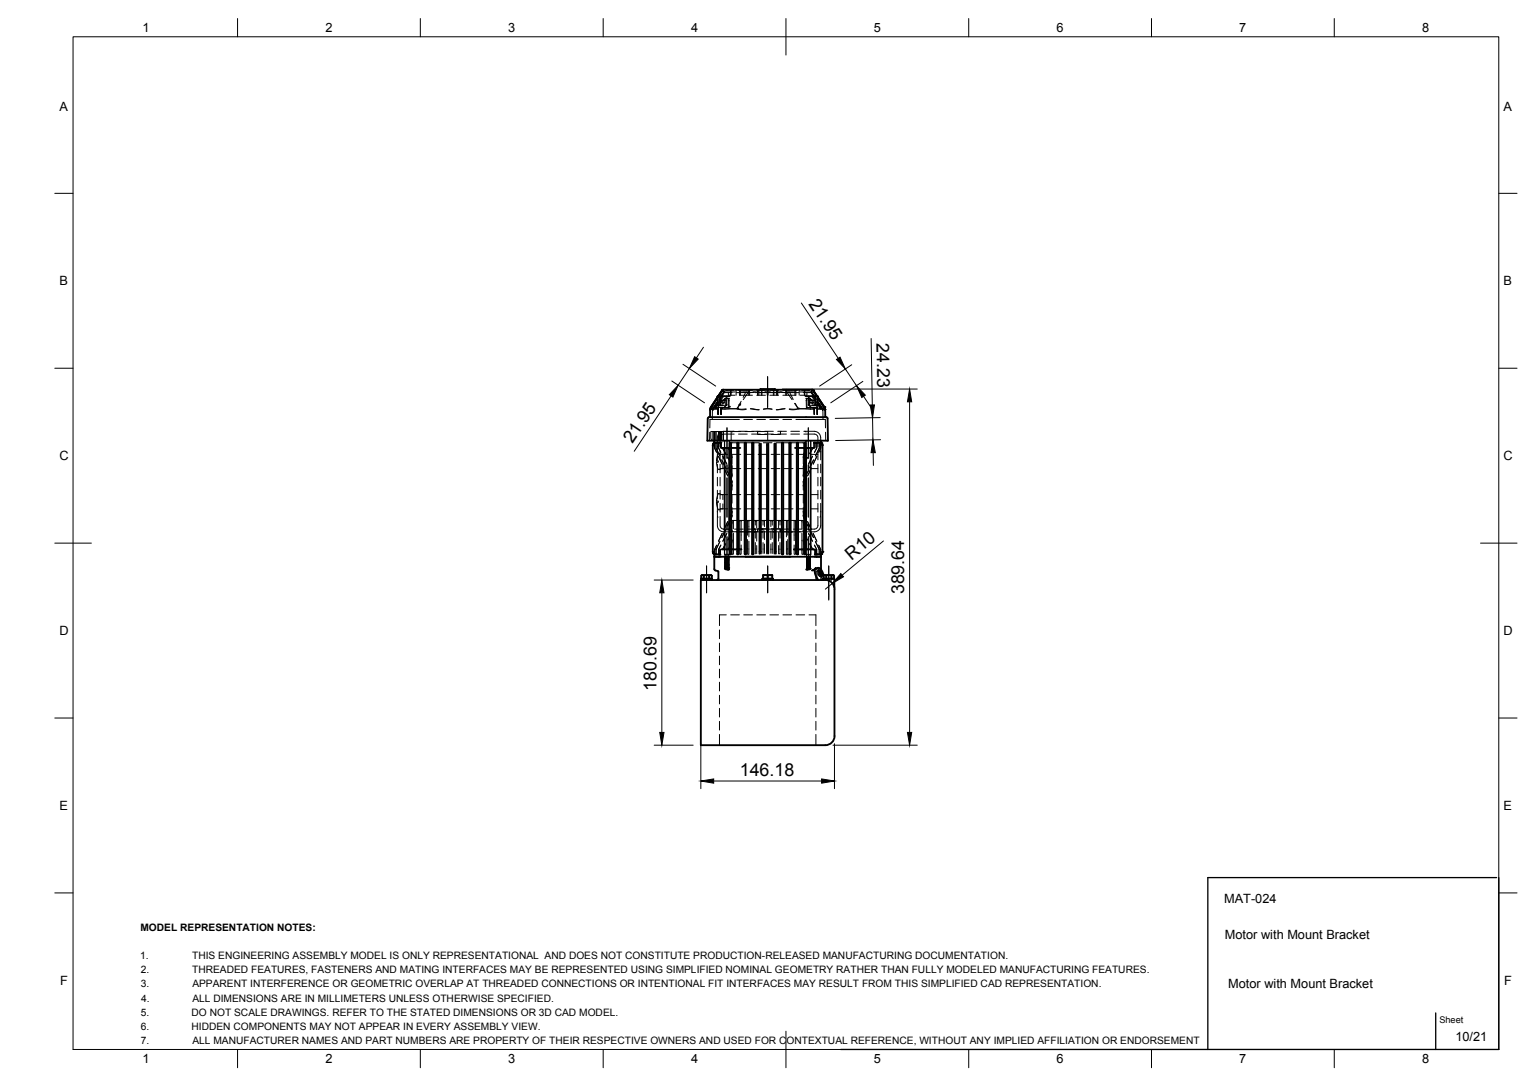
ISO-10303-21;
HEADER;
/* Generated by software containing ST-Developer
 * from STEP Tools, Inc. (www.steptools.com) 
 */

FILE_DESCRIPTION(
/* description */ ('STEP AP214'),
/* implementation_level */ '2;1');

FILE_NAME(
/* name */ 'Motor with Mount Bracket.step',
/* time_stamp */ '2026-11-14T06:34:07-08:00',
/* author */ (''),
/* organization */ (''),
/* preprocessor_version */ 'ST-DEVELOPER v20.2',
/* originating_system */ 'Autodesk Translation Framework v15.17.0.0',
/* authorisation */ '');

FILE_SCHEMA (('AUTOMOTIVE_DESIGN { 1 0 10303 214 3 1 1 }'));
ENDSEC;

DATA;
#10=MECHANICAL_DESIGN_GEOMETRIC_PRESENTATION_REPRESENTATION('',(#7258,#7259,#7260,#7261,#7262,#7263,#7264,#7265,#7266,#7267,#7268,#7269,#7270,#7271,#7272,#7273,#7274,#7275,#7276,#7277),#310623);
#905=B_SPLINE_SURFACE_WITH_KNOTS('',3,3,((#200297,#200298,#200299,#200300,
#200301,#200302,#200303,#200304,#200305,#200306,#200307,#200308,#200309),
(#200310,#200311,#200312,#200313,#200314,#200315,#200316,#200317,#200318,
#200319,#200320,#200321,#200322),(#200323,#200324,#200325,#200326,#200327,
#200328,#200329,#200330,#200331,#200332,#200333,#200334,#200335),(#200336,
#200337,#200338,#200339,#200340,#200341,#200342,#200343,#200344,#200345,
#200346,#200347,#200348),(#200349,#200350,#200351,#200352,#200353,#200354,
#200355,#200356,#200357,#200358,#200359,#200360,#200361),(#200362,#200363,
#200364,#200365,#200366,#200367,#200368,#200369,#200370,#200371,#200372,
#200373,#200374),(#200375,#200376,#200377,#200378,#200379,#200380,#200381,
#200382,#200383,#200384,#200385,#200386,#200387),(#200388,#200389,#200390,
#200391,#200392,#200393,#200394,#200395,#200396,#200397,#200398,#200399,
#200400),(#200401,#200402,#200403,#200404,#200405,#200406,#200407,#200408,
#200409,#200410,#200411,#200412,#200413),(#200414,#200415,#200416,#200417,
#200418,#200419,#200420,#200421,#200422,#200423,#200424,#200425,#200426),
(#200427,#200428,#200429,#200430,#200431,#200432,#200433,#200434,#200435,
#200436,#200437,#200438,#200439),(#200440,#200441,#200442,#200443,#200444,
#200445,#200446,#200447,#200448,#200449,#200450,#200451,#200452),(#200453,
#200454,#200455,#200456,#200457,#200458,#200459,#200460,#200461,#200462,
#200463,#200464,#200465),(#200466,#200467,#200468,#200469,#200470,#200471,
#200472,#200473,#200474,#200475,#200476,#200477,#200478),(#200479,#200480,
#200481,#200482,#200483,#200484,#200485,#200486,#200487,#200488,#200489,
#200490,#200491),(#200492,#200493,#200494,#200495,#200496,#200497,#200498,
#200499,#200500,#200501,#200502,#200503,#200504),(#200505,#200506,#200507,
#200508,#200509,#200510,#200511,#200512,#200513,#200514,#200515,#200516,
#200517),(#200518,#200519,#200520,#200521,#200522,#200523,#200524,#200525,
#200526,#200527,#200528,#200529,#200530),(#200531,#200532,#200533,#200534,
#200535,#200536,#200537,#200538,#200539,#200540,#200541,#200542,#200543),
(#200544,#200545,#200546,#200547,#200548,#200549,#200550,#200551,#200552,
#200553,#200554,#200555,#200556),(#200557,#200558,#200559,#200560,#200561,
#200562,#200563,#200564,#200565,#200566,#200567,#200568,#200569),(#200570,
#200571,#200572,#200573,#200574,#200575,#200576,#200577,#200578,#200579,
#200580,#200581,#200582),(#200583,#200584,#200585,#200586,#200587,#200588,
#200589,#200590,#200591,#200592,#200593,#200594,#200595),(#200596,#200597,
#200598,#200599,#200600,#200601,#200602,#200603,#200604,#200605,#200606,
#200607,#200608),(#200609,#200610,#200611,#200612,#200613,#200614,#200615,
#200616,#200617,#200618,#200619,#200620,#200621),(#200622,#200623,#200624,
#200625,#200626,#200627,#200628,#200629,#200630,#200631,#200632,#200633,
#200634),(#200635,#200636,#200637,#200638,#200639,#200640,#200641,#200642,
#200643,#200644,#200645,#200646,#200647),(#200648,#200649,#200650,#200651,
#200652,#200653,#200654,#200655,#200656,#200657,#200658,#200659,#200660)),
 .UNSPECIFIED.,.F.,.F.,.F.,(4,3,3,3,3,3,3,3,3,4),(4,3,3,3,4),(-3.98343850650087E-6,
0.125000000000275,0.250000000000551,0.375000000000826,0.500000000001101,
0.625000000001376,0.750000000001651,0.875000000001926,0.937500000002063,
1.0000000000022),(0.0305346534395145,0.148544372614449,0.266554091789383,
0.502573530139252,0.97461240683899),.UNSPECIFIED.);
#906=B_SPLINE_SURFACE_WITH_KNOTS('',3,3,((#200724,#200725,#200726,#200727,
#200728,#200729,#200730,#200731,#200732,#200733,#200734,#200735,#200736),
(#200737,#200738,#200739,#200740,#200741,#200742,#200743,#200744,#200745,
#200746,#200747,#200748,#200749),(#200750,#200751,#200752,#200753,#200754,
#200755,#200756,#200757,#200758,#200759,#200760,#200761,#200762),(#200763,
#200764,#200765,#200766,#200767,#200768,#200769,#200770,#200771,#200772,
#200773,#200774,#200775),(#200776,#200777,#200778,#200779,#200780,#200781,
#200782,#200783,#200784,#200785,#200786,#200787,#200788),(#200789,#200790,
#200791,#200792,#200793,#200794,#200795,#200796,#200797,#200798,#200799,
#200800,#200801),(#200802,#200803,#200804,#200805,#200806,#200807,#200808,
#200809,#200810,#200811,#200812,#200813,#200814),(#200815,#200816,#200817,
#200818,#200819,#200820,#200821,#200822,#200823,#200824,#200825,#200826,
#200827),(#200828,#200829,#200830,#200831,#200832,#200833,#200834,#200835,
#200836,#200837,#200838,#200839,#200840),(#200841,#200842,#200843,#200844,
#200845,#200846,#200847,#200848,#200849,#200850,#200851,#200852,#200853),
(#200854,#200855,#200856,#200857,#200858,#200859,#200860,#200861,#200862,
#200863,#200864,#200865,#200866),(#200867,#200868,#200869,#200870,#200871,
#200872,#200873,#200874,#200875,#200876,#200877,#200878,#200879),(#200880,
#200881,#200882,#200883,#200884,#200885,#200886,#200887,#200888,#200889,
#200890,#200891,#200892),(#200893,#200894,#200895,#200896,#200897,#200898,
#200899,#200900,#200901,#200902,#200903,#200904,#200905),(#200906,#200907,
#200908,#200909,#200910,#200911,#200912,#200913,#200914,#200915,#200916,
#200917,#200918),(#200919,#200920,#200921,#200922,#200923,#200924,#200925,
#200926,#200927,#200928,#200929,#200930,#200931),(#200932,#200933,#200934,
#200935,#200936,#200937,#200938,#200939,#200940,#200941,#200942,#200943,
#200944),(#200945,#200946,#200947,#200948,#200949,#200950,#200951,#200952,
#200953,#200954,#200955,#200956,#200957),(#200958,#200959,#200960,#200961,
#200962,#200963,#200964,#200965,#200966,#200967,#200968,#200969,#200970),
(#200971,#200972,#200973,#200974,#200975,#200976,#200977,#200978,#200979,
#200980,#200981,#200982,#200983),(#200984,#200985,#200986,#200987,#200988,
#200989,#200990,#200991,#200992,#200993,#200994,#200995,#200996),(#200997,
#200998,#200999,#201000,#201001,#201002,#201003,#201004,#201005,#201006,
#201007,#201008,#201009),(#201010,#201011,#201012,#201013,#201014,#201015,
#201016,#201017,#201018,#201019,#201020,#201021,#201022),(#201023,#201024,
#201025,#201026,#201027,#201028,#201029,#201030,#201031,#201032,#201033,
#201034,#201035),(#201036,#201037,#201038,#201039,#201040,#201041,#201042,
#201043,#201044,#201045,#201046,#201047,#201048),(#201049,#201050,#201051,
#201052,#201053,#201054,#201055,#201056,#201057,#201058,#201059,#201060,
#201061),(#201062,#201063,#201064,#201065,#201066,#201067,#201068,#201069,
#201070,#201071,#201072,#201073,#201074),(#201075,#201076,#201077,#201078,
#201079,#201080,#201081,#201082,#201083,#201084,#201085,#201086,#201087),
(#201088,#201089,#201090,#201091,#201092,#201093,#201094,#201095,#201096,
#201097,#201098,#201099,#201100),(#201101,#201102,#201103,#201104,#201105,
#201106,#201107,#201108,#201109,#201110,#201111,#201112,#201113),(#201114,
#201115,#201116,#201117,#201118,#201119,#201120,#201121,#201122,#201123,
#201124,#201125,#201126),(#201127,#201128,#201129,#201130,#201131,#201132,
#201133,#201134,#201135,#201136,#201137,#201138,#201139),(#201140,#201141,
#201142,#201143,#201144,#201145,#201146,#201147,#201148,#201149,#201150,
#201151,#201152),(#201153,#201154,#201155,#201156,#201157,#201158,#201159,
#201160,#201161,#201162,#201163,#201164,#201165),(#201166,#201167,#201168,
#201169,#201170,#201171,#201172,#201173,#201174,#201175,#201176,#201177,
#201178),(#201179,#201180,#201181,#201182,#201183,#201184,#201185,#201186,
#201187,#201188,#201189,#201190,#201191),(#201192,#201193,#201194,#201195,
#201196,#201197,#201198,#201199,#201200,#201201,#201202,#201203,#201204),
(#201205,#201206,#201207,#201208,#201209,#201210,#201211,#201212,#201213,
#201214,#201215,#201216,#201217),(#201218,#201219,#201220,#201221,#201222,
#201223,#201224,#201225,#201226,#201227,#201228,#201229,#201230),(#201231,
#201232,#201233,#201234,#201235,#201236,#201237,#201238,#201239,#201240,
#201241,#201242,#201243),(#201244,#201245,#201246,#201247,#201248,#201249,
#201250,#201251,#201252,#201253,#201254,#201255,#201256),(#201257,#201258,
#201259,#201260,#201261,#201262,#201263,#201264,#201265,#201266,#201267,
#201268,#201269),(#201270,#201271,#201272,#201273,#201274,#201275,#201276,
#201277,#201278,#201279,#201280,#201281,#201282)),.UNSPECIFIED.,.F.,.F.,
 .F.,(4,3,3,3,3,3,3,3,3,3,3,3,3,3,4),(4,3,3,3,4),(0.,0.0628750561902459,
0.125750112380492,0.251500224760983,0.377250337141475,0.503000449521967,
0.628750561902459,0.754500674282951,0.817375730473197,0.880250786663443,
0.943125842853689,0.974563370948812,0.990282134996373,0.998141517020154,
1.00600089904393),(0.0313847250337115,0.149350226349808,0.267315727665905,
0.503246730298099,0.975108735562486),.UNSPECIFIED.);
#907=B_SPLINE_SURFACE_WITH_KNOTS('',3,3,((#201360,#201361,#201362,#201363,
#201364,#201365,#201366,#201367,#201368,#201369,#201370,#201371,#201372),
(#201373,#201374,#201375,#201376,#201377,#201378,#201379,#201380,#201381,
#201382,#201383,#201384,#201385),(#201386,#201387,#201388,#201389,#201390,
#201391,#201392,#201393,#201394,#201395,#201396,#201397,#201398),(#201399,
#201400,#201401,#201402,#201403,#201404,#201405,#201406,#201407,#201408,
#201409,#201410,#201411),(#201412,#201413,#201414,#201415,#201416,#201417,
#201418,#201419,#201420,#201421,#201422,#201423,#201424),(#201425,#201426,
#201427,#201428,#201429,#201430,#201431,#201432,#201433,#201434,#201435,
#201436,#201437),(#201438,#201439,#201440,#201441,#201442,#201443,#201444,
#201445,#201446,#201447,#201448,#201449,#201450),(#201451,#201452,#201453,
#201454,#201455,#201456,#201457,#201458,#201459,#201460,#201461,#201462,
#201463),(#201464,#201465,#201466,#201467,#201468,#201469,#201470,#201471,
#201472,#201473,#201474,#201475,#201476),(#201477,#201478,#201479,#201480,
#201481,#201482,#201483,#201484,#201485,#201486,#201487,#201488,#201489),
(#201490,#201491,#201492,#201493,#201494,#201495,#201496,#201497,#201498,
#201499,#201500,#201501,#201502),(#201503,#201504,#201505,#201506,#201507,
#201508,#201509,#201510,#201511,#201512,#201513,#201514,#201515),(#201516,
#201517,#201518,#201519,#201520,#201521,#201522,#201523,#201524,#201525,
#201526,#201527,#201528),(#201529,#201530,#201531,#201532,#201533,#201534,
#201535,#201536,#201537,#201538,#201539,#201540,#201541),(#201542,#201543,
#201544,#201545,#201546,#201547,#201548,#201549,#201550,#201551,#201552,
#201553,#201554),(#201555,#201556,#201557,#201558,#201559,#201560,#201561,
#201562,#201563,#201564,#201565,#201566,#201567),(#201568,#201569,#201570,
#201571,#201572,#201573,#201574,#201575,#201576,#201577,#201578,#201579,
#201580),(#201581,#201582,#201583,#201584,#201585,#201586,#201587,#201588,
#201589,#201590,#201591,#201592,#201593),(#201594,#201595,#201596,#201597,
#201598,#201599,#201600,#201601,#201602,#201603,#201604,#201605,#201606),
(#201607,#201608,#201609,#201610,#201611,#201612,#201613,#201614,#201615,
#201616,#201617,#201618,#201619),(#201620,#201621,#201622,#201623,#201624,
#201625,#201626,#201627,#201628,#201629,#201630,#201631,#201632),(#201633,
#201634,#201635,#201636,#201637,#201638,#201639,#201640,#201641,#201642,
#201643,#201644,#201645),(#201646,#201647,#201648,#201649,#201650,#201651,
#201652,#201653,#201654,#201655,#201656,#201657,#201658),(#201659,#201660,
#201661,#201662,#201663,#201664,#201665,#201666,#201667,#201668,#201669,
#201670,#201671),(#201672,#201673,#201674,#201675,#201676,#201677,#201678,
#201679,#201680,#201681,#201682,#201683,#201684),(#201685,#201686,#201687,
#201688,#201689,#201690,#201691,#201692,#201693,#201694,#201695,#201696,
#201697),(#201698,#201699,#201700,#201701,#201702,#201703,#201704,#201705,
#201706,#201707,#201708,#201709,#201710),(#201711,#201712,#201713,#201714,
#201715,#201716,#201717,#201718,#201719,#201720,#201721,#201722,#201723)),
 .UNSPECIFIED.,.F.,.F.,.F.,(4,3,3,3,3,3,3,3,3,4),(4,3,3,3,4),(0.,0.125000000000521,
0.250000000001042,0.375000000001564,0.500000000002084,0.625000000002606,
0.750000000003127,0.875000000003648,0.937500000003908,1.00000000000417),
(0.035779394199433,0.153116210014097,0.27045302582876,0.505126657458087,
0.97447392071674),.UNSPECIFIED.);
#908=B_SPLINE_SURFACE_WITH_KNOTS('',3,3,((#201796,#201797,#201798,#201799,
#201800,#201801,#201802,#201803,#201804,#201805),(#201806,#201807,#201808,
#201809,#201810,#201811,#201812,#201813,#201814,#201815),(#201816,#201817,
#201818,#201819,#201820,#201821,#201822,#201823,#201824,#201825),(#201826,
#201827,#201828,#201829,#201830,#201831,#201832,#201833,#201834,#201835),
(#201836,#201837,#201838,#201839,#201840,#201841,#201842,#201843,#201844,
#201845),(#201846,#201847,#201848,#201849,#201850,#201851,#201852,#201853,
#201854,#201855),(#201856,#201857,#201858,#201859,#201860,#201861,#201862,
#201863,#201864,#201865),(#201866,#201867,#201868,#201869,#201870,#201871,
#201872,#201873,#201874,#201875),(#201876,#201877,#201878,#201879,#201880,
#201881,#201882,#201883,#201884,#201885),(#201886,#201887,#201888,#201889,
#201890,#201891,#201892,#201893,#201894,#201895),(#201896,#201897,#201898,
#201899,#201900,#201901,#201902,#201903,#201904,#201905),(#201906,#201907,
#201908,#201909,#201910,#201911,#201912,#201913,#201914,#201915),(#201916,
#201917,#201918,#201919,#201920,#201921,#201922,#201923,#201924,#201925),
(#201926,#201927,#201928,#201929,#201930,#201931,#201932,#201933,#201934,
#201935),(#201936,#201937,#201938,#201939,#201940,#201941,#201942,#201943,
#201944,#201945),(#201946,#201947,#201948,#201949,#201950,#201951,#201952,
#201953,#201954,#201955),(#201956,#201957,#201958,#201959,#201960,#201961,
#201962,#201963,#201964,#201965),(#201966,#201967,#201968,#201969,#201970,
#201971,#201972,#201973,#201974,#201975),(#201976,#201977,#201978,#201979,
#201980,#201981,#201982,#201983,#201984,#201985),(#201986,#201987,#201988,
#201989,#201990,#201991,#201992,#201993,#201994,#201995),(#201996,#201997,
#201998,#201999,#202000,#202001,#202002,#202003,#202004,#202005),(#202006,
#202007,#202008,#202009,#202010,#202011,#202012,#202013,#202014,#202015),
(#202016,#202017,#202018,#202019,#202020,#202021,#202022,#202023,#202024,
#202025),(#202026,#202027,#202028,#202029,#202030,#202031,#202032,#202033,
#202034,#202035),(#202036,#202037,#202038,#202039,#202040,#202041,#202042,
#202043,#202044,#202045),(#202046,#202047,#202048,#202049,#202050,#202051,
#202052,#202053,#202054,#202055),(#202056,#202057,#202058,#202059,#202060,
#202061,#202062,#202063,#202064,#202065),(#202066,#202067,#202068,#202069,
#202070,#202071,#202072,#202073,#202074,#202075),(#202076,#202077,#202078,
#202079,#202080,#202081,#202082,#202083,#202084,#202085),(#202086,#202087,
#202088,#202089,#202090,#202091,#202092,#202093,#202094,#202095),(#202096,
#202097,#202098,#202099,#202100,#202101,#202102,#202103,#202104,#202105),
(#202106,#202107,#202108,#202109,#202110,#202111,#202112,#202113,#202114,
#202115),(#202116,#202117,#202118,#202119,#202120,#202121,#202122,#202123,
#202124,#202125),(#202126,#202127,#202128,#202129,#202130,#202131,#202132,
#202133,#202134,#202135),(#202136,#202137,#202138,#202139,#202140,#202141,
#202142,#202143,#202144,#202145),(#202146,#202147,#202148,#202149,#202150,
#202151,#202152,#202153,#202154,#202155),(#202156,#202157,#202158,#202159,
#202160,#202161,#202162,#202163,#202164,#202165),(#202166,#202167,#202168,
#202169,#202170,#202171,#202172,#202173,#202174,#202175),(#202176,#202177,
#202178,#202179,#202180,#202181,#202182,#202183,#202184,#202185),(#202186,
#202187,#202188,#202189,#202190,#202191,#202192,#202193,#202194,#202195),
(#202196,#202197,#202198,#202199,#202200,#202201,#202202,#202203,#202204,
#202205),(#202206,#202207,#202208,#202209,#202210,#202211,#202212,#202213,
#202214,#202215),(#202216,#202217,#202218,#202219,#202220,#202221,#202222,
#202223,#202224,#202225),(#202226,#202227,#202228,#202229,#202230,#202231,
#202232,#202233,#202234,#202235),(#202236,#202237,#202238,#202239,#202240,
#202241,#202242,#202243,#202244,#202245),(#202246,#202247,#202248,#202249,
#202250,#202251,#202252,#202253,#202254,#202255),(#202256,#202257,#202258,
#202259,#202260,#202261,#202262,#202263,#202264,#202265),(#202266,#202267,
#202268,#202269,#202270,#202271,#202272,#202273,#202274,#202275),(#202276,
#202277,#202278,#202279,#202280,#202281,#202282,#202283,#202284,#202285),
(#202286,#202287,#202288,#202289,#202290,#202291,#202292,#202293,#202294,
#202295),(#202296,#202297,#202298,#202299,#202300,#202301,#202302,#202303,
#202304,#202305),(#202306,#202307,#202308,#202309,#202310,#202311,#202312,
#202313,#202314,#202315)),.UNSPECIFIED.,.F.,.F.,.F.,(4,3,3,3,3,3,3,3,3,
3,3,3,3,3,3,3,3,4),(4,3,3,4),(0.,0.00790626166828645,0.0158125233365729,
0.0316250466731458,0.0632500933462917,0.126500186692583,0.189750280038875,
0.253000373385167,0.37950056007775,0.506000746770334,0.632500933462917,
0.7590011201555,0.885501306848084,0.948751400194375,0.980376446867521,0.996188970204094,
1.00409523187238,1.01200149354067),(0.0341113530318832,0.269267250872974,
0.504423148714065,0.974734944396246),.UNSPECIFIED.);
#909=B_SPLINE_SURFACE_WITH_KNOTS('',3,3,((#202498,#202499,#202500,#202501),
(#202502,#202503,#202504,#202505),(#202506,#202507,#202508,#202509),(#202510,
#202511,#202512,#202513)),.UNSPECIFIED.,.F.,.F.,.F.,(4,4),(4,4),(0.,0.27458600745849),
(0.048728470569204,0.974637180848091),.UNSPECIFIED.);
#910=B_SPLINE_SURFACE_WITH_KNOTS('',3,3,((#202534,#202535,#202536,#202537),
(#202538,#202539,#202540,#202541),(#202542,#202543,#202544,#202545),(#202546,
#202547,#202548,#202549)),.UNSPECIFIED.,.F.,.F.,.F.,(4,4),(4,4),(0.,0.276208371820539),
(0.0491493978854403,0.974752225001403),.UNSPECIFIED.);
#911=B_SPLINE_SURFACE_WITH_KNOTS('',3,3,((#202753,#202754,#202755,#202756),
(#202757,#202758,#202759,#202760),(#202761,#202762,#202763,#202764),(#202765,
#202766,#202767,#202768)),.UNSPECIFIED.,.F.,.F.,.F.,(4,4),(4,4),(0.,0.107439860233905),
(0.0511874640850671,0.974440796609261),.UNSPECIFIED.);
#912=B_SPLINE_SURFACE_WITH_KNOTS('',3,3,((#202889,#202890,#202891,#202892),
(#202893,#202894,#202895,#202896),(#202897,#202898,#202899,#202900),(#202901,
#202902,#202903,#202904)),.UNSPECIFIED.,.F.,.F.,.F.,(4,4),(4,4),(0.,0.0948189441871283),
(0.0504405324641688,0.975107277906268),.UNSPECIFIED.);
#913=B_SPLINE_SURFACE_WITH_KNOTS('',3,3,((#202968,#202969,#202970,#202971,
#202972,#202973,#202974),(#202975,#202976,#202977,#202978,#202979,#202980,
#202981),(#202982,#202983,#202984,#202985,#202986,#202987,#202988),(#202989,
#202990,#202991,#202992,#202993,#202994,#202995),(#202996,#202997,#202998,
#202999,#203000,#203001,#203002),(#203003,#203004,#203005,#203006,#203007,
#203008,#203009),(#203010,#203011,#203012,#203013,#203014,#203015,#203016),
(#203017,#203018,#203019,#203020,#203021,#203022,#203023),(#203024,#203025,
#203026,#203027,#203028,#203029,#203030),(#203031,#203032,#203033,#203034,
#203035,#203036,#203037),(#203038,#203039,#203040,#203041,#203042,#203043,
#203044),(#203045,#203046,#203047,#203048,#203049,#203050,#203051),(#203052,
#203053,#203054,#203055,#203056,#203057,#203058),(#203059,#203060,#203061,
#203062,#203063,#203064,#203065),(#203066,#203067,#203068,#203069,#203070,
#203071,#203072),(#203073,#203074,#203075,#203076,#203077,#203078,#203079),
(#203080,#203081,#203082,#203083,#203084,#203085,#203086),(#203087,#203088,
#203089,#203090,#203091,#203092,#203093),(#203094,#203095,#203096,#203097,
#203098,#203099,#203100),(#203101,#203102,#203103,#203104,#203105,#203106,
#203107),(#203108,#203109,#203110,#203111,#203112,#203113,#203114),(#203115,
#203116,#203117,#203118,#203119,#203120,#203121),(#203122,#203123,#203124,
#203125,#203126,#203127,#203128),(#203129,#203130,#203131,#203132,#203133,
#203134,#203135),(#203136,#203137,#203138,#203139,#203140,#203141,#203142),
(#203143,#203144,#203145,#203146,#203147,#203148,#203149),(#203150,#203151,
#203152,#203153,#203154,#203155,#203156),(#203157,#203158,#203159,#203160,
#203161,#203162,#203163)),.UNSPECIFIED.,.F.,.F.,.F.,(4,3,3,3,3,3,3,3,3,
4),(4,3,4),(0.,0.0078125,0.015625,0.03125,0.0625,0.125,0.25,0.5,0.75,1.),
(0.0332750425089971,0.501824549528,0.970374056547004),.UNSPECIFIED.);
#914=B_SPLINE_SURFACE_WITH_KNOTS('',3,3,((#203245,#203246,#203247,#203248,
#203249,#203250,#203251),(#203252,#203253,#203254,#203255,#203256,#203257,
#203258),(#203259,#203260,#203261,#203262,#203263,#203264,#203265),(#203266,
#203267,#203268,#203269,#203270,#203271,#203272),(#203273,#203274,#203275,
#203276,#203277,#203278,#203279),(#203280,#203281,#203282,#203283,#203284,
#203285,#203286),(#203287,#203288,#203289,#203290,#203291,#203292,#203293),
(#203294,#203295,#203296,#203297,#203298,#203299,#203300),(#203301,#203302,
#203303,#203304,#203305,#203306,#203307),(#203308,#203309,#203310,#203311,
#203312,#203313,#203314),(#203315,#203316,#203317,#203318,#203319,#203320,
#203321),(#203322,#203323,#203324,#203325,#203326,#203327,#203328),(#203329,
#203330,#203331,#203332,#203333,#203334,#203335),(#203336,#203337,#203338,
#203339,#203340,#203341,#203342),(#203343,#203344,#203345,#203346,#203347,
#203348,#203349),(#203350,#203351,#203352,#203353,#203354,#203355,#203356),
(#203357,#203358,#203359,#203360,#203361,#203362,#203363),(#203364,#203365,
#203366,#203367,#203368,#203369,#203370),(#203371,#203372,#203373,#203374,
#203375,#203376,#203377),(#203378,#203379,#203380,#203381,#203382,#203383,
#203384),(#203385,#203386,#203387,#203388,#203389,#203390,#203391),(#203392,
#203393,#203394,#203395,#203396,#203397,#203398),(#203399,#203400,#203401,
#203402,#203403,#203404,#203405),(#203406,#203407,#203408,#203409,#203410,
#203411,#203412),(#203413,#203414,#203415,#203416,#203417,#203418,#203419),
(#203420,#203421,#203422,#203423,#203424,#203425,#203426),(#203427,#203428,
#203429,#203430,#203431,#203432,#203433),(#203434,#203435,#203436,#203437,
#203438,#203439,#203440),(#203441,#203442,#203443,#203444,#203445,#203446,
#203447),(#203448,#203449,#203450,#203451,#203452,#203453,#203454),(#203455,
#203456,#203457,#203458,#203459,#203460,#203461),(#203462,#203463,#203464,
#203465,#203466,#203467,#203468),(#203469,#203470,#203471,#203472,#203473,
#203474,#203475),(#203476,#203477,#203478,#203479,#203480,#203481,#203482),
(#203483,#203484,#203485,#203486,#203487,#203488,#203489),(#203490,#203491,
#203492,#203493,#203494,#203495,#203496),(#203497,#203498,#203499,#203500,
#203501,#203502,#203503),(#203504,#203505,#203506,#203507,#203508,#203509,
#203510),(#203511,#203512,#203513,#203514,#203515,#203516,#203517),(#203518,
#203519,#203520,#203521,#203522,#203523,#203524)),.UNSPECIFIED.,.F.,.F.,
 .F.,(4,3,3,3,3,3,3,3,3,3,3,3,3,4),(4,3,4),(0.,0.0078593752336461,0.0157187504672922,
0.0314375009345845,0.0628750018691691,0.125750003738338,0.251500007476676,
0.503000014953352,0.754500022430028,0.880250026168366,0.943125028037535,
0.974562528972119,0.990281279439412,1.0060000299067),(0.0284242133522742,
0.499005960311874,0.969587707271474),.UNSPECIFIED.);
#915=B_SPLINE_SURFACE_WITH_KNOTS('',3,3,((#203732,#203733,#203734,#203735,
#203736,#203737,#203738),(#203739,#203740,#203741,#203742,#203743,#203744,
#203745),(#203746,#203747,#203748,#203749,#203750,#203751,#203752),(#203753,
#203754,#203755,#203756,#203757,#203758,#203759),(#203760,#203761,#203762,
#203763,#203764,#203765,#203766),(#203767,#203768,#203769,#203770,#203771,
#203772,#203773),(#203774,#203775,#203776,#203777,#203778,#203779,#203780),
(#203781,#203782,#203783,#203784,#203785,#203786,#203787),(#203788,#203789,
#203790,#203791,#203792,#203793,#203794),(#203795,#203796,#203797,#203798,
#203799,#203800,#203801),(#203802,#203803,#203804,#203805,#203806,#203807,
#203808),(#203809,#203810,#203811,#203812,#203813,#203814,#203815),(#203816,
#203817,#203818,#203819,#203820,#203821,#203822),(#203823,#203824,#203825,
#203826,#203827,#203828,#203829),(#203830,#203831,#203832,#203833,#203834,
#203835,#203836),(#203837,#203838,#203839,#203840,#203841,#203842,#203843),
(#203844,#203845,#203846,#203847,#203848,#203849,#203850),(#203851,#203852,
#203853,#203854,#203855,#203856,#203857),(#203858,#203859,#203860,#203861,
#203862,#203863,#203864),(#203865,#203866,#203867,#203868,#203869,#203870,
#203871),(#203872,#203873,#203874,#203875,#203876,#203877,#203878),(#203879,
#203880,#203881,#203882,#203883,#203884,#203885),(#203886,#203887,#203888,
#203889,#203890,#203891,#203892),(#203893,#203894,#203895,#203896,#203897,
#203898,#203899),(#203900,#203901,#203902,#203903,#203904,#203905,#203906),
(#203907,#203908,#203909,#203910,#203911,#203912,#203913),(#203914,#203915,
#203916,#203917,#203918,#203919,#203920),(#203921,#203922,#203923,#203924,
#203925,#203926,#203927),(#203928,#203929,#203930,#203931,#203932,#203933,
#203934),(#203935,#203936,#203937,#203938,#203939,#203940,#203941),(#203942,
#203943,#203944,#203945,#203946,#203947,#203948),(#203949,#203950,#203951,
#203952,#203953,#203954,#203955),(#203956,#203957,#203958,#203959,#203960,
#203961,#203962),(#203963,#203964,#203965,#203966,#203967,#203968,#203969),
(#203970,#203971,#203972,#203973,#203974,#203975,#203976),(#203977,#203978,
#203979,#203980,#203981,#203982,#203983),(#203984,#203985,#203986,#203987,
#203988,#203989,#203990),(#203991,#203992,#203993,#203994,#203995,#203996,
#203997),(#203998,#203999,#204000,#204001,#204002,#204003,#204004),(#204005,
#204006,#204007,#204008,#204009,#204010,#204011),(#204012,#204013,#204014,
#204015,#204016,#204017,#204018),(#204019,#204020,#204021,#204022,#204023,
#204024,#204025),(#204026,#204027,#204028,#204029,#204030,#204031,#204032),
(#204033,#204034,#204035,#204036,#204037,#204038,#204039),(#204040,#204041,
#204042,#204043,#204044,#204045,#204046),(#204047,#204048,#204049,#204050,
#204051,#204052,#204053),(#204054,#204055,#204056,#204057,#204058,#204059,
#204060),(#204061,#204062,#204063,#204064,#204065,#204066,#204067),(#204068,
#204069,#204070,#204071,#204072,#204073,#204074),(#204075,#204076,#204077,
#204078,#204079,#204080,#204081),(#204082,#204083,#204084,#204085,#204086,
#204087,#204088),(#204089,#204090,#204091,#204092,#204093,#204094,#204095),
(#204096,#204097,#204098,#204099,#204100,#204101,#204102),(#204103,#204104,
#204105,#204106,#204107,#204108,#204109),(#204110,#204111,#204112,#204113,
#204114,#204115,#204116),(#204117,#204118,#204119,#204120,#204121,#204122,
#204123),(#204124,#204125,#204126,#204127,#204128,#204129,#204130),(#204131,
#204132,#204133,#204134,#204135,#204136,#204137),(#204138,#204139,#204140,
#204141,#204142,#204143,#204144),(#204145,#204146,#204147,#204148,#204149,
#204150,#204151),(#204152,#204153,#204154,#204155,#204156,#204157,#204158),
(#204159,#204160,#204161,#204162,#204163,#204164,#204165),(#204166,#204167,
#204168,#204169,#204170,#204171,#204172),(#204173,#204174,#204175,#204176,
#204177,#204178,#204179),(#204180,#204181,#204182,#204183,#204184,#204185,
#204186),(#204187,#204188,#204189,#204190,#204191,#204192,#204193),(#204194,
#204195,#204196,#204197,#204198,#204199,#204200),(#204201,#204202,#204203,
#204204,#204205,#204206,#204207),(#204208,#204209,#204210,#204211,#204212,
#204213,#204214),(#204215,#204216,#204217,#204218,#204219,#204220,#204221),
(#204222,#204223,#204224,#204225,#204226,#204227,#204228),(#204229,#204230,
#204231,#204232,#204233,#204234,#204235),(#204236,#204237,#204238,#204239,
#204240,#204241,#204242),(#204243,#204244,#204245,#204246,#204247,#204248,
#204249),(#204250,#204251,#204252,#204253,#204254,#204255,#204256),(#204257,
#204258,#204259,#204260,#204261,#204262,#204263),(#204264,#204265,#204266,
#204267,#204268,#204269,#204270),(#204271,#204272,#204273,#204274,#204275,
#204276,#204277),(#204278,#204279,#204280,#204281,#204282,#204283,#204284),
(#204285,#204286,#204287,#204288,#204289,#204290,#204291),(#204292,#204293,
#204294,#204295,#204296,#204297,#204298),(#204299,#204300,#204301,#204302,
#204303,#204304,#204305),(#204306,#204307,#204308,#204309,#204310,#204311,
#204312),(#204313,#204314,#204315,#204316,#204317,#204318,#204319),(#204320,
#204321,#204322,#204323,#204324,#204325,#204326),(#204327,#204328,#204329,
#204330,#204331,#204332,#204333),(#204334,#204335,#204336,#204337,#204338,
#204339,#204340),(#204341,#204342,#204343,#204344,#204345,#204346,#204347),
(#204348,#204349,#204350,#204351,#204352,#204353,#204354),(#204355,#204356,
#204357,#204358,#204359,#204360,#204361),(#204362,#204363,#204364,#204365,
#204366,#204367,#204368),(#204369,#204370,#204371,#204372,#204373,#204374,
#204375),(#204376,#204377,#204378,#204379,#204380,#204381,#204382),(#204383,
#204384,#204385,#204386,#204387,#204388,#204389),(#204390,#204391,#204392,
#204393,#204394,#204395,#204396),(#204397,#204398,#204399,#204400,#204401,
#204402,#204403),(#204404,#204405,#204406,#204407,#204408,#204409,#204410),
(#204411,#204412,#204413,#204414,#204415,#204416,#204417),(#204418,#204419,
#204420,#204421,#204422,#204423,#204424),(#204425,#204426,#204427,#204428,
#204429,#204430,#204431),(#204432,#204433,#204434,#204435,#204436,#204437,
#204438),(#204439,#204440,#204441,#204442,#204443,#204444,#204445),(#204446,
#204447,#204448,#204449,#204450,#204451,#204452),(#204453,#204454,#204455,
#204456,#204457,#204458,#204459),(#204460,#204461,#204462,#204463,#204464,
#204465,#204466),(#204467,#204468,#204469,#204470,#204471,#204472,#204473),
(#204474,#204475,#204476,#204477,#204478,#204479,#204480),(#204481,#204482,
#204483,#204484,#204485,#204486,#204487),(#204488,#204489,#204490,#204491,
#204492,#204493,#204494),(#204495,#204496,#204497,#204498,#204499,#204500,
#204501),(#204502,#204503,#204504,#204505,#204506,#204507,#204508),(#204509,
#204510,#204511,#204512,#204513,#204514,#204515),(#204516,#204517,#204518,
#204519,#204520,#204521,#204522),(#204523,#204524,#204525,#204526,#204527,
#204528,#204529),(#204530,#204531,#204532,#204533,#204534,#204535,#204536),
(#204537,#204538,#204539,#204540,#204541,#204542,#204543),(#204544,#204545,
#204546,#204547,#204548,#204549,#204550),(#204551,#204552,#204553,#204554,
#204555,#204556,#204557),(#204558,#204559,#204560,#204561,#204562,#204563,
#204564),(#204565,#204566,#204567,#204568,#204569,#204570,#204571),(#204572,
#204573,#204574,#204575,#204576,#204577,#204578),(#204579,#204580,#204581,
#204582,#204583,#204584,#204585),(#204586,#204587,#204588,#204589,#204590,
#204591,#204592),(#204593,#204594,#204595,#204596,#204597,#204598,#204599),
(#204600,#204601,#204602,#204603,#204604,#204605,#204606),(#204607,#204608,
#204609,#204610,#204611,#204612,#204613),(#204614,#204615,#204616,#204617,
#204618,#204619,#204620),(#204621,#204622,#204623,#204624,#204625,#204626,
#204627),(#204628,#204629,#204630,#204631,#204632,#204633,#204634),(#204635,
#204636,#204637,#204638,#204639,#204640,#204641),(#204642,#204643,#204644,
#204645,#204646,#204647,#204648),(#204649,#204650,#204651,#204652,#204653,
#204654,#204655),(#204656,#204657,#204658,#204659,#204660,#204661,#204662),
(#204663,#204664,#204665,#204666,#204667,#204668,#204669),(#204670,#204671,
#204672,#204673,#204674,#204675,#204676),(#204677,#204678,#204679,#204680,
#204681,#204682,#204683),(#204684,#204685,#204686,#204687,#204688,#204689,
#204690),(#204691,#204692,#204693,#204694,#204695,#204696,#204697),(#204698,
#204699,#204700,#204701,#204702,#204703,#204704),(#204705,#204706,#204707,
#204708,#204709,#204710,#204711),(#204712,#204713,#204714,#204715,#204716,
#204717,#204718),(#204719,#204720,#204721,#204722,#204723,#204724,#204725),
(#204726,#204727,#204728,#204729,#204730,#204731,#204732),(#204733,#204734,
#204735,#204736,#204737,#204738,#204739),(#204740,#204741,#204742,#204743,
#204744,#204745,#204746),(#204747,#204748,#204749,#204750,#204751,#204752,
#204753),(#204754,#204755,#204756,#204757,#204758,#204759,#204760),(#204761,
#204762,#204763,#204764,#204765,#204766,#204767),(#204768,#204769,#204770,
#204771,#204772,#204773,#204774),(#204775,#204776,#204777,#204778,#204779,
#204780,#204781),(#204782,#204783,#204784,#204785,#204786,#204787,#204788),
(#204789,#204790,#204791,#204792,#204793,#204794,#204795),(#204796,#204797,
#204798,#204799,#204800,#204801,#204802),(#204803,#204804,#204805,#204806,
#204807,#204808,#204809),(#204810,#204811,#204812,#204813,#204814,#204815,
#204816),(#204817,#204818,#204819,#204820,#204821,#204822,#204823),(#204824,
#204825,#204826,#204827,#204828,#204829,#204830)),.UNSPECIFIED.,.F.,.F.,
 .F.,(4,3,3,3,3,3,3,3,3,3,3,3,3,3,3,3,3,3,3,3,3,3,3,3,3,3,3,3,3,3,3,3,3,
3,3,3,3,3,3,3,3,3,3,3,3,3,3,3,3,3,3,3,4),(4,3,4),(0.,0.125100494684528,
0.156375618355659,0.164194399273443,0.165171746888165,0.166149094502889,
0.168103789732334,0.172013180191225,0.187650742026792,0.250200989369055,
0.281476113040187,0.297113674875754,0.299068370105199,0.301023065334645,
0.304932455793537,0.312751236711319,0.375301484053584,0.406576607724715,
0.422214169560281,0.430032950478064,0.431010298092787,0.431498971900149,
0.43198764570751,0.433942340936955,0.437851731395847,0.500401978738111,
0.562952226080375,0.566861616539267,0.568816311768712,0.569793659383435,
0.570771006998158,0.578589787915941,0.594227349751507,0.625502473422639,
0.688052720764903,0.695871501682686,0.699780892141577,0.7007582397563,0.701246913563662,
0.701735587371023,0.703690282600469,0.719327844436035,0.750602968107167,
0.813153215449431,0.828790777284997,0.832700167743888,0.834654862973334,
0.835632210588057,0.836120884395418,0.83660955820278,0.844428339120562,
0.875703462791694,1.00080395747622),(0.0460660594806178,0.548882757239649,
1.05169945499868),.UNSPECIFIED.);
#916=B_SPLINE_SURFACE_WITH_KNOTS('',3,1,((#204924,#204925),(#204926,#204927),
(#204928,#204929),(#204930,#204931),(#204932,#204933),(#204934,#204935),
(#204936,#204937),(#204938,#204939),(#204940,#204941),(#204942,#204943),
(#204944,#204945),(#204946,#204947),(#204948,#204949),(#204950,#204951),
(#204952,#204953),(#204954,#204955),(#204956,#204957),(#204958,#204959),
(#204960,#204961),(#204962,#204963),(#204964,#204965),(#204966,#204967),
(#204968,#204969),(#204970,#204971),(#204972,#204973),(#204974,#204975),
(#204976,#204977),(#204978,#204979),(#204980,#204981),(#204982,#204983),
(#204984,#204985),(#204986,#204987),(#204988,#204989),(#204990,#204991),
(#204992,#204993),(#204994,#204995),(#204996,#204997),(#204998,#204999),
(#205000,#205001),(#205002,#205003),(#205004,#205005),(#205006,#205007)),
 .UNSPECIFIED.,.F.,.F.,.F.,(4,1,1,1,2,1,1,1,2,1,1,1,2,1,1,1,2,1,1,1,2,1,
1,1,2,1,1,1,2,1,1,1,4),(2,2),(-0.130664626928687,0.0411596607520464,0.0823193215040928,
0.123478982256139,0.164638643008186,0.198458137911997,0.232277632815809,
0.26609712771962,0.299916622623432,0.332619014198497,0.365321405773562,
0.398023797348627,0.430726188923692,0.448044641692768,0.465363094461843,
0.482681547230919,0.499999999999994,0.517318452769073,0.534636905538152,
0.55195535830723,0.569273811076309,0.601976202651373,0.634678594226438,
0.667380985801503,0.700083377376568,0.73390287228038,0.767722367184191,
0.801541862088003,0.835361356991815,0.876521017743861,0.917680678495907,
0.958840339247954,1.12208155081997),(-0.184126650858872,1.18095881489235),
 .UNSPECIFIED.);
#917=B_SPLINE_SURFACE_WITH_KNOTS('',3,3,((#205068,#205069,#205070,#205071,
#205072,#205073,#205074),(#205075,#205076,#205077,#205078,#205079,#205080,
#205081),(#205082,#205083,#205084,#205085,#205086,#205087,#205088),(#205089,
#205090,#205091,#205092,#205093,#205094,#205095),(#205096,#205097,#205098,
#205099,#205100,#205101,#205102),(#205103,#205104,#205105,#205106,#205107,
#205108,#205109),(#205110,#205111,#205112,#205113,#205114,#205115,#205116),
(#205117,#205118,#205119,#205120,#205121,#205122,#205123),(#205124,#205125,
#205126,#205127,#205128,#205129,#205130),(#205131,#205132,#205133,#205134,
#205135,#205136,#205137),(#205138,#205139,#205140,#205141,#205142,#205143,
#205144)),.UNSPECIFIED.,.F.,.F.,.F.,(4,1,1,1,1,1,1,1,4),(4,3,4),(0.,0.124999999999998,
0.249999999999996,0.374999999999993,0.500000000000009,0.625000000000007,
0.75,0.875,1.),(0.,1.,1.01),.UNSPECIFIED.);
#918=B_SPLINE_SURFACE_WITH_KNOTS('',3,3,((#205150,#205151,#205152,#205153,
#205154,#205155,#205156),(#205157,#205158,#205159,#205160,#205161,#205162,
#205163),(#205164,#205165,#205166,#205167,#205168,#205169,#205170),(#205171,
#205172,#205173,#205174,#205175,#205176,#205177),(#205178,#205179,#205180,
#205181,#205182,#205183,#205184),(#205185,#205186,#205187,#205188,#205189,
#205190,#205191),(#205192,#205193,#205194,#205195,#205196,#205197,#205198),
(#205199,#205200,#205201,#205202,#205203,#205204,#205205),(#205206,#205207,
#205208,#205209,#205210,#205211,#205212),(#205213,#205214,#205215,#205216,
#205217,#205218,#205219),(#205220,#205221,#205222,#205223,#205224,#205225,
#205226),(#205227,#205228,#205229,#205230,#205231,#205232,#205233),(#205234,
#205235,#205236,#205237,#205238,#205239,#205240),(#205241,#205242,#205243,
#205244,#205245,#205246,#205247)),.UNSPECIFIED.,.F.,.F.,.F.,(4,3,1,1,1,
1,1,1,1,4),(4,3,4),(-0.01,0.,0.124999999999997,0.249999999999995,0.374999999999992,
0.49999999999999,0.624999999999988,0.749999999999985,0.874999999999983,
1.),(0.,1.,1.01),.UNSPECIFIED.);
#919=B_SPLINE_SURFACE_WITH_KNOTS('',3,3,((#205253,#205254,#205255,#205256,
#205257,#205258,#205259),(#205260,#205261,#205262,#205263,#205264,#205265,
#205266),(#205267,#205268,#205269,#205270,#205271,#205272,#205273),(#205274,
#205275,#205276,#205277,#205278,#205279,#205280),(#205281,#205282,#205283,
#205284,#205285,#205286,#205287),(#205288,#205289,#205290,#205291,#205292,
#205293,#205294),(#205295,#205296,#205297,#205298,#205299,#205300,#205301),
(#205302,#205303,#205304,#205305,#205306,#205307,#205308),(#205309,#205310,
#205311,#205312,#205313,#205314,#205315),(#205316,#205317,#205318,#205319,
#205320,#205321,#205322),(#205323,#205324,#205325,#205326,#205327,#205328,
#205329)),.UNSPECIFIED.,.F.,.F.,.F.,(4,1,1,1,1,1,1,1,4),(4,3,4),(0.,0.124999999999997,
0.249999999999998,0.375,0.5,0.625,0.75,0.875,1.),(0.,1.,1.01),
 .UNSPECIFIED.);
#920=B_SPLINE_SURFACE_WITH_KNOTS('',3,3,((#205335,#205336,#205337,#205338,
#205339,#205340,#205341),(#205342,#205343,#205344,#205345,#205346,#205347,
#205348),(#205349,#205350,#205351,#205352,#205353,#205354,#205355),(#205356,
#205357,#205358,#205359,#205360,#205361,#205362),(#205363,#205364,#205365,
#205366,#205367,#205368,#205369),(#205370,#205371,#205372,#205373,#205374,
#205375,#205376),(#205377,#205378,#205379,#205380,#205381,#205382,#205383),
(#205384,#205385,#205386,#205387,#205388,#205389,#205390),(#205391,#205392,
#205393,#205394,#205395,#205396,#205397),(#205398,#205399,#205400,#205401,
#205402,#205403,#205404),(#205405,#205406,#205407,#205408,#205409,#205410,
#205411),(#205412,#205413,#205414,#205415,#205416,#205417,#205418),(#205419,
#205420,#205421,#205422,#205423,#205424,#205425),(#205426,#205427,#205428,
#205429,#205430,#205431,#205432),(#205433,#205434,#205435,#205436,#205437,
#205438,#205439),(#205440,#205441,#205442,#205443,#205444,#205445,#205446),
(#205447,#205448,#205449,#205450,#205451,#205452,#205453)),
 .UNSPECIFIED.,.F.,.F.,.F.,(4,3,1,1,1,1,1,1,1,3,4),(4,3,4),(-0.01,0.,0.125,
0.25,0.375,0.5,0.625,0.75,0.875,1.,1.01),(0.,1.,1.01),.UNSPECIFIED.);
#921=B_SPLINE_SURFACE_WITH_KNOTS('',3,3,((#205503,#205504,#205505,#205506),
(#205507,#205508,#205509,#205510),(#205511,#205512,#205513,#205514),(#205515,
#205516,#205517,#205518),(#205519,#205520,#205521,#205522),(#205523,#205524,
#205525,#205526),(#205527,#205528,#205529,#205530)),.UNSPECIFIED.,.F.,.F.,
 .F.,(4,1,1,1,4),(4,4),(0.,0.25,0.5,0.75,1.),(0.,1.),.UNSPECIFIED.);
#922=B_SPLINE_SURFACE_WITH_KNOTS('',3,3,((#205531,#205532,#205533,#205534,
#205535,#205536,#205537),(#205538,#205539,#205540,#205541,#205542,#205543,
#205544),(#205545,#205546,#205547,#205548,#205549,#205550,#205551),(#205552,
#205553,#205554,#205555,#205556,#205557,#205558),(#205559,#205560,#205561,
#205562,#205563,#205564,#205565),(#205566,#205567,#205568,#205569,#205570,
#205571,#205572),(#205573,#205574,#205575,#205576,#205577,#205578,#205579)),
 .UNSPECIFIED.,.F.,.F.,.F.,(4,1,1,1,4),(4,3,4),(0.,0.25,0.5,0.75,1.),(0.,
1.,1.01),.UNSPECIFIED.);
#923=B_SPLINE_SURFACE_WITH_KNOTS('',3,3,((#205581,#205582,#205583,#205584,
#205585,#205586,#205587),(#205588,#205589,#205590,#205591,#205592,#205593,
#205594),(#205595,#205596,#205597,#205598,#205599,#205600,#205601),(#205602,
#205603,#205604,#205605,#205606,#205607,#205608),(#205609,#205610,#205611,
#205612,#205613,#205614,#205615),(#205616,#205617,#205618,#205619,#205620,
#205621,#205622),(#205623,#205624,#205625,#205626,#205627,#205628,#205629)),
 .UNSPECIFIED.,.F.,.F.,.F.,(4,1,1,1,4),(4,3,4),(0.,0.25,0.5,0.75,1.),(0.,
1.,1.01),.UNSPECIFIED.);
#924=B_SPLINE_SURFACE_WITH_KNOTS('',3,3,((#205630,#205631,#205632,#205633,
#205634,#205635,#205636),(#205637,#205638,#205639,#205640,#205641,#205642,
#205643),(#205644,#205645,#205646,#205647,#205648,#205649,#205650),(#205651,
#205652,#205653,#205654,#205655,#205656,#205657),(#205658,#205659,#205660,
#205661,#205662,#205663,#205664),(#205665,#205666,#205667,#205668,#205669,
#205670,#205671),(#205672,#205673,#205674,#205675,#205676,#205677,#205678)),
 .UNSPECIFIED.,.F.,.F.,.F.,(4,1,1,1,4),(4,3,4),(0.,0.25,0.5,0.75,1.),(0.,
1.,1.01),.UNSPECIFIED.);
#925=B_SPLINE_SURFACE_WITH_KNOTS('',3,3,((#205680,#205681,#205682,#205683,
#205684,#205685,#205686,#205687,#205688,#205689,#205690,#205691,#205692,
#205693,#205694,#205695),(#205696,#205697,#205698,#205699,#205700,#205701,
#205702,#205703,#205704,#205705,#205706,#205707,#205708,#205709,#205710,
#205711),(#205712,#205713,#205714,#205715,#205716,#205717,#205718,#205719,
#205720,#205721,#205722,#205723,#205724,#205725,#205726,#205727),(#205728,
#205729,#205730,#205731,#205732,#205733,#205734,#205735,#205736,#205737,
#205738,#205739,#205740,#205741,#205742,#205743),(#205744,#205745,#205746,
#205747,#205748,#205749,#205750,#205751,#205752,#205753,#205754,#205755,
#205756,#205757,#205758,#205759),(#205760,#205761,#205762,#205763,#205764,
#205765,#205766,#205767,#205768,#205769,#205770,#205771,#205772,#205773,
#205774,#205775),(#205776,#205777,#205778,#205779,#205780,#205781,#205782,
#205783,#205784,#205785,#205786,#205787,#205788,#205789,#205790,#205791),
(#205792,#205793,#205794,#205795,#205796,#205797,#205798,#205799,#205800,
#205801,#205802,#205803,#205804,#205805,#205806,#205807),(#205808,#205809,
#205810,#205811,#205812,#205813,#205814,#205815,#205816,#205817,#205818,
#205819,#205820,#205821,#205822,#205823),(#205824,#205825,#205826,#205827,
#205828,#205829,#205830,#205831,#205832,#205833,#205834,#205835,#205836,
#205837,#205838,#205839),(#205840,#205841,#205842,#205843,#205844,#205845,
#205846,#205847,#205848,#205849,#205850,#205851,#205852,#205853,#205854,
#205855),(#205856,#205857,#205858,#205859,#205860,#205861,#205862,#205863,
#205864,#205865,#205866,#205867,#205868,#205869,#205870,#205871),(#205872,
#205873,#205874,#205875,#205876,#205877,#205878,#205879,#205880,#205881,
#205882,#205883,#205884,#205885,#205886,#205887),(#205888,#205889,#205890,
#205891,#205892,#205893,#205894,#205895,#205896,#205897,#205898,#205899,
#205900,#205901,#205902,#205903),(#205904,#205905,#205906,#205907,#205908,
#205909,#205910,#205911,#205912,#205913,#205914,#205915,#205916,#205917,
#205918,#205919),(#205920,#205921,#205922,#205923,#205924,#205925,#205926,
#205927,#205928,#205929,#205930,#205931,#205932,#205933,#205934,#205935),
(#205936,#205937,#205938,#205939,#205940,#205941,#205942,#205943,#205944,
#205945,#205946,#205947,#205948,#205949,#205950,#205951),(#205952,#205953,
#205954,#205955,#205956,#205957,#205958,#205959,#205960,#205961,#205962,
#205963,#205964,#205965,#205966,#205967),(#205968,#205969,#205970,#205971,
#205972,#205973,#205974,#205975,#205976,#205977,#205978,#205979,#205980,
#205981,#205982,#205983),(#205984,#205985,#205986,#205987,#205988,#205989,
#205990,#205991,#205992,#205993,#205994,#205995,#205996,#205997,#205998,
#205999),(#206000,#206001,#206002,#206003,#206004,#206005,#206006,#206007,
#206008,#206009,#206010,#206011,#206012,#206013,#206014,#206015),(#206016,
#206017,#206018,#206019,#206020,#206021,#206022,#206023,#206024,#206025,
#206026,#206027,#206028,#206029,#206030,#206031),(#206032,#206033,#206034,
#206035,#206036,#206037,#206038,#206039,#206040,#206041,#206042,#206043,
#206044,#206045,#206046,#206047),(#206048,#206049,#206050,#206051,#206052,
#206053,#206054,#206055,#206056,#206057,#206058,#206059,#206060,#206061,
#206062,#206063),(#206064,#206065,#206066,#206067,#206068,#206069,#206070,
#206071,#206072,#206073,#206074,#206075,#206076,#206077,#206078,#206079),
(#206080,#206081,#206082,#206083,#206084,#206085,#206086,#206087,#206088,
#206089,#206090,#206091,#206092,#206093,#206094,#206095),(#206096,#206097,
#206098,#206099,#206100,#206101,#206102,#206103,#206104,#206105,#206106,
#206107,#206108,#206109,#206110,#206111),(#206112,#206113,#206114,#206115,
#206116,#206117,#206118,#206119,#206120,#206121,#206122,#206123,#206124,
#206125,#206126,#206127),(#206128,#206129,#206130,#206131,#206132,#206133,
#206134,#206135,#206136,#206137,#206138,#206139,#206140,#206141,#206142,
#206143),(#206144,#206145,#206146,#206147,#206148,#206149,#206150,#206151,
#206152,#206153,#206154,#206155,#206156,#206157,#206158,#206159),(#206160,
#206161,#206162,#206163,#206164,#206165,#206166,#206167,#206168,#206169,
#206170,#206171,#206172,#206173,#206174,#206175),(#206176,#206177,#206178,
#206179,#206180,#206181,#206182,#206183,#206184,#206185,#206186,#206187,
#206188,#206189,#206190,#206191),(#206192,#206193,#206194,#206195,#206196,
#206197,#206198,#206199,#206200,#206201,#206202,#206203,#206204,#206205,
#206206,#206207),(#206208,#206209,#206210,#206211,#206212,#206213,#206214,
#206215,#206216,#206217,#206218,#206219,#206220,#206221,#206222,#206223),
(#206224,#206225,#206226,#206227,#206228,#206229,#206230,#206231,#206232,
#206233,#206234,#206235,#206236,#206237,#206238,#206239),(#206240,#206241,
#206242,#206243,#206244,#206245,#206246,#206247,#206248,#206249,#206250,
#206251,#206252,#206253,#206254,#206255),(#206256,#206257,#206258,#206259,
#206260,#206261,#206262,#206263,#206264,#206265,#206266,#206267,#206268,
#206269,#206270,#206271),(#206272,#206273,#206274,#206275,#206276,#206277,
#206278,#206279,#206280,#206281,#206282,#206283,#206284,#206285,#206286,
#206287),(#206288,#206289,#206290,#206291,#206292,#206293,#206294,#206295,
#206296,#206297,#206298,#206299,#206300,#206301,#206302,#206303),(#206304,
#206305,#206306,#206307,#206308,#206309,#206310,#206311,#206312,#206313,
#206314,#206315,#206316,#206317,#206318,#206319),(#206320,#206321,#206322,
#206323,#206324,#206325,#206326,#206327,#206328,#206329,#206330,#206331,
#206332,#206333,#206334,#206335),(#206336,#206337,#206338,#206339,#206340,
#206341,#206342,#206343,#206344,#206345,#206346,#206347,#206348,#206349,
#206350,#206351),(#206352,#206353,#206354,#206355,#206356,#206357,#206358,
#206359,#206360,#206361,#206362,#206363,#206364,#206365,#206366,#206367)),
 .UNSPECIFIED.,.F.,.F.,.F.,(4,3,3,3,3,3,3,1,1,1,3,3,3,3,3,3,4),(4,3,3,3,
3,4),(-364.,-121.,-40.,-13.,-4.,-1.,0.,0.25,0.5,0.75,1.,2.,5.,14.,41.,122.,
365.),(-7.07,-3.03,-1.01,0.,1.,1.01),.UNSPECIFIED.);
#926=B_SPLINE_SURFACE_WITH_KNOTS('',3,3,((#206369,#206370,#206371,#206372,
#206373,#206374,#206375,#206376,#206377,#206378,#206379,#206380,#206381,
#206382,#206383,#206384),(#206385,#206386,#206387,#206388,#206389,#206390,
#206391,#206392,#206393,#206394,#206395,#206396,#206397,#206398,#206399,
#206400),(#206401,#206402,#206403,#206404,#206405,#206406,#206407,#206408,
#206409,#206410,#206411,#206412,#206413,#206414,#206415,#206416),(#206417,
#206418,#206419,#206420,#206421,#206422,#206423,#206424,#206425,#206426,
#206427,#206428,#206429,#206430,#206431,#206432),(#206433,#206434,#206435,
#206436,#206437,#206438,#206439,#206440,#206441,#206442,#206443,#206444,
#206445,#206446,#206447,#206448),(#206449,#206450,#206451,#206452,#206453,
#206454,#206455,#206456,#206457,#206458,#206459,#206460,#206461,#206462,
#206463,#206464),(#206465,#206466,#206467,#206468,#206469,#206470,#206471,
#206472,#206473,#206474,#206475,#206476,#206477,#206478,#206479,#206480),
(#206481,#206482,#206483,#206484,#206485,#206486,#206487,#206488,#206489,
#206490,#206491,#206492,#206493,#206494,#206495,#206496),(#206497,#206498,
#206499,#206500,#206501,#206502,#206503,#206504,#206505,#206506,#206507,
#206508,#206509,#206510,#206511,#206512),(#206513,#206514,#206515,#206516,
#206517,#206518,#206519,#206520,#206521,#206522,#206523,#206524,#206525,
#206526,#206527,#206528),(#206529,#206530,#206531,#206532,#206533,#206534,
#206535,#206536,#206537,#206538,#206539,#206540,#206541,#206542,#206543,
#206544),(#206545,#206546,#206547,#206548,#206549,#206550,#206551,#206552,
#206553,#206554,#206555,#206556,#206557,#206558,#206559,#206560),(#206561,
#206562,#206563,#206564,#206565,#206566,#206567,#206568,#206569,#206570,
#206571,#206572,#206573,#206574,#206575,#206576),(#206577,#206578,#206579,
#206580,#206581,#206582,#206583,#206584,#206585,#206586,#206587,#206588,
#206589,#206590,#206591,#206592),(#206593,#206594,#206595,#206596,#206597,
#206598,#206599,#206600,#206601,#206602,#206603,#206604,#206605,#206606,
#206607,#206608),(#206609,#206610,#206611,#206612,#206613,#206614,#206615,
#206616,#206617,#206618,#206619,#206620,#206621,#206622,#206623,#206624),
(#206625,#206626,#206627,#206628,#206629,#206630,#206631,#206632,#206633,
#206634,#206635,#206636,#206637,#206638,#206639,#206640),(#206641,#206642,
#206643,#206644,#206645,#206646,#206647,#206648,#206649,#206650,#206651,
#206652,#206653,#206654,#206655,#206656),(#206657,#206658,#206659,#206660,
#206661,#206662,#206663,#206664,#206665,#206666,#206667,#206668,#206669,
#206670,#206671,#206672),(#206673,#206674,#206675,#206676,#206677,#206678,
#206679,#206680,#206681,#206682,#206683,#206684,#206685,#206686,#206687,
#206688),(#206689,#206690,#206691,#206692,#206693,#206694,#206695,#206696,
#206697,#206698,#206699,#206700,#206701,#206702,#206703,#206704),(#206705,
#206706,#206707,#206708,#206709,#206710,#206711,#206712,#206713,#206714,
#206715,#206716,#206717,#206718,#206719,#206720),(#206721,#206722,#206723,
#206724,#206725,#206726,#206727,#206728,#206729,#206730,#206731,#206732,
#206733,#206734,#206735,#206736),(#206737,#206738,#206739,#206740,#206741,
#206742,#206743,#206744,#206745,#206746,#206747,#206748,#206749,#206750,
#206751,#206752),(#206753,#206754,#206755,#206756,#206757,#206758,#206759,
#206760,#206761,#206762,#206763,#206764,#206765,#206766,#206767,#206768),
(#206769,#206770,#206771,#206772,#206773,#206774,#206775,#206776,#206777,
#206778,#206779,#206780,#206781,#206782,#206783,#206784),(#206785,#206786,
#206787,#206788,#206789,#206790,#206791,#206792,#206793,#206794,#206795,
#206796,#206797,#206798,#206799,#206800),(#206801,#206802,#206803,#206804,
#206805,#206806,#206807,#206808,#206809,#206810,#206811,#206812,#206813,
#206814,#206815,#206816),(#206817,#206818,#206819,#206820,#206821,#206822,
#206823,#206824,#206825,#206826,#206827,#206828,#206829,#206830,#206831,
#206832),(#206833,#206834,#206835,#206836,#206837,#206838,#206839,#206840,
#206841,#206842,#206843,#206844,#206845,#206846,#206847,#206848),(#206849,
#206850,#206851,#206852,#206853,#206854,#206855,#206856,#206857,#206858,
#206859,#206860,#206861,#206862,#206863,#206864),(#206865,#206866,#206867,
#206868,#206869,#206870,#206871,#206872,#206873,#206874,#206875,#206876,
#206877,#206878,#206879,#206880),(#206881,#206882,#206883,#206884,#206885,
#206886,#206887,#206888,#206889,#206890,#206891,#206892,#206893,#206894,
#206895,#206896),(#206897,#206898,#206899,#206900,#206901,#206902,#206903,
#206904,#206905,#206906,#206907,#206908,#206909,#206910,#206911,#206912),
(#206913,#206914,#206915,#206916,#206917,#206918,#206919,#206920,#206921,
#206922,#206923,#206924,#206925,#206926,#206927,#206928),(#206929,#206930,
#206931,#206932,#206933,#206934,#206935,#206936,#206937,#206938,#206939,
#206940,#206941,#206942,#206943,#206944),(#206945,#206946,#206947,#206948,
#206949,#206950,#206951,#206952,#206953,#206954,#206955,#206956,#206957,
#206958,#206959,#206960)),.UNSPECIFIED.,.F.,.F.,.F.,(4,3,3,3,3,3,1,1,1,
3,3,3,3,3,4),(4,3,3,3,3,4),(-121.,-40.,-13.,-4.,-1.,0.,0.25,0.5,0.75,1.,
2.,5.,14.,41.,122.),(-7.07,-3.03,-1.01,0.,1.,1.01),.UNSPECIFIED.);
#927=B_SPLINE_SURFACE_WITH_KNOTS('',3,3,((#223433,#223434,#223435,#223436,
#223437,#223438,#223439),(#223440,#223441,#223442,#223443,#223444,#223445,
#223446),(#223447,#223448,#223449,#223450,#223451,#223452,#223453),(#223454,
#223455,#223456,#223457,#223458,#223459,#223460),(#223461,#223462,#223463,
#223464,#223465,#223466,#223467),(#223468,#223469,#223470,#223471,#223472,
#223473,#223474),(#223475,#223476,#223477,#223478,#223479,#223480,#223481),
(#223482,#223483,#223484,#223485,#223486,#223487,#223488),(#223489,#223490,
#223491,#223492,#223493,#223494,#223495),(#223496,#223497,#223498,#223499,
#223500,#223501,#223502),(#223503,#223504,#223505,#223506,#223507,#223508,
#223509),(#223510,#223511,#223512,#223513,#223514,#223515,#223516),(#223517,
#223518,#223519,#223520,#223521,#223522,#223523),(#223524,#223525,#223526,
#223527,#223528,#223529,#223530),(#223531,#223532,#223533,#223534,#223535,
#223536,#223537),(#223538,#223539,#223540,#223541,#223542,#223543,#223544),
(#223545,#223546,#223547,#223548,#223549,#223550,#223551),(#223552,#223553,
#223554,#223555,#223556,#223557,#223558),(#223559,#223560,#223561,#223562,
#223563,#223564,#223565),(#223566,#223567,#223568,#223569,#223570,#223571,
#223572),(#223573,#223574,#223575,#223576,#223577,#223578,#223579),(#223580,
#223581,#223582,#223583,#223584,#223585,#223586),(#223587,#223588,#223589,
#223590,#223591,#223592,#223593),(#223594,#223595,#223596,#223597,#223598,
#223599,#223600),(#223601,#223602,#223603,#223604,#223605,#223606,#223607),
(#223608,#223609,#223610,#223611,#223612,#223613,#223614),(#223615,#223616,
#223617,#223618,#223619,#223620,#223621),(#223622,#223623,#223624,#223625,
#223626,#223627,#223628),(#223629,#223630,#223631,#223632,#223633,#223634,
#223635),(#223636,#223637,#223638,#223639,#223640,#223641,#223642),(#223643,
#223644,#223645,#223646,#223647,#223648,#223649),(#223650,#223651,#223652,
#223653,#223654,#223655,#223656),(#223657,#223658,#223659,#223660,#223661,
#223662,#223663),(#223664,#223665,#223666,#223667,#223668,#223669,#223670),
(#223671,#223672,#223673,#223674,#223675,#223676,#223677),(#223678,#223679,
#223680,#223681,#223682,#223683,#223684),(#223685,#223686,#223687,#223688,
#223689,#223690,#223691),(#223692,#223693,#223694,#223695,#223696,#223697,
#223698),(#223699,#223700,#223701,#223702,#223703,#223704,#223705),(#223706,
#223707,#223708,#223709,#223710,#223711,#223712),(#223713,#223714,#223715,
#223716,#223717,#223718,#223719),(#223720,#223721,#223722,#223723,#223724,
#223725,#223726),(#223727,#223728,#223729,#223730,#223731,#223732,#223733),
(#223734,#223735,#223736,#223737,#223738,#223739,#223740),(#223741,#223742,
#223743,#223744,#223745,#223746,#223747),(#223748,#223749,#223750,#223751,
#223752,#223753,#223754),(#223755,#223756,#223757,#223758,#223759,#223760,
#223761),(#223762,#223763,#223764,#223765,#223766,#223767,#223768),(#223769,
#223770,#223771,#223772,#223773,#223774,#223775),(#223776,#223777,#223778,
#223779,#223780,#223781,#223782),(#223783,#223784,#223785,#223786,#223787,
#223788,#223789),(#223790,#223791,#223792,#223793,#223794,#223795,#223796),
(#223797,#223798,#223799,#223800,#223801,#223802,#223803),(#223804,#223805,
#223806,#223807,#223808,#223809,#223810),(#223811,#223812,#223813,#223814,
#223815,#223816,#223817),(#223818,#223819,#223820,#223821,#223822,#223823,
#223824),(#223825,#223826,#223827,#223828,#223829,#223830,#223831),(#223832,
#223833,#223834,#223835,#223836,#223837,#223838),(#223839,#223840,#223841,
#223842,#223843,#223844,#223845),(#223846,#223847,#223848,#223849,#223850,
#223851,#223852),(#223853,#223854,#223855,#223856,#223857,#223858,#223859),
(#223860,#223861,#223862,#223863,#223864,#223865,#223866),(#223867,#223868,
#223869,#223870,#223871,#223872,#223873),(#223874,#223875,#223876,#223877,
#223878,#223879,#223880),(#223881,#223882,#223883,#223884,#223885,#223886,
#223887),(#223888,#223889,#223890,#223891,#223892,#223893,#223894),(#223895,
#223896,#223897,#223898,#223899,#223900,#223901),(#223902,#223903,#223904,
#223905,#223906,#223907,#223908),(#223909,#223910,#223911,#223912,#223913,
#223914,#223915),(#223916,#223917,#223918,#223919,#223920,#223921,#223922),
(#223923,#223924,#223925,#223926,#223927,#223928,#223929),(#223930,#223931,
#223932,#223933,#223934,#223935,#223936),(#223937,#223938,#223939,#223940,
#223941,#223942,#223943),(#223944,#223945,#223946,#223947,#223948,#223949,
#223950),(#223951,#223952,#223953,#223954,#223955,#223956,#223957),(#223958,
#223959,#223960,#223961,#223962,#223963,#223964),(#223965,#223966,#223967,
#223968,#223969,#223970,#223971),(#223972,#223973,#223974,#223975,#223976,
#223977,#223978),(#223979,#223980,#223981,#223982,#223983,#223984,#223985),
(#223986,#223987,#223988,#223989,#223990,#223991,#223992),(#223993,#223994,
#223995,#223996,#223997,#223998,#223999),(#224000,#224001,#224002,#224003,
#224004,#224005,#224006),(#224007,#224008,#224009,#224010,#224011,#224012,
#224013),(#224014,#224015,#224016,#224017,#224018,#224019,#224020),(#224021,
#224022,#224023,#224024,#224025,#224026,#224027),(#224028,#224029,#224030,
#224031,#224032,#224033,#224034),(#224035,#224036,#224037,#224038,#224039,
#224040,#224041),(#224042,#224043,#224044,#224045,#224046,#224047,#224048),
(#224049,#224050,#224051,#224052,#224053,#224054,#224055),(#224056,#224057,
#224058,#224059,#224060,#224061,#224062),(#224063,#224064,#224065,#224066,
#224067,#224068,#224069),(#224070,#224071,#224072,#224073,#224074,#224075,
#224076),(#224077,#224078,#224079,#224080,#224081,#224082,#224083),(#224084,
#224085,#224086,#224087,#224088,#224089,#224090),(#224091,#224092,#224093,
#224094,#224095,#224096,#224097),(#224098,#224099,#224100,#224101,#224102,
#224103,#224104),(#224105,#224106,#224107,#224108,#224109,#224110,#224111),
(#224112,#224113,#224114,#224115,#224116,#224117,#224118),(#224119,#224120,
#224121,#224122,#224123,#224124,#224125),(#224126,#224127,#224128,#224129,
#224130,#224131,#224132),(#224133,#224134,#224135,#224136,#224137,#224138,
#224139),(#224140,#224141,#224142,#224143,#224144,#224145,#224146),(#224147,
#224148,#224149,#224150,#224151,#224152,#224153),(#224154,#224155,#224156,
#224157,#224158,#224159,#224160),(#224161,#224162,#224163,#224164,#224165,
#224166,#224167),(#224168,#224169,#224170,#224171,#224172,#224173,#224174),
(#224175,#224176,#224177,#224178,#224179,#224180,#224181),(#224182,#224183,
#224184,#224185,#224186,#224187,#224188),(#224189,#224190,#224191,#224192,
#224193,#224194,#224195),(#224196,#224197,#224198,#224199,#224200,#224201,
#224202),(#224203,#224204,#224205,#224206,#224207,#224208,#224209),(#224210,
#224211,#224212,#224213,#224214,#224215,#224216),(#224217,#224218,#224219,
#224220,#224221,#224222,#224223),(#224224,#224225,#224226,#224227,#224228,
#224229,#224230),(#224231,#224232,#224233,#224234,#224235,#224236,#224237),
(#224238,#224239,#224240,#224241,#224242,#224243,#224244),(#224245,#224246,
#224247,#224248,#224249,#224250,#224251),(#224252,#224253,#224254,#224255,
#224256,#224257,#224258),(#224259,#224260,#224261,#224262,#224263,#224264,
#224265),(#224266,#224267,#224268,#224269,#224270,#224271,#224272),(#224273,
#224274,#224275,#224276,#224277,#224278,#224279),(#224280,#224281,#224282,
#224283,#224284,#224285,#224286),(#224287,#224288,#224289,#224290,#224291,
#224292,#224293),(#224294,#224295,#224296,#224297,#224298,#224299,#224300),
(#224301,#224302,#224303,#224304,#224305,#224306,#224307),(#224308,#224309,
#224310,#224311,#224312,#224313,#224314),(#224315,#224316,#224317,#224318,
#224319,#224320,#224321),(#224322,#224323,#224324,#224325,#224326,#224327,
#224328),(#224329,#224330,#224331,#224332,#224333,#224334,#224335),(#224336,
#224337,#224338,#224339,#224340,#224341,#224342),(#224343,#224344,#224345,
#224346,#224347,#224348,#224349),(#224350,#224351,#224352,#224353,#224354,
#224355,#224356),(#224357,#224358,#224359,#224360,#224361,#224362,#224363),
(#224364,#224365,#224366,#224367,#224368,#224369,#224370),(#224371,#224372,
#224373,#224374,#224375,#224376,#224377),(#224378,#224379,#224380,#224381,
#224382,#224383,#224384),(#224385,#224386,#224387,#224388,#224389,#224390,
#224391),(#224392,#224393,#224394,#224395,#224396,#224397,#224398),(#224399,
#224400,#224401,#224402,#224403,#224404,#224405),(#224406,#224407,#224408,
#224409,#224410,#224411,#224412),(#224413,#224414,#224415,#224416,#224417,
#224418,#224419),(#224420,#224421,#224422,#224423,#224424,#224425,#224426),
(#224427,#224428,#224429,#224430,#224431,#224432,#224433),(#224434,#224435,
#224436,#224437,#224438,#224439,#224440),(#224441,#224442,#224443,#224444,
#224445,#224446,#224447),(#224448,#224449,#224450,#224451,#224452,#224453,
#224454),(#224455,#224456,#224457,#224458,#224459,#224460,#224461),(#224462,
#224463,#224464,#224465,#224466,#224467,#224468),(#224469,#224470,#224471,
#224472,#224473,#224474,#224475),(#224476,#224477,#224478,#224479,#224480,
#224481,#224482),(#224483,#224484,#224485,#224486,#224487,#224488,#224489),
(#224490,#224491,#224492,#224493,#224494,#224495,#224496),(#224497,#224498,
#224499,#224500,#224501,#224502,#224503),(#224504,#224505,#224506,#224507,
#224508,#224509,#224510),(#224511,#224512,#224513,#224514,#224515,#224516,
#224517),(#224518,#224519,#224520,#224521,#224522,#224523,#224524),(#224525,
#224526,#224527,#224528,#224529,#224530,#224531),(#224532,#224533,#224534,
#224535,#224536,#224537,#224538),(#224539,#224540,#224541,#224542,#224543,
#224544,#224545),(#224546,#224547,#224548,#224549,#224550,#224551,#224552),
(#224553,#224554,#224555,#224556,#224557,#224558,#224559),(#224560,#224561,
#224562,#224563,#224564,#224565,#224566),(#224567,#224568,#224569,#224570,
#224571,#224572,#224573),(#224574,#224575,#224576,#224577,#224578,#224579,
#224580),(#224581,#224582,#224583,#224584,#224585,#224586,#224587),(#224588,
#224589,#224590,#224591,#224592,#224593,#224594),(#224595,#224596,#224597,
#224598,#224599,#224600,#224601),(#224602,#224603,#224604,#224605,#224606,
#224607,#224608),(#224609,#224610,#224611,#224612,#224613,#224614,#224615),
(#224616,#224617,#224618,#224619,#224620,#224621,#224622),(#224623,#224624,
#224625,#224626,#224627,#224628,#224629),(#224630,#224631,#224632,#224633,
#224634,#224635,#224636),(#224637,#224638,#224639,#224640,#224641,#224642,
#224643),(#224644,#224645,#224646,#224647,#224648,#224649,#224650),(#224651,
#224652,#224653,#224654,#224655,#224656,#224657)),.UNSPECIFIED.,.F.,.F.,
 .F.,(4,3,3,3,3,3,3,3,3,3,3,3,3,3,3,3,3,3,3,3,3,3,3,3,3,3,3,3,3,3,3,3,3,
3,3,3,3,3,3,3,3,3,3,3,3,3,3,3,3,3,3,3,3,3,3,3,3,3,4),(4,3,4),(-0.00276391227871182,
0.0600815767561073,0.122927065790926,0.138638438049631,0.1396203988158,
0.140111379198885,0.140602359581969,0.142566281114307,0.146494124178983,
0.154349810308336,0.185772554825745,0.248618043860565,0.264329416119269,
0.272185102248622,0.276112945313298,0.277094906079467,0.278076866845636,
0.280040788377974,0.311463532895383,0.374309021930203,0.405731766447612,
0.421443138706317,0.421934119089401,0.422425099472486,0.423407060238655,
0.425370981770993,0.42929882483567,0.437154510965022,0.468577255482431,
0.499999999999841,0.53142274451725,0.56284548903466,0.570701175164012,0.574629018228689,
0.576592939761027,0.577574900527196,0.57806588091028,0.578556861293365,
0.59426823355207,0.625690978069479,0.688536467104298,0.719959211621708,
0.721923133154046,0.722905093920215,0.723887054686384,0.72781489775106,
0.735670583880413,0.751381956139117,0.814227445173936,0.845650189691346,
0.853505875820698,0.857433718885374,0.859397640417713,0.859888620800797,
0.860379601183882,0.861361561950051,0.877072934208755,0.939918423243574,
1.00276391227839),(-0.034810747309642,0.460156458726841,0.955123664763324),
 .UNSPECIFIED.);
#928=B_SPLINE_SURFACE_WITH_KNOTS('',3,3,((#224988,#224989,#224990,#224991),
(#224992,#224993,#224994,#224995),(#224996,#224997,#224998,#224999),(#225000,
#225001,#225002,#225003),(#225004,#225005,#225006,#225007),(#225008,#225009,
#225010,#225011),(#225012,#225013,#225014,#225015),(#225016,#225017,#225018,
#225019),(#225020,#225021,#225022,#225023),(#225024,#225025,#225026,#225027),
(#225028,#225029,#225030,#225031),(#225032,#225033,#225034,#225035),(#225036,
#225037,#225038,#225039),(#225040,#225041,#225042,#225043),(#225044,#225045,
#225046,#225047),(#225048,#225049,#225050,#225051),(#225052,#225053,#225054,
#225055),(#225056,#225057,#225058,#225059),(#225060,#225061,#225062,#225063),
(#225064,#225065,#225066,#225067),(#225068,#225069,#225070,#225071),(#225072,
#225073,#225074,#225075),(#225076,#225077,#225078,#225079),(#225080,#225081,
#225082,#225083),(#225084,#225085,#225086,#225087),(#225088,#225089,#225090,
#225091),(#225092,#225093,#225094,#225095),(#225096,#225097,#225098,#225099),
(#225100,#225101,#225102,#225103),(#225104,#225105,#225106,#225107),(#225108,
#225109,#225110,#225111),(#225112,#225113,#225114,#225115),(#225116,#225117,
#225118,#225119),(#225120,#225121,#225122,#225123),(#225124,#225125,#225126,
#225127),(#225128,#225129,#225130,#225131),(#225132,#225133,#225134,#225135),
(#225136,#225137,#225138,#225139),(#225140,#225141,#225142,#225143),(#225144,
#225145,#225146,#225147),(#225148,#225149,#225150,#225151),(#225152,#225153,
#225154,#225155),(#225156,#225157,#225158,#225159),(#225160,#225161,#225162,
#225163),(#225164,#225165,#225166,#225167),(#225168,#225169,#225170,#225171),
(#225172,#225173,#225174,#225175),(#225176,#225177,#225178,#225179),(#225180,
#225181,#225182,#225183),(#225184,#225185,#225186,#225187),(#225188,#225189,
#225190,#225191),(#225192,#225193,#225194,#225195),(#225196,#225197,#225198,
#225199),(#225200,#225201,#225202,#225203),(#225204,#225205,#225206,#225207),
(#225208,#225209,#225210,#225211),(#225212,#225213,#225214,#225215),(#225216,
#225217,#225218,#225219),(#225220,#225221,#225222,#225223),(#225224,#225225,
#225226,#225227),(#225228,#225229,#225230,#225231),(#225232,#225233,#225234,
#225235),(#225236,#225237,#225238,#225239),(#225240,#225241,#225242,#225243),
(#225244,#225245,#225246,#225247),(#225248,#225249,#225250,#225251),(#225252,
#225253,#225254,#225255),(#225256,#225257,#225258,#225259),(#225260,#225261,
#225262,#225263),(#225264,#225265,#225266,#225267),(#225268,#225269,#225270,
#225271),(#225272,#225273,#225274,#225275),(#225276,#225277,#225278,#225279),
(#225280,#225281,#225282,#225283),(#225284,#225285,#225286,#225287),(#225288,
#225289,#225290,#225291),(#225292,#225293,#225294,#225295),(#225296,#225297,
#225298,#225299),(#225300,#225301,#225302,#225303),(#225304,#225305,#225306,
#225307),(#225308,#225309,#225310,#225311),(#225312,#225313,#225314,#225315),
(#225316,#225317,#225318,#225319),(#225320,#225321,#225322,#225323),(#225324,
#225325,#225326,#225327),(#225328,#225329,#225330,#225331),(#225332,#225333,
#225334,#225335),(#225336,#225337,#225338,#225339),(#225340,#225341,#225342,
#225343),(#225344,#225345,#225346,#225347),(#225348,#225349,#225350,#225351),
(#225352,#225353,#225354,#225355),(#225356,#225357,#225358,#225359),(#225360,
#225361,#225362,#225363),(#225364,#225365,#225366,#225367),(#225368,#225369,
#225370,#225371),(#225372,#225373,#225374,#225375),(#225376,#225377,#225378,
#225379),(#225380,#225381,#225382,#225383),(#225384,#225385,#225386,#225387),
(#225388,#225389,#225390,#225391),(#225392,#225393,#225394,#225395),(#225396,
#225397,#225398,#225399),(#225400,#225401,#225402,#225403),(#225404,#225405,
#225406,#225407),(#225408,#225409,#225410,#225411),(#225412,#225413,#225414,
#225415),(#225416,#225417,#225418,#225419),(#225420,#225421,#225422,#225423),
(#225424,#225425,#225426,#225427),(#225428,#225429,#225430,#225431),(#225432,
#225433,#225434,#225435),(#225436,#225437,#225438,#225439),(#225440,#225441,
#225442,#225443),(#225444,#225445,#225446,#225447),(#225448,#225449,#225450,
#225451),(#225452,#225453,#225454,#225455),(#225456,#225457,#225458,#225459),
(#225460,#225461,#225462,#225463),(#225464,#225465,#225466,#225467),(#225468,
#225469,#225470,#225471),(#225472,#225473,#225474,#225475),(#225476,#225477,
#225478,#225479),(#225480,#225481,#225482,#225483),(#225484,#225485,#225486,
#225487),(#225488,#225489,#225490,#225491),(#225492,#225493,#225494,#225495),
(#225496,#225497,#225498,#225499),(#225500,#225501,#225502,#225503),(#225504,
#225505,#225506,#225507),(#225508,#225509,#225510,#225511),(#225512,#225513,
#225514,#225515),(#225516,#225517,#225518,#225519),(#225520,#225521,#225522,
#225523),(#225524,#225525,#225526,#225527),(#225528,#225529,#225530,#225531),
(#225532,#225533,#225534,#225535),(#225536,#225537,#225538,#225539),(#225540,
#225541,#225542,#225543),(#225544,#225545,#225546,#225547),(#225548,#225549,
#225550,#225551),(#225552,#225553,#225554,#225555),(#225556,#225557,#225558,
#225559),(#225560,#225561,#225562,#225563),(#225564,#225565,#225566,#225567),
(#225568,#225569,#225570,#225571),(#225572,#225573,#225574,#225575),(#225576,
#225577,#225578,#225579),(#225580,#225581,#225582,#225583),(#225584,#225585,
#225586,#225587),(#225588,#225589,#225590,#225591)),.UNSPECIFIED.,.F.,.F.,
 .F.,(4,3,3,3,3,3,3,3,3,3,3,3,3,3,3,3,3,3,3,3,3,3,3,3,3,3,3,3,3,3,3,3,3,
3,3,3,3,3,3,3,3,3,3,3,3,3,3,3,3,3,4),(4,4),(-0.00109644387045235,0.124177669566463,
0.139836933746078,0.147666565835885,0.151581381880788,0.15353878990324,
0.155496197925692,0.186814726284921,0.249451783003379,0.280770311362608,
0.296429575542222,0.300344391587126,0.302301799609578,0.302791151615191,
0.303280503620803,0.304259207632029,0.312088839721837,0.374725896440295,
0.406044424799524,0.421703688979138,0.42366109700159,0.424639801012816,
0.425618505024042,0.429533321068946,0.437362953158753,0.500000009877211,
0.562637066595668,0.570466698685476,0.574381514730379,0.575360218741605,
0.576338922752831,0.578296330775283,0.593955594954897,0.625274123314126,
0.687911180032584,0.695740812122391,0.696719516133617,0.69720886813923,
0.697698220144843,0.699655628167295,0.703570444212198,0.719229708391813,
0.750548236751042,0.8131852934695,0.844503821828729,0.84646122985118,0.848418637873632,
0.852333453918536,0.860163086008343,0.875822350187958,1.00109646362487),
(0.0477813279241126,1.03891804990681),.UNSPECIFIED.);
#929=B_SPLINE_SURFACE_WITH_KNOTS('',3,3,((#225984,#225985,#225986,#225987,
#225988,#225989,#225990,#225991,#225992,#225993,#225994,#225995,#225996),
(#225997,#225998,#225999,#226000,#226001,#226002,#226003,#226004,#226005,
#226006,#226007,#226008,#226009),(#226010,#226011,#226012,#226013,#226014,
#226015,#226016,#226017,#226018,#226019,#226020,#226021,#226022),(#226023,
#226024,#226025,#226026,#226027,#226028,#226029,#226030,#226031,#226032,
#226033,#226034,#226035),(#226036,#226037,#226038,#226039,#226040,#226041,
#226042,#226043,#226044,#226045,#226046,#226047,#226048),(#226049,#226050,
#226051,#226052,#226053,#226054,#226055,#226056,#226057,#226058,#226059,
#226060,#226061),(#226062,#226063,#226064,#226065,#226066,#226067,#226068,
#226069,#226070,#226071,#226072,#226073,#226074),(#226075,#226076,#226077,
#226078,#226079,#226080,#226081,#226082,#226083,#226084,#226085,#226086,
#226087),(#226088,#226089,#226090,#226091,#226092,#226093,#226094,#226095,
#226096,#226097,#226098,#226099,#226100),(#226101,#226102,#226103,#226104,
#226105,#226106,#226107,#226108,#226109,#226110,#226111,#226112,#226113),
(#226114,#226115,#226116,#226117,#226118,#226119,#226120,#226121,#226122,
#226123,#226124,#226125,#226126),(#226127,#226128,#226129,#226130,#226131,
#226132,#226133,#226134,#226135,#226136,#226137,#226138,#226139),(#226140,
#226141,#226142,#226143,#226144,#226145,#226146,#226147,#226148,#226149,
#226150,#226151,#226152),(#226153,#226154,#226155,#226156,#226157,#226158,
#226159,#226160,#226161,#226162,#226163,#226164,#226165),(#226166,#226167,
#226168,#226169,#226170,#226171,#226172,#226173,#226174,#226175,#226176,
#226177,#226178),(#226179,#226180,#226181,#226182,#226183,#226184,#226185,
#226186,#226187,#226188,#226189,#226190,#226191),(#226192,#226193,#226194,
#226195,#226196,#226197,#226198,#226199,#226200,#226201,#226202,#226203,
#226204),(#226205,#226206,#226207,#226208,#226209,#226210,#226211,#226212,
#226213,#226214,#226215,#226216,#226217),(#226218,#226219,#226220,#226221,
#226222,#226223,#226224,#226225,#226226,#226227,#226228,#226229,#226230),
(#226231,#226232,#226233,#226234,#226235,#226236,#226237,#226238,#226239,
#226240,#226241,#226242,#226243),(#226244,#226245,#226246,#226247,#226248,
#226249,#226250,#226251,#226252,#226253,#226254,#226255,#226256),(#226257,
#226258,#226259,#226260,#226261,#226262,#226263,#226264,#226265,#226266,
#226267,#226268,#226269),(#226270,#226271,#226272,#226273,#226274,#226275,
#226276,#226277,#226278,#226279,#226280,#226281,#226282),(#226283,#226284,
#226285,#226286,#226287,#226288,#226289,#226290,#226291,#226292,#226293,
#226294,#226295),(#226296,#226297,#226298,#226299,#226300,#226301,#226302,
#226303,#226304,#226305,#226306,#226307,#226308),(#226309,#226310,#226311,
#226312,#226313,#226314,#226315,#226316,#226317,#226318,#226319,#226320,
#226321),(#226322,#226323,#226324,#226325,#226326,#226327,#226328,#226329,
#226330,#226331,#226332,#226333,#226334),(#226335,#226336,#226337,#226338,
#226339,#226340,#226341,#226342,#226343,#226344,#226345,#226346,#226347)),
 .UNSPECIFIED.,.F.,.F.,.F.,(4,3,3,3,3,3,3,3,3,4),(4,3,3,3,4),(-2.09329281387815E-12,
0.0624999999980442,0.124999999998182,0.249999999998457,0.374999999998732,
0.499999999999007,0.624999999999282,0.749999999999557,0.874999999999832,
1.00000398343861),(0.0305346534395145,0.148544372614449,0.266554091789383,
0.502573530139252,0.97461240683899),.UNSPECIFIED.);
#930=B_SPLINE_SURFACE_WITH_KNOTS('',3,3,((#226418,#226419,#226420,#226421,
#226422,#226423,#226424,#226425,#226426,#226427,#226428,#226429,#226430),
(#226431,#226432,#226433,#226434,#226435,#226436,#226437,#226438,#226439,
#226440,#226441,#226442,#226443),(#226444,#226445,#226446,#226447,#226448,
#226449,#226450,#226451,#226452,#226453,#226454,#226455,#226456),(#226457,
#226458,#226459,#226460,#226461,#226462,#226463,#226464,#226465,#226466,
#226467,#226468,#226469),(#226470,#226471,#226472,#226473,#226474,#226475,
#226476,#226477,#226478,#226479,#226480,#226481,#226482),(#226483,#226484,
#226485,#226486,#226487,#226488,#226489,#226490,#226491,#226492,#226493,
#226494,#226495),(#226496,#226497,#226498,#226499,#226500,#226501,#226502,
#226503,#226504,#226505,#226506,#226507,#226508),(#226509,#226510,#226511,
#226512,#226513,#226514,#226515,#226516,#226517,#226518,#226519,#226520,
#226521),(#226522,#226523,#226524,#226525,#226526,#226527,#226528,#226529,
#226530,#226531,#226532,#226533,#226534),(#226535,#226536,#226537,#226538,
#226539,#226540,#226541,#226542,#226543,#226544,#226545,#226546,#226547),
(#226548,#226549,#226550,#226551,#226552,#226553,#226554,#226555,#226556,
#226557,#226558,#226559,#226560),(#226561,#226562,#226563,#226564,#226565,
#226566,#226567,#226568,#226569,#226570,#226571,#226572,#226573),(#226574,
#226575,#226576,#226577,#226578,#226579,#226580,#226581,#226582,#226583,
#226584,#226585,#226586),(#226587,#226588,#226589,#226590,#226591,#226592,
#226593,#226594,#226595,#226596,#226597,#226598,#226599),(#226600,#226601,
#226602,#226603,#226604,#226605,#226606,#226607,#226608,#226609,#226610,
#226611,#226612),(#226613,#226614,#226615,#226616,#226617,#226618,#226619,
#226620,#226621,#226622,#226623,#226624,#226625),(#226626,#226627,#226628,
#226629,#226630,#226631,#226632,#226633,#226634,#226635,#226636,#226637,
#226638),(#226639,#226640,#226641,#226642,#226643,#226644,#226645,#226646,
#226647,#226648,#226649,#226650,#226651),(#226652,#226653,#226654,#226655,
#226656,#226657,#226658,#226659,#226660,#226661,#226662,#226663,#226664),
(#226665,#226666,#226667,#226668,#226669,#226670,#226671,#226672,#226673,
#226674,#226675,#226676,#226677),(#226678,#226679,#226680,#226681,#226682,
#226683,#226684,#226685,#226686,#226687,#226688,#226689,#226690),(#226691,
#226692,#226693,#226694,#226695,#226696,#226697,#226698,#226699,#226700,
#226701,#226702,#226703),(#226704,#226705,#226706,#226707,#226708,#226709,
#226710,#226711,#226712,#226713,#226714,#226715,#226716),(#226717,#226718,
#226719,#226720,#226721,#226722,#226723,#226724,#226725,#226726,#226727,
#226728,#226729),(#226730,#226731,#226732,#226733,#226734,#226735,#226736,
#226737,#226738,#226739,#226740,#226741,#226742),(#226743,#226744,#226745,
#226746,#226747,#226748,#226749,#226750,#226751,#226752,#226753,#226754,
#226755),(#226756,#226757,#226758,#226759,#226760,#226761,#226762,#226763,
#226764,#226765,#226766,#226767,#226768),(#226769,#226770,#226771,#226772,
#226773,#226774,#226775,#226776,#226777,#226778,#226779,#226780,#226781),
(#226782,#226783,#226784,#226785,#226786,#226787,#226788,#226789,#226790,
#226791,#226792,#226793,#226794),(#226795,#226796,#226797,#226798,#226799,
#226800,#226801,#226802,#226803,#226804,#226805,#226806,#226807),(#226808,
#226809,#226810,#226811,#226812,#226813,#226814,#226815,#226816,#226817,
#226818,#226819,#226820),(#226821,#226822,#226823,#226824,#226825,#226826,
#226827,#226828,#226829,#226830,#226831,#226832,#226833),(#226834,#226835,
#226836,#226837,#226838,#226839,#226840,#226841,#226842,#226843,#226844,
#226845,#226846),(#226847,#226848,#226849,#226850,#226851,#226852,#226853,
#226854,#226855,#226856,#226857,#226858,#226859),(#226860,#226861,#226862,
#226863,#226864,#226865,#226866,#226867,#226868,#226869,#226870,#226871,
#226872),(#226873,#226874,#226875,#226876,#226877,#226878,#226879,#226880,
#226881,#226882,#226883,#226884,#226885),(#226886,#226887,#226888,#226889,
#226890,#226891,#226892,#226893,#226894,#226895,#226896,#226897,#226898),
(#226899,#226900,#226901,#226902,#226903,#226904,#226905,#226906,#226907,
#226908,#226909,#226910,#226911),(#226912,#226913,#226914,#226915,#226916,
#226917,#226918,#226919,#226920,#226921,#226922,#226923,#226924),(#226925,
#226926,#226927,#226928,#226929,#226930,#226931,#226932,#226933,#226934,
#226935,#226936,#226937),(#226938,#226939,#226940,#226941,#226942,#226943,
#226944,#226945,#226946,#226947,#226948,#226949,#226950),(#226951,#226952,
#226953,#226954,#226955,#226956,#226957,#226958,#226959,#226960,#226961,
#226962,#226963),(#226964,#226965,#226966,#226967,#226968,#226969,#226970,
#226971,#226972,#226973,#226974,#226975,#226976)),.UNSPECIFIED.,.F.,.F.,
 .F.,(4,3,3,3,3,3,3,3,3,3,3,3,3,3,4),(4,3,3,3,4),(-0.00600089904390221,
0.00185848297987854,0.00971786500365927,0.0254366290512207,0.0568741571463437,
0.11974921333659,0.182624269526835,0.245499325717081,0.371249438097573,
0.496999550478065,0.622749662858557,0.748499775239049,0.874249887619541,
0.937124943809787,1.00000000000003),(0.0313847250337115,0.149350226349808,
0.267315727665905,0.503246730298099,0.975108735562486),.UNSPECIFIED.);
#931=B_SPLINE_SURFACE_WITH_KNOTS('',3,3,((#227055,#227056,#227057,#227058,
#227059,#227060,#227061,#227062,#227063,#227064,#227065,#227066,#227067),
(#227068,#227069,#227070,#227071,#227072,#227073,#227074,#227075,#227076,
#227077,#227078,#227079,#227080),(#227081,#227082,#227083,#227084,#227085,
#227086,#227087,#227088,#227089,#227090,#227091,#227092,#227093),(#227094,
#227095,#227096,#227097,#227098,#227099,#227100,#227101,#227102,#227103,
#227104,#227105,#227106),(#227107,#227108,#227109,#227110,#227111,#227112,
#227113,#227114,#227115,#227116,#227117,#227118,#227119),(#227120,#227121,
#227122,#227123,#227124,#227125,#227126,#227127,#227128,#227129,#227130,
#227131,#227132),(#227133,#227134,#227135,#227136,#227137,#227138,#227139,
#227140,#227141,#227142,#227143,#227144,#227145),(#227146,#227147,#227148,
#227149,#227150,#227151,#227152,#227153,#227154,#227155,#227156,#227157,
#227158),(#227159,#227160,#227161,#227162,#227163,#227164,#227165,#227166,
#227167,#227168,#227169,#227170,#227171),(#227172,#227173,#227174,#227175,
#227176,#227177,#227178,#227179,#227180,#227181,#227182,#227183,#227184),
(#227185,#227186,#227187,#227188,#227189,#227190,#227191,#227192,#227193,
#227194,#227195,#227196,#227197),(#227198,#227199,#227200,#227201,#227202,
#227203,#227204,#227205,#227206,#227207,#227208,#227209,#227210),(#227211,
#227212,#227213,#227214,#227215,#227216,#227217,#227218,#227219,#227220,
#227221,#227222,#227223),(#227224,#227225,#227226,#227227,#227228,#227229,
#227230,#227231,#227232,#227233,#227234,#227235,#227236),(#227237,#227238,
#227239,#227240,#227241,#227242,#227243,#227244,#227245,#227246,#227247,
#227248,#227249),(#227250,#227251,#227252,#227253,#227254,#227255,#227256,
#227257,#227258,#227259,#227260,#227261,#227262),(#227263,#227264,#227265,
#227266,#227267,#227268,#227269,#227270,#227271,#227272,#227273,#227274,
#227275),(#227276,#227277,#227278,#227279,#227280,#227281,#227282,#227283,
#227284,#227285,#227286,#227287,#227288),(#227289,#227290,#227291,#227292,
#227293,#227294,#227295,#227296,#227297,#227298,#227299,#227300,#227301),
(#227302,#227303,#227304,#227305,#227306,#227307,#227308,#227309,#227310,
#227311,#227312,#227313,#227314),(#227315,#227316,#227317,#227318,#227319,
#227320,#227321,#227322,#227323,#227324,#227325,#227326,#227327),(#227328,
#227329,#227330,#227331,#227332,#227333,#227334,#227335,#227336,#227337,
#227338,#227339,#227340),(#227341,#227342,#227343,#227344,#227345,#227346,
#227347,#227348,#227349,#227350,#227351,#227352,#227353),(#227354,#227355,
#227356,#227357,#227358,#227359,#227360,#227361,#227362,#227363,#227364,
#227365,#227366),(#227367,#227368,#227369,#227370,#227371,#227372,#227373,
#227374,#227375,#227376,#227377,#227378,#227379),(#227380,#227381,#227382,
#227383,#227384,#227385,#227386,#227387,#227388,#227389,#227390,#227391,
#227392),(#227393,#227394,#227395,#227396,#227397,#227398,#227399,#227400,
#227401,#227402,#227403,#227404,#227405),(#227406,#227407,#227408,#227409,
#227410,#227411,#227412,#227413,#227414,#227415,#227416,#227417,#227418)),
 .UNSPECIFIED.,.F.,.F.,.F.,(4,3,3,3,3,3,3,3,3,4),(4,3,3,3,4),(7.97241441451061E-14,
0.0625000000003403,0.125000000000601,0.250000000001122,0.375000000001643,
0.500000000002164,0.625000000002685,0.750000000003206,0.875000000003727,
1.00000000000425),(0.035779394199433,0.153116210014097,0.27045302582876,
0.505126657458087,0.97447392071674),.UNSPECIFIED.);
#932=B_SPLINE_SURFACE_WITH_KNOTS('',3,3,((#227491,#227492,#227493,#227494,
#227495,#227496,#227497,#227498,#227499,#227500),(#227501,#227502,#227503,
#227504,#227505,#227506,#227507,#227508,#227509,#227510),(#227511,#227512,
#227513,#227514,#227515,#227516,#227517,#227518,#227519,#227520),(#227521,
#227522,#227523,#227524,#227525,#227526,#227527,#227528,#227529,#227530),
(#227531,#227532,#227533,#227534,#227535,#227536,#227537,#227538,#227539,
#227540),(#227541,#227542,#227543,#227544,#227545,#227546,#227547,#227548,
#227549,#227550),(#227551,#227552,#227553,#227554,#227555,#227556,#227557,
#227558,#227559,#227560),(#227561,#227562,#227563,#227564,#227565,#227566,
#227567,#227568,#227569,#227570),(#227571,#227572,#227573,#227574,#227575,
#227576,#227577,#227578,#227579,#227580),(#227581,#227582,#227583,#227584,
#227585,#227586,#227587,#227588,#227589,#227590),(#227591,#227592,#227593,
#227594,#227595,#227596,#227597,#227598,#227599,#227600),(#227601,#227602,
#227603,#227604,#227605,#227606,#227607,#227608,#227609,#227610),(#227611,
#227612,#227613,#227614,#227615,#227616,#227617,#227618,#227619,#227620),
(#227621,#227622,#227623,#227624,#227625,#227626,#227627,#227628,#227629,
#227630),(#227631,#227632,#227633,#227634,#227635,#227636,#227637,#227638,
#227639,#227640),(#227641,#227642,#227643,#227644,#227645,#227646,#227647,
#227648,#227649,#227650),(#227651,#227652,#227653,#227654,#227655,#227656,
#227657,#227658,#227659,#227660),(#227661,#227662,#227663,#227664,#227665,
#227666,#227667,#227668,#227669,#227670),(#227671,#227672,#227673,#227674,
#227675,#227676,#227677,#227678,#227679,#227680),(#227681,#227682,#227683,
#227684,#227685,#227686,#227687,#227688,#227689,#227690),(#227691,#227692,
#227693,#227694,#227695,#227696,#227697,#227698,#227699,#227700),(#227701,
#227702,#227703,#227704,#227705,#227706,#227707,#227708,#227709,#227710),
(#227711,#227712,#227713,#227714,#227715,#227716,#227717,#227718,#227719,
#227720),(#227721,#227722,#227723,#227724,#227725,#227726,#227727,#227728,
#227729,#227730),(#227731,#227732,#227733,#227734,#227735,#227736,#227737,
#227738,#227739,#227740),(#227741,#227742,#227743,#227744,#227745,#227746,
#227747,#227748,#227749,#227750),(#227751,#227752,#227753,#227754,#227755,
#227756,#227757,#227758,#227759,#227760),(#227761,#227762,#227763,#227764,
#227765,#227766,#227767,#227768,#227769,#227770),(#227771,#227772,#227773,
#227774,#227775,#227776,#227777,#227778,#227779,#227780),(#227781,#227782,
#227783,#227784,#227785,#227786,#227787,#227788,#227789,#227790),(#227791,
#227792,#227793,#227794,#227795,#227796,#227797,#227798,#227799,#227800),
(#227801,#227802,#227803,#227804,#227805,#227806,#227807,#227808,#227809,
#227810),(#227811,#227812,#227813,#227814,#227815,#227816,#227817,#227818,
#227819,#227820),(#227821,#227822,#227823,#227824,#227825,#227826,#227827,
#227828,#227829,#227830),(#227831,#227832,#227833,#227834,#227835,#227836,
#227837,#227838,#227839,#227840),(#227841,#227842,#227843,#227844,#227845,
#227846,#227847,#227848,#227849,#227850),(#227851,#227852,#227853,#227854,
#227855,#227856,#227857,#227858,#227859,#227860),(#227861,#227862,#227863,
#227864,#227865,#227866,#227867,#227868,#227869,#227870),(#227871,#227872,
#227873,#227874,#227875,#227876,#227877,#227878,#227879,#227880),(#227881,
#227882,#227883,#227884,#227885,#227886,#227887,#227888,#227889,#227890),
(#227891,#227892,#227893,#227894,#227895,#227896,#227897,#227898,#227899,
#227900),(#227901,#227902,#227903,#227904,#227905,#227906,#227907,#227908,
#227909,#227910),(#227911,#227912,#227913,#227914,#227915,#227916,#227917,
#227918,#227919,#227920),(#227921,#227922,#227923,#227924,#227925,#227926,
#227927,#227928,#227929,#227930),(#227931,#227932,#227933,#227934,#227935,
#227936,#227937,#227938,#227939,#227940),(#227941,#227942,#227943,#227944,
#227945,#227946,#227947,#227948,#227949,#227950),(#227951,#227952,#227953,
#227954,#227955,#227956,#227957,#227958,#227959,#227960),(#227961,#227962,
#227963,#227964,#227965,#227966,#227967,#227968,#227969,#227970),(#227971,
#227972,#227973,#227974,#227975,#227976,#227977,#227978,#227979,#227980),
(#227981,#227982,#227983,#227984,#227985,#227986,#227987,#227988,#227989,
#227990),(#227991,#227992,#227993,#227994,#227995,#227996,#227997,#227998,
#227999,#228000),(#228001,#228002,#228003,#228004,#228005,#228006,#228007,
#228008,#228009,#228010)),.UNSPECIFIED.,.F.,.F.,.F.,(4,3,3,3,3,3,3,3,3,
3,3,3,3,3,3,3,3,4),(4,3,3,4),(-0.00600093757051703,0.00190532409776943,
0.00981158576605589,0.0256241091026288,0.0572491557757747,0.120499249122066,
0.24699943581465,0.373499622507233,0.499999809199817,0.6264999958924,0.753000182584983,
0.816250275931275,0.879500369277567,0.942750462623858,0.974375509297004,
0.990188032633577,0.998094294301864,1.00600055597015),(0.0341113530318832,
0.269267250872974,0.504423148714065,0.974734944396246),.UNSPECIFIED.);
#933=B_SPLINE_SURFACE_WITH_KNOTS('',3,3,((#228207,#228208,#228209,#228210),
(#228211,#228212,#228213,#228214),(#228215,#228216,#228217,#228218),(#228219,
#228220,#228221,#228222)),.UNSPECIFIED.,.F.,.F.,.F.,(4,4),(4,4),(-2.26710392139532E-13,
0.274586007458263),(0.048728470569204,0.974637180848091),.UNSPECIFIED.);
#934=B_SPLINE_SURFACE_WITH_KNOTS('',3,3,((#228243,#228244,#228245,#228246),
(#228247,#228248,#228249,#228250),(#228251,#228252,#228253,#228254),(#228255,
#228256,#228257,#228258)),.UNSPECIFIED.,.F.,.F.,.F.,(4,4),(4,4),(0.723791628179461,
1.),(0.0491493978854403,0.974752225001403),.UNSPECIFIED.);
#935=B_SPLINE_SURFACE_WITH_KNOTS('',3,3,((#228461,#228462,#228463,#228464),
(#228465,#228466,#228467,#228468),(#228469,#228470,#228471,#228472),(#228473,
#228474,#228475,#228476)),.UNSPECIFIED.,.F.,.F.,.F.,(4,4),(4,4),(7.07266882820453E-16,
0.107439860233906),(0.0511874640850671,0.974440796609261),.UNSPECIFIED.);
#936=B_SPLINE_SURFACE_WITH_KNOTS('',3,3,((#228512,#228513,#228514,#228515),
(#228516,#228517,#228518,#228519),(#228520,#228521,#228522,#228523),(#228524,
#228525,#228526,#228527)),.UNSPECIFIED.,.F.,.F.,.F.,(4,4),(4,4),(0.905181055822597,
1.00000000000972),(0.0504405324641688,0.975107277906268),.UNSPECIFIED.);
#937=B_SPLINE_SURFACE_WITH_KNOTS('',3,3,((#228544,#228545,#228546,#228547,
#228548,#228549,#228550),(#228551,#228552,#228553,#228554,#228555,#228556,
#228557),(#228558,#228559,#228560,#228561,#228562,#228563,#228564),(#228565,
#228566,#228567,#228568,#228569,#228570,#228571),(#228572,#228573,#228574,
#228575,#228576,#228577,#228578),(#228579,#228580,#228581,#228582,#228583,
#228584,#228585),(#228586,#228587,#228588,#228589,#228590,#228591,#228592),
(#228593,#228594,#228595,#228596,#228597,#228598,#228599),(#228600,#228601,
#228602,#228603,#228604,#228605,#228606),(#228607,#228608,#228609,#228610,
#228611,#228612,#228613),(#228614,#228615,#228616,#228617,#228618,#228619,
#228620),(#228621,#228622,#228623,#228624,#228625,#228626,#228627),(#228628,
#228629,#228630,#228631,#228632,#228633,#228634),(#228635,#228636,#228637,
#228638,#228639,#228640,#228641),(#228642,#228643,#228644,#228645,#228646,
#228647,#228648),(#228649,#228650,#228651,#228652,#228653,#228654,#228655),
(#228656,#228657,#228658,#228659,#228660,#228661,#228662),(#228663,#228664,
#228665,#228666,#228667,#228668,#228669),(#228670,#228671,#228672,#228673,
#228674,#228675,#228676),(#228677,#228678,#228679,#228680,#228681,#228682,
#228683),(#228684,#228685,#228686,#228687,#228688,#228689,#228690),(#228691,
#228692,#228693,#228694,#228695,#228696,#228697),(#228698,#228699,#228700,
#228701,#228702,#228703,#228704),(#228705,#228706,#228707,#228708,#228709,
#228710,#228711),(#228712,#228713,#228714,#228715,#228716,#228717,#228718),
(#228719,#228720,#228721,#228722,#228723,#228724,#228725),(#228726,#228727,
#228728,#228729,#228730,#228731,#228732),(#228733,#228734,#228735,#228736,
#228737,#228738,#228739)),.UNSPECIFIED.,.F.,.F.,.F.,(4,3,3,3,3,3,3,3,3,
4),(4,3,4),(6.8818812944557E-15,0.250000000000005,0.5,0.75,0.875,0.9375,
0.96875,0.984375,0.9921875,1.),(0.0332750425089971,0.501824549528,0.970374056547004),
 .UNSPECIFIED.);
#938=B_SPLINE_SURFACE_WITH_KNOTS('',3,3,((#228821,#228822,#228823,#228824,
#228825,#228826,#228827),(#228828,#228829,#228830,#228831,#228832,#228833,
#228834),(#228835,#228836,#228837,#228838,#228839,#228840,#228841),(#228842,
#228843,#228844,#228845,#228846,#228847,#228848),(#228849,#228850,#228851,
#228852,#228853,#228854,#228855),(#228856,#228857,#228858,#228859,#228860,
#228861,#228862),(#228863,#228864,#228865,#228866,#228867,#228868,#228869),
(#228870,#228871,#228872,#228873,#228874,#228875,#228876),(#228877,#228878,
#228879,#228880,#228881,#228882,#228883),(#228884,#228885,#228886,#228887,
#228888,#228889,#228890),(#228891,#228892,#228893,#228894,#228895,#228896,
#228897),(#228898,#228899,#228900,#228901,#228902,#228903,#228904),(#228905,
#228906,#228907,#228908,#228909,#228910,#228911),(#228912,#228913,#228914,
#228915,#228916,#228917,#228918),(#228919,#228920,#228921,#228922,#228923,
#228924,#228925),(#228926,#228927,#228928,#228929,#228930,#228931,#228932),
(#228933,#228934,#228935,#228936,#228937,#228938,#228939),(#228940,#228941,
#228942,#228943,#228944,#228945,#228946),(#228947,#228948,#228949,#228950,
#228951,#228952,#228953),(#228954,#228955,#228956,#228957,#228958,#228959,
#228960),(#228961,#228962,#228963,#228964,#228965,#228966,#228967),(#228968,
#228969,#228970,#228971,#228972,#228973,#228974),(#228975,#228976,#228977,
#228978,#228979,#228980,#228981),(#228982,#228983,#228984,#228985,#228986,
#228987,#228988),(#228989,#228990,#228991,#228992,#228993,#228994,#228995),
(#228996,#228997,#228998,#228999,#229000,#229001,#229002),(#229003,#229004,
#229005,#229006,#229007,#229008,#229009),(#229010,#229011,#229012,#229013,
#229014,#229015,#229016),(#229017,#229018,#229019,#229020,#229021,#229022,
#229023),(#229024,#229025,#229026,#229027,#229028,#229029,#229030),(#229031,
#229032,#229033,#229034,#229035,#229036,#229037),(#229038,#229039,#229040,
#229041,#229042,#229043,#229044),(#229045,#229046,#229047,#229048,#229049,
#229050,#229051),(#229052,#229053,#229054,#229055,#229056,#229057,#229058),
(#229059,#229060,#229061,#229062,#229063,#229064,#229065),(#229066,#229067,
#229068,#229069,#229070,#229071,#229072),(#229073,#229074,#229075,#229076,
#229077,#229078,#229079),(#229080,#229081,#229082,#229083,#229084,#229085,
#229086),(#229087,#229088,#229089,#229090,#229091,#229092,#229093),(#229094,
#229095,#229096,#229097,#229098,#229099,#229100)),.UNSPECIFIED.,.F.,.F.,
 .F.,(4,3,3,3,3,3,3,3,3,3,3,3,3,4),(4,3,4),(-0.00600002990670325,0.009718720560589,
0.0254374710278812,0.0568749719624657,0.119749973831635,0.245499977569973,
0.496999985046649,0.748499992523325,0.874249996261663,0.937124998130832,
0.968562499065416,0.984281249532708,0.992140624766354,1.),(0.0284242133522742,
0.499005960311874,0.969587707271474),.UNSPECIFIED.);
#939=B_SPLINE_SURFACE_WITH_KNOTS('',3,3,((#229258,#229259,#229260,#229261,
#229262,#229263,#229264),(#229265,#229266,#229267,#229268,#229269,#229270,
#229271),(#229272,#229273,#229274,#229275,#229276,#229277,#229278),(#229279,
#229280,#229281,#229282,#229283,#229284,#229285),(#229286,#229287,#229288,
#229289,#229290,#229291,#229292),(#229293,#229294,#229295,#229296,#229297,
#229298,#229299),(#229300,#229301,#229302,#229303,#229304,#229305,#229306),
(#229307,#229308,#229309,#229310,#229311,#229312,#229313),(#229314,#229315,
#229316,#229317,#229318,#229319,#229320),(#229321,#229322,#229323,#229324,
#229325,#229326,#229327),(#229328,#229329,#229330,#229331,#229332,#229333,
#229334),(#229335,#229336,#229337,#229338,#229339,#229340,#229341),(#229342,
#229343,#229344,#229345,#229346,#229347,#229348),(#229349,#229350,#229351,
#229352,#229353,#229354,#229355),(#229356,#229357,#229358,#229359,#229360,
#229361,#229362),(#229363,#229364,#229365,#229366,#229367,#229368,#229369),
(#229370,#229371,#229372,#229373,#229374,#229375,#229376),(#229377,#229378,
#229379,#229380,#229381,#229382,#229383),(#229384,#229385,#229386,#229387,
#229388,#229389,#229390),(#229391,#229392,#229393,#229394,#229395,#229396,
#229397),(#229398,#229399,#229400,#229401,#229402,#229403,#229404),(#229405,
#229406,#229407,#229408,#229409,#229410,#229411),(#229412,#229413,#229414,
#229415,#229416,#229417,#229418),(#229419,#229420,#229421,#229422,#229423,
#229424,#229425),(#229426,#229427,#229428,#229429,#229430,#229431,#229432),
(#229433,#229434,#229435,#229436,#229437,#229438,#229439),(#229440,#229441,
#229442,#229443,#229444,#229445,#229446),(#229447,#229448,#229449,#229450,
#229451,#229452,#229453),(#229454,#229455,#229456,#229457,#229458,#229459,
#229460),(#229461,#229462,#229463,#229464,#229465,#229466,#229467),(#229468,
#229469,#229470,#229471,#229472,#229473,#229474),(#229475,#229476,#229477,
#229478,#229479,#229480,#229481),(#229482,#229483,#229484,#229485,#229486,
#229487,#229488),(#229489,#229490,#229491,#229492,#229493,#229494,#229495),
(#229496,#229497,#229498,#229499,#229500,#229501,#229502),(#229503,#229504,
#229505,#229506,#229507,#229508,#229509),(#229510,#229511,#229512,#229513,
#229514,#229515,#229516),(#229517,#229518,#229519,#229520,#229521,#229522,
#229523),(#229524,#229525,#229526,#229527,#229528,#229529,#229530),(#229531,
#229532,#229533,#229534,#229535,#229536,#229537),(#229538,#229539,#229540,
#229541,#229542,#229543,#229544),(#229545,#229546,#229547,#229548,#229549,
#229550,#229551),(#229552,#229553,#229554,#229555,#229556,#229557,#229558),
(#229559,#229560,#229561,#229562,#229563,#229564,#229565),(#229566,#229567,
#229568,#229569,#229570,#229571,#229572),(#229573,#229574,#229575,#229576,
#229577,#229578,#229579),(#229580,#229581,#229582,#229583,#229584,#229585,
#229586),(#229587,#229588,#229589,#229590,#229591,#229592,#229593),(#229594,
#229595,#229596,#229597,#229598,#229599,#229600),(#229601,#229602,#229603,
#229604,#229605,#229606,#229607),(#229608,#229609,#229610,#229611,#229612,
#229613,#229614),(#229615,#229616,#229617,#229618,#229619,#229620,#229621),
(#229622,#229623,#229624,#229625,#229626,#229627,#229628),(#229629,#229630,
#229631,#229632,#229633,#229634,#229635),(#229636,#229637,#229638,#229639,
#229640,#229641,#229642),(#229643,#229644,#229645,#229646,#229647,#229648,
#229649),(#229650,#229651,#229652,#229653,#229654,#229655,#229656),(#229657,
#229658,#229659,#229660,#229661,#229662,#229663),(#229664,#229665,#229666,
#229667,#229668,#229669,#229670),(#229671,#229672,#229673,#229674,#229675,
#229676,#229677),(#229678,#229679,#229680,#229681,#229682,#229683,#229684),
(#229685,#229686,#229687,#229688,#229689,#229690,#229691),(#229692,#229693,
#229694,#229695,#229696,#229697,#229698),(#229699,#229700,#229701,#229702,
#229703,#229704,#229705),(#229706,#229707,#229708,#229709,#229710,#229711,
#229712),(#229713,#229714,#229715,#229716,#229717,#229718,#229719),(#229720,
#229721,#229722,#229723,#229724,#229725,#229726),(#229727,#229728,#229729,
#229730,#229731,#229732,#229733),(#229734,#229735,#229736,#229737,#229738,
#229739,#229740),(#229741,#229742,#229743,#229744,#229745,#229746,#229747),
(#229748,#229749,#229750,#229751,#229752,#229753,#229754),(#229755,#229756,
#229757,#229758,#229759,#229760,#229761),(#229762,#229763,#229764,#229765,
#229766,#229767,#229768),(#229769,#229770,#229771,#229772,#229773,#229774,
#229775),(#229776,#229777,#229778,#229779,#229780,#229781,#229782),(#229783,
#229784,#229785,#229786,#229787,#229788,#229789),(#229790,#229791,#229792,
#229793,#229794,#229795,#229796),(#229797,#229798,#229799,#229800,#229801,
#229802,#229803),(#229804,#229805,#229806,#229807,#229808,#229809,#229810),
(#229811,#229812,#229813,#229814,#229815,#229816,#229817),(#229818,#229819,
#229820,#229821,#229822,#229823,#229824),(#229825,#229826,#229827,#229828,
#229829,#229830,#229831),(#229832,#229833,#229834,#229835,#229836,#229837,
#229838),(#229839,#229840,#229841,#229842,#229843,#229844,#229845),(#229846,
#229847,#229848,#229849,#229850,#229851,#229852),(#229853,#229854,#229855,
#229856,#229857,#229858,#229859),(#229860,#229861,#229862,#229863,#229864,
#229865,#229866),(#229867,#229868,#229869,#229870,#229871,#229872,#229873),
(#229874,#229875,#229876,#229877,#229878,#229879,#229880),(#229881,#229882,
#229883,#229884,#229885,#229886,#229887),(#229888,#229889,#229890,#229891,
#229892,#229893,#229894),(#229895,#229896,#229897,#229898,#229899,#229900,
#229901),(#229902,#229903,#229904,#229905,#229906,#229907,#229908),(#229909,
#229910,#229911,#229912,#229913,#229914,#229915),(#229916,#229917,#229918,
#229919,#229920,#229921,#229922),(#229923,#229924,#229925,#229926,#229927,
#229928,#229929),(#229930,#229931,#229932,#229933,#229934,#229935,#229936),
(#229937,#229938,#229939,#229940,#229941,#229942,#229943),(#229944,#229945,
#229946,#229947,#229948,#229949,#229950),(#229951,#229952,#229953,#229954,
#229955,#229956,#229957),(#229958,#229959,#229960,#229961,#229962,#229963,
#229964),(#229965,#229966,#229967,#229968,#229969,#229970,#229971),(#229972,
#229973,#229974,#229975,#229976,#229977,#229978),(#229979,#229980,#229981,
#229982,#229983,#229984,#229985),(#229986,#229987,#229988,#229989,#229990,
#229991,#229992),(#229993,#229994,#229995,#229996,#229997,#229998,#229999),
(#230000,#230001,#230002,#230003,#230004,#230005,#230006),(#230007,#230008,
#230009,#230010,#230011,#230012,#230013),(#230014,#230015,#230016,#230017,
#230018,#230019,#230020),(#230021,#230022,#230023,#230024,#230025,#230026,
#230027),(#230028,#230029,#230030,#230031,#230032,#230033,#230034),(#230035,
#230036,#230037,#230038,#230039,#230040,#230041),(#230042,#230043,#230044,
#230045,#230046,#230047,#230048),(#230049,#230050,#230051,#230052,#230053,
#230054,#230055),(#230056,#230057,#230058,#230059,#230060,#230061,#230062),
(#230063,#230064,#230065,#230066,#230067,#230068,#230069),(#230070,#230071,
#230072,#230073,#230074,#230075,#230076),(#230077,#230078,#230079,#230080,
#230081,#230082,#230083),(#230084,#230085,#230086,#230087,#230088,#230089,
#230090),(#230091,#230092,#230093,#230094,#230095,#230096,#230097),(#230098,
#230099,#230100,#230101,#230102,#230103,#230104),(#230105,#230106,#230107,
#230108,#230109,#230110,#230111),(#230112,#230113,#230114,#230115,#230116,
#230117,#230118),(#230119,#230120,#230121,#230122,#230123,#230124,#230125),
(#230126,#230127,#230128,#230129,#230130,#230131,#230132),(#230133,#230134,
#230135,#230136,#230137,#230138,#230139),(#230140,#230141,#230142,#230143,
#230144,#230145,#230146),(#230147,#230148,#230149,#230150,#230151,#230152,
#230153),(#230154,#230155,#230156,#230157,#230158,#230159,#230160),(#230161,
#230162,#230163,#230164,#230165,#230166,#230167),(#230168,#230169,#230170,
#230171,#230172,#230173,#230174),(#230175,#230176,#230177,#230178,#230179,
#230180,#230181),(#230182,#230183,#230184,#230185,#230186,#230187,#230188),
(#230189,#230190,#230191,#230192,#230193,#230194,#230195),(#230196,#230197,
#230198,#230199,#230200,#230201,#230202),(#230203,#230204,#230205,#230206,
#230207,#230208,#230209),(#230210,#230211,#230212,#230213,#230214,#230215,
#230216),(#230217,#230218,#230219,#230220,#230221,#230222,#230223),(#230224,
#230225,#230226,#230227,#230228,#230229,#230230),(#230231,#230232,#230233,
#230234,#230235,#230236,#230237),(#230238,#230239,#230240,#230241,#230242,
#230243,#230244),(#230245,#230246,#230247,#230248,#230249,#230250,#230251),
(#230252,#230253,#230254,#230255,#230256,#230257,#230258),(#230259,#230260,
#230261,#230262,#230263,#230264,#230265),(#230266,#230267,#230268,#230269,
#230270,#230271,#230272),(#230273,#230274,#230275,#230276,#230277,#230278,
#230279),(#230280,#230281,#230282,#230283,#230284,#230285,#230286),(#230287,
#230288,#230289,#230290,#230291,#230292,#230293),(#230294,#230295,#230296,
#230297,#230298,#230299,#230300),(#230301,#230302,#230303,#230304,#230305,
#230306,#230307),(#230308,#230309,#230310,#230311,#230312,#230313,#230314),
(#230315,#230316,#230317,#230318,#230319,#230320,#230321),(#230322,#230323,
#230324,#230325,#230326,#230327,#230328),(#230329,#230330,#230331,#230332,
#230333,#230334,#230335),(#230336,#230337,#230338,#230339,#230340,#230341,
#230342),(#230343,#230344,#230345,#230346,#230347,#230348,#230349),(#230350,
#230351,#230352,#230353,#230354,#230355,#230356)),.UNSPECIFIED.,.F.,.F.,
 .F.,(4,3,3,3,3,3,3,3,3,3,3,3,3,3,3,3,3,3,3,3,3,3,3,3,3,3,3,3,3,3,3,3,3,
3,3,3,3,3,3,3,3,3,3,3,3,3,3,3,3,3,3,3,4),(4,3,4),(-7.69660169486442E-5,
0.125023528667579,0.156298652338711,0.164117433256494,0.164606107063856,
0.165094780871217,0.16607212848594,0.168026823715385,0.171936214174277,
0.187573776009843,0.250124023352107,0.281399147023239,0.297036708858805,
0.298991404088251,0.299480077895612,0.299968751702973,0.300946099317697,
0.304855489776588,0.312674270694371,0.375224518036634,0.406499641707767,
0.422137203543333,0.429955984461115,0.430933332075839,0.431910679690562,
0.433865374920007,0.437774765378899,0.500325012721163,0.562875260063426,
0.566784650522318,0.568739345751764,0.569228019559125,0.569716693366486,
0.570694040981209,0.578512821898992,0.594150383734558,0.62542550740569,
0.687975754747954,0.695794535665737,0.699703926124629,0.701658621354074,
0.70361331658352,0.719250878419086,0.750526002090218,0.813076249432482,
0.828713811268048,0.832623201726939,0.834577896956385,0.835555244571108,
0.836532592185831,0.844351373103614,0.875626496774746,1.00072699145927),
(0.0460660594806178,0.548882757239649,1.05169945499868),.UNSPECIFIED.);
#940=B_SPLINE_SURFACE_WITH_KNOTS('',3,1,((#230431,#230432),(#230433,#230434),
(#230435,#230436),(#230437,#230438),(#230439,#230440),(#230441,#230442),
(#230443,#230444),(#230445,#230446),(#230447,#230448),(#230449,#230450),
(#230451,#230452),(#230453,#230454),(#230455,#230456),(#230457,#230458),
(#230459,#230460),(#230461,#230462),(#230463,#230464),(#230465,#230466),
(#230467,#230468),(#230469,#230470),(#230471,#230472),(#230473,#230474),
(#230475,#230476),(#230477,#230478),(#230479,#230480),(#230481,#230482),
(#230483,#230484),(#230485,#230486),(#230487,#230488),(#230489,#230490),
(#230491,#230492),(#230493,#230494),(#230495,#230496),(#230497,#230498),
(#230499,#230500),(#230501,#230502),(#230503,#230504),(#230505,#230506),
(#230507,#230508),(#230509,#230510),(#230511,#230512),(#230513,#230514)),
 .UNSPECIFIED.,.F.,.F.,.F.,(4,1,1,1,2,1,1,1,2,1,1,1,2,1,1,1,2,1,1,1,2,1,
1,1,2,1,1,1,2,1,1,1,4),(2,2),(-0.116364947985043,0.0349237439162043,0.0698474878324086,
0.104771231748613,0.139694975664817,0.174004779710855,0.208314583756892,
0.24262438780293,0.276934191848968,0.313293030205055,0.349651868561143,
0.38601070691723,0.422369545273318,0.441777158954989,0.46118477263666,0.480592386318331,
0.5,0.519407613681673,0.538815227363344,0.558222841045015,0.577630454726686,
0.613989293082773,0.65034813143886,0.686706969794946,0.723065808151033,
0.757375612197071,0.791685416243108,0.825995220289146,0.860305024335184,
0.895228768251388,0.930152512167592,0.965076256083796,1.11636494798509),
(-0.174247524918837,1.18461554289192),.UNSPECIFIED.);
#941=B_SPLINE_SURFACE_WITH_KNOTS('',3,3,((#230515,#230516,#230517,#230518),
(#230519,#230520,#230521,#230522),(#230523,#230524,#230525,#230526),(#230527,
#230528,#230529,#230530),(#230531,#230532,#230533,#230534),(#230535,#230536,
#230537,#230538),(#230539,#230540,#230541,#230542),(#230543,#230544,#230545,
#230546),(#230547,#230548,#230549,#230550),(#230551,#230552,#230553,#230554),
(#230555,#230556,#230557,#230558),(#230559,#230560,#230561,#230562),(#230563,
#230564,#230565,#230566),(#230567,#230568,#230569,#230570),(#230571,#230572,
#230573,#230574),(#230575,#230576,#230577,#230578),(#230579,#230580,#230581,
#230582),(#230583,#230584,#230585,#230586),(#230587,#230588,#230589,#230590),
(#230591,#230592,#230593,#230594),(#230595,#230596,#230597,#230598),(#230599,
#230600,#230601,#230602),(#230603,#230604,#230605,#230606),(#230607,#230608,
#230609,#230610),(#230611,#230612,#230613,#230614),(#230615,#230616,#230617,
#230618),(#230619,#230620,#230621,#230622),(#230623,#230624,#230625,#230626),
(#230627,#230628,#230629,#230630),(#230631,#230632,#230633,#230634),(#230635,
#230636,#230637,#230638),(#230639,#230640,#230641,#230642),(#230643,#230644,
#230645,#230646),(#230647,#230648,#230649,#230650),(#230651,#230652,#230653,
#230654),(#230655,#230656,#230657,#230658),(#230659,#230660,#230661,#230662),
(#230663,#230664,#230665,#230666),(#230667,#230668,#230669,#230670),(#230671,
#230672,#230673,#230674),(#230675,#230676,#230677,#230678),(#230679,#230680,
#230681,#230682)),.UNSPECIFIED.,.F.,.F.,.F.,(4,1,1,1,2,1,1,1,2,1,1,1,2,
1,1,1,2,1,1,1,2,1,1,1,2,1,1,1,2,1,1,1,4),(4,4),(-0.0947053917544244,0.0379780806838576,
0.0759561613677151,0.113934242051573,0.15191232273543,0.189669188200293,
0.227426053665157,0.26518291913002,0.302939784594882,0.333326792628875,
0.363713800662868,0.394100808696861,0.424487816730854,0.44336586254814,
0.462243908365427,0.481121954182713,0.5,0.518878045817286,0.537756091634573,
0.55663413745186,0.575512183269147,0.60589919130314,0.636286199337133,0.666673207371127,
0.697060215405119,0.734817080869983,0.772573946334846,0.810330811799709,
0.848087677264572,0.886065757948429,0.924043838632286,0.962021919316143,
1.09470538922058),(-0.176001360689901,1.1748817259388),.UNSPECIFIED.);
#942=B_SPLINE_SURFACE_WITH_KNOTS('',3,1,((#230683,#230684),(#230685,#230686),
(#230687,#230688),(#230689,#230690),(#230691,#230692),(#230693,#230694),
(#230695,#230696),(#230697,#230698),(#230699,#230700),(#230701,#230702),
(#230703,#230704),(#230705,#230706),(#230707,#230708),(#230709,#230710),
(#230711,#230712),(#230713,#230714),(#230715,#230716),(#230717,#230718),
(#230719,#230720),(#230721,#230722),(#230723,#230724),(#230725,#230726),
(#230727,#230728),(#230729,#230730),(#230731,#230732),(#230733,#230734),
(#230735,#230736),(#230737,#230738),(#230739,#230740),(#230741,#230742),
(#230743,#230744),(#230745,#230746),(#230747,#230748),(#230749,#230750),
(#230751,#230752),(#230753,#230754),(#230755,#230756),(#230757,#230758),
(#230759,#230760),(#230761,#230762),(#230763,#230764),(#230765,#230766)),
 .UNSPECIFIED.,.F.,.F.,.F.,(4,1,1,1,2,1,1,1,2,1,1,1,2,1,1,1,2,1,1,1,2,1,
1,1,2,1,1,1,2,1,1,1,4),(2,2),(-0.130664626928687,0.0411596607520464,0.0823193215040928,
0.123478982256139,0.164638643008186,0.198458137911997,0.232277632815809,
0.26609712771962,0.299916622623432,0.332619014198497,0.365321405773562,
0.398023797348627,0.430726188923692,0.448044641692768,0.465363094461843,
0.482681547230919,0.499999999999994,0.517318452769073,0.534636905538152,
0.55195535830723,0.569273811076309,0.601976202651373,0.634678594226438,
0.667380985801503,0.700083377376568,0.73390287228038,0.767722367184191,
0.801541862088003,0.835361356991815,0.876521017743861,0.917680678495907,
0.958840339247954,1.12208155081997),(-0.184126650858872,1.18095881489235),
 .UNSPECIFIED.);
#943=B_SPLINE_SURFACE_WITH_KNOTS('',3,3,((#230837,#230838,#230839,#230840,
#230841,#230842,#230843),(#230844,#230845,#230846,#230847,#230848,#230849,
#230850),(#230851,#230852,#230853,#230854,#230855,#230856,#230857),(#230858,
#230859,#230860,#230861,#230862,#230863,#230864),(#230865,#230866,#230867,
#230868,#230869,#230870,#230871),(#230872,#230873,#230874,#230875,#230876,
#230877,#230878),(#230879,#230880,#230881,#230882,#230883,#230884,#230885),
(#230886,#230887,#230888,#230889,#230890,#230891,#230892),(#230893,#230894,
#230895,#230896,#230897,#230898,#230899),(#230900,#230901,#230902,#230903,
#230904,#230905,#230906),(#230907,#230908,#230909,#230910,#230911,#230912,
#230913)),.UNSPECIFIED.,.F.,.F.,.F.,(4,1,1,1,1,1,1,1,4),(4,3,4),(0.,0.124999999999998,
0.249999999999996,0.374999999999993,0.500000000000009,0.625000000000007,
0.75,0.875,1.),(0.,1.,1.01),.UNSPECIFIED.);
#944=B_SPLINE_SURFACE_WITH_KNOTS('',3,3,((#230919,#230920,#230921,#230922,
#230923,#230924,#230925),(#230926,#230927,#230928,#230929,#230930,#230931,
#230932),(#230933,#230934,#230935,#230936,#230937,#230938,#230939),(#230940,
#230941,#230942,#230943,#230944,#230945,#230946),(#230947,#230948,#230949,
#230950,#230951,#230952,#230953),(#230954,#230955,#230956,#230957,#230958,
#230959,#230960),(#230961,#230962,#230963,#230964,#230965,#230966,#230967),
(#230968,#230969,#230970,#230971,#230972,#230973,#230974),(#230975,#230976,
#230977,#230978,#230979,#230980,#230981),(#230982,#230983,#230984,#230985,
#230986,#230987,#230988),(#230989,#230990,#230991,#230992,#230993,#230994,
#230995),(#230996,#230997,#230998,#230999,#231000,#231001,#231002),(#231003,
#231004,#231005,#231006,#231007,#231008,#231009),(#231010,#231011,#231012,
#231013,#231014,#231015,#231016)),.UNSPECIFIED.,.F.,.F.,.F.,(4,3,1,1,1,
1,1,1,1,4),(4,3,4),(-0.01,0.,0.124999999999997,0.249999999999995,0.374999999999992,
0.49999999999999,0.624999999999988,0.749999999999985,0.874999999999983,
1.),(0.,1.,1.01),.UNSPECIFIED.);
#945=B_SPLINE_SURFACE_WITH_KNOTS('',3,3,((#231022,#231023,#231024,#231025,
#231026,#231027,#231028),(#231029,#231030,#231031,#231032,#231033,#231034,
#231035),(#231036,#231037,#231038,#231039,#231040,#231041,#231042),(#231043,
#231044,#231045,#231046,#231047,#231048,#231049),(#231050,#231051,#231052,
#231053,#231054,#231055,#231056),(#231057,#231058,#231059,#231060,#231061,
#231062,#231063),(#231064,#231065,#231066,#231067,#231068,#231069,#231070),
(#231071,#231072,#231073,#231074,#231075,#231076,#231077),(#231078,#231079,
#231080,#231081,#231082,#231083,#231084),(#231085,#231086,#231087,#231088,
#231089,#231090,#231091),(#231092,#231093,#231094,#231095,#231096,#231097,
#231098)),.UNSPECIFIED.,.F.,.F.,.F.,(4,1,1,1,1,1,1,1,4),(4,3,4),(0.,0.124999999999997,
0.249999999999998,0.375,0.5,0.625,0.75,0.875,1.),(0.,1.,1.01),
 .UNSPECIFIED.);
#946=B_SPLINE_SURFACE_WITH_KNOTS('',3,3,((#231104,#231105,#231106,#231107,
#231108,#231109,#231110),(#231111,#231112,#231113,#231114,#231115,#231116,
#231117),(#231118,#231119,#231120,#231121,#231122,#231123,#231124),(#231125,
#231126,#231127,#231128,#231129,#231130,#231131),(#231132,#231133,#231134,
#231135,#231136,#231137,#231138),(#231139,#231140,#231141,#231142,#231143,
#231144,#231145),(#231146,#231147,#231148,#231149,#231150,#231151,#231152),
(#231153,#231154,#231155,#231156,#231157,#231158,#231159),(#231160,#231161,
#231162,#231163,#231164,#231165,#231166),(#231167,#231168,#231169,#231170,
#231171,#231172,#231173),(#231174,#231175,#231176,#231177,#231178,#231179,
#231180),(#231181,#231182,#231183,#231184,#231185,#231186,#231187),(#231188,
#231189,#231190,#231191,#231192,#231193,#231194),(#231195,#231196,#231197,
#231198,#231199,#231200,#231201),(#231202,#231203,#231204,#231205,#231206,
#231207,#231208),(#231209,#231210,#231211,#231212,#231213,#231214,#231215),
(#231216,#231217,#231218,#231219,#231220,#231221,#231222)),
 .UNSPECIFIED.,.F.,.F.,.F.,(4,3,1,1,1,1,1,1,1,3,4),(4,3,4),(-0.01,0.,0.125,
0.25,0.375,0.5,0.625,0.75,0.875,1.,1.01),(0.,1.,1.01),.UNSPECIFIED.);
#947=B_SPLINE_SURFACE_WITH_KNOTS('',3,3,((#231279,#231280,#231281,#231282),
(#231283,#231284,#231285,#231286),(#231287,#231288,#231289,#231290),(#231291,
#231292,#231293,#231294),(#231295,#231296,#231297,#231298),(#231299,#231300,
#231301,#231302),(#231303,#231304,#231305,#231306)),.UNSPECIFIED.,.F.,.F.,
 .F.,(4,1,1,1,4),(4,4),(0.,0.25,0.5,0.75,1.),(0.,1.),.UNSPECIFIED.);
#948=B_SPLINE_SURFACE_WITH_KNOTS('',3,3,((#231307,#231308,#231309,#231310,
#231311,#231312,#231313),(#231314,#231315,#231316,#231317,#231318,#231319,
#231320),(#231321,#231322,#231323,#231324,#231325,#231326,#231327),(#231328,
#231329,#231330,#231331,#231332,#231333,#231334),(#231335,#231336,#231337,
#231338,#231339,#231340,#231341),(#231342,#231343,#231344,#231345,#231346,
#231347,#231348),(#231349,#231350,#231351,#231352,#231353,#231354,#231355)),
 .UNSPECIFIED.,.F.,.F.,.F.,(4,1,1,1,4),(4,3,4),(0.,0.25,0.5,0.75,1.),(0.,
1.,1.01),.UNSPECIFIED.);
#949=B_SPLINE_SURFACE_WITH_KNOTS('',3,3,((#231357,#231358,#231359,#231360,
#231361,#231362,#231363),(#231364,#231365,#231366,#231367,#231368,#231369,
#231370),(#231371,#231372,#231373,#231374,#231375,#231376,#231377),(#231378,
#231379,#231380,#231381,#231382,#231383,#231384),(#231385,#231386,#231387,
#231388,#231389,#231390,#231391),(#231392,#231393,#231394,#231395,#231396,
#231397,#231398),(#231399,#231400,#231401,#231402,#231403,#231404,#231405)),
 .UNSPECIFIED.,.F.,.F.,.F.,(4,1,1,1,4),(4,3,4),(0.,0.25,0.5,0.75,1.),(0.,
1.,1.01),.UNSPECIFIED.);
#950=B_SPLINE_SURFACE_WITH_KNOTS('',3,3,((#231408,#231409,#231410,#231411,
#231412,#231413,#231414),(#231415,#231416,#231417,#231418,#231419,#231420,
#231421),(#231422,#231423,#231424,#231425,#231426,#231427,#231428),(#231429,
#231430,#231431,#231432,#231433,#231434,#231435),(#231436,#231437,#231438,
#231439,#231440,#231441,#231442),(#231443,#231444,#231445,#231446,#231447,
#231448,#231449),(#231450,#231451,#231452,#231453,#231454,#231455,#231456)),
 .UNSPECIFIED.,.F.,.F.,.F.,(4,1,1,1,4),(4,3,4),(0.,0.25,0.5,0.75,1.),(0.,
1.,1.01),.UNSPECIFIED.);
#951=B_SPLINE_SURFACE_WITH_KNOTS('',3,3,((#231458,#231459,#231460,#231461,
#231462,#231463,#231464,#231465,#231466,#231467,#231468,#231469,#231470,
#231471,#231472,#231473),(#231474,#231475,#231476,#231477,#231478,#231479,
#231480,#231481,#231482,#231483,#231484,#231485,#231486,#231487,#231488,
#231489),(#231490,#231491,#231492,#231493,#231494,#231495,#231496,#231497,
#231498,#231499,#231500,#231501,#231502,#231503,#231504,#231505),(#231506,
#231507,#231508,#231509,#231510,#231511,#231512,#231513,#231514,#231515,
#231516,#231517,#231518,#231519,#231520,#231521),(#231522,#231523,#231524,
#231525,#231526,#231527,#231528,#231529,#231530,#231531,#231532,#231533,
#231534,#231535,#231536,#231537),(#231538,#231539,#231540,#231541,#231542,
#231543,#231544,#231545,#231546,#231547,#231548,#231549,#231550,#231551,
#231552,#231553),(#231554,#231555,#231556,#231557,#231558,#231559,#231560,
#231561,#231562,#231563,#231564,#231565,#231566,#231567,#231568,#231569),
(#231570,#231571,#231572,#231573,#231574,#231575,#231576,#231577,#231578,
#231579,#231580,#231581,#231582,#231583,#231584,#231585),(#231586,#231587,
#231588,#231589,#231590,#231591,#231592,#231593,#231594,#231595,#231596,
#231597,#231598,#231599,#231600,#231601),(#231602,#231603,#231604,#231605,
#231606,#231607,#231608,#231609,#231610,#231611,#231612,#231613,#231614,
#231615,#231616,#231617),(#231618,#231619,#231620,#231621,#231622,#231623,
#231624,#231625,#231626,#231627,#231628,#231629,#231630,#231631,#231632,
#231633),(#231634,#231635,#231636,#231637,#231638,#231639,#231640,#231641,
#231642,#231643,#231644,#231645,#231646,#231647,#231648,#231649),(#231650,
#231651,#231652,#231653,#231654,#231655,#231656,#231657,#231658,#231659,
#231660,#231661,#231662,#231663,#231664,#231665),(#231666,#231667,#231668,
#231669,#231670,#231671,#231672,#231673,#231674,#231675,#231676,#231677,
#231678,#231679,#231680,#231681),(#231682,#231683,#231684,#231685,#231686,
#231687,#231688,#231689,#231690,#231691,#231692,#231693,#231694,#231695,
#231696,#231697),(#231698,#231699,#231700,#231701,#231702,#231703,#231704,
#231705,#231706,#231707,#231708,#231709,#231710,#231711,#231712,#231713),
(#231714,#231715,#231716,#231717,#231718,#231719,#231720,#231721,#231722,
#231723,#231724,#231725,#231726,#231727,#231728,#231729),(#231730,#231731,
#231732,#231733,#231734,#231735,#231736,#231737,#231738,#231739,#231740,
#231741,#231742,#231743,#231744,#231745),(#231746,#231747,#231748,#231749,
#231750,#231751,#231752,#231753,#231754,#231755,#231756,#231757,#231758,
#231759,#231760,#231761),(#231762,#231763,#231764,#231765,#231766,#231767,
#231768,#231769,#231770,#231771,#231772,#231773,#231774,#231775,#231776,
#231777),(#231778,#231779,#231780,#231781,#231782,#231783,#231784,#231785,
#231786,#231787,#231788,#231789,#231790,#231791,#231792,#231793),(#231794,
#231795,#231796,#231797,#231798,#231799,#231800,#231801,#231802,#231803,
#231804,#231805,#231806,#231807,#231808,#231809),(#231810,#231811,#231812,
#231813,#231814,#231815,#231816,#231817,#231818,#231819,#231820,#231821,
#231822,#231823,#231824,#231825),(#231826,#231827,#231828,#231829,#231830,
#231831,#231832,#231833,#231834,#231835,#231836,#231837,#231838,#231839,
#231840,#231841),(#231842,#231843,#231844,#231845,#231846,#231847,#231848,
#231849,#231850,#231851,#231852,#231853,#231854,#231855,#231856,#231857),
(#231858,#231859,#231860,#231861,#231862,#231863,#231864,#231865,#231866,
#231867,#231868,#231869,#231870,#231871,#231872,#231873),(#231874,#231875,
#231876,#231877,#231878,#231879,#231880,#231881,#231882,#231883,#231884,
#231885,#231886,#231887,#231888,#231889),(#231890,#231891,#231892,#231893,
#231894,#231895,#231896,#231897,#231898,#231899,#231900,#231901,#231902,
#231903,#231904,#231905),(#231906,#231907,#231908,#231909,#231910,#231911,
#231912,#231913,#231914,#231915,#231916,#231917,#231918,#231919,#231920,
#231921),(#231922,#231923,#231924,#231925,#231926,#231927,#231928,#231929,
#231930,#231931,#231932,#231933,#231934,#231935,#231936,#231937),(#231938,
#231939,#231940,#231941,#231942,#231943,#231944,#231945,#231946,#231947,
#231948,#231949,#231950,#231951,#231952,#231953),(#231954,#231955,#231956,
#231957,#231958,#231959,#231960,#231961,#231962,#231963,#231964,#231965,
#231966,#231967,#231968,#231969),(#231970,#231971,#231972,#231973,#231974,
#231975,#231976,#231977,#231978,#231979,#231980,#231981,#231982,#231983,
#231984,#231985),(#231986,#231987,#231988,#231989,#231990,#231991,#231992,
#231993,#231994,#231995,#231996,#231997,#231998,#231999,#232000,#232001),
(#232002,#232003,#232004,#232005,#232006,#232007,#232008,#232009,#232010,
#232011,#232012,#232013,#232014,#232015,#232016,#232017),(#232018,#232019,
#232020,#232021,#232022,#232023,#232024,#232025,#232026,#232027,#232028,
#232029,#232030,#232031,#232032,#232033),(#232034,#232035,#232036,#232037,
#232038,#232039,#232040,#232041,#232042,#232043,#232044,#232045,#232046,
#232047,#232048,#232049),(#232050,#232051,#232052,#232053,#232054,#232055,
#232056,#232057,#232058,#232059,#232060,#232061,#232062,#232063,#232064,
#232065),(#232066,#232067,#232068,#232069,#232070,#232071,#232072,#232073,
#232074,#232075,#232076,#232077,#232078,#232079,#232080,#232081),(#232082,
#232083,#232084,#232085,#232086,#232087,#232088,#232089,#232090,#232091,
#232092,#232093,#232094,#232095,#232096,#232097),(#232098,#232099,#232100,
#232101,#232102,#232103,#232104,#232105,#232106,#232107,#232108,#232109,
#232110,#232111,#232112,#232113),(#232114,#232115,#232116,#232117,#232118,
#232119,#232120,#232121,#232122,#232123,#232124,#232125,#232126,#232127,
#232128,#232129),(#232130,#232131,#232132,#232133,#232134,#232135,#232136,
#232137,#232138,#232139,#232140,#232141,#232142,#232143,#232144,#232145)),
 .UNSPECIFIED.,.F.,.F.,.F.,(4,3,3,3,3,3,3,1,1,1,3,3,3,3,3,3,4),(4,3,3,3,
3,4),(-364.,-121.,-40.,-13.,-4.,-1.,0.,0.25,0.5,0.75,1.,2.,5.,14.,41.,122.,
365.),(-7.07,-3.03,-1.01,0.,1.,1.01),.UNSPECIFIED.);
#952=B_SPLINE_SURFACE_WITH_KNOTS('',3,3,((#232147,#232148,#232149,#232150,
#232151,#232152,#232153,#232154,#232155,#232156,#232157,#232158,#232159,
#232160,#232161,#232162),(#232163,#232164,#232165,#232166,#232167,#232168,
#232169,#232170,#232171,#232172,#232173,#232174,#232175,#232176,#232177,
#232178),(#232179,#232180,#232181,#232182,#232183,#232184,#232185,#232186,
#232187,#232188,#232189,#232190,#232191,#232192,#232193,#232194),(#232195,
#232196,#232197,#232198,#232199,#232200,#232201,#232202,#232203,#232204,
#232205,#232206,#232207,#232208,#232209,#232210),(#232211,#232212,#232213,
#232214,#232215,#232216,#232217,#232218,#232219,#232220,#232221,#232222,
#232223,#232224,#232225,#232226),(#232227,#232228,#232229,#232230,#232231,
#232232,#232233,#232234,#232235,#232236,#232237,#232238,#232239,#232240,
#232241,#232242),(#232243,#232244,#232245,#232246,#232247,#232248,#232249,
#232250,#232251,#232252,#232253,#232254,#232255,#232256,#232257,#232258),
(#232259,#232260,#232261,#232262,#232263,#232264,#232265,#232266,#232267,
#232268,#232269,#232270,#232271,#232272,#232273,#232274),(#232275,#232276,
#232277,#232278,#232279,#232280,#232281,#232282,#232283,#232284,#232285,
#232286,#232287,#232288,#232289,#232290),(#232291,#232292,#232293,#232294,
#232295,#232296,#232297,#232298,#232299,#232300,#232301,#232302,#232303,
#232304,#232305,#232306),(#232307,#232308,#232309,#232310,#232311,#232312,
#232313,#232314,#232315,#232316,#232317,#232318,#232319,#232320,#232321,
#232322),(#232323,#232324,#232325,#232326,#232327,#232328,#232329,#232330,
#232331,#232332,#232333,#232334,#232335,#232336,#232337,#232338),(#232339,
#232340,#232341,#232342,#232343,#232344,#232345,#232346,#232347,#232348,
#232349,#232350,#232351,#232352,#232353,#232354),(#232355,#232356,#232357,
#232358,#232359,#232360,#232361,#232362,#232363,#232364,#232365,#232366,
#232367,#232368,#232369,#232370),(#232371,#232372,#232373,#232374,#232375,
#232376,#232377,#232378,#232379,#232380,#232381,#232382,#232383,#232384,
#232385,#232386),(#232387,#232388,#232389,#232390,#232391,#232392,#232393,
#232394,#232395,#232396,#232397,#232398,#232399,#232400,#232401,#232402),
(#232403,#232404,#232405,#232406,#232407,#232408,#232409,#232410,#232411,
#232412,#232413,#232414,#232415,#232416,#232417,#232418),(#232419,#232420,
#232421,#232422,#232423,#232424,#232425,#232426,#232427,#232428,#232429,
#232430,#232431,#232432,#232433,#232434),(#232435,#232436,#232437,#232438,
#232439,#232440,#232441,#232442,#232443,#232444,#232445,#232446,#232447,
#232448,#232449,#232450),(#232451,#232452,#232453,#232454,#232455,#232456,
#232457,#232458,#232459,#232460,#232461,#232462,#232463,#232464,#232465,
#232466),(#232467,#232468,#232469,#232470,#232471,#232472,#232473,#232474,
#232475,#232476,#232477,#232478,#232479,#232480,#232481,#232482),(#232483,
#232484,#232485,#232486,#232487,#232488,#232489,#232490,#232491,#232492,
#232493,#232494,#232495,#232496,#232497,#232498),(#232499,#232500,#232501,
#232502,#232503,#232504,#232505,#232506,#232507,#232508,#232509,#232510,
#232511,#232512,#232513,#232514),(#232515,#232516,#232517,#232518,#232519,
#232520,#232521,#232522,#232523,#232524,#232525,#232526,#232527,#232528,
#232529,#232530),(#232531,#232532,#232533,#232534,#232535,#232536,#232537,
#232538,#232539,#232540,#232541,#232542,#232543,#232544,#232545,#232546),
(#232547,#232548,#232549,#232550,#232551,#232552,#232553,#232554,#232555,
#232556,#232557,#232558,#232559,#232560,#232561,#232562),(#232563,#232564,
#232565,#232566,#232567,#232568,#232569,#232570,#232571,#232572,#232573,
#232574,#232575,#232576,#232577,#232578),(#232579,#232580,#232581,#232582,
#232583,#232584,#232585,#232586,#232587,#232588,#232589,#232590,#232591,
#232592,#232593,#232594),(#232595,#232596,#232597,#232598,#232599,#232600,
#232601,#232602,#232603,#232604,#232605,#232606,#232607,#232608,#232609,
#232610),(#232611,#232612,#232613,#232614,#232615,#232616,#232617,#232618,
#232619,#232620,#232621,#232622,#232623,#232624,#232625,#232626),(#232627,
#232628,#232629,#232630,#232631,#232632,#232633,#232634,#232635,#232636,
#232637,#232638,#232639,#232640,#232641,#232642),(#232643,#232644,#232645,
#232646,#232647,#232648,#232649,#232650,#232651,#232652,#232653,#232654,
#232655,#232656,#232657,#232658),(#232659,#232660,#232661,#232662,#232663,
#232664,#232665,#232666,#232667,#232668,#232669,#232670,#232671,#232672,
#232673,#232674),(#232675,#232676,#232677,#232678,#232679,#232680,#232681,
#232682,#232683,#232684,#232685,#232686,#232687,#232688,#232689,#232690),
(#232691,#232692,#232693,#232694,#232695,#232696,#232697,#232698,#232699,
#232700,#232701,#232702,#232703,#232704,#232705,#232706),(#232707,#232708,
#232709,#232710,#232711,#232712,#232713,#232714,#232715,#232716,#232717,
#232718,#232719,#232720,#232721,#232722),(#232723,#232724,#232725,#232726,
#232727,#232728,#232729,#232730,#232731,#232732,#232733,#232734,#232735,
#232736,#232737,#232738)),.UNSPECIFIED.,.F.,.F.,.F.,(4,3,3,3,3,3,1,1,1,
3,3,3,3,3,4),(4,3,3,3,3,4),(-121.,-40.,-13.,-4.,-1.,0.,0.25,0.5,0.75,1.,
2.,5.,14.,41.,122.),(-7.07,-3.03,-1.01,0.,1.,1.01),.UNSPECIFIED.);
#953=B_SPLINE_SURFACE_WITH_KNOTS('',1,3,((#244024,#244025,#244026,#244027,
#244028,#244029,#244030,#244031,#244032,#244033,#244034,#244035,#244036,
#244037,#244038,#244039,#244040,#244041,#244042,#244043,#244044,#244045,
#244046,#244047,#244048,#244049,#244050,#244051,#244052,#244053,#244054,
#244055,#244056,#244057,#244058,#244059,#244060,#244061,#244062,#244063,
#244064,#244065,#244066,#244067,#244068,#244069,#244070,#244071,#244072,
#244073,#244074,#244075,#244076,#244077,#244078,#244079,#244080,#244081,
#244082,#244083,#244084,#244085,#244086,#244087,#244088,#244089,#244090,
#244091,#244092,#244093,#244094,#244095,#244096,#244097,#244098,#244099,
#244100,#244101,#244102,#244103,#244104,#244105,#244106,#244107,#244108,
#244109,#244110,#244111,#244112,#244113,#244114,#244115,#244116,#244117,
#244118,#244119,#244120,#244121,#244122,#244123,#244124,#244125,#244126,
#244127,#244128,#244129,#244130,#244131,#244132,#244133,#244134,#244135,
#244136,#244137,#244138,#244139,#244140,#244141,#244142,#244143,#244144,
#244145,#244146,#244147,#244148,#244149,#244150,#244151,#244152,#244153,
#244154,#244155,#244156,#244157,#244158,#244159,#244160,#244161,#244162,
#244163,#244164,#244165,#244166,#244167,#244168,#244169,#244170,#244171,
#244172,#244173,#244174,#244175,#244176,#244177,#244178,#244179,#244180,
#244181,#244182,#244183,#244184,#244185,#244186,#244187,#244188,#244189,
#244190,#244191,#244192,#244193,#244194,#244195,#244196,#244197,#244198),
(#244199,#244200,#244201,#244202,#244203,#244204,#244205,#244206,#244207,
#244208,#244209,#244210,#244211,#244212,#244213,#244214,#244215,#244216,
#244217,#244218,#244219,#244220,#244221,#244222,#244223,#244224,#244225,
#244226,#244227,#244228,#244229,#244230,#244231,#244232,#244233,#244234,
#244235,#244236,#244237,#244238,#244239,#244240,#244241,#244242,#244243,
#244244,#244245,#244246,#244247,#244248,#244249,#244250,#244251,#244252,
#244253,#244254,#244255,#244256,#244257,#244258,#244259,#244260,#244261,
#244262,#244263,#244264,#244265,#244266,#244267,#244268,#244269,#244270,
#244271,#244272,#244273,#244274,#244275,#244276,#244277,#244278,#244279,
#244280,#244281,#244282,#244283,#244284,#244285,#244286,#244287,#244288,
#244289,#244290,#244291,#244292,#244293,#244294,#244295,#244296,#244297,
#244298,#244299,#244300,#244301,#244302,#244303,#244304,#244305,#244306,
#244307,#244308,#244309,#244310,#244311,#244312,#244313,#244314,#244315,
#244316,#244317,#244318,#244319,#244320,#244321,#244322,#244323,#244324,
#244325,#244326,#244327,#244328,#244329,#244330,#244331,#244332,#244333,
#244334,#244335,#244336,#244337,#244338,#244339,#244340,#244341,#244342,
#244343,#244344,#244345,#244346,#244347,#244348,#244349,#244350,#244351,
#244352,#244353,#244354,#244355,#244356,#244357,#244358,#244359,#244360,
#244361,#244362,#244363,#244364,#244365,#244366,#244367,#244368,#244369,
#244370,#244371,#244372,#244373)),.UNSPECIFIED.,.F.,.T.,.F.,(2,2),(4,1,
1,2,1,1,1,1,2,2,1,2,2,2,2,1,1,2,2,2,1,1,1,1,2,2,2,2,2,2,2,2,1,1,1,2,2,2,
2,1,1,1,2,2,2,1,1,1,2,2,2,2,2,2,2,1,2,2,2,2,2,1,1,2,2,2,2,1,2,2,2,1,1,2,
2,2,1,1,1,1,2,2,2,2,2,2,2,1,2,1,1,2,2,2,1,2,2,2,2,2,1,2,2,2,2,4),(0.,4.71475608888856),
(-0.000135430429350568,9.25560474171526E-5,0.000320542524184873,0.000548529000952593,
0.000776515477720314,0.00100450195448803,0.00111849519287189,0.00123248843125575,
0.00134648166963961,0.00146047490802347,0.0016884613847912,0.00191644786155891,
0.00203044109994277,0.00214443433832664,0.00225842757671049,0.00237242081509435,
0.00260040729186208,0.00271440053024594,0.0028283937686298,0.00294238700701366,
0.00305638024539752,0.00317037348378138,0.00328436672216524,0.0033983599605491,
0.00351235319893296,0.00362634643731682,0.00374033967570068,0.0039683261524684,
0.00419631262923612,0.00431030586761998,0.00436730248681191,0.00442429910600384,
0.0045382923443877,0.00465228558277156,0.00488027205953928,0.00499426529792314,
0.005108258536307,0.00522225177469086,0.00533624501307472,0.00556423148984244,
0.0056782247282263,0.00579221796661016,0.00590621120499402,0.00602020444337788,
0.00613419768176174,0.0062481909201456,0.00647617739691333,0.00659017063529719,
0.00670416387368105,0.00681815711206491,0.00693215035044876,0.00716013682721649,
0.00727413006560035,0.00738812330398421,0.00761610978075193,0.00784409625751965,
0.00795808949590351,0.00807208273428737,0.0081290793534793,0.00818607597267123,
0.00830006921105509,0.00852805568782281,0.00864204892620667,0.00875604216459053,
0.00887003540297439,0.00898402864135825,0.00921201511812597,0.00944000159489369,
0.00955399483327755,0.00966798807166141,0.00978198131004527,0.00989597454842913,
0.0101239610251968,0.0102379542635807,0.0103519475019646,0.0104659407403484,
0.0105799339787323,0.0106939272171161,0.0108079204555,0.0109219136938839,
0.0110359069322677,0.0111499001706516,0.0112638934090355,0.0114918798858032,
0.0117198663625709,0.0118338596009548,0.0118908562201467,0.0119478528393386,
0.0120618460777225,0.0121758393161063,0.0124038257928741,0.0125178190312579,
0.0126318122696418,0.0127458055080256,0.0129737919847934,0.0130877852231772,
0.0133157716999449,0.0134297649383288,0.0134867615575207,0.0135437581767127,
0.0137717446534804,0.0139997311302481,0.0142277176070158,0.0142847142262077,
0.0143417108453997,0.0144557040837835),.UNSPECIFIED.);
#954=B_SPLINE_SURFACE_WITH_KNOTS('',1,3,((#245024,#245025,#245026,#245027,
#245028,#245029,#245030,#245031,#245032,#245033,#245034,#245035,#245036,
#245037,#245038,#245039,#245040,#245041,#245042,#245043,#245044,#245045,
#245046,#245047,#245048,#245049,#245050,#245051,#245052,#245053,#245054,
#245055,#245056,#245057,#245058,#245059,#245060,#245061,#245062,#245063,
#245064,#245065,#245066,#245067,#245068,#245069,#245070,#245071,#245072,
#245073,#245074,#245075,#245076,#245077,#245078,#245079,#245080,#245081,
#245082,#245083,#245084,#245085,#245086,#245087,#245088,#245089,#245090,
#245091,#245092,#245093,#245094,#245095,#245096,#245097,#245098,#245099,
#245100,#245101,#245102,#245103,#245104,#245105,#245106,#245107,#245108,
#245109,#245110,#245111,#245112,#245113,#245114,#245115,#245116,#245117,
#245118,#245119,#245120,#245121,#245122,#245123,#245124,#245125,#245126,
#245127,#245128,#245129,#245130,#245131,#245132,#245133,#245134,#245135,
#245136,#245137,#245138,#245139,#245140,#245141,#245142,#245143,#245144,
#245145,#245146,#245147,#245148,#245149,#245150,#245151,#245152,#245153,
#245154,#245155,#245156,#245157,#245158,#245159,#245160,#245161,#245162,
#245163,#245164,#245165,#245166,#245167,#245168,#245169,#245170,#245171,
#245172,#245173,#245174,#245175,#245176,#245177,#245178,#245179,#245180,
#245181,#245182,#245183,#245184,#245185,#245186,#245187,#245188,#245189,
#245190,#245191,#245192,#245193,#245194,#245195,#245196,#245197,#245198),
(#245199,#245200,#245201,#245202,#245203,#245204,#245205,#245206,#245207,
#245208,#245209,#245210,#245211,#245212,#245213,#245214,#245215,#245216,
#245217,#245218,#245219,#245220,#245221,#245222,#245223,#245224,#245225,
#245226,#245227,#245228,#245229,#245230,#245231,#245232,#245233,#245234,
#245235,#245236,#245237,#245238,#245239,#245240,#245241,#245242,#245243,
#245244,#245245,#245246,#245247,#245248,#245249,#245250,#245251,#245252,
#245253,#245254,#245255,#245256,#245257,#245258,#245259,#245260,#245261,
#245262,#245263,#245264,#245265,#245266,#245267,#245268,#245269,#245270,
#245271,#245272,#245273,#245274,#245275,#245276,#245277,#245278,#245279,
#245280,#245281,#245282,#245283,#245284,#245285,#245286,#245287,#245288,
#245289,#245290,#245291,#245292,#245293,#245294,#245295,#245296,#245297,
#245298,#245299,#245300,#245301,#245302,#245303,#245304,#245305,#245306,
#245307,#245308,#245309,#245310,#245311,#245312,#245313,#245314,#245315,
#245316,#245317,#245318,#245319,#245320,#245321,#245322,#245323,#245324,
#245325,#245326,#245327,#245328,#245329,#245330,#245331,#245332,#245333,
#245334,#245335,#245336,#245337,#245338,#245339,#245340,#245341,#245342,
#245343,#245344,#245345,#245346,#245347,#245348,#245349,#245350,#245351,
#245352,#245353,#245354,#245355,#245356,#245357,#245358,#245359,#245360,
#245361,#245362,#245363,#245364,#245365,#245366,#245367,#245368,#245369,
#245370,#245371,#245372,#245373)),.UNSPECIFIED.,.F.,.T.,.F.,(2,2),(4,1,
1,2,1,1,1,1,2,2,1,2,2,2,2,1,1,2,2,2,1,1,1,1,2,2,2,2,2,2,2,2,1,1,1,2,2,2,
2,1,1,1,2,2,2,1,1,1,2,2,2,2,2,2,2,1,2,2,2,2,2,1,1,2,2,2,2,1,2,2,2,1,1,2,
2,2,1,1,1,1,2,2,2,2,2,2,2,1,2,1,1,2,2,2,1,2,2,2,2,2,1,2,2,2,2,4),(0.,5.46382276754873),
(-0.000135430429350568,9.25560474171526E-5,0.000320542524184873,0.000548529000952593,
0.000776515477720314,0.00100450195448803,0.00111849519287189,0.00123248843125575,
0.00134648166963961,0.00146047490802347,0.0016884613847912,0.00191644786155891,
0.00203044109994277,0.00214443433832664,0.00225842757671049,0.00237242081509435,
0.00260040729186208,0.00271440053024594,0.0028283937686298,0.00294238700701366,
0.00305638024539752,0.00317037348378138,0.00328436672216524,0.0033983599605491,
0.00351235319893296,0.00362634643731682,0.00374033967570068,0.0039683261524684,
0.00419631262923612,0.00431030586761998,0.00436730248681191,0.00442429910600384,
0.0045382923443877,0.00465228558277156,0.00488027205953928,0.00499426529792314,
0.005108258536307,0.00522225177469086,0.00533624501307472,0.00556423148984244,
0.0056782247282263,0.00579221796661016,0.00590621120499402,0.00602020444337788,
0.00613419768176174,0.0062481909201456,0.00647617739691333,0.00659017063529719,
0.00670416387368105,0.00681815711206491,0.00693215035044876,0.00716013682721649,
0.00727413006560035,0.00738812330398421,0.00761610978075193,0.00784409625751965,
0.00795808949590351,0.00807208273428737,0.0081290793534793,0.00818607597267123,
0.00830006921105509,0.00852805568782281,0.00864204892620667,0.00875604216459053,
0.00887003540297439,0.00898402864135825,0.00921201511812597,0.00944000159489369,
0.00955399483327755,0.00966798807166141,0.00978198131004527,0.00989597454842913,
0.0101239610251968,0.0102379542635807,0.0103519475019646,0.0104659407403484,
0.0105799339787323,0.0106939272171161,0.0108079204555,0.0109219136938839,
0.0110359069322677,0.0111499001706516,0.0112638934090355,0.0114918798858032,
0.0117198663625709,0.0118338596009548,0.0118908562201467,0.0119478528393386,
0.0120618460777225,0.0121758393161063,0.0124038257928741,0.0125178190312579,
0.0126318122696418,0.0127458055080256,0.0129737919847934,0.0130877852231772,
0.0133157716999449,0.0134297649383288,0.0134867615575207,0.0135437581767127,
0.0137717446534804,0.0139997311302481,0.0142277176070158,0.0142847142262077,
0.0143417108453997,0.0144557040837835),.UNSPECIFIED.);
#955=B_SPLINE_SURFACE_WITH_KNOTS('',1,3,((#249188,#249189,#249190,#249191,
#249192,#249193,#249194,#249195,#249196,#249197,#249198,#249199,#249200,
#249201,#249202,#249203,#249204,#249205,#249206,#249207,#249208,#249209,
#249210,#249211,#249212,#249213,#249214,#249215,#249216,#249217,#249218,
#249219,#249220,#249221,#249222,#249223,#249224,#249225,#249226,#249227,
#249228,#249229,#249230,#249231,#249232,#249233,#249234,#249235,#249236,
#249237,#249238,#249239,#249240,#249241,#249242,#249243,#249244,#249245,
#249246,#249247,#249248,#249249,#249250,#249251,#249252,#249253,#249254,
#249255,#249256,#249257,#249258,#249259,#249260,#249261,#249262,#249263,
#249264,#249265,#249266,#249267,#249268,#249269,#249270,#249271,#249272,
#249273,#249274,#249275,#249276,#249277,#249278,#249279,#249280,#249281,
#249282,#249283,#249284,#249285,#249286,#249287,#249288,#249289,#249290,
#249291,#249292,#249293,#249294,#249295,#249296,#249297,#249298,#249299,
#249300,#249301,#249302,#249303,#249304,#249305,#249306,#249307,#249308,
#249309,#249310,#249311,#249312,#249313,#249314,#249315,#249316,#249317,
#249318,#249319,#249320,#249321,#249322,#249323,#249324,#249325,#249326,
#249327,#249328,#249329,#249330,#249331,#249332,#249333,#249334,#249335,
#249336,#249337,#249338,#249339,#249340,#249341,#249342,#249343,#249344,
#249345,#249346,#249347,#249348,#249349,#249350,#249351,#249352,#249353,
#249354,#249355,#249356,#249357,#249358,#249359,#249360,#249361,#249362,
#249363,#249364,#249365,#249366),(#249367,#249368,#249369,#249370,#249371,
#249372,#249373,#249374,#249375,#249376,#249377,#249378,#249379,#249380,
#249381,#249382,#249383,#249384,#249385,#249386,#249387,#249388,#249389,
#249390,#249391,#249392,#249393,#249394,#249395,#249396,#249397,#249398,
#249399,#249400,#249401,#249402,#249403,#249404,#249405,#249406,#249407,
#249408,#249409,#249410,#249411,#249412,#249413,#249414,#249415,#249416,
#249417,#249418,#249419,#249420,#249421,#249422,#249423,#249424,#249425,
#249426,#249427,#249428,#249429,#249430,#249431,#249432,#249433,#249434,
#249435,#249436,#249437,#249438,#249439,#249440,#249441,#249442,#249443,
#249444,#249445,#249446,#249447,#249448,#249449,#249450,#249451,#249452,
#249453,#249454,#249455,#249456,#249457,#249458,#249459,#249460,#249461,
#249462,#249463,#249464,#249465,#249466,#249467,#249468,#249469,#249470,
#249471,#249472,#249473,#249474,#249475,#249476,#249477,#249478,#249479,
#249480,#249481,#249482,#249483,#249484,#249485,#249486,#249487,#249488,
#249489,#249490,#249491,#249492,#249493,#249494,#249495,#249496,#249497,
#249498,#249499,#249500,#249501,#249502,#249503,#249504,#249505,#249506,
#249507,#249508,#249509,#249510,#249511,#249512,#249513,#249514,#249515,
#249516,#249517,#249518,#249519,#249520,#249521,#249522,#249523,#249524,
#249525,#249526,#249527,#249528,#249529,#249530,#249531,#249532,#249533,
#249534,#249535,#249536,#249537,#249538,#249539,#249540,#249541,#249542,
#249543,#249544,#249545)),.UNSPECIFIED.,.F.,.T.,.F.,(2,2),(4,1,1,2,2,2,
2,1,1,1,2,2,2,1,1,2,2,2,2,2,2,2,2,2,1,1,1,2,2,2,1,2,2,2,1,2,2,2,1,1,1,1,
2,2,2,1,1,1,1,2,2,2,2,2,2,2,1,1,2,2,2,2,1,2,2,2,1,1,2,2,2,2,2,2,2,2,2,2,
1,1,1,2,2,2,1,1,2,2,2,1,2,2,2,2,2,1,2,2,2,2,2,1,1,1,2,2,4),(0.,5.45368304321453),
(-0.000118831294053002,0.000109147352845132,0.000337125999743267,0.000451115323192334,
0.000565104646641402,0.000679093970090469,0.000793083293539536,0.00102106194043767,
0.00113505126388674,0.0012490405873358,0.00136302991078487,0.00142002457250941,
0.00147701923423394,0.00170499788113207,0.00193297652803021,0.00204696585147928,
0.00216095517492835,0.00227494449837741,0.00238893382182648,0.00261691246872462,
0.00284489111562275,0.00290188577734728,0.00295888043907182,0.00307286976252088,
0.00330084840941902,0.00341483773286809,0.00352882705631715,0.00364281637976622,
0.00375680570321528,0.00387079502666435,0.00398478435011342,0.00421276299701156,
0.00444074164390969,0.00466872029080782,0.00489669893770596,0.00512467758460409,
0.00518167224632863,0.00523866690805316,0.00535265623150223,0.0054666455549513,
0.00558063487840036,0.00569462420184943,0.0058086135252985,0.00592260284874756,
0.00603659217219663,0.0061505814956457,0.00626457081909477,0.0064925494659929,
0.00660653878944197,0.00672052811289104,0.0068345174363401,0.00694850675978917,
0.00717648540668731,0.00729047473013637,0.00740446405358544,0.00763244270048357,
0.00786042134738171,0.00797441067083078,0.00808839999427985,0.00820238931772891,
0.00831637864117798,0.00854435728807612,0.00877233593497425,0.00888632525842331,
0.00900031458187238,0.00911430390532145,0.00922829322877052,0.00945627187566865,
0.00957026119911772,0.00968425052256679,0.00974124518429132,0.00979823984601585,
0.00991222916946492,0.0101402078163631,0.0103681864632612,0.0104251811249857,
0.0104821757867103,0.0105961651101593,0.0108241437570575,0.0109381330805065,
0.0110521224039556,0.0111661117274047,0.0112801010508537,0.0113940903743028,
0.0115080796977519,0.01173605834465,0.0118500476680991,0.0119640369915481,
0.0120780263149972,0.0121920156384463,0.0124199942853444,0.0126479729322425,
0.0127049675939671,0.0127619622556916,0.0128759515791407,0.0131039302260388,
0.0133319088729369,0.013445898196386,0.0135028928581105,0.0135598875198351,
0.0136738768432841,0.0137878661667332,0.0140158448136313,0.0141298341370804,
0.0142438234605295,0.0143578127839785,0.0144718021074276),.UNSPECIFIED.);
#956=B_SPLINE_SURFACE_WITH_KNOTS('',1,3,((#250322,#250323,#250324,#250325,
#250326,#250327,#250328,#250329,#250330,#250331,#250332,#250333,#250334,
#250335,#250336,#250337,#250338,#250339,#250340,#250341,#250342,#250343,
#250344,#250345,#250346,#250347,#250348,#250349,#250350,#250351,#250352,
#250353,#250354,#250355,#250356,#250357,#250358,#250359,#250360,#250361,
#250362,#250363,#250364,#250365,#250366,#250367,#250368,#250369,#250370,
#250371,#250372,#250373,#250374,#250375,#250376,#250377,#250378,#250379,
#250380,#250381,#250382,#250383,#250384,#250385,#250386,#250387,#250388,
#250389,#250390,#250391,#250392,#250393,#250394,#250395,#250396,#250397,
#250398,#250399,#250400,#250401,#250402,#250403,#250404,#250405,#250406,
#250407,#250408,#250409,#250410,#250411,#250412,#250413,#250414,#250415,
#250416,#250417,#250418,#250419,#250420,#250421,#250422,#250423,#250424,
#250425,#250426,#250427,#250428,#250429,#250430,#250431,#250432,#250433,
#250434,#250435,#250436,#250437,#250438,#250439,#250440,#250441,#250442,
#250443,#250444,#250445,#250446,#250447,#250448,#250449,#250450,#250451,
#250452,#250453,#250454,#250455,#250456,#250457,#250458,#250459,#250460,
#250461,#250462,#250463,#250464,#250465,#250466,#250467,#250468,#250469,
#250470,#250471,#250472,#250473,#250474,#250475,#250476,#250477,#250478,
#250479,#250480,#250481,#250482,#250483,#250484,#250485,#250486,#250487,
#250488,#250489,#250490,#250491,#250492,#250493,#250494,#250495,#250496,
#250497,#250498,#250499,#250500),(#250501,#250502,#250503,#250504,#250505,
#250506,#250507,#250508,#250509,#250510,#250511,#250512,#250513,#250514,
#250515,#250516,#250517,#250518,#250519,#250520,#250521,#250522,#250523,
#250524,#250525,#250526,#250527,#250528,#250529,#250530,#250531,#250532,
#250533,#250534,#250535,#250536,#250537,#250538,#250539,#250540,#250541,
#250542,#250543,#250544,#250545,#250546,#250547,#250548,#250549,#250550,
#250551,#250552,#250553,#250554,#250555,#250556,#250557,#250558,#250559,
#250560,#250561,#250562,#250563,#250564,#250565,#250566,#250567,#250568,
#250569,#250570,#250571,#250572,#250573,#250574,#250575,#250576,#250577,
#250578,#250579,#250580,#250581,#250582,#250583,#250584,#250585,#250586,
#250587,#250588,#250589,#250590,#250591,#250592,#250593,#250594,#250595,
#250596,#250597,#250598,#250599,#250600,#250601,#250602,#250603,#250604,
#250605,#250606,#250607,#250608,#250609,#250610,#250611,#250612,#250613,
#250614,#250615,#250616,#250617,#250618,#250619,#250620,#250621,#250622,
#250623,#250624,#250625,#250626,#250627,#250628,#250629,#250630,#250631,
#250632,#250633,#250634,#250635,#250636,#250637,#250638,#250639,#250640,
#250641,#250642,#250643,#250644,#250645,#250646,#250647,#250648,#250649,
#250650,#250651,#250652,#250653,#250654,#250655,#250656,#250657,#250658,
#250659,#250660,#250661,#250662,#250663,#250664,#250665,#250666,#250667,
#250668,#250669,#250670,#250671,#250672,#250673,#250674,#250675,#250676,
#250677,#250678,#250679)),.UNSPECIFIED.,.F.,.T.,.F.,(2,2),(4,1,1,2,2,2,
2,1,1,1,2,2,2,1,1,2,2,2,2,2,2,2,2,2,1,1,1,2,2,2,1,2,2,2,1,2,2,2,1,1,1,1,
2,2,2,1,1,1,1,2,2,2,2,2,2,2,1,1,2,2,2,2,1,2,2,2,1,1,2,2,2,2,2,2,2,2,2,2,
1,1,1,2,2,2,1,1,2,2,2,1,2,2,2,2,2,1,2,2,2,2,2,1,1,1,2,2,4),(0.,5.45368304321453),
(-0.000118831294053002,0.000109147352845132,0.000337125999743267,0.000451115323192334,
0.000565104646641402,0.000679093970090469,0.000793083293539536,0.00102106194043767,
0.00113505126388674,0.0012490405873358,0.00136302991078487,0.00142002457250941,
0.00147701923423394,0.00170499788113207,0.00193297652803021,0.00204696585147928,
0.00216095517492835,0.00227494449837741,0.00238893382182648,0.00261691246872462,
0.00284489111562275,0.00290188577734728,0.00295888043907182,0.00307286976252088,
0.00330084840941902,0.00341483773286809,0.00352882705631715,0.00364281637976622,
0.00375680570321528,0.00387079502666435,0.00398478435011342,0.00421276299701156,
0.00444074164390969,0.00466872029080782,0.00489669893770596,0.00512467758460409,
0.00518167224632863,0.00523866690805316,0.00535265623150223,0.0054666455549513,
0.00558063487840036,0.00569462420184943,0.0058086135252985,0.00592260284874756,
0.00603659217219663,0.0061505814956457,0.00626457081909477,0.0064925494659929,
0.00660653878944197,0.00672052811289104,0.0068345174363401,0.00694850675978917,
0.00717648540668731,0.00729047473013637,0.00740446405358544,0.00763244270048357,
0.00786042134738171,0.00797441067083078,0.00808839999427985,0.00820238931772891,
0.00831637864117798,0.00854435728807612,0.00877233593497425,0.00888632525842331,
0.00900031458187238,0.00911430390532145,0.00922829322877052,0.00945627187566865,
0.00957026119911772,0.00968425052256679,0.00974124518429132,0.00979823984601585,
0.00991222916946492,0.0101402078163631,0.0103681864632612,0.0104251811249857,
0.0104821757867103,0.0105961651101593,0.0108241437570575,0.0109381330805065,
0.0110521224039556,0.0111661117274047,0.0112801010508537,0.0113940903743028,
0.0115080796977519,0.01173605834465,0.0118500476680991,0.0119640369915481,
0.0120780263149972,0.0121920156384463,0.0124199942853444,0.0126479729322425,
0.0127049675939671,0.0127619622556916,0.0128759515791407,0.0131039302260388,
0.0133319088729369,0.013445898196386,0.0135028928581105,0.0135598875198351,
0.0136738768432841,0.0137878661667332,0.0140158448136313,0.0141298341370804,
0.0142438234605295,0.0143578127839785,0.0144718021074276),.UNSPECIFIED.);
#957=B_SPLINE_SURFACE_WITH_KNOTS('',1,3,((#250704,#250705,#250706,#250707,
#250708,#250709,#250710,#250711,#250712,#250713,#250714,#250715,#250716,
#250717,#250718,#250719,#250720,#250721,#250722,#250723,#250724,#250725,
#250726,#250727,#250728,#250729,#250730,#250731,#250732,#250733,#250734,
#250735,#250736,#250737,#250738,#250739,#250740,#250741,#250742,#250743,
#250744,#250745,#250746,#250747,#250748,#250749,#250750,#250751,#250752,
#250753,#250754,#250755,#250756,#250757,#250758,#250759,#250760,#250761,
#250762,#250763,#250764,#250765,#250766,#250767,#250768,#250769,#250770,
#250771,#250772,#250773,#250774,#250775,#250776,#250777,#250778,#250779,
#250780,#250781,#250782,#250783,#250784,#250785,#250786,#250787,#250788,
#250789,#250790,#250791,#250792,#250793,#250794,#250795,#250796,#250797,
#250798,#250799,#250800,#250801,#250802,#250803,#250804,#250805,#250806,
#250807,#250808,#250809,#250810,#250811,#250812,#250813,#250814,#250815,
#250816,#250817,#250818,#250819,#250820,#250821,#250822,#250823,#250824,
#250825,#250826,#250827,#250828,#250829,#250830,#250831,#250832,#250833,
#250834,#250835,#250836,#250837,#250838,#250839,#250840,#250841,#250842,
#250843,#250844,#250845,#250846,#250847,#250848,#250849,#250850,#250851,
#250852,#250853,#250854,#250855,#250856,#250857,#250858,#250859,#250860,
#250861,#250862,#250863,#250864,#250865,#250866,#250867,#250868,#250869,
#250870,#250871,#250872,#250873,#250874,#250875,#250876,#250877,#250878,
#250879,#250880,#250881,#250882),(#250883,#250884,#250885,#250886,#250887,
#250888,#250889,#250890,#250891,#250892,#250893,#250894,#250895,#250896,
#250897,#250898,#250899,#250900,#250901,#250902,#250903,#250904,#250905,
#250906,#250907,#250908,#250909,#250910,#250911,#250912,#250913,#250914,
#250915,#250916,#250917,#250918,#250919,#250920,#250921,#250922,#250923,
#250924,#250925,#250926,#250927,#250928,#250929,#250930,#250931,#250932,
#250933,#250934,#250935,#250936,#250937,#250938,#250939,#250940,#250941,
#250942,#250943,#250944,#250945,#250946,#250947,#250948,#250949,#250950,
#250951,#250952,#250953,#250954,#250955,#250956,#250957,#250958,#250959,
#250960,#250961,#250962,#250963,#250964,#250965,#250966,#250967,#250968,
#250969,#250970,#250971,#250972,#250973,#250974,#250975,#250976,#250977,
#250978,#250979,#250980,#250981,#250982,#250983,#250984,#250985,#250986,
#250987,#250988,#250989,#250990,#250991,#250992,#250993,#250994,#250995,
#250996,#250997,#250998,#250999,#251000,#251001,#251002,#251003,#251004,
#251005,#251006,#251007,#251008,#251009,#251010,#251011,#251012,#251013,
#251014,#251015,#251016,#251017,#251018,#251019,#251020,#251021,#251022,
#251023,#251024,#251025,#251026,#251027,#251028,#251029,#251030,#251031,
#251032,#251033,#251034,#251035,#251036,#251037,#251038,#251039,#251040,
#251041,#251042,#251043,#251044,#251045,#251046,#251047,#251048,#251049,
#251050,#251051,#251052,#251053,#251054,#251055,#251056,#251057,#251058,
#251059,#251060,#251061)),.UNSPECIFIED.,.F.,.T.,.F.,(2,2),(4,1,1,2,2,2,
2,1,1,1,2,2,2,1,1,2,2,2,2,2,2,2,2,2,1,1,1,2,2,2,1,2,2,2,1,2,2,2,1,1,1,1,
2,2,2,1,1,1,1,2,2,2,2,2,2,2,1,1,2,2,2,2,1,2,2,2,1,1,2,2,2,2,2,2,2,2,2,2,
1,1,1,2,2,2,1,1,2,2,2,1,2,2,2,2,2,1,2,2,2,2,2,1,1,1,2,2,4),(0.,5.45368304321453),
(-0.000118831294053002,0.000109147352845132,0.000337125999743267,0.000451115323192334,
0.000565104646641402,0.000679093970090469,0.000793083293539536,0.00102106194043767,
0.00113505126388674,0.0012490405873358,0.00136302991078487,0.00142002457250941,
0.00147701923423394,0.00170499788113207,0.00193297652803021,0.00204696585147928,
0.00216095517492835,0.00227494449837741,0.00238893382182648,0.00261691246872462,
0.00284489111562275,0.00290188577734728,0.00295888043907182,0.00307286976252088,
0.00330084840941902,0.00341483773286809,0.00352882705631715,0.00364281637976622,
0.00375680570321528,0.00387079502666435,0.00398478435011342,0.00421276299701156,
0.00444074164390969,0.00466872029080782,0.00489669893770596,0.00512467758460409,
0.00518167224632863,0.00523866690805316,0.00535265623150223,0.0054666455549513,
0.00558063487840036,0.00569462420184943,0.0058086135252985,0.00592260284874756,
0.00603659217219663,0.0061505814956457,0.00626457081909477,0.0064925494659929,
0.00660653878944197,0.00672052811289104,0.0068345174363401,0.00694850675978917,
0.00717648540668731,0.00729047473013637,0.00740446405358544,0.00763244270048357,
0.00786042134738171,0.00797441067083078,0.00808839999427985,0.00820238931772891,
0.00831637864117798,0.00854435728807612,0.00877233593497425,0.00888632525842331,
0.00900031458187238,0.00911430390532145,0.00922829322877052,0.00945627187566865,
0.00957026119911772,0.00968425052256679,0.00974124518429132,0.00979823984601585,
0.00991222916946492,0.0101402078163631,0.0103681864632612,0.0104251811249857,
0.0104821757867103,0.0105961651101593,0.0108241437570575,0.0109381330805065,
0.0110521224039556,0.0111661117274047,0.0112801010508537,0.0113940903743028,
0.0115080796977519,0.01173605834465,0.0118500476680991,0.0119640369915481,
0.0120780263149972,0.0121920156384463,0.0124199942853444,0.0126479729322425,
0.0127049675939671,0.0127619622556916,0.0128759515791407,0.0131039302260388,
0.0133319088729369,0.013445898196386,0.0135028928581105,0.0135598875198351,
0.0136738768432841,0.0137878661667332,0.0140158448136313,0.0141298341370804,
0.0142438234605295,0.0143578127839785,0.0144718021074276),.UNSPECIFIED.);
#958=B_SPLINE_SURFACE_WITH_KNOTS('',1,3,((#251106,#251107,#251108,#251109,
#251110,#251111,#251112,#251113,#251114,#251115,#251116,#251117,#251118,
#251119,#251120,#251121,#251122,#251123,#251124,#251125,#251126,#251127,
#251128,#251129,#251130,#251131,#251132,#251133,#251134,#251135,#251136,
#251137,#251138,#251139,#251140,#251141,#251142,#251143,#251144,#251145,
#251146,#251147,#251148,#251149,#251150,#251151,#251152,#251153,#251154,
#251155,#251156,#251157,#251158,#251159,#251160,#251161,#251162,#251163,
#251164,#251165,#251166,#251167,#251168,#251169,#251170,#251171,#251172,
#251173,#251174,#251175,#251176,#251177,#251178,#251179,#251180,#251181,
#251182,#251183,#251184,#251185,#251186,#251187,#251188,#251189,#251190,
#251191,#251192,#251193,#251194,#251195,#251196,#251197,#251198,#251199,
#251200,#251201,#251202,#251203,#251204,#251205,#251206,#251207,#251208,
#251209,#251210,#251211,#251212,#251213,#251214,#251215,#251216,#251217,
#251218,#251219,#251220,#251221,#251222,#251223,#251224,#251225,#251226,
#251227,#251228,#251229,#251230,#251231,#251232,#251233,#251234,#251235,
#251236,#251237,#251238,#251239,#251240,#251241,#251242,#251243,#251244,
#251245,#251246,#251247,#251248,#251249,#251250,#251251,#251252,#251253,
#251254,#251255,#251256,#251257,#251258,#251259,#251260,#251261,#251262,
#251263,#251264,#251265,#251266,#251267,#251268,#251269,#251270,#251271,
#251272,#251273,#251274,#251275,#251276,#251277,#251278,#251279,#251280,
#251281,#251282,#251283,#251284),(#251285,#251286,#251287,#251288,#251289,
#251290,#251291,#251292,#251293,#251294,#251295,#251296,#251297,#251298,
#251299,#251300,#251301,#251302,#251303,#251304,#251305,#251306,#251307,
#251308,#251309,#251310,#251311,#251312,#251313,#251314,#251315,#251316,
#251317,#251318,#251319,#251320,#251321,#251322,#251323,#251324,#251325,
#251326,#251327,#251328,#251329,#251330,#251331,#251332,#251333,#251334,
#251335,#251336,#251337,#251338,#251339,#251340,#251341,#251342,#251343,
#251344,#251345,#251346,#251347,#251348,#251349,#251350,#251351,#251352,
#251353,#251354,#251355,#251356,#251357,#251358,#251359,#251360,#251361,
#251362,#251363,#251364,#251365,#251366,#251367,#251368,#251369,#251370,
#251371,#251372,#251373,#251374,#251375,#251376,#251377,#251378,#251379,
#251380,#251381,#251382,#251383,#251384,#251385,#251386,#251387,#251388,
#251389,#251390,#251391,#251392,#251393,#251394,#251395,#251396,#251397,
#251398,#251399,#251400,#251401,#251402,#251403,#251404,#251405,#251406,
#251407,#251408,#251409,#251410,#251411,#251412,#251413,#251414,#251415,
#251416,#251417,#251418,#251419,#251420,#251421,#251422,#251423,#251424,
#251425,#251426,#251427,#251428,#251429,#251430,#251431,#251432,#251433,
#251434,#251435,#251436,#251437,#251438,#251439,#251440,#251441,#251442,
#251443,#251444,#251445,#251446,#251447,#251448,#251449,#251450,#251451,
#251452,#251453,#251454,#251455,#251456,#251457,#251458,#251459,#251460,
#251461,#251462,#251463)),.UNSPECIFIED.,.F.,.T.,.F.,(2,2),(4,1,1,2,2,2,
2,1,1,1,2,2,2,1,1,2,2,2,2,2,2,2,2,2,1,1,1,2,2,2,1,2,2,2,1,2,2,2,1,1,1,1,
2,2,2,1,1,1,1,2,2,2,2,2,2,2,1,1,2,2,2,2,1,2,2,2,1,1,2,2,2,2,2,2,2,2,2,2,
1,1,1,2,2,2,1,1,2,2,2,1,2,2,2,2,2,1,2,2,2,2,2,1,1,1,2,2,4),(0.,5.45368304321453),
(-0.000118831294053002,0.000109147352845132,0.000337125999743267,0.000451115323192334,
0.000565104646641402,0.000679093970090469,0.000793083293539536,0.00102106194043767,
0.00113505126388674,0.0012490405873358,0.00136302991078487,0.00142002457250941,
0.00147701923423394,0.00170499788113207,0.00193297652803021,0.00204696585147928,
0.00216095517492835,0.00227494449837741,0.00238893382182648,0.00261691246872462,
0.00284489111562275,0.00290188577734728,0.00295888043907182,0.00307286976252088,
0.00330084840941902,0.00341483773286809,0.00352882705631715,0.00364281637976622,
0.00375680570321528,0.00387079502666435,0.00398478435011342,0.00421276299701156,
0.00444074164390969,0.00466872029080782,0.00489669893770596,0.00512467758460409,
0.00518167224632863,0.00523866690805316,0.00535265623150223,0.0054666455549513,
0.00558063487840036,0.00569462420184943,0.0058086135252985,0.00592260284874756,
0.00603659217219663,0.0061505814956457,0.00626457081909477,0.0064925494659929,
0.00660653878944197,0.00672052811289104,0.0068345174363401,0.00694850675978917,
0.00717648540668731,0.00729047473013637,0.00740446405358544,0.00763244270048357,
0.00786042134738171,0.00797441067083078,0.00808839999427985,0.00820238931772891,
0.00831637864117798,0.00854435728807612,0.00877233593497425,0.00888632525842331,
0.00900031458187238,0.00911430390532145,0.00922829322877052,0.00945627187566865,
0.00957026119911772,0.00968425052256679,0.00974124518429132,0.00979823984601585,
0.00991222916946492,0.0101402078163631,0.0103681864632612,0.0104251811249857,
0.0104821757867103,0.0105961651101593,0.0108241437570575,0.0109381330805065,
0.0110521224039556,0.0111661117274047,0.0112801010508537,0.0113940903743028,
0.0115080796977519,0.01173605834465,0.0118500476680991,0.0119640369915481,
0.0120780263149972,0.0121920156384463,0.0124199942853444,0.0126479729322425,
0.0127049675939671,0.0127619622556916,0.0128759515791407,0.0131039302260388,
0.0133319088729369,0.013445898196386,0.0135028928581105,0.0135598875198351,
0.0136738768432841,0.0137878661667332,0.0140158448136313,0.0141298341370804,
0.0142438234605295,0.0143578127839785,0.0144718021074276),.UNSPECIFIED.);
#959=B_SPLINE_SURFACE_WITH_KNOTS('',1,3,((#251561,#251562,#251563,#251564,
#251565,#251566,#251567,#251568,#251569,#251570,#251571,#251572,#251573,
#251574,#251575,#251576,#251577,#251578,#251579,#251580,#251581,#251582,
#251583,#251584,#251585,#251586,#251587,#251588,#251589,#251590,#251591,
#251592,#251593,#251594,#251595,#251596,#251597,#251598,#251599,#251600,
#251601,#251602,#251603,#251604,#251605,#251606,#251607,#251608,#251609,
#251610,#251611,#251612,#251613,#251614,#251615,#251616,#251617,#251618,
#251619,#251620,#251621,#251622,#251623,#251624,#251625,#251626,#251627,
#251628,#251629,#251630,#251631,#251632,#251633,#251634,#251635,#251636,
#251637,#251638,#251639,#251640,#251641,#251642,#251643,#251644,#251645,
#251646,#251647,#251648,#251649,#251650,#251651,#251652,#251653,#251654,
#251655,#251656,#251657,#251658,#251659,#251660,#251661,#251662,#251663,
#251664,#251665,#251666,#251667,#251668,#251669,#251670,#251671,#251672,
#251673,#251674,#251675,#251676,#251677,#251678,#251679,#251680,#251681,
#251682,#251683,#251684,#251685,#251686,#251687,#251688,#251689,#251690,
#251691,#251692,#251693,#251694,#251695,#251696,#251697,#251698,#251699,
#251700,#251701,#251702,#251703,#251704,#251705,#251706,#251707,#251708,
#251709,#251710,#251711,#251712,#251713,#251714,#251715,#251716,#251717,
#251718,#251719,#251720,#251721,#251722,#251723,#251724,#251725,#251726,
#251727,#251728,#251729,#251730,#251731,#251732,#251733,#251734,#251735,
#251736,#251737,#251738,#251739,#251740,#251741,#251742,#251743,#251744,
#251745,#251746,#251747,#251748,#251749,#251750,#251751,#251752,#251753,
#251754,#251755,#251756,#251757,#251758,#251759,#251760,#251761,#251762,
#251763,#251764,#251765,#251766,#251767,#251768,#251769,#251770,#251771,
#251772,#251773,#251774,#251775,#251776,#251777,#251778,#251779,#251780,
#251781,#251782,#251783,#251784,#251785,#251786),(#251787,#251788,#251789,
#251790,#251791,#251792,#251793,#251794,#251795,#251796,#251797,#251798,
#251799,#251800,#251801,#251802,#251803,#251804,#251805,#251806,#251807,
#251808,#251809,#251810,#251811,#251812,#251813,#251814,#251815,#251816,
#251817,#251818,#251819,#251820,#251821,#251822,#251823,#251824,#251825,
#251826,#251827,#251828,#251829,#251830,#251831,#251832,#251833,#251834,
#251835,#251836,#251837,#251838,#251839,#251840,#251841,#251842,#251843,
#251844,#251845,#251846,#251847,#251848,#251849,#251850,#251851,#251852,
#251853,#251854,#251855,#251856,#251857,#251858,#251859,#251860,#251861,
#251862,#251863,#251864,#251865,#251866,#251867,#251868,#251869,#251870,
#251871,#251872,#251873,#251874,#251875,#251876,#251877,#251878,#251879,
#251880,#251881,#251882,#251883,#251884,#251885,#251886,#251887,#251888,
#251889,#251890,#251891,#251892,#251893,#251894,#251895,#251896,#251897,
#251898,#251899,#251900,#251901,#251902,#251903,#251904,#251905,#251906,
#251907,#251908,#251909,#251910,#251911,#251912,#251913,#251914,#251915,
#251916,#251917,#251918,#251919,#251920,#251921,#251922,#251923,#251924,
#251925,#251926,#251927,#251928,#251929,#251930,#251931,#251932,#251933,
#251934,#251935,#251936,#251937,#251938,#251939,#251940,#251941,#251942,
#251943,#251944,#251945,#251946,#251947,#251948,#251949,#251950,#251951,
#251952,#251953,#251954,#251955,#251956,#251957,#251958,#251959,#251960,
#251961,#251962,#251963,#251964,#251965,#251966,#251967,#251968,#251969,
#251970,#251971,#251972,#251973,#251974,#251975,#251976,#251977,#251978,
#251979,#251980,#251981,#251982,#251983,#251984,#251985,#251986,#251987,
#251988,#251989,#251990,#251991,#251992,#251993,#251994,#251995,#251996,
#251997,#251998,#251999,#252000,#252001,#252002,#252003,#252004,#252005,
#252006,#252007,#252008,#252009,#252010,#252011,#252012)),.UNSPECIFIED.,
 .F.,.T.,.F.,(2,2),(4,2,2,2,2,2,2,2,2,2,2,2,2,2,2,2,2,2,2,2,2,2,2,2,2,2,
2,2,2,2,2,2,2,2,2,2,2,2,2,2,2,2,2,2,2,2,2,2,2,2,2,2,2,2,2,2,2,2,2,2,2,2,
2,2,2,2,2,2,2,2,2,2,2,2,2,2,2,2,2,2,2,2,2,2,2,2,2,2,2,2,2,2,2,2,2,2,2,2,
2,2,2,2,2,2,2,2,2,2,2,2,2,2,4),(-1.02033811129603E-7,1.00000163088848),
(-0.000118831294053002,-4.84197060393493E-6,0.000109147352845132,0.000337125999743267,
0.000451115323192334,0.000565104646641402,0.000679093970090469,0.000793083293539536,
0.00102106194043767,0.00113505126388674,0.0012490405873358,0.00136302991078487,
0.00142002457250941,0.00147701923423394,0.00170499788113207,0.00193297652803021,
0.00204696585147928,0.00216095517492835,0.00227494449837741,0.00238893382182648,
0.00261691246872462,0.00284489111562275,0.00290188577734728,0.00295888043907182,
0.00307286976252088,0.00318685908596995,0.00330084840941902,0.00341483773286809,
0.00352882705631715,0.00364281637976622,0.00375680570321528,0.00387079502666435,
0.00398478435011342,0.00421276299701156,0.00444074164390969,0.00466872029080782,
0.00489669893770596,0.00512467758460409,0.00518167224632863,0.00523866690805316,
0.00535265623150223,0.0054666455549513,0.00558063487840036,0.00569462420184943,
0.0058086135252985,0.00592260284874756,0.00603659217219663,0.0061505814956457,
0.00626457081909477,0.0064925494659929,0.00660653878944197,0.00672052811289104,
0.0068345174363401,0.00694850675978917,0.00706249608323824,0.00717648540668731,
0.00729047473013637,0.00740446405358544,0.00763244270048357,0.00786042134738171,
0.00797441067083078,0.00808839999427985,0.00820238931772891,0.00831637864117798,
0.00854435728807612,0.00865834661152518,0.00877233593497425,0.00888632525842331,
0.00900031458187238,0.00911430390532145,0.00922829322877052,0.00945627187566865,
0.00957026119911772,0.00968425052256679,0.00974124518429132,0.00979823984601585,
0.00991222916946492,0.0101402078163631,0.0103681864632612,0.0104251811249857,
0.0104821757867103,0.0105961651101593,0.0107101544336084,0.0108241437570575,
0.0109381330805065,0.0110521224039556,0.0111661117274047,0.0112801010508537,
0.0113940903743028,0.0115080796977519,0.01173605834465,0.0118500476680991,
0.0119640369915481,0.0120780263149972,0.0121920156384463,0.0124199942853444,
0.0126479729322425,0.0127049675939671,0.0127619622556916,0.0128759515791407,
0.0129899409025897,0.0131039302260388,0.0133319088729369,0.013445898196386,
0.0135028928581105,0.0135598875198351,0.0136738768432841,0.0137878661667332,
0.0140158448136313,0.0141298341370804,0.0142438234605295,0.0143578127839785,
0.0144718021074276),.UNSPECIFIED.);
#960=B_SPLINE_SURFACE_WITH_KNOTS('',1,3,((#254568,#254569,#254570,#254571,
#254572,#254573,#254574,#254575,#254576,#254577,#254578,#254579,#254580,
#254581,#254582,#254583,#254584,#254585,#254586,#254587,#254588,#254589,
#254590,#254591,#254592,#254593,#254594,#254595,#254596,#254597,#254598,
#254599,#254600,#254601,#254602,#254603,#254604,#254605,#254606,#254607,
#254608,#254609,#254610,#254611,#254612,#254613,#254614,#254615,#254616,
#254617,#254618,#254619,#254620,#254621,#254622,#254623,#254624,#254625,
#254626,#254627,#254628,#254629,#254630,#254631,#254632,#254633,#254634,
#254635,#254636,#254637,#254638,#254639,#254640,#254641,#254642,#254643,
#254644,#254645,#254646,#254647,#254648,#254649,#254650,#254651,#254652,
#254653,#254654,#254655,#254656,#254657,#254658,#254659,#254660,#254661,
#254662,#254663,#254664,#254665,#254666,#254667,#254668,#254669,#254670,
#254671,#254672,#254673,#254674,#254675,#254676,#254677,#254678,#254679,
#254680,#254681,#254682,#254683,#254684,#254685,#254686,#254687,#254688,
#254689,#254690,#254691,#254692,#254693,#254694,#254695,#254696,#254697,
#254698,#254699,#254700,#254701,#254702,#254703,#254704,#254705,#254706,
#254707,#254708,#254709,#254710,#254711,#254712,#254713,#254714,#254715,
#254716,#254717,#254718,#254719,#254720,#254721,#254722,#254723,#254724,
#254725,#254726,#254727,#254728,#254729,#254730,#254731,#254732,#254733,
#254734,#254735,#254736,#254737,#254738,#254739,#254740,#254741,#254742,
#254743,#254744,#254745,#254746),(#254747,#254748,#254749,#254750,#254751,
#254752,#254753,#254754,#254755,#254756,#254757,#254758,#254759,#254760,
#254761,#254762,#254763,#254764,#254765,#254766,#254767,#254768,#254769,
#254770,#254771,#254772,#254773,#254774,#254775,#254776,#254777,#254778,
#254779,#254780,#254781,#254782,#254783,#254784,#254785,#254786,#254787,
#254788,#254789,#254790,#254791,#254792,#254793,#254794,#254795,#254796,
#254797,#254798,#254799,#254800,#254801,#254802,#254803,#254804,#254805,
#254806,#254807,#254808,#254809,#254810,#254811,#254812,#254813,#254814,
#254815,#254816,#254817,#254818,#254819,#254820,#254821,#254822,#254823,
#254824,#254825,#254826,#254827,#254828,#254829,#254830,#254831,#254832,
#254833,#254834,#254835,#254836,#254837,#254838,#254839,#254840,#254841,
#254842,#254843,#254844,#254845,#254846,#254847,#254848,#254849,#254850,
#254851,#254852,#254853,#254854,#254855,#254856,#254857,#254858,#254859,
#254860,#254861,#254862,#254863,#254864,#254865,#254866,#254867,#254868,
#254869,#254870,#254871,#254872,#254873,#254874,#254875,#254876,#254877,
#254878,#254879,#254880,#254881,#254882,#254883,#254884,#254885,#254886,
#254887,#254888,#254889,#254890,#254891,#254892,#254893,#254894,#254895,
#254896,#254897,#254898,#254899,#254900,#254901,#254902,#254903,#254904,
#254905,#254906,#254907,#254908,#254909,#254910,#254911,#254912,#254913,
#254914,#254915,#254916,#254917,#254918,#254919,#254920,#254921,#254922,
#254923,#254924,#254925)),.UNSPECIFIED.,.F.,.T.,.F.,(2,2),(4,1,1,2,2,2,
2,1,1,1,2,2,2,1,1,2,2,2,2,2,2,2,2,2,1,1,1,2,2,2,1,2,2,2,1,2,2,2,1,1,1,1,
2,2,2,1,1,1,1,2,2,2,2,2,2,2,1,1,2,2,2,2,1,2,2,2,1,1,2,2,2,2,2,2,2,2,2,2,
1,1,1,2,2,2,1,1,2,2,2,1,2,2,2,2,2,1,2,2,2,2,2,1,1,1,2,2,4),(0.,4.74723717073224),
(-0.000118831294053002,0.000109147352845132,0.000337125999743267,0.000451115323192334,
0.000565104646641402,0.000679093970090469,0.000793083293539536,0.00102106194043767,
0.00113505126388674,0.0012490405873358,0.00136302991078487,0.00142002457250941,
0.00147701923423394,0.00170499788113207,0.00193297652803021,0.00204696585147928,
0.00216095517492835,0.00227494449837741,0.00238893382182648,0.00261691246872462,
0.00284489111562275,0.00290188577734728,0.00295888043907182,0.00307286976252088,
0.00330084840941902,0.00341483773286809,0.00352882705631715,0.00364281637976622,
0.00375680570321528,0.00387079502666435,0.00398478435011342,0.00421276299701156,
0.00444074164390969,0.00466872029080782,0.00489669893770596,0.00512467758460409,
0.00518167224632863,0.00523866690805316,0.00535265623150223,0.0054666455549513,
0.00558063487840036,0.00569462420184943,0.0058086135252985,0.00592260284874756,
0.00603659217219663,0.0061505814956457,0.00626457081909477,0.0064925494659929,
0.00660653878944197,0.00672052811289104,0.0068345174363401,0.00694850675978917,
0.00717648540668731,0.00729047473013637,0.00740446405358544,0.00763244270048357,
0.00786042134738171,0.00797441067083078,0.00808839999427985,0.00820238931772891,
0.00831637864117798,0.00854435728807612,0.00877233593497425,0.00888632525842331,
0.00900031458187238,0.00911430390532145,0.00922829322877052,0.00945627187566865,
0.00957026119911772,0.00968425052256679,0.00974124518429132,0.00979823984601585,
0.00991222916946492,0.0101402078163631,0.0103681864632612,0.0104251811249857,
0.0104821757867103,0.0105961651101593,0.0108241437570575,0.0109381330805065,
0.0110521224039556,0.0111661117274047,0.0112801010508537,0.0113940903743028,
0.0115080796977519,0.01173605834465,0.0118500476680991,0.0119640369915481,
0.0120780263149972,0.0121920156384463,0.0124199942853444,0.0126479729322425,
0.0127049675939671,0.0127619622556916,0.0128759515791407,0.0131039302260388,
0.0133319088729369,0.013445898196386,0.0135028928581105,0.0135598875198351,
0.0136738768432841,0.0137878661667332,0.0140158448136313,0.0141298341370804,
0.0142438234605295,0.0143578127839785,0.0144718021074276),.UNSPECIFIED.);
#961=B_SPLINE_SURFACE_WITH_KNOTS('',1,3,((#254948,#254949,#254950,#254951,
#254952,#254953,#254954,#254955,#254956,#254957,#254958,#254959,#254960,
#254961,#254962,#254963,#254964,#254965,#254966,#254967,#254968,#254969,
#254970,#254971,#254972,#254973,#254974,#254975,#254976,#254977,#254978,
#254979,#254980,#254981,#254982,#254983,#254984,#254985,#254986,#254987,
#254988,#254989,#254990,#254991,#254992,#254993,#254994,#254995,#254996,
#254997,#254998,#254999,#255000,#255001,#255002,#255003,#255004,#255005,
#255006,#255007,#255008,#255009,#255010,#255011,#255012,#255013,#255014,
#255015,#255016,#255017,#255018,#255019,#255020,#255021,#255022,#255023,
#255024,#255025,#255026,#255027,#255028,#255029,#255030,#255031,#255032,
#255033,#255034,#255035,#255036,#255037,#255038,#255039,#255040,#255041,
#255042,#255043,#255044,#255045,#255046,#255047,#255048,#255049,#255050,
#255051,#255052,#255053,#255054,#255055,#255056,#255057,#255058,#255059,
#255060,#255061,#255062,#255063,#255064,#255065,#255066,#255067,#255068,
#255069,#255070,#255071,#255072,#255073,#255074,#255075,#255076,#255077,
#255078,#255079,#255080,#255081,#255082,#255083,#255084,#255085,#255086,
#255087,#255088,#255089,#255090,#255091,#255092,#255093,#255094,#255095,
#255096,#255097,#255098,#255099,#255100,#255101,#255102,#255103,#255104,
#255105,#255106,#255107,#255108,#255109,#255110,#255111,#255112,#255113,
#255114,#255115,#255116,#255117,#255118,#255119,#255120,#255121,#255122,
#255123,#255124,#255125,#255126),(#255127,#255128,#255129,#255130,#255131,
#255132,#255133,#255134,#255135,#255136,#255137,#255138,#255139,#255140,
#255141,#255142,#255143,#255144,#255145,#255146,#255147,#255148,#255149,
#255150,#255151,#255152,#255153,#255154,#255155,#255156,#255157,#255158,
#255159,#255160,#255161,#255162,#255163,#255164,#255165,#255166,#255167,
#255168,#255169,#255170,#255171,#255172,#255173,#255174,#255175,#255176,
#255177,#255178,#255179,#255180,#255181,#255182,#255183,#255184,#255185,
#255186,#255187,#255188,#255189,#255190,#255191,#255192,#255193,#255194,
#255195,#255196,#255197,#255198,#255199,#255200,#255201,#255202,#255203,
#255204,#255205,#255206,#255207,#255208,#255209,#255210,#255211,#255212,
#255213,#255214,#255215,#255216,#255217,#255218,#255219,#255220,#255221,
#255222,#255223,#255224,#255225,#255226,#255227,#255228,#255229,#255230,
#255231,#255232,#255233,#255234,#255235,#255236,#255237,#255238,#255239,
#255240,#255241,#255242,#255243,#255244,#255245,#255246,#255247,#255248,
#255249,#255250,#255251,#255252,#255253,#255254,#255255,#255256,#255257,
#255258,#255259,#255260,#255261,#255262,#255263,#255264,#255265,#255266,
#255267,#255268,#255269,#255270,#255271,#255272,#255273,#255274,#255275,
#255276,#255277,#255278,#255279,#255280,#255281,#255282,#255283,#255284,
#255285,#255286,#255287,#255288,#255289,#255290,#255291,#255292,#255293,
#255294,#255295,#255296,#255297,#255298,#255299,#255300,#255301,#255302,
#255303,#255304,#255305)),.UNSPECIFIED.,.F.,.T.,.F.,(2,2),(4,1,1,2,2,2,
2,1,1,1,2,2,2,1,1,2,2,2,2,2,2,2,2,2,1,1,1,2,2,2,1,2,2,2,1,2,2,2,1,1,1,1,
2,2,2,1,1,1,1,2,2,2,2,2,2,2,1,1,2,2,2,2,1,2,2,2,1,1,2,2,2,2,2,2,2,2,2,2,
1,1,1,2,2,2,1,1,2,2,2,1,2,2,2,2,2,1,2,2,2,2,2,1,1,1,2,2,4),(0.,4.74723717073224),
(-0.000118831294053002,0.000109147352845132,0.000337125999743267,0.000451115323192334,
0.000565104646641402,0.000679093970090469,0.000793083293539536,0.00102106194043767,
0.00113505126388674,0.0012490405873358,0.00136302991078487,0.00142002457250941,
0.00147701923423394,0.00170499788113207,0.00193297652803021,0.00204696585147928,
0.00216095517492835,0.00227494449837741,0.00238893382182648,0.00261691246872462,
0.00284489111562275,0.00290188577734728,0.00295888043907182,0.00307286976252088,
0.00330084840941902,0.00341483773286809,0.00352882705631715,0.00364281637976622,
0.00375680570321528,0.00387079502666435,0.00398478435011342,0.00421276299701156,
0.00444074164390969,0.00466872029080782,0.00489669893770596,0.00512467758460409,
0.00518167224632863,0.00523866690805316,0.00535265623150223,0.0054666455549513,
0.00558063487840036,0.00569462420184943,0.0058086135252985,0.00592260284874756,
0.00603659217219663,0.0061505814956457,0.00626457081909477,0.0064925494659929,
0.00660653878944197,0.00672052811289104,0.0068345174363401,0.00694850675978917,
0.00717648540668731,0.00729047473013637,0.00740446405358544,0.00763244270048357,
0.00786042134738171,0.00797441067083078,0.00808839999427985,0.00820238931772891,
0.00831637864117798,0.00854435728807612,0.00877233593497425,0.00888632525842331,
0.00900031458187238,0.00911430390532145,0.00922829322877052,0.00945627187566865,
0.00957026119911772,0.00968425052256679,0.00974124518429132,0.00979823984601585,
0.00991222916946492,0.0101402078163631,0.0103681864632612,0.0104251811249857,
0.0104821757867103,0.0105961651101593,0.0108241437570575,0.0109381330805065,
0.0110521224039556,0.0111661117274047,0.0112801010508537,0.0113940903743028,
0.0115080796977519,0.01173605834465,0.0118500476680991,0.0119640369915481,
0.0120780263149972,0.0121920156384463,0.0124199942853444,0.0126479729322425,
0.0127049675939671,0.0127619622556916,0.0128759515791407,0.0131039302260388,
0.0133319088729369,0.013445898196386,0.0135028928581105,0.0135598875198351,
0.0136738768432841,0.0137878661667332,0.0140158448136313,0.0141298341370804,
0.0142438234605295,0.0143578127839785,0.0144718021074276),.UNSPECIFIED.);
#962=B_SPLINE_SURFACE_WITH_KNOTS('',1,3,((#255358,#255359,#255360,#255361,
#255362,#255363,#255364,#255365,#255366,#255367,#255368,#255369,#255370,
#255371,#255372,#255373,#255374,#255375,#255376,#255377,#255378,#255379,
#255380,#255381,#255382,#255383,#255384,#255385,#255386,#255387,#255388,
#255389,#255390,#255391,#255392,#255393,#255394,#255395,#255396,#255397,
#255398,#255399,#255400,#255401,#255402,#255403,#255404,#255405,#255406,
#255407,#255408,#255409,#255410,#255411,#255412,#255413,#255414,#255415,
#255416,#255417,#255418,#255419,#255420,#255421,#255422,#255423,#255424,
#255425,#255426,#255427,#255428,#255429,#255430,#255431,#255432,#255433,
#255434,#255435,#255436,#255437,#255438,#255439,#255440,#255441,#255442,
#255443,#255444,#255445,#255446,#255447,#255448,#255449,#255450,#255451,
#255452,#255453,#255454,#255455,#255456,#255457,#255458,#255459,#255460,
#255461,#255462,#255463,#255464,#255465,#255466,#255467,#255468,#255469,
#255470,#255471,#255472,#255473,#255474,#255475,#255476,#255477,#255478,
#255479,#255480,#255481,#255482,#255483,#255484,#255485,#255486,#255487,
#255488,#255489,#255490,#255491,#255492,#255493,#255494,#255495,#255496,
#255497,#255498,#255499,#255500,#255501,#255502,#255503,#255504,#255505,
#255506,#255507,#255508,#255509,#255510,#255511,#255512,#255513,#255514,
#255515,#255516,#255517,#255518,#255519,#255520,#255521,#255522,#255523,
#255524,#255525,#255526,#255527,#255528,#255529,#255530,#255531,#255532,
#255533,#255534,#255535,#255536),(#255537,#255538,#255539,#255540,#255541,
#255542,#255543,#255544,#255545,#255546,#255547,#255548,#255549,#255550,
#255551,#255552,#255553,#255554,#255555,#255556,#255557,#255558,#255559,
#255560,#255561,#255562,#255563,#255564,#255565,#255566,#255567,#255568,
#255569,#255570,#255571,#255572,#255573,#255574,#255575,#255576,#255577,
#255578,#255579,#255580,#255581,#255582,#255583,#255584,#255585,#255586,
#255587,#255588,#255589,#255590,#255591,#255592,#255593,#255594,#255595,
#255596,#255597,#255598,#255599,#255600,#255601,#255602,#255603,#255604,
#255605,#255606,#255607,#255608,#255609,#255610,#255611,#255612,#255613,
#255614,#255615,#255616,#255617,#255618,#255619,#255620,#255621,#255622,
#255623,#255624,#255625,#255626,#255627,#255628,#255629,#255630,#255631,
#255632,#255633,#255634,#255635,#255636,#255637,#255638,#255639,#255640,
#255641,#255642,#255643,#255644,#255645,#255646,#255647,#255648,#255649,
#255650,#255651,#255652,#255653,#255654,#255655,#255656,#255657,#255658,
#255659,#255660,#255661,#255662,#255663,#255664,#255665,#255666,#255667,
#255668,#255669,#255670,#255671,#255672,#255673,#255674,#255675,#255676,
#255677,#255678,#255679,#255680,#255681,#255682,#255683,#255684,#255685,
#255686,#255687,#255688,#255689,#255690,#255691,#255692,#255693,#255694,
#255695,#255696,#255697,#255698,#255699,#255700,#255701,#255702,#255703,
#255704,#255705,#255706,#255707,#255708,#255709,#255710,#255711,#255712,
#255713,#255714,#255715)),.UNSPECIFIED.,.F.,.T.,.F.,(2,2),(4,1,1,2,2,2,
2,1,1,1,2,2,2,1,1,2,2,2,2,2,2,2,2,2,1,1,1,2,2,2,1,2,2,2,1,2,2,2,1,1,1,1,
2,2,2,1,1,1,1,2,2,2,2,2,2,2,1,1,2,2,2,2,1,2,2,2,1,1,2,2,2,2,2,2,2,2,2,2,
1,1,1,2,2,2,1,1,2,2,2,1,2,2,2,2,2,1,2,2,2,2,2,1,1,1,2,2,4),(0.,4.74723717073224),
(-0.000118831294053002,0.000109147352845132,0.000337125999743267,0.000451115323192334,
0.000565104646641402,0.000679093970090469,0.000793083293539536,0.00102106194043767,
0.00113505126388674,0.0012490405873358,0.00136302991078487,0.00142002457250941,
0.00147701923423394,0.00170499788113207,0.00193297652803021,0.00204696585147928,
0.00216095517492835,0.00227494449837741,0.00238893382182648,0.00261691246872462,
0.00284489111562275,0.00290188577734728,0.00295888043907182,0.00307286976252088,
0.00330084840941902,0.00341483773286809,0.00352882705631715,0.00364281637976622,
0.00375680570321528,0.00387079502666435,0.00398478435011342,0.00421276299701156,
0.00444074164390969,0.00466872029080782,0.00489669893770596,0.00512467758460409,
0.00518167224632863,0.00523866690805316,0.00535265623150223,0.0054666455549513,
0.00558063487840036,0.00569462420184943,0.0058086135252985,0.00592260284874756,
0.00603659217219663,0.0061505814956457,0.00626457081909477,0.0064925494659929,
0.00660653878944197,0.00672052811289104,0.0068345174363401,0.00694850675978917,
0.00717648540668731,0.00729047473013637,0.00740446405358544,0.00763244270048357,
0.00786042134738171,0.00797441067083078,0.00808839999427985,0.00820238931772891,
0.00831637864117798,0.00854435728807612,0.00877233593497425,0.00888632525842331,
0.00900031458187238,0.00911430390532145,0.00922829322877052,0.00945627187566865,
0.00957026119911772,0.00968425052256679,0.00974124518429132,0.00979823984601585,
0.00991222916946492,0.0101402078163631,0.0103681864632612,0.0104251811249857,
0.0104821757867103,0.0105961651101593,0.0108241437570575,0.0109381330805065,
0.0110521224039556,0.0111661117274047,0.0112801010508537,0.0113940903743028,
0.0115080796977519,0.01173605834465,0.0118500476680991,0.0119640369915481,
0.0120780263149972,0.0121920156384463,0.0124199942853444,0.0126479729322425,
0.0127049675939671,0.0127619622556916,0.0128759515791407,0.0131039302260388,
0.0133319088729369,0.013445898196386,0.0135028928581105,0.0135598875198351,
0.0136738768432841,0.0137878661667332,0.0140158448136313,0.0141298341370804,
0.0142438234605295,0.0143578127839785,0.0144718021074276),.UNSPECIFIED.);
#963=B_SPLINE_SURFACE_WITH_KNOTS('',1,3,((#255726,#255727,#255728,#255729,
#255730,#255731,#255732,#255733,#255734,#255735,#255736,#255737,#255738,
#255739,#255740,#255741,#255742,#255743,#255744,#255745,#255746,#255747,
#255748,#255749,#255750,#255751,#255752,#255753,#255754,#255755,#255756,
#255757,#255758,#255759,#255760,#255761,#255762,#255763,#255764,#255765,
#255766,#255767,#255768,#255769,#255770,#255771,#255772,#255773,#255774,
#255775,#255776,#255777,#255778,#255779,#255780,#255781,#255782,#255783,
#255784,#255785,#255786,#255787,#255788,#255789,#255790,#255791,#255792,
#255793,#255794,#255795,#255796,#255797,#255798,#255799,#255800,#255801,
#255802,#255803,#255804,#255805,#255806,#255807,#255808,#255809,#255810,
#255811,#255812,#255813,#255814,#255815,#255816,#255817,#255818,#255819,
#255820,#255821,#255822,#255823,#255824,#255825,#255826,#255827,#255828,
#255829,#255830,#255831,#255832,#255833,#255834,#255835,#255836,#255837,
#255838,#255839,#255840,#255841),(#255842,#255843,#255844,#255845,#255846,
#255847,#255848,#255849,#255850,#255851,#255852,#255853,#255854,#255855,
#255856,#255857,#255858,#255859,#255860,#255861,#255862,#255863,#255864,
#255865,#255866,#255867,#255868,#255869,#255870,#255871,#255872,#255873,
#255874,#255875,#255876,#255877,#255878,#255879,#255880,#255881,#255882,
#255883,#255884,#255885,#255886,#255887,#255888,#255889,#255890,#255891,
#255892,#255893,#255894,#255895,#255896,#255897,#255898,#255899,#255900,
#255901,#255902,#255903,#255904,#255905,#255906,#255907,#255908,#255909,
#255910,#255911,#255912,#255913,#255914,#255915,#255916,#255917,#255918,
#255919,#255920,#255921,#255922,#255923,#255924,#255925,#255926,#255927,
#255928,#255929,#255930,#255931,#255932,#255933,#255934,#255935,#255936,
#255937,#255938,#255939,#255940,#255941,#255942,#255943,#255944,#255945,
#255946,#255947,#255948,#255949,#255950,#255951,#255952,#255953,#255954,
#255955,#255956,#255957)),.UNSPECIFIED.,.F.,.F.,.F.,(2,2),(4,2,2,2,2,2,
2,2,2,2,2,2,2,2,2,2,2,2,2,2,2,2,2,2,2,2,2,2,2,2,2,2,2,2,2,2,2,2,2,2,2,2,
2,2,2,2,2,2,2,2,2,2,2,2,2,2,2,4),(0.,1.00000324318157),(0.00717648540668731,
0.00729047473013637,0.00740446405358544,0.00763244270048357,0.00786042134738171,
0.00797441067083078,0.00808839999427985,0.00820238931772891,0.00831637864117798,
0.00854435728807612,0.00865834661152518,0.00877233593497425,0.00888632525842331,
0.00900031458187238,0.00911430390532145,0.00922829322877052,0.00945627187566865,
0.00957026119911772,0.00968425052256679,0.00974124518429132,0.00979823984601585,
0.00991222916946492,0.0101402078163631,0.0103681864632612,0.0104251811249857,
0.0104821757867103,0.0105961651101593,0.0107101544336084,0.0108241437570575,
0.0109381330805065,0.0110521224039556,0.0111661117274047,0.0112801010508537,
0.0113940903743028,0.0115080796977519,0.01173605834465,0.0118500476680991,
0.0119640369915481,0.0120780263149972,0.0121920156384463,0.0124199942853444,
0.0126479729322425,0.0127049675939671,0.0127619622556916,0.0128759515791407,
0.0129899409025897,0.0131039302260388,0.0133319088729369,0.013445898196386,
0.0135028928581105,0.0135598875198351,0.0136738768432841,0.0137878661667332,
0.0140158448136313,0.0141298341370804,0.0142438234605295,0.0143578127839785,
0.0144718021074276),.UNSPECIFIED.);
#964=B_SPLINE_SURFACE_WITH_KNOTS('',1,3,((#258767,#258768,#258769,#258770,
#258771,#258772,#258773,#258774,#258775,#258776,#258777,#258778,#258779,
#258780,#258781,#258782,#258783,#258784,#258785,#258786,#258787,#258788,
#258789,#258790,#258791,#258792,#258793,#258794,#258795,#258796,#258797,
#258798,#258799,#258800,#258801,#258802,#258803,#258804,#258805,#258806,
#258807,#258808,#258809,#258810,#258811,#258812,#258813,#258814,#258815,
#258816,#258817,#258818,#258819,#258820,#258821,#258822,#258823,#258824,
#258825,#258826,#258827,#258828,#258829,#258830,#258831,#258832,#258833,
#258834,#258835,#258836,#258837,#258838,#258839,#258840,#258841,#258842,
#258843,#258844,#258845,#258846,#258847,#258848,#258849,#258850,#258851,
#258852,#258853,#258854,#258855,#258856,#258857,#258858,#258859,#258860,
#258861,#258862,#258863,#258864,#258865,#258866,#258867,#258868,#258869,
#258870,#258871,#258872,#258873,#258874,#258875,#258876,#258877,#258878,
#258879,#258880,#258881,#258882,#258883,#258884,#258885,#258886,#258887,
#258888,#258889,#258890,#258891,#258892,#258893,#258894,#258895,#258896,
#258897,#258898,#258899,#258900,#258901,#258902,#258903,#258904,#258905,
#258906,#258907,#258908,#258909,#258910,#258911,#258912,#258913,#258914,
#258915,#258916,#258917,#258918,#258919,#258920,#258921,#258922,#258923,
#258924,#258925,#258926,#258927,#258928,#258929,#258930,#258931,#258932,
#258933,#258934,#258935,#258936,#258937,#258938,#258939,#258940,#258941),
(#258942,#258943,#258944,#258945,#258946,#258947,#258948,#258949,#258950,
#258951,#258952,#258953,#258954,#258955,#258956,#258957,#258958,#258959,
#258960,#258961,#258962,#258963,#258964,#258965,#258966,#258967,#258968,
#258969,#258970,#258971,#258972,#258973,#258974,#258975,#258976,#258977,
#258978,#258979,#258980,#258981,#258982,#258983,#258984,#258985,#258986,
#258987,#258988,#258989,#258990,#258991,#258992,#258993,#258994,#258995,
#258996,#258997,#258998,#258999,#259000,#259001,#259002,#259003,#259004,
#259005,#259006,#259007,#259008,#259009,#259010,#259011,#259012,#259013,
#259014,#259015,#259016,#259017,#259018,#259019,#259020,#259021,#259022,
#259023,#259024,#259025,#259026,#259027,#259028,#259029,#259030,#259031,
#259032,#259033,#259034,#259035,#259036,#259037,#259038,#259039,#259040,
#259041,#259042,#259043,#259044,#259045,#259046,#259047,#259048,#259049,
#259050,#259051,#259052,#259053,#259054,#259055,#259056,#259057,#259058,
#259059,#259060,#259061,#259062,#259063,#259064,#259065,#259066,#259067,
#259068,#259069,#259070,#259071,#259072,#259073,#259074,#259075,#259076,
#259077,#259078,#259079,#259080,#259081,#259082,#259083,#259084,#259085,
#259086,#259087,#259088,#259089,#259090,#259091,#259092,#259093,#259094,
#259095,#259096,#259097,#259098,#259099,#259100,#259101,#259102,#259103,
#259104,#259105,#259106,#259107,#259108,#259109,#259110,#259111,#259112,
#259113,#259114,#259115,#259116)),.UNSPECIFIED.,.F.,.T.,.F.,(2,2),(4,1,
1,2,1,1,1,1,2,2,1,2,2,2,2,1,1,2,2,2,1,1,1,1,2,2,2,2,2,2,2,2,1,1,1,2,2,2,
2,1,1,1,2,2,2,1,1,1,2,2,2,2,2,2,2,1,2,2,2,2,2,1,1,2,2,2,2,1,2,2,2,1,1,2,
2,2,1,1,1,1,2,2,2,2,2,2,2,1,2,1,1,2,2,2,1,2,2,2,2,2,1,2,2,2,2,4),(0.,4.71475608888856),
(-0.000135430429350568,9.25560474171526E-5,0.000320542524184873,0.000548529000952593,
0.000776515477720314,0.00100450195448803,0.00111849519287189,0.00123248843125575,
0.00134648166963961,0.00146047490802347,0.0016884613847912,0.00191644786155891,
0.00203044109994277,0.00214443433832664,0.00225842757671049,0.00237242081509435,
0.00260040729186208,0.00271440053024594,0.0028283937686298,0.00294238700701366,
0.00305638024539752,0.00317037348378138,0.00328436672216524,0.0033983599605491,
0.00351235319893296,0.00362634643731682,0.00374033967570068,0.0039683261524684,
0.00419631262923612,0.00431030586761998,0.00436730248681191,0.00442429910600384,
0.0045382923443877,0.00465228558277156,0.00488027205953928,0.00499426529792314,
0.005108258536307,0.00522225177469086,0.00533624501307472,0.00556423148984244,
0.0056782247282263,0.00579221796661016,0.00590621120499402,0.00602020444337788,
0.00613419768176174,0.0062481909201456,0.00647617739691333,0.00659017063529719,
0.00670416387368105,0.00681815711206491,0.00693215035044876,0.00716013682721649,
0.00727413006560035,0.00738812330398421,0.00761610978075193,0.00784409625751965,
0.00795808949590351,0.00807208273428737,0.0081290793534793,0.00818607597267123,
0.00830006921105509,0.00852805568782281,0.00864204892620667,0.00875604216459053,
0.00887003540297439,0.00898402864135825,0.00921201511812597,0.00944000159489369,
0.00955399483327755,0.00966798807166141,0.00978198131004527,0.00989597454842913,
0.0101239610251968,0.0102379542635807,0.0103519475019646,0.0104659407403484,
0.0105799339787323,0.0106939272171161,0.0108079204555,0.0109219136938839,
0.0110359069322677,0.0111499001706516,0.0112638934090355,0.0114918798858032,
0.0117198663625709,0.0118338596009548,0.0118908562201467,0.0119478528393386,
0.0120618460777225,0.0121758393161063,0.0124038257928741,0.0125178190312579,
0.0126318122696418,0.0127458055080256,0.0129737919847934,0.0130877852231772,
0.0133157716999449,0.0134297649383288,0.0134867615575207,0.0135437581767127,
0.0137717446534804,0.0139997311302481,0.0142277176070158,0.0142847142262077,
0.0143417108453997,0.0144557040837835),.UNSPECIFIED.);
#965=B_SPLINE_SURFACE_WITH_KNOTS('',1,3,((#259139,#259140,#259141,#259142,
#259143,#259144,#259145,#259146,#259147,#259148,#259149,#259150,#259151,
#259152,#259153,#259154,#259155,#259156,#259157,#259158,#259159,#259160,
#259161,#259162,#259163,#259164,#259165,#259166,#259167,#259168,#259169,
#259170,#259171,#259172,#259173,#259174,#259175,#259176,#259177,#259178,
#259179,#259180,#259181,#259182,#259183,#259184,#259185,#259186,#259187,
#259188,#259189,#259190,#259191,#259192,#259193,#259194,#259195,#259196,
#259197,#259198,#259199,#259200,#259201,#259202,#259203,#259204,#259205,
#259206,#259207,#259208,#259209,#259210,#259211,#259212,#259213,#259214,
#259215,#259216,#259217,#259218,#259219,#259220,#259221,#259222,#259223,
#259224,#259225,#259226,#259227,#259228,#259229,#259230,#259231,#259232,
#259233,#259234,#259235,#259236,#259237,#259238,#259239,#259240,#259241,
#259242,#259243,#259244,#259245,#259246,#259247,#259248,#259249,#259250,
#259251,#259252,#259253,#259254,#259255,#259256,#259257,#259258,#259259,
#259260,#259261,#259262,#259263,#259264,#259265,#259266,#259267,#259268,
#259269,#259270,#259271,#259272,#259273,#259274,#259275,#259276,#259277,
#259278,#259279,#259280,#259281,#259282,#259283,#259284,#259285,#259286,
#259287,#259288,#259289,#259290,#259291,#259292,#259293,#259294,#259295,
#259296,#259297,#259298,#259299,#259300,#259301,#259302,#259303,#259304,
#259305,#259306,#259307,#259308,#259309,#259310,#259311,#259312,#259313),
(#259314,#259315,#259316,#259317,#259318,#259319,#259320,#259321,#259322,
#259323,#259324,#259325,#259326,#259327,#259328,#259329,#259330,#259331,
#259332,#259333,#259334,#259335,#259336,#259337,#259338,#259339,#259340,
#259341,#259342,#259343,#259344,#259345,#259346,#259347,#259348,#259349,
#259350,#259351,#259352,#259353,#259354,#259355,#259356,#259357,#259358,
#259359,#259360,#259361,#259362,#259363,#259364,#259365,#259366,#259367,
#259368,#259369,#259370,#259371,#259372,#259373,#259374,#259375,#259376,
#259377,#259378,#259379,#259380,#259381,#259382,#259383,#259384,#259385,
#259386,#259387,#259388,#259389,#259390,#259391,#259392,#259393,#259394,
#259395,#259396,#259397,#259398,#259399,#259400,#259401,#259402,#259403,
#259404,#259405,#259406,#259407,#259408,#259409,#259410,#259411,#259412,
#259413,#259414,#259415,#259416,#259417,#259418,#259419,#259420,#259421,
#259422,#259423,#259424,#259425,#259426,#259427,#259428,#259429,#259430,
#259431,#259432,#259433,#259434,#259435,#259436,#259437,#259438,#259439,
#259440,#259441,#259442,#259443,#259444,#259445,#259446,#259447,#259448,
#259449,#259450,#259451,#259452,#259453,#259454,#259455,#259456,#259457,
#259458,#259459,#259460,#259461,#259462,#259463,#259464,#259465,#259466,
#259467,#259468,#259469,#259470,#259471,#259472,#259473,#259474,#259475,
#259476,#259477,#259478,#259479,#259480,#259481,#259482,#259483,#259484,
#259485,#259486,#259487,#259488)),.UNSPECIFIED.,.F.,.T.,.F.,(2,2),(4,1,
1,2,1,1,1,1,2,2,1,2,2,2,2,1,1,2,2,2,1,1,1,1,2,2,2,2,2,2,2,2,1,1,1,2,2,2,
2,1,1,1,2,2,2,1,1,1,2,2,2,2,2,2,2,1,2,2,2,2,2,1,1,2,2,2,2,1,2,2,2,1,1,2,
2,2,1,1,1,1,2,2,2,2,2,2,2,1,2,1,1,2,2,2,1,2,2,2,2,2,1,2,2,2,2,4),(0.,4.71475608888856),
(-0.000135430429350568,9.25560474171526E-5,0.000320542524184873,0.000548529000952593,
0.000776515477720314,0.00100450195448803,0.00111849519287189,0.00123248843125575,
0.00134648166963961,0.00146047490802347,0.0016884613847912,0.00191644786155891,
0.00203044109994277,0.00214443433832664,0.00225842757671049,0.00237242081509435,
0.00260040729186208,0.00271440053024594,0.0028283937686298,0.00294238700701366,
0.00305638024539752,0.00317037348378138,0.00328436672216524,0.0033983599605491,
0.00351235319893296,0.00362634643731682,0.00374033967570068,0.0039683261524684,
0.00419631262923612,0.00431030586761998,0.00436730248681191,0.00442429910600384,
0.0045382923443877,0.00465228558277156,0.00488027205953928,0.00499426529792314,
0.005108258536307,0.00522225177469086,0.00533624501307472,0.00556423148984244,
0.0056782247282263,0.00579221796661016,0.00590621120499402,0.00602020444337788,
0.00613419768176174,0.0062481909201456,0.00647617739691333,0.00659017063529719,
0.00670416387368105,0.00681815711206491,0.00693215035044876,0.00716013682721649,
0.00727413006560035,0.00738812330398421,0.00761610978075193,0.00784409625751965,
0.00795808949590351,0.00807208273428737,0.0081290793534793,0.00818607597267123,
0.00830006921105509,0.00852805568782281,0.00864204892620667,0.00875604216459053,
0.00887003540297439,0.00898402864135825,0.00921201511812597,0.00944000159489369,
0.00955399483327755,0.00966798807166141,0.00978198131004527,0.00989597454842913,
0.0101239610251968,0.0102379542635807,0.0103519475019646,0.0104659407403484,
0.0105799339787323,0.0106939272171161,0.0108079204555,0.0109219136938839,
0.0110359069322677,0.0111499001706516,0.0112638934090355,0.0114918798858032,
0.0117198663625709,0.0118338596009548,0.0118908562201467,0.0119478528393386,
0.0120618460777225,0.0121758393161063,0.0124038257928741,0.0125178190312579,
0.0126318122696418,0.0127458055080256,0.0129737919847934,0.0130877852231772,
0.0133157716999449,0.0134297649383288,0.0134867615575207,0.0135437581767127,
0.0137717446534804,0.0139997311302481,0.0142277176070158,0.0142847142262077,
0.0143417108453997,0.0144557040837835),.UNSPECIFIED.);
#966=B_SPLINE_SURFACE_WITH_KNOTS('',1,3,((#259536,#259537,#259538,#259539,
#259540,#259541,#259542,#259543,#259544,#259545,#259546,#259547,#259548,
#259549,#259550,#259551,#259552,#259553,#259554,#259555,#259556,#259557,
#259558,#259559,#259560,#259561,#259562,#259563,#259564,#259565,#259566,
#259567,#259568,#259569,#259570,#259571,#259572,#259573,#259574,#259575,
#259576,#259577,#259578,#259579,#259580,#259581,#259582,#259583,#259584,
#259585,#259586,#259587,#259588,#259589,#259590,#259591,#259592,#259593,
#259594,#259595,#259596,#259597,#259598,#259599,#259600,#259601,#259602,
#259603,#259604,#259605,#259606,#259607,#259608,#259609,#259610,#259611,
#259612,#259613,#259614,#259615,#259616,#259617,#259618,#259619,#259620,
#259621,#259622,#259623,#259624,#259625,#259626,#259627,#259628,#259629,
#259630,#259631,#259632,#259633,#259634,#259635,#259636,#259637,#259638,
#259639,#259640,#259641,#259642,#259643,#259644,#259645,#259646,#259647,
#259648,#259649,#259650,#259651,#259652,#259653,#259654,#259655,#259656,
#259657,#259658,#259659,#259660,#259661,#259662,#259663,#259664,#259665,
#259666,#259667,#259668,#259669,#259670,#259671,#259672,#259673,#259674,
#259675,#259676,#259677,#259678,#259679,#259680,#259681,#259682,#259683,
#259684,#259685,#259686,#259687,#259688,#259689,#259690,#259691,#259692,
#259693,#259694,#259695,#259696,#259697,#259698,#259699,#259700,#259701,
#259702,#259703,#259704,#259705,#259706,#259707,#259708,#259709,#259710),
(#259711,#259712,#259713,#259714,#259715,#259716,#259717,#259718,#259719,
#259720,#259721,#259722,#259723,#259724,#259725,#259726,#259727,#259728,
#259729,#259730,#259731,#259732,#259733,#259734,#259735,#259736,#259737,
#259738,#259739,#259740,#259741,#259742,#259743,#259744,#259745,#259746,
#259747,#259748,#259749,#259750,#259751,#259752,#259753,#259754,#259755,
#259756,#259757,#259758,#259759,#259760,#259761,#259762,#259763,#259764,
#259765,#259766,#259767,#259768,#259769,#259770,#259771,#259772,#259773,
#259774,#259775,#259776,#259777,#259778,#259779,#259780,#259781,#259782,
#259783,#259784,#259785,#259786,#259787,#259788,#259789,#259790,#259791,
#259792,#259793,#259794,#259795,#259796,#259797,#259798,#259799,#259800,
#259801,#259802,#259803,#259804,#259805,#259806,#259807,#259808,#259809,
#259810,#259811,#259812,#259813,#259814,#259815,#259816,#259817,#259818,
#259819,#259820,#259821,#259822,#259823,#259824,#259825,#259826,#259827,
#259828,#259829,#259830,#259831,#259832,#259833,#259834,#259835,#259836,
#259837,#259838,#259839,#259840,#259841,#259842,#259843,#259844,#259845,
#259846,#259847,#259848,#259849,#259850,#259851,#259852,#259853,#259854,
#259855,#259856,#259857,#259858,#259859,#259860,#259861,#259862,#259863,
#259864,#259865,#259866,#259867,#259868,#259869,#259870,#259871,#259872,
#259873,#259874,#259875,#259876,#259877,#259878,#259879,#259880,#259881,
#259882,#259883,#259884,#259885)),.UNSPECIFIED.,.F.,.T.,.F.,(2,2),(4,1,
1,2,1,1,1,1,2,2,1,2,2,2,2,1,1,2,2,2,1,1,1,1,2,2,2,2,2,2,2,2,1,1,1,2,2,2,
2,1,1,1,2,2,2,1,1,1,2,2,2,2,2,2,2,1,2,2,2,2,2,1,1,2,2,2,2,1,2,2,2,1,1,2,
2,2,1,1,1,1,2,2,2,2,2,2,2,1,2,1,1,2,2,2,1,2,2,2,2,2,1,2,2,2,2,4),(0.,4.71475608888856),
(-0.000135430429350568,9.25560474171526E-5,0.000320542524184873,0.000548529000952593,
0.000776515477720314,0.00100450195448803,0.00111849519287189,0.00123248843125575,
0.00134648166963961,0.00146047490802347,0.0016884613847912,0.00191644786155891,
0.00203044109994277,0.00214443433832664,0.00225842757671049,0.00237242081509435,
0.00260040729186208,0.00271440053024594,0.0028283937686298,0.00294238700701366,
0.00305638024539752,0.00317037348378138,0.00328436672216524,0.0033983599605491,
0.00351235319893296,0.00362634643731682,0.00374033967570068,0.0039683261524684,
0.00419631262923612,0.00431030586761998,0.00436730248681191,0.00442429910600384,
0.0045382923443877,0.00465228558277156,0.00488027205953928,0.00499426529792314,
0.005108258536307,0.00522225177469086,0.00533624501307472,0.00556423148984244,
0.0056782247282263,0.00579221796661016,0.00590621120499402,0.00602020444337788,
0.00613419768176174,0.0062481909201456,0.00647617739691333,0.00659017063529719,
0.00670416387368105,0.00681815711206491,0.00693215035044876,0.00716013682721649,
0.00727413006560035,0.00738812330398421,0.00761610978075193,0.00784409625751965,
0.00795808949590351,0.00807208273428737,0.0081290793534793,0.00818607597267123,
0.00830006921105509,0.00852805568782281,0.00864204892620667,0.00875604216459053,
0.00887003540297439,0.00898402864135825,0.00921201511812597,0.00944000159489369,
0.00955399483327755,0.00966798807166141,0.00978198131004527,0.00989597454842913,
0.0101239610251968,0.0102379542635807,0.0103519475019646,0.0104659407403484,
0.0105799339787323,0.0106939272171161,0.0108079204555,0.0109219136938839,
0.0110359069322677,0.0111499001706516,0.0112638934090355,0.0114918798858032,
0.0117198663625709,0.0118338596009548,0.0118908562201467,0.0119478528393386,
0.0120618460777225,0.0121758393161063,0.0124038257928741,0.0125178190312579,
0.0126318122696418,0.0127458055080256,0.0129737919847934,0.0130877852231772,
0.0133157716999449,0.0134297649383288,0.0134867615575207,0.0135437581767127,
0.0137717446534804,0.0139997311302481,0.0142277176070158,0.0142847142262077,
0.0143417108453997,0.0144557040837835),.UNSPECIFIED.);
#967=B_SPLINE_SURFACE_WITH_KNOTS('',1,3,((#259896,#259897,#259898,#259899,
#259900,#259901,#259902,#259903,#259904,#259905,#259906,#259907,#259908,
#259909,#259910,#259911,#259912,#259913,#259914,#259915,#259916,#259917,
#259918,#259919,#259920,#259921,#259922,#259923,#259924,#259925,#259926,
#259927,#259928,#259929,#259930,#259931,#259932,#259933,#259934,#259935,
#259936,#259937,#259938,#259939,#259940,#259941,#259942,#259943,#259944,
#259945,#259946,#259947,#259948,#259949,#259950,#259951,#259952,#259953,
#259954,#259955,#259956,#259957,#259958,#259959,#259960,#259961,#259962,
#259963,#259964,#259965,#259966,#259967,#259968,#259969,#259970,#259971,
#259972,#259973,#259974,#259975,#259976,#259977,#259978,#259979,#259980,
#259981,#259982,#259983,#259984,#259985,#259986,#259987,#259988,#259989,
#259990,#259991,#259992,#259993,#259994,#259995,#259996,#259997,#259998,
#259999,#260000,#260001,#260002,#260003,#260004,#260005,#260006,#260007,
#260008,#260009),(#260010,#260011,#260012,#260013,#260014,#260015,#260016,
#260017,#260018,#260019,#260020,#260021,#260022,#260023,#260024,#260025,
#260026,#260027,#260028,#260029,#260030,#260031,#260032,#260033,#260034,
#260035,#260036,#260037,#260038,#260039,#260040,#260041,#260042,#260043,
#260044,#260045,#260046,#260047,#260048,#260049,#260050,#260051,#260052,
#260053,#260054,#260055,#260056,#260057,#260058,#260059,#260060,#260061,
#260062,#260063,#260064,#260065,#260066,#260067,#260068,#260069,#260070,
#260071,#260072,#260073,#260074,#260075,#260076,#260077,#260078,#260079,
#260080,#260081,#260082,#260083,#260084,#260085,#260086,#260087,#260088,
#260089,#260090,#260091,#260092,#260093,#260094,#260095,#260096,#260097,
#260098,#260099,#260100,#260101,#260102,#260103,#260104,#260105,#260106,
#260107,#260108,#260109,#260110,#260111,#260112,#260113,#260114,#260115,
#260116,#260117,#260118,#260119,#260120,#260121,#260122,#260123)),
 .UNSPECIFIED.,.F.,.F.,.F.,(2,2),(4,2,2,2,2,2,2,2,2,2,2,2,2,2,2,2,2,2,2,
2,2,2,2,2,2,2,2,2,2,2,2,2,2,2,2,2,2,2,2,2,2,2,2,2,2,2,2,2,2,2,2,2,2,2,2,
2,4),(0.,1.00000135803625),(0.00716013682721649,0.00727413006560035,0.00738812330398421,
0.00761610978075193,0.00784409625751965,0.00795808949590351,0.00807208273428737,
0.0081290793534793,0.00818607597267123,0.00830006921105509,0.00852805568782281,
0.00864204892620667,0.00875604216459053,0.00887003540297439,0.00898402864135825,
0.00921201511812597,0.00944000159489369,0.00955399483327755,0.00966798807166141,
0.00978198131004527,0.00989597454842913,0.0101239610251968,0.0102379542635807,
0.0103519475019646,0.0104659407403484,0.0105799339787323,0.0106939272171161,
0.0108079204555,0.0109219136938839,0.0110359069322677,0.0111499001706516,
0.0112638934090355,0.0114918798858032,0.0117198663625709,0.0118338596009548,
0.0118908562201467,0.0119478528393386,0.0120618460777225,0.0121758393161063,
0.0124038257928741,0.0125178190312579,0.0126318122696418,0.0127458055080256,
0.0128597987464095,0.0129737919847934,0.0130877852231772,0.0133157716999449,
0.0134297649383288,0.0134867615575207,0.0135437581767127,0.0136577514150965,
0.0137717446534804,0.0139997311302481,0.0142277176070158,0.0142847142262077,
0.0143417108453997,0.0144557040837835),.UNSPECIFIED.);
#968=B_SPLINE_SURFACE_WITH_KNOTS('',1,3,((#262733,#262734,#262735,#262736,
#262737,#262738,#262739,#262740,#262741,#262742,#262743,#262744,#262745,
#262746,#262747,#262748,#262749,#262750,#262751,#262752,#262753,#262754,
#262755,#262756,#262757,#262758,#262759,#262760,#262761,#262762,#262763,
#262764,#262765,#262766,#262767,#262768,#262769,#262770,#262771,#262772,
#262773,#262774,#262775,#262776,#262777,#262778,#262779,#262780,#262781,
#262782,#262783,#262784,#262785,#262786,#262787,#262788,#262789,#262790,
#262791,#262792,#262793,#262794,#262795,#262796,#262797,#262798,#262799,
#262800,#262801,#262802,#262803,#262804,#262805,#262806,#262807,#262808,
#262809,#262810,#262811,#262812,#262813,#262814,#262815,#262816,#262817,
#262818,#262819,#262820,#262821,#262822,#262823,#262824,#262825,#262826,
#262827,#262828,#262829,#262830,#262831,#262832,#262833,#262834,#262835,
#262836,#262837,#262838,#262839,#262840,#262841,#262842,#262843,#262844,
#262845,#262846,#262847,#262848,#262849,#262850,#262851,#262852,#262853,
#262854,#262855,#262856,#262857,#262858,#262859,#262860,#262861,#262862,
#262863,#262864,#262865,#262866,#262867,#262868,#262869,#262870,#262871,
#262872,#262873,#262874,#262875,#262876,#262877,#262878,#262879,#262880,
#262881,#262882,#262883,#262884,#262885,#262886,#262887,#262888,#262889,
#262890,#262891,#262892,#262893,#262894,#262895,#262896,#262897,#262898,
#262899,#262900,#262901,#262902,#262903,#262904,#262905,#262906,#262907),
(#262908,#262909,#262910,#262911,#262912,#262913,#262914,#262915,#262916,
#262917,#262918,#262919,#262920,#262921,#262922,#262923,#262924,#262925,
#262926,#262927,#262928,#262929,#262930,#262931,#262932,#262933,#262934,
#262935,#262936,#262937,#262938,#262939,#262940,#262941,#262942,#262943,
#262944,#262945,#262946,#262947,#262948,#262949,#262950,#262951,#262952,
#262953,#262954,#262955,#262956,#262957,#262958,#262959,#262960,#262961,
#262962,#262963,#262964,#262965,#262966,#262967,#262968,#262969,#262970,
#262971,#262972,#262973,#262974,#262975,#262976,#262977,#262978,#262979,
#262980,#262981,#262982,#262983,#262984,#262985,#262986,#262987,#262988,
#262989,#262990,#262991,#262992,#262993,#262994,#262995,#262996,#262997,
#262998,#262999,#263000,#263001,#263002,#263003,#263004,#263005,#263006,
#263007,#263008,#263009,#263010,#263011,#263012,#263013,#263014,#263015,
#263016,#263017,#263018,#263019,#263020,#263021,#263022,#263023,#263024,
#263025,#263026,#263027,#263028,#263029,#263030,#263031,#263032,#263033,
#263034,#263035,#263036,#263037,#263038,#263039,#263040,#263041,#263042,
#263043,#263044,#263045,#263046,#263047,#263048,#263049,#263050,#263051,
#263052,#263053,#263054,#263055,#263056,#263057,#263058,#263059,#263060,
#263061,#263062,#263063,#263064,#263065,#263066,#263067,#263068,#263069,
#263070,#263071,#263072,#263073,#263074,#263075,#263076,#263077,#263078,
#263079,#263080,#263081,#263082)),.UNSPECIFIED.,.F.,.T.,.F.,(2,2),(4,1,
1,2,1,1,1,1,2,2,1,2,2,2,2,1,1,2,2,2,1,1,1,1,2,2,2,2,2,2,2,2,1,1,1,2,2,2,
2,1,1,1,2,2,2,1,1,1,2,2,2,2,2,2,2,1,2,2,2,2,2,1,1,2,2,2,2,1,2,2,2,1,1,2,
2,2,1,1,1,1,2,2,2,2,2,2,2,1,2,1,1,2,2,2,1,2,2,2,2,2,1,2,2,2,2,4),(0.,5.46382276754873),
(-0.000135430429350568,9.25560474171526E-5,0.000320542524184873,0.000548529000952593,
0.000776515477720314,0.00100450195448803,0.00111849519287189,0.00123248843125575,
0.00134648166963961,0.00146047490802347,0.0016884613847912,0.00191644786155891,
0.00203044109994277,0.00214443433832664,0.00225842757671049,0.00237242081509435,
0.00260040729186208,0.00271440053024594,0.0028283937686298,0.00294238700701366,
0.00305638024539752,0.00317037348378138,0.00328436672216524,0.0033983599605491,
0.00351235319893296,0.00362634643731682,0.00374033967570068,0.0039683261524684,
0.00419631262923612,0.00431030586761998,0.00436730248681191,0.00442429910600384,
0.0045382923443877,0.00465228558277156,0.00488027205953928,0.00499426529792314,
0.005108258536307,0.00522225177469086,0.00533624501307472,0.00556423148984244,
0.0056782247282263,0.00579221796661016,0.00590621120499402,0.00602020444337788,
0.00613419768176174,0.0062481909201456,0.00647617739691333,0.00659017063529719,
0.00670416387368105,0.00681815711206491,0.00693215035044876,0.00716013682721649,
0.00727413006560035,0.00738812330398421,0.00761610978075193,0.00784409625751965,
0.00795808949590351,0.00807208273428737,0.0081290793534793,0.00818607597267123,
0.00830006921105509,0.00852805568782281,0.00864204892620667,0.00875604216459053,
0.00887003540297439,0.00898402864135825,0.00921201511812597,0.00944000159489369,
0.00955399483327755,0.00966798807166141,0.00978198131004527,0.00989597454842913,
0.0101239610251968,0.0102379542635807,0.0103519475019646,0.0104659407403484,
0.0105799339787323,0.0106939272171161,0.0108079204555,0.0109219136938839,
0.0110359069322677,0.0111499001706516,0.0112638934090355,0.0114918798858032,
0.0117198663625709,0.0118338596009548,0.0118908562201467,0.0119478528393386,
0.0120618460777225,0.0121758393161063,0.0124038257928741,0.0125178190312579,
0.0126318122696418,0.0127458055080256,0.0129737919847934,0.0130877852231772,
0.0133157716999449,0.0134297649383288,0.0134867615575207,0.0135437581767127,
0.0137717446534804,0.0139997311302481,0.0142277176070158,0.0142847142262077,
0.0143417108453997,0.0144557040837835),.UNSPECIFIED.);
#969=B_SPLINE_SURFACE_WITH_KNOTS('',1,3,((#263107,#263108,#263109,#263110,
#263111,#263112,#263113,#263114,#263115,#263116,#263117,#263118,#263119,
#263120,#263121,#263122,#263123,#263124,#263125,#263126,#263127,#263128,
#263129,#263130,#263131,#263132,#263133,#263134,#263135,#263136,#263137,
#263138,#263139,#263140,#263141,#263142,#263143,#263144,#263145,#263146,
#263147,#263148,#263149,#263150,#263151,#263152,#263153,#263154,#263155,
#263156,#263157,#263158,#263159,#263160,#263161,#263162,#263163,#263164,
#263165,#263166,#263167,#263168,#263169,#263170,#263171,#263172,#263173,
#263174,#263175,#263176,#263177,#263178,#263179,#263180,#263181,#263182,
#263183,#263184,#263185,#263186,#263187,#263188,#263189,#263190,#263191,
#263192,#263193,#263194,#263195,#263196,#263197,#263198,#263199,#263200,
#263201,#263202,#263203,#263204,#263205,#263206,#263207,#263208,#263209,
#263210,#263211,#263212,#263213,#263214,#263215,#263216,#263217,#263218,
#263219,#263220,#263221,#263222,#263223,#263224,#263225,#263226,#263227,
#263228,#263229,#263230,#263231,#263232,#263233,#263234,#263235,#263236,
#263237,#263238,#263239,#263240,#263241,#263242,#263243,#263244,#263245,
#263246,#263247,#263248,#263249,#263250,#263251,#263252,#263253,#263254,
#263255,#263256,#263257,#263258,#263259,#263260,#263261,#263262,#263263,
#263264,#263265,#263266,#263267,#263268,#263269,#263270,#263271,#263272,
#263273,#263274,#263275,#263276,#263277,#263278,#263279,#263280,#263281),
(#263282,#263283,#263284,#263285,#263286,#263287,#263288,#263289,#263290,
#263291,#263292,#263293,#263294,#263295,#263296,#263297,#263298,#263299,
#263300,#263301,#263302,#263303,#263304,#263305,#263306,#263307,#263308,
#263309,#263310,#263311,#263312,#263313,#263314,#263315,#263316,#263317,
#263318,#263319,#263320,#263321,#263322,#263323,#263324,#263325,#263326,
#263327,#263328,#263329,#263330,#263331,#263332,#263333,#263334,#263335,
#263336,#263337,#263338,#263339,#263340,#263341,#263342,#263343,#263344,
#263345,#263346,#263347,#263348,#263349,#263350,#263351,#263352,#263353,
#263354,#263355,#263356,#263357,#263358,#263359,#263360,#263361,#263362,
#263363,#263364,#263365,#263366,#263367,#263368,#263369,#263370,#263371,
#263372,#263373,#263374,#263375,#263376,#263377,#263378,#263379,#263380,
#263381,#263382,#263383,#263384,#263385,#263386,#263387,#263388,#263389,
#263390,#263391,#263392,#263393,#263394,#263395,#263396,#263397,#263398,
#263399,#263400,#263401,#263402,#263403,#263404,#263405,#263406,#263407,
#263408,#263409,#263410,#263411,#263412,#263413,#263414,#263415,#263416,
#263417,#263418,#263419,#263420,#263421,#263422,#263423,#263424,#263425,
#263426,#263427,#263428,#263429,#263430,#263431,#263432,#263433,#263434,
#263435,#263436,#263437,#263438,#263439,#263440,#263441,#263442,#263443,
#263444,#263445,#263446,#263447,#263448,#263449,#263450,#263451,#263452,
#263453,#263454,#263455,#263456)),.UNSPECIFIED.,.F.,.T.,.F.,(2,2),(4,1,
1,2,1,1,1,1,2,2,1,2,2,2,2,1,1,2,2,2,1,1,1,1,2,2,2,2,2,2,2,2,1,1,1,2,2,2,
2,1,1,1,2,2,2,1,1,1,2,2,2,2,2,2,2,1,2,2,2,2,2,1,1,2,2,2,2,1,2,2,2,1,1,2,
2,2,1,1,1,1,2,2,2,2,2,2,2,1,2,1,1,2,2,2,1,2,2,2,2,2,1,2,2,2,2,4),(0.,5.46382276754873),
(-0.000135430429350568,9.25560474171526E-5,0.000320542524184873,0.000548529000952593,
0.000776515477720314,0.00100450195448803,0.00111849519287189,0.00123248843125575,
0.00134648166963961,0.00146047490802347,0.0016884613847912,0.00191644786155891,
0.00203044109994277,0.00214443433832664,0.00225842757671049,0.00237242081509435,
0.00260040729186208,0.00271440053024594,0.0028283937686298,0.00294238700701366,
0.00305638024539752,0.00317037348378138,0.00328436672216524,0.0033983599605491,
0.00351235319893296,0.00362634643731682,0.00374033967570068,0.0039683261524684,
0.00419631262923612,0.00431030586761998,0.00436730248681191,0.00442429910600384,
0.0045382923443877,0.00465228558277156,0.00488027205953928,0.00499426529792314,
0.005108258536307,0.00522225177469086,0.00533624501307472,0.00556423148984244,
0.0056782247282263,0.00579221796661016,0.00590621120499402,0.00602020444337788,
0.00613419768176174,0.0062481909201456,0.00647617739691333,0.00659017063529719,
0.00670416387368105,0.00681815711206491,0.00693215035044876,0.00716013682721649,
0.00727413006560035,0.00738812330398421,0.00761610978075193,0.00784409625751965,
0.00795808949590351,0.00807208273428737,0.0081290793534793,0.00818607597267123,
0.00830006921105509,0.00852805568782281,0.00864204892620667,0.00875604216459053,
0.00887003540297439,0.00898402864135825,0.00921201511812597,0.00944000159489369,
0.00955399483327755,0.00966798807166141,0.00978198131004527,0.00989597454842913,
0.0101239610251968,0.0102379542635807,0.0103519475019646,0.0104659407403484,
0.0105799339787323,0.0106939272171161,0.0108079204555,0.0109219136938839,
0.0110359069322677,0.0111499001706516,0.0112638934090355,0.0114918798858032,
0.0117198663625709,0.0118338596009548,0.0118908562201467,0.0119478528393386,
0.0120618460777225,0.0121758393161063,0.0124038257928741,0.0125178190312579,
0.0126318122696418,0.0127458055080256,0.0129737919847934,0.0130877852231772,
0.0133157716999449,0.0134297649383288,0.0134867615575207,0.0135437581767127,
0.0137717446534804,0.0139997311302481,0.0142277176070158,0.0142847142262077,
0.0143417108453997,0.0144557040837835),.UNSPECIFIED.);
#970=B_SPLINE_SURFACE_WITH_KNOTS('',1,3,((#263501,#263502,#263503,#263504,
#263505,#263506,#263507,#263508,#263509,#263510,#263511,#263512,#263513,
#263514,#263515,#263516,#263517,#263518,#263519,#263520,#263521,#263522,
#263523,#263524,#263525,#263526,#263527,#263528,#263529,#263530,#263531,
#263532,#263533,#263534,#263535,#263536,#263537,#263538,#263539,#263540,
#263541,#263542,#263543,#263544,#263545,#263546,#263547,#263548,#263549,
#263550,#263551,#263552,#263553,#263554,#263555,#263556,#263557,#263558,
#263559,#263560,#263561,#263562,#263563,#263564,#263565,#263566,#263567,
#263568,#263569,#263570,#263571,#263572,#263573,#263574,#263575,#263576,
#263577,#263578,#263579,#263580,#263581,#263582,#263583,#263584,#263585,
#263586,#263587,#263588,#263589,#263590,#263591,#263592,#263593,#263594,
#263595,#263596,#263597,#263598,#263599,#263600,#263601,#263602,#263603,
#263604,#263605,#263606,#263607,#263608,#263609,#263610,#263611,#263612,
#263613,#263614,#263615,#263616,#263617,#263618,#263619,#263620,#263621,
#263622,#263623,#263624,#263625,#263626,#263627,#263628,#263629,#263630,
#263631,#263632,#263633,#263634,#263635,#263636,#263637,#263638,#263639,
#263640,#263641,#263642,#263643,#263644,#263645,#263646,#263647,#263648,
#263649,#263650,#263651,#263652,#263653,#263654,#263655,#263656,#263657,
#263658,#263659,#263660,#263661,#263662,#263663,#263664,#263665,#263666,
#263667,#263668,#263669,#263670,#263671,#263672,#263673,#263674,#263675),
(#263676,#263677,#263678,#263679,#263680,#263681,#263682,#263683,#263684,
#263685,#263686,#263687,#263688,#263689,#263690,#263691,#263692,#263693,
#263694,#263695,#263696,#263697,#263698,#263699,#263700,#263701,#263702,
#263703,#263704,#263705,#263706,#263707,#263708,#263709,#263710,#263711,
#263712,#263713,#263714,#263715,#263716,#263717,#263718,#263719,#263720,
#263721,#263722,#263723,#263724,#263725,#263726,#263727,#263728,#263729,
#263730,#263731,#263732,#263733,#263734,#263735,#263736,#263737,#263738,
#263739,#263740,#263741,#263742,#263743,#263744,#263745,#263746,#263747,
#263748,#263749,#263750,#263751,#263752,#263753,#263754,#263755,#263756,
#263757,#263758,#263759,#263760,#263761,#263762,#263763,#263764,#263765,
#263766,#263767,#263768,#263769,#263770,#263771,#263772,#263773,#263774,
#263775,#263776,#263777,#263778,#263779,#263780,#263781,#263782,#263783,
#263784,#263785,#263786,#263787,#263788,#263789,#263790,#263791,#263792,
#263793,#263794,#263795,#263796,#263797,#263798,#263799,#263800,#263801,
#263802,#263803,#263804,#263805,#263806,#263807,#263808,#263809,#263810,
#263811,#263812,#263813,#263814,#263815,#263816,#263817,#263818,#263819,
#263820,#263821,#263822,#263823,#263824,#263825,#263826,#263827,#263828,
#263829,#263830,#263831,#263832,#263833,#263834,#263835,#263836,#263837,
#263838,#263839,#263840,#263841,#263842,#263843,#263844,#263845,#263846,
#263847,#263848,#263849,#263850)),.UNSPECIFIED.,.F.,.T.,.F.,(2,2),(4,1,
1,2,1,1,1,1,2,2,1,2,2,2,2,1,1,2,2,2,1,1,1,1,2,2,2,2,2,2,2,2,1,1,1,2,2,2,
2,1,1,1,2,2,2,1,1,1,2,2,2,2,2,2,2,1,2,2,2,2,2,1,1,2,2,2,2,1,2,2,2,1,1,2,
2,2,1,1,1,1,2,2,2,2,2,2,2,1,2,1,1,2,2,2,1,2,2,2,2,2,1,2,2,2,2,4),(0.,5.46382276754873),
(-0.000135430429350568,9.25560474171526E-5,0.000320542524184873,0.000548529000952593,
0.000776515477720314,0.00100450195448803,0.00111849519287189,0.00123248843125575,
0.00134648166963961,0.00146047490802347,0.0016884613847912,0.00191644786155891,
0.00203044109994277,0.00214443433832664,0.00225842757671049,0.00237242081509435,
0.00260040729186208,0.00271440053024594,0.0028283937686298,0.00294238700701366,
0.00305638024539752,0.00317037348378138,0.00328436672216524,0.0033983599605491,
0.00351235319893296,0.00362634643731682,0.00374033967570068,0.0039683261524684,
0.00419631262923612,0.00431030586761998,0.00436730248681191,0.00442429910600384,
0.0045382923443877,0.00465228558277156,0.00488027205953928,0.00499426529792314,
0.005108258536307,0.00522225177469086,0.00533624501307472,0.00556423148984244,
0.0056782247282263,0.00579221796661016,0.00590621120499402,0.00602020444337788,
0.00613419768176174,0.0062481909201456,0.00647617739691333,0.00659017063529719,
0.00670416387368105,0.00681815711206491,0.00693215035044876,0.00716013682721649,
0.00727413006560035,0.00738812330398421,0.00761610978075193,0.00784409625751965,
0.00795808949590351,0.00807208273428737,0.0081290793534793,0.00818607597267123,
0.00830006921105509,0.00852805568782281,0.00864204892620667,0.00875604216459053,
0.00887003540297439,0.00898402864135825,0.00921201511812597,0.00944000159489369,
0.00955399483327755,0.00966798807166141,0.00978198131004527,0.00989597454842913,
0.0101239610251968,0.0102379542635807,0.0103519475019646,0.0104659407403484,
0.0105799339787323,0.0106939272171161,0.0108079204555,0.0109219136938839,
0.0110359069322677,0.0111499001706516,0.0112638934090355,0.0114918798858032,
0.0117198663625709,0.0118338596009548,0.0118908562201467,0.0119478528393386,
0.0120618460777225,0.0121758393161063,0.0124038257928741,0.0125178190312579,
0.0126318122696418,0.0127458055080256,0.0129737919847934,0.0130877852231772,
0.0133157716999449,0.0134297649383288,0.0134867615575207,0.0135437581767127,
0.0137717446534804,0.0139997311302481,0.0142277176070158,0.0142847142262077,
0.0143417108453997,0.0144557040837835),.UNSPECIFIED.);
#971=B_SPLINE_SURFACE_WITH_KNOTS('',1,3,((#263926,#263927,#263928,#263929,
#263930,#263931,#263932,#263933,#263934,#263935,#263936,#263937,#263938,
#263939,#263940,#263941,#263942,#263943,#263944,#263945,#263946,#263947,
#263948,#263949,#263950,#263951,#263952,#263953,#263954,#263955,#263956,
#263957,#263958,#263959,#263960,#263961,#263962,#263963,#263964,#263965,
#263966,#263967,#263968,#263969,#263970,#263971,#263972,#263973,#263974,
#263975,#263976,#263977,#263978,#263979,#263980,#263981,#263982,#263983,
#263984,#263985,#263986,#263987,#263988,#263989,#263990,#263991,#263992,
#263993,#263994,#263995,#263996,#263997,#263998,#263999,#264000,#264001,
#264002,#264003,#264004,#264005,#264006,#264007,#264008,#264009,#264010,
#264011,#264012,#264013,#264014,#264015,#264016,#264017,#264018,#264019,
#264020,#264021,#264022,#264023,#264024,#264025,#264026,#264027,#264028,
#264029,#264030,#264031,#264032,#264033,#264034,#264035,#264036,#264037,
#264038,#264039,#264040,#264041,#264042,#264043,#264044,#264045,#264046,
#264047,#264048,#264049,#264050,#264051,#264052,#264053,#264054,#264055,
#264056,#264057,#264058,#264059,#264060,#264061,#264062,#264063,#264064,
#264065,#264066,#264067,#264068,#264069,#264070,#264071,#264072,#264073,
#264074,#264075,#264076,#264077,#264078,#264079,#264080,#264081,#264082,
#264083,#264084,#264085,#264086,#264087,#264088,#264089,#264090,#264091,
#264092,#264093,#264094,#264095,#264096,#264097,#264098,#264099,#264100,
#264101,#264102,#264103,#264104,#264105,#264106,#264107,#264108,#264109,
#264110,#264111,#264112,#264113,#264114,#264115,#264116,#264117,#264118,
#264119,#264120,#264121,#264122,#264123,#264124,#264125,#264126,#264127,
#264128,#264129,#264130,#264131,#264132,#264133,#264134,#264135,#264136,
#264137,#264138,#264139,#264140,#264141,#264142,#264143,#264144,#264145,
#264146,#264147,#264148,#264149),(#264150,#264151,#264152,#264153,#264154,
#264155,#264156,#264157,#264158,#264159,#264160,#264161,#264162,#264163,
#264164,#264165,#264166,#264167,#264168,#264169,#264170,#264171,#264172,
#264173,#264174,#264175,#264176,#264177,#264178,#264179,#264180,#264181,
#264182,#264183,#264184,#264185,#264186,#264187,#264188,#264189,#264190,
#264191,#264192,#264193,#264194,#264195,#264196,#264197,#264198,#264199,
#264200,#264201,#264202,#264203,#264204,#264205,#264206,#264207,#264208,
#264209,#264210,#264211,#264212,#264213,#264214,#264215,#264216,#264217,
#264218,#264219,#264220,#264221,#264222,#264223,#264224,#264225,#264226,
#264227,#264228,#264229,#264230,#264231,#264232,#264233,#264234,#264235,
#264236,#264237,#264238,#264239,#264240,#264241,#264242,#264243,#264244,
#264245,#264246,#264247,#264248,#264249,#264250,#264251,#264252,#264253,
#264254,#264255,#264256,#264257,#264258,#264259,#264260,#264261,#264262,
#264263,#264264,#264265,#264266,#264267,#264268,#264269,#264270,#264271,
#264272,#264273,#264274,#264275,#264276,#264277,#264278,#264279,#264280,
#264281,#264282,#264283,#264284,#264285,#264286,#264287,#264288,#264289,
#264290,#264291,#264292,#264293,#264294,#264295,#264296,#264297,#264298,
#264299,#264300,#264301,#264302,#264303,#264304,#264305,#264306,#264307,
#264308,#264309,#264310,#264311,#264312,#264313,#264314,#264315,#264316,
#264317,#264318,#264319,#264320,#264321,#264322,#264323,#264324,#264325,
#264326,#264327,#264328,#264329,#264330,#264331,#264332,#264333,#264334,
#264335,#264336,#264337,#264338,#264339,#264340,#264341,#264342,#264343,
#264344,#264345,#264346,#264347,#264348,#264349,#264350,#264351,#264352,
#264353,#264354,#264355,#264356,#264357,#264358,#264359,#264360,#264361,
#264362,#264363,#264364,#264365,#264366,#264367,#264368,#264369,#264370,
#264371,#264372,#264373)),.UNSPECIFIED.,.F.,.T.,.F.,(2,2),(4,2,2,2,2,2,
2,2,2,2,2,2,2,2,2,2,2,2,2,2,2,2,2,2,2,2,2,2,2,2,2,2,2,2,2,2,2,2,2,2,2,2,
2,2,2,2,2,2,2,2,2,2,2,2,2,2,2,2,2,2,2,2,2,2,2,2,2,2,2,2,2,2,2,2,2,2,2,2,
2,2,2,2,2,2,2,2,2,2,2,2,2,2,2,2,2,2,2,2,2,2,2,2,2,2,2,2,2,2,2,2,2,4),(-1.37747249376985E-7,
1.00000777338949),(-0.000135430429350568,-2.14371909667077E-5,9.25560474171526E-5,
0.000320542524184873,0.000548529000952593,0.000776515477720314,0.00100450195448803,
0.00111849519287189,0.00123248843125575,0.00134648166963961,0.00146047490802347,
0.00157446814640733,0.0016884613847912,0.00191644786155891,0.00203044109994277,
0.00214443433832664,0.00225842757671049,0.00237242081509435,0.00260040729186208,
0.00271440053024594,0.0028283937686298,0.00294238700701366,0.00305638024539752,
0.00317037348378138,0.00328436672216524,0.0033983599605491,0.00351235319893296,
0.00362634643731682,0.00374033967570068,0.0039683261524684,0.00419631262923612,
0.00431030586761998,0.00436730248681191,0.00442429910600384,0.0045382923443877,
0.00465228558277156,0.00488027205953928,0.00499426529792314,0.005108258536307,
0.00522225177469086,0.00533624501307472,0.00545023825145858,0.00556423148984244,
0.0056782247282263,0.00579221796661016,0.00590621120499402,0.00602020444337788,
0.00613419768176174,0.0062481909201456,0.00647617739691333,0.00659017063529719,
0.00670416387368105,0.00681815711206491,0.00693215035044876,0.00704614358883263,
0.00716013682721649,0.00727413006560035,0.00738812330398421,0.00761610978075193,
0.00784409625751965,0.00795808949590351,0.00807208273428737,0.0081290793534793,
0.00818607597267123,0.00830006921105509,0.00852805568782281,0.00864204892620667,
0.00875604216459053,0.00887003540297439,0.00898402864135825,0.00921201511812597,
0.00944000159489369,0.00955399483327755,0.00966798807166141,0.00978198131004527,
0.00989597454842913,0.0101239610251968,0.0102379542635807,0.0103519475019646,
0.0104659407403484,0.0105799339787323,0.0106939272171161,0.0108079204555,
0.0109219136938839,0.0110359069322677,0.0111499001706516,0.0112638934090355,
0.0114918798858032,0.0117198663625709,0.0118338596009548,0.0118908562201467,
0.0119478528393386,0.0120618460777225,0.0121758393161063,0.0124038257928741,
0.0125178190312579,0.0126318122696418,0.0127458055080256,0.0128597987464095,
0.0129737919847934,0.0130877852231772,0.0133157716999449,0.0134297649383288,
0.0134867615575207,0.0135437581767127,0.0136577514150965,0.0137717446534804,
0.0139997311302481,0.0142277176070158,0.0142847142262077,0.0143417108453997,
0.0144557040837835),.UNSPECIFIED.);
#972=B_SPLINE_SURFACE_WITH_KNOTS('',1,3,((#266971,#266972,#266973,#266974,
#266975,#266976,#266977,#266978,#266979,#266980,#266981,#266982,#266983,
#266984,#266985,#266986,#266987,#266988,#266989,#266990,#266991,#266992,
#266993,#266994,#266995,#266996,#266997,#266998,#266999,#267000,#267001,
#267002,#267003,#267004,#267005,#267006,#267007,#267008,#267009,#267010,
#267011,#267012,#267013,#267014,#267015,#267016,#267017,#267018,#267019,
#267020,#267021,#267022,#267023,#267024,#267025,#267026,#267027,#267028,
#267029,#267030,#267031,#267032,#267033,#267034,#267035,#267036,#267037,
#267038,#267039,#267040,#267041,#267042,#267043,#267044,#267045,#267046,
#267047,#267048,#267049,#267050,#267051,#267052,#267053,#267054,#267055,
#267056,#267057,#267058,#267059,#267060,#267061,#267062,#267063,#267064,
#267065,#267066,#267067,#267068,#267069,#267070,#267071,#267072,#267073,
#267074,#267075,#267076,#267077,#267078,#267079,#267080,#267081,#267082,
#267083,#267084,#267085,#267086,#267087,#267088,#267089,#267090,#267091,
#267092,#267093,#267094,#267095,#267096,#267097,#267098,#267099,#267100,
#267101,#267102,#267103,#267104,#267105,#267106,#267107,#267108,#267109,
#267110,#267111,#267112,#267113,#267114,#267115,#267116,#267117,#267118,
#267119,#267120,#267121,#267122,#267123,#267124,#267125,#267126,#267127,
#267128,#267129,#267130,#267131,#267132,#267133,#267134,#267135,#267136,
#267137,#267138,#267139,#267140,#267141,#267142,#267143,#267144,#267145,
#267146,#267147,#267148,#267149,#267150,#267151,#267152,#267153,#267154,
#267155,#267156,#267157,#267158,#267159,#267160,#267161,#267162,#267163,
#267164,#267165,#267166,#267167,#267168,#267169,#267170,#267171,#267172,
#267173,#267174,#267175,#267176,#267177,#267178,#267179,#267180,#267181,
#267182,#267183,#267184,#267185,#267186,#267187,#267188,#267189,#267190,
#267191,#267192,#267193,#267194),(#267195,#267196,#267197,#267198,#267199,
#267200,#267201,#267202,#267203,#267204,#267205,#267206,#267207,#267208,
#267209,#267210,#267211,#267212,#267213,#267214,#267215,#267216,#267217,
#267218,#267219,#267220,#267221,#267222,#267223,#267224,#267225,#267226,
#267227,#267228,#267229,#267230,#267231,#267232,#267233,#267234,#267235,
#267236,#267237,#267238,#267239,#267240,#267241,#267242,#267243,#267244,
#267245,#267246,#267247,#267248,#267249,#267250,#267251,#267252,#267253,
#267254,#267255,#267256,#267257,#267258,#267259,#267260,#267261,#267262,
#267263,#267264,#267265,#267266,#267267,#267268,#267269,#267270,#267271,
#267272,#267273,#267274,#267275,#267276,#267277,#267278,#267279,#267280,
#267281,#267282,#267283,#267284,#267285,#267286,#267287,#267288,#267289,
#267290,#267291,#267292,#267293,#267294,#267295,#267296,#267297,#267298,
#267299,#267300,#267301,#267302,#267303,#267304,#267305,#267306,#267307,
#267308,#267309,#267310,#267311,#267312,#267313,#267314,#267315,#267316,
#267317,#267318,#267319,#267320,#267321,#267322,#267323,#267324,#267325,
#267326,#267327,#267328,#267329,#267330,#267331,#267332,#267333,#267334,
#267335,#267336,#267337,#267338,#267339,#267340,#267341,#267342,#267343,
#267344,#267345,#267346,#267347,#267348,#267349,#267350,#267351,#267352,
#267353,#267354,#267355,#267356,#267357,#267358,#267359,#267360,#267361,
#267362,#267363,#267364,#267365,#267366,#267367,#267368,#267369,#267370,
#267371,#267372,#267373,#267374,#267375,#267376,#267377,#267378,#267379,
#267380,#267381,#267382,#267383,#267384,#267385,#267386,#267387,#267388,
#267389,#267390,#267391,#267392,#267393,#267394,#267395,#267396,#267397,
#267398,#267399,#267400,#267401,#267402,#267403,#267404,#267405,#267406,
#267407,#267408,#267409,#267410,#267411,#267412,#267413,#267414,#267415,
#267416,#267417,#267418)),.UNSPECIFIED.,.F.,.T.,.F.,(2,2),(4,2,2,2,2,2,
2,2,2,2,2,2,2,2,2,2,2,2,2,2,2,2,2,2,2,2,2,2,2,2,2,2,2,2,2,2,2,2,2,2,2,2,
2,2,2,2,2,2,2,2,2,2,2,2,2,2,2,2,2,2,2,2,2,2,2,2,2,2,2,2,2,2,2,2,2,2,2,2,
2,2,2,2,2,2,2,2,2,2,2,2,2,2,2,2,2,2,2,2,2,2,2,2,2,2,2,2,2,2,2,2,2,4),(-3.14488534446183E-8,
1.00000561805477),(-0.000135430429350568,-2.14371909667077E-5,9.25560474171526E-5,
0.000320542524184873,0.000548529000952593,0.000776515477720314,0.00100450195448803,
0.00111849519287189,0.00123248843125575,0.00134648166963961,0.00146047490802347,
0.00157446814640733,0.0016884613847912,0.00191644786155891,0.00203044109994277,
0.00214443433832664,0.00225842757671049,0.00237242081509435,0.00260040729186208,
0.00271440053024594,0.0028283937686298,0.00294238700701366,0.00305638024539752,
0.00317037348378138,0.00328436672216524,0.0033983599605491,0.00351235319893296,
0.00362634643731682,0.00374033967570068,0.0039683261524684,0.00419631262923612,
0.00431030586761998,0.00436730248681191,0.00442429910600384,0.0045382923443877,
0.00465228558277156,0.00488027205953928,0.00499426529792314,0.005108258536307,
0.00522225177469086,0.00533624501307472,0.00545023825145858,0.00556423148984244,
0.0056782247282263,0.00579221796661016,0.00590621120499402,0.00602020444337788,
0.00613419768176174,0.0062481909201456,0.00647617739691333,0.00659017063529719,
0.00670416387368105,0.00681815711206491,0.00693215035044876,0.00704614358883263,
0.00716013682721649,0.00727413006560035,0.00738812330398421,0.00761610978075193,
0.00784409625751965,0.00795808949590351,0.00807208273428737,0.0081290793534793,
0.00818607597267123,0.00830006921105509,0.00852805568782281,0.00864204892620667,
0.00875604216459053,0.00887003540297439,0.00898402864135825,0.00921201511812597,
0.00944000159489369,0.00955399483327755,0.00966798807166141,0.00978198131004527,
0.00989597454842913,0.0101239610251968,0.0102379542635807,0.0103519475019646,
0.0104659407403484,0.0105799339787323,0.0106939272171161,0.0108079204555,
0.0109219136938839,0.0110359069322677,0.0111499001706516,0.0112638934090355,
0.0114918798858032,0.0117198663625709,0.0118338596009548,0.0118908562201467,
0.0119478528393386,0.0120618460777225,0.0121758393161063,0.0124038257928741,
0.0125178190312579,0.0126318122696418,0.0127458055080256,0.0128597987464095,
0.0129737919847934,0.0130877852231772,0.0133157716999449,0.0134297649383288,
0.0134867615575207,0.0135437581767127,0.0136577514150965,0.0137717446534804,
0.0139997311302481,0.0142277176070158,0.0142847142262077,0.0143417108453997,
0.0144557040837835),.UNSPECIFIED.);
#973=B_SPLINE_SURFACE_WITH_KNOTS('',1,3,((#267480,#267481,#267482,#267483,
#267484,#267485,#267486,#267487,#267488,#267489,#267490,#267491,#267492,
#267493,#267494,#267495,#267496,#267497,#267498,#267499,#267500,#267501,
#267502,#267503,#267504,#267505,#267506,#267507,#267508,#267509,#267510,
#267511,#267512,#267513,#267514,#267515,#267516,#267517,#267518,#267519,
#267520,#267521,#267522,#267523,#267524,#267525,#267526,#267527,#267528,
#267529,#267530,#267531,#267532,#267533,#267534,#267535,#267536,#267537,
#267538,#267539,#267540,#267541,#267542,#267543,#267544,#267545,#267546,
#267547,#267548,#267549,#267550,#267551,#267552,#267553,#267554,#267555,
#267556,#267557,#267558,#267559,#267560,#267561,#267562,#267563,#267564,
#267565,#267566,#267567,#267568,#267569,#267570,#267571,#267572,#267573,
#267574,#267575,#267576,#267577,#267578,#267579,#267580,#267581,#267582,
#267583,#267584,#267585,#267586,#267587,#267588,#267589,#267590,#267591,
#267592,#267593,#267594,#267595,#267596,#267597,#267598,#267599,#267600,
#267601,#267602,#267603,#267604,#267605,#267606,#267607,#267608,#267609,
#267610,#267611,#267612,#267613,#267614,#267615,#267616,#267617,#267618,
#267619,#267620,#267621,#267622,#267623,#267624,#267625,#267626,#267627,
#267628,#267629,#267630,#267631,#267632,#267633,#267634,#267635,#267636,
#267637,#267638,#267639,#267640,#267641,#267642,#267643,#267644,#267645,
#267646,#267647,#267648,#267649,#267650,#267651,#267652,#267653,#267654),
(#267655,#267656,#267657,#267658,#267659,#267660,#267661,#267662,#267663,
#267664,#267665,#267666,#267667,#267668,#267669,#267670,#267671,#267672,
#267673,#267674,#267675,#267676,#267677,#267678,#267679,#267680,#267681,
#267682,#267683,#267684,#267685,#267686,#267687,#267688,#267689,#267690,
#267691,#267692,#267693,#267694,#267695,#267696,#267697,#267698,#267699,
#267700,#267701,#267702,#267703,#267704,#267705,#267706,#267707,#267708,
#267709,#267710,#267711,#267712,#267713,#267714,#267715,#267716,#267717,
#267718,#267719,#267720,#267721,#267722,#267723,#267724,#267725,#267726,
#267727,#267728,#267729,#267730,#267731,#267732,#267733,#267734,#267735,
#267736,#267737,#267738,#267739,#267740,#267741,#267742,#267743,#267744,
#267745,#267746,#267747,#267748,#267749,#267750,#267751,#267752,#267753,
#267754,#267755,#267756,#267757,#267758,#267759,#267760,#267761,#267762,
#267763,#267764,#267765,#267766,#267767,#267768,#267769,#267770,#267771,
#267772,#267773,#267774,#267775,#267776,#267777,#267778,#267779,#267780,
#267781,#267782,#267783,#267784,#267785,#267786,#267787,#267788,#267789,
#267790,#267791,#267792,#267793,#267794,#267795,#267796,#267797,#267798,
#267799,#267800,#267801,#267802,#267803,#267804,#267805,#267806,#267807,
#267808,#267809,#267810,#267811,#267812,#267813,#267814,#267815,#267816,
#267817,#267818,#267819,#267820,#267821,#267822,#267823,#267824,#267825,
#267826,#267827,#267828,#267829)),.UNSPECIFIED.,.F.,.T.,.F.,(2,2),(4,1,
1,2,1,1,1,1,2,2,1,2,2,2,2,1,1,2,2,2,1,1,1,1,2,2,2,2,2,2,2,2,1,1,1,2,2,2,
2,1,1,1,2,2,2,1,1,1,2,2,2,2,2,2,2,1,2,2,2,2,2,1,1,2,2,2,2,1,2,2,2,1,1,2,
2,2,1,1,1,1,2,2,2,2,2,2,2,1,2,1,1,2,2,2,1,2,2,2,2,2,1,2,2,2,2,4),(0.,5.46382276754873),
(-0.000135430429350568,9.25560474171526E-5,0.000320542524184873,0.000548529000952593,
0.000776515477720314,0.00100450195448803,0.00111849519287189,0.00123248843125575,
0.00134648166963961,0.00146047490802347,0.0016884613847912,0.00191644786155891,
0.00203044109994277,0.00214443433832664,0.00225842757671049,0.00237242081509435,
0.00260040729186208,0.00271440053024594,0.0028283937686298,0.00294238700701366,
0.00305638024539752,0.00317037348378138,0.00328436672216524,0.0033983599605491,
0.00351235319893296,0.00362634643731682,0.00374033967570068,0.0039683261524684,
0.00419631262923612,0.00431030586761998,0.00436730248681191,0.00442429910600384,
0.0045382923443877,0.00465228558277156,0.00488027205953928,0.00499426529792314,
0.005108258536307,0.00522225177469086,0.00533624501307472,0.00556423148984244,
0.0056782247282263,0.00579221796661016,0.00590621120499402,0.00602020444337788,
0.00613419768176174,0.0062481909201456,0.00647617739691333,0.00659017063529719,
0.00670416387368105,0.00681815711206491,0.00693215035044876,0.00716013682721649,
0.00727413006560035,0.00738812330398421,0.00761610978075193,0.00784409625751965,
0.00795808949590351,0.00807208273428737,0.0081290793534793,0.00818607597267123,
0.00830006921105509,0.00852805568782281,0.00864204892620667,0.00875604216459053,
0.00887003540297439,0.00898402864135825,0.00921201511812597,0.00944000159489369,
0.00955399483327755,0.00966798807166141,0.00978198131004527,0.00989597454842913,
0.0101239610251968,0.0102379542635807,0.0103519475019646,0.0104659407403484,
0.0105799339787323,0.0106939272171161,0.0108079204555,0.0109219136938839,
0.0110359069322677,0.0111499001706516,0.0112638934090355,0.0114918798858032,
0.0117198663625709,0.0118338596009548,0.0118908562201467,0.0119478528393386,
0.0120618460777225,0.0121758393161063,0.0124038257928741,0.0125178190312579,
0.0126318122696418,0.0127458055080256,0.0129737919847934,0.0130877852231772,
0.0133157716999449,0.0134297649383288,0.0134867615575207,0.0135437581767127,
0.0137717446534804,0.0139997311302481,0.0142277176070158,0.0142847142262077,
0.0143417108453997,0.0144557040837835),.UNSPECIFIED.);
#974=B_SPLINE_SURFACE_WITH_KNOTS('',1,3,((#267830,#267831,#267832,#267833,
#267834,#267835,#267836,#267837,#267838,#267839,#267840,#267841,#267842,
#267843,#267844,#267845,#267846,#267847,#267848,#267849,#267850,#267851,
#267852,#267853,#267854,#267855,#267856,#267857,#267858,#267859,#267860,
#267861,#267862,#267863,#267864,#267865,#267866,#267867,#267868,#267869,
#267870,#267871,#267872,#267873,#267874,#267875,#267876,#267877,#267878,
#267879,#267880,#267881,#267882,#267883,#267884,#267885,#267886,#267887,
#267888,#267889,#267890,#267891,#267892,#267893,#267894,#267895,#267896,
#267897,#267898,#267899,#267900,#267901,#267902,#267903,#267904,#267905,
#267906,#267907,#267908,#267909,#267910,#267911,#267912,#267913,#267914,
#267915,#267916,#267917,#267918,#267919,#267920,#267921,#267922,#267923,
#267924,#267925,#267926,#267927,#267928,#267929,#267930,#267931,#267932,
#267933,#267934,#267935,#267936,#267937,#267938,#267939,#267940,#267941,
#267942,#267943,#267944,#267945,#267946,#267947,#267948,#267949,#267950,
#267951,#267952,#267953,#267954,#267955,#267956,#267957,#267958,#267959,
#267960,#267961,#267962,#267963,#267964,#267965,#267966,#267967,#267968,
#267969,#267970,#267971,#267972,#267973,#267974,#267975,#267976,#267977,
#267978,#267979,#267980,#267981,#267982,#267983,#267984,#267985,#267986,
#267987,#267988,#267989,#267990,#267991,#267992,#267993,#267994,#267995,
#267996,#267997,#267998,#267999,#268000,#268001,#268002,#268003,#268004),
(#268005,#268006,#268007,#268008,#268009,#268010,#268011,#268012,#268013,
#268014,#268015,#268016,#268017,#268018,#268019,#268020,#268021,#268022,
#268023,#268024,#268025,#268026,#268027,#268028,#268029,#268030,#268031,
#268032,#268033,#268034,#268035,#268036,#268037,#268038,#268039,#268040,
#268041,#268042,#268043,#268044,#268045,#268046,#268047,#268048,#268049,
#268050,#268051,#268052,#268053,#268054,#268055,#268056,#268057,#268058,
#268059,#268060,#268061,#268062,#268063,#268064,#268065,#268066,#268067,
#268068,#268069,#268070,#268071,#268072,#268073,#268074,#268075,#268076,
#268077,#268078,#268079,#268080,#268081,#268082,#268083,#268084,#268085,
#268086,#268087,#268088,#268089,#268090,#268091,#268092,#268093,#268094,
#268095,#268096,#268097,#268098,#268099,#268100,#268101,#268102,#268103,
#268104,#268105,#268106,#268107,#268108,#268109,#268110,#268111,#268112,
#268113,#268114,#268115,#268116,#268117,#268118,#268119,#268120,#268121,
#268122,#268123,#268124,#268125,#268126,#268127,#268128,#268129,#268130,
#268131,#268132,#268133,#268134,#268135,#268136,#268137,#268138,#268139,
#268140,#268141,#268142,#268143,#268144,#268145,#268146,#268147,#268148,
#268149,#268150,#268151,#268152,#268153,#268154,#268155,#268156,#268157,
#268158,#268159,#268160,#268161,#268162,#268163,#268164,#268165,#268166,
#268167,#268168,#268169,#268170,#268171,#268172,#268173,#268174,#268175,
#268176,#268177,#268178,#268179)),.UNSPECIFIED.,.F.,.T.,.F.,(2,2),(4,1,
1,2,1,1,1,1,2,2,1,2,2,2,2,1,1,2,2,2,1,1,1,1,2,2,2,2,2,2,2,2,1,1,1,2,2,2,
2,1,1,1,2,2,2,1,1,1,2,2,2,2,2,2,2,1,2,2,2,2,2,1,1,2,2,2,2,1,2,2,2,1,1,2,
2,2,1,1,1,1,2,2,2,2,2,2,2,1,2,1,1,2,2,2,1,2,2,2,2,2,1,2,2,2,2,4),(0.,5.46382276754873),
(-0.000135430429350568,9.25560474171526E-5,0.000320542524184873,0.000548529000952593,
0.000776515477720314,0.00100450195448803,0.00111849519287189,0.00123248843125575,
0.00134648166963961,0.00146047490802347,0.0016884613847912,0.00191644786155891,
0.00203044109994277,0.00214443433832664,0.00225842757671049,0.00237242081509435,
0.00260040729186208,0.00271440053024594,0.0028283937686298,0.00294238700701366,
0.00305638024539752,0.00317037348378138,0.00328436672216524,0.0033983599605491,
0.00351235319893296,0.00362634643731682,0.00374033967570068,0.0039683261524684,
0.00419631262923612,0.00431030586761998,0.00436730248681191,0.00442429910600384,
0.0045382923443877,0.00465228558277156,0.00488027205953928,0.00499426529792314,
0.005108258536307,0.00522225177469086,0.00533624501307472,0.00556423148984244,
0.0056782247282263,0.00579221796661016,0.00590621120499402,0.00602020444337788,
0.00613419768176174,0.0062481909201456,0.00647617739691333,0.00659017063529719,
0.00670416387368105,0.00681815711206491,0.00693215035044876,0.00716013682721649,
0.00727413006560035,0.00738812330398421,0.00761610978075193,0.00784409625751965,
0.00795808949590351,0.00807208273428737,0.0081290793534793,0.00818607597267123,
0.00830006921105509,0.00852805568782281,0.00864204892620667,0.00875604216459053,
0.00887003540297439,0.00898402864135825,0.00921201511812597,0.00944000159489369,
0.00955399483327755,0.00966798807166141,0.00978198131004527,0.00989597454842913,
0.0101239610251968,0.0102379542635807,0.0103519475019646,0.0104659407403484,
0.0105799339787323,0.0106939272171161,0.0108079204555,0.0109219136938839,
0.0110359069322677,0.0111499001706516,0.0112638934090355,0.0114918798858032,
0.0117198663625709,0.0118338596009548,0.0118908562201467,0.0119478528393386,
0.0120618460777225,0.0121758393161063,0.0124038257928741,0.0125178190312579,
0.0126318122696418,0.0127458055080256,0.0129737919847934,0.0130877852231772,
0.0133157716999449,0.0134297649383288,0.0134867615575207,0.0135437581767127,
0.0137717446534804,0.0139997311302481,0.0142277176070158,0.0142847142262077,
0.0143417108453997,0.0144557040837835),.UNSPECIFIED.);
#975=B_SPLINE_SURFACE_WITH_KNOTS('',1,3,((#268180,#268181,#268182,#268183,
#268184,#268185,#268186,#268187,#268188,#268189,#268190,#268191,#268192,
#268193,#268194,#268195,#268196,#268197,#268198,#268199,#268200,#268201,
#268202,#268203,#268204,#268205,#268206,#268207,#268208,#268209,#268210,
#268211,#268212,#268213,#268214,#268215,#268216,#268217,#268218,#268219,
#268220,#268221,#268222,#268223,#268224,#268225,#268226,#268227,#268228,
#268229,#268230,#268231,#268232,#268233,#268234,#268235,#268236,#268237,
#268238,#268239,#268240,#268241,#268242,#268243,#268244,#268245,#268246,
#268247,#268248,#268249,#268250,#268251,#268252,#268253,#268254,#268255,
#268256,#268257,#268258,#268259,#268260,#268261,#268262,#268263,#268264,
#268265,#268266,#268267,#268268,#268269,#268270,#268271,#268272,#268273,
#268274,#268275,#268276,#268277,#268278,#268279,#268280,#268281,#268282,
#268283,#268284,#268285,#268286,#268287,#268288,#268289,#268290,#268291),
(#268292,#268293,#268294,#268295,#268296,#268297,#268298,#268299,#268300,
#268301,#268302,#268303,#268304,#268305,#268306,#268307,#268308,#268309,
#268310,#268311,#268312,#268313,#268314,#268315,#268316,#268317,#268318,
#268319,#268320,#268321,#268322,#268323,#268324,#268325,#268326,#268327,
#268328,#268329,#268330,#268331,#268332,#268333,#268334,#268335,#268336,
#268337,#268338,#268339,#268340,#268341,#268342,#268343,#268344,#268345,
#268346,#268347,#268348,#268349,#268350,#268351,#268352,#268353,#268354,
#268355,#268356,#268357,#268358,#268359,#268360,#268361,#268362,#268363,
#268364,#268365,#268366,#268367,#268368,#268369,#268370,#268371,#268372,
#268373,#268374,#268375,#268376,#268377,#268378,#268379,#268380,#268381,
#268382,#268383,#268384,#268385,#268386,#268387,#268388,#268389,#268390,
#268391,#268392,#268393,#268394,#268395,#268396,#268397,#268398,#268399,
#268400,#268401,#268402,#268403)),.UNSPECIFIED.,.F.,.F.,.F.,(2,2),(4,2,
2,2,2,2,2,2,2,2,2,2,2,2,2,2,2,2,2,2,2,2,2,2,2,2,2,2,2,2,2,2,2,2,2,2,2,2,
2,2,2,2,2,2,2,2,2,2,2,2,2,2,2,2,2,4),(0.,1.),(-0.000135430429350568,-2.14371909667077E-5,
9.25560474171526E-5,0.000320542524184873,0.000548529000952593,0.000776515477720314,
0.00100450195448803,0.00111849519287189,0.00123248843125575,0.00134648166963961,
0.00146047490802347,0.00157446814640733,0.0016884613847912,0.00191644786155891,
0.00203044109994277,0.00214443433832664,0.00225842757671049,0.00237242081509435,
0.00260040729186208,0.00271440053024594,0.0028283937686298,0.00294238700701366,
0.00305638024539752,0.00317037348378138,0.00328436672216524,0.0033983599605491,
0.00351235319893296,0.00362634643731682,0.00374033967570068,0.0039683261524684,
0.00419631262923612,0.00431030586761998,0.00436730248681191,0.00442429910600384,
0.0045382923443877,0.00465228558277156,0.00488027205953928,0.00499426529792314,
0.005108258536307,0.00522225177469086,0.00533624501307472,0.00545023825145858,
0.00556423148984244,0.0056782247282263,0.00579221796661016,0.00590621120499402,
0.00602020444337788,0.00613419768176174,0.0062481909201456,0.00647617739691333,
0.00659017063529719,0.00670416387368105,0.00681815711206491,0.00693215035044876,
0.00704614358883263,0.00716013682721649),.UNSPECIFIED.);
#976=B_SPLINE_SURFACE_WITH_KNOTS('',1,3,((#268440,#268441,#268442,#268443,
#268444,#268445,#268446,#268447,#268448,#268449,#268450,#268451,#268452,
#268453,#268454,#268455,#268456,#268457,#268458,#268459,#268460,#268461,
#268462,#268463,#268464,#268465,#268466,#268467,#268468,#268469,#268470,
#268471,#268472,#268473,#268474,#268475,#268476,#268477,#268478,#268479,
#268480,#268481,#268482,#268483,#268484,#268485,#268486,#268487,#268488,
#268489,#268490,#268491,#268492,#268493,#268494,#268495,#268496,#268497,
#268498,#268499,#268500,#268501,#268502,#268503,#268504,#268505,#268506,
#268507,#268508,#268509,#268510,#268511,#268512,#268513,#268514,#268515,
#268516,#268517,#268518,#268519,#268520,#268521,#268522,#268523,#268524,
#268525,#268526,#268527,#268528,#268529,#268530,#268531,#268532,#268533,
#268534,#268535,#268536,#268537,#268538,#268539,#268540,#268541,#268542,
#268543,#268544,#268545,#268546,#268547,#268548,#268549,#268550,#268551,
#268552,#268553,#268554,#268555,#268556,#268557,#268558,#268559,#268560,
#268561,#268562,#268563,#268564,#268565,#268566,#268567,#268568,#268569,
#268570,#268571,#268572,#268573,#268574,#268575,#268576,#268577,#268578,
#268579,#268580,#268581,#268582,#268583,#268584,#268585,#268586,#268587,
#268588,#268589,#268590,#268591,#268592,#268593,#268594,#268595,#268596,
#268597,#268598,#268599,#268600,#268601,#268602,#268603,#268604,#268605,
#268606,#268607,#268608,#268609,#268610,#268611,#268612,#268613,#268614),
(#268615,#268616,#268617,#268618,#268619,#268620,#268621,#268622,#268623,
#268624,#268625,#268626,#268627,#268628,#268629,#268630,#268631,#268632,
#268633,#268634,#268635,#268636,#268637,#268638,#268639,#268640,#268641,
#268642,#268643,#268644,#268645,#268646,#268647,#268648,#268649,#268650,
#268651,#268652,#268653,#268654,#268655,#268656,#268657,#268658,#268659,
#268660,#268661,#268662,#268663,#268664,#268665,#268666,#268667,#268668,
#268669,#268670,#268671,#268672,#268673,#268674,#268675,#268676,#268677,
#268678,#268679,#268680,#268681,#268682,#268683,#268684,#268685,#268686,
#268687,#268688,#268689,#268690,#268691,#268692,#268693,#268694,#268695,
#268696,#268697,#268698,#268699,#268700,#268701,#268702,#268703,#268704,
#268705,#268706,#268707,#268708,#268709,#268710,#268711,#268712,#268713,
#268714,#268715,#268716,#268717,#268718,#268719,#268720,#268721,#268722,
#268723,#268724,#268725,#268726,#268727,#268728,#268729,#268730,#268731,
#268732,#268733,#268734,#268735,#268736,#268737,#268738,#268739,#268740,
#268741,#268742,#268743,#268744,#268745,#268746,#268747,#268748,#268749,
#268750,#268751,#268752,#268753,#268754,#268755,#268756,#268757,#268758,
#268759,#268760,#268761,#268762,#268763,#268764,#268765,#268766,#268767,
#268768,#268769,#268770,#268771,#268772,#268773,#268774,#268775,#268776,
#268777,#268778,#268779,#268780,#268781,#268782,#268783,#268784,#268785,
#268786,#268787,#268788,#268789)),.UNSPECIFIED.,.F.,.T.,.F.,(2,2),(4,1,
1,2,1,1,1,1,2,2,1,2,2,2,2,1,1,2,2,2,1,1,1,1,2,2,2,2,2,2,2,2,1,1,1,2,2,2,
2,1,1,1,2,2,2,1,1,1,2,2,2,2,2,2,2,1,2,2,2,2,2,1,1,2,2,2,2,1,2,2,2,1,1,2,
2,2,1,1,1,1,2,2,2,2,2,2,2,1,2,1,1,2,2,2,1,2,2,2,2,2,1,2,2,2,2,4),(0.,4.71475608888856),
(-0.000135430429350568,9.25560474171526E-5,0.000320542524184873,0.000548529000952593,
0.000776515477720314,0.00100450195448803,0.00111849519287189,0.00123248843125575,
0.00134648166963961,0.00146047490802347,0.0016884613847912,0.00191644786155891,
0.00203044109994277,0.00214443433832664,0.00225842757671049,0.00237242081509435,
0.00260040729186208,0.00271440053024594,0.0028283937686298,0.00294238700701366,
0.00305638024539752,0.00317037348378138,0.00328436672216524,0.0033983599605491,
0.00351235319893296,0.00362634643731682,0.00374033967570068,0.0039683261524684,
0.00419631262923612,0.00431030586761998,0.00436730248681191,0.00442429910600384,
0.0045382923443877,0.00465228558277156,0.00488027205953928,0.00499426529792314,
0.005108258536307,0.00522225177469086,0.00533624501307472,0.00556423148984244,
0.0056782247282263,0.00579221796661016,0.00590621120499402,0.00602020444337788,
0.00613419768176174,0.0062481909201456,0.00647617739691333,0.00659017063529719,
0.00670416387368105,0.00681815711206491,0.00693215035044876,0.00716013682721649,
0.00727413006560035,0.00738812330398421,0.00761610978075193,0.00784409625751965,
0.00795808949590351,0.00807208273428737,0.0081290793534793,0.00818607597267123,
0.00830006921105509,0.00852805568782281,0.00864204892620667,0.00875604216459053,
0.00887003540297439,0.00898402864135825,0.00921201511812597,0.00944000159489369,
0.00955399483327755,0.00966798807166141,0.00978198131004527,0.00989597454842913,
0.0101239610251968,0.0102379542635807,0.0103519475019646,0.0104659407403484,
0.0105799339787323,0.0106939272171161,0.0108079204555,0.0109219136938839,
0.0110359069322677,0.0111499001706516,0.0112638934090355,0.0114918798858032,
0.0117198663625709,0.0118338596009548,0.0118908562201467,0.0119478528393386,
0.0120618460777225,0.0121758393161063,0.0124038257928741,0.0125178190312579,
0.0126318122696418,0.0127458055080256,0.0129737919847934,0.0130877852231772,
0.0133157716999449,0.0134297649383288,0.0134867615575207,0.0135437581767127,
0.0137717446534804,0.0139997311302481,0.0142277176070158,0.0142847142262077,
0.0143417108453997,0.0144557040837835),.UNSPECIFIED.);
#977=B_SPLINE_SURFACE_WITH_KNOTS('',1,3,((#268791,#268792,#268793,#268794,
#268795,#268796,#268797,#268798,#268799,#268800,#268801,#268802,#268803,
#268804,#268805,#268806,#268807,#268808,#268809,#268810,#268811,#268812,
#268813,#268814,#268815,#268816,#268817,#268818,#268819,#268820,#268821,
#268822,#268823,#268824,#268825,#268826,#268827,#268828,#268829,#268830,
#268831,#268832,#268833,#268834,#268835,#268836,#268837,#268838,#268839,
#268840,#268841,#268842,#268843,#268844,#268845,#268846,#268847,#268848,
#268849,#268850,#268851,#268852,#268853,#268854,#268855,#268856,#268857,
#268858,#268859,#268860,#268861,#268862,#268863,#268864,#268865,#268866,
#268867,#268868,#268869,#268870,#268871,#268872,#268873,#268874,#268875,
#268876,#268877,#268878,#268879,#268880,#268881,#268882,#268883,#268884,
#268885,#268886,#268887,#268888,#268889,#268890,#268891,#268892,#268893,
#268894,#268895,#268896,#268897,#268898,#268899,#268900,#268901,#268902,
#268903,#268904,#268905,#268906,#268907,#268908,#268909,#268910,#268911,
#268912,#268913,#268914,#268915,#268916,#268917,#268918,#268919,#268920,
#268921,#268922,#268923,#268924,#268925,#268926,#268927,#268928,#268929,
#268930,#268931,#268932,#268933,#268934,#268935,#268936,#268937,#268938,
#268939,#268940,#268941,#268942,#268943,#268944,#268945,#268946,#268947,
#268948,#268949,#268950,#268951,#268952,#268953,#268954,#268955,#268956,
#268957,#268958,#268959,#268960,#268961,#268962,#268963,#268964,#268965),
(#268966,#268967,#268968,#268969,#268970,#268971,#268972,#268973,#268974,
#268975,#268976,#268977,#268978,#268979,#268980,#268981,#268982,#268983,
#268984,#268985,#268986,#268987,#268988,#268989,#268990,#268991,#268992,
#268993,#268994,#268995,#268996,#268997,#268998,#268999,#269000,#269001,
#269002,#269003,#269004,#269005,#269006,#269007,#269008,#269009,#269010,
#269011,#269012,#269013,#269014,#269015,#269016,#269017,#269018,#269019,
#269020,#269021,#269022,#269023,#269024,#269025,#269026,#269027,#269028,
#269029,#269030,#269031,#269032,#269033,#269034,#269035,#269036,#269037,
#269038,#269039,#269040,#269041,#269042,#269043,#269044,#269045,#269046,
#269047,#269048,#269049,#269050,#269051,#269052,#269053,#269054,#269055,
#269056,#269057,#269058,#269059,#269060,#269061,#269062,#269063,#269064,
#269065,#269066,#269067,#269068,#269069,#269070,#269071,#269072,#269073,
#269074,#269075,#269076,#269077,#269078,#269079,#269080,#269081,#269082,
#269083,#269084,#269085,#269086,#269087,#269088,#269089,#269090,#269091,
#269092,#269093,#269094,#269095,#269096,#269097,#269098,#269099,#269100,
#269101,#269102,#269103,#269104,#269105,#269106,#269107,#269108,#269109,
#269110,#269111,#269112,#269113,#269114,#269115,#269116,#269117,#269118,
#269119,#269120,#269121,#269122,#269123,#269124,#269125,#269126,#269127,
#269128,#269129,#269130,#269131,#269132,#269133,#269134,#269135,#269136,
#269137,#269138,#269139,#269140)),.UNSPECIFIED.,.F.,.T.,.F.,(2,2),(4,1,
1,2,1,1,1,1,2,2,1,2,2,2,2,1,1,2,2,2,1,1,1,1,2,2,2,2,2,2,2,2,1,1,1,2,2,2,
2,1,1,1,2,2,2,1,1,1,2,2,2,2,2,2,2,1,2,2,2,2,2,1,1,2,2,2,2,1,2,2,2,1,1,2,
2,2,1,1,1,1,2,2,2,2,2,2,2,1,2,1,1,2,2,2,1,2,2,2,2,2,1,2,2,2,2,4),(0.,4.71475608888856),
(-0.000135430429350568,9.25560474171526E-5,0.000320542524184873,0.000548529000952593,
0.000776515477720314,0.00100450195448803,0.00111849519287189,0.00123248843125575,
0.00134648166963961,0.00146047490802347,0.0016884613847912,0.00191644786155891,
0.00203044109994277,0.00214443433832664,0.00225842757671049,0.00237242081509435,
0.00260040729186208,0.00271440053024594,0.0028283937686298,0.00294238700701366,
0.00305638024539752,0.00317037348378138,0.00328436672216524,0.0033983599605491,
0.00351235319893296,0.00362634643731682,0.00374033967570068,0.0039683261524684,
0.00419631262923612,0.00431030586761998,0.00436730248681191,0.00442429910600384,
0.0045382923443877,0.00465228558277156,0.00488027205953928,0.00499426529792314,
0.005108258536307,0.00522225177469086,0.00533624501307472,0.00556423148984244,
0.0056782247282263,0.00579221796661016,0.00590621120499402,0.00602020444337788,
0.00613419768176174,0.0062481909201456,0.00647617739691333,0.00659017063529719,
0.00670416387368105,0.00681815711206491,0.00693215035044876,0.00716013682721649,
0.00727413006560035,0.00738812330398421,0.00761610978075193,0.00784409625751965,
0.00795808949590351,0.00807208273428737,0.0081290793534793,0.00818607597267123,
0.00830006921105509,0.00852805568782281,0.00864204892620667,0.00875604216459053,
0.00887003540297439,0.00898402864135825,0.00921201511812597,0.00944000159489369,
0.00955399483327755,0.00966798807166141,0.00978198131004527,0.00989597454842913,
0.0101239610251968,0.0102379542635807,0.0103519475019646,0.0104659407403484,
0.0105799339787323,0.0106939272171161,0.0108079204555,0.0109219136938839,
0.0110359069322677,0.0111499001706516,0.0112638934090355,0.0114918798858032,
0.0117198663625709,0.0118338596009548,0.0118908562201467,0.0119478528393386,
0.0120618460777225,0.0121758393161063,0.0124038257928741,0.0125178190312579,
0.0126318122696418,0.0127458055080256,0.0129737919847934,0.0130877852231772,
0.0133157716999449,0.0134297649383288,0.0134867615575207,0.0135437581767127,
0.0137717446534804,0.0139997311302481,0.0142277176070158,0.0142847142262077,
0.0143417108453997,0.0144557040837835),.UNSPECIFIED.);
#978=B_SPLINE_SURFACE_WITH_KNOTS('',1,3,((#269141,#269142,#269143,#269144,
#269145,#269146,#269147,#269148,#269149,#269150,#269151,#269152,#269153,
#269154,#269155,#269156,#269157,#269158,#269159,#269160,#269161,#269162,
#269163,#269164,#269165,#269166,#269167,#269168,#269169,#269170,#269171,
#269172,#269173,#269174,#269175,#269176,#269177,#269178,#269179,#269180,
#269181,#269182,#269183,#269184,#269185,#269186,#269187,#269188,#269189,
#269190,#269191,#269192,#269193,#269194,#269195,#269196,#269197,#269198,
#269199,#269200,#269201,#269202,#269203,#269204,#269205,#269206,#269207,
#269208,#269209,#269210,#269211,#269212,#269213,#269214,#269215,#269216,
#269217,#269218,#269219,#269220,#269221,#269222,#269223,#269224,#269225,
#269226,#269227,#269228,#269229,#269230,#269231,#269232,#269233,#269234,
#269235,#269236,#269237,#269238,#269239,#269240,#269241,#269242,#269243,
#269244,#269245,#269246,#269247,#269248,#269249,#269250,#269251,#269252),
(#269253,#269254,#269255,#269256,#269257,#269258,#269259,#269260,#269261,
#269262,#269263,#269264,#269265,#269266,#269267,#269268,#269269,#269270,
#269271,#269272,#269273,#269274,#269275,#269276,#269277,#269278,#269279,
#269280,#269281,#269282,#269283,#269284,#269285,#269286,#269287,#269288,
#269289,#269290,#269291,#269292,#269293,#269294,#269295,#269296,#269297,
#269298,#269299,#269300,#269301,#269302,#269303,#269304,#269305,#269306,
#269307,#269308,#269309,#269310,#269311,#269312,#269313,#269314,#269315,
#269316,#269317,#269318,#269319,#269320,#269321,#269322,#269323,#269324,
#269325,#269326,#269327,#269328,#269329,#269330,#269331,#269332,#269333,
#269334,#269335,#269336,#269337,#269338,#269339,#269340,#269341,#269342,
#269343,#269344,#269345,#269346,#269347,#269348,#269349,#269350,#269351,
#269352,#269353,#269354,#269355,#269356,#269357,#269358,#269359,#269360,
#269361,#269362,#269363,#269364)),.UNSPECIFIED.,.F.,.F.,.F.,(2,2),(4,2,
2,2,2,2,2,2,2,2,2,2,2,2,2,2,2,2,2,2,2,2,2,2,2,2,2,2,2,2,2,2,2,2,2,2,2,2,
2,2,2,2,2,2,2,2,2,2,2,2,2,2,2,2,2,4),(0.,1.),(-0.000118831294053002,-4.84197060393493E-6,
0.000109147352845132,0.000337125999743267,0.000451115323192334,0.000565104646641402,
0.000679093970090469,0.000793083293539536,0.00102106194043767,0.00113505126388674,
0.0012490405873358,0.00136302991078487,0.00142002457250941,0.00147701923423394,
0.00170499788113207,0.00193297652803021,0.00204696585147928,0.00216095517492835,
0.00227494449837741,0.00238893382182648,0.00261691246872462,0.00284489111562275,
0.00290188577734728,0.00295888043907182,0.00307286976252088,0.00318685908596995,
0.00330084840941902,0.00341483773286809,0.00352882705631715,0.00364281637976622,
0.00375680570321528,0.00387079502666435,0.00398478435011342,0.00421276299701156,
0.00444074164390969,0.00466872029080782,0.00489669893770596,0.00512467758460409,
0.00518167224632863,0.00523866690805316,0.00535265623150223,0.0054666455549513,
0.00558063487840036,0.00569462420184943,0.0058086135252985,0.00592260284874756,
0.00603659217219663,0.0061505814956457,0.00626457081909477,0.0064925494659929,
0.00660653878944197,0.00672052811289104,0.0068345174363401,0.00694850675978917,
0.00706249608323824,0.00717648540668731),.UNSPECIFIED.);
#979=B_SPLINE_SURFACE_WITH_KNOTS('',1,3,((#269442,#269443,#269444,#269445,
#269446,#269447,#269448,#269449,#269450,#269451,#269452,#269453,#269454,
#269455,#269456,#269457,#269458,#269459,#269460),(#269461,#269462,#269463,
#269464,#269465,#269466,#269467,#269468,#269469,#269470,#269471,#269472,
#269473,#269474,#269475,#269476,#269477,#269478,#269479)),.UNSPECIFIED.,
 .F.,.F.,.F.,(2,2),(4,2,2,2,2,1,1,1,2,2,4),(0.,4.74723717073224),(0.013418536150584,
0.013445898196386,0.0135028928581105,0.0135598875198351,0.0136738768432841,
0.0137878661667332,0.0140158448136313,0.0141298341370804,0.0142438234605295,
0.0143578127839785,0.0144718021074276),.UNSPECIFIED.);
#980=B_SPLINE_SURFACE_WITH_KNOTS('',1,3,((#269481,#269482,#269483,#269484,
#269485,#269486,#269487,#269488,#269489,#269490,#269491,#269492,#269493,
#269494,#269495,#269496,#269497,#269498,#269499,#269500,#269501,#269502,
#269503,#269504,#269505,#269506,#269507,#269508,#269509,#269510,#269511,
#269512,#269513,#269514,#269515,#269516,#269517,#269518,#269519,#269520,
#269521,#269522,#269523,#269524,#269525,#269526,#269527,#269528,#269529,
#269530,#269531,#269532,#269533,#269534,#269535,#269536,#269537,#269538,
#269539,#269540,#269541,#269542,#269543,#269544,#269545,#269546,#269547,
#269548,#269549,#269550,#269551,#269552,#269553,#269554,#269555,#269556,
#269557,#269558,#269559,#269560,#269561,#269562,#269563,#269564,#269565,
#269566,#269567,#269568,#269569,#269570,#269571,#269572,#269573,#269574,
#269575,#269576,#269577,#269578,#269579,#269580,#269581,#269582,#269583,
#269584,#269585,#269586,#269587,#269588,#269589,#269590,#269591,#269592,
#269593,#269594,#269595,#269596,#269597,#269598,#269599,#269600,#269601,
#269602,#269603,#269604,#269605,#269606,#269607,#269608,#269609,#269610,
#269611,#269612,#269613,#269614,#269615,#269616,#269617,#269618,#269619,
#269620,#269621,#269622,#269623,#269624,#269625,#269626,#269627,#269628,
#269629,#269630,#269631,#269632,#269633,#269634,#269635,#269636,#269637,
#269638,#269639,#269640,#269641,#269642,#269643,#269644,#269645,#269646,
#269647,#269648,#269649,#269650,#269651,#269652,#269653,#269654,#269655,
#269656,#269657,#269658,#269659),(#269660,#269661,#269662,#269663,#269664,
#269665,#269666,#269667,#269668,#269669,#269670,#269671,#269672,#269673,
#269674,#269675,#269676,#269677,#269678,#269679,#269680,#269681,#269682,
#269683,#269684,#269685,#269686,#269687,#269688,#269689,#269690,#269691,
#269692,#269693,#269694,#269695,#269696,#269697,#269698,#269699,#269700,
#269701,#269702,#269703,#269704,#269705,#269706,#269707,#269708,#269709,
#269710,#269711,#269712,#269713,#269714,#269715,#269716,#269717,#269718,
#269719,#269720,#269721,#269722,#269723,#269724,#269725,#269726,#269727,
#269728,#269729,#269730,#269731,#269732,#269733,#269734,#269735,#269736,
#269737,#269738,#269739,#269740,#269741,#269742,#269743,#269744,#269745,
#269746,#269747,#269748,#269749,#269750,#269751,#269752,#269753,#269754,
#269755,#269756,#269757,#269758,#269759,#269760,#269761,#269762,#269763,
#269764,#269765,#269766,#269767,#269768,#269769,#269770,#269771,#269772,
#269773,#269774,#269775,#269776,#269777,#269778,#269779,#269780,#269781,
#269782,#269783,#269784,#269785,#269786,#269787,#269788,#269789,#269790,
#269791,#269792,#269793,#269794,#269795,#269796,#269797,#269798,#269799,
#269800,#269801,#269802,#269803,#269804,#269805,#269806,#269807,#269808,
#269809,#269810,#269811,#269812,#269813,#269814,#269815,#269816,#269817,
#269818,#269819,#269820,#269821,#269822,#269823,#269824,#269825,#269826,
#269827,#269828,#269829,#269830,#269831,#269832,#269833,#269834,#269835,
#269836,#269837,#269838)),.UNSPECIFIED.,.F.,.T.,.F.,(2,2),(4,1,1,2,2,2,
2,1,1,1,2,2,2,1,1,2,2,2,2,2,2,2,2,2,1,1,1,2,2,2,1,2,2,2,1,2,2,2,1,1,1,1,
2,2,2,1,1,1,1,2,2,2,2,2,2,2,1,1,2,2,2,2,1,2,2,2,1,1,2,2,2,2,2,2,2,2,2,2,
1,1,1,2,2,2,1,1,2,2,2,1,2,2,2,2,2,1,2,2,2,2,2,1,1,1,2,2,4),(0.,4.74723717073224),
(-0.000118831294053002,0.000109147352845132,0.000337125999743267,0.000451115323192334,
0.000565104646641402,0.000679093970090469,0.000793083293539536,0.00102106194043767,
0.00113505126388674,0.0012490405873358,0.00136302991078487,0.00142002457250941,
0.00147701923423394,0.00170499788113207,0.00193297652803021,0.00204696585147928,
0.00216095517492835,0.00227494449837741,0.00238893382182648,0.00261691246872462,
0.00284489111562275,0.00290188577734728,0.00295888043907182,0.00307286976252088,
0.00330084840941902,0.00341483773286809,0.00352882705631715,0.00364281637976622,
0.00375680570321528,0.00387079502666435,0.00398478435011342,0.00421276299701156,
0.00444074164390969,0.00466872029080782,0.00489669893770596,0.00512467758460409,
0.00518167224632863,0.00523866690805316,0.00535265623150223,0.0054666455549513,
0.00558063487840036,0.00569462420184943,0.0058086135252985,0.00592260284874756,
0.00603659217219663,0.0061505814956457,0.00626457081909477,0.0064925494659929,
0.00660653878944197,0.00672052811289104,0.0068345174363401,0.00694850675978917,
0.00717648540668731,0.00729047473013637,0.00740446405358544,0.00763244270048357,
0.00786042134738171,0.00797441067083078,0.00808839999427985,0.00820238931772891,
0.00831637864117798,0.00854435728807612,0.00877233593497425,0.00888632525842331,
0.00900031458187238,0.00911430390532145,0.00922829322877052,0.00945627187566865,
0.00957026119911772,0.00968425052256679,0.00974124518429132,0.00979823984601585,
0.00991222916946492,0.0101402078163631,0.0103681864632612,0.0104251811249857,
0.0104821757867103,0.0105961651101593,0.0108241437570575,0.0109381330805065,
0.0110521224039556,0.0111661117274047,0.0112801010508537,0.0113940903743028,
0.0115080796977519,0.01173605834465,0.0118500476680991,0.0119640369915481,
0.0120780263149972,0.0121920156384463,0.0124199942853444,0.0126479729322425,
0.0127049675939671,0.0127619622556916,0.0128759515791407,0.0131039302260388,
0.0133319088729369,0.013445898196386,0.0135028928581105,0.0135598875198351,
0.0136738768432841,0.0137878661667332,0.0140158448136313,0.0141298341370804,
0.0142438234605295,0.0143578127839785,0.0144718021074276),.UNSPECIFIED.);
#981=B_SPLINE_SURFACE_WITH_KNOTS('',1,3,((#269839,#269840,#269841,#269842,
#269843,#269844,#269845,#269846,#269847,#269848,#269849,#269850,#269851,
#269852,#269853,#269854,#269855,#269856,#269857,#269858,#269859,#269860,
#269861,#269862,#269863,#269864,#269865,#269866,#269867,#269868,#269869,
#269870,#269871,#269872,#269873,#269874,#269875,#269876,#269877,#269878,
#269879,#269880,#269881,#269882,#269883,#269884,#269885,#269886,#269887,
#269888,#269889,#269890,#269891,#269892,#269893,#269894,#269895,#269896,
#269897,#269898,#269899,#269900,#269901,#269902,#269903,#269904,#269905,
#269906,#269907,#269908,#269909,#269910,#269911,#269912,#269913,#269914,
#269915,#269916,#269917,#269918,#269919,#269920,#269921,#269922,#269923,
#269924,#269925,#269926,#269927,#269928,#269929,#269930,#269931,#269932,
#269933,#269934,#269935,#269936,#269937,#269938,#269939,#269940,#269941,
#269942,#269943,#269944,#269945,#269946,#269947,#269948,#269949,#269950,
#269951,#269952,#269953,#269954,#269955,#269956,#269957,#269958,#269959,
#269960,#269961,#269962,#269963,#269964,#269965,#269966,#269967,#269968,
#269969,#269970,#269971,#269972,#269973,#269974,#269975,#269976,#269977,
#269978,#269979,#269980,#269981,#269982,#269983,#269984,#269985,#269986,
#269987,#269988,#269989,#269990,#269991,#269992,#269993,#269994,#269995,
#269996,#269997,#269998,#269999,#270000,#270001,#270002,#270003,#270004,
#270005,#270006,#270007,#270008,#270009,#270010,#270011,#270012,#270013,
#270014,#270015,#270016,#270017,#270018,#270019,#270020,#270021,#270022,
#270023,#270024,#270025,#270026,#270027,#270028,#270029,#270030,#270031,
#270032,#270033,#270034,#270035,#270036,#270037,#270038,#270039,#270040,
#270041,#270042,#270043,#270044,#270045,#270046,#270047,#270048,#270049,
#270050,#270051,#270052,#270053,#270054,#270055,#270056,#270057,#270058,
#270059,#270060,#270061,#270062,#270063,#270064),(#270065,#270066,#270067,
#270068,#270069,#270070,#270071,#270072,#270073,#270074,#270075,#270076,
#270077,#270078,#270079,#270080,#270081,#270082,#270083,#270084,#270085,
#270086,#270087,#270088,#270089,#270090,#270091,#270092,#270093,#270094,
#270095,#270096,#270097,#270098,#270099,#270100,#270101,#270102,#270103,
#270104,#270105,#270106,#270107,#270108,#270109,#270110,#270111,#270112,
#270113,#270114,#270115,#270116,#270117,#270118,#270119,#270120,#270121,
#270122,#270123,#270124,#270125,#270126,#270127,#270128,#270129,#270130,
#270131,#270132,#270133,#270134,#270135,#270136,#270137,#270138,#270139,
#270140,#270141,#270142,#270143,#270144,#270145,#270146,#270147,#270148,
#270149,#270150,#270151,#270152,#270153,#270154,#270155,#270156,#270157,
#270158,#270159,#270160,#270161,#270162,#270163,#270164,#270165,#270166,
#270167,#270168,#270169,#270170,#270171,#270172,#270173,#270174,#270175,
#270176,#270177,#270178,#270179,#270180,#270181,#270182,#270183,#270184,
#270185,#270186,#270187,#270188,#270189,#270190,#270191,#270192,#270193,
#270194,#270195,#270196,#270197,#270198,#270199,#270200,#270201,#270202,
#270203,#270204,#270205,#270206,#270207,#270208,#270209,#270210,#270211,
#270212,#270213,#270214,#270215,#270216,#270217,#270218,#270219,#270220,
#270221,#270222,#270223,#270224,#270225,#270226,#270227,#270228,#270229,
#270230,#270231,#270232,#270233,#270234,#270235,#270236,#270237,#270238,
#270239,#270240,#270241,#270242,#270243,#270244,#270245,#270246,#270247,
#270248,#270249,#270250,#270251,#270252,#270253,#270254,#270255,#270256,
#270257,#270258,#270259,#270260,#270261,#270262,#270263,#270264,#270265,
#270266,#270267,#270268,#270269,#270270,#270271,#270272,#270273,#270274,
#270275,#270276,#270277,#270278,#270279,#270280,#270281,#270282,#270283,
#270284,#270285,#270286,#270287,#270288,#270289,#270290)),.UNSPECIFIED.,
 .F.,.T.,.F.,(2,2),(4,2,2,2,2,2,2,2,2,2,2,2,2,2,2,2,2,2,2,2,2,2,2,2,2,2,
2,2,2,2,2,2,2,2,2,2,2,2,2,2,2,2,2,2,2,2,2,2,2,2,2,2,2,2,2,2,2,2,2,2,2,2,
2,2,2,2,2,2,2,2,2,2,2,2,2,2,2,2,2,2,2,2,2,2,2,2,2,2,2,2,2,2,2,2,2,2,2,2,
2,2,2,2,2,2,2,2,2,2,2,2,2,2,4),(-1.67052866871372E-8,1.00000923646777),
(-0.000118831294053002,-4.84197060393493E-6,0.000109147352845132,0.000337125999743267,
0.000451115323192334,0.000565104646641402,0.000679093970090469,0.000793083293539536,
0.00102106194043767,0.00113505126388674,0.0012490405873358,0.00136302991078487,
0.00142002457250941,0.00147701923423394,0.00170499788113207,0.00193297652803021,
0.00204696585147928,0.00216095517492835,0.00227494449837741,0.00238893382182648,
0.00261691246872462,0.00284489111562275,0.00290188577734728,0.00295888043907182,
0.00307286976252088,0.00318685908596995,0.00330084840941902,0.00341483773286809,
0.00352882705631715,0.00364281637976622,0.00375680570321528,0.00387079502666435,
0.00398478435011342,0.00421276299701156,0.00444074164390969,0.00466872029080782,
0.00489669893770596,0.00512467758460409,0.00518167224632863,0.00523866690805316,
0.00535265623150223,0.0054666455549513,0.00558063487840036,0.00569462420184943,
0.0058086135252985,0.00592260284874756,0.00603659217219663,0.0061505814956457,
0.00626457081909477,0.0064925494659929,0.00660653878944197,0.00672052811289104,
0.0068345174363401,0.00694850675978917,0.00706249608323824,0.00717648540668731,
0.00729047473013637,0.00740446405358544,0.00763244270048357,0.00786042134738171,
0.00797441067083078,0.00808839999427985,0.00820238931772891,0.00831637864117798,
0.00854435728807612,0.00865834661152518,0.00877233593497425,0.00888632525842331,
0.00900031458187238,0.00911430390532145,0.00922829322877052,0.00945627187566865,
0.00957026119911772,0.00968425052256679,0.00974124518429132,0.00979823984601585,
0.00991222916946492,0.0101402078163631,0.0103681864632612,0.0104251811249857,
0.0104821757867103,0.0105961651101593,0.0107101544336084,0.0108241437570575,
0.0109381330805065,0.0110521224039556,0.0111661117274047,0.0112801010508537,
0.0113940903743028,0.0115080796977519,0.01173605834465,0.0118500476680991,
0.0119640369915481,0.0120780263149972,0.0121920156384463,0.0124199942853444,
0.0126479729322425,0.0127049675939671,0.0127619622556916,0.0128759515791407,
0.0129899409025897,0.0131039302260388,0.0133319088729369,0.013445898196386,
0.0135028928581105,0.0135598875198351,0.0136738768432841,0.0137878661667332,
0.0140158448136313,0.0141298341370804,0.0142438234605295,0.0143578127839785,
0.0144718021074276),.UNSPECIFIED.);
#982=B_SPLINE_SURFACE_WITH_KNOTS('',1,3,((#270358,#270359,#270360,#270361,
#270362,#270363,#270364,#270365,#270366,#270367,#270368,#270369,#270370,
#270371,#270372,#270373,#270374,#270375,#270376,#270377,#270378,#270379,
#270380,#270381,#270382,#270383,#270384,#270385,#270386,#270387,#270388,
#270389,#270390,#270391,#270392,#270393,#270394,#270395,#270396,#270397,
#270398,#270399,#270400,#270401,#270402,#270403,#270404,#270405,#270406,
#270407,#270408,#270409,#270410,#270411,#270412,#270413,#270414,#270415,
#270416,#270417,#270418,#270419,#270420,#270421,#270422,#270423,#270424,
#270425,#270426,#270427,#270428,#270429,#270430,#270431,#270432,#270433,
#270434,#270435,#270436,#270437,#270438,#270439,#270440,#270441,#270442,
#270443,#270444,#270445,#270446,#270447,#270448,#270449,#270450,#270451,
#270452,#270453,#270454,#270455,#270456,#270457,#270458,#270459,#270460,
#270461,#270462,#270463,#270464,#270465,#270466,#270467,#270468,#270469,
#270470,#270471,#270472,#270473,#270474,#270475,#270476,#270477,#270478,
#270479,#270480,#270481,#270482,#270483,#270484,#270485,#270486,#270487,
#270488,#270489,#270490,#270491,#270492,#270493,#270494,#270495,#270496,
#270497,#270498,#270499,#270500,#270501,#270502,#270503,#270504,#270505,
#270506,#270507,#270508,#270509,#270510,#270511,#270512,#270513,#270514,
#270515,#270516,#270517,#270518,#270519,#270520,#270521,#270522,#270523,
#270524,#270525,#270526,#270527,#270528,#270529,#270530,#270531,#270532,
#270533,#270534,#270535,#270536),(#270537,#270538,#270539,#270540,#270541,
#270542,#270543,#270544,#270545,#270546,#270547,#270548,#270549,#270550,
#270551,#270552,#270553,#270554,#270555,#270556,#270557,#270558,#270559,
#270560,#270561,#270562,#270563,#270564,#270565,#270566,#270567,#270568,
#270569,#270570,#270571,#270572,#270573,#270574,#270575,#270576,#270577,
#270578,#270579,#270580,#270581,#270582,#270583,#270584,#270585,#270586,
#270587,#270588,#270589,#270590,#270591,#270592,#270593,#270594,#270595,
#270596,#270597,#270598,#270599,#270600,#270601,#270602,#270603,#270604,
#270605,#270606,#270607,#270608,#270609,#270610,#270611,#270612,#270613,
#270614,#270615,#270616,#270617,#270618,#270619,#270620,#270621,#270622,
#270623,#270624,#270625,#270626,#270627,#270628,#270629,#270630,#270631,
#270632,#270633,#270634,#270635,#270636,#270637,#270638,#270639,#270640,
#270641,#270642,#270643,#270644,#270645,#270646,#270647,#270648,#270649,
#270650,#270651,#270652,#270653,#270654,#270655,#270656,#270657,#270658,
#270659,#270660,#270661,#270662,#270663,#270664,#270665,#270666,#270667,
#270668,#270669,#270670,#270671,#270672,#270673,#270674,#270675,#270676,
#270677,#270678,#270679,#270680,#270681,#270682,#270683,#270684,#270685,
#270686,#270687,#270688,#270689,#270690,#270691,#270692,#270693,#270694,
#270695,#270696,#270697,#270698,#270699,#270700,#270701,#270702,#270703,
#270704,#270705,#270706,#270707,#270708,#270709,#270710,#270711,#270712,
#270713,#270714,#270715)),.UNSPECIFIED.,.F.,.T.,.F.,(2,2),(4,1,1,2,2,2,
2,1,1,1,2,2,2,1,1,2,2,2,2,2,2,2,2,2,1,1,1,2,2,2,1,2,2,2,1,2,2,2,1,1,1,1,
2,2,2,1,1,1,1,2,2,2,2,2,2,2,1,1,2,2,2,2,1,2,2,2,1,1,2,2,2,2,2,2,2,2,2,2,
1,1,1,2,2,2,1,1,2,2,2,1,2,2,2,2,2,1,2,2,2,2,2,1,1,1,2,2,4),(0.,5.45368304321453),
(-0.000118831294053002,0.000109147352845132,0.000337125999743267,0.000451115323192334,
0.000565104646641402,0.000679093970090469,0.000793083293539536,0.00102106194043767,
0.00113505126388674,0.0012490405873358,0.00136302991078487,0.00142002457250941,
0.00147701923423394,0.00170499788113207,0.00193297652803021,0.00204696585147928,
0.00216095517492835,0.00227494449837741,0.00238893382182648,0.00261691246872462,
0.00284489111562275,0.00290188577734728,0.00295888043907182,0.00307286976252088,
0.00330084840941902,0.00341483773286809,0.00352882705631715,0.00364281637976622,
0.00375680570321528,0.00387079502666435,0.00398478435011342,0.00421276299701156,
0.00444074164390969,0.00466872029080782,0.00489669893770596,0.00512467758460409,
0.00518167224632863,0.00523866690805316,0.00535265623150223,0.0054666455549513,
0.00558063487840036,0.00569462420184943,0.0058086135252985,0.00592260284874756,
0.00603659217219663,0.0061505814956457,0.00626457081909477,0.0064925494659929,
0.00660653878944197,0.00672052811289104,0.0068345174363401,0.00694850675978917,
0.00717648540668731,0.00729047473013637,0.00740446405358544,0.00763244270048357,
0.00786042134738171,0.00797441067083078,0.00808839999427985,0.00820238931772891,
0.00831637864117798,0.00854435728807612,0.00877233593497425,0.00888632525842331,
0.00900031458187238,0.00911430390532145,0.00922829322877052,0.00945627187566865,
0.00957026119911772,0.00968425052256679,0.00974124518429132,0.00979823984601585,
0.00991222916946492,0.0101402078163631,0.0103681864632612,0.0104251811249857,
0.0104821757867103,0.0105961651101593,0.0108241437570575,0.0109381330805065,
0.0110521224039556,0.0111661117274047,0.0112801010508537,0.0113940903743028,
0.0115080796977519,0.01173605834465,0.0118500476680991,0.0119640369915481,
0.0120780263149972,0.0121920156384463,0.0124199942853444,0.0126479729322425,
0.0127049675939671,0.0127619622556916,0.0128759515791407,0.0131039302260388,
0.0133319088729369,0.013445898196386,0.0135028928581105,0.0135598875198351,
0.0136738768432841,0.0137878661667332,0.0140158448136313,0.0141298341370804,
0.0142438234605295,0.0143578127839785,0.0144718021074276),.UNSPECIFIED.);
#983=B_SPLINE_SURFACE_WITH_KNOTS('',1,3,((#270716,#270717,#270718,#270719,
#270720,#270721,#270722,#270723,#270724,#270725,#270726,#270727,#270728,
#270729,#270730,#270731,#270732,#270733,#270734,#270735,#270736,#270737,
#270738,#270739,#270740,#270741,#270742,#270743,#270744,#270745,#270746,
#270747,#270748,#270749,#270750,#270751,#270752,#270753,#270754,#270755,
#270756,#270757,#270758,#270759,#270760,#270761,#270762,#270763,#270764,
#270765,#270766,#270767,#270768,#270769,#270770,#270771,#270772,#270773,
#270774,#270775,#270776,#270777,#270778,#270779,#270780,#270781,#270782,
#270783,#270784,#270785,#270786,#270787,#270788,#270789,#270790,#270791,
#270792,#270793,#270794,#270795,#270796,#270797,#270798,#270799,#270800,
#270801,#270802,#270803,#270804,#270805,#270806,#270807,#270808,#270809,
#270810,#270811,#270812,#270813,#270814,#270815,#270816,#270817,#270818,
#270819,#270820,#270821,#270822,#270823,#270824,#270825,#270826,#270827,
#270828,#270829,#270830,#270831,#270832,#270833,#270834,#270835,#270836,
#270837,#270838,#270839,#270840,#270841,#270842,#270843,#270844,#270845,
#270846,#270847,#270848,#270849,#270850,#270851,#270852,#270853,#270854,
#270855,#270856,#270857,#270858,#270859,#270860,#270861,#270862,#270863,
#270864,#270865,#270866,#270867,#270868,#270869,#270870,#270871,#270872,
#270873,#270874,#270875,#270876,#270877,#270878,#270879,#270880,#270881,
#270882,#270883,#270884,#270885,#270886,#270887,#270888,#270889,#270890,
#270891,#270892,#270893,#270894),(#270895,#270896,#270897,#270898,#270899,
#270900,#270901,#270902,#270903,#270904,#270905,#270906,#270907,#270908,
#270909,#270910,#270911,#270912,#270913,#270914,#270915,#270916,#270917,
#270918,#270919,#270920,#270921,#270922,#270923,#270924,#270925,#270926,
#270927,#270928,#270929,#270930,#270931,#270932,#270933,#270934,#270935,
#270936,#270937,#270938,#270939,#270940,#270941,#270942,#270943,#270944,
#270945,#270946,#270947,#270948,#270949,#270950,#270951,#270952,#270953,
#270954,#270955,#270956,#270957,#270958,#270959,#270960,#270961,#270962,
#270963,#270964,#270965,#270966,#270967,#270968,#270969,#270970,#270971,
#270972,#270973,#270974,#270975,#270976,#270977,#270978,#270979,#270980,
#270981,#270982,#270983,#270984,#270985,#270986,#270987,#270988,#270989,
#270990,#270991,#270992,#270993,#270994,#270995,#270996,#270997,#270998,
#270999,#271000,#271001,#271002,#271003,#271004,#271005,#271006,#271007,
#271008,#271009,#271010,#271011,#271012,#271013,#271014,#271015,#271016,
#271017,#271018,#271019,#271020,#271021,#271022,#271023,#271024,#271025,
#271026,#271027,#271028,#271029,#271030,#271031,#271032,#271033,#271034,
#271035,#271036,#271037,#271038,#271039,#271040,#271041,#271042,#271043,
#271044,#271045,#271046,#271047,#271048,#271049,#271050,#271051,#271052,
#271053,#271054,#271055,#271056,#271057,#271058,#271059,#271060,#271061,
#271062,#271063,#271064,#271065,#271066,#271067,#271068,#271069,#271070,
#271071,#271072,#271073)),.UNSPECIFIED.,.F.,.T.,.F.,(2,2),(4,1,1,2,2,2,
2,1,1,1,2,2,2,1,1,2,2,2,2,2,2,2,2,2,1,1,1,2,2,2,1,2,2,2,1,2,2,2,1,1,1,1,
2,2,2,1,1,1,1,2,2,2,2,2,2,2,1,1,2,2,2,2,1,2,2,2,1,1,2,2,2,2,2,2,2,2,2,2,
1,1,1,2,2,2,1,1,2,2,2,1,2,2,2,2,2,1,2,2,2,2,2,1,1,1,2,2,4),(0.,5.45368304321453),
(-0.000118831294053002,0.000109147352845132,0.000337125999743267,0.000451115323192334,
0.000565104646641402,0.000679093970090469,0.000793083293539536,0.00102106194043767,
0.00113505126388674,0.0012490405873358,0.00136302991078487,0.00142002457250941,
0.00147701923423394,0.00170499788113207,0.00193297652803021,0.00204696585147928,
0.00216095517492835,0.00227494449837741,0.00238893382182648,0.00261691246872462,
0.00284489111562275,0.00290188577734728,0.00295888043907182,0.00307286976252088,
0.00330084840941902,0.00341483773286809,0.00352882705631715,0.00364281637976622,
0.00375680570321528,0.00387079502666435,0.00398478435011342,0.00421276299701156,
0.00444074164390969,0.00466872029080782,0.00489669893770596,0.00512467758460409,
0.00518167224632863,0.00523866690805316,0.00535265623150223,0.0054666455549513,
0.00558063487840036,0.00569462420184943,0.0058086135252985,0.00592260284874756,
0.00603659217219663,0.0061505814956457,0.00626457081909477,0.0064925494659929,
0.00660653878944197,0.00672052811289104,0.0068345174363401,0.00694850675978917,
0.00717648540668731,0.00729047473013637,0.00740446405358544,0.00763244270048357,
0.00786042134738171,0.00797441067083078,0.00808839999427985,0.00820238931772891,
0.00831637864117798,0.00854435728807612,0.00877233593497425,0.00888632525842331,
0.00900031458187238,0.00911430390532145,0.00922829322877052,0.00945627187566865,
0.00957026119911772,0.00968425052256679,0.00974124518429132,0.00979823984601585,
0.00991222916946492,0.0101402078163631,0.0103681864632612,0.0104251811249857,
0.0104821757867103,0.0105961651101593,0.0108241437570575,0.0109381330805065,
0.0110521224039556,0.0111661117274047,0.0112801010508537,0.0113940903743028,
0.0115080796977519,0.01173605834465,0.0118500476680991,0.0119640369915481,
0.0120780263149972,0.0121920156384463,0.0124199942853444,0.0126479729322425,
0.0127049675939671,0.0127619622556916,0.0128759515791407,0.0131039302260388,
0.0133319088729369,0.013445898196386,0.0135028928581105,0.0135598875198351,
0.0136738768432841,0.0137878661667332,0.0140158448136313,0.0141298341370804,
0.0142438234605295,0.0143578127839785,0.0144718021074276),.UNSPECIFIED.);
#1016=SPHERICAL_SURFACE('',#95826,0.5);
#1017=SPHERICAL_SURFACE('',#96300,0.5);
#1018=SPHERICAL_SURFACE('',#97991,0.5);
#1019=SPHERICAL_SURFACE('',#98013,0.5);
#1020=SPHERICAL_SURFACE('',#98021,0.5);
#1021=SPHERICAL_SURFACE('',#98031,0.5);
#1022=SPHERICAL_SURFACE('',#99893,0.5);
#1023=SPHERICAL_SURFACE('',#99915,0.5);
#1024=SPHERICAL_SURFACE('',#99923,0.5);
#1025=SPHERICAL_SURFACE('',#99933,0.5);
#1026=SPHERICAL_SURFACE('',#101999,20.36);
#1027=SPHERICAL_SURFACE('',#102137,20.36);
#1028=SPHERICAL_SURFACE('',#102743,0.75);
#1029=SPHERICAL_SURFACE('',#102749,0.75);
#1030=SPHERICAL_SURFACE('',#102756,0.75);
#1031=SPHERICAL_SURFACE('',#102764,0.75);
#1032=SPHERICAL_SURFACE('',#102790,0.75);
#1033=SPHERICAL_SURFACE('',#102796,0.75);
#1034=SPHERICAL_SURFACE('',#102803,0.75);
#1035=SPHERICAL_SURFACE('',#102811,0.75);
#1036=SPHERICAL_SURFACE('',#103151,1.);
#1037=SPHERICAL_SURFACE('',#103161,1.);
#1038=SPHERICAL_SURFACE('',#103323,10.);
#1039=SPHERICAL_SURFACE('',#103325,10.);
#1068=(
BOUNDED_CURVE()
B_SPLINE_CURVE(3,(#134716,#134717,#134718,#134719,#134720,#134721),
 .UNSPECIFIED.,.F.,.F.)
B_SPLINE_CURVE_WITH_KNOTS((4,2,4),(0.,0.5,1.),.UNSPECIFIED.)
CURVE()
GEOMETRIC_REPRESENTATION_ITEM()
RATIONAL_B_SPLINE_CURVE((0.999999968420324,0.999999972427659,0.999999976025392,
0.999999982652427,0.99999998567993,0.999999988486397))
REPRESENTATION_ITEM('')
);
#1069=(
BOUNDED_CURVE()
B_SPLINE_CURVE(3,(#135210,#135211,#135212,#135213,#135214,#135215,#135216,
#135217,#135218,#135219,#135220,#135221,#135222,#135223),.UNSPECIFIED.,
 .F.,.F.)
B_SPLINE_CURVE_WITH_KNOTS((4,2,2,2,2,2,4),(0.,0.0419812889255314,0.201651074104609,
0.361320859283688,0.520990644462766,0.680660429641844,1.),.UNSPECIFIED.)
CURVE()
GEOMETRIC_REPRESENTATION_ITEM()
RATIONAL_B_SPLINE_CURVE((0.999998374495664,0.999998374493274,0.999998374583376,
0.999998375464702,0.999998377524268,0.999998384150543,0.999998388666334,
0.999998400123408,0.999998406847051,0.999998422090857,0.99999843067397,
0.999998457730094,0.999998478258162,0.999998498329814))
REPRESENTATION_ITEM('')
);
#1070=(
BOUNDED_CURVE()
B_SPLINE_CURVE(3,(#135565,#135566,#135567,#135568,#135569,#135570,#135571,
#135572,#135573,#135574),.UNSPECIFIED.,.F.,.F.)
B_SPLINE_CURVE_WITH_KNOTS((4,2,2,2,4),(4.71238898038469,5.10508806208341,
5.49778714378214,5.89048622548086,6.28318530717959),.UNSPECIFIED.)
CURVE()
GEOMETRIC_REPRESENTATION_ITEM()
RATIONAL_B_SPLINE_CURVE((1.,1.,1.,1.,1.,1.,1.,1.,1.,1.))
REPRESENTATION_ITEM('')
);
#1071=(
BOUNDED_CURVE()
B_SPLINE_CURVE(3,(#136470,#136471,#136472,#136473,#136474,#136475,#136476,
#136477,#136478,#136479),.UNSPECIFIED.,.F.,.F.)
B_SPLINE_CURVE_WITH_KNOTS((4,2,2,2,4),(0.,0.245429606613382,0.496953071075587,
0.748476535537792,1.),.UNSPECIFIED.)
CURVE()
GEOMETRIC_REPRESENTATION_ITEM()
RATIONAL_B_SPLINE_CURVE((0.999999984853823,0.999999984852031,0.99999998484993,
0.999999984845045,0.999999984842238,0.999999984836252,0.999999984832989,
0.999999984826274,0.999999984822825,0.99999998481928))
REPRESENTATION_ITEM('')
);
#1072=(
BOUNDED_CURVE()
B_SPLINE_CURVE(3,(#136618,#136619,#136620,#136621),.UNSPECIFIED.,.F.,.F.)
B_SPLINE_CURVE_WITH_KNOTS((4,4),(0.,0.038317388945353),.UNSPECIFIED.)
CURVE()
GEOMETRIC_REPRESENTATION_ITEM()
RATIONAL_B_SPLINE_CURVE((1.,1.,1.,1.))
REPRESENTATION_ITEM('')
);
#1073=(
BOUNDED_CURVE()
B_SPLINE_CURVE(3,(#136629,#136630,#136631,#136632),.UNSPECIFIED.,.F.,.F.)
B_SPLINE_CURVE_WITH_KNOTS((4,4),(0.,0.0385835973699829),.UNSPECIFIED.)
CURVE()
GEOMETRIC_REPRESENTATION_ITEM()
RATIONAL_B_SPLINE_CURVE((1.,1.,1.,1.))
REPRESENTATION_ITEM('')
);
#1074=(
BOUNDED_CURVE()
B_SPLINE_CURVE(3,(#136756,#136757,#136758,#136759),.UNSPECIFIED.,.F.,.F.)
B_SPLINE_CURVE_WITH_KNOTS((4,4),(0.,0.0372541843113205),.UNSPECIFIED.)
CURVE()
GEOMETRIC_REPRESENTATION_ITEM()
RATIONAL_B_SPLINE_CURVE((1.,1.,1.,1.))
REPRESENTATION_ITEM('')
);
#1075=(
BOUNDED_CURVE()
B_SPLINE_CURVE(3,(#136790,#136791,#136792,#136793),.UNSPECIFIED.,.F.,.F.)
B_SPLINE_CURVE_WITH_KNOTS((4,4),(0.,0.0369876550821707),.UNSPECIFIED.)
CURVE()
GEOMETRIC_REPRESENTATION_ITEM()
RATIONAL_B_SPLINE_CURVE((1.,1.,1.,1.))
REPRESENTATION_ITEM('')
);
#1076=(
BOUNDED_CURVE()
B_SPLINE_CURVE(3,(#136837,#136838,#136839,#136840,#136841,#136842,#136843,
#136844,#136845,#136846,#136847,#136848,#136849,#136850),.UNSPECIFIED.,
 .F.,.F.)
B_SPLINE_CURVE_WITH_KNOTS((4,2,2,2,2,2,4),(0.,0.245468499204218,0.371223749336846,
0.496978999469476,0.622734249602107,0.748489499734738,1.),.UNSPECIFIED.)
CURVE()
GEOMETRIC_REPRESENTATION_ITEM()
RATIONAL_B_SPLINE_CURVE((0.99999993495641,0.999999935048577,0.999999935181178,
0.999999935424418,0.999999935514307,0.999999935708972,0.999999935814682,
0.999999936034834,0.999999936149644,0.999999936388505,0.999999936513549,
0.999999936895779,0.999999937156295,0.999999937422256))
REPRESENTATION_ITEM('')
);
#1077=(
BOUNDED_CURVE()
B_SPLINE_CURVE(3,(#137033,#137034,#137035,#137036),.UNSPECIFIED.,.F.,.F.)
B_SPLINE_CURVE_WITH_KNOTS((4,4),(0.,0.0358270578054484),.UNSPECIFIED.)
CURVE()
GEOMETRIC_REPRESENTATION_ITEM()
RATIONAL_B_SPLINE_CURVE((1.,1.,1.,1.))
REPRESENTATION_ITEM('')
);
#1078=(
BOUNDED_CURVE()
B_SPLINE_CURVE(3,(#137068,#137069,#137070,#137071),.UNSPECIFIED.,.F.,.F.)
B_SPLINE_CURVE_WITH_KNOTS((4,4),(0.,0.0360938777358061),.UNSPECIFIED.)
CURVE()
GEOMETRIC_REPRESENTATION_ITEM()
RATIONAL_B_SPLINE_CURVE((1.,1.,1.,1.))
REPRESENTATION_ITEM('')
);
#1079=(
BOUNDED_CURVE()
B_SPLINE_CURVE(3,(#137082,#137083,#137084,#137085),.UNSPECIFIED.,.F.,.F.)
B_SPLINE_CURVE_WITH_KNOTS((4,4),(0.,1.),.UNSPECIFIED.)
CURVE()
GEOMETRIC_REPRESENTATION_ITEM()
RATIONAL_B_SPLINE_CURVE((0.999999995222607,0.999999995303701,0.999999995402298,
0.999999995544337))
REPRESENTATION_ITEM('')
);
#1080=(
BOUNDED_CURVE()
B_SPLINE_CURVE(3,(#137248,#137249,#137250,#137251),.UNSPECIFIED.,.F.,.F.)
B_SPLINE_CURVE_WITH_KNOTS((4,4),(0.,1.),.UNSPECIFIED.)
CURVE()
GEOMETRIC_REPRESENTATION_ITEM()
RATIONAL_B_SPLINE_CURVE((0.999999920677172,0.999999923035118,0.999999925829014,
0.999999929482952))
REPRESENTATION_ITEM('')
);
#1081=(
BOUNDED_CURVE()
B_SPLINE_CURVE(3,(#137464,#137465,#137466,#137467),.UNSPECIFIED.,.F.,.F.)
B_SPLINE_CURVE_WITH_KNOTS((4,4),(0.,1.),.UNSPECIFIED.)
CURVE()
GEOMETRIC_REPRESENTATION_ITEM()
RATIONAL_B_SPLINE_CURVE((0.999999954619029,0.999999952528045,0.999999951009961,
0.999999949748637))
REPRESENTATION_ITEM('')
);
#1082=(
BOUNDED_CURVE()
B_SPLINE_CURVE(3,(#137900,#137901,#137902,#137903),.UNSPECIFIED.,.F.,.F.)
B_SPLINE_CURVE_WITH_KNOTS((4,4),(-1.38777878078145E-17,0.0332202089949022),
 .UNSPECIFIED.)
CURVE()
GEOMETRIC_REPRESENTATION_ITEM()
RATIONAL_B_SPLINE_CURVE((1.,1.,1.,1.))
REPRESENTATION_ITEM('')
);
#1083=(
BOUNDED_CURVE()
B_SPLINE_CURVE(3,(#137941,#137942,#137943,#137944,#137945,#137946,#137947,
#137948,#137949,#137950,#137951,#137952),.UNSPECIFIED.,.F.,.F.)
B_SPLINE_CURVE_WITH_KNOTS((4,2,2,2,2,4),(0.,0.244321743484906,0.496214495656607,
0.622160871742453,0.748107247828304,1.),.UNSPECIFIED.)
CURVE()
GEOMETRIC_REPRESENTATION_ITEM()
RATIONAL_B_SPLINE_CURVE((0.999999971111316,0.999999971052111,0.999999970982043,
0.999999970817943,0.99999997072254,0.999999970569587,0.999999970516657,
0.999999970406767,0.999999970349674,0.999999970177141,0.999999970058889,
0.999999969937273))
REPRESENTATION_ITEM('')
);
#1084=(
BOUNDED_CURVE()
B_SPLINE_CURVE(3,(#138175,#138176,#138177,#138178,#138179,#138180),
 .UNSPECIFIED.,.F.,.F.)
B_SPLINE_CURVE_WITH_KNOTS((4,2,4),(0.,0.5,1.),.UNSPECIFIED.)
CURVE()
GEOMETRIC_REPRESENTATION_ITEM()
RATIONAL_B_SPLINE_CURVE((0.999999994912409,0.999999994848392,0.999999994777208,
0.999999994613678,0.999999994521381,0.999999994413334))
REPRESENTATION_ITEM('')
);
#1085=(
BOUNDED_CURVE()
B_SPLINE_CURVE(3,(#138365,#138366,#138367,#138368),.UNSPECIFIED.,.F.,.F.)
B_SPLINE_CURVE_WITH_KNOTS((4,4),(0.,1.),.UNSPECIFIED.)
CURVE()
GEOMETRIC_REPRESENTATION_ITEM()
RATIONAL_B_SPLINE_CURVE((0.999999987573952,0.999999987041702,0.999999986704629,
0.99999998643111))
REPRESENTATION_ITEM('')
);
#1086=(
BOUNDED_CURVE()
B_SPLINE_CURVE(3,(#138745,#138746,#138747,#138748),.UNSPECIFIED.,.F.,.F.)
B_SPLINE_CURVE_WITH_KNOTS((4,4),(0.,0.0430361525536219),.UNSPECIFIED.)
CURVE()
GEOMETRIC_REPRESENTATION_ITEM()
RATIONAL_B_SPLINE_CURVE((1.,1.,1.,1.))
REPRESENTATION_ITEM('')
);
#1087=(
BOUNDED_CURVE()
B_SPLINE_CURVE(3,(#138780,#138781,#138782,#138783),.UNSPECIFIED.,.F.,.F.)
B_SPLINE_CURVE_WITH_KNOTS((4,4),(-2.77555756156289E-17,0.0433026927553429),
 .UNSPECIFIED.)
CURVE()
GEOMETRIC_REPRESENTATION_ITEM()
RATIONAL_B_SPLINE_CURVE((1.,1.,1.,1.))
REPRESENTATION_ITEM('')
);
#1088=(
BOUNDED_CURVE()
B_SPLINE_CURVE(3,(#138796,#138797,#138798,#138799),.UNSPECIFIED.,.F.,.F.)
B_SPLINE_CURVE_WITH_KNOTS((4,4),(0.,1.),.UNSPECIFIED.)
CURVE()
GEOMETRIC_REPRESENTATION_ITEM()
RATIONAL_B_SPLINE_CURVE((0.999999999134233,0.999999999123191,0.999999999109547,
0.999999999086375))
REPRESENTATION_ITEM('')
);
#1089=(
BOUNDED_CURVE()
B_SPLINE_CURVE(3,(#138882,#138883,#138884,#138885),.UNSPECIFIED.,.F.,.F.)
B_SPLINE_CURVE_WITH_KNOTS((4,4),(0.,0.044753309356401),.UNSPECIFIED.)
CURVE()
GEOMETRIC_REPRESENTATION_ITEM()
RATIONAL_B_SPLINE_CURVE((1.,1.,1.,1.))
REPRESENTATION_ITEM('')
);
#1090=(
BOUNDED_CURVE()
B_SPLINE_CURVE(3,(#138892,#138893,#138894,#138895),.UNSPECIFIED.,.F.,.F.)
B_SPLINE_CURVE_WITH_KNOTS((4,4),(0.,0.0444870989094409),.UNSPECIFIED.)
CURVE()
GEOMETRIC_REPRESENTATION_ITEM()
RATIONAL_B_SPLINE_CURVE((1.,1.,1.,1.))
REPRESENTATION_ITEM('')
);
#1091=(
BOUNDED_CURVE()
B_SPLINE_CURVE(3,(#138927,#138928,#138929,#138930,#138931,#138932,#138933,
#138934,#138935,#138936),.UNSPECIFIED.,.F.,.F.)
B_SPLINE_CURVE_WITH_KNOTS((4,2,2,2,4),(0.,0.245398115008223,0.49693207667215,
0.748466038336073,1.),.UNSPECIFIED.)
CURVE()
GEOMETRIC_REPRESENTATION_ITEM()
RATIONAL_B_SPLINE_CURVE((0.999999977858779,0.999999977854974,0.999999977850512,
0.999999977840136,0.999999977834171,0.999999977821454,0.999999977814521,
0.999999977800252,0.999999977792922,0.999999977785388))
REPRESENTATION_ITEM('')
);
#1092=(
BOUNDED_CURVE()
B_SPLINE_CURVE(3,(#138951,#138952,#138953,#138954,#138955,#138956,#138957,
#138958,#138959,#138960),.UNSPECIFIED.,.F.,.F.)
B_SPLINE_CURVE_WITH_KNOTS((4,2,2,2,4),(0.,0.251502574391383,0.503005148782772,
0.754507723174155,1.),.UNSPECIFIED.)
CURVE()
GEOMETRIC_REPRESENTATION_ITEM()
RATIONAL_B_SPLINE_CURVE((0.999999995351172,0.999999995351771,0.999999995352353,
0.999999995353486,0.999999995354037,0.999999995355048,0.999999995355522,
0.999999995356347,0.999999995356702,0.999999995357005))
REPRESENTATION_ITEM('')
);
#1093=(
BOUNDED_CURVE()
B_SPLINE_CURVE(3,(#139039,#139040,#139041,#139042),.UNSPECIFIED.,.F.,.F.)
B_SPLINE_CURVE_WITH_KNOTS((4,4),(0.,0.0445045070401677),.UNSPECIFIED.)
CURVE()
GEOMETRIC_REPRESENTATION_ITEM()
RATIONAL_B_SPLINE_CURVE((1.,1.,1.,1.))
REPRESENTATION_ITEM('')
);
#1094=(
BOUNDED_CURVE()
B_SPLINE_CURVE(3,(#139088,#139089,#139090,#139091,#139092,#139093,#139094,
#139095),.UNSPECIFIED.,.F.,.F.)
B_SPLINE_CURVE_WITH_KNOTS((4,2,2,4),(0.,0.233211998637451,0.490844615148963,
1.),.UNSPECIFIED.)
CURVE()
GEOMETRIC_REPRESENTATION_ITEM()
RATIONAL_B_SPLINE_CURVE((0.999999996506968,0.999999996496103,0.99999999647882,
0.999999996429016,0.999999996394958,0.999999996273789,0.999999996166972,
0.999999996039415))
REPRESENTATION_ITEM('')
);
#1095=(
BOUNDED_CURVE()
B_SPLINE_CURVE(3,(#139100,#139101,#139102,#139103),.UNSPECIFIED.,.F.,.F.)
B_SPLINE_CURVE_WITH_KNOTS((4,4),(0.,1.),.UNSPECIFIED.)
CURVE()
GEOMETRIC_REPRESENTATION_ITEM()
RATIONAL_B_SPLINE_CURVE((0.999999998576403,0.999999998611592,0.999999998632289,
0.999999998649038))
REPRESENTATION_ITEM('')
);
#1096=(
BOUNDED_CURVE()
B_SPLINE_CURVE(3,(#139203,#139204,#139205,#139206),.UNSPECIFIED.,.F.,.F.)
B_SPLINE_CURVE_WITH_KNOTS((4,4),(0.,0.0433970829567688),.UNSPECIFIED.)
CURVE()
GEOMETRIC_REPRESENTATION_ITEM()
RATIONAL_B_SPLINE_CURVE((1.,1.,1.,1.))
REPRESENTATION_ITEM('')
);
#1097=(
BOUNDED_CURVE()
B_SPLINE_CURVE(3,(#139237,#139238,#139239,#139240),.UNSPECIFIED.,.F.,.F.)
B_SPLINE_CURVE_WITH_KNOTS((4,4),(-1.38777878078145E-17,0.0431305646498159),
 .UNSPECIFIED.)
CURVE()
GEOMETRIC_REPRESENTATION_ITEM()
RATIONAL_B_SPLINE_CURVE((1.,1.,1.,1.))
REPRESENTATION_ITEM('')
);
#1098=(
BOUNDED_CURVE()
B_SPLINE_CURVE(3,(#139284,#139285,#139286,#139287,#139288,#139289,#139290,
#139291,#139292,#139293,#139294,#139295,#139296,#139297),.UNSPECIFIED.,
 .F.,.F.)
B_SPLINE_CURVE_WITH_KNOTS((4,2,2,2,2,2,4),(0.,0.245486421447413,0.371238684539511,
0.496990947631609,0.622743210723706,0.748495473815804,1.),.UNSPECIFIED.)
CURVE()
GEOMETRIC_REPRESENTATION_ITEM()
RATIONAL_B_SPLINE_CURVE((0.999999936096482,0.999999936209566,0.999999936365119,
0.999999936644208,0.999999936746728,0.999999936967832,0.999999937086967,
0.999999937333646,0.999999937462032,0.999999937728739,0.999999937868259,
0.999999938292486,0.99999993858141,0.99999993887622))
REPRESENTATION_ITEM('')
);
#1099=(
BOUNDED_CURVE()
B_SPLINE_CURVE(3,(#139524,#139525,#139526,#139527),.UNSPECIFIED.,.F.,.F.)
B_SPLINE_CURVE_WITH_KNOTS((4,4),(0.,1.),.UNSPECIFIED.)
CURVE()
GEOMETRIC_REPRESENTATION_ITEM()
RATIONAL_B_SPLINE_CURVE((0.999999988352499,0.999999988581759,0.999999988864347,
0.999999989311818))
REPRESENTATION_ITEM('')
);
#1100=(
BOUNDED_CURVE()
B_SPLINE_CURVE(3,(#139703,#139704,#139705,#139706,#139707,#139708),
 .UNSPECIFIED.,.F.,.F.)
B_SPLINE_CURVE_WITH_KNOTS((4,2,4),(0.,0.500000000000001,1.),
 .UNSPECIFIED.)
CURVE()
GEOMETRIC_REPRESENTATION_ITEM()
RATIONAL_B_SPLINE_CURVE((0.999999994872226,0.999999994962405,0.999999995062978,
0.999999995295095,0.999999995426566,0.999999995581248))
REPRESENTATION_ITEM('')
);
#1101=(
BOUNDED_CURVE()
B_SPLINE_CURVE(3,(#139709,#139710,#139711,#139712,#139713,#139714),
 .UNSPECIFIED.,.F.,.F.)
B_SPLINE_CURVE_WITH_KNOTS((4,2,4),(0.,0.5,1.),.UNSPECIFIED.)
CURVE()
GEOMETRIC_REPRESENTATION_ITEM()
RATIONAL_B_SPLINE_CURVE((0.999999988435972,0.999999988660851,0.999999988852627,
0.999999989192075,0.999999989339638,0.999999989472243))
REPRESENTATION_ITEM('')
);
#1102=(
BOUNDED_CURVE()
B_SPLINE_CURVE(3,(#139852,#139853,#139854,#139855,#139856,#139857,#139858,
#139859,#139860,#139861),.UNSPECIFIED.,.F.,.F.)
B_SPLINE_CURVE_WITH_KNOTS((4,2,2,2,4),(1.18015353016497E-15,0.392699081698726,
0.785398163397449,1.17809724509617,1.5707963267949),.UNSPECIFIED.)
CURVE()
GEOMETRIC_REPRESENTATION_ITEM()
RATIONAL_B_SPLINE_CURVE((1.,1.,1.,1.,1.,1.,1.,1.,1.,1.))
REPRESENTATION_ITEM('')
);
#1103=(
BOUNDED_CURVE()
B_SPLINE_CURVE(3,(#139894,#139895,#139896,#139897,#139898,#139899,#139900,
#139901,#139902,#139903),.UNSPECIFIED.,.F.,.F.)
B_SPLINE_CURVE_WITH_KNOTS((4,2,2,2,4),(4.71238898038469,5.10508806208341,
5.49778714378214,5.89048622548086,6.28318530717959),.UNSPECIFIED.)
CURVE()
GEOMETRIC_REPRESENTATION_ITEM()
RATIONAL_B_SPLINE_CURVE((1.,1.,1.,1.,1.,1.,1.,1.,1.,1.))
REPRESENTATION_ITEM('')
);
#1104=(
BOUNDED_CURVE()
B_SPLINE_CURVE(3,(#139907,#139908,#139909,#139910,#139911,#139912,#139913,
#139914,#139915,#139916),.UNSPECIFIED.,.F.,.F.)
B_SPLINE_CURVE_WITH_KNOTS((4,2,2,2,4),(1.5707963267949,1.96349540849362,
2.35619449019234,2.74889357189107,3.1415926535898),.UNSPECIFIED.)
CURVE()
GEOMETRIC_REPRESENTATION_ITEM()
RATIONAL_B_SPLINE_CURVE((1.,1.,1.,1.,1.,1.,1.,1.,1.,1.))
REPRESENTATION_ITEM('')
);
#1105=(
BOUNDED_CURVE()
B_SPLINE_CURVE(3,(#140064,#140065,#140066,#140067,#140068,#140069,#140070,
#140071,#140072,#140073),.UNSPECIFIED.,.F.,.F.)
B_SPLINE_CURVE_WITH_KNOTS((4,2,2,2,4),(3.1415926535898,3.53429173528852,
3.92699081698724,4.31968989868597,4.71238898038469),.UNSPECIFIED.)
CURVE()
GEOMETRIC_REPRESENTATION_ITEM()
RATIONAL_B_SPLINE_CURVE((1.,1.,1.,1.,1.,1.,1.,1.,1.,1.))
REPRESENTATION_ITEM('')
);
#1106=(
BOUNDED_CURVE()
B_SPLINE_CURVE(3,(#140084,#140085,#140086,#140087,#140088,#140089,#140090,
#140091,#140092,#140093),.UNSPECIFIED.,.F.,.F.)
B_SPLINE_CURVE_WITH_KNOTS((4,2,2,2,4),(4.71238898038469,5.10508806208342,
5.49778714378214,5.89048622548086,6.28318530717959),.UNSPECIFIED.)
CURVE()
GEOMETRIC_REPRESENTATION_ITEM()
RATIONAL_B_SPLINE_CURVE((1.,1.,1.,1.,1.,1.,1.,1.,1.,1.))
REPRESENTATION_ITEM('')
);
#1107=(
BOUNDED_CURVE()
B_SPLINE_CURVE(3,(#140350,#140351,#140352,#140353,#140354,#140355,#140356,
#140357,#140358,#140359),.UNSPECIFIED.,.F.,.F.)
B_SPLINE_CURVE_WITH_KNOTS((4,2,2,2,4),(0.,0.392699081698724,0.785398163397448,
1.17809724509617,1.5707963267949),.UNSPECIFIED.)
CURVE()
GEOMETRIC_REPRESENTATION_ITEM()
RATIONAL_B_SPLINE_CURVE((1.,1.,1.,1.,1.,1.,1.,1.,1.,1.))
REPRESENTATION_ITEM('')
);
#1108=(
BOUNDED_CURVE()
B_SPLINE_CURVE(3,(#140374,#140375,#140376,#140377,#140378,#140379,#140380,
#140381,#140382,#140383),.UNSPECIFIED.,.F.,.F.)
B_SPLINE_CURVE_WITH_KNOTS((4,2,2,2,4),(1.5707963267949,1.96349540849362,
2.35619449019234,2.74889357189107,3.1415926535898),.UNSPECIFIED.)
CURVE()
GEOMETRIC_REPRESENTATION_ITEM()
RATIONAL_B_SPLINE_CURVE((1.,1.,1.,1.,1.,1.,1.,1.,1.,1.))
REPRESENTATION_ITEM('')
);
#1109=(
BOUNDED_CURVE()
B_SPLINE_CURVE(3,(#140585,#140586,#140587,#140588,#140589,#140590,#140591,
#140592,#140593,#140594),.UNSPECIFIED.,.F.,.F.)
B_SPLINE_CURVE_WITH_KNOTS((4,2,2,2,4),(3.1415926535898,3.53429173528852,
3.92699081698724,4.31968989868597,4.71238898038469),.UNSPECIFIED.)
CURVE()
GEOMETRIC_REPRESENTATION_ITEM()
RATIONAL_B_SPLINE_CURVE((1.,1.,1.,1.,1.,1.,1.,1.,1.,1.))
REPRESENTATION_ITEM('')
);
#1110=(
BOUNDED_CURVE()
B_SPLINE_CURVE(3,(#140633,#140634,#140635,#140636,#140637,#140638,#140639,
#140640,#140641,#140642),.UNSPECIFIED.,.F.,.F.)
B_SPLINE_CURVE_WITH_KNOTS((4,2,2,2,4),(3.1415926535898,3.53429173528852,
3.92699081698724,4.31968989868597,4.71238898038469),.UNSPECIFIED.)
CURVE()
GEOMETRIC_REPRESENTATION_ITEM()
RATIONAL_B_SPLINE_CURVE((1.,1.,1.,1.,1.,1.,1.,1.,1.,1.))
REPRESENTATION_ITEM('')
);
#1111=(
BOUNDED_CURVE()
B_SPLINE_CURVE(3,(#140676,#140677,#140678,#140679,#140680,#140681,#140682,
#140683,#140684,#140685),.UNSPECIFIED.,.F.,.F.)
B_SPLINE_CURVE_WITH_KNOTS((4,2,2,2,4),(1.5707963267949,1.96349540849362,
2.35619449019234,2.74889357189106,3.14159265358979),.UNSPECIFIED.)
CURVE()
GEOMETRIC_REPRESENTATION_ITEM()
RATIONAL_B_SPLINE_CURVE((1.,1.,1.,1.,1.,1.,1.,1.,1.,1.))
REPRESENTATION_ITEM('')
);
#1112=(
BOUNDED_CURVE()
B_SPLINE_CURVE(3,(#140968,#140969,#140970,#140971),.UNSPECIFIED.,.F.,.F.)
B_SPLINE_CURVE_WITH_KNOTS((4,4),(0.,0.00407947372412412),.UNSPECIFIED.)
CURVE()
GEOMETRIC_REPRESENTATION_ITEM()
RATIONAL_B_SPLINE_CURVE((1.,1.,1.,1.))
REPRESENTATION_ITEM('')
);
#1113=(
BOUNDED_CURVE()
B_SPLINE_CURVE(3,(#141029,#141030,#141031,#141032,#141033,#141034,#141035,
#141036,#141037,#141038),.UNSPECIFIED.,.F.,.F.)
B_SPLINE_CURVE_WITH_KNOTS((4,2,2,2,4),(-1.77635683940025E-15,0.392699081698723,
0.785398163397447,1.17809724509617,1.5707963267949),.UNSPECIFIED.)
CURVE()
GEOMETRIC_REPRESENTATION_ITEM()
RATIONAL_B_SPLINE_CURVE((1.,1.,1.,1.,1.,1.,1.,1.,1.,1.))
REPRESENTATION_ITEM('')
);
#1114=(
BOUNDED_CURVE()
B_SPLINE_CURVE(3,(#141072,#141073,#141074,#141075,#141076,#141077,#141078,
#141079,#141080,#141081),.UNSPECIFIED.,.F.,.F.)
B_SPLINE_CURVE_WITH_KNOTS((4,2,2,2,4),(4.71238898038469,5.10508806208342,
5.49778714378214,5.89048622548086,6.28318530717959),.UNSPECIFIED.)
CURVE()
GEOMETRIC_REPRESENTATION_ITEM()
RATIONAL_B_SPLINE_CURVE((1.,1.,1.,1.,1.,1.,1.,1.,1.,1.))
REPRESENTATION_ITEM('')
);
#1115=(
BOUNDED_CURVE()
B_SPLINE_CURVE(3,(#141085,#141086,#141087,#141088,#141089,#141090,#141091,
#141092,#141093,#141094),.UNSPECIFIED.,.F.,.F.)
B_SPLINE_CURVE_WITH_KNOTS((4,2,2,2,4),(1.5707963267949,1.96349540849362,
2.35619449019234,2.74889357189107,3.14159265358979),.UNSPECIFIED.)
CURVE()
GEOMETRIC_REPRESENTATION_ITEM()
RATIONAL_B_SPLINE_CURVE((1.,1.,1.,1.,1.,1.,1.,1.,1.,1.))
REPRESENTATION_ITEM('')
);
#1116=(
BOUNDED_CURVE()
B_SPLINE_CURVE(3,(#141118,#141119,#141120,#141121),.UNSPECIFIED.,.F.,.F.)
B_SPLINE_CURVE_WITH_KNOTS((4,4),(-1.00613961606655E-16,0.00454919832189776),
 .UNSPECIFIED.)
CURVE()
GEOMETRIC_REPRESENTATION_ITEM()
RATIONAL_B_SPLINE_CURVE((1.,1.,1.,1.))
REPRESENTATION_ITEM('')
);
#1117=(
BOUNDED_CURVE()
B_SPLINE_CURVE(3,(#141162,#141163,#141164,#141165),.UNSPECIFIED.,.F.,.F.)
B_SPLINE_CURVE_WITH_KNOTS((4,4),(1.7347234759768E-18,0.00426411906192034),
 .UNSPECIFIED.)
CURVE()
GEOMETRIC_REPRESENTATION_ITEM()
RATIONAL_B_SPLINE_CURVE((1.,1.,1.,1.))
REPRESENTATION_ITEM('')
);
#1118=(
BOUNDED_CURVE()
B_SPLINE_CURVE(3,(#141236,#141237,#141238,#141239,#141240,#141241,#141242,
#141243,#141244,#141245),.UNSPECIFIED.,.F.,.F.)
B_SPLINE_CURVE_WITH_KNOTS((4,2,2,2,4),(4.71238898038469,5.10508806208342,
5.49778714378214,5.89048622548086,6.28318530717959),.UNSPECIFIED.)
CURVE()
GEOMETRIC_REPRESENTATION_ITEM()
RATIONAL_B_SPLINE_CURVE((1.,1.,1.,1.,1.,1.,1.,1.,1.,1.))
REPRESENTATION_ITEM('')
);
#1119=(
BOUNDED_CURVE()
B_SPLINE_CURVE(3,(#141275,#141276,#141277,#141278,#141279,#141280,#141281,
#141282,#141283,#141284),.UNSPECIFIED.,.F.,.F.)
B_SPLINE_CURVE_WITH_KNOTS((4,2,2,2,4),(3.1415926535898,3.53429173528852,
3.92699081698724,4.31968989868597,4.71238898038469),.UNSPECIFIED.)
CURVE()
GEOMETRIC_REPRESENTATION_ITEM()
RATIONAL_B_SPLINE_CURVE((1.,1.,1.,1.,1.,1.,1.,1.,1.,1.))
REPRESENTATION_ITEM('')
);
#1120=(
BOUNDED_CURVE()
B_SPLINE_CURVE(3,(#141500,#141501,#141502,#141503,#141504,#141505,#141506,
#141507,#141508,#141509),.UNSPECIFIED.,.F.,.F.)
B_SPLINE_CURVE_WITH_KNOTS((4,2,2,2,4),(-1.77635683940025E-15,0.392699081698723,
0.785398163397447,1.17809724509617,1.5707963267949),.UNSPECIFIED.)
CURVE()
GEOMETRIC_REPRESENTATION_ITEM()
RATIONAL_B_SPLINE_CURVE((1.,1.,1.,1.,1.,1.,1.,1.,1.,1.))
REPRESENTATION_ITEM('')
);
#1121=(
BOUNDED_CURVE()
B_SPLINE_CURVE(3,(#141524,#141525,#141526,#141527,#141528,#141529,#141530,
#141531,#141532,#141533),.UNSPECIFIED.,.F.,.F.)
B_SPLINE_CURVE_WITH_KNOTS((4,2,2,2,4),(1.5707963267949,1.96349540849362,
2.35619449019234,2.74889357189107,3.14159265358979),.UNSPECIFIED.)
CURVE()
GEOMETRIC_REPRESENTATION_ITEM()
RATIONAL_B_SPLINE_CURVE((1.,1.,1.,1.,1.,1.,1.,1.,1.,1.))
REPRESENTATION_ITEM('')
);
#1122=(
BOUNDED_CURVE()
B_SPLINE_CURVE(3,(#141732,#141733,#141734,#141735,#141736,#141737,#141738,
#141739,#141740,#141741),.UNSPECIFIED.,.F.,.F.)
B_SPLINE_CURVE_WITH_KNOTS((4,2,2,2,4),(3.1415926535898,3.53429173528852,
3.92699081698724,4.31968989868597,4.71238898038469),.UNSPECIFIED.)
CURVE()
GEOMETRIC_REPRESENTATION_ITEM()
RATIONAL_B_SPLINE_CURVE((1.,1.,1.,1.,1.,1.,1.,1.,1.,1.))
REPRESENTATION_ITEM('')
);
#1123=(
BOUNDED_CURVE()
B_SPLINE_CURVE(3,(#141935,#141936,#141937,#141938,#141939,#141940,#141941,
#141942,#141943,#141944),.UNSPECIFIED.,.F.,.F.)
B_SPLINE_CURVE_WITH_KNOTS((4,2,2,2,4),(3.1415926535898,3.53429173528852,
3.92699081698724,4.31968989868597,4.71238898038469),.UNSPECIFIED.)
CURVE()
GEOMETRIC_REPRESENTATION_ITEM()
RATIONAL_B_SPLINE_CURVE((1.,1.,1.,1.,1.,1.,1.,1.,1.,1.))
REPRESENTATION_ITEM('')
);
#1124=(
BOUNDED_CURVE()
B_SPLINE_CURVE(3,(#141948,#141949,#141950,#141951,#141952,#141953,#141954,
#141955,#141956,#141957),.UNSPECIFIED.,.F.,.F.)
B_SPLINE_CURVE_WITH_KNOTS((4,2,2,2,4),(4.71238898038469,5.10508806208341,
5.49778714378214,5.89048622548086,6.28318530717959),.UNSPECIFIED.)
CURVE()
GEOMETRIC_REPRESENTATION_ITEM()
RATIONAL_B_SPLINE_CURVE((1.,1.,1.,1.,1.,1.,1.,1.,1.,1.))
REPRESENTATION_ITEM('')
);
#1125=(
BOUNDED_CURVE()
B_SPLINE_CURVE(3,(#142061,#142062,#142063,#142064,#142065,#142066,#142067,
#142068,#142069,#142070),.UNSPECIFIED.,.F.,.F.)
B_SPLINE_CURVE_WITH_KNOTS((4,2,2,2,4),(1.5707963267949,1.96349540849362,
2.35619449019234,2.74889357189107,3.14159265358979),.UNSPECIFIED.)
CURVE()
GEOMETRIC_REPRESENTATION_ITEM()
RATIONAL_B_SPLINE_CURVE((1.,1.,1.,1.,1.,1.,1.,1.,1.,1.))
REPRESENTATION_ITEM('')
);
#1126=(
BOUNDED_CURVE()
B_SPLINE_CURVE(3,(#142094,#142095,#142096,#142097),.UNSPECIFIED.,.F.,.F.)
B_SPLINE_CURVE_WITH_KNOTS((4,4),(-5.03069808033274E-17,0.00385726433182564),
 .UNSPECIFIED.)
CURVE()
GEOMETRIC_REPRESENTATION_ITEM()
RATIONAL_B_SPLINE_CURVE((1.,1.,1.,1.))
REPRESENTATION_ITEM('')
);
#1127=(
BOUNDED_CURVE()
B_SPLINE_CURVE(3,(#142138,#142139,#142140,#142141),.UNSPECIFIED.,.F.,.F.)
B_SPLINE_CURVE_WITH_KNOTS((4,4),(0.,0.00414272899747597),.UNSPECIFIED.)
CURVE()
GEOMETRIC_REPRESENTATION_ITEM()
RATIONAL_B_SPLINE_CURVE((1.,1.,1.,1.))
REPRESENTATION_ITEM('')
);
#1128=(
BOUNDED_CURVE()
B_SPLINE_CURVE(3,(#142159,#142160,#142161,#142162,#142163,#142164,#142165,
#142166,#142167,#142168),.UNSPECIFIED.,.F.,.F.)
B_SPLINE_CURVE_WITH_KNOTS((4,2,2,2,4),(-8.88178419700125E-16,0.392699081698724,
0.785398163397448,1.17809724509617,1.5707963267949),.UNSPECIFIED.)
CURVE()
GEOMETRIC_REPRESENTATION_ITEM()
RATIONAL_B_SPLINE_CURVE((1.,1.,1.,1.,1.,1.,1.,1.,1.,1.))
REPRESENTATION_ITEM('')
);
#1129=(
BOUNDED_CURVE()
B_SPLINE_CURVE(3,(#142266,#142267,#142268,#142269,#142270,#142271,#142272,
#142273,#142274,#142275),.UNSPECIFIED.,.F.,.F.)
B_SPLINE_CURVE_WITH_KNOTS((4,2,2,2,4),(4.71238898038469,5.10508806208341,
5.49778714378214,5.89048622548086,6.28318530717959),.UNSPECIFIED.)
CURVE()
GEOMETRIC_REPRESENTATION_ITEM()
RATIONAL_B_SPLINE_CURVE((1.,1.,1.,1.,1.,1.,1.,1.,1.,1.))
REPRESENTATION_ITEM('')
);
#1130=(
BOUNDED_CURVE()
B_SPLINE_CURVE(3,(#142412,#142413,#142414,#142415,#142416,#142417,#142418,
#142419,#142420,#142421),.UNSPECIFIED.,.F.,.F.)
B_SPLINE_CURVE_WITH_KNOTS((4,2,2,2,4),(1.5707963267949,1.96349540849362,
2.35619449019234,2.74889357189107,3.14159265358979),.UNSPECIFIED.)
CURVE()
GEOMETRIC_REPRESENTATION_ITEM()
RATIONAL_B_SPLINE_CURVE((1.,1.,1.,1.,1.,1.,1.,1.,1.,1.))
REPRESENTATION_ITEM('')
);
#1131=(
BOUNDED_CURVE()
B_SPLINE_CURVE(3,(#142528,#142529,#142530,#142531,#142532,#142533,#142534,
#142535,#142536,#142537),.UNSPECIFIED.,.F.,.F.)
B_SPLINE_CURVE_WITH_KNOTS((4,2,2,2,4),(-8.88178419700125E-16,0.392699081698724,
0.785398163397448,1.17809724509617,1.5707963267949),.UNSPECIFIED.)
CURVE()
GEOMETRIC_REPRESENTATION_ITEM()
RATIONAL_B_SPLINE_CURVE((1.,1.,1.,1.,1.,1.,1.,1.,1.,1.))
REPRESENTATION_ITEM('')
);
#1132=(
BOUNDED_CURVE()
B_SPLINE_CURVE(3,(#144003,#144004,#144005,#144006),.UNSPECIFIED.,.F.,.F.)
B_SPLINE_CURVE_WITH_KNOTS((4,4),(0.,1.),.UNSPECIFIED.)
CURVE()
GEOMETRIC_REPRESENTATION_ITEM()
RATIONAL_B_SPLINE_CURVE((0.999999927380708,0.999999923584106,0.999999920688567,
0.999999918247059))
REPRESENTATION_ITEM('')
);
#1133=(
BOUNDED_CURVE()
B_SPLINE_CURVE(3,(#144057,#144058,#144059,#144060),.UNSPECIFIED.,.F.,.F.)
B_SPLINE_CURVE_WITH_KNOTS((4,4),(0.,1.),.UNSPECIFIED.)
CURVE()
GEOMETRIC_REPRESENTATION_ITEM()
RATIONAL_B_SPLINE_CURVE((0.999999995487232,0.999999995342312,0.999999995242007,
0.999999995159558))
REPRESENTATION_ITEM('')
);
#1134=(
BOUNDED_CURVE()
B_SPLINE_CURVE(3,(#144253,#144254,#144255,#144256),.UNSPECIFIED.,.F.,.F.)
B_SPLINE_CURVE_WITH_KNOTS((4,4),(0.,1.),.UNSPECIFIED.)
CURVE()
GEOMETRIC_REPRESENTATION_ITEM()
RATIONAL_B_SPLINE_CURVE((0.999999999408156,0.999999999401785,0.999999999393965,
0.999999999382027))
REPRESENTATION_ITEM('')
);
#1135=(
BOUNDED_CURVE()
B_SPLINE_CURVE(3,(#144311,#144312,#144313,#144314),.UNSPECIFIED.,.F.,.F.)
B_SPLINE_CURVE_WITH_KNOTS((4,4),(0.,1.),.UNSPECIFIED.)
CURVE()
GEOMETRIC_REPRESENTATION_ITEM()
RATIONAL_B_SPLINE_CURVE((0.99999987960117,0.999999865674974,0.999999841276082,
0.999999808047049))
REPRESENTATION_ITEM('')
);
#1136=(
BOUNDED_CURVE()
B_SPLINE_CURVE(3,(#144668,#144669,#144670,#144671,#144672,#144673),
 .UNSPECIFIED.,.F.,.F.)
B_SPLINE_CURVE_WITH_KNOTS((4,2,4),(0.,0.5,1.),.UNSPECIFIED.)
CURVE()
GEOMETRIC_REPRESENTATION_ITEM()
RATIONAL_B_SPLINE_CURVE((0.999999999903741,0.999999999897905,0.999999999891833,
0.999999999879122,0.999999999872429,0.999999999865662))
REPRESENTATION_ITEM('')
);
#1137=(
BOUNDED_CURVE()
B_SPLINE_CURVE(3,(#144928,#144929,#144930,#144931,#144932,#144933),
 .UNSPECIFIED.,.F.,.F.)
B_SPLINE_CURVE_WITH_KNOTS((4,2,4),(0.,0.499999999999999,0.999999989281006),
 .UNSPECIFIED.)
CURVE()
GEOMETRIC_REPRESENTATION_ITEM()
RATIONAL_B_SPLINE_CURVE((0.999999999934743,0.999999999928937,0.999999999922868,
0.999999999909996,0.99999999990313,0.999999999896125))
REPRESENTATION_ITEM('')
);
#1138=(
BOUNDED_CURVE()
B_SPLINE_CURVE(3,(#145054,#145055,#145056,#145057),.UNSPECIFIED.,.F.,.F.)
B_SPLINE_CURVE_WITH_KNOTS((4,4),(0.,1.),.UNSPECIFIED.)
CURVE()
GEOMETRIC_REPRESENTATION_ITEM()
RATIONAL_B_SPLINE_CURVE((0.999999907463791,0.99999990228317,0.999999898054214,
0.999999894391216))
REPRESENTATION_ITEM('')
);
#1139=(
BOUNDED_CURVE()
B_SPLINE_CURVE(3,(#145708,#145709,#145710,#145711,#145712,#145713),
 .UNSPECIFIED.,.F.,.F.)
B_SPLINE_CURVE_WITH_KNOTS((4,2,4),(0.,0.5,1.),.UNSPECIFIED.)
CURVE()
GEOMETRIC_REPRESENTATION_ITEM()
RATIONAL_B_SPLINE_CURVE((0.999999998284567,0.999999998319219,0.99999999834714,
0.999999998395064,0.999999998415023,0.999999998432575))
REPRESENTATION_ITEM('')
);
#1140=(
BOUNDED_CURVE()
B_SPLINE_CURVE(3,(#145734,#145735,#145736,#145737,#145738,#145739),
 .UNSPECIFIED.,.F.,.F.)
B_SPLINE_CURVE_WITH_KNOTS((4,2,4),(0.,0.499999999999999,1.),
 .UNSPECIFIED.)
CURVE()
GEOMETRIC_REPRESENTATION_ITEM()
RATIONAL_B_SPLINE_CURVE((0.99999999988276,0.999999999875186,0.999999999867293,
0.999999999850728,0.999999999841986,0.999999999833128))
REPRESENTATION_ITEM('')
);
#1141=(
BOUNDED_CURVE()
B_SPLINE_CURVE(3,(#145935,#145936,#145937,#145938),.UNSPECIFIED.,.F.,.F.)
B_SPLINE_CURVE_WITH_KNOTS((4,4),(0.,1.),.UNSPECIFIED.)
CURVE()
GEOMETRIC_REPRESENTATION_ITEM()
RATIONAL_B_SPLINE_CURVE((0.999999985881004,0.999999986166315,0.999999986518015,
0.99999998707511))
REPRESENTATION_ITEM('')
);
#1142=(
BOUNDED_CURVE()
B_SPLINE_CURVE(3,(#146091,#146092,#146093,#146094,#146095,#146096,#146097,
#146098,#146099,#146100,#146101,#146102,#146103,#146104),.UNSPECIFIED.,
 .F.,.F.)
B_SPLINE_CURVE_WITH_KNOTS((4,2,2,2,2,2,4),(0.,0.245502202551198,0.371251835459332,
0.497001468367467,0.622751101275599,0.748500734183734,1.),.UNSPECIFIED.)
CURVE()
GEOMETRIC_REPRESENTATION_ITEM()
RATIONAL_B_SPLINE_CURVE((0.999999945516601,0.999999945630438,0.999999945782265,
0.999999946051757,0.999999946150377,0.999999946362488,0.999999946475958,
0.99999994671043,0.999999946832282,0.999999947085115,0.999999947217219,
0.999999947617593,0.999999947890007,0.999999948167728))
REPRESENTATION_ITEM('')
);
#1143=(
BOUNDED_CURVE()
B_SPLINE_CURVE(3,(#146180,#146181,#146182,#146183),.UNSPECIFIED.,.F.,.F.)
B_SPLINE_CURVE_WITH_KNOTS((4,4),(0.,1.),.UNSPECIFIED.)
CURVE()
GEOMETRIC_REPRESENTATION_ITEM()
RATIONAL_B_SPLINE_CURVE((0.999999999051513,0.999999999075715,0.999999999089916,
0.999999999101407))
REPRESENTATION_ITEM('')
);
#1144=(
BOUNDED_CURVE()
B_SPLINE_CURVE(3,(#146412,#146413,#146414,#146415,#146416,#146417,#146418,
#146419,#146420,#146421),.UNSPECIFIED.,.F.,.F.)
B_SPLINE_CURVE_WITH_KNOTS((4,2,2,2,4),(0.,0.251507516180303,0.50301503236061,
0.754522548540912,1.),.UNSPECIFIED.)
CURVE()
GEOMETRIC_REPRESENTATION_ITEM()
RATIONAL_B_SPLINE_CURVE((0.999999987939898,0.999999987944251,0.999999987948487,
0.999999987956739,0.999999987960767,0.999999987968182,0.999999987971664,
0.999999987977827,0.999999987980498,0.999999987982808))
REPRESENTATION_ITEM('')
);
#1145=(
BOUNDED_CURVE()
B_SPLINE_CURVE(3,(#146520,#146521,#146522,#146523,#146524,#146525,#146526,
#146527,#146528,#146529),.UNSPECIFIED.,.F.,.F.)
B_SPLINE_CURVE_WITH_KNOTS((4,2,2,2,4),(0.,0.24546127409179,0.496974182727859,
0.748487091363931,1.),.UNSPECIFIED.)
CURVE()
GEOMETRIC_REPRESENTATION_ITEM()
RATIONAL_B_SPLINE_CURVE((0.999999992164428,0.999999992163856,0.999999992163196,
0.999999992161673,0.999999992160813,0.999999992158981,0.999999992157986,
0.999999992155948,0.999999992154902,0.999999992153827))
REPRESENTATION_ITEM('')
);
#1146=(
BOUNDED_CURVE()
B_SPLINE_CURVE(3,(#146762,#146763,#146764,#146765),.UNSPECIFIED.,.F.,.F.)
B_SPLINE_CURVE_WITH_KNOTS((4,4),(0.,1.),.UNSPECIFIED.)
CURVE()
GEOMETRIC_REPRESENTATION_ITEM()
RATIONAL_B_SPLINE_CURVE((0.999999998598817,0.999999998581398,0.999999998559873,
0.999999998523147))
REPRESENTATION_ITEM('')
);
#1147=(
BOUNDED_CURVE()
B_SPLINE_CURVE(3,(#147003,#147004,#147005,#147006),.UNSPECIFIED.,.F.,.F.)
B_SPLINE_CURVE_WITH_KNOTS((4,4),(0.,1.),.UNSPECIFIED.)
CURVE()
GEOMETRIC_REPRESENTATION_ITEM()
RATIONAL_B_SPLINE_CURVE((0.99999998938962,0.999999988942626,0.999999988661227,
0.999999988432992))
REPRESENTATION_ITEM('')
);
#1148=(
BOUNDED_CURVE()
B_SPLINE_CURVE(3,(#147124,#147125,#147126,#147127,#147128,#147129),
 .UNSPECIFIED.,.F.,.F.)
B_SPLINE_CURVE_WITH_KNOTS((4,2,4),(0.,0.5,1.),.UNSPECIFIED.)
CURVE()
GEOMETRIC_REPRESENTATION_ITEM()
RATIONAL_B_SPLINE_CURVE((0.999999999894234,0.999999999887496,0.999999999880475,
0.999999999865743,0.999999999857971,0.999999999850097))
REPRESENTATION_ITEM('')
);
#1149=(
BOUNDED_CURVE()
B_SPLINE_CURVE(3,(#148141,#148142,#148143,#148144),.UNSPECIFIED.,.F.,.F.)
B_SPLINE_CURVE_WITH_KNOTS((4,4),(0.,1.),.UNSPECIFIED.)
CURVE()
GEOMETRIC_REPRESENTATION_ITEM()
RATIONAL_B_SPLINE_CURVE((0.999999927469661,0.999999923649506,0.999999920386278,
0.999999917494068))
REPRESENTATION_ITEM('')
);
#1150=(
BOUNDED_CURVE()
B_SPLINE_CURVE(3,(#148246,#148247,#148248,#148249),.UNSPECIFIED.,.F.,.F.)
B_SPLINE_CURVE_WITH_KNOTS((4,4),(0.,1.),.UNSPECIFIED.)
CURVE()
GEOMETRIC_REPRESENTATION_ITEM()
RATIONAL_B_SPLINE_CURVE((0.999999892411738,0.999999896151516,0.999999900365766,
0.999999905288505))
REPRESENTATION_ITEM('')
);
#1151=(
BOUNDED_CURVE()
B_SPLINE_CURVE(3,(#148262,#148263,#148264,#148265),.UNSPECIFIED.,.F.,.F.)
B_SPLINE_CURVE_WITH_KNOTS((4,4),(0.,1.),.UNSPECIFIED.)
CURVE()
GEOMETRIC_REPRESENTATION_ITEM()
RATIONAL_B_SPLINE_CURVE((0.999999978616913,0.999999978977049,0.999999979295994,
0.999999979585313))
REPRESENTATION_ITEM('')
);
#1152=(
BOUNDED_CURVE()
B_SPLINE_CURVE(3,(#148432,#148433,#148434,#148435),.UNSPECIFIED.,.F.,.F.)
B_SPLINE_CURVE_WITH_KNOTS((4,4),(0.,1.),.UNSPECIFIED.)
CURVE()
GEOMETRIC_REPRESENTATION_ITEM()
RATIONAL_B_SPLINE_CURVE((0.999999998794032,0.999999998776629,0.99999999875741,
0.999999998735649))
REPRESENTATION_ITEM('')
);
#1153=(
BOUNDED_CURVE()
B_SPLINE_CURVE(3,(#149798,#149799,#149800,#149801,#149802,#149803),
 .UNSPECIFIED.,.F.,.F.)
B_SPLINE_CURVE_WITH_KNOTS((4,2,4),(0.,0.5,1.),.UNSPECIFIED.)
CURVE()
GEOMETRIC_REPRESENTATION_ITEM()
RATIONAL_B_SPLINE_CURVE((0.999999996854374,0.999999996923258,0.999999996997747,
0.999999997161208,0.999999997250172,0.999999997348475))
REPRESENTATION_ITEM('')
);
#1154=(
BOUNDED_CURVE()
B_SPLINE_CURVE(3,(#150640,#150641,#150642,#150643,#150644,#150645),
 .UNSPECIFIED.,.F.,.F.)
B_SPLINE_CURVE_WITH_KNOTS((4,2,4),(0.,0.5,1.),.UNSPECIFIED.)
CURVE()
GEOMETRIC_REPRESENTATION_ITEM()
RATIONAL_B_SPLINE_CURVE((0.999999996756183,0.999999996827757,0.999999996905132,
0.999999997074846,0.999999997167179,0.999999997269145))
REPRESENTATION_ITEM('')
);
#1155=(
BOUNDED_CURVE()
B_SPLINE_CURVE(3,(#151836,#151837,#151838,#151839,#151840,#151841),
 .UNSPECIFIED.,.F.,.F.)
B_SPLINE_CURVE_WITH_KNOTS((4,2,4),(0.,0.5,1.),.UNSPECIFIED.)
CURVE()
GEOMETRIC_REPRESENTATION_ITEM()
RATIONAL_B_SPLINE_CURVE((0.999999999990438,0.999999999987754,0.999999999984833,
0.999999999978368,0.999999999974827,0.999999999970832))
REPRESENTATION_ITEM('')
);
#1156=(
BOUNDED_CURVE()
B_SPLINE_CURVE(3,(#151873,#151874,#151875,#151876),.UNSPECIFIED.,.F.,.F.)
B_SPLINE_CURVE_WITH_KNOTS((4,4),(0.,1.),.UNSPECIFIED.)
CURVE()
GEOMETRIC_REPRESENTATION_ITEM()
RATIONAL_B_SPLINE_CURVE((0.999999764205276,0.999999729074058,0.999999662874959,
0.999999569832623))
REPRESENTATION_ITEM('')
);
#1157=(
BOUNDED_CURVE()
B_SPLINE_CURVE(3,(#152419,#152420,#152421,#152422,#152423,#152424),
 .UNSPECIFIED.,.F.,.F.)
B_SPLINE_CURVE_WITH_KNOTS((4,2,4),(0.,0.5,1.),.UNSPECIFIED.)
CURVE()
GEOMETRIC_REPRESENTATION_ITEM()
RATIONAL_B_SPLINE_CURVE((0.999999938557239,0.999999946973332,0.999999954433094,
0.999999968051422,0.999999974205021,0.999999979856827))
REPRESENTATION_ITEM('')
);
#1158=(
BOUNDED_CURVE()
B_SPLINE_CURVE(3,(#152846,#152847,#152848,#152849,#152850,#152851,#152852,
#152853),.UNSPECIFIED.,.F.,.F.)
B_SPLINE_CURVE_WITH_KNOTS((4,2,2,4),(0.,0.230529842217703,0.489063635927588,
1.),.UNSPECIFIED.)
CURVE()
GEOMETRIC_REPRESENTATION_ITEM()
RATIONAL_B_SPLINE_CURVE((0.999999995461409,0.999999995444687,0.999999995419802,
0.999999995349838,0.999999995302614,0.999999995136626,0.999999994992415,
0.999999994821643))
REPRESENTATION_ITEM('')
);
#1159=(
BOUNDED_CURVE()
B_SPLINE_CURVE(3,(#165191,#165192,#165193,#165194,#165195,#165196,#165197,
#165198,#165199,#165200),.UNSPECIFIED.,.F.,.F.)
B_SPLINE_CURVE_WITH_KNOTS((4,2,2,2,4),(-8.88178419700125E-16,0.392699081698724,
0.785398163397448,1.17809724509617,1.5707963267949),.UNSPECIFIED.)
CURVE()
GEOMETRIC_REPRESENTATION_ITEM()
RATIONAL_B_SPLINE_CURVE((1.,1.,1.,1.,1.,1.,1.,1.,1.,1.))
REPRESENTATION_ITEM('')
);
#1160=(
BOUNDED_CURVE()
B_SPLINE_CURVE(3,(#165277,#165278,#165279,#165280,#165281,#165282,#165283,
#165284,#165285,#165286),.UNSPECIFIED.,.F.,.F.)
B_SPLINE_CURVE_WITH_KNOTS((4,2,2,2,4),(4.71238898038469,5.10508806208341,
5.49778714378214,5.89048622548086,6.28318530717959),.UNSPECIFIED.)
CURVE()
GEOMETRIC_REPRESENTATION_ITEM()
RATIONAL_B_SPLINE_CURVE((1.,1.,1.,1.,1.,1.,1.,1.,1.,1.))
REPRESENTATION_ITEM('')
);
#1161=(
BOUNDED_CURVE()
B_SPLINE_CURVE(3,(#165729,#165730,#165731,#165732),.UNSPECIFIED.,.F.,.F.)
B_SPLINE_CURVE_WITH_KNOTS((4,4),(-5.03069808033274E-17,0.00385726433182564),
 .UNSPECIFIED.)
CURVE()
GEOMETRIC_REPRESENTATION_ITEM()
RATIONAL_B_SPLINE_CURVE((1.,1.,1.,1.))
REPRESENTATION_ITEM('')
);
#1162=(
BOUNDED_CURVE()
B_SPLINE_CURVE(3,(#165857,#165858,#165859,#165860),.UNSPECIFIED.,.F.,.F.)
B_SPLINE_CURVE_WITH_KNOTS((4,4),(0.,0.00414272899747597),.UNSPECIFIED.)
CURVE()
GEOMETRIC_REPRESENTATION_ITEM()
RATIONAL_B_SPLINE_CURVE((1.,1.,1.,1.))
REPRESENTATION_ITEM('')
);
#1163=(
BOUNDED_CURVE()
B_SPLINE_CURVE(3,(#165944,#165945,#165946,#165947,#165948,#165949,#165950,
#165951,#165952,#165953),.UNSPECIFIED.,.F.,.F.)
B_SPLINE_CURVE_WITH_KNOTS((4,2,2,2,4),(-8.88178419700125E-16,0.392699081698724,
0.785398163397448,1.17809724509617,1.5707963267949),.UNSPECIFIED.)
CURVE()
GEOMETRIC_REPRESENTATION_ITEM()
RATIONAL_B_SPLINE_CURVE((1.,1.,1.,1.,1.,1.,1.,1.,1.,1.))
REPRESENTATION_ITEM('')
);
#1164=(
BOUNDED_CURVE()
B_SPLINE_CURVE(3,(#166125,#166126,#166127,#166128,#166129,#166130,#166131,
#166132,#166133,#166134),.UNSPECIFIED.,.F.,.F.)
B_SPLINE_CURVE_WITH_KNOTS((4,2,2,2,4),(4.71238898038469,5.10508806208341,
5.49778714378214,5.89048622548086,6.28318530717959),.UNSPECIFIED.)
CURVE()
GEOMETRIC_REPRESENTATION_ITEM()
RATIONAL_B_SPLINE_CURVE((1.,1.,1.,1.,1.,1.,1.,1.,1.,1.))
REPRESENTATION_ITEM('')
);
#1165=(
BOUNDED_CURVE()
B_SPLINE_CURVE(3,(#166770,#166771,#166772,#166773,#166774,#166775,#166776,
#166777,#166778,#166779),.UNSPECIFIED.,.F.,.F.)
B_SPLINE_CURVE_WITH_KNOTS((4,2,2,2,4),(3.1415926535898,3.53429173528852,
3.92699081698724,4.31968989868597,4.71238898038469),.UNSPECIFIED.)
CURVE()
GEOMETRIC_REPRESENTATION_ITEM()
RATIONAL_B_SPLINE_CURVE((1.,1.,1.,1.,1.,1.,1.,1.,1.,1.))
REPRESENTATION_ITEM('')
);
#1166=(
BOUNDED_CURVE()
B_SPLINE_CURVE(3,(#166847,#166848,#166849,#166850,#166851,#166852,#166853,
#166854,#166855,#166856),.UNSPECIFIED.,.F.,.F.)
B_SPLINE_CURVE_WITH_KNOTS((4,2,2,2,4),(1.5707963267949,1.96349540849362,
2.35619449019234,2.74889357189107,3.14159265358979),.UNSPECIFIED.)
CURVE()
GEOMETRIC_REPRESENTATION_ITEM()
RATIONAL_B_SPLINE_CURVE((1.,1.,1.,1.,1.,1.,1.,1.,1.,1.))
REPRESENTATION_ITEM('')
);
#1167=(
BOUNDED_CURVE()
B_SPLINE_CURVE(3,(#167521,#167522,#167523,#167524,#167525,#167526,#167527,
#167528,#167529,#167530),.UNSPECIFIED.,.F.,.F.)
B_SPLINE_CURVE_WITH_KNOTS((4,2,2,2,4),(3.1415926535898,3.53429173528852,
3.92699081698724,4.31968989868597,4.71238898038469),.UNSPECIFIED.)
CURVE()
GEOMETRIC_REPRESENTATION_ITEM()
RATIONAL_B_SPLINE_CURVE((1.,1.,1.,1.,1.,1.,1.,1.,1.,1.))
REPRESENTATION_ITEM('')
);
#1168=(
BOUNDED_CURVE()
B_SPLINE_CURVE(3,(#167735,#167736,#167737,#167738),.UNSPECIFIED.,.F.,.F.)
B_SPLINE_CURVE_WITH_KNOTS((4,4),(-1.00613961606655E-16,0.00454919832189776),
 .UNSPECIFIED.)
CURVE()
GEOMETRIC_REPRESENTATION_ITEM()
RATIONAL_B_SPLINE_CURVE((1.,1.,1.,1.))
REPRESENTATION_ITEM('')
);
#1169=(
BOUNDED_CURVE()
B_SPLINE_CURVE(3,(#167862,#167863,#167864,#167865),.UNSPECIFIED.,.F.,.F.)
B_SPLINE_CURVE_WITH_KNOTS((4,4),(1.7347234759768E-18,0.00426411906192034),
 .UNSPECIFIED.)
CURVE()
GEOMETRIC_REPRESENTATION_ITEM()
RATIONAL_B_SPLINE_CURVE((1.,1.,1.,1.))
REPRESENTATION_ITEM('')
);
#1170=(
BOUNDED_CURVE()
B_SPLINE_CURVE(3,(#168044,#168045,#168046,#168047,#168048,#168049,#168050,
#168051,#168052,#168053),.UNSPECIFIED.,.F.,.F.)
B_SPLINE_CURVE_WITH_KNOTS((4,2,2,2,4),(1.5707963267949,1.96349540849362,
2.35619449019234,2.74889357189107,3.14159265358979),.UNSPECIFIED.)
CURVE()
GEOMETRIC_REPRESENTATION_ITEM()
RATIONAL_B_SPLINE_CURVE((1.,1.,1.,1.,1.,1.,1.,1.,1.,1.))
REPRESENTATION_ITEM('')
);
#1171=(
BOUNDED_CURVE()
B_SPLINE_CURVE(3,(#168202,#168203,#168204,#168205),.UNSPECIFIED.,.F.,.F.)
B_SPLINE_CURVE_WITH_KNOTS((4,4),(0.,0.00407947372412412),.UNSPECIFIED.)
CURVE()
GEOMETRIC_REPRESENTATION_ITEM()
RATIONAL_B_SPLINE_CURVE((1.,1.,1.,1.))
REPRESENTATION_ITEM('')
);
#1172=(
BOUNDED_CURVE()
B_SPLINE_CURVE(3,(#169018,#169019,#169020,#169021,#169022,#169023,#169024,
#169025,#169026,#169027),.UNSPECIFIED.,.F.,.F.)
B_SPLINE_CURVE_WITH_KNOTS((4,2,2,2,4),(3.1415926535898,3.53429173528852,
3.92699081698724,4.31968989868597,4.71238898038469),.UNSPECIFIED.)
CURVE()
GEOMETRIC_REPRESENTATION_ITEM()
RATIONAL_B_SPLINE_CURVE((1.,1.,1.,1.,1.,1.,1.,1.,1.,1.))
REPRESENTATION_ITEM('')
);
#1173=(
BOUNDED_CURVE()
B_SPLINE_CURVE(3,(#169095,#169096,#169097,#169098,#169099,#169100,#169101,
#169102,#169103,#169104),.UNSPECIFIED.,.F.,.F.)
B_SPLINE_CURVE_WITH_KNOTS((4,2,2,2,4),(1.5707963267949,1.96349540849362,
2.35619449019234,2.74889357189107,3.1415926535898),.UNSPECIFIED.)
CURVE()
GEOMETRIC_REPRESENTATION_ITEM()
RATIONAL_B_SPLINE_CURVE((1.,1.,1.,1.,1.,1.,1.,1.,1.,1.))
REPRESENTATION_ITEM('')
);
#1174=(
BOUNDED_CURVE()
B_SPLINE_CURVE(3,(#169731,#169732,#169733,#169734,#169735,#169736,#169737,
#169738,#169739,#169740),.UNSPECIFIED.,.F.,.F.)
B_SPLINE_CURVE_WITH_KNOTS((4,2,2,2,4),(3.1415926535898,3.53429173528852,
3.92699081698724,4.31968989868597,4.71238898038469),.UNSPECIFIED.)
CURVE()
GEOMETRIC_REPRESENTATION_ITEM()
RATIONAL_B_SPLINE_CURVE((1.,1.,1.,1.,1.,1.,1.,1.,1.,1.))
REPRESENTATION_ITEM('')
);
#1175=(
BOUNDED_CURVE()
B_SPLINE_CURVE(3,(#170157,#170158,#170159,#170160,#170161,#170162,#170163,
#170164,#170165,#170166),.UNSPECIFIED.,.F.,.F.)
B_SPLINE_CURVE_WITH_KNOTS((4,2,2,2,4),(1.5707963267949,1.96349540849362,
2.35619449019234,2.74889357189107,3.1415926535898),.UNSPECIFIED.)
CURVE()
GEOMETRIC_REPRESENTATION_ITEM()
RATIONAL_B_SPLINE_CURVE((1.,1.,1.,1.,1.,1.,1.,1.,1.,1.))
REPRESENTATION_ITEM('')
);
#1176=(
BOUNDED_CURVE()
B_SPLINE_CURVE(3,(#171513,#171514,#171515,#171516),.UNSPECIFIED.,.F.,.F.)
B_SPLINE_CURVE_WITH_KNOTS((4,4),(0.,0.0433970829567688),.UNSPECIFIED.)
CURVE()
GEOMETRIC_REPRESENTATION_ITEM()
RATIONAL_B_SPLINE_CURVE((1.,1.,1.,1.))
REPRESENTATION_ITEM('')
);
#1177=(
BOUNDED_CURVE()
B_SPLINE_CURVE(3,(#171666,#171667,#171668,#171669),.UNSPECIFIED.,.F.,.F.)
B_SPLINE_CURVE_WITH_KNOTS((4,4),(-1.38777878078145E-17,0.0431305646498159),
 .UNSPECIFIED.)
CURVE()
GEOMETRIC_REPRESENTATION_ITEM()
RATIONAL_B_SPLINE_CURVE((1.,1.,1.,1.))
REPRESENTATION_ITEM('')
);
#1178=(
BOUNDED_CURVE()
B_SPLINE_CURVE(3,(#171908,#171909,#171910,#171911),.UNSPECIFIED.,.F.,.F.)
B_SPLINE_CURVE_WITH_KNOTS((4,4),(0.,0.0445045070401677),.UNSPECIFIED.)
CURVE()
GEOMETRIC_REPRESENTATION_ITEM()
RATIONAL_B_SPLINE_CURVE((1.,1.,1.,1.))
REPRESENTATION_ITEM('')
);
#1179=(
BOUNDED_CURVE()
B_SPLINE_CURVE(3,(#172016,#172017,#172018,#172019),.UNSPECIFIED.,.F.,.F.)
B_SPLINE_CURVE_WITH_KNOTS((4,4),(0.,0.044753309356401),.UNSPECIFIED.)
CURVE()
GEOMETRIC_REPRESENTATION_ITEM()
RATIONAL_B_SPLINE_CURVE((1.,1.,1.,1.))
REPRESENTATION_ITEM('')
);
#1180=(
BOUNDED_CURVE()
B_SPLINE_CURVE(3,(#172070,#172071,#172072,#172073),.UNSPECIFIED.,.F.,.F.)
B_SPLINE_CURVE_WITH_KNOTS((4,4),(0.,0.0444870989094409),.UNSPECIFIED.)
CURVE()
GEOMETRIC_REPRESENTATION_ITEM()
RATIONAL_B_SPLINE_CURVE((1.,1.,1.,1.))
REPRESENTATION_ITEM('')
);
#1181=(
BOUNDED_CURVE()
B_SPLINE_CURVE(3,(#172295,#172296,#172297,#172298),.UNSPECIFIED.,.F.,.F.)
B_SPLINE_CURVE_WITH_KNOTS((4,4),(-2.77555756156289E-17,0.0433026927553429),
 .UNSPECIFIED.)
CURVE()
GEOMETRIC_REPRESENTATION_ITEM()
RATIONAL_B_SPLINE_CURVE((1.,1.,1.,1.))
REPRESENTATION_ITEM('')
);
#1182=(
BOUNDED_CURVE()
B_SPLINE_CURVE(3,(#172425,#172426,#172427,#172428),.UNSPECIFIED.,.F.,.F.)
B_SPLINE_CURVE_WITH_KNOTS((4,4),(0.,0.0430361525536219),.UNSPECIFIED.)
CURVE()
GEOMETRIC_REPRESENTATION_ITEM()
RATIONAL_B_SPLINE_CURVE((1.,1.,1.,1.))
REPRESENTATION_ITEM('')
);
#1183=(
BOUNDED_CURVE()
B_SPLINE_CURVE(3,(#173780,#173781,#173782,#173783),.UNSPECIFIED.,.F.,.F.)
B_SPLINE_CURVE_WITH_KNOTS((4,4),(-1.38777878078145E-17,0.0332202089949022),
 .UNSPECIFIED.)
CURVE()
GEOMETRIC_REPRESENTATION_ITEM()
RATIONAL_B_SPLINE_CURVE((1.,1.,1.,1.))
REPRESENTATION_ITEM('')
);
#1184=(
BOUNDED_CURVE()
B_SPLINE_CURVE(3,(#175236,#175237,#175238,#175239),.UNSPECIFIED.,.F.,.F.)
B_SPLINE_CURVE_WITH_KNOTS((4,4),(0.,0.0360938777358061),.UNSPECIFIED.)
CURVE()
GEOMETRIC_REPRESENTATION_ITEM()
RATIONAL_B_SPLINE_CURVE((1.,1.,1.,1.))
REPRESENTATION_ITEM('')
);
#1185=(
BOUNDED_CURVE()
B_SPLINE_CURVE(3,(#175270,#175271,#175272,#175273),.UNSPECIFIED.,.F.,.F.)
B_SPLINE_CURVE_WITH_KNOTS((4,4),(0.,0.0358270578054484),.UNSPECIFIED.)
CURVE()
GEOMETRIC_REPRESENTATION_ITEM()
RATIONAL_B_SPLINE_CURVE((1.,1.,1.,1.))
REPRESENTATION_ITEM('')
);
#1186=(
BOUNDED_CURVE()
B_SPLINE_CURVE(3,(#175317,#175318,#175319,#175320),.UNSPECIFIED.,.F.,.F.)
B_SPLINE_CURVE_WITH_KNOTS((4,4),(0.,0.0372541843113205),.UNSPECIFIED.)
CURVE()
GEOMETRIC_REPRESENTATION_ITEM()
RATIONAL_B_SPLINE_CURVE((1.,1.,1.,1.))
REPRESENTATION_ITEM('')
);
#1187=(
BOUNDED_CURVE()
B_SPLINE_CURVE(3,(#175490,#175491,#175492,#175493),.UNSPECIFIED.,.F.,.F.)
B_SPLINE_CURVE_WITH_KNOTS((4,4),(0.,0.0369876550821707),.UNSPECIFIED.)
CURVE()
GEOMETRIC_REPRESENTATION_ITEM()
RATIONAL_B_SPLINE_CURVE((1.,1.,1.,1.))
REPRESENTATION_ITEM('')
);
#1188=(
BOUNDED_CURVE()
B_SPLINE_CURVE(3,(#175650,#175651,#175652,#175653),.UNSPECIFIED.,.F.,.F.)
B_SPLINE_CURVE_WITH_KNOTS((4,4),(0.,0.0385835973699829),.UNSPECIFIED.)
CURVE()
GEOMETRIC_REPRESENTATION_ITEM()
RATIONAL_B_SPLINE_CURVE((1.,1.,1.,1.))
REPRESENTATION_ITEM('')
);
#1189=(
BOUNDED_CURVE()
B_SPLINE_CURVE(3,(#175681,#175682,#175683,#175684),.UNSPECIFIED.,.F.,.F.)
B_SPLINE_CURVE_WITH_KNOTS((4,4),(0.,0.038317388945353),.UNSPECIFIED.)
CURVE()
GEOMETRIC_REPRESENTATION_ITEM()
RATIONAL_B_SPLINE_CURVE((1.,1.,1.,1.))
REPRESENTATION_ITEM('')
);
#1190=(
BOUNDED_CURVE()
B_SPLINE_CURVE(3,(#176882,#176883,#176884,#176885,#176886,#176887,#176888,
#176889,#176890,#176891),.UNSPECIFIED.,.F.,.F.)
B_SPLINE_CURVE_WITH_KNOTS((4,2,2,2,4),(4.71238898038469,5.10508806208341,
5.49778714378214,5.89048622548086,6.28318530717959),.UNSPECIFIED.)
CURVE()
GEOMETRIC_REPRESENTATION_ITEM()
RATIONAL_B_SPLINE_CURVE((1.,1.,1.,1.,1.,1.,1.,1.,1.,1.))
REPRESENTATION_ITEM('')
);
#1191=(
BOUNDED_CURVE()
B_SPLINE_CURVE(3,(#177941,#177942,#177943,#177944,#177945,#177946,#177947,
#177948,#177949,#177950),.UNSPECIFIED.,.F.,.F.)
B_SPLINE_CURVE_WITH_KNOTS((4,2,2,2,4),(1.5707963267949,1.96349540849362,
2.35619449019234,2.74889357189107,3.14159265358979),.UNSPECIFIED.)
CURVE()
GEOMETRIC_REPRESENTATION_ITEM()
RATIONAL_B_SPLINE_CURVE((1.,1.,1.,1.,1.,1.,1.,1.,1.,1.))
REPRESENTATION_ITEM('')
);
#1192=(
BOUNDED_CURVE()
B_SPLINE_CURVE(3,(#178325,#178326,#178327,#178328,#178329,#178330,#178331,
#178332,#178333,#178334),.UNSPECIFIED.,.F.,.F.)
B_SPLINE_CURVE_WITH_KNOTS((4,2,2,2,4),(1.5707963267949,1.96349540849362,
2.35619449019234,2.74889357189107,3.14159265358979),.UNSPECIFIED.)
CURVE()
GEOMETRIC_REPRESENTATION_ITEM()
RATIONAL_B_SPLINE_CURVE((1.,1.,1.,1.,1.,1.,1.,1.,1.,1.))
REPRESENTATION_ITEM('')
);
#1193=(
BOUNDED_CURVE()
B_SPLINE_CURVE(3,(#178526,#178527,#178528,#178529,#178530,#178531,#178532,
#178533,#178534,#178535),.UNSPECIFIED.,.F.,.F.)
B_SPLINE_CURVE_WITH_KNOTS((4,2,2,2,4),(3.1415926535898,3.53429173528852,
3.92699081698724,4.31968989868597,4.71238898038469),.UNSPECIFIED.)
CURVE()
GEOMETRIC_REPRESENTATION_ITEM()
RATIONAL_B_SPLINE_CURVE((1.,1.,1.,1.,1.,1.,1.,1.,1.,1.))
REPRESENTATION_ITEM('')
);
#1194=(
BOUNDED_CURVE()
B_SPLINE_CURVE(3,(#178822,#178823,#178824,#178825,#178826,#178827,#178828,
#178829,#178830,#178831),.UNSPECIFIED.,.F.,.F.)
B_SPLINE_CURVE_WITH_KNOTS((4,2,2,2,4),(4.71238898038469,5.10508806208342,
5.49778714378214,5.89048622548086,6.28318530717959),.UNSPECIFIED.)
CURVE()
GEOMETRIC_REPRESENTATION_ITEM()
RATIONAL_B_SPLINE_CURVE((1.,1.,1.,1.,1.,1.,1.,1.,1.,1.))
REPRESENTATION_ITEM('')
);
#1195=(
BOUNDED_CURVE()
B_SPLINE_CURVE(3,(#178949,#178950,#178951,#178952,#178953,#178954,#178955,
#178956,#178957,#178958),.UNSPECIFIED.,.F.,.F.)
B_SPLINE_CURVE_WITH_KNOTS((4,2,2,2,4),(-1.77635683940025E-15,0.392699081698723,
0.785398163397447,1.17809724509617,1.5707963267949),.UNSPECIFIED.)
CURVE()
GEOMETRIC_REPRESENTATION_ITEM()
RATIONAL_B_SPLINE_CURVE((1.,1.,1.,1.,1.,1.,1.,1.,1.,1.))
REPRESENTATION_ITEM('')
);
#1196=(
BOUNDED_CURVE()
B_SPLINE_CURVE(3,(#179176,#179177,#179178,#179179,#179180,#179181,#179182,
#179183,#179184,#179185),.UNSPECIFIED.,.F.,.F.)
B_SPLINE_CURVE_WITH_KNOTS((4,2,2,2,4),(4.71238898038469,5.10508806208342,
5.49778714378214,5.89048622548086,6.28318530717959),.UNSPECIFIED.)
CURVE()
GEOMETRIC_REPRESENTATION_ITEM()
RATIONAL_B_SPLINE_CURVE((1.,1.,1.,1.,1.,1.,1.,1.,1.,1.))
REPRESENTATION_ITEM('')
);
#1197=(
BOUNDED_CURVE()
B_SPLINE_CURVE(3,(#179405,#179406,#179407,#179408,#179409,#179410,#179411,
#179412,#179413,#179414),.UNSPECIFIED.,.F.,.F.)
B_SPLINE_CURVE_WITH_KNOTS((4,2,2,2,4),(-1.77635683940025E-15,0.392699081698723,
0.785398163397447,1.17809724509617,1.5707963267949),.UNSPECIFIED.)
CURVE()
GEOMETRIC_REPRESENTATION_ITEM()
RATIONAL_B_SPLINE_CURVE((1.,1.,1.,1.,1.,1.,1.,1.,1.,1.))
REPRESENTATION_ITEM('')
);
#1198=(
BOUNDED_CURVE()
B_SPLINE_CURVE(3,(#179630,#179631,#179632,#179633,#179634,#179635,#179636,
#179637,#179638,#179639),.UNSPECIFIED.,.F.,.F.)
B_SPLINE_CURVE_WITH_KNOTS((4,2,2,2,4),(1.5707963267949,1.96349540849362,
2.35619449019234,2.74889357189106,3.14159265358979),.UNSPECIFIED.)
CURVE()
GEOMETRIC_REPRESENTATION_ITEM()
RATIONAL_B_SPLINE_CURVE((1.,1.,1.,1.,1.,1.,1.,1.,1.,1.))
REPRESENTATION_ITEM('')
);
#1199=(
BOUNDED_CURVE()
B_SPLINE_CURVE(3,(#180140,#180141,#180142,#180143,#180144,#180145,#180146,
#180147,#180148,#180149),.UNSPECIFIED.,.F.,.F.)
B_SPLINE_CURVE_WITH_KNOTS((4,2,2,2,4),(3.1415926535898,3.53429173528852,
3.92699081698724,4.31968989868597,4.71238898038469),.UNSPECIFIED.)
CURVE()
GEOMETRIC_REPRESENTATION_ITEM()
RATIONAL_B_SPLINE_CURVE((1.,1.,1.,1.,1.,1.,1.,1.,1.,1.))
REPRESENTATION_ITEM('')
);
#1200=(
BOUNDED_CURVE()
B_SPLINE_CURVE(3,(#180362,#180363,#180364,#180365,#180366,#180367,#180368,
#180369,#180370,#180371),.UNSPECIFIED.,.F.,.F.)
B_SPLINE_CURVE_WITH_KNOTS((4,2,2,2,4),(4.71238898038469,5.10508806208341,
5.49778714378214,5.89048622548086,6.28318530717959),.UNSPECIFIED.)
CURVE()
GEOMETRIC_REPRESENTATION_ITEM()
RATIONAL_B_SPLINE_CURVE((1.,1.,1.,1.,1.,1.,1.,1.,1.,1.))
REPRESENTATION_ITEM('')
);
#1201=(
BOUNDED_CURVE()
B_SPLINE_CURVE(3,(#180489,#180490,#180491,#180492,#180493,#180494,#180495,
#180496,#180497,#180498),.UNSPECIFIED.,.F.,.F.)
B_SPLINE_CURVE_WITH_KNOTS((4,2,2,2,4),(0.,0.392699081698724,0.785398163397448,
1.17809724509617,1.5707963267949),.UNSPECIFIED.)
CURVE()
GEOMETRIC_REPRESENTATION_ITEM()
RATIONAL_B_SPLINE_CURVE((1.,1.,1.,1.,1.,1.,1.,1.,1.,1.))
REPRESENTATION_ITEM('')
);
#1202=(
BOUNDED_CURVE()
B_SPLINE_CURVE(3,(#180738,#180739,#180740,#180741,#180742,#180743,#180744,
#180745,#180746,#180747),.UNSPECIFIED.,.F.,.F.)
B_SPLINE_CURVE_WITH_KNOTS((4,2,2,2,4),(4.71238898038469,5.10508806208342,
5.49778714378214,5.89048622548086,6.28318530717959),.UNSPECIFIED.)
CURVE()
GEOMETRIC_REPRESENTATION_ITEM()
RATIONAL_B_SPLINE_CURVE((1.,1.,1.,1.,1.,1.,1.,1.,1.,1.))
REPRESENTATION_ITEM('')
);
#1203=(
BOUNDED_CURVE()
B_SPLINE_CURVE(3,(#180936,#180937,#180938,#180939,#180940,#180941,#180942,
#180943,#180944,#180945),.UNSPECIFIED.,.F.,.F.)
B_SPLINE_CURVE_WITH_KNOTS((4,2,2,2,4),(1.18015353016497E-15,0.392699081698726,
0.785398163397449,1.17809724509617,1.5707963267949),.UNSPECIFIED.)
CURVE()
GEOMETRIC_REPRESENTATION_ITEM()
RATIONAL_B_SPLINE_CURVE((1.,1.,1.,1.,1.,1.,1.,1.,1.,1.))
REPRESENTATION_ITEM('')
);
#1204=(
BOUNDED_CURVE()
B_SPLINE_CURVE(2,(#189315,#189316,#189317),.UNSPECIFIED.,.F.,.F.)
B_SPLINE_CURVE_WITH_KNOTS((3,3),(0.130611113351463,0.388312804292302),
 .UNSPECIFIED.)
CURVE()
GEOMETRIC_REPRESENTATION_ITEM()
RATIONAL_B_SPLINE_CURVE((1.30940107675848,1.51196612828735,1.30940107675849))
REPRESENTATION_ITEM('')
);
#1205=(
BOUNDED_CURVE()
B_SPLINE_CURVE(2,(#189320,#189321,#189322),.UNSPECIFIED.,.F.,.F.)
B_SPLINE_CURVE_WITH_KNOTS((3,3),(-1.16209721084497,-0.594066455576381),
 .UNSPECIFIED.)
CURVE()
GEOMETRIC_REPRESENTATION_ITEM()
RATIONAL_B_SPLINE_CURVE((2.95854811567268,3.41623710198805,2.95854811567267))
REPRESENTATION_ITEM('')
);
#1206=(
BOUNDED_CURVE()
B_SPLINE_CURVE(2,(#189327,#189328,#189329),.UNSPECIFIED.,.F.,.F.)
B_SPLINE_CURVE_WITH_KNOTS((3,3),(0.130611113351462,0.388312804292336),
 .UNSPECIFIED.)
CURVE()
GEOMETRIC_REPRESENTATION_ITEM()
RATIONAL_B_SPLINE_CURVE((1.30940107675853,1.51196612828747,1.30940107675849))
REPRESENTATION_ITEM('')
);
#1207=(
BOUNDED_CURVE()
B_SPLINE_CURVE(2,(#189330,#189331,#189332),.UNSPECIFIED.,.F.,.F.)
B_SPLINE_CURVE_WITH_KNOTS((3,3),(-1.16209721084502,-0.594066455576397),
 .UNSPECIFIED.)
CURVE()
GEOMETRIC_REPRESENTATION_ITEM()
RATIONAL_B_SPLINE_CURVE((2.95854811567274,3.41623710198818,2.95854811567276))
REPRESENTATION_ITEM('')
);
#1208=(
BOUNDED_CURVE()
B_SPLINE_CURVE(2,(#189337,#189338,#189339),.UNSPECIFIED.,.F.,.F.)
B_SPLINE_CURVE_WITH_KNOTS((3,3),(0.130611113351459,0.388312804292314),
 .UNSPECIFIED.)
CURVE()
GEOMETRIC_REPRESENTATION_ITEM()
RATIONAL_B_SPLINE_CURVE((1.30940107675849,1.51196612828739,1.3094010767585))
REPRESENTATION_ITEM('')
);
#1209=(
BOUNDED_CURVE()
B_SPLINE_CURVE(2,(#189340,#189341,#189342),.UNSPECIFIED.,.F.,.F.)
B_SPLINE_CURVE_WITH_KNOTS((3,3),(-1.16209721084514,-0.594066455576369),
 .UNSPECIFIED.)
CURVE()
GEOMETRIC_REPRESENTATION_ITEM()
RATIONAL_B_SPLINE_CURVE((2.95854811567259,3.4162371019884,2.95854811567281))
REPRESENTATION_ITEM('')
);
#1210=(
BOUNDED_CURVE()
B_SPLINE_CURVE(2,(#189347,#189348,#189349),.UNSPECIFIED.,.F.,.F.)
B_SPLINE_CURVE_WITH_KNOTS((3,3),(0.130611113351462,0.388312804292323),
 .UNSPECIFIED.)
CURVE()
GEOMETRIC_REPRESENTATION_ITEM()
RATIONAL_B_SPLINE_CURVE((1.30940107675851,1.51196612828743,1.30940107675851))
REPRESENTATION_ITEM('')
);
#1211=(
BOUNDED_CURVE()
B_SPLINE_CURVE(2,(#189350,#189351,#189352),.UNSPECIFIED.,.F.,.F.)
B_SPLINE_CURVE_WITH_KNOTS((3,3),(-1.16209721084512,-0.594066455576527),
 .UNSPECIFIED.)
CURVE()
GEOMETRIC_REPRESENTATION_ITEM()
RATIONAL_B_SPLINE_CURVE((2.95854811567258,3.41623710198823,2.95854811567305))
REPRESENTATION_ITEM('')
);
#1212=(
BOUNDED_CURVE()
B_SPLINE_CURVE(2,(#189357,#189358,#189359),.UNSPECIFIED.,.F.,.F.)
B_SPLINE_CURVE_WITH_KNOTS((3,3),(0.130611113351459,0.388312804292301),
 .UNSPECIFIED.)
CURVE()
GEOMETRIC_REPRESENTATION_ITEM()
RATIONAL_B_SPLINE_CURVE((1.30940107675849,1.51196612828738,1.30940107675852))
REPRESENTATION_ITEM('')
);
#1213=(
BOUNDED_CURVE()
B_SPLINE_CURVE(2,(#189360,#189361,#189362),.UNSPECIFIED.,.F.,.F.)
B_SPLINE_CURVE_WITH_KNOTS((3,3),(-1.16209721084525,-0.594066455576358),
 .UNSPECIFIED.)
CURVE()
GEOMETRIC_REPRESENTATION_ITEM()
RATIONAL_B_SPLINE_CURVE((2.95854811567222,3.41623710198829,2.95854811567264))
REPRESENTATION_ITEM('')
);
#1214=(
BOUNDED_CURVE()
B_SPLINE_CURVE(2,(#189364,#189365,#189366),.UNSPECIFIED.,.F.,.F.)
B_SPLINE_CURVE_WITH_KNOTS((3,3),(0.130611113351455,0.388312804292296),
 .UNSPECIFIED.)
CURVE()
GEOMETRIC_REPRESENTATION_ITEM()
RATIONAL_B_SPLINE_CURVE((1.30940107675851,1.51196612828741,1.30940107675853))
REPRESENTATION_ITEM('')
);
#1215=(
BOUNDED_CURVE()
B_SPLINE_CURVE(2,(#189367,#189368,#189369),.UNSPECIFIED.,.F.,.F.)
B_SPLINE_CURVE_WITH_KNOTS((3,3),(-1.16209721084501,-0.594066455576361),
 .UNSPECIFIED.)
CURVE()
GEOMETRIC_REPRESENTATION_ITEM()
RATIONAL_B_SPLINE_CURVE((2.95854811567265,3.41623710198812,2.95854811567266))
REPRESENTATION_ITEM('')
);
#1216=(
BOUNDED_CURVE()
B_SPLINE_CURVE(3,(#189448,#189449,#189450,#189451,#189452,#189453),
 .UNSPECIFIED.,.F.,.F.)
B_SPLINE_CURVE_WITH_KNOTS((4,2,4),(0.,0.5,1.),.UNSPECIFIED.)
CURVE()
GEOMETRIC_REPRESENTATION_ITEM()
RATIONAL_B_SPLINE_CURVE((0.999999993165193,0.99999999218853,0.99999999162755,
0.999999991625647,0.999999992188242,0.999999993165193))
REPRESENTATION_ITEM('')
);
#1217=(
BOUNDED_CURVE()
B_SPLINE_CURVE(3,(#195905,#195906,#195907,#195908),.UNSPECIFIED.,.F.,.F.)
B_SPLINE_CURVE_WITH_KNOTS((4,4),(0.,1.),.UNSPECIFIED.)
CURVE()
GEOMETRIC_REPRESENTATION_ITEM()
RATIONAL_B_SPLINE_CURVE((0.999999992674717,0.999999992656022,0.999999992624103,
0.999999992588127))
REPRESENTATION_ITEM('')
);
#1218=(
BOUNDED_CURVE()
B_SPLINE_CURVE(3,(#198545,#198546,#198547,#198548),.UNSPECIFIED.,.F.,.F.)
B_SPLINE_CURVE_WITH_KNOTS((4,4),(0.,1.),.UNSPECIFIED.)
CURVE()
GEOMETRIC_REPRESENTATION_ITEM()
RATIONAL_B_SPLINE_CURVE((0.999999999851496,0.999999999851229,0.999999999850917,
0.999999999850552))
REPRESENTATION_ITEM('')
);
#1219=(
BOUNDED_CURVE()
B_SPLINE_CURVE(3,(#198765,#198766,#198767,#198768,#198769,#198770,#198771,
#198772,#198773,#198774,#198775,#198776,#198777,#198778,#198779,#198780,
#198781,#198782,#198783,#198784),.UNSPECIFIED.,.F.,.F.)
B_SPLINE_CURVE_WITH_KNOTS((4,2,2,2,2,2,2,2,2,4),(0.,0.12500000000001,0.25,
0.37499999999999,0.437500000000004,0.5,0.62499999999999,0.75,0.87499999999999,
1.),.UNSPECIFIED.)
CURVE()
GEOMETRIC_REPRESENTATION_ITEM()
RATIONAL_B_SPLINE_CURVE((0.999999999812713,0.999999999813312,0.999999999814157,
0.999999999815449,0.999999999817637,0.999999999820964,0.999999999822179,
0.999999999824503,0.999999999825349,0.999999999827408,0.999999999828626,
0.999999999831746,0.999999999833571,0.999999999837455,0.999999999839621,
0.999999999844372,0.999999999846902,0.999999999851427,0.999999999853478,
0.999999999855875))
REPRESENTATION_ITEM('')
);
#1220=(
BOUNDED_CURVE()
B_SPLINE_CURVE(3,(#198941,#198942,#198943,#198944),.UNSPECIFIED.,.F.,.F.)
B_SPLINE_CURVE_WITH_KNOTS((4,4),(0.,1.),.UNSPECIFIED.)
CURVE()
GEOMETRIC_REPRESENTATION_ITEM()
RATIONAL_B_SPLINE_CURVE((0.999999998386268,0.999999998378396,0.999999998366988,
0.999999998354755))
REPRESENTATION_ITEM('')
);
#1221=(
BOUNDED_CURVE()
B_SPLINE_CURVE(3,(#199096,#199097,#199098,#199099,#199100,#199101),
 .UNSPECIFIED.,.F.,.F.)
B_SPLINE_CURVE_WITH_KNOTS((4,2,4),(0.,0.494420432466491,1.),
 .UNSPECIFIED.)
CURVE()
GEOMETRIC_REPRESENTATION_ITEM()
RATIONAL_B_SPLINE_CURVE((0.999999966703371,0.999999968198516,0.999999968156611,
0.999999966169366,0.999999964170887,0.999999961536821))
REPRESENTATION_ITEM('')
);
#1222=(
BOUNDED_CURVE()
B_SPLINE_CURVE(2,(#200177,#200178,#200179),.UNSPECIFIED.,.F.,.F.)
B_SPLINE_CURVE_WITH_KNOTS((3,3),(-0.866812823403001,-0.259568682604973),
 .UNSPECIFIED.)
CURVE()
GEOMETRIC_REPRESENTATION_ITEM()
RATIONAL_B_SPLINE_CURVE((1.00000103881537,1.00000117281535,1.00000060925137))
REPRESENTATION_ITEM('')
);
#1223=(
BOUNDED_CURVE()
B_SPLINE_CURVE(2,(#200193,#200194,#200195),.UNSPECIFIED.,.F.,.F.)
B_SPLINE_CURVE_WITH_KNOTS((3,3),(-1.23967788329125,-0.633513201114164),
 .UNSPECIFIED.)
CURVE()
GEOMETRIC_REPRESENTATION_ITEM()
RATIONAL_B_SPLINE_CURVE((1.00000061114393,1.00000117236832,1.00000103863036))
REPRESENTATION_ITEM('')
);
#1224=(
BOUNDED_CURVE()
B_SPLINE_CURVE(2,(#200212,#200213,#200214),.UNSPECIFIED.,.F.,.F.)
B_SPLINE_CURVE_WITH_KNOTS((3,3),(-1.24811202076719,-0.633513201181538),
 .UNSPECIFIED.)
CURVE()
GEOMETRIC_REPRESENTATION_ITEM()
RATIONAL_B_SPLINE_CURVE((1.00000059564287,1.00000117472449,1.00000103906851))
REPRESENTATION_ITEM('')
);
#1225=(
BOUNDED_CURVE()
B_SPLINE_CURVE(2,(#200228,#200229,#200230),.UNSPECIFIED.,.F.,.F.)
B_SPLINE_CURVE_WITH_KNOTS((3,3),(-0.866812823519123,-0.251975230958864),
 .UNSPECIFIED.)
CURVE()
GEOMETRIC_REPRESENTATION_ITEM()
RATIONAL_B_SPLINE_CURVE((1.00000103877905,1.00000117444993,1.00000059502701))
REPRESENTATION_ITEM('')
);
#1226=(
BOUNDED_CURVE()
B_SPLINE_CURVE(2,(#223366,#223367,#223368),.UNSPECIFIED.,.F.,.F.)
B_SPLINE_CURVE_WITH_KNOTS((3,3),(0.633513201322797,1.24075734212083),
 .UNSPECIFIED.)
CURVE()
GEOMETRIC_REPRESENTATION_ITEM()
RATIONAL_B_SPLINE_CURVE((1.00000103881537,1.00000117281535,1.00000060925137))
REPRESENTATION_ITEM('')
);
#1227=(
BOUNDED_CURVE()
B_SPLINE_CURVE(2,(#223382,#223383,#223384),.UNSPECIFIED.,.F.,.F.)
B_SPLINE_CURVE_WITH_KNOTS((3,3),(0.260648141434546,0.866812823611635),
 .UNSPECIFIED.)
CURVE()
GEOMETRIC_REPRESENTATION_ITEM()
RATIONAL_B_SPLINE_CURVE((1.00000061114393,1.00000117236832,1.00000103863036))
REPRESENTATION_ITEM('')
);
#1228=(
BOUNDED_CURVE()
B_SPLINE_CURVE(2,(#223401,#223402,#223403),.UNSPECIFIED.,.F.,.F.)
B_SPLINE_CURVE_WITH_KNOTS((3,3),(0.252214003958614,0.866812823544261),
 .UNSPECIFIED.)
CURVE()
GEOMETRIC_REPRESENTATION_ITEM()
RATIONAL_B_SPLINE_CURVE((1.00000059564287,1.00000117472449,1.00000103906851))
REPRESENTATION_ITEM('')
);
#1229=(
BOUNDED_CURVE()
B_SPLINE_CURVE(2,(#223417,#223418,#223419),.UNSPECIFIED.,.F.,.F.)
B_SPLINE_CURVE_WITH_KNOTS((3,3),(0.633513201206708,1.24835079376697),
 .UNSPECIFIED.)
CURVE()
GEOMETRIC_REPRESENTATION_ITEM()
RATIONAL_B_SPLINE_CURVE((1.00000103877905,1.00000117444993,1.00000059502701))
REPRESENTATION_ITEM('')
);
#1230=(
BOUNDED_CURVE()
B_SPLINE_CURVE(2,(#232817,#232818,#232819),.UNSPECIFIED.,.F.,.F.)
B_SPLINE_CURVE_WITH_KNOTS((3,3),(0.594066455576382,1.16209721084497),
 .UNSPECIFIED.)
CURVE()
GEOMETRIC_REPRESENTATION_ITEM()
RATIONAL_B_SPLINE_CURVE((2.95854811567267,3.41623710198805,2.95854811567268))
REPRESENTATION_ITEM('')
);
#1231=(
BOUNDED_CURVE()
B_SPLINE_CURVE(2,(#232822,#232823,#232824),.UNSPECIFIED.,.F.,.F.)
B_SPLINE_CURVE_WITH_KNOTS((3,3),(-0.388312804292316,-0.130611113351459),
 .UNSPECIFIED.)
CURVE()
GEOMETRIC_REPRESENTATION_ITEM()
RATIONAL_B_SPLINE_CURVE((1.30940107675847,1.51196612828737,1.30940107675848))
REPRESENTATION_ITEM('')
);
#1232=(
BOUNDED_CURVE()
B_SPLINE_CURVE(2,(#232829,#232830,#232831),.UNSPECIFIED.,.F.,.F.)
B_SPLINE_CURVE_WITH_KNOTS((3,3),(0.594066455576367,1.16209721084493),
 .UNSPECIFIED.)
CURVE()
GEOMETRIC_REPRESENTATION_ITEM()
RATIONAL_B_SPLINE_CURVE((2.95854811567267,3.41623710198805,2.95854811567278))
REPRESENTATION_ITEM('')
);
#1233=(
BOUNDED_CURVE()
B_SPLINE_CURVE(2,(#232832,#232833,#232834),.UNSPECIFIED.,.F.,.F.)
B_SPLINE_CURVE_WITH_KNOTS((3,3),(-0.388312804292315,-0.130611113351461),
 .UNSPECIFIED.)
CURVE()
GEOMETRIC_REPRESENTATION_ITEM()
RATIONAL_B_SPLINE_CURVE((1.30940107675852,1.51196612828742,1.30940107675851))
REPRESENTATION_ITEM('')
);
#1234=(
BOUNDED_CURVE()
B_SPLINE_CURVE(2,(#232839,#232840,#232841),.UNSPECIFIED.,.F.,.F.)
B_SPLINE_CURVE_WITH_KNOTS((3,3),(0.594066455576351,1.16209721084505),
 .UNSPECIFIED.)
CURVE()
GEOMETRIC_REPRESENTATION_ITEM()
RATIONAL_B_SPLINE_CURVE((2.95854811567277,3.41623710198832,2.95854811567269))
REPRESENTATION_ITEM('')
);
#1235=(
BOUNDED_CURVE()
B_SPLINE_CURVE(2,(#232842,#232843,#232844),.UNSPECIFIED.,.F.,.F.)
B_SPLINE_CURVE_WITH_KNOTS((3,3),(-0.388312804292322,-0.130611113351455),
 .UNSPECIFIED.)
CURVE()
GEOMETRIC_REPRESENTATION_ITEM()
RATIONAL_B_SPLINE_CURVE((1.30940107675848,1.5119661282874,1.30940107675849))
REPRESENTATION_ITEM('')
);
#1236=(
BOUNDED_CURVE()
B_SPLINE_CURVE(2,(#232849,#232850,#232851),.UNSPECIFIED.,.F.,.F.)
B_SPLINE_CURVE_WITH_KNOTS((3,3),(0.594066455576352,1.16209721084485),
 .UNSPECIFIED.)
CURVE()
GEOMETRIC_REPRESENTATION_ITEM()
RATIONAL_B_SPLINE_CURVE((2.95854811567277,3.41623710198815,2.95854811567302))
REPRESENTATION_ITEM('')
);
#1237=(
BOUNDED_CURVE()
B_SPLINE_CURVE(2,(#232852,#232853,#232854),.UNSPECIFIED.,.F.,.F.)
B_SPLINE_CURVE_WITH_KNOTS((3,3),(-0.388312804292316,-0.130611113351461),
 .UNSPECIFIED.)
CURVE()
GEOMETRIC_REPRESENTATION_ITEM()
RATIONAL_B_SPLINE_CURVE((1.30940107675852,1.51196612828743,1.30940107675851))
REPRESENTATION_ITEM('')
);
#1238=(
BOUNDED_CURVE()
B_SPLINE_CURVE(2,(#232859,#232860,#232861),.UNSPECIFIED.,.F.,.F.)
B_SPLINE_CURVE_WITH_KNOTS((3,3),(0.594066455576162,1.16209721084505),
 .UNSPECIFIED.)
CURVE()
GEOMETRIC_REPRESENTATION_ITEM()
RATIONAL_B_SPLINE_CURVE((2.95854811567234,3.41623710198832,2.95854811567258))
REPRESENTATION_ITEM('')
);
#1239=(
BOUNDED_CURVE()
B_SPLINE_CURVE(2,(#232862,#232863,#232864),.UNSPECIFIED.,.F.,.F.)
B_SPLINE_CURVE_WITH_KNOTS((3,3),(-0.388312804292327,-0.130611113351463),
 .UNSPECIFIED.)
CURVE()
GEOMETRIC_REPRESENTATION_ITEM()
RATIONAL_B_SPLINE_CURVE((1.30940107675851,1.51196612828743,1.30940107675852))
REPRESENTATION_ITEM('')
);
#1240=(
BOUNDED_CURVE()
B_SPLINE_CURVE(2,(#232866,#232867,#232868),.UNSPECIFIED.,.F.,.F.)
B_SPLINE_CURVE_WITH_KNOTS((3,3),(0.594066455576369,1.16209721084496),
 .UNSPECIFIED.)
CURVE()
GEOMETRIC_REPRESENTATION_ITEM()
RATIONAL_B_SPLINE_CURVE((2.95854811567278,3.4162371019882,2.95854811567281))
REPRESENTATION_ITEM('')
);
#1241=(
BOUNDED_CURVE()
B_SPLINE_CURVE(2,(#232869,#232870,#232871),.UNSPECIFIED.,.F.,.F.)
B_SPLINE_CURVE_WITH_KNOTS((3,3),(-0.388312804292311,-0.130611113351464),
 .UNSPECIFIED.)
CURVE()
GEOMETRIC_REPRESENTATION_ITEM()
RATIONAL_B_SPLINE_CURVE((1.30940107675851,1.51196612828742,1.30940107675852))
REPRESENTATION_ITEM('')
);
#1242=(
BOUNDED_CURVE()
B_SPLINE_CURVE(2,(#232916,#232917,#232918),.UNSPECIFIED.,.F.,.F.)
B_SPLINE_CURVE_WITH_KNOTS((3,3),(-1.46410161513778,-1.00000000000002),
 .UNSPECIFIED.)
CURVE()
GEOMETRIC_REPRESENTATION_ITEM()
RATIONAL_B_SPLINE_CURVE((1.39230484541328,1.50000000000003,1.50000000000003))
REPRESENTATION_ITEM('')
);
#1243=(
BOUNDED_CURVE()
B_SPLINE_CURVE(2,(#232919,#232920,#232921),.UNSPECIFIED.,.F.,.F.)
B_SPLINE_CURVE_WITH_KNOTS((3,3),(-1.00000000000002,-0.535898384862265),
 .UNSPECIFIED.)
CURVE()
GEOMETRIC_REPRESENTATION_ITEM()
RATIONAL_B_SPLINE_CURVE((1.50000000000001,1.50000000000001,1.39230484541328))
REPRESENTATION_ITEM('')
);
#1244=(
BOUNDED_CURVE()
B_SPLINE_CURVE(2,(#232924,#232925,#232926),.UNSPECIFIED.,.F.,.F.)
B_SPLINE_CURVE_WITH_KNOTS((3,3),(-1.00000000000002,-0.535898384862256),
 .UNSPECIFIED.)
CURVE()
GEOMETRIC_REPRESENTATION_ITEM()
RATIONAL_B_SPLINE_CURVE((1.50000000000003,1.50000000000003,1.39230484541329))
REPRESENTATION_ITEM('')
);
#1245=(
BOUNDED_CURVE()
B_SPLINE_CURVE(2,(#232927,#232928,#232929),.UNSPECIFIED.,.F.,.F.)
B_SPLINE_CURVE_WITH_KNOTS((3,3),(-1.46410161513777,-1.00000000000001),
 .UNSPECIFIED.)
CURVE()
GEOMETRIC_REPRESENTATION_ITEM()
RATIONAL_B_SPLINE_CURVE((1.39230484541327,1.50000000000001,1.50000000000001))
REPRESENTATION_ITEM('')
);
#1246=(
BOUNDED_CURVE()
B_SPLINE_CURVE(2,(#232932,#232933,#232934),.UNSPECIFIED.,.F.,.F.)
B_SPLINE_CURVE_WITH_KNOTS((3,3),(-1.00000000000001,-0.535898384862254),
 .UNSPECIFIED.)
CURVE()
GEOMETRIC_REPRESENTATION_ITEM()
RATIONAL_B_SPLINE_CURVE((1.50000000000001,1.50000000000001,1.39230484541328))
REPRESENTATION_ITEM('')
);
#1247=(
BOUNDED_CURVE()
B_SPLINE_CURVE(2,(#232935,#232936,#232937),.UNSPECIFIED.,.F.,.F.)
B_SPLINE_CURVE_WITH_KNOTS((3,3),(-1.46410161513775,-1.),.UNSPECIFIED.)
CURVE()
GEOMETRIC_REPRESENTATION_ITEM()
RATIONAL_B_SPLINE_CURVE((1.39230484541327,1.5,1.5))
REPRESENTATION_ITEM('')
);
#1248=(
BOUNDED_CURVE()
B_SPLINE_CURVE(2,(#232940,#232941,#232942),.UNSPECIFIED.,.F.,.F.)
B_SPLINE_CURVE_WITH_KNOTS((3,3),(-1.,-0.535898384862256),.UNSPECIFIED.)
CURVE()
GEOMETRIC_REPRESENTATION_ITEM()
RATIONAL_B_SPLINE_CURVE((1.5,1.5,1.39230484541327))
REPRESENTATION_ITEM('')
);
#1249=(
BOUNDED_CURVE()
B_SPLINE_CURVE(2,(#232943,#232944,#232945),.UNSPECIFIED.,.F.,.F.)
B_SPLINE_CURVE_WITH_KNOTS((3,3),(-1.46410161513776,-1.00000000000001),
 .UNSPECIFIED.)
CURVE()
GEOMETRIC_REPRESENTATION_ITEM()
RATIONAL_B_SPLINE_CURVE((1.39230484541327,1.5,1.5))
REPRESENTATION_ITEM('')
);
#1250=(
BOUNDED_CURVE()
B_SPLINE_CURVE(2,(#232948,#232949,#232950),.UNSPECIFIED.,.F.,.F.)
B_SPLINE_CURVE_WITH_KNOTS((3,3),(-1.00000000000001,-0.535898384862251),
 .UNSPECIFIED.)
CURVE()
GEOMETRIC_REPRESENTATION_ITEM()
RATIONAL_B_SPLINE_CURVE((1.5,1.50000000000001,1.39230484541327))
REPRESENTATION_ITEM('')
);
#1251=(
BOUNDED_CURVE()
B_SPLINE_CURVE(2,(#232951,#232952,#232953),.UNSPECIFIED.,.F.,.F.)
B_SPLINE_CURVE_WITH_KNOTS((3,3),(-1.46410161513775,-1.00000000000001),
 .UNSPECIFIED.)
CURVE()
GEOMETRIC_REPRESENTATION_ITEM()
RATIONAL_B_SPLINE_CURVE((1.39230484541326,1.49999999999999,1.49999999999999))
REPRESENTATION_ITEM('')
);
#1252=(
BOUNDED_CURVE()
B_SPLINE_CURVE(2,(#232956,#232957,#232958),.UNSPECIFIED.,.F.,.F.)
B_SPLINE_CURVE_WITH_KNOTS((3,3),(-1.00000000000001,-0.535898384862264),
 .UNSPECIFIED.)
CURVE()
GEOMETRIC_REPRESENTATION_ITEM()
RATIONAL_B_SPLINE_CURVE((1.49999999999999,1.49999999999999,1.39230484541326))
REPRESENTATION_ITEM('')
);
#1253=(
BOUNDED_CURVE()
B_SPLINE_CURVE(2,(#232959,#232960,#232961),.UNSPECIFIED.,.F.,.F.)
B_SPLINE_CURVE_WITH_KNOTS((3,3),(-1.46410161513776,-1.00000000000002),
 .UNSPECIFIED.)
CURVE()
GEOMETRIC_REPRESENTATION_ITEM()
RATIONAL_B_SPLINE_CURVE((1.39230484541327,1.5,1.50000000000001))
REPRESENTATION_ITEM('')
);
#1254=(
BOUNDED_CURVE()
B_SPLINE_CURVE(2,(#232977,#232978,#232979),.UNSPECIFIED.,.F.,.F.)
B_SPLINE_CURVE_WITH_KNOTS((3,3),(0.82874043787133,1.36602540378442),
 .UNSPECIFIED.)
CURVE()
GEOMETRIC_REPRESENTATION_ITEM()
RATIONAL_B_SPLINE_CURVE((1.73205080756822,1.86602540378445,1.86602540378445))
REPRESENTATION_ITEM('')
);
#1255=(
BOUNDED_CURVE()
B_SPLINE_CURVE(2,(#232980,#232981,#232982),.UNSPECIFIED.,.F.,.F.)
B_SPLINE_CURVE_WITH_KNOTS((3,3),(1.36602540378443,1.90331036969748),
 .UNSPECIFIED.)
CURVE()
GEOMETRIC_REPRESENTATION_ITEM()
RATIONAL_B_SPLINE_CURVE((1.86602540378443,1.86602540378443,1.73205080756823))
REPRESENTATION_ITEM('')
);
#1256=(
BOUNDED_CURVE()
B_SPLINE_CURVE(2,(#232985,#232986,#232987),.UNSPECIFIED.,.F.,.F.)
B_SPLINE_CURVE_WITH_KNOTS((3,3),(0.82874043787135,1.36602540378443),
 .UNSPECIFIED.)
CURVE()
GEOMETRIC_REPRESENTATION_ITEM()
RATIONAL_B_SPLINE_CURVE((1.73205080756821,1.86602540378443,1.86602540378443))
REPRESENTATION_ITEM('')
);
#1257=(
BOUNDED_CURVE()
B_SPLINE_CURVE(2,(#232988,#232989,#232990),.UNSPECIFIED.,.F.,.F.)
B_SPLINE_CURVE_WITH_KNOTS((3,3),(1.36602540378445,1.90331036969754),
 .UNSPECIFIED.)
CURVE()
GEOMETRIC_REPRESENTATION_ITEM()
RATIONAL_B_SPLINE_CURVE((1.86602540378445,1.86602540378445,1.73205080756823))
REPRESENTATION_ITEM('')
);
#1258=(
BOUNDED_CURVE()
B_SPLINE_CURVE(2,(#232993,#232994,#232995),.UNSPECIFIED.,.F.,.F.)
B_SPLINE_CURVE_WITH_KNOTS((3,3),(0.828740437871358,1.36602540378445),
 .UNSPECIFIED.)
CURVE()
GEOMETRIC_REPRESENTATION_ITEM()
RATIONAL_B_SPLINE_CURVE((1.73205080756824,1.86602540378446,1.86602540378445))
REPRESENTATION_ITEM('')
);
#1259=(
BOUNDED_CURVE()
B_SPLINE_CURVE(2,(#232996,#232997,#232998),.UNSPECIFIED.,.F.,.F.)
B_SPLINE_CURVE_WITH_KNOTS((3,3),(1.36602540378445,1.90331036969753),
 .UNSPECIFIED.)
CURVE()
GEOMETRIC_REPRESENTATION_ITEM()
RATIONAL_B_SPLINE_CURVE((1.86602540378444,1.86602540378444,1.73205080756822))
REPRESENTATION_ITEM('')
);
#1260=(
BOUNDED_CURVE()
B_SPLINE_CURVE(2,(#233001,#233002,#233003),.UNSPECIFIED.,.F.,.F.)
B_SPLINE_CURVE_WITH_KNOTS((3,3),(0.828740437871363,1.36602540378445),
 .UNSPECIFIED.)
CURVE()
GEOMETRIC_REPRESENTATION_ITEM()
RATIONAL_B_SPLINE_CURVE((1.73205080756823,1.86602540378444,1.86602540378444))
REPRESENTATION_ITEM('')
);
#1261=(
BOUNDED_CURVE()
B_SPLINE_CURVE(2,(#233004,#233005,#233006),.UNSPECIFIED.,.F.,.F.)
B_SPLINE_CURVE_WITH_KNOTS((3,3),(1.36602540378447,1.90331036969755),
 .UNSPECIFIED.)
CURVE()
GEOMETRIC_REPRESENTATION_ITEM()
RATIONAL_B_SPLINE_CURVE((1.86602540378447,1.86602540378447,1.73205080756825))
REPRESENTATION_ITEM('')
);
#1262=(
BOUNDED_CURVE()
B_SPLINE_CURVE(2,(#233009,#233010,#233011),.UNSPECIFIED.,.F.,.F.)
B_SPLINE_CURVE_WITH_KNOTS((3,3),(0.828740437871365,1.36602540378447),
 .UNSPECIFIED.)
CURVE()
GEOMETRIC_REPRESENTATION_ITEM()
RATIONAL_B_SPLINE_CURVE((1.73205080756825,1.86602540378447,1.86602540378447))
REPRESENTATION_ITEM('')
);
#1263=(
BOUNDED_CURVE()
B_SPLINE_CURVE(2,(#233012,#233013,#233014),.UNSPECIFIED.,.F.,.F.)
B_SPLINE_CURVE_WITH_KNOTS((3,3),(1.36602540378446,1.90331036969757),
 .UNSPECIFIED.)
CURVE()
GEOMETRIC_REPRESENTATION_ITEM()
RATIONAL_B_SPLINE_CURVE((1.8660254037845,1.8660254037845,1.73205080756827))
REPRESENTATION_ITEM('')
);
#1264=(
BOUNDED_CURVE()
B_SPLINE_CURVE(2,(#233017,#233018,#233019),.UNSPECIFIED.,.F.,.F.)
B_SPLINE_CURVE_WITH_KNOTS((3,3),(1.36602540378442,1.90331036969753),
 .UNSPECIFIED.)
CURVE()
GEOMETRIC_REPRESENTATION_ITEM()
RATIONAL_B_SPLINE_CURVE((1.86602540378445,1.86602540378446,1.73205080756824))
REPRESENTATION_ITEM('')
);
#1265=(
BOUNDED_CURVE()
B_SPLINE_CURVE(2,(#233020,#233021,#233022),.UNSPECIFIED.,.F.,.F.)
B_SPLINE_CURVE_WITH_KNOTS((3,3),(0.82874043787136,1.36602540378446),
 .UNSPECIFIED.)
CURVE()
GEOMETRIC_REPRESENTATION_ITEM()
RATIONAL_B_SPLINE_CURVE((1.73205080756826,1.86602540378449,1.8660254037845))
REPRESENTATION_ITEM('')
);
#1266=(
BOUNDED_CURVE()
B_SPLINE_CURVE(2,(#233050,#233051,#233052),.UNSPECIFIED.,.F.,.F.)
B_SPLINE_CURVE_WITH_KNOTS((3,3),(-1.46410161513776,-1.00000000000001),
 .UNSPECIFIED.)
CURVE()
GEOMETRIC_REPRESENTATION_ITEM()
RATIONAL_B_SPLINE_CURVE((1.39230484541327,1.50000000000001,1.50000000000001))
REPRESENTATION_ITEM('')
);
#1267=(
BOUNDED_CURVE()
B_SPLINE_CURVE(2,(#233053,#233054,#233055),.UNSPECIFIED.,.F.,.F.)
B_SPLINE_CURVE_WITH_KNOTS((3,3),(-1.,-0.535898384862256),.UNSPECIFIED.)
CURVE()
GEOMETRIC_REPRESENTATION_ITEM()
RATIONAL_B_SPLINE_CURVE((1.5,1.5,1.39230484541327))
REPRESENTATION_ITEM('')
);
#1268=(
BOUNDED_CURVE()
B_SPLINE_CURVE(2,(#233058,#233059,#233060),.UNSPECIFIED.,.F.,.F.)
B_SPLINE_CURVE_WITH_KNOTS((3,3),(-1.00000000000001,-0.535898384862251),
 .UNSPECIFIED.)
CURVE()
GEOMETRIC_REPRESENTATION_ITEM()
RATIONAL_B_SPLINE_CURVE((1.50000000000001,1.50000000000001,1.39230484541327))
REPRESENTATION_ITEM('')
);
#1269=(
BOUNDED_CURVE()
B_SPLINE_CURVE(2,(#233061,#233062,#233063),.UNSPECIFIED.,.F.,.F.)
B_SPLINE_CURVE_WITH_KNOTS((3,3),(-1.46410161513775,-1.),.UNSPECIFIED.)
CURVE()
GEOMETRIC_REPRESENTATION_ITEM()
RATIONAL_B_SPLINE_CURVE((1.39230484541326,1.5,1.5))
REPRESENTATION_ITEM('')
);
#1270=(
BOUNDED_CURVE()
B_SPLINE_CURVE(2,(#233066,#233067,#233068),.UNSPECIFIED.,.F.,.F.)
B_SPLINE_CURVE_WITH_KNOTS((3,3),(-1.,-0.535898384862256),.UNSPECIFIED.)
CURVE()
GEOMETRIC_REPRESENTATION_ITEM()
RATIONAL_B_SPLINE_CURVE((1.5,1.5,1.39230484541327))
REPRESENTATION_ITEM('')
);
#1271=(
BOUNDED_CURVE()
B_SPLINE_CURVE(2,(#233069,#233070,#233071),.UNSPECIFIED.,.F.,.F.)
B_SPLINE_CURVE_WITH_KNOTS((3,3),(-1.46410161513777,-1.),.UNSPECIFIED.)
CURVE()
GEOMETRIC_REPRESENTATION_ITEM()
RATIONAL_B_SPLINE_CURVE((1.39230484541326,1.5,1.5))
REPRESENTATION_ITEM('')
);
#1272=(
BOUNDED_CURVE()
B_SPLINE_CURVE(2,(#233074,#233075,#233076),.UNSPECIFIED.,.F.,.F.)
B_SPLINE_CURVE_WITH_KNOTS((3,3),(-1.,-0.535898384862258),.UNSPECIFIED.)
CURVE()
GEOMETRIC_REPRESENTATION_ITEM()
RATIONAL_B_SPLINE_CURVE((1.5,1.5,1.39230484541327))
REPRESENTATION_ITEM('')
);
#1273=(
BOUNDED_CURVE()
B_SPLINE_CURVE(2,(#233077,#233078,#233079),.UNSPECIFIED.,.F.,.F.)
B_SPLINE_CURVE_WITH_KNOTS((3,3),(-1.46410161513776,-1.),.UNSPECIFIED.)
CURVE()
GEOMETRIC_REPRESENTATION_ITEM()
RATIONAL_B_SPLINE_CURVE((1.39230484541327,1.50000000000001,1.50000000000001))
REPRESENTATION_ITEM('')
);
#1274=(
BOUNDED_CURVE()
B_SPLINE_CURVE(2,(#233082,#233083,#233084),.UNSPECIFIED.,.F.,.F.)
B_SPLINE_CURVE_WITH_KNOTS((3,3),(-1.,-0.535898384862256),.UNSPECIFIED.)
CURVE()
GEOMETRIC_REPRESENTATION_ITEM()
RATIONAL_B_SPLINE_CURVE((1.50000000000001,1.5,1.39230484541327))
REPRESENTATION_ITEM('')
);
#1275=(
BOUNDED_CURVE()
B_SPLINE_CURVE(2,(#233085,#233086,#233087),.UNSPECIFIED.,.F.,.F.)
B_SPLINE_CURVE_WITH_KNOTS((3,3),(-1.46410161513776,-1.00000000000001),
 .UNSPECIFIED.)
CURVE()
GEOMETRIC_REPRESENTATION_ITEM()
RATIONAL_B_SPLINE_CURVE((1.39230484541328,1.50000000000002,1.50000000000002))
REPRESENTATION_ITEM('')
);
#1276=(
BOUNDED_CURVE()
B_SPLINE_CURVE(2,(#233090,#233091,#233092),.UNSPECIFIED.,.F.,.F.)
B_SPLINE_CURVE_WITH_KNOTS((3,3),(-1.00000000000001,-0.535898384862248),
 .UNSPECIFIED.)
CURVE()
GEOMETRIC_REPRESENTATION_ITEM()
RATIONAL_B_SPLINE_CURVE((1.50000000000002,1.50000000000002,1.39230484541328))
REPRESENTATION_ITEM('')
);
#1277=(
BOUNDED_CURVE()
B_SPLINE_CURVE(2,(#233093,#233094,#233095),.UNSPECIFIED.,.F.,.F.)
B_SPLINE_CURVE_WITH_KNOTS((3,3),(-1.46410161513775,-1.),.UNSPECIFIED.)
CURVE()
GEOMETRIC_REPRESENTATION_ITEM()
RATIONAL_B_SPLINE_CURVE((1.39230484541327,1.5,1.5))
REPRESENTATION_ITEM('')
);
#1278=(
BOUNDED_CURVE()
B_SPLINE_CURVE(2,(#233111,#233112,#233113),.UNSPECIFIED.,.F.,.F.)
B_SPLINE_CURVE_WITH_KNOTS((3,3),(0.828740437871337,1.36602540378444),
 .UNSPECIFIED.)
CURVE()
GEOMETRIC_REPRESENTATION_ITEM()
RATIONAL_B_SPLINE_CURVE((1.73205080756821,1.86602540378444,1.86602540378444))
REPRESENTATION_ITEM('')
);
#1279=(
BOUNDED_CURVE()
B_SPLINE_CURVE(2,(#233114,#233115,#233116),.UNSPECIFIED.,.F.,.F.)
B_SPLINE_CURVE_WITH_KNOTS((3,3),(1.36602540378446,1.90331036969753),
 .UNSPECIFIED.)
CURVE()
GEOMETRIC_REPRESENTATION_ITEM()
RATIONAL_B_SPLINE_CURVE((1.86602540378447,1.86602540378447,1.73205080756826))
REPRESENTATION_ITEM('')
);
#1280=(
BOUNDED_CURVE()
B_SPLINE_CURVE(2,(#233119,#233120,#233121),.UNSPECIFIED.,.F.,.F.)
B_SPLINE_CURVE_WITH_KNOTS((3,3),(0.828740437871367,1.36602540378446),
 .UNSPECIFIED.)
CURVE()
GEOMETRIC_REPRESENTATION_ITEM()
RATIONAL_B_SPLINE_CURVE((1.73205080756825,1.86602540378447,1.86602540378447))
REPRESENTATION_ITEM('')
);
#1281=(
BOUNDED_CURVE()
B_SPLINE_CURVE(2,(#233122,#233123,#233124),.UNSPECIFIED.,.F.,.F.)
B_SPLINE_CURVE_WITH_KNOTS((3,3),(1.36602540378445,1.90331036969753),
 .UNSPECIFIED.)
CURVE()
GEOMETRIC_REPRESENTATION_ITEM()
RATIONAL_B_SPLINE_CURVE((1.86602540378445,1.86602540378445,1.73205080756823))
REPRESENTATION_ITEM('')
);
#1282=(
BOUNDED_CURVE()
B_SPLINE_CURVE(2,(#233127,#233128,#233129),.UNSPECIFIED.,.F.,.F.)
B_SPLINE_CURVE_WITH_KNOTS((3,3),(0.828740437871355,1.36602540378445),
 .UNSPECIFIED.)
CURVE()
GEOMETRIC_REPRESENTATION_ITEM()
RATIONAL_B_SPLINE_CURVE((1.73205080756823,1.86602540378445,1.86602540378445))
REPRESENTATION_ITEM('')
);
#1283=(
BOUNDED_CURVE()
B_SPLINE_CURVE(2,(#233130,#233131,#233132),.UNSPECIFIED.,.F.,.F.)
B_SPLINE_CURVE_WITH_KNOTS((3,3),(1.36602540378444,1.90331036969752),
 .UNSPECIFIED.)
CURVE()
GEOMETRIC_REPRESENTATION_ITEM()
RATIONAL_B_SPLINE_CURVE((1.86602540378444,1.86602540378444,1.73205080756823))
REPRESENTATION_ITEM('')
);
#1284=(
BOUNDED_CURVE()
B_SPLINE_CURVE(2,(#233135,#233136,#233137),.UNSPECIFIED.,.F.,.F.)
B_SPLINE_CURVE_WITH_KNOTS((3,3),(0.828740437871347,1.36602540378444),
 .UNSPECIFIED.)
CURVE()
GEOMETRIC_REPRESENTATION_ITEM()
RATIONAL_B_SPLINE_CURVE((1.73205080756822,1.86602540378444,1.86602540378444))
REPRESENTATION_ITEM('')
);
#1285=(
BOUNDED_CURVE()
B_SPLINE_CURVE(2,(#233138,#233139,#233140),.UNSPECIFIED.,.F.,.F.)
B_SPLINE_CURVE_WITH_KNOTS((3,3),(1.36602540378443,1.90331036969751),
 .UNSPECIFIED.)
CURVE()
GEOMETRIC_REPRESENTATION_ITEM()
RATIONAL_B_SPLINE_CURVE((1.86602540378443,1.86602540378444,1.73205080756823))
REPRESENTATION_ITEM('')
);
#1286=(
BOUNDED_CURVE()
B_SPLINE_CURVE(2,(#233143,#233144,#233145),.UNSPECIFIED.,.F.,.F.)
B_SPLINE_CURVE_WITH_KNOTS((3,3),(0.828740437871352,1.36602540378443),
 .UNSPECIFIED.)
CURVE()
GEOMETRIC_REPRESENTATION_ITEM()
RATIONAL_B_SPLINE_CURVE((1.73205080756822,1.86602540378443,1.86602540378443))
REPRESENTATION_ITEM('')
);
#1287=(
BOUNDED_CURVE()
B_SPLINE_CURVE(2,(#233146,#233147,#233148),.UNSPECIFIED.,.F.,.F.)
B_SPLINE_CURVE_WITH_KNOTS((3,3),(1.36602540378444,1.90331036969754),
 .UNSPECIFIED.)
CURVE()
GEOMETRIC_REPRESENTATION_ITEM()
RATIONAL_B_SPLINE_CURVE((1.86602540378445,1.86602540378445,1.73205080756823))
REPRESENTATION_ITEM('')
);
#1288=(
BOUNDED_CURVE()
B_SPLINE_CURVE(2,(#233151,#233152,#233153),.UNSPECIFIED.,.F.,.F.)
B_SPLINE_CURVE_WITH_KNOTS((3,3),(1.36602540378444,1.90331036969753),
 .UNSPECIFIED.)
CURVE()
GEOMETRIC_REPRESENTATION_ITEM()
RATIONAL_B_SPLINE_CURVE((1.86602540378444,1.86602540378444,1.73205080756822))
REPRESENTATION_ITEM('')
);
#1289=(
BOUNDED_CURVE()
B_SPLINE_CURVE(2,(#233154,#233155,#233156),.UNSPECIFIED.,.F.,.F.)
B_SPLINE_CURVE_WITH_KNOTS((3,3),(0.828740437871356,1.36602540378444),
 .UNSPECIFIED.)
CURVE()
GEOMETRIC_REPRESENTATION_ITEM()
RATIONAL_B_SPLINE_CURVE((1.73205080756823,1.86602540378445,1.86602540378445))
REPRESENTATION_ITEM('')
);
#1290=(
BOUNDED_CURVE()
B_SPLINE_CURVE(2,(#233174,#233175,#233176),.UNSPECIFIED.,.F.,.F.)
B_SPLINE_CURVE_WITH_KNOTS((3,3),(0.130611113351464,0.388312804292288),
 .UNSPECIFIED.)
CURVE()
GEOMETRIC_REPRESENTATION_ITEM()
RATIONAL_B_SPLINE_CURVE((1.30940107675847,1.51196612828731,1.30940107675848))
REPRESENTATION_ITEM('')
);
#1291=(
BOUNDED_CURVE()
B_SPLINE_CURVE(2,(#233179,#233180,#233181),.UNSPECIFIED.,.F.,.F.)
B_SPLINE_CURVE_WITH_KNOTS((3,3),(-1.16209721084502,-0.594066455576398),
 .UNSPECIFIED.)
CURVE()
GEOMETRIC_REPRESENTATION_ITEM()
RATIONAL_B_SPLINE_CURVE((2.95854811567252,3.41623710198795,2.95854811567259))
REPRESENTATION_ITEM('')
);
#1292=(
BOUNDED_CURVE()
B_SPLINE_CURVE(2,(#233186,#233187,#233188),.UNSPECIFIED.,.F.,.F.)
B_SPLINE_CURVE_WITH_KNOTS((3,3),(0.130611113351459,0.388312804292326),
 .UNSPECIFIED.)
CURVE()
GEOMETRIC_REPRESENTATION_ITEM()
RATIONAL_B_SPLINE_CURVE((1.30940107675853,1.51196612828746,1.30940107675851))
REPRESENTATION_ITEM('')
);
#1293=(
BOUNDED_CURVE()
B_SPLINE_CURVE(2,(#233189,#233190,#233191),.UNSPECIFIED.,.F.,.F.)
B_SPLINE_CURVE_WITH_KNOTS((3,3),(-1.16209721084504,-0.594066455576386),
 .UNSPECIFIED.)
CURVE()
GEOMETRIC_REPRESENTATION_ITEM()
RATIONAL_B_SPLINE_CURVE((2.95854811567252,3.416237101988,2.95854811567259))
REPRESENTATION_ITEM('')
);
#1294=(
BOUNDED_CURVE()
B_SPLINE_CURVE(2,(#233196,#233197,#233198),.UNSPECIFIED.,.F.,.F.)
B_SPLINE_CURVE_WITH_KNOTS((3,3),(0.130611113351456,0.388312804292303),
 .UNSPECIFIED.)
CURVE()
GEOMETRIC_REPRESENTATION_ITEM()
RATIONAL_B_SPLINE_CURVE((1.30940107675853,1.51196612828745,1.30940107675855))
REPRESENTATION_ITEM('')
);
#1295=(
BOUNDED_CURVE()
B_SPLINE_CURVE(2,(#233199,#233200,#233201),.UNSPECIFIED.,.F.,.F.)
B_SPLINE_CURVE_WITH_KNOTS((3,3),(-1.16209721084501,-0.594066455576338),
 .UNSPECIFIED.)
CURVE()
GEOMETRIC_REPRESENTATION_ITEM()
RATIONAL_B_SPLINE_CURVE((2.95854811567261,3.41623710198812,2.9585481156726))
REPRESENTATION_ITEM('')
);
#1296=(
BOUNDED_CURVE()
B_SPLINE_CURVE(2,(#233206,#233207,#233208),.UNSPECIFIED.,.F.,.F.)
B_SPLINE_CURVE_WITH_KNOTS((3,3),(0.130611113351459,0.388312804292329),
 .UNSPECIFIED.)
CURVE()
GEOMETRIC_REPRESENTATION_ITEM()
RATIONAL_B_SPLINE_CURVE((1.30940107675851,1.51196612828744,1.3094010767585))
REPRESENTATION_ITEM('')
);
#1297=(
BOUNDED_CURVE()
B_SPLINE_CURVE(2,(#233209,#233210,#233211),.UNSPECIFIED.,.F.,.F.)
B_SPLINE_CURVE_WITH_KNOTS((3,3),(-1.16209721084508,-0.594066455576527),
 .UNSPECIFIED.)
CURVE()
GEOMETRIC_REPRESENTATION_ITEM()
RATIONAL_B_SPLINE_CURVE((2.95854811567269,3.41623710198822,2.95854811567307))
REPRESENTATION_ITEM('')
);
#1298=(
BOUNDED_CURVE()
B_SPLINE_CURVE(2,(#233216,#233217,#233218),.UNSPECIFIED.,.F.,.F.)
B_SPLINE_CURVE_WITH_KNOTS((3,3),(0.130611113351453,0.388312804292305),
 .UNSPECIFIED.)
CURVE()
GEOMETRIC_REPRESENTATION_ITEM()
RATIONAL_B_SPLINE_CURVE((1.30940107675848,1.51196612828739,1.30940107675851))
REPRESENTATION_ITEM('')
);
#1299=(
BOUNDED_CURVE()
B_SPLINE_CURVE(2,(#233219,#233220,#233221),.UNSPECIFIED.,.F.,.F.)
B_SPLINE_CURVE_WITH_KNOTS((3,3),(-1.16209721084514,-0.594066455576349),
 .UNSPECIFIED.)
CURVE()
GEOMETRIC_REPRESENTATION_ITEM()
RATIONAL_B_SPLINE_CURVE((2.9585481156724,3.41623710198821,2.95854811567262))
REPRESENTATION_ITEM('')
);
#1300=(
BOUNDED_CURVE()
B_SPLINE_CURVE(2,(#233223,#233224,#233225),.UNSPECIFIED.,.F.,.F.)
B_SPLINE_CURVE_WITH_KNOTS((3,3),(0.130611113351457,0.388312804292304),
 .UNSPECIFIED.)
CURVE()
GEOMETRIC_REPRESENTATION_ITEM()
RATIONAL_B_SPLINE_CURVE((1.30940107675851,1.51196612828742,1.30940107675852))
REPRESENTATION_ITEM('')
);
#1301=(
BOUNDED_CURVE()
B_SPLINE_CURVE(2,(#233226,#233227,#233228),.UNSPECIFIED.,.F.,.F.)
B_SPLINE_CURVE_WITH_KNOTS((3,3),(-1.16209721084494,-0.594066455576379),
 .UNSPECIFIED.)
CURVE()
GEOMETRIC_REPRESENTATION_ITEM()
RATIONAL_B_SPLINE_CURVE((2.95854811567261,3.41623710198787,2.95854811567254))
REPRESENTATION_ITEM('')
);
#1302=(
BOUNDED_CURVE()
B_SPLINE_CURVE(2,(#234764,#234765,#234766),.UNSPECIFIED.,.F.,.F.)
B_SPLINE_CURVE_WITH_KNOTS((3,3),(-1.46410161513777,-1.00000000000001),
 .UNSPECIFIED.)
CURVE()
GEOMETRIC_REPRESENTATION_ITEM()
RATIONAL_B_SPLINE_CURVE((1.39230484541328,1.50000000000002,1.50000000000002))
REPRESENTATION_ITEM('')
);
#1303=(
BOUNDED_CURVE()
B_SPLINE_CURVE(2,(#234767,#234768,#234769),.UNSPECIFIED.,.F.,.F.)
B_SPLINE_CURVE_WITH_KNOTS((3,3),(-1.00000000000001,-0.535898384862261),
 .UNSPECIFIED.)
CURVE()
GEOMETRIC_REPRESENTATION_ITEM()
RATIONAL_B_SPLINE_CURVE((1.5,1.5,1.39230484541327))
REPRESENTATION_ITEM('')
);
#1304=(
BOUNDED_CURVE()
B_SPLINE_CURVE(2,(#234772,#234773,#234774),.UNSPECIFIED.,.F.,.F.)
B_SPLINE_CURVE_WITH_KNOTS((3,3),(-1.00000000000001,-0.535898384862254),
 .UNSPECIFIED.)
CURVE()
GEOMETRIC_REPRESENTATION_ITEM()
RATIONAL_B_SPLINE_CURVE((1.50000000000002,1.50000000000002,1.39230484541328))
REPRESENTATION_ITEM('')
);
#1305=(
BOUNDED_CURVE()
B_SPLINE_CURVE(2,(#234775,#234776,#234777),.UNSPECIFIED.,.F.,.F.)
B_SPLINE_CURVE_WITH_KNOTS((3,3),(-1.46410161513777,-1.),.UNSPECIFIED.)
CURVE()
GEOMETRIC_REPRESENTATION_ITEM()
RATIONAL_B_SPLINE_CURVE((1.39230484541327,1.50000000000001,1.50000000000001))
REPRESENTATION_ITEM('')
);
#1306=(
BOUNDED_CURVE()
B_SPLINE_CURVE(2,(#234780,#234781,#234782),.UNSPECIFIED.,.F.,.F.)
B_SPLINE_CURVE_WITH_KNOTS((3,3),(-1.,-0.535898384862249),.UNSPECIFIED.)
CURVE()
GEOMETRIC_REPRESENTATION_ITEM()
RATIONAL_B_SPLINE_CURVE((1.50000000000001,1.50000000000001,1.39230484541327))
REPRESENTATION_ITEM('')
);
#1307=(
BOUNDED_CURVE()
B_SPLINE_CURVE(2,(#234783,#234784,#234785),.UNSPECIFIED.,.F.,.F.)
B_SPLINE_CURVE_WITH_KNOTS((3,3),(-1.46410161513774,-0.99999999999999),
 .UNSPECIFIED.)
CURVE()
GEOMETRIC_REPRESENTATION_ITEM()
RATIONAL_B_SPLINE_CURVE((1.39230484541328,1.50000000000001,1.50000000000001))
REPRESENTATION_ITEM('')
);
#1308=(
BOUNDED_CURVE()
B_SPLINE_CURVE(2,(#234788,#234789,#234790),.UNSPECIFIED.,.F.,.F.)
B_SPLINE_CURVE_WITH_KNOTS((3,3),(-0.99999999999999,-0.535898384862251),
 .UNSPECIFIED.)
CURVE()
GEOMETRIC_REPRESENTATION_ITEM()
RATIONAL_B_SPLINE_CURVE((1.50000000000001,1.5,1.39230484541327))
REPRESENTATION_ITEM('')
);
#1309=(
BOUNDED_CURVE()
B_SPLINE_CURVE(2,(#234791,#234792,#234793),.UNSPECIFIED.,.F.,.F.)
B_SPLINE_CURVE_WITH_KNOTS((3,3),(-1.46410161513775,-1.),.UNSPECIFIED.)
CURVE()
GEOMETRIC_REPRESENTATION_ITEM()
RATIONAL_B_SPLINE_CURVE((1.39230484541327,1.5,1.5))
REPRESENTATION_ITEM('')
);
#1310=(
BOUNDED_CURVE()
B_SPLINE_CURVE(2,(#234796,#234797,#234798),.UNSPECIFIED.,.F.,.F.)
B_SPLINE_CURVE_WITH_KNOTS((3,3),(-1.,-0.53589838486225),.UNSPECIFIED.)
CURVE()
GEOMETRIC_REPRESENTATION_ITEM()
RATIONAL_B_SPLINE_CURVE((1.5,1.5,1.39230484541326))
REPRESENTATION_ITEM('')
);
#1311=(
BOUNDED_CURVE()
B_SPLINE_CURVE(2,(#234799,#234800,#234801),.UNSPECIFIED.,.F.,.F.)
B_SPLINE_CURVE_WITH_KNOTS((3,3),(-1.46410161513774,-1.),.UNSPECIFIED.)
CURVE()
GEOMETRIC_REPRESENTATION_ITEM()
RATIONAL_B_SPLINE_CURVE((1.39230484541326,1.49999999999999,1.49999999999999))
REPRESENTATION_ITEM('')
);
#1312=(
BOUNDED_CURVE()
B_SPLINE_CURVE(2,(#234804,#234805,#234806),.UNSPECIFIED.,.F.,.F.)
B_SPLINE_CURVE_WITH_KNOTS((3,3),(-1.,-0.535898384862254),.UNSPECIFIED.)
CURVE()
GEOMETRIC_REPRESENTATION_ITEM()
RATIONAL_B_SPLINE_CURVE((1.49999999999999,1.49999999999999,1.39230484541326))
REPRESENTATION_ITEM('')
);
#1313=(
BOUNDED_CURVE()
B_SPLINE_CURVE(2,(#234807,#234808,#234809),.UNSPECIFIED.,.F.,.F.)
B_SPLINE_CURVE_WITH_KNOTS((3,3),(-1.46410161513775,-1.00000000000001),
 .UNSPECIFIED.)
CURVE()
GEOMETRIC_REPRESENTATION_ITEM()
RATIONAL_B_SPLINE_CURVE((1.39230484541327,1.5,1.5))
REPRESENTATION_ITEM('')
);
#1314=(
BOUNDED_CURVE()
B_SPLINE_CURVE(2,(#234825,#234826,#234827),.UNSPECIFIED.,.F.,.F.)
B_SPLINE_CURVE_WITH_KNOTS((3,3),(0.828740437871318,1.36602540378443),
 .UNSPECIFIED.)
CURVE()
GEOMETRIC_REPRESENTATION_ITEM()
RATIONAL_B_SPLINE_CURVE((1.73205080756821,1.86602540378444,1.86602540378444))
REPRESENTATION_ITEM('')
);
#1315=(
BOUNDED_CURVE()
B_SPLINE_CURVE(2,(#234828,#234829,#234830),.UNSPECIFIED.,.F.,.F.)
B_SPLINE_CURVE_WITH_KNOTS((3,3),(1.36602540378443,1.90331036969749),
 .UNSPECIFIED.)
CURVE()
GEOMETRIC_REPRESENTATION_ITEM()
RATIONAL_B_SPLINE_CURVE((1.86602540378444,1.86602540378444,1.73205080756824))
REPRESENTATION_ITEM('')
);
#1316=(
BOUNDED_CURVE()
B_SPLINE_CURVE(2,(#234833,#234834,#234835),.UNSPECIFIED.,.F.,.F.)
B_SPLINE_CURVE_WITH_KNOTS((3,3),(0.828740437871351,1.36602540378443),
 .UNSPECIFIED.)
CURVE()
GEOMETRIC_REPRESENTATION_ITEM()
RATIONAL_B_SPLINE_CURVE((1.73205080756822,1.86602540378444,1.86602540378444))
REPRESENTATION_ITEM('')
);
#1317=(
BOUNDED_CURVE()
B_SPLINE_CURVE(2,(#234836,#234837,#234838),.UNSPECIFIED.,.F.,.F.)
B_SPLINE_CURVE_WITH_KNOTS((3,3),(1.36602540378444,1.90331036969753),
 .UNSPECIFIED.)
CURVE()
GEOMETRIC_REPRESENTATION_ITEM()
RATIONAL_B_SPLINE_CURVE((1.86602540378444,1.86602540378444,1.73205080756822))
REPRESENTATION_ITEM('')
);
#1318=(
BOUNDED_CURVE()
B_SPLINE_CURVE(2,(#234841,#234842,#234843),.UNSPECIFIED.,.F.,.F.)
B_SPLINE_CURVE_WITH_KNOTS((3,3),(0.82874043787136,1.36602540378444),
 .UNSPECIFIED.)
CURVE()
GEOMETRIC_REPRESENTATION_ITEM()
RATIONAL_B_SPLINE_CURVE((1.73205080756822,1.86602540378444,1.86602540378444))
REPRESENTATION_ITEM('')
);
#1319=(
BOUNDED_CURVE()
B_SPLINE_CURVE(2,(#234844,#234845,#234846),.UNSPECIFIED.,.F.,.F.)
B_SPLINE_CURVE_WITH_KNOTS((3,3),(1.36602540378446,1.90331036969753),
 .UNSPECIFIED.)
CURVE()
GEOMETRIC_REPRESENTATION_ITEM()
RATIONAL_B_SPLINE_CURVE((1.86602540378445,1.86602540378444,1.73205080756823))
REPRESENTATION_ITEM('')
);
#1320=(
BOUNDED_CURVE()
B_SPLINE_CURVE(2,(#234849,#234850,#234851),.UNSPECIFIED.,.F.,.F.)
B_SPLINE_CURVE_WITH_KNOTS((3,3),(0.82874043787137,1.36602540378446),
 .UNSPECIFIED.)
CURVE()
GEOMETRIC_REPRESENTATION_ITEM()
RATIONAL_B_SPLINE_CURVE((1.73205080756824,1.86602540378445,1.86602540378445))
REPRESENTATION_ITEM('')
);
#1321=(
BOUNDED_CURVE()
B_SPLINE_CURVE(2,(#234852,#234853,#234854),.UNSPECIFIED.,.F.,.F.)
B_SPLINE_CURVE_WITH_KNOTS((3,3),(1.36602540378446,1.90331036969755),
 .UNSPECIFIED.)
CURVE()
GEOMETRIC_REPRESENTATION_ITEM()
RATIONAL_B_SPLINE_CURVE((1.86602540378447,1.86602540378446,1.73205080756824))
REPRESENTATION_ITEM('')
);
#1322=(
BOUNDED_CURVE()
B_SPLINE_CURVE(2,(#234857,#234858,#234859),.UNSPECIFIED.,.F.,.F.)
B_SPLINE_CURVE_WITH_KNOTS((3,3),(0.828740437871358,1.36602540378446),
 .UNSPECIFIED.)
CURVE()
GEOMETRIC_REPRESENTATION_ITEM()
RATIONAL_B_SPLINE_CURVE((1.73205080756824,1.86602540378447,1.86602540378447))
REPRESENTATION_ITEM('')
);
#1323=(
BOUNDED_CURVE()
B_SPLINE_CURVE(2,(#234860,#234861,#234862),.UNSPECIFIED.,.F.,.F.)
B_SPLINE_CURVE_WITH_KNOTS((3,3),(1.36602540378446,1.90331036969755),
 .UNSPECIFIED.)
CURVE()
GEOMETRIC_REPRESENTATION_ITEM()
RATIONAL_B_SPLINE_CURVE((1.86602540378446,1.86602540378446,1.73205080756824))
REPRESENTATION_ITEM('')
);
#1324=(
BOUNDED_CURVE()
B_SPLINE_CURVE(2,(#234865,#234866,#234867),.UNSPECIFIED.,.F.,.F.)
B_SPLINE_CURVE_WITH_KNOTS((3,3),(1.36602540378443,1.90331036969752),
 .UNSPECIFIED.)
CURVE()
GEOMETRIC_REPRESENTATION_ITEM()
RATIONAL_B_SPLINE_CURVE((1.86602540378444,1.86602540378445,1.73205080756823))
REPRESENTATION_ITEM('')
);
#1325=(
BOUNDED_CURVE()
B_SPLINE_CURVE(2,(#234868,#234869,#234870),.UNSPECIFIED.,.F.,.F.)
B_SPLINE_CURVE_WITH_KNOTS((3,3),(0.828740437871363,1.36602540378446),
 .UNSPECIFIED.)
CURVE()
GEOMETRIC_REPRESENTATION_ITEM()
RATIONAL_B_SPLINE_CURVE((1.73205080756824,1.86602540378447,1.86602540378446))
REPRESENTATION_ITEM('')
);
#1326=(
BOUNDED_CURVE()
B_SPLINE_CURVE(2,(#234898,#234899,#234900),.UNSPECIFIED.,.F.,.F.)
B_SPLINE_CURVE_WITH_KNOTS((3,3),(-1.46410161513776,-1.00000000000001),
 .UNSPECIFIED.)
CURVE()
GEOMETRIC_REPRESENTATION_ITEM()
RATIONAL_B_SPLINE_CURVE((1.39230484541327,1.5,1.5))
REPRESENTATION_ITEM('')
);
#1327=(
BOUNDED_CURVE()
B_SPLINE_CURVE(2,(#234901,#234902,#234903),.UNSPECIFIED.,.F.,.F.)
B_SPLINE_CURVE_WITH_KNOTS((3,3),(-1.,-0.535898384862256),.UNSPECIFIED.)
CURVE()
GEOMETRIC_REPRESENTATION_ITEM()
RATIONAL_B_SPLINE_CURVE((1.5,1.5,1.39230484541327))
REPRESENTATION_ITEM('')
);
#1328=(
BOUNDED_CURVE()
B_SPLINE_CURVE(2,(#234906,#234907,#234908),.UNSPECIFIED.,.F.,.F.)
B_SPLINE_CURVE_WITH_KNOTS((3,3),(-1.00000000000001,-0.535898384862261),
 .UNSPECIFIED.)
CURVE()
GEOMETRIC_REPRESENTATION_ITEM()
RATIONAL_B_SPLINE_CURVE((1.5,1.5,1.39230484541327))
REPRESENTATION_ITEM('')
);
#1329=(
BOUNDED_CURVE()
B_SPLINE_CURVE(2,(#234909,#234910,#234911),.UNSPECIFIED.,.F.,.F.)
B_SPLINE_CURVE_WITH_KNOTS((3,3),(-1.46410161513776,-1.),.UNSPECIFIED.)
CURVE()
GEOMETRIC_REPRESENTATION_ITEM()
RATIONAL_B_SPLINE_CURVE((1.39230484541328,1.50000000000002,1.50000000000002))
REPRESENTATION_ITEM('')
);
#1330=(
BOUNDED_CURVE()
B_SPLINE_CURVE(2,(#234914,#234915,#234916),.UNSPECIFIED.,.F.,.F.)
B_SPLINE_CURVE_WITH_KNOTS((3,3),(-1.,-0.53589838486225),.UNSPECIFIED.)
CURVE()
GEOMETRIC_REPRESENTATION_ITEM()
RATIONAL_B_SPLINE_CURVE((1.50000000000002,1.50000000000002,1.39230484541328))
REPRESENTATION_ITEM('')
);
#1331=(
BOUNDED_CURVE()
B_SPLINE_CURVE(2,(#234917,#234918,#234919),.UNSPECIFIED.,.F.,.F.)
B_SPLINE_CURVE_WITH_KNOTS((3,3),(-1.46410161513775,-1.00000000000001),
 .UNSPECIFIED.)
CURVE()
GEOMETRIC_REPRESENTATION_ITEM()
RATIONAL_B_SPLINE_CURVE((1.39230484541327,1.5,1.50000000000001))
REPRESENTATION_ITEM('')
);
#1332=(
BOUNDED_CURVE()
B_SPLINE_CURVE(2,(#234922,#234923,#234924),.UNSPECIFIED.,.F.,.F.)
B_SPLINE_CURVE_WITH_KNOTS((3,3),(-1.00000000000001,-0.535898384862254),
 .UNSPECIFIED.)
CURVE()
GEOMETRIC_REPRESENTATION_ITEM()
RATIONAL_B_SPLINE_CURVE((1.50000000000001,1.50000000000001,1.39230484541327))
REPRESENTATION_ITEM('')
);
#1333=(
BOUNDED_CURVE()
B_SPLINE_CURVE(2,(#234925,#234926,#234927),.UNSPECIFIED.,.F.,.F.)
B_SPLINE_CURVE_WITH_KNOTS((3,3),(-1.46410161513775,-1.00000000000001),
 .UNSPECIFIED.)
CURVE()
GEOMETRIC_REPRESENTATION_ITEM()
RATIONAL_B_SPLINE_CURVE((1.39230484541328,1.50000000000001,1.50000000000001))
REPRESENTATION_ITEM('')
);
#1334=(
BOUNDED_CURVE()
B_SPLINE_CURVE(2,(#234930,#234931,#234932),.UNSPECIFIED.,.F.,.F.)
B_SPLINE_CURVE_WITH_KNOTS((3,3),(-1.00000000000001,-0.535898384862257),
 .UNSPECIFIED.)
CURVE()
GEOMETRIC_REPRESENTATION_ITEM()
RATIONAL_B_SPLINE_CURVE((1.5,1.5,1.39230484541327))
REPRESENTATION_ITEM('')
);
#1335=(
BOUNDED_CURVE()
B_SPLINE_CURVE(2,(#234933,#234934,#234935),.UNSPECIFIED.,.F.,.F.)
B_SPLINE_CURVE_WITH_KNOTS((3,3),(-1.46410161513775,-1.00000000000001),
 .UNSPECIFIED.)
CURVE()
GEOMETRIC_REPRESENTATION_ITEM()
RATIONAL_B_SPLINE_CURVE((1.39230484541328,1.50000000000001,1.50000000000001))
REPRESENTATION_ITEM('')
);
#1336=(
BOUNDED_CURVE()
B_SPLINE_CURVE(2,(#234938,#234939,#234940),.UNSPECIFIED.,.F.,.F.)
B_SPLINE_CURVE_WITH_KNOTS((3,3),(-1.00000000000001,-0.535898384862249),
 .UNSPECIFIED.)
CURVE()
GEOMETRIC_REPRESENTATION_ITEM()
RATIONAL_B_SPLINE_CURVE((1.50000000000002,1.50000000000002,1.39230484541328))
REPRESENTATION_ITEM('')
);
#1337=(
BOUNDED_CURVE()
B_SPLINE_CURVE(2,(#234941,#234942,#234943),.UNSPECIFIED.,.F.,.F.)
B_SPLINE_CURVE_WITH_KNOTS((3,3),(-1.46410161513775,-1.),.UNSPECIFIED.)
CURVE()
GEOMETRIC_REPRESENTATION_ITEM()
RATIONAL_B_SPLINE_CURVE((1.39230484541327,1.5,1.5))
REPRESENTATION_ITEM('')
);
#1338=(
BOUNDED_CURVE()
B_SPLINE_CURVE(2,(#234959,#234960,#234961),.UNSPECIFIED.,.F.,.F.)
B_SPLINE_CURVE_WITH_KNOTS((3,3),(0.828740437871322,1.36602540378445),
 .UNSPECIFIED.)
CURVE()
GEOMETRIC_REPRESENTATION_ITEM()
RATIONAL_B_SPLINE_CURVE((1.7320508075682,1.86602540378444,1.86602540378444))
REPRESENTATION_ITEM('')
);
#1339=(
BOUNDED_CURVE()
B_SPLINE_CURVE(2,(#234962,#234963,#234964),.UNSPECIFIED.,.F.,.F.)
B_SPLINE_CURVE_WITH_KNOTS((3,3),(1.36602540378446,1.90331036969753),
 .UNSPECIFIED.)
CURVE()
GEOMETRIC_REPRESENTATION_ITEM()
RATIONAL_B_SPLINE_CURVE((1.86602540378447,1.86602540378447,1.73205080756826))
REPRESENTATION_ITEM('')
);
#1340=(
BOUNDED_CURVE()
B_SPLINE_CURVE(2,(#234967,#234968,#234969),.UNSPECIFIED.,.F.,.F.)
B_SPLINE_CURVE_WITH_KNOTS((3,3),(0.828740437871366,1.36602540378446),
 .UNSPECIFIED.)
CURVE()
GEOMETRIC_REPRESENTATION_ITEM()
RATIONAL_B_SPLINE_CURVE((1.73205080756825,1.86602540378447,1.86602540378447))
REPRESENTATION_ITEM('')
);
#1341=(
BOUNDED_CURVE()
B_SPLINE_CURVE(2,(#234970,#234971,#234972),.UNSPECIFIED.,.F.,.F.)
B_SPLINE_CURVE_WITH_KNOTS((3,3),(1.36602540378446,1.90331036969754),
 .UNSPECIFIED.)
CURVE()
GEOMETRIC_REPRESENTATION_ITEM()
RATIONAL_B_SPLINE_CURVE((1.86602540378445,1.86602540378445,1.73205080756824))
REPRESENTATION_ITEM('')
);
#1342=(
BOUNDED_CURVE()
B_SPLINE_CURVE(2,(#234975,#234976,#234977),.UNSPECIFIED.,.F.,.F.)
B_SPLINE_CURVE_WITH_KNOTS((3,3),(0.828740437871359,1.36602540378446),
 .UNSPECIFIED.)
CURVE()
GEOMETRIC_REPRESENTATION_ITEM()
RATIONAL_B_SPLINE_CURVE((1.73205080756823,1.86602540378446,1.86602540378445))
REPRESENTATION_ITEM('')
);
#1343=(
BOUNDED_CURVE()
B_SPLINE_CURVE(2,(#234978,#234979,#234980),.UNSPECIFIED.,.F.,.F.)
B_SPLINE_CURVE_WITH_KNOTS((3,3),(1.36602540378444,1.90331036969751),
 .UNSPECIFIED.)
CURVE()
GEOMETRIC_REPRESENTATION_ITEM()
RATIONAL_B_SPLINE_CURVE((1.86602540378444,1.86602540378444,1.73205080756823))
REPRESENTATION_ITEM('')
);
#1344=(
BOUNDED_CURVE()
B_SPLINE_CURVE(2,(#234983,#234984,#234985),.UNSPECIFIED.,.F.,.F.)
B_SPLINE_CURVE_WITH_KNOTS((3,3),(0.828740437871355,1.36602540378444),
 .UNSPECIFIED.)
CURVE()
GEOMETRIC_REPRESENTATION_ITEM()
RATIONAL_B_SPLINE_CURVE((1.73205080756823,1.86602540378444,1.86602540378444))
REPRESENTATION_ITEM('')
);
#1345=(
BOUNDED_CURVE()
B_SPLINE_CURVE(2,(#234986,#234987,#234988),.UNSPECIFIED.,.F.,.F.)
B_SPLINE_CURVE_WITH_KNOTS((3,3),(1.36602540378447,1.90331036969758),
 .UNSPECIFIED.)
CURVE()
GEOMETRIC_REPRESENTATION_ITEM()
RATIONAL_B_SPLINE_CURVE((1.8660254037845,1.86602540378449,1.73205080756826))
REPRESENTATION_ITEM('')
);
#1346=(
BOUNDED_CURVE()
B_SPLINE_CURVE(2,(#234991,#234992,#234993),.UNSPECIFIED.,.F.,.F.)
B_SPLINE_CURVE_WITH_KNOTS((3,3),(0.828740437871367,1.36602540378446),
 .UNSPECIFIED.)
CURVE()
GEOMETRIC_REPRESENTATION_ITEM()
RATIONAL_B_SPLINE_CURVE((1.73205080756826,1.86602540378449,1.86602540378449))
REPRESENTATION_ITEM('')
);
#1347=(
BOUNDED_CURVE()
B_SPLINE_CURVE(2,(#234994,#234995,#234996),.UNSPECIFIED.,.F.,.F.)
B_SPLINE_CURVE_WITH_KNOTS((3,3),(1.36602540378445,1.90331036969752),
 .UNSPECIFIED.)
CURVE()
GEOMETRIC_REPRESENTATION_ITEM()
RATIONAL_B_SPLINE_CURVE((1.86602540378444,1.86602540378444,1.73205080756823))
REPRESENTATION_ITEM('')
);
#1348=(
BOUNDED_CURVE()
B_SPLINE_CURVE(2,(#234999,#235000,#235001),.UNSPECIFIED.,.F.,.F.)
B_SPLINE_CURVE_WITH_KNOTS((3,3),(1.36602540378445,1.90331036969753),
 .UNSPECIFIED.)
CURVE()
GEOMETRIC_REPRESENTATION_ITEM()
RATIONAL_B_SPLINE_CURVE((1.86602540378444,1.86602540378444,1.73205080756822))
REPRESENTATION_ITEM('')
);
#1349=(
BOUNDED_CURVE()
B_SPLINE_CURVE(2,(#235002,#235003,#235004),.UNSPECIFIED.,.F.,.F.)
B_SPLINE_CURVE_WITH_KNOTS((3,3),(0.828740437871357,1.36602540378444),
 .UNSPECIFIED.)
CURVE()
GEOMETRIC_REPRESENTATION_ITEM()
RATIONAL_B_SPLINE_CURVE((1.73205080756823,1.86602540378444,1.86602540378444))
REPRESENTATION_ITEM('')
);
#1350=(
BOUNDED_CURVE()
B_SPLINE_CURVE(2,(#235022,#235023,#235024),.UNSPECIFIED.,.F.,.F.)
B_SPLINE_CURVE_WITH_KNOTS((3,3),(0.594066455576395,1.16209721084489),
 .UNSPECIFIED.)
CURVE()
GEOMETRIC_REPRESENTATION_ITEM()
RATIONAL_B_SPLINE_CURVE((2.95854811567256,3.4162371019878,2.95854811567265))
REPRESENTATION_ITEM('')
);
#1351=(
BOUNDED_CURVE()
B_SPLINE_CURVE(2,(#235027,#235028,#235029),.UNSPECIFIED.,.F.,.F.)
B_SPLINE_CURVE_WITH_KNOTS((3,3),(-0.388312804292301,-0.130611113351461),
 .UNSPECIFIED.)
CURVE()
GEOMETRIC_REPRESENTATION_ITEM()
RATIONAL_B_SPLINE_CURVE((1.30940107675846,1.51196612828732,1.30940107675846))
REPRESENTATION_ITEM('')
);
#1352=(
BOUNDED_CURVE()
B_SPLINE_CURVE(2,(#235034,#235035,#235036),.UNSPECIFIED.,.F.,.F.)
B_SPLINE_CURVE_WITH_KNOTS((3,3),(0.594066455576358,1.16209721084491),
 .UNSPECIFIED.)
CURVE()
GEOMETRIC_REPRESENTATION_ITEM()
RATIONAL_B_SPLINE_CURVE((2.95854811567265,3.41623710198804,2.95854811567281))
REPRESENTATION_ITEM('')
);
#1353=(
BOUNDED_CURVE()
B_SPLINE_CURVE(2,(#235037,#235038,#235039),.UNSPECIFIED.,.F.,.F.)
B_SPLINE_CURVE_WITH_KNOTS((3,3),(-0.388312804292316,-0.130611113351459),
 .UNSPECIFIED.)
CURVE()
GEOMETRIC_REPRESENTATION_ITEM()
RATIONAL_B_SPLINE_CURVE((1.30940107675852,1.51196612828743,1.30940107675851))
REPRESENTATION_ITEM('')
);
#1354=(
BOUNDED_CURVE()
B_SPLINE_CURVE(2,(#235044,#235045,#235046),.UNSPECIFIED.,.F.,.F.)
B_SPLINE_CURVE_WITH_KNOTS((3,3),(0.59406645557637,1.16209721084499),
 .UNSPECIFIED.)
CURVE()
GEOMETRIC_REPRESENTATION_ITEM()
RATIONAL_B_SPLINE_CURVE((2.95854811567266,3.41623710198807,2.95854811567265))
REPRESENTATION_ITEM('')
);
#1355=(
BOUNDED_CURVE()
B_SPLINE_CURVE(2,(#235047,#235048,#235049),.UNSPECIFIED.,.F.,.F.)
B_SPLINE_CURVE_WITH_KNOTS((3,3),(-0.38831280429231,-0.130611113351455),
 .UNSPECIFIED.)
CURVE()
GEOMETRIC_REPRESENTATION_ITEM()
RATIONAL_B_SPLINE_CURVE((1.30940107675854,1.51196612828746,1.30940107675852))
REPRESENTATION_ITEM('')
);
#1356=(
BOUNDED_CURVE()
B_SPLINE_CURVE(2,(#235054,#235055,#235056),.UNSPECIFIED.,.F.,.F.)
B_SPLINE_CURVE_WITH_KNOTS((3,3),(0.594066455576365,1.16209721084486),
 .UNSPECIFIED.)
CURVE()
GEOMETRIC_REPRESENTATION_ITEM()
RATIONAL_B_SPLINE_CURVE((2.95854811567265,3.41623710198797,2.95854811567285))
REPRESENTATION_ITEM('')
);
#1357=(
BOUNDED_CURVE()
B_SPLINE_CURVE(2,(#235057,#235058,#235059),.UNSPECIFIED.,.F.,.F.)
B_SPLINE_CURVE_WITH_KNOTS((3,3),(-0.388312804292318,-0.13061111335146),
 .UNSPECIFIED.)
CURVE()
GEOMETRIC_REPRESENTATION_ITEM()
RATIONAL_B_SPLINE_CURVE((1.30940107675852,1.51196612828743,1.30940107675851))
REPRESENTATION_ITEM('')
);
#1358=(
BOUNDED_CURVE()
B_SPLINE_CURVE(2,(#235064,#235065,#235066),.UNSPECIFIED.,.F.,.F.)
B_SPLINE_CURVE_WITH_KNOTS((3,3),(0.594066455576169,1.16209721084492),
 .UNSPECIFIED.)
CURVE()
GEOMETRIC_REPRESENTATION_ITEM()
RATIONAL_B_SPLINE_CURVE((2.95854811567235,3.41623710198821,2.95854811567279))
REPRESENTATION_ITEM('')
);
#1359=(
BOUNDED_CURVE()
B_SPLINE_CURVE(2,(#235067,#235068,#235069),.UNSPECIFIED.,.F.,.F.)
B_SPLINE_CURVE_WITH_KNOTS((3,3),(-0.388312804292328,-0.130611113351469),
 .UNSPECIFIED.)
CURVE()
GEOMETRIC_REPRESENTATION_ITEM()
RATIONAL_B_SPLINE_CURVE((1.3094010767585,1.51196612828743,1.30940107675853))
REPRESENTATION_ITEM('')
);
#1360=(
BOUNDED_CURVE()
B_SPLINE_CURVE(2,(#235071,#235072,#235073),.UNSPECIFIED.,.F.,.F.)
B_SPLINE_CURVE_WITH_KNOTS((3,3),(0.594066455576378,1.16209721084502),
 .UNSPECIFIED.)
CURVE()
GEOMETRIC_REPRESENTATION_ITEM()
RATIONAL_B_SPLINE_CURVE((2.95854811567253,3.41623710198792,2.95854811567244))
REPRESENTATION_ITEM('')
);
#1361=(
BOUNDED_CURVE()
B_SPLINE_CURVE(2,(#235074,#235075,#235076),.UNSPECIFIED.,.F.,.F.)
B_SPLINE_CURVE_WITH_KNOTS((3,3),(-0.388312804292317,-0.13061111335146),
 .UNSPECIFIED.)
CURVE()
GEOMETRIC_REPRESENTATION_ITEM()
RATIONAL_B_SPLINE_CURVE((1.3094010767585,1.51196612828743,1.30940107675851))
REPRESENTATION_ITEM('')
);
#1362=(
BOUNDED_CURVE()
B_SPLINE_CURVE(3,(#235504,#235505,#235506,#235507,#235508,#235509,#235510,
#235511,#235512,#235513),.UNSPECIFIED.,.F.,.F.)
B_SPLINE_CURVE_WITH_KNOTS((4,2,2,2,4),(4.71238898038469,5.10508806208341,
5.49778714378214,5.89048622548086,6.28318530717959),.UNSPECIFIED.)
CURVE()
GEOMETRIC_REPRESENTATION_ITEM()
RATIONAL_B_SPLINE_CURVE((1.,1.,1.,1.,1.,1.,1.,1.,1.,1.))
REPRESENTATION_ITEM('')
);
#1363=(
BOUNDED_CURVE()
B_SPLINE_CURVE(3,(#235591,#235592,#235593,#235594,#235595,#235596,#235597,
#235598,#235599,#235600),.UNSPECIFIED.,.F.,.F.)
B_SPLINE_CURVE_WITH_KNOTS((4,2,2,2,4),(4.71238898038469,5.10508806208341,
5.49778714378214,5.89048622548086,6.28318530717959),.UNSPECIFIED.)
CURVE()
GEOMETRIC_REPRESENTATION_ITEM()
RATIONAL_B_SPLINE_CURVE((1.,1.,1.,1.,1.,1.,1.,1.,1.,1.))
REPRESENTATION_ITEM('')
);
#1364=(
BOUNDED_CURVE()
B_SPLINE_CURVE(2,(#238415,#238416,#238417),.UNSPECIFIED.,.F.,.F.)
B_SPLINE_CURVE_WITH_KNOTS((3,3),(0.809350832147077,0.812919471044032),
 .UNSPECIFIED.)
CURVE()
GEOMETRIC_REPRESENTATION_ITEM()
RATIONAL_B_SPLINE_CURVE((1.,0.934429088195473,0.933042650109519))
REPRESENTATION_ITEM('')
);
#1365=(
BOUNDED_CURVE()
B_SPLINE_CURVE(2,(#238425,#238426,#238427),.UNSPECIFIED.,.F.,.F.)
B_SPLINE_CURVE_WITH_KNOTS((3,3),(0.804347826086956,0.80995470719394),
 .UNSPECIFIED.)
CURVE()
GEOMETRIC_REPRESENTATION_ITEM()
RATIONAL_B_SPLINE_CURVE((1.,0.89633721073752,0.953092503428239))
REPRESENTATION_ITEM('')
);
#1366=(
BOUNDED_CURVE()
B_SPLINE_CURVE(2,(#238433,#238434,#238435,#238436,#238437,#238438,#238439),
 .UNSPECIFIED.,.F.,.F.)
B_SPLINE_CURVE_WITH_KNOTS((3,2,2,3),(0.76560213851751,0.772893587455772,
0.780185036394034,0.78020664750063),.UNSPECIFIED.)
CURVE()
GEOMETRIC_REPRESENTATION_ITEM()
RATIONAL_B_SPLINE_CURVE((1.,0.866025403784439,1.,0.866025403784439,1.,0.99960291304177,
0.999208179933552))
REPRESENTATION_ITEM('')
);
#1367=(
BOUNDED_CURVE()
B_SPLINE_CURVE(2,(#238453,#238454,#238455,#238456,#238457,#238458,#238459),
 .UNSPECIFIED.,.F.,.F.)
B_SPLINE_CURVE_WITH_KNOTS((3,2,2,3),(0.787646415600072,0.794767934270535,
0.802059383208806,0.809350832147077),.UNSPECIFIED.)
CURVE()
GEOMETRIC_REPRESENTATION_ITEM()
RATIONAL_B_SPLINE_CURVE((0.993900866577314,0.86914773779612,1.,0.866025403784439,
1.,0.866025403784439,1.))
REPRESENTATION_ITEM('')
);
#1368=(
BOUNDED_CURVE()
B_SPLINE_CURVE(2,(#238460,#238461,#238462,#238463,#238464,#238465,#238466,
#238467,#238468,#238469,#238470,#238471,#238472),.UNSPECIFIED.,.F.,.F.)
B_SPLINE_CURVE_WITH_KNOTS((3,2,2,2,2,2,3),(0.760869565217391,0.768115942028986,
0.77536231884058,0.782608695652174,0.789855072463768,0.797101449275362,
0.804347826086956),.UNSPECIFIED.)
CURVE()
GEOMETRIC_REPRESENTATION_ITEM()
RATIONAL_B_SPLINE_CURVE((1.,0.866025403784439,1.,0.866025403784439,1.,0.866025403784439,
1.,0.866025403784439,1.,0.866025403784439,1.,0.866025403784439,1.))
REPRESENTATION_ITEM('')
);
#1369=(
BOUNDED_CURVE()
B_SPLINE_CURVE(2,(#238477,#238478,#238479,#238480,#238481,#238482,#238483,
#238484,#238485,#238486,#238487,#238488,#238489),.UNSPECIFIED.,.F.,.F.)
B_SPLINE_CURVE_WITH_KNOTS((3,2,2,2,2,2,3),(0.721853444887938,0.7291448938262,
0.736436342764462,0.743727791702724,0.751019240640986,0.758310689579248,
0.76560213851751),.UNSPECIFIED.)
CURVE()
GEOMETRIC_REPRESENTATION_ITEM()
RATIONAL_B_SPLINE_CURVE((1.,0.866025403784439,1.,0.866025403784439,1.,0.866025403784439,
1.,0.866025403784439,1.,0.866025403784439,1.,0.866025403784439,1.))
REPRESENTATION_ITEM('')
);
#1370=(
BOUNDED_CURVE()
B_SPLINE_CURVE(2,(#238490,#238491,#238492,#238493,#238494,#238495,#238496,
#238497,#238498,#238499,#238500,#238501,#238502),.UNSPECIFIED.,.F.,.F.)
B_SPLINE_CURVE_WITH_KNOTS((3,2,2,2,2,2,3),(0.717391304347826,0.72463768115942,
0.731884057971015,0.739130434782609,0.746376811594203,0.753623188405797,
0.760869565217391),.UNSPECIFIED.)
CURVE()
GEOMETRIC_REPRESENTATION_ITEM()
RATIONAL_B_SPLINE_CURVE((1.,0.866025403784439,1.,0.866025403784439,1.,0.866025403784439,
1.,0.866025403784439,1.,0.866025403784439,1.,0.866025403784439,1.))
REPRESENTATION_ITEM('')
);
#1371=(
BOUNDED_CURVE()
B_SPLINE_CURVE(2,(#238507,#238508,#238509,#238510,#238511,#238512,#238513,
#238514,#238515,#238516,#238517,#238518,#238519),.UNSPECIFIED.,.F.,.F.)
B_SPLINE_CURVE_WITH_KNOTS((3,2,2,2,2,2,3),(0.678104751258366,0.685396200196628,
0.69268764913489,0.699979098073152,0.707270547011414,0.714561995949676,
0.721853444887938),.UNSPECIFIED.)
CURVE()
GEOMETRIC_REPRESENTATION_ITEM()
RATIONAL_B_SPLINE_CURVE((1.,0.866025403784439,1.,0.866025403784439,1.,0.866025403784439,
1.,0.866025403784439,1.,0.866025403784439,1.,0.866025403784439,1.))
REPRESENTATION_ITEM('')
);
#1372=(
BOUNDED_CURVE()
B_SPLINE_CURVE(2,(#238520,#238521,#238522,#238523,#238524,#238525,#238526,
#238527,#238528,#238529,#238530,#238531,#238532),.UNSPECIFIED.,.F.,.F.)
B_SPLINE_CURVE_WITH_KNOTS((3,2,2,2,2,2,3),(0.673913043478261,0.681159420289855,
0.688405797101449,0.695652173913044,0.702898550724638,0.710144927536232,
0.717391304347826),.UNSPECIFIED.)
CURVE()
GEOMETRIC_REPRESENTATION_ITEM()
RATIONAL_B_SPLINE_CURVE((1.,0.866025403784439,1.,0.866025403784439,1.,0.866025403784439,
1.,0.866025403784439,1.,0.866025403784439,1.,0.866025403784439,1.))
REPRESENTATION_ITEM('')
);
#1373=(
BOUNDED_CURVE()
B_SPLINE_CURVE(2,(#238537,#238538,#238539,#238540,#238541,#238542,#238543,
#238544,#238545,#238546,#238547,#238548,#238549),.UNSPECIFIED.,.F.,.F.)
B_SPLINE_CURVE_WITH_KNOTS((3,2,2,2,2,2,3),(0.634356057628794,0.641647506567056,
0.648938955505318,0.65623040444358,0.663521853381842,0.670813302320104,
0.678104751258366),.UNSPECIFIED.)
CURVE()
GEOMETRIC_REPRESENTATION_ITEM()
RATIONAL_B_SPLINE_CURVE((1.,0.866025403784439,1.,0.866025403784439,1.,0.866025403784439,
1.,0.866025403784439,1.,0.866025403784439,1.,0.866025403784439,1.))
REPRESENTATION_ITEM('')
);
#1374=(
BOUNDED_CURVE()
B_SPLINE_CURVE(2,(#238550,#238551,#238552,#238553,#238554,#238555,#238556,
#238557,#238558,#238559,#238560,#238561,#238562),.UNSPECIFIED.,.F.,.F.)
B_SPLINE_CURVE_WITH_KNOTS((3,2,2,2,2,2,3),(0.630434782608696,0.63768115942029,
0.644927536231884,0.652173913043478,0.659420289855073,0.666666666666667,
0.673913043478261),.UNSPECIFIED.)
CURVE()
GEOMETRIC_REPRESENTATION_ITEM()
RATIONAL_B_SPLINE_CURVE((1.,0.866025403784439,1.,0.866025403784439,1.,0.866025403784439,
1.,0.866025403784439,1.,0.866025403784439,1.,0.866025403784439,1.))
REPRESENTATION_ITEM('')
);
#1375=(
BOUNDED_CURVE()
B_SPLINE_CURVE(2,(#238567,#238568,#238569,#238570,#238571,#238572,#238573,
#238574,#238575,#238576,#238577,#238578,#238579),.UNSPECIFIED.,.F.,.F.)
B_SPLINE_CURVE_WITH_KNOTS((3,2,2,2,2,2,3),(0.590607363999222,0.597898812937484,
0.605190261875746,0.612481710814008,0.61977315975227,0.627064608690532,
0.634356057628794),.UNSPECIFIED.)
CURVE()
GEOMETRIC_REPRESENTATION_ITEM()
RATIONAL_B_SPLINE_CURVE((1.,0.866025403784439,1.,0.866025403784439,1.,0.866025403784439,
1.,0.866025403784439,1.,0.866025403784439,1.,0.866025403784439,1.))
REPRESENTATION_ITEM('')
);
#1376=(
BOUNDED_CURVE()
B_SPLINE_CURVE(2,(#238580,#238581,#238582,#238583,#238584,#238585,#238586,
#238587,#238588,#238589,#238590,#238591,#238592),.UNSPECIFIED.,.F.,.F.)
B_SPLINE_CURVE_WITH_KNOTS((3,2,2,2,2,2,3),(0.586956521739131,0.594202898550725,
0.601449275362319,0.608695652173913,0.615942028985507,0.623188405797102,
0.630434782608696),.UNSPECIFIED.)
CURVE()
GEOMETRIC_REPRESENTATION_ITEM()
RATIONAL_B_SPLINE_CURVE((1.,0.866025403784439,1.,0.866025403784439,1.,0.866025403784439,
1.,0.866025403784439,1.,0.866025403784439,1.,0.866025403784439,1.))
REPRESENTATION_ITEM('')
);
#1377=(
BOUNDED_CURVE()
B_SPLINE_CURVE(2,(#238597,#238598,#238599,#238600,#238601,#238602,#238603,
#238604,#238605,#238606,#238607,#238608,#238609),.UNSPECIFIED.,.F.,.F.)
B_SPLINE_CURVE_WITH_KNOTS((3,2,2,2,2,2,3),(0.54685867036965,0.554150119307912,
0.561441568246174,0.568733017184436,0.576024466122698,0.58331591506096,
0.590607363999222),.UNSPECIFIED.)
CURVE()
GEOMETRIC_REPRESENTATION_ITEM()
RATIONAL_B_SPLINE_CURVE((1.,0.866025403784439,1.,0.866025403784439,1.,0.866025403784439,
1.,0.866025403784439,1.,0.866025403784439,1.,0.866025403784439,1.))
REPRESENTATION_ITEM('')
);
#1378=(
BOUNDED_CURVE()
B_SPLINE_CURVE(2,(#238610,#238611,#238612,#238613,#238614,#238615,#238616,
#238617,#238618,#238619,#238620,#238621,#238622),.UNSPECIFIED.,.F.,.F.)
B_SPLINE_CURVE_WITH_KNOTS((3,2,2,2,2,2,3),(0.543478260869565,0.550724637681159,
0.557971014492754,0.565217391304348,0.572463768115942,0.579710144927536,
0.586956521739131),.UNSPECIFIED.)
CURVE()
GEOMETRIC_REPRESENTATION_ITEM()
RATIONAL_B_SPLINE_CURVE((1.,0.866025403784439,1.,0.866025403784439,1.,0.866025403784439,
1.,0.866025403784439,1.,0.866025403784439,1.,0.866025403784439,1.))
REPRESENTATION_ITEM('')
);
#1379=(
BOUNDED_CURVE()
B_SPLINE_CURVE(2,(#238627,#238628,#238629,#238630,#238631,#238632,#238633,
#238634,#238635,#238636,#238637,#238638,#238639),.UNSPECIFIED.,.F.,.F.)
B_SPLINE_CURVE_WITH_KNOTS((3,2,2,2,2,2,3),(0.503109976740078,0.51040142567834,
0.517692874616602,0.524984323554864,0.532275772493126,0.539567221431388,
0.54685867036965),.UNSPECIFIED.)
CURVE()
GEOMETRIC_REPRESENTATION_ITEM()
RATIONAL_B_SPLINE_CURVE((1.,0.866025403784439,1.,0.866025403784439,1.,0.866025403784439,
1.,0.866025403784439,1.,0.866025403784439,1.,0.866025403784439,1.))
REPRESENTATION_ITEM('')
);
#1380=(
BOUNDED_CURVE()
B_SPLINE_CURVE(2,(#238640,#238641,#238642,#238643,#238644,#238645,#238646,
#238647,#238648,#238649,#238650,#238651,#238652),.UNSPECIFIED.,.F.,.F.)
B_SPLINE_CURVE_WITH_KNOTS((3,2,2,2,2,2,3),(0.5,0.507246376811594,0.514492753623189,
0.521739130434783,0.528985507246377,0.536231884057971,0.543478260869565),
 .UNSPECIFIED.)
CURVE()
GEOMETRIC_REPRESENTATION_ITEM()
RATIONAL_B_SPLINE_CURVE((1.,0.866025403784439,1.,0.866025403784439,1.,0.866025403784439,
1.,0.866025403784439,1.,0.866025403784439,1.,0.866025403784439,1.))
REPRESENTATION_ITEM('')
);
#1381=(
BOUNDED_CURVE()
B_SPLINE_CURVE(2,(#238657,#238658,#238659,#238660,#238661,#238662,#238663,
#238664,#238665,#238666,#238667,#238668,#238669),.UNSPECIFIED.,.F.,.F.)
B_SPLINE_CURVE_WITH_KNOTS((3,2,2,2,2,2,3),(0.459361283110506,0.466652732048768,
0.47394418098703,0.481235629925292,0.488527078863554,0.495818527801816,
0.503109976740078),.UNSPECIFIED.)
CURVE()
GEOMETRIC_REPRESENTATION_ITEM()
RATIONAL_B_SPLINE_CURVE((1.,0.866025403784439,1.,0.866025403784439,1.,0.866025403784439,
1.,0.866025403784439,1.,0.866025403784439,1.,0.866025403784439,1.))
REPRESENTATION_ITEM('')
);
#1382=(
BOUNDED_CURVE()
B_SPLINE_CURVE(2,(#238670,#238671,#238672,#238673,#238674,#238675,#238676,
#238677,#238678,#238679,#238680,#238681,#238682),.UNSPECIFIED.,.F.,.F.)
B_SPLINE_CURVE_WITH_KNOTS((3,2,2,2,2,2,3),(0.456521739130435,0.463768115942029,
0.471014492753623,0.478260869565218,0.485507246376812,0.492753623188406,
0.5),.UNSPECIFIED.)
CURVE()
GEOMETRIC_REPRESENTATION_ITEM()
RATIONAL_B_SPLINE_CURVE((1.,0.866025403784439,1.,0.866025403784439,1.,0.866025403784439,
1.,0.866025403784439,1.,0.866025403784439,1.,0.866025403784439,1.))
REPRESENTATION_ITEM('')
);
#1383=(
BOUNDED_CURVE()
B_SPLINE_CURVE(2,(#238687,#238688,#238689,#238690,#238691,#238692,#238693,
#238694,#238695,#238696,#238697,#238698,#238699),.UNSPECIFIED.,.F.,.F.)
B_SPLINE_CURVE_WITH_KNOTS((3,2,2,2,2,2,3),(0.415612589480934,0.422904038419196,
0.430195487357458,0.43748693629572,0.444778385233982,0.452069834172244,
0.459361283110506),.UNSPECIFIED.)
CURVE()
GEOMETRIC_REPRESENTATION_ITEM()
RATIONAL_B_SPLINE_CURVE((1.,0.866025403784439,1.,0.866025403784439,1.,0.866025403784439,
1.,0.866025403784439,1.,0.866025403784439,1.,0.866025403784439,1.))
REPRESENTATION_ITEM('')
);
#1384=(
BOUNDED_CURVE()
B_SPLINE_CURVE(2,(#238700,#238701,#238702,#238703,#238704,#238705,#238706,
#238707,#238708,#238709,#238710,#238711,#238712),.UNSPECIFIED.,.F.,.F.)
B_SPLINE_CURVE_WITH_KNOTS((3,2,2,2,2,2,3),(0.41304347826087,0.420289855072464,
0.427536231884058,0.434782608695652,0.442028985507247,0.449275362318841,
0.456521739130435),.UNSPECIFIED.)
CURVE()
GEOMETRIC_REPRESENTATION_ITEM()
RATIONAL_B_SPLINE_CURVE((1.,0.866025403784439,1.,0.866025403784439,1.,0.866025403784439,
1.,0.866025403784439,1.,0.866025403784439,1.,0.866025403784439,1.))
REPRESENTATION_ITEM('')
);
#1385=(
BOUNDED_CURVE()
B_SPLINE_CURVE(2,(#238717,#238718,#238719,#238720,#238721,#238722,#238723,
#238724,#238725,#238726,#238727,#238728,#238729),.UNSPECIFIED.,.F.,.F.)
B_SPLINE_CURVE_WITH_KNOTS((3,2,2,2,2,2,3),(0.371863895851362,0.379155344789624,
0.386446793727886,0.393738242666148,0.40102969160441,0.408321140542672,
0.415612589480934),.UNSPECIFIED.)
CURVE()
GEOMETRIC_REPRESENTATION_ITEM()
RATIONAL_B_SPLINE_CURVE((1.,0.866025403784439,1.,0.866025403784439,1.,0.866025403784439,
1.,0.866025403784439,1.,0.866025403784439,1.,0.866025403784439,1.))
REPRESENTATION_ITEM('')
);
#1386=(
BOUNDED_CURVE()
B_SPLINE_CURVE(2,(#238730,#238731,#238732,#238733,#238734,#238735,#238736,
#238737,#238738,#238739,#238740,#238741,#238742),.UNSPECIFIED.,.F.,.F.)
B_SPLINE_CURVE_WITH_KNOTS((3,2,2,2,2,2,3),(0.369565217391304,0.376811594202899,
0.384057971014493,0.391304347826087,0.398550724637681,0.405797101449275,
0.41304347826087),.UNSPECIFIED.)
CURVE()
GEOMETRIC_REPRESENTATION_ITEM()
RATIONAL_B_SPLINE_CURVE((1.,0.866025403784439,1.,0.866025403784439,1.,0.866025403784439,
1.,0.866025403784439,1.,0.866025403784439,1.,0.866025403784439,1.))
REPRESENTATION_ITEM('')
);
#1387=(
BOUNDED_CURVE()
B_SPLINE_CURVE(2,(#238747,#238748,#238749,#238750,#238751,#238752,#238753,
#238754,#238755,#238756,#238757,#238758,#238759),.UNSPECIFIED.,.F.,.F.)
B_SPLINE_CURVE_WITH_KNOTS((3,2,2,2,2,2,3),(0.32811520222179,0.335406651160052,
0.342698100098314,0.349989549036576,0.357280997974838,0.3645724469131,0.371863895851362),
 .UNSPECIFIED.)
CURVE()
GEOMETRIC_REPRESENTATION_ITEM()
RATIONAL_B_SPLINE_CURVE((1.,0.866025403784439,1.,0.866025403784439,1.,0.866025403784439,
1.,0.866025403784439,1.,0.866025403784439,1.,0.866025403784439,1.))
REPRESENTATION_ITEM('')
);
#1388=(
BOUNDED_CURVE()
B_SPLINE_CURVE(2,(#238760,#238761,#238762,#238763,#238764,#238765,#238766,
#238767,#238768,#238769,#238770,#238771,#238772),.UNSPECIFIED.,.F.,.F.)
B_SPLINE_CURVE_WITH_KNOTS((3,2,2,2,2,2,3),(0.326086956521739,0.333333333333334,
0.340579710144927,0.347826086956522,0.355072463768116,0.36231884057971,
0.369565217391304),.UNSPECIFIED.)
CURVE()
GEOMETRIC_REPRESENTATION_ITEM()
RATIONAL_B_SPLINE_CURVE((1.,0.866025403784439,1.,0.866025403784439,1.,0.866025403784439,
1.,0.866025403784439,1.,0.866025403784439,1.,0.866025403784439,1.))
REPRESENTATION_ITEM('')
);
#1389=(
BOUNDED_CURVE()
B_SPLINE_CURVE(2,(#238777,#238778,#238779,#238780,#238781,#238782,#238783,
#238784,#238785,#238786,#238787,#238788,#238789),.UNSPECIFIED.,.F.,.F.)
B_SPLINE_CURVE_WITH_KNOTS((3,2,2,2,2,2,3),(0.284366508592218,0.29165795753048,
0.298949406468742,0.306240855407004,0.313532304345266,0.320823753283528,
0.32811520222179),.UNSPECIFIED.)
CURVE()
GEOMETRIC_REPRESENTATION_ITEM()
RATIONAL_B_SPLINE_CURVE((1.,0.866025403784439,1.,0.866025403784439,1.,0.866025403784439,
1.,0.866025403784439,1.,0.866025403784439,1.,0.866025403784439,1.))
REPRESENTATION_ITEM('')
);
#1390=(
BOUNDED_CURVE()
B_SPLINE_CURVE(2,(#238790,#238791,#238792,#238793,#238794,#238795,#238796,
#238797,#238798,#238799,#238800,#238801,#238802),.UNSPECIFIED.,.F.,.F.)
B_SPLINE_CURVE_WITH_KNOTS((3,2,2,2,2,2,3),(0.282608695652174,0.289855072463769,
0.297101449275363,0.304347826086956,0.311594202898551,0.318840579710145,
0.326086956521739),.UNSPECIFIED.)
CURVE()
GEOMETRIC_REPRESENTATION_ITEM()
RATIONAL_B_SPLINE_CURVE((1.,0.866025403784439,1.,0.866025403784439,1.,0.866025403784439,
1.,0.866025403784439,1.,0.866025403784439,1.,0.866025403784439,1.))
REPRESENTATION_ITEM('')
);
#1391=(
BOUNDED_CURVE()
B_SPLINE_CURVE(2,(#238807,#238808,#238809,#238810,#238811,#238812,#238813,
#238814,#238815,#238816,#238817,#238818,#238819),.UNSPECIFIED.,.F.,.F.)
B_SPLINE_CURVE_WITH_KNOTS((3,2,2,2,2,2,3),(0.240617814962646,0.247909263900908,
0.25520071283917,0.262492161777432,0.269783610715694,0.277075059653956,
0.284366508592218),.UNSPECIFIED.)
CURVE()
GEOMETRIC_REPRESENTATION_ITEM()
RATIONAL_B_SPLINE_CURVE((1.,0.866025403784439,1.,0.866025403784439,1.,0.866025403784439,
1.,0.866025403784439,1.,0.866025403784439,1.,0.866025403784439,1.))
REPRESENTATION_ITEM('')
);
#1392=(
BOUNDED_CURVE()
B_SPLINE_CURVE(2,(#238820,#238821,#238822,#238823,#238824,#238825,#238826,
#238827,#238828,#238829,#238830,#238831,#238832),.UNSPECIFIED.,.F.,.F.)
B_SPLINE_CURVE_WITH_KNOTS((3,2,2,2,2,2,3),(0.239130434782609,0.246376811594203,
0.253623188405797,0.260869565217392,0.268115942028985,0.27536231884058,
0.282608695652174),.UNSPECIFIED.)
CURVE()
GEOMETRIC_REPRESENTATION_ITEM()
RATIONAL_B_SPLINE_CURVE((1.,0.866025403784439,1.,0.866025403784439,1.,0.866025403784439,
1.,0.866025403784439,1.,0.866025403784439,1.,0.866025403784439,1.))
REPRESENTATION_ITEM('')
);
#1393=(
BOUNDED_CURVE()
B_SPLINE_CURVE(2,(#238837,#238838,#238839,#238840,#238841,#238842,#238843,
#238844,#238845,#238846,#238847,#238848,#238849),.UNSPECIFIED.,.F.,.F.)
B_SPLINE_CURVE_WITH_KNOTS((3,2,2,2,2,2,3),(0.196869121333074,0.204160570271336,
0.211452019209598,0.21874346814786,0.226034917086122,0.233326366024384,
0.240617814962646),.UNSPECIFIED.)
CURVE()
GEOMETRIC_REPRESENTATION_ITEM()
RATIONAL_B_SPLINE_CURVE((1.,0.866025403784439,1.,0.866025403784439,1.,0.866025403784439,
1.,0.866025403784439,1.,0.866025403784439,1.,0.866025403784439,1.))
REPRESENTATION_ITEM('')
);
#1394=(
BOUNDED_CURVE()
B_SPLINE_CURVE(2,(#238850,#238851,#238852,#238853,#238854,#238855,#238856,
#238857,#238858,#238859,#238860,#238861,#238862),.UNSPECIFIED.,.F.,.F.)
B_SPLINE_CURVE_WITH_KNOTS((3,2,2,2,2,2,3),(0.195652173913044,0.202898550724638,
0.210144927536232,0.217391304347826,0.224637681159421,0.231884057971014,
0.239130434782609),.UNSPECIFIED.)
CURVE()
GEOMETRIC_REPRESENTATION_ITEM()
RATIONAL_B_SPLINE_CURVE((1.,0.866025403784439,1.,0.866025403784439,1.,0.866025403784439,
1.,0.866025403784439,1.,0.866025403784439,1.,0.866025403784439,1.))
REPRESENTATION_ITEM('')
);
#1395=(
BOUNDED_CURVE()
B_SPLINE_CURVE(2,(#238867,#238868,#238869,#238870,#238871,#238872,#238873,
#238874,#238875,#238876,#238877,#238878,#238879),.UNSPECIFIED.,.F.,.F.)
B_SPLINE_CURVE_WITH_KNOTS((3,2,2,2,2,2,3),(0.153120427703502,0.160411876641764,
0.167703325580026,0.174994774518288,0.18228622345655,0.189577672394812,
0.196869121333074),.UNSPECIFIED.)
CURVE()
GEOMETRIC_REPRESENTATION_ITEM()
RATIONAL_B_SPLINE_CURVE((1.,0.866025403784439,1.,0.866025403784439,1.,0.866025403784439,
1.,0.866025403784439,1.,0.866025403784439,1.,0.866025403784439,1.))
REPRESENTATION_ITEM('')
);
#1396=(
BOUNDED_CURVE()
B_SPLINE_CURVE(2,(#238880,#238881,#238882,#238883,#238884,#238885,#238886,
#238887,#238888,#238889,#238890,#238891,#238892),.UNSPECIFIED.,.F.,.F.)
B_SPLINE_CURVE_WITH_KNOTS((3,2,2,2,2,2,3),(0.152173913043478,0.159420289855073,
0.166666666666667,0.173913043478261,0.181159420289855,0.18840579710145,
0.195652173913044),.UNSPECIFIED.)
CURVE()
GEOMETRIC_REPRESENTATION_ITEM()
RATIONAL_B_SPLINE_CURVE((1.,0.866025403784439,1.,0.866025403784439,1.,0.866025403784439,
1.,0.866025403784439,1.,0.866025403784439,1.,0.866025403784439,1.))
REPRESENTATION_ITEM('')
);
#1397=(
BOUNDED_CURVE()
B_SPLINE_CURVE(2,(#238897,#238898,#238899,#238900,#238901,#238902,#238903,
#238904,#238905,#238906,#238907,#238908,#238909),.UNSPECIFIED.,.F.,.F.)
B_SPLINE_CURVE_WITH_KNOTS((3,2,2,2,2,2,3),(0.10937173407393,0.116663183012192,
0.123954631950454,0.131246080888716,0.138537529826978,0.14582897876524,
0.153120427703502),.UNSPECIFIED.)
CURVE()
GEOMETRIC_REPRESENTATION_ITEM()
RATIONAL_B_SPLINE_CURVE((1.,0.866025403784439,1.,0.866025403784439,1.,0.866025403784439,
1.,0.866025403784439,1.,0.866025403784439,1.,0.866025403784439,1.))
REPRESENTATION_ITEM('')
);
#1398=(
BOUNDED_CURVE()
B_SPLINE_CURVE(2,(#238910,#238911,#238912,#238913,#238914,#238915,#238916,
#238917,#238918,#238919,#238920,#238921,#238922),.UNSPECIFIED.,.F.,.F.)
B_SPLINE_CURVE_WITH_KNOTS((3,2,2,2,2,2,3),(0.108695652173913,0.115942028985507,
0.123188405797102,0.130434782608696,0.13768115942029,0.144927536231884,
0.152173913043478),.UNSPECIFIED.)
CURVE()
GEOMETRIC_REPRESENTATION_ITEM()
RATIONAL_B_SPLINE_CURVE((1.,0.866025403784439,1.,0.866025403784439,1.,0.866025403784439,
1.,0.866025403784439,1.,0.866025403784439,1.,0.866025403784439,1.))
REPRESENTATION_ITEM('')
);
#1399=(
BOUNDED_CURVE()
B_SPLINE_CURVE(2,(#238927,#238928,#238929,#238930,#238931,#238932,#238933,
#238934,#238935,#238936,#238937,#238938,#238939),.UNSPECIFIED.,.F.,.F.)
B_SPLINE_CURVE_WITH_KNOTS((3,2,2,2,2,2,3),(0.065623040444358,0.07291448938262,
0.080205938320882,0.087497387259144,0.094788836197406,0.102080285135668,
0.10937173407393),.UNSPECIFIED.)
CURVE()
GEOMETRIC_REPRESENTATION_ITEM()
RATIONAL_B_SPLINE_CURVE((1.,0.866025403784439,1.,0.866025403784439,1.,0.866025403784439,
1.,0.866025403784439,1.,0.866025403784439,1.,0.866025403784439,1.))
REPRESENTATION_ITEM('')
);
#1400=(
BOUNDED_CURVE()
B_SPLINE_CURVE(2,(#238940,#238941,#238942,#238943,#238944,#238945,#238946,
#238947,#238948,#238949,#238950,#238951,#238952),.UNSPECIFIED.,.F.,.F.)
B_SPLINE_CURVE_WITH_KNOTS((3,2,2,2,2,2,3),(0.065217391304348,0.0724637681159422,
0.0797101449275364,0.0869565217391306,0.0942028985507248,0.101449275362319,
0.108695652173913),.UNSPECIFIED.)
CURVE()
GEOMETRIC_REPRESENTATION_ITEM()
RATIONAL_B_SPLINE_CURVE((1.,0.866025403784439,1.,0.866025403784439,1.,0.866025403784439,
1.,0.866025403784439,1.,0.866025403784439,1.,0.866025403784439,1.))
REPRESENTATION_ITEM('')
);
#1401=(
BOUNDED_CURVE()
B_SPLINE_CURVE(2,(#238959,#238960,#238961,#238962,#238963),
 .UNSPECIFIED.,.F.,.F.)
B_SPLINE_CURVE_WITH_KNOTS((3,2,3),(0.0118893770663295,0.014582897876524,
0.021874346814786),.UNSPECIFIED.)
CURVE()
GEOMETRIC_REPRESENTATION_ITEM()
RATIONAL_B_SPLINE_CURVE((0.937582367981151,0.950508689562319,1.,0.866025403784439,
1.))
REPRESENTATION_ITEM('')
);
#1402=(
BOUNDED_CURVE()
B_SPLINE_CURVE(2,(#240349,#240350,#240351),.UNSPECIFIED.,.F.,.F.)
B_SPLINE_CURVE_WITH_KNOTS((3,3),(0.809350832147077,0.812919456587346),
 .UNSPECIFIED.)
CURVE()
GEOMETRIC_REPRESENTATION_ITEM()
RATIONAL_B_SPLINE_CURVE((1.,0.934429353825615,0.933042661343594))
REPRESENTATION_ITEM('')
);
#1403=(
BOUNDED_CURVE()
B_SPLINE_CURVE(2,(#240369,#240370,#240371),.UNSPECIFIED.,.F.,.F.)
B_SPLINE_CURVE_WITH_KNOTS((3,3),(0.804347826086956,0.809954707839571),
 .UNSPECIFIED.)
CURVE()
GEOMETRIC_REPRESENTATION_ITEM()
RATIONAL_B_SPLINE_CURVE((1.,0.896337198800779,0.953092516498953))
REPRESENTATION_ITEM('')
);
#1404=(
BOUNDED_CURVE()
B_SPLINE_CURVE(2,(#240377,#240378,#240379,#240380,#240381,#240382,#240383),
 .UNSPECIFIED.,.F.,.F.)
B_SPLINE_CURVE_WITH_KNOTS((3,2,2,3),(0.76560213851751,0.772893587455772,
0.780185036394034,0.780206648355897),.UNSPECIFIED.)
CURVE()
GEOMETRIC_REPRESENTATION_ITEM()
RATIONAL_B_SPLINE_CURVE((1.,0.866025403784439,1.,0.866025403784439,1.,0.99960289732691,
0.999208148690144))
REPRESENTATION_ITEM('')
);
#1405=(
BOUNDED_CURVE()
B_SPLINE_CURVE(2,(#240397,#240398,#240399,#240400,#240401,#240402,#240403),
 .UNSPECIFIED.,.F.,.F.)
B_SPLINE_CURVE_WITH_KNOTS((3,2,2,3),(0.787646397966073,0.794767934270535,
0.802059383208806,0.809350832147077),.UNSPECIFIED.)
CURVE()
GEOMETRIC_REPRESENTATION_ITEM()
RATIONAL_B_SPLINE_CURVE((0.99390148439558,0.869147413785358,1.,0.866025403784439,
1.,0.866025403784439,1.))
REPRESENTATION_ITEM('')
);
#1406=(
BOUNDED_CURVE()
B_SPLINE_CURVE(2,(#240404,#240405,#240406,#240407,#240408,#240409,#240410,
#240411,#240412,#240413,#240414,#240415,#240416),.UNSPECIFIED.,.F.,.F.)
B_SPLINE_CURVE_WITH_KNOTS((3,2,2,2,2,2,3),(0.760869565217391,0.768115942028986,
0.77536231884058,0.782608695652174,0.789855072463768,0.797101449275362,
0.804347826086956),.UNSPECIFIED.)
CURVE()
GEOMETRIC_REPRESENTATION_ITEM()
RATIONAL_B_SPLINE_CURVE((1.,0.866025403784439,1.,0.866025403784439,1.,0.866025403784439,
1.,0.866025403784439,1.,0.866025403784439,1.,0.866025403784439,1.))
REPRESENTATION_ITEM('')
);
#1407=(
BOUNDED_CURVE()
B_SPLINE_CURVE(2,(#240421,#240422,#240423,#240424,#240425,#240426,#240427,
#240428,#240429,#240430,#240431,#240432,#240433),.UNSPECIFIED.,.F.,.F.)
B_SPLINE_CURVE_WITH_KNOTS((3,2,2,2,2,2,3),(0.721853444887938,0.7291448938262,
0.736436342764462,0.743727791702724,0.751019240640986,0.758310689579248,
0.76560213851751),.UNSPECIFIED.)
CURVE()
GEOMETRIC_REPRESENTATION_ITEM()
RATIONAL_B_SPLINE_CURVE((1.,0.866025403784439,1.,0.866025403784439,1.,0.866025403784439,
1.,0.866025403784439,1.,0.866025403784439,1.,0.866025403784439,1.))
REPRESENTATION_ITEM('')
);
#1408=(
BOUNDED_CURVE()
B_SPLINE_CURVE(2,(#240434,#240435,#240436,#240437,#240438,#240439,#240440,
#240441,#240442,#240443,#240444,#240445,#240446),.UNSPECIFIED.,.F.,.F.)
B_SPLINE_CURVE_WITH_KNOTS((3,2,2,2,2,2,3),(0.717391304347826,0.724637681159421,
0.731884057971015,0.739130434782609,0.746376811594203,0.753623188405797,
0.760869565217391),.UNSPECIFIED.)
CURVE()
GEOMETRIC_REPRESENTATION_ITEM()
RATIONAL_B_SPLINE_CURVE((1.,0.866025403784439,1.,0.866025403784439,1.,0.866025403784439,
1.,0.866025403784439,1.,0.866025403784439,1.,0.866025403784439,1.))
REPRESENTATION_ITEM('')
);
#1409=(
BOUNDED_CURVE()
B_SPLINE_CURVE(2,(#240451,#240452,#240453,#240454,#240455,#240456,#240457,
#240458,#240459,#240460,#240461,#240462,#240463),.UNSPECIFIED.,.F.,.F.)
B_SPLINE_CURVE_WITH_KNOTS((3,2,2,2,2,2,3),(0.678104751258366,0.685396200196628,
0.69268764913489,0.699979098073152,0.707270547011414,0.714561995949676,
0.721853444887938),.UNSPECIFIED.)
CURVE()
GEOMETRIC_REPRESENTATION_ITEM()
RATIONAL_B_SPLINE_CURVE((1.,0.866025403784439,1.,0.866025403784439,1.,0.866025403784439,
1.,0.866025403784439,1.,0.866025403784439,1.,0.866025403784439,1.))
REPRESENTATION_ITEM('')
);
#1410=(
BOUNDED_CURVE()
B_SPLINE_CURVE(2,(#240464,#240465,#240466,#240467,#240468,#240469,#240470,
#240471,#240472,#240473,#240474,#240475,#240476),.UNSPECIFIED.,.F.,.F.)
B_SPLINE_CURVE_WITH_KNOTS((3,2,2,2,2,2,3),(0.673913043478261,0.681159420289855,
0.688405797101449,0.695652173913044,0.702898550724638,0.710144927536232,
0.717391304347826),.UNSPECIFIED.)
CURVE()
GEOMETRIC_REPRESENTATION_ITEM()
RATIONAL_B_SPLINE_CURVE((1.,0.866025403784439,1.,0.866025403784439,1.,0.866025403784439,
1.,0.866025403784439,1.,0.866025403784439,1.,0.866025403784439,1.))
REPRESENTATION_ITEM('')
);
#1411=(
BOUNDED_CURVE()
B_SPLINE_CURVE(2,(#240481,#240482,#240483,#240484,#240485,#240486,#240487,
#240488,#240489,#240490,#240491,#240492,#240493),.UNSPECIFIED.,.F.,.F.)
B_SPLINE_CURVE_WITH_KNOTS((3,2,2,2,2,2,3),(0.634356057628794,0.641647506567056,
0.648938955505318,0.65623040444358,0.663521853381842,0.670813302320104,
0.678104751258366),.UNSPECIFIED.)
CURVE()
GEOMETRIC_REPRESENTATION_ITEM()
RATIONAL_B_SPLINE_CURVE((1.,0.866025403784439,1.,0.866025403784439,1.,0.866025403784439,
1.,0.866025403784439,1.,0.866025403784439,1.,0.866025403784439,1.))
REPRESENTATION_ITEM('')
);
#1412=(
BOUNDED_CURVE()
B_SPLINE_CURVE(2,(#240494,#240495,#240496,#240497,#240498,#240499,#240500,
#240501,#240502,#240503,#240504,#240505,#240506),.UNSPECIFIED.,.F.,.F.)
B_SPLINE_CURVE_WITH_KNOTS((3,2,2,2,2,2,3),(0.630434782608696,0.63768115942029,
0.644927536231884,0.652173913043478,0.659420289855073,0.666666666666667,
0.673913043478261),.UNSPECIFIED.)
CURVE()
GEOMETRIC_REPRESENTATION_ITEM()
RATIONAL_B_SPLINE_CURVE((1.,0.866025403784439,1.,0.866025403784439,1.,0.866025403784439,
1.,0.866025403784439,1.,0.866025403784439,1.,0.866025403784439,1.))
REPRESENTATION_ITEM('')
);
#1413=(
BOUNDED_CURVE()
B_SPLINE_CURVE(2,(#240511,#240512,#240513,#240514,#240515,#240516,#240517,
#240518,#240519,#240520,#240521,#240522,#240523),.UNSPECIFIED.,.F.,.F.)
B_SPLINE_CURVE_WITH_KNOTS((3,2,2,2,2,2,3),(0.590607363999222,0.597898812937484,
0.605190261875746,0.612481710814008,0.61977315975227,0.627064608690532,
0.634356057628794),.UNSPECIFIED.)
CURVE()
GEOMETRIC_REPRESENTATION_ITEM()
RATIONAL_B_SPLINE_CURVE((1.,0.866025403784439,1.,0.866025403784439,1.,0.866025403784439,
1.,0.866025403784439,1.,0.866025403784439,1.,0.866025403784439,1.))
REPRESENTATION_ITEM('')
);
#1414=(
BOUNDED_CURVE()
B_SPLINE_CURVE(2,(#240524,#240525,#240526,#240527,#240528,#240529,#240530,
#240531,#240532,#240533,#240534,#240535,#240536),.UNSPECIFIED.,.F.,.F.)
B_SPLINE_CURVE_WITH_KNOTS((3,2,2,2,2,2,3),(0.586956521739131,0.594202898550725,
0.601449275362319,0.608695652173913,0.615942028985507,0.623188405797101,
0.630434782608696),.UNSPECIFIED.)
CURVE()
GEOMETRIC_REPRESENTATION_ITEM()
RATIONAL_B_SPLINE_CURVE((1.,0.866025403784439,1.,0.866025403784439,1.,0.866025403784439,
1.,0.866025403784439,1.,0.866025403784439,1.,0.866025403784439,1.))
REPRESENTATION_ITEM('')
);
#1415=(
BOUNDED_CURVE()
B_SPLINE_CURVE(2,(#240541,#240542,#240543,#240544,#240545,#240546,#240547,
#240548,#240549,#240550,#240551,#240552,#240553),.UNSPECIFIED.,.F.,.F.)
B_SPLINE_CURVE_WITH_KNOTS((3,2,2,2,2,2,3),(0.54685867036965,0.554150119307912,
0.561441568246174,0.568733017184436,0.576024466122698,0.58331591506096,
0.590607363999222),.UNSPECIFIED.)
CURVE()
GEOMETRIC_REPRESENTATION_ITEM()
RATIONAL_B_SPLINE_CURVE((1.,0.866025403784439,1.,0.866025403784439,1.,0.866025403784439,
1.,0.866025403784439,1.,0.866025403784439,1.,0.866025403784439,1.))
REPRESENTATION_ITEM('')
);
#1416=(
BOUNDED_CURVE()
B_SPLINE_CURVE(2,(#240554,#240555,#240556,#240557,#240558,#240559,#240560,
#240561,#240562,#240563,#240564,#240565,#240566),.UNSPECIFIED.,.F.,.F.)
B_SPLINE_CURVE_WITH_KNOTS((3,2,2,2,2,2,3),(0.543478260869565,0.55072463768116,
0.557971014492754,0.565217391304348,0.572463768115942,0.579710144927536,
0.586956521739131),.UNSPECIFIED.)
CURVE()
GEOMETRIC_REPRESENTATION_ITEM()
RATIONAL_B_SPLINE_CURVE((1.,0.866025403784439,1.,0.866025403784439,1.,0.866025403784439,
1.,0.866025403784439,1.,0.866025403784439,1.,0.866025403784439,1.))
REPRESENTATION_ITEM('')
);
#1417=(
BOUNDED_CURVE()
B_SPLINE_CURVE(2,(#240571,#240572,#240573,#240574,#240575,#240576,#240577,
#240578,#240579,#240580,#240581,#240582,#240583),.UNSPECIFIED.,.F.,.F.)
B_SPLINE_CURVE_WITH_KNOTS((3,2,2,2,2,2,3),(0.503109976740078,0.51040142567834,
0.517692874616602,0.524984323554864,0.532275772493126,0.539567221431388,
0.54685867036965),.UNSPECIFIED.)
CURVE()
GEOMETRIC_REPRESENTATION_ITEM()
RATIONAL_B_SPLINE_CURVE((1.,0.866025403784439,1.,0.866025403784439,1.,0.866025403784439,
1.,0.866025403784439,1.,0.866025403784439,1.,0.866025403784439,1.))
REPRESENTATION_ITEM('')
);
#1418=(
BOUNDED_CURVE()
B_SPLINE_CURVE(2,(#240584,#240585,#240586,#240587,#240588,#240589,#240590,
#240591,#240592,#240593,#240594,#240595,#240596),.UNSPECIFIED.,.F.,.F.)
B_SPLINE_CURVE_WITH_KNOTS((3,2,2,2,2,2,3),(0.5,0.507246376811594,0.514492753623189,
0.521739130434783,0.528985507246377,0.536231884057971,0.543478260869565),
 .UNSPECIFIED.)
CURVE()
GEOMETRIC_REPRESENTATION_ITEM()
RATIONAL_B_SPLINE_CURVE((1.,0.866025403784439,1.,0.866025403784439,1.,0.866025403784439,
1.,0.866025403784439,1.,0.866025403784439,1.,0.866025403784439,1.))
REPRESENTATION_ITEM('')
);
#1419=(
BOUNDED_CURVE()
B_SPLINE_CURVE(2,(#240601,#240602,#240603,#240604,#240605,#240606,#240607,
#240608,#240609,#240610,#240611,#240612,#240613),.UNSPECIFIED.,.F.,.F.)
B_SPLINE_CURVE_WITH_KNOTS((3,2,2,2,2,2,3),(0.459361283110506,0.466652732048768,
0.47394418098703,0.481235629925292,0.488527078863554,0.495818527801816,
0.503109976740078),.UNSPECIFIED.)
CURVE()
GEOMETRIC_REPRESENTATION_ITEM()
RATIONAL_B_SPLINE_CURVE((1.,0.866025403784439,1.,0.866025403784439,1.,0.866025403784439,
1.,0.866025403784439,1.,0.866025403784439,1.,0.866025403784439,1.))
REPRESENTATION_ITEM('')
);
#1420=(
BOUNDED_CURVE()
B_SPLINE_CURVE(2,(#240614,#240615,#240616,#240617,#240618,#240619,#240620,
#240621,#240622,#240623,#240624,#240625,#240626),.UNSPECIFIED.,.F.,.F.)
B_SPLINE_CURVE_WITH_KNOTS((3,2,2,2,2,2,3),(0.456521739130435,0.463768115942029,
0.471014492753623,0.478260869565218,0.485507246376812,0.492753623188406,
0.5),.UNSPECIFIED.)
CURVE()
GEOMETRIC_REPRESENTATION_ITEM()
RATIONAL_B_SPLINE_CURVE((1.,0.866025403784439,1.,0.866025403784439,1.,0.866025403784439,
1.,0.866025403784439,1.,0.866025403784439,1.,0.866025403784439,1.))
REPRESENTATION_ITEM('')
);
#1421=(
BOUNDED_CURVE()
B_SPLINE_CURVE(2,(#240631,#240632,#240633,#240634,#240635,#240636,#240637,
#240638,#240639,#240640,#240641,#240642,#240643),.UNSPECIFIED.,.F.,.F.)
B_SPLINE_CURVE_WITH_KNOTS((3,2,2,2,2,2,3),(0.415612589480934,0.422904038419196,
0.430195487357458,0.43748693629572,0.444778385233982,0.452069834172244,
0.459361283110506),.UNSPECIFIED.)
CURVE()
GEOMETRIC_REPRESENTATION_ITEM()
RATIONAL_B_SPLINE_CURVE((1.,0.866025403784439,1.,0.866025403784439,1.,0.866025403784439,
1.,0.866025403784439,1.,0.866025403784439,1.,0.866025403784439,1.))
REPRESENTATION_ITEM('')
);
#1422=(
BOUNDED_CURVE()
B_SPLINE_CURVE(2,(#240644,#240645,#240646,#240647,#240648,#240649,#240650,
#240651,#240652,#240653,#240654,#240655,#240656),.UNSPECIFIED.,.F.,.F.)
B_SPLINE_CURVE_WITH_KNOTS((3,2,2,2,2,2,3),(0.413043478260869,0.420289855072464,
0.427536231884058,0.434782608695652,0.442028985507246,0.449275362318841,
0.456521739130435),.UNSPECIFIED.)
CURVE()
GEOMETRIC_REPRESENTATION_ITEM()
RATIONAL_B_SPLINE_CURVE((1.,0.866025403784439,1.,0.866025403784439,1.,0.866025403784439,
1.,0.866025403784439,1.,0.866025403784439,1.,0.866025403784439,1.))
REPRESENTATION_ITEM('')
);
#1423=(
BOUNDED_CURVE()
B_SPLINE_CURVE(2,(#240661,#240662,#240663,#240664,#240665,#240666,#240667,
#240668,#240669,#240670,#240671,#240672,#240673),.UNSPECIFIED.,.F.,.F.)
B_SPLINE_CURVE_WITH_KNOTS((3,2,2,2,2,2,3),(0.371863895851362,0.379155344789624,
0.386446793727886,0.393738242666148,0.40102969160441,0.408321140542672,
0.415612589480934),.UNSPECIFIED.)
CURVE()
GEOMETRIC_REPRESENTATION_ITEM()
RATIONAL_B_SPLINE_CURVE((1.,0.866025403784439,1.,0.866025403784439,1.,0.866025403784439,
1.,0.866025403784439,1.,0.866025403784439,1.,0.866025403784439,1.))
REPRESENTATION_ITEM('')
);
#1424=(
BOUNDED_CURVE()
B_SPLINE_CURVE(2,(#240674,#240675,#240676,#240677,#240678,#240679,#240680,
#240681,#240682,#240683,#240684,#240685,#240686),.UNSPECIFIED.,.F.,.F.)
B_SPLINE_CURVE_WITH_KNOTS((3,2,2,2,2,2,3),(0.369565217391304,0.376811594202899,
0.384057971014493,0.391304347826087,0.398550724637682,0.405797101449275,
0.413043478260869),.UNSPECIFIED.)
CURVE()
GEOMETRIC_REPRESENTATION_ITEM()
RATIONAL_B_SPLINE_CURVE((1.,0.866025403784439,1.,0.866025403784439,1.,0.866025403784439,
1.,0.866025403784439,1.,0.866025403784439,1.,0.866025403784439,1.))
REPRESENTATION_ITEM('')
);
#1425=(
BOUNDED_CURVE()
B_SPLINE_CURVE(2,(#240691,#240692,#240693,#240694,#240695,#240696,#240697,
#240698,#240699,#240700,#240701,#240702,#240703),.UNSPECIFIED.,.F.,.F.)
B_SPLINE_CURVE_WITH_KNOTS((3,2,2,2,2,2,3),(0.32811520222179,0.335406651160052,
0.342698100098314,0.349989549036576,0.357280997974838,0.3645724469131,0.371863895851362),
 .UNSPECIFIED.)
CURVE()
GEOMETRIC_REPRESENTATION_ITEM()
RATIONAL_B_SPLINE_CURVE((1.,0.866025403784439,1.,0.866025403784439,1.,0.866025403784439,
1.,0.866025403784439,1.,0.866025403784439,1.,0.866025403784439,1.))
REPRESENTATION_ITEM('')
);
#1426=(
BOUNDED_CURVE()
B_SPLINE_CURVE(2,(#240704,#240705,#240706,#240707,#240708,#240709,#240710,
#240711,#240712,#240713,#240714,#240715,#240716),.UNSPECIFIED.,.F.,.F.)
B_SPLINE_CURVE_WITH_KNOTS((3,2,2,2,2,2,3),(0.326086956521739,0.333333333333334,
0.340579710144927,0.347826086956522,0.355072463768116,0.36231884057971,
0.369565217391304),.UNSPECIFIED.)
CURVE()
GEOMETRIC_REPRESENTATION_ITEM()
RATIONAL_B_SPLINE_CURVE((1.,0.866025403784439,1.,0.866025403784439,1.,0.866025403784439,
1.,0.866025403784439,1.,0.866025403784439,1.,0.866025403784439,1.))
REPRESENTATION_ITEM('')
);
#1427=(
BOUNDED_CURVE()
B_SPLINE_CURVE(2,(#240721,#240722,#240723,#240724,#240725,#240726,#240727,
#240728,#240729,#240730,#240731,#240732,#240733),.UNSPECIFIED.,.F.,.F.)
B_SPLINE_CURVE_WITH_KNOTS((3,2,2,2,2,2,3),(0.284366508592218,0.29165795753048,
0.298949406468742,0.306240855407004,0.313532304345266,0.320823753283528,
0.32811520222179),.UNSPECIFIED.)
CURVE()
GEOMETRIC_REPRESENTATION_ITEM()
RATIONAL_B_SPLINE_CURVE((1.,0.866025403784439,1.,0.866025403784439,1.,0.866025403784439,
1.,0.866025403784439,1.,0.866025403784439,1.,0.866025403784439,1.))
REPRESENTATION_ITEM('')
);
#1428=(
BOUNDED_CURVE()
B_SPLINE_CURVE(2,(#240734,#240735,#240736,#240737,#240738,#240739,#240740,
#240741,#240742,#240743,#240744,#240745,#240746),.UNSPECIFIED.,.F.,.F.)
B_SPLINE_CURVE_WITH_KNOTS((3,2,2,2,2,2,3),(0.282608695652174,0.289855072463769,
0.297101449275363,0.304347826086956,0.311594202898551,0.318840579710145,
0.326086956521739),.UNSPECIFIED.)
CURVE()
GEOMETRIC_REPRESENTATION_ITEM()
RATIONAL_B_SPLINE_CURVE((1.,0.866025403784439,1.,0.866025403784439,1.,0.866025403784439,
1.,0.866025403784439,1.,0.866025403784439,1.,0.866025403784439,1.))
REPRESENTATION_ITEM('')
);
#1429=(
BOUNDED_CURVE()
B_SPLINE_CURVE(2,(#240751,#240752,#240753,#240754,#240755,#240756,#240757,
#240758,#240759,#240760,#240761,#240762,#240763),.UNSPECIFIED.,.F.,.F.)
B_SPLINE_CURVE_WITH_KNOTS((3,2,2,2,2,2,3),(0.240617814962646,0.247909263900908,
0.25520071283917,0.262492161777432,0.269783610715694,0.277075059653956,
0.284366508592218),.UNSPECIFIED.)
CURVE()
GEOMETRIC_REPRESENTATION_ITEM()
RATIONAL_B_SPLINE_CURVE((1.,0.866025403784439,1.,0.866025403784439,1.,0.866025403784439,
1.,0.866025403784439,1.,0.866025403784439,1.,0.866025403784439,1.))
REPRESENTATION_ITEM('')
);
#1430=(
BOUNDED_CURVE()
B_SPLINE_CURVE(2,(#240764,#240765,#240766,#240767,#240768,#240769,#240770,
#240771,#240772,#240773,#240774,#240775,#240776),.UNSPECIFIED.,.F.,.F.)
B_SPLINE_CURVE_WITH_KNOTS((3,2,2,2,2,2,3),(0.239130434782609,0.246376811594203,
0.253623188405797,0.260869565217392,0.268115942028985,0.27536231884058,
0.282608695652174),.UNSPECIFIED.)
CURVE()
GEOMETRIC_REPRESENTATION_ITEM()
RATIONAL_B_SPLINE_CURVE((1.,0.866025403784439,1.,0.866025403784439,1.,0.866025403784439,
1.,0.866025403784439,1.,0.866025403784439,1.,0.866025403784439,1.))
REPRESENTATION_ITEM('')
);
#1431=(
BOUNDED_CURVE()
B_SPLINE_CURVE(2,(#240781,#240782,#240783,#240784,#240785,#240786,#240787,
#240788,#240789,#240790,#240791,#240792,#240793),.UNSPECIFIED.,.F.,.F.)
B_SPLINE_CURVE_WITH_KNOTS((3,2,2,2,2,2,3),(0.196869121333074,0.204160570271336,
0.211452019209598,0.21874346814786,0.226034917086122,0.233326366024384,
0.240617814962646),.UNSPECIFIED.)
CURVE()
GEOMETRIC_REPRESENTATION_ITEM()
RATIONAL_B_SPLINE_CURVE((1.,0.866025403784439,1.,0.866025403784439,1.,0.866025403784439,
1.,0.866025403784439,1.,0.866025403784439,1.,0.866025403784439,1.))
REPRESENTATION_ITEM('')
);
#1432=(
BOUNDED_CURVE()
B_SPLINE_CURVE(2,(#240794,#240795,#240796,#240797,#240798,#240799,#240800,
#240801,#240802,#240803,#240804,#240805,#240806),.UNSPECIFIED.,.F.,.F.)
B_SPLINE_CURVE_WITH_KNOTS((3,2,2,2,2,2,3),(0.195652173913044,0.202898550724638,
0.210144927536232,0.217391304347826,0.224637681159421,0.231884057971015,
0.239130434782609),.UNSPECIFIED.)
CURVE()
GEOMETRIC_REPRESENTATION_ITEM()
RATIONAL_B_SPLINE_CURVE((1.,0.866025403784439,1.,0.866025403784439,1.,0.866025403784439,
1.,0.866025403784439,1.,0.866025403784439,1.,0.866025403784439,1.))
REPRESENTATION_ITEM('')
);
#1433=(
BOUNDED_CURVE()
B_SPLINE_CURVE(2,(#240811,#240812,#240813,#240814,#240815,#240816,#240817,
#240818,#240819,#240820,#240821,#240822,#240823),.UNSPECIFIED.,.F.,.F.)
B_SPLINE_CURVE_WITH_KNOTS((3,2,2,2,2,2,3),(0.153120427703502,0.160411876641764,
0.167703325580026,0.174994774518288,0.18228622345655,0.189577672394812,
0.196869121333074),.UNSPECIFIED.)
CURVE()
GEOMETRIC_REPRESENTATION_ITEM()
RATIONAL_B_SPLINE_CURVE((1.,0.866025403784439,1.,0.866025403784439,1.,0.866025403784439,
1.,0.866025403784439,1.,0.866025403784439,1.,0.866025403784439,1.))
REPRESENTATION_ITEM('')
);
#1434=(
BOUNDED_CURVE()
B_SPLINE_CURVE(2,(#240824,#240825,#240826,#240827,#240828,#240829,#240830,
#240831,#240832,#240833,#240834,#240835,#240836),.UNSPECIFIED.,.F.,.F.)
B_SPLINE_CURVE_WITH_KNOTS((3,2,2,2,2,2,3),(0.152173913043478,0.159420289855073,
0.166666666666667,0.173913043478261,0.181159420289855,0.18840579710145,
0.195652173913044),.UNSPECIFIED.)
CURVE()
GEOMETRIC_REPRESENTATION_ITEM()
RATIONAL_B_SPLINE_CURVE((1.,0.866025403784439,1.,0.866025403784439,1.,0.866025403784439,
1.,0.866025403784439,1.,0.866025403784439,1.,0.866025403784439,1.))
REPRESENTATION_ITEM('')
);
#1435=(
BOUNDED_CURVE()
B_SPLINE_CURVE(2,(#240841,#240842,#240843,#240844,#240845,#240846,#240847,
#240848,#240849,#240850,#240851,#240852,#240853),.UNSPECIFIED.,.F.,.F.)
B_SPLINE_CURVE_WITH_KNOTS((3,2,2,2,2,2,3),(0.10937173407393,0.116663183012192,
0.123954631950454,0.131246080888716,0.138537529826978,0.14582897876524,
0.153120427703502),.UNSPECIFIED.)
CURVE()
GEOMETRIC_REPRESENTATION_ITEM()
RATIONAL_B_SPLINE_CURVE((1.,0.866025403784439,1.,0.866025403784439,1.,0.866025403784439,
1.,0.866025403784439,1.,0.866025403784439,1.,0.866025403784439,1.))
REPRESENTATION_ITEM('')
);
#1436=(
BOUNDED_CURVE()
B_SPLINE_CURVE(2,(#240854,#240855,#240856,#240857,#240858,#240859,#240860,
#240861,#240862,#240863,#240864,#240865,#240866),.UNSPECIFIED.,.F.,.F.)
B_SPLINE_CURVE_WITH_KNOTS((3,2,2,2,2,2,3),(0.108695652173913,0.115942028985507,
0.123188405797102,0.130434782608696,0.13768115942029,0.144927536231884,
0.152173913043478),.UNSPECIFIED.)
CURVE()
GEOMETRIC_REPRESENTATION_ITEM()
RATIONAL_B_SPLINE_CURVE((1.,0.866025403784439,1.,0.866025403784439,1.,0.866025403784439,
1.,0.866025403784439,1.,0.866025403784439,1.,0.866025403784439,1.))
REPRESENTATION_ITEM('')
);
#1437=(
BOUNDED_CURVE()
B_SPLINE_CURVE(2,(#240871,#240872,#240873,#240874,#240875,#240876,#240877,
#240878,#240879,#240880,#240881,#240882,#240883),.UNSPECIFIED.,.F.,.F.)
B_SPLINE_CURVE_WITH_KNOTS((3,2,2,2,2,2,3),(0.065623040444358,0.07291448938262,
0.080205938320882,0.087497387259144,0.094788836197406,0.102080285135668,
0.10937173407393),.UNSPECIFIED.)
CURVE()
GEOMETRIC_REPRESENTATION_ITEM()
RATIONAL_B_SPLINE_CURVE((1.,0.866025403784439,1.,0.866025403784439,1.,0.866025403784439,
1.,0.866025403784439,1.,0.866025403784439,1.,0.866025403784439,1.))
REPRESENTATION_ITEM('')
);
#1438=(
BOUNDED_CURVE()
B_SPLINE_CURVE(2,(#240884,#240885,#240886,#240887,#240888,#240889,#240890,
#240891,#240892,#240893,#240894,#240895,#240896),.UNSPECIFIED.,.F.,.F.)
B_SPLINE_CURVE_WITH_KNOTS((3,2,2,2,2,2,3),(0.065217391304348,0.0724637681159421,
0.0797101449275364,0.0869565217391305,0.0942028985507248,0.101449275362319,
0.108695652173913),.UNSPECIFIED.)
CURVE()
GEOMETRIC_REPRESENTATION_ITEM()
RATIONAL_B_SPLINE_CURVE((1.,0.866025403784439,1.,0.866025403784439,1.,0.866025403784439,
1.,0.866025403784439,1.,0.866025403784439,1.,0.866025403784439,1.))
REPRESENTATION_ITEM('')
);
#1439=(
BOUNDED_CURVE()
B_SPLINE_CURVE(2,(#240903,#240904,#240905,#240906,#240907),
 .UNSPECIFIED.,.F.,.F.)
B_SPLINE_CURVE_WITH_KNOTS((3,2,3),(0.0118893770663288,0.014582897876524,
0.021874346814786),.UNSPECIFIED.)
CURVE()
GEOMETRIC_REPRESENTATION_ITEM()
RATIONAL_B_SPLINE_CURVE((0.937582367981144,0.950508689562306,1.,0.866025403784439,
1.))
REPRESENTATION_ITEM('')
);
#1440=(
BOUNDED_CURVE()
B_SPLINE_CURVE(2,(#242295,#242296,#242297),.UNSPECIFIED.,.F.,.F.)
B_SPLINE_CURVE_WITH_KNOTS((3,3),(0.809350832147077,0.81291946675533),
 .UNSPECIFIED.)
CURVE()
GEOMETRIC_REPRESENTATION_ITEM()
RATIONAL_B_SPLINE_CURVE((1.,0.934429166996968,0.933042653441986))
REPRESENTATION_ITEM('')
);
#1441=(
BOUNDED_CURVE()
B_SPLINE_CURVE(2,(#242305,#242306,#242307),.UNSPECIFIED.,.F.,.F.)
B_SPLINE_CURVE_WITH_KNOTS((3,3),(0.804347826086956,0.809954704477924),
 .UNSPECIFIED.)
CURVE()
GEOMETRIC_REPRESENTATION_ITEM()
RATIONAL_B_SPLINE_CURVE((1.,0.896337260952566,0.953092448442884))
REPRESENTATION_ITEM('')
);
#1442=(
BOUNDED_CURVE()
B_SPLINE_CURVE(2,(#242313,#242314,#242315,#242316,#242317,#242318,#242319),
 .UNSPECIFIED.,.F.,.F.)
B_SPLINE_CURVE_WITH_KNOTS((3,2,2,3),(0.76560213851751,0.772893587455772,
0.780185036394034,0.780206651397652),.UNSPECIFIED.)
CURVE()
GEOMETRIC_REPRESENTATION_ITEM()
RATIONAL_B_SPLINE_CURVE((1.,0.866025403784439,1.,0.866025403784439,1.,0.999602841437075,
0.999208037573154))
REPRESENTATION_ITEM('')
);
#1443=(
BOUNDED_CURVE()
B_SPLINE_CURVE(2,(#242333,#242334,#242335,#242336,#242337,#242338,#242339),
 .UNSPECIFIED.,.F.,.F.)
B_SPLINE_CURVE_WITH_KNOTS((3,2,2,3),(0.787646407455994,0.794767934270535,
0.802059383208806,0.809350832147077),.UNSPECIFIED.)
CURVE()
GEOMETRIC_REPRESENTATION_ITEM()
RATIONAL_B_SPLINE_CURVE((0.993901151909826,0.86914758815514,1.,0.866025403784439,
1.,0.866025403784439,1.))
REPRESENTATION_ITEM('')
);
#1444=(
BOUNDED_CURVE()
B_SPLINE_CURVE(2,(#242340,#242341,#242342,#242343,#242344,#242345,#242346,
#242347,#242348,#242349,#242350,#242351,#242352),.UNSPECIFIED.,.F.,.F.)
B_SPLINE_CURVE_WITH_KNOTS((3,2,2,2,2,2,3),(0.760869565217391,0.768115942028986,
0.77536231884058,0.782608695652174,0.789855072463768,0.797101449275362,
0.804347826086956),.UNSPECIFIED.)
CURVE()
GEOMETRIC_REPRESENTATION_ITEM()
RATIONAL_B_SPLINE_CURVE((1.,0.866025403784439,1.,0.866025403784439,1.,0.866025403784439,
1.,0.866025403784439,1.,0.866025403784439,1.,0.866025403784439,1.))
REPRESENTATION_ITEM('')
);
#1445=(
BOUNDED_CURVE()
B_SPLINE_CURVE(2,(#242357,#242358,#242359,#242360,#242361,#242362,#242363,
#242364,#242365,#242366,#242367,#242368,#242369),.UNSPECIFIED.,.F.,.F.)
B_SPLINE_CURVE_WITH_KNOTS((3,2,2,2,2,2,3),(0.721853444887938,0.7291448938262,
0.736436342764462,0.743727791702724,0.751019240640986,0.758310689579248,
0.76560213851751),.UNSPECIFIED.)
CURVE()
GEOMETRIC_REPRESENTATION_ITEM()
RATIONAL_B_SPLINE_CURVE((1.,0.866025403784439,1.,0.866025403784439,1.,0.866025403784439,
1.,0.866025403784439,1.,0.866025403784439,1.,0.866025403784439,1.))
REPRESENTATION_ITEM('')
);
#1446=(
BOUNDED_CURVE()
B_SPLINE_CURVE(2,(#242370,#242371,#242372,#242373,#242374,#242375,#242376,
#242377,#242378,#242379,#242380,#242381,#242382),.UNSPECIFIED.,.F.,.F.)
B_SPLINE_CURVE_WITH_KNOTS((3,2,2,2,2,2,3),(0.717391304347826,0.72463768115942,
0.731884057971015,0.739130434782609,0.746376811594203,0.753623188405797,
0.760869565217391),.UNSPECIFIED.)
CURVE()
GEOMETRIC_REPRESENTATION_ITEM()
RATIONAL_B_SPLINE_CURVE((1.,0.866025403784439,1.,0.866025403784439,1.,0.866025403784439,
1.,0.866025403784439,1.,0.866025403784439,1.,0.866025403784439,1.))
REPRESENTATION_ITEM('')
);
#1447=(
BOUNDED_CURVE()
B_SPLINE_CURVE(2,(#242387,#242388,#242389,#242390,#242391,#242392,#242393,
#242394,#242395,#242396,#242397,#242398,#242399),.UNSPECIFIED.,.F.,.F.)
B_SPLINE_CURVE_WITH_KNOTS((3,2,2,2,2,2,3),(0.678104751258366,0.685396200196628,
0.69268764913489,0.699979098073152,0.707270547011414,0.714561995949676,
0.721853444887938),.UNSPECIFIED.)
CURVE()
GEOMETRIC_REPRESENTATION_ITEM()
RATIONAL_B_SPLINE_CURVE((1.,0.866025403784439,1.,0.866025403784439,1.,0.866025403784439,
1.,0.866025403784439,1.,0.866025403784439,1.,0.866025403784439,1.))
REPRESENTATION_ITEM('')
);
#1448=(
BOUNDED_CURVE()
B_SPLINE_CURVE(2,(#242400,#242401,#242402,#242403,#242404,#242405,#242406,
#242407,#242408,#242409,#242410,#242411,#242412),.UNSPECIFIED.,.F.,.F.)
B_SPLINE_CURVE_WITH_KNOTS((3,2,2,2,2,2,3),(0.673913043478261,0.681159420289855,
0.688405797101449,0.695652173913044,0.702898550724638,0.710144927536232,
0.717391304347826),.UNSPECIFIED.)
CURVE()
GEOMETRIC_REPRESENTATION_ITEM()
RATIONAL_B_SPLINE_CURVE((1.,0.866025403784439,1.,0.866025403784439,1.,0.866025403784439,
1.,0.866025403784439,1.,0.866025403784439,1.,0.866025403784439,1.))
REPRESENTATION_ITEM('')
);
#1449=(
BOUNDED_CURVE()
B_SPLINE_CURVE(2,(#242417,#242418,#242419,#242420,#242421,#242422,#242423,
#242424,#242425,#242426,#242427,#242428,#242429),.UNSPECIFIED.,.F.,.F.)
B_SPLINE_CURVE_WITH_KNOTS((3,2,2,2,2,2,3),(0.634356057628794,0.641647506567056,
0.648938955505318,0.65623040444358,0.663521853381842,0.670813302320104,
0.678104751258366),.UNSPECIFIED.)
CURVE()
GEOMETRIC_REPRESENTATION_ITEM()
RATIONAL_B_SPLINE_CURVE((1.,0.866025403784439,1.,0.866025403784439,1.,0.866025403784439,
1.,0.866025403784439,1.,0.866025403784439,1.,0.866025403784439,1.))
REPRESENTATION_ITEM('')
);
#1450=(
BOUNDED_CURVE()
B_SPLINE_CURVE(2,(#242430,#242431,#242432,#242433,#242434,#242435,#242436,
#242437,#242438,#242439,#242440,#242441,#242442),.UNSPECIFIED.,.F.,.F.)
B_SPLINE_CURVE_WITH_KNOTS((3,2,2,2,2,2,3),(0.630434782608696,0.63768115942029,
0.644927536231884,0.652173913043478,0.659420289855073,0.666666666666667,
0.673913043478261),.UNSPECIFIED.)
CURVE()
GEOMETRIC_REPRESENTATION_ITEM()
RATIONAL_B_SPLINE_CURVE((1.,0.866025403784439,1.,0.866025403784439,1.,0.866025403784439,
1.,0.866025403784439,1.,0.866025403784439,1.,0.866025403784439,1.))
REPRESENTATION_ITEM('')
);
#1451=(
BOUNDED_CURVE()
B_SPLINE_CURVE(2,(#242447,#242448,#242449,#242450,#242451,#242452,#242453,
#242454,#242455,#242456,#242457,#242458,#242459),.UNSPECIFIED.,.F.,.F.)
B_SPLINE_CURVE_WITH_KNOTS((3,2,2,2,2,2,3),(0.590607363999222,0.597898812937484,
0.605190261875746,0.612481710814008,0.61977315975227,0.627064608690532,
0.634356057628794),.UNSPECIFIED.)
CURVE()
GEOMETRIC_REPRESENTATION_ITEM()
RATIONAL_B_SPLINE_CURVE((1.,0.866025403784439,1.,0.866025403784439,1.,0.866025403784439,
1.,0.866025403784439,1.,0.866025403784439,1.,0.866025403784439,1.))
REPRESENTATION_ITEM('')
);
#1452=(
BOUNDED_CURVE()
B_SPLINE_CURVE(2,(#242460,#242461,#242462,#242463,#242464,#242465,#242466,
#242467,#242468,#242469,#242470,#242471,#242472),.UNSPECIFIED.,.F.,.F.)
B_SPLINE_CURVE_WITH_KNOTS((3,2,2,2,2,2,3),(0.586956521739131,0.594202898550725,
0.601449275362319,0.608695652173913,0.615942028985507,0.623188405797101,
0.630434782608696),.UNSPECIFIED.)
CURVE()
GEOMETRIC_REPRESENTATION_ITEM()
RATIONAL_B_SPLINE_CURVE((1.,0.866025403784439,1.,0.866025403784439,1.,0.866025403784439,
1.,0.866025403784439,1.,0.866025403784439,1.,0.866025403784439,1.))
REPRESENTATION_ITEM('')
);
#1453=(
BOUNDED_CURVE()
B_SPLINE_CURVE(2,(#242477,#242478,#242479,#242480,#242481,#242482,#242483,
#242484,#242485,#242486,#242487,#242488,#242489),.UNSPECIFIED.,.F.,.F.)
B_SPLINE_CURVE_WITH_KNOTS((3,2,2,2,2,2,3),(0.54685867036965,0.554150119307912,
0.561441568246174,0.568733017184436,0.576024466122698,0.58331591506096,
0.590607363999222),.UNSPECIFIED.)
CURVE()
GEOMETRIC_REPRESENTATION_ITEM()
RATIONAL_B_SPLINE_CURVE((1.,0.866025403784439,1.,0.866025403784439,1.,0.866025403784439,
1.,0.866025403784439,1.,0.866025403784439,1.,0.866025403784439,1.))
REPRESENTATION_ITEM('')
);
#1454=(
BOUNDED_CURVE()
B_SPLINE_CURVE(2,(#242490,#242491,#242492,#242493,#242494,#242495,#242496,
#242497,#242498,#242499,#242500,#242501,#242502),.UNSPECIFIED.,.F.,.F.)
B_SPLINE_CURVE_WITH_KNOTS((3,2,2,2,2,2,3),(0.543478260869565,0.55072463768116,
0.557971014492754,0.565217391304348,0.572463768115942,0.579710144927536,
0.586956521739131),.UNSPECIFIED.)
CURVE()
GEOMETRIC_REPRESENTATION_ITEM()
RATIONAL_B_SPLINE_CURVE((1.,0.866025403784439,1.,0.866025403784439,1.,0.866025403784439,
1.,0.866025403784439,1.,0.866025403784439,1.,0.866025403784439,1.))
REPRESENTATION_ITEM('')
);
#1455=(
BOUNDED_CURVE()
B_SPLINE_CURVE(2,(#242507,#242508,#242509,#242510,#242511,#242512,#242513,
#242514,#242515,#242516,#242517,#242518,#242519),.UNSPECIFIED.,.F.,.F.)
B_SPLINE_CURVE_WITH_KNOTS((3,2,2,2,2,2,3),(0.503109976740078,0.51040142567834,
0.517692874616602,0.524984323554864,0.532275772493126,0.539567221431388,
0.54685867036965),.UNSPECIFIED.)
CURVE()
GEOMETRIC_REPRESENTATION_ITEM()
RATIONAL_B_SPLINE_CURVE((1.,0.866025403784439,1.,0.866025403784439,1.,0.866025403784439,
1.,0.866025403784439,1.,0.866025403784439,1.,0.866025403784439,1.))
REPRESENTATION_ITEM('')
);
#1456=(
BOUNDED_CURVE()
B_SPLINE_CURVE(2,(#242520,#242521,#242522,#242523,#242524,#242525,#242526,
#242527,#242528,#242529,#242530,#242531,#242532),.UNSPECIFIED.,.F.,.F.)
B_SPLINE_CURVE_WITH_KNOTS((3,2,2,2,2,2,3),(0.5,0.507246376811594,0.514492753623188,
0.521739130434783,0.528985507246377,0.536231884057971,0.543478260869565),
 .UNSPECIFIED.)
CURVE()
GEOMETRIC_REPRESENTATION_ITEM()
RATIONAL_B_SPLINE_CURVE((1.,0.866025403784439,1.,0.866025403784439,1.,0.866025403784439,
1.,0.866025403784439,1.,0.866025403784439,1.,0.866025403784439,1.))
REPRESENTATION_ITEM('')
);
#1457=(
BOUNDED_CURVE()
B_SPLINE_CURVE(2,(#242537,#242538,#242539,#242540,#242541,#242542,#242543,
#242544,#242545,#242546,#242547,#242548,#242549),.UNSPECIFIED.,.F.,.F.)
B_SPLINE_CURVE_WITH_KNOTS((3,2,2,2,2,2,3),(0.459361283110506,0.466652732048768,
0.47394418098703,0.481235629925292,0.488527078863554,0.495818527801816,
0.503109976740078),.UNSPECIFIED.)
CURVE()
GEOMETRIC_REPRESENTATION_ITEM()
RATIONAL_B_SPLINE_CURVE((1.,0.866025403784439,1.,0.866025403784439,1.,0.866025403784439,
1.,0.866025403784439,1.,0.866025403784439,1.,0.866025403784439,1.))
REPRESENTATION_ITEM('')
);
#1458=(
BOUNDED_CURVE()
B_SPLINE_CURVE(2,(#242550,#242551,#242552,#242553,#242554,#242555,#242556,
#242557,#242558,#242559,#242560,#242561,#242562),.UNSPECIFIED.,.F.,.F.)
B_SPLINE_CURVE_WITH_KNOTS((3,2,2,2,2,2,3),(0.456521739130435,0.463768115942029,
0.471014492753623,0.478260869565218,0.485507246376812,0.492753623188406,
0.5),.UNSPECIFIED.)
CURVE()
GEOMETRIC_REPRESENTATION_ITEM()
RATIONAL_B_SPLINE_CURVE((1.,0.866025403784439,1.,0.866025403784439,1.,0.866025403784439,
1.,0.866025403784439,1.,0.866025403784439,1.,0.866025403784439,1.))
REPRESENTATION_ITEM('')
);
#1459=(
BOUNDED_CURVE()
B_SPLINE_CURVE(2,(#242567,#242568,#242569,#242570,#242571,#242572,#242573,
#242574,#242575,#242576,#242577,#242578,#242579),.UNSPECIFIED.,.F.,.F.)
B_SPLINE_CURVE_WITH_KNOTS((3,2,2,2,2,2,3),(0.415612589480934,0.422904038419196,
0.430195487357458,0.43748693629572,0.444778385233982,0.452069834172244,
0.459361283110506),.UNSPECIFIED.)
CURVE()
GEOMETRIC_REPRESENTATION_ITEM()
RATIONAL_B_SPLINE_CURVE((1.,0.866025403784439,1.,0.866025403784439,1.,0.866025403784439,
1.,0.866025403784439,1.,0.866025403784439,1.,0.866025403784439,1.))
REPRESENTATION_ITEM('')
);
#1460=(
BOUNDED_CURVE()
B_SPLINE_CURVE(2,(#242580,#242581,#242582,#242583,#242584,#242585,#242586,
#242587,#242588,#242589,#242590,#242591,#242592),.UNSPECIFIED.,.F.,.F.)
B_SPLINE_CURVE_WITH_KNOTS((3,2,2,2,2,2,3),(0.41304347826087,0.420289855072464,
0.427536231884058,0.434782608695652,0.442028985507247,0.449275362318841,
0.456521739130435),.UNSPECIFIED.)
CURVE()
GEOMETRIC_REPRESENTATION_ITEM()
RATIONAL_B_SPLINE_CURVE((1.,0.866025403784439,1.,0.866025403784439,1.,0.866025403784439,
1.,0.866025403784439,1.,0.866025403784439,1.,0.866025403784439,1.))
REPRESENTATION_ITEM('')
);
#1461=(
BOUNDED_CURVE()
B_SPLINE_CURVE(2,(#242597,#242598,#242599,#242600,#242601,#242602,#242603,
#242604,#242605,#242606,#242607,#242608,#242609),.UNSPECIFIED.,.F.,.F.)
B_SPLINE_CURVE_WITH_KNOTS((3,2,2,2,2,2,3),(0.371863895851362,0.379155344789624,
0.386446793727886,0.393738242666148,0.40102969160441,0.408321140542672,
0.415612589480934),.UNSPECIFIED.)
CURVE()
GEOMETRIC_REPRESENTATION_ITEM()
RATIONAL_B_SPLINE_CURVE((1.,0.866025403784439,1.,0.866025403784439,1.,0.866025403784439,
1.,0.866025403784439,1.,0.866025403784439,1.,0.866025403784439,1.))
REPRESENTATION_ITEM('')
);
#1462=(
BOUNDED_CURVE()
B_SPLINE_CURVE(2,(#242610,#242611,#242612,#242613,#242614,#242615,#242616,
#242617,#242618,#242619,#242620,#242621,#242622),.UNSPECIFIED.,.F.,.F.)
B_SPLINE_CURVE_WITH_KNOTS((3,2,2,2,2,2,3),(0.369565217391304,0.376811594202899,
0.384057971014493,0.391304347826087,0.398550724637681,0.405797101449275,
0.41304347826087),.UNSPECIFIED.)
CURVE()
GEOMETRIC_REPRESENTATION_ITEM()
RATIONAL_B_SPLINE_CURVE((1.,0.866025403784439,1.,0.866025403784439,1.,0.866025403784439,
1.,0.866025403784439,1.,0.866025403784439,1.,0.866025403784439,1.))
REPRESENTATION_ITEM('')
);
#1463=(
BOUNDED_CURVE()
B_SPLINE_CURVE(2,(#242627,#242628,#242629,#242630,#242631,#242632,#242633,
#242634,#242635,#242636,#242637,#242638,#242639),.UNSPECIFIED.,.F.,.F.)
B_SPLINE_CURVE_WITH_KNOTS((3,2,2,2,2,2,3),(0.32811520222179,0.335406651160052,
0.342698100098314,0.349989549036576,0.357280997974838,0.3645724469131,0.371863895851362),
 .UNSPECIFIED.)
CURVE()
GEOMETRIC_REPRESENTATION_ITEM()
RATIONAL_B_SPLINE_CURVE((1.,0.866025403784439,1.,0.866025403784439,1.,0.866025403784439,
1.,0.866025403784439,1.,0.866025403784439,1.,0.866025403784439,1.))
REPRESENTATION_ITEM('')
);
#1464=(
BOUNDED_CURVE()
B_SPLINE_CURVE(2,(#242640,#242641,#242642,#242643,#242644,#242645,#242646,
#242647,#242648,#242649,#242650,#242651,#242652),.UNSPECIFIED.,.F.,.F.)
B_SPLINE_CURVE_WITH_KNOTS((3,2,2,2,2,2,3),(0.326086956521739,0.333333333333334,
0.340579710144927,0.347826086956522,0.355072463768116,0.36231884057971,
0.369565217391304),.UNSPECIFIED.)
CURVE()
GEOMETRIC_REPRESENTATION_ITEM()
RATIONAL_B_SPLINE_CURVE((1.,0.866025403784439,1.,0.866025403784439,1.,0.866025403784439,
1.,0.866025403784439,1.,0.866025403784439,1.,0.866025403784439,1.))
REPRESENTATION_ITEM('')
);
#1465=(
BOUNDED_CURVE()
B_SPLINE_CURVE(2,(#242657,#242658,#242659,#242660,#242661,#242662,#242663,
#242664,#242665,#242666,#242667,#242668,#242669),.UNSPECIFIED.,.F.,.F.)
B_SPLINE_CURVE_WITH_KNOTS((3,2,2,2,2,2,3),(0.284366508592218,0.29165795753048,
0.298949406468742,0.306240855407004,0.313532304345266,0.320823753283528,
0.32811520222179),.UNSPECIFIED.)
CURVE()
GEOMETRIC_REPRESENTATION_ITEM()
RATIONAL_B_SPLINE_CURVE((1.,0.866025403784439,1.,0.866025403784439,1.,0.866025403784439,
1.,0.866025403784439,1.,0.866025403784439,1.,0.866025403784439,1.))
REPRESENTATION_ITEM('')
);
#1466=(
BOUNDED_CURVE()
B_SPLINE_CURVE(2,(#242670,#242671,#242672,#242673,#242674,#242675,#242676,
#242677,#242678,#242679,#242680,#242681,#242682),.UNSPECIFIED.,.F.,.F.)
B_SPLINE_CURVE_WITH_KNOTS((3,2,2,2,2,2,3),(0.282608695652174,0.289855072463769,
0.297101449275363,0.304347826086956,0.311594202898551,0.318840579710145,
0.326086956521739),.UNSPECIFIED.)
CURVE()
GEOMETRIC_REPRESENTATION_ITEM()
RATIONAL_B_SPLINE_CURVE((1.,0.866025403784439,1.,0.866025403784439,1.,0.866025403784439,
1.,0.866025403784439,1.,0.866025403784439,1.,0.866025403784439,1.))
REPRESENTATION_ITEM('')
);
#1467=(
BOUNDED_CURVE()
B_SPLINE_CURVE(2,(#242687,#242688,#242689,#242690,#242691,#242692,#242693,
#242694,#242695,#242696,#242697,#242698,#242699),.UNSPECIFIED.,.F.,.F.)
B_SPLINE_CURVE_WITH_KNOTS((3,2,2,2,2,2,3),(0.240617814962646,0.247909263900908,
0.25520071283917,0.262492161777432,0.269783610715694,0.277075059653956,
0.284366508592218),.UNSPECIFIED.)
CURVE()
GEOMETRIC_REPRESENTATION_ITEM()
RATIONAL_B_SPLINE_CURVE((1.,0.866025403784439,1.,0.866025403784439,1.,0.866025403784439,
1.,0.866025403784439,1.,0.866025403784439,1.,0.866025403784439,1.))
REPRESENTATION_ITEM('')
);
#1468=(
BOUNDED_CURVE()
B_SPLINE_CURVE(2,(#242700,#242701,#242702,#242703,#242704,#242705,#242706,
#242707,#242708,#242709,#242710,#242711,#242712),.UNSPECIFIED.,.F.,.F.)
B_SPLINE_CURVE_WITH_KNOTS((3,2,2,2,2,2,3),(0.239130434782609,0.246376811594203,
0.253623188405797,0.260869565217392,0.268115942028985,0.27536231884058,
0.282608695652174),.UNSPECIFIED.)
CURVE()
GEOMETRIC_REPRESENTATION_ITEM()
RATIONAL_B_SPLINE_CURVE((1.,0.866025403784439,1.,0.866025403784439,1.,0.866025403784439,
1.,0.866025403784439,1.,0.866025403784439,1.,0.866025403784439,1.))
REPRESENTATION_ITEM('')
);
#1469=(
BOUNDED_CURVE()
B_SPLINE_CURVE(2,(#242717,#242718,#242719,#242720,#242721,#242722,#242723,
#242724,#242725,#242726,#242727,#242728,#242729),.UNSPECIFIED.,.F.,.F.)
B_SPLINE_CURVE_WITH_KNOTS((3,2,2,2,2,2,3),(0.196869121333074,0.204160570271336,
0.211452019209598,0.21874346814786,0.226034917086122,0.233326366024384,
0.240617814962646),.UNSPECIFIED.)
CURVE()
GEOMETRIC_REPRESENTATION_ITEM()
RATIONAL_B_SPLINE_CURVE((1.,0.866025403784439,1.,0.866025403784439,1.,0.866025403784439,
1.,0.866025403784439,1.,0.866025403784439,1.,0.866025403784439,1.))
REPRESENTATION_ITEM('')
);
#1470=(
BOUNDED_CURVE()
B_SPLINE_CURVE(2,(#242730,#242731,#242732,#242733,#242734,#242735,#242736,
#242737,#242738,#242739,#242740,#242741,#242742),.UNSPECIFIED.,.F.,.F.)
B_SPLINE_CURVE_WITH_KNOTS((3,2,2,2,2,2,3),(0.195652173913044,0.202898550724638,
0.210144927536232,0.217391304347826,0.224637681159421,0.231884057971014,
0.239130434782609),.UNSPECIFIED.)
CURVE()
GEOMETRIC_REPRESENTATION_ITEM()
RATIONAL_B_SPLINE_CURVE((1.,0.866025403784439,1.,0.866025403784439,1.,0.866025403784439,
1.,0.866025403784439,1.,0.866025403784439,1.,0.866025403784439,1.))
REPRESENTATION_ITEM('')
);
#1471=(
BOUNDED_CURVE()
B_SPLINE_CURVE(2,(#242747,#242748,#242749,#242750,#242751,#242752,#242753,
#242754,#242755,#242756,#242757,#242758,#242759),.UNSPECIFIED.,.F.,.F.)
B_SPLINE_CURVE_WITH_KNOTS((3,2,2,2,2,2,3),(0.153120427703502,0.160411876641764,
0.167703325580026,0.174994774518288,0.18228622345655,0.189577672394812,
0.196869121333074),.UNSPECIFIED.)
CURVE()
GEOMETRIC_REPRESENTATION_ITEM()
RATIONAL_B_SPLINE_CURVE((1.,0.866025403784439,1.,0.866025403784439,1.,0.866025403784439,
1.,0.866025403784439,1.,0.866025403784439,1.,0.866025403784439,1.))
REPRESENTATION_ITEM('')
);
#1472=(
BOUNDED_CURVE()
B_SPLINE_CURVE(2,(#242760,#242761,#242762,#242763,#242764,#242765,#242766,
#242767,#242768,#242769,#242770,#242771,#242772),.UNSPECIFIED.,.F.,.F.)
B_SPLINE_CURVE_WITH_KNOTS((3,2,2,2,2,2,3),(0.152173913043478,0.159420289855073,
0.166666666666667,0.173913043478261,0.181159420289855,0.18840579710145,
0.195652173913044),.UNSPECIFIED.)
CURVE()
GEOMETRIC_REPRESENTATION_ITEM()
RATIONAL_B_SPLINE_CURVE((1.,0.866025403784439,1.,0.866025403784439,1.,0.866025403784439,
1.,0.866025403784439,1.,0.866025403784439,1.,0.866025403784439,1.))
REPRESENTATION_ITEM('')
);
#1473=(
BOUNDED_CURVE()
B_SPLINE_CURVE(2,(#242777,#242778,#242779,#242780,#242781,#242782,#242783,
#242784,#242785,#242786,#242787,#242788,#242789),.UNSPECIFIED.,.F.,.F.)
B_SPLINE_CURVE_WITH_KNOTS((3,2,2,2,2,2,3),(0.10937173407393,0.116663183012192,
0.123954631950454,0.131246080888716,0.138537529826978,0.14582897876524,
0.153120427703502),.UNSPECIFIED.)
CURVE()
GEOMETRIC_REPRESENTATION_ITEM()
RATIONAL_B_SPLINE_CURVE((1.,0.866025403784439,1.,0.866025403784439,1.,0.866025403784439,
1.,0.866025403784439,1.,0.866025403784439,1.,0.866025403784439,1.))
REPRESENTATION_ITEM('')
);
#1474=(
BOUNDED_CURVE()
B_SPLINE_CURVE(2,(#242790,#242791,#242792,#242793,#242794,#242795,#242796,
#242797,#242798,#242799,#242800,#242801,#242802),.UNSPECIFIED.,.F.,.F.)
B_SPLINE_CURVE_WITH_KNOTS((3,2,2,2,2,2,3),(0.108695652173913,0.115942028985507,
0.123188405797102,0.130434782608696,0.13768115942029,0.144927536231884,
0.152173913043478),.UNSPECIFIED.)
CURVE()
GEOMETRIC_REPRESENTATION_ITEM()
RATIONAL_B_SPLINE_CURVE((1.,0.866025403784439,1.,0.866025403784439,1.,0.866025403784439,
1.,0.866025403784439,1.,0.866025403784439,1.,0.866025403784439,1.))
REPRESENTATION_ITEM('')
);
#1475=(
BOUNDED_CURVE()
B_SPLINE_CURVE(2,(#242807,#242808,#242809,#242810,#242811,#242812,#242813,
#242814,#242815,#242816,#242817,#242818,#242819),.UNSPECIFIED.,.F.,.F.)
B_SPLINE_CURVE_WITH_KNOTS((3,2,2,2,2,2,3),(0.065623040444358,0.07291448938262,
0.080205938320882,0.087497387259144,0.094788836197406,0.102080285135668,
0.10937173407393),.UNSPECIFIED.)
CURVE()
GEOMETRIC_REPRESENTATION_ITEM()
RATIONAL_B_SPLINE_CURVE((1.,0.866025403784439,1.,0.866025403784439,1.,0.866025403784439,
1.,0.866025403784439,1.,0.866025403784439,1.,0.866025403784439,1.))
REPRESENTATION_ITEM('')
);
#1476=(
BOUNDED_CURVE()
B_SPLINE_CURVE(2,(#242820,#242821,#242822,#242823,#242824,#242825,#242826,
#242827,#242828,#242829,#242830,#242831,#242832),.UNSPECIFIED.,.F.,.F.)
B_SPLINE_CURVE_WITH_KNOTS((3,2,2,2,2,2,3),(0.065217391304348,0.0724637681159422,
0.0797101449275364,0.0869565217391306,0.0942028985507248,0.101449275362319,
0.108695652173913),.UNSPECIFIED.)
CURVE()
GEOMETRIC_REPRESENTATION_ITEM()
RATIONAL_B_SPLINE_CURVE((1.,0.866025403784439,1.,0.866025403784439,1.,0.866025403784439,
1.,0.866025403784439,1.,0.866025403784439,1.,0.866025403784439,1.))
REPRESENTATION_ITEM('')
);
#1477=(
BOUNDED_CURVE()
B_SPLINE_CURVE(2,(#242839,#242840,#242841,#242842,#242843),
 .UNSPECIFIED.,.F.,.F.)
B_SPLINE_CURVE_WITH_KNOTS((3,2,3),(0.0118893770663289,0.014582897876524,
0.021874346814786),.UNSPECIFIED.)
CURVE()
GEOMETRIC_REPRESENTATION_ITEM()
RATIONAL_B_SPLINE_CURVE((0.937582367981145,0.950508689562308,1.,0.866025403784439,
1.))
REPRESENTATION_ITEM('')
);
#1478=(
BOUNDED_CURVE()
B_SPLINE_CURVE(2,(#242849,#242850,#242851),.UNSPECIFIED.,.F.,.F.)
B_SPLINE_CURVE_WITH_KNOTS((3,3),(0.809350832147077,0.812919467682267),
 .UNSPECIFIED.)
CURVE()
GEOMETRIC_REPRESENTATION_ITEM()
RATIONAL_B_SPLINE_CURVE((1.,0.934429149965244,0.933042652721709))
REPRESENTATION_ITEM('')
);
#1479=(
BOUNDED_CURVE()
B_SPLINE_CURVE(2,(#242859,#242860,#242861),.UNSPECIFIED.,.F.,.F.)
B_SPLINE_CURVE_WITH_KNOTS((3,3),(0.804347826086957,0.809954707320484),
 .UNSPECIFIED.)
CURVE()
GEOMETRIC_REPRESENTATION_ITEM()
RATIONAL_B_SPLINE_CURVE((1.,0.896337208397912,0.953092505990106))
REPRESENTATION_ITEM('')
);
#1480=(
BOUNDED_CURVE()
B_SPLINE_CURVE(2,(#242867,#242868,#242869,#242870,#242871,#242872,#242873),
 .UNSPECIFIED.,.F.,.F.)
B_SPLINE_CURVE_WITH_KNOTS((3,2,2,3),(0.76560213851751,0.772893587455772,
0.780185036394034,0.780206571546235),.UNSPECIFIED.)
CURVE()
GEOMETRIC_REPRESENTATION_ITEM()
RATIONAL_B_SPLINE_CURVE((1.,0.866025403784439,1.,0.866025403784439,1.,0.99960430864359,
0.999210954620584))
REPRESENTATION_ITEM('')
);
#1481=(
BOUNDED_CURVE()
B_SPLINE_CURVE(2,(#242887,#242888,#242889,#242890,#242891,#242892,#242893),
 .UNSPECIFIED.,.F.,.F.)
B_SPLINE_CURVE_WITH_KNOTS((3,2,2,3),(0.787646418746451,0.794767934270535,
0.802059383208806,0.809350832147077),.UNSPECIFIED.)
CURVE()
GEOMETRIC_REPRESENTATION_ITEM()
RATIONAL_B_SPLINE_CURVE((0.993900756342288,0.869147795608333,1.,0.866025403784439,
1.,0.866025403784439,1.))
REPRESENTATION_ITEM('')
);
#1482=(
BOUNDED_CURVE()
B_SPLINE_CURVE(2,(#242894,#242895,#242896,#242897,#242898,#242899,#242900,
#242901,#242902,#242903,#242904,#242905,#242906),.UNSPECIFIED.,.F.,.F.)
B_SPLINE_CURVE_WITH_KNOTS((3,2,2,2,2,2,3),(0.760869565217391,0.768115942028986,
0.77536231884058,0.782608695652174,0.789855072463768,0.797101449275362,
0.804347826086957),.UNSPECIFIED.)
CURVE()
GEOMETRIC_REPRESENTATION_ITEM()
RATIONAL_B_SPLINE_CURVE((1.,0.866025403784439,1.,0.866025403784439,1.,0.866025403784439,
1.,0.866025403784439,1.,0.866025403784439,1.,0.866025403784439,1.))
REPRESENTATION_ITEM('')
);
#1483=(
BOUNDED_CURVE()
B_SPLINE_CURVE(2,(#242911,#242912,#242913,#242914,#242915,#242916,#242917,
#242918,#242919,#242920,#242921,#242922,#242923),.UNSPECIFIED.,.F.,.F.)
B_SPLINE_CURVE_WITH_KNOTS((3,2,2,2,2,2,3),(0.721853444887938,0.7291448938262,
0.736436342764462,0.743727791702724,0.751019240640986,0.758310689579248,
0.76560213851751),.UNSPECIFIED.)
CURVE()
GEOMETRIC_REPRESENTATION_ITEM()
RATIONAL_B_SPLINE_CURVE((1.,0.866025403784439,1.,0.866025403784439,1.,0.866025403784439,
1.,0.866025403784439,1.,0.866025403784439,1.,0.866025403784439,1.))
REPRESENTATION_ITEM('')
);
#1484=(
BOUNDED_CURVE()
B_SPLINE_CURVE(2,(#242924,#242925,#242926,#242927,#242928,#242929,#242930,
#242931,#242932,#242933,#242934,#242935,#242936),.UNSPECIFIED.,.F.,.F.)
B_SPLINE_CURVE_WITH_KNOTS((3,2,2,2,2,2,3),(0.717391304347826,0.72463768115942,
0.731884057971015,0.739130434782609,0.746376811594203,0.753623188405797,
0.760869565217391),.UNSPECIFIED.)
CURVE()
GEOMETRIC_REPRESENTATION_ITEM()
RATIONAL_B_SPLINE_CURVE((1.,0.866025403784439,1.,0.866025403784439,1.,0.866025403784439,
1.,0.866025403784439,1.,0.866025403784439,1.,0.866025403784439,1.))
REPRESENTATION_ITEM('')
);
#1485=(
BOUNDED_CURVE()
B_SPLINE_CURVE(2,(#242941,#242942,#242943,#242944,#242945,#242946,#242947,
#242948,#242949,#242950,#242951,#242952,#242953),.UNSPECIFIED.,.F.,.F.)
B_SPLINE_CURVE_WITH_KNOTS((3,2,2,2,2,2,3),(0.678104751258366,0.685396200196628,
0.69268764913489,0.699979098073152,0.707270547011414,0.714561995949676,
0.721853444887938),.UNSPECIFIED.)
CURVE()
GEOMETRIC_REPRESENTATION_ITEM()
RATIONAL_B_SPLINE_CURVE((1.,0.866025403784439,1.,0.866025403784439,1.,0.866025403784439,
1.,0.866025403784439,1.,0.866025403784439,1.,0.866025403784439,1.))
REPRESENTATION_ITEM('')
);
#1486=(
BOUNDED_CURVE()
B_SPLINE_CURVE(2,(#242954,#242955,#242956,#242957,#242958,#242959,#242960,
#242961,#242962,#242963,#242964,#242965,#242966),.UNSPECIFIED.,.F.,.F.)
B_SPLINE_CURVE_WITH_KNOTS((3,2,2,2,2,2,3),(0.673913043478261,0.681159420289855,
0.688405797101449,0.695652173913044,0.702898550724638,0.710144927536232,
0.717391304347826),.UNSPECIFIED.)
CURVE()
GEOMETRIC_REPRESENTATION_ITEM()
RATIONAL_B_SPLINE_CURVE((1.,0.866025403784439,1.,0.866025403784439,1.,0.866025403784439,
1.,0.866025403784439,1.,0.866025403784439,1.,0.866025403784439,1.))
REPRESENTATION_ITEM('')
);
#1487=(
BOUNDED_CURVE()
B_SPLINE_CURVE(2,(#242971,#242972,#242973,#242974,#242975,#242976,#242977,
#242978,#242979,#242980,#242981,#242982,#242983),.UNSPECIFIED.,.F.,.F.)
B_SPLINE_CURVE_WITH_KNOTS((3,2,2,2,2,2,3),(0.634356057628794,0.641647506567056,
0.648938955505318,0.65623040444358,0.663521853381842,0.670813302320104,
0.678104751258366),.UNSPECIFIED.)
CURVE()
GEOMETRIC_REPRESENTATION_ITEM()
RATIONAL_B_SPLINE_CURVE((1.,0.866025403784439,1.,0.866025403784439,1.,0.866025403784439,
1.,0.866025403784439,1.,0.866025403784439,1.,0.866025403784439,1.))
REPRESENTATION_ITEM('')
);
#1488=(
BOUNDED_CURVE()
B_SPLINE_CURVE(2,(#242984,#242985,#242986,#242987,#242988,#242989,#242990,
#242991,#242992,#242993,#242994,#242995,#242996),.UNSPECIFIED.,.F.,.F.)
B_SPLINE_CURVE_WITH_KNOTS((3,2,2,2,2,2,3),(0.630434782608696,0.63768115942029,
0.644927536231884,0.652173913043478,0.659420289855073,0.666666666666667,
0.673913043478261),.UNSPECIFIED.)
CURVE()
GEOMETRIC_REPRESENTATION_ITEM()
RATIONAL_B_SPLINE_CURVE((1.,0.866025403784439,1.,0.866025403784439,1.,0.866025403784439,
1.,0.866025403784439,1.,0.866025403784439,1.,0.866025403784439,1.))
REPRESENTATION_ITEM('')
);
#1489=(
BOUNDED_CURVE()
B_SPLINE_CURVE(2,(#243001,#243002,#243003,#243004,#243005,#243006,#243007,
#243008,#243009,#243010,#243011,#243012,#243013),.UNSPECIFIED.,.F.,.F.)
B_SPLINE_CURVE_WITH_KNOTS((3,2,2,2,2,2,3),(0.590607363999222,0.597898812937484,
0.605190261875746,0.612481710814008,0.61977315975227,0.627064608690532,
0.634356057628794),.UNSPECIFIED.)
CURVE()
GEOMETRIC_REPRESENTATION_ITEM()
RATIONAL_B_SPLINE_CURVE((1.,0.866025403784439,1.,0.866025403784439,1.,0.866025403784439,
1.,0.866025403784439,1.,0.866025403784439,1.,0.866025403784439,1.))
REPRESENTATION_ITEM('')
);
#1490=(
BOUNDED_CURVE()
B_SPLINE_CURVE(2,(#243014,#243015,#243016,#243017,#243018,#243019,#243020,
#243021,#243022,#243023,#243024,#243025,#243026),.UNSPECIFIED.,.F.,.F.)
B_SPLINE_CURVE_WITH_KNOTS((3,2,2,2,2,2,3),(0.586956521739131,0.594202898550725,
0.601449275362319,0.608695652173913,0.615942028985507,0.623188405797101,
0.630434782608696),.UNSPECIFIED.)
CURVE()
GEOMETRIC_REPRESENTATION_ITEM()
RATIONAL_B_SPLINE_CURVE((1.,0.866025403784439,1.,0.866025403784439,1.,0.866025403784439,
1.,0.866025403784439,1.,0.866025403784439,1.,0.866025403784439,1.))
REPRESENTATION_ITEM('')
);
#1491=(
BOUNDED_CURVE()
B_SPLINE_CURVE(2,(#243031,#243032,#243033,#243034,#243035,#243036,#243037,
#243038,#243039,#243040,#243041,#243042,#243043),.UNSPECIFIED.,.F.,.F.)
B_SPLINE_CURVE_WITH_KNOTS((3,2,2,2,2,2,3),(0.54685867036965,0.554150119307912,
0.561441568246174,0.568733017184436,0.576024466122698,0.58331591506096,
0.590607363999222),.UNSPECIFIED.)
CURVE()
GEOMETRIC_REPRESENTATION_ITEM()
RATIONAL_B_SPLINE_CURVE((1.,0.866025403784439,1.,0.866025403784439,1.,0.866025403784439,
1.,0.866025403784439,1.,0.866025403784439,1.,0.866025403784439,1.))
REPRESENTATION_ITEM('')
);
#1492=(
BOUNDED_CURVE()
B_SPLINE_CURVE(2,(#243044,#243045,#243046,#243047,#243048,#243049,#243050,
#243051,#243052,#243053,#243054,#243055,#243056),.UNSPECIFIED.,.F.,.F.)
B_SPLINE_CURVE_WITH_KNOTS((3,2,2,2,2,2,3),(0.543478260869565,0.55072463768116,
0.557971014492754,0.565217391304348,0.572463768115942,0.579710144927536,
0.586956521739131),.UNSPECIFIED.)
CURVE()
GEOMETRIC_REPRESENTATION_ITEM()
RATIONAL_B_SPLINE_CURVE((1.,0.866025403784439,1.,0.866025403784439,1.,0.866025403784439,
1.,0.866025403784439,1.,0.866025403784439,1.,0.866025403784439,1.))
REPRESENTATION_ITEM('')
);
#1493=(
BOUNDED_CURVE()
B_SPLINE_CURVE(2,(#243061,#243062,#243063,#243064,#243065,#243066,#243067,
#243068,#243069,#243070,#243071,#243072,#243073),.UNSPECIFIED.,.F.,.F.)
B_SPLINE_CURVE_WITH_KNOTS((3,2,2,2,2,2,3),(0.503109976740078,0.51040142567834,
0.517692874616602,0.524984323554864,0.532275772493126,0.539567221431388,
0.54685867036965),.UNSPECIFIED.)
CURVE()
GEOMETRIC_REPRESENTATION_ITEM()
RATIONAL_B_SPLINE_CURVE((1.,0.866025403784439,1.,0.866025403784439,1.,0.866025403784439,
1.,0.866025403784439,1.,0.866025403784439,1.,0.866025403784439,1.))
REPRESENTATION_ITEM('')
);
#1494=(
BOUNDED_CURVE()
B_SPLINE_CURVE(2,(#243074,#243075,#243076,#243077,#243078,#243079,#243080,
#243081,#243082,#243083,#243084,#243085,#243086),.UNSPECIFIED.,.F.,.F.)
B_SPLINE_CURVE_WITH_KNOTS((3,2,2,2,2,2,3),(0.5,0.507246376811594,0.514492753623189,
0.521739130434783,0.528985507246377,0.536231884057971,0.543478260869565),
 .UNSPECIFIED.)
CURVE()
GEOMETRIC_REPRESENTATION_ITEM()
RATIONAL_B_SPLINE_CURVE((1.,0.866025403784439,1.,0.866025403784439,1.,0.866025403784439,
1.,0.866025403784439,1.,0.866025403784439,1.,0.866025403784439,1.))
REPRESENTATION_ITEM('')
);
#1495=(
BOUNDED_CURVE()
B_SPLINE_CURVE(2,(#243091,#243092,#243093,#243094,#243095,#243096,#243097,
#243098,#243099,#243100,#243101,#243102,#243103),.UNSPECIFIED.,.F.,.F.)
B_SPLINE_CURVE_WITH_KNOTS((3,2,2,2,2,2,3),(0.459361283110506,0.466652732048768,
0.47394418098703,0.481235629925292,0.488527078863554,0.495818527801816,
0.503109976740078),.UNSPECIFIED.)
CURVE()
GEOMETRIC_REPRESENTATION_ITEM()
RATIONAL_B_SPLINE_CURVE((1.,0.866025403784439,1.,0.866025403784439,1.,0.866025403784439,
1.,0.866025403784439,1.,0.866025403784439,1.,0.866025403784439,1.))
REPRESENTATION_ITEM('')
);
#1496=(
BOUNDED_CURVE()
B_SPLINE_CURVE(2,(#243104,#243105,#243106,#243107,#243108,#243109,#243110,
#243111,#243112,#243113,#243114,#243115,#243116),.UNSPECIFIED.,.F.,.F.)
B_SPLINE_CURVE_WITH_KNOTS((3,2,2,2,2,2,3),(0.456521739130435,0.463768115942029,
0.471014492753623,0.478260869565218,0.485507246376812,0.492753623188406,
0.5),.UNSPECIFIED.)
CURVE()
GEOMETRIC_REPRESENTATION_ITEM()
RATIONAL_B_SPLINE_CURVE((1.,0.866025403784439,1.,0.866025403784439,1.,0.866025403784439,
1.,0.866025403784439,1.,0.866025403784439,1.,0.866025403784439,1.))
REPRESENTATION_ITEM('')
);
#1497=(
BOUNDED_CURVE()
B_SPLINE_CURVE(2,(#243121,#243122,#243123,#243124,#243125,#243126,#243127,
#243128,#243129,#243130,#243131,#243132,#243133),.UNSPECIFIED.,.F.,.F.)
B_SPLINE_CURVE_WITH_KNOTS((3,2,2,2,2,2,3),(0.415612589480934,0.422904038419196,
0.430195487357458,0.43748693629572,0.444778385233982,0.452069834172244,
0.459361283110506),.UNSPECIFIED.)
CURVE()
GEOMETRIC_REPRESENTATION_ITEM()
RATIONAL_B_SPLINE_CURVE((1.,0.866025403784439,1.,0.866025403784439,1.,0.866025403784439,
1.,0.866025403784439,1.,0.866025403784439,1.,0.866025403784439,1.))
REPRESENTATION_ITEM('')
);
#1498=(
BOUNDED_CURVE()
B_SPLINE_CURVE(2,(#243134,#243135,#243136,#243137,#243138,#243139,#243140,
#243141,#243142,#243143,#243144,#243145,#243146),.UNSPECIFIED.,.F.,.F.)
B_SPLINE_CURVE_WITH_KNOTS((3,2,2,2,2,2,3),(0.41304347826087,0.420289855072464,
0.427536231884058,0.434782608695652,0.442028985507247,0.449275362318841,
0.456521739130435),.UNSPECIFIED.)
CURVE()
GEOMETRIC_REPRESENTATION_ITEM()
RATIONAL_B_SPLINE_CURVE((1.,0.866025403784439,1.,0.866025403784439,1.,0.866025403784439,
1.,0.866025403784439,1.,0.866025403784439,1.,0.866025403784439,1.))
REPRESENTATION_ITEM('')
);
#1499=(
BOUNDED_CURVE()
B_SPLINE_CURVE(2,(#243151,#243152,#243153,#243154,#243155,#243156,#243157,
#243158,#243159,#243160,#243161,#243162,#243163),.UNSPECIFIED.,.F.,.F.)
B_SPLINE_CURVE_WITH_KNOTS((3,2,2,2,2,2,3),(0.371863895851362,0.379155344789624,
0.386446793727886,0.393738242666148,0.40102969160441,0.408321140542672,
0.415612589480934),.UNSPECIFIED.)
CURVE()
GEOMETRIC_REPRESENTATION_ITEM()
RATIONAL_B_SPLINE_CURVE((1.,0.866025403784439,1.,0.866025403784439,1.,0.866025403784439,
1.,0.866025403784439,1.,0.866025403784439,1.,0.866025403784439,1.))
REPRESENTATION_ITEM('')
);
#1500=(
BOUNDED_CURVE()
B_SPLINE_CURVE(2,(#243164,#243165,#243166,#243167,#243168,#243169,#243170,
#243171,#243172,#243173,#243174,#243175,#243176),.UNSPECIFIED.,.F.,.F.)
B_SPLINE_CURVE_WITH_KNOTS((3,2,2,2,2,2,3),(0.369565217391304,0.376811594202899,
0.384057971014493,0.391304347826087,0.398550724637682,0.405797101449275,
0.41304347826087),.UNSPECIFIED.)
CURVE()
GEOMETRIC_REPRESENTATION_ITEM()
RATIONAL_B_SPLINE_CURVE((1.,0.866025403784439,1.,0.866025403784439,1.,0.866025403784439,
1.,0.866025403784439,1.,0.866025403784439,1.,0.866025403784439,1.))
REPRESENTATION_ITEM('')
);
#1501=(
BOUNDED_CURVE()
B_SPLINE_CURVE(2,(#243181,#243182,#243183,#243184,#243185,#243186,#243187,
#243188,#243189,#243190,#243191,#243192,#243193),.UNSPECIFIED.,.F.,.F.)
B_SPLINE_CURVE_WITH_KNOTS((3,2,2,2,2,2,3),(0.32811520222179,0.335406651160052,
0.342698100098314,0.349989549036576,0.357280997974838,0.3645724469131,0.371863895851362),
 .UNSPECIFIED.)
CURVE()
GEOMETRIC_REPRESENTATION_ITEM()
RATIONAL_B_SPLINE_CURVE((1.,0.866025403784439,1.,0.866025403784439,1.,0.866025403784439,
1.,0.866025403784439,1.,0.866025403784439,1.,0.866025403784439,1.))
REPRESENTATION_ITEM('')
);
#1502=(
BOUNDED_CURVE()
B_SPLINE_CURVE(2,(#243194,#243195,#243196,#243197,#243198,#243199,#243200,
#243201,#243202,#243203,#243204,#243205,#243206),.UNSPECIFIED.,.F.,.F.)
B_SPLINE_CURVE_WITH_KNOTS((3,2,2,2,2,2,3),(0.326086956521739,0.333333333333334,
0.340579710144927,0.347826086956522,0.355072463768116,0.36231884057971,
0.369565217391304),.UNSPECIFIED.)
CURVE()
GEOMETRIC_REPRESENTATION_ITEM()
RATIONAL_B_SPLINE_CURVE((1.,0.866025403784439,1.,0.866025403784439,1.,0.866025403784439,
1.,0.866025403784439,1.,0.866025403784439,1.,0.866025403784439,1.))
REPRESENTATION_ITEM('')
);
#1503=(
BOUNDED_CURVE()
B_SPLINE_CURVE(2,(#243211,#243212,#243213,#243214,#243215,#243216,#243217,
#243218,#243219,#243220,#243221,#243222,#243223),.UNSPECIFIED.,.F.,.F.)
B_SPLINE_CURVE_WITH_KNOTS((3,2,2,2,2,2,3),(0.284366508592218,0.29165795753048,
0.298949406468742,0.306240855407004,0.313532304345266,0.320823753283528,
0.32811520222179),.UNSPECIFIED.)
CURVE()
GEOMETRIC_REPRESENTATION_ITEM()
RATIONAL_B_SPLINE_CURVE((1.,0.866025403784439,1.,0.866025403784439,1.,0.866025403784439,
1.,0.866025403784439,1.,0.866025403784439,1.,0.866025403784439,1.))
REPRESENTATION_ITEM('')
);
#1504=(
BOUNDED_CURVE()
B_SPLINE_CURVE(2,(#243224,#243225,#243226,#243227,#243228,#243229,#243230,
#243231,#243232,#243233,#243234,#243235,#243236),.UNSPECIFIED.,.F.,.F.)
B_SPLINE_CURVE_WITH_KNOTS((3,2,2,2,2,2,3),(0.282608695652174,0.289855072463769,
0.297101449275363,0.304347826086956,0.311594202898551,0.318840579710145,
0.326086956521739),.UNSPECIFIED.)
CURVE()
GEOMETRIC_REPRESENTATION_ITEM()
RATIONAL_B_SPLINE_CURVE((1.,0.866025403784439,1.,0.866025403784439,1.,0.866025403784439,
1.,0.866025403784439,1.,0.866025403784439,1.,0.866025403784439,1.))
REPRESENTATION_ITEM('')
);
#1505=(
BOUNDED_CURVE()
B_SPLINE_CURVE(2,(#243241,#243242,#243243,#243244,#243245,#243246,#243247,
#243248,#243249,#243250,#243251,#243252,#243253),.UNSPECIFIED.,.F.,.F.)
B_SPLINE_CURVE_WITH_KNOTS((3,2,2,2,2,2,3),(0.240617814962646,0.247909263900908,
0.25520071283917,0.262492161777432,0.269783610715694,0.277075059653956,
0.284366508592218),.UNSPECIFIED.)
CURVE()
GEOMETRIC_REPRESENTATION_ITEM()
RATIONAL_B_SPLINE_CURVE((1.,0.866025403784439,1.,0.866025403784439,1.,0.866025403784439,
1.,0.866025403784439,1.,0.866025403784439,1.,0.866025403784439,1.))
REPRESENTATION_ITEM('')
);
#1506=(
BOUNDED_CURVE()
B_SPLINE_CURVE(2,(#243254,#243255,#243256,#243257,#243258,#243259,#243260,
#243261,#243262,#243263,#243264,#243265,#243266),.UNSPECIFIED.,.F.,.F.)
B_SPLINE_CURVE_WITH_KNOTS((3,2,2,2,2,2,3),(0.239130434782609,0.246376811594203,
0.253623188405797,0.260869565217392,0.268115942028985,0.27536231884058,
0.282608695652174),.UNSPECIFIED.)
CURVE()
GEOMETRIC_REPRESENTATION_ITEM()
RATIONAL_B_SPLINE_CURVE((1.,0.866025403784439,1.,0.866025403784439,1.,0.866025403784439,
1.,0.866025403784439,1.,0.866025403784439,1.,0.866025403784439,1.))
REPRESENTATION_ITEM('')
);
#1507=(
BOUNDED_CURVE()
B_SPLINE_CURVE(2,(#243271,#243272,#243273,#243274,#243275,#243276,#243277,
#243278,#243279,#243280,#243281,#243282,#243283),.UNSPECIFIED.,.F.,.F.)
B_SPLINE_CURVE_WITH_KNOTS((3,2,2,2,2,2,3),(0.196869121333074,0.204160570271336,
0.211452019209598,0.21874346814786,0.226034917086122,0.233326366024384,
0.240617814962646),.UNSPECIFIED.)
CURVE()
GEOMETRIC_REPRESENTATION_ITEM()
RATIONAL_B_SPLINE_CURVE((1.,0.866025403784439,1.,0.866025403784439,1.,0.866025403784439,
1.,0.866025403784439,1.,0.866025403784439,1.,0.866025403784439,1.))
REPRESENTATION_ITEM('')
);
#1508=(
BOUNDED_CURVE()
B_SPLINE_CURVE(2,(#243284,#243285,#243286,#243287,#243288,#243289,#243290,
#243291,#243292,#243293,#243294,#243295,#243296),.UNSPECIFIED.,.F.,.F.)
B_SPLINE_CURVE_WITH_KNOTS((3,2,2,2,2,2,3),(0.195652173913044,0.202898550724638,
0.210144927536232,0.217391304347826,0.224637681159421,0.231884057971015,
0.239130434782609),.UNSPECIFIED.)
CURVE()
GEOMETRIC_REPRESENTATION_ITEM()
RATIONAL_B_SPLINE_CURVE((1.,0.866025403784439,1.,0.866025403784439,1.,0.866025403784439,
1.,0.866025403784439,1.,0.866025403784439,1.,0.866025403784439,1.))
REPRESENTATION_ITEM('')
);
#1509=(
BOUNDED_CURVE()
B_SPLINE_CURVE(2,(#243301,#243302,#243303,#243304,#243305,#243306,#243307,
#243308,#243309,#243310,#243311,#243312,#243313),.UNSPECIFIED.,.F.,.F.)
B_SPLINE_CURVE_WITH_KNOTS((3,2,2,2,2,2,3),(0.153120427703502,0.160411876641764,
0.167703325580026,0.174994774518288,0.18228622345655,0.189577672394812,
0.196869121333074),.UNSPECIFIED.)
CURVE()
GEOMETRIC_REPRESENTATION_ITEM()
RATIONAL_B_SPLINE_CURVE((1.,0.866025403784439,1.,0.866025403784439,1.,0.866025403784439,
1.,0.866025403784439,1.,0.866025403784439,1.,0.866025403784439,1.))
REPRESENTATION_ITEM('')
);
#1510=(
BOUNDED_CURVE()
B_SPLINE_CURVE(2,(#243314,#243315,#243316,#243317,#243318,#243319,#243320,
#243321,#243322,#243323,#243324,#243325,#243326),.UNSPECIFIED.,.F.,.F.)
B_SPLINE_CURVE_WITH_KNOTS((3,2,2,2,2,2,3),(0.152173913043478,0.159420289855073,
0.166666666666667,0.173913043478261,0.181159420289855,0.18840579710145,
0.195652173913044),.UNSPECIFIED.)
CURVE()
GEOMETRIC_REPRESENTATION_ITEM()
RATIONAL_B_SPLINE_CURVE((1.,0.866025403784439,1.,0.866025403784439,1.,0.866025403784439,
1.,0.866025403784439,1.,0.866025403784439,1.,0.866025403784439,1.))
REPRESENTATION_ITEM('')
);
#1511=(
BOUNDED_CURVE()
B_SPLINE_CURVE(2,(#243331,#243332,#243333,#243334,#243335,#243336,#243337,
#243338,#243339,#243340,#243341,#243342,#243343),.UNSPECIFIED.,.F.,.F.)
B_SPLINE_CURVE_WITH_KNOTS((3,2,2,2,2,2,3),(0.10937173407393,0.116663183012192,
0.123954631950454,0.131246080888716,0.138537529826978,0.14582897876524,
0.153120427703502),.UNSPECIFIED.)
CURVE()
GEOMETRIC_REPRESENTATION_ITEM()
RATIONAL_B_SPLINE_CURVE((1.,0.866025403784439,1.,0.866025403784439,1.,0.866025403784439,
1.,0.866025403784439,1.,0.866025403784439,1.,0.866025403784439,1.))
REPRESENTATION_ITEM('')
);
#1512=(
BOUNDED_CURVE()
B_SPLINE_CURVE(2,(#243344,#243345,#243346,#243347,#243348,#243349,#243350,
#243351,#243352,#243353,#243354,#243355,#243356),.UNSPECIFIED.,.F.,.F.)
B_SPLINE_CURVE_WITH_KNOTS((3,2,2,2,2,2,3),(0.108695652173913,0.115942028985507,
0.123188405797102,0.130434782608696,0.13768115942029,0.144927536231884,
0.152173913043478),.UNSPECIFIED.)
CURVE()
GEOMETRIC_REPRESENTATION_ITEM()
RATIONAL_B_SPLINE_CURVE((1.,0.866025403784439,1.,0.866025403784439,1.,0.866025403784439,
1.,0.866025403784439,1.,0.866025403784439,1.,0.866025403784439,1.))
REPRESENTATION_ITEM('')
);
#1513=(
BOUNDED_CURVE()
B_SPLINE_CURVE(2,(#243361,#243362,#243363,#243364,#243365,#243366,#243367,
#243368,#243369,#243370,#243371,#243372,#243373),.UNSPECIFIED.,.F.,.F.)
B_SPLINE_CURVE_WITH_KNOTS((3,2,2,2,2,2,3),(0.065623040444358,0.07291448938262,
0.080205938320882,0.087497387259144,0.094788836197406,0.102080285135668,
0.10937173407393),.UNSPECIFIED.)
CURVE()
GEOMETRIC_REPRESENTATION_ITEM()
RATIONAL_B_SPLINE_CURVE((1.,0.866025403784439,1.,0.866025403784439,1.,0.866025403784439,
1.,0.866025403784439,1.,0.866025403784439,1.,0.866025403784439,1.))
REPRESENTATION_ITEM('')
);
#1514=(
BOUNDED_CURVE()
B_SPLINE_CURVE(2,(#243374,#243375,#243376,#243377,#243378,#243379,#243380,
#243381,#243382,#243383,#243384,#243385,#243386),.UNSPECIFIED.,.F.,.F.)
B_SPLINE_CURVE_WITH_KNOTS((3,2,2,2,2,2,3),(0.065217391304348,0.0724637681159422,
0.0797101449275364,0.0869565217391306,0.0942028985507248,0.101449275362319,
0.108695652173913),.UNSPECIFIED.)
CURVE()
GEOMETRIC_REPRESENTATION_ITEM()
RATIONAL_B_SPLINE_CURVE((1.,0.866025403784439,1.,0.866025403784439,1.,0.866025403784439,
1.,0.866025403784439,1.,0.866025403784439,1.,0.866025403784439,1.))
REPRESENTATION_ITEM('')
);
#1515=(
BOUNDED_CURVE()
B_SPLINE_CURVE(2,(#243393,#243394,#243395,#243396,#243397),
 .UNSPECIFIED.,.F.,.F.)
B_SPLINE_CURVE_WITH_KNOTS((3,2,3),(0.0118893770663285,0.014582897876524,
0.021874346814786),.UNSPECIFIED.)
CURVE()
GEOMETRIC_REPRESENTATION_ITEM()
RATIONAL_B_SPLINE_CURVE((0.937582367981142,0.950508689562301,1.,0.866025403784439,
1.))
REPRESENTATION_ITEM('')
);
#1516=(
BOUNDED_CURVE()
B_SPLINE_CURVE(2,(#243949,#243950,#243951),.UNSPECIFIED.,.F.,.F.)
B_SPLINE_CURVE_WITH_KNOTS((3,3),(0.305379135947461,0.795630657118022),
 .UNSPECIFIED.)
CURVE()
GEOMETRIC_REPRESENTATION_ITEM()
RATIONAL_B_SPLINE_CURVE((1.45513171305057,1.68024137247218,1.45513171305058))
REPRESENTATION_ITEM('')
);
#1517=(
BOUNDED_CURVE()
B_SPLINE_CURVE(2,(#243954,#243955,#243956),.UNSPECIFIED.,.F.,.F.)
B_SPLINE_CURVE_WITH_KNOTS((3,3),(-1.92744743716646,-0.984663180908388),
 .UNSPECIFIED.)
CURVE()
GEOMETRIC_REPRESENTATION_ITEM()
RATIONAL_B_SPLINE_CURVE((2.94675698395174,3.40262187584188,2.94675698395181))
REPRESENTATION_ITEM('')
);
#1518=(
BOUNDED_CURVE()
B_SPLINE_CURVE(2,(#243961,#243962,#243963),.UNSPECIFIED.,.F.,.F.)
B_SPLINE_CURVE_WITH_KNOTS((3,3),(0.313853530401117,0.810060947929668),
 .UNSPECIFIED.)
CURVE()
GEOMETRIC_REPRESENTATION_ITEM()
RATIONAL_B_SPLINE_CURVE((1.46945873729773,1.69678479508373,1.46945873729773))
REPRESENTATION_ITEM('')
);
#1519=(
BOUNDED_CURVE()
B_SPLINE_CURVE(2,(#243964,#243965,#243966),.UNSPECIFIED.,.F.,.F.)
B_SPLINE_CURVE_WITH_KNOTS((3,3),(-1.9274474371665,-0.98466318090834),
 .UNSPECIFIED.)
CURVE()
GEOMETRIC_REPRESENTATION_ITEM()
RATIONAL_B_SPLINE_CURVE((2.94675698395173,3.40262187584197,2.94675698395179))
REPRESENTATION_ITEM('')
);
#1520=(
BOUNDED_CURVE()
B_SPLINE_CURVE(2,(#243971,#243972,#243973),.UNSPECIFIED.,.F.,.F.)
B_SPLINE_CURVE_WITH_KNOTS((3,3),(0.337455036462552,0.850307797466422),
 .UNSPECIFIED.)
CURVE()
GEOMETRIC_REPRESENTATION_ITEM()
RATIONAL_B_SPLINE_CURVE((1.5095308677303,1.74305610566815,1.5095308677303))
REPRESENTATION_ITEM('')
);
#1521=(
BOUNDED_CURVE()
B_SPLINE_CURVE(2,(#243974,#243975,#243976),.UNSPECIFIED.,.F.,.F.)
B_SPLINE_CURVE_WITH_KNOTS((3,3),(-1.75023669514897,-0.881692746819963),
 .UNSPECIFIED.)
CURVE()
GEOMETRIC_REPRESENTATION_ITEM()
RATIONAL_B_SPLINE_CURVE((2.72423919983985,3.14568047072895,2.72423919983986))
REPRESENTATION_ITEM('')
);
#1522=(
BOUNDED_CURVE()
B_SPLINE_CURVE(2,(#243981,#243982,#243983),.UNSPECIFIED.,.F.,.F.)
B_SPLINE_CURVE_WITH_KNOTS((3,3),(0.296747814710797,0.78094561467123),
 .UNSPECIFIED.)
CURVE()
GEOMETRIC_REPRESENTATION_ITEM()
RATIONAL_B_SPLINE_CURVE((1.44057579043547,1.66343364079194,1.44057579043547))
REPRESENTATION_ITEM('')
);
#1523=(
BOUNDED_CURVE()
B_SPLINE_CURVE(2,(#243984,#243985,#243986),.UNSPECIFIED.,.F.,.F.)
B_SPLINE_CURVE_WITH_KNOTS((3,3),(-1.65890795248092,-0.828567311293231),
 .UNSPECIFIED.)
CURVE()
GEOMETRIC_REPRESENTATION_ITEM()
RATIONAL_B_SPLINE_CURVE((2.60974794608846,3.01347735838248,2.60974794608845))
REPRESENTATION_ITEM('')
);
#1524=(
BOUNDED_CURVE()
B_SPLINE_CURVE(2,(#243991,#243992,#243993),.UNSPECIFIED.,.F.,.F.)
B_SPLINE_CURVE_WITH_KNOTS((3,3),(0.327461385305039,0.833256095326246),
 .UNSPECIFIED.)
CURVE()
GEOMETRIC_REPRESENTATION_ITEM()
RATIONAL_B_SPLINE_CURVE((1.49253377429497,1.72342955272753,1.49253377429496))
REPRESENTATION_ITEM('')
);
#1525=(
BOUNDED_CURVE()
B_SPLINE_CURVE(2,(#243994,#243995,#243996),.UNSPECIFIED.,.F.,.F.)
B_SPLINE_CURVE_WITH_KNOTS((3,3),(-1.63785199431076,-0.816312569741005),
 .UNSPECIFIED.)
CURVE()
GEOMETRIC_REPRESENTATION_ITEM()
RATIONAL_B_SPLINE_CURVE((2.58337319633923,2.9830224206474,2.58337319633922))
REPRESENTATION_ITEM('')
);
#1526=(
BOUNDED_CURVE()
B_SPLINE_CURVE(2,(#243998,#243999,#244000),.UNSPECIFIED.,.F.,.F.)
B_SPLINE_CURVE_WITH_KNOTS((3,3),(0.336410883504879,0.848525565411443),
 .UNSPECIFIED.)
CURVE()
GEOMETRIC_REPRESENTATION_ITEM()
RATIONAL_B_SPLINE_CURVE((1.50775306979144,1.74100328143105,1.50775306979145))
REPRESENTATION_ITEM('')
);
#1527=(
BOUNDED_CURVE()
B_SPLINE_CURVE(2,(#244001,#244002,#244003),.UNSPECIFIED.,.F.,.F.)
B_SPLINE_CURVE_WITH_KNOTS((3,3),(-1.93645569281037,-0.989894173396402),
 .UNSPECIFIED.)
CURVE()
GEOMETRIC_REPRESENTATION_ITEM()
RATIONAL_B_SPLINE_CURVE((2.9580792886783,3.41569574720537,2.9580792886783))
REPRESENTATION_ITEM('')
);
#1528=(
BOUNDED_CURVE()
B_SPLINE_CURVE(2,(#247964,#247965,#247966),.UNSPECIFIED.,.F.,.F.)
B_SPLINE_CURVE_WITH_KNOTS((3,3),(-1.19817642475198,-1.13405670867392),
 .UNSPECIFIED.)
CURVE()
GEOMETRIC_REPRESENTATION_ITEM()
RATIONAL_B_SPLINE_CURVE((1.00675929761165,1.00683091269735,1.00687550567357))
REPRESENTATION_ITEM('')
);
#1529=(
BOUNDED_CURVE()
B_SPLINE_CURVE(3,(#248095,#248096,#248097,#248098,#248099,#248100),
 .UNSPECIFIED.,.F.,.F.)
B_SPLINE_CURVE_WITH_KNOTS((4,2,4),(0.,0.5,1.),.UNSPECIFIED.)
CURVE()
GEOMETRIC_REPRESENTATION_ITEM()
RATIONAL_B_SPLINE_CURVE((0.99999997576651,0.999999976303432,0.999999976712256,
0.999999977274856,0.999999977413013,0.999999977414642))
REPRESENTATION_ITEM('')
);
#1530=(
BOUNDED_CURVE()
B_SPLINE_CURVE(3,(#248243,#248244,#248245,#248246,#248247,#248248),
 .UNSPECIFIED.,.F.,.F.)
B_SPLINE_CURVE_WITH_KNOTS((4,2,4),(0.,0.5,1.),.UNSPECIFIED.)
CURVE()
GEOMETRIC_REPRESENTATION_ITEM()
RATIONAL_B_SPLINE_CURVE((0.999999975766518,0.999999976303441,0.999999976712265,
0.999999977274864,0.999999977413021,0.99999997741465))
REPRESENTATION_ITEM('')
);
#1531=(
BOUNDED_CURVE()
B_SPLINE_CURVE(2,(#252039,#252040,#252041,#252042,#252043,#252044,#252045,
#252046,#252047,#252048,#252049,#252050,#252051),.UNSPECIFIED.,.F.,.F.)
B_SPLINE_CURVE_WITH_KNOTS((3,2,2,2,2,2,3),(0.021874346814786,0.029165795753048,
0.03645724469131,0.043748693629572,0.051040142567834,0.058331591506096,
0.065623040444358),.UNSPECIFIED.)
CURVE()
GEOMETRIC_REPRESENTATION_ITEM()
RATIONAL_B_SPLINE_CURVE((1.,0.866025403784439,1.,0.866025403784439,1.,0.866025403784439,
1.,0.866025403784439,1.,0.866025403784439,1.,0.866025403784439,1.))
REPRESENTATION_ITEM('')
);
#1532=(
BOUNDED_CURVE()
B_SPLINE_CURVE(2,(#252052,#252053,#252054,#252055,#252056,#252057,#252058,
#252059,#252060,#252061,#252062,#252063,#252064),.UNSPECIFIED.,.F.,.F.)
B_SPLINE_CURVE_WITH_KNOTS((3,2,2,2,2,2,3),(0.0217391304347828,0.028985507246377,
0.0362318840579712,0.0434782608695654,0.0507246376811596,0.0579710144927538,
0.065217391304348),.UNSPECIFIED.)
CURVE()
GEOMETRIC_REPRESENTATION_ITEM()
RATIONAL_B_SPLINE_CURVE((1.,0.866025403784442,1.,0.866025403784439,1.,0.866025403784439,
1.,0.866025403784439,1.,0.866025403784439,1.,0.866025403784439,1.))
REPRESENTATION_ITEM('')
);
#1533=(
BOUNDED_CURVE()
B_SPLINE_CURVE(2,(#256140,#256141,#256142,#256143,#256144,#256145,#256146,
#256147,#256148,#256149,#256150,#256151,#256152),.UNSPECIFIED.,.F.,.F.)
B_SPLINE_CURVE_WITH_KNOTS((3,2,2,2,2,2,3),(0.021874346814786,0.029165795753048,
0.03645724469131,0.043748693629572,0.051040142567834,0.058331591506096,
0.065623040444358),.UNSPECIFIED.)
CURVE()
GEOMETRIC_REPRESENTATION_ITEM()
RATIONAL_B_SPLINE_CURVE((1.,0.866025403784439,1.,0.866025403784439,1.,0.866025403784439,
1.,0.866025403784439,1.,0.866025403784439,1.,0.866025403784439,1.))
REPRESENTATION_ITEM('')
);
#1534=(
BOUNDED_CURVE()
B_SPLINE_CURVE(2,(#256153,#256154,#256155,#256156,#256157,#256158,#256159,
#256160,#256161,#256162,#256163,#256164,#256165),.UNSPECIFIED.,.F.,.F.)
B_SPLINE_CURVE_WITH_KNOTS((3,2,2,2,2,2,3),(0.0217391304347828,0.028985507246377,
0.0362318840579712,0.0434782608695654,0.0507246376811596,0.0579710144927538,
0.065217391304348),.UNSPECIFIED.)
CURVE()
GEOMETRIC_REPRESENTATION_ITEM()
RATIONAL_B_SPLINE_CURVE((1.,0.866025403784442,1.,0.866025403784439,1.,0.866025403784439,
1.,0.866025403784439,1.,0.866025403784439,1.,0.866025403784439,1.))
REPRESENTATION_ITEM('')
);
#1535=(
BOUNDED_CURVE()
B_SPLINE_CURVE(2,(#260278,#260279,#260280,#260281,#260282,#260283,#260284,
#260285,#260286,#260287,#260288,#260289,#260290),.UNSPECIFIED.,.F.,.F.)
B_SPLINE_CURVE_WITH_KNOTS((3,2,2,2,2,2,3),(0.021874346814786,0.029165795753048,
0.03645724469131,0.043748693629572,0.051040142567834,0.058331591506096,
0.065623040444358),.UNSPECIFIED.)
CURVE()
GEOMETRIC_REPRESENTATION_ITEM()
RATIONAL_B_SPLINE_CURVE((1.,0.866025403784439,1.,0.866025403784439,1.,0.866025403784439,
1.,0.866025403784439,1.,0.866025403784439,1.,0.866025403784439,1.))
REPRESENTATION_ITEM('')
);
#1536=(
BOUNDED_CURVE()
B_SPLINE_CURVE(2,(#260291,#260292,#260293,#260294,#260295,#260296,#260297,
#260298,#260299,#260300,#260301,#260302,#260303),.UNSPECIFIED.,.F.,.F.)
B_SPLINE_CURVE_WITH_KNOTS((3,2,2,2,2,2,3),(0.0217391304347828,0.028985507246377,
0.0362318840579711,0.0434782608695653,0.0507246376811596,0.0579710144927538,
0.065217391304348),.UNSPECIFIED.)
CURVE()
GEOMETRIC_REPRESENTATION_ITEM()
RATIONAL_B_SPLINE_CURVE((1.,0.866025403784441,1.,0.866025403784439,1.,0.866025403784439,
1.,0.866025403784439,1.,0.866025403784439,1.,0.866025403784439,1.))
REPRESENTATION_ITEM('')
);
#1537=(
BOUNDED_CURVE()
B_SPLINE_CURVE(2,(#264429,#264430,#264431,#264432,#264433,#264434,#264435,
#264436,#264437,#264438,#264439,#264440,#264441),.UNSPECIFIED.,.F.,.F.)
B_SPLINE_CURVE_WITH_KNOTS((3,2,2,2,2,2,3),(0.021874346814786,0.029165795753048,
0.03645724469131,0.043748693629572,0.051040142567834,0.058331591506096,
0.065623040444358),.UNSPECIFIED.)
CURVE()
GEOMETRIC_REPRESENTATION_ITEM()
RATIONAL_B_SPLINE_CURVE((1.,0.866025403784439,1.,0.866025403784439,1.,0.866025403784439,
1.,0.866025403784439,1.,0.866025403784439,1.,0.866025403784439,1.))
REPRESENTATION_ITEM('')
);
#1538=(
BOUNDED_CURVE()
B_SPLINE_CURVE(2,(#264442,#264443,#264444,#264445,#264446,#264447,#264448,
#264449,#264450,#264451,#264452,#264453,#264454),.UNSPECIFIED.,.F.,.F.)
B_SPLINE_CURVE_WITH_KNOTS((3,2,2,2,2,2,3),(0.0217391304347828,0.028985507246377,
0.0362318840579712,0.0434782608695654,0.0507246376811596,0.0579710144927538,
0.065217391304348),.UNSPECIFIED.)
CURVE()
GEOMETRIC_REPRESENTATION_ITEM()
RATIONAL_B_SPLINE_CURVE((1.,0.866025403784442,1.,0.866025403784439,1.,0.866025403784439,
1.,0.866025403784439,1.,0.866025403784439,1.,0.866025403784439,1.))
REPRESENTATION_ITEM('')
);
#1771=ELLIPSE('',#94133,0.937885965405836,0.86675406492929);
#1772=ELLIPSE('',#94142,1.46972525436131,1.19984572304843);
#1773=ELLIPSE('',#94157,1.04665693996376,1.00906146746166);
#1774=ELLIPSE('',#94159,1.37504974877692,1.13183911208508);
#1775=ELLIPSE('',#94174,1.14567646024684,1.02014379851209);
#1776=ELLIPSE('',#94176,1.25196838933939,1.02863480032067);
#1777=ELLIPSE('',#94203,1.29935811091585,1.07153805568279);
#1778=ELLIPSE('',#94205,1.09610411986708,1.01541339803192);
#1779=ELLIPSE('',#94218,1.42337813156552,1.16710237101683);
#1780=ELLIPSE('',#94264,0.908597175301873,0.820141976513812);
#1781=ELLIPSE('',#94283,1.06703722879645,0.943876034909289);
#1782=ELLIPSE('',#94284,1.14336482056826,1.01842172929862);
#1783=ELLIPSE('',#94297,1.3737241452667,1.13065652311915);
#1784=ELLIPSE('',#94298,1.04669178748828,1.00873018684506);
#1785=ELLIPSE('',#94310,1.46903943622045,1.1992965413372);
#1786=ELLIPSE('',#94324,1.47061008469222,1.20045580538409);
#1787=ELLIPSE('',#94336,1.04558723045975,1.0088761098663);
#1788=ELLIPSE('',#94337,1.37669607957637,1.13307292819281);
#1789=ELLIPSE('',#94350,1.14413769841436,1.02008736650461);
#1790=ELLIPSE('',#94351,1.25359260924378,1.03019400968285);
#1791=ELLIPSE('',#94415,0.455015549306865,0.414682781673397);
#1792=ELLIPSE('',#94434,0.470322150347728,0.437408695773927);
#1793=ELLIPSE('',#94470,2.23591051322783,1.82312386243465);
#1794=ELLIPSE('',#94471,1.49234872661747,1.21529881462133);
#1795=ELLIPSE('',#94499,0.796819240888165,0.626540578311605);
#1796=ELLIPSE('',#94501,0.817675517046813,0.657962952441664);
#1797=ELLIPSE('',#94642,1.14142675533965,1.0183769149773);
#1798=ELLIPSE('',#94644,1.25155489583491,1.02861695892357);
#1799=ELLIPSE('',#94658,1.04546867609948,1.00852772291651);
#1800=ELLIPSE('',#94660,1.37581189656266,1.13221924904961);
#1801=ELLIPSE('',#94675,1.47003669918833,1.19998639117251);
#1802=ELLIPSE('',#94690,2.24478172556828,1.82751302619863);
#1803=ELLIPSE('',#94692,6.74379813677969,5.49640701624088);
#1804=ELLIPSE('',#94693,6.74471830677379,5.49677536022385);
#1805=ELLIPSE('',#94694,2.24478717905741,1.82751618959032);
#1806=ELLIPSE('',#94697,2.19060648404767,1.80054773483043);
#1807=ELLIPSE('',#94699,2.19081358780445,1.80064181344396);
#1808=ELLIPSE('',#94703,1.43187143532244,1.37961189378668);
#1809=ELLIPSE('',#94705,2.14457779788183,1.77729531483311);
#1810=ELLIPSE('',#94708,1.45260602254477,1.42951177173056);
#1811=ELLIPSE('',#94712,1.45276135118972,1.42923490730472);
#1812=ELLIPSE('',#94719,1.48146874195372,1.44883544422854);
#1813=ELLIPSE('',#94723,1.48049428484162,1.44867655321776);
#1814=ELLIPSE('',#94726,1.59183749500213,1.48024250564481);
#1815=ELLIPSE('',#94730,1.59230054944377,1.48054973563609);
#1816=ELLIPSE('',#94736,1.34503947636183,1.23514518656413);
#1817=ELLIPSE('',#94748,1.52235692825161,1.4619644584823);
#1818=ELLIPSE('',#94753,1.44688208751335,1.42026986218873);
#1819=ELLIPSE('',#94761,1.43683810397249,1.39553674726878);
#1820=ELLIPSE('',#94764,2.21081023708958,1.81065351492543);
#1821=ELLIPSE('',#94783,1.4677889282425,1.40956355520622);
#1822=ELLIPSE('',#94784,1.59354891790328,1.48067275522773);
#1823=ELLIPSE('',#94787,1.48261995869119,1.44952139994979);
#1824=ELLIPSE('',#94792,1.48262920837846,1.44930064696724);
#1825=ELLIPSE('',#94799,1.45380901900664,1.43054003732522);
#1826=ELLIPSE('',#94801,1.45322066357761,1.43028995785239);
#1827=ELLIPSE('',#94806,2.14181401024915,1.77588874339951);
#1828=ELLIPSE('',#94808,1.43208157244053,1.38029189146704);
#1829=ELLIPSE('',#94812,2.18879207398525,1.79962727559316);
#1830=ELLIPSE('',#94814,2.18901509550273,1.79974914074665);
#1831=ELLIPSE('',#94817,2.2444282619244,1.82733890923556);
#1832=ELLIPSE('',#94819,2.24443876108746,1.82734353773875);
#1833=ELLIPSE('',#94820,6.74573450851259,5.50047048351084);
#1834=ELLIPSE('',#94821,6.74598671172703,5.50057144500526);
#1835=ELLIPSE('',#94826,2.24510297414266,1.8276717674473);
#1836=ELLIPSE('',#94828,6.74390240939121,5.49585078304806);
#1837=ELLIPSE('',#94829,6.74404990886307,5.4959097928901);
#1838=ELLIPSE('',#94830,2.24510748390125,1.82767438434328);
#1839=ELLIPSE('',#94833,2.19238797298482,1.80144123645576);
#1840=ELLIPSE('',#94835,2.19259034569564,1.80153305864657);
#1841=ELLIPSE('',#94839,1.4316254101432,1.37881184106309);
#1842=ELLIPSE('',#94841,2.14692927256853,1.77849116248874);
#1843=ELLIPSE('',#94843,1.45181104759523,1.42845526063355);
#1844=ELLIPSE('',#94848,1.45196348821223,1.42817952802932);
#1845=ELLIPSE('',#94855,1.47984354908539,1.44816756164213);
#1846=ELLIPSE('',#94857,1.47888863188348,1.44801453428131);
#1847=ELLIPSE('',#94861,1.58904382174786,1.4795419860971);
#1848=ELLIPSE('',#94864,1.58949098795625,1.47983751651523);
#1849=ELLIPSE('',#94887,0.749685754907703,0.60185647341446);
#1850=ELLIPSE('',#94890,1.41328440310968,1.18460827309285);
#1851=ELLIPSE('',#94952,2.88179127866164,2.12564226548654);
#1852=ELLIPSE('',#94953,1.43722552537773,1.32204636451836);
#1853=ELLIPSE('',#94954,0.987429753876356,0.693960884248331);
#1854=ELLIPSE('',#94958,1.87599164352097,1.3631837367251);
#1855=ELLIPSE('',#94976,0.977632591669663,0.93380624359465);
#1856=ELLIPSE('',#94979,0.523318313869799,0.469519600058616);
#1857=ELLIPSE('',#95067,17.5713723065032,4.52112060210991);
#1858=ELLIPSE('',#95068,4.50277672631039,3.19320827117429);
#1859=ELLIPSE('',#95108,9.1303217691259,3.27937044288807);
#1860=ELLIPSE('',#95112,5.58690768783904,2.31976556616765);
#1861=ELLIPSE('',#95177,7.49339813124813,6.10504954200232);
#1862=ELLIPSE('',#95180,7.49235439337033,6.10463249190312);
#1863=ELLIPSE('',#95265,1.25100010657953,1.02769269305806);
#1864=ELLIPSE('',#95282,1.14675177068285,1.02017737933149);
#1865=ELLIPSE('',#95308,1.37382679960868,1.13091857689604);
#1866=ELLIPSE('',#95320,1.04756140277279,1.00921649017983);
#1867=ELLIPSE('',#95333,1.46893565132849,1.19930046752296);
#1868=ELLIPSE('',#95338,7.49433291871596,6.10831258037442);
#1869=ELLIPSE('',#95344,7.4940138380099,6.10818593644246);
#1870=ELLIPSE('',#95364,7.49253505210954,6.10416626992353);
#1871=ELLIPSE('',#95367,7.49234362041712,6.10409043317082);
#1872=ELLIPSE('',#95375,1.47091283278985,1.20059247389518);
#1873=ELLIPSE('',#95388,1.04442811078714,1.00835504871987);
#1874=ELLIPSE('',#95400,1.3774591382642,1.13345236867699);
#1875=ELLIPSE('',#95426,1.13994052039406,1.01834002153806);
#1876=ELLIPSE('',#95434,1.25321023290178,1.03018791386508);
#1877=ELLIPSE('',#95475,11.6751690359376,3.71302998352787);
#1878=ELLIPSE('',#95715,0.678690131415711,0.494805844211885);
#1879=ELLIPSE('',#95726,34.5904711318704,5.84597391203818);
#1880=ELLIPSE('',#96078,11.7565014068008,3.72593447424617);
#1881=ELLIPSE('',#96110,7.46086400325983,6.09136338114254);
#1882=ELLIPSE('',#96116,7.53518791407952,6.1247960459708);
#1883=ELLIPSE('',#96150,7.45763201025,6.09058811436398);
#1884=ELLIPSE('',#96203,9.1303217691259,3.27937044288807);
#1885=ELLIPSE('',#96205,6.16525689027633,2.36185455359168);
#1886=ELLIPSE('',#96212,1.33669592490101,1.1019523707532);
#1887=ELLIPSE('',#96213,1.25109689071003,1.02773417463857);
#1888=ELLIPSE('',#96221,5.58690768783904,2.31976556616765);
#1889=ELLIPSE('',#96224,1.44645360831276,1.18341499862822);
#1890=ELLIPSE('',#96225,1.37376569032744,1.13089346959656);
#1891=ELLIPSE('',#96233,1.49685474119579,1.21828695523177);
#1892=ELLIPSE('',#96234,1.46882736484448,1.19925664387663);
#1893=ELLIPSE('',#96242,1.47121822864674,1.20071603818299);
#1894=ELLIPSE('',#96243,1.49679583489779,1.21835526315613);
#1895=ELLIPSE('',#96251,1.37792699674947,1.13364466418821);
#1896=ELLIPSE('',#96252,1.44801280663984,1.18476784522542);
#1897=ELLIPSE('',#96262,1.25404132664573,1.03054296143257);
#1898=ELLIPSE('',#96263,1.3394502339077,1.10450276996805);
#1899=ELLIPSE('',#96432,0.979743096898815,0.937213104467219);
#1900=ELLIPSE('',#96433,0.523318313830269,0.469519600018551);
#1901=ELLIPSE('',#96496,1.43722552532624,1.32204636444341);
#1902=ELLIPSE('',#96498,0.987429753852244,0.693960884240177);
#1903=ELLIPSE('',#96500,1.01009247479397,0.982994833669031);
#1904=ELLIPSE('',#96682,0.749685755431834,0.601856473637416);
#1905=ELLIPSE('',#96752,1.58949098802822,1.479837516555);
#1906=ELLIPSE('',#96760,1.47888863176487,1.4480145341903);
#1907=ELLIPSE('',#96787,1.45196348827863,1.42817952812272);
#1908=ELLIPSE('',#96802,2.14692927256853,1.77849116248874);
#1909=ELLIPSE('',#96814,2.19259034569564,1.80153305864657);
#1910=ELLIPSE('',#96822,7.53325800757047,6.12058869275862);
#1911=ELLIPSE('',#96825,6.74390240934933,5.49585078303102);
#1912=ELLIPSE('',#96829,6.74404990885783,5.49590979288799);
#1913=ELLIPSE('',#96832,2.24510748390125,1.82767438434328);
#1914=ELLIPSE('',#96845,2.24443876108746,1.82734353773875);
#1915=ELLIPSE('',#96848,6.7457345089557,5.50047048368992);
#1916=ELLIPSE('',#96852,6.7459867118041,5.50057144503682);
#1917=ELLIPSE('',#96854,7.46237077505305,6.09538628449527);
#1918=ELLIPSE('',#96863,2.18901509550273,1.79974914074665);
#1919=ELLIPSE('',#96875,1.43208157237843,1.38029189134632);
#1920=ELLIPSE('',#96889,1.45322066372077,1.43028995804929);
#1921=ELLIPSE('',#96916,1.48262920850352,1.44930064705618);
#1922=ELLIPSE('',#96937,1.59354891806686,1.48067275531);
#1923=ELLIPSE('',#96964,4.50277672631039,3.19320827117429);
#1924=ELLIPSE('',#97067,7.540726371712,6.12413561514585);
#1925=ELLIPSE('',#97070,6.743798136932,5.49640701630224);
#1926=ELLIPSE('',#97074,6.74471830680559,5.49677536023675);
#1927=ELLIPSE('',#97084,1.49663539150943,1.21824685106957);
#1928=ELLIPSE('',#97085,2.24478717905741,1.82751618959032);
#1929=ELLIPSE('',#97089,2.19081358780445,1.80064181344396);
#1930=ELLIPSE('',#97090,1.47034339388813,1.20011049466526);
#1931=ELLIPSE('',#97093,1.4468541246316,1.18395401892993);
#1932=ELLIPSE('',#97094,2.14457779788183,1.77729531483311);
#1933=ELLIPSE('',#97098,1.45276135105947,1.42923490713001);
#1934=ELLIPSE('',#97099,1.37628311373034,1.13241299577346);
#1935=ELLIPSE('',#97105,1.33772997969343,1.1031395948871);
#1936=ELLIPSE('',#97106,1.48049428500572,1.4486765533338);
#1937=ELLIPSE('',#97110,1.59230054967801,1.48054973575714);
#1938=ELLIPSE('',#97111,1.25239319344149,1.02897532635693);
#1939=ELLIPSE('',#97183,17.5713723091178,4.52112060324491);
#1940=ELLIPSE('',#97197,0.872532027987849,0.761015579916806);
#1941=ELLIPSE('',#97198,0.872242253742692,0.756153787356879);
#1942=ELLIPSE('',#97289,2.88179127901306,2.12564226561543);
#1943=ELLIPSE('',#97336,1.58904382162818,1.47954198603725);
#1944=ELLIPSE('',#97338,1.25368354036916,1.03023294677774);
#1945=ELLIPSE('',#97342,1.47984354894719,1.44816756153839);
#1946=ELLIPSE('',#97343,1.33964027941621,1.10428915808927);
#1947=ELLIPSE('',#97350,1.45181104761723,1.42845526066408);
#1948=ELLIPSE('',#97352,1.37663299645276,1.13304702413717);
#1949=ELLIPSE('',#97356,1.4316254101432,1.37881184106309);
#1950=ELLIPSE('',#97357,1.44858750676641,1.18492005208182);
#1951=ELLIPSE('',#97361,2.19238797298482,1.80144123645576);
#1952=ELLIPSE('',#97363,1.47050130285363,1.20041179042018);
#1953=ELLIPSE('',#97367,2.24510297414266,1.8276717674473);
#1954=ELLIPSE('',#97368,1.49718443147311,1.21851081499056);
#1955=ELLIPSE('',#97372,2.2444282619244,1.82733890923556);
#1956=ELLIPSE('',#97374,1.496455657919,1.21812538939567);
#1957=ELLIPSE('',#97378,2.18879207398525,1.79962727559316);
#1958=ELLIPSE('',#97379,1.46934753477481,1.19942122868132);
#1959=ELLIPSE('',#97383,2.14181401024915,1.77588874339951);
#1960=ELLIPSE('',#97385,1.44549176500332,1.18299703423917);
#1961=ELLIPSE('',#97389,1.45380901901781,1.43054003733421);
#1962=ELLIPSE('',#97390,1.37419951292197,1.13085206801441);
#1963=ELLIPSE('',#97397,1.48261995859359,1.44952139988389);
#1964=ELLIPSE('',#97399,1.33548546759184,1.10135868188479);
#1965=ELLIPSE('',#97403,1.46778892822304,1.40956355519549);
#1966=ELLIPSE('',#97409,0.470344661252933,0.437456112172233);
#1967=ELLIPSE('',#97411,0.455017224729773,0.414686073541653);
#1968=ELLIPSE('',#97416,2.23591051322783,1.82312386243465);
#1969=ELLIPSE('',#97419,2.21081023703135,1.81065351490182);
#1970=ELLIPSE('',#97421,1.47966360607638,1.20670524509602);
#1971=ELLIPSE('',#97426,1.43683810399907,1.39553674731997);
#1972=ELLIPSE('',#97427,1.42375962264705,1.16725779022872);
#1973=ELLIPSE('',#97431,1.44688208750104,1.42026986217179);
#1974=ELLIPSE('',#97433,1.39004657997782,1.14302890167313);
#1975=ELLIPSE('',#97437,1.52235692801125,1.4619644583464);
#1976=ELLIPSE('',#97438,1.30002012621557,1.07181606140101);
#1977=ELLIPSE('',#97445,1.34503947637202,1.23514518658134);
#1978=ELLIPSE('',#97451,1.59183749527776,1.48024250578175);
#1979=ELLIPSE('',#97453,1.25206291218026,1.02867529869755);
#1980=ELLIPSE('',#97457,1.48146874171335,1.4488354440584);
#1981=ELLIPSE('',#97458,1.33790496197122,1.1029159114908);
#1982=ELLIPSE('',#97465,1.45260602245606,1.42951177160569);
#1983=ELLIPSE('',#97468,1.37498779933069,1.13181366553965);
#1984=ELLIPSE('',#97472,1.4318714352199,1.37961189358987);
#1985=ELLIPSE('',#97473,1.44743072160946,1.18410503354282);
#1986=ELLIPSE('',#97477,2.19060648404767,1.80054773483043);
#1987=ELLIPSE('',#97480,1.46961676159926,1.19980182022532);
#1988=ELLIPSE('',#97484,2.24478172556828,1.82751302619863);
#1989=ELLIPSE('',#97485,1.49702492666268,1.21840253533698);
#1990=ELLIPSE('',#97642,0.872188006859956,0.755196727163197);
#1991=ELLIPSE('',#97644,1.49262340192896,1.21540966767209);
#1992=ELLIPSE('',#97677,0.937885965402937,0.866754064923446);
#1993=ELLIPSE('',#97692,0.908597175301873,0.820141976513812);
#1994=ELLIPSE('',#98012,3.52383305788943,2.05269137889129);
#1995=ELLIPSE('',#98075,61.9730832448324,42.9788571518931);
#1996=ELLIPSE('',#99192,13.1271153497978,2.2815651398259);
#1997=ELLIPSE('',#99195,1.19618791882944,0.501602687323024);
#1998=ELLIPSE('',#99196,1.29981244177848,1.04628846257511);
#1999=ELLIPSE('',#99204,12.6883691454053,2.13068730228645);
#2000=ELLIPSE('',#99207,1.1878650987102,0.0615784629608745);
#2001=ELLIPSE('',#99209,9.77817556377705,5.31069546080688);
#2002=ELLIPSE('',#99212,88.5846814729442,33.7972522652792);
#2003=ELLIPSE('',#99914,3.52785922818763,2.05416344169751);
#2004=ELLIPSE('',#99983,61.9730832448324,42.9788571518931);
#2005=ELLIPSE('',#101082,2.92401254191216,2.73356722767542);
#2006=ELLIPSE('',#101109,5.10101304780922,2.0080086469997);
#2007=ELLIPSE('',#101114,5.6075381031809,3.56592930826501);
#2008=ELLIPSE('',#101127,13.1302942292056,2.28259278464871);
#2009=ELLIPSE('',#101129,4.57456085127438,4.1484359323234);
#2010=ELLIPSE('',#101131,1.29981239432824,1.04628842702785);
#2011=ELLIPSE('',#101132,1.19618830369613,0.501602775052797);
#2012=ELLIPSE('',#101140,12.6871422926546,2.13028400375921);
#2013=ELLIPSE('',#101142,9.77817556377705,5.31069546080688);
#2014=ELLIPSE('',#101144,1.18790481732873,0.0615825826882351);
#2015=ELLIPSE('',#101147,88.5846058090516,33.7973158081396);
#2016=ELLIPSE('',#102738,0.922279678089193,0.749999999999809);
#2017=ELLIPSE('',#102739,1.28870175757961,0.749999999999421);
#2018=ELLIPSE('',#102741,1.2887017575839,0.750000000003065);
#2019=ELLIPSE('',#102777,0.859134505046975,0.499999999989815);
#2020=ELLIPSE('',#102778,0.614853118726872,0.500000000000419);
#2021=ELLIPSE('',#102780,0.859134505053703,0.499999999999708);
#2022=ELLIPSE('',#102785,1.28870175757994,0.749999999999587);
#2023=ELLIPSE('',#102786,0.922279678089253,0.749999999999816);
#2024=ELLIPSE('',#102789,1.28870175760062,0.750000000020496);
#2025=ELLIPSE('',#102824,0.859134505046725,0.499999999989502);
#2026=ELLIPSE('',#102825,0.614853118726913,0.500000000000432);
#2027=ELLIPSE('',#102827,0.859134505054217,0.500000000000012);
#2028=ELLIPSE('',#103055,20.4666308011442,7.0000000000003);
#2029=ELLIPSE('',#103124,2.41725606676382,0.463770738124485);
#2030=ELLIPSE('',#103128,18.7300337971543,16.644499908438);
#2031=ELLIPSE('',#103129,18.4563717977211,16.4307217995611);
#2032=ELLIPSE('',#103137,1.99975887730092,1.99623716560152);
#2033=ELLIPSE('',#103142,2.00289288489225,1.97864499243066);
#2034=ELLIPSE('',#103145,1.70825186416551,1.63934150110833);
#2035=ELLIPSE('',#103294,2.05999726017368,1.96170207629362);
#2036=ELLIPSE('',#103328,14.1421356237285,9.99999999999842);
#2037=ELLIPSE('',#103330,14.14213562373,9.99999999999928);
#2038=(
BOUNDED_SURFACE()
B_SPLINE_SURFACE(3,2,((#131389,#131390,#131391),(#131392,#131393,#131394),
(#131395,#131396,#131397),(#131398,#131399,#131400)),.UNSPECIFIED.,.F.,
 .F.,.F.)
B_SPLINE_SURFACE_WITH_KNOTS((4,4),(3,3),(0.,0.00040046484477139),(0.,1.),
 .UNSPECIFIED.)
GEOMETRIC_REPRESENTATION_ITEM()
RATIONAL_B_SPLINE_SURFACE(((1.,0.707106781186548,1.),(1.,0.718332690797356,
1.),(1.,0.721890377876178,1.),(1.,0.71893387489533,1.)))
REPRESENTATION_ITEM('')
SURFACE()
);
#2039=(
BOUNDED_SURFACE()
B_SPLINE_SURFACE(3,2,((#131632,#131633,#131634),(#131635,#131636,#131637),
(#131638,#131639,#131640),(#131641,#131642,#131643),(#131644,#131645,#131646),
(#131647,#131648,#131649),(#131650,#131651,#131652),(#131653,#131654,#131655)),
 .UNSPECIFIED.,.F.,.F.,.F.)
B_SPLINE_SURFACE_WITH_KNOTS((4,2,2,4),(3,3),(-6.93889390390723E-18,0.000883592517330617,
0.00132538877599593,0.00176718503466124),(0.,1.),.UNSPECIFIED.)
GEOMETRIC_REPRESENTATION_ITEM()
RATIONAL_B_SPLINE_SURFACE(((1.,0.714572220188102,1.),(1.,0.766482020905858,
1.),(1.,0.804713539964754,1.),(1.,0.843200382681728,1.),(1.,0.852495764772597,
1.),(1.,0.865090875406593,1.),(1.,0.86808633519291,1.),(1.,0.868041451421723,
1.)))
REPRESENTATION_ITEM('')
SURFACE()
);
#2040=(
BOUNDED_SURFACE()
B_SPLINE_SURFACE(3,2,((#131704,#131705,#131706),(#131707,#131708,#131709),
(#131710,#131711,#131712),(#131713,#131714,#131715),(#131716,#131717,#131718),
(#131719,#131720,#131721),(#131722,#131723,#131724),(#131725,#131726,#131727),
(#131728,#131729,#131730),(#131731,#131732,#131733)),.UNSPECIFIED.,.F.,
 .F.,.F.)
B_SPLINE_SURFACE_WITH_KNOTS((4,2,2,2,4),(3,3),(-4.62791697325438E-16,0.00043428534736775,
0.000868570694735964,0.00130285604210418,0.00173714138947239),(0.,1.),
 .UNSPECIFIED.)
GEOMETRIC_REPRESENTATION_ITEM()
RATIONAL_B_SPLINE_SURFACE(((1.,0.823084066989561,1.),(1.,0.819254444805576,
1.),(1.,0.813299508531675,1.),(1.,0.797300511206505,1.),(1.,0.787129420739965,
1.),(1.,0.761999300344554,1.),(1.,0.746886433981532,1.),(1.,0.710597168436061,
1.),(1.,0.68930848675479,1.),(1.,0.664389729441784,1.)))
REPRESENTATION_ITEM('')
SURFACE()
);
#2041=(
BOUNDED_SURFACE()
B_SPLINE_SURFACE(3,2,((#131793,#131794,#131795),(#131796,#131797,#131798),
(#131799,#131800,#131801),(#131802,#131803,#131804)),.UNSPECIFIED.,.F.,
 .F.,.F.)
B_SPLINE_SURFACE_WITH_KNOTS((4,4),(3,3),(0.,0.000503800937603746),(0.,1.),
 .UNSPECIFIED.)
GEOMETRIC_REPRESENTATION_ITEM()
RATIONAL_B_SPLINE_SURFACE(((1.,0.816955285488328,1.),(1.,0.819071576866324,
1.),(1.,0.821113754793722,1.),(1.,0.823084066989369,1.)))
REPRESENTATION_ITEM('')
SURFACE()
);
#2042=(
BOUNDED_SURFACE()
B_SPLINE_SURFACE(3,2,((#131810,#131811,#131812),(#131813,#131814,#131815),
(#131816,#131817,#131818),(#131819,#131820,#131821),(#131822,#131823,#131824),
(#131825,#131826,#131827),(#131828,#131829,#131830),(#131831,#131832,#131833),
(#131834,#131835,#131836),(#131837,#131838,#131839)),.UNSPECIFIED.,.F.,
 .F.,.F.)
B_SPLINE_SURFACE_WITH_KNOTS((4,2,2,2,4),(3,3),(-7.15573433840433E-18,0.000392138229924569,
0.000784276459849145,0.00117641468977372,0.00156855291969829),(0.,1.),
 .UNSPECIFIED.)
GEOMETRIC_REPRESENTATION_ITEM()
RATIONAL_B_SPLINE_SURFACE(((1.,0.761454662564716,1.),(1.,0.777350220421001,
1.),(1.,0.789525254479917,1.),(1.,0.80808932428192,1.),(1.,0.814267286660623,
1.),(1.,0.822043050215882,1.),(1.,0.8235601071816,1.),(1.,0.82291335354639,
1.),(1.,0.820747192732019,1.),(1.,0.816955285488498,1.)))
REPRESENTATION_ITEM('')
SURFACE()
);
#2043=(
BOUNDED_SURFACE()
B_SPLINE_SURFACE(3,2,((#131914,#131915,#131916),(#131917,#131918,#131919),
(#131920,#131921,#131922),(#131923,#131924,#131925),(#131926,#131927,#131928),
(#131929,#131930,#131931)),.UNSPECIFIED.,.F.,.F.,.F.)
B_SPLINE_SURFACE_WITH_KNOTS((4,2,4),(3,3),(-9.86081875875566E-17,0.000795696580732677,
0.00159139316146545),(0.,1.),.UNSPECIFIED.)
GEOMETRIC_REPRESENTATION_ITEM()
RATIONAL_B_SPLINE_SURFACE(((1.,0.707106781186548,1.),(1.,0.682426263182222,
1.),(1.,0.657497772192221,1.),(1.,0.621173394621865,1.),(1.,0.609936188780092,
1.),(1.,0.610093408676581,1.)))
REPRESENTATION_ITEM('')
SURFACE()
);
#2044=(
BOUNDED_SURFACE()
B_SPLINE_SURFACE(3,2,((#131953,#131954,#131955),(#131956,#131957,#131958),
(#131959,#131960,#131961),(#131962,#131963,#131964),(#131965,#131966,#131967),
(#131968,#131969,#131970),(#131971,#131972,#131973),(#131974,#131975,#131976),
(#131977,#131978,#131979),(#131980,#131981,#131982)),.UNSPECIFIED.,.F.,
 .F.,.F.)
B_SPLINE_SURFACE_WITH_KNOTS((4,2,2,2,4),(3,3),(0.,0.000399257182160439,
0.000798514364320879,0.00119777154648132,0.00159702872864176),(0.,1.),
 .UNSPECIFIED.)
GEOMETRIC_REPRESENTATION_ITEM()
RATIONAL_B_SPLINE_SURFACE(((1.,0.805613398857371,1.),(1.,0.805643268651268,
1.),(1.,0.802937363700045,1.),(1.,0.792810049002322,1.),(1.,0.785336419192136,
1.),(1.,0.767086380955436,1.),(1.,0.756158224894836,1.),(1.,0.732687821688199,
1.),(1.,0.719866291289219,1.),(1.,0.707106781186559,1.)))
REPRESENTATION_ITEM('')
SURFACE()
);
#2045=(
BOUNDED_SURFACE()
B_SPLINE_SURFACE(3,2,((#132088,#132089,#132090),(#132091,#132092,#132093),
(#132094,#132095,#132096),(#132097,#132098,#132099),(#132100,#132101,#132102),
(#132103,#132104,#132105),(#132106,#132107,#132108),(#132109,#132110,#132111),
(#132112,#132113,#132114),(#132115,#132116,#132117)),.UNSPECIFIED.,.F.,
 .F.,.F.)
B_SPLINE_SURFACE_WITH_KNOTS((4,2,2,2,4),(3,3),(0.,0.000408971318093432,
0.000817942636186865,0.0012269139542803,0.00163588527237373),(0.,1.),
 .UNSPECIFIED.)
GEOMETRIC_REPRESENTATION_ITEM()
RATIONAL_B_SPLINE_SURFACE(((1.,0.707106781186548,1.),(1.,0.688859876352089,
1.),(1.,0.670469148037181,1.),(1.,0.634232875326911,1.),(1.,0.617116919953528,
1.),(1.,0.586509610415134,1.),(1.,0.573603373050602,1.),(1.,0.555466576286827,
1.),(1.,0.550482231415542,1.),(1.,0.55046727607882,1.)))
REPRESENTATION_ITEM('')
SURFACE()
);
#2046=(
BOUNDED_SURFACE()
B_SPLINE_SURFACE(3,2,((#132223,#132224,#132225),(#132226,#132227,#132228),
(#132229,#132230,#132231),(#132232,#132233,#132234),(#132235,#132236,#132237),
(#132238,#132239,#132240)),.UNSPECIFIED.,.F.,.F.,.F.)
B_SPLINE_SURFACE_WITH_KNOTS((4,2,4),(3,3),(0.,0.0008117357936932,0.0016234715873864),
(0.,1.),.UNSPECIFIED.)
GEOMETRIC_REPRESENTATION_ITEM()
RATIONAL_B_SPLINE_SURFACE(((1.,0.707106781186543,1.),(1.,0.739826804639566,
1.),(1.,0.771134330273905,1.),(1.,0.817260896513624,1.),(1.,0.831377708695547,
1.),(1.,0.831289505264087,1.)))
REPRESENTATION_ITEM('')
SURFACE()
);
#2047=(
BOUNDED_SURFACE()
B_SPLINE_SURFACE(3,2,((#132262,#132263,#132264),(#132265,#132266,#132267),
(#132268,#132269,#132270),(#132271,#132272,#132273),(#132274,#132275,#132276),
(#132277,#132278,#132279),(#132280,#132281,#132282),(#132283,#132284,#132285),
(#132286,#132287,#132288),(#132289,#132290,#132291)),.UNSPECIFIED.,.F.,
 .F.,.F.)
B_SPLINE_SURFACE_WITH_KNOTS((4,2,2,2,4),(3,3),(0.,0.000403813407730069,
0.00080762681546014,0.00121144022319021,0.00161525363092028),(0.,1.),
 .UNSPECIFIED.)
GEOMETRIC_REPRESENTATION_ITEM()
RATIONAL_B_SPLINE_SURFACE(((1.,0.574616980402532,1.),(1.,0.574559944255782,
1.),(1.,0.578580805360036,1.),(1.,0.593205211704828,1.),(1.,0.603887596362185,
1.),(1.,0.629170763939607,1.),(1.,0.643946507952345,1.),(1.,0.674809145535283,
1.),(1.,0.691194307570675,1.),(1.,0.707106781186543,1.)))
REPRESENTATION_ITEM('')
SURFACE()
);
#2048=(
BOUNDED_SURFACE()
B_SPLINE_SURFACE(3,2,((#132373,#132374,#132375),(#132376,#132377,#132378),
(#132379,#132380,#132381),(#132382,#132383,#132384),(#132385,#132386,#132387),
(#132388,#132389,#132390),(#132391,#132392,#132393),(#132394,#132395,#132396),
(#132397,#132398,#132399),(#132400,#132401,#132402)),.UNSPECIFIED.,.F.,
 .F.,.F.)
B_SPLINE_SURFACE_WITH_KNOTS((4,2,2,2,4),(3,3),(-3.25260651745651E-18,0.000393055033931551,
0.000786110067863104,0.00117916510179466,0.00157222013572621),(0.,1.),
 .UNSPECIFIED.)
GEOMETRIC_REPRESENTATION_ITEM()
RATIONAL_B_SPLINE_SURFACE(((1.,0.759233451646328,1.),(1.,0.765853834182409,
1.),(1.,0.77182063876785,1.),(1.,0.782085007421256,1.),(1.,0.786377884755709,
1.),(1.,0.792439775573655,1.),(1.,0.794229619467717,1.),(1.,0.793882695203775,
1.),(1.,0.791736824593394,1.),(1.,0.786683372191859,1.)))
REPRESENTATION_ITEM('')
SURFACE()
);
#2049=(
BOUNDED_SURFACE()
B_SPLINE_SURFACE(3,2,((#132459,#132460,#132461),(#132462,#132463,#132464),
(#132465,#132466,#132467),(#132468,#132469,#132470)),.UNSPECIFIED.,.F.,
 .F.,.F.)
B_SPLINE_SURFACE_WITH_KNOTS((4,4),(3,3),(2.16840434497101E-19,0.000504355062152837),
(0.,1.),.UNSPECIFIED.)
GEOMETRIC_REPRESENTATION_ITEM()
RATIONAL_B_SPLINE_SURFACE(((1.,0.759233451646319,1.),(1.,0.762871393877082,
1.),(1.,0.766403968732707,1.),(1.,0.769836971136898,1.)))
REPRESENTATION_ITEM('')
SURFACE()
);
#2050=(
BOUNDED_SURFACE()
B_SPLINE_SURFACE(3,2,((#132476,#132477,#132478),(#132479,#132480,#132481),
(#132482,#132483,#132484),(#132485,#132486,#132487),(#132488,#132489,#132490),
(#132491,#132492,#132493)),.UNSPECIFIED.,.F.,.F.,.F.)
B_SPLINE_SURFACE_WITH_KNOTS((4,2,4),(3,3),(-7.10152422978005E-18,0.000826467086096255,
0.00165293417219252),(0.,1.),.UNSPECIFIED.)
GEOMETRIC_REPRESENTATION_ITEM()
RATIONAL_B_SPLINE_SURFACE(((1.,0.634315526883885,1.),(1.,0.669226935131166,
1.),(1.,0.696507858185965,1.),(1.,0.739984504397939,1.),(1.,0.756420113602562,
1.),(1.,0.769836971137166,1.)))
REPRESENTATION_ITEM('')
SURFACE()
);
#2051=(
BOUNDED_SURFACE()
B_SPLINE_SURFACE(3,2,((#132531,#132532,#132533),(#132534,#132535,#132536),
(#132537,#132538,#132539),(#132540,#132541,#132542),(#132543,#132544,#132545),
(#132546,#132547,#132548),(#132549,#132550,#132551),(#132552,#132553,#132554),
(#132555,#132556,#132557),(#132558,#132559,#132560)),.UNSPECIFIED.,.F.,
 .F.,.F.)
B_SPLINE_SURFACE_WITH_KNOTS((4,2,2,2,4),(3,3),(-9.01822866961737E-5,0.000428050429885702,
0.000856100859773762,0.00128415128966182,0.0018023840062437),(-0.000709751295981599,
1.),.UNSPECIFIED.)
GEOMETRIC_REPRESENTATION_ITEM()
RATIONAL_B_SPLINE_SURFACE(((1.00018329866537,0.870871200656103,1.),(1.00017803427841,
0.874579814490897,1.),(1.00017912606777,0.873810679327735,1.),(1.00019317825117,
0.863911307902413,1.),(1.000204118,0.856204559855697,1.),(1.00023569027009,
0.833962775819186,1.),(1.00025618433367,0.819525279404997,1.),(1.00031175778272,
0.780375333947188,1.),(1.00034836088001,0.754589472410892,1.),(1.00039261225142,
0.723415614990589,1.)))
REPRESENTATION_ITEM('')
SURFACE()
);
#2052=(
BOUNDED_SURFACE()
B_SPLINE_SURFACE(3,2,((#132586,#132587,#132588),(#132589,#132590,#132591),
(#132592,#132593,#132594),(#132595,#132596,#132597)),.UNSPECIFIED.,.F.,
 .F.,.F.)
B_SPLINE_SURFACE_WITH_KNOTS((4,4),(3,3),(0.,0.000504208024932662),(0.,1.),
 .UNSPECIFIED.)
GEOMETRIC_REPRESENTATION_ITEM()
RATIONAL_B_SPLINE_SURFACE(((1.,0.872490094680101,1.),(1.,0.873532316568381,
1.),(1.,0.874514063294085,1.),(1.,0.875436198637085,1.)))
REPRESENTATION_ITEM('')
SURFACE()
);
#2053=(
BOUNDED_SURFACE()
B_SPLINE_SURFACE(3,2,((#132603,#132604,#132605),(#132606,#132607,#132608),
(#132609,#132610,#132611),(#132612,#132613,#132614),(#132615,#132616,#132617),
(#132618,#132619,#132620),(#132621,#132622,#132623),(#132624,#132625,#132626),
(#132627,#132628,#132629),(#132630,#132631,#132632),(#132633,#132634,#132635),
(#132636,#132637,#132638)),.UNSPECIFIED.,.F.,.F.,.F.)
B_SPLINE_SURFACE_WITH_KNOTS((4,2,2,2,2,4),(3,3),(0.,0.000471787629256711,
0.000943575258513421,0.00117946907314178,0.00141536288777013,0.00188715051702685),
(0.,1.),.UNSPECIFIED.)
GEOMETRIC_REPRESENTATION_ITEM()
RATIONAL_B_SPLINE_SURFACE(((1.,0.688859710774758,1.),(1.,0.717278497414175,
1.),(1.,0.742415568607548,1.),(1.,0.786827943379553,1.),(1.,0.806155596178757,
1.),(1.,0.829868996905786,1.),(1.,0.837032764561711,1.),(1.,0.849395444084014,
1.),(1.,0.854694123459555,1.),(1.,0.86824784980175,1.),(1.,0.873676740317145,
1.),(1.,0.875436198637081,1.)))
REPRESENTATION_ITEM('')
SURFACE()
);
#2054=(
BOUNDED_SURFACE()
B_SPLINE_SURFACE(3,2,((#132703,#132704,#132705),(#132706,#132707,#132708),
(#132709,#132710,#132711),(#132712,#132713,#132714)),.UNSPECIFIED.,.F.,
 .F.,.F.)
B_SPLINE_SURFACE_WITH_KNOTS((4,4),(3,3),(0.000909429960036056,0.00157021148057203),
(0.,1.),.UNSPECIFIED.)
GEOMETRIC_REPRESENTATION_ITEM()
RATIONAL_B_SPLINE_SURFACE(((1.,0.72569894652024,1.),(1.,0.728856973451895,
1.),(1.,0.724481780670466,1.),(1.,0.707106781186543,1.)))
REPRESENTATION_ITEM('')
SURFACE()
);
#2055=(
BOUNDED_SURFACE()
B_SPLINE_SURFACE(3,2,((#132727,#132728,#132729),(#132730,#132731,#132732),
(#132733,#132734,#132735),(#132736,#132737,#132738)),.UNSPECIFIED.,.F.,
 .F.,.F.)
B_SPLINE_SURFACE_WITH_KNOTS((4,4),(3,3),(-1.50704101975485E-17,0.000358861832009556),
(0.,1.),.UNSPECIFIED.)
GEOMETRIC_REPRESENTATION_ITEM()
RATIONAL_B_SPLINE_SURFACE(((1.,0.707106781186544,1.),(1.,0.693584131808955,
1.),(1.,0.67719600445086,1.),(1.,0.65799444631037,1.)))
REPRESENTATION_ITEM('')
SURFACE()
);
#2056=(
BOUNDED_SURFACE()
B_SPLINE_SURFACE(3,2,((#133123,#133124,#133125),(#133126,#133127,#133128),
(#133129,#133130,#133131),(#133132,#133133,#133134)),.UNSPECIFIED.,.F.,
 .F.,.F.)
B_SPLINE_SURFACE_WITH_KNOTS((4,4),(3,3),(5.42101086242752E-20,0.000113625826113285),
(0.,1.),.UNSPECIFIED.)
GEOMETRIC_REPRESENTATION_ITEM()
RATIONAL_B_SPLINE_SURFACE(((1.,0.691935594449019,1.),(1.,0.697297182114951,
1.),(1.,0.702351867303478,1.),(1.,0.70710678118654,1.)))
REPRESENTATION_ITEM('')
SURFACE()
);
#2057=(
BOUNDED_SURFACE()
B_SPLINE_SURFACE(3,2,((#133147,#133148,#133149),(#133150,#133151,#133152),
(#133153,#133154,#133155),(#133156,#133157,#133158),(#133159,#133160,#133161),
(#133162,#133163,#133164)),.UNSPECIFIED.,.F.,.F.,.F.)
B_SPLINE_SURFACE_WITH_KNOTS((4,2,4),(3,3),(0.,0.000500133683539797,0.00100026736707959),
(0.,1.),.UNSPECIFIED.)
GEOMETRIC_REPRESENTATION_ITEM()
RATIONAL_B_SPLINE_SURFACE(((1.,0.707106781186538,1.),(1.,0.722794581177,
1.),(1.,0.731463278267736,1.),(1.,0.737752025312339,1.),(1.,0.735567484186947,
1.),(1.,0.732423362569068,1.)))
REPRESENTATION_ITEM('')
SURFACE()
);
#2058=(
BOUNDED_SURFACE()
B_SPLINE_SURFACE(3,2,((#133347,#133348,#133349),(#133350,#133351,#133352),
(#133353,#133354,#133355),(#133356,#133357,#133358),(#133359,#133360,#133361),
(#133362,#133363,#133364)),.UNSPECIFIED.,.F.,.F.,.F.)
B_SPLINE_SURFACE_WITH_KNOTS((4,2,4),(3,3),(0.,0.000635851334990063,0.00127170266998013),
(0.,1.),.UNSPECIFIED.)
GEOMETRIC_REPRESENTATION_ITEM()
RATIONAL_B_SPLINE_SURFACE(((1.,0.549598954535088,1.),(1.,0.549481216714779,
1.),(1.,0.561870616792487,1.),(1.,0.602538835999935,1.),(1.,0.629604434612806,
1.),(1.,0.65799444631184,1.)))
REPRESENTATION_ITEM('')
SURFACE()
);
#2059=(
BOUNDED_SURFACE()
B_SPLINE_SURFACE(3,2,((#133389,#133390,#133391),(#133392,#133393,#133394),
(#133395,#133396,#133397),(#133398,#133399,#133400),(#133401,#133402,#133403),
(#133404,#133405,#133406),(#133407,#133408,#133409),(#133410,#133411,#133412)),
 .UNSPECIFIED.,.F.,.F.,.F.)
B_SPLINE_SURFACE_WITH_KNOTS((4,2,2,4),(3,3),(0.,0.000399389907139719,0.000798779814279438,
0.00159755962855888),(0.,1.),.UNSPECIFIED.)
GEOMETRIC_REPRESENTATION_ITEM()
RATIONAL_B_SPLINE_SURFACE(((1.,0.707106781186543,1.),(1.,0.719972059607527,
1.),(1.,0.732679659198347,1.),(1.,0.756479572209125,1.),(1.,0.767365377234031,
1.),(1.,0.79501980381119,1.),(1.,0.806340389868128,1.),(1.,0.806206028026398,
1.)))
REPRESENTATION_ITEM('')
SURFACE()
);
#2060=(
BOUNDED_SURFACE()
B_SPLINE_SURFACE(3,2,((#133427,#133428,#133429),(#133430,#133431,#133432),
(#133433,#133434,#133435),(#133436,#133437,#133438),(#133439,#133440,#133441),
(#133442,#133443,#133444),(#133445,#133446,#133447),(#133448,#133449,#133450),
(#133451,#133452,#133453),(#133454,#133455,#133456)),.UNSPECIFIED.,.F.,
 .F.,.F.)
B_SPLINE_SURFACE_WITH_KNOTS((4,2,2,2,4),(3,3),(0.,0.000397955182835291,
0.000795910365670582,0.00119386554850587,0.00159182073134117),(0.,1.),
 .UNSPECIFIED.)
GEOMETRIC_REPRESENTATION_ITEM()
RATIONAL_B_SPLINE_SURFACE(((1.,0.60931006565052,1.),(1.,0.60928110676943,
1.),(1.,0.611992414032709,1.),(1.,0.622151576786515,1.),(1.,0.629646305612374,
1.),(1.,0.647895096091951,1.),(1.,0.658798646820943,1.),(1.,0.682038372243284,
1.),(1.,0.694657643733687,1.),(1.,0.707106781186553,1.)))
REPRESENTATION_ITEM('')
SURFACE()
);
#2061=(
BOUNDED_SURFACE()
B_SPLINE_SURFACE(3,2,((#133485,#133486,#133487),(#133488,#133489,#133490),
(#133491,#133492,#133493),(#133494,#133495,#133496),(#133497,#133498,#133499),
(#133500,#133501,#133502),(#133503,#133504,#133505),(#133506,#133507,#133508),
(#133509,#133510,#133511),(#133512,#133513,#133514)),.UNSPECIFIED.,.F.,
 .F.,.F.)
B_SPLINE_SURFACE_WITH_KNOTS((4,2,2,2,4),(3,3),(0.,0.00039329942356206,0.000786598847124121,
0.00117989827068618,0.00157319769424824),(0.,1.),.UNSPECIFIED.)
GEOMETRIC_REPRESENTATION_ITEM()
RATIONAL_B_SPLINE_SURFACE(((1.,0.825370895892916,1.),(1.,0.829081051796027,
1.),(1.,0.831084991111337,1.),(1.,0.831059675364535,1.),(1.,0.829021889329635,
1.),(1.,0.819977402296451,1.),(1.,0.812885056457023,1.),(1.,0.792515337687537,
1.),(1.,0.779105591645567,1.),(1.,0.762081632340355,1.)))
REPRESENTATION_ITEM('')
SURFACE()
);
#2062=(
BOUNDED_SURFACE()
B_SPLINE_SURFACE(3,2,((#133527,#133528,#133529),(#133530,#133531,#133532),
(#133533,#133534,#133535),(#133536,#133537,#133538)),.UNSPECIFIED.,.F.,
 .F.,.F.)
B_SPLINE_SURFACE_WITH_KNOTS((4,4),(3,3),(-2.62810606610486E-16,0.000504136652582459),
(0.,1.),.UNSPECIFIED.)
GEOMETRIC_REPRESENTATION_ITEM()
RATIONAL_B_SPLINE_SURFACE(((1.,0.831517473467334,1.),(1.,0.829540548856785,
1.),(1.,0.827492428459287,1.),(1.,0.825370895892945,1.)))
REPRESENTATION_ITEM('')
SURFACE()
);
#2063=(
BOUNDED_SURFACE()
B_SPLINE_SURFACE(3,2,((#133542,#133543,#133544),(#133545,#133546,#133547),
(#133548,#133549,#133550),(#133551,#133552,#133553),(#133554,#133555,#133556),
(#133557,#133558,#133559),(#133560,#133561,#133562),(#133563,#133564,#133565),
(#133566,#133567,#133568),(#133569,#133570,#133571),(#133572,#133573,#133574),
(#133575,#133576,#133577)),.UNSPECIFIED.,.F.,.F.,.F.)
B_SPLINE_SURFACE_WITH_KNOTS((4,2,2,2,2,4),(3,3),(-0.000176150978763801,
0.000440377446917856,0.000880754893835713,0.00110094361729464,0.00132113234075357,
0.00193766076643857),(0.,1.00051287559994),.UNSPECIFIED.)
GEOMETRIC_REPRESENTATION_ITEM()
RATIONAL_B_SPLINE_SURFACE(((1.,0.629431973271816,1.00038011059806),(1.,
0.671936522340933,1.00033651150585),(1.,0.704322705400091,1.00030329133971),
(1.,0.750691692792477,1.00025572829526),(1.,0.766670204641027,1.00023933831756),
(1.,0.786800026967206,1.00021869012815),(1.,0.792954061695274,1.00021237761965),
(1.,0.80379124513689,1.00020126136573),(1.,0.808563806838397,1.00019636590484),
(1.,0.824745084867243,1.00017976793948),(1.,0.832099980342898,1.00017222364662),
(1.,0.835028609003294,1.00016921960226)))
REPRESENTATION_ITEM('')
SURFACE()
);
#2064=(
BOUNDED_SURFACE()
B_SPLINE_SURFACE(3,2,((#133645,#133646,#133647),(#133648,#133649,#133650),
(#133651,#133652,#133653),(#133654,#133655,#133656),(#133657,#133658,#133659),
(#133660,#133661,#133662),(#133663,#133664,#133665),(#133666,#133667,#133668),
(#133669,#133670,#133671),(#133672,#133673,#133674)),.UNSPECIFIED.,.F.,
 .F.,.F.)
B_SPLINE_SURFACE_WITH_KNOTS((4,2,2,2,4),(3,3),(-0.000135704889425893,0.000453061765036137,
0.000906123530072295,0.00135918529510845,0.00194795194957144),(-0.000781731935573401,
1.00013570488943),.UNSPECIFIED.)
GEOMETRIC_REPRESENTATION_ITEM()
RATIONAL_B_SPLINE_SURFACE(((1.00019390081514,0.8759631402042,1.00003363851682),
(1.00018914318116,0.879006562062377,1.00003281314767),(1.00019402369835,
0.875884532760928,1.00003365983498),(1.00021859753591,0.860164837917186,
1.00003792298079),(1.00023473046334,0.84984472834809,1.00004072177124),
(1.00027794935235,0.822197937521576,1.0000482195186),(1.00030475494617,
0.805050605368179,1.00005286983644),(1.00037753551171,0.758493437481938,
1.00006549603544),(1.00042634862193,0.727268066383258,1.0000739642857),
(1.00048406431786,0.690347779692363,1.00008397698424)))
REPRESENTATION_ITEM('')
SURFACE()
);
#2065=(
BOUNDED_SURFACE()
B_SPLINE_SURFACE(3,2,((#133726,#133727,#133728),(#133729,#133730,#133731),
(#133732,#133733,#133734),(#133735,#133736,#133737)),.UNSPECIFIED.,.F.,
 .F.,.F.)
B_SPLINE_SURFACE_WITH_KNOTS((4,4),(3,3),(0.,0.000503779257761556),(0.,1.),
 .UNSPECIFIED.)
GEOMETRIC_REPRESENTATION_ITEM()
RATIONAL_B_SPLINE_SURFACE(((1.,0.877279917170998,1.),(1.,0.877311423474687,
1.),(1.,0.877285649811871,1.),(1.,0.877202574460126,1.)))
REPRESENTATION_ITEM('')
SURFACE()
);
#2066=(
BOUNDED_SURFACE()
B_SPLINE_SURFACE(3,2,((#133741,#133742,#133743),(#133744,#133745,#133746),
(#133747,#133748,#133749),(#133750,#133751,#133752),(#133753,#133754,#133755),
(#133756,#133757,#133758),(#133759,#133760,#133761),(#133762,#133763,#133764),
(#133765,#133766,#133767),(#133768,#133769,#133770)),.UNSPECIFIED.,.F.,
 .F.,.F.)
B_SPLINE_SURFACE_WITH_KNOTS((4,2,2,2,4),(3,3),(-0.000155617325212005,0.000907880296577857,
0.00113485037072232,0.00136182044486679,0.00197137791837065),(0.,1.00015561732522),
 .UNSPECIFIED.)
GEOMETRIC_REPRESENTATION_ITEM()
RATIONAL_B_SPLINE_SURFACE(((1.,0.68550557359324,1.00009788156287),(1.,0.752540961090915,
1.00007701782747),(1.,0.80291249495684,1.00006134046074),(1.,0.8425596182679,
1.00004900090217),(1.,0.848571644906788,1.00004712975116),(1.,0.858970162163407,
1.00004389337228),(1.,0.8633849038709,1.00004251935169),(1.,0.876162786879574,
1.00003854243174),(1.,0.879321122197454,1.00003755944835),(1.,0.875948401811248,
1.0000386091558)))
REPRESENTATION_ITEM('')
SURFACE()
);
#2067=(
BOUNDED_SURFACE()
B_SPLINE_SURFACE(3,2,((#133838,#133839,#133840),(#133841,#133842,#133843),
(#133844,#133845,#133846),(#133847,#133848,#133849),(#133850,#133851,#133852),
(#133853,#133854,#133855),(#133856,#133857,#133858),(#133859,#133860,#133861),
(#133862,#133863,#133864),(#133865,#133866,#133867)),.UNSPECIFIED.,.F.,
 .F.,.F.)
B_SPLINE_SURFACE_WITH_KNOTS((4,2,2,2,4),(3,3),(-8.34022521184474E-16,0.000443043867974425,
0.000886087735949684,0.00132913160392494,0.00177217547190021),(0.,1.),
 .UNSPECIFIED.)
GEOMETRIC_REPRESENTATION_ITEM()
RATIONAL_B_SPLINE_SURFACE(((1.,0.834143101464621,1.),(1.,0.83044410875076,
1.),(1.,0.824302497883951,1.),(1.,0.80744078994961,1.),(1.,0.79657978834944,
1.),(1.,0.769588124839812,1.),(1.,0.753384767045469,1.),(1.,0.714346006222175,
1.),(1.,0.691706791956038,1.),(1.,0.665108204576645,1.)))
REPRESENTATION_ITEM('')
SURFACE()
);
#2068=(
BOUNDED_SURFACE()
B_SPLINE_SURFACE(3,2,((#133880,#133881,#133882),(#133883,#133884,#133885),
(#133886,#133887,#133888),(#133889,#133890,#133891)),.UNSPECIFIED.,.F.,
 .F.,.F.)
B_SPLINE_SURFACE_WITH_KNOTS((4,4),(3,3),(0.,0.000504125640440226),(0.,1.),
 .UNSPECIFIED.)
GEOMETRIC_REPRESENTATION_ITEM()
RATIONAL_B_SPLINE_SURFACE(((1.,0.828190603154496,1.),(1.,0.830246482056442,
1.),(1.,0.832229943187683,1.),(1.,0.834143101464675,1.)))
REPRESENTATION_ITEM('')
SURFACE()
);
#2069=(
BOUNDED_SURFACE()
B_SPLINE_SURFACE(3,2,((#133895,#133896,#133897),(#133898,#133899,#133900),
(#133901,#133902,#133903),(#133904,#133905,#133906),(#133907,#133908,#133909),
(#133910,#133911,#133912),(#133913,#133914,#133915),(#133916,#133917,#133918)),
 .UNSPECIFIED.,.F.,.F.,.F.)
B_SPLINE_SURFACE_WITH_KNOTS((4,2,2,4),(3,3),(0.,0.000394166264145648,0.000788332528291295,
0.00157666505658259),(0.,1.),.UNSPECIFIED.)
GEOMETRIC_REPRESENTATION_ITEM()
RATIONAL_B_SPLINE_SURFACE(((1.,0.760827176127386,1.),(1.,0.778398802886113,
1.),(1.,0.792083552136379,1.),(1.,0.813520155171949,1.),(1.,0.820889309284053,
1.),(1.,0.835705990917082,1.),(1.,0.835268319089816,1.),(1.,0.828190603154679,
1.)))
REPRESENTATION_ITEM('')
SURFACE()
);
#2070=(
BOUNDED_SURFACE()
B_SPLINE_SURFACE(3,2,((#133945,#133946,#133947),(#133948,#133949,#133950),
(#133951,#133952,#133953),(#133954,#133955,#133956),(#133957,#133958,#133959),
(#133960,#133961,#133962)),.UNSPECIFIED.,.F.,.F.,.F.)
B_SPLINE_SURFACE_WITH_KNOTS((4,2,4),(3,3),(0.,0.000795474163050539,0.00159094832610108),
(0.,1.),.UNSPECIFIED.)
GEOMETRIC_REPRESENTATION_ITEM()
RATIONAL_B_SPLINE_SURFACE(((1.,0.707106781186543,1.),(1.,0.682590952101739,
1.),(1.,0.657853637690047,1.),(1.,0.62184399984072,1.),(1.,0.610720170210845,
1.),(1.,0.610875747200839,1.)))
REPRESENTATION_ITEM('')
SURFACE()
);
#2071=(
BOUNDED_SURFACE()
B_SPLINE_SURFACE(3,2,((#133975,#133976,#133977),(#133978,#133979,#133980),
(#133981,#133982,#133983),(#133984,#133985,#133986),(#133987,#133988,#133989),
(#133990,#133991,#133992),(#133993,#133994,#133995),(#133996,#133997,#133998),
(#133999,#134000,#134001),(#134002,#134003,#134004)),.UNSPECIFIED.,.F.,
 .F.,.F.)
B_SPLINE_SURFACE_WITH_KNOTS((4,2,2,2,4),(3,3),(0.,0.000399133477242608,
0.000798266954485216,0.00119740043172782,0.00159653390897044),(0.,1.),
 .UNSPECIFIED.)
GEOMETRIC_REPRESENTATION_ITEM()
RATIONAL_B_SPLINE_SURFACE(((1.,0.805020333414601,1.),(1.,0.805049923545582,
1.),(1.,0.802360394037482,1.),(1.,0.792292516045722,1.),(1.,0.784862653088995,
1.),(1.,0.766719225973379,1.),(1.,0.755854623801483,1.),(1.,0.732526059701691,
1.),(1.,0.719783513455905,1.),(1.,0.707106781186554,1.)))
REPRESENTATION_ITEM('')
SURFACE()
);
#2072=(
BOUNDED_SURFACE()
B_SPLINE_SURFACE(3,2,((#134060,#134061,#134062),(#134063,#134064,#134065),
(#134066,#134067,#134068),(#134069,#134070,#134071),(#134072,#134073,#134074),
(#134075,#134076,#134077),(#134078,#134079,#134080),(#134081,#134082,#134083)),
 .UNSPECIFIED.,.F.,.F.,.F.)
B_SPLINE_SURFACE_WITH_KNOTS((4,2,2,4),(3,3),(-3.14418630020796E-18,0.000761037462531171,
0.00114155619379676,0.00152207492506235),(0.,1.),.UNSPECIFIED.)
GEOMETRIC_REPRESENTATION_ITEM()
RATIONAL_B_SPLINE_SURFACE(((1.,0.691935594449023,1.),(1.,0.657938057153071,
1.),(1.,0.623321566128117,1.),(1.,0.582569634693765,1.),(1.,0.571407182182735,
1.),(1.,0.5555307216223,1.),(1.,0.551373498869702,1.),(1.,0.551334230064852,
1.)))
REPRESENTATION_ITEM('')
SURFACE()
);
#2073=(
BOUNDED_SURFACE()
B_SPLINE_SURFACE(3,2,((#134122,#134123,#134124),(#134125,#134126,#134127),
(#134128,#134129,#134130),(#134131,#134132,#134133),(#134134,#134135,#134136),
(#134137,#134138,#134139)),.UNSPECIFIED.,.F.,.F.,.F.)
B_SPLINE_SURFACE_WITH_KNOTS((4,2,4),(3,3),(4.71238898038469,5.49778714378214,
6.28318530717959),(0.,1.),.UNSPECIFIED.)
GEOMETRIC_REPRESENTATION_ITEM()
RATIONAL_B_SPLINE_SURFACE(((1.,0.707106781186548,1.),(1.,0.699025295935929,
1.),(1.,0.690860049127223,1.),(1.,0.679082711198032,1.),(1.,0.675526278180878,
1.),(1.,0.675590207615665,1.)))
REPRESENTATION_ITEM('')
SURFACE()
);
#2074=(
BOUNDED_SURFACE()
B_SPLINE_SURFACE(3,2,((#134152,#134153,#134154),(#134155,#134156,#134157),
(#134158,#134159,#134160),(#134161,#134162,#134163),(#134164,#134165,#134166),
(#134167,#134168,#134169)),.UNSPECIFIED.,.F.,.F.,.F.)
B_SPLINE_SURFACE_WITH_KNOTS((4,2,4),(3,3),(1.41124413247309E-15,0.78539816339745,
1.5707963267949),(0.,1.),.UNSPECIFIED.)
GEOMETRIC_REPRESENTATION_ITEM()
RATIONAL_B_SPLINE_SURFACE(((1.,0.73727733681012,1.),(1.,0.737326538316275,
1.),(1.,0.734106258287724,1.),(1.,0.723033691556635,1.),(1.,0.715202981902879,
1.),(1.,0.707106781186548,1.)))
REPRESENTATION_ITEM('')
SURFACE()
);
#2075=(
BOUNDED_SURFACE()
B_SPLINE_SURFACE(3,2,((#134195,#134196,#134197),(#134198,#134199,#134200),
(#134201,#134202,#134203),(#134204,#134205,#134206),(#134207,#134208,#134209),
(#134210,#134211,#134212)),.UNSPECIFIED.,.F.,.F.,.F.)
B_SPLINE_SURFACE_WITH_KNOTS((4,2,4),(3,3),(3.1415926535898,3.72828696246945,
4.31498127134909),(0.,1.),.UNSPECIFIED.)
GEOMETRIC_REPRESENTATION_ITEM()
RATIONAL_B_SPLINE_SURFACE(((1.,0.737277336810115,1.),(1.,0.73729299178243,
1.),(1.,0.735539930277599,1.),(1.,0.729097328045697,1.),(1.,0.724411344440144,
1.),(1.,0.71893387489533,1.)))
REPRESENTATION_ITEM('')
SURFACE()
);
#2076=(
BOUNDED_SURFACE()
B_SPLINE_SURFACE(3,2,((#134225,#134226,#134227),(#134228,#134229,#134230),
(#134231,#134232,#134233),(#134234,#134235,#134236),(#134237,#134238,#134239),
(#134240,#134241,#134242)),.UNSPECIFIED.,.F.,.F.,.F.)
B_SPLINE_SURFACE_WITH_KNOTS((4,2,4),(3,3),(0.,0.00169934430350512,0.00339868860701024),
(0.,1.),.UNSPECIFIED.)
GEOMETRIC_REPRESENTATION_ITEM()
RATIONAL_B_SPLINE_SURFACE(((1.,0.707106781186547,1.),(1.,0.74482559038907,
1.),(1.,0.778551967557851,1.),(1.,0.840511428018892,1.),(1.,0.868726285027217,
1.),(1.,0.894799245647903,1.)))
REPRESENTATION_ITEM('')
SURFACE()
);
#2077=(
BOUNDED_SURFACE()
B_SPLINE_SURFACE(3,2,((#134277,#134278,#134279),(#134280,#134281,#134282),
(#134283,#134284,#134285),(#134286,#134287,#134288),(#134289,#134290,#134291),
(#134292,#134293,#134294)),.UNSPECIFIED.,.F.,.F.,.F.)
B_SPLINE_SURFACE_WITH_KNOTS((4,2,4),(3,3),(4.71238898038469,5.49778714378214,
6.28318530717959),(0.,1.),.UNSPECIFIED.)
GEOMETRIC_REPRESENTATION_ITEM()
RATIONAL_B_SPLINE_SURFACE(((1.,0.707106781186548,1.),(1.,0.699025295935929,
1.),(1.,0.690860049127223,1.),(1.,0.679082711198032,1.),(1.,0.675526278180878,
1.),(1.,0.675590207615665,1.)))
REPRESENTATION_ITEM('')
SURFACE()
);
#2078=(
BOUNDED_SURFACE()
B_SPLINE_SURFACE(3,2,((#134307,#134308,#134309),(#134310,#134311,#134312),
(#134313,#134314,#134315),(#134316,#134317,#134318),(#134319,#134320,#134321),
(#134322,#134323,#134324)),.UNSPECIFIED.,.F.,.F.,.F.)
B_SPLINE_SURFACE_WITH_KNOTS((4,2,4),(3,3),(3.1415926535898,3.92699081698724,
4.71238898038469),(0.,1.),.UNSPECIFIED.)
GEOMETRIC_REPRESENTATION_ITEM()
RATIONAL_B_SPLINE_SURFACE(((1.,0.73727733681012,1.),(1.,0.737326538316634,
1.),(1.,0.734106258287243,1.),(1.,0.723033691557116,1.),(1.,0.715202981902516,
1.),(1.,0.707106781186548,1.)))
REPRESENTATION_ITEM('')
SURFACE()
);
#2079=(
BOUNDED_SURFACE()
B_SPLINE_SURFACE(3,2,((#134339,#134340,#134341),(#134342,#134343,#134344),
(#134345,#134346,#134347),(#134348,#134349,#134350),(#134351,#134352,#134353),
(#134354,#134355,#134356)),.UNSPECIFIED.,.F.,.F.,.F.)
B_SPLINE_SURFACE_WITH_KNOTS((4,2,4),(3,3),(-3.25260651745651E-18,0.00101351621082632,
0.00202703242165263),(0.,1.),.UNSPECIFIED.)
GEOMETRIC_REPRESENTATION_ITEM()
RATIONAL_B_SPLINE_SURFACE(((1.,0.893214344719542,1.),(1.,0.912305000874927,
1.),(1.,0.927255525935639,1.),(1.,0.94789383214718,1.),(1.,0.953590869545161,
1.),(1.,0.953555223991885,1.)))
REPRESENTATION_ITEM('')
SURFACE()
);
#2080=(
BOUNDED_SURFACE()
B_SPLINE_SURFACE(3,2,((#134395,#134396,#134397),(#134398,#134399,#134400),
(#134401,#134402,#134403),(#134404,#134405,#134406),(#134407,#134408,#134409),
(#134410,#134411,#134412)),.UNSPECIFIED.,.F.,.F.,.F.)
B_SPLINE_SURFACE_WITH_KNOTS((4,2,4),(3,3),(4.71238898038469,5.49778714378214,
6.28318530717959),(0.,1.),.UNSPECIFIED.)
GEOMETRIC_REPRESENTATION_ITEM()
RATIONAL_B_SPLINE_SURFACE(((1.,0.707106781186543,1.),(1.,0.715202981902221,
1.),(1.,0.723033691557525,1.),(1.,0.734106258286841,1.),(1.,0.737326538316939,
1.),(1.,0.737277336810125,1.)))
REPRESENTATION_ITEM('')
SURFACE()
);
#2081=(
BOUNDED_SURFACE()
B_SPLINE_SURFACE(3,2,((#134425,#134426,#134427),(#134428,#134429,#134430),
(#134431,#134432,#134433),(#134434,#134435,#134436),(#134437,#134438,#134439),
(#134440,#134441,#134442)),.UNSPECIFIED.,.F.,.F.,.F.)
B_SPLINE_SURFACE_WITH_KNOTS((4,2,4),(3,3),(3.1415926535898,3.92699081698724,
4.71238898038469),(0.,1.),.UNSPECIFIED.)
GEOMETRIC_REPRESENTATION_ITEM()
RATIONAL_B_SPLINE_SURFACE(((1.,0.675590207615659,1.),(1.,0.675526278181242,
1.),(1.,0.679082711197541,1.),(1.,0.690860049127717,1.),(1.,0.699025295935567,
1.),(1.,0.707106781186543,1.)))
REPRESENTATION_ITEM('')
SURFACE()
);
#2082=(
BOUNDED_SURFACE()
B_SPLINE_SURFACE(3,2,((#134455,#134456,#134457),(#134458,#134459,#134460),
(#134461,#134462,#134463),(#134464,#134465,#134466),(#134467,#134468,#134469),
(#134470,#134471,#134472)),.UNSPECIFIED.,.F.,.F.,.F.)
B_SPLINE_SURFACE_WITH_KNOTS((4,2,4),(3,3),(0.,0.00162565899344706,0.00325131798689413),
(0.,1.),.UNSPECIFIED.)
GEOMETRIC_REPRESENTATION_ITEM()
RATIONAL_B_SPLINE_SURFACE(((1.,0.893214344719539,1.),(1.,0.868075018581634,
1.),(1.,0.841018189595232,1.),(1.,0.782003386508022,1.),(1.,0.750058517040659,
1.),(1.,0.714668958264373,1.)))
REPRESENTATION_ITEM('')
SURFACE()
);
#2083=(
BOUNDED_SURFACE()
B_SPLINE_SURFACE(3,2,((#134511,#134512,#134513),(#134514,#134515,#134516),
(#134517,#134518,#134519),(#134520,#134521,#134522),(#134523,#134524,#134525),
(#134526,#134527,#134528)),.UNSPECIFIED.,.F.,.F.,.F.)
B_SPLINE_SURFACE_WITH_KNOTS((4,2,4),(3,3),(1.5707963267949,2.35619449019234,
3.1415926535898),(0.,1.),.UNSPECIFIED.)
GEOMETRIC_REPRESENTATION_ITEM()
RATIONAL_B_SPLINE_SURFACE(((1.,0.707106781186543,1.),(1.,0.71520298190223,
1.),(1.,0.723033691557516,1.),(1.,0.734106258286857,1.),(1.,0.737326538316932,
1.),(1.,0.737277336810125,1.)))
REPRESENTATION_ITEM('')
SURFACE()
);
#2084=(
BOUNDED_SURFACE()
B_SPLINE_SURFACE(3,2,((#134541,#134542,#134543),(#134544,#134545,#134546),
(#134547,#134548,#134549),(#134550,#134551,#134552),(#134553,#134554,#134555),
(#134556,#134557,#134558)),.UNSPECIFIED.,.F.,.F.,.F.)
B_SPLINE_SURFACE_WITH_KNOTS((4,2,4),(3,3),(3.1415926535898,3.92699081698724,
4.71238898038469),(0.,1.),.UNSPECIFIED.)
GEOMETRIC_REPRESENTATION_ITEM()
RATIONAL_B_SPLINE_SURFACE(((1.,0.675590207615659,1.),(1.,0.675526278181249,
1.),(1.,0.679082711197525,1.),(1.,0.69086004912773,1.),(1.,0.699025295935556,
1.),(1.,0.707106781186543,1.)))
REPRESENTATION_ITEM('')
SURFACE()
);
#2085=(
BOUNDED_SURFACE()
B_SPLINE_SURFACE(3,2,((#134603,#134604,#134605),(#134606,#134607,#134608),
(#134609,#134610,#134611),(#134612,#134613,#134614),(#134615,#134616,#134617),
(#134618,#134619,#134620)),.UNSPECIFIED.,.F.,.F.,.F.)
B_SPLINE_SURFACE_WITH_KNOTS((4,2,4),(3,3),(4.71238898038469,5.49778714378214,
6.28318530717959),(0.,1.),.UNSPECIFIED.)
GEOMETRIC_REPRESENTATION_ITEM()
RATIONAL_B_SPLINE_SURFACE(((1.,0.707106781186543,1.),(1.,0.699025295935225,
1.),(1.,0.690860049128176,1.),(1.,0.679082711197064,1.),(1.,0.6755262781816,
1.),(1.,0.675590207615662,1.)))
REPRESENTATION_ITEM('')
SURFACE()
);
#2086=(
BOUNDED_SURFACE()
B_SPLINE_SURFACE(3,2,((#134633,#134634,#134635),(#134636,#134637,#134638),
(#134639,#134640,#134641),(#134642,#134643,#134644),(#134645,#134646,#134647),
(#134648,#134649,#134650)),.UNSPECIFIED.,.F.,.F.,.F.)
B_SPLINE_SURFACE_WITH_KNOTS((4,2,4),(3,3),(0.,0.785398163397448,1.5707963267949),
(0.,1.),.UNSPECIFIED.)
GEOMETRIC_REPRESENTATION_ITEM()
RATIONAL_B_SPLINE_SURFACE(((1.,0.737277336810127,1.),(1.,0.737326538316762,
1.),(1.,0.734106258287074,1.),(1.,0.723033691557295,1.),(1.,0.715202981902387,
1.),(1.,0.707106781186548,1.)))
REPRESENTATION_ITEM('')
SURFACE()
);
#2087=(
BOUNDED_SURFACE()
B_SPLINE_SURFACE(3,2,((#134676,#134677,#134678),(#134679,#134680,#134681),
(#134682,#134683,#134684),(#134685,#134686,#134687)),.UNSPECIFIED.,.F.,
 .F.,.F.)
B_SPLINE_SURFACE_WITH_KNOTS((4,4),(3,3),(3.1415926535898,3.72189740710945),
(0.,1.),.UNSPECIFIED.)
GEOMETRIC_REPRESENTATION_ITEM()
RATIONAL_B_SPLINE_SURFACE(((1.,0.737277336810124,1.),(1.,0.737285953283754,
1.),(1.,0.735586930398308,1.),(1.,0.732423362569238,1.)))
REPRESENTATION_ITEM('')
SURFACE()
);
#2088=(
BOUNDED_SURFACE()
B_SPLINE_SURFACE(3,2,((#134695,#134696,#134697),(#134698,#134699,#134700),
(#134701,#134702,#134703),(#134704,#134705,#134706),(#134707,#134708,#134709),
(#134710,#134711,#134712)),.UNSPECIFIED.,.F.,.F.,.F.)
B_SPLINE_SURFACE_WITH_KNOTS((4,2,4),(3,3),(0.,0.00168309713341273,0.00336619426682545),
(0.,1.),.UNSPECIFIED.)
GEOMETRIC_REPRESENTATION_ITEM()
RATIONAL_B_SPLINE_SURFACE(((1.,0.707106781186545,1.),(1.,0.744273762477552,
1.),(1.,0.7776417896067,1.),(1.,0.83910580954319,1.),(1.,0.867185102973278,
1.),(1.,0.89321434471954,1.)))
REPRESENTATION_ITEM('')
SURFACE()
);
#2089=(
BOUNDED_SURFACE()
B_SPLINE_SURFACE(3,2,((#134756,#134757,#134758),(#134759,#134760,#134761),
(#134762,#134763,#134764),(#134765,#134766,#134767),(#134768,#134769,#134770),
(#134771,#134772,#134773)),.UNSPECIFIED.,.F.,.F.,.F.)
B_SPLINE_SURFACE_WITH_KNOTS((4,2,4),(3,3),(4.71238898038469,5.49778714378214,
6.28318530717959),(0.,1.),.UNSPECIFIED.)
GEOMETRIC_REPRESENTATION_ITEM()
RATIONAL_B_SPLINE_SURFACE(((1.,0.707106781186543,1.),(1.,0.699025295935037,
1.),(1.,0.690860049128415,1.),(1.,0.679082711196836,1.),(1.,0.675526278181767,
1.),(1.,0.675590207615662,1.)))
REPRESENTATION_ITEM('')
SURFACE()
);
#2090=(
BOUNDED_SURFACE()
B_SPLINE_SURFACE(3,2,((#134786,#134787,#134788),(#134789,#134790,#134791),
(#134792,#134793,#134794),(#134795,#134796,#134797),(#134798,#134799,#134800),
(#134801,#134802,#134803)),.UNSPECIFIED.,.F.,.F.,.F.)
B_SPLINE_SURFACE_WITH_KNOTS((4,2,4),(3,3),(3.1415926535898,3.92699081698724,
4.71238898038469),(0.,1.),.UNSPECIFIED.)
GEOMETRIC_REPRESENTATION_ITEM()
RATIONAL_B_SPLINE_SURFACE(((1.,0.737277336810123,1.),(1.,0.737326538316937,
1.),(1.,0.73410625828684,1.),(1.,0.723033691557529,1.),(1.,0.715202981902217,
1.),(1.,0.707106781186543,1.)))
REPRESENTATION_ITEM('')
SURFACE()
);
#2091=(
BOUNDED_SURFACE()
B_SPLINE_SURFACE(3,2,((#134816,#134817,#134818),(#134819,#134820,#134821),
(#134822,#134823,#134824),(#134825,#134826,#134827),(#134828,#134829,#134830),
(#134831,#134832,#134833)),.UNSPECIFIED.,.F.,.F.,.F.)
B_SPLINE_SURFACE_WITH_KNOTS((4,2,4),(3,3),(9.63948754967748E-5,0.00173129457116097,
0.00336619426682516),(0.,1.),.UNSPECIFIED.)
GEOMETRIC_REPRESENTATION_ITEM()
RATIONAL_B_SPLINE_SURFACE(((1.,0.88872394157032,1.),(1.,0.863203710383462,
1.),(1.,0.835728844788038,1.),(1.,0.775725241916869,1.),(1.,0.743211702946043,
1.),(1.,0.707106781186548,1.)))
REPRESENTATION_ITEM('')
SURFACE()
);
#2092=(
BOUNDED_SURFACE()
B_SPLINE_SURFACE(3,2,((#134855,#134856,#134857),(#134858,#134859,#134860),
(#134861,#134862,#134863),(#134864,#134865,#134866)),.UNSPECIFIED.,.F.,
 .F.,.F.)
B_SPLINE_SURFACE_WITH_KNOTS((4,4),(3,3),(2.22847122787664,3.14161440295379),
(-2.1749363990258E-5,1.),.UNSPECIFIED.)
GEOMETRIC_REPRESENTATION_ITEM()
RATIONAL_B_SPLINE_SURFACE(((1.00001193202905,0.725692460307629,1.),(1.00001161526324,
0.732974645844473,1.),(1.00001142611057,0.737323110435419,1.),(1.00001142835037,
0.737271619087495,0.999999999999999)))
REPRESENTATION_ITEM('')
SURFACE()
);
#2093=(
BOUNDED_SURFACE()
B_SPLINE_SURFACE(3,2,((#134887,#134888,#134889),(#134890,#134891,#134892),
(#134893,#134894,#134895),(#134896,#134897,#134898),(#134899,#134900,#134901),
(#134902,#134903,#134904)),.UNSPECIFIED.,.F.,.F.,.F.)
B_SPLINE_SURFACE_WITH_KNOTS((4,2,4),(3,3),(4.71238898038469,5.49778714378214,
6.28318530717959),(0.,1.),.UNSPECIFIED.)
GEOMETRIC_REPRESENTATION_ITEM()
RATIONAL_B_SPLINE_SURFACE(((1.,0.707106781186538,1.),(1.,0.715202981902668,
1.),(1.,0.723033691556936,1.),(1.,0.734106258287417,1.),(1.,0.737326538316498,
1.),(1.,0.737277336810125,1.)))
REPRESENTATION_ITEM('')
SURFACE()
);
#2094=(
BOUNDED_SURFACE()
B_SPLINE_SURFACE(3,2,((#134917,#134918,#134919),(#134920,#134921,#134922),
(#134923,#134924,#134925),(#134926,#134927,#134928),(#134929,#134930,#134931),
(#134932,#134933,#134934)),.UNSPECIFIED.,.F.,.F.,.F.)
B_SPLINE_SURFACE_WITH_KNOTS((4,2,4),(3,3),(0.,0.785398163397448,1.5707963267949),
(0.,1.),.UNSPECIFIED.)
GEOMETRIC_REPRESENTATION_ITEM()
RATIONAL_B_SPLINE_SURFACE(((1.,0.675590207615664,1.),(1.,0.675526278181461,
1.),(1.,0.679082711197251,1.),(1.,0.690860049128011,1.),(1.,0.699025295935341,
1.),(1.,0.707106781186543,1.)))
REPRESENTATION_ITEM('')
SURFACE()
);
#2095=(
BOUNDED_SURFACE()
B_SPLINE_SURFACE(3,2,((#134977,#134978,#134979),(#134980,#134981,#134982),
(#134983,#134984,#134985),(#134986,#134987,#134988),(#134989,#134990,#134991),
(#134992,#134993,#134994)),.UNSPECIFIED.,.F.,.F.,.F.)
B_SPLINE_SURFACE_WITH_KNOTS((4,2,4),(3,3),(1.5707963267949,2.35619449019234,
3.1415926535898),(0.,1.),.UNSPECIFIED.)
GEOMETRIC_REPRESENTATION_ITEM()
RATIONAL_B_SPLINE_SURFACE(((1.,0.707106781186543,1.),(1.,0.715202981902222,
1.),(1.,0.723033691557528,1.),(1.,0.73410625828684,1.),(1.,0.737326538316928,
1.),(1.,0.737277336810125,1.)))
REPRESENTATION_ITEM('')
SURFACE()
);
#2096=(
BOUNDED_SURFACE()
B_SPLINE_SURFACE(3,2,((#135007,#135008,#135009),(#135010,#135011,#135012),
(#135013,#135014,#135015),(#135016,#135017,#135018),(#135019,#135020,#135021),
(#135022,#135023,#135024)),.UNSPECIFIED.,.F.,.F.,.F.)
B_SPLINE_SURFACE_WITH_KNOTS((4,2,4),(3,3),(0.,0.785398163397448,1.5707963267949),
(0.,1.),.UNSPECIFIED.)
GEOMETRIC_REPRESENTATION_ITEM()
RATIONAL_B_SPLINE_SURFACE(((1.,0.675590207615664,1.),(1.,0.675526278181762,
1.),(1.,0.679082711196844,1.),(1.,0.690860049128418,1.),(1.,0.699025295935035,
1.),(1.,0.707106781186543,1.)))
REPRESENTATION_ITEM('')
SURFACE()
);
#2097=(
BOUNDED_SURFACE()
B_SPLINE_SURFACE(3,2,((#135086,#135087,#135088),(#135089,#135090,#135091),
(#135092,#135093,#135094),(#135095,#135096,#135097)),.UNSPECIFIED.,.F.,
 .F.,.F.)
B_SPLINE_SURFACE_WITH_KNOTS((4,4),(3,3),(0.,0.000650162698700256),(0.,1.),
 .UNSPECIFIED.)
GEOMETRIC_REPRESENTATION_ITEM()
RATIONAL_B_SPLINE_SURFACE(((1.,0.690549802660026,1.),(1.,0.689437188232559,
1.),(1.,0.688863085247593,1.),(1.,0.688859710772113,1.)))
REPRESENTATION_ITEM('')
SURFACE()
);
#2098=(
BOUNDED_SURFACE()
B_SPLINE_SURFACE(3,2,((#135103,#135104,#135105),(#135106,#135107,#135108),
(#135109,#135110,#135111),(#135112,#135113,#135114)),.UNSPECIFIED.,.F.,
 .F.,.F.)
B_SPLINE_SURFACE_WITH_KNOTS((4,4),(3,3),(-6.93889390390723E-18,0.0331958858056162),
(0.,1.),.UNSPECIFIED.)
GEOMETRIC_REPRESENTATION_ITEM()
RATIONAL_B_SPLINE_SURFACE(((1.,0.685275128444715,1.),(1.,0.687584548418076,
1.),(1.,0.689209215689052,1.),(1.,0.690549802660031,1.)))
REPRESENTATION_ITEM('')
SURFACE()
);
#2099=(
BOUNDED_SURFACE()
B_SPLINE_SURFACE(3,2,((#135126,#135127,#135128),(#135129,#135130,#135131),
(#135132,#135133,#135134),(#135135,#135136,#135137),(#135138,#135139,#135140),
(#135141,#135142,#135143),(#135144,#135145,#135146),(#135147,#135148,#135149),
(#135150,#135151,#135152),(#135153,#135154,#135155),(#135156,#135157,#135158),
(#135159,#135160,#135161),(#135162,#135163,#135164),(#135165,#135166,#135167)),
 .UNSPECIFIED.,.F.,.F.,.F.)
B_SPLINE_SURFACE_WITH_KNOTS((4,2,2,2,2,2,4),(3,3),(-9.99593665452618E-5,
0.000249898416362892,0.000374847624544338,0.000499796832725785,0.000624746040907231,
0.000749695249088677,0.00109955303199673),(-0.00121399112232759,1.00003012118409),
 .UNSPECIFIED.)
GEOMETRIC_REPRESENTATION_ITEM()
RATIONAL_B_SPLINE_SURFACE(((1.00075881319157,0.687462263241503,1.0000188051834),
(1.0007674207464,0.683917008974209,1.00001901849894),(1.00077151552536,
0.682230463507457,1.00001911997723),(1.00077025819397,0.682748329448053,
1.00001908881759),(1.00076928167011,0.683150537212566,1.00001906461702),
(1.00076613988363,0.684444566951248,1.00001898675613),(1.00076399876361,
0.685326445139633,1.00001893369412),(1.00075856649934,0.687563870106642,
1.00001879906978),(1.000755378547,0.688876914504211,1.00001872006479),(1.0007481508392,
0.69185384145156,1.00001854094512),(1.00074408123656,0.693530017369103,
1.00001844009075),(1.00072783192001,0.700222737891797,1.0000180373943),
(1.00071354413798,0.706107547365276,1.00001768330931),(1.00070077601211,
0.711366445349713,1.00001736688499)))
REPRESENTATION_ITEM('')
SURFACE()
);
#2100=(
BOUNDED_SURFACE()
B_SPLINE_SURFACE(3,2,((#135420,#135421,#135422),(#135423,#135424,#135425),
(#135426,#135427,#135428),(#135429,#135430,#135431),(#135432,#135433,#135434),
(#135435,#135436,#135437)),.UNSPECIFIED.,.F.,.F.,.F.)
B_SPLINE_SURFACE_WITH_KNOTS((4,2,4),(3,3),(0.0202634924775631,0.0220347355863407,
0.0238059786951184),(0.,1.),.UNSPECIFIED.)
GEOMETRIC_REPRESENTATION_ITEM()
RATIONAL_B_SPLINE_SURFACE(((1.,0.707106781186538,1.),(1.,0.681614664404396,
1.),(1.,0.655059254259685,1.),(1.,0.598852069172831,1.),(1.,0.569209502658738,
1.),(1.,0.537299608347133,1.)))
REPRESENTATION_ITEM('')
SURFACE()
);
#2101=(
BOUNDED_SURFACE()
B_SPLINE_SURFACE(3,2,((#135836,#135837,#135838),(#135839,#135840,#135841),
(#135842,#135843,#135844),(#135845,#135846,#135847),(#135848,#135849,#135850),
(#135851,#135852,#135853),(#135854,#135855,#135856),(#135857,#135858,#135859),
(#135860,#135861,#135862),(#135863,#135864,#135865)),.UNSPECIFIED.,.F.,
 .F.,.F.)
B_SPLINE_SURFACE_WITH_KNOTS((4,2,2,2,4),(3,3),(-4.08272591082004E-15,0.000408890006701704,
0.000817780013407491,0.00122667002011328,0.00163556002681907),(0.,1.),
 .UNSPECIFIED.)
GEOMETRIC_REPRESENTATION_ITEM()
RATIONAL_B_SPLINE_SURFACE(((1.,0.707106781186878,1.),(1.,0.688891921544893,
1.),(1.,0.670532818962991,1.),(1.,0.634368444020432,1.),(1.,0.617287210907485,
1.),(1.,0.586753298958185,1.),(1.,0.573879231151052,1.),(1.,0.555793216592158,
1.),(1.,0.550823008344725,1.),(1.,0.550808342809435,1.)))
REPRESENTATION_ITEM('')
SURFACE()
);
#2102=(
BOUNDED_SURFACE()
B_SPLINE_SURFACE(3,2,((#135947,#135948,#135949),(#135950,#135951,#135952),
(#135953,#135954,#135955),(#135956,#135957,#135958),(#135959,#135960,#135961),
(#135962,#135963,#135964),(#135965,#135966,#135967),(#135968,#135969,#135970),
(#135971,#135972,#135973),(#135974,#135975,#135976)),.UNSPECIFIED.,.F.,
 .F.,.F.)
B_SPLINE_SURFACE_WITH_KNOTS((4,2,2,2,4),(3,3),(-5.38853734303535E-5,0.000399221470224828,
0.000798442940449655,0.00119766441067448,0.00165077125432966),(-5.38853734303535E-5,
1.),.UNSPECIFIED.)
GEOMETRIC_REPRESENTATION_ITEM()
RATIONAL_B_SPLINE_SURFACE(((1.00002098681007,0.805264316328848,1.),(1.00002089216129,
0.806142558161274,1.),(1.00002118366649,0.803437694284019,1.),(1.00002234668521,
0.79264609497424,1.),(1.00002315070481,0.785185632613891,1.),(1.00002511413113,
0.766967086537006,1.),(1.0000262898705,0.756057452790845,1.),(1.00002898535259,
0.731046193594127,1.),(1.00003056885291,0.716352964024592,1.),(1.00003212218393,
0.701939674122364,1.)))
REPRESENTATION_ITEM('')
SURFACE()
);
#2103=(
BOUNDED_SURFACE()
B_SPLINE_SURFACE(3,2,((#136069,#136070,#136071),(#136072,#136073,#136074),
(#136075,#136076,#136077),(#136078,#136079,#136080),(#136081,#136082,#136083),
(#136084,#136085,#136086)),.UNSPECIFIED.,.F.,.F.,.F.)
B_SPLINE_SURFACE_WITH_KNOTS((4,2,4),(3,3),(-1.94017978766281E-16,0.000795637462001992,
0.00159127492400417),(0.,1.),.UNSPECIFIED.)
GEOMETRIC_REPRESENTATION_ITEM()
RATIONAL_B_SPLINE_SURFACE(((1.,0.707106781186555,1.),(1.,0.682471170316176,
1.),(1.,0.657591859959034,1.),(1.,0.621346223380964,1.),(1.,0.610136165392898,
1.),(1.,0.610293066582478,1.)))
REPRESENTATION_ITEM('')
SURFACE()
);
#2104=(
BOUNDED_SURFACE()
B_SPLINE_SURFACE(3,2,((#136124,#136125,#136126),(#136127,#136128,#136129),
(#136130,#136131,#136132),(#136133,#136134,#136135),(#136136,#136137,#136138),
(#136139,#136140,#136141),(#136142,#136143,#136144),(#136145,#136146,#136147)),
 .UNSPECIFIED.,.F.,.F.,.F.)
B_SPLINE_SURFACE_WITH_KNOTS((4,2,2,4),(3,3),(0.,0.000393730579424048,0.000787461158848096,
0.00157492231769619),(0.,1.),.UNSPECIFIED.)
GEOMETRIC_REPRESENTATION_ITEM()
RATIONAL_B_SPLINE_SURFACE(((1.,0.761354724782829,1.),(1.,0.778699482201342,
1.),(1.,0.792177303062869,1.),(1.,0.813203501689393,1.),(1.,0.820397856397578,
1.),(1.,0.834724000629532,1.),(1.,0.834081767050111,1.),(1.,0.826892724830075,
1.)))
REPRESENTATION_ITEM('')
SURFACE()
);
#2105=(
BOUNDED_SURFACE()
B_SPLINE_SURFACE(3,2,((#136167,#136168,#136169),(#136170,#136171,#136172),
(#136173,#136174,#136175),(#136176,#136177,#136178)),.UNSPECIFIED.,.F.,
 .F.,.F.)
B_SPLINE_SURFACE_WITH_KNOTS((4,4),(3,3),(-2.30501381870419E-16,0.000504122926429285),
(0.,1.),.UNSPECIFIED.)
GEOMETRIC_REPRESENTATION_ITEM()
RATIONAL_B_SPLINE_SURFACE(((1.,0.832929291663028,1.),(1.,0.830988393206304,
1.),(1.,0.828976922242354,1.),(1.,0.82689272482991,1.)))
REPRESENTATION_ITEM('')
SURFACE()
);
#2106=(
BOUNDED_SURFACE()
B_SPLINE_SURFACE(3,2,((#136184,#136185,#136186),(#136187,#136188,#136189),
(#136190,#136191,#136192),(#136193,#136194,#136195),(#136196,#136197,#136198),
(#136199,#136200,#136201),(#136202,#136203,#136204),(#136205,#136206,#136207),
(#136208,#136209,#136210),(#136211,#136212,#136213)),.UNSPECIFIED.,.F.,
 .F.,.F.)
B_SPLINE_SURFACE_WITH_KNOTS((4,2,2,2,4),(3,3),(-1.86157513015761E-16,0.000442340065143073,
0.000884680130286332,0.00132702019542959,0.00176936026057285),(0.,1.),
 .UNSPECIFIED.)
GEOMETRIC_REPRESENTATION_ITEM()
RATIONAL_B_SPLINE_SURFACE(((1.,0.83292929166297,1.),(1.,0.829173169481911,
1.),(1.,0.823008202027213,1.),(1.,0.806154887727085,1.),(1.,0.795326013033949,
1.),(1.,0.768452086196073,1.),(1.,0.752322946736307,1.),(1.,0.713492386952618,
1.),(1.,0.69094524448308,1.),(1.,0.664473794614023,1.)))
REPRESENTATION_ITEM('')
SURFACE()
);
#2107=(
BOUNDED_SURFACE()
B_SPLINE_SURFACE(3,2,((#136301,#136302,#136303),(#136304,#136305,#136306),
(#136307,#136308,#136309),(#136310,#136311,#136312),(#136313,#136314,#136315),
(#136316,#136317,#136318),(#136319,#136320,#136321),(#136322,#136323,#136324),
(#136325,#136326,#136327),(#136328,#136329,#136330)),.UNSPECIFIED.,.F.,
 .F.,.F.)
B_SPLINE_SURFACE_WITH_KNOTS((4,2,2,2,4),(3,3),(-0.000154485852495398,0.000906588491342359,
0.00113323561417795,0.00135988273701354,0.00196766283517968),(-0.000154485852495398,
1.),.UNSPECIFIED.)
GEOMETRIC_REPRESENTATION_ITEM()
RATIONAL_B_SPLINE_SURFACE(((1.00009689723556,0.686387996056344,1.),(1.00007625016334,
0.753213119168533,1.),(1.00006074765387,0.803387647186572,1.),(1.00004855990641,
0.842833807662968,1.),(1.00004671134296,0.848816761518043,1.),(1.00004351687879,
0.859155779998294,1.),(1.0000421620718,0.863540670176529,1.),(1.00003825071871,
0.876199929974803,1.),(1.00003729591827,0.879290182030031,1.),(1.00003834620117,
0.875890896968986,1.)))
REPRESENTATION_ITEM('')
SURFACE()
);
#2108=(
BOUNDED_SURFACE()
B_SPLINE_SURFACE(3,2,((#136411,#136412,#136413),(#136414,#136415,#136416),
(#136417,#136418,#136419),(#136420,#136421,#136422)),.UNSPECIFIED.,.F.,
 .F.,.F.)
B_SPLINE_SURFACE_WITH_KNOTS((4,4),(3,3),(-2.91650384398601E-17,0.000810744804887501),
(0.,1.),.UNSPECIFIED.)
GEOMETRIC_REPRESENTATION_ITEM()
RATIONAL_B_SPLINE_SURFACE(((1.,0.804104907750019,1.),(1.,0.778265384411316,
1.),(1.,0.743775615594857,1.),(1.,0.707106781186549,1.)))
REPRESENTATION_ITEM('')
SURFACE()
);
#2109=(
BOUNDED_SURFACE()
B_SPLINE_SURFACE(3,2,((#136439,#136440,#136441),(#136442,#136443,#136444),
(#136445,#136446,#136447),(#136448,#136449,#136450),(#136451,#136452,#136453),
(#136454,#136455,#136456),(#136457,#136458,#136459),(#136460,#136461,#136462),
(#136463,#136464,#136465),(#136466,#136467,#136468)),.UNSPECIFIED.,.F.,
 .F.,.F.)
B_SPLINE_SURFACE_WITH_KNOTS((4,2,2,2,4),(3,3),(0.00807567872552143,0.00870243807057167,
0.0093291974156219,0.00995595676067213,0.0105827161057224),(0.,1.),
 .UNSPECIFIED.)
GEOMETRIC_REPRESENTATION_ITEM()
RATIONAL_B_SPLINE_SURFACE(((1.,0.707106781186547,1.),(1.,0.707175173315664,
1.),(1.,0.707241719347897,1.),(1.,0.707371272007346,1.),(1.,0.70743422794471,
1.),(1.,0.707549712034256,1.),(1.,0.707603875852248,1.),(1.,0.707699291327501,
1.),(1.,0.707740674853624,1.),(1.,0.707775806502368,1.)))
REPRESENTATION_ITEM('')
SURFACE()
);
#2110=(
BOUNDED_SURFACE()
B_SPLINE_SURFACE(3,2,((#136516,#136517,#136518),(#136519,#136520,#136521),
(#136522,#136523,#136524),(#136525,#136526,#136527),(#136528,#136529,#136530),
(#136531,#136532,#136533),(#136534,#136535,#136536),(#136537,#136538,#136539),
(#136540,#136541,#136542),(#136543,#136544,#136545),(#136546,#136547,#136548),
(#136549,#136550,#136551)),.UNSPECIFIED.,.F.,.F.,.F.)
B_SPLINE_SURFACE_WITH_KNOTS((4,2,2,2,2,4),(3,3),(0.00807567643991074,0.0087258483708248,
0.00905093433628183,0.00937602030173886,0.0100261922326529,0.010676364163567),
(0.,1.),.UNSPECIFIED.)
GEOMETRIC_REPRESENTATION_ITEM()
RATIONAL_B_SPLINE_SURFACE(((1.,0.707106781186547,1.),(1.,0.707170635637275,
1.),(1.,0.707232744268554,1.),(1.,0.70732338528182,1.),(1.,0.707353375007997,
1.),(1.,0.707410998957093,1.),(1.,0.707438747129451,1.),(1.,0.707518900645085,
1.),(1.,0.707568814651682,1.),(1.,0.707655521042551,1.),(1.,0.707692858707996,
1.),(1.,0.707723858215708,1.)))
REPRESENTATION_ITEM('')
SURFACE()
);
#2111=(
BOUNDED_SURFACE()
B_SPLINE_SURFACE(3,2,((#136601,#136602,#136603),(#136604,#136605,#136606),
(#136607,#136608,#136609),(#136610,#136611,#136612)),.UNSPECIFIED.,.F.,
 .F.,.F.)
B_SPLINE_SURFACE_WITH_KNOTS((4,4),(3,3),(0.,0.000650122897330092),(0.,1.),
 .UNSPECIFIED.)
GEOMETRIC_REPRESENTATION_ITEM()
RATIONAL_B_SPLINE_SURFACE(((1.,0.713892198341303,1.),(1.,0.714340614318511,
1.),(1.,0.714570777789516,1.),(1.,0.714572220188112,1.)))
REPRESENTATION_ITEM('')
SURFACE()
);
#2112=(
BOUNDED_SURFACE()
B_SPLINE_SURFACE(3,2,((#136660,#136661,#136662),(#136663,#136664,#136665),
(#136666,#136667,#136668),(#136669,#136670,#136671)),.UNSPECIFIED.,.F.,
 .F.,.F.)
B_SPLINE_SURFACE_WITH_KNOTS((4,4),(3,3),(0.,0.000650368158908551),(0.,1.),
 .UNSPECIFIED.)
GEOMETRIC_REPRESENTATION_ITEM()
RATIONAL_B_SPLINE_SURFACE(((1.,0.66438972944168,1.),(1.,0.664393217905862,
1.),(1.,0.665747114157887,1.),(1.,0.66841287307604,1.)))
REPRESENTATION_ITEM('')
SURFACE()
);
#2113=(
BOUNDED_SURFACE()
B_SPLINE_SURFACE(3,2,((#136794,#136795,#136796),(#136797,#136798,#136799),
(#136800,#136801,#136802),(#136803,#136804,#136805),(#136806,#136807,#136808),
(#136809,#136810,#136811),(#136812,#136813,#136814),(#136815,#136816,#136817),
(#136818,#136819,#136820),(#136821,#136822,#136823),(#136824,#136825,#136826),
(#136827,#136828,#136829),(#136830,#136831,#136832),(#136833,#136834,#136835)),
 .UNSPECIFIED.,.F.,.F.,.F.)
B_SPLINE_SURFACE_WITH_KNOTS((4,2,2,2,2,2,4),(3,3),(0.00807831625971351,
0.00883535021604665,0.00921386719421322,0.00959238417237979,0.00997090115054636,
0.0103494181287129,0.0111064520850461),(0.,1.),.UNSPECIFIED.)
GEOMETRIC_REPRESENTATION_ITEM()
RATIONAL_B_SPLINE_SURFACE(((1.,0.707106781186548,1.),(1.,0.705861961062141,
1.),(1.,0.704642623504988,1.),(1.,0.702853606538468,1.),(1.,0.702268342990035,
1.),(1.,0.701150362247141,1.),(1.,0.700612993986993,1.),(1.,0.699582583564998,
1.),(1.,0.699087807793684,1.),(1.,0.698176683118393,1.),(1.,0.697755963868462,
1.),(1.,0.696598958196255,1.),(1.,0.695966377684547,1.),(1.,0.695533955710884,
1.)))
REPRESENTATION_ITEM('')
SURFACE()
);
#2114=(
BOUNDED_SURFACE()
B_SPLINE_SURFACE(3,2,((#136852,#136853,#136854),(#136855,#136856,#136857),
(#136858,#136859,#136860),(#136861,#136862,#136863)),.UNSPECIFIED.,.F.,
 .F.,.F.)
B_SPLINE_SURFACE_WITH_KNOTS((4,4),(3,3),(0.0316780996002149,0.0322721596780966),
(0.0854777406552673,1.),.UNSPECIFIED.)
GEOMETRIC_REPRESENTATION_ITEM()
RATIONAL_B_SPLINE_SURFACE(((0.96702384016161,0.807106741558701,1.),(0.966583587972177,
0.804531496904019,1.),(0.966125339262662,0.801850982035457,1.),(0.96564868941755,
0.799062830164232,1.)))
REPRESENTATION_ITEM('')
SURFACE()
);
#2115=(
BOUNDED_SURFACE()
B_SPLINE_SURFACE(3,2,((#136881,#136882,#136883),(#136884,#136885,#136886),
(#136887,#136888,#136889),(#136890,#136891,#136892),(#136893,#136894,#136895),
(#136896,#136897,#136898),(#136899,#136900,#136901),(#136902,#136903,#136904),
(#136905,#136906,#136907),(#136908,#136909,#136910),(#136911,#136912,#136913),
(#136914,#136915,#136916)),.UNSPECIFIED.,.F.,.F.,.F.)
B_SPLINE_SURFACE_WITH_KNOTS((4,2,2,2,2,4),(3,3),(0.00807807165860127,0.00885401549830484,
0.00962995933800841,0.0100179312578602,0.010405903177712,0.0111818470174155),
(0.,1.),.UNSPECIFIED.)
GEOMETRIC_REPRESENTATION_ITEM()
RATIONAL_B_SPLINE_SURFACE(((1.,0.707106781186548,1.),(1.,0.708323960348238,
1.),(1.,0.709510365636766,1.),(1.,0.711820403892163,1.),(1.,0.712901935204825,
1.),(1.,0.714375984986412,1.),(1.,0.714843782196838,1.),(1.,0.715700614088123,
1.),(1.,0.716094239791898,1.),(1.,0.71717000694229,1.),(1.,0.717742537382462,
1.),(1.,0.718120418666571,1.)))
REPRESENTATION_ITEM('')
SURFACE()
);
#2116=(
BOUNDED_SURFACE()
B_SPLINE_SURFACE(3,2,((#136965,#136966,#136967),(#136968,#136969,#136970),
(#136971,#136972,#136973),(#136974,#136975,#136976)),.UNSPECIFIED.,.F.,
 .F.,.F.)
B_SPLINE_SURFACE_WITH_KNOTS((4,4),(3,3),(-6.50599722386063E-5,0.000715659694624667),
(0.,1.00019764385803),.UNSPECIFIED.)
GEOMETRIC_REPRESENTATION_ITEM()
RATIONAL_B_SPLINE_SURFACE(((1.,0.755595413549798,1.00009661013077),(1.,
0.759778183122694,1.00009495673334),(1.,0.761738166948689,1.00009418197581),
(1.,0.761362101277913,1.00009433062995)))
REPRESENTATION_ITEM('')
SURFACE()
);
#2117=(
BOUNDED_SURFACE()
B_SPLINE_SURFACE(3,2,((#137090,#137091,#137092),(#137093,#137094,#137095),
(#137096,#137097,#137098),(#137099,#137100,#137101)),.UNSPECIFIED.,.F.,
 .F.,.F.)
B_SPLINE_SURFACE_WITH_KNOTS((4,4),(3,3),(-6.51392861930307E-5,0.000716532148123338),
(0.,1.00012789259532),.UNSPECIFIED.)
GEOMETRIC_REPRESENTATION_ITEM()
RATIONAL_B_SPLINE_SURFACE(((1.,0.610140967503591,1.00009972016695),(1.,
0.609358872291236,1.00009992021532),(1.,0.613297600455477,1.00009891274699),
(1.,0.621522254435954,1.0000968090023)))
REPRESENTATION_ITEM('')
SURFACE()
);
#2118=(
BOUNDED_SURFACE()
B_SPLINE_SURFACE(3,2,((#137171,#137172,#137173),(#137174,#137175,#137176),
(#137177,#137178,#137179),(#137180,#137181,#137182)),.UNSPECIFIED.,.F.,
 .F.,.F.)
B_SPLINE_SURFACE_WITH_KNOTS((4,4),(3,3),(-6.51938878740145E-5,0.000717132766614092),
(0.,1.00014042207762),.UNSPECIFIED.)
GEOMETRIC_REPRESENTATION_ITEM()
RATIONAL_B_SPLINE_SURFACE(((1.,0.795313299193259,1.00005748506358),(1.,
0.802685972468766,1.00005541449138),(1.,0.806177096184803,1.00005443402969),
(1.,0.805504544806421,1.00005462291181)))
REPRESENTATION_ITEM('')
SURFACE()
);
#2119=(
BOUNDED_SURFACE()
B_SPLINE_SURFACE(3,2,((#137256,#137257,#137258),(#137259,#137260,#137261),
(#137262,#137263,#137264),(#137265,#137266,#137267)),.UNSPECIFIED.,.F.,
 .F.,.F.)
B_SPLINE_SURFACE_WITH_KNOTS((4,4),(3,3),(-3.51472717058904E-5,0.00068864672702981),
(0.,1.00003514727171),.UNSPECIFIED.)
GEOMETRIC_REPRESENTATION_ITEM()
RATIONAL_B_SPLINE_SURFACE(((1.,0.550503741378763,1.00003159713427),(1.,
0.549804011257131,1.00003164632147),(1.,0.556145239310861,1.00003120056774),
(1.,0.568324276981185,1.00003034444785)))
REPRESENTATION_ITEM('')
SURFACE()
);
#2120=(
BOUNDED_SURFACE()
B_SPLINE_SURFACE(3,2,((#137355,#137356,#137357),(#137358,#137359,#137360),
(#137361,#137362,#137363),(#137364,#137365,#137366)),.UNSPECIFIED.,.F.,
 .F.,.F.)
B_SPLINE_SURFACE_WITH_KNOTS((4,4),(3,3),(0.,0.000921798889909707),(0.,1.),
 .UNSPECIFIED.)
GEOMETRIC_REPRESENTATION_ITEM()
RATIONAL_B_SPLINE_SURFACE(((1.,0.831289505264087,1.),(1.,0.831333394817592,
1.),(1.,0.824011622363235,1.),(1.,0.810617639934149,1.)))
REPRESENTATION_ITEM('')
SURFACE()
);
#2121=(
BOUNDED_SURFACE()
B_SPLINE_SURFACE(3,2,((#137438,#137439,#137440),(#137441,#137442,#137443),
(#137444,#137445,#137446),(#137447,#137448,#137449)),.UNSPECIFIED.,.F.,
 .F.,.F.)
B_SPLINE_SURFACE_WITH_KNOTS((4,4),(3,3),(-6.52563961816919E-5,0.000717820357998483),
(0.,1.00007660676733),.UNSPECIFIED.)
GEOMETRIC_REPRESENTATION_ITEM()
RATIONAL_B_SPLINE_SURFACE(((1.,0.590666869146129,1.00006271537583),(1.,
0.579347829852759,1.00006444960585),(1.,0.573596789585218,1.00006533074306),
(0.999999999999999,0.574723554882887,1.00006515810736)))
REPRESENTATION_ITEM('')
SURFACE()
);
#2122=(
BOUNDED_SURFACE()
B_SPLINE_SURFACE(3,2,((#137468,#137469,#137470),(#137471,#137472,#137473),
(#137474,#137475,#137476),(#137477,#137478,#137479)),.UNSPECIFIED.,.F.,
 .F.,.F.)
B_SPLINE_SURFACE_WITH_KNOTS((4,4),(3,3),(-6.51209638471727E-5,0.000716330602318899),
(0.,1.00017301493665),.UNSPECIFIED.)
GEOMETRIC_REPRESENTATION_ITEM()
RATIONAL_B_SPLINE_SURFACE(((1.,0.786579319308494,1.0000738499311),(1.,0.787125222591245,
1.00007366103225),(1.,0.784342967102359,1.00007462377577),(1.,0.778244201129582,
1.00007673413099)))
REPRESENTATION_ITEM('')
SURFACE()
);
#2123=(
BOUNDED_SURFACE()
B_SPLINE_SURFACE(3,2,((#137596,#137597,#137598),(#137599,#137600,#137601),
(#137602,#137603,#137604),(#137605,#137606,#137607),(#137608,#137609,#137610),
(#137611,#137612,#137613),(#137614,#137615,#137616),(#137617,#137618,#137619),
(#137620,#137621,#137622),(#137623,#137624,#137625),(#137626,#137627,#137628),
(#137629,#137630,#137631),(#137632,#137633,#137634),(#137635,#137636,#137637)),
 .UNSPECIFIED.,.F.,.F.,.F.)
B_SPLINE_SURFACE_WITH_KNOTS((4,2,2,2,2,2,4),(3,3),(0.00807568025026493,
0.00898700204274496,0.00944266293898498,0.009898323835225,0.010353984731465,
0.010809645627705,0.0117209674201851),(0.,1.),.UNSPECIFIED.)
GEOMETRIC_REPRESENTATION_ITEM()
RATIONAL_B_SPLINE_SURFACE(((1.,0.707106781186546,1.),(1.,0.707214557916128,
1.),(1.,0.707322930753557,1.),(1.,0.707478596210236,1.),(1.,0.707528365558662,
1.),(1.,0.70762361150633,1.),(1.,0.70766951928712,1.),(1.,0.70775397022188,
1.),(1.,0.707792549798564,1.),(1.,0.707862266510969,1.),(1.,0.707893578069266,
1.),(1.,0.707972242595767,1.),(1.,0.70800597758526,1.),(1.,0.708018339291814,
1.)))
REPRESENTATION_ITEM('')
SURFACE()
);
#2124=(
BOUNDED_SURFACE()
B_SPLINE_SURFACE(3,2,((#137654,#137655,#137656),(#137657,#137658,#137659),
(#137660,#137661,#137662),(#137663,#137664,#137665)),.UNSPECIFIED.,.F.,
 .F.,.F.)
B_SPLINE_SURFACE_WITH_KNOTS((4,4),(3,3),(0.0370067204754696,0.0375452288399126),
(0.,0.906596046514924),.UNSPECIFIED.)
GEOMETRIC_REPRESENTATION_ITEM()
RATIONAL_B_SPLINE_SURFACE(((1.,0.74984328911729,0.953268748425464),(1.,
0.745960134338133,0.952543344408728),(1.,0.741971405566699,0.951798218335465),
(1.,0.737872605222811,0.951032530022135)))
REPRESENTATION_ITEM('')
SURFACE()
);
#2125=(
BOUNDED_SURFACE()
B_SPLINE_SURFACE(3,2,((#137680,#137681,#137682),(#137683,#137684,#137685),
(#137686,#137687,#137688),(#137689,#137690,#137691),(#137692,#137693,#137694),
(#137695,#137696,#137697),(#137698,#137699,#137700),(#137701,#137702,#137703),
(#137704,#137705,#137706),(#137707,#137708,#137709),(#137710,#137711,#137712),
(#137713,#137714,#137715)),.UNSPECIFIED.,.F.,.F.,.F.)
B_SPLINE_SURFACE_WITH_KNOTS((4,2,2,2,2,4),(3,3),(0.00807589507756136,0.00894079878156724,
0.00980570248557312,0.010238154337576,0.010670606189579,0.0115355098935849),
(0.,1.),.UNSPECIFIED.)
GEOMETRIC_REPRESENTATION_ITEM()
RATIONAL_B_SPLINE_SURFACE(((1.,0.707106781186548,1.),(1.,0.706684802682679,
1.),(1.,0.706265611788784,1.),(1.,0.705449765784865,1.),(1.,0.705070572349072,
1.),(1.,0.704559600788765,1.),(1.,0.704402907652403,1.),(1.,0.7041166887103,
1.),(1.,0.703986299022118,1.),(1.,0.703645597188673,1.),(1.,0.703488957328521,
1.),(1.,0.703406029216022,1.)))
REPRESENTATION_ITEM('')
SURFACE()
);
#2126=(
BOUNDED_SURFACE()
B_SPLINE_SURFACE(3,2,((#137779,#137780,#137781),(#137782,#137783,#137784),
(#137785,#137786,#137787),(#137788,#137789,#137790)),.UNSPECIFIED.,.F.,
 .F.,.F.)
B_SPLINE_SURFACE_WITH_KNOTS((4,4),(3,3),(-6.50851503337948E-5,0.000715936653671955),
(0.,1.00015557324313),.UNSPECIFIED.)
GEOMETRIC_REPRESENTATION_ITEM()
RATIONAL_B_SPLINE_SURFACE(((0.999999999999999,0.64270572393334,1.00011117085856),
(1.,0.636685742162938,1.00011304395473),(1.,0.633761479841935,1.00011395382868),
(1.,0.634327701648552,1.00011377765075)))
REPRESENTATION_ITEM('')
SURFACE()
);
#2127=(
BOUNDED_SURFACE()
B_SPLINE_SURFACE(3,2,((#137844,#137845,#137846),(#137847,#137848,#137849),
(#137850,#137851,#137852),(#137853,#137854,#137855)),.UNSPECIFIED.,.F.,
 .F.,.F.)
B_SPLINE_SURFACE_WITH_KNOTS((4,4),(3,3),(0.,0.000650274811908555),(0.,1.),
 .UNSPECIFIED.)
GEOMETRIC_REPRESENTATION_ITEM()
RATIONAL_B_SPLINE_SURFACE(((1.,0.73939111071482,1.),(1.,0.73938749716724,
1.),(1.,0.738423154307972,1.),(1.,0.736495153922513,1.)))
REPRESENTATION_ITEM('')
SURFACE()
);
#2128=(
BOUNDED_SURFACE()
B_SPLINE_SURFACE(3,2,((#137904,#137905,#137906),(#137907,#137908,#137909),
(#137910,#137911,#137912),(#137913,#137914,#137915),(#137916,#137917,#137918),
(#137919,#137920,#137921),(#137922,#137923,#137924),(#137925,#137926,#137927),
(#137928,#137929,#137930),(#137931,#137932,#137933),(#137934,#137935,#137936),
(#137937,#137938,#137939)),.UNSPECIFIED.,.F.,.F.,.F.)
B_SPLINE_SURFACE_WITH_KNOTS((4,2,2,2,2,4),(3,3),(0.00807907499033046,0.00872002967587247,
0.00904050701864348,0.00936098436141448,0.0100019390469565,0.0106428937324985),
(0.,1.),.UNSPECIFIED.)
GEOMETRIC_REPRESENTATION_ITEM()
RATIONAL_B_SPLINE_SURFACE(((1.,0.707106781186548,1.),(1.,0.708291653108703,
1.),(1.,0.709443749235048,1.),(1.,0.71112469687116,1.),(1.,0.711680940824733,
1.),(1.,0.712751570007901,1.),(1.,0.713267249229028,1.),(1.,0.714757432797168,
1.),(1.,0.715686917775259,1.),(1.,0.717310091250008,1.),(1.,0.718010566750711,
1.),(1.,0.718598488256614,1.)))
REPRESENTATION_ITEM('')
SURFACE()
);
#2129=(
BOUNDED_SURFACE()
B_SPLINE_SURFACE(3,2,((#137954,#137955,#137956),(#137957,#137958,#137959),
(#137960,#137961,#137962),(#137963,#137964,#137965)),.UNSPECIFIED.,.F.,
 .F.,.F.)
B_SPLINE_SURFACE_WITH_KNOTS((4,4),(3,3),(0.0283524505452003,0.0289409470909155),
(0.,0.920633110097118),.UNSPECIFIED.)
GEOMETRIC_REPRESENTATION_ITEM()
RATIONAL_B_SPLINE_SURFACE(((1.,0.864312975626627,0.978461885750618),(1.,
0.86308788835206,0.978267423016934),(1.,0.861770510916135,0.978058310717099),
(1.,0.860360064997711,0.977834425305256)))
REPRESENTATION_ITEM('')
SURFACE()
);
#2130=(
BOUNDED_SURFACE()
B_SPLINE_SURFACE(3,2,((#137981,#137982,#137983),(#137984,#137985,#137986),
(#137987,#137988,#137989),(#137990,#137991,#137992),(#137993,#137994,#137995),
(#137996,#137997,#137998),(#137999,#138000,#138001),(#138002,#138003,#138004),
(#138005,#138006,#138007),(#138008,#138009,#138010)),.UNSPECIFIED.,.F.,
 .F.,.F.)
B_SPLINE_SURFACE_WITH_KNOTS((4,2,2,2,4),(3,3),(0.00807856278467327,0.00871080510931882,
0.00934304743396438,0.00997528975860994,0.0106075320832555),(0.,1.),
 .UNSPECIFIED.)
GEOMETRIC_REPRESENTATION_ITEM()
RATIONAL_B_SPLINE_SURFACE(((1.,0.707106781186548,1.),(1.,0.706030220592194,
1.),(1.,0.704978540375902,1.),(1.,0.702923837367757,1.),(1.,0.701922380471311,
1.),(1.,0.700080728636545,1.),(1.,0.699214393311896,1.),(1.,0.697689255248067,
1.),(1.,0.697026914527849,1.),(1.,0.696465765714756,1.)))
REPRESENTATION_ITEM('')
SURFACE()
);
#2131=(
BOUNDED_SURFACE()
B_SPLINE_SURFACE(3,2,((#138152,#138153,#138154),(#138155,#138156,#138157),
(#138158,#138159,#138160),(#138161,#138162,#138163)),.UNSPECIFIED.,.F.,
 .F.,.F.)
B_SPLINE_SURFACE_WITH_KNOTS((4,4),(3,3),(0.00489732211254449,0.00554953903232782),
(0.,1.),.UNSPECIFIED.)
GEOMETRIC_REPRESENTATION_ITEM()
RATIONAL_B_SPLINE_SURFACE(((1.,0.565840417962196,1.),(1.,0.555341099754398,
1.),(1.,0.549566935115175,1.),(1.,0.549598954535096,1.)))
REPRESENTATION_ITEM('')
SURFACE()
);
#2132=(
BOUNDED_SURFACE()
B_SPLINE_SURFACE(3,2,((#138187,#138188,#138189),(#138190,#138191,#138192),
(#138193,#138194,#138195),(#138196,#138197,#138198)),.UNSPECIFIED.,.F.,
 .F.,.F.)
B_SPLINE_SURFACE_WITH_KNOTS((4,4),(3,3),(-6.51926395977061E-5,0.000717119035574751),
(0.,1.00013881592609),.UNSPECIFIED.)
GEOMETRIC_REPRESENTATION_ITEM()
RATIONAL_B_SPLINE_SURFACE(((1.,0.806095432842625,1.00005383408413),(1.,
0.806773570717767,1.00005364581145),(1.,0.803329499666744,1.00005460199528),
(0.999999999999999,0.795829536739348,1.00005668422387)))
REPRESENTATION_ITEM('')
SURFACE()
);
#2133=(
BOUNDED_SURFACE()
B_SPLINE_SURFACE(3,2,((#138272,#138273,#138274),(#138275,#138276,#138277),
(#138278,#138279,#138280),(#138281,#138282,#138283)),.UNSPECIFIED.,.F.,
 .F.,.F.)
B_SPLINE_SURFACE_WITH_KNOTS((4,4),(3,3),(-6.51439314691727E-5,0.000716583246160882),
(0.,1.00012692018127),.UNSPECIFIED.)
GEOMETRIC_REPRESENTATION_ITEM()
RATIONAL_B_SPLINE_SURFACE(((1.,0.620818202688319,1.0000962516449),(1.,0.612618963298309,
1.0000983329428),(1.,0.608569430840875,1.00009936087759),(1.,0.609356995261979,
1.00009916096195)))
REPRESENTATION_ITEM('')
SURFACE()
);
#2134=(
BOUNDED_SURFACE()
B_SPLINE_SURFACE(3,2,((#138369,#138370,#138371),(#138372,#138373,#138374),
(#138375,#138376,#138377),(#138378,#138379,#138380)),.UNSPECIFIED.,.F.,
 .F.,.F.)
B_SPLINE_SURFACE_WITH_KNOTS((4,4),(3,3),(0.,0.00065060314950297),(0.,1.),
 .UNSPECIFIED.)
GEOMETRIC_REPRESENTATION_ITEM()
RATIONAL_B_SPLINE_SURFACE(((1.,0.762081632339421,1.),(1.,0.762075781187422,
1.),(1.,0.760455646763466,1.),(1.,0.757216058458816,1.)))
REPRESENTATION_ITEM('')
SURFACE()
);
#2135=(
BOUNDED_SURFACE()
B_SPLINE_SURFACE(3,2,((#138521,#138522,#138523),(#138524,#138525,#138526),
(#138527,#138528,#138529),(#138530,#138531,#138532),(#138533,#138534,#138535),
(#138536,#138537,#138538),(#138539,#138540,#138541),(#138542,#138543,#138544),
(#138545,#138546,#138547),(#138548,#138549,#138550),(#138551,#138552,#138553),
(#138554,#138555,#138556),(#138557,#138558,#138559),(#138560,#138561,#138562)),
 .UNSPECIFIED.,.F.,.F.,.F.)
B_SPLINE_SURFACE_WITH_KNOTS((4,2,2,2,2,2,4),(3,3),(0.00807895877935271,
0.00883634587130868,0.00921503941728666,0.00959373296326465,0.00997242650924264,
0.0103511200552206,0.0111085071471766),(0.,1.),.UNSPECIFIED.)
GEOMETRIC_REPRESENTATION_ITEM()
RATIONAL_B_SPLINE_SURFACE(((1.,0.707106781186548,1.),(1.,0.708496200821205,
1.),(1.,0.70985049824013,1.),(1.,0.711828637936002,1.),(1.,0.712474210732742,
1.),(1.,0.71370482119381,1.),(1.,0.714294998379545,1.),(1.,0.715424510819791,
1.),(1.,0.715965704866287,1.),(1.,0.716960611510995,1.),(1.,0.71741913219781,
1.),(1.,0.71867831515119,1.),(1.,0.719364099598229,1.),(1.,0.719832136235989,
1.)))
REPRESENTATION_ITEM('')
SURFACE()
);
#2136=(
BOUNDED_SURFACE()
B_SPLINE_SURFACE(3,2,((#138579,#138580,#138581),(#138582,#138583,#138584),
(#138585,#138586,#138587),(#138588,#138589,#138590)),.UNSPECIFIED.,.F.,
 .F.,.F.)
B_SPLINE_SURFACE_WITH_KNOTS((4,4),(3,3),(0.0154746506919765,0.0160816000283851),
(0.0845570889131019,1.),.UNSPECIFIED.)
GEOMETRIC_REPRESENTATION_ITEM()
RATIONAL_B_SPLINE_SURFACE(((0.967520924037566,0.807945871955148,1.),(0.96800421232544,
0.810803635237245,1.),(0.968468725982054,0.813550381031034,1.),(0.968914883389343,
0.81618858329783,1.)))
REPRESENTATION_ITEM('')
SURFACE()
);
#2137=(
BOUNDED_SURFACE()
B_SPLINE_SURFACE(3,2,((#138610,#138611,#138612),(#138613,#138614,#138615),
(#138616,#138617,#138618),(#138619,#138620,#138621),(#138622,#138623,#138624),
(#138625,#138626,#138627),(#138628,#138629,#138630),(#138631,#138632,#138633),
(#138634,#138635,#138636),(#138637,#138638,#138639),(#138640,#138641,#138642),
(#138643,#138644,#138645),(#138646,#138647,#138648),(#138649,#138650,#138651)),
 .UNSPECIFIED.,.F.,.F.,.F.)
B_SPLINE_SURFACE_WITH_KNOTS((4,2,2,2,2,2,4),(3,3),(0.00807922902311453,
0.00881773053780572,0.00918698129515131,0.0095562320524969,0.0099254828098425,
0.0102947335671881,0.0110332350818793),(0.,1.),.UNSPECIFIED.)
GEOMETRIC_REPRESENTATION_ITEM()
RATIONAL_B_SPLINE_SURFACE(((1.,0.707106781186548,1.),(1.,0.705699386801107,
1.),(1.,0.704319784944778,1.),(1.,0.702293838625036,1.),(1.,0.701628229397446,
1.),(1.,0.700355977320158,1.),(1.,0.699743668156969,1.),(1.,0.698567591087498,
1.),(1.,0.698000119405105,1.),(1.,0.696949115865192,1.),(1.,0.696462203809247,
1.),(1.,0.695116916536575,1.),(1.,0.694367821279467,1.),(1.,0.693837065201558,
1.)))
REPRESENTATION_ITEM('')
SURFACE()
);
#2138=(
BOUNDED_SURFACE()
B_SPLINE_SURFACE(3,2,((#138691,#138692,#138693),(#138694,#138695,#138696),
(#138697,#138698,#138699),(#138700,#138701,#138702)),.UNSPECIFIED.,.F.,
 .F.,.F.)
B_SPLINE_SURFACE_WITH_KNOTS((4,4),(3,3),(0.,0.0006503810773206),(0.,1.),
 .UNSPECIFIED.)
GEOMETRIC_REPRESENTATION_ITEM()
RATIONAL_B_SPLINE_SURFACE(((1.,0.667763418073535,1.),(1.,0.665075430476096,
1.),(1.,0.663677894706716,1.),(1.,0.663670476501713,1.)))
REPRESENTATION_ITEM('')
SURFACE()
);
#2139=(
BOUNDED_SURFACE()
B_SPLINE_SURFACE(3,2,((#138804,#138805,#138806),(#138807,#138808,#138809),
(#138810,#138811,#138812),(#138813,#138814,#138815)),.UNSPECIFIED.,.F.,
 .F.,.F.)
B_SPLINE_SURFACE_WITH_KNOTS((4,4),(3,3),(0.,0.000650124307745721),(0.,1.),
 .UNSPECIFIED.)
GEOMETRIC_REPRESENTATION_ITEM()
RATIONAL_B_SPLINE_SURFACE(((1.,0.715240287646145,1.),(1.,0.715239393380683,
1.),(1.,0.714992351911572,1.),(1.,0.71449972514277,1.)))
REPRESENTATION_ITEM('')
SURFACE()
);
#2140=(
BOUNDED_SURFACE()
B_SPLINE_SURFACE(3,2,((#138896,#138897,#138898),(#138899,#138900,#138901),
(#138902,#138903,#138904),(#138905,#138906,#138907),(#138908,#138909,#138910),
(#138911,#138912,#138913),(#138914,#138915,#138916),(#138917,#138918,#138919),
(#138920,#138921,#138922),(#138923,#138924,#138925)),.UNSPECIFIED.,.F.,
 .F.,.F.)
B_SPLINE_SURFACE_WITH_KNOTS((4,2,2,2,4),(3,3),(0.00807569195610403,0.00870260410927289,
0.00932951626244174,0.0099564284156106,0.0105833405687795),(0.,1.),
 .UNSPECIFIED.)
GEOMETRIC_REPRESENTATION_ITEM()
RATIONAL_B_SPLINE_SURFACE(((1.,0.707106781186548,1.),(1.,0.707206112905989,
1.),(1.,0.707302756119535,1.),(1.,0.707490889447615,1.),(1.,0.707582303244654,
1.),(1.,0.707749976398179,1.),(1.,0.707828611057685,1.),(1.,0.70796711497316,
1.),(1.,0.708027180199908,1.),(1.,0.708078164615097,1.)))
REPRESENTATION_ITEM('')
SURFACE()
);
#2141=(
BOUNDED_SURFACE()
B_SPLINE_SURFACE(3,2,((#138938,#138939,#138940),(#138941,#138942,#138943),
(#138944,#138945,#138946),(#138947,#138948,#138949)),.UNSPECIFIED.,.F.,
 .F.,.F.)
B_SPLINE_SURFACE_WITH_KNOTS((4,4),(3,3),(0.0237206528291238,0.0242322821884044),
(0.0789621674491627,1.),.UNSPECIFIED.)
GEOMETRIC_REPRESENTATION_ITEM()
RATIONAL_B_SPLINE_SURFACE(((0.978911250155251,0.866462949751686,1.),(0.978926955451664,
0.866562397986968,1.),(0.9789317875721,0.866592995680722,1.),(0.978925751378407,
0.866554773618892,1.)))
REPRESENTATION_ITEM('')
SURFACE()
);
#2142=(
BOUNDED_SURFACE()
B_SPLINE_SURFACE(3,2,((#138962,#138963,#138964),(#138965,#138966,#138967),
(#138968,#138969,#138970),(#138971,#138972,#138973),(#138974,#138975,#138976),
(#138977,#138978,#138979),(#138980,#138981,#138982),(#138983,#138984,#138985),
(#138986,#138987,#138988),(#138989,#138990,#138991)),.UNSPECIFIED.,.F.,
 .F.,.F.)
B_SPLINE_SURFACE_WITH_KNOTS((4,2,2,2,4),(3,3),(0.00807567041695258,0.00870229794915108,
0.00932892548134959,0.00995555301354809,0.0105821805457466),(0.,1.),
 .UNSPECIFIED.)
GEOMETRIC_REPRESENTATION_ITEM()
RATIONAL_B_SPLINE_SURFACE(((1.,0.707106781186548,1.),(1.,0.707144476742774,
1.),(1.,0.707181156772813,1.),(1.,0.707252569458078,1.),(1.,0.707287275051322,
1.),(1.,0.707350941456054,1.),(1.,0.707380803865577,1.),(1.,0.707433415861318,
1.),(1.,0.707456236659423,1.),(1.,0.707475611987371,1.)))
REPRESENTATION_ITEM('')
SURFACE()
);
#2143=(
BOUNDED_SURFACE()
B_SPLINE_SURFACE(3,2,((#139022,#139023,#139024),(#139025,#139026,#139027),
(#139028,#139029,#139030),(#139031,#139032,#139033)),.UNSPECIFIED.,.F.,
 .F.,.F.)
B_SPLINE_SURFACE_WITH_KNOTS((4,4),(3,3),(0.,0.000650121463573334),(0.,1.),
 .UNSPECIFIED.)
GEOMETRIC_REPRESENTATION_ITEM()
RATIONAL_B_SPLINE_SURFACE(((1.,0.713284154090124,1.),(1.,0.713692564168438,
1.),(1.,0.713902215282654,1.),(1.,0.713903527556066,1.)))
REPRESENTATION_ITEM('')
SURFACE()
);
#2144=(
BOUNDED_SURFACE()
B_SPLINE_SURFACE(3,2,((#139104,#139105,#139106),(#139107,#139108,#139109),
(#139110,#139111,#139112),(#139113,#139114,#139115)),.UNSPECIFIED.,.F.,
 .F.,.F.)
B_SPLINE_SURFACE_WITH_KNOTS((4,4),(3,3),(0.,0.000650359837711272),(0.,1.),
 .UNSPECIFIED.)
GEOMETRIC_REPRESENTATION_ITEM()
RATIONAL_B_SPLINE_SURFACE(((1.,0.665108204576639,1.),(1.,0.66511166059484,
1.),(1.,0.666441892349684,1.),(1.,0.669061697655964,1.)))
REPRESENTATION_ITEM('')
SURFACE()
);
#2145=(
BOUNDED_SURFACE()
B_SPLINE_SURFACE(3,2,((#139241,#139242,#139243),(#139244,#139245,#139246),
(#139247,#139248,#139249),(#139250,#139251,#139252),(#139253,#139254,#139255),
(#139256,#139257,#139258),(#139259,#139260,#139261),(#139262,#139263,#139264),
(#139265,#139266,#139267),(#139268,#139269,#139270),(#139271,#139272,#139273),
(#139274,#139275,#139276),(#139277,#139278,#139279),(#139280,#139281,#139282)),
 .UNSPECIFIED.,.F.,.F.,.F.)
B_SPLINE_SURFACE_WITH_KNOTS((4,2,2,2,2,2,4),(3,3),(0.00807931853788568,
0.00881187542632408,0.00917815387054328,0.00954443231476248,0.00991071075898168,
0.0102769892032009,0.0110095460916393),(0.,1.),.UNSPECIFIED.)
GEOMETRIC_REPRESENTATION_ITEM()
RATIONAL_B_SPLINE_SURFACE(((1.,0.707106781186552,1.),(1.,0.705694108475444,
1.),(1.,0.704309639709031,1.),(1.,0.702276829363826,1.),(1.,0.701608277715413,
1.),(1.,0.700330266875156,1.),(1.,0.699715065357364,1.),(1.,0.698533028725346,
1.),(1.,0.697962156582885,1.),(1.,0.696902668323859,1.),(1.,0.696411414935025,
1.),(1.,0.695052392645847,1.),(1.,0.69429223033984,1.),(1.,0.69374733452232,
1.)))
REPRESENTATION_ITEM('')
SURFACE()
);
#2146=(
BOUNDED_SURFACE()
B_SPLINE_SURFACE(3,2,((#139299,#139300,#139301),(#139302,#139303,#139304),
(#139305,#139306,#139307),(#139308,#139309,#139310)),.UNSPECIFIED.,.F.,
 .F.,.F.)
B_SPLINE_SURFACE_WITH_KNOTS((4,4),(3,3),(0.0318721040045715,0.0324798405467945),
(0.0842204782052437,1.),.UNSPECIFIED.)
GEOMETRIC_REPRESENTATION_ITEM()
RATIONAL_B_SPLINE_SURFACE(((0.96952117077485,0.819053335514945,1.),(0.96908988447244,
0.816492875686171,1.),(0.968640411425079,0.813824444819121,1.),(0.968172353055208,
0.811045676639188,1.)))
REPRESENTATION_ITEM('')
SURFACE()
);
#2147=(
BOUNDED_SURFACE()
B_SPLINE_SURFACE(3,2,((#139330,#139331,#139332),(#139333,#139334,#139335),
(#139336,#139337,#139338),(#139339,#139340,#139341),(#139342,#139343,#139344),
(#139345,#139346,#139347),(#139348,#139349,#139350),(#139351,#139352,#139353),
(#139354,#139355,#139356),(#139357,#139358,#139359),(#139360,#139361,#139362),
(#139363,#139364,#139365),(#139366,#139367,#139368),(#139369,#139370,#139371)),
 .UNSPECIFIED.,.F.,.F.,.F.)
B_SPLINE_SURFACE_WITH_KNOTS((4,2,2,2,2,2,4),(3,3),(0.00807909221698663,
0.00882982802565525,0.00920519592998956,0.00958056383432386,0.00995593173865817,
0.0103312996429925,0.0110820354516611),(0.,1.),.UNSPECIFIED.)
GEOMETRIC_REPRESENTATION_ITEM()
RATIONAL_B_SPLINE_SURFACE(((1.,0.707106781186556,1.),(1.,0.708510771074171,
1.),(1.,0.709878889431803,1.),(1.,0.711876867675041,1.),(1.,0.712529775389558,
1.),(1.,0.713774284861137,1.),(1.,0.714371256763372,1.),(1.,0.715514222535529,
1.),(1.,0.716062813357328,1.),(1.,0.717072969030255,1.),(1.,0.717538977439758,
1.),(1.,0.718820706504871,1.),(1.,0.719523481892828,1.),(1.,0.720009098745653,
1.)))
REPRESENTATION_ITEM('')
SURFACE()
);
#2148=(
BOUNDED_SURFACE()
B_SPLINE_SURFACE(3,2,((#139411,#139412,#139413),(#139414,#139415,#139416),
(#139417,#139418,#139419),(#139420,#139421,#139422)),.UNSPECIFIED.,.F.,
 .F.,.F.)
B_SPLINE_SURFACE_WITH_KNOTS((4,4),(3,3),(-6.50587846610038E-5,0.000715646631271042),
(0.,1.00019802018696),.UNSPECIFIED.)
GEOMETRIC_REPRESENTATION_ITEM()
RATIONAL_B_SPLINE_SURFACE(((1.,0.755032712249889,1.00009701693624),(1.,
0.75916874975514,1.0000953788984),(1.,0.761106752395798,1.00009461137111),
(1.,0.760734912009425,1.00009475863492)))
REPRESENTATION_ITEM('')
SURFACE()
);
#2149=(
BOUNDED_SURFACE()
B_SPLINE_SURFACE(3,2,((#139534,#139535,#139536),(#139537,#139538,#139539),
(#139540,#139541,#139542),(#139543,#139544,#139545)),.UNSPECIFIED.,.F.,
 .F.,.F.)
B_SPLINE_SURFACE_WITH_KNOTS((4,4),(3,3),(-6.5137241604418E-5,0.000716509657648589),
(0.,1.00012888352926),.UNSPECIFIED.)
GEOMETRIC_REPRESENTATION_ITEM()
RATIONAL_B_SPLINE_SURFACE(((1.,0.610922104164594,1.00010029146475),(1.,
0.610147227047923,1.00010049120254),(1.,0.614050298485334,1.0000994851193),
(1.,0.622205101827845,1.00009738307963)))
REPRESENTATION_ITEM('')
SURFACE()
);
#2150=(
BOUNDED_SURFACE()
B_SPLINE_SURFACE(3,2,((#139622,#139623,#139624),(#139625,#139626,#139627),
(#139628,#139629,#139630),(#139631,#139632,#139633)),.UNSPECIFIED.,.F.,
 .F.,.F.)
B_SPLINE_SURFACE_WITH_KNOTS((4,4),(3,3),(-6.51913040321435E-5,0.00071710434435357),
(0.,1.00014170095501),.UNSPECIFIED.)
GEOMETRIC_REPRESENTATION_ITEM()
RATIONAL_B_SPLINE_SURFACE(((1.,0.794778369766658,1.00005816020198),(1.,
0.80210956676765,1.00005608252675),(1.,0.805580179391815,1.0000550989485),
(1.,0.804911641151859,1.00005528841352)))
REPRESENTATION_ITEM('')
SURFACE()
);
#2151=(
BOUNDED_SURFACE()
B_SPLINE_SURFACE(3,2,((#139715,#139716,#139717),(#139718,#139719,#139720),
(#139721,#139722,#139723),(#139724,#139725,#139726)),.UNSPECIFIED.,.F.,
 .F.,.F.)
B_SPLINE_SURFACE_WITH_KNOTS((4,4),(3,3),(-3.67368196064713E-5,0.0006901971826107),
(0.,1.00003673681961),.UNSPECIFIED.)
GEOMETRIC_REPRESENTATION_ITEM()
RATIONAL_B_SPLINE_SURFACE(((1.,0.551374288254534,1.00003296216369),(1.,
0.550645752158029,1.00003301569188),(1.,0.556973926885096,1.00003255073786),
(0.999999999999999,0.569158328192581,1.00003165550555)))
REPRESENTATION_ITEM('')
SURFACE()
);
#2152=(
BOUNDED_SURFACE()
B_SPLINE_SURFACE(3,2,((#139820,#139821,#139822),(#139823,#139824,#139825),
(#139826,#139827,#139828),(#139829,#139830,#139831),(#139832,#139833,#139834),
(#139835,#139836,#139837),(#139838,#139839,#139840),(#139841,#139842,#139843),
(#139844,#139845,#139846),(#139847,#139848,#139849)),.UNSPECIFIED.,.F.,
 .F.,.F.)
B_SPLINE_SURFACE_WITH_KNOTS((4,2,2,2,4),(3,3),(1.18015353016497E-15,0.392699081698726,
0.785398163397449,1.17809724509617,1.5707963267949),(0.,1.),
 .UNSPECIFIED.)
GEOMETRIC_REPRESENTATION_ITEM()
RATIONAL_B_SPLINE_SURFACE(((1.,0.67559020761567,1.),(1.,0.675585785528194,
1.),(1.,0.676431027860885,1.),(1.,0.679650528045421,1.),(1.,0.682027045382314,
1.),(1.,0.687915714942951,1.),(1.,0.691424416305301,1.),(1.,0.699004971484679,
1.),(1.,0.703073130220216,1.),(1.,0.707106781186548,1.)))
REPRESENTATION_ITEM('')
SURFACE()
);
#2153=(
BOUNDED_SURFACE()
B_SPLINE_SURFACE(3,2,((#139862,#139863,#139864),(#139865,#139866,#139867),
(#139868,#139869,#139870),(#139871,#139872,#139873),(#139874,#139875,#139876),
(#139877,#139878,#139879),(#139880,#139881,#139882),(#139883,#139884,#139885),
(#139886,#139887,#139888),(#139889,#139890,#139891)),.UNSPECIFIED.,.F.,
 .F.,.F.)
B_SPLINE_SURFACE_WITH_KNOTS((4,2,2,2,4),(3,3),(4.71238898038469,5.10508806208341,
5.49778714378214,5.89048622548086,6.28318530717959),(0.,1.),
 .UNSPECIFIED.)
GEOMETRIC_REPRESENTATION_ITEM()
RATIONAL_B_SPLINE_SURFACE(((1.,0.707106781186548,1.),(1.,0.71114164850559,
1.),(1.,0.71513624913423,1.),(1.,0.722468048845566,1.),(1.,0.725801833007554,
1.),(1.,0.731338116836806,1.),(1.,0.733539335051299,1.),(1.,0.736509240245015,
1.),(1.,0.737280525008035,1.),(1.,0.73727733681012,1.)))
REPRESENTATION_ITEM('')
SURFACE()
);
#2154=(
BOUNDED_SURFACE()
B_SPLINE_SURFACE(3,2,((#140139,#140140,#140141),(#140142,#140143,#140144),
(#140145,#140146,#140147),(#140148,#140149,#140150),(#140151,#140152,#140153),
(#140154,#140155,#140156),(#140157,#140158,#140159),(#140160,#140161,#140162),
(#140163,#140164,#140165),(#140166,#140167,#140168)),.UNSPECIFIED.,.F.,
 .F.,.F.)
B_SPLINE_SURFACE_WITH_KNOTS((4,2,2,2,4),(3,3),(4.71238898038469,5.10508806208342,
5.49778714378214,5.89048622548086,6.28318530717959),(0.,1.),
 .UNSPECIFIED.)
GEOMETRIC_REPRESENTATION_ITEM()
RATIONAL_B_SPLINE_SURFACE(((1.,0.707106781186548,1.),(1.,0.711141648505921,
1.),(1.,0.715136249133786,1.),(1.,0.722468048846019,1.),(1.,0.725801833007554,
1.),(1.,0.731338116836806,1.),(1.,0.733539335051135,1.),(1.,0.736509240245178,
1.),(1.,0.737280525007913,1.),(1.,0.73727733681012,1.)))
REPRESENTATION_ITEM('')
SURFACE()
);
#2155=(
BOUNDED_SURFACE()
B_SPLINE_SURFACE(3,2,((#140170,#140171,#140172),(#140173,#140174,#140175),
(#140176,#140177,#140178),(#140179,#140180,#140181),(#140182,#140183,#140184),
(#140185,#140186,#140187)),.UNSPECIFIED.,.F.,.F.,.F.)
B_SPLINE_SURFACE_WITH_KNOTS((4,2,4),(3,3),(0.,0.00070803381389838,0.00141606762779676),
(0.,1.),.UNSPECIFIED.)
GEOMETRIC_REPRESENTATION_ITEM()
RATIONAL_B_SPLINE_SURFACE(((1.,0.800108937437262,1.),(1.,0.794442999342884,
1.),(1.,0.785169683107043,1.),(1.,0.763289065038484,1.),(1.,0.750458153314313,
1.),(1.,0.737277336810115,1.)))
REPRESENTATION_ITEM('')
SURFACE()
);
#2156=(
BOUNDED_SURFACE()
B_SPLINE_SURFACE(3,2,((#140318,#140319,#140320),(#140321,#140322,#140323),
(#140324,#140325,#140326),(#140327,#140328,#140329),(#140330,#140331,#140332),
(#140333,#140334,#140335),(#140336,#140337,#140338),(#140339,#140340,#140341),
(#140342,#140343,#140344),(#140345,#140346,#140347)),.UNSPECIFIED.,.F.,
 .F.,.F.)
B_SPLINE_SURFACE_WITH_KNOTS((4,2,2,2,4),(3,3),(0.,0.392699081698724,0.785398163397448,
1.17809724509617,1.5707963267949),(0.,1.),.UNSPECIFIED.)
GEOMETRIC_REPRESENTATION_ITEM()
RATIONAL_B_SPLINE_SURFACE(((1.,0.67559020761567,1.),(1.,0.675585785528568,
1.),(1.,0.676431027860386,1.),(1.,0.679650528045925,1.),(1.,0.682027045382314,
1.),(1.,0.687915714942951,1.),(1.,0.69142441630529,1.),(1.,0.69900497148469,
1.),(1.,0.703073130220208,1.),(1.,0.707106781186548,1.)))
REPRESENTATION_ITEM('')
SURFACE()
);
#2157=(
BOUNDED_SURFACE()
B_SPLINE_SURFACE(3,2,((#140602,#140603,#140604),(#140605,#140606,#140607),
(#140608,#140609,#140610),(#140611,#140612,#140613),(#140614,#140615,#140616),
(#140617,#140618,#140619),(#140620,#140621,#140622),(#140623,#140624,#140625),
(#140626,#140627,#140628),(#140629,#140630,#140631)),.UNSPECIFIED.,.F.,
 .F.,.F.)
B_SPLINE_SURFACE_WITH_KNOTS((4,2,2,2,4),(3,3),(3.1415926535898,3.53429173528852,
3.92699081698724,4.31968989868597,4.71238898038469),(0.,1.),
 .UNSPECIFIED.)
GEOMETRIC_REPRESENTATION_ITEM()
RATIONAL_B_SPLINE_SURFACE(((1.,0.737277336810125,1.),(1.,0.737280525008216,
1.),(1.,0.736509240244793,1.),(1.,0.733539335051535,1.),(1.,0.731338116837053,
1.),(1.,0.725801833007317,1.),(1.,0.722468048845379,1.),(1.,0.715136249134436,
1.),(1.,0.711141648505436,1.),(1.,0.707106781186548,1.)))
REPRESENTATION_ITEM('')
SURFACE()
);
#2158=(
BOUNDED_SURFACE()
B_SPLINE_SURFACE(3,2,((#140644,#140645,#140646),(#140647,#140648,#140649),
(#140650,#140651,#140652),(#140653,#140654,#140655),(#140656,#140657,#140658),
(#140659,#140660,#140661),(#140662,#140663,#140664),(#140665,#140666,#140667),
(#140668,#140669,#140670),(#140671,#140672,#140673)),.UNSPECIFIED.,.F.,
 .F.,.F.)
B_SPLINE_SURFACE_WITH_KNOTS((4,2,2,2,4),(3,3),(1.5707963267949,1.96349540849362,
2.35619449019234,2.74889357189106,3.14159265358979),(0.,1.),
 .UNSPECIFIED.)
GEOMETRIC_REPRESENTATION_ITEM()
RATIONAL_B_SPLINE_SURFACE(((1.,0.707106781186548,1.),(1.,0.703073130219847,
1.),(1.,0.699004971485165,1.),(1.,0.691424416304824,1.),(1.,0.687915714942826,
1.),(1.,0.682027045382428,1.),(1.,0.679650528045614,1.),(1.,0.676431027860685,
1.),(1.,0.675585785528338,1.),(1.,0.675590207615664,1.)))
REPRESENTATION_ITEM('')
SURFACE()
);
#2159=(
BOUNDED_SURFACE()
B_SPLINE_SURFACE(3,2,((#140835,#140836,#140837),(#140838,#140839,#140840),
(#140841,#140842,#140843),(#140844,#140845,#140846),(#140847,#140848,#140849),
(#140850,#140851,#140852),(#140853,#140854,#140855),(#140856,#140857,#140858),
(#140859,#140860,#140861),(#140862,#140863,#140864),(#140865,#140866,#140867),
(#140868,#140869,#140870)),.UNSPECIFIED.,.F.,.F.,.F.)
B_SPLINE_SURFACE_WITH_KNOTS((4,2,2,2,2,4),(3,3),(0.00373720614906648,0.00431441150266452,
0.00489161685626256,0.00518021953306157,0.00546882220986059,0.00604602756345863),
(0.,1.),.UNSPECIFIED.)
GEOMETRIC_REPRESENTATION_ITEM()
RATIONAL_B_SPLINE_SURFACE(((1.,0.702399276808564,1.),(1.,0.697901374758016,
1.),(1.,0.693446103155503,1.),(1.,0.685742881148842,1.),(1.,0.682394877642487,
1.),(1.,0.6786862147386,1.),(1.,0.677675780152448,1.),(1.,0.676083839724519,
1.),(1.,0.675500346164623,1.),(1.,0.674441428307327,1.),(1.,0.674627601820987,
1.),(1.,0.675590207615657,1.)))
REPRESENTATION_ITEM('')
SURFACE()
);
#2160=(
BOUNDED_SURFACE()
B_SPLINE_SURFACE(3,2,((#140872,#140873,#140874),(#140875,#140876,#140877),
(#140878,#140879,#140880),(#140881,#140882,#140883),(#140884,#140885,#140886),
(#140887,#140888,#140889),(#140890,#140891,#140892),(#140893,#140894,#140895),
(#140896,#140897,#140898),(#140899,#140900,#140901)),.UNSPECIFIED.,.F.,
 .F.,.F.)
B_SPLINE_SURFACE_WITH_KNOTS((4,2,2,2,4),(3,3),(1.5707963267949,1.96349540849362,
2.35619449019234,2.74889357189107,3.1415926535898),(0.,1.),
 .UNSPECIFIED.)
GEOMETRIC_REPRESENTATION_ITEM()
RATIONAL_B_SPLINE_SURFACE(((1.,0.707106781186548,1.),(1.,0.711141648505595,
1.),(1.,0.715136249134216,1.),(1.,0.722468048845599,1.),(1.,0.725801833007891,
1.),(1.,0.731338116836469,1.),(1.,0.733539335051304,1.),(1.,0.73650924024502,
1.),(1.,0.737280525008041,1.),(1.,0.737277336810125,1.)))
REPRESENTATION_ITEM('')
SURFACE()
);
#2161=(
BOUNDED_SURFACE()
B_SPLINE_SURFACE(3,2,((#140998,#140999,#141000),(#141001,#141002,#141003),
(#141004,#141005,#141006),(#141007,#141008,#141009),(#141010,#141011,#141012),
(#141013,#141014,#141015),(#141016,#141017,#141018),(#141019,#141020,#141021),
(#141022,#141023,#141024),(#141025,#141026,#141027)),.UNSPECIFIED.,.F.,
 .F.,.F.)
B_SPLINE_SURFACE_WITH_KNOTS((4,2,2,2,4),(3,3),(-1.77635683940025E-15,0.392699081698723,
0.785398163397447,1.17809724509617,1.5707963267949),(0.,1.),
 .UNSPECIFIED.)
GEOMETRIC_REPRESENTATION_ITEM()
RATIONAL_B_SPLINE_SURFACE(((1.,0.675590207615668,1.),(1.,0.675585785528724,
1.),(1.,0.676431027860173,1.),(1.,0.679650528046127,1.),(1.,0.682027045382925,
1.),(1.,0.687915714942339,1.),(1.,0.69142441630503,1.),(1.,0.699004971484955,
1.),(1.,0.703073130220009,1.),(1.,0.70710678118655,1.)))
REPRESENTATION_ITEM('')
SURFACE()
);
#2162=(
BOUNDED_SURFACE()
B_SPLINE_SURFACE(3,2,((#141040,#141041,#141042),(#141043,#141044,#141045),
(#141046,#141047,#141048),(#141049,#141050,#141051),(#141052,#141053,#141054),
(#141055,#141056,#141057),(#141058,#141059,#141060),(#141061,#141062,#141063),
(#141064,#141065,#141066),(#141067,#141068,#141069)),.UNSPECIFIED.,.F.,
 .F.,.F.)
B_SPLINE_SURFACE_WITH_KNOTS((4,2,2,2,4),(3,3),(4.71238898038469,5.10508806208342,
5.49778714378214,5.89048622548086,6.28318530717959),(0.,1.),
 .UNSPECIFIED.)
GEOMETRIC_REPRESENTATION_ITEM()
RATIONAL_B_SPLINE_SURFACE(((1.,0.707106781186545,1.),(1.,0.711141648505882,
1.),(1.,0.715136249133832,1.),(1.,0.722468048845978,1.),(1.,0.725801833007229,
1.),(1.,0.731338116837136,1.),(1.,0.733539335051522,1.),(1.,0.736509240244802,
1.),(1.,0.737280525008203,1.),(1.,0.737277336810123,1.)))
REPRESENTATION_ITEM('')
SURFACE()
);
#2163=(
BOUNDED_SURFACE()
B_SPLINE_SURFACE(3,2,((#141204,#141205,#141206),(#141207,#141208,#141209),
(#141210,#141211,#141212),(#141213,#141214,#141215),(#141216,#141217,#141218),
(#141219,#141220,#141221),(#141222,#141223,#141224),(#141225,#141226,#141227),
(#141228,#141229,#141230),(#141231,#141232,#141233)),.UNSPECIFIED.,.F.,
 .F.,.F.)
B_SPLINE_SURFACE_WITH_KNOTS((4,2,2,2,4),(3,3),(4.71238898038469,5.10508806208342,
5.49778714378214,5.89048622548086,6.28318530717959),(0.,1.),
 .UNSPECIFIED.)
GEOMETRIC_REPRESENTATION_ITEM()
RATIONAL_B_SPLINE_SURFACE(((1.,0.707106781186545,1.),(1.,0.711141648505767,
1.),(1.,0.715136249133983,1.),(1.,0.722468048845823,1.),(1.,0.725801833007033,
1.),(1.,0.731338116837333,1.),(1.,0.73353933505153,1.),(1.,0.736509240244789,
1.),(1.,0.737280525008216,1.),(1.,0.737277336810123,1.)))
REPRESENTATION_ITEM('')
SURFACE()
);
#2164=(
BOUNDED_SURFACE()
B_SPLINE_SURFACE(3,2,((#141417,#141418,#141419),(#141420,#141421,#141422),
(#141423,#141424,#141425),(#141426,#141427,#141428)),.UNSPECIFIED.,.F.,
 .F.,.F.)
B_SPLINE_SURFACE_WITH_KNOTS((4,4),(3,3),(-5.74627151417317E-18,0.000655078443521525),
(0.,1.),.UNSPECIFIED.)
GEOMETRIC_REPRESENTATION_ITEM()
RATIONAL_B_SPLINE_SURFACE(((1.,0.773398994756356,1.),(1.,0.76231666392952,
1.),(1.,0.750153503473797,1.),(1.,0.737277336810164,1.)))
REPRESENTATION_ITEM('')
SURFACE()
);
#2165=(
BOUNDED_SURFACE()
B_SPLINE_SURFACE(3,2,((#141430,#141431,#141432),(#141433,#141434,#141435),
(#141436,#141437,#141438),(#141439,#141440,#141441)),.UNSPECIFIED.,.F.,
 .F.,.F.)
B_SPLINE_SURFACE_WITH_KNOTS((4,4),(3,3),(-8.23993651088983E-18,0.000144871551798125),
(0.,0.546238879221174),.UNSPECIFIED.)
GEOMETRIC_REPRESENTATION_ITEM()
RATIONAL_B_SPLINE_SURFACE(((1.,0.941669523342704,0.947063795072844),(1.,
0.94316141436526,0.948417719357794),(1.,0.944606420735039,0.949729094777561),
(1.,0.946004055482066,0.950997479396062)))
REPRESENTATION_ITEM('')
SURFACE()
);
#2166=(
BOUNDED_SURFACE()
B_SPLINE_SURFACE(3,2,((#141468,#141469,#141470),(#141471,#141472,#141473),
(#141474,#141475,#141476),(#141477,#141478,#141479),(#141480,#141481,#141482),
(#141483,#141484,#141485),(#141486,#141487,#141488),(#141489,#141490,#141491),
(#141492,#141493,#141494),(#141495,#141496,#141497)),.UNSPECIFIED.,.F.,
 .F.,.F.)
B_SPLINE_SURFACE_WITH_KNOTS((4,2,2,2,4),(3,3),(-1.77635683940025E-15,0.392699081698723,
0.785398163397447,1.17809724509617,1.5707963267949),(0.,1.),
 .UNSPECIFIED.)
GEOMETRIC_REPRESENTATION_ITEM()
RATIONAL_B_SPLINE_SURFACE(((1.,0.675590207615662,1.),(1.,0.675585785528387,
1.),(1.,0.676431027860615,1.),(1.,0.679650528045674,1.),(1.,0.682027045382935,
1.),(1.,0.687915714942327,1.),(1.,0.691424416304369,1.),(1.,0.699004971485606,
1.),(1.,0.703073130219524,1.),(1.,0.707106781186548,1.)))
REPRESENTATION_ITEM('')
SURFACE()
);
#2167=(
BOUNDED_SURFACE()
B_SPLINE_SURFACE(3,2,((#141760,#141761,#141762),(#141763,#141764,#141765),
(#141766,#141767,#141768),(#141769,#141770,#141771),(#141772,#141773,#141774),
(#141775,#141776,#141777)),.UNSPECIFIED.,.F.,.F.,.F.)
B_SPLINE_SURFACE_WITH_KNOTS((4,2,4),(3,3),(0.00432986646256736,0.00505584518302534,
0.00578182390348332),(0.,1.),.UNSPECIFIED.)
GEOMETRIC_REPRESENTATION_ITEM()
RATIONAL_B_SPLINE_SURFACE(((1.,0.737277336810087,1.),(1.,0.750110373322841,
1.),(1.,0.762782449795825,1.),(1.,0.783852338027907,1.),(1.,0.792419881107176,
1.),(1.,0.79736306112227,1.)))
REPRESENTATION_ITEM('')
SURFACE()
);
#2168=(
BOUNDED_SURFACE()
B_SPLINE_SURFACE(3,2,((#141903,#141904,#141905),(#141906,#141907,#141908),
(#141909,#141910,#141911),(#141912,#141913,#141914),(#141915,#141916,#141917),
(#141918,#141919,#141920),(#141921,#141922,#141923),(#141924,#141925,#141926),
(#141927,#141928,#141929),(#141930,#141931,#141932)),.UNSPECIFIED.,.F.,
 .F.,.F.)
B_SPLINE_SURFACE_WITH_KNOTS((4,2,2,2,4),(3,3),(3.1415926535898,3.53429173528852,
3.92699081698724,4.31968989868597,4.71238898038469),(0.,1.),
 .UNSPECIFIED.)
GEOMETRIC_REPRESENTATION_ITEM()
RATIONAL_B_SPLINE_SURFACE(((1.,0.73727733681012,1.),(1.,0.737280525007918,
1.),(1.,0.736509240245177,1.),(1.,0.733539335051133,1.),(1.,0.731338116836513,
1.),(1.,0.725801833007847,1.),(1.,0.722468048844965,1.),(1.,0.715136249134831,
1.),(1.,0.711141648505139,1.),(1.,0.707106781186548,1.)))
REPRESENTATION_ITEM('')
SURFACE()
);
#2169=(
BOUNDED_SURFACE()
B_SPLINE_SURFACE(3,2,((#142170,#142171,#142172),(#142173,#142174,#142175),
(#142176,#142177,#142178),(#142179,#142180,#142181),(#142182,#142183,#142184),
(#142185,#142186,#142187),(#142188,#142189,#142190),(#142191,#142192,#142193),
(#142194,#142195,#142196),(#142197,#142198,#142199)),.UNSPECIFIED.,.F.,
 .F.,.F.)
B_SPLINE_SURFACE_WITH_KNOTS((4,2,2,2,4),(3,3),(1.5707963267949,1.96349540849362,
2.35619449019234,2.74889357189107,3.14159265358979),(0.,1.),
 .UNSPECIFIED.)
GEOMETRIC_REPRESENTATION_ITEM()
RATIONAL_B_SPLINE_SURFACE(((1.,0.707106781186548,1.),(1.,0.703073130219484,
1.),(1.,0.699004971485652,1.),(1.,0.691424416304328,1.),(1.,0.687915714942076,
1.),(1.,0.682027045383186,1.),(1.,0.679650528045925,1.),(1.,0.676431027860385,
1.),(1.,0.675585785528569,1.),(1.,0.67559020761567,1.)))
REPRESENTATION_ITEM('')
SURFACE()
);
#2170=(
BOUNDED_SURFACE()
B_SPLINE_SURFACE(3,2,((#142207,#142208,#142209),(#142210,#142211,#142212),
(#142213,#142214,#142215),(#142216,#142217,#142218),(#142219,#142220,#142221),
(#142222,#142223,#142224),(#142225,#142226,#142227),(#142228,#142229,#142230),
(#142231,#142232,#142233),(#142234,#142235,#142236)),.UNSPECIFIED.,.F.,
 .F.,.F.)
B_SPLINE_SURFACE_WITH_KNOTS((4,2,2,2,4),(3,3),(3.1415926535898,3.53429173528852,
3.92699081698724,4.31968989868597,4.71238898038469),(0.,1.),
 .UNSPECIFIED.)
GEOMETRIC_REPRESENTATION_ITEM()
RATIONAL_B_SPLINE_SURFACE(((1.,0.73727733681012,1.),(1.,0.737280525007918,
1.),(1.,0.736509240245186,1.),(1.,0.733539335051142,1.),(1.,0.731338116837293,
1.),(1.,0.725801833007076,1.),(1.,0.722468048845319,1.),(1.,0.715136249134486,
1.),(1.,0.711141648505406,1.),(1.,0.707106781186552,1.)))
REPRESENTATION_ITEM('')
SURFACE()
);
#2171=(
BOUNDED_SURFACE()
B_SPLINE_SURFACE(3,2,((#142380,#142381,#142382),(#142383,#142384,#142385),
(#142386,#142387,#142388),(#142389,#142390,#142391),(#142392,#142393,#142394),
(#142395,#142396,#142397),(#142398,#142399,#142400),(#142401,#142402,#142403),
(#142404,#142405,#142406),(#142407,#142408,#142409)),.UNSPECIFIED.,.F.,
 .F.,.F.)
B_SPLINE_SURFACE_WITH_KNOTS((4,2,2,2,4),(3,3),(1.5707963267949,1.96349540849362,
2.35619449019234,2.74889357189107,3.14159265358979),(0.,1.),
 .UNSPECIFIED.)
GEOMETRIC_REPRESENTATION_ITEM()
RATIONAL_B_SPLINE_SURFACE(((1.,0.707106781186543,1.),(1.,0.703073130219691,
1.),(1.,0.699004971485369,1.),(1.,0.691424416304591,1.),(1.,0.687915714942475,
1.),(1.,0.682027045382777,1.),(1.,0.679650528045923,1.),(1.,0.676431027860383,
1.),(1.,0.675585785528567,1.),(1.,0.675590207615659,1.)))
REPRESENTATION_ITEM('')
SURFACE()
);
#2172=(
BOUNDED_SURFACE()
B_SPLINE_SURFACE(2,2,((#142574,#142575,#142576),(#142577,#142578,#142579),
(#142580,#142581,#142582)),.UNSPECIFIED.,.F.,.F.,.F.)
B_SPLINE_SURFACE_WITH_KNOTS((3,3),(3,3),(-1.5707963267949,-1.75915766232281E-16),
(2.36370134837197,3.14159265358979),.UNSPECIFIED.)
GEOMETRIC_REPRESENTATION_ITEM()
RATIONAL_B_SPLINE_SURFACE(((1.,0.925309396359852,1.),(0.707106781186554,
0.654292548861688,0.707106781186554),(1.,0.925309396359852,1.)))
REPRESENTATION_ITEM('')
SURFACE()
);
#2173=(
BOUNDED_SURFACE()
B_SPLINE_SURFACE(2,2,((#142590,#142591,#142592),(#142593,#142594,#142595),
(#142596,#142597,#142598)),.UNSPECIFIED.,.F.,.F.,.F.)
B_SPLINE_SURFACE_WITH_KNOTS((3,3),(3,3),(-1.5707963267949,0.),(1.5707963267949,
2.40432329481773),.UNSPECIFIED.)
GEOMETRIC_REPRESENTATION_ITEM()
RATIONAL_B_SPLINE_SURFACE(((1.,0.914403878918655,1.),(0.707106781186554,
0.64658118352667,0.707106781186554),(1.,0.914403878918655,1.)))
REPRESENTATION_ITEM('')
SURFACE()
);
#2174=(
BOUNDED_SURFACE()
B_SPLINE_SURFACE(3,2,((#142680,#142681,#142682),(#142683,#142684,#142685),
(#142686,#142687,#142688),(#142689,#142690,#142691),(#142692,#142693,#142694),
(#142695,#142696,#142697),(#142698,#142699,#142700),(#142701,#142702,#142703),
(#142704,#142705,#142706),(#142707,#142708,#142709)),.UNSPECIFIED.,.F.,
 .F.,.F.)
B_SPLINE_SURFACE_WITH_KNOTS((4,2,2,2,4),(3,3),(0.00328497804042337,0.00367780251889487,
0.00407062699736637,0.00446345147583787,0.00485627595430937),(0.,1.),
 .UNSPECIFIED.)
GEOMETRIC_REPRESENTATION_ITEM()
RATIONAL_B_SPLINE_SURFACE(((1.,0.801783725737274,1.),(1.,0.801875346909261,
1.),(1.,0.796940392589261,1.),(1.,0.780100098278086,1.),(1.,0.768150144755555,
1.),(1.,0.743627445145758,1.),(1.,0.730956034974261,1.),(1.,0.712691010436091,
1.),(1.,0.706946596929733,1.),(1.,0.707106781186548,1.)))
REPRESENTATION_ITEM('')
SURFACE()
);
#2175=(
BOUNDED_SURFACE()
B_SPLINE_SURFACE(3,2,((#142721,#142722,#142723),(#142724,#142725,#142726),
(#142727,#142728,#142729),(#142730,#142731,#142732),(#142733,#142734,#142735),
(#142736,#142737,#142738)),.UNSPECIFIED.,.F.,.F.,.F.)
B_SPLINE_SURFACE_WITH_KNOTS((4,2,4),(3,3),(-1.97866896478604E-18,0.00038804539867497,
0.000776090797349943),(0.,1.),.UNSPECIFIED.)
GEOMETRIC_REPRESENTATION_ITEM()
RATIONAL_B_SPLINE_SURFACE(((1.,0.889512696472455,1.),(1.,0.863343118435834,
1.),(1.,0.832896241151233,1.),(1.,0.770252595987774,1.),(1.,0.738321744191135,
1.),(1.,0.707106781186616,1.)))
REPRESENTATION_ITEM('')
SURFACE()
);
#2176=(
BOUNDED_SURFACE()
B_SPLINE_SURFACE(3,2,((#142752,#142753,#142754),(#142755,#142756,#142757),
(#142758,#142759,#142760),(#142761,#142762,#142763)),.UNSPECIFIED.,.F.,
 .F.,.F.)
B_SPLINE_SURFACE_WITH_KNOTS((4,4),(3,3),(-3.41523684332934E-18,0.000418670815451504),
(0.,1.),.UNSPECIFIED.)
GEOMETRIC_REPRESENTATION_ITEM()
RATIONAL_B_SPLINE_SURFACE(((1.,0.80178372573727,1.),(1.,0.801581038760284,
1.),(1.,0.797360979426379,1.),(1.,0.782160982635977,1.)))
REPRESENTATION_ITEM('')
SURFACE()
);
#2177=(
BOUNDED_SURFACE()
B_SPLINE_SURFACE(3,2,((#142770,#142771,#142772),(#142773,#142774,#142775),
(#142776,#142777,#142778),(#142779,#142780,#142781),(#142782,#142783,#142784),
(#142785,#142786,#142787)),.UNSPECIFIED.,.F.,.F.,.F.)
B_SPLINE_SURFACE_WITH_KNOTS((4,2,4),(3,3),(0.,0.00138008432392828,0.00276016864785656),
(0.,1.),.UNSPECIFIED.)
GEOMETRIC_REPRESENTATION_ITEM()
RATIONAL_B_SPLINE_SURFACE(((1.,0.889512696472458,1.),(1.,0.875621469665309,
1.),(1.,0.859481975708513,1.),(1.,0.823331923932046,1.),(1.,0.803217377248123,
1.),(1.,0.782160982635976,1.)))
REPRESENTATION_ITEM('')
SURFACE()
);
#2178=(
BOUNDED_SURFACE()
B_SPLINE_SURFACE(3,2,((#142799,#142800,#142801),(#142802,#142803,#142804),
(#142805,#142806,#142807),(#142808,#142809,#142810),(#142811,#142812,#142813),
(#142814,#142815,#142816),(#142817,#142818,#142819),(#142820,#142821,#142822),
(#142823,#142824,#142825),(#142826,#142827,#142828),(#142829,#142830,#142831),
(#142832,#142833,#142834)),.UNSPECIFIED.,.F.,.F.,.F.)
B_SPLINE_SURFACE_WITH_KNOTS((4,2,2,2,2,4),(3,3),(0.,0.000250417359226946,
0.000375626038840418,0.000500834718453891,0.000751252077680836,0.00100166943690778),
(-0.00140468204160171,1.),.UNSPECIFIED.)
GEOMETRIC_REPRESENTATION_ITEM()
RATIONAL_B_SPLINE_SURFACE(((1.0008239995229,0.706695359341974,1.),(1.00080388922191,
0.713853670046833,1.),(1.00078381509905,0.720999103057124,1.),(1.00075782359272,
0.7302508431544,1.),(1.00074967829203,0.73315018280726,1.),(1.00073524706918,
0.738287011792902,1.),(1.00072896513201,0.740523082654128,1.),(1.00071294399062,
0.746225847024512,1.),(1.00070666903946,0.748459431199004,1.),(1.00070405563711,
0.749389678142165,1.),(1.00070770913775,0.748089205673413,1.),(1.00071606406546,
0.745115248770045,1.)))
REPRESENTATION_ITEM('')
SURFACE()
);
#2179=(
BOUNDED_SURFACE()
B_SPLINE_SURFACE(3,2,((#142836,#142837,#142838),(#142839,#142840,#142841),
(#142842,#142843,#142844),(#142845,#142846,#142847),(#142848,#142849,#142850),
(#142851,#142852,#142853),(#142854,#142855,#142856),(#142857,#142858,#142859),
(#142860,#142861,#142862),(#142863,#142864,#142865),(#142866,#142867,#142868),
(#142869,#142870,#142871)),.UNSPECIFIED.,.F.,.F.,.F.)
B_SPLINE_SURFACE_WITH_KNOTS((4,2,2,2,2,4),(3,3),(-2.00577401909819E-18,
0.000253295312002929,0.000379942968004394,0.00050659062400586,0.000759885936008791,
0.00101318124801172),(0.,1.),.UNSPECIFIED.)
GEOMETRIC_REPRESENTATION_ITEM()
RATIONAL_B_SPLINE_SURFACE(((1.,0.619253049823351,1.),(1.,0.611711019709536,
1.),(1.,0.608322651255403,1.),(1.,0.610256821027379,1.),(1.,0.612081873728276,
1.),(1.,0.61778814027945,1.),(1.,0.621690668847742,1.),(1.,0.636005795097188,
1.),(1.,0.648854597242623,1.),(1.,0.676998182563378,1.),(1.,0.692438011698887,
1.),(1.,0.707106781186548,1.)))
REPRESENTATION_ITEM('')
SURFACE()
);
#2180=(
BOUNDED_SURFACE()
B_SPLINE_SURFACE(3,2,((#142878,#142879,#142880),(#142881,#142882,#142883),
(#142884,#142885,#142886),(#142887,#142888,#142889)),.UNSPECIFIED.,.F.,
 .F.,.F.)
B_SPLINE_SURFACE_WITH_KNOTS((4,4),(3,3),(0.00165976994196512,0.00175987143987977),
(0.,1.),.UNSPECIFIED.)
GEOMETRIC_REPRESENTATION_ITEM()
RATIONAL_B_SPLINE_SURFACE(((1.,0.707106781186549,1.),(1.,0.714158119082749,
1.),(1.,0.721010468727715,1.),(1.,0.727682857483054,1.)))
REPRESENTATION_ITEM('')
SURFACE()
);
#2181=(
BOUNDED_SURFACE()
B_SPLINE_SURFACE(3,2,((#142891,#142892,#142893),(#142894,#142895,#142896),
(#142897,#142898,#142899),(#142900,#142901,#142902),(#142903,#142904,#142905),
(#142906,#142907,#142908),(#142909,#142910,#142911),(#142912,#142913,#142914),
(#142915,#142916,#142917),(#142918,#142919,#142920)),.UNSPECIFIED.,.F.,
 .F.,.F.)
B_SPLINE_SURFACE_WITH_KNOTS((4,2,2,2,4),(3,3),(0.00166905748884283,0.00189688228523533,
0.00212470708162783,0.00235253187802032,0.00258035667441282),(0.,1.),
 .UNSPECIFIED.)
GEOMETRIC_REPRESENTATION_ITEM()
RATIONAL_B_SPLINE_SURFACE(((1.,0.727682857482998,1.),(1.,0.742747587336582,
1.),(1.,0.756565090576503,1.),(1.,0.779563382898484,1.),(1.,0.788904601358709,
1.),(1.,0.801793098601248,1.),(1.,0.805447378128131,1.),(1.,0.806422615061365,
1.),(1.,0.803776299349016,1.),(1.,0.798143461625347,1.)))
REPRESENTATION_ITEM('')
SURFACE()
);
#2182=(
BOUNDED_SURFACE()
B_SPLINE_SURFACE(3,2,((#142922,#142923,#142924),(#142925,#142926,#142927),
(#142928,#142929,#142930),(#142931,#142932,#142933),(#142934,#142935,#142936),
(#142937,#142938,#142939)),.UNSPECIFIED.,.F.,.F.,.F.)
B_SPLINE_SURFACE_WITH_KNOTS((4,2,4),(3,3),(0.19058679356565,0.194723599184011,
0.198860404802373),(0.,1.),.UNSPECIFIED.)
GEOMETRIC_REPRESENTATION_ITEM()
RATIONAL_B_SPLINE_SURFACE(((1.,0.954062806827576,1.),(1.,0.95589180838713,
1.),(1.,0.957713181483215,1.),(1.,0.961295526062221,1.),(1.,0.963047831711069,
1.),(1.,0.964700553047209,1.)))
REPRESENTATION_ITEM('')
SURFACE()
);
#2183=(
BOUNDED_SURFACE()
B_SPLINE_SURFACE(2,2,((#142973,#142974,#142975),(#142976,#142977,#142978),
(#142979,#142980,#142981)),.UNSPECIFIED.,.F.,.F.,.F.)
B_SPLINE_SURFACE_WITH_KNOTS((3,3),(3,3),(-3.74064361396611E-16,1.57079632679501),
(0.,1.5707963267949),.UNSPECIFIED.)
GEOMETRIC_REPRESENTATION_ITEM()
RATIONAL_B_SPLINE_SURFACE(((1.,0.707106781186548,1.),(0.707106781186506,
0.49999999999997,0.707106781186506),(1.,0.707106781186548,1.)))
REPRESENTATION_ITEM('')
SURFACE()
);
#2184=(
BOUNDED_SURFACE()
B_SPLINE_SURFACE(2,2,((#142993,#142994,#142995),(#142996,#142997,#142998),
(#142999,#143000,#143001)),.UNSPECIFIED.,.F.,.F.,.F.)
B_SPLINE_SURFACE_WITH_KNOTS((3,3),(3,3),(0.,1.57079632679501),(1.5707963267949,
3.14159265358979),.UNSPECIFIED.)
GEOMETRIC_REPRESENTATION_ITEM()
RATIONAL_B_SPLINE_SURFACE(((1.,0.707106781186548,1.),(0.707106781186506,
0.49999999999997,0.707106781186506),(1.,0.707106781186548,1.)))
REPRESENTATION_ITEM('')
SURFACE()
);
#2185=(
BOUNDED_SURFACE()
B_SPLINE_SURFACE(2,2,((#143024,#143025,#143026),(#143027,#143028,#143029),
(#143030,#143031,#143032)),.UNSPECIFIED.,.F.,.F.,.F.)
B_SPLINE_SURFACE_WITH_KNOTS((3,3),(3,3),(-3.74064361396611E-16,1.57079632679492),
(0.,1.5707963267949),.UNSPECIFIED.)
GEOMETRIC_REPRESENTATION_ITEM()
RATIONAL_B_SPLINE_SURFACE(((1.,0.707106781186548,1.),(0.707106781186552,
0.500000000000003,0.707106781186552),(1.,0.707106781186548,1.)))
REPRESENTATION_ITEM('')
SURFACE()
);
#2186=(
BOUNDED_SURFACE()
B_SPLINE_SURFACE(2,2,((#143044,#143045,#143046),(#143047,#143048,#143049),
(#143050,#143051,#143052)),.UNSPECIFIED.,.F.,.F.,.F.)
B_SPLINE_SURFACE_WITH_KNOTS((3,3),(3,3),(0.,1.57079632679492),(1.5707963267949,
3.14159265358979),.UNSPECIFIED.)
GEOMETRIC_REPRESENTATION_ITEM()
RATIONAL_B_SPLINE_SURFACE(((1.,0.707106781186548,1.),(0.707106781186552,
0.500000000000003,0.707106781186552),(1.,0.707106781186548,1.)))
REPRESENTATION_ITEM('')
SURFACE()
);
#2187=(
BOUNDED_SURFACE()
B_SPLINE_SURFACE(2,2,((#143072,#143073,#143074),(#143075,#143076,#143077),
(#143078,#143079,#143080)),.UNSPECIFIED.,.F.,.F.,.F.)
B_SPLINE_SURFACE_WITH_KNOTS((3,3),(3,3),(-3.74064361396611E-16,1.57079632679492),
(0.,1.5707963267949),.UNSPECIFIED.)
GEOMETRIC_REPRESENTATION_ITEM()
RATIONAL_B_SPLINE_SURFACE(((1.,0.707106781186548,1.),(0.707106781186552,
0.500000000000003,0.707106781186552),(1.,0.707106781186548,1.)))
REPRESENTATION_ITEM('')
SURFACE()
);
#2188=(
BOUNDED_SURFACE()
B_SPLINE_SURFACE(3,2,((#143089,#143090,#143091),(#143092,#143093,#143094),
(#143095,#143096,#143097),(#143098,#143099,#143100),(#143101,#143102,#143103),
(#143104,#143105,#143106),(#143107,#143108,#143109),(#143110,#143111,#143112),
(#143113,#143114,#143115),(#143116,#143117,#143118)),.UNSPECIFIED.,.F.,
 .F.,.F.)
B_SPLINE_SURFACE_WITH_KNOTS((4,2,2,2,4),(3,3),(0.00116892975483561,0.00173273620432837,
0.00229654265382113,0.00286034910331391,0.00342415555280667),(-8.73672651670295E-5,
1.),.UNSPECIFIED.)
GEOMETRIC_REPRESENTATION_ITEM()
RATIONAL_B_SPLINE_SURFACE(((1.00005118303036,0.707081191907034,1.),(1.00004250803408,
0.75672791175003,1.),(1.00003576403205,0.795323614743255,1.),(1.0000266067815,
0.847730260009664,1.),(1.00002422236724,0.86137618483401,1.),(1.00002421067414,
0.861443104051655,1.),(1.0000265855687,0.847851660205381,1.),(1.00003574715403,
0.795420207077597,1.),(1.00004250128307,0.756766547571557,1.),(1.00005118303036,
0.707081191907034,1.)))
REPRESENTATION_ITEM('')
SURFACE()
);
#2189=(
BOUNDED_SURFACE()
B_SPLINE_SURFACE(3,2,((#143124,#143125,#143126),(#143127,#143128,#143129),
(#143130,#143131,#143132),(#143133,#143134,#143135),(#143136,#143137,#143138),
(#143139,#143140,#143141),(#143142,#143143,#143144),(#143145,#143146,#143147),
(#143148,#143149,#143150),(#143151,#143152,#143153)),.UNSPECIFIED.,.F.,
 .F.,.F.)
B_SPLINE_SURFACE_WITH_KNOTS((4,2,2,2,4),(3,3),(4.71238898038469,5.10508806208341,
5.49778714378214,5.89048622548086,6.28318530717959),(0.,1.),
 .UNSPECIFIED.)
GEOMETRIC_REPRESENTATION_ITEM()
RATIONAL_B_SPLINE_SURFACE(((1.,0.707106781186548,1.),(1.,0.71355026185156,
1.),(1.,0.719894264862189,1.),(1.,0.73149075639733,1.),(1.,0.73673812929671,
1.),(1.,0.745429366938189,1.),(1.,0.748871927696634,1.),(1.,0.753512297096161,
1.),(1.,0.754714219730837,1.),(1.,0.754709580222772,1.)))
REPRESENTATION_ITEM('')
SURFACE()
);
#2190=(
BOUNDED_SURFACE()
B_SPLINE_SURFACE(3,2,((#143170,#143171,#143172),(#143173,#143174,#143175),
(#143176,#143177,#143178),(#143179,#143180,#143181),(#143182,#143183,#143184),
(#143185,#143186,#143187),(#143188,#143189,#143190),(#143191,#143192,#143193),
(#143194,#143195,#143196),(#143197,#143198,#143199)),.UNSPECIFIED.,.F.,
 .F.,.F.)
B_SPLINE_SURFACE_WITH_KNOTS((4,2,2,2,4),(3,3),(8.78519494496445E-16,0.392699081698725,
0.785398163397449,1.17809724509617,1.5707963267949),(0.,1.),
 .UNSPECIFIED.)
GEOMETRIC_REPRESENTATION_ITEM()
RATIONAL_B_SPLINE_SURFACE(((1.,0.754709580222768,1.),(1.,0.754714219644573,
1.),(1.,0.753512297211018,1.),(1.,0.748871927581762,1.),(1.,0.745429367161016,
1.),(1.,0.736738129073881,1.),(1.,0.73149075671205,1.),(1.,0.719894264547496,
1.),(1.,0.713550262087909,1.),(1.,0.707106781186548,1.)))
REPRESENTATION_ITEM('')
SURFACE()
);
#2191=(
BOUNDED_SURFACE()
B_SPLINE_SURFACE(3,2,((#143854,#143855,#143856),(#143857,#143858,#143859),
(#143860,#143861,#143862),(#143863,#143864,#143865),(#143866,#143867,#143868),
(#143869,#143870,#143871),(#143872,#143873,#143874),(#143875,#143876,#143877),
(#143878,#143879,#143880),(#143881,#143882,#143883)),.UNSPECIFIED.,.F.,
 .F.,.F.)
B_SPLINE_SURFACE_WITH_KNOTS((4,2,2,2,4),(3,3),(0.00116892975483565,0.00173273620432837,
0.00229654265382108,0.0028603491033138,0.00342415555280651),(-8.73672651410431E-5,
1.),.UNSPECIFIED.)
GEOMETRIC_REPRESENTATION_ITEM()
RATIONAL_B_SPLINE_SURFACE(((1.00005118303034,0.707081191907037,1.),(1.00004250803407,
0.756727911750281,1.),(1.00003576403204,0.795323614742893,1.),(1.00002660678149,
0.847730260009987,1.),(1.00002422236723,0.861376184832614,1.),(1.00002421067413,
0.861443104052995,1.),(1.00002658556869,0.847851660205354,1.),(1.00003574715402,
0.795420207077597,1.),(1.00004250128306,0.756766547571537,1.),(1.00005118303034,
0.707081191907037,1.)))
REPRESENTATION_ITEM('')
SURFACE()
);
#2192=(
BOUNDED_SURFACE()
B_SPLINE_SURFACE(3,2,((#143900,#143901,#143902),(#143903,#143904,#143905),
(#143906,#143907,#143908),(#143909,#143910,#143911),(#143912,#143913,#143914),
(#143915,#143916,#143917),(#143918,#143919,#143920),(#143921,#143922,#143923),
(#143924,#143925,#143926),(#143927,#143928,#143929)),.UNSPECIFIED.,.F.,
 .F.,.F.)
B_SPLINE_SURFACE_WITH_KNOTS((4,2,2,2,4),(3,3),(0.00108313181642967,0.00175636478508591,
0.00242959775374216,0.0031028307223984,0.00377606369105465),(-0.000209460012303618,
1.),.UNSPECIFIED.)
GEOMETRIC_REPRESENTATION_ITEM()
RATIONAL_B_SPLINE_SURFACE(((1.00012272453493,0.707045431769336,1.),(1.00009434426229,
0.774791710231057,1.),(1.00007166829574,0.828921293970649,1.),(1.0000403086156,
0.903779687679754,1.),(1.00003179560244,0.924101020320101,1.),(1.00003154660919,
0.92469538973271,1.),(1.00003985538718,0.90486158494707,1.),(1.00007114262335,
0.830176121522528,1.),(1.00009383870822,0.775998513536341,1.),(1.00012272453493,
0.707045431769336,1.)))
REPRESENTATION_ITEM('')
SURFACE()
);
#2193=(
BOUNDED_SURFACE()
B_SPLINE_SURFACE(3,2,((#143938,#143939,#143940),(#143941,#143942,#143943),
(#143944,#143945,#143946),(#143947,#143948,#143949),(#143950,#143951,#143952),
(#143953,#143954,#143955),(#143956,#143957,#143958),(#143959,#143960,#143961),
(#143962,#143963,#143964),(#143965,#143966,#143967)),.UNSPECIFIED.,.F.,
 .F.,.F.)
B_SPLINE_SURFACE_WITH_KNOTS((4,2,2,2,4),(3,3),(0.00131180726843869,0.00173116479138241,
0.00215052231432612,0.00256987983726984,0.00298923736021356),(-7.19536616060548E-6,
1.),.UNSPECIFIED.)
GEOMETRIC_REPRESENTATION_ITEM()
RATIONAL_B_SPLINE_SURFACE(((1.00000421497824,0.707104673712593,1.),(1.00000380693473,
0.735459277067922,1.),(1.00000349584298,0.757076784024011,1.),(1.00000307861086,
0.78606989643,1.),(1.00000297270686,0.793429076618424,1.),(1.00000297242631,
0.793448571747567,1.),(1.00000307812254,0.786103829136133,1.),(1.0000034951559,
0.757124528684544,1.),(1.00000380600669,0.735523766261729,1.),(1.00000421497824,
0.707104673712593,1.)))
REPRESENTATION_ITEM('')
SURFACE()
);
#2194=(
BOUNDED_SURFACE()
B_SPLINE_SURFACE(3,2,((#143988,#143989,#143990),(#143991,#143992,#143993),
(#143994,#143995,#143996),(#143997,#143998,#143999)),.UNSPECIFIED.,.F.,
 .F.,.F.)
B_SPLINE_SURFACE_WITH_KNOTS((4,4),(3,3),(-3.51851606259766E-5,0.000688755160509476),
(0.,1.00003518516063),.UNSPECIFIED.)
GEOMETRIC_REPRESENTATION_ITEM()
RATIONAL_B_SPLINE_SURFACE(((1.,0.568606220888424,1.00003035731882),(1.,
0.556584756681385,1.00003120327312),(1.,0.550157943671747,1.00003165553002),
(1.,0.550842070368378,1.0000316073878)))
REPRESENTATION_ITEM('')
SURFACE()
);
#2195=(
BOUNDED_SURFACE()
B_SPLINE_SURFACE(3,2,((#144019,#144020,#144021),(#144022,#144023,#144024),
(#144025,#144026,#144027),(#144028,#144029,#144030)),.UNSPECIFIED.,.F.,
 .F.,.F.)
B_SPLINE_SURFACE_WITH_KNOTS((4,4),(3,3),(-6.51893458122614E-5,0.000717082803934822),
(0.,1.00014047630858),.UNSPECIFIED.)
GEOMETRIC_REPRESENTATION_ITEM()
RATIONAL_B_SPLINE_SURFACE(((1.,0.80532666321776,1.00005469398346),(1.,0.805999592802023,
1.00005450492213),(1.,0.80258142750598,1.00005546526462),(1.,0.795135566176566,
1.00005755719884)))
REPRESENTATION_ITEM('')
SURFACE()
);
#2196=(
BOUNDED_SURFACE()
B_SPLINE_SURFACE(3,2,((#144042,#144043,#144044),(#144045,#144046,#144047),
(#144048,#144049,#144050),(#144051,#144052,#144053)),.UNSPECIFIED.,.F.,
 .F.,.F.)
B_SPLINE_SURFACE_WITH_KNOTS((4,4),(3,3),(-6.51412822692208E-5,0.000716554104961429),
(0.,1.00012817146333),.UNSPECIFIED.)
GEOMETRIC_REPRESENTATION_ITEM()
RATIONAL_B_SPLINE_SURFACE(((1.,0.62167678976432,1.00009698047894),(1.,0.613563994562104,
1.0000990601366),(1.,0.609559936451189,1.00010008654858),(1.,0.610338513229397,
1.00009988696593)))
REPRESENTATION_ITEM('')
SURFACE()
);
#2197=(
BOUNDED_SURFACE()
B_SPLINE_SURFACE(3,2,((#144072,#144073,#144074),(#144075,#144076,#144077),
(#144078,#144079,#144080),(#144081,#144082,#144083)),.UNSPECIFIED.,.F.,
 .F.,.F.)
B_SPLINE_SURFACE_WITH_KNOTS((4,4),(3,3),(0.,0.000650589467290063),(0.,1.),
 .UNSPECIFIED.)
GEOMETRIC_REPRESENTATION_ITEM()
RATIONAL_B_SPLINE_SURFACE(((1.,0.761354724782838,1.),(1.,0.761348936155314,
1.),(1.,0.759749503531854,1.),(1.,0.756551244268667,1.)))
REPRESENTATION_ITEM('')
SURFACE()
);
#2198=(
BOUNDED_SURFACE()
B_SPLINE_SURFACE(3,2,((#144085,#144086,#144087),(#144088,#144089,#144090),
(#144091,#144092,#144093),(#144094,#144095,#144096),(#144097,#144098,#144099),
(#144100,#144101,#144102),(#144103,#144104,#144105),(#144106,#144107,#144108),
(#144109,#144110,#144111),(#144112,#144113,#144114),(#144115,#144116,#144117),
(#144118,#144119,#144120),(#144121,#144122,#144123),(#144124,#144125,#144126)),
 .UNSPECIFIED.,.F.,.F.,.F.)
B_SPLINE_SURFACE_WITH_KNOTS((4,2,2,2,2,2,4),(3,3),(0.00807902625150492,
0.00883280378349999,0.00920969254949752,0.00958658131549505,0.00996347008149258,
0.0103403588474901,0.0110941363794852),(0.,1.),.UNSPECIFIED.)
GEOMETRIC_REPRESENTATION_ITEM()
RATIONAL_B_SPLINE_SURFACE(((1.,0.707106781186548,1.),(1.,0.708503208405905,
1.),(1.,0.709864127404626,1.),(1.,0.711851747119499,1.),(1.,0.712500882329163,
1.),(1.,0.713738228851022,1.),(1.,0.714331705876986,1.),(1.,0.715467776552351,
1.),(1.,0.716012641761659,1.),(1.,0.71701515809269,1.),(1.,0.717477434704573,
1.),(1.,0.718748007011303,1.),(1.,0.719442582755427,1.),(1.,0.719919801430648,
1.)))
REPRESENTATION_ITEM('')
SURFACE()
);
#2199=(
BOUNDED_SURFACE()
B_SPLINE_SURFACE(3,2,((#144143,#144144,#144145),(#144146,#144147,#144148),
(#144149,#144150,#144151),(#144152,#144153,#144154)),.UNSPECIFIED.,.F.,
 .F.,.F.)
B_SPLINE_SURFACE_WITH_KNOTS((4,4),(3,3),(0.0156098999423859,0.0162171358932854),
(0.0843742085712764,1.),.UNSPECIFIED.)
GEOMETRIC_REPRESENTATION_ITEM()
RATIONAL_B_SPLINE_SURFACE(((0.967873953213285,0.809621640719886,1.),(0.968348523789084,
0.812433937177747,1.),(0.968804462122364,0.815135819310926,1.),(0.969242174215226,
0.817729693080374,1.)))
REPRESENTATION_ITEM('')
SURFACE()
);
#2200=(
BOUNDED_SURFACE()
B_SPLINE_SURFACE(3,2,((#144174,#144175,#144176),(#144177,#144178,#144179),
(#144180,#144181,#144182),(#144183,#144184,#144185),(#144186,#144187,#144188),
(#144189,#144190,#144191),(#144192,#144193,#144194),(#144195,#144196,#144197),
(#144198,#144199,#144200),(#144201,#144202,#144203),(#144204,#144205,#144206),
(#144207,#144208,#144209),(#144210,#144211,#144212),(#144213,#144214,#144215)),
 .UNSPECIFIED.,.F.,.F.,.F.)
B_SPLINE_SURFACE_WITH_KNOTS((4,2,2,2,2,2,4),(3,3),(0.00807927244133089,
0.00881458117408921,0.00918223554046837,0.00954988990684753,0.0099175442732267,
0.0102851986396059,0.0110205073723642),(0.,1.),.UNSPECIFIED.)
GEOMETRIC_REPRESENTATION_ITEM()
RATIONAL_B_SPLINE_SURFACE(((1.,0.707106781186548,1.),(1.,0.705697402766896,
1.),(1.,0.704316028414221,1.),(1.,0.702287640598182,1.),(1.,0.70162085852966,
1.),(1.,0.700346303389684,1.),(1.,0.699732822392533,1.),(1.,0.69855427952325,
1.),(1.,0.697985323371657,1.),(1.,0.696930428409623,1.),(1.,0.69644149384419,
1.),(1.,0.695089684342733,1.),(1.,0.694335092820993,1.),(1.,0.693797102764879,
1.)))
REPRESENTATION_ITEM('')
SURFACE()
);
#2201=(
BOUNDED_SURFACE()
B_SPLINE_SURFACE(3,2,((#144217,#144218,#144219),(#144220,#144221,#144222),
(#144223,#144224,#144225),(#144226,#144227,#144228)),.UNSPECIFIED.,.F.,
 .F.,.F.)
B_SPLINE_SURFACE_WITH_KNOTS((4,4),(3,3),(-1.0842021724855E-19,0.000650371461981817),
(0.,1.),.UNSPECIFIED.)
GEOMETRIC_REPRESENTATION_ITEM()
RATIONAL_B_SPLINE_SURFACE(((1.,0.668488966322264,1.),(1.,0.665851831765851,
1.),(1.,0.664481097979681,1.),(1.,0.664473794614064,1.)))
REPRESENTATION_ITEM('')
SURFACE()
);
#2202=(
BOUNDED_SURFACE()
B_SPLINE_SURFACE(3,2,((#144257,#144258,#144259),(#144260,#144261,#144262),
(#144263,#144264,#144265),(#144266,#144267,#144268)),.UNSPECIFIED.,.F.,
 .F.,.F.)
B_SPLINE_SURFACE_WITH_KNOTS((4,4),(3,3),(0.,0.000650122732446382),(0.,1.),
 .UNSPECIFIED.)
GEOMETRIC_REPRESENTATION_ITEM()
RATIONAL_B_SPLINE_SURFACE(((1.,0.714558059459819,1.),(1.,0.714557241617472,
1.),(1.,0.714330794970796,1.),(1.,0.71387929067142,1.)))
REPRESENTATION_ITEM('')
SURFACE()
);
#2203=(
BOUNDED_SURFACE()
B_SPLINE_SURFACE(3,2,((#144273,#144274,#144275),(#144276,#144277,#144278),
(#144279,#144280,#144281),(#144282,#144283,#144284),(#144285,#144286,#144287),
(#144288,#144289,#144290)),.UNSPECIFIED.,.F.,.F.,.F.)
B_SPLINE_SURFACE_WITH_KNOTS((4,2,4),(3,3),(0.,0.000414679582686121,0.000829359165372242),
(0.,1.),.UNSPECIFIED.)
GEOMETRIC_REPRESENTATION_ITEM()
RATIONAL_B_SPLINE_SURFACE(((1.,0.807089511457031,1.),(1.,0.806982451123016,
1.),(1.,0.808254776113455,1.),(1.,0.809251473726326,1.),(1.,0.80886183729917,
1.),(1.,0.804104907750028,1.)))
REPRESENTATION_ITEM('')
SURFACE()
);
#2204=(
BOUNDED_SURFACE()
B_SPLINE_SURFACE(3,2,((#144297,#144298,#144299),(#144300,#144301,#144302),
(#144303,#144304,#144305),(#144306,#144307,#144308)),.UNSPECIFIED.,.F.,
 .F.,.F.)
B_SPLINE_SURFACE_WITH_KNOTS((4,4),(3,3),(2.16840434497101E-19,0.000794016598505311),
(0.,1.),.UNSPECIFIED.)
GEOMETRIC_REPRESENTATION_ITEM()
RATIONAL_B_SPLINE_SURFACE(((1.,0.917068097704896,1.),(1.,0.931812274712855,
1.),(1.,0.942532558511199,1.),(1.,0.948460216910911,1.)))
REPRESENTATION_ITEM('')
SURFACE()
);
#2205=(
BOUNDED_SURFACE()
B_SPLINE_SURFACE(3,2,((#144328,#144329,#144330),(#144331,#144332,#144333),
(#144334,#144335,#144336),(#144337,#144338,#144339)),.UNSPECIFIED.,.F.,
 .F.,.F.)
B_SPLINE_SURFACE_WITH_KNOTS((4,4),(3,3),(0.,0.038317388945353),(0.,1.),
 .UNSPECIFIED.)
GEOMETRIC_REPRESENTATION_ITEM()
RATIONAL_B_SPLINE_SURFACE(((1.,0.716457303923414,1.),(1.,0.715285870443621,
1.),(1.,0.714517981140503,1.),(1.,0.713892198341303,1.)))
REPRESENTATION_ITEM('')
SURFACE()
);
#2206=(
BOUNDED_SURFACE()
B_SPLINE_SURFACE(3,2,((#144341,#144342,#144343),(#144344,#144345,#144346),
(#144347,#144348,#144349),(#144350,#144351,#144352)),.UNSPECIFIED.,.F.,
 .F.,.F.)
B_SPLINE_SURFACE_WITH_KNOTS((4,4),(3,3),(0.,0.0385835973699829),(0.,1.),
 .UNSPECIFIED.)
GEOMETRIC_REPRESENTATION_ITEM()
RATIONAL_B_SPLINE_SURFACE(((1.,0.713879290671428,1.),(1.,0.71450712730611,
1.),(1.,0.715277846561214,1.),(1.,0.716457303923418,1.)))
REPRESENTATION_ITEM('')
SURFACE()
);
#2207=(
BOUNDED_SURFACE()
B_SPLINE_SURFACE(3,2,((#144354,#144355,#144356),(#144357,#144358,#144359),
(#144360,#144361,#144362),(#144363,#144364,#144365)),.UNSPECIFIED.,.F.,
 .F.,.F.)
B_SPLINE_SURFACE_WITH_KNOTS((4,4),(3,3),(0.,0.00195778753723149),(0.,1.),
 .UNSPECIFIED.)
GEOMETRIC_REPRESENTATION_ITEM()
RATIONAL_B_SPLINE_SURFACE(((1.,0.707106781186543,1.),(1.,0.710074099671655,
1.),(1.,0.713236629341983,1.),(1.,0.716457303923398,1.)))
REPRESENTATION_ITEM('')
SURFACE()
);
#2208=(
BOUNDED_SURFACE()
B_SPLINE_SURFACE(3,2,((#144373,#144374,#144375),(#144376,#144377,#144378),
(#144379,#144380,#144381),(#144382,#144383,#144384)),.UNSPECIFIED.,.F.,
 .F.,.F.)
B_SPLINE_SURFACE_WITH_KNOTS((4,4),(3,3),(-4.11996825544492E-18,0.00195778789380024),
(0.,1.),.UNSPECIFIED.)
GEOMETRIC_REPRESENTATION_ITEM()
RATIONAL_B_SPLINE_SURFACE(((1.,0.716457303923414,1.),(1.,0.713268765085681,
1.),(1.,0.710104564531573,1.),(1.,0.707106781186529,1.)))
REPRESENTATION_ITEM('')
SURFACE()
);
#2209=(
BOUNDED_SURFACE()
B_SPLINE_SURFACE(3,2,((#144386,#144387,#144388),(#144389,#144390,#144391),
(#144392,#144393,#144394),(#144395,#144396,#144397),(#144398,#144399,#144400),
(#144401,#144402,#144403)),.UNSPECIFIED.,.F.,.F.,.F.)
B_SPLINE_SURFACE_WITH_KNOTS((4,2,4),(3,3),(0.024832888249526,0.028058706716499,
0.0312845251834718),(0.,1.),.UNSPECIFIED.)
GEOMETRIC_REPRESENTATION_ITEM()
RATIONAL_B_SPLINE_SURFACE(((1.,0.973275621725783,1.),(1.,0.974072863725218,
1.),(1.,0.974738796346974,1.),(1.,0.975743605366306,1.),(1.,0.976080910223402,
1.),(1.,0.976217656750926,1.)))
REPRESENTATION_ITEM('')
SURFACE()
);
#2210=(
BOUNDED_SURFACE()
B_SPLINE_SURFACE(3,2,((#144437,#144438,#144439),(#144440,#144441,#144442),
(#144443,#144444,#144445),(#144446,#144447,#144448)),.UNSPECIFIED.,.F.,
 .F.,.F.)
B_SPLINE_SURFACE_WITH_KNOTS((4,4),(3,3),(0.,0.0369876550821707),(0.,1.),
 .UNSPECIFIED.)
GEOMETRIC_REPRESENTATION_ITEM()
RATIONAL_B_SPLINE_SURFACE(((1.,0.668412873076039,1.),(1.,0.66485630627401,
1.),(1.,0.660493096380151,1.),(1.,0.653853118868808,1.)))
REPRESENTATION_ITEM('')
SURFACE()
);
#2211=(
BOUNDED_SURFACE()
B_SPLINE_SURFACE(3,2,((#144450,#144451,#144452),(#144453,#144454,#144455),
(#144456,#144457,#144458),(#144459,#144460,#144461),(#144462,#144463,#144464),
(#144465,#144466,#144467)),.UNSPECIFIED.,.F.,.F.,.F.)
B_SPLINE_SURFACE_WITH_KNOTS((4,2,4),(3,3),(0.,0.00108572934543333,0.00217145869086666),
(0.,1.),.UNSPECIFIED.)
GEOMETRIC_REPRESENTATION_ITEM()
RATIONAL_B_SPLINE_SURFACE(((1.,0.707106781186548,1.),(1.,0.698862672165929,
1.),(1.,0.690309395332211,1.),(1.,0.672521089753096,1.),(1.,0.663221545283971,
1.),(1.,0.653853118868808,1.)))
REPRESENTATION_ITEM('')
SURFACE()
);
#2212=(
BOUNDED_SURFACE()
B_SPLINE_SURFACE(3,2,((#144473,#144474,#144475),(#144476,#144477,#144478),
(#144479,#144480,#144481),(#144482,#144483,#144484),(#144485,#144486,#144487),
(#144488,#144489,#144490)),.UNSPECIFIED.,.F.,.F.,.F.)
B_SPLINE_SURFACE_WITH_KNOTS((4,2,4),(3,3),(-3.59995409638982E-5,0.00108574887884081,
0.00220749732422829),(0.,1.00003599956655),.UNSPECIFIED.)
GEOMETRIC_REPRESENTATION_ITEM()
RATIONAL_B_SPLINE_SURFACE(((1.,0.652908618523184,1.00002499027857),(1.,
0.662597041194131,1.00002429272054),(1.,0.672048287583566,1.00002361223899),
(1.,0.690435350993111,1.00002228838636),(1.,0.699430385989609,1.00002164075164),
(1.,0.70791464495416,1.00002102989235)))
REPRESENTATION_ITEM('')
SURFACE()
);
#2213=(
BOUNDED_SURFACE()
B_SPLINE_SURFACE(3,2,((#144517,#144518,#144519),(#144520,#144521,#144522),
(#144523,#144524,#144525),(#144526,#144527,#144528)),.UNSPECIFIED.,.F.,
 .F.,.F.)
B_SPLINE_SURFACE_WITH_KNOTS((4,4),(3,3),(0.,0.0372541843113205),(0.,1.),
 .UNSPECIFIED.)
GEOMETRIC_REPRESENTATION_ITEM()
RATIONAL_B_SPLINE_SURFACE(((1.,0.653853118868809,1.),(1.,0.660540277946251,
1.),(1.,0.664920252154014,1.),(1.,0.668488966322263,1.)))
REPRESENTATION_ITEM('')
SURFACE()
);
#2214=(
BOUNDED_SURFACE()
B_SPLINE_SURFACE(3,2,((#144534,#144535,#144536),(#144537,#144538,#144539),
(#144540,#144541,#144542),(#144543,#144544,#144545)),.UNSPECIFIED.,.F.,
 .F.,.F.)
B_SPLINE_SURFACE_WITH_KNOTS((4,4),(3,3),(0.,0.0358270578054484),(0.,1.),
 .UNSPECIFIED.)
GEOMETRIC_REPRESENTATION_ITEM()
RATIONAL_B_SPLINE_SURFACE(((1.,0.773031559588625,1.),(1.,0.765796148320668,
1.),(1.,0.760773695826815,1.),(1.,0.756642830410354,1.)))
REPRESENTATION_ITEM('')
SURFACE()
);
#2215=(
BOUNDED_SURFACE()
B_SPLINE_SURFACE(3,2,((#144547,#144548,#144549),(#144550,#144551,#144552),
(#144553,#144554,#144555),(#144556,#144557,#144558)),.UNSPECIFIED.,.F.,
 .F.,.F.)
B_SPLINE_SURFACE_WITH_KNOTS((4,4),(3,3),(0.,0.0360938777358061),(0.,1.),
 .UNSPECIFIED.)
GEOMETRIC_REPRESENTATION_ITEM()
RATIONAL_B_SPLINE_SURFACE(((1.,0.756551244268665,1.),(1.,0.760698019999951,
1.),(1.,0.765742819248909,1.),(1.,0.77303155958863,1.)))
REPRESENTATION_ITEM('')
SURFACE()
);
#2216=(
BOUNDED_SURFACE()
B_SPLINE_SURFACE(3,2,((#144560,#144561,#144562),(#144563,#144564,#144565),
(#144566,#144567,#144568),(#144569,#144570,#144571),(#144572,#144573,#144574),
(#144575,#144576,#144577)),.UNSPECIFIED.,.F.,.F.,.F.)
B_SPLINE_SURFACE_WITH_KNOTS((4,2,4),(3,3),(-2.53870287234617E-5,0.00117590500970525,
0.00237716614312564),(0.,1.00002538702872),.UNSPECIFIED.)
GEOMETRIC_REPRESENTATION_ITEM()
RATIONAL_B_SPLINE_SURFACE(((1.,0.706372183938724,1.0000149086756),(1.,0.717843868865426,
1.00001432621161),(1.,0.729214574731599,1.00001374887474),(1.,0.751742343795836,
1.0000126050485),(1.,0.762975777222459,1.0000120346815),(1.,0.773705940022985,
1.0000114898676)))
REPRESENTATION_ITEM('')
SURFACE()
);
#2217=(
BOUNDED_SURFACE()
B_SPLINE_SURFACE(3,2,((#144609,#144610,#144611),(#144612,#144613,#144614),
(#144615,#144616,#144617),(#144618,#144619,#144620),(#144621,#144622,#144623),
(#144624,#144625,#144626)),.UNSPECIFIED.,.F.,.F.,.F.)
B_SPLINE_SURFACE_WITH_KNOTS((4,2,4),(3,3),(0.,0.00117596609447381,0.00235193218894761),
(0.,1.),.UNSPECIFIED.)
GEOMETRIC_REPRESENTATION_ITEM()
RATIONAL_B_SPLINE_SURFACE(((1.,0.773031559588625,1.),(1.,0.762507689934388,
1.),(1.,0.751714784265694,1.),(1.,0.729663967046365,1.),(1.,0.718328240933523,
1.),(1.,0.707106781186548,1.)))
REPRESENTATION_ITEM('')
SURFACE()
);
#2218=(
BOUNDED_SURFACE()
B_SPLINE_SURFACE(3,2,((#144633,#144634,#144635),(#144636,#144637,#144638),
(#144639,#144640,#144641),(#144642,#144643,#144644),(#144645,#144646,#144647),
(#144648,#144649,#144650)),.UNSPECIFIED.,.F.,.F.,.F.)
B_SPLINE_SURFACE_WITH_KNOTS((4,2,4),(3,3),(0.0131958327712131,0.0172517018793722,
0.0213075709875312),(0.,1.),.UNSPECIFIED.)
GEOMETRIC_REPRESENTATION_ITEM()
RATIONAL_B_SPLINE_SURFACE(((1.,0.962986864031359,1.),(1.,0.964634124968522,
1.),(1.,0.966223563289428,1.),(1.,0.969200421482677,1.),(1.,0.970562510847277,
1.),(1.,0.97174760310377,1.)))
REPRESENTATION_ITEM('')
SURFACE()
);
#2219=(
BOUNDED_SURFACE()
B_SPLINE_SURFACE(3,2,((#144674,#144675,#144676),(#144677,#144678,#144679),
(#144680,#144681,#144682),(#144683,#144684,#144685)),.UNSPECIFIED.,.F.,
 .F.,.F.)
B_SPLINE_SURFACE_WITH_KNOTS((4,4),(3,3),(0.,0.0319950621716305),(0.,1.),
 .UNSPECIFIED.)
GEOMETRIC_REPRESENTATION_ITEM()
RATIONAL_B_SPLINE_SURFACE(((1.,0.619604282534389,1.),(1.,0.612421729644488,
1.),(1.,0.603704627405285,1.),(1.,0.591243989422539,1.)))
REPRESENTATION_ITEM('')
SURFACE()
);
#2220=(
BOUNDED_SURFACE()
B_SPLINE_SURFACE(3,2,((#144687,#144688,#144689),(#144690,#144691,#144692),
(#144693,#144694,#144695),(#144696,#144697,#144698),(#144699,#144700,#144701),
(#144702,#144703,#144704)),.UNSPECIFIED.,.F.,.F.,.F.)
B_SPLINE_SURFACE_WITH_KNOTS((4,2,4),(3,3),(0.,0.00145467289932797,0.00290934579865593),
(0.,1.),.UNSPECIFIED.)
GEOMETRIC_REPRESENTATION_ITEM()
RATIONAL_B_SPLINE_SURFACE(((1.,0.707106781186548,1.),(1.,0.689351003959322,
1.),(1.,0.670875374619751,1.),(1.,0.63219865253591,1.),(1.,0.61183462187758,
1.),(1.,0.591243989422533,1.)))
REPRESENTATION_ITEM('')
SURFACE()
);
#2221=(
BOUNDED_SURFACE()
B_SPLINE_SURFACE(3,2,((#144710,#144711,#144712),(#144713,#144714,#144715),
(#144716,#144717,#144718),(#144719,#144720,#144721),(#144722,#144723,#144724),
(#144725,#144726,#144727)),.UNSPECIFIED.,.F.,.F.,.F.)
B_SPLINE_SURFACE_WITH_KNOTS((4,2,4),(3,3),(-0.000112903673830276,0.00145505538520654,
0.00302301461672063),(0.,1.00011290384629),.UNSPECIFIED.)
GEOMETRIC_REPRESENTATION_ITEM()
RATIONAL_B_SPLINE_SURFACE(((0.999999999999999,0.586393787062724,1.00009339546458),
(1.,0.608684432923124,1.00008836206527),(1.,0.630255928913141,1.00008349105554),
(1.,0.671993040490121,1.00007406649468),(1.,0.692297992883085,1.00006948148023),
(1.,0.711173028308929,1.00006521935203)))
REPRESENTATION_ITEM('')
SURFACE()
);
#2222=(
BOUNDED_SURFACE()
B_SPLINE_SURFACE(3,2,((#144757,#144758,#144759),(#144760,#144761,#144762),
(#144763,#144764,#144765),(#144766,#144767,#144768)),.UNSPECIFIED.,.F.,
 .F.,.F.)
B_SPLINE_SURFACE_WITH_KNOTS((4,4),(3,3),(0.,0.0322629186945109),(0.,1.),
 .UNSPECIFIED.)
GEOMETRIC_REPRESENTATION_ITEM()
RATIONAL_B_SPLINE_SURFACE(((1.,0.591243989422541,1.),(1.,0.603807915079894,
1.),(1.,0.612569262394175,1.),(1.,0.619783312569531,1.)))
REPRESENTATION_ITEM('')
SURFACE()
);
#2223=(
BOUNDED_SURFACE()
B_SPLINE_SURFACE(3,2,((#144785,#144786,#144787),(#144788,#144789,#144790),
(#144791,#144792,#144793),(#144794,#144795,#144796)),.UNSPECIFIED.,.F.,
 .F.,.F.)
B_SPLINE_SURFACE_WITH_KNOTS((4,4),(3,3),(0.,0.0298008594779328),(0.,1.),
 .UNSPECIFIED.)
GEOMETRIC_REPRESENTATION_ITEM()
RATIONAL_B_SPLINE_SURFACE(((1.,0.819627815321769,1.),(1.,0.81028158060527,
1.),(1.,0.803135207628788,1.),(1.,0.797103929716951,1.)))
REPRESENTATION_ITEM('')
SURFACE()
);
#2224=(
BOUNDED_SURFACE()
B_SPLINE_SURFACE(3,2,((#144798,#144799,#144800),(#144801,#144802,#144803),
(#144804,#144805,#144806),(#144807,#144808,#144809)),.UNSPECIFIED.,.F.,
 .F.,.F.)
B_SPLINE_SURFACE_WITH_KNOTS((4,4),(3,3),(0.,0.0300693678107436),(0.,1.),
 .UNSPECIFIED.)
GEOMETRIC_REPRESENTATION_ITEM()
RATIONAL_B_SPLINE_SURFACE(((1.,0.79694160937888,1.),(1.,0.803005840650144,
1.),(1.,0.810197796192684,1.),(1.,0.819627815321757,1.)))
REPRESENTATION_ITEM('')
SURFACE()
);
#2225=(
BOUNDED_SURFACE()
B_SPLINE_SURFACE(3,2,((#144811,#144812,#144813),(#144814,#144815,#144816),
(#144817,#144818,#144819),(#144820,#144821,#144822),(#144823,#144824,#144825),
(#144826,#144827,#144828)),.UNSPECIFIED.,.F.,.F.,.F.)
B_SPLINE_SURFACE_WITH_KNOTS((4,2,4),(3,3),(-8.43401684374147E-5,0.00160216910094088,
0.00328860201455053),(0.,1.00008434016844),.UNSPECIFIED.)
GEOMETRIC_REPRESENTATION_ITEM()
RATIONAL_B_SPLINE_SURFACE(((1.,0.703841529342767,1.0000499561106),(1.,0.725491849855086,
1.00004630412724),(1.,0.746131243723142,1.00004282266733),(1.,0.785697186856154,
1.00003614867071),(1.,0.804770925859817,1.00003293130599),(1.,0.822243584210538,
1.0000299840121)))
REPRESENTATION_ITEM('')
SURFACE()
);
#2226=(
BOUNDED_SURFACE()
B_SPLINE_SURFACE(3,2,((#144863,#144864,#144865),(#144866,#144867,#144868),
(#144869,#144870,#144871),(#144872,#144873,#144874),(#144875,#144876,#144877),
(#144878,#144879,#144880)),.UNSPECIFIED.,.F.,.F.,.F.)
B_SPLINE_SURFACE_WITH_KNOTS((4,2,4),(3,3),(0.,0.00160286774303482,0.00320573548606963),
(0.,1.),.UNSPECIFIED.)
GEOMETRIC_REPRESENTATION_ITEM()
RATIONAL_B_SPLINE_SURFACE(((1.,0.819627815321769,1.),(1.,0.802865620897526,
1.),(1.,0.785107826354221,1.),(1.,0.747495184421159,1.),(1.,0.727508688529169,
1.),(1.,0.707106781186548,1.)))
REPRESENTATION_ITEM('')
SURFACE()
);
#2227=(
BOUNDED_SURFACE()
B_SPLINE_SURFACE(3,2,((#144893,#144894,#144895),(#144896,#144897,#144898),
(#144899,#144900,#144901),(#144902,#144903,#144904),(#144905,#144906,#144907),
(#144908,#144909,#144910)),.UNSPECIFIED.,.F.,.F.,.F.)
B_SPLINE_SURFACE_WITH_KNOTS((4,2,4),(3,3),(0.28787290846928,0.292960043496213,
0.298047178523145),(0.,1.),.UNSPECIFIED.)
GEOMETRIC_REPRESENTATION_ITEM()
RATIONAL_B_SPLINE_SURFACE(((1.,0.948000837587232,1.),(1.,0.950253148926149,
1.),(1.,0.952526342948766,1.),(1.,0.957029990073055,1.),(1.,0.959243464400477,
1.),(1.,0.961372004230729,1.)))
REPRESENTATION_ITEM('')
SURFACE()
);
#2228=(
BOUNDED_SURFACE()
B_SPLINE_SURFACE(3,2,((#144934,#144935,#144936),(#144937,#144938,#144939),
(#144940,#144941,#144942),(#144943,#144944,#144945)),.UNSPECIFIED.,.F.,
 .F.,.F.)
B_SPLINE_SURFACE_WITH_KNOTS((4,4),(3,3),(1.38777878078145E-17,0.0238258198664154),
(0.,1.),.UNSPECIFIED.)
GEOMETRIC_REPRESENTATION_ITEM()
RATIONAL_B_SPLINE_SURFACE(((1.,0.566606711022863,1.),(1.,0.557709627588123,
1.),(1.,0.547241836069268,1.),(1.,0.533775524284033,1.)))
REPRESENTATION_ITEM('')
SURFACE()
);
#2229=(
BOUNDED_SURFACE()
B_SPLINE_SURFACE(3,2,((#144947,#144948,#144949),(#144950,#144951,#144952),
(#144953,#144954,#144955),(#144956,#144957,#144958),(#144959,#144960,#144961),
(#144962,#144963,#144964)),.UNSPECIFIED.,.F.,.F.,.F.)
B_SPLINE_SURFACE_WITH_KNOTS((4,2,4),(3,3),(0.,0.00196532227871992,0.00393064455743984),
(0.,1.),.UNSPECIFIED.)
GEOMETRIC_REPRESENTATION_ITEM()
RATIONAL_B_SPLINE_SURFACE(((1.,0.70710678118655,1.),(1.,0.681045297773967,
1.),(1.,0.653805231917789,1.),(1.,0.596033371554667,1.),(1.,0.565216504169612,
1.),(1.,0.533775524284038,1.)))
REPRESENTATION_ITEM('')
SURFACE()
);
#2230=(
BOUNDED_SURFACE()
B_SPLINE_SURFACE(3,2,((#144970,#144971,#144972),(#144973,#144974,#144975),
(#144976,#144977,#144978),(#144979,#144980,#144981),(#144982,#144983,#144984),
(#144985,#144986,#144987)),.UNSPECIFIED.,.F.,.F.,.F.)
B_SPLINE_SURFACE_WITH_KNOTS((4,2,4),(3,3),(-0.000393284609852448,0.00196642364705715,
0.00432613202352569),(0.,1.00045991623863),.UNSPECIFIED.)
GEOMETRIC_REPRESENTATION_ITEM()
RATIONAL_B_SPLINE_SURFACE(((1.,0.514485821122662,1.0004465917099),(1.,0.552975432690279,
1.00041118771514),(1.,0.589408021414007,1.0003776758368),(1.,0.658978456167228,
1.00031368269146),(1.,0.692168964479326,1.00028315298398),(1.,0.722275405990915,
1.0002554601013)))
REPRESENTATION_ITEM('')
SURFACE()
);
#2231=(
BOUNDED_SURFACE()
B_SPLINE_SURFACE(3,2,((#145020,#145021,#145022),(#145023,#145024,#145025),
(#145026,#145027,#145028),(#145029,#145030,#145031)),.UNSPECIFIED.,.F.,
 .F.,.F.)
B_SPLINE_SURFACE_WITH_KNOTS((4,4),(3,3),(0.,0.0240963563036403),(0.,1.),
 .UNSPECIFIED.)
GEOMETRIC_REPRESENTATION_ITEM()
RATIONAL_B_SPLINE_SURFACE(((1.,0.533775524284036,1.),(1.,0.547394060950047,
1.),(1.,0.557948204678947,1.),(1.,0.566908467907053,1.)))
REPRESENTATION_ITEM('')
SURFACE()
);
#2232=(
BOUNDED_SURFACE()
B_SPLINE_SURFACE(3,2,((#145058,#145059,#145060),(#145061,#145062,#145063),
(#145064,#145065,#145066),(#145067,#145068,#145069)),.UNSPECIFIED.,.F.,
 .F.,.F.)
B_SPLINE_SURFACE_WITH_KNOTS((4,4),(3,3),(0.,8.95703543583319E-5),(0.,1.),
 .UNSPECIFIED.)
GEOMETRIC_REPRESENTATION_ITEM()
RATIONAL_B_SPLINE_SURFACE(((1.,0.821022196159299,1.),(1.,0.818079073177133,
1.),(1.,0.814610488520586,1.),(1.,0.810617639934139,1.)))
REPRESENTATION_ITEM('')
SURFACE()
);
#2233=(
BOUNDED_SURFACE()
B_SPLINE_SURFACE(3,2,((#145071,#145072,#145073),(#145074,#145075,#145076),
(#145077,#145078,#145079),(#145080,#145081,#145082),(#145083,#145084,#145085),
(#145086,#145087,#145088),(#145089,#145090,#145091),(#145092,#145093,#145094)),
 .UNSPECIFIED.,.F.,.F.,.F.)
B_SPLINE_SURFACE_WITH_KNOTS((4,2,2,4),(3,3),(0.,0.000301902853038141,0.000452854279557211,
0.000603805706076282),(0.,1.),.UNSPECIFIED.)
GEOMETRIC_REPRESENTATION_ITEM()
RATIONAL_B_SPLINE_SURFACE(((1.,0.702399276808562,1.),(1.,0.672208297052869,
1.),(1.,0.639172707788597,1.),(1.,0.593013313775285,1.),(1.,0.577958663413849,
1.),(1.,0.550545486207946,1.),(1.,0.538469268822416,1.),(1.,0.528679393385783,
1.)))
REPRESENTATION_ITEM('')
SURFACE()
);
#2234=(
BOUNDED_SURFACE()
B_SPLINE_SURFACE(3,2,((#145096,#145097,#145098),(#145099,#145100,#145101),
(#145102,#145103,#145104),(#145105,#145106,#145107)),.UNSPECIFIED.,.F.,
 .F.,.F.)
B_SPLINE_SURFACE_WITH_KNOTS((4,4),(3,3),(0.,0.024690830875569),(0.,1.),
 .UNSPECIFIED.)
GEOMETRIC_REPRESENTATION_ITEM()
RATIONAL_B_SPLINE_SURFACE(((1.,0.821022196159299,1.),(1.,0.827229968384993,
1.),(1.,0.834396885388283,1.),(1.,0.84317661051583,1.)))
REPRESENTATION_ITEM('')
SURFACE()
);
#2235=(
BOUNDED_SURFACE()
B_SPLINE_SURFACE(3,2,((#145109,#145110,#145111),(#145112,#145113,#145114),
(#145115,#145116,#145117),(#145118,#145119,#145120),(#145121,#145122,#145123),
(#145124,#145125,#145126)),.UNSPECIFIED.,.F.,.F.,.F.)
B_SPLINE_SURFACE_WITH_KNOTS((4,2,4),(3,3),(-0.000125633631190664,0.00192660600180124,
0.00397876574878657),(0.,1.00012563363119),.UNSPECIFIED.)
GEOMETRIC_REPRESENTATION_ITEM()
RATIONAL_B_SPLINE_SURFACE(((1.,0.702058786892261,1.00007486287297),(1.,
0.729454174087526,1.00006797930903),(1.,0.755057429332917,1.00006154604917),
(1.,0.803448625603955,1.00004938692576),(1.,0.826420664059153,1.00004361480455),
(1.,0.846952528006408,1.0000384558193)))
REPRESENTATION_ITEM('')
SURFACE()
);
#2236=(
BOUNDED_SURFACE()
B_SPLINE_SURFACE(3,2,((#145167,#145168,#145169),(#145170,#145171,#145172),
(#145173,#145174,#145175),(#145176,#145177,#145178),(#145179,#145180,#145181),
(#145182,#145183,#145184)),.UNSPECIFIED.,.F.,.F.,.F.)
B_SPLINE_SURFACE_WITH_KNOTS((4,2,4),(3,3),(-0.000277756685671561,0.00176358033920161,
0.00380491746723071),(0.,1.00027775678883),.UNSPECIFIED.)
GEOMETRIC_REPRESENTATION_ITEM()
RATIONAL_B_SPLINE_SURFACE(((1.,0.541612572103269,1.00025464044002),(1.,
0.573730160641759,1.00023679868351),(1.,0.60443290548972,1.00021974289187),
(1.,0.66339296977674,1.00018698977562),(1.,0.691792553884413,1.00017121342105),
(1.,0.717755310902421,1.00015679075701)))
REPRESENTATION_ITEM('')
SURFACE()
);
#2237=(
BOUNDED_SURFACE()
B_SPLINE_SURFACE(3,2,((#145186,#145187,#145188),(#145189,#145190,#145191),
(#145192,#145193,#145194),(#145195,#145196,#145197)),.UNSPECIFIED.,.F.,
 .F.,.F.)
B_SPLINE_SURFACE_WITH_KNOTS((4,4),(3,3),(0.,0.0278605201857756),(0.,1.),
 .UNSPECIFIED.)
GEOMETRIC_REPRESENTATION_ITEM()
RATIONAL_B_SPLINE_SURFACE(((1.,0.55476848021506,1.),(1.,0.56887897086178,
1.),(1.,0.579290070452688,1.),(1.,0.587985430396658,1.)))
REPRESENTATION_ITEM('')
SURFACE()
);
#2238=(
BOUNDED_SURFACE()
B_SPLINE_SURFACE(3,2,((#145198,#145199,#145200),(#145201,#145202,#145203),
(#145204,#145205,#145206),(#145207,#145208,#145209)),.UNSPECIFIED.,.F.,
 .F.,.F.)
B_SPLINE_SURFACE_WITH_KNOTS((4,4),(3,3),(-1.38777878078145E-17,0.0333345287175385),
(0.,1.),.UNSPECIFIED.)
GEOMETRIC_REPRESENTATION_ITEM()
RATIONAL_B_SPLINE_SURFACE(((1.,0.779737900546642,1.),(1.,0.785266544814036,
1.),(1.,0.791920621206337,1.),(1.,0.801085834760578,1.)))
REPRESENTATION_ITEM('')
SURFACE()
);
#2239=(
BOUNDED_SURFACE()
B_SPLINE_SURFACE(3,2,((#145211,#145212,#145213),(#145214,#145215,#145216),
(#145217,#145218,#145219),(#145220,#145221,#145222)),.UNSPECIFIED.,.F.,
 .F.,.F.)
B_SPLINE_SURFACE_WITH_KNOTS((4,4),(3,3),(0.,9.64176041888312E-5),(0.,1.),
 .UNSPECIFIED.)
GEOMETRIC_REPRESENTATION_ITEM()
RATIONAL_B_SPLINE_SURFACE(((1.,0.801085834760579,1.),(1.,0.800109483270879,
1.),(1.,0.799128688610329,1.),(1.,0.798143461627153,1.)))
REPRESENTATION_ITEM('')
SURFACE()
);
#2240=(
BOUNDED_SURFACE()
B_SPLINE_SURFACE(3,2,((#145223,#145224,#145225),(#145226,#145227,#145228),
(#145229,#145230,#145231),(#145232,#145233,#145234)),.UNSPECIFIED.,.F.,
 .F.,.F.)
B_SPLINE_SURFACE_WITH_KNOTS((4,4),(3,3),(0.,0.0333425790106738),(0.,1.),
 .UNSPECIFIED.)
GEOMETRIC_REPRESENTATION_ITEM()
RATIONAL_B_SPLINE_SURFACE(((1.,0.619253049823353,1.),(1.,0.62903050118076,
1.),(1.,0.635777469330956,1.),(1.,0.641321251913794,1.)))
REPRESENTATION_ITEM('')
SURFACE()
);
#2241=(
BOUNDED_SURFACE()
B_SPLINE_SURFACE(3,2,((#145235,#145236,#145237),(#145238,#145239,#145240),
(#145241,#145242,#145243),(#145244,#145245,#145246)),.UNSPECIFIED.,.F.,
 .F.,.F.)
B_SPLINE_SURFACE_WITH_KNOTS((4,4),(3,3),(-1.38777878078145E-17,0.0332202089949022),
(0.,1.),.UNSPECIFIED.)
GEOMETRIC_REPRESENTATION_ITEM()
RATIONAL_B_SPLINE_SURFACE(((1.,0.736495153922513,1.),(1.,0.738798609451216,
1.),(1.,0.741580133014481,1.),(1.,0.745472778587061,1.)))
REPRESENTATION_ITEM('')
SURFACE()
);
#2242=(
BOUNDED_SURFACE()
B_SPLINE_SURFACE(3,2,((#145285,#145286,#145287),(#145288,#145289,#145290),
(#145291,#145292,#145293),(#145294,#145295,#145296)),.UNSPECIFIED.,.F.,
 .F.,.F.)
B_SPLINE_SURFACE_WITH_KNOTS((4,4),(3,3),(-3.41800396632663E-5,0.000687703280430334),
(0.,1.00003418003966),.UNSPECIFIED.)
GEOMETRIC_REPRESENTATION_ITEM()
RATIONAL_B_SPLINE_SURFACE(((1.,0.549976566282829,1.00003076363763),(1.,
0.549294416403988,1.00003081026945),(1.,0.555643671106273,1.00003037623389),
(1.,0.567819410633178,1.00002954389937)))
REPRESENTATION_ITEM('')
SURFACE()
);
#2243=(
BOUNDED_SURFACE()
B_SPLINE_SURFACE(3,2,((#145300,#145301,#145302),(#145303,#145304,#145305),
(#145306,#145307,#145308),(#145309,#145310,#145311),(#145312,#145313,#145314),
(#145315,#145316,#145317)),.UNSPECIFIED.,.F.,.F.,.F.)
B_SPLINE_SURFACE_WITH_KNOTS((4,2,4),(3,3),(1.38777878078145E-17,0.0146992078328598,
0.0293984156657196),(0.,1.),.UNSPECIFIED.)
GEOMETRIC_REPRESENTATION_ITEM()
RATIONAL_B_SPLINE_SURFACE(((1.,0.566144048133053,1.),(1.,0.560653267979146,
1.),(1.,0.554543800692172,1.),(1.,0.540492753126539,1.),(1.,0.532555598048173,
1.),(1.,0.523250899838466,1.)))
REPRESENTATION_ITEM('')
SURFACE()
);
#2244=(
BOUNDED_SURFACE()
B_SPLINE_SURFACE(3,2,((#145326,#145327,#145328),(#145329,#145330,#145331),
(#145332,#145333,#145334),(#145335,#145336,#145337),(#145338,#145339,#145340),
(#145341,#145342,#145343)),.UNSPECIFIED.,.F.,.F.,.F.)
B_SPLINE_SURFACE_WITH_KNOTS((4,2,4),(3,3),(0.,0.00207126900955203,0.00414253801910405),
(0.,1.),.UNSPECIFIED.)
GEOMETRIC_REPRESENTATION_ITEM()
RATIONAL_B_SPLINE_SURFACE(((1.,0.707106781186548,1.),(1.,0.679626330234824,
1.),(1.,0.650848145227602,1.),(1.,0.589569252159033,1.),(1.,0.556778618705704,
1.),(1.,0.523250899838466,1.)))
REPRESENTATION_ITEM('')
SURFACE()
);
#2245=(
BOUNDED_SURFACE()
B_SPLINE_SURFACE(3,2,((#145356,#145357,#145358),(#145359,#145360,#145361),
(#145362,#145363,#145364),(#145365,#145366,#145367),(#145368,#145369,#145370),
(#145371,#145372,#145373)),.UNSPECIFIED.,.F.,.F.,.F.)
B_SPLINE_SURFACE_WITH_KNOTS((4,2,4),(3,3),(-0.000414433024293954,0.00207216577676188,
0.00455876470887616),(0.,1.00057450279771),.UNSPECIFIED.)
GEOMETRIC_REPRESENTATION_ITEM()
RATIONAL_B_SPLINE_SURFACE(((1.,0.502594029997045,1.00057152224273),(1.,
0.543754583372273,1.00052422853659),(1.,0.582517660127345,1.0004796895445),
(1.,0.656326486548337,1.00039488278995),(1.,0.691338987574868,1.00035465323036),
(1.,0.723071803322265,1.00031819204751)))
REPRESENTATION_ITEM('')
SURFACE()
);
#2246=(
BOUNDED_SURFACE()
B_SPLINE_SURFACE(3,2,((#145406,#145407,#145408),(#145409,#145410,#145411),
(#145412,#145413,#145414),(#145415,#145416,#145417),(#145418,#145419,#145420),
(#145421,#145422,#145423)),.UNSPECIFIED.,.F.,.F.,.F.)
B_SPLINE_SURFACE_WITH_KNOTS((4,2,4),(3,3),(0.,0.0145632072393804,0.0291264144787609),
(0.,1.),.UNSPECIFIED.)
GEOMETRIC_REPRESENTATION_ITEM()
RATIONAL_B_SPLINE_SURFACE(((1.,0.523250899838464,1.),(1.,0.532471350763147,
1.),(1.,0.540347653844846,1.),(1.,0.554302832144208,1.),(1.,0.560377433574518,
1.),(1.,0.565840417962188,1.)))
REPRESENTATION_ITEM('')
SURFACE()
);
#2247=(
BOUNDED_SURFACE()
B_SPLINE_SURFACE(3,2,((#145430,#145431,#145432),(#145433,#145434,#145435),
(#145436,#145437,#145438),(#145439,#145440,#145441),(#145442,#145443,#145444),
(#145445,#145446,#145447)),.UNSPECIFIED.,.F.,.F.,.F.)
B_SPLINE_SURFACE_WITH_KNOTS((4,2,4),(3,3),(0.320579494062015,0.325851056440119,
0.331122618818223),(0.,1.),.UNSPECIFIED.)
GEOMETRIC_REPRESENTATION_ITEM()
RATIONAL_B_SPLINE_SURFACE(((1.,0.944716550693843,1.),(1.,0.947183014496352,
1.),(1.,0.949681733718157,1.),(1.,0.954674150124444,1.),(1.,0.957142659869515,
1.),(1.,0.959530911310534,1.)))
REPRESENTATION_ITEM('')
SURFACE()
);
#2248=(
BOUNDED_SURFACE()
B_SPLINE_SURFACE(3,2,((#145499,#145500,#145501),(#145502,#145503,#145504),
(#145505,#145506,#145507),(#145508,#145509,#145510),(#145511,#145512,#145513),
(#145514,#145515,#145516)),.UNSPECIFIED.,.F.,.F.,.F.)
B_SPLINE_SURFACE_WITH_KNOTS((4,2,4),(3,3),(0.,0.0176980703187956,0.0353961406375911),
(0.,1.),.UNSPECIFIED.)
GEOMETRIC_REPRESENTATION_ITEM()
RATIONAL_B_SPLINE_SURFACE(((1.,0.797648081014877,1.),(1.,0.801243745289675,
1.),(1.,0.805251011590647,1.),(1.,0.814487862093865,1.),(1.,0.819714636457853,
1.),(1.,0.825853968826193,1.)))
REPRESENTATION_ITEM('')
SURFACE()
);
#2249=(
BOUNDED_SURFACE()
B_SPLINE_SURFACE(3,2,((#145518,#145519,#145520),(#145521,#145522,#145523),
(#145524,#145525,#145526),(#145527,#145528,#145529),(#145530,#145531,#145532),
(#145533,#145534,#145535)),.UNSPECIFIED.,.F.,.F.,.F.)
B_SPLINE_SURFACE_WITH_KNOTS((4,2,4),(3,3),(-9.9063038639367E-5,0.00167878022781669,
0.00345653198876773),(0.,1.00009906303864),.UNSPECIFIED.)
GEOMETRIC_REPRESENTATION_ITEM()
RATIONAL_B_SPLINE_SURFACE(((0.999999999999999,0.70321690031505,1.00005880047134),
(1.,0.726378747565388,1.0000542115054),(1.,0.748363388483742,1.00004985577474),
(1.,0.790366013422709,1.00004153395942),(1.,0.810543585884598,1.00003753625614),
(1.,0.828922930782749,1.00003389482864)))
REPRESENTATION_ITEM('')
SURFACE()
);
#2250=(
BOUNDED_SURFACE()
B_SPLINE_SURFACE(3,2,((#145541,#145542,#145543),(#145544,#145545,#145546),
(#145547,#145548,#145549),(#145550,#145551,#145552),(#145553,#145554,#145555),
(#145556,#145557,#145558)),.UNSPECIFIED.,.F.,.F.,.F.)
B_SPLINE_SURFACE_WITH_KNOTS((4,2,4),(3,3),(-3.90312782094781E-18,0.00167965794371986,
0.00335931588743972),(0.,1.),.UNSPECIFIED.)
GEOMETRIC_REPRESENTATION_ITEM()
RATIONAL_B_SPLINE_SURFACE(((1.,0.825853968826192,1.),(1.,0.808295365083271,
1.),(1.,0.789625920673805,1.),(1.,0.749928217285841,1.),(1.,0.728769006116152,
1.),(1.,0.707106781186548,1.)))
REPRESENTATION_ITEM('')
SURFACE()
);
#2251=(
BOUNDED_SURFACE()
B_SPLINE_SURFACE(3,2,((#145567,#145568,#145569),(#145570,#145571,#145572),
(#145573,#145574,#145575),(#145576,#145577,#145578),(#145579,#145580,#145581),
(#145582,#145583,#145584)),.UNSPECIFIED.,.F.,.F.,.F.)
B_SPLINE_SURFACE_WITH_KNOTS((4,2,4),(3,3),(0.,0.0178323395635859,0.0356646791271718),
(0.,1.),.UNSPECIFIED.)
GEOMETRIC_REPRESENTATION_ITEM()
RATIONAL_B_SPLINE_SURFACE(((1.,0.825853968826192,1.),(1.,0.819668171116131,
1.),(1.,0.814408476706928,1.),(1.,0.80512037347301,1.),(1.,0.801094867709694,
1.),(1.,0.79748483152198,1.)))
REPRESENTATION_ITEM('')
SURFACE()
);
#2252=(
BOUNDED_SURFACE()
B_SPLINE_SURFACE(3,2,((#145593,#145594,#145595),(#145596,#145597,#145598),
(#145599,#145600,#145601),(#145602,#145603,#145604)),.UNSPECIFIED.,.F.,
 .F.,.F.)
B_SPLINE_SURFACE_WITH_KNOTS((4,4),(3,3),(-6.51957114117417E-5,0.000717152825529202),
(0.,1.0001395156952),.UNSPECIFIED.)
GEOMETRIC_REPRESENTATION_ITEM()
RATIONAL_B_SPLINE_SURFACE(((1.,0.795687417707187,1.00005700962391),(1.,
0.80308940810469,1.00005494423624),(1.,0.806595093358397,1.00005396604001),
(1.,0.80591968995395,1.00005415449876)))
REPRESENTATION_ITEM('')
SURFACE()
);
#2253=(
BOUNDED_SURFACE()
B_SPLINE_SURFACE(3,2,((#145638,#145639,#145640),(#145641,#145642,#145643),
(#145644,#145645,#145646),(#145647,#145648,#145649),(#145650,#145651,#145652),
(#145653,#145654,#145655)),.UNSPECIFIED.,.F.,.F.,.F.)
B_SPLINE_SURFACE_WITH_KNOTS((4,2,4),(3,3),(0.,0.0188568492058762,0.0377136984117525),
(0.,1.),.UNSPECIFIED.)
GEOMETRIC_REPRESENTATION_ITEM()
RATIONAL_B_SPLINE_SURFACE(((1.,0.583115115460263,1.),(1.,0.591477165975886,
1.),(1.,0.59822556054293,1.),(1.,0.609817503669346,1.),(1.,0.614651018359553,
1.),(1.,0.618903611686376,1.)))
REPRESENTATION_ITEM('')
SURFACE()
);
#2254=(
BOUNDED_SURFACE()
B_SPLINE_SURFACE(3,2,((#145673,#145674,#145675),(#145676,#145677,#145678),
(#145679,#145680,#145681),(#145682,#145683,#145684)),.UNSPECIFIED.,.F.,
 .F.,.F.)
B_SPLINE_SURFACE_WITH_KNOTS((4,4),(3,3),(-6.51408174375087E-5,0.000716548991812596),
(0.,1.00012715075799),.UNSPECIFIED.)
GEOMETRIC_REPRESENTATION_ITEM()
RATIONAL_B_SPLINE_SURFACE(((1.,0.609559938200355,1.00009928949961),(1.,
0.608772413245087,1.0000994897684),(1.,0.612737943163139,1.00009848132813),
(1.,0.621014916147782,1.00009637648136)))
REPRESENTATION_ITEM('')
SURFACE()
);
#2255=(
BOUNDED_SURFACE()
B_SPLINE_SURFACE(3,2,((#145688,#145689,#145690),(#145691,#145692,#145693),
(#145694,#145695,#145696),(#145697,#145698,#145699),(#145700,#145701,#145702),
(#145703,#145704,#145705)),.UNSPECIFIED.,.F.,.F.,.F.)
B_SPLINE_SURFACE_WITH_KNOTS((4,2,4),(3,3),(0.,0.018990790064314,0.0379815801286281),
(0.,1.),.UNSPECIFIED.)
GEOMETRIC_REPRESENTATION_ITEM()
RATIONAL_B_SPLINE_SURFACE(((1.,0.619084183929308,1.),(1.,0.61481875400451,
1.),(1.,0.609968099232784,1.),(1.,0.598321687913226,1.),(1.,0.591536257853193,
1.),(1.,0.583115115460264,1.)))
REPRESENTATION_ITEM('')
SURFACE()
);
#2256=(
BOUNDED_SURFACE()
B_SPLINE_SURFACE(3,2,((#145714,#145715,#145716),(#145717,#145718,#145719),
(#145720,#145721,#145722),(#145723,#145724,#145725),(#145726,#145727,#145728),
(#145729,#145730,#145731)),.UNSPECIFIED.,.F.,.F.,.F.)
B_SPLINE_SURFACE_WITH_KNOTS((4,2,4),(3,3),(0.,0.00151694200897944,0.00303388401795888),
(0.,1.),.UNSPECIFIED.)
GEOMETRIC_REPRESENTATION_ITEM()
RATIONAL_B_SPLINE_SURFACE(((1.,0.70710678118655,1.),(1.,0.688185240537986,
1.),(1.,0.6684652198449,1.),(1.,0.627083641349078,1.),(1.,0.605243055947471,
1.),(1.,0.583115115460264,1.)))
REPRESENTATION_ITEM('')
SURFACE()
);
#2257=(
BOUNDED_SURFACE()
B_SPLINE_SURFACE(3,2,((#145744,#145745,#145746),(#145747,#145748,#145749),
(#145750,#145751,#145752),(#145753,#145754,#145755),(#145756,#145757,#145758),
(#145759,#145760,#145761)),.UNSPECIFIED.,.F.,.F.,.F.)
B_SPLINE_SURFACE_WITH_KNOTS((4,2,4),(3,3),(-0.000134068678628998,0.00151741931723474,
0.00316890735964793),(0.,1.00013406872517),.UNSPECIFIED.)
GEOMETRIC_REPRESENTATION_ITEM()
RATIONAL_B_SPLINE_SURFACE(((1.,0.577176787432037,1.00011337473816),(1.,
0.601399673404762,1.00010687967528),(1.,0.624769559778014,1.00010061333353),
(1.,0.669881131114838,1.00008851723181),(1.,0.691769778729462,1.00008264806565),
(1.,0.712034386796128,1.00007721436531)))
REPRESENTATION_ITEM('')
SURFACE()
);
#2258=(
BOUNDED_SURFACE()
B_SPLINE_SURFACE(3,2,((#145790,#145791,#145792),(#145793,#145794,#145795),
(#145796,#145797,#145798),(#145799,#145800,#145801),(#145802,#145803,#145804),
(#145805,#145806,#145807),(#145808,#145809,#145810),(#145811,#145812,#145813)),
 .UNSPECIFIED.,.F.,.F.,.F.)
B_SPLINE_SURFACE_WITH_KNOTS((4,2,2,4),(3,3),(0.017818580704263,0.0199004486313254,
0.0219823165583878,0.0261460524125126),(0.,1.),.UNSPECIFIED.)
GEOMETRIC_REPRESENTATION_ITEM()
RATIONAL_B_SPLINE_SURFACE(((1.,0.961171308030857,1.),(1.,0.962092810628593,
1.),(1.,0.963001088261132,1.),(1.,0.964780402726978,1.),(1.,0.965653853257041,
1.),(1.,0.968176214233281,1.),(1.,0.969729042204957,1.),(1.,0.971089731516655,
1.)))
REPRESENTATION_ITEM('')
SURFACE()
);
#2259=(
BOUNDED_SURFACE()
B_SPLINE_SURFACE(3,2,((#145859,#145860,#145861),(#145862,#145863,#145864),
(#145865,#145866,#145867),(#145868,#145869,#145870)),.UNSPECIFIED.,.F.,
 .F.,.F.)
B_SPLINE_SURFACE_WITH_KNOTS((4,4),(3,3),(-8.32667268468867E-17,0.0417901757617077),
(0.,1.),.UNSPECIFIED.)
GEOMETRIC_REPRESENTATION_ITEM()
RATIONAL_B_SPLINE_SURFACE(((1.,0.757216058458815,1.),(1.,0.76211005468913,
1.),(1.,0.768141195659961,1.),(1.,0.777664586555055,1.)))
REPRESENTATION_ITEM('')
SURFACE()
);
#2260=(
BOUNDED_SURFACE()
B_SPLINE_SURFACE(3,2,((#145872,#145873,#145874),(#145875,#145876,#145877),
(#145878,#145879,#145880),(#145881,#145882,#145883),(#145884,#145885,#145886),
(#145887,#145888,#145889)),.UNSPECIFIED.,.F.,.F.,.F.)
B_SPLINE_SURFACE_WITH_KNOTS((4,2,4),(3,3),(-2.92956119863222E-5,0.00120613678608598,
0.00244151698435041),(0.,1.00002929561199),.UNSPECIFIED.)
GEOMETRIC_REPRESENTATION_ITEM()
RATIONAL_B_SPLINE_SURFACE(((1.,0.706220266280328,1.00001721291418),(1.,
0.718564407685336,1.00001648965582),(1.,0.730784372547602,1.00001577367312),
(1.,0.754961474849659,1.00001435710711),(1.,0.767001288465581,1.00001365167969),
(1.,0.778473732954666,1.00001297949513)))
REPRESENTATION_ITEM('')
SURFACE()
);
#2261=(
BOUNDED_SURFACE()
B_SPLINE_SURFACE(3,2,((#145895,#145896,#145897),(#145898,#145899,#145900),
(#145901,#145902,#145903),(#145904,#145905,#145906),(#145907,#145908,#145909),
(#145910,#145911,#145912)),.UNSPECIFIED.,.F.,.F.,.F.)
B_SPLINE_SURFACE_WITH_KNOTS((4,2,4),(3,3),(0.,0.00120620763625507,0.00241241527251014),
(0.,1.),.UNSPECIFIED.)
GEOMETRIC_REPRESENTATION_ITEM()
RATIONAL_B_SPLINE_SURFACE(((1.,0.777664586555049,1.),(1.,0.766436783957212,
1.),(1.,0.754901973237173,1.),(1.,0.73129895059372,1.),(1.,0.719146552484787,
1.),(1.,0.707106781186548,1.)))
REPRESENTATION_ITEM('')
SURFACE()
);
#2262=(
BOUNDED_SURFACE()
B_SPLINE_SURFACE(3,2,((#145921,#145922,#145923),(#145924,#145925,#145926),
(#145927,#145928,#145929),(#145930,#145931,#145932)),.UNSPECIFIED.,.F.,
 .F.,.F.)
B_SPLINE_SURFACE_WITH_KNOTS((4,4),(3,3),(0.,0.0420570108120997),(0.,1.),
 .UNSPECIFIED.)
GEOMETRIC_REPRESENTATION_ITEM()
RATIONAL_B_SPLINE_SURFACE(((1.,0.777664586555049,1.),(1.,0.768081385918698,
1.),(1.,0.762031405880593,1.),(1.,0.757123446310248,1.)))
REPRESENTATION_ITEM('')
SURFACE()
);
#2263=(
BOUNDED_SURFACE()
B_SPLINE_SURFACE(3,2,((#145939,#145940,#145941),(#145942,#145943,#145944),
(#145945,#145946,#145947),(#145948,#145949,#145950)),.UNSPECIFIED.,.F.,
 .F.,.F.)
B_SPLINE_SURFACE_WITH_KNOTS((4,4),(3,3),(-6.50609804213592E-5,0.000715670784634903),
(0.,1.00019732104438),.UNSPECIFIED.)
GEOMETRIC_REPRESENTATION_ITEM()
RATIONAL_B_SPLINE_SURFACE(((1.,0.756066809424476,1.00009626630384),(1.,
0.760288887453374,1.00009460009415),(1.,0.762267398805321,1.0000938192903),
(1.,0.761887769744426,1.00009396910791)))
REPRESENTATION_ITEM('')
SURFACE()
);
#2264=(
BOUNDED_SURFACE()
B_SPLINE_SURFACE(3,2,((#145955,#145956,#145957),(#145958,#145959,#145960),
(#145961,#145962,#145963),(#145964,#145965,#145966),(#145967,#145968,#145969),
(#145970,#145971,#145972),(#145973,#145974,#145975),(#145976,#145977,#145978),
(#145979,#145980,#145981),(#145982,#145983,#145984),(#145985,#145986,#145987),
(#145988,#145989,#145990),(#145991,#145992,#145993),(#145994,#145995,#145996)),
 .UNSPECIFIED.,.F.,.F.,.F.)
B_SPLINE_SURFACE_WITH_KNOTS((4,2,2,2,2,2,4),(3,3),(0.00808011141552929,
0.00881517523662049,0.00918270714716608,0.00955023905771168,0.00991777096825728,
0.0102853028788029,0.0110203666998941),(0.,1.),.UNSPECIFIED.)
GEOMETRIC_REPRESENTATION_ITEM()
RATIONAL_B_SPLINE_SURFACE(((1.,0.707106781186548,1.),(1.,0.708672362536739,
1.),(1.,0.710198222857537,1.),(1.,0.712427305746575,1.),(1.,0.71315813872198,
1.),(1.,0.714551782754775,1.),(1.,0.715220876802376,1.),(1.,0.71650348303418,
1.),(1.,0.717121230234592,1.),(1.,0.718264550261012,1.),(1.,0.718793336138408,
1.),(1.,0.720253112545596,1.),(1.,0.721064801594907,1.),(1.,0.721643051700349,
1.)))
REPRESENTATION_ITEM('')
SURFACE()
);
#2265=(
BOUNDED_SURFACE()
B_SPLINE_SURFACE(3,2,((#146035,#146036,#146037),(#146038,#146039,#146040),
(#146041,#146042,#146043),(#146044,#146045,#146046)),.UNSPECIFIED.,.F.,
 .F.,.F.)
B_SPLINE_SURFACE_WITH_KNOTS((4,4),(3,3),(0.,0.0430361525536219),(0.,1.),
 .UNSPECIFIED.)
GEOMETRIC_REPRESENTATION_ITEM()
RATIONAL_B_SPLINE_SURFACE(((1.,0.649397749909071,1.),(1.,0.658290092659334,
1.),(1.,0.663526138769308,1.),(1.,0.667763418073535,1.)))
REPRESENTATION_ITEM('')
SURFACE()
);
#2266=(
BOUNDED_SURFACE()
B_SPLINE_SURFACE(3,2,((#146048,#146049,#146050),(#146051,#146052,#146053),
(#146054,#146055,#146056),(#146057,#146058,#146059),(#146060,#146061,#146062),
(#146063,#146064,#146065),(#146066,#146067,#146068),(#146069,#146070,#146071),
(#146072,#146073,#146074),(#146075,#146076,#146077),(#146078,#146079,#146080),
(#146081,#146082,#146083),(#146084,#146085,#146086),(#146087,#146088,#146089)),
 .UNSPECIFIED.,.F.,.F.,.F.)
B_SPLINE_SURFACE_WITH_KNOTS((4,2,2,2,2,2,4),(3,3),(0.0080803797182093,0.00879690254712659,
0.00915516396158524,0.00951342537604388,0.00987168679050253,0.0102299482049612,
0.0109464710338785),(0.,1.),.UNSPECIFIED.)
GEOMETRIC_REPRESENTATION_ITEM()
RATIONAL_B_SPLINE_SURFACE(((1.,0.707106781186548,1.),(1.,0.705537440672151,
1.),(1.,0.703998083945123,1.),(1.,0.701735656940981,1.),(1.,0.700989163179782,
1.),(1.,0.699560461823081,1.),(1.,0.698871897343629,1.),(1.,0.697546947950716,
1.),(1.,0.696905752213842,1.),(1.,0.695707159507179,1.),(1.,0.695149875554341,
1.),(1.,0.693602432259692,1.),(1.,0.692727265033204,1.),(1.,0.692079067931822,
1.)))
REPRESENTATION_ITEM('')
SURFACE()
);
#2267=(
BOUNDED_SURFACE()
B_SPLINE_SURFACE(3,2,((#146151,#146152,#146153),(#146154,#146155,#146156),
(#146157,#146158,#146159),(#146160,#146161,#146162)),.UNSPECIFIED.,.F.,
 .F.,.F.)
B_SPLINE_SURFACE_WITH_KNOTS((4,4),(3,3),(0.,0.000650375609766158),(0.,1.),
 .UNSPECIFIED.)
GEOMETRIC_REPRESENTATION_ITEM()
RATIONAL_B_SPLINE_SURFACE(((1.,0.663756004792833,1.),(1.,0.663759519746911,
1.),(1.,0.665134391960157,1.),(1.,0.66784082710355,1.)))
REPRESENTATION_ITEM('')
SURFACE()
);
#2268=(
BOUNDED_SURFACE()
B_SPLINE_SURFACE(3,2,((#146166,#146167,#146168),(#146169,#146170,#146171),
(#146172,#146173,#146174),(#146175,#146176,#146177)),.UNSPECIFIED.,.F.,
 .F.,.F.)
B_SPLINE_SURFACE_WITH_KNOTS((4,4),(3,3),(-2.77555756156289E-17,0.0433026927553429),
(0.,1.),.UNSPECIFIED.)
GEOMETRIC_REPRESENTATION_ITEM()
RATIONAL_B_SPLINE_SURFACE(((1.,0.667840827103545,1.),(1.,0.66359300941018,
1.),(1.,0.658343952018749,1.),(1.,0.649397749909072,1.)))
REPRESENTATION_ITEM('')
SURFACE()
);
#2269=(
BOUNDED_SURFACE()
B_SPLINE_SURFACE(3,2,((#146184,#146185,#146186),(#146187,#146188,#146189),
(#146190,#146191,#146192),(#146193,#146194,#146195),(#146196,#146197,#146198),
(#146199,#146200,#146201)),.UNSPECIFIED.,.F.,.F.,.F.)
B_SPLINE_SURFACE_WITH_KNOTS((4,2,4),(3,3),(0.,0.00110388220976991,0.00220776441953981),
(0.,1.),.UNSPECIFIED.)
GEOMETRIC_REPRESENTATION_ITEM()
RATIONAL_B_SPLINE_SURFACE(((1.,0.707106781186548,1.),(1.,0.69822152219183,
1.),(1.,0.68897986867167,1.),(1.,0.66970545013756,1.),(1.,0.659601845960695,
1.),(1.,0.649397749909072,1.)))
REPRESENTATION_ITEM('')
SURFACE()
);
#2270=(
BOUNDED_SURFACE()
B_SPLINE_SURFACE(3,2,((#146215,#146216,#146217),(#146218,#146219,#146220),
(#146221,#146222,#146223),(#146224,#146225,#146226),(#146227,#146228,#146229),
(#146230,#146231,#146232)),.UNSPECIFIED.,.F.,.F.,.F.)
B_SPLINE_SURFACE_WITH_KNOTS((4,2,4),(3,3),(-4.18082381682501E-5,0.00110390261829224,
0.00224961359036052),(0.,1.00004180835378),.UNSPECIFIED.)
GEOMETRIC_REPRESENTATION_ITEM()
RATIONAL_B_SPLINE_SURFACE(((1.,0.648223184306046,1.00002941441912),(1.,
0.658829102191687,1.00002852758719),(1.,0.669145628051642,1.00002766495326),
(1.,0.68916060951258,1.00002599136641),(1.,0.698923845802076,1.00002517499674),
(1.,0.708101577151724,1.00002440758506)))
REPRESENTATION_ITEM('')
SURFACE()
);
#2271=(
BOUNDED_SURFACE()
B_SPLINE_SURFACE(3,2,((#146258,#146259,#146260),(#146261,#146262,#146263),
(#146264,#146265,#146266),(#146267,#146268,#146269),(#146270,#146271,#146272),
(#146273,#146274,#146275)),.UNSPECIFIED.,.F.,.F.,.F.)
B_SPLINE_SURFACE_WITH_KNOTS((4,2,4),(3,3),(0.012499301108314,0.0157975372010094,
0.0190957732937049),(0.,1.),.UNSPECIFIED.)
GEOMETRIC_REPRESENTATION_ITEM()
RATIONAL_B_SPLINE_SURFACE(((1.,0.976191060180328,1.),(1.,0.976018964367352,
1.),(1.,0.975629721882182,1.),(1.,0.974451430140223,1.),(1.,0.97367913510036,
1.),(1.,0.972768244198254,1.)))
REPRESENTATION_ITEM('')
SURFACE()
);
#2272=(
BOUNDED_SURFACE()
B_SPLINE_SURFACE(3,2,((#146300,#146301,#146302),(#146303,#146304,#146305),
(#146306,#146307,#146308),(#146309,#146310,#146311)),.UNSPECIFIED.,.F.,
 .F.,.F.)
B_SPLINE_SURFACE_WITH_KNOTS((4,4),(3,3),(0.,0.0444870989094409),(0.,1.),
 .UNSPECIFIED.)
GEOMETRIC_REPRESENTATION_ITEM()
RATIONAL_B_SPLINE_SURFACE(((1.,0.71449972514277,1.),(1.,0.715296138993144,
1.),(1.,0.71628014758797,1.),(1.,0.717952606100523,1.)))
REPRESENTATION_ITEM('')
SURFACE()
);
#2273=(
BOUNDED_SURFACE()
B_SPLINE_SURFACE(3,2,((#146313,#146314,#146315),(#146316,#146317,#146318),
(#146319,#146320,#146321),(#146322,#146323,#146324)),.UNSPECIFIED.,.F.,
 .F.,.F.)
B_SPLINE_SURFACE_WITH_KNOTS((4,4),(3,3),(0.,0.00196035438616165),(0.,1.),
 .UNSPECIFIED.)
GEOMETRIC_REPRESENTATION_ITEM()
RATIONAL_B_SPLINE_SURFACE(((1.,0.707106781186548,1.),(1.,0.710533388681839,
1.),(1.,0.714200483631581,1.),(1.,0.717952606100467,1.)))
REPRESENTATION_ITEM('')
SURFACE()
);
#2274=(
BOUNDED_SURFACE()
B_SPLINE_SURFACE(3,2,((#146330,#146331,#146332),(#146333,#146334,#146335),
(#146336,#146337,#146338),(#146339,#146340,#146341)),.UNSPECIFIED.,.F.,
 .F.,.F.)
B_SPLINE_SURFACE_WITH_KNOTS((4,4),(3,3),(-3.90312782094781E-18,0.0019603544817943),
(0.,1.),.UNSPECIFIED.)
GEOMETRIC_REPRESENTATION_ITEM()
RATIONAL_B_SPLINE_SURFACE(((1.,0.717952606100523,1.),(1.,0.714237876912109,
1.),(1.,0.710568615888393,1.),(1.,0.707106781186514,1.)))
REPRESENTATION_ITEM('')
SURFACE()
);
#2275=(
BOUNDED_SURFACE()
B_SPLINE_SURFACE(3,2,((#146345,#146346,#146347),(#146348,#146349,#146350),
(#146351,#146352,#146353),(#146354,#146355,#146356)),.UNSPECIFIED.,.F.,
 .F.,.F.)
B_SPLINE_SURFACE_WITH_KNOTS((4,4),(3,3),(0.,0.044753309356401),(0.,1.),
 .UNSPECIFIED.)
GEOMETRIC_REPRESENTATION_ITEM()
RATIONAL_B_SPLINE_SURFACE(((1.,0.717952606100523,1.),(1.,0.716270361073643,
1.),(1.,0.715283994577086,1.),(1.,0.714485667734334,1.)))
REPRESENTATION_ITEM('')
SURFACE()
);
#2276=(
BOUNDED_SURFACE()
B_SPLINE_SURFACE(3,2,((#146363,#146364,#146365),(#146366,#146367,#146368),
(#146369,#146370,#146371),(#146372,#146373,#146374)),.UNSPECIFIED.,.F.,
 .F.,.F.)
B_SPLINE_SURFACE_WITH_KNOTS((4,4),(3,3),(0.,0.000650124428678587),(0.,1.),
 .UNSPECIFIED.)
GEOMETRIC_REPRESENTATION_ITEM()
RATIONAL_B_SPLINE_SURFACE(((1.,0.714485667734326,1.),(1.,0.714973119513317,
1.),(1.,0.715223297464931,1.),(1.,0.715224866856049,1.)))
REPRESENTATION_ITEM('')
SURFACE()
);
#2277=(
BOUNDED_SURFACE()
B_SPLINE_SURFACE(3,2,((#146379,#146380,#146381),(#146382,#146383,#146384),
(#146385,#146386,#146387),(#146388,#146389,#146390),(#146391,#146392,#146393),
(#146394,#146395,#146396),(#146397,#146398,#146399),(#146400,#146401,#146402),
(#146403,#146404,#146405),(#146406,#146407,#146408)),.UNSPECIFIED.,.F.,
 .F.,.F.)
B_SPLINE_SURFACE_WITH_KNOTS((4,2,2,2,4),(3,3),(0.00807569768389314,0.00867847980331418,
0.00928126192273523,0.00988404404215627,0.0104868261615773),(0.,1.),
 .UNSPECIFIED.)
GEOMETRIC_REPRESENTATION_ITEM()
RATIONAL_B_SPLINE_SURFACE(((1.,0.707106781186548,1.),(1.,0.707212493429049,
1.),(1.,0.707315385014487,1.),(1.,0.707515784384109,1.),(1.,0.707613608127955,
1.),(1.,0.707793680404111,1.),(1.,0.707878261047732,1.),(1.,0.708029744860286,
1.),(1.,0.7080959680978,1.),(1.,0.708153025875396,1.)))
REPRESENTATION_ITEM('')
SURFACE()
);
#2278=(
BOUNDED_SURFACE()
B_SPLINE_SURFACE(3,2,((#146476,#146477,#146478),(#146479,#146480,#146481),
(#146482,#146483,#146484),(#146485,#146486,#146487)),.UNSPECIFIED.,.F.,
 .F.,.F.)
B_SPLINE_SURFACE_WITH_KNOTS((4,4),(3,3),(0.,0.0445045070401677),(0.,1.),
 .UNSPECIFIED.)
GEOMETRIC_REPRESENTATION_ITEM()
RATIONAL_B_SPLINE_SURFACE(((1.,0.71617462512364,1.),(1.,0.714773807595299,
1.),(1.,0.713950503107743,1.),(1.,0.713284154090124,1.)))
REPRESENTATION_ITEM('')
SURFACE()
);
#2279=(
BOUNDED_SURFACE()
B_SPLINE_SURFACE(3,2,((#146489,#146490,#146491),(#146492,#146493,#146494),
(#146495,#146496,#146497),(#146498,#146499,#146500),(#146501,#146502,#146503),
(#146504,#146505,#146506),(#146507,#146508,#146509),(#146510,#146511,#146512),
(#146513,#146514,#146515),(#146516,#146517,#146518)),.UNSPECIFIED.,.F.,
 .F.,.F.)
B_SPLINE_SURFACE_WITH_KNOTS((4,2,2,2,4),(3,3),(0.0080756712423913,0.00867825313759154,
0.00928083503279179,0.00988341692799203,0.0104859988231923),(0.,1.),
 .UNSPECIFIED.)
GEOMETRIC_REPRESENTATION_ITEM()
RATIONAL_B_SPLINE_SURFACE(((1.,0.707106781186548,1.),(1.,0.707146901961909,
1.),(1.,0.707185957443845,1.),(1.,0.707262034097608,1.),(1.,0.707299176477847,
1.),(1.,0.7073675568103,1.),(1.,0.707399679105567,1.),(1.,0.707457223307409,
1.),(1.,0.707482383732919,1.),(1.,0.707504065565917,1.)))
REPRESENTATION_ITEM('')
SURFACE()
);
#2280=(
BOUNDED_SURFACE()
B_SPLINE_SURFACE(3,2,((#146545,#146546,#146547),(#146548,#146549,#146550),
(#146551,#146552,#146553),(#146554,#146555,#146556)),.UNSPECIFIED.,.F.,
 .F.,.F.)
B_SPLINE_SURFACE_WITH_KNOTS((4,4),(3,3),(0.,0.000650121327073412),(0.,1.),
 .UNSPECIFIED.)
GEOMETRIC_REPRESENTATION_ITEM()
RATIONAL_B_SPLINE_SURFACE(((1.,0.713890629234418,1.),(1.,0.713889885788569,
1.),(1.,0.71368362023966,1.),(1.,0.713272398106985,1.)))
REPRESENTATION_ITEM('')
SURFACE()
);
#2281=(
BOUNDED_SURFACE()
B_SPLINE_SURFACE(3,2,((#146560,#146561,#146562),(#146563,#146564,#146565),
(#146566,#146567,#146568),(#146569,#146570,#146571)),.UNSPECIFIED.,.F.,
 .F.,.F.)
B_SPLINE_SURFACE_WITH_KNOTS((4,4),(3,3),(0.,0.0447707136167657),(0.,1.),
 .UNSPECIFIED.)
GEOMETRIC_REPRESENTATION_ITEM()
RATIONAL_B_SPLINE_SURFACE(((1.,0.713272398106993,1.),(1.,0.713940344609358,
1.),(1.,0.714765614654658,1.),(1.,0.71617462512364,1.)))
REPRESENTATION_ITEM('')
SURFACE()
);
#2282=(
BOUNDED_SURFACE()
B_SPLINE_SURFACE(3,2,((#146578,#146579,#146580),(#146581,#146582,#146583),
(#146584,#146585,#146586),(#146587,#146588,#146589)),.UNSPECIFIED.,.F.,
 .F.,.F.)
B_SPLINE_SURFACE_WITH_KNOTS((4,4),(3,3),(0.,0.00195732360009946),(0.,1.),
 .UNSPECIFIED.)
GEOMETRIC_REPRESENTATION_ITEM()
RATIONAL_B_SPLINE_SURFACE(((1.,0.707106781186548,1.),(1.,0.709967301734631,
1.),(1.,0.713032729764421,1.),(1.,0.716174625123614,1.)))
REPRESENTATION_ITEM('')
SURFACE()
);
#2283=(
BOUNDED_SURFACE()
B_SPLINE_SURFACE(3,2,((#146597,#146598,#146599),(#146600,#146601,#146602),
(#146603,#146604,#146605),(#146606,#146607,#146608)),.UNSPECIFIED.,.F.,
 .F.,.F.)
B_SPLINE_SURFACE_WITH_KNOTS((4,4),(3,3),(0.,0.00195732365556561),(0.,1.),
 .UNSPECIFIED.)
GEOMETRIC_REPRESENTATION_ITEM()
RATIONAL_B_SPLINE_SURFACE(((1.,0.71617462512364,1.),(1.,0.713064019807532,
1.),(1.,0.709996713322441,1.),(1.,0.707106781186534,1.)))
REPRESENTATION_ITEM('')
SURFACE()
);
#2284=(
BOUNDED_SURFACE()
B_SPLINE_SURFACE(3,2,((#146610,#146611,#146612),(#146613,#146614,#146615),
(#146616,#146617,#146618),(#146619,#146620,#146621),(#146622,#146623,#146624),
(#146625,#146626,#146627),(#146628,#146629,#146630),(#146631,#146632,#146633)),
 .UNSPECIFIED.,.F.,.F.,.F.)
B_SPLINE_SURFACE_WITH_KNOTS((4,2,2,4),(3,3),(0.023727979672696,0.0269788291349169,
0.0286042538660274,0.0302296785971378),(0.,1.),.UNSPECIFIED.)
GEOMETRIC_REPRESENTATION_ITEM()
RATIONAL_B_SPLINE_SURFACE(((1.,0.972985060853882,1.),(1.,0.973867966894579,
1.),(1.,0.974606628833735,1.),(1.,0.975438732489742,1.),(1.,0.975670772749385,
1.),(1.,0.976026965697327,1.),(1.,0.976152018462137,1.),(1.,0.976223679017856,
1.)))
REPRESENTATION_ITEM('')
SURFACE()
);
#2285=(
BOUNDED_SURFACE()
B_SPLINE_SURFACE(3,2,((#146667,#146668,#146669),(#146670,#146671,#146672),
(#146673,#146674,#146675),(#146676,#146677,#146678)),.UNSPECIFIED.,.F.,
 .F.,.F.)
B_SPLINE_SURFACE_WITH_KNOTS((4,4),(3,3),(-1.38777878078145E-17,0.0431305646498159),
(0.,1.),.UNSPECIFIED.)
GEOMETRIC_REPRESENTATION_ITEM()
RATIONAL_B_SPLINE_SURFACE(((1.,0.669061697655964,1.),(1.,0.66495869705799,
1.),(1.,0.659888610517475,1.),(1.,0.65126854630498,1.)))
REPRESENTATION_ITEM('')
SURFACE()
);
#2286=(
BOUNDED_SURFACE()
B_SPLINE_SURFACE(3,2,((#146680,#146681,#146682),(#146683,#146684,#146685),
(#146686,#146687,#146688),(#146689,#146690,#146691),(#146692,#146693,#146694),
(#146695,#146696,#146697)),.UNSPECIFIED.,.F.,.F.,.F.)
B_SPLINE_SURFACE_WITH_KNOTS((4,2,4),(3,3),(0.,0.00109598668217933,0.00219197336435865),
(0.,1.),.UNSPECIFIED.)
GEOMETRIC_REPRESENTATION_ITEM()
RATIONAL_B_SPLINE_SURFACE(((1.,0.707106781186548,1.),(1.,0.698507203291837,
1.),(1.,0.689563761715544,1.),(1.,0.670914228806854,1.),(1.,0.661139818833385,
1.),(1.,0.65126854630498,1.)))
REPRESENTATION_ITEM('')
SURFACE()
);
#2287=(
BOUNDED_SURFACE()
B_SPLINE_SURFACE(3,2,((#146703,#146704,#146705),(#146706,#146707,#146708),
(#146709,#146710,#146711),(#146712,#146713,#146714),(#146715,#146716,#146717),
(#146718,#146719,#146720)),.UNSPECIFIED.,.F.,.F.,.F.)
B_SPLINE_SURFACE_WITH_KNOTS((4,2,4),(3,3),(-4.05963276307181E-5,0.00109600456666539,
0.0022326050184341),(0.,1.00004059633081),.UNSPECIFIED.)
GEOMETRIC_REPRESENTATION_ITEM()
RATIONAL_B_SPLINE_SURFACE(((1.,0.650157040100188,1.00002840468107),(1.,
0.660408047293388,1.00002757237451),(1.,0.670380682621654,1.0000267626697),
(1.,0.689731025456819,1.00002519156386),(1.,0.699171182287062,1.0000244250924),
(1.,0.708048211870778,1.00002370434275)))
REPRESENTATION_ITEM('')
SURFACE()
);
#2288=(
BOUNDED_SURFACE()
B_SPLINE_SURFACE(3,2,((#146748,#146749,#146750),(#146751,#146752,#146753),
(#146754,#146755,#146756),(#146757,#146758,#146759)),.UNSPECIFIED.,.F.,
 .F.,.F.)
B_SPLINE_SURFACE_WITH_KNOTS((4,4),(3,3),(0.,0.0433970829567688),(0.,1.),
 .UNSPECIFIED.)
GEOMETRIC_REPRESENTATION_ITEM()
RATIONAL_B_SPLINE_SURFACE(((1.,0.651268546304981,1.),(1.,0.659940697395559,
1.),(1.,0.665023311775857,1.),(1.,0.669136477740405,1.)))
REPRESENTATION_ITEM('')
SURFACE()
);
#2289=(
BOUNDED_SURFACE()
B_SPLINE_SURFACE(3,2,((#146766,#146767,#146768),(#146769,#146770,#146771),
(#146772,#146773,#146774),(#146775,#146776,#146777)),.UNSPECIFIED.,.F.,
 .F.,.F.)
B_SPLINE_SURFACE_WITH_KNOTS((4,4),(3,3),(0.,0.000650363027228679),(0.,1.),
 .UNSPECIFIED.)
GEOMETRIC_REPRESENTATION_ITEM()
RATIONAL_B_SPLINE_SURFACE(((1.,0.66913647774042,1.),(1.,0.666544790513632,
1.),(1.,0.665198010610878,1.),(1.,0.665190809887722,1.)))
REPRESENTATION_ITEM('')
SURFACE()
);
#2290=(
BOUNDED_SURFACE()
B_SPLINE_SURFACE(3,2,((#146782,#146783,#146784),(#146785,#146786,#146787),
(#146788,#146789,#146790),(#146791,#146792,#146793),(#146794,#146795,#146796),
(#146797,#146798,#146799),(#146800,#146801,#146802),(#146803,#146804,#146805),
(#146806,#146807,#146808),(#146809,#146810,#146811),(#146812,#146813,#146814),
(#146815,#146816,#146817),(#146818,#146819,#146820),(#146821,#146822,#146823)),
 .UNSPECIFIED.,.F.,.F.,.F.)
B_SPLINE_SURFACE_WITH_KNOTS((4,2,2,2,2,2,4),(3,3),(0.00808046157075938,
0.00879095475051749,0.00914620134039654,0.0095014479302756,0.00985669452015465,
0.0102119411100337,0.0109224342897918),(0.,1.),.UNSPECIFIED.)
GEOMETRIC_REPRESENTATION_ITEM()
RATIONAL_B_SPLINE_SURFACE(((1.,0.707106781186552,1.),(1.,0.705538120216095,
1.),(1.,0.703999772329756,1.),(1.,0.701739154413458,1.),(1.,0.700992634705956,
1.),(1.,0.699563445722461,1.),(1.,0.698874516085242,1.),(1.,0.697548436732303,
1.),(1.,0.696906638208049,1.),(1.,0.695703451829647,1.),(1.,0.695143596113536,
1.),(1.,0.693587190992306,1.),(1.,0.692704331853457,1.),(1.,0.69204248906153,
1.)))
REPRESENTATION_ITEM('')
SURFACE()
);
#2291=(
BOUNDED_SURFACE()
B_SPLINE_SURFACE(3,2,((#146895,#146896,#146897),(#146898,#146899,#146900),
(#146901,#146902,#146903),(#146904,#146905,#146906)),.UNSPECIFIED.,.F.,
 .F.,.F.)
B_SPLINE_SURFACE_WITH_KNOTS((4,4),(3,3),(0.,0.0419168978153696),(0.,1.),
 .UNSPECIFIED.)
GEOMETRIC_REPRESENTATION_ITEM()
RATIONAL_B_SPLINE_SURFACE(((1.,0.776159951988518,1.),(1.,0.766788671732685,
1.),(1.,0.760870494736068,1.),(1.,0.756069167758398,1.)))
REPRESENTATION_ITEM('')
SURFACE()
);
#2292=(
BOUNDED_SURFACE()
B_SPLINE_SURFACE(3,2,((#146908,#146909,#146910),(#146911,#146912,#146913),
(#146914,#146915,#146916),(#146917,#146918,#146919),(#146920,#146921,#146922),
(#146923,#146924,#146925),(#146926,#146927,#146928),(#146929,#146930,#146931),
(#146932,#146933,#146934),(#146935,#146936,#146937),(#146938,#146939,#146940),
(#146941,#146942,#146943),(#146944,#146945,#146946),(#146947,#146948,#146949)),
 .UNSPECIFIED.,.F.,.F.,.F.)
B_SPLINE_SURFACE_WITH_KNOTS((4,2,2,2,2,2,4),(3,3),(0.00808024661615471,
0.00880850598034447,0.00917263566243935,0.00953676534453423,0.00990089502662911,
0.010265024708724,0.0109932840729137),(0.,1.),.UNSPECIFIED.)
GEOMETRIC_REPRESENTATION_ITEM()
RATIONAL_B_SPLINE_SURFACE(((1.,0.707106781186552,1.),(1.,0.7086803042033,
1.),(1.,0.710213526000588,1.),(1.,0.712453026336305,1.),(1.,0.713188114139461,
1.),(1.,0.714590095265908,1.),(1.,0.715263343050717,1.),(1.,0.716554408796435,
1.),(1.,0.71717678241798,1.),(1.,0.718331565221162,1.),(1.,0.718866152975084,
1.),(1.,0.720344053893136,1.),(1.,0.721169771392395,1.),(1.,0.721765931188049,
1.)))
REPRESENTATION_ITEM('')
SURFACE()
);
#2293=(
BOUNDED_SURFACE()
B_SPLINE_SURFACE(3,2,((#146974,#146975,#146976),(#146977,#146978,#146979),
(#146980,#146981,#146982),(#146983,#146984,#146985)),.UNSPECIFIED.,.F.,
 .F.,.F.)
B_SPLINE_SURFACE_WITH_KNOTS((4,4),(3,3),(0.,0.000650577858517379),(0.,1.),
 .UNSPECIFIED.)
GEOMETRIC_REPRESENTATION_ITEM()
RATIONAL_B_SPLINE_SURFACE(((1.,0.760728353039955,1.),(1.,0.760722617942438,
1.),(1.,0.759141109939139,1.),(1.,0.755978609126096,1.)))
REPRESENTATION_ITEM('')
SURFACE()
);
#2294=(
BOUNDED_SURFACE()
B_SPLINE_SURFACE(3,2,((#146989,#146990,#146991),(#146992,#146993,#146994),
(#146995,#146996,#146997),(#146998,#146999,#147000)),.UNSPECIFIED.,.F.,
 .F.,.F.)
B_SPLINE_SURFACE_WITH_KNOTS((4,4),(3,3),(0.,0.0421837023697854),(0.,1.),
 .UNSPECIFIED.)
GEOMETRIC_REPRESENTATION_ITEM()
RATIONAL_B_SPLINE_SURFACE(((1.,0.755978609126094,1.),(1.,0.760793534959097,
1.),(1.,0.766730014383061,1.),(1.,0.776159951988524,1.)))
REPRESENTATION_ITEM('')
SURFACE()
);
#2295=(
BOUNDED_SURFACE()
B_SPLINE_SURFACE(3,2,((#147007,#147008,#147009),(#147010,#147011,#147012),
(#147013,#147014,#147015),(#147016,#147017,#147018),(#147019,#147020,#147021),
(#147022,#147023,#147024)),.UNSPECIFIED.,.F.,.F.,.F.)
B_SPLINE_SURFACE_WITH_KNOTS((4,2,4),(3,3),(-2.81603468776107E-5,0.00119589979970271,
0.00241995509742885),(0.,1.00002816034688),.UNSPECIFIED.)
GEOMETRIC_REPRESENTATION_ITEM()
RATIONAL_B_SPLINE_SURFACE(((1.,0.706267412093565,1.00001654322313),(1.,
0.718312133068377,1.00001586485609),(1.,0.730249727038935,1.00001519252251),
(1.,0.753894775002322,1.00001386081701),(1.,0.765682964669419,1.00001319689799),
(1.,0.776930652130126,1.00001256342043)))
REPRESENTATION_ITEM('')
SURFACE()
);
#2296=(
BOUNDED_SURFACE()
B_SPLINE_SURFACE(3,2,((#147056,#147057,#147058),(#147059,#147060,#147061),
(#147062,#147063,#147064),(#147065,#147066,#147067),(#147068,#147069,#147070),
(#147071,#147072,#147073)),.UNSPECIFIED.,.F.,.F.,.F.)
B_SPLINE_SURFACE_WITH_KNOTS((4,2,4),(3,3),(0.,0.00119596402151854,0.00239192804303707),
(0.,1.),.UNSPECIFIED.)
GEOMETRIC_REPRESENTATION_ITEM()
RATIONAL_B_SPLINE_SURFACE(((1.,0.776159951988518,1.),(1.,0.765146332033717,
1.),(1.,0.753844155392208,1.),(1.,0.730744284614809,1.),(1.,0.718864587348138,
1.),(1.,0.707106781186548,1.)))
REPRESENTATION_ITEM('')
SURFACE()
);
#2297=(
BOUNDED_SURFACE()
B_SPLINE_SURFACE(3,2,((#147080,#147081,#147082),(#147083,#147084,#147085),
(#147086,#147087,#147088),(#147089,#147090,#147091),(#147092,#147093,#147094),
(#147095,#147096,#147097),(#147098,#147099,#147100),(#147101,#147102,#147103)),
 .UNSPECIFIED.,.F.,.F.,.F.)
B_SPLINE_SURFACE_WITH_KNOTS((4,2,2,4),(3,3),(0.0758061741912965,0.0799264930317429,
0.081986652451966,0.0840468118721892),(0.,1.),.UNSPECIFIED.)
GEOMETRIC_REPRESENTATION_ITEM()
RATIONAL_B_SPLINE_SURFACE(((1.,0.961573839605902,1.),(1.,0.963379794804551,
1.),(1.,0.965135301445735,1.),(1.,0.967619049505042,1.),(1.,0.968423938543271,
1.),(1.,0.96994350882013,1.),(1.,0.970660771468208,1.),(1.,0.971327129982678,
1.)))
REPRESENTATION_ITEM('')
SURFACE()
);
#2298=(
BOUNDED_SURFACE()
B_SPLINE_SURFACE(3,2,((#147130,#147131,#147132),(#147133,#147134,#147135),
(#147136,#147137,#147138),(#147139,#147140,#147141),(#147142,#147143,#147144),
(#147145,#147146,#147147)),.UNSPECIFIED.,.F.,.F.,.F.)
B_SPLINE_SURFACE_WITH_KNOTS((4,2,4),(3,3),(-1.38777878078145E-17,0.0189537577590876,
0.0379075155181751),(0.,1.),.UNSPECIFIED.)
GEOMETRIC_REPRESENTATION_ITEM()
RATIONAL_B_SPLINE_SURFACE(((1.,0.620304161933054,1.),(1.,0.616101722702546,
1.),(1.,0.61132314280393,1.),(1.,0.599852065362239,1.),(1.,0.593169697629851,
1.),(1.,0.584878694958868,1.)))
REPRESENTATION_ITEM('')
SURFACE()
);
#2299=(
BOUNDED_SURFACE()
B_SPLINE_SURFACE(3,2,((#147149,#147150,#147151),(#147152,#147153,#147154),
(#147155,#147156,#147157),(#147158,#147159,#147160),(#147161,#147162,#147163),
(#147164,#147165,#147166)),.UNSPECIFIED.,.F.,.F.,.F.)
B_SPLINE_SURFACE_WITH_KNOTS((4,2,4),(3,3),(-1.06251812903579E-17,0.00150294083257491,
0.00300588166514984),(0.,1.),.UNSPECIFIED.)
GEOMETRIC_REPRESENTATION_ITEM()
RATIONAL_B_SPLINE_SURFACE(((1.,0.707106781186548,1.),(1.,0.688447591630839,
1.),(1.,0.669002122235948,1.),(1.,0.628207099426844,1.),(1.,0.606682052630604,
1.),(1.,0.584878694958868,1.)))
REPRESENTATION_ITEM('')
SURFACE()
);
#2300=(
BOUNDED_SURFACE()
B_SPLINE_SURFACE(3,2,((#147172,#147173,#147174),(#147175,#147176,#147177),
(#147178,#147179,#147180),(#147181,#147182,#147183),(#147184,#147185,#147186),
(#147187,#147188,#147189)),.UNSPECIFIED.,.F.,.F.,.F.)
B_SPLINE_SURFACE_WITH_KNOTS((4,2,4),(3,3),(-0.000128927283350436,0.00150339017752321,
0.00313570783234569),(0.,1.00012892747725),.UNSPECIFIED.)
GEOMETRIC_REPRESENTATION_ITEM()
RATIONAL_B_SPLINE_SURFACE(((1.,0.579199953812914,1.00010850537676),(1.,
0.603005180155982,1.0001023670812),(1.,0.625981897604081,1.00009644242077),
(1.,0.670345420760658,1.00008500306653),(1.,0.691877771030212,1.00007945084333),
(1.,0.711824716728862,1.00007430742455)))
REPRESENTATION_ITEM('')
SURFACE()
);
#2301=(
BOUNDED_SURFACE()
B_SPLINE_SURFACE(3,2,((#147220,#147221,#147222),(#147223,#147224,#147225),
(#147226,#147227,#147228),(#147229,#147230,#147231),(#147232,#147233,#147234),
(#147235,#147236,#147237)),.UNSPECIFIED.,.F.,.F.,.F.)
B_SPLINE_SURFACE_WITH_KNOTS((4,2,4),(3,3),(0.,0.0190876722191456,0.0381753444382913),
(0.,1.),.UNSPECIFIED.)
GEOMETRIC_REPRESENTATION_ITEM()
RATIONAL_B_SPLINE_SURFACE(((1.,0.584878694958869,1.),(1.,0.593227971935905,
1.),(1.,0.599946751815832,1.),(1.,0.611471310523657,1.),(1.,0.616266665820404,
1.),(1.,0.620481653466,1.)))
REPRESENTATION_ITEM('')
SURFACE()
);
#2302=(
BOUNDED_SURFACE()
B_SPLINE_SURFACE(3,2,((#147246,#147247,#147248),(#147249,#147250,#147251),
(#147252,#147253,#147254),(#147255,#147256,#147257)),.UNSPECIFIED.,.F.,
 .F.,.F.)
B_SPLINE_SURFACE_WITH_KNOTS((4,4),(3,3),(-6.51391992791641E-5,0.000716531192070805),
(0.,1.00012915786925),.UNSPECIFIED.)
GEOMETRIC_REPRESENTATION_ITEM()
RATIONAL_B_SPLINE_SURFACE(((1.,0.622358323103107,1.00009755078866),(1.,
0.614314362823104,1.0000996286702),(1.,0.610346508423654,1.00010065362944),
(1.,0.611117930705946,1.00010045435892)))
REPRESENTATION_ITEM('')
SURFACE()
);
#2303=(
BOUNDED_SURFACE()
B_SPLINE_SURFACE(3,2,((#147285,#147286,#147287),(#147288,#147289,#147290),
(#147291,#147292,#147293),(#147294,#147295,#147296),(#147297,#147298,#147299),
(#147300,#147301,#147302)),.UNSPECIFIED.,.F.,.F.,.F.)
B_SPLINE_SURFACE_WITH_KNOTS((4,2,4),(3,3),(0.,0.0178083890192188,0.0356167780384377),
(0.,1.),.UNSPECIFIED.)
GEOMETRIC_REPRESENTATION_ITEM()
RATIONAL_B_SPLINE_SURFACE(((1.,0.824689321081978,1.),(1.,0.818552442915159,
1.),(1.,0.813336414682689,1.),(1.,0.80412734431217,1.),(1.,0.800137214821899,
1.),(1.,0.796559406694623,1.)))
REPRESENTATION_ITEM('')
SURFACE()
);
#2304=(
BOUNDED_SURFACE()
B_SPLINE_SURFACE(3,2,((#147355,#147356,#147357),(#147358,#147359,#147360),
(#147361,#147362,#147363),(#147364,#147365,#147366)),.UNSPECIFIED.,.F.,
 .F.,.F.)
B_SPLINE_SURFACE_WITH_KNOTS((4,4),(3,3),(-6.5186839171593E-5,0.000717055230887516),
(0.,1.00014173624585),.UNSPECIFIED.)
GEOMETRIC_REPRESENTATION_ITEM()
RATIONAL_B_SPLINE_SURFACE(((1.,0.804734778555417,1.00005535231887),(1.,
0.805403669437747,1.0000551627067),(1.,0.802005595787365,1.00005612596711),
(1.,0.794601667527971,1.0000582247771)))
REPRESENTATION_ITEM('')
SURFACE()
);
#2305=(
BOUNDED_SURFACE()
B_SPLINE_SURFACE(3,2,((#147370,#147371,#147372),(#147373,#147374,#147375),
(#147376,#147377,#147378),(#147379,#147380,#147381),(#147382,#147383,#147384),
(#147385,#147386,#147387)),.UNSPECIFIED.,.F.,.F.,.F.)
B_SPLINE_SURFACE_WITH_KNOTS((4,2,4),(3,3),(0.,0.0179426259581151,0.0358852519162302),
(0.,1.),.UNSPECIFIED.)
GEOMETRIC_REPRESENTATION_ITEM()
RATIONAL_B_SPLINE_SURFACE(((1.,0.796398016704685,1.),(1.,0.799989941027341,
1.),(1.,0.80399801610487,1.),(1.,0.81325769888663,1.),(1.,0.81850629826423,
1.),(1.,0.824689321081979,1.)))
REPRESENTATION_ITEM('')
SURFACE()
);
#2306=(
BOUNDED_SURFACE()
B_SPLINE_SURFACE(3,2,((#147396,#147397,#147398),(#147399,#147400,#147401),
(#147402,#147403,#147404),(#147405,#147406,#147407),(#147408,#147409,#147410),
(#147411,#147412,#147413)),.UNSPECIFIED.,.F.,.F.,.F.)
B_SPLINE_SURFACE_WITH_KNOTS((4,2,4),(3,3),(-9.67458881849461E-5,0.0016638050806964,
0.00342426416910809),(0.,1.00009674588818),.UNSPECIFIED.)
GEOMETRIC_REPRESENTATION_ITEM()
RATIONAL_B_SPLINE_SURFACE(((1.,0.703317663028854,1.0000574055924),(1.,0.726192599003532,
1.0000529794804),(1.,0.747928069556768,1.00004877384559),(1.,0.789487375132482,
1.00004073246173),(1.,0.809468493425914,1.00003686627966),(1.,0.827689223724241,
1.00003334071819)))
REPRESENTATION_ITEM('')
SURFACE()
);
#2307=(
BOUNDED_SURFACE()
B_SPLINE_SURFACE(3,2,((#147448,#147449,#147450),(#147451,#147452,#147453),
(#147454,#147455,#147456),(#147457,#147458,#147459),(#147460,#147461,#147462),
(#147463,#147464,#147465)),.UNSPECIFIED.,.F.,.F.,.F.)
B_SPLINE_SURFACE_WITH_KNOTS((4,2,4),(3,3),(0.,0.00166463949867057,0.00332927899734113),
(0.,1.),.UNSPECIFIED.)
GEOMETRIC_REPRESENTATION_ITEM()
RATIONAL_B_SPLINE_SURFACE(((1.,0.824689321081979,1.),(1.,0.807273117786527,
1.),(1.,0.78876985537206,1.),(1.,0.749461319834452,1.),(1.,0.728524445804063,
1.),(1.,0.707106781186548,1.)))
REPRESENTATION_ITEM('')
SURFACE()
);
#2308=(
BOUNDED_SURFACE()
B_SPLINE_SURFACE(3,2,((#147473,#147474,#147475),(#147476,#147477,#147478),
(#147479,#147480,#147481),(#147482,#147483,#147484),(#147485,#147486,#147487),
(#147488,#147489,#147490)),.UNSPECIFIED.,.F.,.F.,.F.)
B_SPLINE_SURFACE_WITH_KNOTS((4,2,4),(3,3),(0.312244141975826,0.317485429411984,
0.322726716848141),(0.,1.),.UNSPECIFIED.)
GEOMETRIC_REPRESENTATION_ITEM()
RATIONAL_B_SPLINE_SURFACE(((1.,0.945205509755643,1.),(1.,0.94765942841632,
1.),(1.,0.950143082313928,1.),(1.,0.955101624050304,1.),(1.,0.957550590969702,
1.),(1.,0.959916006973269,1.)))
REPRESENTATION_ITEM('')
SURFACE()
);
#2309=(
BOUNDED_SURFACE()
B_SPLINE_SURFACE(3,2,((#147517,#147518,#147519),(#147520,#147521,#147522),
(#147523,#147524,#147525),(#147526,#147527,#147528),(#147529,#147530,#147531),
(#147532,#147533,#147534)),.UNSPECIFIED.,.F.,.F.,.F.)
B_SPLINE_SURFACE_WITH_KNOTS((4,2,4),(3,3),(0.,0.0147014688781887,0.0294029377563774),
(0.,1.),.UNSPECIFIED.)
GEOMETRIC_REPRESENTATION_ITEM()
RATIONAL_B_SPLINE_SURFACE(((1.,0.567371969128416,1.),(1.,0.561922702387361,
1.),(1.,0.555858739311734,1.),(1.,0.541909480588213,1.),(1.,0.534028604774054,
1.),(1.,0.524787419125872,1.)))
REPRESENTATION_ITEM('')
SURFACE()
);
#2310=(
BOUNDED_SURFACE()
B_SPLINE_SURFACE(3,2,((#147536,#147537,#147538),(#147539,#147540,#147541),
(#147542,#147543,#147544),(#147545,#147546,#147547)),.UNSPECIFIED.,.F.,
 .F.,.F.)
B_SPLINE_SURFACE_WITH_KNOTS((4,4),(3,3),(-3.67928601655754E-5,0.000690322634236133),
(0.,1.00003679286017),.UNSPECIFIED.)
GEOMETRIC_REPRESENTATION_ITEM()
RATIONAL_B_SPLINE_SURFACE(((1.,0.569438382608578,1.00003168318676),(1.,
0.557411392496524,1.00003256820149),(1.,0.550996682930264,1.00003304023252),
(1.,0.551710399363625,1.00003298771318)))
REPRESENTATION_ITEM('')
SURFACE()
);
#2311=(
BOUNDED_SURFACE()
B_SPLINE_SURFACE(3,2,((#147575,#147576,#147577),(#147578,#147579,#147580),
(#147581,#147582,#147583),(#147584,#147585,#147586),(#147587,#147588,#147589),
(#147590,#147591,#147592)),.UNSPECIFIED.,.F.,.F.,.F.)
B_SPLINE_SURFACE_WITH_KNOTS((4,2,4),(3,3),(0.,0.002055311285568,0.00411062257113599),
(0.,1.),.UNSPECIFIED.)
GEOMETRIC_REPRESENTATION_ITEM()
RATIONAL_B_SPLINE_SURFACE(((1.,0.707106781186549,1.),(1.,0.67983601545864,
1.),(1.,0.651283059470391,1.),(1.,0.590515772030266,1.),(1.,0.55801180255865,
1.),(1.,0.524787419125864,1.)))
REPRESENTATION_ITEM('')
SURFACE()
);
#2312=(
BOUNDED_SURFACE()
B_SPLINE_SURFACE(3,2,((#147598,#147599,#147600),(#147601,#147602,#147603),
(#147604,#147605,#147606),(#147607,#147608,#147609),(#147610,#147611,#147612),
(#147613,#147614,#147615)),.UNSPECIFIED.,.F.,.F.,.F.)
B_SPLINE_SURFACE_WITH_KNOTS((4,2,4),(3,3),(-0.000411246537817809,0.00205623335330194,
0.00452371337726426),(0.,1.00055466892243),.UNSPECIFIED.)
GEOMETRIC_REPRESENTATION_ITEM()
RATIONAL_B_SPLINE_SURFACE(((1.,0.50433079517456,1.00054986460745),(1.,0.545103499610019,
1.00050463390338),(1.,0.583527669535412,1.00046200851752),(1.,0.656716898757763,
1.00038081693571),(1.,0.691464019865608,1.00034227063927),(1.,0.722954371107003,
1.00030733720088)))
REPRESENTATION_ITEM('')
SURFACE()
);
#2313=(
BOUNDED_SURFACE()
B_SPLINE_SURFACE(3,2,((#147649,#147650,#147651),(#147652,#147653,#147654),
(#147655,#147656,#147657),(#147658,#147659,#147660),(#147661,#147662,#147663),
(#147664,#147665,#147666)),.UNSPECIFIED.,.F.,.F.,.F.)
B_SPLINE_SURFACE_WITH_KNOTS((4,2,4),(3,3),(-6.93889390390723E-18,0.0148367096635454,
0.0296734193270908),(0.,1.),.UNSPECIFIED.)
GEOMETRIC_REPRESENTATION_ITEM()
RATIONAL_B_SPLINE_SURFACE(((1.,0.524787419125867,1.),(1.,0.534113414550019,
1.),(1.,0.542054608658765,1.),(1.,0.556098130983184,1.),(1.,0.562195863398439,
1.),(1.,0.56767185832395,1.)))
REPRESENTATION_ITEM('')
SURFACE()
);
#2314=(
BOUNDED_SURFACE()
B_SPLINE_SURFACE(3,2,((#147673,#147674,#147675),(#147676,#147677,#147678),
(#147679,#147680,#147681),(#147682,#147683,#147684)),.UNSPECIFIED.,.F.,
 .F.,.F.)
B_SPLINE_SURFACE_WITH_KNOTS((4,4),(3,3),(0.,0.000433489251034108),(0.,1.),
 .UNSPECIFIED.)
GEOMETRIC_REPRESENTATION_ITEM()
RATIONAL_B_SPLINE_SURFACE(((1.,0.843391445812886,1.),(1.,0.83955525384858,
1.),(1.,0.835558949072738,1.),(1.,0.831408647420015,1.)))
REPRESENTATION_ITEM('')
SURFACE()
);
#2315=(
BOUNDED_SURFACE()
B_SPLINE_SURFACE(3,2,((#147715,#147716,#147717),(#147718,#147719,#147720),
(#147721,#147722,#147723),(#147724,#147725,#147726),(#147727,#147728,#147729),
(#147730,#147731,#147732),(#147733,#147734,#147735),(#147736,#147737,#147738),
(#147739,#147740,#147741),(#147742,#147743,#147744)),.UNSPECIFIED.,.F.,
 .F.,.F.)
B_SPLINE_SURFACE_WITH_KNOTS((4,2,2,2,4),(3,3),(1.5707963267949,1.96349540849362,
2.35619449019234,2.74889357189107,3.1415926535898),(0.,1.),
 .UNSPECIFIED.)
GEOMETRIC_REPRESENTATION_ITEM()
RATIONAL_B_SPLINE_SURFACE(((1.,0.707106781186548,1.),(1.,0.700666378834291,
1.),(1.,0.694134907060803,1.),(1.,0.681903435451243,1.),(1.,0.676209154064001,
1.),(1.,0.666616044204474,1.),(1.,0.662724068472647,1.),(1.,0.657443209221265,
1.),(1.,0.656051196071914,1.),(1.,0.656059028990508,1.)))
REPRESENTATION_ITEM('')
SURFACE()
);
#2316=(
BOUNDED_SURFACE()
B_SPLINE_SURFACE(3,2,((#147783,#147784,#147785),(#147786,#147787,#147788),
(#147789,#147790,#147791),(#147792,#147793,#147794),(#147795,#147796,#147797),
(#147798,#147799,#147800),(#147801,#147802,#147803),(#147804,#147805,#147806),
(#147807,#147808,#147809),(#147810,#147811,#147812)),.UNSPECIFIED.,.F.,
 .F.,.F.)
B_SPLINE_SURFACE_WITH_KNOTS((4,2,2,2,4),(3,3),(0.,0.000174105410412539,
0.000348210820825077,0.000522316231237617,0.000696421641650155),(0.,1.),
 .UNSPECIFIED.)
GEOMETRIC_REPRESENTATION_ITEM()
RATIONAL_B_SPLINE_SURFACE(((1.,0.4747595709467,1.),(1.,0.487194273605061,
1.),(1.,0.503322485825965,1.),(1.,0.54047069549172,1.),(1.,0.560568699342516,
1.),(1.,0.602438533850501,1.),(1.,0.623450047599376,1.),(1.,0.665484286819028,
1.),(1.,0.686628698725959,1.),(1.,0.707106781186548,1.)))
REPRESENTATION_ITEM('')
SURFACE()
);
#2317=(
BOUNDED_SURFACE()
B_SPLINE_SURFACE(3,2,((#147814,#147815,#147816),(#147817,#147818,#147819),
(#147820,#147821,#147822),(#147823,#147824,#147825),(#147826,#147827,#147828),
(#147829,#147830,#147831),(#147832,#147833,#147834),(#147835,#147836,#147837)),
 .UNSPECIFIED.,.F.,.F.,.F.)
B_SPLINE_SURFACE_WITH_KNOTS((4,2,2,4),(3,3),(0.,0.00267885639561352,0.00401828459342028,
0.00535771279122705),(0.,1.),.UNSPECIFIED.)
GEOMETRIC_REPRESENTATION_ITEM()
RATIONAL_B_SPLINE_SURFACE(((1.,0.707106781186871,1.),(1.,0.673473842386368,
1.),(1.,0.638019211186003,1.),(1.,0.580269195298477,1.),(1.,0.560144321783745,
1.),(1.,0.518526712842715,1.),(1.,0.497044145980004,1.),(1.,0.474759570947005,
1.)))
REPRESENTATION_ITEM('')
SURFACE()
);
#2318=(
BOUNDED_SURFACE()
B_SPLINE_SURFACE(3,2,((#147854,#147855,#147856),(#147857,#147858,#147859),
(#147860,#147861,#147862),(#147863,#147864,#147865),(#147866,#147867,#147868),
(#147869,#147870,#147871),(#147872,#147873,#147874),(#147875,#147876,#147877),
(#147878,#147879,#147880),(#147881,#147882,#147883)),.UNSPECIFIED.,.F.,
 .F.,.F.)
B_SPLINE_SURFACE_WITH_KNOTS((4,2,2,2,4),(3,3),(-0.000563963881013773,0.00140990970253443,
0.00281981940506887,0.0042297291076033,0.0062036026911515),(0.,1.00067621131492),
 .UNSPECIFIED.)
GEOMETRIC_REPRESENTATION_ITEM()
RATIONAL_B_SPLINE_SURFACE(((1.,0.431302648803683,1.00076911916729),(1.,
0.465713233921,1.00072258151327),(1.,0.498089262024449,1.0006787954402),
(1.,0.550868342653017,1.00060741581717),(1.,0.572053437981938,1.00057876461484),
(1.,0.613155696744348,1.00052317698995),(1.,0.632943112728916,1.00049641604078),
(1.,0.678527474844668,1.00043476671789),(1.,0.703702763966988,1.00040071908717),
(1.,0.727897090333189,1.00036799813268)))
REPRESENTATION_ITEM('')
SURFACE()
);
#2319=(
BOUNDED_SURFACE()
B_SPLINE_SURFACE(3,2,((#147929,#147930,#147931),(#147932,#147933,#147934),
(#147935,#147936,#147937),(#147938,#147939,#147940),(#147941,#147942,#147943),
(#147944,#147945,#147946)),.UNSPECIFIED.,.F.,.F.,.F.)
B_SPLINE_SURFACE_WITH_KNOTS((4,2,4),(3,3),(0.00191966951912585,0.00217079434687949,
0.00242191917463315),(0.,1.),.UNSPECIFIED.)
GEOMETRIC_REPRESENTATION_ITEM()
RATIONAL_B_SPLINE_SURFACE(((1.,0.460674285272032,1.),(1.,0.480581991146479,
1.),(1.,0.508992468088204,1.),(1.,0.568988175192947,1.),(1.,0.601196374063936,
1.),(1.,0.631879234223659,1.)))
REPRESENTATION_ITEM('')
SURFACE()
);
#2320=(
BOUNDED_SURFACE()
B_SPLINE_SURFACE(3,2,((#147955,#147956,#147957),(#147958,#147959,#147960),
(#147961,#147962,#147963),(#147964,#147965,#147966)),.UNSPECIFIED.,.F.,
 .F.,.F.)
B_SPLINE_SURFACE_WITH_KNOTS((4,4),(3,3),(-6.9931040125315E-18,0.000203650363220118),
(0.,1.),.UNSPECIFIED.)
GEOMETRIC_REPRESENTATION_ITEM()
RATIONAL_B_SPLINE_SURFACE(((1.,0.707106781186548,1.),(1.,0.683088481213104,
1.),(1.,0.658130799535722,1.),(1.,0.631879234223615,1.)))
REPRESENTATION_ITEM('')
SURFACE()
);
#2321=(
BOUNDED_SURFACE()
B_SPLINE_SURFACE(3,2,((#147988,#147989,#147990),(#147991,#147992,#147993),
(#147994,#147995,#147996),(#147997,#147998,#147999),(#148000,#148001,#148002),
(#148003,#148004,#148005),(#148006,#148007,#148008),(#148009,#148010,#148011),
(#148012,#148013,#148014),(#148015,#148016,#148017)),.UNSPECIFIED.,.F.,
 .F.,.F.)
B_SPLINE_SURFACE_WITH_KNOTS((4,2,2,2,4),(3,3),(0.00116892975483546,0.00173273620432841,
0.00229654265382136,0.0028603491033143,0.00342415555280725),(0.,1.00008736726511),
 .UNSPECIFIED.)
GEOMETRIC_REPRESENTATION_ITEM()
RATIONAL_B_SPLINE_SURFACE(((1.,0.707081191907056,1.00005118303032),(1.,
0.756727911750155,1.00004250803406),(1.,0.795323614743188,1.00003576403202),
(1.,0.847730260009882,1.00002660678148),(1.,0.86137618483429,1.00002422236722),
(1.,0.861443104051581,1.00002421067412),(1.,0.847851660205464,1.00002658556868),
(1.,0.795420207077645,1.00003574715401),(1.,0.756766547571617,1.00004250128304),
(1.,0.707081191907056,1.00005118303032)))
REPRESENTATION_ITEM('')
SURFACE()
);
#2322=(
BOUNDED_SURFACE()
B_SPLINE_SURFACE(3,2,((#148038,#148039,#148040),(#148041,#148042,#148043),
(#148044,#148045,#148046),(#148047,#148048,#148049),(#148050,#148051,#148052),
(#148053,#148054,#148055),(#148056,#148057,#148058),(#148059,#148060,#148061),
(#148062,#148063,#148064),(#148065,#148066,#148067)),.UNSPECIFIED.,.F.,
 .F.,.F.)
B_SPLINE_SURFACE_WITH_KNOTS((4,2,2,2,4),(3,3),(3.1415926535898,3.53429173528852,
3.92699081698724,4.31968989868597,4.71238898038469),(0.,1.),
 .UNSPECIFIED.)
GEOMETRIC_REPRESENTATION_ITEM()
RATIONAL_B_SPLINE_SURFACE(((1.,0.754709580222767,1.),(1.,0.754714219730801,
1.),(1.,0.753512297096199,1.),(1.,0.748871927696587,1.),(1.,0.745429366938708,
1.),(1.,0.736738129296182,1.),(1.,0.731490756397336,1.),(1.,0.719894264862173,
1.),(1.,0.71355026185156,1.),(1.,0.707106781186543,1.)))
REPRESENTATION_ITEM('')
SURFACE()
);
#2323=(
BOUNDED_SURFACE()
B_SPLINE_SURFACE(3,2,((#148080,#148081,#148082),(#148083,#148084,#148085),
(#148086,#148087,#148088),(#148089,#148090,#148091)),.UNSPECIFIED.,.F.,
 .F.,.F.)
B_SPLINE_SURFACE_WITH_KNOTS((4,4),(3,3),(-2.71050543121376E-20,0.00022779825406313),
(0.,1.),.UNSPECIFIED.)
GEOMETRIC_REPRESENTATION_ITEM()
RATIONAL_B_SPLINE_SURFACE(((1.,0.800108937437274,1.),(1.,0.815261773270244,
1.),(1.,0.827452668690902,1.),(1.,0.835963592436001,1.)))
REPRESENTATION_ITEM('')
SURFACE()
);
#2324=(
BOUNDED_SURFACE()
B_SPLINE_SURFACE(3,2,((#148093,#148094,#148095),(#148096,#148097,#148098),
(#148099,#148100,#148101),(#148102,#148103,#148104),(#148105,#148106,#148107),
(#148108,#148109,#148110)),.UNSPECIFIED.,.F.,.F.,.F.)
B_SPLINE_SURFACE_WITH_KNOTS((4,2,4),(3,3),(0.,0.000488238270881924,0.000976476541763847),
(0.,1.),.UNSPECIFIED.)
GEOMETRIC_REPRESENTATION_ITEM()
RATIONAL_B_SPLINE_SURFACE(((1.,0.807089511457258,1.),(1.,0.816558112905035,
1.),(1.,0.821286794224823,1.),(1.,0.825205555407875,1.),(1.,0.824318362071196,
1.),(1.,0.822092089912778,1.)))
REPRESENTATION_ITEM('')
SURFACE()
);
#2325=(
BOUNDED_SURFACE()
B_SPLINE_SURFACE(3,2,((#148112,#148113,#148114),(#148115,#148116,#148117),
(#148118,#148119,#148120),(#148121,#148122,#148123)),.UNSPECIFIED.,.F.,
 .F.,.F.)
B_SPLINE_SURFACE_WITH_KNOTS((4,4),(3,3),(0.,0.000103369667661675),(0.,1.),
 .UNSPECIFIED.)
GEOMETRIC_REPRESENTATION_ITEM()
RATIONAL_B_SPLINE_SURFACE(((1.,0.835735574810027,1.),(1.,0.831946521393585,
1.),(1.,0.827395718030991,1.),(1.,0.822092089912784,1.)))
REPRESENTATION_ITEM('')
SURFACE()
);
#2326=(
BOUNDED_SURFACE()
B_SPLINE_SURFACE(3,2,((#148127,#148128,#148129),(#148130,#148131,#148132),
(#148133,#148134,#148135),(#148136,#148137,#148138)),.UNSPECIFIED.,.F.,
 .F.,.F.)
B_SPLINE_SURFACE_WITH_KNOTS((4,4),(3,3),(0.,0.0206148669995797),(0.,1.),
 .UNSPECIFIED.)
GEOMETRIC_REPRESENTATION_ITEM()
RATIONAL_B_SPLINE_SURFACE(((1.,0.835735574810025,1.),(1.,0.841493793210698,
1.),(1.,0.847990686938055,1.),(1.,0.855596390789697,1.)))
REPRESENTATION_ITEM('')
SURFACE()
);
#2327=(
BOUNDED_SURFACE()
B_SPLINE_SURFACE(3,2,((#148145,#148146,#148147),(#148148,#148149,#148150),
(#148151,#148152,#148153),(#148154,#148155,#148156),(#148157,#148158,#148159),
(#148160,#148161,#148162)),.UNSPECIFIED.,.F.,.F.,.F.)
B_SPLINE_SURFACE_WITH_KNOTS((4,2,4),(3,3),(-0.000138519827310576,0.00213206083322637,
0.00440235036966729),(0.,1.00013851982731),.UNSPECIFIED.)
GEOMETRIC_REPRESENTATION_ITEM()
RATIONAL_B_SPLINE_SURFACE(((1.,0.701536032441349,1.00008268635449),(1.,
0.731888497336716,1.0000742775181),(1.,0.759999697565549,1.0000664896009),
(1.,0.812818114669199,1.00005185680486),(1.,0.837690840276735,1.00004496607355),
(1.,0.859613164458893,1.00003889272043)))
REPRESENTATION_ITEM('')
SURFACE()
);
#2328=(
BOUNDED_SURFACE()
B_SPLINE_SURFACE(3,2,((#148200,#148201,#148202),(#148203,#148204,#148205),
(#148206,#148207,#148208),(#148209,#148210,#148211),(#148212,#148213,#148214),
(#148215,#148216,#148217),(#148218,#148219,#148220),(#148221,#148222,#148223)),
 .UNSPECIFIED.,.F.,.F.,.F.)
B_SPLINE_SURFACE_WITH_KNOTS((4,2,2,4),(3,3),(0.,0.00213290337237644,0.00319935505856466,
0.00426580674475288),(0.,1.),.UNSPECIFIED.)
GEOMETRIC_REPRESENTATION_ITEM()
RATIONAL_B_SPLINE_SURFACE(((1.,0.855596390789701,1.),(1.,0.834565892891844,
1.),(1.,0.811730594666637,1.),(1.,0.77446817058652,1.),(1.,0.761499431653623,
1.),(1.,0.734903385695778,1.),(1.,0.721225679237929,1.),(1.,0.707106781186545,
1.)))
REPRESENTATION_ITEM('')
SURFACE()
);
#2329=(
BOUNDED_SURFACE()
B_SPLINE_SURFACE(3,2,((#148234,#148235,#148236),(#148237,#148238,#148239),
(#148240,#148241,#148242),(#148243,#148244,#148245)),.UNSPECIFIED.,.F.,
 .F.,.F.)
B_SPLINE_SURFACE_WITH_KNOTS((4,4),(3,3),(-2.08166817117217E-17,0.0203430832871546),
(0.,1.),.UNSPECIFIED.)
GEOMETRIC_REPRESENTATION_ITEM()
RATIONAL_B_SPLINE_SURFACE(((1.,0.855596390789699,1.),(1.,0.848090845809161,
1.),(1.,0.841665513049531,1.),(1.,0.835963592435998,1.)))
REPRESENTATION_ITEM('')
SURFACE()
);
#2330=(
BOUNDED_SURFACE()
B_SPLINE_SURFACE(3,2,((#148266,#148267,#148268),(#148269,#148270,#148271),
(#148272,#148273,#148274),(#148275,#148276,#148277),(#148278,#148279,#148280),
(#148281,#148282,#148283),(#148284,#148285,#148286),(#148287,#148288,#148289)),
 .UNSPECIFIED.,.F.,.F.,.F.)
B_SPLINE_SURFACE_WITH_KNOTS((4,2,2,4),(3,3),(-1.5368565794982E-17,0.000158339556725866,
0.000316679113451747,0.000633358226903509),(0.,1.),.UNSPECIFIED.)
GEOMETRIC_REPRESENTATION_ITEM()
RATIONAL_B_SPLINE_SURFACE(((1.,0.507397370006824,1.),(1.,0.519070630879541,
1.),(1.,0.533426892711081,1.),(1.,0.565658432465259,1.),(1.,0.583100719918817,
1.),(1.,0.636529920575075,1.),(1.,0.673198940992506,1.),(1.,0.707106781186548,
1.)))
REPRESENTATION_ITEM('')
SURFACE()
);
#2331=(
BOUNDED_SURFACE()
B_SPLINE_SURFACE(3,2,((#148293,#148294,#148295),(#148296,#148297,#148298),
(#148299,#148300,#148301),(#148302,#148303,#148304)),.UNSPECIFIED.,.F.,
 .F.,.F.)
B_SPLINE_SURFACE_WITH_KNOTS((4,4),(3,3),(0.,0.0125680158145827),(0.,1.),
 .UNSPECIFIED.)
GEOMETRIC_REPRESENTATION_ITEM()
RATIONAL_B_SPLINE_SURFACE(((1.,0.507397370006812,1.),(1.,0.500416139715127,
1.),(1.,0.49272006913241,1.),(1.,0.484030052331115,1.)))
REPRESENTATION_ITEM('')
SURFACE()
);
#2332=(
BOUNDED_SURFACE()
B_SPLINE_SURFACE(3,2,((#148306,#148307,#148308),(#148309,#148310,#148311),
(#148312,#148313,#148314),(#148315,#148316,#148317),(#148318,#148319,#148320),
(#148321,#148322,#148323),(#148324,#148325,#148326),(#148327,#148328,#148329)),
 .UNSPECIFIED.,.F.,.F.,.F.)
B_SPLINE_SURFACE_WITH_KNOTS((4,2,2,4),(3,3),(-5.42101086242752E-20,0.00250485829616721,
0.00375728744425081,0.00500971659233441),(0.,1.),.UNSPECIFIED.)
GEOMETRIC_REPRESENTATION_ITEM()
RATIONAL_B_SPLINE_SURFACE(((1.,0.70710678118722,1.),(1.,0.674452105060394,
1.),(1.,0.640073400404409,1.),(1.,0.584341050151977,1.),(1.,0.564951135845581,
1.),(1.,0.525261922605914,1.),(1.,0.504912110655119,1.),(1.,0.484030052331115,
1.)))
REPRESENTATION_ITEM('')
SURFACE()
);
#2333=(
BOUNDED_SURFACE()
B_SPLINE_SURFACE(3,2,((#148346,#148347,#148348),(#148349,#148350,#148351),
(#148352,#148353,#148354),(#148355,#148356,#148357),(#148358,#148359,#148360),
(#148361,#148362,#148363),(#148364,#148365,#148366),(#148367,#148368,#148369),
(#148370,#148371,#148372),(#148373,#148374,#148375)),.UNSPECIFIED.,.F.,
 .F.,.F.)
B_SPLINE_SURFACE_WITH_KNOTS((4,2,2,2,4),(3,3),(-0.000453575048684217,0.00125260629929845,
0.00250521259859689,0.00375781889789535,0.00546400047376828),(0.,1.00045357527164),
 .UNSPECIFIED.)
GEOMETRIC_REPRESENTATION_ITEM()
RATIONAL_B_SPLINE_SURFACE(((1.,0.460833248862991,1.00048910541122),(1.,
0.4899429330804,1.00046269854536),(1.,0.517846279275575,1.0004373860097),
(1.,0.564400235579759,1.00039515456295),(1.,0.583541342515348,1.00037779069739),
(1.,0.620882778440762,1.00034391639351),(1.,0.63899642320703,1.00032748459082),
(1.,0.680146964965137,1.0002901548545),(1.,0.702746029066762,1.00026965410123),
(1.,0.724519821938228,1.00024990199319)))
REPRESENTATION_ITEM('')
SURFACE()
);
#2334=(
BOUNDED_SURFACE()
B_SPLINE_SURFACE(3,2,((#148418,#148419,#148420),(#148421,#148422,#148423),
(#148424,#148425,#148426),(#148427,#148428,#148429)),.UNSPECIFIED.,.F.,
 .F.,.F.)
B_SPLINE_SURFACE_WITH_KNOTS((4,4),(3,3),(0.,0.01284355850178),(0.,1.),
 .UNSPECIFIED.)
GEOMETRIC_REPRESENTATION_ITEM()
RATIONAL_B_SPLINE_SURFACE(((1.,0.484030052331127,1.),(1.,0.492910462848522,
1.),(1.,0.500753390328389,1.),(1.,0.507855360856573,1.)))
REPRESENTATION_ITEM('')
SURFACE()
);
#2335=(
BOUNDED_SURFACE()
B_SPLINE_SURFACE(3,2,((#148436,#148437,#148438),(#148439,#148440,#148441),
(#148442,#148443,#148444),(#148445,#148446,#148447),(#148448,#148449,#148450),
(#148451,#148452,#148453),(#148454,#148455,#148456),(#148457,#148458,#148459),
(#148460,#148461,#148462),(#148463,#148464,#148465)),.UNSPECIFIED.,.F.,
 .F.,.F.)
B_SPLINE_SURFACE_WITH_KNOTS((4,2,2,2,4),(3,3),(0.,0.000158019212117338,
0.000316038424234677,0.000474057636352015,0.000632076848469353),(0.,1.),
 .UNSPECIFIED.)
GEOMETRIC_REPRESENTATION_ITEM()
RATIONAL_B_SPLINE_SURFACE(((1.,0.707106781186548,1.),(1.,0.690072170678528,
1.),(1.,0.67275310971826,1.),(1.,0.637401910188738,1.),(1.,0.619074074320766,
1.),(1.,0.5836606862513,1.),(1.,0.566468213012793,1.),(1.,0.53406367243224,
1.),(1.,0.519473083497879,1.),(1.,0.507855360856575,1.)))
REPRESENTATION_ITEM('')
SURFACE()
);
#2336=(
BOUNDED_SURFACE()
B_SPLINE_SURFACE(3,2,((#148482,#148483,#148484),(#148485,#148486,#148487),
(#148488,#148489,#148490),(#148491,#148492,#148493),(#148494,#148495,#148496),
(#148497,#148498,#148499),(#148500,#148501,#148502),(#148503,#148504,#148505),
(#148506,#148507,#148508),(#148509,#148510,#148511)),.UNSPECIFIED.,.F.,
 .F.,.F.)
B_SPLINE_SURFACE_WITH_KNOTS((4,2,2,2,4),(3,3),(1.5707963267949,1.96349540849362,
2.35619449019234,2.74889357189107,3.1415926535898),(0.,1.),
 .UNSPECIFIED.)
GEOMETRIC_REPRESENTATION_ITEM()
RATIONAL_B_SPLINE_SURFACE(((1.,0.707106781186548,1.),(1.,0.700666378834307,
1.),(1.,0.694134907060781,1.),(1.,0.681903435451265,1.),(1.,0.676209154064001,
1.),(1.,0.666616044204474,1.),(1.,0.662724068472647,1.),(1.,0.657443209221265,
1.),(1.,0.656051196071904,1.),(1.,0.656059028990508,1.)))
REPRESENTATION_ITEM('')
SURFACE()
);
#2337=(
BOUNDED_SURFACE()
B_SPLINE_SURFACE(3,2,((#148566,#148567,#148568),(#148569,#148570,#148571),
(#148572,#148573,#148574),(#148575,#148576,#148577),(#148578,#148579,#148580),
(#148581,#148582,#148583),(#148584,#148585,#148586),(#148587,#148588,#148589),
(#148590,#148591,#148592),(#148593,#148594,#148595)),.UNSPECIFIED.,.F.,
 .F.,.F.)
B_SPLINE_SURFACE_WITH_KNOTS((4,2,2,2,4),(3,3),(3.1415926535898,3.53429173528852,
3.92699081698724,4.31968989868597,4.71238898038469),(0.,1.),
 .UNSPECIFIED.)
GEOMETRIC_REPRESENTATION_ITEM()
RATIONAL_B_SPLINE_SURFACE(((1.,0.754709580222772,1.),(1.,0.754714219730806,
1.),(1.,0.753512297096203,1.),(1.,0.748871927696591,1.),(1.,0.745429366938691,
1.),(1.,0.736738129296209,1.),(1.,0.73149075639733,1.),(1.,0.719894264862189,
1.),(1.,0.713550261851557,1.),(1.,0.707106781186548,1.)))
REPRESENTATION_ITEM('')
SURFACE()
);
#2338=(
BOUNDED_SURFACE()
B_SPLINE_SURFACE(3,2,((#148612,#148613,#148614),(#148615,#148616,#148617),
(#148618,#148619,#148620),(#148621,#148622,#148623),(#148624,#148625,#148626),
(#148627,#148628,#148629)),.UNSPECIFIED.,.F.,.F.,.F.)
B_SPLINE_SURFACE_WITH_KNOTS((4,2,4),(3,3),(-3.07642366442762E-17,0.000324428028333684,
0.000648856056667399),(0.,1.),.UNSPECIFIED.)
GEOMETRIC_REPRESENTATION_ITEM()
RATIONAL_B_SPLINE_SURFACE(((1.,0.872575378690131,1.),(1.,0.857798601408145,
1.),(1.,0.834121076196936,1.),(1.,0.776835192876573,1.),(1.,0.743446077163894,
1.),(1.,0.707106781186548,1.)))
REPRESENTATION_ITEM('')
SURFACE()
);
#2339=(
BOUNDED_SURFACE()
B_SPLINE_SURFACE(3,2,((#148638,#148639,#148640),(#148641,#148642,#148643),
(#148644,#148645,#148646),(#148647,#148648,#148649)),.UNSPECIFIED.,.F.,
 .F.,.F.)
B_SPLINE_SURFACE_WITH_KNOTS((4,4),(3,3),(-3.46944695195361E-18,0.00904291806877092),
(0.,1.),.UNSPECIFIED.)
GEOMETRIC_REPRESENTATION_ITEM()
RATIONAL_B_SPLINE_SURFACE(((1.,0.872575378690133,1.),(1.,0.875691129720726,
1.),(1.,0.878972255663315,1.),(1.,0.882443751548002,1.)))
REPRESENTATION_ITEM('')
SURFACE()
);
#2340=(
BOUNDED_SURFACE()
B_SPLINE_SURFACE(3,2,((#148656,#148657,#148658),(#148659,#148660,#148661),
(#148662,#148663,#148664),(#148665,#148666,#148667),(#148668,#148669,#148670),
(#148671,#148672,#148673),(#148674,#148675,#148676),(#148677,#148678,#148679)),
 .UNSPECIFIED.,.F.,.F.,.F.)
B_SPLINE_SURFACE_WITH_KNOTS((4,2,2,4),(3,3),(-0.000144062567305207,0.0026640399986995,
0.00399605999804924,0.00547189964699229),(0.,1.00014406256731),
 .UNSPECIFIED.)
GEOMETRIC_REPRESENTATION_ITEM()
RATIONAL_B_SPLINE_SURFACE(((1.,0.701472497284949,1.0000860132769),(1.,0.73797281472355,
1.00007549661803),(1.,0.771217551452112,1.00006591797378),(1.,0.816811286567555,
1.00005278127272),(1.,0.831011743157808,1.00004868976425),(1.,0.859267298198093,
1.00004054862865),(1.,0.873224671977378,1.00003652715845),(1.,0.886265321053273,
1.00003276981968)))
REPRESENTATION_ITEM('')
SURFACE()
);
#2341=(
BOUNDED_SURFACE()
B_SPLINE_SURFACE(3,2,((#148726,#148727,#148728),(#148729,#148730,#148731),
(#148732,#148733,#148734),(#148735,#148736,#148737),(#148738,#148739,#148740),
(#148741,#148742,#148743),(#148744,#148745,#148746),(#148747,#148748,#148749)),
 .UNSPECIFIED.,.F.,.F.,.F.)
B_SPLINE_SURFACE_WITH_KNOTS((4,2,2,4),(3,3),(0.,0.00133214690895888,0.00266429381791776,
0.00532858763583552),(0.,1.),.UNSPECIFIED.)
GEOMETRIC_REPRESENTATION_ITEM()
RATIONAL_B_SPLINE_SURFACE(((1.,0.882443751548025,1.),(1.,0.870504695835311,
1.),(1.,0.857867656996629,1.),(1.,0.831237498116469,1.),(1.,0.81724531074011,
1.),(1.,0.773060112442974,1.),(1.,0.741342239036411,1.),(1.,0.707106781185704,
1.)))
REPRESENTATION_ITEM('')
SURFACE()
);
#2342=(
BOUNDED_SURFACE()
B_SPLINE_SURFACE(3,2,((#148760,#148761,#148762),(#148763,#148764,#148765),
(#148766,#148767,#148768),(#148769,#148770,#148771)),.UNSPECIFIED.,.F.,
 .F.,.F.)
B_SPLINE_SURFACE_WITH_KNOTS((4,4),(3,3),(0.,0.00876509433037234),(0.,1.),
 .UNSPECIFIED.)
GEOMETRIC_REPRESENTATION_ITEM()
RATIONAL_B_SPLINE_SURFACE(((1.,0.882443751548025,1.),(1.,0.879078911067312,
1.),(1.,0.875892933141997,1.),(1.,0.872863017557589,1.)))
REPRESENTATION_ITEM('')
SURFACE()
);
#2343=(
BOUNDED_SURFACE()
B_SPLINE_SURFACE(3,2,((#148777,#148778,#148779),(#148780,#148781,#148782),
(#148783,#148784,#148785),(#148786,#148787,#148788),(#148789,#148790,#148791),
(#148792,#148793,#148794)),.UNSPECIFIED.,.F.,.F.,.F.)
B_SPLINE_SURFACE_WITH_KNOTS((4,2,4),(3,3),(0.,0.000324772070278169,0.000649544140556338),
(0.,1.),.UNSPECIFIED.)
GEOMETRIC_REPRESENTATION_ITEM()
RATIONAL_B_SPLINE_SURFACE(((1.,0.707106781186543,1.),(1.,0.743104095569232,
1.),(1.,0.776957430466177,1.),(1.,0.834022397797079,1.),(1.,0.857828418485942,
1.),(1.,0.872863017557589,1.)))
REPRESENTATION_ITEM('')
SURFACE()
);
#2344=(
BOUNDED_SURFACE()
B_SPLINE_SURFACE(3,2,((#148823,#148824,#148825),(#148826,#148827,#148828),
(#148829,#148830,#148831),(#148832,#148833,#148834),(#148835,#148836,#148837),
(#148838,#148839,#148840)),.UNSPECIFIED.,.F.,.F.,.F.)
B_SPLINE_SURFACE_WITH_KNOTS((4,2,4),(3,3),(0.,0.000315675390911493,0.000631350781822986),
(0.,1.),.UNSPECIFIED.)
GEOMETRIC_REPRESENTATION_ITEM()
RATIONAL_B_SPLINE_SURFACE(((1.,0.860139545375527,1.),(1.,0.846673137247607,
1.),(1.,0.824923291377528,1.),(1.,0.771907958235216,1.),(1.,0.740773829846737,
1.),(1.,0.70710678118655,1.)))
REPRESENTATION_ITEM('')
SURFACE()
);
#2345=(
BOUNDED_SURFACE()
B_SPLINE_SURFACE(3,2,((#148842,#148843,#148844),(#148845,#148846,#148847),
(#148848,#148849,#148850),(#148851,#148852,#148853)),.UNSPECIFIED.,.F.,
 .F.,.F.)
B_SPLINE_SURFACE_WITH_KNOTS((4,4),(3,3),(0.,0.0135233968444947),(0.,1.),
 .UNSPECIFIED.)
GEOMETRIC_REPRESENTATION_ITEM()
RATIONAL_B_SPLINE_SURFACE(((1.,0.860139545375529,1.),(1.,0.864525021855929,
1.),(1.,0.869269442591942,1.),(1.,0.874466916621369,1.)))
REPRESENTATION_ITEM('')
SURFACE()
);
#2346=(
BOUNDED_SURFACE()
B_SPLINE_SURFACE(3,2,((#148860,#148861,#148862),(#148863,#148864,#148865),
(#148866,#148867,#148868),(#148869,#148870,#148871),(#148872,#148873,#148874),
(#148875,#148876,#148877),(#148878,#148879,#148880),(#148881,#148882,#148883)),
 .UNSPECIFIED.,.F.,.F.,.F.)
B_SPLINE_SURFACE_WITH_KNOTS((4,2,2,4),(3,3),(-0.000144843990829094,0.00249252731595781,
0.00373879097393672,0.00512986098279815),(0.,1.00014484399083),
 .UNSPECIFIED.)
GEOMETRIC_REPRESENTATION_ITEM()
RATIONAL_B_SPLINE_SURFACE(((1.,0.70137438171017,1.00008650825263),(1.,0.736070522946198,
1.00007645719751),(1.,0.767818414112902,1.00006726021499),(1.,0.811420652293743,
1.00005462917062),(1.,0.824998507459968,1.00005069582916),(1.,0.852223941818717,
1.00004280894803),(1.,0.865751049224885,1.00003889030759),(1.,0.878438086880466,
1.00003521502526)))
REPRESENTATION_ITEM('')
SURFACE()
);
#2347=(
BOUNDED_SURFACE()
B_SPLINE_SURFACE(3,2,((#148933,#148934,#148935),(#148936,#148937,#148938),
(#148939,#148940,#148941),(#148942,#148943,#148944),(#148945,#148946,#148947),
(#148948,#148949,#148950),(#148951,#148952,#148953),(#148954,#148955,#148956),
(#148957,#148958,#148959),(#148960,#148961,#148962)),.UNSPECIFIED.,.F.,
 .F.,.F.)
B_SPLINE_SURFACE_WITH_KNOTS((4,2,2,2,4),(3,3),(-0.000328574018954638,0.00116432048255243,
0.00232864096510486,0.0034929614476573,0.00498585604475646),(0.,1.00032857411453),
 .UNSPECIFIED.)
GEOMETRIC_REPRESENTATION_ITEM()
RATIONAL_B_SPLINE_SURFACE(((1.,0.483022826201985,1.00033973063422),(1.,
0.508075627896709,1.00032326722996),(1.,0.53225061289853,1.00030738068138),
(1.,0.573877072079261,1.00028002592744),(1.,0.591639012002754,1.00026835370008),
(1.,0.626354777911338,1.00024554029599),(1.,0.643300055532478,1.00023440473681),
(1.,0.680527266030163,1.00020994094136),(1.,0.700545105936671,1.00019678625332),
(1.,0.719876715686407,1.0001840825202)))
REPRESENTATION_ITEM('')
SURFACE()
);
#2348=(
BOUNDED_SURFACE()
B_SPLINE_SURFACE(3,2,((#149004,#149005,#149006),(#149007,#149008,#149009),
(#149010,#149011,#149012),(#149013,#149014,#149015)),.UNSPECIFIED.,.F.,
 .F.,.F.)
B_SPLINE_SURFACE_WITH_KNOTS((4,4),(3,3),(-1.7347234759768E-18,0.0170848224870981),
(0.,1.),.UNSPECIFIED.)
GEOMETRIC_REPRESENTATION_ITEM()
RATIONAL_B_SPLINE_SURFACE(((1.,0.499602392377301,1.),(1.,0.510855798801923,
1.),(1.,0.520331406035946,1.),(1.,0.528679393385783,1.)))
REPRESENTATION_ITEM('')
SURFACE()
);
#2349=(
BOUNDED_SURFACE()
B_SPLINE_SURFACE(3,2,((#149027,#149028,#149029),(#149030,#149031,#149032),
(#149033,#149034,#149035),(#149036,#149037,#149038),(#149039,#149040,#149041),
(#149042,#149043,#149044),(#149045,#149046,#149047),(#149048,#149049,#149050)),
 .UNSPECIFIED.,.F.,.F.,.F.)
B_SPLINE_SURFACE_WITH_KNOTS((4,2,2,4),(3,3),(0.,0.001434338214324,0.002868676428648,
0.005737352857296),(0.,1.),.UNSPECIFIED.)
GEOMETRIC_REPRESENTATION_ITEM()
RATIONAL_B_SPLINE_SURFACE(((1.,0.45339384727684,1.),(1.,0.47771228976057,
1.),(1.,0.501151853233145,1.),(1.,0.546461020466456,1.),(1.,0.568350660511087,
1.),(1.,0.632070189677047,1.),(1.,0.670684004768455,1.),(1.,0.707106781186548,
1.)))
REPRESENTATION_ITEM('')
SURFACE()
);
#2350=(
BOUNDED_SURFACE()
B_SPLINE_SURFACE(3,2,((#149061,#149062,#149063),(#149064,#149065,#149066),
(#149067,#149068,#149069),(#149070,#149071,#149072)),.UNSPECIFIED.,.F.,
 .F.,.F.)
B_SPLINE_SURFACE_WITH_KNOTS((4,4),(3,3),(0.,0.00407947372412412),(0.,1.),
 .UNSPECIFIED.)
GEOMETRIC_REPRESENTATION_ITEM()
RATIONAL_B_SPLINE_SURFACE(((1.,0.453393847276564,1.),(1.,0.456475766016567,
1.),(1.,0.459447353892611,1.),(1.,0.462319489161104,1.)))
REPRESENTATION_ITEM('')
SURFACE()
);
#2351=(
BOUNDED_SURFACE()
B_SPLINE_SURFACE(3,2,((#149078,#149079,#149080),(#149081,#149082,#149083),
(#149084,#149085,#149086),(#149087,#149088,#149089),(#149090,#149091,#149092),
(#149093,#149094,#149095),(#149096,#149097,#149098),(#149099,#149100,#149101)),
 .UNSPECIFIED.,.F.,.F.,.F.)
B_SPLINE_SURFACE_WITH_KNOTS((4,2,2,4),(3,3),(0.,0.000337961269725901,0.000506941904588851,
0.000675922539451801),(0.,1.),.UNSPECIFIED.)
GEOMETRIC_REPRESENTATION_ITEM()
RATIONAL_B_SPLINE_SURFACE(((1.,0.707106781186548,1.),(1.,0.66833529952704,
1.),(1.,0.625126311995779,1.),(1.,0.560329805282816,1.),(1.,0.53845874286336,
1.),(1.,0.497198802480914,1.),(1.,0.478168468596388,1.),(1.,0.462319489161107,
1.)))
REPRESENTATION_ITEM('')
SURFACE()
);
#2352=(
BOUNDED_SURFACE()
B_SPLINE_SURFACE(3,2,((#149126,#149127,#149128),(#149129,#149130,#149131),
(#149132,#149133,#149134),(#149135,#149136,#149137),(#149138,#149139,#149140),
(#149141,#149142,#149143),(#149144,#149145,#149146),(#149147,#149148,#149149),
(#149150,#149151,#149152),(#149153,#149154,#149155)),.UNSPECIFIED.,.F.,
 .F.,.F.)
B_SPLINE_SURFACE_WITH_KNOTS((4,2,2,2,4),(3,3),(1.5707963267949,1.96349540849362,
2.35619449019234,2.74889357189107,3.14159265358979),(0.,1.),
 .UNSPECIFIED.)
GEOMETRIC_REPRESENTATION_ITEM()
RATIONAL_B_SPLINE_SURFACE(((1.,0.70710678118655,1.),(1.,0.7006663788345,
1.),(1.,0.694134907060529,1.),(1.,0.681903435451519,1.),(1.,0.676209154063276,
1.),(1.,0.666616044205195,1.),(1.,0.662724068472661,1.),(1.,0.657443209221257,
1.),(1.,0.656051196071916,1.),(1.,0.656059028990507,1.)))
REPRESENTATION_ITEM('')
SURFACE()
);
#2353=(
BOUNDED_SURFACE()
B_SPLINE_SURFACE(3,2,((#149194,#149195,#149196),(#149197,#149198,#149199),
(#149200,#149201,#149202),(#149203,#149204,#149205),(#149206,#149207,#149208),
(#149209,#149210,#149211),(#149212,#149213,#149214),(#149215,#149216,#149217),
(#149218,#149219,#149220),(#149221,#149222,#149223)),.UNSPECIFIED.,.F.,
 .F.,.F.)
B_SPLINE_SURFACE_WITH_KNOTS((4,2,2,2,4),(3,3),(0.,0.000175112702239915,
0.000350225404479831,0.000525338106719747,0.000700450808959663),(0.,1.),
 .UNSPECIFIED.)
GEOMETRIC_REPRESENTATION_ITEM()
RATIONAL_B_SPLINE_SURFACE(((1.,0.441891116431771,1.),(1.,0.459945578495206,
1.),(1.,0.481391225572596,1.),(1.,0.52725624746098,1.),(1.,0.550835433567685,
1.),(1.,0.597437830540943,1.),(1.,0.62070290968502,1.),(1.,0.665021344579013,
1.),(1.,0.68636937449165,1.),(1.,0.707106781186548,1.)))
REPRESENTATION_ITEM('')
SURFACE()
);
#2354=(
BOUNDED_SURFACE()
B_SPLINE_SURFACE(3,2,((#149225,#149226,#149227),(#149228,#149229,#149230),
(#149231,#149232,#149233),(#149234,#149235,#149236)),.UNSPECIFIED.,.F.,
 .F.,.F.)
B_SPLINE_SURFACE_WITH_KNOTS((4,4),(3,3),(1.7347234759768E-18,0.00426411906192034),
(0.,1.),.UNSPECIFIED.)
GEOMETRIC_REPRESENTATION_ITEM()
RATIONAL_B_SPLINE_SURFACE(((1.,0.441891116431774,1.),(1.,0.438589787881315,
1.),(1.,0.435168043398159,1.),(1.,0.431612184895232,1.)))
REPRESENTATION_ITEM('')
SURFACE()
);
#2355=(
BOUNDED_SURFACE()
B_SPLINE_SURFACE(3,2,((#149243,#149244,#149245),(#149246,#149247,#149248),
(#149249,#149250,#149251),(#149252,#149253,#149254),(#149255,#149256,#149257),
(#149258,#149259,#149260),(#149261,#149262,#149263),(#149264,#149265,#149266),
(#149267,#149268,#149269),(#149270,#149271,#149272)),.UNSPECIFIED.,.F.,
 .F.,.F.)
B_SPLINE_SURFACE_WITH_KNOTS((4,2,2,2,4),(3,3),(-0.000627077628646835,0.00156769407161709,
0.00313538814323418,0.00470308221485126,0.00689785374126868),(0.,1.00120059479706),
 .UNSPECIFIED.)
GEOMETRIC_REPRESENTATION_ITEM()
RATIONAL_B_SPLINE_SURFACE(((1.,0.729847250011682,1.00064868797209),(1.,
0.70323368126333,1.00071259219644),(1.,0.675527972127855,1.00077911885691),
(1.,0.62520314302849,1.00089995831287),(1.,0.603398245983805,1.00095231600475),
(1.,0.55753734457264,1.001062436724),(1.,0.533442814445538,1.00112029225901),
(1.,0.47370313538274,1.00126373855474),(1.,0.436994504158806,1.00135188293805),
(1.,0.398153145892338,1.00144514840334)))
REPRESENTATION_ITEM('')
SURFACE()
);
#2356=(
BOUNDED_SURFACE()
B_SPLINE_SURFACE(3,2,((#149328,#149329,#149330),(#149331,#149332,#149333),
(#149334,#149335,#149336),(#149337,#149338,#149339),(#149340,#149341,#149342),
(#149343,#149344,#149345),(#149346,#149347,#149348),(#149349,#149350,#149351),
(#149352,#149353,#149354),(#149355,#149356,#149357),(#149358,#149359,#149360),
(#149361,#149362,#149363)),.UNSPECIFIED.,.F.,.F.,.F.)
B_SPLINE_SURFACE_WITH_KNOTS((4,2,2,2,2,4),(3,3),(-0.000627228261712472,
0.0015680710888481,0.00235210663327216,0.0031361421776962,0.00470421326654431,
0.00689951279093165),(0.,1.00121732095691),.UNSPECIFIED.)
GEOMETRIC_REPRESENTATION_ITEM()
RATIONAL_B_SPLINE_SURFACE(((1.,0.398113494737596,1.00146537811308),(1.,
0.437012270486998,1.00137067352324),(1.,0.473696248960092,1.00128136117168),
(1.,0.520905142750056,1.00116642442016),(1.,0.533089323815758,1.00113676030225),
(1.,0.557031366991619,1.00107847000043),(1.,0.568823900888959,1.00104975940313),
(1.,0.603302051221277,1.00096581745322),(1.,0.625142666027295,1.00091264337699),
(1.,0.675522559468756,1.00078998637681),(1.,0.703234839482815,1.00072251689836),
(1.,0.729837417574121,1.00065774914672)))
REPRESENTATION_ITEM('')
SURFACE()
);
#2357=(
BOUNDED_SURFACE()
B_SPLINE_SURFACE(3,2,((#149415,#149416,#149417),(#149418,#149419,#149420),
(#149421,#149422,#149423),(#149424,#149425,#149426)),.UNSPECIFIED.,.F.,
 .F.,.F.)
B_SPLINE_SURFACE_WITH_KNOTS((4,4),(3,3),(-1.00613961606655E-16,0.00454919832189776),
(0.,1.),.UNSPECIFIED.)
GEOMETRIC_REPRESENTATION_ITEM()
RATIONAL_B_SPLINE_SURFACE(((1.,0.43161218489519,1.),(1.,0.4354057728044,
1.),(1.,0.439046733702441,1.),(1.,0.442551630563568,1.)))
REPRESENTATION_ITEM('')
SURFACE()
);
#2358=(
BOUNDED_SURFACE()
B_SPLINE_SURFACE(3,2,((#149433,#149434,#149435),(#149436,#149437,#149438),
(#149439,#149440,#149441),(#149442,#149443,#149444),(#149445,#149446,#149447),
(#149448,#149449,#149450),(#149451,#149452,#149453),(#149454,#149455,#149456)),
 .UNSPECIFIED.,.F.,.F.,.F.)
B_SPLINE_SURFACE_WITH_KNOTS((4,2,2,4),(3,3),(0.,0.000350059279280428,0.000525088918920643,
0.000700118558560857),(0.,1.),.UNSPECIFIED.)
GEOMETRIC_REPRESENTATION_ITEM()
RATIONAL_B_SPLINE_SURFACE(((1.,0.707106781186548,1.),(1.,0.666269021153261,
1.),(1.,0.620643690025591,1.),(1.,0.551020195303415,1.),(1.,0.527243635346707,
1.),(1.,0.48184496425994,1.),(1.,0.460546552679624,1.),(1.,0.442551630563558,
1.)))
REPRESENTATION_ITEM('')
SURFACE()
);
#2359=(
BOUNDED_SURFACE()
B_SPLINE_SURFACE(3,2,((#149477,#149478,#149479),(#149480,#149481,#149482),
(#149483,#149484,#149485),(#149486,#149487,#149488),(#149489,#149490,#149491),
(#149492,#149493,#149494),(#149495,#149496,#149497),(#149498,#149499,#149500),
(#149501,#149502,#149503),(#149504,#149505,#149506)),.UNSPECIFIED.,.F.,
 .F.,.F.)
B_SPLINE_SURFACE_WITH_KNOTS((4,2,2,2,4),(3,3),(0.00131180726843867,0.00173116479138242,
0.00215052231432617,0.00256987983726992,0.00298923736021366),(0.,1.00000719536586),
 .UNSPECIFIED.)
GEOMETRIC_REPRESENTATION_ITEM()
RATIONAL_B_SPLINE_SURFACE(((1.,0.70710467371268,1.00000421497806),(1.,0.735459277069437,
1.00000380693457),(1.,0.75707678402216,1.00000349584283),(1.,0.786069896432003,
1.00000307861073),(1.,0.793429076618853,1.00000297270674),(1.,0.793448571747271,
1.00000297242619),(1.,0.786103829137559,1.00000307812241),(1.,0.757124528683257,
1.00000349515575),(1.,0.735523766262829,1.00000380600653),(1.,0.70710467371268,
1.00000421497806)))
REPRESENTATION_ITEM('')
SURFACE()
);
#2360=(
BOUNDED_SURFACE()
B_SPLINE_SURFACE(3,2,((#149527,#149528,#149529),(#149530,#149531,#149532),
(#149533,#149534,#149535),(#149536,#149537,#149538),(#149539,#149540,#149541),
(#149542,#149543,#149544),(#149545,#149546,#149547),(#149548,#149549,#149550),
(#149551,#149552,#149553),(#149554,#149555,#149556)),.UNSPECIFIED.,.F.,
 .F.,.F.)
B_SPLINE_SURFACE_WITH_KNOTS((4,2,2,2,4),(3,3),(3.1415926535898,3.53429173528852,
3.92699081698724,4.31968989868597,4.71238898038469),(0.,1.),
 .UNSPECIFIED.)
GEOMETRIC_REPRESENTATION_ITEM()
RATIONAL_B_SPLINE_SURFACE(((1.,0.754709580222776,1.),(1.,0.75471421973084,
1.),(1.,0.753512297096162,1.),(1.,0.748871927696637,1.),(1.,0.745429366938649,
1.),(1.,0.736738129296255,1.),(1.,0.73149075639724,1.),(1.,0.719894264862275,
1.),(1.,0.713550261851491,1.),(1.,0.707106781186548,1.)))
REPRESENTATION_ITEM('')
SURFACE()
);
#2361=(
BOUNDED_SURFACE()
B_SPLINE_SURFACE(3,2,((#149596,#149597,#149598),(#149599,#149600,#149601),
(#149602,#149603,#149604),(#149605,#149606,#149607),(#149608,#149609,#149610),
(#149611,#149612,#149613)),.UNSPECIFIED.,.F.,.F.,.F.)
B_SPLINE_SURFACE_WITH_KNOTS((4,2,4),(3,3),(-3.80119597236557E-5,0.000488761174293955,
0.00101555203427385),(-3.80296856860089E-5,1.),.UNSPECIFIED.)
GEOMETRIC_REPRESENTATION_ITEM()
RATIONAL_B_SPLINE_SURFACE(((1.00001434166179,0.81144122631948,1.),(1.00001374938095,
0.819228311950262,1.),(1.00001345333693,0.823120587367281,1.),(1.00001327853937,
0.825418760007561,1.),(1.00001340351003,0.823775692776788,1.),(1.00001365395156,
0.820482981788876,1.)))
REPRESENTATION_ITEM('')
SURFACE()
);
#2362=(
BOUNDED_SURFACE()
B_SPLINE_SURFACE(3,2,((#149641,#149642,#149643),(#149644,#149645,#149646),
(#149647,#149648,#149649),(#149650,#149651,#149652)),.UNSPECIFIED.,.F.,
 .F.,.F.)
B_SPLINE_SURFACE_WITH_KNOTS((4,4),(3,3),(0.,0.000106239733749475),(0.,1.),
 .UNSPECIFIED.)
GEOMETRIC_REPRESENTATION_ITEM()
RATIONAL_B_SPLINE_SURFACE(((1.,0.835215680136664,1.),(1.,0.831333836917881,
1.),(1.,0.826651097750167,1.),(1.,0.821176675475199,1.)))
REPRESENTATION_ITEM('')
SURFACE()
);
#2363=(
BOUNDED_SURFACE()
B_SPLINE_SURFACE(3,2,((#149656,#149657,#149658),(#149659,#149660,#149661),
(#149662,#149663,#149664),(#149665,#149666,#149667),(#149668,#149669,#149670),
(#149671,#149672,#149673)),.UNSPECIFIED.,.F.,.F.,.F.)
B_SPLINE_SURFACE_WITH_KNOTS((4,2,4),(3,3),(0.,0.0130414224518927,0.0260828449037854),
(0.,1.),.UNSPECIFIED.)
GEOMETRIC_REPRESENTATION_ITEM()
RATIONAL_B_SPLINE_SURFACE(((1.,0.835215680136663,1.),(1.,0.838844513950773,
1.),(1.,0.842771271110783,1.),(1.,0.851396246528345,1.),(1.,0.856094111052002,
1.),(1.,0.861290731803024,1.)))
REPRESENTATION_ITEM('')
SURFACE()
);
#2364=(
BOUNDED_SURFACE()
B_SPLINE_SURFACE(3,2,((#149682,#149683,#149684),(#149685,#149686,#149687),
(#149688,#149689,#149690),(#149691,#149692,#149693),(#149694,#149695,#149696),
(#149697,#149698,#149699)),.UNSPECIFIED.,.F.,.F.,.F.)
B_SPLINE_SURFACE_WITH_KNOTS((4,2,4),(3,3),(-0.00015233523741089,0.0022325368353913,
0.00461734601372613),(0.,1.00015233523741),.UNSPECIFIED.)
GEOMETRIC_REPRESENTATION_ITEM()
RATIONAL_B_SPLINE_SURFACE(((1.,0.700994279879693,1.00009109821472),(1.,
0.732815663384495,1.0000814031787),(1.,0.762177009942305,1.0000724576433),
(1.,0.817213761356616,1.00005568957012),(1.,0.843031394120544,1.00004782369969),
(1.,0.865639026170535,1.00004093582169)))
REPRESENTATION_ITEM('')
SURFACE()
);
#2365=(
BOUNDED_SURFACE()
B_SPLINE_SURFACE(3,2,((#149743,#149744,#149745),(#149746,#149747,#149748),
(#149749,#149750,#149751),(#149752,#149753,#149754),(#149755,#149756,#149757),
(#149758,#149759,#149760),(#149761,#149762,#149763),(#149764,#149765,#149766)),
 .UNSPECIFIED.,.F.,.F.,.F.)
B_SPLINE_SURFACE_WITH_KNOTS((4,2,2,4),(3,3),(0.,0.00223318354977648,0.00334977532466471,
0.00446636709955295),(0.,1.),.UNSPECIFIED.)
GEOMETRIC_REPRESENTATION_ITEM()
RATIONAL_B_SPLINE_SURFACE(((1.,0.861290731803006,1.),(1.,0.839613661895165,
1.),(1.,0.815980432119487,1.),(1.,0.777267373295742,1.),(1.,0.763786842194511,
1.),(1.,0.736109943319361,1.),(1.,0.721853181403518,1.),(1.,0.707106781186545,
1.)))
REPRESENTATION_ITEM('')
SURFACE()
);
#2366=(
BOUNDED_SURFACE()
B_SPLINE_SURFACE(3,2,((#149779,#149780,#149781),(#149782,#149783,#149784),
(#149785,#149786,#149787),(#149788,#149789,#149790),(#149791,#149792,#149793),
(#149794,#149795,#149796)),.UNSPECIFIED.,.F.,.F.,.F.)
B_SPLINE_SURFACE_WITH_KNOTS((4,2,4),(3,3),(0.,0.0129055642122842,0.0258111284245685),
(0.,1.),.UNSPECIFIED.)
GEOMETRIC_REPRESENTATION_ITEM()
RATIONAL_B_SPLINE_SURFACE(((1.,0.861290731803006,1.),(1.,0.856148221578915,
1.),(1.,0.851494227257712,1.),(1.,0.842943112520738,1.),(1.,0.839046328378941,
1.),(1.,0.835442841040481,1.)))
REPRESENTATION_ITEM('')
SURFACE()
);
#2367=(
BOUNDED_SURFACE()
B_SPLINE_SURFACE(3,2,((#149804,#149805,#149806),(#149807,#149808,#149809),
(#149810,#149811,#149812),(#149813,#149814,#149815)),.UNSPECIFIED.,.F.,
 .F.,.F.)
B_SPLINE_SURFACE_WITH_KNOTS((4,4),(3,3),(0.,0.000212668013534773),(0.,1.),
 .UNSPECIFIED.)
GEOMETRIC_REPRESENTATION_ITEM()
RATIONAL_B_SPLINE_SURFACE(((1.,0.802684671197877,1.),(1.,0.816456497832501,
1.),(1.,0.82752079624252,1.),(1.,0.835442841040483,1.)))
REPRESENTATION_ITEM('')
SURFACE()
);
#2368=(
BOUNDED_SURFACE()
B_SPLINE_SURFACE(3,2,((#149817,#149818,#149819),(#149820,#149821,#149822),
(#149823,#149824,#149825),(#149826,#149827,#149828)),.UNSPECIFIED.,.F.,
 .F.,.F.)
B_SPLINE_SURFACE_WITH_KNOTS((4,4),(3,3),(-1.1328828500301E-15,0.000723745383907254),
(0.,1.),.UNSPECIFIED.)
GEOMETRIC_REPRESENTATION_ITEM()
RATIONAL_B_SPLINE_SURFACE(((1.,0.802684671198269,1.),(1.,0.797620722711664,
1.),(1.,0.787749610789602,1.),(1.,0.773398994756355,1.)))
REPRESENTATION_ITEM('')
SURFACE()
);
#2369=(
BOUNDED_SURFACE()
B_SPLINE_SURFACE(3,2,((#149848,#149849,#149850),(#149851,#149852,#149853),
(#149854,#149855,#149856),(#149857,#149858,#149859),(#149860,#149861,#149862),
(#149863,#149864,#149865),(#149866,#149867,#149868),(#149869,#149870,#149871)),
 .UNSPECIFIED.,.F.,.F.,.F.)
B_SPLINE_SURFACE_WITH_KNOTS((4,2,2,4),(3,3),(-6.50521303491303E-18,0.000158176853950714,
0.000316353707901435,0.000632707415802875),(0.,1.),.UNSPECIFIED.)
GEOMETRIC_REPRESENTATION_ITEM()
RATIONAL_B_SPLINE_SURFACE(((1.,0.50825434412561,1.),(1.,0.519857702736613,
1.),(1.,0.534132547044037,1.),(1.,0.566198696596924,1.),(1.,0.583560620774966,
1.),(1.,0.636763258069658,1.),(1.,0.673308410857549,1.),(1.,0.707106781186552,
1.)))
REPRESENTATION_ITEM('')
SURFACE()
);
#2370=(
BOUNDED_SURFACE()
B_SPLINE_SURFACE(3,2,((#149875,#149876,#149877),(#149878,#149879,#149880),
(#149881,#149882,#149883),(#149884,#149885,#149886)),.UNSPECIFIED.,.F.,
 .F.,.F.)
B_SPLINE_SURFACE_WITH_KNOTS((4,4),(3,3),(-6.93889390390723E-18,0.0177935197894076),
(0.,1.),.UNSPECIFIED.)
GEOMETRIC_REPRESENTATION_ITEM()
RATIONAL_B_SPLINE_SURFACE(((1.,0.508254344125608,1.),(1.,0.498412666571477,
1.),(1.,0.487173250319529,1.),(1.,0.473671517629131,1.)))
REPRESENTATION_ITEM('')
SURFACE()
);
#2371=(
BOUNDED_SURFACE()
B_SPLINE_SURFACE(3,2,((#149888,#149889,#149890),(#149891,#149892,#149893),
(#149894,#149895,#149896),(#149897,#149898,#149899),(#149900,#149901,#149902),
(#149903,#149904,#149905),(#149906,#149907,#149908),(#149909,#149910,#149911)),
 .UNSPECIFIED.,.F.,.F.,.F.)
B_SPLINE_SURFACE_WITH_KNOTS((4,2,2,4),(3,3),(0.,0.00262348010799063,0.00393522016198593,
0.00524696021598125),(0.,1.),.UNSPECIFIED.)
GEOMETRIC_REPRESENTATION_ITEM()
RATIONAL_B_SPLINE_SURFACE(((1.,0.70710678118732,1.),(1.,0.673159051373371,
1.),(1.,0.637356734328886,1.),(1.,0.579048422068377,1.),(1.,0.558729842945168,
1.),(1.,0.517089292555981,1.),(1.,0.495689661102028,1.),(1.,0.473671517629131,
1.)))
REPRESENTATION_ITEM('')
SURFACE()
);
#2372=(
BOUNDED_SURFACE()
B_SPLINE_SURFACE(3,2,((#149928,#149929,#149930),(#149931,#149932,#149933),
(#149934,#149935,#149936),(#149937,#149938,#149939),(#149940,#149941,#149942),
(#149943,#149944,#149945),(#149946,#149947,#149948),(#149949,#149950,#149951),
(#149952,#149953,#149954),(#149955,#149956,#149957)),.UNSPECIFIED.,.F.,
 .F.,.F.)
B_SPLINE_SURFACE_WITH_KNOTS((4,2,2,2,4),(3,3),(-4.33680868994201E-18,0.00131184996336558,
0.00262369992673117,0.00393554989009676,0.00524739985346235),(0.,1.),
 .UNSPECIFIED.)
GEOMETRIC_REPRESENTATION_ITEM()
RATIONAL_B_SPLINE_SURFACE(((1.,0.473671517629133,1.),(1.,0.495707594803631,
1.),(1.,0.517034522428114,1.),(1.,0.558412152901823,1.),(1.,0.578466470542957,
1.),(1.,0.617536962037478,1.),(1.,0.636393525150058,1.),(1.,0.672664546785766,
1.),(1.,0.690145348310819,1.),(1.,0.707106781186548,1.)))
REPRESENTATION_ITEM('')
SURFACE()
);
#2373=(
BOUNDED_SURFACE()
B_SPLINE_SURFACE(3,2,((#149970,#149971,#149972),(#149973,#149974,#149975),
(#149976,#149977,#149978),(#149979,#149980,#149981)),.UNSPECIFIED.,.F.,
 .F.,.F.)
B_SPLINE_SURFACE_WITH_KNOTS((4,4),(3,3),(0.,0.0180689587739334),(0.,1.),
 .UNSPECIFIED.)
GEOMETRIC_REPRESENTATION_ITEM()
RATIONAL_B_SPLINE_SURFACE(((1.,0.473671517629134,1.),(1.,0.487381853083234,
1.),(1.,0.49876090260372,1.),(1.,0.508709923441297,1.)))
REPRESENTATION_ITEM('')
SURFACE()
);
#2374=(
BOUNDED_SURFACE()
B_SPLINE_SURFACE(3,2,((#149988,#149989,#149990),(#149991,#149992,#149993),
(#149994,#149995,#149996),(#149997,#149998,#149999),(#150000,#150001,#150002),
(#150003,#150004,#150005),(#150006,#150007,#150008),(#150009,#150010,#150011),
(#150012,#150013,#150014),(#150015,#150016,#150017)),.UNSPECIFIED.,.F.,
 .F.,.F.)
B_SPLINE_SURFACE_WITH_KNOTS((4,2,2,2,4),(3,3),(0.,0.000157845161260656,
0.000315690322521312,0.000473535483781968,0.000631380645042625),(0.,1.),
 .UNSPECIFIED.)
GEOMETRIC_REPRESENTATION_ITEM()
RATIONAL_B_SPLINE_SURFACE(((1.,0.707106781186548,1.),(1.,0.690126575842363,
1.),(1.,0.672866331348439,1.),(1.,0.637644189799934,1.),(1.,0.619386686649187,
1.),(1.,0.584119465416144,1.),(1.,0.567005655158962,1.),(1.,0.534765171917349,
1.),(1.,0.520258799319389,1.),(1.,0.508709923441296,1.)))
REPRESENTATION_ITEM('')
SURFACE()
);
#2375=(
BOUNDED_SURFACE()
B_SPLINE_SURFACE(3,2,((#150034,#150035,#150036),(#150037,#150038,#150039),
(#150040,#150041,#150042),(#150043,#150044,#150045),(#150046,#150047,#150048),
(#150049,#150050,#150051),(#150052,#150053,#150054),(#150055,#150056,#150057),
(#150058,#150059,#150060),(#150061,#150062,#150063)),.UNSPECIFIED.,.F.,
 .F.,.F.)
B_SPLINE_SURFACE_WITH_KNOTS((4,2,2,2,4),(3,3),(1.5707963267949,1.96349540849362,
2.35619449019234,2.74889357189107,3.14159265358979),(0.,1.),
 .UNSPECIFIED.)
GEOMETRIC_REPRESENTATION_ITEM()
RATIONAL_B_SPLINE_SURFACE(((1.,0.707106781186548,1.),(1.,0.700666378834645,
1.),(1.,0.694134907060333,1.),(1.,0.681903435451719,1.),(1.,0.676209154063922,
1.),(1.,0.666616044204548,1.),(1.,0.662724068472644,1.),(1.,0.657443209221262,
1.),(1.,0.656051196071901,1.),(1.,0.656059028990513,1.)))
REPRESENTATION_ITEM('')
SURFACE()
);
#2376=(
BOUNDED_SURFACE()
B_SPLINE_SURFACE(3,2,((#150118,#150119,#150120),(#150121,#150122,#150123),
(#150124,#150125,#150126),(#150127,#150128,#150129),(#150130,#150131,#150132),
(#150133,#150134,#150135),(#150136,#150137,#150138),(#150139,#150140,#150141),
(#150142,#150143,#150144),(#150145,#150146,#150147)),.UNSPECIFIED.,.F.,
 .F.,.F.)
B_SPLINE_SURFACE_WITH_KNOTS((4,2,2,2,4),(3,3),(3.1415926535898,3.53429173528852,
3.92699081698724,4.31968989868597,4.71238898038469),(0.,1.),
 .UNSPECIFIED.)
GEOMETRIC_REPRESENTATION_ITEM()
RATIONAL_B_SPLINE_SURFACE(((1.,0.754709580222772,1.),(1.,0.754714219730848,
1.),(1.,0.753512297096158,1.),(1.,0.748871927696634,1.),(1.,0.745429366938649,
1.),(1.,0.736738129296255,1.),(1.,0.731490756397077,1.),(1.,0.719894264862441,
1.),(1.,0.713550261851367,1.),(1.,0.707106781186548,1.)))
REPRESENTATION_ITEM('')
SURFACE()
);
#2377=(
BOUNDED_SURFACE()
B_SPLINE_SURFACE(3,2,((#150164,#150165,#150166),(#150167,#150168,#150169),
(#150170,#150171,#150172),(#150173,#150174,#150175),(#150176,#150177,#150178),
(#150179,#150180,#150181)),.UNSPECIFIED.,.F.,.F.,.F.)
B_SPLINE_SURFACE_WITH_KNOTS((4,2,4),(3,3),(0.,0.000324038763230374,0.000648077526460748),
(0.,1.),.UNSPECIFIED.)
GEOMETRIC_REPRESENTATION_ITEM()
RATIONAL_B_SPLINE_SURFACE(((1.,0.87207744658335,1.),(1.,0.857354948275163,
1.),(1.,0.833755771861677,1.),(1.,0.776640613237984,1.),(1.,0.743340108181467,
1.),(1.,0.707106781186543,1.)))
REPRESENTATION_ITEM('')
SURFACE()
);
#2378=(
BOUNDED_SURFACE()
B_SPLINE_SURFACE(3,2,((#150190,#150191,#150192),(#150193,#150194,#150195),
(#150196,#150197,#150198),(#150199,#150200,#150201)),.UNSPECIFIED.,.F.,
 .F.,.F.)
B_SPLINE_SURFACE_WITH_KNOTS((4,4),(3,3),(0.,0.0141656229616797),(0.,1.),
 .UNSPECIFIED.)
GEOMETRIC_REPRESENTATION_ITEM()
RATIONAL_B_SPLINE_SURFACE(((1.,0.872077446583348,1.),(1.,0.876947206822174,
1.),(1.,0.882221222508023,1.),(1.,0.887998771276578,1.)))
REPRESENTATION_ITEM('')
SURFACE()
);
#2379=(
BOUNDED_SURFACE()
B_SPLINE_SURFACE(3,2,((#150208,#150209,#150210),(#150211,#150212,#150213),
(#150214,#150215,#150216),(#150217,#150218,#150219),(#150220,#150221,#150222),
(#150223,#150224,#150225),(#150226,#150227,#150228),(#150229,#150230,#150231)),
 .UNSPECIFIED.,.F.,.F.,.F.)
B_SPLINE_SURFACE_WITH_KNOTS((4,2,2,4),(3,3),(-0.000151407848110819,0.00278824321172774,
0.00418236481759161,0.0057276222743267),(0.,1.00015140784811),
 .UNSPECIFIED.)
GEOMETRIC_REPRESENTATION_ITEM()
RATIONAL_B_SPLINE_SURFACE(((1.,0.701236390783137,1.00009047031033),(1.,
0.739120426865072,1.00007899842957),(1.,0.773512306563008,1.00006858402857),
(1.,0.820586923934616,1.00005432909554),(1.,0.835217331499987,1.00004989877849),
(1.,0.864264001665827,1.00004110299084),(1.,0.878586452051055,1.00003676592805),
(1.,0.891923360613614,1.0000327273028)))
REPRESENTATION_ITEM('')
SURFACE()
);
#2380=(
BOUNDED_SURFACE()
B_SPLINE_SURFACE(3,2,((#150278,#150279,#150280),(#150281,#150282,#150283),
(#150284,#150285,#150286),(#150287,#150288,#150289),(#150290,#150291,#150292),
(#150293,#150294,#150295),(#150296,#150297,#150298),(#150299,#150300,#150301)),
 .UNSPECIFIED.,.F.,.F.,.F.)
B_SPLINE_SURFACE_WITH_KNOTS((4,2,2,4),(3,3),(-8.78076470147105E-5,0.00139422219513554,
0.00278844439027108,0.0056649682329014),(0.,1.00008807945236),
 .UNSPECIFIED.)
GEOMETRIC_REPRESENTATION_ITEM()
RATIONAL_B_SPLINE_SURFACE(((1.,0.890287745294558,1.00001932679062),(1.,
0.87740523386917,1.00002159615973),(1.,0.863663500716923,1.00002401688839),
(1.,0.835397058527914,1.00002899627389),(1.,0.820967815861932,1.00003153811347),
(1.,0.774347259046824,1.0000397507397),(1.,0.740581186868133,1.00004569893399),
(0.999999999999999,0.703701983503653,1.00005219553406)))
REPRESENTATION_ITEM('')
SURFACE()
);
#2381=(
BOUNDED_SURFACE()
B_SPLINE_SURFACE(3,2,((#150350,#150351,#150352),(#150353,#150354,#150355),
(#150356,#150357,#150358),(#150359,#150360,#150361)),.UNSPECIFIED.,.F.,
 .F.,.F.)
B_SPLINE_SURFACE_WITH_KNOTS((4,4),(3,3),(0.,0.0138879247081574),(0.,1.),
 .UNSPECIFIED.)
GEOMETRIC_REPRESENTATION_ITEM()
RATIONAL_B_SPLINE_SURFACE(((1.,0.887998771276556,1.),(1.,0.882334484690674,
1.),(1.,0.877154223922122,1.),(1.,0.872364293278347,1.)))
REPRESENTATION_ITEM('')
SURFACE()
);
#2382=(
BOUNDED_SURFACE()
B_SPLINE_SURFACE(3,2,((#150367,#150368,#150369),(#150370,#150371,#150372),
(#150373,#150374,#150375),(#150376,#150377,#150378),(#150379,#150380,#150381),
(#150382,#150383,#150384)),.UNSPECIFIED.,.F.,.F.,.F.)
B_SPLINE_SURFACE_WITH_KNOTS((4,2,4),(3,3),(0.,0.000324353517959648,0.000648707035919297),
(0.,1.),.UNSPECIFIED.)
GEOMETRIC_REPRESENTATION_ITEM()
RATIONAL_B_SPLINE_SURFACE(((1.,0.707106781186548,1.),(1.,0.742998991655634,
1.),(1.,0.776756965569408,1.),(1.,0.833658724502819,1.),(1.,0.857385369677227,
1.),(1.,0.872364293278349,1.)))
REPRESENTATION_ITEM('')
SURFACE()
);
#2383=(
BOUNDED_SURFACE()
B_SPLINE_SURFACE(3,2,((#150411,#150412,#150413),(#150414,#150415,#150416),
(#150417,#150418,#150419),(#150420,#150421,#150422)),.UNSPECIFIED.,.F.,
 .F.,.F.)
B_SPLINE_SURFACE_WITH_KNOTS((4,4),(3,3),(0.00167806205423436,0.0019221164224989),
(0.,1.),.UNSPECIFIED.)
GEOMETRIC_REPRESENTATION_ITEM()
RATIONAL_B_SPLINE_SURFACE(((1.,0.83648401963888,1.),(1.,0.827500667105214,
1.),(1.,0.81402442184051,1.),(1.,0.797363061122239,1.)))
REPRESENTATION_ITEM('')
SURFACE()
);
#2384=(
BOUNDED_SURFACE()
B_SPLINE_SURFACE(3,2,((#150424,#150425,#150426),(#150427,#150428,#150429),
(#150430,#150431,#150432),(#150433,#150434,#150435),(#150436,#150437,#150438),
(#150439,#150440,#150441),(#150442,#150443,#150444),(#150445,#150446,#150447),
(#150448,#150449,#150450),(#150451,#150452,#150453)),.UNSPECIFIED.,.F.,
 .F.,.F.)
B_SPLINE_SURFACE_WITH_KNOTS((4,2,2,2,4),(3,3),(0.,0.000158289020679031,
0.000316578041358062,0.000474867062037094,0.000633156082716125),(0.,1.),
 .UNSPECIFIED.)
GEOMETRIC_REPRESENTATION_ITEM()
RATIONAL_B_SPLINE_SURFACE(((1.,0.707106781186548,1.),(1.,0.689988873362392,
1.),(1.,0.672579653000586,1.),(1.,0.63703033863955,1.),(1.,0.61859446393025,
1.),(1.,0.582956103977724,1.),(1.,0.565642356156971,1.),(1.,0.532984405418804,
1.),(1.,0.518263379167526,1.),(1.,0.506538946041792,1.)))
REPRESENTATION_ITEM('')
SURFACE()
);
#2385=(
BOUNDED_SURFACE()
B_SPLINE_SURFACE(3,2,((#150456,#150457,#150458),(#150459,#150460,#150461),
(#150462,#150463,#150464),(#150465,#150466,#150467),(#150468,#150469,#150470),
(#150471,#150472,#150473)),.UNSPECIFIED.,.F.,.F.,.F.)
B_SPLINE_SURFACE_WITH_KNOTS((4,2,4),(3,3),(0.,0.000518347860385374,0.00103669572077075),
(0.,1.),.UNSPECIFIED.)
GEOMETRIC_REPRESENTATION_ITEM()
RATIONAL_B_SPLINE_SURFACE(((1.,0.819851970694872,1.),(1.,0.821199393891468,
1.),(1.,0.820620061026224,1.),(1.,0.813565992888811,1.),(1.,0.807280082867884,
1.),(1.,0.797551754323293,1.)))
REPRESENTATION_ITEM('')
SURFACE()
);
#2386=(
BOUNDED_SURFACE()
B_SPLINE_SURFACE(3,2,((#150504,#150505,#150506),(#150507,#150508,#150509),
(#150510,#150511,#150512),(#150513,#150514,#150515),(#150516,#150517,#150518),
(#150519,#150520,#150521)),.UNSPECIFIED.,.F.,.F.,.F.)
B_SPLINE_SURFACE_WITH_KNOTS((4,2,4),(3,3),(0.,0.0127570403976527,0.0255140807953054),
(0.,1.),.UNSPECIFIED.)
GEOMETRIC_REPRESENTATION_ITEM()
RATIONAL_B_SPLINE_SURFACE(((1.,0.83648401963888,1.),(1.,0.840071262854844,
1.),(1.,0.843946769546665,1.),(1.,0.852439323016447,1.),(1.,0.857056062862677,
1.),(1.,0.862148985649771,1.)))
REPRESENTATION_ITEM('')
SURFACE()
);
#2387=(
BOUNDED_SURFACE()
B_SPLINE_SURFACE(3,2,((#150523,#150524,#150525),(#150526,#150527,#150528),
(#150529,#150530,#150531),(#150532,#150533,#150534),(#150535,#150536,#150537),
(#150538,#150539,#150540)),.UNSPECIFIED.,.F.,.F.,.F.)
B_SPLINE_SURFACE_WITH_KNOTS((4,2,4),(3,3),(-0.000152927716596379,0.00224843555189379,
0.00464973688355988),(0.,1.0001529277166),.UNSPECIFIED.)
GEOMETRIC_REPRESENTATION_ITEM()
RATIONAL_B_SPLINE_SURFACE(((1.,0.700973962712928,1.00009145873817),(1.,
0.732997839700047,1.0000816640614),(1.,0.76252859926943,1.00007263191814),
(1.,0.817862932084816,1.00005570761181),(1.,0.843804501741489,1.00004777324178),
(1.,0.866501623387319,1.00004083120381)))
REPRESENTATION_ITEM('')
SURFACE()
);
#2388=(
BOUNDED_SURFACE()
B_SPLINE_SURFACE(3,2,((#150584,#150585,#150586),(#150587,#150588,#150589),
(#150590,#150591,#150592),(#150593,#150594,#150595),(#150596,#150597,#150598),
(#150599,#150600,#150601),(#150602,#150603,#150604),(#150605,#150606,#150607)),
 .UNSPECIFIED.,.F.,.F.,.F.)
B_SPLINE_SURFACE_WITH_KNOTS((4,2,2,4),(3,3),(2.16840434497101E-19,0.00224905873968498,
0.00337358810952747,0.00449811747936996),(0.,1.),.UNSPECIFIED.)
GEOMETRIC_REPRESENTATION_ITEM()
RATIONAL_B_SPLINE_SURFACE(((1.,0.862148985649768,1.),(1.,0.840377424690098,
1.),(1.,0.816625499326475,1.),(1.,0.777693385283957,1.),(1.,0.764135973582955,
1.),(1.,0.736295007876384,1.),(1.,0.721949804627483,1.),(1.,0.707106781186548,
1.)))
REPRESENTATION_ITEM('')
SURFACE()
);
#2389=(
BOUNDED_SURFACE()
B_SPLINE_SURFACE(3,2,((#150620,#150621,#150622),(#150623,#150624,#150625),
(#150626,#150627,#150628),(#150629,#150630,#150631),(#150632,#150633,#150634),
(#150635,#150636,#150637)),.UNSPECIFIED.,.F.,.F.,.F.)
B_SPLINE_SURFACE_WITH_KNOTS((4,2,4),(3,3),(0.,0.0128929585057523,0.0257859170115046),
(0.,1.),.UNSPECIFIED.)
GEOMETRIC_REPRESENTATION_ITEM()
RATIONAL_B_SPLINE_SURFACE(((1.,0.862148985649771,1.),(1.,0.857001824466315,
1.),(1.,0.852340953158334,1.),(1.,0.843773924789864,1.),(1.,0.839868090827823,
1.),(1.,0.83625514626814,1.)))
REPRESENTATION_ITEM('')
SURFACE()
);
#2390=(
BOUNDED_SURFACE()
B_SPLINE_SURFACE(3,2,((#150646,#150647,#150648),(#150649,#150650,#150651),
(#150652,#150653,#150654),(#150655,#150656,#150657)),.UNSPECIFIED.,.F.,
 .F.,.F.)
B_SPLINE_SURFACE_WITH_KNOTS((4,4),(3,3),(-1.68213967061126E-16,0.000120540380538488),
(0.,1.),.UNSPECIFIED.)
GEOMETRIC_REPRESENTATION_ITEM()
RATIONAL_B_SPLINE_SURFACE(((1.,0.819851970694933,1.),(1.,0.826338730586804,
1.),(1.,0.831810971765196,1.),(1.,0.836255146268139,1.)))
REPRESENTATION_ITEM('')
SURFACE()
);
#2391=(
BOUNDED_SURFACE()
B_SPLINE_SURFACE(3,2,((#150659,#150660,#150661),(#150662,#150663,#150664),
(#150665,#150666,#150667),(#150668,#150669,#150670),(#150671,#150672,#150673),
(#150674,#150675,#150676),(#150677,#150678,#150679),(#150680,#150681,#150682),
(#150683,#150684,#150685),(#150686,#150687,#150688)),.UNSPECIFIED.,.F.,
 .F.,.F.)
B_SPLINE_SURFACE_WITH_KNOTS((4,2,2,2,4),(3,3),(4.71238898038469,5.10508806208341,
5.49778714378214,5.89048622548086,6.28318530717959),(0.,1.),
 .UNSPECIFIED.)
GEOMETRIC_REPRESENTATION_ITEM()
RATIONAL_B_SPLINE_SURFACE(((1.,0.707106781186552,1.),(1.,0.713550261851678,
1.),(1.,0.71989426486204,1.),(1.,0.731490756397489,1.),(1.,0.736738129296849,
1.),(1.,0.745429366938066,1.),(1.,0.748871927696599,1.),(1.,0.753512297096214,
1.),(1.,0.754714219730812,1.),(1.,0.754709580222777,1.)))
REPRESENTATION_ITEM('')
SURFACE()
);
#2392=(
BOUNDED_SURFACE()
B_SPLINE_SURFACE(3,2,((#150724,#150725,#150726),(#150727,#150728,#150729),
(#150730,#150731,#150732),(#150733,#150734,#150735),(#150736,#150737,#150738),
(#150739,#150740,#150741),(#150742,#150743,#150744),(#150745,#150746,#150747),
(#150748,#150749,#150750),(#150751,#150752,#150753)),.UNSPECIFIED.,.F.,
 .F.,.F.)
B_SPLINE_SURFACE_WITH_KNOTS((4,2,2,2,4),(3,3),(0.00108313181642978,0.00175636478508586,
0.00242959775374195,0.00310283072239804,0.00377606369105412),(0.,1.00020946001193),
 .UNSPECIFIED.)
GEOMETRIC_REPRESENTATION_ITEM()
RATIONAL_B_SPLINE_SURFACE(((1.,0.707045431769442,1.00012272453471),(1.,
0.774791710231453,1.00009434426212),(1.,0.828921293970199,1.00007166829561),
(1.,0.90377968768014,1.00004030861553),(1.,0.924101020320238,1.00003179560238),
(1.,0.924695389732398,1.00003154660913),(1.,0.904861584946617,1.0000398553871),
(1.,0.830176121522932,1.00007114262322),(1.,0.775998513536094,1.00009383870805),
(1.,0.707045431769442,1.00012272453471)))
REPRESENTATION_ITEM('')
SURFACE()
);
#2393=(
BOUNDED_SURFACE()
B_SPLINE_SURFACE(3,2,((#150784,#150785,#150786),(#150787,#150788,#150789),
(#150790,#150791,#150792),(#150793,#150794,#150795),(#150796,#150797,#150798),
(#150799,#150800,#150801),(#150802,#150803,#150804),(#150805,#150806,#150807),
(#150808,#150809,#150810),(#150811,#150812,#150813)),.UNSPECIFIED.,.F.,
 .F.,.F.)
B_SPLINE_SURFACE_WITH_KNOTS((4,2,2,2,4),(3,3),(-8.88178419700125E-16,0.392699081698724,
0.785398163397448,1.17809724509617,1.5707963267949),(0.,1.),
 .UNSPECIFIED.)
GEOMETRIC_REPRESENTATION_ITEM()
RATIONAL_B_SPLINE_SURFACE(((1.,0.656059028990513,1.),(1.,0.656051196071901,
1.),(1.,0.657443209221259,1.),(1.,0.662724068472642,1.),(1.,0.666616044204551,
1.),(1.,0.676209154063925,1.),(1.,0.681903435451265,1.),(1.,0.694134907060781,
1.),(1.,0.70066637883431,1.),(1.,0.707106781186548,1.)))
REPRESENTATION_ITEM('')
SURFACE()
);
#2394=(
BOUNDED_SURFACE()
B_SPLINE_SURFACE(3,2,((#150830,#150831,#150832),(#150833,#150834,#150835),
(#150836,#150837,#150838),(#150839,#150840,#150841),(#150842,#150843,#150844),
(#150845,#150846,#150847),(#150848,#150849,#150850),(#150851,#150852,#150853),
(#150854,#150855,#150856),(#150857,#150858,#150859)),.UNSPECIFIED.,.F.,
 .F.,.F.)
B_SPLINE_SURFACE_WITH_KNOTS((4,2,2,2,4),(3,3),(-6.16097884514888E-17,0.000175529658750937,
0.000351059317501936,0.000526588976252934,0.000702118635003933),(0.,1.),
 .UNSPECIFIED.)
GEOMETRIC_REPRESENTATION_ITEM()
RATIONAL_B_SPLINE_SURFACE(((1.,0.440584280700845,1.),(1.,0.458788905458512,
1.),(1.,0.480391768923104,1.),(1.,0.526541516020855,1.),(1.,0.550240391579637,
1.),(1.,0.597052366816548,1.),(1.,0.620407250394368,1.),(1.,0.664886737818671,
1.),(1.,0.686305427599538,1.),(1.,0.707106781186548,1.)))
REPRESENTATION_ITEM('')
SURFACE()
);
#2395=(
BOUNDED_SURFACE()
B_SPLINE_SURFACE(3,2,((#150872,#150873,#150874),(#150875,#150876,#150877),
(#150878,#150879,#150880),(#150881,#150882,#150883)),.UNSPECIFIED.,.F.,
 .F.,.F.)
B_SPLINE_SURFACE_WITH_KNOTS((4,4),(3,3),(0.,0.00414272899747597),(0.,1.),
 .UNSPECIFIED.)
GEOMETRIC_REPRESENTATION_ITEM()
RATIONAL_B_SPLINE_SURFACE(((1.,0.440584280700845,1.),(1.,0.437364321804866,
1.),(1.,0.434030421143282,1.),(1.,0.43057004911423,1.)))
REPRESENTATION_ITEM('')
SURFACE()
);
#2396=(
BOUNDED_SURFACE()
B_SPLINE_SURFACE(3,2,((#150890,#150891,#150892),(#150893,#150894,#150895),
(#150896,#150897,#150898),(#150899,#150900,#150901),(#150902,#150903,#150904),
(#150905,#150906,#150907),(#150908,#150909,#150910),(#150911,#150912,#150913),
(#150914,#150915,#150916),(#150917,#150918,#150919)),.UNSPECIFIED.,.F.,
 .F.,.F.)
B_SPLINE_SURFACE_WITH_KNOTS((4,2,2,2,4),(3,3),(-0.000629686196911106,0.00157421549227777,
0.00314843098455553,0.0047226464768333,0.00692654799509362),(0.,1.00122484286925),
 .UNSPECIFIED.)
GEOMETRIC_REPRESENTATION_ITEM()
RATIONAL_B_SPLINE_SURFACE(((1.,0.729910044545915,1.00066163551199),(1.,
0.703216914697168,1.00072702529149),(1.,0.675425262315014,1.00079510610598),
(1.,0.62493198685998,1.00091879876276),(1.,0.603050731781505,1.00097240096126),
(1.,0.557017477276785,1.00108516796832),(1.,0.532829811862376,1.00114442014733),
(1.,0.472843951657849,1.00129136665359),(1.,0.435970647158995,1.00138169466175),
(1.,0.396939037364919,1.00147730983961)))
REPRESENTATION_ITEM('')
SURFACE()
);
#2397=(
BOUNDED_SURFACE()
B_SPLINE_SURFACE(3,2,((#150975,#150976,#150977),(#150978,#150979,#150980),
(#150981,#150982,#150983),(#150984,#150985,#150986),(#150987,#150988,#150989),
(#150990,#150991,#150992),(#150993,#150994,#150995),(#150996,#150997,#150998),
(#150999,#151000,#151001),(#151002,#151003,#151004),(#151005,#151006,#151007),
(#151008,#151009,#151010)),.UNSPECIFIED.,.F.,.F.,.F.)
B_SPLINE_SURFACE_WITH_KNOTS((4,2,2,2,2,4),(3,3),(-0.000629845251684256,
0.00157461356268982,0.00236192034403473,0.00314922712537965,0.00472384068806947,
0.00692829967583523),(0.,1.00123997501886),.UNSPECIFIED.)
GEOMETRIC_REPRESENTATION_ITEM()
RATIONAL_B_SPLINE_SURFACE(((1.,0.396902198869997,1.00149565241467),(1.,
0.435987544303699,1.00139872271078),(1.,0.47283780294273,1.00130733591048),
(1.,0.520247360808013,1.00118976257566),(1.,0.532482074736246,1.0011594210964),
(1.,0.556521348730162,1.00109980489795),(1.,0.568360302311468,1.00107044488457),
(1.,0.602961724073934,1.00098463508736),(1.,0.624876074265694,1.00093028859378),
(1.,0.67542036326162,1.00080494128238),(1.,0.703218088558977,1.00073600431248),
(1.,0.72990104380667,1.0006698319166)))
REPRESENTATION_ITEM('')
SURFACE()
);
#2398=(
BOUNDED_SURFACE()
B_SPLINE_SURFACE(3,2,((#151062,#151063,#151064),(#151065,#151066,#151067),
(#151068,#151069,#151070),(#151071,#151072,#151073)),.UNSPECIFIED.,.F.,
 .F.,.F.)
B_SPLINE_SURFACE_WITH_KNOTS((4,4),(3,3),(-5.03069808033274E-17,0.00385726433182564),
(0.,1.),.UNSPECIFIED.)
GEOMETRIC_REPRESENTATION_ITEM()
RATIONAL_B_SPLINE_SURFACE(((1.,0.430570049114201,1.),(1.,0.433791974258431,
1.),(1.,0.436904245661489,1.),(1.,0.439917019807019,1.)))
REPRESENTATION_ITEM('')
SURFACE()
);
#2399=(
BOUNDED_SURFACE()
B_SPLINE_SURFACE(3,2,((#151080,#151081,#151082),(#151083,#151084,#151085),
(#151086,#151087,#151088),(#151089,#151090,#151091),(#151092,#151093,#151094),
(#151095,#151096,#151097),(#151098,#151099,#151100),(#151101,#151102,#151103)),
 .UNSPECIFIED.,.F.,.F.,.F.)
B_SPLINE_SURFACE_WITH_KNOTS((4,2,2,4),(3,3),(0.,0.000351812098911224,0.000527718148366836,
0.000703624197822447),(0.,1.),.UNSPECIFIED.)
GEOMETRIC_REPRESENTATION_ITEM()
RATIONAL_B_SPLINE_SURFACE(((1.,0.707106781186548,1.),(1.,0.666004685610564,
1.),(1.,0.620075381085077,1.),(1.,0.549819108711631,1.),(1.,0.525790037137517,
1.),(1.,0.479829608303299,1.),(1.,0.458216765529125,1.),(1.,0.439917019807004,
1.)))
REPRESENTATION_ITEM('')
SURFACE()
);
#2400=(
BOUNDED_SURFACE()
B_SPLINE_SURFACE(3,2,((#151131,#151132,#151133),(#151134,#151135,#151136),
(#151137,#151138,#151139),(#151140,#151141,#151142),(#151143,#151144,#151145),
(#151146,#151147,#151148)),.UNSPECIFIED.,.F.,.F.,.F.)
B_SPLINE_SURFACE_WITH_KNOTS((4,2,4),(3,3),(-6.47810798060089E-18,0.000325048915579083,
0.000650097831158172),(0.,1.),.UNSPECIFIED.)
GEOMETRIC_REPRESENTATION_ITEM()
RATIONAL_B_SPLINE_SURFACE(((1.,0.873361457045401,1.),(1.,0.85849847792363,
1.),(1.,0.834696857457215,1.),(1.,0.77714142509596,1.),(1.,0.743612803250452,
1.),(1.,0.707106781186552,1.)))
REPRESENTATION_ITEM('')
SURFACE()
);
#2401=(
BOUNDED_SURFACE()
B_SPLINE_SURFACE(3,2,((#151150,#151151,#151152),(#151153,#151154,#151155),
(#151156,#151157,#151158),(#151159,#151160,#151161)),.UNSPECIFIED.,.F.,
 .F.,.F.)
B_SPLINE_SURFACE_WITH_KNOTS((4,4),(3,3),(-6.93889390390723E-18,0.0135258923233721),
(0.,1.),.UNSPECIFIED.)
GEOMETRIC_REPRESENTATION_ITEM()
RATIONAL_B_SPLINE_SURFACE(((1.,0.873361457045398,1.),(1.,0.878048383336236,
1.),(1.,0.883106305929072,1.),(1.,0.888620714475961,1.)))
REPRESENTATION_ITEM('')
SURFACE()
);
#2402=(
BOUNDED_SURFACE()
B_SPLINE_SURFACE(3,2,((#151168,#151169,#151170),(#151171,#151172,#151173),
(#151174,#151175,#151176),(#151177,#151178,#151179),(#151180,#151181,#151182),
(#151183,#151184,#151185),(#151186,#151187,#151188),(#151189,#151190,#151191)),
 .UNSPECIFIED.,.F.,.F.,.F.)
B_SPLINE_SURFACE_WITH_KNOTS((4,2,2,4),(3,3),(-0.000151078666148884,0.00280275939636971,
0.00420413909455456,0.00575632475223853),(0.,1.00015107866615),
 .UNSPECIFIED.)
GEOMETRIC_REPRESENTATION_ITEM()
RATIONAL_B_SPLINE_SURFACE(((1.,0.701255881851812,1.00009026772578),(1.,
0.739278029586967,1.00007877905505),(1.,0.773783756716406,1.00006835289659),
(1.,0.82101132809148,1.00005408273962),(1.,0.835689666549691,1.00004964757202),
(1.,0.864812919803629,1.00004084776751),(1.,0.879165644906446,1.00003651098639),
(1.,0.892526157585967,1.00003247400952)))
REPRESENTATION_ITEM('')
SURFACE()
);
#2403=(
BOUNDED_SURFACE()
B_SPLINE_SURFACE(3,2,((#151241,#151242,#151243),(#151244,#151245,#151246),
(#151247,#151248,#151249),(#151250,#151251,#151252),(#151253,#151254,#151255),
(#151256,#151257,#151258),(#151259,#151260,#151261),(#151262,#151263,#151264)),
 .UNSPECIFIED.,.F.,.F.,.F.)
B_SPLINE_SURFACE_WITH_KNOTS((4,2,2,4),(3,3),(-9.4832710962814E-5,0.00140148291572316,
0.00280296583144632,0.00570103232705891),(0.,1.00009510066417),
 .UNSPECIFIED.)
GEOMETRIC_REPRESENTATION_ITEM()
RATIONAL_B_SPLINE_SURFACE(((1.,0.891085304843231,1.0000207157197),(1.,0.878122527114681,
1.00002318125724),(1.,0.864284413164116,1.00002581328489),(1.,0.835864397104656,
1.0000312188097),(1.,0.821386039943232,1.00003397261246),(1.,0.774524182759367,
1.00004288579995),(1.,0.740570301233833,1.00004934387332),(1.,0.703433195559746,
1.00005640740015)))
REPRESENTATION_ITEM('')
SURFACE()
);
#2404=(
BOUNDED_SURFACE()
B_SPLINE_SURFACE(3,2,((#151313,#151314,#151315),(#151316,#151317,#151318),
(#151319,#151320,#151321),(#151322,#151323,#151324)),.UNSPECIFIED.,.F.,
 .F.,.F.)
B_SPLINE_SURFACE_WITH_KNOTS((4,4),(3,3),(-6.93889390390723E-18,0.0138038180377133),
(0.,1.),.UNSPECIFIED.)
GEOMETRIC_REPRESENTATION_ITEM()
RATIONAL_B_SPLINE_SURFACE(((1.,0.888620714475959,1.),(1.,0.882992994712188,
1.),(1.,0.877840677983261,1.),(1.,0.873073026815702,1.)))
REPRESENTATION_ITEM('')
SURFACE()
);
#2405=(
BOUNDED_SURFACE()
B_SPLINE_SURFACE(3,2,((#151331,#151332,#151333),(#151334,#151335,#151336),
(#151337,#151338,#151339),(#151340,#151341,#151342),(#151343,#151344,#151345),
(#151346,#151347,#151348)),.UNSPECIFIED.,.F.,.F.,.F.)
B_SPLINE_SURFACE_WITH_KNOTS((4,2,4),(3,3),(0.,0.000324950456877623,0.000649900913755246),
(0.,1.),.UNSPECIFIED.)
GEOMETRIC_REPRESENTATION_ITEM()
RATIONAL_B_SPLINE_SURFACE(((1.,0.707106781186552,1.),(1.,0.743148709395921,
1.),(1.,0.777042261126144,1.),(1.,0.834175818048995,1.),(1.,0.858015095896893,
1.),(1.,0.873073026815704,1.)))
REPRESENTATION_ITEM('')
SURFACE()
);
#2406=(
BOUNDED_SURFACE()
B_SPLINE_SURFACE(3,2,((#151361,#151362,#151363),(#151364,#151365,#151366),
(#151367,#151368,#151369),(#151370,#151371,#151372),(#151373,#151374,#151375),
(#151376,#151377,#151378),(#151379,#151380,#151381),(#151382,#151383,#151384),
(#151385,#151386,#151387),(#151388,#151389,#151390)),.UNSPECIFIED.,.F.,
 .F.,.F.)
B_SPLINE_SURFACE_WITH_KNOTS((4,2,2,2,4),(3,3),(4.71238898038469,5.10508806208341,
5.49778714378214,5.89048622548086,6.28318530717959),(0.,1.),
 .UNSPECIFIED.)
GEOMETRIC_REPRESENTATION_ITEM()
RATIONAL_B_SPLINE_SURFACE(((1.,0.707106781186552,1.),(1.,0.713550261851565,
1.),(1.,0.719894264862192,1.),(1.,0.731490756397333,1.),(1.,0.736738129296254,
1.),(1.,0.745429366938654,1.),(1.,0.748871927696603,1.),(1.,0.753512297096217,
1.),(1.,0.754714219730812,1.),(1.,0.754709580222777,1.)))
REPRESENTATION_ITEM('')
SURFACE()
);
#2407=(
BOUNDED_SURFACE()
B_SPLINE_SURFACE(3,2,((#151448,#151449,#151450),(#151451,#151452,#151453),
(#151454,#151455,#151456),(#151457,#151458,#151459),(#151460,#151461,#151462),
(#151463,#151464,#151465),(#151466,#151467,#151468),(#151469,#151470,#151471),
(#151472,#151473,#151474),(#151475,#151476,#151477)),.UNSPECIFIED.,.F.,
 .F.,.F.)
B_SPLINE_SURFACE_WITH_KNOTS((4,2,2,2,4),(3,3),(-8.88178419700125E-16,0.392699081698724,
0.785398163397448,1.17809724509617,1.5707963267949),(0.,1.),
 .UNSPECIFIED.)
GEOMETRIC_REPRESENTATION_ITEM()
RATIONAL_B_SPLINE_SURFACE(((1.,0.656059028990507,1.),(1.,0.65605119607191,
1.),(1.,0.657443209221259,1.),(1.,0.662724068472642,1.),(1.,0.666616044204551,
1.),(1.,0.676209154063925,1.),(1.,0.681903435451068,1.),(1.,0.694134907060979,
1.),(1.,0.70066637883416,1.),(1.,0.707106781186548,1.)))
REPRESENTATION_ITEM('')
SURFACE()
);
#2408=(
BOUNDED_SURFACE()
B_SPLINE_SURFACE(3,2,((#151494,#151495,#151496),(#151497,#151498,#151499),
(#151500,#151501,#151502),(#151503,#151504,#151505),(#151506,#151507,#151508),
(#151509,#151510,#151511),(#151512,#151513,#151514),(#151515,#151516,#151517)),
 .UNSPECIFIED.,.F.,.F.,.F.)
B_SPLINE_SURFACE_WITH_KNOTS((4,2,2,4),(3,3),(-2.83789918648081E-17,0.000158415844625727,
0.000316831689251482,0.000633663378502992),(0.,1.),.UNSPECIFIED.)
GEOMETRIC_REPRESENTATION_ITEM()
RATIONAL_B_SPLINE_SURFACE(((1.,0.506999357883079,1.),(1.,0.518705031372287,
1.),(1.,0.533099046918872,1.),(1.,0.565407295868411,1.),(1.,0.582886848388227,
1.),(1.,0.636421215472814,1.),(1.,0.67314781771756,1.),(1.,0.707106781186543,
1.)))
REPRESENTATION_ITEM('')
SURFACE()
);
#2409=(
BOUNDED_SURFACE()
B_SPLINE_SURFACE(3,2,((#151528,#151529,#151530),(#151531,#151532,#151533),
(#151534,#151535,#151536),(#151537,#151538,#151539)),.UNSPECIFIED.,.F.,
 .F.,.F.)
B_SPLINE_SURFACE_WITH_KNOTS((4,4),(3,3),(6.93889390390723E-18,0.0177264565684137),
(0.,1.),.UNSPECIFIED.)
GEOMETRIC_REPRESENTATION_ITEM()
RATIONAL_B_SPLINE_SURFACE(((1.,0.506999357883079,1.),(1.,0.497142617029225,
1.),(1.,0.485892200859361,1.),(1.,0.472392340793768,1.)))
REPRESENTATION_ITEM('')
SURFACE()
);
#2410=(
BOUNDED_SURFACE()
B_SPLINE_SURFACE(3,2,((#151546,#151547,#151548),(#151549,#151550,#151551),
(#151552,#151553,#151554),(#151555,#151556,#151557),(#151558,#151559,#151560),
(#151561,#151562,#151563),(#151564,#151565,#151566),(#151567,#151568,#151569)),
 .UNSPECIFIED.,.F.,.F.,.F.)
B_SPLINE_SURFACE_WITH_KNOTS((4,2,2,4),(3,3),(0.,0.00263855694108943,0.00395783541163415,
0.00527711388217887),(0.,1.),.UNSPECIFIED.)
GEOMETRIC_REPRESENTATION_ITEM()
RATIONAL_B_SPLINE_SURFACE(((1.,0.707106781186999,1.),(1.,0.673000035720727,
1.),(1.,0.63702309328796,1.),(1.,0.578397249219397,1.),(1.,0.557964247865131,
1.),(1.,0.516081850109694,1.),(1.,0.494551837223282,1.),(1.,0.472392340793768,
1.)))
REPRESENTATION_ITEM('')
SURFACE()
);
#2411=(
BOUNDED_SURFACE()
B_SPLINE_SURFACE(3,2,((#151586,#151587,#151588),(#151589,#151590,#151591),
(#151592,#151593,#151594),(#151595,#151596,#151597),(#151598,#151599,#151600),
(#151601,#151602,#151603),(#151604,#151605,#151606),(#151607,#151608,#151609)),
 .UNSPECIFIED.,.F.,.F.,.F.)
B_SPLINE_SURFACE_WITH_KNOTS((4,2,2,4),(3,3),(-0.00052775387520704,0.0013193848583342,
0.00263876971666841,0.00580529337667048),(0.,1.00056372827132),
 .UNSPECIFIED.)
GEOMETRIC_REPRESENTATION_ITEM()
RATIONAL_B_SPLINE_SURFACE(((1.,0.445116797210528,1.00062560669739),(1.,
0.477005124809063,1.0005896539938),(1.,0.507425993631993,1.00055535578622),
(1.,0.557401754212246,1.00049901028798),(1.,0.577581621789236,1.00047625836425),
(1.,0.644406491906409,1.00040091622722),(1.,0.687357348800982,1.0003524910026),
(1.,0.727074127757439,1.00030771206032)))
REPRESENTATION_ITEM('')
SURFACE()
);
#2412=(
BOUNDED_SURFACE()
B_SPLINE_SURFACE(3,2,((#151654,#151655,#151656),(#151657,#151658,#151659),
(#151660,#151661,#151662),(#151663,#151664,#151665)),.UNSPECIFIED.,.F.,
 .F.,.F.)
B_SPLINE_SURFACE_WITH_KNOTS((4,4),(3,3),(0.,0.0174508326761739),(0.,1.),
 .UNSPECIFIED.)
GEOMETRIC_REPRESENTATION_ITEM()
RATIONAL_B_SPLINE_SURFACE(((1.,0.472392340793765,1.),(1.,0.485682667654673,
1.),(1.,0.49679147679375,1.),(1.,0.506538946041787,1.)))
REPRESENTATION_ITEM('')
SURFACE()
);
#2413=(
BOUNDED_SURFACE()
B_SPLINE_SURFACE(3,2,((#151677,#151678,#151679),(#151680,#151681,#151682),
(#151683,#151684,#151685),(#151686,#151687,#151688),(#151689,#151690,#151691),
(#151692,#151693,#151694)),.UNSPECIFIED.,.F.,.F.,.F.)
B_SPLINE_SURFACE_WITH_KNOTS((4,2,4),(3,3),(0.269041526988586,0.27511900362718,
0.281196480265774),(0.,1.),.UNSPECIFIED.)
GEOMETRIC_REPRESENTATION_ITEM()
RATIONAL_B_SPLINE_SURFACE(((1.,0.936757701036177,1.),(1.,0.939378149853558,
1.),(1.,0.942051042550488,1.),(1.,0.947449038066665,1.),(1.,0.950158897999453,
1.),(1.,0.952840299126697,1.)))
REPRESENTATION_ITEM('')
SURFACE()
);
#2414=(
BOUNDED_SURFACE()
B_SPLINE_SURFACE(3,2,((#151695,#151696,#151697),(#151698,#151699,#151700),
(#151701,#151702,#151703),(#151704,#151705,#151706),(#151707,#151708,#151709),
(#151710,#151711,#151712)),.UNSPECIFIED.,.F.,.F.,.F.)
B_SPLINE_SURFACE_WITH_KNOTS((4,2,4),(3,3),(0.0740543944727613,0.0811932403219739,
0.0883320861711864),(0.,1.),.UNSPECIFIED.)
GEOMETRIC_REPRESENTATION_ITEM()
RATIONAL_B_SPLINE_SURFACE(((1.,0.918849788108586,1.),(1.,0.921623427170992,
1.),(1.,0.924482745526459,1.),(1.,0.930368049939493,1.),(1.,0.933390296558584,
1.),(1.,0.936467000373499,1.)))
REPRESENTATION_ITEM('')
SURFACE()
);
#2415=(
BOUNDED_SURFACE()
B_SPLINE_SURFACE(3,2,((#151730,#151731,#151732),(#151733,#151734,#151735),
(#151736,#151737,#151738),(#151739,#151740,#151741),(#151742,#151743,#151744),
(#151745,#151746,#151747)),.UNSPECIFIED.,.F.,.F.,.F.)
B_SPLINE_SURFACE_WITH_KNOTS((4,2,4),(3,3),(4.71238898038469,5.49778714378214,
6.28318530717959),(0.,1.),.UNSPECIFIED.)
GEOMETRIC_REPRESENTATION_ITEM()
RATIONAL_B_SPLINE_SURFACE(((1.,0.707106781186552,1.),(1.,0.720039765645528,
1.),(1.,0.732392511163776,1.),(1.,0.749774985071127,1.),(1.,0.754782222113857,
1.),(1.,0.754709580222772,1.)))
REPRESENTATION_ITEM('')
SURFACE()
);
#2416=(
BOUNDED_SURFACE()
B_SPLINE_SURFACE(3,2,((#151752,#151753,#151754),(#151755,#151756,#151757),
(#151758,#151759,#151760),(#151761,#151762,#151763),(#151764,#151765,#151766),
(#151767,#151768,#151769)),.UNSPECIFIED.,.F.,.F.,.F.)
B_SPLINE_SURFACE_WITH_KNOTS((4,2,4),(3,3),(0.,0.785398163397448,1.5707963267949),
(0.,1.),.UNSPECIFIED.)
GEOMETRIC_REPRESENTATION_ITEM()
RATIONAL_B_SPLINE_SURFACE(((1.,0.656059028990507,1.),(1.,0.655948674699742,
1.),(1.,0.661819490286637,1.),(1.,0.681005707981833,1.),(1.,0.694211427469263,
1.),(1.,0.707106781186548,1.)))
REPRESENTATION_ITEM('')
SURFACE()
);
#2417=(
BOUNDED_SURFACE()
B_SPLINE_SURFACE(3,2,((#151772,#151773,#151774),(#151775,#151776,#151777),
(#151778,#151779,#151780),(#151781,#151782,#151783),(#151784,#151785,#151786),
(#151787,#151788,#151789)),.UNSPECIFIED.,.F.,.F.,.F.)
B_SPLINE_SURFACE_WITH_KNOTS((4,2,4),(3,3),(1.5707963267949,2.35619449019234,
3.1415926535898),(0.,1.),.UNSPECIFIED.)
GEOMETRIC_REPRESENTATION_ITEM()
RATIONAL_B_SPLINE_SURFACE(((1.,0.707106781186548,1.),(1.,0.72003976564552,
1.),(1.,0.732392511163791,1.),(1.,0.749774985071113,1.),(1.,0.75478222211386,
1.),(1.,0.754709580222772,1.)))
REPRESENTATION_ITEM('')
SURFACE()
);
#2418=(
BOUNDED_SURFACE()
B_SPLINE_SURFACE(3,2,((#151794,#151795,#151796),(#151797,#151798,#151799),
(#151800,#151801,#151802),(#151803,#151804,#151805),(#151806,#151807,#151808),
(#151809,#151810,#151811)),.UNSPECIFIED.,.F.,.F.,.F.)
B_SPLINE_SURFACE_WITH_KNOTS((4,2,4),(3,3),(0.,0.785398163397448,1.5707963267949),
(0.,1.),.UNSPECIFIED.)
GEOMETRIC_REPRESENTATION_ITEM()
RATIONAL_B_SPLINE_SURFACE(((1.,0.656059028990507,1.),(1.,0.655948674699894,
1.),(1.,0.661819490286433,1.),(1.,0.681005707982038,1.),(1.,0.694211427469109,
1.),(1.,0.707106781186548,1.)))
REPRESENTATION_ITEM('')
SURFACE()
);
#2419=(
BOUNDED_SURFACE()
B_SPLINE_SURFACE(3,2,((#151816,#151817,#151818),(#151819,#151820,#151821),
(#151822,#151823,#151824),(#151825,#151826,#151827),(#151828,#151829,#151830),
(#151831,#151832,#151833)),.UNSPECIFIED.,.F.,.F.,.F.)
B_SPLINE_SURFACE_WITH_KNOTS((4,2,4),(3,3),(-4.77048955893622E-18,0.00191432655883667,
0.00382865311767335),(0.,1.),.UNSPECIFIED.)
GEOMETRIC_REPRESENTATION_ITEM()
RATIONAL_B_SPLINE_SURFACE(((1.,0.903978945212085,1.),(1.,0.877037193452108,
1.),(1.,0.847703426978615,1.),(1.,0.782785838918396,1.),(1.,0.74722569047758,
1.),(1.,0.707106781186548,1.)))
REPRESENTATION_ITEM('')
SURFACE()
);
#2420=(
BOUNDED_SURFACE()
B_SPLINE_SURFACE(3,2,((#151842,#151843,#151844),(#151845,#151846,#151847),
(#151848,#151849,#151850),(#151851,#151852,#151853),(#151854,#151855,#151856),
(#151857,#151858,#151859)),.UNSPECIFIED.,.F.,.F.,.F.)
B_SPLINE_SURFACE_WITH_KNOTS((4,2,4),(3,3),(0.,0.000512893057734432,0.00102578611546886),
(0.,1.),.UNSPECIFIED.)
GEOMETRIC_REPRESENTATION_ITEM()
RATIONAL_B_SPLINE_SURFACE(((1.,0.813073674901549,1.),(1.,0.812982901655522,
1.),(1.,0.811992001632673,1.),(1.,0.803971289951385,1.),(1.,0.796694115012665,
1.),(1.,0.78334887142417,1.)))
REPRESENTATION_ITEM('')
SURFACE()
);
#2421=(
BOUNDED_SURFACE()
B_SPLINE_SURFACE(3,2,((#151861,#151862,#151863),(#151864,#151865,#151866),
(#151867,#151868,#151869),(#151870,#151871,#151872)),.UNSPECIFIED.,.F.,
 .F.,.F.)
B_SPLINE_SURFACE_WITH_KNOTS((4,4),(3,3),(0.,0.00123332093723591),(0.,1.),
 .UNSPECIFIED.)
GEOMETRIC_REPRESENTATION_ITEM()
RATIONAL_B_SPLINE_SURFACE(((1.,0.903978945212084,1.),(1.,0.925250261712233,
1.),(1.,0.940236171156205,1.),(1.,0.947923524237147,1.)))
REPRESENTATION_ITEM('')
SURFACE()
);
#2422=(
BOUNDED_SURFACE()
B_SPLINE_SURFACE(3,2,((#151877,#151878,#151879),(#151880,#151881,#151882),
(#151883,#151884,#151885),(#151886,#151887,#151888)),.UNSPECIFIED.,.F.,
 .F.,.F.)
B_SPLINE_SURFACE_WITH_KNOTS((4,4),(3,3),(-2.22874639202747E-5,0.000633198052120762),
(-2.22874639202404E-5,1.),.UNSPECIFIED.)
GEOMETRIC_REPRESENTATION_ITEM()
RATIONAL_B_SPLINE_SURFACE(((1.00000954900466,0.785776329440857,1.),(1.00001060519385,
0.762081637234299,1.),(1.0000118597036,0.733937794771298,1.),(1.00001319156803,
0.70405856681235,1.)))
REPRESENTATION_ITEM('')
SURFACE()
);
#2423=(
BOUNDED_SURFACE()
B_SPLINE_SURFACE(3,2,((#151893,#151894,#151895),(#151896,#151897,#151898),
(#151899,#151900,#151901),(#151902,#151903,#151904),(#151905,#151906,#151907),
(#151908,#151909,#151910),(#151911,#151912,#151913),(#151914,#151915,#151916),
(#151917,#151918,#151919),(#151920,#151921,#151922)),.UNSPECIFIED.,.F.,
 .F.,.F.)
B_SPLINE_SURFACE_WITH_KNOTS((4,2,2,2,4),(3,3),(0.,0.000408689684844658,
0.000817379369689317,0.00122606905453398,0.00163475873937863),(0.,1.),
 .UNSPECIFIED.)
GEOMETRIC_REPRESENTATION_ITEM()
RATIONAL_B_SPLINE_SURFACE(((1.,0.707106781186864,1.),(1.,0.688970136944317,
1.),(1.,0.670689426918774,1.),(1.,0.634705388858963,1.),(1.,0.617712576312848,
1.),(1.,0.58736619029857,1.),(1.,0.574575334017929,1.),(1.,0.556620432342278,
1.),(1.,0.551687087704826,1.),(1.,0.55167311003777,1.)))
REPRESENTATION_ITEM('')
SURFACE()
);
#2424=(
BOUNDED_SURFACE()
B_SPLINE_SURFACE(3,2,((#151925,#151926,#151927),(#151928,#151929,#151930),
(#151931,#151932,#151933),(#151934,#151935,#151936),(#151937,#151938,#151939),
(#151940,#151941,#151942),(#151943,#151944,#151945),(#151946,#151947,#151948),
(#151949,#151950,#151951),(#151952,#151953,#151954)),.UNSPECIFIED.,.F.,
 .F.,.F.)
B_SPLINE_SURFACE_WITH_KNOTS((4,2,2,2,4),(3,3),(-5.33083174934941E-5,0.000399098307138592,
0.000798196614277184,0.00119729492141578,0.00164970154604786),(-5.33083174934941E-5,
1.),.UNSPECIFIED.)
GEOMETRIC_REPRESENTATION_ITEM()
RATIONAL_B_SPLINE_SURFACE(((1.00002082472519,0.804676585507141,1.),(1.00002073272724,
0.805539470966454,1.),(1.00002101939354,0.802850713304667,1.),(1.00002216245292,
0.792129502840601,1.),(1.0000229532041,0.784712731694325,1.),(1.00002488425564,
0.766600628144248,1.),(1.00002604063762,0.755754459706965,1.),(1.00002868939129,
0.730910741180952,1.),(1.00003024414844,0.716328052911061,1.),(1.00003176891541,
0.702026654549035,1.)))
REPRESENTATION_ITEM('')
SURFACE()
);
#2425=(
BOUNDED_SURFACE()
B_SPLINE_SURFACE(3,2,((#151960,#151961,#151962),(#151963,#151964,#151965),
(#151966,#151967,#151968),(#151969,#151970,#151971)),.UNSPECIFIED.,.F.,
 .F.,.F.)
B_SPLINE_SURFACE_WITH_KNOTS((4,4),(3,3),(0.00330239163309442,0.00410592895993832),
(0.,1.),.UNSPECIFIED.)
GEOMETRIC_REPRESENTATION_ITEM()
RATIONAL_B_SPLINE_SURFACE(((1.,0.707106781186551,1.),(1.,0.682330721002586,
1.),(1.,0.657517255942454,1.),(1.,0.639433225268795,1.)))
REPRESENTATION_ITEM('')
SURFACE()
);
#2426=(
BOUNDED_SURFACE()
B_SPLINE_SURFACE(3,2,((#151977,#151978,#151979),(#151980,#151981,#151982),
(#151983,#151984,#151985),(#151986,#151987,#151988)),.UNSPECIFIED.,.F.,
 .F.,.F.)
B_SPLINE_SURFACE_WITH_KNOTS((4,4),(3,3),(-3.25260651745652E-19,0.0007884708222344),
(0.,1.),.UNSPECIFIED.)
GEOMETRIC_REPRESENTATION_ITEM()
RATIONAL_B_SPLINE_SURFACE(((1.,0.639433225268789,1.),(1.,0.625985289878347,
1.),(1.,0.614551947533885,1.),(1.,0.61107365918432,1.)))
REPRESENTATION_ITEM('')
SURFACE()
);
#2427=(
BOUNDED_SURFACE()
B_SPLINE_SURFACE(3,2,((#151991,#151992,#151993),(#151994,#151995,#151996),
(#151997,#151998,#151999),(#152000,#152001,#152002),(#152003,#152004,#152005),
(#152006,#152007,#152008)),.UNSPECIFIED.,.F.,.F.,.F.)
B_SPLINE_SURFACE_WITH_KNOTS((4,2,4),(3,3),(0.,0.000792989481313416,0.00158597896262684),
(0.,1.),.UNSPECIFIED.)
GEOMETRIC_REPRESENTATION_ITEM()
RATIONAL_B_SPLINE_SURFACE(((1.,0.760728353039959,1.),(1.,0.798498231399495,
1.),(1.,0.82089578223655,1.),(1.,0.844341385725833,1.),(1.,0.844813563409958,
1.),(1.,0.837989542743388,1.)))
REPRESENTATION_ITEM('')
SURFACE()
);
#2428=(
BOUNDED_SURFACE()
B_SPLINE_SURFACE(3,2,((#152010,#152011,#152012),(#152013,#152014,#152015),
(#152016,#152017,#152018),(#152019,#152020,#152021)),.UNSPECIFIED.,.F.,
 .F.,.F.)
B_SPLINE_SURFACE_WITH_KNOTS((4,4),(3,3),(0.,0.000504443591143906),(0.,1.),
 .UNSPECIFIED.)
GEOMETRIC_REPRESENTATION_ITEM()
RATIONAL_B_SPLINE_SURFACE(((1.,0.843854525156016,1.),(1.,0.841969285469978,
1.),(1.,0.840014967913779,1.),(1.,0.837989542743208,1.)))
REPRESENTATION_ITEM('')
SURFACE()
);
#2429=(
BOUNDED_SURFACE()
B_SPLINE_SURFACE(3,2,((#152024,#152025,#152026),(#152027,#152028,#152029),
(#152030,#152031,#152032),(#152033,#152034,#152035),(#152036,#152037,#152038),
(#152039,#152040,#152041),(#152042,#152043,#152044),(#152045,#152046,#152047),
(#152048,#152049,#152050),(#152051,#152052,#152053)),.UNSPECIFIED.,.F.,
 .F.,.F.)
B_SPLINE_SURFACE_WITH_KNOTS((4,2,2,2,4),(3,3),(-0.000180960259681038,0.00045240064920256,
0.00090480129840513,0.0013572019476077,0.0019905628564913),(-0.000555000723925246,
1.),.UNSPECIFIED.)
GEOMETRIC_REPRESENTATION_ITEM()
RATIONAL_B_SPLINE_SURFACE(((1.00017007065858,0.846783390316832,1.),(1.00017222379657,
0.844843628895718,1.),(1.00018057705553,0.837318180189595,1.),(1.00020429784683,
0.815948125808373,1.),(1.00021713987135,0.804378749442043,1.),(1.00024916216878,
0.775529870463418,1.),(1.00026828613008,0.758301098979412,1.),(1.00032368050176,
0.708396324719543,1.),(1.00036234037351,0.673567656857712,1.),(1.00041151994587,
0.629261793605653,1.)))
REPRESENTATION_ITEM('')
SURFACE()
);
#2430=(
BOUNDED_SURFACE()
B_SPLINE_SURFACE(3,2,((#152056,#152057,#152058),(#152059,#152060,#152061),
(#152062,#152063,#152064),(#152065,#152066,#152067),(#152068,#152069,#152070),
(#152071,#152072,#152073),(#152074,#152075,#152076),(#152077,#152078,#152079),
(#152080,#152081,#152082),(#152083,#152084,#152085),(#152086,#152087,#152088),
(#152089,#152090,#152091)),.UNSPECIFIED.,.F.,.F.,.F.)
B_SPLINE_SURFACE_WITH_KNOTS((4,2,2,2,2,4),(3,3),(0.,0.000464847896993965,
0.00092969579398793,0.00116211974248491,0.00139454369098189,0.00185939158797586),
(0.,1.),.UNSPECIFIED.)
GEOMETRIC_REPRESENTATION_ITEM()
RATIONAL_B_SPLINE_SURFACE(((1.,0.713890629234418,1.),(1.,0.74043984709427,
1.),(1.,0.764405928904485,1.),(1.,0.806784773788238,1.),(1.,0.825414433535011,
1.),(1.,0.847876574774264,1.),(1.,0.854606009430438,1.),(1.,0.866028143804753,
1.),(1.,0.87079122929337,1.),(1.,0.882487982894785,1.),(1.,0.886433234017275,
1.),(1.,0.886392435203049,1.)))
REPRESENTATION_ITEM('')
SURFACE()
);
#2431=(
BOUNDED_SURFACE()
B_SPLINE_SURFACE(3,2,((#152093,#152094,#152095),(#152096,#152097,#152098),
(#152099,#152100,#152101),(#152102,#152103,#152104)),.UNSPECIFIED.,.F.,
 .F.,.F.)
B_SPLINE_SURFACE_WITH_KNOTS((4,4),(3,3),(0.,0.000504070263719173),(0.,1.),
 .UNSPECIFIED.)
GEOMETRIC_REPRESENTATION_ITEM()
RATIONAL_B_SPLINE_SURFACE(((1.,0.886316114436169,1.),(1.,0.886398092028818,
1.),(1.,0.886423525277845,1.),(1.,0.886392435202391,1.)))
REPRESENTATION_ITEM('')
SURFACE()
);
#2432=(
BOUNDED_SURFACE()
B_SPLINE_SURFACE(3,2,((#152107,#152108,#152109),(#152110,#152111,#152112),
(#152113,#152114,#152115),(#152116,#152117,#152118),(#152119,#152120,#152121),
(#152122,#152123,#152124),(#152125,#152126,#152127),(#152128,#152129,#152130)),
 .UNSPECIFIED.,.F.,.F.,.F.)
B_SPLINE_SURFACE_WITH_KNOTS((4,2,2,4),(3,3),(-0.00017279642425018,0.000466811173310166,
0.000933622346620337,0.00204004111749139),(-0.000172796424253642,1.),
 .UNSPECIFIED.)
GEOMETRIC_REPRESENTATION_ITEM()
RATIONAL_B_SPLINE_SURFACE(((1.00003993733279,0.884438196676905,1.),(1.00003842620951,
0.888810750363417,1.),(1.00003959918162,0.885416663590792,1.),(1.00004581699226,
0.867424941052306,1.),(1.00004978263944,0.855950030055177,1.),(1.00006709382113,
0.805858768736276,1.),(1.0000858454205,0.751599545903121,1.),(1.0001089190889,
0.684834077514369,1.)))
REPRESENTATION_ITEM('')
SURFACE()
);
#2433=(
BOUNDED_SURFACE()
B_SPLINE_SURFACE(3,2,((#152133,#152134,#152135),(#152136,#152137,#152138),
(#152139,#152140,#152141),(#152142,#152143,#152144),(#152145,#152146,#152147),
(#152148,#152149,#152150),(#152151,#152152,#152153),(#152154,#152155,#152156)),
 .UNSPECIFIED.,.F.,.F.,.F.)
B_SPLINE_SURFACE_WITH_KNOTS((4,2,2,4),(3,3),(-0.00017992504535195,0.000899625226760169,
0.00134943784014025,0.00197917549887237),(-0.000964860374386562,1.),
 .UNSPECIFIED.)
GEOMETRIC_REPRESENTATION_ITEM()
RATIONAL_B_SPLINE_SURFACE(((1.00071732884499,0.628273238267874,1.),(1.00057400293934,
0.702546112070203,1.),(1.00047742991241,0.75259119087058,1.),(1.00038270957014,
0.801676190515576,1.),(1.00036092726382,0.812963992823138,1.),(1.00031924704205,
0.83456308781941,1.),(1.00030545716438,0.841709136113667,1.),(1.00029954974065,
0.844770420362849,1.)))
REPRESENTATION_ITEM('')
SURFACE()
);
#2434=(
BOUNDED_SURFACE()
B_SPLINE_SURFACE(3,2,((#152158,#152159,#152160),(#152161,#152162,#152163),
(#152164,#152165,#152166),(#152167,#152168,#152169)),.UNSPECIFIED.,.F.,
 .F.,.F.)
B_SPLINE_SURFACE_WITH_KNOTS((4,4),(3,3),(-2.16840434497101E-19,0.000504456607560921),
(0.,1.),.UNSPECIFIED.)
GEOMETRIC_REPRESENTATION_ITEM()
RATIONAL_B_SPLINE_SURFACE(((1.,0.835211735760659,1.),(1.,0.83730162444359,
1.),(1.,0.839319452171524,1.),(1.,0.841267344812682,1.)))
REPRESENTATION_ITEM('')
SURFACE()
);
#2435=(
BOUNDED_SURFACE()
B_SPLINE_SURFACE(3,2,((#152172,#152173,#152174),(#152175,#152176,#152177),
(#152178,#152179,#152180),(#152181,#152182,#152183),(#152184,#152185,#152186),
(#152187,#152188,#152189),(#152190,#152191,#152192),(#152193,#152194,#152195),
(#152196,#152197,#152198),(#152199,#152200,#152201)),.UNSPECIFIED.,.F.,
 .F.,.F.)
B_SPLINE_SURFACE_WITH_KNOTS((4,2,2,2,4),(3,3),(0.,0.00039540981677153,0.00079081963354306,
0.00118622945031459,0.00158163926708612),(0.,1.),.UNSPECIFIED.)
GEOMETRIC_REPRESENTATION_ITEM()
RATIONAL_B_SPLINE_SURFACE(((1.,0.835211735760644,1.),(1.,0.838806334780784,
1.),(1.,0.840513202341181,1.),(1.,0.839504260685003,1.),(1.,0.836771095032971,
1.),(1.,0.825966649242057,1.),(1.,0.817815337411177,1.),(1.,0.795024845130666,
1.),(1.,0.780342956064905,1.),(1.,0.761980581628842,1.)))
REPRESENTATION_ITEM('')
SURFACE()
);
#2436=(
BOUNDED_SURFACE()
B_SPLINE_SURFACE(3,2,((#152204,#152205,#152206),(#152207,#152208,#152209),
(#152210,#152211,#152212),(#152213,#152214,#152215)),.UNSPECIFIED.,.F.,
 .F.,.F.)
B_SPLINE_SURFACE_WITH_KNOTS((4,4),(3,3),(0.,0.000372129922795447),(0.,1.),
 .UNSPECIFIED.)
GEOMETRIC_REPRESENTATION_ITEM()
RATIONAL_B_SPLINE_SURFACE(((1.,0.609511474287707,1.),(1.,0.609908567799612,
1.),(1.,0.612427474748796,1.),(1.,0.616304832905386,1.)))
REPRESENTATION_ITEM('')
SURFACE()
);
#2437=(
BOUNDED_SURFACE()
B_SPLINE_SURFACE(3,2,((#152217,#152218,#152219),(#152220,#152221,#152222),
(#152223,#152224,#152225),(#152226,#152227,#152228),(#152229,#152230,#152231),
(#152232,#152233,#152234)),.UNSPECIFIED.,.F.,.F.,.F.)
B_SPLINE_SURFACE_WITH_KNOTS((4,2,4),(3,3),(0.0033044647217104,0.00391466500066162,
0.00452486527961284),(0.,1.),.UNSPECIFIED.)
GEOMETRIC_REPRESENTATION_ITEM()
RATIONAL_B_SPLINE_SURFACE(((1.,0.707106781186548,1.),(1.,0.688071275370979,
1.),(1.,0.668909963668733,1.),(1.,0.636714772442526,1.),(1.,0.623520947306417,
1.),(1.,0.61630483290538,1.)))
REPRESENTATION_ITEM('')
SURFACE()
);
#2438=(
BOUNDED_SURFACE()
B_SPLINE_SURFACE(3,2,((#152246,#152247,#152248),(#152249,#152250,#152251),
(#152252,#152253,#152254),(#152255,#152256,#152257),(#152258,#152259,#152260),
(#152261,#152262,#152263),(#152264,#152265,#152266),(#152267,#152268,#152269)),
 .UNSPECIFIED.,.F.,.F.,.F.)
B_SPLINE_SURFACE_WITH_KNOTS((4,2,2,4),(3,3),(-1.29128478743024E-16,0.000399353616616221,
0.00079870723323257,0.00159741446646527),(0.,1.),.UNSPECIFIED.)
GEOMETRIC_REPRESENTATION_ITEM()
RATIONAL_B_SPLINE_SURFACE(((1.,0.70710678118656,1.),(1.,0.719948338626786,
1.),(1.,0.732633692835949,1.),(1.,0.756391361283625,1.),(1.,0.767258343653063,
1.),(1.,0.794863148134095,1.),(1.,0.806163077037293,1.),(1.,0.806028661642745,
1.)))
REPRESENTATION_ITEM('')
SURFACE()
);
#2439=(
BOUNDED_SURFACE()
B_SPLINE_SURFACE(3,2,((#152272,#152273,#152274),(#152275,#152276,#152277),
(#152278,#152279,#152280),(#152281,#152282,#152283),(#152284,#152285,#152286),
(#152287,#152288,#152289),(#152290,#152291,#152292),(#152293,#152294,#152295),
(#152296,#152297,#152298),(#152299,#152300,#152301)),.UNSPECIFIED.,.F.,
 .F.,.F.)
B_SPLINE_SURFACE_WITH_KNOTS((4,2,2,2,4),(3,3),(0.,0.000409091700616903,
0.000818183401233805,0.00122727510185071,0.00163636680246761),(0.,1.),
 .UNSPECIFIED.)
GEOMETRIC_REPRESENTATION_ITEM()
RATIONAL_B_SPLINE_SURFACE(((1.,0.549942215762897,1.),(1.,0.54985788278214,
1.),(1.,0.554957454495403,1.),(1.,0.573078296428378,1.),(1.,0.58619337630722,
1.),(1.,0.61662144853447,1.),(1.,0.634085743304818,1.),(1.,0.670152902628418,
1.),(1.,0.688944445542904,1.),(1.,0.707106781186548,1.)))
REPRESENTATION_ITEM('')
SURFACE()
);
#2440=(
BOUNDED_SURFACE()
B_SPLINE_SURFACE(3,2,((#152306,#152307,#152308),(#152309,#152310,#152311),
(#152312,#152313,#152314),(#152315,#152316,#152317)),.UNSPECIFIED.,.F.,
 .F.,.F.)
B_SPLINE_SURFACE_WITH_KNOTS((4,4),(3,3),(0.,0.000344272120907045),(0.,1.),
 .UNSPECIFIED.)
GEOMETRIC_REPRESENTATION_ITEM()
RATIONAL_B_SPLINE_SURFACE(((1.,0.707106781186548,1.),(1.,0.722743638846974,
1.),(1.,0.737730816488031,1.),(1.,0.752153393551655,1.)))
REPRESENTATION_ITEM('')
SURFACE()
);
#2441=(
BOUNDED_SURFACE()
B_SPLINE_SURFACE(3,2,((#152319,#152320,#152321),(#152322,#152323,#152324),
(#152325,#152326,#152327),(#152328,#152329,#152330),(#152331,#152332,#152333),
(#152334,#152335,#152336)),.UNSPECIFIED.,.F.,.F.,.F.)
B_SPLINE_SURFACE_WITH_KNOTS((4,2,4),(3,3),(-1.54498809579185E-17,0.000643111039450966,
0.00128622207890195),(0.,1.),.UNSPECIFIED.)
GEOMETRIC_REPRESENTATION_ITEM()
RATIONAL_B_SPLINE_SURFACE(((1.,0.752153393551656,1.),(1.,0.774602351077688,
1.),(1.,0.786049290204429,1.),(1.,0.797170335299084,1.),(1.,0.797315472489739,
1.),(1.,0.797551754323297,1.)))
REPRESENTATION_ITEM('')
SURFACE()
);
#2442=(
BOUNDED_SURFACE()
B_SPLINE_SURFACE(3,2,((#152337,#152338,#152339),(#152340,#152341,#152342),
(#152343,#152344,#152345),(#152346,#152347,#152348)),.UNSPECIFIED.,.F.,
 .F.,.F.)
B_SPLINE_SURFACE_WITH_KNOTS((4,4),(3,3),(0.,0.00096907076046529),(0.,1.),
 .UNSPECIFIED.)
GEOMETRIC_REPRESENTATION_ITEM()
RATIONAL_B_SPLINE_SURFACE(((1.,0.903978945212084,1.),(1.,0.920702565586523,
1.),(1.,0.933513016958348,1.),(1.,0.941989694367876,1.)))
REPRESENTATION_ITEM('')
SURFACE()
);
#2443=(
BOUNDED_SURFACE()
B_SPLINE_SURFACE(3,2,((#152357,#152358,#152359),(#152360,#152361,#152362),
(#152363,#152364,#152365),(#152366,#152367,#152368),(#152369,#152370,#152371),
(#152372,#152373,#152374)),.UNSPECIFIED.,.F.,.F.,.F.)
B_SPLINE_SURFACE_WITH_KNOTS((4,2,4),(3,3),(4.71238898038469,5.49778714378214,
6.28318530717959),(0.,1.),.UNSPECIFIED.)
GEOMETRIC_REPRESENTATION_ITEM()
RATIONAL_B_SPLINE_SURFACE(((1.,0.707106781186552,1.),(1.,0.694211427469738,
1.),(1.,0.681005707981193,1.),(1.,0.661819490287278,1.),(1.,0.65594867469926,
1.),(1.,0.656059028990507,1.)))
REPRESENTATION_ITEM('')
SURFACE()
);
#2444=(
BOUNDED_SURFACE()
B_SPLINE_SURFACE(3,2,((#152379,#152380,#152381),(#152382,#152383,#152384),
(#152385,#152386,#152387),(#152388,#152389,#152390),(#152391,#152392,#152393),
(#152394,#152395,#152396)),.UNSPECIFIED.,.F.,.F.,.F.)
B_SPLINE_SURFACE_WITH_KNOTS((4,2,4),(3,3),(0.,0.785398163397448,1.5707963267949),
(0.,1.),.UNSPECIFIED.)
GEOMETRIC_REPRESENTATION_ITEM()
RATIONAL_B_SPLINE_SURFACE(((1.,0.754709580222772,1.),(1.,0.754782222114301,
1.),(1.,0.749774985070531,1.),(1.,0.732392511164381,1.),(1.,0.720039765645079,
1.),(1.,0.707106781186548,1.)))
REPRESENTATION_ITEM('')
SURFACE()
);
#2445=(
BOUNDED_SURFACE()
B_SPLINE_SURFACE(3,2,((#152399,#152400,#152401),(#152402,#152403,#152404),
(#152405,#152406,#152407),(#152408,#152409,#152410),(#152411,#152412,#152413),
(#152414,#152415,#152416)),.UNSPECIFIED.,.F.,.F.,.F.)
B_SPLINE_SURFACE_WITH_KNOTS((4,2,4),(3,3),(0.,0.00191432655883665,0.0038286531176733),
(0.,1.),.UNSPECIFIED.)
GEOMETRIC_REPRESENTATION_ITEM()
RATIONAL_B_SPLINE_SURFACE(((1.,0.707106781186548,1.),(1.,0.747225690478532,
1.),(1.,0.78278583891712,1.),(1.,0.847703426979888,1.),(1.,0.877037193451153,
1.),(1.,0.903978945212084,1.)))
REPRESENTATION_ITEM('')
SURFACE()
);
#2446=(
BOUNDED_SURFACE()
B_SPLINE_SURFACE(3,2,((#152427,#152428,#152429),(#152430,#152431,#152432),
(#152433,#152434,#152435),(#152436,#152437,#152438),(#152439,#152440,#152441),
(#152442,#152443,#152444)),.UNSPECIFIED.,.F.,.F.,.F.)
B_SPLINE_SURFACE_WITH_KNOTS((4,2,4),(3,3),(4.71238898038469,5.49778714378214,
6.28318530717959),(0.,1.),.UNSPECIFIED.)
GEOMETRIC_REPRESENTATION_ITEM()
RATIONAL_B_SPLINE_SURFACE(((1.,0.707106781186548,1.),(1.,0.694211427468419,
1.),(1.,0.68100570798296,1.),(1.,0.661819490285511,1.),(1.,0.655948674700594,
1.),(1.,0.656059028990501,1.)))
REPRESENTATION_ITEM('')
SURFACE()
);
#2447=(
BOUNDED_SURFACE()
B_SPLINE_SURFACE(3,2,((#152449,#152450,#152451),(#152452,#152453,#152454),
(#152455,#152456,#152457),(#152458,#152459,#152460),(#152461,#152462,#152463),
(#152464,#152465,#152466)),.UNSPECIFIED.,.F.,.F.,.F.)
B_SPLINE_SURFACE_WITH_KNOTS((4,2,4),(3,3),(3.1415926535898,3.92699081698724,
4.71238898038469),(0.,1.),.UNSPECIFIED.)
GEOMETRIC_REPRESENTATION_ITEM()
RATIONAL_B_SPLINE_SURFACE(((1.,0.754709580222777,1.),(1.,0.754782222115066,
1.),(1.,0.749774985069503,1.),(1.,0.732392511165393,1.),(1.,0.720039765644325,
1.),(1.,0.707106781186548,1.)))
REPRESENTATION_ITEM('')
SURFACE()
);
#2448=(
BOUNDED_SURFACE()
B_SPLINE_SURFACE(3,2,((#152474,#152475,#152476),(#152477,#152478,#152479),
(#152480,#152481,#152482),(#152483,#152484,#152485),(#152486,#152487,#152488),
(#152489,#152490,#152491)),.UNSPECIFIED.,.F.,.F.,.F.)
B_SPLINE_SURFACE_WITH_KNOTS((4,2,4),(3,3),(4.71238898038469,5.49778714378214,
6.28318530717959),(0.,1.),.UNSPECIFIED.)
GEOMETRIC_REPRESENTATION_ITEM()
RATIONAL_B_SPLINE_SURFACE(((1.,0.707106781186548,1.),(1.,0.720039765645103,
1.),(1.,0.732392511164345,1.),(1.,0.749774985070558,1.),(1.,0.754782222114279,
1.),(1.,0.754709580222763,1.)))
REPRESENTATION_ITEM('')
SURFACE()
);
#2449=(
BOUNDED_SURFACE()
B_SPLINE_SURFACE(3,2,((#152496,#152497,#152498),(#152499,#152500,#152501),
(#152502,#152503,#152504),(#152505,#152506,#152507),(#152508,#152509,#152510),
(#152511,#152512,#152513)),.UNSPECIFIED.,.F.,.F.,.F.)
B_SPLINE_SURFACE_WITH_KNOTS((4,2,4),(3,3),(8.78519494496442E-16,0.785398163397449,
1.5707963267949),(0.,1.),.UNSPECIFIED.)
GEOMETRIC_REPRESENTATION_ITEM()
RATIONAL_B_SPLINE_SURFACE(((1.,0.656059028990513,1.),(1.,0.655948674700453,
1.),(1.,0.661819490285707,1.),(1.,0.681005707982772,1.),(1.,0.694211427468564,
1.),(1.,0.707106781186548,1.)))
REPRESENTATION_ITEM('')
SURFACE()
);
#2450=(
BOUNDED_SURFACE()
B_SPLINE_SURFACE(3,2,((#152516,#152517,#152518),(#152519,#152520,#152521),
(#152522,#152523,#152524),(#152525,#152526,#152527),(#152528,#152529,#152530),
(#152531,#152532,#152533)),.UNSPECIFIED.,.F.,.F.,.F.)
B_SPLINE_SURFACE_WITH_KNOTS((4,2,4),(3,3),(1.5707963267949,2.35619449019234,
3.1415926535898),(0.,1.),.UNSPECIFIED.)
GEOMETRIC_REPRESENTATION_ITEM()
RATIONAL_B_SPLINE_SURFACE(((1.,0.707106781186548,1.),(1.,0.720039765645106,
1.),(1.,0.732392511164342,1.),(1.,0.749774985070554,1.),(1.,0.754782222114274,
1.),(1.,0.754709580222767,1.)))
REPRESENTATION_ITEM('')
SURFACE()
);
#2451=(
BOUNDED_SURFACE()
B_SPLINE_SURFACE(3,2,((#152538,#152539,#152540),(#152541,#152542,#152543),
(#152544,#152545,#152546),(#152547,#152548,#152549),(#152550,#152551,#152552),
(#152553,#152554,#152555)),.UNSPECIFIED.,.F.,.F.,.F.)
B_SPLINE_SURFACE_WITH_KNOTS((4,2,4),(3,3),(8.78519494496442E-16,0.785398163397449,
1.5707963267949),(0.,1.),.UNSPECIFIED.)
GEOMETRIC_REPRESENTATION_ITEM()
RATIONAL_B_SPLINE_SURFACE(((1.,0.656059028990513,1.),(1.,0.65594867470042,
1.),(1.,0.661819490285751,1.),(1.,0.681005707982728,1.),(1.,0.694211427468597,
1.),(1.,0.707106781186548,1.)))
REPRESENTATION_ITEM('')
SURFACE()
);
#2452=(
BOUNDED_SURFACE()
B_SPLINE_SURFACE(3,2,((#152560,#152561,#152562),(#152563,#152564,#152565),
(#152566,#152567,#152568),(#152569,#152570,#152571),(#152572,#152573,#152574),
(#152575,#152576,#152577),(#152578,#152579,#152580),(#152581,#152582,#152583)),
 .UNSPECIFIED.,.F.,.F.,.F.)
B_SPLINE_SURFACE_WITH_KNOTS((4,2,2,4),(3,3),(0.,0.00103600378053286,0.00207200756106572,
0.00414401512213144),(0.,1.),.UNSPECIFIED.)
GEOMETRIC_REPRESENTATION_ITEM()
RATIONAL_B_SPLINE_SURFACE(((1.,0.917068097704898,1.),(1.,0.902969174287913,
1.),(1.,0.888154932928049,1.),(1.,0.856959094818643,1.),(1.,0.840579087750432,
1.),(1.,0.788725570722382,1.),(1.,0.750598222445163,1.),(1.,0.707106781186548,
1.)))
REPRESENTATION_ITEM('')
SURFACE()
);
#2453=(
BOUNDED_SURFACE()
B_SPLINE_SURFACE(2,2,((#152592,#152593,#152594),(#152595,#152596,#152597),
(#152598,#152599,#152600)),.UNSPECIFIED.,.F.,.F.,.F.)
B_SPLINE_SURFACE_WITH_KNOTS((3,3),(3,3),(0.,1.5707963267949),(0.,1.5707963267949),
 .UNSPECIFIED.)
GEOMETRIC_REPRESENTATION_ITEM()
RATIONAL_B_SPLINE_SURFACE(((1.,0.707106781186547,1.),(0.707106781186621,
0.500000000000052,0.707106781186621),(1.,0.707106781186547,1.)))
REPRESENTATION_ITEM('')
SURFACE()
);
#2454=(
BOUNDED_SURFACE()
B_SPLINE_SURFACE(3,2,((#152601,#152602,#152603),(#152604,#152605,#152606),
(#152607,#152608,#152609),(#152610,#152611,#152612),(#152613,#152614,#152615),
(#152616,#152617,#152618)),.UNSPECIFIED.,.F.,.F.,.F.)
B_SPLINE_SURFACE_WITH_KNOTS((4,2,4),(3,3),(0.283188163394013,0.288276169473932,
0.293364175553851),(0.,1.),.UNSPECIFIED.)
GEOMETRIC_REPRESENTATION_ITEM()
RATIONAL_B_SPLINE_SURFACE(((1.,0.948000855586274,1.),(1.,0.950253931198463,
1.),(1.,0.952523267214703,1.),(1.,0.957028867337525,1.),(1.,0.959243070764605,
1.),(1.,0.961372018922465,1.)))
REPRESENTATION_ITEM('')
SURFACE()
);
#2455=(
BOUNDED_SURFACE()
B_SPLINE_SURFACE(3,2,((#152640,#152641,#152642),(#152643,#152644,#152645),
(#152646,#152647,#152648),(#152649,#152650,#152651),(#152652,#152653,#152654),
(#152655,#152656,#152657)),.UNSPECIFIED.,.F.,.F.,.F.)
B_SPLINE_SURFACE_WITH_KNOTS((4,2,4),(3,3),(0.0131888298509929,0.0172446796820237,
0.0213005295130545),(0.,1.),.UNSPECIFIED.)
GEOMETRIC_REPRESENTATION_ITEM()
RATIONAL_B_SPLINE_SURFACE(((1.,0.962986864789684,1.),(1.,0.964634105108703,
1.),(1.,0.96622351418111,1.),(1.,0.969200309542686,1.),(1.,0.970562566403692,
1.),(1.,0.971747603318281,1.)))
REPRESENTATION_ITEM('')
SURFACE()
);
#2456=(
BOUNDED_SURFACE()
B_SPLINE_SURFACE(3,2,((#152674,#152675,#152676),(#152677,#152678,#152679),
(#152680,#152681,#152682),(#152683,#152684,#152685),(#152686,#152687,#152688),
(#152689,#152690,#152691),(#152692,#152693,#152694),(#152695,#152696,#152697)),
 .UNSPECIFIED.,.F.,.F.,.F.)
B_SPLINE_SURFACE_WITH_KNOTS((4,2,2,4),(3,3),(0.0122567706991037,0.0155118977534076,
0.0171394612805594,0.0187670248077113),(0.,1.),.UNSPECIFIED.)
GEOMETRIC_REPRESENTATION_ITEM()
RATIONAL_B_SPLINE_SURFACE(((1.,0.976217638119343,1.),(1.,0.976078404720299,
1.),(1.,0.975752989031438,1.),(1.,0.975002468017128,1.),(1.,0.974707022042782,
1.),(1.,0.97404359369431,1.),(1.,0.973675473821347,1.),(1.,0.973275528580344,
1.)))
REPRESENTATION_ITEM('')
SURFACE()
);
#2457=(
BOUNDED_SURFACE()
B_SPLINE_SURFACE(3,2,((#152745,#152746,#152747),(#152748,#152749,#152750),
(#152751,#152752,#152753),(#152754,#152755,#152756),(#152757,#152758,#152759),
(#152760,#152761,#152762)),.UNSPECIFIED.,.F.,.F.,.F.)
B_SPLINE_SURFACE_WITH_KNOTS((4,2,4),(3,3),(0.320593732793275,0.325865292398914,
0.331136852004555),(0.,1.),.UNSPECIFIED.)
GEOMETRIC_REPRESENTATION_ITEM()
RATIONAL_B_SPLINE_SURFACE(((1.,0.944716550630948,1.),(1.,0.947183012056064,
1.),(1.,0.949681743560583,1.),(1.,0.954674153969892,1.),(1.,0.957142661330136,
1.),(1.,0.959530911256235,1.)))
REPRESENTATION_ITEM('')
SURFACE()
);
#2458=(
BOUNDED_SURFACE()
B_SPLINE_SURFACE(3,2,((#152798,#152799,#152800),(#152801,#152802,#152803),
(#152804,#152805,#152806),(#152807,#152808,#152809),(#152810,#152811,#152812),
(#152813,#152814,#152815)),.UNSPECIFIED.,.F.,.F.,.F.)
B_SPLINE_SURFACE_WITH_KNOTS((4,2,4),(3,3),(0.0161036610523817,0.0202680863362144,
0.0244325116200472),(0.,1.),.UNSPECIFIED.)
GEOMETRIC_REPRESENTATION_ITEM()
RATIONAL_B_SPLINE_SURFACE(((1.,0.961171400688072,1.),(1.,0.963011198169074,
1.),(1.,0.964799382389448,1.),(1.,0.968173271553358,1.),(1.,0.969728922082773,
1.),(1.,0.971089741366958,1.)))
REPRESENTATION_ITEM('')
SURFACE()
);
#2459=(
BOUNDED_SURFACE()
B_SPLINE_SURFACE(3,2,((#152833,#152834,#152835),(#152836,#152837,#152838),
(#152839,#152840,#152841),(#152842,#152843,#152844)),.UNSPECIFIED.,.F.,
 .F.,.F.)
B_SPLINE_SURFACE_WITH_KNOTS((4,4),(3,3),(0.0324061838408421,0.0330259723062236),
(0.0834883624373275,1.),.UNSPECIFIED.)
GEOMETRIC_REPRESENTATION_ITEM()
RATIONAL_B_SPLINE_SURFACE(((0.97106385378676,0.826705510992856,1.),(0.97062009002177,
0.824047872538613,1.),(0.970157734863912,0.821278892860728,1.),(0.969676371182953,
0.8183960738252,1.)))
REPRESENTATION_ITEM('')
SURFACE()
);
#2460=(
BOUNDED_SURFACE()
B_SPLINE_SURFACE(3,2,((#152854,#152855,#152856),(#152857,#152858,#152859),
(#152860,#152861,#152862),(#152863,#152864,#152865),(#152866,#152867,#152868),
(#152869,#152870,#152871),(#152872,#152873,#152874),(#152875,#152876,#152877)),
 .UNSPECIFIED.,.F.,.F.,.F.)
B_SPLINE_SURFACE_WITH_KNOTS((4,2,2,4),(3,3),(0.0238269657788709,0.0270983492768517,
0.0287340410258421,0.0303697327748325),(0.,1.),.UNSPECIFIED.)
GEOMETRIC_REPRESENTATION_ITEM()
RATIONAL_B_SPLINE_SURFACE(((1.,0.972768240458926,1.),(1.,0.973679370262107,
1.),(1.,0.974448100441956,1.),(1.,0.975326902749563,1.),(1.,0.975574944117527,
1.),(1.,0.975963474394985,1.),(1.,0.976104268047958,1.),(1.,0.976191081059459,
1.)))
REPRESENTATION_ITEM('')
SURFACE()
);
#2461=(
BOUNDED_SURFACE()
B_SPLINE_SURFACE(3,2,((#152904,#152905,#152906),(#152907,#152908,#152909),
(#152910,#152911,#152912),(#152913,#152914,#152915)),.UNSPECIFIED.,.F.,
 .F.,.F.)
B_SPLINE_SURFACE_WITH_KNOTS((4,4),(3,3),(0.0242632023351278,0.0247749981337221),
(0.078087948024069,1.),.UNSPECIFIED.)
GEOMETRIC_REPRESENTATION_ITEM()
RATIONAL_B_SPLINE_SURFACE(((0.980707816377885,0.876471439509661,1.),(0.980713728265565,
0.876509293543672,1.),(0.98070899383337,0.876478978800394,1.),(0.980693615408901,
0.876380510183544,1.)))
REPRESENTATION_ITEM('')
SURFACE()
);
#2462=(
BOUNDED_SURFACE()
B_SPLINE_SURFACE(3,2,((#152923,#152924,#152925),(#152926,#152927,#152928),
(#152929,#152930,#152931),(#152932,#152933,#152934),(#152935,#152936,#152937),
(#152938,#152939,#152940)),.UNSPECIFIED.,.F.,.F.,.F.)
B_SPLINE_SURFACE_WITH_KNOTS((4,2,4),(3,3),(0.0123698333451925,0.0156488944469233,
0.018927955548654),(0.,1.),.UNSPECIFIED.)
GEOMETRIC_REPRESENTATION_ITEM()
RATIONAL_B_SPLINE_SURFACE(((1.,0.976223664541016,1.),(1.,0.976080968954893,
1.),(1.,0.975725566325668,1.),(1.,0.974611093487067,1.),(1.,0.973867270455976,
1.),(1.,0.972985060473524,1.)))
REPRESENTATION_ITEM('')
SURFACE()
);
#2463=(
BOUNDED_SURFACE()
B_SPLINE_SURFACE(3,2,((#152961,#152962,#152963),(#152964,#152965,#152966),
(#152967,#152968,#152969),(#152970,#152971,#152972)),.UNSPECIFIED.,.F.,
 .F.,.F.)
B_SPLINE_SURFACE_WITH_KNOTS((4,4),(3,3),(0.0160154644119955,0.0166352988433916),
(0.0831643362494566,1.),.UNSPECIFIED.)
GEOMETRIC_REPRESENTATION_ITEM()
RATIONAL_B_SPLINE_SURFACE(((0.970304695662226,0.821466113499056,1.),(0.970770685596721,
0.824267734695772,1.),(0.971217880665933,0.826956357544095,1.),(0.971646673892332,
0.829534344970778,1.)))
REPRESENTATION_ITEM('')
SURFACE()
);
#2464=(
BOUNDED_SURFACE()
B_SPLINE_SURFACE(3,2,((#152982,#152983,#152984),(#152985,#152986,#152987),
(#152988,#152989,#152990),(#152991,#152992,#152993),(#152994,#152995,#152996),
(#152997,#152998,#152999),(#153000,#153001,#153002),(#153003,#153004,#153005)),
 .UNSPECIFIED.,.F.,.F.,.F.)
B_SPLINE_SURFACE_WITH_KNOTS((4,2,2,4),(3,3),(0.0125275809691397,0.0146002660392865,
0.0166729511094333,0.0208183212497269),(0.,1.),.UNSPECIFIED.)
GEOMETRIC_REPRESENTATION_ITEM()
RATIONAL_B_SPLINE_SURFACE(((1.,0.971326932216839,1.),(1.,0.970663335907126,
1.),(1.,0.969949535519179,1.),(1.,0.968438208203061,1.),(1.,0.967638304877362,
1.),(1.,0.965155032314022,1.),(1.,0.963392662012641,1.),(1.,0.961573369372794,
1.)))
REPRESENTATION_ITEM('')
SURFACE()
);
#2465=(
BOUNDED_SURFACE()
B_SPLINE_SURFACE(3,2,((#153041,#153042,#153043),(#153044,#153045,#153046),
(#153047,#153048,#153049),(#153050,#153051,#153052),(#153053,#153054,#153055),
(#153056,#153057,#153058)),.UNSPECIFIED.,.F.,.F.,.F.)
B_SPLINE_SURFACE_WITH_KNOTS((4,2,4),(3,3),(0.312823500866356,0.318064669632816,
0.323305838399276),(0.,1.),.UNSPECIFIED.)
GEOMETRIC_REPRESENTATION_ITEM()
RATIONAL_B_SPLINE_SURFACE(((1.,0.945205507217168,1.),(1.,0.947659322083022,
1.),(1.,0.950143491189858,1.),(1.,0.955101782056076,1.),(1.,0.957550650194803,
1.),(1.,0.959916004770377,1.)))
REPRESENTATION_ITEM('')
SURFACE()
);
#2466=(
BOUNDED_SURFACE()
B_SPLINE_SURFACE(3,2,((#153082,#153083,#153084),(#153085,#153086,#153087),
(#153088,#153089,#153090),(#153091,#153092,#153093)),.UNSPECIFIED.,.F.,
 .F.,.F.)
B_SPLINE_SURFACE_WITH_KNOTS((4,4),(3,3),(0.419404298305653,0.433181348372439),
(0.,1.),.UNSPECIFIED.)
GEOMETRIC_REPRESENTATION_ITEM()
RATIONAL_B_SPLINE_SURFACE(((1.,0.914650799019394,1.),(1.,0.919810342661608,
1.),(1.,0.925303402418372,1.),(1.,0.931052782541994,1.)))
REPRESENTATION_ITEM('')
SURFACE()
);
#2467=(
BOUNDED_SURFACE()
B_SPLINE_SURFACE(3,2,((#153113,#153114,#153115),(#153116,#153117,#153118),
(#153119,#153120,#153121),(#153122,#153123,#153124)),.UNSPECIFIED.,.F.,
 .F.,.F.)
B_SPLINE_SURFACE_WITH_KNOTS((4,4),(3,3),(0.419208811459411,0.43319545022518),
(0.,1.),.UNSPECIFIED.)
GEOMETRIC_REPRESENTATION_ITEM()
RATIONAL_B_SPLINE_SURFACE(((1.,0.914416798650558,1.),(1.,0.91964499776707,
1.),(1.,0.925217323809603,1.),(1.,0.931054338234342,1.)))
REPRESENTATION_ITEM('')
SURFACE()
);
#2468=(
BOUNDED_SURFACE()
B_SPLINE_SURFACE(3,2,((#153131,#153132,#153133),(#153134,#153135,#153136),
(#153137,#153138,#153139),(#153140,#153141,#153142)),.UNSPECIFIED.,.F.,
 .F.,.F.)
B_SPLINE_SURFACE_WITH_KNOTS((4,4),(3,3),(0.,0.000244695081784474),(0.27005445281224,
1.),.UNSPECIFIED.)
GEOMETRIC_REPRESENTATION_ITEM()
RATIONAL_B_SPLINE_SURFACE(((0.938257063314061,0.885684283219602,1.),(0.937405524229094,
0.884107676953533,1.),(0.936533776434415,0.882493654696909,1.),(0.935642351405452,
0.88084320046503,1.)))
REPRESENTATION_ITEM('')
SURFACE()
);
#2469=(
BOUNDED_SURFACE()
B_SPLINE_SURFACE(2,2,((#153148,#153149,#153150),(#153151,#153152,#153153),
(#153154,#153155,#153156)),.UNSPECIFIED.,.F.,.F.,.F.)
B_SPLINE_SURFACE_WITH_KNOTS((3,3),(3,3),(-1.5707963267949,2.46935726117696E-16),
(0.,1.5707963267949),.UNSPECIFIED.)
GEOMETRIC_REPRESENTATION_ITEM()
RATIONAL_B_SPLINE_SURFACE(((1.,0.707106781186548,1.),(0.707106781186554,
0.500000000000005,0.707106781186554),(1.,0.707106781186548,1.)))
REPRESENTATION_ITEM('')
SURFACE()
);
#2470=(
BOUNDED_SURFACE()
B_SPLINE_SURFACE(3,2,((#153162,#153163,#153164),(#153165,#153166,#153167),
(#153168,#153169,#153170),(#153171,#153172,#153173)),.UNSPECIFIED.,.F.,
 .F.,.F.)
B_SPLINE_SURFACE_WITH_KNOTS((4,4),(3,3),(0.38512996553569,0.397461118597566),
(0.,1.),.UNSPECIFIED.)
GEOMETRIC_REPRESENTATION_ITEM()
RATIONAL_B_SPLINE_SURFACE(((1.,0.93107684669709,1.),(1.,0.936225605355842,
1.),(1.,0.941660652469138,1.),(1.,0.947109873173451,1.)))
REPRESENTATION_ITEM('')
SURFACE()
);
#2471=(
BOUNDED_SURFACE()
B_SPLINE_SURFACE(3,2,((#153183,#153184,#153185),(#153186,#153187,#153188),
(#153189,#153190,#153191),(#153192,#153193,#153194)),.UNSPECIFIED.,.F.,
 .F.,.F.)
B_SPLINE_SURFACE_WITH_KNOTS((4,4),(3,3),(0.385104144430477,0.397435259869197),
(0.,1.),.UNSPECIFIED.)
GEOMETRIC_REPRESENTATION_ITEM()
RATIONAL_B_SPLINE_SURFACE(((1.,0.931076847239609,1.),(1.,0.936225547402437,
1.),(1.,0.941660619426866,1.),(1.,0.947109873449768,1.)))
REPRESENTATION_ITEM('')
SURFACE()
);
#2472=(
BOUNDED_SURFACE()
B_SPLINE_SURFACE(3,2,((#153213,#153214,#153215),(#153216,#153217,#153218),
(#153219,#153220,#153221),(#153222,#153223,#153224)),.UNSPECIFIED.,.F.,
 .F.,.F.)
B_SPLINE_SURFACE_WITH_KNOTS((4,4),(3,3),(0.404488952792596,0.419203847024178),
(0.,1.),.UNSPECIFIED.)
GEOMETRIC_REPRESENTATION_ITEM()
RATIONAL_B_SPLINE_SURFACE(((1.,0.909299925506085,1.),(1.,0.914893743921987,
1.),(1.,0.920902622704526,1.),(1.,0.927264329586823,1.)))
REPRESENTATION_ITEM('')
SURFACE()
);
#2473=(
BOUNDED_SURFACE()
B_SPLINE_SURFACE(3,2,((#153234,#153235,#153236),(#153237,#153238,#153239),
(#153240,#153241,#153242),(#153243,#153244,#153245)),.UNSPECIFIED.,.F.,
 .F.,.F.)
B_SPLINE_SURFACE_WITH_KNOTS((4,4),(3,3),(0.404502936988592,0.419217840791179),
(0.,1.),.UNSPECIFIED.)
GEOMETRIC_REPRESENTATION_ITEM()
RATIONAL_B_SPLINE_SURFACE(((1.,0.909299925389086,1.),(1.,0.914893755639716,
1.),(1.,0.920902631303307,1.),(1.,0.927264329485076,1.)))
REPRESENTATION_ITEM('')
SURFACE()
);
#2474=(
BOUNDED_SURFACE()
B_SPLINE_SURFACE(3,2,((#153266,#153267,#153268),(#153269,#153270,#153271),
(#153272,#153273,#153274),(#153275,#153276,#153277),(#153278,#153279,#153280),
(#153281,#153282,#153283)),.UNSPECIFIED.,.F.,.F.,.F.)
B_SPLINE_SURFACE_WITH_KNOTS((4,2,4),(3,3),(0.369267573830044,0.375649620241937,
0.382031666653828),(0.,1.),.UNSPECIFIED.)
GEOMETRIC_REPRESENTATION_ITEM()
RATIONAL_B_SPLINE_SURFACE(((1.,0.927093956641406,1.),(1.,0.929854789980195,
1.),(1.,0.932694024545401,1.),(1.,0.938495042437814,1.),(1.,0.941445780893249,
1.),(1.,0.944420998665188,1.)))
REPRESENTATION_ITEM('')
SURFACE()
);
#2475=(
BOUNDED_SURFACE()
B_SPLINE_SURFACE(3,2,((#153311,#153312,#153313),(#153314,#153315,#153316),
(#153317,#153318,#153319),(#153320,#153321,#153322),(#153323,#153324,#153325),
(#153326,#153327,#153328)),.UNSPECIFIED.,.F.,.F.,.F.)
B_SPLINE_SURFACE_WITH_KNOTS((4,2,4),(3,3),(0.369297600957186,0.375679664308256,
0.382061727659326),(0.,1.),.UNSPECIFIED.)
GEOMETRIC_REPRESENTATION_ITEM()
RATIONAL_B_SPLINE_SURFACE(((1.,0.927093956100417,1.),(1.,0.929854781017749,
1.),(1.,0.932694090912752,1.),(1.,0.938495064212398,1.),(1.,0.941445786720263,
1.),(1.,0.944420998446809,1.)))
REPRESENTATION_ITEM('')
SURFACE()
);
#2476=(
BOUNDED_SURFACE()
B_SPLINE_SURFACE(3,2,((#153335,#153336,#153337),(#153338,#153339,#153340),
(#153341,#153342,#153343),(#153344,#153345,#153346),(#153347,#153348,#153349),
(#153350,#153351,#153352)),.UNSPECIFIED.,.F.,.F.,.F.)
B_SPLINE_SURFACE_WITH_KNOTS((4,2,4),(3,3),(0.370125164623157,0.376536577097884,
0.382947989572612),(0.,1.),.UNSPECIFIED.)
GEOMETRIC_REPRESENTATION_ITEM()
RATIONAL_B_SPLINE_SURFACE(((1.,0.926591820711723,1.),(1.,0.929356779319319,
1.),(1.,0.932200966596534,1.),(1.,0.938014929520768,1.),(1.,0.94097390228205,
1.),(1.,0.943959859033813,1.)))
REPRESENTATION_ITEM('')
SURFACE()
);
#2477=(
BOUNDED_SURFACE()
B_SPLINE_SURFACE(3,2,((#153380,#153381,#153382),(#153383,#153384,#153385),
(#153386,#153387,#153388),(#153389,#153390,#153391),(#153392,#153393,#153394),
(#153395,#153396,#153397)),.UNSPECIFIED.,.F.,.F.,.F.)
B_SPLINE_SURFACE_WITH_KNOTS((4,2,4),(3,3),(0.370163239489449,0.376574672522443,
0.382986105555437),(0.,1.),.UNSPECIFIED.)
GEOMETRIC_REPRESENTATION_ITEM()
RATIONAL_B_SPLINE_SURFACE(((1.,0.926591820049981,1.),(1.,0.929356768176447,
1.),(1.,0.932201048041363,1.),(1.,0.938014956099503,1.),(1.,0.940973909290998,
1.),(1.,0.943959858771035,1.)))
REPRESENTATION_ITEM('')
SURFACE()
);
#2478=(
BOUNDED_SURFACE()
B_SPLINE_SURFACE(3,2,((#153423,#153424,#153425),(#153426,#153427,#153428),
(#153429,#153430,#153431),(#153432,#153433,#153434)),.UNSPECIFIED.,.F.,
 .F.,.F.)
B_SPLINE_SURFACE_WITH_KNOTS((4,4),(3,3),(0.405561464018681,0.420324995017399),
(0.,1.),.UNSPECIFIED.)
GEOMETRIC_REPRESENTATION_ITEM()
RATIONAL_B_SPLINE_SURFACE(((1.,0.908824629255916,1.),(1.,0.914415103092982,
1.),(1.,0.920421753472993,1.),(1.,0.926785562004255,1.)))
REPRESENTATION_ITEM('')
SURFACE()
);
#2479=(
BOUNDED_SURFACE()
B_SPLINE_SURFACE(3,2,((#153444,#153445,#153446),(#153447,#153448,#153449),
(#153450,#153451,#153452),(#153453,#153454,#153455)),.UNSPECIFIED.,.F.,
 .F.,.F.)
B_SPLINE_SURFACE_WITH_KNOTS((4,4),(3,3),(0.410308427502393,0.42507565892922),
(0.,1.),.UNSPECIFIED.)
GEOMETRIC_REPRESENTATION_ITEM()
RATIONAL_B_SPLINE_SURFACE(((1.,0.908824587192128,1.),(1.,0.914419456338754,
1.),(1.,0.920423871098494,1.),(1.,0.926785532009406,1.)))
REPRESENTATION_ITEM('')
SURFACE()
);
#2480=(
BOUNDED_SURFACE()
B_SPLINE_SURFACE(3,2,((#153537,#153538,#153539),(#153540,#153541,#153542),
(#153543,#153544,#153545),(#153546,#153547,#153548)),.UNSPECIFIED.,.F.,
 .F.,.F.)
B_SPLINE_SURFACE_WITH_KNOTS((4,4),(3,3),(0.410308427502393,0.42507565892922),
(0.,1.),.UNSPECIFIED.)
GEOMETRIC_REPRESENTATION_ITEM()
RATIONAL_B_SPLINE_SURFACE(((1.,0.908824587192128,1.),(1.,0.914419456338754,
1.),(1.,0.920423871098494,1.),(1.,0.926785532009406,1.)))
REPRESENTATION_ITEM('')
SURFACE()
);
#2481=(
BOUNDED_SURFACE()
B_SPLINE_SURFACE(3,2,((#153800,#153801,#153802),(#153803,#153804,#153805),
(#153806,#153807,#153808),(#153809,#153810,#153811)),.UNSPECIFIED.,.F.,
 .F.,.F.)
B_SPLINE_SURFACE_WITH_KNOTS((4,4),(3,3),(0.405561464018681,0.420324995017399),
(0.,1.),.UNSPECIFIED.)
GEOMETRIC_REPRESENTATION_ITEM()
RATIONAL_B_SPLINE_SURFACE(((1.,0.908824629255916,1.),(1.,0.914415103092982,
1.),(1.,0.920421753472993,1.),(1.,0.926785562004255,1.)))
REPRESENTATION_ITEM('')
SURFACE()
);
#2482=(
BOUNDED_SURFACE()
B_SPLINE_SURFACE(3,2,((#154434,#154435,#154436),(#154437,#154438,#154439),
(#154440,#154441,#154442),(#154443,#154444,#154445),(#154446,#154447,#154448),
(#154449,#154450,#154451)),.UNSPECIFIED.,.F.,.F.,.F.)
B_SPLINE_SURFACE_WITH_KNOTS((4,2,4),(3,3),(0.370163239489449,0.376574672522443,
0.382986105555437),(0.,1.),.UNSPECIFIED.)
GEOMETRIC_REPRESENTATION_ITEM()
RATIONAL_B_SPLINE_SURFACE(((1.,0.926591820049981,1.),(1.,0.929356768176447,
1.),(1.,0.932201048041363,1.),(1.,0.938014956099503,1.),(1.,0.940973909290998,
1.),(1.,0.943959858771035,1.)))
REPRESENTATION_ITEM('')
SURFACE()
);
#2483=(
BOUNDED_SURFACE()
B_SPLINE_SURFACE(3,2,((#154619,#154620,#154621),(#154622,#154623,#154624),
(#154625,#154626,#154627),(#154628,#154629,#154630),(#154631,#154632,#154633),
(#154634,#154635,#154636)),.UNSPECIFIED.,.F.,.F.,.F.)
B_SPLINE_SURFACE_WITH_KNOTS((4,2,4),(3,3),(0.370125164623157,0.376536577097884,
0.382947989572612),(0.,1.),.UNSPECIFIED.)
GEOMETRIC_REPRESENTATION_ITEM()
RATIONAL_B_SPLINE_SURFACE(((1.,0.926591820711723,1.),(1.,0.929356779319319,
1.),(1.,0.932200966596534,1.),(1.,0.938014929520768,1.),(1.,0.94097390228205,
1.),(1.,0.943959859033813,1.)))
REPRESENTATION_ITEM('')
SURFACE()
);
#2484=(
BOUNDED_SURFACE()
B_SPLINE_SURFACE(3,2,((#154835,#154836,#154837),(#154838,#154839,#154840),
(#154841,#154842,#154843),(#154844,#154845,#154846),(#154847,#154848,#154849),
(#154850,#154851,#154852)),.UNSPECIFIED.,.F.,.F.,.F.)
B_SPLINE_SURFACE_WITH_KNOTS((4,2,4),(3,3),(0.369297600957186,0.375679664308256,
0.382061727659326),(0.,1.),.UNSPECIFIED.)
GEOMETRIC_REPRESENTATION_ITEM()
RATIONAL_B_SPLINE_SURFACE(((1.,0.927093956100417,1.),(1.,0.929854781017749,
1.),(1.,0.932694090912752,1.),(1.,0.938495064212398,1.),(1.,0.941445786720263,
1.),(1.,0.944420998446809,1.)))
REPRESENTATION_ITEM('')
SURFACE()
);
#2485=(
BOUNDED_SURFACE()
B_SPLINE_SURFACE(3,2,((#154999,#155000,#155001),(#155002,#155003,#155004),
(#155005,#155006,#155007),(#155008,#155009,#155010),(#155011,#155012,#155013),
(#155014,#155015,#155016)),.UNSPECIFIED.,.F.,.F.,.F.)
B_SPLINE_SURFACE_WITH_KNOTS((4,2,4),(3,3),(0.369267573830044,0.375649620241937,
0.382031666653828),(0.,1.),.UNSPECIFIED.)
GEOMETRIC_REPRESENTATION_ITEM()
RATIONAL_B_SPLINE_SURFACE(((1.,0.927093956641406,1.),(1.,0.929854789980195,
1.),(1.,0.932694024545401,1.),(1.,0.938495042437814,1.),(1.,0.941445780893249,
1.),(1.,0.944420998665188,1.)))
REPRESENTATION_ITEM('')
SURFACE()
);
#2486=(
BOUNDED_SURFACE()
B_SPLINE_SURFACE(3,2,((#155557,#155558,#155559),(#155560,#155561,#155562),
(#155563,#155564,#155565),(#155566,#155567,#155568)),.UNSPECIFIED.,.F.,
 .F.,.F.)
B_SPLINE_SURFACE_WITH_KNOTS((4,4),(3,3),(0.404502936988592,0.419217840791179),
(0.,1.),.UNSPECIFIED.)
GEOMETRIC_REPRESENTATION_ITEM()
RATIONAL_B_SPLINE_SURFACE(((1.,0.909299925389086,1.),(1.,0.914893755639716,
1.),(1.,0.920902631303307,1.),(1.,0.927264329485076,1.)))
REPRESENTATION_ITEM('')
SURFACE()
);
#2487=(
BOUNDED_SURFACE()
B_SPLINE_SURFACE(3,2,((#155817,#155818,#155819),(#155820,#155821,#155822),
(#155823,#155824,#155825),(#155826,#155827,#155828)),.UNSPECIFIED.,.F.,
 .F.,.F.)
B_SPLINE_SURFACE_WITH_KNOTS((4,4),(3,3),(0.404488952792596,0.419203847024178),
(0.,1.00010378411472),.UNSPECIFIED.)
GEOMETRIC_REPRESENTATION_ITEM()
RATIONAL_B_SPLINE_SURFACE(((1.,0.909290512279149,1.00001882840776),(1.,
0.914884911244543,1.00001766718827),(1.,0.920894413653247,1.0000164198065),
(1.,0.927256780779661,1.00001509918122)))
REPRESENTATION_ITEM('')
SURFACE()
);
#2488=(
BOUNDED_SURFACE()
B_SPLINE_SURFACE(3,2,((#156265,#156266,#156267),(#156268,#156269,#156270),
(#156271,#156272,#156273),(#156274,#156275,#156276)),.UNSPECIFIED.,.F.,
 .F.,.F.)
B_SPLINE_SURFACE_WITH_KNOTS((4,4),(3,3),(0.385104144430477,0.397435259869197),
(0.,1.),.UNSPECIFIED.)
GEOMETRIC_REPRESENTATION_ITEM()
RATIONAL_B_SPLINE_SURFACE(((1.,0.931076847239609,1.),(1.,0.936225547402437,
1.),(1.,0.941660619426866,1.),(1.,0.947109873449768,1.)))
REPRESENTATION_ITEM('')
SURFACE()
);
#2489=(
BOUNDED_SURFACE()
B_SPLINE_SURFACE(3,2,((#156429,#156430,#156431),(#156432,#156433,#156434),
(#156435,#156436,#156437),(#156438,#156439,#156440)),.UNSPECIFIED.,.F.,
 .F.,.F.)
B_SPLINE_SURFACE_WITH_KNOTS((4,4),(3,3),(0.38512996553569,0.397461118597566),
(0.,1.),.UNSPECIFIED.)
GEOMETRIC_REPRESENTATION_ITEM()
RATIONAL_B_SPLINE_SURFACE(((1.,0.93107684669709,1.),(1.,0.936225605355842,
1.),(1.,0.941660652469138,1.),(1.,0.947109873173451,1.)))
REPRESENTATION_ITEM('')
SURFACE()
);
#2490=(
BOUNDED_SURFACE()
B_SPLINE_SURFACE(2,2,((#156689,#156690,#156691),(#156692,#156693,#156694),
(#156695,#156696,#156697)),.UNSPECIFIED.,.F.,.F.,.F.)
B_SPLINE_SURFACE_WITH_KNOTS((3,3),(3,3),(-1.5707963267949,2.46935726117696E-16),
(-1.5707963267949,0.),.UNSPECIFIED.)
GEOMETRIC_REPRESENTATION_ITEM()
RATIONAL_B_SPLINE_SURFACE(((1.,0.707106781186548,1.),(0.707106781186554,
0.500000000000005,0.707106781186554),(1.,0.707106781186548,1.)))
REPRESENTATION_ITEM('')
SURFACE()
);
#2491=(
BOUNDED_SURFACE()
B_SPLINE_SURFACE(3,2,((#156786,#156787,#156788),(#156789,#156790,#156791),
(#156792,#156793,#156794),(#156795,#156796,#156797)),.UNSPECIFIED.,.F.,
 .F.,.F.)
B_SPLINE_SURFACE_WITH_KNOTS((4,4),(3,3),(0.,0.000244695081784474),(0.,0.729945547187775),
 .UNSPECIFIED.)
GEOMETRIC_REPRESENTATION_ITEM()
RATIONAL_B_SPLINE_SURFACE(((1.,0.8856842832196,0.938257063314063),(1.,0.884107676953531,
0.937405524229096),(1.,0.882493654696906,0.936533776434417),(1.,0.880843200465028,
0.935642351405454)))
REPRESENTATION_ITEM('')
SURFACE()
);
#2492=(
BOUNDED_SURFACE()
B_SPLINE_SURFACE(3,2,((#156852,#156853,#156854),(#156855,#156856,#156857),
(#156858,#156859,#156860),(#156861,#156862,#156863)),.UNSPECIFIED.,.F.,
 .F.,.F.)
B_SPLINE_SURFACE_WITH_KNOTS((4,4),(3,3),(0.419208811459411,0.43319545022518),
(0.,1.),.UNSPECIFIED.)
GEOMETRIC_REPRESENTATION_ITEM()
RATIONAL_B_SPLINE_SURFACE(((1.,0.914416798650558,1.),(1.,0.91964499776707,
1.),(1.,0.925217323809603,1.),(1.,0.931054338234342,1.)))
REPRESENTATION_ITEM('')
SURFACE()
);
#2493=(
BOUNDED_SURFACE()
B_SPLINE_SURFACE(3,2,((#157146,#157147,#157148),(#157149,#157150,#157151),
(#157152,#157153,#157154),(#157155,#157156,#157157)),.UNSPECIFIED.,.F.,
 .F.,.F.)
B_SPLINE_SURFACE_WITH_KNOTS((4,4),(3,3),(0.419404298305653,0.433181348372439),
(0.,1.),.UNSPECIFIED.)
GEOMETRIC_REPRESENTATION_ITEM()
RATIONAL_B_SPLINE_SURFACE(((1.,0.914650799019394,1.),(1.,0.919810342661608,
1.),(1.,0.925303402418372,1.),(1.,0.931052782541994,1.)))
REPRESENTATION_ITEM('')
SURFACE()
);
#2494=(
BOUNDED_SURFACE()
B_SPLINE_SURFACE(3,2,((#157401,#157402,#157403),(#157404,#157405,#157406),
(#157407,#157408,#157409),(#157410,#157411,#157412),(#157413,#157414,#157415),
(#157416,#157417,#157418)),.UNSPECIFIED.,.F.,.F.,.F.)
B_SPLINE_SURFACE_WITH_KNOTS((4,2,4),(3,3),(0.312823500866356,0.318064669632816,
0.323305838399276),(-5.72660618870878E-8,1.),.UNSPECIFIED.)
GEOMETRIC_REPRESENTATION_ITEM()
RATIONAL_B_SPLINE_SURFACE(((1.00000000627573,0.945205504079303,1.),(1.00000000599469,
0.947659319085678,1.),(1.00000000571017,0.950143488334772,1.),(1.00000000514229,
0.955101779484932,1.),(1.00000000486181,0.957550647763896,1.),(1.00000000459091,
0.959916002474924,1.)))
REPRESENTATION_ITEM('')
SURFACE()
);
#2495=(
BOUNDED_SURFACE()
B_SPLINE_SURFACE(3,2,((#157744,#157745,#157746),(#157747,#157748,#157749),
(#157750,#157751,#157752),(#157753,#157754,#157755),(#157756,#157757,#157758),
(#157759,#157760,#157761),(#157762,#157763,#157764),(#157765,#157766,#157767)),
 .UNSPECIFIED.,.F.,.F.,.F.)
B_SPLINE_SURFACE_WITH_KNOTS((4,2,2,4),(3,3),(0.0125275809691397,0.0146002660392865,
0.0166729511094333,0.0208183212497269),(0.,1.),.UNSPECIFIED.)
GEOMETRIC_REPRESENTATION_ITEM()
RATIONAL_B_SPLINE_SURFACE(((1.,0.971326932216839,1.),(1.,0.970663335907126,
1.),(1.,0.969949535519179,1.),(1.,0.968438208203061,1.),(1.,0.967638304877362,
1.),(1.,0.965155032314022,1.),(1.,0.963392662012641,1.),(1.,0.961573369372794,
1.)))
REPRESENTATION_ITEM('')
SURFACE()
);
#2496=(
BOUNDED_SURFACE()
B_SPLINE_SURFACE(3,2,((#157998,#157999,#158000),(#158001,#158002,#158003),
(#158004,#158005,#158006),(#158007,#158008,#158009)),.UNSPECIFIED.,.F.,
 .F.,.F.)
B_SPLINE_SURFACE_WITH_KNOTS((4,4),(3,3),(0.0160154644119955,0.0166352988433916),
(0.,0.916835663750545),.UNSPECIFIED.)
GEOMETRIC_REPRESENTATION_ITEM()
RATIONAL_B_SPLINE_SURFACE(((1.,0.821466113499055,0.970304695662227),(1.,
0.824267734695769,0.970770685596721),(1.,0.826956357544096,0.971217880665933),
(1.,0.829534344970778,0.971646673892332)))
REPRESENTATION_ITEM('')
SURFACE()
);
#2497=(
BOUNDED_SURFACE()
B_SPLINE_SURFACE(3,2,((#158282,#158283,#158284),(#158285,#158286,#158287),
(#158288,#158289,#158290),(#158291,#158292,#158293),(#158294,#158295,#158296),
(#158297,#158298,#158299)),.UNSPECIFIED.,.F.,.F.,.F.)
B_SPLINE_SURFACE_WITH_KNOTS((4,2,4),(3,3),(0.0123698333451925,0.0156488944469233,
0.018927955548654),(0.,1.00002228978397),.UNSPECIFIED.)
GEOMETRIC_REPRESENTATION_ITEM()
RATIONAL_B_SPLINE_SURFACE(((1.,0.976223134571635,1.00000105996239),(1.,
0.976080435804858,1.00000106632384),(1.,0.975725025253786,1.00000108216789),
(1.,0.974610527573826,1.00000113185171),(1.,0.97386668796308,1.00000116501176),
(1.,0.972984458316358,1.00000120434118)))
REPRESENTATION_ITEM('')
SURFACE()
);
#2498=(
BOUNDED_SURFACE()
B_SPLINE_SURFACE(3,2,((#158421,#158422,#158423),(#158424,#158425,#158426),
(#158427,#158428,#158429),(#158430,#158431,#158432)),.UNSPECIFIED.,.F.,
 .F.,.F.)
B_SPLINE_SURFACE_WITH_KNOTS((4,4),(3,3),(0.0242632023351278,0.0247749981337221),
(0.,0.921912051975923),.UNSPECIFIED.)
GEOMETRIC_REPRESENTATION_ITEM()
RATIONAL_B_SPLINE_SURFACE(((1.,0.876471439509662,0.980707816377883),(1.,
0.876509293543674,0.980713728265564),(1.,0.876478978800395,0.980708993833368),
(1.,0.876380510183545,0.980693615408899)))
REPRESENTATION_ITEM('')
SURFACE()
);
#2499=(
BOUNDED_SURFACE()
B_SPLINE_SURFACE(3,2,((#158594,#158595,#158596),(#158597,#158598,#158599),
(#158600,#158601,#158602),(#158603,#158604,#158605),(#158606,#158607,#158608),
(#158609,#158610,#158611),(#158612,#158613,#158614),(#158615,#158616,#158617)),
 .UNSPECIFIED.,.F.,.F.,.F.)
B_SPLINE_SURFACE_WITH_KNOTS((4,2,2,4),(3,3),(0.0238269657788709,0.0270983492768517,
0.0287340410258421,0.0303697327748325),(0.,1.),.UNSPECIFIED.)
GEOMETRIC_REPRESENTATION_ITEM()
RATIONAL_B_SPLINE_SURFACE(((1.,0.972768240458926,1.),(1.,0.973679370262107,
1.),(1.,0.974448100441956,1.),(1.,0.975326902749563,1.),(1.,0.975574944117527,
1.),(1.,0.975963474394985,1.),(1.,0.976104268047958,1.),(1.,0.976191081059459,
1.)))
REPRESENTATION_ITEM('')
SURFACE()
);
#2500=(
BOUNDED_SURFACE()
B_SPLINE_SURFACE(3,2,((#158773,#158774,#158775),(#158776,#158777,#158778),
(#158779,#158780,#158781),(#158782,#158783,#158784)),.UNSPECIFIED.,.F.,
 .F.,.F.)
B_SPLINE_SURFACE_WITH_KNOTS((4,4),(3,3),(0.0324061838408421,0.0330259723062236),
(0.,0.916511637562676),.UNSPECIFIED.)
GEOMETRIC_REPRESENTATION_ITEM()
RATIONAL_B_SPLINE_SURFACE(((1.,0.826705510992856,0.971063853786761),(1.,
0.824047872538611,0.970620090021771),(1.,0.821278892860727,0.970157734863913),
(1.,0.818396073825199,0.969676371182954)))
REPRESENTATION_ITEM('')
SURFACE()
);
#2501=(
BOUNDED_SURFACE()
B_SPLINE_SURFACE(3,2,((#158996,#158997,#158998),(#158999,#159000,#159001),
(#159002,#159003,#159004),(#159005,#159006,#159007),(#159008,#159009,#159010),
(#159011,#159012,#159013)),.UNSPECIFIED.,.F.,.F.,.F.)
B_SPLINE_SURFACE_WITH_KNOTS((4,2,4),(3,3),(0.0161036610523817,0.0202680863362144,
0.0244325116200472),(0.,1.),.UNSPECIFIED.)
GEOMETRIC_REPRESENTATION_ITEM()
RATIONAL_B_SPLINE_SURFACE(((1.,0.961171400688072,1.),(1.,0.963011198169074,
1.),(1.,0.964799382389448,1.),(1.,0.968173271553358,1.),(1.,0.969728922082773,
1.),(1.,0.971089741366958,1.)))
REPRESENTATION_ITEM('')
SURFACE()
);
#2502=(
BOUNDED_SURFACE()
B_SPLINE_SURFACE(3,2,((#159339,#159340,#159341),(#159342,#159343,#159344),
(#159345,#159346,#159347),(#159348,#159349,#159350),(#159351,#159352,#159353),
(#159354,#159355,#159356)),.UNSPECIFIED.,.F.,.F.,.F.)
B_SPLINE_SURFACE_WITH_KNOTS((4,2,4),(3,3),(0.320593732793275,0.325865292398914,
0.331136852004555),(0.,1.),.UNSPECIFIED.)
GEOMETRIC_REPRESENTATION_ITEM()
RATIONAL_B_SPLINE_SURFACE(((1.,0.944716550630948,1.),(1.,0.947183012056064,
1.),(1.,0.949681743560583,1.),(1.,0.954674153969892,1.),(1.,0.957142661330136,
1.),(1.,0.959530911256235,1.)))
REPRESENTATION_ITEM('')
SURFACE()
);
#2503=(
BOUNDED_SURFACE()
B_SPLINE_SURFACE(3,2,((#159807,#159808,#159809),(#159810,#159811,#159812),
(#159813,#159814,#159815),(#159816,#159817,#159818),(#159819,#159820,#159821),
(#159822,#159823,#159824),(#159825,#159826,#159827),(#159828,#159829,#159830)),
 .UNSPECIFIED.,.F.,.F.,.F.)
B_SPLINE_SURFACE_WITH_KNOTS((4,2,2,4),(3,3),(0.0122567706991037,0.0155118977534076,
0.0171394612805594,0.0187670248077113),(0.,1.00001496733849),
 .UNSPECIFIED.)
GEOMETRIC_REPRESENTATION_ITEM()
RATIONAL_B_SPLINE_SURFACE(((1.,0.976217282160683,1.00000071192798),(1.,
0.976078046677685,1.00000071609595),(1.,0.975752626118217,1.0000007258373),
(1.,0.975002093870605,1.00000074830424),(1.,0.97470664347422,1.00000075714846),
(1.,0.974043205195991,1.00000077700827),(1.,0.973675079813253,1.00000078802798),
(1.,0.973275128586134,1.00000080000039)))
REPRESENTATION_ITEM('')
SURFACE()
);
#2504=(
BOUNDED_SURFACE()
B_SPLINE_SURFACE(3,2,((#159910,#159911,#159912),(#159913,#159914,#159915),
(#159916,#159917,#159918),(#159919,#159920,#159921),(#159922,#159923,#159924),
(#159925,#159926,#159927)),.UNSPECIFIED.,.F.,.F.,.F.)
B_SPLINE_SURFACE_WITH_KNOTS((4,2,4),(3,3),(0.0131888298509929,0.0172446796820237,
0.0213005295130545),(0.,1.),.UNSPECIFIED.)
GEOMETRIC_REPRESENTATION_ITEM()
RATIONAL_B_SPLINE_SURFACE(((1.,0.962986864789684,1.),(1.,0.964634105108703,
1.),(1.,0.96622351418111,1.),(1.,0.969200309542686,1.),(1.,0.970562566403692,
1.),(1.,0.971747603318281,1.)))
REPRESENTATION_ITEM('')
SURFACE()
);
#2505=(
BOUNDED_SURFACE()
B_SPLINE_SURFACE(3,2,((#160107,#160108,#160109),(#160110,#160111,#160112),
(#160113,#160114,#160115),(#160116,#160117,#160118),(#160119,#160120,#160121),
(#160122,#160123,#160124)),.UNSPECIFIED.,.F.,.F.,.F.)
B_SPLINE_SURFACE_WITH_KNOTS((4,2,4),(3,3),(0.283188163394013,0.288276169473932,
0.293364175553851),(0.,1.),.UNSPECIFIED.)
GEOMETRIC_REPRESENTATION_ITEM()
RATIONAL_B_SPLINE_SURFACE(((1.,0.948000855586274,1.),(1.,0.950253931198463,
1.),(1.,0.952523267214703,1.),(1.,0.957028867337525,1.),(1.,0.959243070764605,
1.),(1.,0.961372018922465,1.)))
REPRESENTATION_ITEM('')
SURFACE()
);
#2506=(
BOUNDED_SURFACE()
B_SPLINE_SURFACE(2,2,((#160355,#160356,#160357),(#160358,#160359,#160360),
(#160361,#160362,#160363)),.UNSPECIFIED.,.F.,.F.,.F.)
B_SPLINE_SURFACE_WITH_KNOTS((3,3),(3,3),(0.,1.5707963267949),(-1.5707963267949,
0.),.UNSPECIFIED.)
GEOMETRIC_REPRESENTATION_ITEM()
RATIONAL_B_SPLINE_SURFACE(((1.,0.707106781186547,1.),(0.707106781186621,
0.500000000000052,0.707106781186621),(1.,0.707106781186547,1.)))
REPRESENTATION_ITEM('')
SURFACE()
);
#2507=(
BOUNDED_SURFACE()
B_SPLINE_SURFACE(3,2,((#160372,#160373,#160374),(#160375,#160376,#160377),
(#160378,#160379,#160380),(#160381,#160382,#160383),(#160384,#160385,#160386),
(#160387,#160388,#160389),(#160390,#160391,#160392),(#160393,#160394,#160395)),
 .UNSPECIFIED.,.F.,.F.,.F.)
B_SPLINE_SURFACE_WITH_KNOTS((4,2,2,4),(3,3),(0.,0.00103600378053286,0.00207200756106572,
0.00414401512213144),(0.,1.),.UNSPECIFIED.)
GEOMETRIC_REPRESENTATION_ITEM()
RATIONAL_B_SPLINE_SURFACE(((1.,0.917068097704898,1.),(1.,0.902969174287913,
1.),(1.,0.888154932928049,1.),(1.,0.856959094818643,1.),(1.,0.840579087750432,
1.),(1.,0.788725570722382,1.),(1.,0.750598222445163,1.),(1.,0.707106781186548,
1.)))
REPRESENTATION_ITEM('')
SURFACE()
);
#2508=(
BOUNDED_SURFACE()
B_SPLINE_SURFACE(3,2,((#160489,#160490,#160491),(#160492,#160493,#160494),
(#160495,#160496,#160497),(#160498,#160499,#160500),(#160501,#160502,#160503),
(#160504,#160505,#160506)),.UNSPECIFIED.,.F.,.F.,.F.)
B_SPLINE_SURFACE_WITH_KNOTS((4,2,4),(3,3),(8.78519494496442E-16,0.785398163397449,
1.5707963267949),(0.,1.),.UNSPECIFIED.)
GEOMETRIC_REPRESENTATION_ITEM()
RATIONAL_B_SPLINE_SURFACE(((1.,0.656059028990513,1.),(1.,0.65594867470042,
1.),(1.,0.661819490285751,1.),(1.,0.681005707982728,1.),(1.,0.694211427468597,
1.),(1.,0.707106781186548,1.)))
REPRESENTATION_ITEM('')
SURFACE()
);
#2509=(
BOUNDED_SURFACE()
B_SPLINE_SURFACE(3,2,((#160578,#160579,#160580),(#160581,#160582,#160583),
(#160584,#160585,#160586),(#160587,#160588,#160589),(#160590,#160591,#160592),
(#160593,#160594,#160595)),.UNSPECIFIED.,.F.,.F.,.F.)
B_SPLINE_SURFACE_WITH_KNOTS((4,2,4),(3,3),(1.5707963267949,2.35619449019234,
3.1415926535898),(0.,1.),.UNSPECIFIED.)
GEOMETRIC_REPRESENTATION_ITEM()
RATIONAL_B_SPLINE_SURFACE(((1.,0.707106781186548,1.),(1.,0.720039765645106,
1.),(1.,0.732392511164342,1.),(1.,0.749774985070554,1.),(1.,0.754782222114274,
1.),(1.,0.754709580222767,1.)))
REPRESENTATION_ITEM('')
SURFACE()
);
#2510=(
BOUNDED_SURFACE()
B_SPLINE_SURFACE(3,2,((#160799,#160800,#160801),(#160802,#160803,#160804),
(#160805,#160806,#160807),(#160808,#160809,#160810),(#160811,#160812,#160813),
(#160814,#160815,#160816)),.UNSPECIFIED.,.F.,.F.,.F.)
B_SPLINE_SURFACE_WITH_KNOTS((4,2,4),(3,3),(8.78519494496442E-16,0.785398163397449,
1.5707963267949),(0.,1.),.UNSPECIFIED.)
GEOMETRIC_REPRESENTATION_ITEM()
RATIONAL_B_SPLINE_SURFACE(((1.,0.656059028990513,1.),(1.,0.655948674700453,
1.),(1.,0.661819490285707,1.),(1.,0.681005707982772,1.),(1.,0.694211427468564,
1.),(1.,0.707106781186548,1.)))
REPRESENTATION_ITEM('')
SURFACE()
);
#2511=(
BOUNDED_SURFACE()
B_SPLINE_SURFACE(3,2,((#160888,#160889,#160890),(#160891,#160892,#160893),
(#160894,#160895,#160896),(#160897,#160898,#160899),(#160900,#160901,#160902),
(#160903,#160904,#160905)),.UNSPECIFIED.,.F.,.F.,.F.)
B_SPLINE_SURFACE_WITH_KNOTS((4,2,4),(3,3),(4.71238898038469,5.49778714378214,
6.28318530717959),(0.,1.),.UNSPECIFIED.)
GEOMETRIC_REPRESENTATION_ITEM()
RATIONAL_B_SPLINE_SURFACE(((1.,0.707106781186548,1.),(1.,0.720039765645103,
1.),(1.,0.732392511164345,1.),(1.,0.749774985070558,1.),(1.,0.754782222114279,
1.),(1.,0.754709580222763,1.)))
REPRESENTATION_ITEM('')
SURFACE()
);
#2512=(
BOUNDED_SURFACE()
B_SPLINE_SURFACE(3,2,((#161058,#161059,#161060),(#161061,#161062,#161063),
(#161064,#161065,#161066),(#161067,#161068,#161069),(#161070,#161071,#161072),
(#161073,#161074,#161075)),.UNSPECIFIED.,.F.,.F.,.F.)
B_SPLINE_SURFACE_WITH_KNOTS((4,2,4),(3,3),(3.1415926535898,3.92699081698724,
4.71238898038469),(0.,1.),.UNSPECIFIED.)
GEOMETRIC_REPRESENTATION_ITEM()
RATIONAL_B_SPLINE_SURFACE(((1.,0.754709580222777,1.),(1.,0.754782222115066,
1.),(1.,0.749774985069503,1.),(1.,0.732392511165393,1.),(1.,0.720039765644325,
1.),(1.,0.707106781186548,1.)))
REPRESENTATION_ITEM('')
SURFACE()
);
#2513=(
BOUNDED_SURFACE()
B_SPLINE_SURFACE(3,2,((#161141,#161142,#161143),(#161144,#161145,#161146),
(#161147,#161148,#161149),(#161150,#161151,#161152),(#161153,#161154,#161155),
(#161156,#161157,#161158)),.UNSPECIFIED.,.F.,.F.,.F.)
B_SPLINE_SURFACE_WITH_KNOTS((4,2,4),(3,3),(4.71232237546293,5.49778714378214,
6.28325191210135),(-6.66049217571579E-5,1.),.UNSPECIFIED.)
GEOMETRIC_REPRESENTATION_ITEM()
RATIONAL_B_SPLINE_SURFACE(((1.00003901842147,0.707090554001954,1.),(1.0000407364626,
0.694193300415841,1.),(1.0000424959016,0.680985274981482,1.),(1.00004505208164,
0.661796152210739,1.),(1.00004583420842,0.655924763411915,1.),(1.00004581937076,
0.656036149035425,1.)))
REPRESENTATION_ITEM('')
SURFACE()
);
#2514=(
BOUNDED_SURFACE()
B_SPLINE_SURFACE(3,2,((#161302,#161303,#161304),(#161305,#161306,#161307),
(#161308,#161309,#161310),(#161311,#161312,#161313),(#161314,#161315,#161316),
(#161317,#161318,#161319)),.UNSPECIFIED.,.F.,.F.,.F.)
B_SPLINE_SURFACE_WITH_KNOTS((4,2,4),(3,3),(0.,0.00191432655883665,0.0038286531176733),
(0.,1.),.UNSPECIFIED.)
GEOMETRIC_REPRESENTATION_ITEM()
RATIONAL_B_SPLINE_SURFACE(((1.,0.707106781186548,1.),(1.,0.747225690478532,
1.),(1.,0.78278583891712,1.),(1.,0.847703426979888,1.),(1.,0.877037193451153,
1.),(1.,0.903978945212084,1.)))
REPRESENTATION_ITEM('')
SURFACE()
);
#2515=(
BOUNDED_SURFACE()
B_SPLINE_SURFACE(3,2,((#161410,#161411,#161412),(#161413,#161414,#161415),
(#161416,#161417,#161418),(#161419,#161420,#161421),(#161422,#161423,#161424),
(#161425,#161426,#161427)),.UNSPECIFIED.,.F.,.F.,.F.)
B_SPLINE_SURFACE_WITH_KNOTS((4,2,4),(3,3),(0.,0.785398163397448,1.5707963267949),
(0.,1.),.UNSPECIFIED.)
GEOMETRIC_REPRESENTATION_ITEM()
RATIONAL_B_SPLINE_SURFACE(((1.,0.754709580222772,1.),(1.,0.754782222114301,
1.),(1.,0.749774985070531,1.),(1.,0.732392511164381,1.),(1.,0.720039765645079,
1.),(1.,0.707106781186548,1.)))
REPRESENTATION_ITEM('')
SURFACE()
);
#2516=(
BOUNDED_SURFACE()
B_SPLINE_SURFACE(3,2,((#161493,#161494,#161495),(#161496,#161497,#161498),
(#161499,#161500,#161501),(#161502,#161503,#161504),(#161505,#161506,#161507),
(#161508,#161509,#161510)),.UNSPECIFIED.,.F.,.F.,.F.)
B_SPLINE_SURFACE_WITH_KNOTS((4,2,4),(3,3),(4.71232237546302,5.49778714378214,
6.28325191210126),(-6.6604921673139E-5,1.),.UNSPECIFIED.)
GEOMETRIC_REPRESENTATION_ITEM()
RATIONAL_B_SPLINE_SURFACE(((1.00003901842142,0.707090554001977,0.999999999999999),
(1.00004073646254,0.694193300417183,1.),(1.00004249590154,0.68098527497974,
1.),(1.00004505208158,0.661796152212536,1.),(1.00004583420837,0.65592476341061,
1.),(1.0000458193707,0.65603614903546,1.)))
REPRESENTATION_ITEM('')
SURFACE()
);
#2517=(
BOUNDED_SURFACE()
B_SPLINE_SURFACE(3,2,((#161723,#161724,#161725),(#161726,#161727,#161728),
(#161729,#161730,#161731),(#161732,#161733,#161734)),.UNSPECIFIED.,.F.,
 .F.,.F.)
B_SPLINE_SURFACE_WITH_KNOTS((4,4),(3,3),(0.,0.00096907076046529),(0.,1.),
 .UNSPECIFIED.)
GEOMETRIC_REPRESENTATION_ITEM()
RATIONAL_B_SPLINE_SURFACE(((1.,0.903978945212084,1.),(1.,0.920702565586523,
1.),(1.,0.933513016958348,1.),(1.,0.941989694367876,1.)))
REPRESENTATION_ITEM('')
SURFACE()
);
#2518=(
BOUNDED_SURFACE()
B_SPLINE_SURFACE(3,2,((#161807,#161808,#161809),(#161810,#161811,#161812),
(#161813,#161814,#161815),(#161816,#161817,#161818),(#161819,#161820,#161821),
(#161822,#161823,#161824)),.UNSPECIFIED.,.F.,.F.,.F.)
B_SPLINE_SURFACE_WITH_KNOTS((4,2,4),(3,3),(-0.000128622207890212,0.000643111039450966,
0.00141484428679216),(-0.00251732068448168,1.),.UNSPECIFIED.)
GEOMETRIC_REPRESENTATION_ITEM()
RATIONAL_B_SPLINE_SURFACE(((1.00132581435537,0.736661609395596,1.),(1.00116195192182,
0.769208601633366,1.),(1.0010854898064,0.784395803624051,1.),(1.00101813210278,
0.797774652021856,1.),(1.00102381299662,0.796646290850486,1.),(1.00102082699956,
0.797239381168936,1.)))
REPRESENTATION_ITEM('')
SURFACE()
);
#2519=(
BOUNDED_SURFACE()
B_SPLINE_SURFACE(3,2,((#161873,#161874,#161875),(#161876,#161877,#161878),
(#161879,#161880,#161881),(#161882,#161883,#161884)),.UNSPECIFIED.,.F.,
 .F.,.F.)
B_SPLINE_SURFACE_WITH_KNOTS((4,4),(3,3),(0.,0.000344272120907045),(0.,1.),
 .UNSPECIFIED.)
GEOMETRIC_REPRESENTATION_ITEM()
RATIONAL_B_SPLINE_SURFACE(((1.,0.707106781186548,1.),(1.,0.722743638846974,
1.),(1.,0.737730816488031,1.),(1.,0.752153393551655,1.)))
REPRESENTATION_ITEM('')
SURFACE()
);
#2520=(
BOUNDED_SURFACE()
B_SPLINE_SURFACE(3,2,((#161893,#161894,#161895),(#161896,#161897,#161898),
(#161899,#161900,#161901),(#161902,#161903,#161904),(#161905,#161906,#161907),
(#161908,#161909,#161910),(#161911,#161912,#161913),(#161914,#161915,#161916),
(#161917,#161918,#161919),(#161920,#161921,#161922)),.UNSPECIFIED.,.F.,
 .F.,.F.)
B_SPLINE_SURFACE_WITH_KNOTS((4,2,2,2,4),(3,3),(0.,0.000409091700616903,
0.000818183401233805,0.00122727510185071,0.00163636680246761),(0.,1.),
 .UNSPECIFIED.)
GEOMETRIC_REPRESENTATION_ITEM()
RATIONAL_B_SPLINE_SURFACE(((1.,0.549942215762897,1.),(1.,0.54985788278214,
1.),(1.,0.554957454495403,1.),(1.,0.573078296428378,1.),(1.,0.58619337630722,
1.),(1.,0.61662144853447,1.),(1.,0.634085743304818,1.),(1.,0.670152902628418,
1.),(1.,0.688944445542904,1.),(1.,0.707106781186548,1.)))
REPRESENTATION_ITEM('')
SURFACE()
);
#2521=(
BOUNDED_SURFACE()
B_SPLINE_SURFACE(3,2,((#162039,#162040,#162041),(#162042,#162043,#162044),
(#162045,#162046,#162047),(#162048,#162049,#162050),(#162051,#162052,#162053),
(#162054,#162055,#162056),(#162057,#162058,#162059),(#162060,#162061,#162062)),
 .UNSPECIFIED.,.F.,.F.,.F.)
B_SPLINE_SURFACE_WITH_KNOTS((4,2,2,4),(3,3),(-0.000109471601813517,0.000399353616616221,
0.00079870723323257,0.00170688606827854),(-0.000609991948385842,1.),
 .UNSPECIFIED.)
GEOMETRIC_REPRESENTATION_ITEM()
RATIONAL_B_SPLINE_SURFACE(((1.00037046105782,0.696339387097673,1.),(1.00035043066668,
0.712757957212574,1.),(1.00033035655321,0.729212365766033,1.),(1.00029737990511,
0.756242761975451,1.),(1.00028411427462,0.767116373116637,1.),(1.00024733719763,
0.797261916093909,1.),(1.00023300379127,0.809010764906677,1.),(1.00023765398644,
0.805199079207076,1.)))
REPRESENTATION_ITEM('')
SURFACE()
);
#2522=(
BOUNDED_SURFACE()
B_SPLINE_SURFACE(3,2,((#162155,#162156,#162157),(#162158,#162159,#162160),
(#162161,#162162,#162163),(#162164,#162165,#162166),(#162167,#162168,#162169),
(#162170,#162171,#162172)),.UNSPECIFIED.,.F.,.F.,.F.)
B_SPLINE_SURFACE_WITH_KNOTS((4,2,4),(3,3),(0.0033044647217104,0.00391466500066162,
0.00452486527961284),(0.,1.),.UNSPECIFIED.)
GEOMETRIC_REPRESENTATION_ITEM()
RATIONAL_B_SPLINE_SURFACE(((1.,0.707106781186548,1.),(1.,0.688071275370979,
1.),(1.,0.668909963668733,1.),(1.,0.636714772442526,1.),(1.,0.623520947306417,
1.),(1.,0.61630483290538,1.)))
REPRESENTATION_ITEM('')
SURFACE()
);
#2523=(
BOUNDED_SURFACE()
B_SPLINE_SURFACE(3,2,((#162206,#162207,#162208),(#162209,#162210,#162211),
(#162212,#162213,#162214),(#162215,#162216,#162217)),.UNSPECIFIED.,.F.,
 .F.,.F.)
B_SPLINE_SURFACE_WITH_KNOTS((4,4),(3,3),(-3.72129922795447E-5,0.000409342915074972),
(0.,1.00007018282617),.UNSPECIFIED.)
GEOMETRIC_REPRESENTATION_ITEM()
RATIONAL_B_SPLINE_SURFACE(((1.,0.609429354571442,1.00005482270343),(1.,
0.60938746827453,1.00005482858282),(1.,0.612511139640593,1.00005439012666),
(1.,0.617481186158951,1.00005369250283)))
REPRESENTATION_ITEM('')
SURFACE()
);
#2524=(
BOUNDED_SURFACE()
B_SPLINE_SURFACE(3,2,((#162238,#162239,#162240),(#162241,#162242,#162243),
(#162244,#162245,#162246),(#162247,#162248,#162249),(#162250,#162251,#162252),
(#162253,#162254,#162255),(#162256,#162257,#162258),(#162259,#162260,#162261),
(#162262,#162263,#162264),(#162265,#162266,#162267)),.UNSPECIFIED.,.F.,
 .F.,.F.)
B_SPLINE_SURFACE_WITH_KNOTS((4,2,2,2,4),(3,3),(0.,0.00039540981677153,0.00079081963354306,
0.00118622945031459,0.00158163926708612),(0.,1.),.UNSPECIFIED.)
GEOMETRIC_REPRESENTATION_ITEM()
RATIONAL_B_SPLINE_SURFACE(((1.,0.835211735760644,1.),(1.,0.838806334780784,
1.),(1.,0.840513202341181,1.),(1.,0.839504260685003,1.),(1.,0.836771095032971,
1.),(1.,0.825966649242057,1.),(1.,0.817815337411177,1.),(1.,0.795024845130666,
1.),(1.,0.780342956064905,1.),(1.,0.761980581628842,1.)))
REPRESENTATION_ITEM('')
SURFACE()
);
#2525=(
BOUNDED_SURFACE()
B_SPLINE_SURFACE(3,2,((#162380,#162381,#162382),(#162383,#162384,#162385),
(#162386,#162387,#162388),(#162389,#162390,#162391)),.UNSPECIFIED.,.F.,
 .F.,.F.)
B_SPLINE_SURFACE_WITH_KNOTS((4,4),(3,3),(-2.16840434497101E-19,0.000504456607560921),
(0.,1.),.UNSPECIFIED.)
GEOMETRIC_REPRESENTATION_ITEM()
RATIONAL_B_SPLINE_SURFACE(((1.,0.835211735760659,1.),(1.,0.83730162444359,
1.),(1.,0.839319452171524,1.),(1.,0.841267344812682,1.)))
REPRESENTATION_ITEM('')
SURFACE()
);
#2526=(
BOUNDED_SURFACE()
B_SPLINE_SURFACE(3,2,((#162395,#162396,#162397),(#162398,#162399,#162400),
(#162401,#162402,#162403),(#162404,#162405,#162406),(#162407,#162408,#162409),
(#162410,#162411,#162412),(#162413,#162414,#162415),(#162416,#162417,#162418)),
 .UNSPECIFIED.,.F.,.F.,.F.)
B_SPLINE_SURFACE_WITH_KNOTS((4,2,2,4),(3,3),(-0.000179925045351958,0.000899625226760169,
0.00134943784014025,0.00197917549887236),(0.,1.00242125618315),
 .UNSPECIFIED.)
GEOMETRIC_REPRESENTATION_ITEM()
RATIONAL_B_SPLINE_SURFACE(((1.,0.627732378823926,1.00180271055912),(1.,
0.702113319059347,1.00144251993621),(1.,0.752231213046251,1.00119982341481),
(1.,0.801387630970335,1.00096178285313),(1.,0.812691856939329,1.00090704199908),
(1.,0.834322378444833,1.0008022959312),(1.,0.841478824181795,1.00076764075422),
(1.,0.8445445625749,1.00075279487814)))
REPRESENTATION_ITEM('')
SURFACE()
);
#2527=(
BOUNDED_SURFACE()
B_SPLINE_SURFACE(3,2,((#162525,#162526,#162527),(#162528,#162529,#162530),
(#162531,#162532,#162533),(#162534,#162535,#162536),(#162537,#162538,#162539),
(#162540,#162541,#162542),(#162543,#162544,#162545),(#162546,#162547,#162548)),
 .UNSPECIFIED.,.F.,.F.,.F.)
B_SPLINE_SURFACE_WITH_KNOTS((4,2,2,4),(3,3),(-5.14996031930615E-18,0.000466811173310166,
0.000933622346620337,0.00186724469324068),(-0.00180391133637782,1.),
 .UNSPECIFIED.)
GEOMETRIC_REPRESENTATION_ITEM()
RATIONAL_B_SPLINE_SURFACE(((1.00041089117644,0.886111038786231,1.),(1.00041028049095,
0.886280305833524,1.),(1.0004242246253,0.882415333629096,1.),(1.0004790873429,
0.867208733256615,1.),(1.00052055430255,0.855715108594697,1.),(1.00068168753861,
0.811052925699315,1.),(1.00083807861781,0.767705152435299,1.),(1.00102927155329,
0.714711157767394,1.)))
REPRESENTATION_ITEM('')
SURFACE()
);
#2528=(
BOUNDED_SURFACE()
B_SPLINE_SURFACE(3,2,((#162647,#162648,#162649),(#162650,#162651,#162652),
(#162653,#162654,#162655),(#162656,#162657,#162658)),.UNSPECIFIED.,.F.,
 .F.,.F.)
B_SPLINE_SURFACE_WITH_KNOTS((4,4),(3,3),(0.,0.000504070263719173),(0.,1.),
 .UNSPECIFIED.)
GEOMETRIC_REPRESENTATION_ITEM()
RATIONAL_B_SPLINE_SURFACE(((1.,0.886316114436169,1.),(1.,0.886398092028818,
1.),(1.,0.886423525277845,1.),(1.,0.886392435202391,1.)))
REPRESENTATION_ITEM('')
SURFACE()
);
#2529=(
BOUNDED_SURFACE()
B_SPLINE_SURFACE(3,2,((#162662,#162663,#162664),(#162665,#162666,#162667),
(#162668,#162669,#162670),(#162671,#162672,#162673),(#162674,#162675,#162676),
(#162677,#162678,#162679),(#162680,#162681,#162682),(#162683,#162684,#162685),
(#162686,#162687,#162688),(#162689,#162690,#162691),(#162692,#162693,#162694),
(#162695,#162696,#162697)),.UNSPECIFIED.,.F.,.F.,.F.)
B_SPLINE_SURFACE_WITH_KNOTS((4,2,2,2,2,4),(3,3),(0.,0.000464847896993965,
0.00092969579398793,0.00116211974248491,0.00139454369098189,0.00185939158797586),
(0.,1.),.UNSPECIFIED.)
GEOMETRIC_REPRESENTATION_ITEM()
RATIONAL_B_SPLINE_SURFACE(((1.,0.713890629234418,1.),(1.,0.74043984709427,
1.),(1.,0.764405928904485,1.),(1.,0.806784773788238,1.),(1.,0.825414433535011,
1.),(1.,0.847876574774264,1.),(1.,0.854606009430438,1.),(1.,0.866028143804753,
1.),(1.,0.87079122929337,1.),(1.,0.882487982894785,1.),(1.,0.886433234017274,
1.),(1.,0.886392435203049,1.)))
REPRESENTATION_ITEM('')
SURFACE()
);
#2530=(
BOUNDED_SURFACE()
B_SPLINE_SURFACE(3,2,((#162835,#162836,#162837),(#162838,#162839,#162840),
(#162841,#162842,#162843),(#162844,#162845,#162846),(#162847,#162848,#162849),
(#162850,#162851,#162852),(#162853,#162854,#162855),(#162856,#162857,#162858),
(#162859,#162860,#162861),(#162862,#162863,#162864)),.UNSPECIFIED.,.F.,
 .F.,.F.)
B_SPLINE_SURFACE_WITH_KNOTS((4,2,2,2,4),(3,3),(-1.01915004213637E-17,0.00045240064920256,
0.00090480129840513,0.0013572019476077,0.00180960259681027),(0.,1.),
 .UNSPECIFIED.)
GEOMETRIC_REPRESENTATION_ITEM()
RATIONAL_B_SPLINE_SURFACE(((1.,0.843854525155974,1.),(1.,0.840228746359808,
1.),(1.,0.833848718540882,1.),(1.,0.81605021807051,1.),(1.,0.804487259154749,
1.),(1.,0.775654382443571,1.),(1.,0.758435167636249,1.),(1.,0.716870923938366,
1.),(1.,0.693173303079418,1.),(1.,0.665190809887608,1.)))
REPRESENTATION_ITEM('')
SURFACE()
);
#2531=(
BOUNDED_SURFACE()
B_SPLINE_SURFACE(3,2,((#162989,#162990,#162991),(#162992,#162993,#162994),
(#162995,#162996,#162997),(#162998,#162999,#163000)),.UNSPECIFIED.,.F.,
 .F.,.F.)
B_SPLINE_SURFACE_WITH_KNOTS((4,4),(3,3),(0.,0.000504443591143906),(0.,1.),
 .UNSPECIFIED.)
GEOMETRIC_REPRESENTATION_ITEM()
RATIONAL_B_SPLINE_SURFACE(((1.,0.843854525156016,1.),(1.,0.841969285469978,
1.),(1.,0.840014967913779,1.),(1.,0.837989542743208,1.)))
REPRESENTATION_ITEM('')
SURFACE()
);
#2532=(
BOUNDED_SURFACE()
B_SPLINE_SURFACE(3,2,((#163004,#163005,#163006),(#163007,#163008,#163009),
(#163010,#163011,#163012),(#163013,#163014,#163015),(#163016,#163017,#163018),
(#163019,#163020,#163021)),.UNSPECIFIED.,.F.,.F.,.F.)
B_SPLINE_SURFACE_WITH_KNOTS((4,2,4),(3,3),(-0.000158597896262736,0.000792989481313416,
0.00174457685888895),(-0.00240453499929849,1.),.UNSPECIFIED.)
GEOMETRIC_REPRESENTATION_ITEM()
RATIONAL_B_SPLINE_SURFACE(((1.00127175946673,0.735549811688094,1.),(1.00101661270767,
0.788605134055686,1.),(1.00087469807204,0.81811492195007,1.),(1.00073907087598,
0.846317297066205,1.),(1.00074935587393,0.844178630349327,1.),(1.00080479888491,
0.832649787767144,1.)))
REPRESENTATION_ITEM('')
SURFACE()
);
#2533=(
BOUNDED_SURFACE()
B_SPLINE_SURFACE(3,2,((#163108,#163109,#163110),(#163111,#163112,#163113),
(#163114,#163115,#163116),(#163117,#163118,#163119)),.UNSPECIFIED.,.F.,
 .F.,.F.)
B_SPLINE_SURFACE_WITH_KNOTS((4,4),(3,3),(-3.25260651745652E-19,0.0007884708222344),
(0.,1.),.UNSPECIFIED.)
GEOMETRIC_REPRESENTATION_ITEM()
RATIONAL_B_SPLINE_SURFACE(((1.,0.639433225268789,1.),(1.,0.625985289878347,
1.),(1.,0.614551947533885,1.),(1.,0.61107365918432,1.)))
REPRESENTATION_ITEM('')
SURFACE()
);
#2534=(
BOUNDED_SURFACE()
B_SPLINE_SURFACE(3,2,((#163168,#163169,#163170),(#163171,#163172,#163173),
(#163174,#163175,#163176),(#163177,#163178,#163179)),.UNSPECIFIED.,.F.,
 .F.,.F.)
B_SPLINE_SURFACE_WITH_KNOTS((4,4),(3,3),(0.00330239163309442,0.00410592895993832),
(0.,1.),.UNSPECIFIED.)
GEOMETRIC_REPRESENTATION_ITEM()
RATIONAL_B_SPLINE_SURFACE(((1.,0.707106781186551,1.),(1.,0.682330721002586,
1.),(1.,0.657517255942454,1.),(1.,0.639433225268795,1.)))
REPRESENTATION_ITEM('')
SURFACE()
);
#2535=(
BOUNDED_SURFACE()
B_SPLINE_SURFACE(3,2,((#163214,#163215,#163216),(#163217,#163218,#163219),
(#163220,#163221,#163222),(#163223,#163224,#163225),(#163226,#163227,#163228),
(#163229,#163230,#163231),(#163232,#163233,#163234),(#163235,#163236,#163237),
(#163238,#163239,#163240),(#163241,#163242,#163243)),.UNSPECIFIED.,.F.,
 .F.,.F.)
B_SPLINE_SURFACE_WITH_KNOTS((4,2,2,2,4),(3,3),(-0.000159639322855436,0.000399098307138592,
0.000798196614277184,0.00119729492141578,0.0017560325514098),(0.,1.00227173482475),
 .UNSPECIFIED.)
GEOMETRIC_REPRESENTATION_ITEM()
RATIONAL_B_SPLINE_SURFACE(((1.,0.803036549228823,1.00089489746064),(1.,
0.806208297931994,1.00088048671667),(1.,0.80375514797508,1.00089163252905),
(1.,0.791668382001202,1.00094654838341),(1.,0.784235158170282,1.00098032101028),
(1.,0.766082876391421,1.00106279535161),(1.,0.755212647809181,1.00111218390526),
(1.,0.727204596596005,1.00123943763589),(1.,0.708752138742072,1.00132327581811),
(1.,0.691327715635498,1.00140244315565)))
REPRESENTATION_ITEM('')
SURFACE()
);
#2536=(
BOUNDED_SURFACE()
B_SPLINE_SURFACE(3,2,((#163315,#163316,#163317),(#163318,#163319,#163320),
(#163321,#163322,#163323),(#163324,#163325,#163326),(#163327,#163328,#163329),
(#163330,#163331,#163332),(#163333,#163334,#163335),(#163336,#163337,#163338),
(#163339,#163340,#163341),(#163342,#163343,#163344)),.UNSPECIFIED.,.F.,
 .F.,.F.)
B_SPLINE_SURFACE_WITH_KNOTS((4,2,2,2,4),(3,3),(0.,0.000408689684844658,
0.000817379369689317,0.00122606905453398,0.00163475873937863),(0.,1.),
 .UNSPECIFIED.)
GEOMETRIC_REPRESENTATION_ITEM()
RATIONAL_B_SPLINE_SURFACE(((1.,0.707106781186864,1.),(1.,0.688970136944317,
1.),(1.,0.670689426918774,1.),(1.,0.634705388858963,1.),(1.,0.617712576312848,
1.),(1.,0.58736619029857,1.),(1.,0.574575334017929,1.),(1.,0.556620432342278,
1.),(1.,0.551687087704826,1.),(1.,0.55167311003777,1.)))
REPRESENTATION_ITEM('')
SURFACE()
);
#2537=(
BOUNDED_SURFACE()
B_SPLINE_SURFACE(3,2,((#163467,#163468,#163469),(#163470,#163471,#163472),
(#163473,#163474,#163475),(#163476,#163477,#163478)),.UNSPECIFIED.,.F.,
 .F.,.F.)
B_SPLINE_SURFACE_WITH_KNOTS((4,4),(3,3),(-6.10910588200899E-5,0.000672001647020572),
(-0.000116090865111071,1.),.UNSPECIFIED.)
GEOMETRIC_REPRESENTATION_ITEM()
RATIONAL_B_SPLINE_SURFACE(((1.00004877735551,0.789917339908843,1.),(1.00005479149462,
0.764014616617302,1.),(1.00006214451632,0.73234536470319,1.),(1.00006995490833,
0.698706232130948,1.)))
REPRESENTATION_ITEM('')
SURFACE()
);
#2538=(
BOUNDED_SURFACE()
B_SPLINE_SURFACE(3,2,((#163526,#163527,#163528),(#163529,#163530,#163531),
(#163532,#163533,#163534),(#163535,#163536,#163537)),.UNSPECIFIED.,.F.,
 .F.,.F.)
B_SPLINE_SURFACE_WITH_KNOTS((4,4),(3,3),(0.,0.00123332093723591),(0.,1.),
 .UNSPECIFIED.)
GEOMETRIC_REPRESENTATION_ITEM()
RATIONAL_B_SPLINE_SURFACE(((1.,0.903978945212084,1.),(1.,0.925250261712233,
1.),(1.,0.940236171156205,1.),(1.,0.947923524237147,1.)))
REPRESENTATION_ITEM('')
SURFACE()
);
#2539=(
BOUNDED_SURFACE()
B_SPLINE_SURFACE(3,2,((#163612,#163613,#163614),(#163615,#163616,#163617),
(#163618,#163619,#163620),(#163621,#163622,#163623),(#163624,#163625,#163626),
(#163627,#163628,#163629)),.UNSPECIFIED.,.F.,.F.,.F.)
B_SPLINE_SURFACE_WITH_KNOTS((4,2,4),(3,3),(-2.91766628346879E-5,0.000512893057734432,
0.00105496277830351),(-0.00146324405675922,1.00002917666283),
 .UNSPECIFIED.)
GEOMETRIC_REPRESENTATION_ITEM()
RATIONAL_B_SPLINE_SURFACE(((1.00054781718412,0.812801839713216,1.00001090767416),
(1.0005478023828,0.812806897568977,1.00001090737945),(1.00055033964304,
0.811939873927939,1.00001095789923),(1.00057518372836,0.80345024052436,
1.00001145257373),(1.00059830034578,0.795550911371957,1.00001191285233),
(1.00064180365305,0.780685114305911,1.00001277905353)))
REPRESENTATION_ITEM('')
SURFACE()
);
#2540=(
BOUNDED_SURFACE()
B_SPLINE_SURFACE(3,2,((#163651,#163652,#163653),(#163654,#163655,#163656),
(#163657,#163658,#163659),(#163660,#163661,#163662),(#163663,#163664,#163665),
(#163666,#163667,#163668)),.UNSPECIFIED.,.F.,.F.,.F.)
B_SPLINE_SURFACE_WITH_KNOTS((4,2,4),(3,3),(-4.77048955893622E-18,0.00191432655883667,
0.00382865311767335),(0.,1.),.UNSPECIFIED.)
GEOMETRIC_REPRESENTATION_ITEM()
RATIONAL_B_SPLINE_SURFACE(((1.,0.903978945212085,1.),(1.,0.877037193452108,
1.),(1.,0.847703426978615,1.),(1.,0.782785838918396,1.),(1.,0.74722569047758,
1.),(1.,0.707106781186548,1.)))
REPRESENTATION_ITEM('')
SURFACE()
);
#2541=(
BOUNDED_SURFACE()
B_SPLINE_SURFACE(3,2,((#163760,#163761,#163762),(#163763,#163764,#163765),
(#163766,#163767,#163768),(#163769,#163770,#163771),(#163772,#163773,#163774),
(#163775,#163776,#163777)),.UNSPECIFIED.,.F.,.F.,.F.)
B_SPLINE_SURFACE_WITH_KNOTS((4,2,4),(3,3),(0.,0.785398163397448,1.5707963267949),
(0.,1.),.UNSPECIFIED.)
GEOMETRIC_REPRESENTATION_ITEM()
RATIONAL_B_SPLINE_SURFACE(((1.,0.656059028990507,1.),(1.,0.655948674699894,
1.),(1.,0.661819490286433,1.),(1.,0.681005707982038,1.),(1.,0.694211427469109,
1.),(1.,0.707106781186548,1.)))
REPRESENTATION_ITEM('')
SURFACE()
);
#2542=(
BOUNDED_SURFACE()
B_SPLINE_SURFACE(3,2,((#163849,#163850,#163851),(#163852,#163853,#163854),
(#163855,#163856,#163857),(#163858,#163859,#163860),(#163861,#163862,#163863),
(#163864,#163865,#163866)),.UNSPECIFIED.,.F.,.F.,.F.)
B_SPLINE_SURFACE_WITH_KNOTS((4,2,4),(3,3),(1.5707963267949,2.35619449019234,
3.1415926535898),(0.,1.),.UNSPECIFIED.)
GEOMETRIC_REPRESENTATION_ITEM()
RATIONAL_B_SPLINE_SURFACE(((1.,0.707106781186548,1.),(1.,0.72003976564552,
1.),(1.,0.732392511163791,1.),(1.,0.749774985071113,1.),(1.,0.75478222211386,
1.),(1.,0.754709580222772,1.)))
REPRESENTATION_ITEM('')
SURFACE()
);
#2543=(
BOUNDED_SURFACE()
B_SPLINE_SURFACE(3,2,((#164070,#164071,#164072),(#164073,#164074,#164075),
(#164076,#164077,#164078),(#164079,#164080,#164081),(#164082,#164083,#164084),
(#164085,#164086,#164087)),.UNSPECIFIED.,.F.,.F.,.F.)
B_SPLINE_SURFACE_WITH_KNOTS((4,2,4),(3,3),(0.,0.785398163397448,1.5707963267949),
(0.,1.),.UNSPECIFIED.)
GEOMETRIC_REPRESENTATION_ITEM()
RATIONAL_B_SPLINE_SURFACE(((1.,0.656059028990507,1.),(1.,0.655948674699742,
1.),(1.,0.661819490286637,1.),(1.,0.681005707981833,1.),(1.,0.694211427469263,
1.),(1.,0.707106781186548,1.)))
REPRESENTATION_ITEM('')
SURFACE()
);
#2544=(
BOUNDED_SURFACE()
B_SPLINE_SURFACE(3,2,((#164159,#164160,#164161),(#164162,#164163,#164164),
(#164165,#164166,#164167),(#164168,#164169,#164170),(#164171,#164172,#164173),
(#164174,#164175,#164176)),.UNSPECIFIED.,.F.,.F.,.F.)
B_SPLINE_SURFACE_WITH_KNOTS((4,2,4),(3,3),(4.71238898038469,5.49778714378214,
6.28318530717959),(0.,1.),.UNSPECIFIED.)
GEOMETRIC_REPRESENTATION_ITEM()
RATIONAL_B_SPLINE_SURFACE(((1.,0.707106781186552,1.),(1.,0.720039765645528,
1.),(1.,0.732392511163776,1.),(1.,0.749774985071127,1.),(1.,0.754782222113857,
1.),(1.,0.754709580222772,1.)))
REPRESENTATION_ITEM('')
SURFACE()
);
#2545=(
BOUNDED_SURFACE()
B_SPLINE_SURFACE(3,2,((#164411,#164412,#164413),(#164414,#164415,#164416),
(#164417,#164418,#164419),(#164420,#164421,#164422),(#164423,#164424,#164425),
(#164426,#164427,#164428)),.UNSPECIFIED.,.F.,.F.,.F.)
B_SPLINE_SURFACE_WITH_KNOTS((4,2,4),(3,3),(0.0740543944727613,0.0811932403219739,
0.0883320861711864),(0.,1.),.UNSPECIFIED.)
GEOMETRIC_REPRESENTATION_ITEM()
RATIONAL_B_SPLINE_SURFACE(((1.,0.918849788108586,1.),(1.,0.921623427170992,
1.),(1.,0.924482745526459,1.),(1.,0.930368049939493,1.),(1.,0.933390296558584,
1.),(1.,0.936467000373499,1.)))
REPRESENTATION_ITEM('')
SURFACE()
);
#2546=(
BOUNDED_SURFACE()
B_SPLINE_SURFACE(3,2,((#164641,#164642,#164643),(#164644,#164645,#164646),
(#164647,#164648,#164649),(#164650,#164651,#164652),(#164653,#164654,#164655),
(#164656,#164657,#164658)),.UNSPECIFIED.,.F.,.F.,.F.)
B_SPLINE_SURFACE_WITH_KNOTS((4,2,4),(3,3),(0.269041526988586,0.27511900362718,
0.281196480265774),(0.,1.),.UNSPECIFIED.)
GEOMETRIC_REPRESENTATION_ITEM()
RATIONAL_B_SPLINE_SURFACE(((1.,0.936757701036177,1.),(1.,0.939378149853558,
1.),(1.,0.942051042550488,1.),(1.,0.947449038066665,1.),(1.,0.950158897999453,
1.),(1.,0.952840299126697,1.)))
REPRESENTATION_ITEM('')
SURFACE()
);
#2547=(
BOUNDED_SURFACE()
B_SPLINE_SURFACE(3,2,((#164959,#164960,#164961),(#164962,#164963,#164964),
(#164965,#164966,#164967),(#164968,#164969,#164970)),.UNSPECIFIED.,.F.,
 .F.,.F.)
B_SPLINE_SURFACE_WITH_KNOTS((4,4),(3,3),(0.,0.0174508326761739),(0.,1.),
 .UNSPECIFIED.)
GEOMETRIC_REPRESENTATION_ITEM()
RATIONAL_B_SPLINE_SURFACE(((1.,0.472392340793765,1.),(1.,0.485682667654673,
1.),(1.,0.49679147679375,1.),(1.,0.506538946041787,1.)))
REPRESENTATION_ITEM('')
SURFACE()
);
#2548=(
BOUNDED_SURFACE()
B_SPLINE_SURFACE(3,2,((#164996,#164997,#164998),(#164999,#165000,#165001),
(#165002,#165003,#165004),(#165005,#165006,#165007),(#165008,#165009,#165010),
(#165011,#165012,#165013),(#165014,#165015,#165016),(#165017,#165018,#165019)),
 .UNSPECIFIED.,.F.,.F.,.F.)
B_SPLINE_SURFACE_WITH_KNOTS((4,2,2,4),(3,3),(0.,0.0013193848583342,0.00263876971666841,
0.00527753943333681),(0.,1.),.UNSPECIFIED.)
GEOMETRIC_REPRESENTATION_ITEM()
RATIONAL_B_SPLINE_SURFACE(((1.,0.472392340793765,1.),(1.,0.494569863951139,
1.),(1.,0.516028114800238,1.),(1.,0.557651118782376,1.),(1.,0.577819616806839,
1.),(1.,0.636749517047671,1.),(1.,0.673107462854922,1.),(1.,0.707106781186548,
1.)))
REPRESENTATION_ITEM('')
SURFACE()
);
#2549=(
BOUNDED_SURFACE()
B_SPLINE_SURFACE(3,2,((#165054,#165055,#165056),(#165057,#165058,#165059),
(#165060,#165061,#165062),(#165063,#165064,#165065),(#165066,#165067,#165068),
(#165069,#165070,#165071),(#165072,#165073,#165074),(#165075,#165076,#165077)),
 .UNSPECIFIED.,.F.,.F.,.F.)
B_SPLINE_SURFACE_WITH_KNOTS((4,2,2,4),(3,3),(-0.000342067638939368,0.00263855694108943,
0.00395783541163415,0.00561918145328965),(-0.00153661657981784,1.),
 .UNSPECIFIED.)
GEOMETRIC_REPRESENTATION_ITEM()
RATIONAL_B_SPLINE_SURFACE(((1.00086096519304,0.71985035032541,1.),(1.00097794016698,
0.681787838351873,1.),(1.00110163105103,0.641540034937012,1.),(1.00129767452272,
0.577749407442451,1.),(1.00136056639245,0.557285008399528,1.),(1.00150619096957,
0.509900195875283,1.),(1.00159023347395,0.482553587266646,1.),(1.00167739996307,
0.454190464588956,1.)))
REPRESENTATION_ITEM('')
SURFACE()
);
#2550=(
BOUNDED_SURFACE()
B_SPLINE_SURFACE(3,2,((#165096,#165097,#165098),(#165099,#165100,#165101),
(#165102,#165103,#165104),(#165105,#165106,#165107)),.UNSPECIFIED.,.F.,
 .F.,.F.)
B_SPLINE_SURFACE_WITH_KNOTS((4,4),(3,3),(6.93889390390723E-18,0.0177264565684137),
(0.,1.),.UNSPECIFIED.)
GEOMETRIC_REPRESENTATION_ITEM()
RATIONAL_B_SPLINE_SURFACE(((1.,0.506999357883079,1.),(1.,0.497142617029225,
1.),(1.,0.485892200859361,1.),(1.,0.472392340793768,1.)))
REPRESENTATION_ITEM('')
SURFACE()
);
#2551=(
BOUNDED_SURFACE()
B_SPLINE_SURFACE(3,2,((#165114,#165115,#165116),(#165117,#165118,#165119),
(#165120,#165121,#165122),(#165123,#165124,#165125),(#165126,#165127,#165128),
(#165129,#165130,#165131),(#165132,#165133,#165134),(#165135,#165136,#165137)),
 .UNSPECIFIED.,.F.,.F.,.F.)
B_SPLINE_SURFACE_WITH_KNOTS((4,2,2,4),(3,3),(-2.83789918648081E-17,0.000158415844625727,
0.000316831689251482,0.000633663378502992),(0.,1.),.UNSPECIFIED.)
GEOMETRIC_REPRESENTATION_ITEM()
RATIONAL_B_SPLINE_SURFACE(((1.,0.506999357883079,1.),(1.,0.518705031372287,
1.),(1.,0.533099046918872,1.),(1.,0.565407295868411,1.),(1.,0.582886848388227,
1.),(1.,0.636421215472814,1.),(1.,0.67314781771756,1.),(1.,0.707106781186543,
1.)))
REPRESENTATION_ITEM('')
SURFACE()
);
#2552=(
BOUNDED_SURFACE()
B_SPLINE_SURFACE(3,2,((#165157,#165158,#165159),(#165160,#165161,#165162),
(#165163,#165164,#165165),(#165166,#165167,#165168),(#165169,#165170,#165171),
(#165172,#165173,#165174),(#165175,#165176,#165177),(#165178,#165179,#165180),
(#165181,#165182,#165183),(#165184,#165185,#165186)),.UNSPECIFIED.,.F.,
 .F.,.F.)
B_SPLINE_SURFACE_WITH_KNOTS((4,2,2,2,4),(3,3),(-8.88178419700125E-16,0.392699081698724,
0.785398163397448,1.17809724509617,1.5707963267949),(0.,1.),
 .UNSPECIFIED.)
GEOMETRIC_REPRESENTATION_ITEM()
RATIONAL_B_SPLINE_SURFACE(((1.,0.656059028990507,1.),(1.,0.65605119607191,
1.),(1.,0.657443209221259,1.),(1.,0.662724068472642,1.),(1.,0.666616044204551,
1.),(1.,0.676209154063925,1.),(1.,0.681903435451068,1.),(1.,0.694134907060979,
1.),(1.,0.70066637883416,1.),(1.,0.707106781186548,1.)))
REPRESENTATION_ITEM('')
SURFACE()
);
#2553=(
BOUNDED_SURFACE()
B_SPLINE_SURFACE(3,2,((#165246,#165247,#165248),(#165249,#165250,#165251),
(#165252,#165253,#165254),(#165255,#165256,#165257),(#165258,#165259,#165260),
(#165261,#165262,#165263),(#165264,#165265,#165266),(#165267,#165268,#165269),
(#165270,#165271,#165272),(#165273,#165274,#165275)),.UNSPECIFIED.,.F.,
 .F.,.F.)
B_SPLINE_SURFACE_WITH_KNOTS((4,2,2,2,4),(3,3),(4.71238898038469,5.10508806208341,
5.49778714378214,5.89048622548086,6.28318530717959),(0.,1.),
 .UNSPECIFIED.)
GEOMETRIC_REPRESENTATION_ITEM()
RATIONAL_B_SPLINE_SURFACE(((1.,0.707106781186552,1.),(1.,0.713550261851565,
1.),(1.,0.719894264862192,1.),(1.,0.731490756397333,1.),(1.,0.736738129296254,
1.),(1.,0.745429366938654,1.),(1.,0.748871927696603,1.),(1.,0.753512297096217,
1.),(1.,0.754714219730812,1.),(1.,0.754709580222777,1.)))
REPRESENTATION_ITEM('')
SURFACE()
);
#2554=(
BOUNDED_SURFACE()
B_SPLINE_SURFACE(3,2,((#165292,#165293,#165294),(#165295,#165296,#165297),
(#165298,#165299,#165300),(#165301,#165302,#165303),(#165304,#165305,#165306),
(#165307,#165308,#165309)),.UNSPECIFIED.,.F.,.F.,.F.)
B_SPLINE_SURFACE_WITH_KNOTS((4,2,4),(3,3),(-6.49900913755202E-5,0.000324950456877623,
0.000714891005130771),(-0.0004124377275279,1.),.UNSPECIFIED.)
GEOMETRIC_REPRESENTATION_ITEM()
RATIONAL_B_SPLINE_SURFACE(((1.0002597372525,0.685119431172141,1.),(1.00022332133393,
0.7292666031402,1.),(1.00018870296933,0.771234592847265,1.),(1.00013212596193,
0.839823137995945,1.),(1.00010945519713,0.867307001975368,1.),(1.00009818284526,
0.880972521781153,1.)))
REPRESENTATION_ITEM('')
SURFACE()
);
#2555=(
BOUNDED_SURFACE()
B_SPLINE_SURFACE(3,2,((#165334,#165335,#165336),(#165337,#165338,#165339),
(#165340,#165341,#165342),(#165343,#165344,#165345)),.UNSPECIFIED.,.F.,
 .F.,.F.)
B_SPLINE_SURFACE_WITH_KNOTS((4,4),(3,3),(-6.93889390390723E-18,0.0138038180377133),
(0.,1.),.UNSPECIFIED.)
GEOMETRIC_REPRESENTATION_ITEM()
RATIONAL_B_SPLINE_SURFACE(((1.,0.888620714475959,1.),(1.,0.882992994712188,
1.),(1.,0.877840677983261,1.),(1.,0.873073026815702,1.)))
REPRESENTATION_ITEM('')
SURFACE()
);
#2556=(
BOUNDED_SURFACE()
B_SPLINE_SURFACE(3,2,((#165352,#165353,#165354),(#165355,#165356,#165357),
(#165358,#165359,#165360),(#165361,#165362,#165363),(#165364,#165365,#165366),
(#165367,#165368,#165369),(#165370,#165371,#165372),(#165373,#165374,#165375)),
 .UNSPECIFIED.,.F.,.F.,.F.)
B_SPLINE_SURFACE_WITH_KNOTS((4,2,2,4),(3,3),(0.,0.00140148291572316,0.00280296583144632,
0.00560593166289265),(0.,1.),.UNSPECIFIED.)
GEOMETRIC_REPRESENTATION_ITEM()
RATIONAL_B_SPLINE_SURFACE(((1.,0.888620714475959,1.),(1.,0.876376872535401,
1.),(1.,0.863367339892611,1.),(1.,0.835880005025182,1.),(1.,0.821403024634208,
1.),(1.,0.775582050820272,1.),(1.,0.742820617730576,1.),(1.,0.707106781185993,
1.)))
REPRESENTATION_ITEM('')
SURFACE()
);
#2557=(
BOUNDED_SURFACE()
B_SPLINE_SURFACE(3,2,((#165401,#165402,#165403),(#165404,#165405,#165406),
(#165407,#165408,#165409),(#165410,#165411,#165412),(#165413,#165414,#165415),
(#165416,#165417,#165418),(#165419,#165420,#165421),(#165422,#165423,#165424)),
 .UNSPECIFIED.,.F.,.F.,.F.)
B_SPLINE_SURFACE_WITH_KNOTS((4,2,2,4),(3,3),(0.,0.00280275939636971,0.00420413909455456,
0.00560551879273941),(0.,1.),.UNSPECIFIED.)
GEOMETRIC_REPRESENTATION_ITEM()
RATIONAL_B_SPLINE_SURFACE(((1.,0.707106781186548,1.),(1.,0.742840106247676,
1.),(1.,0.77545596336237,1.),(1.,0.821038365376531,1.),(1.,0.835714486585925,
1.),(1.,0.863346562356171,1.),(1.,0.876386389875133,1.),(1.,0.888620714475965,
1.)))
REPRESENTATION_ITEM('')
SURFACE()
);
#2558=(
BOUNDED_SURFACE()
B_SPLINE_SURFACE(3,2,((#165443,#165444,#165445),(#165446,#165447,#165448),
(#165449,#165450,#165451),(#165452,#165453,#165454)),.UNSPECIFIED.,.F.,
 .F.,.F.)
B_SPLINE_SURFACE_WITH_KNOTS((4,4),(3,3),(-6.93889390390723E-18,0.0135258923233721),
(0.,1.),.UNSPECIFIED.)
GEOMETRIC_REPRESENTATION_ITEM()
RATIONAL_B_SPLINE_SURFACE(((1.,0.873361457045398,1.),(1.,0.878048383336236,
1.),(1.,0.883106305929072,1.),(1.,0.888620714475961,1.)))
REPRESENTATION_ITEM('')
SURFACE()
);
#2559=(
BOUNDED_SURFACE()
B_SPLINE_SURFACE(3,2,((#165461,#165462,#165463),(#165464,#165465,#165466),
(#165467,#165468,#165469),(#165470,#165471,#165472),(#165473,#165474,#165475),
(#165476,#165477,#165478)),.UNSPECIFIED.,.F.,.F.,.F.)
B_SPLINE_SURFACE_WITH_KNOTS((4,2,4),(3,3),(-6.47810798060089E-18,0.000325048915579083,
0.000650097831158172),(0.,1.),.UNSPECIFIED.)
GEOMETRIC_REPRESENTATION_ITEM()
RATIONAL_B_SPLINE_SURFACE(((1.,0.873361457045401,1.),(1.,0.85849847792363,
1.),(1.,0.834696857457215,1.),(1.,0.77714142509596,1.),(1.,0.743612803250452,
1.),(1.,0.707106781186552,1.)))
REPRESENTATION_ITEM('')
SURFACE()
);
#2560=(
BOUNDED_SURFACE()
B_SPLINE_SURFACE(3,2,((#165671,#165672,#165673),(#165674,#165675,#165676),
(#165677,#165678,#165679),(#165680,#165681,#165682),(#165683,#165684,#165685),
(#165686,#165687,#165688),(#165689,#165690,#165691),(#165692,#165693,#165694)),
 .UNSPECIFIED.,.F.,.F.,.F.)
B_SPLINE_SURFACE_WITH_KNOTS((4,2,2,4),(3,3),(0.,0.000351812098911224,0.000527718148366836,
0.000703624197822447),(0.,1.),.UNSPECIFIED.)
GEOMETRIC_REPRESENTATION_ITEM()
RATIONAL_B_SPLINE_SURFACE(((1.,0.707106781186548,1.),(1.,0.666004685610564,
1.),(1.,0.620075381085077,1.),(1.,0.549819108711631,1.),(1.,0.525790037137517,
1.),(1.,0.479829608303299,1.),(1.,0.458216765529125,1.),(1.,0.439917019807004,
1.)))
REPRESENTATION_ITEM('')
SURFACE()
);
#2561=(
BOUNDED_SURFACE()
B_SPLINE_SURFACE(3,2,((#165716,#165717,#165718),(#165719,#165720,#165721),
(#165722,#165723,#165724),(#165725,#165726,#165727)),.UNSPECIFIED.,.F.,
 .F.,.F.)
B_SPLINE_SURFACE_WITH_KNOTS((4,4),(3,3),(-5.03069808033274E-17,0.00385726433182564),
(0.,1.),.UNSPECIFIED.)
GEOMETRIC_REPRESENTATION_ITEM()
RATIONAL_B_SPLINE_SURFACE(((1.,0.430570049114201,1.),(1.,0.433791974258431,
1.),(1.,0.436904245661489,1.),(1.,0.439917019807019,1.)))
REPRESENTATION_ITEM('')
SURFACE()
);
#2562=(
BOUNDED_SURFACE()
B_SPLINE_SURFACE(3,2,((#165734,#165735,#165736),(#165737,#165738,#165739),
(#165740,#165741,#165742),(#165743,#165744,#165745),(#165746,#165747,#165748),
(#165749,#165750,#165751),(#165752,#165753,#165754),(#165755,#165756,#165757),
(#165758,#165759,#165760),(#165761,#165762,#165763),(#165764,#165765,#165766),
(#165767,#165768,#165769)),.UNSPECIFIED.,.F.,.F.,.F.)
B_SPLINE_SURFACE_WITH_KNOTS((4,2,2,2,2,4),(3,3),(0.,0.00157461356268982,
0.00236192034403473,0.00314922712537965,0.00472384068806947,0.0062984542507593),
(0.,1.),.UNSPECIFIED.)
GEOMETRIC_REPRESENTATION_ITEM()
RATIONAL_B_SPLINE_SURFACE(((1.,0.430570049114667,1.),(1.,0.457560960025303,
1.),(1.,0.483459257940472,1.),(1.,0.520841505371429,1.),(1.,0.533061067348069,
1.),(1.,0.557070570158285,1.),(1.,0.5688948619132,1.),(1.,0.603453431912179,
1.),(1.,0.625340642509566,1.),(1.,0.667408719974356,1.),(1.,0.687583394050722,
1.),(1.,0.707106781186543,1.)))
REPRESENTATION_ITEM('')
SURFACE()
);
#2563=(
BOUNDED_SURFACE()
B_SPLINE_SURFACE(3,2,((#165795,#165796,#165797),(#165798,#165799,#165800),
(#165801,#165802,#165803),(#165804,#165805,#165806),(#165807,#165808,#165809),
(#165810,#165811,#165812),(#165813,#165814,#165815),(#165816,#165817,#165818),
(#165819,#165820,#165821),(#165822,#165823,#165824)),.UNSPECIFIED.,.F.,
 .F.,.F.)
B_SPLINE_SURFACE_WITH_KNOTS((4,2,2,2,4),(3,3),(0.,0.00157421549227777,0.00314843098455553,
0.0047226464768333,0.00629686196911106),(0.,1.),.UNSPECIFIED.)
GEOMETRIC_REPRESENTATION_ITEM()
RATIONAL_B_SPLINE_SURFACE(((1.,0.707106781187362,1.),(1.,0.68758289696825,
1.),(1.,0.667417078226011,1.),(1.,0.625390824237668,1.),(1.,0.60353633747147,
1.),(1.,0.557559397493831,1.),(1.,0.533401321926016,1.),(1.,0.483474255638482,
1.),(1.,0.457551920277023,1.),(1.,0.430570049114227,1.)))
REPRESENTATION_ITEM('')
SURFACE()
);
#2564=(
BOUNDED_SURFACE()
B_SPLINE_SURFACE(3,2,((#165843,#165844,#165845),(#165846,#165847,#165848),
(#165849,#165850,#165851),(#165852,#165853,#165854)),.UNSPECIFIED.,.F.,
 .F.,.F.)
B_SPLINE_SURFACE_WITH_KNOTS((4,4),(3,3),(0.,0.00414272899747597),(0.,1.),
 .UNSPECIFIED.)
GEOMETRIC_REPRESENTATION_ITEM()
RATIONAL_B_SPLINE_SURFACE(((1.,0.440584280700845,1.),(1.,0.437364321804866,
1.),(1.,0.434030421143282,1.),(1.,0.43057004911423,1.)))
REPRESENTATION_ITEM('')
SURFACE()
);
#2565=(
BOUNDED_SURFACE()
B_SPLINE_SURFACE(3,2,((#165861,#165862,#165863),(#165864,#165865,#165866),
(#165867,#165868,#165869),(#165870,#165871,#165872),(#165873,#165874,#165875),
(#165876,#165877,#165878),(#165879,#165880,#165881),(#165882,#165883,#165884),
(#165885,#165886,#165887),(#165888,#165889,#165890)),.UNSPECIFIED.,.F.,
 .F.,.F.)
B_SPLINE_SURFACE_WITH_KNOTS((4,2,2,2,4),(3,3),(-6.16097884514888E-17,0.000175529658750937,
0.000351059317501936,0.000526588976252934,0.000702118635003933),(0.,1.),
 .UNSPECIFIED.)
GEOMETRIC_REPRESENTATION_ITEM()
RATIONAL_B_SPLINE_SURFACE(((1.,0.440584280700845,1.),(1.,0.458788905458512,
1.),(1.,0.480391768923104,1.),(1.,0.526541516020855,1.),(1.,0.550240391579637,
1.),(1.,0.597052366816548,1.),(1.,0.620407250394368,1.),(1.,0.664886737818671,
1.),(1.,0.686305427599538,1.),(1.,0.707106781186548,1.)))
REPRESENTATION_ITEM('')
SURFACE()
);
#2566=(
BOUNDED_SURFACE()
B_SPLINE_SURFACE(3,2,((#165910,#165911,#165912),(#165913,#165914,#165915),
(#165916,#165917,#165918),(#165919,#165920,#165921),(#165922,#165923,#165924),
(#165925,#165926,#165927),(#165928,#165929,#165930),(#165931,#165932,#165933),
(#165934,#165935,#165936),(#165937,#165938,#165939)),.UNSPECIFIED.,.F.,
 .F.,.F.)
B_SPLINE_SURFACE_WITH_KNOTS((4,2,2,2,4),(3,3),(-8.88178419700125E-16,0.392699081698724,
0.785398163397448,1.17809724509617,1.5707963267949),(0.,1.),
 .UNSPECIFIED.)
GEOMETRIC_REPRESENTATION_ITEM()
RATIONAL_B_SPLINE_SURFACE(((1.,0.656059028990513,1.),(1.,0.656051196071901,
1.),(1.,0.657443209221259,1.),(1.,0.662724068472642,1.),(1.,0.666616044204551,
1.),(1.,0.676209154063925,1.),(1.,0.681903435451265,1.),(1.,0.694134907060781,
1.),(1.,0.70066637883431,1.),(1.,0.707106781186548,1.)))
REPRESENTATION_ITEM('')
SURFACE()
);
#2567=(
BOUNDED_SURFACE()
B_SPLINE_SURFACE(3,2,((#165987,#165988,#165989),(#165990,#165991,#165992),
(#165993,#165994,#165995),(#165996,#165997,#165998),(#165999,#166000,#166001),
(#166002,#166003,#166004),(#166005,#166006,#166007),(#166008,#166009,#166010),
(#166011,#166012,#166013),(#166014,#166015,#166016)),.UNSPECIFIED.,.F.,
 .F.,.F.)
B_SPLINE_SURFACE_WITH_KNOTS((4,2,2,2,4),(3,3),(0.00108313181642978,0.00175636478508586,
0.00242959775374195,0.00310283072239804,0.00377606369105412),(-0.000209460012389645,
1.),.UNSPECIFIED.)
GEOMETRIC_REPRESENTATION_ITEM()
RATIONAL_B_SPLINE_SURFACE(((1.00012272453498,0.707045431769307,1.),(1.00009434426233,
0.774791710231349,1.),(1.00007166829577,0.82892129397012,1.),(1.00004030861562,
0.903779687680096,1.),(1.00003179560245,0.924101020320203,1.),(1.0000315466092,
0.924695389732363,1.),(1.00003985538719,0.904861584947119,1.),(1.00007114262338,
0.830176121522307,1.),(1.00009383870826,0.775998513536397,1.),(1.00012272453498,
0.707045431769307,1.)))
REPRESENTATION_ITEM('')
SURFACE()
);
#2568=(
BOUNDED_SURFACE()
B_SPLINE_SURFACE(3,2,((#166095,#166096,#166097),(#166098,#166099,#166100),
(#166101,#166102,#166103),(#166104,#166105,#166106),(#166107,#166108,#166109),
(#166110,#166111,#166112),(#166113,#166114,#166115),(#166116,#166117,#166118),
(#166119,#166120,#166121),(#166122,#166123,#166124)),.UNSPECIFIED.,.F.,
 .F.,.F.)
B_SPLINE_SURFACE_WITH_KNOTS((4,2,2,2,4),(3,3),(4.71238898038469,5.10508806208341,
5.49778714378214,5.89048622548086,6.28318530717959),(0.,1.),
 .UNSPECIFIED.)
GEOMETRIC_REPRESENTATION_ITEM()
RATIONAL_B_SPLINE_SURFACE(((1.,0.707106781186552,1.),(1.,0.713550261851678,
1.),(1.,0.71989426486204,1.),(1.,0.731490756397489,1.),(1.,0.736738129296849,
1.),(1.,0.745429366938066,1.),(1.,0.748871927696599,1.),(1.,0.753512297096214,
1.),(1.,0.754714219730812,1.),(1.,0.754709580222777,1.)))
REPRESENTATION_ITEM('')
SURFACE()
);
#2569=(
BOUNDED_SURFACE()
B_SPLINE_SURFACE(3,2,((#166135,#166136,#166137),(#166138,#166139,#166140),
(#166141,#166142,#166143),(#166144,#166145,#166146)),.UNSPECIFIED.,.F.,
 .F.,.F.)
B_SPLINE_SURFACE_WITH_KNOTS((4,4),(3,3),(-1.68213967061126E-16,0.000120540380538488),
(0.,1.),.UNSPECIFIED.)
GEOMETRIC_REPRESENTATION_ITEM()
RATIONAL_B_SPLINE_SURFACE(((1.,0.819851970694933,1.),(1.,0.826338730586804,
1.),(1.,0.831810971765196,1.),(1.,0.836255146268139,1.)))
REPRESENTATION_ITEM('')
SURFACE()
);
#2570=(
BOUNDED_SURFACE()
B_SPLINE_SURFACE(3,2,((#166155,#166156,#166157),(#166158,#166159,#166160),
(#166161,#166162,#166163),(#166164,#166165,#166166),(#166167,#166168,#166169),
(#166170,#166171,#166172)),.UNSPECIFIED.,.F.,.F.,.F.)
B_SPLINE_SURFACE_WITH_KNOTS((4,2,4),(3,3),(0.,0.0128929585057523,0.0257859170115046),
(0.,1.),.UNSPECIFIED.)
GEOMETRIC_REPRESENTATION_ITEM()
RATIONAL_B_SPLINE_SURFACE(((1.,0.862148985649771,1.),(1.,0.857001824466315,
1.),(1.,0.852340953158334,1.),(1.,0.843773924789864,1.),(1.,0.839868090827823,
1.),(1.,0.83625514626814,1.)))
REPRESENTATION_ITEM('')
SURFACE()
);
#2571=(
BOUNDED_SURFACE()
B_SPLINE_SURFACE(3,2,((#166182,#166183,#166184),(#166185,#166186,#166187),
(#166188,#166189,#166190),(#166191,#166192,#166193),(#166194,#166195,#166196),
(#166197,#166198,#166199),(#166200,#166201,#166202),(#166203,#166204,#166205)),
 .UNSPECIFIED.,.F.,.F.,.F.)
B_SPLINE_SURFACE_WITH_KNOTS((4,2,2,4),(3,3),(-0.000114297678441313,0.00224905873968498,
0.00337358810952747,0.00461247683191633),(-0.000114359352546393,1.),
 .UNSPECIFIED.)
GEOMETRIC_REPRESENTATION_ITEM()
RATIONAL_B_SPLINE_SURFACE(((1.0000307769399,0.865437591192138,1.),(1.00003596191931,
0.842767913115381,1.),(1.0000416442543,0.817923705527529,1.),(1.00005085149573,
0.777667962443431,1.),(1.00005395268399,0.764109000325605,1.),(1.00006064498396,
0.734849041160352,1.),(1.00006427096229,0.718995600871095,1.),(1.00006803721689,
0.702528847114332,1.)))
REPRESENTATION_ITEM('')
SURFACE()
);
#2572=(
BOUNDED_SURFACE()
B_SPLINE_SURFACE(3,2,((#166228,#166229,#166230),(#166231,#166232,#166233),
(#166234,#166235,#166236),(#166237,#166238,#166239),(#166240,#166241,#166242),
(#166243,#166244,#166245)),.UNSPECIFIED.,.F.,.F.,.F.)
B_SPLINE_SURFACE_WITH_KNOTS((4,2,4),(3,3),(0.,0.00224843555189379,0.00449687110378757),
(0.,1.),.UNSPECIFIED.)
GEOMETRIC_REPRESENTATION_ITEM()
RATIONAL_B_SPLINE_SURFACE(((1.,0.707106781186548,1.),(1.,0.736791791485942,
1.),(1.,0.764326610725229,1.),(1.,0.81612979408374,1.),(1.,0.840519041516535,
1.),(1.,0.862148985649773,1.)))
REPRESENTATION_ITEM('')
SURFACE()
);
#2573=(
BOUNDED_SURFACE()
B_SPLINE_SURFACE(3,2,((#166273,#166274,#166275),(#166276,#166277,#166278),
(#166279,#166280,#166281),(#166282,#166283,#166284),(#166285,#166286,#166287),
(#166288,#166289,#166290)),.UNSPECIFIED.,.F.,.F.,.F.)
B_SPLINE_SURFACE_WITH_KNOTS((4,2,4),(3,3),(0.,0.0127570403976527,0.0255140807953054),
(0.,1.),.UNSPECIFIED.)
GEOMETRIC_REPRESENTATION_ITEM()
RATIONAL_B_SPLINE_SURFACE(((1.,0.83648401963888,1.),(1.,0.840071262854844,
1.),(1.,0.843946769546665,1.),(1.,0.852439323016447,1.),(1.,0.857056062862677,
1.),(1.,0.862148985649771,1.)))
REPRESENTATION_ITEM('')
SURFACE()
);
#2574=(
BOUNDED_SURFACE()
B_SPLINE_SURFACE(3,2,((#166346,#166347,#166348),(#166349,#166350,#166351),
(#166352,#166353,#166354),(#166355,#166356,#166357),(#166358,#166359,#166360),
(#166361,#166362,#166363)),.UNSPECIFIED.,.F.,.F.,.F.)
B_SPLINE_SURFACE_WITH_KNOTS((4,2,4),(3,3),(0.,0.000518347860385374,0.00103669572077075),
(0.,1.),.UNSPECIFIED.)
GEOMETRIC_REPRESENTATION_ITEM()
RATIONAL_B_SPLINE_SURFACE(((1.,0.819851970694872,1.),(1.,0.821199393891468,
1.),(1.,0.820620061026224,1.),(1.,0.813565992888811,1.),(1.,0.807280082867884,
1.),(1.,0.797551754323293,1.)))
REPRESENTATION_ITEM('')
SURFACE()
);
#2575=(
BOUNDED_SURFACE()
B_SPLINE_SURFACE(3,2,((#166377,#166378,#166379),(#166380,#166381,#166382),
(#166383,#166384,#166385),(#166386,#166387,#166388),(#166389,#166390,#166391),
(#166392,#166393,#166394),(#166395,#166396,#166397),(#166398,#166399,#166400),
(#166401,#166402,#166403),(#166404,#166405,#166406)),.UNSPECIFIED.,.F.,
 .F.,.F.)
B_SPLINE_SURFACE_WITH_KNOTS((4,2,2,2,4),(3,3),(0.,0.000158289020679031,
0.000316578041358062,0.000474867062037094,0.000633156082716125),(-0.000663546784200084,
1.),.UNSPECIFIED.)
GEOMETRIC_REPRESENTATION_ITEM()
RATIONAL_B_SPLINE_SURFACE(((1.00038895462537,0.70691243283309,1.),(1.00041168676458,
0.689783166476245,1.),(1.00043480575931,0.672362394282253,1.),(1.00048201433009,
0.636789491287992,1.),(1.00050649669526,0.618341383513315,1.),(1.00055382351628,
0.582679375841648,1.),(1.00057681572595,0.565354139539206,1.),(1.00062018464055,
0.532674518722848,1.),(1.00063973378298,0.517943724381941,1.),(1.00065530352718,
0.50621151154631,1.)))
REPRESENTATION_ITEM('')
SURFACE()
);
#2576=(
BOUNDED_SURFACE()
B_SPLINE_SURFACE(3,2,((#166442,#166443,#166444),(#166445,#166446,#166447),
(#166448,#166449,#166450),(#166451,#166452,#166453)),.UNSPECIFIED.,.F.,
 .F.,.F.)
B_SPLINE_SURFACE_WITH_KNOTS((4,4),(3,3),(0.00167806205423436,0.0019221164224989),
(0.,1.),.UNSPECIFIED.)
GEOMETRIC_REPRESENTATION_ITEM()
RATIONAL_B_SPLINE_SURFACE(((1.,0.83648401963888,1.),(1.,0.827500667105214,
1.),(1.,0.81402442184051,1.),(1.,0.797363061122239,1.)))
REPRESENTATION_ITEM('')
SURFACE()
);
#2577=(
BOUNDED_SURFACE()
B_SPLINE_SURFACE(3,2,((#166471,#166472,#166473),(#166474,#166475,#166476),
(#166477,#166478,#166479),(#166480,#166481,#166482),(#166483,#166484,#166485),
(#166486,#166487,#166488)),.UNSPECIFIED.,.F.,.F.,.F.)
B_SPLINE_SURFACE_WITH_KNOTS((4,2,4),(3,3),(-6.48707035919281E-5,0.000324353517959648,
0.000713577739511227),(-0.000405636278254878,1.),.UNSPECIFIED.)
GEOMETRIC_REPRESENTATION_ITEM()
RATIONAL_B_SPLINE_SURFACE(((1.00025537797947,0.685213092166142,1.),(1.00021971394,
0.729173705886148,1.),(1.00018580256851,0.770973926060662,1.),(1.0001303846956,
0.839283734482019,1.),(1.0001081970018,0.866632981809814,1.),(1.00009717328087,
0.88022116601206,1.)))
REPRESENTATION_ITEM('')
SURFACE()
);
#2578=(
BOUNDED_SURFACE()
B_SPLINE_SURFACE(3,2,((#166571,#166572,#166573),(#166574,#166575,#166576),
(#166577,#166578,#166579),(#166580,#166581,#166582)),.UNSPECIFIED.,.F.,
 .F.,.F.)
B_SPLINE_SURFACE_WITH_KNOTS((4,4),(3,3),(0.,0.0138879247081574),(0.,1.),
 .UNSPECIFIED.)
GEOMETRIC_REPRESENTATION_ITEM()
RATIONAL_B_SPLINE_SURFACE(((1.,0.887998771276556,1.),(1.,0.882334484690674,
1.),(1.,0.877154223922122,1.),(1.,0.872364293278347,1.)))
REPRESENTATION_ITEM('')
SURFACE()
);
#2579=(
BOUNDED_SURFACE()
B_SPLINE_SURFACE(3,2,((#166589,#166590,#166591),(#166592,#166593,#166594),
(#166595,#166596,#166597),(#166598,#166599,#166600),(#166601,#166602,#166603),
(#166604,#166605,#166606),(#166607,#166608,#166609),(#166610,#166611,#166612)),
 .UNSPECIFIED.,.F.,.F.,.F.)
B_SPLINE_SURFACE_WITH_KNOTS((4,2,2,4),(3,3),(0.,0.00139422219513554,0.00278844439027108,
0.00557688878054216),(-0.000307172053122608,1.),.UNSPECIFIED.)
GEOMETRIC_REPRESENTATION_ITEM()
RATIONAL_B_SPLINE_SURFACE(((1.00006882843044,0.887964367629177,1.),(1.00007633423115,
0.875746783638711,1.),(1.00008430612713,0.862770512034486,1.),(1.00010114500028,
0.835360998417529,1.),(1.00011001146245,0.820928594689669,1.),(1.00013806798131,
0.775259533038872,1.),(1.00015813805149,0.742590431185938,1.),(1.00017999249442,
0.707016812574673,1.)))
REPRESENTATION_ITEM('')
SURFACE()
);
#2580=(
BOUNDED_SURFACE()
B_SPLINE_SURFACE(3,2,((#166638,#166639,#166640),(#166641,#166642,#166643),
(#166644,#166645,#166646),(#166647,#166648,#166649),(#166650,#166651,#166652),
(#166653,#166654,#166655),(#166656,#166657,#166658),(#166659,#166660,#166661)),
 .UNSPECIFIED.,.F.,.F.,.F.)
B_SPLINE_SURFACE_WITH_KNOTS((4,2,2,4),(3,3),(0.,0.00278824321172774,0.00418236481759161,
0.00557648642345548),(0.,1.),.UNSPECIFIED.)
GEOMETRIC_REPRESENTATION_ITEM()
RATIONAL_B_SPLINE_SURFACE(((1.,0.707106781186548,1.),(1.,0.742695591047798,
1.),(1.,0.775190977638611,1.),(1.,0.820614084370083,1.),(1.,0.835242277112269,
1.),(1.,0.862791265741296,1.),(1.,0.875794541967241,1.),(1.,0.887998771276056,
1.)))
REPRESENTATION_ITEM('')
SURFACE()
);
#2581=(
BOUNDED_SURFACE()
B_SPLINE_SURFACE(3,2,((#166680,#166681,#166682),(#166683,#166684,#166685),
(#166686,#166687,#166688),(#166689,#166690,#166691)),.UNSPECIFIED.,.F.,
 .F.,.F.)
B_SPLINE_SURFACE_WITH_KNOTS((4,4),(3,3),(0.,0.0141656229616797),(0.,1.),
 .UNSPECIFIED.)
GEOMETRIC_REPRESENTATION_ITEM()
RATIONAL_B_SPLINE_SURFACE(((1.,0.872077446583348,1.),(1.,0.876947206822174,
1.),(1.,0.882221222508023,1.),(1.,0.887998771276578,1.)))
REPRESENTATION_ITEM('')
SURFACE()
);
#2582=(
BOUNDED_SURFACE()
B_SPLINE_SURFACE(3,2,((#166698,#166699,#166700),(#166701,#166702,#166703),
(#166704,#166705,#166706),(#166707,#166708,#166709),(#166710,#166711,#166712),
(#166713,#166714,#166715)),.UNSPECIFIED.,.F.,.F.,.F.)
B_SPLINE_SURFACE_WITH_KNOTS((4,2,4),(3,3),(-6.48077526460634E-5,0.000324038763230374,
0.000712885279106823),(-0.000106163867131493,1.),.UNSPECIFIED.)
GEOMETRIC_REPRESENTATION_ITEM()
RATIONAL_B_SPLINE_SURFACE(((1.00002552144573,0.879801638625688,1.),(1.00002832831616,
0.866582120070106,1.),(1.00003408916573,0.839450244950509,1.),(1.00004864326935,
0.770904778322745,1.),(1.00005737063385,0.729801506857169,1.),(1.00006688410924,
0.684995888682771,1.)))
REPRESENTATION_ITEM('')
SURFACE()
);
#2583=(
BOUNDED_SURFACE()
B_SPLINE_SURFACE(3,2,((#166738,#166739,#166740),(#166741,#166742,#166743),
(#166744,#166745,#166746),(#166747,#166748,#166749),(#166750,#166751,#166752),
(#166753,#166754,#166755),(#166756,#166757,#166758),(#166759,#166760,#166761),
(#166762,#166763,#166764),(#166765,#166766,#166767)),.UNSPECIFIED.,.F.,
 .F.,.F.)
B_SPLINE_SURFACE_WITH_KNOTS((4,2,2,2,4),(3,3),(3.1415926535898,3.53429173528852,
3.92699081698724,4.31968989868597,4.71238898038469),(0.,1.),
 .UNSPECIFIED.)
GEOMETRIC_REPRESENTATION_ITEM()
RATIONAL_B_SPLINE_SURFACE(((1.,0.754709580222772,1.),(1.,0.754714219730848,
1.),(1.,0.753512297096158,1.),(1.,0.748871927696634,1.),(1.,0.745429366938649,
1.),(1.,0.736738129296255,1.),(1.,0.731490756397077,1.),(1.,0.719894264862441,
1.),(1.,0.713550261851367,1.),(1.,0.707106781186548,1.)))
REPRESENTATION_ITEM('')
SURFACE()
);
#2584=(
BOUNDED_SURFACE()
B_SPLINE_SURFACE(3,2,((#166816,#166817,#166818),(#166819,#166820,#166821),
(#166822,#166823,#166824),(#166825,#166826,#166827),(#166828,#166829,#166830),
(#166831,#166832,#166833),(#166834,#166835,#166836),(#166837,#166838,#166839),
(#166840,#166841,#166842),(#166843,#166844,#166845)),.UNSPECIFIED.,.F.,
 .F.,.F.)
B_SPLINE_SURFACE_WITH_KNOTS((4,2,2,2,4),(3,3),(1.5706633618744,1.96349540849362,
2.35619449019234,2.74889357189107,3.14172561851029),(0.,1.0001329649205),
 .UNSPECIFIED.)
GEOMETRIC_REPRESENTATION_ITEM()
RATIONAL_B_SPLINE_SURFACE(((1.,0.707074379515176,1.00007789766368),(1.,
0.700631001612551,1.00007961115014),(1.,0.694096308749504,1.00008134891997),
(1.,0.681861139767303,1.00008460261652),(1.,0.676166101239835,1.00008611709721),
(1.,0.666571715833371,1.00008866853059),(1.,0.662679222605223,1.0000897036607),
(1.,0.657396767036559,1.00009110842327),(1.,0.656004520314218,1.00009147866321),
(0.999999999999999,0.65601330534573,1.00009147632701)))
REPRESENTATION_ITEM('')
SURFACE()
);
#2585=(
BOUNDED_SURFACE()
B_SPLINE_SURFACE(3,2,((#166862,#166863,#166864),(#166865,#166866,#166867),
(#166868,#166869,#166870),(#166871,#166872,#166873),(#166874,#166875,#166876),
(#166877,#166878,#166879),(#166880,#166881,#166882),(#166883,#166884,#166885),
(#166886,#166887,#166888),(#166889,#166890,#166891)),.UNSPECIFIED.,.F.,
 .F.,.F.)
B_SPLINE_SURFACE_WITH_KNOTS((4,2,2,2,4),(3,3),(0.,0.000157845161260656,
0.000315690322521312,0.000473535483781968,0.000631380645042625),(-0.000656128803624682,
1.),.UNSPECIFIED.)
GEOMETRIC_REPRESENTATION_ITEM()
RATIONAL_B_SPLINE_SURFACE(((1.00038460353849,0.706914605509298,1.),(1.00040690056226,
0.689923258963295,1.),(1.00042956531064,0.672651689525801,1.),(1.00047581616045,
0.637406437715701,1.),(1.00049979042774,0.619136955291255,1.),(1.00054610047252,
0.583846594218537,1.),(1.00056857293538,0.566721555097505,1.),(1.00061090851415,
0.534459917946195,1.),(1.00062995710208,0.519944027299337,1.),(1.00064512214601,
0.508387573871131,1.)))
REPRESENTATION_ITEM('')
SURFACE()
);
#2586=(
BOUNDED_SURFACE()
B_SPLINE_SURFACE(3,2,((#166913,#166914,#166915),(#166916,#166917,#166918),
(#166919,#166920,#166921),(#166922,#166923,#166924)),.UNSPECIFIED.,.F.,
 .F.,.F.)
B_SPLINE_SURFACE_WITH_KNOTS((4,4),(3,3),(0.,0.0180689587739334),(0.,1.),
 .UNSPECIFIED.)
GEOMETRIC_REPRESENTATION_ITEM()
RATIONAL_B_SPLINE_SURFACE(((1.,0.473671517629134,1.),(1.,0.487381853083234,
1.),(1.,0.49876090260372,1.),(1.,0.508709923441297,1.)))
REPRESENTATION_ITEM('')
SURFACE()
);
#2587=(
BOUNDED_SURFACE()
B_SPLINE_SURFACE(3,2,((#166931,#166932,#166933),(#166934,#166935,#166936),
(#166937,#166938,#166939),(#166940,#166941,#166942),(#166943,#166944,#166945),
(#166946,#166947,#166948),(#166949,#166950,#166951),(#166952,#166953,#166954),
(#166955,#166956,#166957),(#166958,#166959,#166960)),.UNSPECIFIED.,.F.,
 .F.,.F.)
B_SPLINE_SURFACE_WITH_KNOTS((4,2,2,2,4),(3,3),(-4.33680868994201E-18,0.00131184996336558,
0.00262369992673117,0.00393554989009676,0.00524739985346235),(0.,1.),
 .UNSPECIFIED.)
GEOMETRIC_REPRESENTATION_ITEM()
RATIONAL_B_SPLINE_SURFACE(((1.,0.473671517629133,1.),(1.,0.495707594803631,
1.),(1.,0.517034522428114,1.),(1.,0.558412152901823,1.),(1.,0.578466470542957,
1.),(1.,0.617536962037478,1.),(1.,0.636393525150058,1.),(1.,0.672664546785766,
1.),(1.,0.690145348310819,1.),(1.,0.707106781186548,1.)))
REPRESENTATION_ITEM('')
SURFACE()
);
#2588=(
BOUNDED_SURFACE()
B_SPLINE_SURFACE(3,2,((#166983,#166984,#166985),(#166986,#166987,#166988),
(#166989,#166990,#166991),(#166992,#166993,#166994),(#166995,#166996,#166997),
(#166998,#166999,#167000),(#167001,#167002,#167003),(#167004,#167005,#167006)),
 .UNSPECIFIED.,.F.,.F.,.F.)
B_SPLINE_SURFACE_WITH_KNOTS((4,2,2,4),(3,3),(0.,0.00262348010799063,0.00393522016198593,
0.00524696021598125),(0.,1.),.UNSPECIFIED.)
GEOMETRIC_REPRESENTATION_ITEM()
RATIONAL_B_SPLINE_SURFACE(((1.,0.70710678118732,1.),(1.,0.673159051373371,
1.),(1.,0.637356734328886,1.),(1.,0.579048422068377,1.),(1.,0.558729842945168,
1.),(1.,0.517089292555981,1.),(1.,0.495689661102028,1.),(1.,0.473671517629131,
1.)))
REPRESENTATION_ITEM('')
SURFACE()
);
#2589=(
BOUNDED_SURFACE()
B_SPLINE_SURFACE(3,2,((#167025,#167026,#167027),(#167028,#167029,#167030),
(#167031,#167032,#167033),(#167034,#167035,#167036)),.UNSPECIFIED.,.F.,
 .F.,.F.)
B_SPLINE_SURFACE_WITH_KNOTS((4,4),(3,3),(-6.93889390390723E-18,0.0177935197894076),
(0.,1.),.UNSPECIFIED.)
GEOMETRIC_REPRESENTATION_ITEM()
RATIONAL_B_SPLINE_SURFACE(((1.,0.508254344125608,1.),(1.,0.498412666571477,
1.),(1.,0.487173250319529,1.),(1.,0.473671517629131,1.)))
REPRESENTATION_ITEM('')
SURFACE()
);
#2590=(
BOUNDED_SURFACE()
B_SPLINE_SURFACE(3,2,((#167072,#167073,#167074),(#167075,#167076,#167077),
(#167078,#167079,#167080),(#167081,#167082,#167083),(#167084,#167085,#167086),
(#167087,#167088,#167089),(#167090,#167091,#167092),(#167093,#167094,#167095)),
 .UNSPECIFIED.,.F.,.F.,.F.)
B_SPLINE_SURFACE_WITH_KNOTS((4,2,2,4),(3,3),(-6.50521303491303E-18,0.000158176853950714,
0.000316353707901435,0.000632707415802875),(0.,1.),.UNSPECIFIED.)
GEOMETRIC_REPRESENTATION_ITEM()
RATIONAL_B_SPLINE_SURFACE(((1.,0.50825434412561,1.),(1.,0.519857702736613,
1.),(1.,0.534132547044037,1.),(1.,0.566198696596924,1.),(1.,0.583560620774966,
1.),(1.,0.636763258069658,1.),(1.,0.673308410857549,1.),(1.,0.707106781186552,
1.)))
REPRESENTATION_ITEM('')
SURFACE()
);
#2591=(
BOUNDED_SURFACE()
B_SPLINE_SURFACE(3,2,((#167226,#167227,#167228),(#167229,#167230,#167231),
(#167232,#167233,#167234),(#167235,#167236,#167237)),.UNSPECIFIED.,.F.,
 .F.,.F.)
B_SPLINE_SURFACE_WITH_KNOTS((4,4),(3,3),(-1.1328828500301E-15,0.000723745383907254),
(0.,1.),.UNSPECIFIED.)
GEOMETRIC_REPRESENTATION_ITEM()
RATIONAL_B_SPLINE_SURFACE(((1.,0.802684671198269,1.),(1.,0.797620722711664,
1.),(1.,0.787749610789602,1.),(1.,0.773398994756355,1.)))
REPRESENTATION_ITEM('')
SURFACE()
);
#2592=(
BOUNDED_SURFACE()
B_SPLINE_SURFACE(3,2,((#167258,#167259,#167260),(#167261,#167262,#167263),
(#167264,#167265,#167266),(#167267,#167268,#167269)),.UNSPECIFIED.,.F.,
 .F.,.F.)
B_SPLINE_SURFACE_WITH_KNOTS((4,4),(3,3),(-2.12668013510612E-5,0.00023393481488825),
(-2.58890273307494E-5,1.),.UNSPECIFIED.)
GEOMETRIC_REPRESENTATION_ITEM()
RATIONAL_B_SPLINE_SURFACE(((1.00001043498075,0.798467114731324,1.),(1.00000954588804,
0.815638341296739,1.),(1.00000885543353,0.828973228358054,1.),(1.00000840251418,
0.837720550997796,0.999999999999999)))
REPRESENTATION_ITEM('')
SURFACE()
);
#2593=(
BOUNDED_SURFACE()
B_SPLINE_SURFACE(3,2,((#167274,#167275,#167276),(#167277,#167278,#167279),
(#167280,#167281,#167282),(#167283,#167284,#167285),(#167286,#167287,#167288),
(#167289,#167290,#167291)),.UNSPECIFIED.,.F.,.F.,.F.)
B_SPLINE_SURFACE_WITH_KNOTS((4,2,4),(3,3),(0.,0.0129055642122842,0.0258111284245685),
(0.,1.),.UNSPECIFIED.)
GEOMETRIC_REPRESENTATION_ITEM()
RATIONAL_B_SPLINE_SURFACE(((1.,0.861290731803006,1.),(1.,0.856148221578915,
1.),(1.,0.851494227257712,1.),(1.,0.842943112520738,1.),(1.,0.839046328378941,
1.),(1.,0.835442841040481,1.)))
REPRESENTATION_ITEM('')
SURFACE()
);
#2594=(
BOUNDED_SURFACE()
B_SPLINE_SURFACE(3,2,((#167301,#167302,#167303),(#167304,#167305,#167306),
(#167307,#167308,#167309),(#167310,#167311,#167312),(#167313,#167314,#167315),
(#167316,#167317,#167318),(#167319,#167320,#167321),(#167322,#167323,#167324)),
 .UNSPECIFIED.,.F.,.F.,.F.)
B_SPLINE_SURFACE_WITH_KNOTS((4,2,2,4),(3,3),(-0.000118679703551729,0.00223318354977648,
0.00334977532466471,0.00458504680310467),(-0.000118679703551729,1.),
 .UNSPECIFIED.)
GEOMETRIC_REPRESENTATION_ITEM()
RATIONAL_B_SPLINE_SURFACE(((1.00003211137202,0.864714137900249,1.),(1.00003747888505,
0.842100696538067,1.),(1.00004335836542,0.817330326405749,1.),(1.00005287395854,
0.777240939453633,1.),(1.00005607406915,0.763758808486968,1.),(1.00006299338349,
0.734607596724851,1.),(1.00006674915501,0.718784455078024,1.),(1.00007064938466,
0.702352708408401,0.999999999999999)))
REPRESENTATION_ITEM('')
SURFACE()
);
#2595=(
BOUNDED_SURFACE()
B_SPLINE_SURFACE(3,2,((#167347,#167348,#167349),(#167350,#167351,#167352),
(#167353,#167354,#167355),(#167356,#167357,#167358),(#167359,#167360,#167361),
(#167362,#167363,#167364)),.UNSPECIFIED.,.F.,.F.,.F.)
B_SPLINE_SURFACE_WITH_KNOTS((4,2,4),(3,3),(4.33680868994202E-19,0.0022325368353913,
0.00446507367078261),(0.,1.),.UNSPECIFIED.)
GEOMETRIC_REPRESENTATION_ITEM()
RATIONAL_B_SPLINE_SURFACE(((1.,0.707106781186548,1.),(1.,0.736599220372578,
1.),(1.,0.763970742639471,1.),(1.,0.815484818127782,1.),(1.,0.839751912193024,
1.),(1.,0.861290731802537,1.)))
REPRESENTATION_ITEM('')
SURFACE()
);
#2596=(
BOUNDED_SURFACE()
B_SPLINE_SURFACE(3,2,((#167392,#167393,#167394),(#167395,#167396,#167397),
(#167398,#167399,#167400),(#167401,#167402,#167403),(#167404,#167405,#167406),
(#167407,#167408,#167409)),.UNSPECIFIED.,.F.,.F.,.F.)
B_SPLINE_SURFACE_WITH_KNOTS((4,2,4),(3,3),(0.,0.0130414224518927,0.0260828449037854),
(0.,1.),.UNSPECIFIED.)
GEOMETRIC_REPRESENTATION_ITEM()
RATIONAL_B_SPLINE_SURFACE(((1.,0.835215680136663,1.),(1.,0.838844513950773,
1.),(1.,0.842771271110783,1.),(1.,0.851396246528345,1.),(1.,0.856094111052002,
1.),(1.,0.861290731803024,1.)))
REPRESENTATION_ITEM('')
SURFACE()
);
#2597=(
BOUNDED_SURFACE()
B_SPLINE_SURFACE(3,2,((#167419,#167420,#167421),(#167422,#167423,#167424),
(#167425,#167426,#167427),(#167428,#167429,#167430)),.UNSPECIFIED.,.F.,
 .F.,.F.)
B_SPLINE_SURFACE_WITH_KNOTS((4,4),(3,3),(0.,0.000106239733749475),(0.,1.),
 .UNSPECIFIED.)
GEOMETRIC_REPRESENTATION_ITEM()
RATIONAL_B_SPLINE_SURFACE(((1.,0.835215680136664,1.),(1.,0.831333836917881,
1.),(1.,0.826651097750167,1.),(1.,0.821176675475199,1.)))
REPRESENTATION_ITEM('')
SURFACE()
);
#2598=(
BOUNDED_SURFACE()
B_SPLINE_SURFACE(3,2,((#167437,#167438,#167439),(#167440,#167441,#167442),
(#167443,#167444,#167445),(#167446,#167447,#167448),(#167449,#167450,#167451),
(#167452,#167453,#167454)),.UNSPECIFIED.,.F.,.F.,.F.)
B_SPLINE_SURFACE_WITH_KNOTS((4,2,4),(3,3),(0.,0.000488761174293955,0.00097752234858791),
(0.,1.),.UNSPECIFIED.)
GEOMETRIC_REPRESENTATION_ITEM()
RATIONAL_B_SPLINE_SURFACE(((1.,0.813073674901529,1.),(1.,0.819782614828204,
1.),(1.,0.82321022732318,1.),(1.,0.825342446816795,1.),(1.,0.824005064313242,
1.),(1.,0.821176675475194,1.)))
REPRESENTATION_ITEM('')
SURFACE()
);
#2599=(
BOUNDED_SURFACE()
B_SPLINE_SURFACE(3,2,((#167489,#167490,#167491),(#167492,#167493,#167494),
(#167495,#167496,#167497),(#167498,#167499,#167500),(#167501,#167502,#167503),
(#167504,#167505,#167506),(#167507,#167508,#167509),(#167510,#167511,#167512),
(#167513,#167514,#167515),(#167516,#167517,#167518)),.UNSPECIFIED.,.F.,
 .F.,.F.)
B_SPLINE_SURFACE_WITH_KNOTS((4,2,2,2,4),(3,3),(3.1415926535898,3.53429173528852,
3.92699081698724,4.31968989868597,4.71238898038469),(0.,1.),
 .UNSPECIFIED.)
GEOMETRIC_REPRESENTATION_ITEM()
RATIONAL_B_SPLINE_SURFACE(((1.,0.754709580222776,1.),(1.,0.75471421973084,
1.),(1.,0.753512297096162,1.),(1.,0.748871927696637,1.),(1.,0.745429366938649,
1.),(1.,0.736738129296255,1.),(1.,0.73149075639724,1.),(1.,0.719894264862275,
1.),(1.,0.713550261851491,1.),(1.,0.707106781186548,1.)))
REPRESENTATION_ITEM('')
SURFACE()
);
#2600=(
BOUNDED_SURFACE()
B_SPLINE_SURFACE(3,2,((#167546,#167547,#167548),(#167549,#167550,#167551),
(#167552,#167553,#167554),(#167555,#167556,#167557),(#167558,#167559,#167560),
(#167561,#167562,#167563),(#167564,#167565,#167566),(#167567,#167568,#167569),
(#167570,#167571,#167572),(#167573,#167574,#167575)),.UNSPECIFIED.,.F.,
 .F.,.F.)
B_SPLINE_SURFACE_WITH_KNOTS((4,2,2,2,4),(3,3),(0.00131180726843867,0.00173116479138242,
0.00215052231432617,0.00256987983726992,0.00298923736021366),(-7.19536585550859E-6,
1.),.UNSPECIFIED.)
GEOMETRIC_REPRESENTATION_ITEM()
RATIONAL_B_SPLINE_SURFACE(((1.00000421497806,0.707104673712682,1.),(1.00000380693457,
0.735459277069438,1.),(1.00000349584283,0.757076784022164,1.),(1.00000307861073,
0.786069896432006,1.),(1.00000297270674,0.793429076618855,1.),(1.00000297242619,
0.793448571747273,1.),(1.00000307812241,0.786103829137561,1.),(1.00000349515575,
0.757124528683259,1.),(1.00000380600652,0.735523766262835,1.),(1.00000421497806,
0.707104673712682,1.)))
REPRESENTATION_ITEM('')
SURFACE()
);
#2601=(
BOUNDED_SURFACE()
B_SPLINE_SURFACE(3,2,((#167676,#167677,#167678),(#167679,#167680,#167681),
(#167682,#167683,#167684),(#167685,#167686,#167687),(#167688,#167689,#167690),
(#167691,#167692,#167693),(#167694,#167695,#167696),(#167697,#167698,#167699)),
 .UNSPECIFIED.,.F.,.F.,.F.)
B_SPLINE_SURFACE_WITH_KNOTS((4,2,2,4),(3,3),(0.,0.000350059279280428,0.000525088918920643,
0.000700118558560857),(0.,1.),.UNSPECIFIED.)
GEOMETRIC_REPRESENTATION_ITEM()
RATIONAL_B_SPLINE_SURFACE(((1.,0.707106781186548,1.),(1.,0.666269021153261,
1.),(1.,0.620643690025591,1.),(1.,0.551020195303415,1.),(1.,0.527243635346707,
1.),(1.,0.48184496425994,1.),(1.,0.460546552679624,1.),(1.,0.442551630563558,
1.)))
REPRESENTATION_ITEM('')
SURFACE()
);
#2602=(
BOUNDED_SURFACE()
B_SPLINE_SURFACE(3,2,((#167721,#167722,#167723),(#167724,#167725,#167726),
(#167727,#167728,#167729),(#167730,#167731,#167732)),.UNSPECIFIED.,.F.,
 .F.,.F.)
B_SPLINE_SURFACE_WITH_KNOTS((4,4),(3,3),(-1.00613961606655E-16,0.00454919832189776),
(0.,1.),.UNSPECIFIED.)
GEOMETRIC_REPRESENTATION_ITEM()
RATIONAL_B_SPLINE_SURFACE(((1.,0.43161218489519,1.),(1.,0.4354057728044,
1.),(1.,0.439046733702441,1.),(1.,0.442551630563568,1.)))
REPRESENTATION_ITEM('')
SURFACE()
);
#2603=(
BOUNDED_SURFACE()
B_SPLINE_SURFACE(3,2,((#167739,#167740,#167741),(#167742,#167743,#167744),
(#167745,#167746,#167747),(#167748,#167749,#167750),(#167751,#167752,#167753),
(#167754,#167755,#167756),(#167757,#167758,#167759),(#167760,#167761,#167762),
(#167763,#167764,#167765),(#167766,#167767,#167768),(#167769,#167770,#167771),
(#167772,#167773,#167774)),.UNSPECIFIED.,.F.,.F.,.F.)
B_SPLINE_SURFACE_WITH_KNOTS((4,2,2,2,2,4),(3,3),(0.,0.0015680710888481,
0.00235210663327216,0.0031361421776962,0.00470421326654431,0.00627228435539241),
(0.,1.),.UNSPECIFIED.)
GEOMETRIC_REPRESENTATION_ITEM()
RATIONAL_B_SPLINE_SURFACE(((1.,0.431612184896198,1.),(1.,0.458478767119797,
1.),(1.,0.484262778995081,1.),(1.,0.521487645866883,1.),(1.,0.533657012907055,
1.),(1.,0.557569946367873,1.),(1.,0.569348142420323,1.),(1.,0.603784372807714,
1.),(1.,0.625598432901225,1.),(1.,0.667530632490446,1.),(1.,0.687642674416921,
1.),(1.,0.707106781186545,1.)))
REPRESENTATION_ITEM('')
SURFACE()
);
#2604=(
BOUNDED_SURFACE()
B_SPLINE_SURFACE(3,2,((#167800,#167801,#167802),(#167803,#167804,#167805),
(#167806,#167807,#167808),(#167809,#167810,#167811),(#167812,#167813,#167814),
(#167815,#167816,#167817),(#167818,#167819,#167820),(#167821,#167822,#167823),
(#167824,#167825,#167826),(#167827,#167828,#167829)),.UNSPECIFIED.,.F.,
 .F.,.F.)
B_SPLINE_SURFACE_WITH_KNOTS((4,2,2,2,4),(3,3),(0.,0.00156769407161709,0.00313538814323418,
0.00470308221485126,0.00627077628646835),(0.,1.),.UNSPECIFIED.)
GEOMETRIC_REPRESENTATION_ITEM()
RATIONAL_B_SPLINE_SURFACE(((1.,0.707106781185944,1.),(1.,0.687642132810167,
1.),(1.,0.6675396507768,1.),(1.,0.625652582590125,1.),(1.,0.603873832998886,
1.),(1.,0.558067925921433,1.),(1.,0.534002288872959,1.),(1.,0.484278918307038,
1.),(1.,0.458469143464434,1.),(1.,0.431612184895232,1.)))
REPRESENTATION_ITEM('')
SURFACE()
);
#2605=(
BOUNDED_SURFACE()
B_SPLINE_SURFACE(3,2,((#167848,#167849,#167850),(#167851,#167852,#167853),
(#167854,#167855,#167856),(#167857,#167858,#167859)),.UNSPECIFIED.,.F.,
 .F.,.F.)
B_SPLINE_SURFACE_WITH_KNOTS((4,4),(3,3),(1.7347234759768E-18,0.00426411906192034),
(0.,1.),.UNSPECIFIED.)
GEOMETRIC_REPRESENTATION_ITEM()
RATIONAL_B_SPLINE_SURFACE(((1.,0.441891116431774,1.),(1.,0.438589787881315,
1.),(1.,0.435168043398159,1.),(1.,0.431612184895232,1.)))
REPRESENTATION_ITEM('')
SURFACE()
);
#2606=(
BOUNDED_SURFACE()
B_SPLINE_SURFACE(3,2,((#167866,#167867,#167868),(#167869,#167870,#167871),
(#167872,#167873,#167874),(#167875,#167876,#167877),(#167878,#167879,#167880),
(#167881,#167882,#167883),(#167884,#167885,#167886),(#167887,#167888,#167889),
(#167890,#167891,#167892),(#167893,#167894,#167895)),.UNSPECIFIED.,.F.,
 .F.,.F.)
B_SPLINE_SURFACE_WITH_KNOTS((4,2,2,2,4),(3,3),(0.,0.000175112702239915,
0.000350225404479831,0.000525338106719747,0.000700450808959663),(0.,1.),
 .UNSPECIFIED.)
GEOMETRIC_REPRESENTATION_ITEM()
RATIONAL_B_SPLINE_SURFACE(((1.,0.441891116431771,1.),(1.,0.459945578495206,
1.),(1.,0.481391225572596,1.),(1.,0.52725624746098,1.),(1.,0.550835433567685,
1.),(1.,0.597437830540943,1.),(1.,0.62070290968502,1.),(1.,0.665021344579013,
1.),(1.,0.68636937449165,1.),(1.,0.707106781186548,1.)))
REPRESENTATION_ITEM('')
SURFACE()
);
#2607=(
BOUNDED_SURFACE()
B_SPLINE_SURFACE(3,2,((#168014,#168015,#168016),(#168017,#168018,#168019),
(#168020,#168021,#168022),(#168023,#168024,#168025),(#168026,#168027,#168028),
(#168029,#168030,#168031),(#168032,#168033,#168034),(#168035,#168036,#168037),
(#168038,#168039,#168040),(#168041,#168042,#168043)),.UNSPECIFIED.,.F.,
 .F.,.F.)
B_SPLINE_SURFACE_WITH_KNOTS((4,2,2,2,4),(3,3),(1.57066336187496,1.96349540849362,
2.35619449019234,2.74889357189107,3.14172561850969),(0.,1.00013296491993),
 .UNSPECIFIED.)
GEOMETRIC_REPRESENTATION_ITEM()
RATIONAL_B_SPLINE_SURFACE(((1.,0.707074379515315,1.00007789766335),(1.,
0.700631001612556,1.0000796111498),(1.,0.694096308749865,1.00008134891963),
(1.,0.681861139767284,1.00008460261615),(1.,0.676166101239372,1.00008611709684),
(1.,0.666571715834207,1.00008866853021),(1.,0.662679222605431,1.00008970366031),
(1.,0.657396767036752,1.00009110842288),(1.,0.656004520314433,1.00009147866283),
(1.,0.656013305345919,1.00009147632662)))
REPRESENTATION_ITEM('')
SURFACE()
);
#2608=(
BOUNDED_SURFACE()
B_SPLINE_SURFACE(3,2,((#168068,#168069,#168070),(#168071,#168072,#168073),
(#168074,#168075,#168076),(#168077,#168078,#168079),(#168080,#168081,#168082),
(#168083,#168084,#168085),(#168086,#168087,#168088),(#168089,#168090,#168091)),
 .UNSPECIFIED.,.F.,.F.,.F.)
B_SPLINE_SURFACE_WITH_KNOTS((4,2,2,4),(3,3),(0.,0.000337961269725901,0.000506941904588851,
0.000675922539451801),(0.,1.),.UNSPECIFIED.)
GEOMETRIC_REPRESENTATION_ITEM()
RATIONAL_B_SPLINE_SURFACE(((1.,0.707106781186548,1.),(1.,0.66833529952704,
1.),(1.,0.625126311995779,1.),(1.,0.560329805282816,1.),(1.,0.53845874286336,
1.),(1.,0.497198802480914,1.),(1.,0.478168468596388,1.),(1.,0.462319489161107,
1.)))
REPRESENTATION_ITEM('')
SURFACE()
);
#2609=(
BOUNDED_SURFACE()
B_SPLINE_SURFACE(3,2,((#168189,#168190,#168191),(#168192,#168193,#168194),
(#168195,#168196,#168197),(#168198,#168199,#168200)),.UNSPECIFIED.,.F.,
 .F.,.F.)
B_SPLINE_SURFACE_WITH_KNOTS((4,4),(3,3),(0.,0.00407947372412412),(0.,1.),
 .UNSPECIFIED.)
GEOMETRIC_REPRESENTATION_ITEM()
RATIONAL_B_SPLINE_SURFACE(((1.,0.453393847276564,1.),(1.,0.456475766016567,
1.),(1.,0.459447353892611,1.),(1.,0.462319489161104,1.)))
REPRESENTATION_ITEM('')
SURFACE()
);
#2610=(
BOUNDED_SURFACE()
B_SPLINE_SURFACE(3,2,((#168207,#168208,#168209),(#168210,#168211,#168212),
(#168213,#168214,#168215),(#168216,#168217,#168218),(#168219,#168220,#168221),
(#168222,#168223,#168224),(#168225,#168226,#168227),(#168228,#168229,#168230)),
 .UNSPECIFIED.,.F.,.F.,.F.)
B_SPLINE_SURFACE_WITH_KNOTS((4,2,2,4),(3,3),(0.,0.001434338214324,0.002868676428648,
0.005737352857296),(0.,1.),.UNSPECIFIED.)
GEOMETRIC_REPRESENTATION_ITEM()
RATIONAL_B_SPLINE_SURFACE(((1.,0.45339384727684,1.),(1.,0.47771228976057,
1.),(1.,0.501151853233145,1.),(1.,0.546461020466456,1.),(1.,0.568350660511087,
1.),(1.,0.632070189677047,1.),(1.,0.670684004768455,1.),(1.,0.707106781186548,
1.)))
REPRESENTATION_ITEM('')
SURFACE()
);
#2611=(
BOUNDED_SURFACE()
B_SPLINE_SURFACE(3,2,((#168399,#168400,#168401),(#168402,#168403,#168404),
(#168405,#168406,#168407),(#168408,#168409,#168410)),.UNSPECIFIED.,.F.,
 .F.,.F.)
B_SPLINE_SURFACE_WITH_KNOTS((4,4),(3,3),(-1.7347234759768E-18,0.0170848224870981),
(0.,1.),.UNSPECIFIED.)
GEOMETRIC_REPRESENTATION_ITEM()
RATIONAL_B_SPLINE_SURFACE(((1.,0.499602392377301,1.),(1.,0.510855798801923,
1.),(1.,0.520331406035946,1.),(1.,0.528679393385783,1.)))
REPRESENTATION_ITEM('')
SURFACE()
);
#2612=(
BOUNDED_SURFACE()
B_SPLINE_SURFACE(3,2,((#168436,#168437,#168438),(#168439,#168440,#168441),
(#168442,#168443,#168444),(#168445,#168446,#168447),(#168448,#168449,#168450),
(#168451,#168452,#168453),(#168454,#168455,#168456),(#168457,#168458,#168459),
(#168460,#168461,#168462),(#168463,#168464,#168465)),.UNSPECIFIED.,.F.,
 .F.,.F.)
B_SPLINE_SURFACE_WITH_KNOTS((4,2,2,2,4),(3,3),(-1.8702487475375E-18,0.00116432048255243,
0.00232864096510486,0.0034929614476573,0.00465728193020974),(0.,1.),
 .UNSPECIFIED.)
GEOMETRIC_REPRESENTATION_ITEM()
RATIONAL_B_SPLINE_SURFACE(((1.,0.499602392377304,1.),(1.,0.518836986211321,
1.),(1.,0.537549820773013,1.),(1.,0.574017039053458,1.),(1.,0.591773144780234,
1.),(1.,0.62647750773349,1.),(1.,0.643417219403868,1.),(1.,0.676030436791849,
1.),(1.,0.691791372953169,1.),(1.,0.707106781186548,1.)))
REPRESENTATION_ITEM('')
SURFACE()
);
#2613=(
BOUNDED_SURFACE()
B_SPLINE_SURFACE(3,2,((#168516,#168517,#168518),(#168519,#168520,#168521),
(#168522,#168523,#168524),(#168525,#168526,#168527),(#168528,#168529,#168530),
(#168531,#168532,#168533),(#168534,#168535,#168536),(#168537,#168538,#168539)),
 .UNSPECIFIED.,.F.,.F.,.F.)
B_SPLINE_SURFACE_WITH_KNOTS((4,2,2,4),(3,3),(-4.33680868994202E-19,0.00249252731595781,
0.00373879097393672,0.00498505463191562),(0.,1.),.UNSPECIFIED.)
GEOMETRIC_REPRESENTATION_ITEM()
RATIONAL_B_SPLINE_SURFACE(((1.,0.70710678118655,1.),(1.,0.739588972045703,
1.),(1.,0.769477992255324,1.),(1.,0.811447962923272,1.),(1.,0.825023851703587,
1.),(1.,0.850750710603259,1.),(1.,0.862945608551043,1.),(1.,0.874466916621005,
1.)))
REPRESENTATION_ITEM('')
SURFACE()
);
#2614=(
BOUNDED_SURFACE()
B_SPLINE_SURFACE(3,2,((#168555,#168556,#168557),(#168558,#168559,#168560),
(#168561,#168562,#168563),(#168564,#168565,#168566)),.UNSPECIFIED.,.F.,
 .F.,.F.)
B_SPLINE_SURFACE_WITH_KNOTS((4,4),(3,3),(0.,0.0135233968444947),(0.,1.),
 .UNSPECIFIED.)
GEOMETRIC_REPRESENTATION_ITEM()
RATIONAL_B_SPLINE_SURFACE(((1.,0.860139545375529,1.),(1.,0.864525021855929,
1.),(1.,0.869269442591942,1.),(1.,0.874466916621369,1.)))
REPRESENTATION_ITEM('')
SURFACE()
);
#2615=(
BOUNDED_SURFACE()
B_SPLINE_SURFACE(3,2,((#168573,#168574,#168575),(#168576,#168577,#168578),
(#168579,#168580,#168581),(#168582,#168583,#168584),(#168585,#168586,#168587),
(#168588,#168589,#168590)),.UNSPECIFIED.,.F.,.F.,.F.)
B_SPLINE_SURFACE_WITH_KNOTS((4,2,4),(3,3),(0.,0.000315675390911493,0.000631350781822986),
(0.,1.),.UNSPECIFIED.)
GEOMETRIC_REPRESENTATION_ITEM()
RATIONAL_B_SPLINE_SURFACE(((1.,0.860139545375527,1.),(1.,0.846673137247607,
1.),(1.,0.824923291377528,1.),(1.,0.771907958235216,1.),(1.,0.740773829846737,
1.),(1.,0.70710678118655,1.)))
REPRESENTATION_ITEM('')
SURFACE()
);
#2616=(
BOUNDED_SURFACE()
B_SPLINE_SURFACE(3,2,((#168713,#168714,#168715),(#168716,#168717,#168718),
(#168719,#168720,#168721),(#168722,#168723,#168724),(#168725,#168726,#168727),
(#168728,#168729,#168730)),.UNSPECIFIED.,.F.,.F.,.F.)
B_SPLINE_SURFACE_WITH_KNOTS((4,2,4),(3,3),(-6.4954414055628E-5,0.000324772070278169,
0.000714498554611972),(-0.000410438713922671,1.),.UNSPECIFIED.)
GEOMETRIC_REPRESENTATION_ITEM()
RATIONAL_B_SPLINE_SURFACE(((1.00025845542913,0.685147355296338,1.),(1.0002222617227,
0.729238842293541,1.),(1.00018785201525,0.771157046260518,1.),(1.00013161693134,
0.839663113063761,1.),(1.00010908866185,0.867107246289421,1.),(1.00009788969732,
0.880749921969343,1.)))
REPRESENTATION_ITEM('')
SURFACE()
);
#2617=(
BOUNDED_SURFACE()
B_SPLINE_SURFACE(3,2,((#168813,#168814,#168815),(#168816,#168817,#168818),
(#168819,#168820,#168821),(#168822,#168823,#168824)),.UNSPECIFIED.,.F.,
 .F.,.F.)
B_SPLINE_SURFACE_WITH_KNOTS((4,4),(3,3),(0.,0.00876509433037234),(0.,1.),
 .UNSPECIFIED.)
GEOMETRIC_REPRESENTATION_ITEM()
RATIONAL_B_SPLINE_SURFACE(((1.,0.882443751548025,1.),(1.,0.879078911067312,
1.),(1.,0.875892933141997,1.),(1.,0.872863017557589,1.)))
REPRESENTATION_ITEM('')
SURFACE()
);
#2618=(
BOUNDED_SURFACE()
B_SPLINE_SURFACE(3,2,((#168831,#168832,#168833),(#168834,#168835,#168836),
(#168837,#168838,#168839),(#168840,#168841,#168842),(#168843,#168844,#168845),
(#168846,#168847,#168848),(#168849,#168850,#168851),(#168852,#168853,#168854)),
 .UNSPECIFIED.,.F.,.F.,.F.)
B_SPLINE_SURFACE_WITH_KNOTS((4,2,2,4),(3,3),(-4.21496351932344E-5,0.00133214690895888,
0.00266429381791776,0.00537073727101886),(-0.000298701407012629,1.),
 .UNSPECIFIED.)
GEOMETRIC_REPRESENTATION_ITEM()
RATIONAL_B_SPLINE_SURFACE(((1.00006957344384,0.883540147100468,1.),(1.0000769064979,
0.871265256709866,1.),(1.00008468386698,0.858246621887947,1.),(1.00010084930836,
0.831187088519705,1.),(1.00010921077731,0.81719072165729,1.),(1.00013589350388,
0.772526173817441,1.),(1.00015516908062,0.740260546179961,1.),(1.00017599959926,
0.705392081983662,0.999999999999999)))
REPRESENTATION_ITEM('')
SURFACE()
);
#2619=(
BOUNDED_SURFACE()
B_SPLINE_SURFACE(3,2,((#168886,#168887,#168888),(#168889,#168890,#168891),
(#168892,#168893,#168894),(#168895,#168896,#168897),(#168898,#168899,#168900),
(#168901,#168902,#168903),(#168904,#168905,#168906),(#168907,#168908,#168909)),
 .UNSPECIFIED.,.F.,.F.,.F.)
B_SPLINE_SURFACE_WITH_KNOTS((4,2,2,4),(3,3),(0.,0.0026640399986995,0.00399605999804924,
0.00532807999739899),(0.,1.),.UNSPECIFIED.)
GEOMETRIC_REPRESENTATION_ITEM()
RATIONAL_B_SPLINE_SURFACE(((1.,0.707106781186548,1.),(1.,0.741415034329509,
1.),(1.,0.772836788298617,1.),(1.,0.816837673402558,1.),(1.,0.831036084533252,
1.),(1.,0.857840517676878,1.),(1.,0.87051456122688,1.),(1.,0.882443751548482,
1.)))
REPRESENTATION_ITEM('')
SURFACE()
);
#2620=(
BOUNDED_SURFACE()
B_SPLINE_SURFACE(3,2,((#168928,#168929,#168930),(#168931,#168932,#168933),
(#168934,#168935,#168936),(#168937,#168938,#168939)),.UNSPECIFIED.,.F.,
 .F.,.F.)
B_SPLINE_SURFACE_WITH_KNOTS((4,4),(3,3),(-3.46944695195361E-18,0.00904291806877092),
(0.,1.),.UNSPECIFIED.)
GEOMETRIC_REPRESENTATION_ITEM()
RATIONAL_B_SPLINE_SURFACE(((1.,0.872575378690133,1.),(1.,0.875691129720726,
1.),(1.,0.878972255663315,1.),(1.,0.882443751548002,1.)))
REPRESENTATION_ITEM('')
SURFACE()
);
#2621=(
BOUNDED_SURFACE()
B_SPLINE_SURFACE(3,2,((#168946,#168947,#168948),(#168949,#168950,#168951),
(#168952,#168953,#168954),(#168955,#168956,#168957),(#168958,#168959,#168960),
(#168961,#168962,#168963)),.UNSPECIFIED.,.F.,.F.,.F.)
B_SPLINE_SURFACE_WITH_KNOTS((4,2,4),(3,3),(-6.48856056667737E-5,0.000324428028333684,
0.000713741662334142),(-0.000106621799618699,1.),.UNSPECIFIED.)
GEOMETRIC_REPRESENTATION_ITEM()
RATIONAL_B_SPLINE_SURFACE(((1.00002551905035,0.880329114491097,1.),(1.00002834928183,
0.867056821704917,1.),(1.0000341546752,0.839832589011995,1.),(1.0000488152557,
0.771082199518792,1.),(1.00005760311273,0.729871785430903,1.),(1.00006718666931,
0.68492996016543,1.)))
REPRESENTATION_ITEM('')
SURFACE()
);
#2622=(
BOUNDED_SURFACE()
B_SPLINE_SURFACE(3,2,((#168986,#168987,#168988),(#168989,#168990,#168991),
(#168992,#168993,#168994),(#168995,#168996,#168997),(#168998,#168999,#169000),
(#169001,#169002,#169003),(#169004,#169005,#169006),(#169007,#169008,#169009),
(#169010,#169011,#169012),(#169013,#169014,#169015)),.UNSPECIFIED.,.F.,
 .F.,.F.)
B_SPLINE_SURFACE_WITH_KNOTS((4,2,2,2,4),(3,3),(3.1415926535898,3.53429173528852,
3.92699081698724,4.31968989868597,4.71238898038469),(0.,1.),
 .UNSPECIFIED.)
GEOMETRIC_REPRESENTATION_ITEM()
RATIONAL_B_SPLINE_SURFACE(((1.,0.754709580222772,1.),(1.,0.754714219730806,
1.),(1.,0.753512297096203,1.),(1.,0.748871927696591,1.),(1.,0.745429366938691,
1.),(1.,0.736738129296209,1.),(1.,0.73149075639733,1.),(1.,0.719894264862189,
1.),(1.,0.713550261851557,1.),(1.,0.707106781186548,1.)))
REPRESENTATION_ITEM('')
SURFACE()
);
#2623=(
BOUNDED_SURFACE()
B_SPLINE_SURFACE(3,2,((#169064,#169065,#169066),(#169067,#169068,#169069),
(#169070,#169071,#169072),(#169073,#169074,#169075),(#169076,#169077,#169078),
(#169079,#169080,#169081),(#169082,#169083,#169084),(#169085,#169086,#169087),
(#169088,#169089,#169090),(#169091,#169092,#169093)),.UNSPECIFIED.,.F.,
 .F.,.F.)
B_SPLINE_SURFACE_WITH_KNOTS((4,2,2,2,4),(3,3),(1.57066336187449,1.96349540849362,
2.35619449019234,2.74889357189107,3.1417256185102),(0.,1.00013296492041),
 .UNSPECIFIED.)
GEOMETRIC_REPRESENTATION_ITEM()
RATIONAL_B_SPLINE_SURFACE(((1.,0.707074379515197,1.00007789766363),(1.,
0.700631001612236,1.00007961115009),(1.,0.694096308749978,1.00008134891992),
(1.,0.681861139766877,1.00008460261646),(1.,0.676166101239942,1.00008611709715),
(1.,0.666571715833326,1.00008866853053),(1.,0.662679222605256,1.00008970366064),
(1.,0.657396767036593,1.00009110842321),(1.,0.656004520314252,1.00009147866316),
(1.,0.656013305345755,1.00009147632695)))
REPRESENTATION_ITEM('')
SURFACE()
);
#2624=(
BOUNDED_SURFACE()
B_SPLINE_SURFACE(3,2,((#169110,#169111,#169112),(#169113,#169114,#169115),
(#169116,#169117,#169118),(#169119,#169120,#169121),(#169122,#169123,#169124),
(#169125,#169126,#169127),(#169128,#169129,#169130),(#169131,#169132,#169133),
(#169134,#169135,#169136),(#169137,#169138,#169139)),.UNSPECIFIED.,.F.,
 .F.,.F.)
B_SPLINE_SURFACE_WITH_KNOTS((4,2,2,2,4),(3,3),(0.,0.000158019212117338,
0.000316038424234677,0.000474057636352015,0.000632076848469353),(-0.000659009817274179,
1.),.UNSPECIFIED.)
GEOMETRIC_REPRESENTATION_ITEM()
RATIONAL_B_SPLINE_SURFACE(((1.00038629341672,0.706913761679937,1.),(1.00040876016389,
0.689867925196359,1.),(1.00043160206942,0.672537450804892,1.),(1.00047822635013,
0.637162954487827,1.),(1.000502398717,0.618823040396089,1.),(1.00054910501744,
0.583386314556222,1.),(1.0005717799679,0.566182511309068,1.),(1.00061451793483,
0.533756615818148,1.),(1.00063376129073,0.519156411542439,1.),(1.0006490837683,
0.507531032707861,1.)))
REPRESENTATION_ITEM('')
SURFACE()
);
#2625=(
BOUNDED_SURFACE()
B_SPLINE_SURFACE(3,2,((#169161,#169162,#169163),(#169164,#169165,#169166),
(#169167,#169168,#169169),(#169170,#169171,#169172)),.UNSPECIFIED.,.F.,
 .F.,.F.)
B_SPLINE_SURFACE_WITH_KNOTS((4,4),(3,3),(0.,0.01284355850178),(0.,1.),
 .UNSPECIFIED.)
GEOMETRIC_REPRESENTATION_ITEM()
RATIONAL_B_SPLINE_SURFACE(((1.,0.484030052331127,1.),(1.,0.492910462848522,
1.),(1.,0.500753390328389,1.),(1.,0.507855360856573,1.)))
REPRESENTATION_ITEM('')
SURFACE()
);
#2626=(
BOUNDED_SURFACE()
B_SPLINE_SURFACE(3,2,((#169179,#169180,#169181),(#169182,#169183,#169184),
(#169185,#169186,#169187),(#169188,#169189,#169190),(#169191,#169192,#169193),
(#169194,#169195,#169196),(#169197,#169198,#169199),(#169200,#169201,#169202),
(#169203,#169204,#169205),(#169206,#169207,#169208)),.UNSPECIFIED.,.F.,
 .F.,.F.)
B_SPLINE_SURFACE_WITH_KNOTS((4,2,2,2,4),(3,3),(-4.33680868994201E-18,0.00125260629929845,
0.00250521259859689,0.00375781889789535,0.0050104251971938),(0.,1.),
 .UNSPECIFIED.)
GEOMETRIC_REPRESENTATION_ITEM()
RATIONAL_B_SPLINE_SURFACE(((1.,0.484030052331112,1.),(1.,0.504928485114276,
1.),(1.,0.525198247435633,1.),(1.,0.564597723285694,1.),(1.,0.583730152224629,
1.),(1.,0.62105465867689,1.),(1.,0.639160091266653,1.),(1.,0.67398655458045,
1.),(1.,0.690790819130117,1.),(1.,0.707106781186548,1.)))
REPRESENTATION_ITEM('')
SURFACE()
);
#2627=(
BOUNDED_SURFACE()
B_SPLINE_SURFACE(3,2,((#169231,#169232,#169233),(#169234,#169235,#169236),
(#169237,#169238,#169239),(#169240,#169241,#169242),(#169243,#169244,#169245),
(#169246,#169247,#169248),(#169249,#169250,#169251),(#169252,#169253,#169254)),
 .UNSPECIFIED.,.F.,.F.,.F.)
B_SPLINE_SURFACE_WITH_KNOTS((4,2,2,4),(3,3),(-5.42101086242752E-20,0.00250485829616721,
0.00375728744425081,0.00500971659233441),(0.,1.),.UNSPECIFIED.)
GEOMETRIC_REPRESENTATION_ITEM()
RATIONAL_B_SPLINE_SURFACE(((1.,0.70710678118722,1.),(1.,0.674452105060394,
1.),(1.,0.640073400404409,1.),(1.,0.584341050151977,1.),(1.,0.564951135845581,
1.),(1.,0.525261922605914,1.),(1.,0.504912110655119,1.),(1.,0.484030052331115,
1.)))
REPRESENTATION_ITEM('')
SURFACE()
);
#2628=(
BOUNDED_SURFACE()
B_SPLINE_SURFACE(3,2,((#169270,#169271,#169272),(#169273,#169274,#169275),
(#169276,#169277,#169278),(#169279,#169280,#169281)),.UNSPECIFIED.,.F.,
 .F.,.F.)
B_SPLINE_SURFACE_WITH_KNOTS((4,4),(3,3),(0.,0.0125680158145827),(0.,1.),
 .UNSPECIFIED.)
GEOMETRIC_REPRESENTATION_ITEM()
RATIONAL_B_SPLINE_SURFACE(((1.,0.507397370006812,1.),(1.,0.500416139715127,
1.),(1.,0.49272006913241,1.),(1.,0.484030052331115,1.)))
REPRESENTATION_ITEM('')
SURFACE()
);
#2629=(
BOUNDED_SURFACE()
B_SPLINE_SURFACE(3,2,((#169311,#169312,#169313),(#169314,#169315,#169316),
(#169317,#169318,#169319),(#169320,#169321,#169322),(#169323,#169324,#169325),
(#169326,#169327,#169328),(#169329,#169330,#169331),(#169332,#169333,#169334)),
 .UNSPECIFIED.,.F.,.F.,.F.)
B_SPLINE_SURFACE_WITH_KNOTS((4,2,2,4),(3,3),(-1.5368565794982E-17,0.000158339556725866,
0.000316679113451747,0.000633358226903509),(0.,1.),.UNSPECIFIED.)
GEOMETRIC_REPRESENTATION_ITEM()
RATIONAL_B_SPLINE_SURFACE(((1.,0.507397370006824,1.),(1.,0.519070630879541,
1.),(1.,0.533426892711081,1.),(1.,0.565658432465259,1.),(1.,0.583100719918817,
1.),(1.,0.636529920575075,1.),(1.,0.673198940992506,1.),(1.,0.707106781186548,
1.)))
REPRESENTATION_ITEM('')
SURFACE()
);
#2630=(
BOUNDED_SURFACE()
B_SPLINE_SURFACE(3,2,((#169453,#169454,#169455),(#169456,#169457,#169458),
(#169459,#169460,#169461),(#169462,#169463,#169464)),.UNSPECIFIED.,.F.,
 .F.,.F.)
B_SPLINE_SURFACE_WITH_KNOTS((4,4),(3,3),(-2.08166817117217E-17,0.0203430832871546),
(0.,1.),.UNSPECIFIED.)
GEOMETRIC_REPRESENTATION_ITEM()
RATIONAL_B_SPLINE_SURFACE(((1.,0.855596390789699,1.),(1.,0.848090845809161,
1.),(1.,0.841665513049531,1.),(1.,0.835963592435998,1.)))
REPRESENTATION_ITEM('')
SURFACE()
);
#2631=(
BOUNDED_SURFACE()
B_SPLINE_SURFACE(3,2,((#169473,#169474,#169475),(#169476,#169477,#169478),
(#169479,#169480,#169481),(#169482,#169483,#169484),(#169485,#169486,#169487),
(#169488,#169489,#169490),(#169491,#169492,#169493),(#169494,#169495,#169496)),
 .UNSPECIFIED.,.F.,.F.,.F.)
B_SPLINE_SURFACE_WITH_KNOTS((4,2,2,4),(3,3),(-0.000280270643381287,0.00213290337237644,
0.00319935505856466,0.00454607738813407),(-0.00139944814386632,1.),
 .UNSPECIFIED.)
GEOMETRIC_REPRESENTATION_ITEM()
RATIONAL_B_SPLINE_SURFACE(((1.0003817605577,0.863603178378214,1.),(1.00044695755931,
0.840309352917159,1.),(1.00051853483077,0.814735961086389,1.),(1.00063212358804,
0.774152550486465,1.),(1.00066847254068,0.76116566247594,1.),(1.00075281158742,
0.731032696452739,1.),(1.00080157579018,0.713610042037807,1.),(1.00085238418929,
0.695457029605283,1.)))
REPRESENTATION_ITEM('')
SURFACE()
);
#2632=(
BOUNDED_SURFACE()
B_SPLINE_SURFACE(3,2,((#169516,#169517,#169518),(#169519,#169520,#169521),
(#169522,#169523,#169524),(#169525,#169526,#169527),(#169528,#169529,#169530),
(#169531,#169532,#169533)),.UNSPECIFIED.,.F.,.F.,.F.)
B_SPLINE_SURFACE_WITH_KNOTS((4,2,4),(3,3),(0.,0.00213206083322637,0.00426412166645274),
(0.,1.),.UNSPECIFIED.)
GEOMETRIC_REPRESENTATION_ITEM()
RATIONAL_B_SPLINE_SURFACE(((1.,0.707106781186545,1.),(1.,0.735348751818402,
1.),(1.,0.761643947187706,1.),(1.,0.811236415877723,1.),(1.,0.834679252508647,
1.),(1.,0.855596390789698,1.)))
REPRESENTATION_ITEM('')
SURFACE()
);
#2633=(
BOUNDED_SURFACE()
B_SPLINE_SURFACE(3,2,((#169558,#169559,#169560),(#169561,#169562,#169563),
(#169564,#169565,#169566),(#169567,#169568,#169569)),.UNSPECIFIED.,.F.,
 .F.,.F.)
B_SPLINE_SURFACE_WITH_KNOTS((4,4),(3,3),(0.,0.0206148669995797),(0.,1.),
 .UNSPECIFIED.)
GEOMETRIC_REPRESENTATION_ITEM()
RATIONAL_B_SPLINE_SURFACE(((1.,0.835735574810025,1.),(1.,0.841493793210698,
1.),(1.,0.847990686938055,1.),(1.,0.855596390789697,1.)))
REPRESENTATION_ITEM('')
SURFACE()
);
#2634=(
BOUNDED_SURFACE()
B_SPLINE_SURFACE(3,2,((#169576,#169577,#169578),(#169579,#169580,#169581),
(#169582,#169583,#169584),(#169585,#169586,#169587)),.UNSPECIFIED.,.F.,
 .F.,.F.)
B_SPLINE_SURFACE_WITH_KNOTS((4,4),(3,3),(0.,0.000103369667661675),(0.,1.),
 .UNSPECIFIED.)
GEOMETRIC_REPRESENTATION_ITEM()
RATIONAL_B_SPLINE_SURFACE(((1.,0.835735574810027,1.),(1.,0.831946521393585,
1.),(1.,0.827395718030991,1.),(1.,0.822092089912784,1.)))
REPRESENTATION_ITEM('')
SURFACE()
);
#2635=(
BOUNDED_SURFACE()
B_SPLINE_SURFACE(3,2,((#169594,#169595,#169596),(#169597,#169598,#169599),
(#169600,#169601,#169602),(#169603,#169604,#169605),(#169606,#169607,#169608),
(#169609,#169610,#169611)),.UNSPECIFIED.,.F.,.F.,.F.)
B_SPLINE_SURFACE_WITH_KNOTS((4,2,4),(3,3),(0.,0.000488238270881924,0.000976476541763847),
(0.,1.),.UNSPECIFIED.)
GEOMETRIC_REPRESENTATION_ITEM()
RATIONAL_B_SPLINE_SURFACE(((1.,0.807089511457258,1.),(1.,0.816558112905035,
1.),(1.,0.821286794224823,1.),(1.,0.825205555407875,1.),(1.,0.824318362071196,
1.),(1.,0.822092089912778,1.)))
REPRESENTATION_ITEM('')
SURFACE()
);
#2636=(
BOUNDED_SURFACE()
B_SPLINE_SURFACE(3,2,((#169662,#169663,#169664),(#169665,#169666,#169667),
(#169668,#169669,#169670),(#169671,#169672,#169673)),.UNSPECIFIED.,.F.,
 .F.,.F.)
B_SPLINE_SURFACE_WITH_KNOTS((4,4),(3,3),(-2.2779825405953E-5,0.000250578079469443),
(-9.62977912475538E-5,1.),.UNSPECIFIED.)
GEOMETRIC_REPRESENTATION_ITEM()
RATIONAL_B_SPLINE_SURFACE(((1.00003939441504,0.795455251195445,1.),(1.00003575677157,
0.814342722165374,1.),(1.00003292074913,0.829067994671566,1.),(1.00003112533526,
0.838390191208877,1.)))
REPRESENTATION_ITEM('')
SURFACE()
);
#2637=(
BOUNDED_SURFACE()
B_SPLINE_SURFACE(3,2,((#169699,#169700,#169701),(#169702,#169703,#169704),
(#169705,#169706,#169707),(#169708,#169709,#169710),(#169711,#169712,#169713),
(#169714,#169715,#169716),(#169717,#169718,#169719),(#169720,#169721,#169722),
(#169723,#169724,#169725),(#169726,#169727,#169728)),.UNSPECIFIED.,.F.,
 .F.,.F.)
B_SPLINE_SURFACE_WITH_KNOTS((4,2,2,2,4),(3,3),(3.1415926535898,3.53429173528852,
3.92699081698724,4.31968989868597,4.71238898038469),(0.,1.),
 .UNSPECIFIED.)
GEOMETRIC_REPRESENTATION_ITEM()
RATIONAL_B_SPLINE_SURFACE(((1.,0.754709580222767,1.),(1.,0.754714219730801,
1.),(1.,0.753512297096199,1.),(1.,0.748871927696587,1.),(1.,0.745429366938708,
1.),(1.,0.736738129296182,1.),(1.,0.731490756397336,1.),(1.,0.719894264862173,
1.),(1.,0.71355026185156,1.),(1.,0.707106781186543,1.)))
REPRESENTATION_ITEM('')
SURFACE()
);
#2638=(
BOUNDED_SURFACE()
B_SPLINE_SURFACE(3,2,((#169756,#169757,#169758),(#169759,#169760,#169761),
(#169762,#169763,#169764),(#169765,#169766,#169767),(#169768,#169769,#169770),
(#169771,#169772,#169773),(#169774,#169775,#169776),(#169777,#169778,#169779),
(#169780,#169781,#169782),(#169783,#169784,#169785)),.UNSPECIFIED.,.F.,
 .F.,.F.)
B_SPLINE_SURFACE_WITH_KNOTS((4,2,2,2,4),(3,3),(0.00116892975483546,0.00173273620432841,
0.00229654265382136,0.0028603491033143,0.00342415555280725),(-8.73672651017134E-5,
1.),.UNSPECIFIED.)
GEOMETRIC_REPRESENTATION_ITEM()
RATIONAL_B_SPLINE_SURFACE(((1.00005118303032,0.707081191907057,1.),(1.00004250803405,
0.756727911750157,1.),(1.00003576403202,0.795323614743189,1.),(1.00002660678148,
0.847730260009883,1.),(1.00002422236722,0.86137618483429,1.),(1.00002421067412,
0.861443104051582,1.),(1.00002658556867,0.847851660205465,1.),(1.00003574715401,
0.795420207077646,1.),(1.00004250128304,0.756766547571618,1.),(1.00005118303032,
0.707081191907057,1.)))
REPRESENTATION_ITEM('')
SURFACE()
);
#2639=(
BOUNDED_SURFACE()
B_SPLINE_SURFACE(3,2,((#169873,#169874,#169875),(#169876,#169877,#169878),
(#169879,#169880,#169881),(#169882,#169883,#169884)),.UNSPECIFIED.,.F.,
 .F.,.F.)
B_SPLINE_SURFACE_WITH_KNOTS((4,4),(3,3),(-6.9931040125315E-18,0.000203650363220118),
(0.,1.),.UNSPECIFIED.)
GEOMETRIC_REPRESENTATION_ITEM()
RATIONAL_B_SPLINE_SURFACE(((1.,0.707106781186548,1.),(1.,0.683088481213104,
1.),(1.,0.658130799535722,1.),(1.,0.631879234223615,1.)))
REPRESENTATION_ITEM('')
SURFACE()
);
#2640=(
BOUNDED_SURFACE()
B_SPLINE_SURFACE(3,2,((#169891,#169892,#169893),(#169894,#169895,#169896),
(#169897,#169898,#169899),(#169900,#169901,#169902),(#169903,#169904,#169905),
(#169906,#169907,#169908)),.UNSPECIFIED.,.F.,.F.,.F.)
B_SPLINE_SURFACE_WITH_KNOTS((4,2,4),(3,3),(0.00191966951912585,0.00217079434687949,
0.00242191917463315),(0.,1.),.UNSPECIFIED.)
GEOMETRIC_REPRESENTATION_ITEM()
RATIONAL_B_SPLINE_SURFACE(((1.,0.460674285272032,1.),(1.,0.480581991146479,
1.),(1.,0.508992468088204,1.),(1.,0.568988175192947,1.),(1.,0.601196374063936,
1.),(1.,0.631879234223659,1.)))
REPRESENTATION_ITEM('')
SURFACE()
);
#2641=(
BOUNDED_SURFACE()
B_SPLINE_SURFACE(3,2,((#169936,#169937,#169938),(#169939,#169940,#169941),
(#169942,#169943,#169944),(#169945,#169946,#169947),(#169948,#169949,#169950),
(#169951,#169952,#169953),(#169954,#169955,#169956),(#169957,#169958,#169959),
(#169960,#169961,#169962),(#169963,#169964,#169965)),.UNSPECIFIED.,.F.,
 .F.,.F.)
B_SPLINE_SURFACE_WITH_KNOTS((4,2,2,2,4),(3,3),(0.,0.00140990970253443,0.00281981940506887,
0.0042297291076033,0.00563963881013773),(0.,1.),.UNSPECIFIED.)
GEOMETRIC_REPRESENTATION_ITEM()
RATIONAL_B_SPLINE_SURFACE(((1.,0.460674285271834,1.),(1.,0.484432802265468,
1.),(1.,0.507218999550826,1.),(1.,0.55117184532966,1.),(1.,0.572342624738,
1.),(1.,0.613417108469756,1.),(1.,0.633191153021656,1.),(1.,0.671152451591827,
1.),(1.,0.689411349760462,1.),(1.,0.707106781186548,1.)))
REPRESENTATION_ITEM('')
SURFACE()
);
#2642=(
BOUNDED_SURFACE()
B_SPLINE_SURFACE(3,2,((#169988,#169989,#169990),(#169991,#169992,#169993),
(#169994,#169995,#169996),(#169997,#169998,#169999),(#170000,#170001,#170002),
(#170003,#170004,#170005),(#170006,#170007,#170008),(#170009,#170010,#170011)),
 .UNSPECIFIED.,.F.,.F.,.F.)
B_SPLINE_SURFACE_WITH_KNOTS((4,2,2,4),(3,3),(0.,0.00267885639561352,0.00401828459342028,
0.00535771279122705),(0.,1.),.UNSPECIFIED.)
GEOMETRIC_REPRESENTATION_ITEM()
RATIONAL_B_SPLINE_SURFACE(((1.,0.707106781186871,1.),(1.,0.673473842386368,
1.),(1.,0.638019211186003,1.),(1.,0.580269195298477,1.),(1.,0.560144321783745,
1.),(1.,0.518526712842715,1.),(1.,0.497044145980004,1.),(1.,0.474759570947005,
1.)))
REPRESENTATION_ITEM('')
SURFACE()
);
#2643=(
BOUNDED_SURFACE()
B_SPLINE_SURFACE(3,2,((#170027,#170028,#170029),(#170030,#170031,#170032),
(#170033,#170034,#170035),(#170036,#170037,#170038),(#170039,#170040,#170041),
(#170042,#170043,#170044),(#170045,#170046,#170047),(#170048,#170049,#170050),
(#170051,#170052,#170053),(#170054,#170055,#170056)),.UNSPECIFIED.,.F.,
 .F.,.F.)
B_SPLINE_SURFACE_WITH_KNOTS((4,2,2,2,4),(3,3),(0.,0.000174105410412539,
0.000348210820825077,0.000522316231237617,0.000696421641650155),(-0.000483059379797502,
1.),.UNSPECIFIED.)
GEOMETRIC_REPRESENTATION_ITEM()
RATIONAL_B_SPLINE_SURFACE(((1.0005076897577,0.474505848630797,1.),(1.000495670555,
0.486946557988912,1.),(1.0004800812597,0.503082561094009,1.),(1.00044417434065,
0.540248715550885,1.),(1.00042474790251,0.560356427930957,1.),(1.00038427712958,
0.602246488055232,1.),(1.00036396770606,0.623268151612906,1.),(1.00032333802193,
0.665322695866086,1.),(1.00030290014099,0.686477321779519,1.),(1.00028310632439,
0.706965296369921,1.)))
REPRESENTATION_ITEM('')
SURFACE()
);
#2644=(
BOUNDED_SURFACE()
B_SPLINE_SURFACE(3,2,((#170127,#170128,#170129),(#170130,#170131,#170132),
(#170133,#170134,#170135),(#170136,#170137,#170138),(#170139,#170140,#170141),
(#170142,#170143,#170144),(#170145,#170146,#170147),(#170148,#170149,#170150),
(#170151,#170152,#170153),(#170154,#170155,#170156)),.UNSPECIFIED.,.F.,
 .F.,.F.)
B_SPLINE_SURFACE_WITH_KNOTS((4,2,2,2,4),(3,3),(1.57066336187483,1.96349540849362,
2.35619449019234,2.74889357189107,3.14172561850986),(0.,1.00013296492006),
 .UNSPECIFIED.)
GEOMETRIC_REPRESENTATION_ITEM()
RATIONAL_B_SPLINE_SURFACE(((1.,0.707074379515281,1.00007789766343),(1.,
0.700631001612311,1.00007961114988),(1.,0.6940963087501,1.00008134891971),
(1.,0.681861139766965,1.00008460261624),(1.,0.676166101240053,1.00008611709693),
(1.,0.666571715833441,1.0000886685303),(1.,0.662679222605372,1.00008970366041),
(1.,0.657396767036713,1.00009110842297),(1.,0.656004520314383,1.00009147866292),
(1.,0.656013305345874,1.00009147632672)))
REPRESENTATION_ITEM('')
SURFACE()
);
#2645=(
BOUNDED_SURFACE()
B_SPLINE_SURFACE(3,2,((#170183,#170184,#170185),(#170186,#170187,#170188),
(#170189,#170190,#170191),(#170192,#170193,#170194)),.UNSPECIFIED.,.F.,
 .F.,.F.)
B_SPLINE_SURFACE_WITH_KNOTS((4,4),(3,3),(0.,0.000433489251034108),(0.,1.),
 .UNSPECIFIED.)
GEOMETRIC_REPRESENTATION_ITEM()
RATIONAL_B_SPLINE_SURFACE(((1.,0.843391445812886,1.),(1.,0.83955525384858,
1.),(1.,0.835558949072738,1.),(1.,0.831408647420015,1.)))
REPRESENTATION_ITEM('')
SURFACE()
);
#2646=(
BOUNDED_SURFACE()
B_SPLINE_SURFACE(3,2,((#170199,#170200,#170201),(#170202,#170203,#170204),
(#170205,#170206,#170207),(#170208,#170209,#170210),(#170211,#170212,#170213),
(#170214,#170215,#170216)),.UNSPECIFIED.,.F.,.F.,.F.)
B_SPLINE_SURFACE_WITH_KNOTS((4,2,4),(3,3),(-6.93889390390723E-18,0.0148367096635454,
0.0296734193270908),(0.,1.),.UNSPECIFIED.)
GEOMETRIC_REPRESENTATION_ITEM()
RATIONAL_B_SPLINE_SURFACE(((1.,0.524787419125867,1.),(1.,0.534113414550019,
1.),(1.,0.542054608658765,1.),(1.,0.556098130983184,1.),(1.,0.562195863398439,
1.),(1.,0.56767185832395,1.)))
REPRESENTATION_ITEM('')
SURFACE()
);
#2647=(
BOUNDED_SURFACE()
B_SPLINE_SURFACE(3,2,((#170228,#170229,#170230),(#170231,#170232,#170233),
(#170234,#170235,#170236),(#170237,#170238,#170239),(#170240,#170241,#170242),
(#170243,#170244,#170245)),.UNSPECIFIED.,.F.,.F.,.F.)
B_SPLINE_SURFACE_WITH_KNOTS((4,2,4),(3,3),(-0.000210164559996447,0.00205623335330194,
0.00432263126660034),(-0.000445187292128403,1.),.UNSPECIFIED.)
GEOMETRIC_REPRESENTATION_ITEM()
RATIONAL_B_SPLINE_SURFACE(((1.0004324500486,0.514305488672343,1.),(1.00039941933963,
0.551403031161431,1.),(1.00036812081892,0.58655511350849,1.),(1.00030827208983,
0.653772585966662,1.),(1.00027973535443,0.68582284425181,1.),(1.00025355847735,
0.71522269184906,1.)))
REPRESENTATION_ITEM('')
SURFACE()
);
#2648=(
BOUNDED_SURFACE()
B_SPLINE_SURFACE(3,2,((#170277,#170278,#170279),(#170280,#170281,#170282),
(#170283,#170284,#170285),(#170286,#170287,#170288),(#170289,#170290,#170291),
(#170292,#170293,#170294)),.UNSPECIFIED.,.F.,.F.,.F.)
B_SPLINE_SURFACE_WITH_KNOTS((4,2,4),(3,3),(0.,0.002055311285568,0.00411062257113599),
(0.,1.),.UNSPECIFIED.)
GEOMETRIC_REPRESENTATION_ITEM()
RATIONAL_B_SPLINE_SURFACE(((1.,0.707106781186549,1.),(1.,0.67983601545864,
1.),(1.,0.651283059470391,1.),(1.,0.590515772030266,1.),(1.,0.55801180255865,
1.),(1.,0.524787419125864,1.)))
REPRESENTATION_ITEM('')
SURFACE()
);
#2649=(
BOUNDED_SURFACE()
B_SPLINE_SURFACE(3,2,((#170376,#170377,#170378),(#170379,#170380,#170381),
(#170382,#170383,#170384),(#170385,#170386,#170387)),.UNSPECIFIED.,.F.,
 .F.,.F.)
B_SPLINE_SURFACE_WITH_KNOTS((4,4),(3,3),(-3.67928601881599E-5,0.000690322634258718),
(-3.67928601881599E-5,1.),.UNSPECIFIED.)
GEOMETRIC_REPRESENTATION_ITEM()
RATIONAL_B_SPLINE_SURFACE(((1.00003168318678,0.569438382609689,1.),(1.00003256820151,
0.557411392496539,1.),(1.00003304023254,0.550996682929833,1.),(1.0000329877132,
0.551710399363681,1.)))
REPRESENTATION_ITEM('')
SURFACE()
);
#2650=(
BOUNDED_SURFACE()
B_SPLINE_SURFACE(3,2,((#170389,#170390,#170391),(#170392,#170393,#170394),
(#170395,#170396,#170397),(#170398,#170399,#170400),(#170401,#170402,#170403),
(#170404,#170405,#170406)),.UNSPECIFIED.,.F.,.F.,.F.)
B_SPLINE_SURFACE_WITH_KNOTS((4,2,4),(3,3),(-3.37037386498138E-5,0.0147014688781887,
0.0294366414950272),(0.,1.00003370373865),.UNSPECIFIED.)
GEOMETRIC_REPRESENTATION_ITEM()
RATIONAL_B_SPLINE_SURFACE(((1.,0.567394857543477,1.00002916082132),(1.,
0.561935737478507,1.00002952880683),(1.,0.555859760262213,1.00002993837313),
(1.,0.541878051053617,1.00003088084487),(1.,0.533976759333239,1.00003141345102),
(1.,0.524707821662759,1.00003203824672)))
REPRESENTATION_ITEM('')
SURFACE()
);
#2651=(
BOUNDED_SURFACE()
B_SPLINE_SURFACE(3,2,((#170433,#170434,#170435),(#170436,#170437,#170438),
(#170439,#170440,#170441),(#170442,#170443,#170444),(#170445,#170446,#170447),
(#170448,#170449,#170450)),.UNSPECIFIED.,.F.,.F.,.F.)
B_SPLINE_SURFACE_WITH_KNOTS((4,2,4),(3,3),(0.312244141975826,0.317485429411984,
0.322726716848141),(0.,1.),.UNSPECIFIED.)
GEOMETRIC_REPRESENTATION_ITEM()
RATIONAL_B_SPLINE_SURFACE(((1.,0.945205509755643,1.),(1.,0.94765942841632,
1.),(1.,0.950143082313928,1.),(1.,0.955101624050304,1.),(1.,0.957550590969702,
1.),(1.,0.959916006973269,1.)))
REPRESENTATION_ITEM('')
SURFACE()
);
#2652=(
BOUNDED_SURFACE()
B_SPLINE_SURFACE(3,2,((#170550,#170551,#170552),(#170553,#170554,#170555),
(#170556,#170557,#170558),(#170559,#170560,#170561),(#170562,#170563,#170564),
(#170565,#170566,#170567)),.UNSPECIFIED.,.F.,.F.,.F.)
B_SPLINE_SURFACE_WITH_KNOTS((4,2,4),(3,3),(0.,0.00166463949867057,0.00332927899734113),
(0.,1.),.UNSPECIFIED.)
GEOMETRIC_REPRESENTATION_ITEM()
RATIONAL_B_SPLINE_SURFACE(((1.,0.824689321081979,1.),(1.,0.807273117786527,
1.),(1.,0.78876985537206,1.),(1.,0.749461319834452,1.),(1.,0.728524445804063,
1.),(1.,0.707106781186548,1.)))
REPRESENTATION_ITEM('')
SURFACE()
);
#2653=(
BOUNDED_SURFACE()
B_SPLINE_SURFACE(3,2,((#170584,#170585,#170586),(#170587,#170588,#170589),
(#170590,#170591,#170592),(#170593,#170594,#170595),(#170596,#170597,#170598),
(#170599,#170600,#170601)),.UNSPECIFIED.,.F.,.F.,.F.)
B_SPLINE_SURFACE_WITH_KNOTS((4,2,4),(3,3),(0.,0.0016638050806964,0.0033276101613928),
(0.,1.),.UNSPECIFIED.)
GEOMETRIC_REPRESENTATION_ITEM()
RATIONAL_B_SPLINE_SURFACE(((1.,0.707106781186548,1.),(1.,0.728604788113201,
1.),(1.,0.749094258011124,1.),(1.,0.788367019884298,1.),(1.,0.807290696029469,
1.),(1.,0.824689321081979,1.)))
REPRESENTATION_ITEM('')
SURFACE()
);
#2654=(
BOUNDED_SURFACE()
B_SPLINE_SURFACE(3,2,((#170620,#170621,#170622),(#170623,#170624,#170625),
(#170626,#170627,#170628),(#170629,#170630,#170631),(#170632,#170633,#170634),
(#170635,#170636,#170637)),.UNSPECIFIED.,.F.,.F.,.F.)
B_SPLINE_SURFACE_WITH_KNOTS((4,2,4),(3,3),(0.,0.0179426259581151,0.0358852519162302),
(0.,1.),.UNSPECIFIED.)
GEOMETRIC_REPRESENTATION_ITEM()
RATIONAL_B_SPLINE_SURFACE(((1.,0.796398016704685,1.),(1.,0.799989941027341,
1.),(1.,0.80399801610487,1.),(1.,0.81325769888663,1.),(1.,0.81850629826423,
1.),(1.,0.824689321081979,1.)))
REPRESENTATION_ITEM('')
SURFACE()
);
#2655=(
BOUNDED_SURFACE()
B_SPLINE_SURFACE(3,2,((#170647,#170648,#170649),(#170650,#170651,#170652),
(#170653,#170654,#170655),(#170656,#170657,#170658)),.UNSPECIFIED.,.F.,
 .F.,.F.)
B_SPLINE_SURFACE_WITH_KNOTS((4,4),(3,3),(-6.51868391715497E-5,0.000717055230887523),
(-0.00014173624593116,1.),.UNSPECIFIED.)
GEOMETRIC_REPRESENTATION_ITEM()
RATIONAL_B_SPLINE_SURFACE(((1.0000553523189,0.804734778555401,1.),(1.00005516270673,
0.805403669437731,1.),(1.00005612596714,0.802005595787349,1.),(1.00005822477713,
0.794601667527954,1.)))
REPRESENTATION_ITEM('')
SURFACE()
);
#2656=(
BOUNDED_SURFACE()
B_SPLINE_SURFACE(3,2,((#170677,#170678,#170679),(#170680,#170681,#170682),
(#170683,#170684,#170685),(#170686,#170687,#170688),(#170689,#170690,#170691),
(#170692,#170693,#170694)),.UNSPECIFIED.,.F.,.F.,.F.)
B_SPLINE_SURFACE_WITH_KNOTS((4,2,4),(3,3),(0.,0.0178083890192188,0.0356167780384377),
(0.,1.),.UNSPECIFIED.)
GEOMETRIC_REPRESENTATION_ITEM()
RATIONAL_B_SPLINE_SURFACE(((1.,0.824689321081978,1.),(1.,0.818552442915159,
1.),(1.,0.813336414682689,1.),(1.,0.80412734431217,1.),(1.,0.800137214821899,
1.),(1.,0.796559406694623,1.)))
REPRESENTATION_ITEM('')
SURFACE()
);
#2657=(
BOUNDED_SURFACE()
B_SPLINE_SURFACE(3,2,((#170763,#170764,#170765),(#170766,#170767,#170768),
(#170769,#170770,#170771),(#170772,#170773,#170774)),.UNSPECIFIED.,.F.,
 .F.,.F.)
B_SPLINE_SURFACE_WITH_KNOTS((4,4),(3,3),(-6.51391992791641E-5,0.00071653119207077),
(-0.000129157869248124,1.),.UNSPECIFIED.)
GEOMETRIC_REPRESENTATION_ITEM()
RATIONAL_B_SPLINE_SURFACE(((1.00009755078865,0.622358323103109,1.),(1.00009962867019,
0.614314362823106,1.),(1.00010065362943,0.610346508423656,1.),(1.00010045435892,
0.611117930705948,1.)))
REPRESENTATION_ITEM('')
SURFACE()
);
#2658=(
BOUNDED_SURFACE()
B_SPLINE_SURFACE(3,2,((#170778,#170779,#170780),(#170781,#170782,#170783),
(#170784,#170785,#170786),(#170787,#170788,#170789),(#170790,#170791,#170792),
(#170793,#170794,#170795)),.UNSPECIFIED.,.F.,.F.,.F.)
B_SPLINE_SURFACE_WITH_KNOTS((4,2,4),(3,3),(0.,0.0190876722191456,0.0381753444382913),
(0.,1.),.UNSPECIFIED.)
GEOMETRIC_REPRESENTATION_ITEM()
RATIONAL_B_SPLINE_SURFACE(((1.,0.584878694958869,1.),(1.,0.593227971935905,
1.),(1.,0.599946751815832,1.),(1.,0.611471310523657,1.),(1.,0.616266665820404,
1.),(1.,0.620481653466,1.)))
REPRESENTATION_ITEM('')
SURFACE()
);
#2659=(
BOUNDED_SURFACE()
B_SPLINE_SURFACE(3,2,((#170805,#170806,#170807),(#170808,#170809,#170810),
(#170811,#170812,#170813),(#170814,#170815,#170816),(#170817,#170818,#170819),
(#170820,#170821,#170822)),.UNSPECIFIED.,.F.,.F.,.F.)
B_SPLINE_SURFACE_WITH_KNOTS((4,2,4),(3,3),(-3.90312782094781E-18,0.00150339017752321,
0.00300678035504644),(0.,1.),.UNSPECIFIED.)
GEOMETRIC_REPRESENTATION_ITEM()
RATIONAL_B_SPLINE_SURFACE(((1.,0.58487869495887,1.),(1.,0.60668052563981,
1.),(1.,0.627781895260115,1.),(1.,0.668636131517873,1.),(1.,0.688512443471572,
1.),(1.,0.707106781186547,1.)))
REPRESENTATION_ITEM('')
SURFACE()
);
#2660=(
BOUNDED_SURFACE()
B_SPLINE_SURFACE(3,2,((#170845,#170846,#170847),(#170848,#170849,#170850),
(#170851,#170852,#170853),(#170854,#170855,#170856),(#170857,#170858,#170859),
(#170860,#170861,#170862)),.UNSPECIFIED.,.F.,.F.,.F.)
B_SPLINE_SURFACE_WITH_KNOTS((4,2,4),(3,3),(-1.06251812903579E-17,0.00150294083257491,
0.00300588166514984),(0.,1.),.UNSPECIFIED.)
GEOMETRIC_REPRESENTATION_ITEM()
RATIONAL_B_SPLINE_SURFACE(((1.,0.707106781186548,1.),(1.,0.688447591630839,
1.),(1.,0.669002122235948,1.),(1.,0.628207099426844,1.),(1.,0.606682052630604,
1.),(1.,0.584878694958868,1.)))
REPRESENTATION_ITEM('')
SURFACE()
);
#2661=(
BOUNDED_SURFACE()
B_SPLINE_SURFACE(3,2,((#170982,#170983,#170984),(#170985,#170986,#170987),
(#170988,#170989,#170990),(#170991,#170992,#170993),(#170994,#170995,#170996),
(#170997,#170998,#170999)),.UNSPECIFIED.,.F.,.F.,.F.)
B_SPLINE_SURFACE_WITH_KNOTS((4,2,4),(3,3),(-1.83478794364492E-5,0.0189537577590876,
0.0379258633976115),(0.,1.00001834787944),.UNSPECIFIED.)
GEOMETRIC_REPRESENTATION_ITEM()
RATIONAL_B_SPLINE_SURFACE(((0.999999999999999,0.620309398234657,1.00001393303477),
(1.,0.616103929910579,1.00001408735762),(1.,0.611321563705418,1.00001426285018),
(1.,0.599839171198574,1.00001468420528),(1.,0.593149294515289,1.00001492969539),
(0.999999999999999,0.584846995484289,1.00001523435455)))
REPRESENTATION_ITEM('')
SURFACE()
);
#2662=(
BOUNDED_SURFACE()
B_SPLINE_SURFACE(3,2,((#171026,#171027,#171028),(#171029,#171030,#171031),
(#171032,#171033,#171034),(#171035,#171036,#171037),(#171038,#171039,#171040),
(#171041,#171042,#171043),(#171044,#171045,#171046),(#171047,#171048,#171049)),
 .UNSPECIFIED.,.F.,.F.,.F.)
B_SPLINE_SURFACE_WITH_KNOTS((4,2,2,4),(3,3),(0.0758061741912965,0.0799264930317429,
0.081986652451966,0.0840468118721892),(0.,1.00000233834524),
 .UNSPECIFIED.)
GEOMETRIC_REPRESENTATION_ITEM()
RATIONAL_B_SPLINE_SURFACE(((1.,0.961573749752273,1.00000017970768),(1.,
0.963379709173868,1.00000017126177),(1.,0.965135219920033,1.00000016305179),
(1.,0.9676189737872,1.00000015143604),(1.,0.968423864707538,1.00000014767181),
(1.,0.969943438537677,1.00000014056524),(1.,0.970660702862963,1.00000013721081),
(1.,0.971327062935609,1.00000013409445)))
REPRESENTATION_ITEM('')
SURFACE()
);
#2663=(
BOUNDED_SURFACE()
B_SPLINE_SURFACE(3,2,((#171155,#171156,#171157),(#171158,#171159,#171160),
(#171161,#171162,#171163),(#171164,#171165,#171166),(#171167,#171168,#171169),
(#171170,#171171,#171172)),.UNSPECIFIED.,.F.,.F.,.F.)
B_SPLINE_SURFACE_WITH_KNOTS((4,2,4),(3,3),(-0.00011033835690659,0.00119596402151854,
0.00250226639994571),(-0.000284389303992256,1.),.UNSPECIFIED.)
GEOMETRIC_REPRESENTATION_ITEM()
RATIONAL_B_SPLINE_SURFACE(((1.00012562153941,0.779138072972314,1.),(1.00013243243221,
0.767163479163878,1.),(1.00013944174136,0.754840038985303,1.),(1.00015379669844,
0.729601823486879,1.),(1.00016119800703,0.716589188185346,1.),(1.00016848829712,
0.703771740441114,1.)))
REPRESENTATION_ITEM('')
SURFACE()
);
#2664=(
BOUNDED_SURFACE()
B_SPLINE_SURFACE(3,2,((#171194,#171195,#171196),(#171197,#171198,#171199),
(#171200,#171201,#171202),(#171203,#171204,#171205),(#171206,#171207,#171208),
(#171209,#171210,#171211)),.UNSPECIFIED.,.F.,.F.,.F.)
B_SPLINE_SURFACE_WITH_KNOTS((4,2,4),(3,3),(0.,0.00119589979970271,0.00239179959940542),
(0.,1.),.UNSPECIFIED.)
GEOMETRIC_REPRESENTATION_ITEM()
RATIONAL_B_SPLINE_SURFACE(((1.,0.707106781186548,1.),(1.,0.718869254063191,
1.),(1.,0.730529301274249,1.),(1.,0.753629773858896,1.),(1.,0.765147260447909,
1.),(1.,0.776159951988232,1.)))
REPRESENTATION_ITEM('')
SURFACE()
);
#2665=(
BOUNDED_SURFACE()
B_SPLINE_SURFACE(3,2,((#171227,#171228,#171229),(#171230,#171231,#171232),
(#171233,#171234,#171235),(#171236,#171237,#171238)),.UNSPECIFIED.,.F.,
 .F.,.F.)
B_SPLINE_SURFACE_WITH_KNOTS((4,4),(3,3),(0.,0.0421837023697854),(0.,1.),
 .UNSPECIFIED.)
GEOMETRIC_REPRESENTATION_ITEM()
RATIONAL_B_SPLINE_SURFACE(((1.,0.755978609126094,1.),(1.,0.760793534959097,
1.),(1.,0.766730014383061,1.),(1.,0.776159951988524,1.)))
REPRESENTATION_ITEM('')
SURFACE()
);
#2666=(
BOUNDED_SURFACE()
B_SPLINE_SURFACE(3,2,((#171245,#171246,#171247),(#171248,#171249,#171250),
(#171251,#171252,#171253),(#171254,#171255,#171256)),.UNSPECIFIED.,.F.,
 .F.,.F.)
B_SPLINE_SURFACE_WITH_KNOTS((4,4),(3,3),(0.,0.000650577858517379),(0.,1.),
 .UNSPECIFIED.)
GEOMETRIC_REPRESENTATION_ITEM()
RATIONAL_B_SPLINE_SURFACE(((1.,0.760728353039955,1.),(1.,0.760722617942438,
1.),(1.,0.759141109939139,1.),(1.,0.755978609126096,1.)))
REPRESENTATION_ITEM('')
SURFACE()
);
#2667=(
BOUNDED_SURFACE()
B_SPLINE_SURFACE(3,2,((#171263,#171264,#171265),(#171266,#171267,#171268),
(#171269,#171270,#171271),(#171272,#171273,#171274),(#171275,#171276,#171277),
(#171278,#171279,#171280),(#171281,#171282,#171283),(#171284,#171285,#171286),
(#171287,#171288,#171289),(#171290,#171291,#171292),(#171293,#171294,#171295),
(#171296,#171297,#171298),(#171299,#171300,#171301),(#171302,#171303,#171304)),
 .UNSPECIFIED.,.F.,.F.,.F.)
B_SPLINE_SURFACE_WITH_KNOTS((4,2,2,2,2,2,4),(3,3),(0.00808024661615471,
0.00880850598034447,0.00917263566243935,0.00953676534453423,0.00990089502662911,
0.010265024708724,0.0109932840729137),(0.,1.),.UNSPECIFIED.)
GEOMETRIC_REPRESENTATION_ITEM()
RATIONAL_B_SPLINE_SURFACE(((1.,0.707106781186552,1.),(1.,0.7086803042033,
1.),(1.,0.710213526000588,1.),(1.,0.712453026336305,1.),(1.,0.713188114139461,
1.),(1.,0.714590095265908,1.),(1.,0.715263343050717,1.),(1.,0.716554408796435,
1.),(1.,0.71717678241798,1.),(1.,0.718331565221162,1.),(1.,0.718866152975084,
1.),(1.,0.720344053893136,1.),(1.,0.721169771392395,1.),(1.,0.721765931188049,
1.)))
REPRESENTATION_ITEM('')
SURFACE()
);
#2668=(
BOUNDED_SURFACE()
B_SPLINE_SURFACE(3,2,((#171347,#171348,#171349),(#171350,#171351,#171352),
(#171353,#171354,#171355),(#171356,#171357,#171358)),.UNSPECIFIED.,.F.,
 .F.,.F.)
B_SPLINE_SURFACE_WITH_KNOTS((4,4),(3,3),(0.,0.0419168978153696),(0.,1.),
 .UNSPECIFIED.)
GEOMETRIC_REPRESENTATION_ITEM()
RATIONAL_B_SPLINE_SURFACE(((1.,0.776159951988518,1.),(1.,0.766788671732685,
1.),(1.,0.760870494736068,1.),(1.,0.756069167758398,1.)))
REPRESENTATION_ITEM('')
SURFACE()
);
#2669=(
BOUNDED_SURFACE()
B_SPLINE_SURFACE(3,2,((#171401,#171402,#171403),(#171404,#171405,#171406),
(#171407,#171408,#171409),(#171410,#171411,#171412),(#171413,#171414,#171415),
(#171416,#171417,#171418),(#171419,#171420,#171421),(#171422,#171423,#171424),
(#171425,#171426,#171427),(#171428,#171429,#171430),(#171431,#171432,#171433),
(#171434,#171435,#171436),(#171437,#171438,#171439),(#171440,#171441,#171442)),
 .UNSPECIFIED.,.F.,.F.,.F.)
B_SPLINE_SURFACE_WITH_KNOTS((4,2,2,2,2,2,4),(3,3),(0.00808046157075938,
0.00879095475051749,0.00914620134039654,0.0095014479302756,0.00985669452015465,
0.0102119411100337,0.0109224342897918),(0.,1.),.UNSPECIFIED.)
GEOMETRIC_REPRESENTATION_ITEM()
RATIONAL_B_SPLINE_SURFACE(((1.,0.707106781186552,1.),(1.,0.705538120216095,
1.),(1.,0.703999772329756,1.),(1.,0.701739154413458,1.),(1.,0.700992634705956,
1.),(1.,0.699563445722461,1.),(1.,0.698874516085242,1.),(1.,0.697548436732303,
1.),(1.,0.696906638208049,1.),(1.,0.695703451829647,1.),(1.,0.695143596113536,
1.),(1.,0.693587190992306,1.),(1.,0.692704331853457,1.),(1.,0.69204248906153,
1.)))
REPRESENTATION_ITEM('')
SURFACE()
);
#2670=(
BOUNDED_SURFACE()
B_SPLINE_SURFACE(3,2,((#171485,#171486,#171487),(#171488,#171489,#171490),
(#171491,#171492,#171493),(#171494,#171495,#171496)),.UNSPECIFIED.,.F.,
 .F.,.F.)
B_SPLINE_SURFACE_WITH_KNOTS((4,4),(3,3),(0.,0.000650363027228679),(0.,1.),
 .UNSPECIFIED.)
GEOMETRIC_REPRESENTATION_ITEM()
RATIONAL_B_SPLINE_SURFACE(((1.,0.66913647774042,1.),(1.,0.666544790513632,
1.),(1.,0.665198010610878,1.),(1.,0.665190809887722,1.)))
REPRESENTATION_ITEM('')
SURFACE()
);
#2671=(
BOUNDED_SURFACE()
B_SPLINE_SURFACE(3,2,((#171500,#171501,#171502),(#171503,#171504,#171505),
(#171506,#171507,#171508),(#171509,#171510,#171511)),.UNSPECIFIED.,.F.,
 .F.,.F.)
B_SPLINE_SURFACE_WITH_KNOTS((4,4),(3,3),(0.,0.0433970829567688),(0.,1.),
 .UNSPECIFIED.)
GEOMETRIC_REPRESENTATION_ITEM()
RATIONAL_B_SPLINE_SURFACE(((1.,0.651268546304981,1.),(1.,0.659940697395559,
1.),(1.,0.665023311775857,1.),(1.,0.669136477740405,1.)))
REPRESENTATION_ITEM('')
SURFACE()
);
#2672=(
BOUNDED_SURFACE()
B_SPLINE_SURFACE(3,2,((#171518,#171519,#171520),(#171521,#171522,#171523),
(#171524,#171525,#171526),(#171527,#171528,#171529),(#171530,#171531,#171532),
(#171533,#171534,#171535)),.UNSPECIFIED.,.F.,.F.,.F.)
B_SPLINE_SURFACE_WITH_KNOTS((4,2,4),(3,3),(-0.00017231904915643,0.00109600456666539,
0.00236432773995983),(-0.000172319052339097,1.),.UNSPECIFIED.)
GEOMETRIC_REPRESENTATION_ITEM()
RATIONAL_B_SPLINE_SURFACE(((1.00012181741146,0.646535279167556,1.),(1.00011784985333,
0.658047523674751,1.),(1.0001140008242,0.669215845107308,1.),(1.00010655811155,
0.690811578565519,1.),(1.00010293762449,0.701316763613497,1.),(1.00009957515527,
0.711073285509502,1.)))
REPRESENTATION_ITEM('')
SURFACE()
);
#2673=(
BOUNDED_SURFACE()
B_SPLINE_SURFACE(3,2,((#171555,#171556,#171557),(#171558,#171559,#171560),
(#171561,#171562,#171563),(#171564,#171565,#171566),(#171567,#171568,#171569),
(#171570,#171571,#171572)),.UNSPECIFIED.,.F.,.F.,.F.)
B_SPLINE_SURFACE_WITH_KNOTS((4,2,4),(3,3),(0.,0.00109598668217933,0.00219197336435865),
(0.,1.),.UNSPECIFIED.)
GEOMETRIC_REPRESENTATION_ITEM()
RATIONAL_B_SPLINE_SURFACE(((1.,0.707106781186548,1.),(1.,0.698507203291837,
1.),(1.,0.689563761715544,1.),(1.,0.670914228806854,1.),(1.,0.661139818833385,
1.),(1.,0.65126854630498,1.)))
REPRESENTATION_ITEM('')
SURFACE()
);
#2674=(
BOUNDED_SURFACE()
B_SPLINE_SURFACE(3,2,((#171653,#171654,#171655),(#171656,#171657,#171658),
(#171659,#171660,#171661),(#171662,#171663,#171664)),.UNSPECIFIED.,.F.,
 .F.,.F.)
B_SPLINE_SURFACE_WITH_KNOTS((4,4),(3,3),(-1.38777878078145E-17,0.0431305646498159),
(0.,1.),.UNSPECIFIED.)
GEOMETRIC_REPRESENTATION_ITEM()
RATIONAL_B_SPLINE_SURFACE(((1.,0.669061697655964,1.),(1.,0.66495869705799,
1.),(1.,0.659888610517475,1.),(1.,0.65126854630498,1.)))
REPRESENTATION_ITEM('')
SURFACE()
);
#2675=(
BOUNDED_SURFACE()
B_SPLINE_SURFACE(3,2,((#171688,#171689,#171690),(#171691,#171692,#171693),
(#171694,#171695,#171696),(#171697,#171698,#171699),(#171700,#171701,#171702),
(#171703,#171704,#171705),(#171706,#171707,#171708),(#171709,#171710,#171711)),
 .UNSPECIFIED.,.F.,.F.,.F.)
B_SPLINE_SURFACE_WITH_KNOTS((4,2,2,4),(3,3),(0.023727979672696,0.0269788291349169,
0.0286042538660274,0.0302296785971378),(0.,1.),.UNSPECIFIED.)
GEOMETRIC_REPRESENTATION_ITEM()
RATIONAL_B_SPLINE_SURFACE(((1.,0.972985060853882,1.),(1.,0.973867966894579,
1.),(1.,0.974606628833735,1.),(1.,0.975438732489742,1.),(1.,0.975670772749385,
1.),(1.,0.976026965697327,1.),(1.,0.976152018462137,1.),(1.,0.976223679017856,
1.)))
REPRESENTATION_ITEM('')
SURFACE()
);
#2676=(
BOUNDED_SURFACE()
B_SPLINE_SURFACE(3,2,((#171754,#171755,#171756),(#171757,#171758,#171759),
(#171760,#171761,#171762),(#171763,#171764,#171765)),.UNSPECIFIED.,.F.,
 .F.,.F.)
B_SPLINE_SURFACE_WITH_KNOTS((4,4),(3,3),(0.,0.00195732365556561),(0.,1.),
 .UNSPECIFIED.)
GEOMETRIC_REPRESENTATION_ITEM()
RATIONAL_B_SPLINE_SURFACE(((1.,0.71617462512364,1.),(1.,0.713064019807532,
1.),(1.,0.709996713322441,1.),(1.,0.707106781186534,1.)))
REPRESENTATION_ITEM('')
SURFACE()
);
#2677=(
BOUNDED_SURFACE()
B_SPLINE_SURFACE(3,2,((#171775,#171776,#171777),(#171778,#171779,#171780),
(#171781,#171782,#171783),(#171784,#171785,#171786)),.UNSPECIFIED.,.F.,
 .F.,.F.)
B_SPLINE_SURFACE_WITH_KNOTS((4,4),(3,3),(0.,0.00195732360009946),(0.,1.),
 .UNSPECIFIED.)
GEOMETRIC_REPRESENTATION_ITEM()
RATIONAL_B_SPLINE_SURFACE(((1.,0.707106781186548,1.),(1.,0.709967301734631,
1.),(1.,0.713032729764421,1.),(1.,0.716174625123614,1.)))
REPRESENTATION_ITEM('')
SURFACE()
);
#2678=(
BOUNDED_SURFACE()
B_SPLINE_SURFACE(3,2,((#171790,#171791,#171792),(#171793,#171794,#171795),
(#171796,#171797,#171798),(#171799,#171800,#171801)),.UNSPECIFIED.,.F.,
 .F.,.F.)
B_SPLINE_SURFACE_WITH_KNOTS((4,4),(3,3),(0.,0.0447707136167657),(0.,1.),
 .UNSPECIFIED.)
GEOMETRIC_REPRESENTATION_ITEM()
RATIONAL_B_SPLINE_SURFACE(((1.,0.713272398106993,1.),(1.,0.713940344609358,
1.),(1.,0.714765614654658,1.),(1.,0.71617462512364,1.)))
REPRESENTATION_ITEM('')
SURFACE()
);
#2679=(
BOUNDED_SURFACE()
B_SPLINE_SURFACE(3,2,((#171808,#171809,#171810),(#171811,#171812,#171813),
(#171814,#171815,#171816),(#171817,#171818,#171819)),.UNSPECIFIED.,.F.,
 .F.,.F.)
B_SPLINE_SURFACE_WITH_KNOTS((4,4),(3,3),(0.,0.000650121327073412),(0.,1.),
 .UNSPECIFIED.)
GEOMETRIC_REPRESENTATION_ITEM()
RATIONAL_B_SPLINE_SURFACE(((1.,0.713890629234418,1.),(1.,0.713889885788569,
1.),(1.,0.71368362023966,1.),(1.,0.713272398106985,1.)))
REPRESENTATION_ITEM('')
SURFACE()
);
#2680=(
BOUNDED_SURFACE()
B_SPLINE_SURFACE(3,2,((#171826,#171827,#171828),(#171829,#171830,#171831),
(#171832,#171833,#171834),(#171835,#171836,#171837),(#171838,#171839,#171840),
(#171841,#171842,#171843),(#171844,#171845,#171846),(#171847,#171848,#171849),
(#171850,#171851,#171852),(#171853,#171854,#171855)),.UNSPECIFIED.,.F.,
 .F.,.F.)
B_SPLINE_SURFACE_WITH_KNOTS((4,2,2,2,4),(3,3),(0.0080756712423913,0.00867825313759154,
0.00928083503279179,0.00988341692799203,0.0104859988231923),(0.,1.),
 .UNSPECIFIED.)
GEOMETRIC_REPRESENTATION_ITEM()
RATIONAL_B_SPLINE_SURFACE(((1.,0.707106781186548,1.),(1.,0.707146901961909,
1.),(1.,0.707185957443845,1.),(1.,0.707262034097608,1.),(1.,0.707299176477847,
1.),(1.,0.7073675568103,1.),(1.,0.707399679105567,1.),(1.,0.707457223307409,
1.),(1.,0.707482383732919,1.),(1.,0.707504065565917,1.)))
REPRESENTATION_ITEM('')
SURFACE()
);
#2681=(
BOUNDED_SURFACE()
B_SPLINE_SURFACE(3,2,((#171883,#171884,#171885),(#171886,#171887,#171888),
(#171889,#171890,#171891),(#171892,#171893,#171894)),.UNSPECIFIED.,.F.,
 .F.,.F.)
B_SPLINE_SURFACE_WITH_KNOTS((4,4),(3,3),(0.,0.0445045070401677),(0.,1.),
 .UNSPECIFIED.)
GEOMETRIC_REPRESENTATION_ITEM()
RATIONAL_B_SPLINE_SURFACE(((1.,0.71617462512364,1.),(1.,0.714773807595299,
1.),(1.,0.713950503107743,1.),(1.,0.713284154090124,1.)))
REPRESENTATION_ITEM('')
SURFACE()
);
#2682=(
BOUNDED_SURFACE()
B_SPLINE_SURFACE(3,2,((#171928,#171929,#171930),(#171931,#171932,#171933),
(#171934,#171935,#171936),(#171937,#171938,#171939),(#171940,#171941,#171942),
(#171943,#171944,#171945),(#171946,#171947,#171948),(#171949,#171950,#171951),
(#171952,#171953,#171954),(#171955,#171956,#171957)),.UNSPECIFIED.,.F.,
 .F.,.F.)
B_SPLINE_SURFACE_WITH_KNOTS((4,2,2,2,4),(3,3),(0.00807569768389314,0.00867847980331418,
0.00928126192273523,0.00988404404215627,0.0104868261615773),(0.,1.),
 .UNSPECIFIED.)
GEOMETRIC_REPRESENTATION_ITEM()
RATIONAL_B_SPLINE_SURFACE(((1.,0.707106781186548,1.),(1.,0.707212493429049,
1.),(1.,0.707315385014487,1.),(1.,0.707515784384109,1.),(1.,0.707613608127955,
1.),(1.,0.707793680404111,1.),(1.,0.707878261047732,1.),(1.,0.708029744860286,
1.),(1.,0.7080959680978,1.),(1.,0.708153025875396,1.)))
REPRESENTATION_ITEM('')
SURFACE()
);
#2683=(
BOUNDED_SURFACE()
B_SPLINE_SURFACE(3,2,((#171988,#171989,#171990),(#171991,#171992,#171993),
(#171994,#171995,#171996),(#171997,#171998,#171999)),.UNSPECIFIED.,.F.,
 .F.,.F.)
B_SPLINE_SURFACE_WITH_KNOTS((4,4),(3,3),(0.,0.000650124428678587),(0.,1.),
 .UNSPECIFIED.)
GEOMETRIC_REPRESENTATION_ITEM()
RATIONAL_B_SPLINE_SURFACE(((1.,0.714485667734326,1.),(1.,0.714973119513317,
1.),(1.,0.715223297464931,1.),(1.,0.715224866856049,1.)))
REPRESENTATION_ITEM('')
SURFACE()
);
#2684=(
BOUNDED_SURFACE()
B_SPLINE_SURFACE(3,2,((#172003,#172004,#172005),(#172006,#172007,#172008),
(#172009,#172010,#172011),(#172012,#172013,#172014)),.UNSPECIFIED.,.F.,
 .F.,.F.)
B_SPLINE_SURFACE_WITH_KNOTS((4,4),(3,3),(0.,0.044753309356401),(0.,1.),
 .UNSPECIFIED.)
GEOMETRIC_REPRESENTATION_ITEM()
RATIONAL_B_SPLINE_SURFACE(((1.,0.717952606100523,1.),(1.,0.716270361073643,
1.),(1.,0.715283994577086,1.),(1.,0.714485667734334,1.)))
REPRESENTATION_ITEM('')
SURFACE()
);
#2685=(
BOUNDED_SURFACE()
B_SPLINE_SURFACE(3,2,((#172021,#172022,#172023),(#172024,#172025,#172026),
(#172027,#172028,#172029),(#172030,#172031,#172032)),.UNSPECIFIED.,.F.,
 .F.,.F.)
B_SPLINE_SURFACE_WITH_KNOTS((4,4),(3,3),(-3.90312782094781E-18,0.0019603544817943),
(0.,1.),.UNSPECIFIED.)
GEOMETRIC_REPRESENTATION_ITEM()
RATIONAL_B_SPLINE_SURFACE(((1.,0.717952606100523,1.),(1.,0.714237876912109,
1.),(1.,0.710568615888393,1.),(1.,0.707106781186514,1.)))
REPRESENTATION_ITEM('')
SURFACE()
);
#2686=(
BOUNDED_SURFACE()
B_SPLINE_SURFACE(3,2,((#172040,#172041,#172042),(#172043,#172044,#172045),
(#172046,#172047,#172048),(#172049,#172050,#172051)),.UNSPECIFIED.,.F.,
 .F.,.F.)
B_SPLINE_SURFACE_WITH_KNOTS((4,4),(3,3),(0.,0.00196035438616165),(0.,1.),
 .UNSPECIFIED.)
GEOMETRIC_REPRESENTATION_ITEM()
RATIONAL_B_SPLINE_SURFACE(((1.,0.707106781186548,1.),(1.,0.710533388681839,
1.),(1.,0.714200483631581,1.),(1.,0.717952606100467,1.)))
REPRESENTATION_ITEM('')
SURFACE()
);
#2687=(
BOUNDED_SURFACE()
B_SPLINE_SURFACE(3,2,((#172057,#172058,#172059),(#172060,#172061,#172062),
(#172063,#172064,#172065),(#172066,#172067,#172068)),.UNSPECIFIED.,.F.,
 .F.,.F.)
B_SPLINE_SURFACE_WITH_KNOTS((4,4),(3,3),(0.,0.0444870989094409),(0.,1.),
 .UNSPECIFIED.)
GEOMETRIC_REPRESENTATION_ITEM()
RATIONAL_B_SPLINE_SURFACE(((1.,0.71449972514277,1.),(1.,0.715296138993144,
1.),(1.,0.71628014758797,1.),(1.,0.717952606100523,1.)))
REPRESENTATION_ITEM('')
SURFACE()
);
#2688=(
BOUNDED_SURFACE()
B_SPLINE_SURFACE(3,2,((#172101,#172102,#172103),(#172104,#172105,#172106),
(#172107,#172108,#172109),(#172110,#172111,#172112),(#172113,#172114,#172115),
(#172116,#172117,#172118)),.UNSPECIFIED.,.F.,.F.,.F.)
B_SPLINE_SURFACE_WITH_KNOTS((4,2,4),(3,3),(0.012499301108314,0.0157975372010094,
0.0190957732937049),(0.,1.),.UNSPECIFIED.)
GEOMETRIC_REPRESENTATION_ITEM()
RATIONAL_B_SPLINE_SURFACE(((1.,0.976191060180328,1.),(1.,0.976018964367352,
1.),(1.,0.975629721882182,1.),(1.,0.974451430140223,1.),(1.,0.97367913510036,
1.),(1.,0.972768244198254,1.)))
REPRESENTATION_ITEM('')
SURFACE()
);
#2689=(
BOUNDED_SURFACE()
B_SPLINE_SURFACE(3,2,((#172209,#172210,#172211),(#172212,#172213,#172214),
(#172215,#172216,#172217),(#172218,#172219,#172220),(#172221,#172222,#172223),
(#172224,#172225,#172226)),.UNSPECIFIED.,.F.,.F.,.F.)
B_SPLINE_SURFACE_WITH_KNOTS((4,2,4),(3,3),(-0.00018317133585458,0.00110390261829224,
0.00239097668804685),(-0.000183171451462374,1.),.UNSPECIFIED.)
GEOMETRIC_REPRESENTATION_ITEM()
RATIONAL_B_SPLINE_SURFACE(((1.00013033238588,0.644233899891368,1.),(1.00012593769652,
0.656230008786567,1.),(1.00012167569773,0.667863914494213,1.),(1.00011343748823,
0.690351615044338,1.),(1.00010943132374,0.701287174225601,1.),(1.00010571535824,
0.711430582116219,1.)))
REPRESENTATION_ITEM('')
SURFACE()
);
#2690=(
BOUNDED_SURFACE()
B_SPLINE_SURFACE(3,2,((#172248,#172249,#172250),(#172251,#172252,#172253),
(#172254,#172255,#172256),(#172257,#172258,#172259),(#172260,#172261,#172262),
(#172263,#172264,#172265)),.UNSPECIFIED.,.F.,.F.,.F.)
B_SPLINE_SURFACE_WITH_KNOTS((4,2,4),(3,3),(0.,0.00110388220976991,0.00220776441953981),
(0.,1.),.UNSPECIFIED.)
GEOMETRIC_REPRESENTATION_ITEM()
RATIONAL_B_SPLINE_SURFACE(((1.,0.707106781186548,1.),(1.,0.69822152219183,
1.),(1.,0.68897986867167,1.),(1.,0.66970545013756,1.),(1.,0.659601845960695,
1.),(1.,0.649397749909072,1.)))
REPRESENTATION_ITEM('')
SURFACE()
);
#2691=(
BOUNDED_SURFACE()
B_SPLINE_SURFACE(3,2,((#172281,#172282,#172283),(#172284,#172285,#172286),
(#172287,#172288,#172289),(#172290,#172291,#172292)),.UNSPECIFIED.,.F.,
 .F.,.F.)
B_SPLINE_SURFACE_WITH_KNOTS((4,4),(3,3),(-2.77555756156289E-17,0.0433026927553429),
(0.,1.),.UNSPECIFIED.)
GEOMETRIC_REPRESENTATION_ITEM()
RATIONAL_B_SPLINE_SURFACE(((1.,0.667840827103545,1.),(1.,0.66359300941018,
1.),(1.,0.658343952018749,1.),(1.,0.649397749909072,1.)))
REPRESENTATION_ITEM('')
SURFACE()
);
#2692=(
BOUNDED_SURFACE()
B_SPLINE_SURFACE(3,2,((#172299,#172300,#172301),(#172302,#172303,#172304),
(#172305,#172306,#172307),(#172308,#172309,#172310)),.UNSPECIFIED.,.F.,
 .F.,.F.)
B_SPLINE_SURFACE_WITH_KNOTS((4,4),(3,3),(0.,0.000650375609766158),(0.,1.),
 .UNSPECIFIED.)
GEOMETRIC_REPRESENTATION_ITEM()
RATIONAL_B_SPLINE_SURFACE(((1.,0.663756004792833,1.),(1.,0.663759519746911,
1.),(1.,0.665134391960157,1.),(1.,0.66784082710355,1.)))
REPRESENTATION_ITEM('')
SURFACE()
);
#2693=(
BOUNDED_SURFACE()
B_SPLINE_SURFACE(3,2,((#172317,#172318,#172319),(#172320,#172321,#172322),
(#172323,#172324,#172325),(#172326,#172327,#172328),(#172329,#172330,#172331),
(#172332,#172333,#172334),(#172335,#172336,#172337),(#172338,#172339,#172340),
(#172341,#172342,#172343),(#172344,#172345,#172346),(#172347,#172348,#172349),
(#172350,#172351,#172352),(#172353,#172354,#172355),(#172356,#172357,#172358)),
 .UNSPECIFIED.,.F.,.F.,.F.)
B_SPLINE_SURFACE_WITH_KNOTS((4,2,2,2,2,2,4),(3,3),(0.0080803797182093,0.00879690254712659,
0.00915516396158524,0.00951342537604388,0.00987168679050253,0.0102299482049612,
0.0109464710338785),(0.,1.),.UNSPECIFIED.)
GEOMETRIC_REPRESENTATION_ITEM()
RATIONAL_B_SPLINE_SURFACE(((1.,0.707106781186548,1.),(1.,0.705537440672151,
1.),(1.,0.703998083945123,1.),(1.,0.701735656940981,1.),(1.,0.700989163179782,
1.),(1.,0.699560461823081,1.),(1.,0.698871897343629,1.),(1.,0.697546947950716,
1.),(1.,0.696905752213842,1.),(1.,0.695707159507179,1.),(1.,0.695149875554341,
1.),(1.,0.693602432259692,1.),(1.,0.692727265033204,1.),(1.,0.692079067931822,
1.)))
REPRESENTATION_ITEM('')
SURFACE()
);
#2694=(
BOUNDED_SURFACE()
B_SPLINE_SURFACE(3,2,((#172395,#172396,#172397),(#172398,#172399,#172400),
(#172401,#172402,#172403),(#172404,#172405,#172406)),.UNSPECIFIED.,.F.,
 .F.,.F.)
B_SPLINE_SURFACE_WITH_KNOTS((4,4),(3,3),(0.,0.0430361525536219),(0.,1.),
 .UNSPECIFIED.)
GEOMETRIC_REPRESENTATION_ITEM()
RATIONAL_B_SPLINE_SURFACE(((1.,0.649397749909071,1.),(1.,0.658290092659334,
1.),(1.,0.663526138769308,1.),(1.,0.667763418073535,1.)))
REPRESENTATION_ITEM('')
SURFACE()
);
#2695=(
BOUNDED_SURFACE()
B_SPLINE_SURFACE(3,2,((#172448,#172449,#172450),(#172451,#172452,#172453),
(#172454,#172455,#172456),(#172457,#172458,#172459),(#172460,#172461,#172462),
(#172463,#172464,#172465),(#172466,#172467,#172468),(#172469,#172470,#172471),
(#172472,#172473,#172474),(#172475,#172476,#172477),(#172478,#172479,#172480),
(#172481,#172482,#172483),(#172484,#172485,#172486),(#172487,#172488,#172489)),
 .UNSPECIFIED.,.F.,.F.,.F.)
B_SPLINE_SURFACE_WITH_KNOTS((4,2,2,2,2,2,4),(3,3),(0.00808011141552929,
0.00881517523662049,0.00918270714716608,0.00955023905771168,0.00991777096825728,
0.0102853028788029,0.0110203666998941),(0.,1.),.UNSPECIFIED.)
GEOMETRIC_REPRESENTATION_ITEM()
RATIONAL_B_SPLINE_SURFACE(((1.,0.707106781186548,1.),(1.,0.708672362536739,
1.),(1.,0.710198222857537,1.),(1.,0.712427305746575,1.),(1.,0.71315813872198,
1.),(1.,0.714551782754775,1.),(1.,0.715220876802376,1.),(1.,0.71650348303418,
1.),(1.,0.717121230234592,1.),(1.,0.718264550261012,1.),(1.,0.718793336138408,
1.),(1.,0.720253112545596,1.),(1.,0.721064801594907,1.),(1.,0.721643051700349,
1.)))
REPRESENTATION_ITEM('')
SURFACE()
);
#2696=(
BOUNDED_SURFACE()
B_SPLINE_SURFACE(3,2,((#172532,#172533,#172534),(#172535,#172536,#172537),
(#172538,#172539,#172540),(#172541,#172542,#172543)),.UNSPECIFIED.,.F.,
 .F.,.F.)
B_SPLINE_SURFACE_WITH_KNOTS((4,4),(3,3),(-6.5060980421357E-5,0.000715670784634951),
(-0.000197321044369628,1.),.UNSPECIFIED.)
GEOMETRIC_REPRESENTATION_ITEM()
RATIONAL_B_SPLINE_SURFACE(((1.00009626630384,0.756066809424477,1.),(1.00009460009415,
0.760288887453376,1.),(1.0000938192903,0.762267398805323,1.),(1.0000939691079,
0.761887769744427,1.)))
REPRESENTATION_ITEM('')
SURFACE()
);
#2697=(
BOUNDED_SURFACE()
B_SPLINE_SURFACE(3,2,((#172547,#172548,#172549),(#172550,#172551,#172552),
(#172553,#172554,#172555),(#172556,#172557,#172558)),.UNSPECIFIED.,.F.,
 .F.,.F.)
B_SPLINE_SURFACE_WITH_KNOTS((4,4),(3,3),(0.,0.0420570108120997),(0.,1.),
 .UNSPECIFIED.)
GEOMETRIC_REPRESENTATION_ITEM()
RATIONAL_B_SPLINE_SURFACE(((1.,0.777664586555049,1.),(1.,0.768081385918698,
1.),(1.,0.762031405880593,1.),(1.,0.757123446310248,1.)))
REPRESENTATION_ITEM('')
SURFACE()
);
#2698=(
BOUNDED_SURFACE()
B_SPLINE_SURFACE(3,2,((#172565,#172566,#172567),(#172568,#172569,#172570),
(#172571,#172572,#172573),(#172574,#172575,#172576),(#172577,#172578,#172579),
(#172580,#172581,#172582)),.UNSPECIFIED.,.F.,.F.,.F.)
B_SPLINE_SURFACE_WITH_KNOTS((4,2,4),(3,3),(0.,0.00120620763625507,0.00241241527251014),
(0.,1.),.UNSPECIFIED.)
GEOMETRIC_REPRESENTATION_ITEM()
RATIONAL_B_SPLINE_SURFACE(((1.,0.777664586555049,1.),(1.,0.766436783957212,
1.),(1.,0.754901973237173,1.),(1.,0.73129895059372,1.),(1.,0.719146552484787,
1.),(1.,0.707106781186548,1.)))
REPRESENTATION_ITEM('')
SURFACE()
);
#2699=(
BOUNDED_SURFACE()
B_SPLINE_SURFACE(3,2,((#172602,#172603,#172604),(#172605,#172606,#172607),
(#172608,#172609,#172610),(#172611,#172612,#172613),(#172614,#172615,#172616),
(#172617,#172618,#172619)),.UNSPECIFIED.,.F.,.F.,.F.)
B_SPLINE_SURFACE_WITH_KNOTS((4,2,4),(3,3),(0.,0.00120613678608598,0.00241227357217196),
(0.,1.),.UNSPECIFIED.)
GEOMETRIC_REPRESENTATION_ITEM()
RATIONAL_B_SPLINE_SURFACE(((1.,0.707106781186548,1.),(1.,0.719152101713129,
1.),(1.,0.731078910702522,1.),(1.,0.754682512407923,1.),(1.,0.766438100601174,
1.),(1.,0.777664586554854,1.)))
REPRESENTATION_ITEM('')
SURFACE()
);
#2700=(
BOUNDED_SURFACE()
B_SPLINE_SURFACE(3,2,((#172700,#172701,#172702),(#172703,#172704,#172705),
(#172706,#172707,#172708),(#172709,#172710,#172711)),.UNSPECIFIED.,.F.,
 .F.,.F.)
B_SPLINE_SURFACE_WITH_KNOTS((4,4),(3,3),(-8.32667268468867E-17,0.0417901757617077),
(0.,1.),.UNSPECIFIED.)
GEOMETRIC_REPRESENTATION_ITEM()
RATIONAL_B_SPLINE_SURFACE(((1.,0.757216058458815,1.),(1.,0.76211005468913,
1.),(1.,0.768141195659961,1.),(1.,0.777664586555055,1.)))
REPRESENTATION_ITEM('')
SURFACE()
);
#2701=(
BOUNDED_SURFACE()
B_SPLINE_SURFACE(3,2,((#172735,#172736,#172737),(#172738,#172739,#172740),
(#172741,#172742,#172743),(#172744,#172745,#172746),(#172747,#172748,#172749),
(#172750,#172751,#172752),(#172753,#172754,#172755),(#172756,#172757,#172758)),
 .UNSPECIFIED.,.F.,.F.,.F.)
B_SPLINE_SURFACE_WITH_KNOTS((4,2,2,4),(3,3),(0.017818580704263,0.0199004486313254,
0.0219823165583878,0.0261460524125126),(0.,1.),.UNSPECIFIED.)
GEOMETRIC_REPRESENTATION_ITEM()
RATIONAL_B_SPLINE_SURFACE(((1.,0.961171308030857,1.),(1.,0.962092810628593,
1.),(1.,0.963001088261132,1.),(1.,0.964780402726978,1.),(1.,0.965653853257041,
1.),(1.,0.968176214233281,1.),(1.,0.969729042204957,1.),(1.,0.971089731516655,
1.)))
REPRESENTATION_ITEM('')
SURFACE()
);
#2702=(
BOUNDED_SURFACE()
B_SPLINE_SURFACE(3,2,((#172864,#172865,#172866),(#172867,#172868,#172869),
(#172870,#172871,#172872),(#172873,#172874,#172875),(#172876,#172877,#172878),
(#172879,#172880,#172881)),.UNSPECIFIED.,.F.,.F.,.F.)
B_SPLINE_SURFACE_WITH_KNOTS((4,2,4),(3,3),(-1.5178830414797E-17,0.00151741931723474,
0.0030348386344695),(0.,1.),.UNSPECIFIED.)
GEOMETRIC_REPRESENTATION_ITEM()
RATIONAL_B_SPLINE_SURFACE(((1.,0.583115115460263,1.),(1.,0.605241592753533,
1.),(1.,0.62665070495839,1.),(1.,0.668094537904905,1.),(1.,0.688253312209368,
1.),(1.,0.70710678118655,1.)))
REPRESENTATION_ITEM('')
SURFACE()
);
#2703=(
BOUNDED_SURFACE()
B_SPLINE_SURFACE(3,2,((#172906,#172907,#172908),(#172909,#172910,#172911),
(#172912,#172913,#172914),(#172915,#172916,#172917),(#172918,#172919,#172920),
(#172921,#172922,#172923)),.UNSPECIFIED.,.F.,.F.,.F.)
B_SPLINE_SURFACE_WITH_KNOTS((4,2,4),(3,3),(0.,0.00151694200897944,0.00303388401795888),
(0.,1.),.UNSPECIFIED.)
GEOMETRIC_REPRESENTATION_ITEM()
RATIONAL_B_SPLINE_SURFACE(((1.,0.70710678118655,1.),(1.,0.688185240537986,
1.),(1.,0.6684652198449,1.),(1.,0.627083641349078,1.),(1.,0.605243055947471,
1.),(1.,0.583115115460264,1.)))
REPRESENTATION_ITEM('')
SURFACE()
);
#2704=(
BOUNDED_SURFACE()
B_SPLINE_SURFACE(3,2,((#172939,#172940,#172941),(#172942,#172943,#172944),
(#172945,#172946,#172947),(#172948,#172949,#172950),(#172951,#172952,#172953),
(#172954,#172955,#172956)),.UNSPECIFIED.,.F.,.F.,.F.)
B_SPLINE_SURFACE_WITH_KNOTS((4,2,4),(3,3),(-1.94201995013153E-5,0.018990790064314,
0.0380010003281294),(0.,1.0000194201995),.UNSPECIFIED.)
GEOMETRIC_REPRESENTATION_ITEM()
RATIONAL_B_SPLINE_SURFACE(((1.,0.619089870519235,1.00001479470141),(1.,
0.61482119355377,1.00001496049853),(1.,0.60996647972793,1.00001514905755),
(1.,0.5983079322478,1.00001560188019),(1.,0.59151444641303,1.00001586574189),
(0.999999999999999,0.58308117916846,1.00001619329335)))
REPRESENTATION_ITEM('')
SURFACE()
);
#2705=(
BOUNDED_SURFACE()
B_SPLINE_SURFACE(3,2,((#172966,#172967,#172968),(#172969,#172970,#172971),
(#172972,#172973,#172974),(#172975,#172976,#172977)),.UNSPECIFIED.,.F.,
 .F.,.F.)
B_SPLINE_SURFACE_WITH_KNOTS((4,4),(3,3),(-6.51408174375083E-5,0.000716548991812596),
(-0.000127150757950157,1.),.UNSPECIFIED.)
GEOMETRIC_REPRESENTATION_ITEM()
RATIONAL_B_SPLINE_SURFACE(((1.00009928949958,0.60955993820037,1.),(1.00009948976837,
0.608772413245102,1.),(1.0000984813281,0.612737943163154,1.),(1.00009637648133,
0.621014916147796,1.)))
REPRESENTATION_ITEM('')
SURFACE()
);
#2706=(
BOUNDED_SURFACE()
B_SPLINE_SURFACE(3,2,((#172992,#172993,#172994),(#172995,#172996,#172997),
(#172998,#172999,#173000),(#173001,#173002,#173003),(#173004,#173005,#173006),
(#173007,#173008,#173009)),.UNSPECIFIED.,.F.,.F.,.F.)
B_SPLINE_SURFACE_WITH_KNOTS((4,2,4),(3,3),(0.,0.0188568492058762,0.0377136984117525),
(0.,1.),.UNSPECIFIED.)
GEOMETRIC_REPRESENTATION_ITEM()
RATIONAL_B_SPLINE_SURFACE(((1.,0.583115115460263,1.),(1.,0.591477165975886,
1.),(1.,0.59822556054293,1.),(1.,0.609817503669346,1.),(1.,0.614651018359553,
1.),(1.,0.618903611686376,1.)))
REPRESENTATION_ITEM('')
SURFACE()
);
#2707=(
BOUNDED_SURFACE()
B_SPLINE_SURFACE(3,2,((#173094,#173095,#173096),(#173097,#173098,#173099),
(#173100,#173101,#173102),(#173103,#173104,#173105)),.UNSPECIFIED.,.F.,
 .F.,.F.)
B_SPLINE_SURFACE_WITH_KNOTS((4,4),(3,3),(-6.51957114117336E-5,0.000717152825529202),
(-0.000139515695195982,1.),.UNSPECIFIED.)
GEOMETRIC_REPRESENTATION_ITEM()
RATIONAL_B_SPLINE_SURFACE(((1.00005700962391,0.795687417707188,1.),(1.00005494423624,
0.80308940810469,1.),(1.00005396604001,0.806595093358397,1.),(1.00005415449876,
0.805919689953951,1.)))
REPRESENTATION_ITEM('')
SURFACE()
);
#2708=(
BOUNDED_SURFACE()
B_SPLINE_SURFACE(3,2,((#173109,#173110,#173111),(#173112,#173113,#173114),
(#173115,#173116,#173117),(#173118,#173119,#173120),(#173121,#173122,#173123),
(#173124,#173125,#173126)),.UNSPECIFIED.,.F.,.F.,.F.)
B_SPLINE_SURFACE_WITH_KNOTS((4,2,4),(3,3),(0.,0.0178323395635859,0.0356646791271718),
(0.,1.),.UNSPECIFIED.)
GEOMETRIC_REPRESENTATION_ITEM()
RATIONAL_B_SPLINE_SURFACE(((1.,0.825853968826192,1.),(1.,0.819668171116131,
1.),(1.,0.814408476706928,1.),(1.,0.80512037347301,1.),(1.,0.801094867709694,
1.),(1.,0.79748483152198,1.)))
REPRESENTATION_ITEM('')
SURFACE()
);
#2709=(
BOUNDED_SURFACE()
B_SPLINE_SURFACE(3,2,((#173136,#173137,#173138),(#173139,#173140,#173141),
(#173142,#173143,#173144),(#173145,#173146,#173147),(#173148,#173149,#173150),
(#173151,#173152,#173153)),.UNSPECIFIED.,.F.,.F.,.F.)
B_SPLINE_SURFACE_WITH_KNOTS((4,2,4),(3,3),(-3.90312782094781E-18,0.00167965794371986,
0.00335931588743972),(0.,1.),.UNSPECIFIED.)
GEOMETRIC_REPRESENTATION_ITEM()
RATIONAL_B_SPLINE_SURFACE(((1.,0.825853968826192,1.),(1.,0.808295365083271,
1.),(1.,0.789625920673805,1.),(1.,0.749928217285841,1.),(1.,0.728769006116152,
1.),(1.,0.707106781186548,1.)))
REPRESENTATION_ITEM('')
SURFACE()
);
#2710=(
BOUNDED_SURFACE()
B_SPLINE_SURFACE(3,2,((#173168,#173169,#173170),(#173171,#173172,#173173),
(#173174,#173175,#173176),(#173177,#173178,#173179),(#173180,#173181,#173182),
(#173183,#173184,#173185)),.UNSPECIFIED.,.F.,.F.,.F.)
B_SPLINE_SURFACE_WITH_KNOTS((4,2,4),(3,3),(0.,0.00167878022781669,0.00335756045563338),
(0.,1.),.UNSPECIFIED.)
GEOMETRIC_REPRESENTATION_ITEM()
RATIONAL_B_SPLINE_SURFACE(((1.,0.707106781186548,1.),(1.,0.728852565122502,
1.),(1.,0.749558440272865,1.),(1.,0.789217732831704,1.),(1.,0.808313359696353,
1.),(1.,0.825853968826191,1.)))
REPRESENTATION_ITEM('')
SURFACE()
);
#2711=(
BOUNDED_SURFACE()
B_SPLINE_SURFACE(3,2,((#173302,#173303,#173304),(#173305,#173306,#173307),
(#173308,#173309,#173310),(#173311,#173312,#173313),(#173314,#173315,#173316),
(#173317,#173318,#173319)),.UNSPECIFIED.,.F.,.F.,.F.)
B_SPLINE_SURFACE_WITH_KNOTS((4,2,4),(3,3),(0.,0.0176980703187956,0.0353961406375911),
(0.,1.),.UNSPECIFIED.)
GEOMETRIC_REPRESENTATION_ITEM()
RATIONAL_B_SPLINE_SURFACE(((1.,0.797648081014877,1.),(1.,0.801243745289675,
1.),(1.,0.805251011590647,1.),(1.,0.814487862093865,1.),(1.,0.819714636457853,
1.),(1.,0.825853968826193,1.)))
REPRESENTATION_ITEM('')
SURFACE()
);
#2712=(
BOUNDED_SURFACE()
B_SPLINE_SURFACE(3,2,((#173361,#173362,#173363),(#173364,#173365,#173366),
(#173367,#173368,#173369),(#173370,#173371,#173372),(#173373,#173374,#173375),
(#173376,#173377,#173378)),.UNSPECIFIED.,.F.,.F.,.F.)
B_SPLINE_SURFACE_WITH_KNOTS((4,2,4),(3,3),(0.320579494062015,0.325851056440119,
0.331122618818223),(0.,1.),.UNSPECIFIED.)
GEOMETRIC_REPRESENTATION_ITEM()
RATIONAL_B_SPLINE_SURFACE(((1.,0.944716550693843,1.),(1.,0.947183014496352,
1.),(1.,0.949681733718157,1.),(1.,0.954674150124444,1.),(1.,0.957142659869515,
1.),(1.,0.959530911310534,1.)))
REPRESENTATION_ITEM('')
SURFACE()
);
#2713=(
BOUNDED_SURFACE()
B_SPLINE_SURFACE(3,2,((#173512,#173513,#173514),(#173515,#173516,#173517),
(#173518,#173519,#173520),(#173521,#173522,#173523),(#173524,#173525,#173526),
(#173527,#173528,#173529)),.UNSPECIFIED.,.F.,.F.,.F.)
B_SPLINE_SURFACE_WITH_KNOTS((4,2,4),(3,3),(0.,0.0145632072393804,0.0291264144787609),
(0.,1.),.UNSPECIFIED.)
GEOMETRIC_REPRESENTATION_ITEM()
RATIONAL_B_SPLINE_SURFACE(((1.,0.523250899838464,1.),(1.,0.532471350763147,
1.),(1.,0.540347653844846,1.),(1.,0.554302832144208,1.),(1.,0.560377433574518,
1.),(1.,0.565840417962188,1.)))
REPRESENTATION_ITEM('')
SURFACE()
);
#2714=(
BOUNDED_SURFACE()
B_SPLINE_SURFACE(3,2,((#173582,#173583,#173584),(#173585,#173586,#173587),
(#173588,#173589,#173590),(#173591,#173592,#173593),(#173594,#173595,#173596),
(#173597,#173598,#173599)),.UNSPECIFIED.,.F.,.F.,.F.)
B_SPLINE_SURFACE_WITH_KNOTS((4,2,4),(3,3),(-0.000106024816734168,0.00207216577676188,
0.00425035650131637),(-0.000106024947792593,1.),.UNSPECIFIED.)
GEOMETRIC_REPRESENTATION_ITEM()
RATIONAL_B_SPLINE_SURFACE(((1.00010220266629,0.518025387314371,1.),(1.00009466956028,
0.553550545186674,1.),(1.00008751550017,0.587288171340496,1.),(1.00007381194872,
0.651912355251542,1.),(1.00006726786479,0.682773412363203,1.),(1.00006122918042,
0.711251070175717,1.)))
REPRESENTATION_ITEM('')
SURFACE()
);
#2715=(
BOUNDED_SURFACE()
B_SPLINE_SURFACE(3,2,((#173631,#173632,#173633),(#173634,#173635,#173636),
(#173637,#173638,#173639),(#173640,#173641,#173642),(#173643,#173644,#173645),
(#173646,#173647,#173648)),.UNSPECIFIED.,.F.,.F.,.F.)
B_SPLINE_SURFACE_WITH_KNOTS((4,2,4),(3,3),(0.,0.00207126900955203,0.00414253801910405),
(0.,1.),.UNSPECIFIED.)
GEOMETRIC_REPRESENTATION_ITEM()
RATIONAL_B_SPLINE_SURFACE(((1.,0.707106781186548,1.),(1.,0.679626330234824,
1.),(1.,0.650848145227602,1.),(1.,0.589569252159033,1.),(1.,0.556778618705704,
1.),(1.,0.523250899838466,1.)))
REPRESENTATION_ITEM('')
SURFACE()
);
#2716=(
BOUNDED_SURFACE()
B_SPLINE_SURFACE(3,2,((#173673,#173674,#173675),(#173676,#173677,#173678),
(#173679,#173680,#173681),(#173682,#173683,#173684),(#173685,#173686,#173687),
(#173688,#173689,#173690)),.UNSPECIFIED.,.F.,.F.,.F.)
B_SPLINE_SURFACE_WITH_KNOTS((4,2,4),(3,3),(-3.45632130015141E-5,0.0146992078328598,
0.029432978878721),(0.,1.000034563213),.UNSPECIFIED.)
GEOMETRIC_REPRESENTATION_ITEM()
RATIONAL_B_SPLINE_SURFACE(((1.,0.566167776253824,1.00002998927111),(1.,
0.560666809856082,1.00003036953326),(1.,0.554544924441235,1.00003079271732),
(1.,0.540460350933127,1.00003176633355),(1.,0.532502109028823,1.00003231645837),
(1.,0.523168760654905,1.00003296163938)))
REPRESENTATION_ITEM('')
SURFACE()
);
#2717=(
BOUNDED_SURFACE()
B_SPLINE_SURFACE(3,2,((#173700,#173701,#173702),(#173703,#173704,#173705),
(#173706,#173707,#173708),(#173709,#173710,#173711)),.UNSPECIFIED.,.F.,
 .F.,.F.)
B_SPLINE_SURFACE_WITH_KNOTS((4,4),(3,3),(-3.41800396463488E-5,0.000687703280413445),
(-3.41800396463774E-5,1.),.UNSPECIFIED.)
GEOMETRIC_REPRESENTATION_ITEM()
RATIONAL_B_SPLINE_SURFACE(((1.00003076363761,0.549976566282789,1.),(1.00003081026943,
0.549294416404309,1.),(1.00003037623388,0.555643671106268,1.),(1.00002954389936,
0.56781941063233,1.)))
REPRESENTATION_ITEM('')
SURFACE()
);
#2718=(
BOUNDED_SURFACE()
B_SPLINE_SURFACE(3,2,((#173748,#173749,#173750),(#173751,#173752,#173753),
(#173754,#173755,#173756),(#173757,#173758,#173759)),.UNSPECIFIED.,.F.,
 .F.,.F.)
B_SPLINE_SURFACE_WITH_KNOTS((4,4),(3,3),(-1.38777878078145E-17,0.0332202089949022),
(0.,1.),.UNSPECIFIED.)
GEOMETRIC_REPRESENTATION_ITEM()
RATIONAL_B_SPLINE_SURFACE(((1.,0.736495153922513,1.),(1.,0.738798609451216,
1.),(1.,0.741580133014481,1.),(1.,0.745472778587061,1.)))
REPRESENTATION_ITEM('')
SURFACE()
);
#2719=(
BOUNDED_SURFACE()
B_SPLINE_SURFACE(3,2,((#173784,#173785,#173786),(#173787,#173788,#173789),
(#173790,#173791,#173792),(#173793,#173794,#173795)),.UNSPECIFIED.,.F.,
 .F.,.F.)
B_SPLINE_SURFACE_WITH_KNOTS((4,4),(3,3),(0.,0.0333425790106738),(0.,1.),
 .UNSPECIFIED.)
GEOMETRIC_REPRESENTATION_ITEM()
RATIONAL_B_SPLINE_SURFACE(((1.,0.619253049823353,1.),(1.,0.62903050118076,
1.),(1.,0.635777469330956,1.),(1.,0.641321251913794,1.)))
REPRESENTATION_ITEM('')
SURFACE()
);
#2720=(
BOUNDED_SURFACE()
B_SPLINE_SURFACE(3,2,((#173820,#173821,#173822),(#173823,#173824,#173825),
(#173826,#173827,#173828),(#173829,#173830,#173831)),.UNSPECIFIED.,.F.,
 .F.,.F.)
B_SPLINE_SURFACE_WITH_KNOTS((4,4),(3,3),(0.,9.64176041888312E-5),(0.,1.),
 .UNSPECIFIED.)
GEOMETRIC_REPRESENTATION_ITEM()
RATIONAL_B_SPLINE_SURFACE(((1.,0.801085834760579,1.),(1.,0.800109483270879,
1.),(1.,0.799128688610329,1.),(1.,0.798143461627153,1.)))
REPRESENTATION_ITEM('')
SURFACE()
);
#2721=(
BOUNDED_SURFACE()
B_SPLINE_SURFACE(3,2,((#173843,#173844,#173845),(#173846,#173847,#173848),
(#173849,#173850,#173851),(#173852,#173853,#173854)),.UNSPECIFIED.,.F.,
 .F.,.F.)
B_SPLINE_SURFACE_WITH_KNOTS((4,4),(3,3),(-1.38777878078145E-17,0.0333345287175385),
(0.,1.),.UNSPECIFIED.)
GEOMETRIC_REPRESENTATION_ITEM()
RATIONAL_B_SPLINE_SURFACE(((1.,0.779737900546642,1.),(1.,0.785266544814036,
1.),(1.,0.791920621206337,1.),(1.,0.801085834760578,1.)))
REPRESENTATION_ITEM('')
SURFACE()
);
#2722=(
BOUNDED_SURFACE()
B_SPLINE_SURFACE(3,2,((#173881,#173882,#173883),(#173884,#173885,#173886),
(#173887,#173888,#173889),(#173890,#173891,#173892)),.UNSPECIFIED.,.F.,
 .F.,.F.)
B_SPLINE_SURFACE_WITH_KNOTS((4,4),(3,3),(0.,0.0278605201857756),(0.,1.),
 .UNSPECIFIED.)
GEOMETRIC_REPRESENTATION_ITEM()
RATIONAL_B_SPLINE_SURFACE(((1.,0.55476848021506,1.),(1.,0.56887897086178,
1.),(1.,0.579290070452688,1.),(1.,0.587985430396658,1.)))
REPRESENTATION_ITEM('')
SURFACE()
);
#2723=(
BOUNDED_SURFACE()
B_SPLINE_SURFACE(3,2,((#173922,#173923,#173924),(#173925,#173926,#173927),
(#173928,#173929,#173930),(#173931,#173932,#173933),(#173934,#173935,#173936),
(#173937,#173938,#173939)),.UNSPECIFIED.,.F.,.F.,.F.)
B_SPLINE_SURFACE_WITH_KNOTS((4,2,4),(3,3),(-1.95156391047391E-18,0.00176358033920161,
0.00352716067840323),(0.,1.),.UNSPECIFIED.)
GEOMETRIC_REPRESENTATION_ITEM()
RATIONAL_B_SPLINE_SURFACE(((1.,0.554768480215054,1.),(1.,0.582178779071266,
1.),(1.,0.608552864303934,1.),(1.,0.659476319336264,1.),(1.,0.684131843499319,
1.),(1.,0.707106781186548,1.)))
REPRESENTATION_ITEM('')
SURFACE()
);
#2724=(
BOUNDED_SURFACE()
B_SPLINE_SURFACE(3,2,((#174089,#174090,#174091),(#174092,#174093,#174094),
(#174095,#174096,#174097),(#174098,#174099,#174100),(#174101,#174102,#174103),
(#174104,#174105,#174106)),.UNSPECIFIED.,.F.,.F.,.F.)
B_SPLINE_SURFACE_WITH_KNOTS((4,2,4),(3,3),(0.,0.00192660600180124,0.00385321200360248),
(0.,1.),.UNSPECIFIED.)
GEOMETRIC_REPRESENTATION_ITEM()
RATIONAL_B_SPLINE_SURFACE(((1.,0.707106781186548,1.),(1.,0.732617243564259,
1.),(1.,0.7565692429617,1.),(1.,0.801993213239136,1.),(1.,0.823627327095932,
1.),(1.,0.843176610515832,1.)))
REPRESENTATION_ITEM('')
SURFACE()
);
#2725=(
BOUNDED_SURFACE()
B_SPLINE_SURFACE(3,2,((#174125,#174126,#174127),(#174128,#174129,#174130),
(#174131,#174132,#174133),(#174134,#174135,#174136)),.UNSPECIFIED.,.F.,
 .F.,.F.)
B_SPLINE_SURFACE_WITH_KNOTS((4,4),(3,3),(0.,0.024690830875569),(0.,1.),
 .UNSPECIFIED.)
GEOMETRIC_REPRESENTATION_ITEM()
RATIONAL_B_SPLINE_SURFACE(((1.,0.821022196159299,1.),(1.,0.827229968384993,
1.),(1.,0.834396885388283,1.),(1.,0.84317661051583,1.)))
REPRESENTATION_ITEM('')
SURFACE()
);
#2726=(
BOUNDED_SURFACE()
B_SPLINE_SURFACE(3,2,((#174163,#174164,#174165),(#174166,#174167,#174168),
(#174169,#174170,#174171),(#174172,#174173,#174174),(#174175,#174176,#174177),
(#174178,#174179,#174180),(#174181,#174182,#174183),(#174184,#174185,#174186)),
 .UNSPECIFIED.,.F.,.F.,.F.)
B_SPLINE_SURFACE_WITH_KNOTS((4,2,2,4),(3,3),(0.,0.000301902853038141,0.000452854279557211,
0.000603805706076282),(0.,1.),.UNSPECIFIED.)
GEOMETRIC_REPRESENTATION_ITEM()
RATIONAL_B_SPLINE_SURFACE(((1.,0.702399276808562,1.),(1.,0.672208297052869,
1.),(1.,0.639172707788597,1.),(1.,0.593013313775285,1.),(1.,0.577958663413849,
1.),(1.,0.550545486207946,1.),(1.,0.538469268822416,1.),(1.,0.528679393385783,
1.)))
REPRESENTATION_ITEM('')
SURFACE()
);
#2727=(
BOUNDED_SURFACE()
B_SPLINE_SURFACE(3,2,((#174264,#174265,#174266),(#174267,#174268,#174269),
(#174270,#174271,#174272),(#174273,#174274,#174275)),.UNSPECIFIED.,.F.,
 .F.,.F.)
B_SPLINE_SURFACE_WITH_KNOTS((4,4),(3,3),(0.,8.95703543583319E-5),(0.,1.),
 .UNSPECIFIED.)
GEOMETRIC_REPRESENTATION_ITEM()
RATIONAL_B_SPLINE_SURFACE(((1.,0.821022196159299,1.),(1.,0.818079073177133,
1.),(1.,0.814610488520586,1.),(1.,0.810617639934139,1.)))
REPRESENTATION_ITEM('')
SURFACE()
);
#2728=(
BOUNDED_SURFACE()
B_SPLINE_SURFACE(3,2,((#174299,#174300,#174301),(#174302,#174303,#174304),
(#174305,#174306,#174307),(#174308,#174309,#174310)),.UNSPECIFIED.,.F.,
 .F.,.F.)
B_SPLINE_SURFACE_WITH_KNOTS((4,4),(3,3),(0.,0.0240963563036403),(0.,1.),
 .UNSPECIFIED.)
GEOMETRIC_REPRESENTATION_ITEM()
RATIONAL_B_SPLINE_SURFACE(((1.,0.533775524284036,1.),(1.,0.547394060950047,
1.),(1.,0.557948204678947,1.),(1.,0.566908467907053,1.)))
REPRESENTATION_ITEM('')
SURFACE()
);
#2729=(
BOUNDED_SURFACE()
B_SPLINE_SURFACE(3,2,((#174339,#174340,#174341),(#174342,#174343,#174344),
(#174345,#174346,#174347),(#174348,#174349,#174350),(#174351,#174352,#174353),
(#174354,#174355,#174356)),.UNSPECIFIED.,.F.,.F.,.F.)
B_SPLINE_SURFACE_WITH_KNOTS((4,2,4),(3,3),(0.,0.00196642364705715,0.0039328472941143),
(0.,1.),.UNSPECIFIED.)
GEOMETRIC_REPRESENTATION_ITEM()
RATIONAL_B_SPLINE_SURFACE(((1.,0.533775524284043,1.),(1.,0.565273803175765,
1.),(1.,0.595391641981992,1.),(1.,0.653340354191305,1.),(1.,0.681207781927973,
1.),(1.,0.707106781186552,1.)))
REPRESENTATION_ITEM('')
SURFACE()
);
#2730=(
BOUNDED_SURFACE()
B_SPLINE_SURFACE(3,2,((#174388,#174389,#174390),(#174391,#174392,#174393),
(#174394,#174395,#174396),(#174397,#174398,#174399),(#174400,#174401,#174402),
(#174403,#174404,#174405)),.UNSPECIFIED.,.F.,.F.,.F.)
B_SPLINE_SURFACE_WITH_KNOTS((4,2,4),(3,3),(0.,0.00196532227871992,0.00393064455743984),
(0.,1.),.UNSPECIFIED.)
GEOMETRIC_REPRESENTATION_ITEM()
RATIONAL_B_SPLINE_SURFACE(((1.,0.70710678118655,1.),(1.,0.681045297773967,
1.),(1.,0.653805231917789,1.),(1.,0.596033371554667,1.),(1.,0.565216504169612,
1.),(1.,0.533775524284038,1.)))
REPRESENTATION_ITEM('')
SURFACE()
);
#2731=(
BOUNDED_SURFACE()
B_SPLINE_SURFACE(3,2,((#174467,#174468,#174469),(#174470,#174471,#174472),
(#174473,#174474,#174475),(#174476,#174477,#174478)),.UNSPECIFIED.,.F.,
 .F.,.F.)
B_SPLINE_SURFACE_WITH_KNOTS((4,4),(3,3),(1.38777878078145E-17,0.0238258198664154),
(0.,1.),.UNSPECIFIED.)
GEOMETRIC_REPRESENTATION_ITEM()
RATIONAL_B_SPLINE_SURFACE(((1.,0.566606711022863,1.),(1.,0.557709627588123,
1.),(1.,0.547241836069268,1.),(1.,0.533775524284033,1.)))
REPRESENTATION_ITEM('')
SURFACE()
);
#2732=(
BOUNDED_SURFACE()
B_SPLINE_SURFACE(3,2,((#174505,#174506,#174507),(#174508,#174509,#174510),
(#174511,#174512,#174513),(#174514,#174515,#174516),(#174517,#174518,#174519),
(#174520,#174521,#174522)),.UNSPECIFIED.,.F.,.F.,.F.)
B_SPLINE_SURFACE_WITH_KNOTS((4,2,4),(3,3),(0.28787290846928,0.292960043496213,
0.298047178523145),(0.,1.),.UNSPECIFIED.)
GEOMETRIC_REPRESENTATION_ITEM()
RATIONAL_B_SPLINE_SURFACE(((1.,0.948000837587232,1.),(1.,0.950253148926149,
1.),(1.,0.952526342948766,1.),(1.,0.957029990073055,1.),(1.,0.959243464400477,
1.),(1.,0.961372004230729,1.)))
REPRESENTATION_ITEM('')
SURFACE()
);
#2733=(
BOUNDED_SURFACE()
B_SPLINE_SURFACE(3,2,((#174589,#174590,#174591),(#174592,#174593,#174594),
(#174595,#174596,#174597),(#174598,#174599,#174600),(#174601,#174602,#174603),
(#174604,#174605,#174606)),.UNSPECIFIED.,.F.,.F.,.F.)
B_SPLINE_SURFACE_WITH_KNOTS((4,2,4),(3,3),(0.,0.00160286774303482,0.00320573548606963),
(0.,1.),.UNSPECIFIED.)
GEOMETRIC_REPRESENTATION_ITEM()
RATIONAL_B_SPLINE_SURFACE(((1.,0.819627815321769,1.),(1.,0.802865620897526,
1.),(1.,0.785107826354221,1.),(1.,0.747495184421159,1.),(1.,0.727508688529169,
1.),(1.,0.707106781186548,1.)))
REPRESENTATION_ITEM('')
SURFACE()
);
#2734=(
BOUNDED_SURFACE()
B_SPLINE_SURFACE(3,2,((#174631,#174632,#174633),(#174634,#174635,#174636),
(#174637,#174638,#174639),(#174640,#174641,#174642),(#174643,#174644,#174645),
(#174646,#174647,#174648)),.UNSPECIFIED.,.F.,.F.,.F.)
B_SPLINE_SURFACE_WITH_KNOTS((4,2,4),(3,3),(0.,0.00160216910094088,0.00320433820188177),
(0.,1.),.UNSPECIFIED.)
GEOMETRIC_REPRESENTATION_ITEM()
RATIONAL_B_SPLINE_SURFACE(((1.,0.707106781186548,1.),(1.,0.727576984679287,
1.),(1.,0.747141913282259,1.),(1.,0.784726895243881,1.),(1.,0.80287971578069,
1.),(1.,0.819627815322113,1.)))
REPRESENTATION_ITEM('')
SURFACE()
);
#2735=(
BOUNDED_SURFACE()
B_SPLINE_SURFACE(3,2,((#174664,#174665,#174666),(#174667,#174668,#174669),
(#174670,#174671,#174672),(#174673,#174674,#174675)),.UNSPECIFIED.,.F.,
 .F.,.F.)
B_SPLINE_SURFACE_WITH_KNOTS((4,4),(3,3),(0.,0.0300693678107436),(0.,1.),
 .UNSPECIFIED.)
GEOMETRIC_REPRESENTATION_ITEM()
RATIONAL_B_SPLINE_SURFACE(((1.,0.79694160937888,1.),(1.,0.803005840650144,
1.),(1.,0.810197796192684,1.),(1.,0.819627815321757,1.)))
REPRESENTATION_ITEM('')
SURFACE()
);
#2736=(
BOUNDED_SURFACE()
B_SPLINE_SURFACE(3,2,((#174702,#174703,#174704),(#174705,#174706,#174707),
(#174708,#174709,#174710),(#174711,#174712,#174713)),.UNSPECIFIED.,.F.,
 .F.,.F.)
B_SPLINE_SURFACE_WITH_KNOTS((4,4),(3,3),(0.,0.0298008594779328),(0.,1.),
 .UNSPECIFIED.)
GEOMETRIC_REPRESENTATION_ITEM()
RATIONAL_B_SPLINE_SURFACE(((1.,0.819627815321769,1.),(1.,0.81028158060527,
1.),(1.,0.803135207628788,1.),(1.,0.797103929716951,1.)))
REPRESENTATION_ITEM('')
SURFACE()
);
#2737=(
BOUNDED_SURFACE()
B_SPLINE_SURFACE(3,2,((#174764,#174765,#174766),(#174767,#174768,#174769),
(#174770,#174771,#174772),(#174773,#174774,#174775)),.UNSPECIFIED.,.F.,
 .F.,.F.)
B_SPLINE_SURFACE_WITH_KNOTS((4,4),(3,3),(0.,0.0322629186945109),(0.,1.),
 .UNSPECIFIED.)
GEOMETRIC_REPRESENTATION_ITEM()
RATIONAL_B_SPLINE_SURFACE(((1.,0.591243989422541,1.),(1.,0.603807915079894,
1.),(1.,0.612569262394175,1.),(1.,0.619783312569531,1.)))
REPRESENTATION_ITEM('')
SURFACE()
);
#2738=(
BOUNDED_SURFACE()
B_SPLINE_SURFACE(3,2,((#174804,#174805,#174806),(#174807,#174808,#174809),
(#174810,#174811,#174812),(#174813,#174814,#174815),(#174816,#174817,#174818),
(#174819,#174820,#174821)),.UNSPECIFIED.,.F.,.F.,.F.)
B_SPLINE_SURFACE_WITH_KNOTS((4,2,4),(3,3),(-4.11996825544492E-18,0.00145505538520654,
0.00291011077041309),(0.,1.),.UNSPECIFIED.)
GEOMETRIC_REPRESENTATION_ITEM()
RATIONAL_B_SPLINE_SURFACE(((1.,0.591243989422539,1.),(1.,0.611831201619161,
1.),(1.,0.631800177390031,1.),(1.,0.67052755959961,1.),(1.,0.68940594547505,
1.),(1.,0.707106781186548,1.)))
REPRESENTATION_ITEM('')
SURFACE()
);
#2739=(
BOUNDED_SURFACE()
B_SPLINE_SURFACE(3,2,((#174844,#174845,#174846),(#174847,#174848,#174849),
(#174850,#174851,#174852),(#174853,#174854,#174855),(#174856,#174857,#174858),
(#174859,#174860,#174861)),.UNSPECIFIED.,.F.,.F.,.F.)
B_SPLINE_SURFACE_WITH_KNOTS((4,2,4),(3,3),(0.,0.00145467289932797,0.00290934579865593),
(0.,1.),.UNSPECIFIED.)
GEOMETRIC_REPRESENTATION_ITEM()
RATIONAL_B_SPLINE_SURFACE(((1.,0.707106781186548,1.),(1.,0.689351003959322,
1.),(1.,0.670875374619751,1.),(1.,0.63219865253591,1.),(1.,0.61183462187758,
1.),(1.,0.591243989422533,1.)))
REPRESENTATION_ITEM('')
SURFACE()
);
#2740=(
BOUNDED_SURFACE()
B_SPLINE_SURFACE(3,2,((#174975,#174976,#174977),(#174978,#174979,#174980),
(#174981,#174982,#174983),(#174984,#174985,#174986)),.UNSPECIFIED.,.F.,
 .F.,.F.)
B_SPLINE_SURFACE_WITH_KNOTS((4,4),(3,3),(0.,0.0319950621716305),(0.,1.),
 .UNSPECIFIED.)
GEOMETRIC_REPRESENTATION_ITEM()
RATIONAL_B_SPLINE_SURFACE(((1.,0.619604282534389,1.),(1.,0.612421729644488,
1.),(1.,0.603704627405285,1.),(1.,0.591243989422539,1.)))
REPRESENTATION_ITEM('')
SURFACE()
);
#2741=(
BOUNDED_SURFACE()
B_SPLINE_SURFACE(3,2,((#175013,#175014,#175015),(#175016,#175017,#175018),
(#175019,#175020,#175021),(#175022,#175023,#175024),(#175025,#175026,#175027),
(#175028,#175029,#175030)),.UNSPECIFIED.,.F.,.F.,.F.)
B_SPLINE_SURFACE_WITH_KNOTS((4,2,4),(3,3),(0.0131958327712131,0.0172517018793722,
0.0213075709875312),(0.,1.),.UNSPECIFIED.)
GEOMETRIC_REPRESENTATION_ITEM()
RATIONAL_B_SPLINE_SURFACE(((1.,0.962986864031359,1.),(1.,0.964634124968522,
1.),(1.,0.966223563289428,1.),(1.,0.969200421482677,1.),(1.,0.970562510847277,
1.),(1.,0.97174760310377,1.)))
REPRESENTATION_ITEM('')
SURFACE()
);
#2742=(
BOUNDED_SURFACE()
B_SPLINE_SURFACE(3,2,((#175133,#175134,#175135),(#175136,#175137,#175138),
(#175139,#175140,#175141),(#175142,#175143,#175144),(#175145,#175146,#175147),
(#175148,#175149,#175150)),.UNSPECIFIED.,.F.,.F.,.F.)
B_SPLINE_SURFACE_WITH_KNOTS((4,2,4),(3,3),(0.,0.00117596609447381,0.00235193218894761),
(0.,1.),.UNSPECIFIED.)
GEOMETRIC_REPRESENTATION_ITEM()
RATIONAL_B_SPLINE_SURFACE(((1.,0.773031559588625,1.),(1.,0.762507689934388,
1.),(1.,0.751714784265694,1.),(1.,0.729663967046365,1.),(1.,0.718328240933523,
1.),(1.,0.707106781186548,1.)))
REPRESENTATION_ITEM('')
SURFACE()
);
#2743=(
BOUNDED_SURFACE()
B_SPLINE_SURFACE(3,2,((#175172,#175173,#175174),(#175175,#175176,#175177),
(#175178,#175179,#175180),(#175181,#175182,#175183),(#175184,#175185,#175186),
(#175187,#175188,#175189)),.UNSPECIFIED.,.F.,.F.,.F.)
B_SPLINE_SURFACE_WITH_KNOTS((4,2,4),(3,3),(0.,0.00117590500970525,0.00235181001941051),
(0.,1.),.UNSPECIFIED.)
GEOMETRIC_REPRESENTATION_ITEM()
RATIONAL_B_SPLINE_SURFACE(((1.,0.707106781186548,1.),(1.,0.718331568550412,
1.),(1.,0.729459486848599,1.),(1.,0.751510898082342,1.),(1.,0.762507564122321,
1.),(1.,0.773031559588357,1.)))
REPRESENTATION_ITEM('')
SURFACE()
);
#2744=(
BOUNDED_SURFACE()
B_SPLINE_SURFACE(3,2,((#175205,#175206,#175207),(#175208,#175209,#175210),
(#175211,#175212,#175213),(#175214,#175215,#175216)),.UNSPECIFIED.,.F.,
 .F.,.F.)
B_SPLINE_SURFACE_WITH_KNOTS((4,4),(3,3),(0.,0.0360938777358061),(0.,1.),
 .UNSPECIFIED.)
GEOMETRIC_REPRESENTATION_ITEM()
RATIONAL_B_SPLINE_SURFACE(((1.,0.756551244268665,1.),(1.,0.760698019999951,
1.),(1.,0.765742819248909,1.),(1.,0.77303155958863,1.)))
REPRESENTATION_ITEM('')
SURFACE()
);
#2745=(
BOUNDED_SURFACE()
B_SPLINE_SURFACE(3,2,((#175240,#175241,#175242),(#175243,#175244,#175245),
(#175246,#175247,#175248),(#175249,#175250,#175251)),.UNSPECIFIED.,.F.,
 .F.,.F.)
B_SPLINE_SURFACE_WITH_KNOTS((4,4),(3,3),(0.,0.0358270578054484),(0.,1.),
 .UNSPECIFIED.)
GEOMETRIC_REPRESENTATION_ITEM()
RATIONAL_B_SPLINE_SURFACE(((1.,0.773031559588625,1.),(1.,0.765796148320668,
1.),(1.,0.760773695826815,1.),(1.,0.756642830410354,1.)))
REPRESENTATION_ITEM('')
SURFACE()
);
#2746=(
BOUNDED_SURFACE()
B_SPLINE_SURFACE(3,2,((#175301,#175302,#175303),(#175304,#175305,#175306),
(#175307,#175308,#175309),(#175310,#175311,#175312)),.UNSPECIFIED.,.F.,
 .F.,.F.)
B_SPLINE_SURFACE_WITH_KNOTS((4,4),(3,3),(0.,0.0372541843113205),(0.,1.),
 .UNSPECIFIED.)
GEOMETRIC_REPRESENTATION_ITEM()
RATIONAL_B_SPLINE_SURFACE(((1.,0.653853118868809,1.),(1.,0.660540277946251,
1.),(1.,0.664920252154014,1.),(1.,0.668488966322263,1.)))
REPRESENTATION_ITEM('')
SURFACE()
);
#2747=(
BOUNDED_SURFACE()
B_SPLINE_SURFACE(3,2,((#175336,#175337,#175338),(#175339,#175340,#175341),
(#175342,#175343,#175344),(#175345,#175346,#175347),(#175348,#175349,#175350),
(#175351,#175352,#175353)),.UNSPECIFIED.,.F.,.F.,.F.)
B_SPLINE_SURFACE_WITH_KNOTS((4,2,4),(3,3),(-0.000172720172426045,0.00108574887884081,
0.00234421795569043),(-0.000172720198008812,1.),.UNSPECIFIED.)
GEOMETRIC_REPRESENTATION_ITEM()
RATIONAL_B_SPLINE_SURFACE(((1.00012114331385,0.649307622257087,1.),(1.00011736582696,
0.660242900607159,1.),(1.00011369038462,0.670882774756897,1.),(1.0001065636278,
0.691513705317947,1.),(1.00010308656314,0.70157930476702,1.),(1.00009984815327,
0.710954033119057,1.)))
REPRESENTATION_ITEM('')
SURFACE()
);
#2748=(
BOUNDED_SURFACE()
B_SPLINE_SURFACE(3,2,((#175373,#175374,#175375),(#175376,#175377,#175378),
(#175379,#175380,#175381),(#175382,#175383,#175384),(#175385,#175386,#175387),
(#175388,#175389,#175390)),.UNSPECIFIED.,.F.,.F.,.F.)
B_SPLINE_SURFACE_WITH_KNOTS((4,2,4),(3,3),(0.,0.00108572934543333,0.00217145869086666),
(0.,1.),.UNSPECIFIED.)
GEOMETRIC_REPRESENTATION_ITEM()
RATIONAL_B_SPLINE_SURFACE(((1.,0.707106781186548,1.),(1.,0.698862672165929,
1.),(1.,0.690309395332211,1.),(1.,0.672521089753096,1.),(1.,0.663221545283971,
1.),(1.,0.653853118868808,1.)))
REPRESENTATION_ITEM('')
SURFACE()
);
#2749=(
BOUNDED_SURFACE()
B_SPLINE_SURFACE(3,2,((#175477,#175478,#175479),(#175480,#175481,#175482),
(#175483,#175484,#175485),(#175486,#175487,#175488)),.UNSPECIFIED.,.F.,
 .F.,.F.)
B_SPLINE_SURFACE_WITH_KNOTS((4,4),(3,3),(0.,0.0369876550821707),(0.,1.),
 .UNSPECIFIED.)
GEOMETRIC_REPRESENTATION_ITEM()
RATIONAL_B_SPLINE_SURFACE(((1.,0.668412873076039,1.),(1.,0.66485630627401,
1.),(1.,0.660493096380151,1.),(1.,0.653853118868808,1.)))
REPRESENTATION_ITEM('')
SURFACE()
);
#2750=(
BOUNDED_SURFACE()
B_SPLINE_SURFACE(3,2,((#175554,#175555,#175556),(#175557,#175558,#175559),
(#175560,#175561,#175562),(#175563,#175564,#175565),(#175566,#175567,#175568),
(#175569,#175570,#175571)),.UNSPECIFIED.,.F.,.F.,.F.)
B_SPLINE_SURFACE_WITH_KNOTS((4,2,4),(3,3),(0.024832888249526,0.028058706716499,
0.0312845251834718),(0.,1.),.UNSPECIFIED.)
GEOMETRIC_REPRESENTATION_ITEM()
RATIONAL_B_SPLINE_SURFACE(((1.,0.973275621725783,1.),(1.,0.974072863725218,
1.),(1.,0.974738796346974,1.),(1.,0.975743605366306,1.),(1.,0.976080910223402,
1.),(1.,0.976217656750926,1.)))
REPRESENTATION_ITEM('')
SURFACE()
);
#2751=(
BOUNDED_SURFACE()
B_SPLINE_SURFACE(3,2,((#175587,#175588,#175589),(#175590,#175591,#175592),
(#175593,#175594,#175595),(#175596,#175597,#175598)),.UNSPECIFIED.,.F.,
 .F.,.F.)
B_SPLINE_SURFACE_WITH_KNOTS((4,4),(3,3),(-4.11996825544492E-18,0.00195778789380024),
(0.,1.),.UNSPECIFIED.)
GEOMETRIC_REPRESENTATION_ITEM()
RATIONAL_B_SPLINE_SURFACE(((1.,0.716457303923414,1.),(1.,0.713268765085681,
1.),(1.,0.710104564531573,1.),(1.,0.707106781186529,1.)))
REPRESENTATION_ITEM('')
SURFACE()
);
#2752=(
BOUNDED_SURFACE()
B_SPLINE_SURFACE(3,2,((#175608,#175609,#175610),(#175611,#175612,#175613),
(#175614,#175615,#175616),(#175617,#175618,#175619)),.UNSPECIFIED.,.F.,
 .F.,.F.)
B_SPLINE_SURFACE_WITH_KNOTS((4,4),(3,3),(0.,0.00195778753723149),(0.,1.),
 .UNSPECIFIED.)
GEOMETRIC_REPRESENTATION_ITEM()
RATIONAL_B_SPLINE_SURFACE(((1.,0.707106781186543,1.),(1.,0.710074099671655,
1.),(1.,0.713236629341983,1.),(1.,0.716457303923398,1.)))
REPRESENTATION_ITEM('')
SURFACE()
);
#2753=(
BOUNDED_SURFACE()
B_SPLINE_SURFACE(3,2,((#175623,#175624,#175625),(#175626,#175627,#175628),
(#175629,#175630,#175631),(#175632,#175633,#175634)),.UNSPECIFIED.,.F.,
 .F.,.F.)
B_SPLINE_SURFACE_WITH_KNOTS((4,4),(3,3),(0.,0.0385835973699829),(0.,1.),
 .UNSPECIFIED.)
GEOMETRIC_REPRESENTATION_ITEM()
RATIONAL_B_SPLINE_SURFACE(((1.,0.713879290671428,1.),(1.,0.71450712730611,
1.),(1.,0.715277846561214,1.),(1.,0.716457303923418,1.)))
REPRESENTATION_ITEM('')
SURFACE()
);
#2754=(
BOUNDED_SURFACE()
B_SPLINE_SURFACE(3,2,((#175654,#175655,#175656),(#175657,#175658,#175659),
(#175660,#175661,#175662),(#175663,#175664,#175665)),.UNSPECIFIED.,.F.,
 .F.,.F.)
B_SPLINE_SURFACE_WITH_KNOTS((4,4),(3,3),(0.,0.038317388945353),(0.,1.),
 .UNSPECIFIED.)
GEOMETRIC_REPRESENTATION_ITEM()
RATIONAL_B_SPLINE_SURFACE(((1.,0.716457303923414,1.),(1.,0.715285870443621,
1.),(1.,0.714517981140503,1.),(1.,0.713892198341303,1.)))
REPRESENTATION_ITEM('')
SURFACE()
);
#2755=(
BOUNDED_SURFACE()
B_SPLINE_SURFACE(3,2,((#175747,#175748,#175749),(#175750,#175751,#175752),
(#175753,#175754,#175755),(#175756,#175757,#175758)),.UNSPECIFIED.,.F.,
 .F.,.F.)
B_SPLINE_SURFACE_WITH_KNOTS((4,4),(3,3),(-1.62187915626604E-5,0.000794016598505311),
(0.,1.00001621879156),.UNSPECIFIED.)
GEOMETRIC_REPRESENTATION_ITEM()
RATIONAL_B_SPLINE_SURFACE(((1.,0.916158202477454,1.00000271962528),(1.,
0.931371211352859,1.00000222615204),(1.,0.942410544587803,1.00000186806275),
(1.,0.948459380997912,1.00000167185311)))
REPRESENTATION_ITEM('')
SURFACE()
);
#2756=(
BOUNDED_SURFACE()
B_SPLINE_SURFACE(3,2,((#175770,#175771,#175772),(#175773,#175774,#175775),
(#175776,#175777,#175778),(#175779,#175780,#175781),(#175782,#175783,#175784),
(#175785,#175786,#175787)),.UNSPECIFIED.,.F.,.F.,.F.)
B_SPLINE_SURFACE_WITH_KNOTS((4,2,4),(3,3),(-2.35539541778838E-5,0.000414679582686121,
0.000852913119550131),(-0.00068744155822166,1.00002355395418),
 .UNSPECIFIED.)
GEOMETRIC_REPRESENTATION_ITEM()
RATIONAL_B_SPLINE_SURFACE(((1.00026536769246,0.806984358134055,1.00000908631671),
(1.00026576129372,0.806698071587169,1.00000909979381),(1.00026384744406,
0.80809011338651,1.00000903426268),(1.00026239826983,0.809144172726734,
1.00000898464226),(1.00026303812725,0.808678771345985,1.00000900655128),
(1.00027069226676,0.803111519968988,1.00000926863268)))
REPRESENTATION_ITEM('')
SURFACE()
);
#2757=(
BOUNDED_SURFACE()
B_SPLINE_SURFACE(3,2,((#175807,#175808,#175809),(#175810,#175811,#175812),
(#175813,#175814,#175815),(#175816,#175817,#175818)),.UNSPECIFIED.,.F.,
 .F.,.F.)
B_SPLINE_SURFACE_WITH_KNOTS((4,4),(3,3),(0.,0.000650122732446382),(0.,1.),
 .UNSPECIFIED.)
GEOMETRIC_REPRESENTATION_ITEM()
RATIONAL_B_SPLINE_SURFACE(((1.,0.714558059459819,1.),(1.,0.714557241617472,
1.),(1.,0.714330794970796,1.),(1.,0.71387929067142,1.)))
REPRESENTATION_ITEM('')
SURFACE()
);
#2758=(
BOUNDED_SURFACE()
B_SPLINE_SURFACE(3,2,((#175826,#175827,#175828),(#175829,#175830,#175831),
(#175832,#175833,#175834),(#175835,#175836,#175837)),.UNSPECIFIED.,.F.,
 .F.,.F.)
B_SPLINE_SURFACE_WITH_KNOTS((4,4),(3,3),(-1.0842021724855E-19,0.000650371461981817),
(0.,1.),.UNSPECIFIED.)
GEOMETRIC_REPRESENTATION_ITEM()
RATIONAL_B_SPLINE_SURFACE(((1.,0.668488966322264,1.),(1.,0.665851831765851,
1.),(1.,0.664481097979681,1.),(1.,0.664473794614064,1.)))
REPRESENTATION_ITEM('')
SURFACE()
);
#2759=(
BOUNDED_SURFACE()
B_SPLINE_SURFACE(3,2,((#175843,#175844,#175845),(#175846,#175847,#175848),
(#175849,#175850,#175851),(#175852,#175853,#175854),(#175855,#175856,#175857),
(#175858,#175859,#175860),(#175861,#175862,#175863),(#175864,#175865,#175866),
(#175867,#175868,#175869),(#175870,#175871,#175872),(#175873,#175874,#175875),
(#175876,#175877,#175878),(#175879,#175880,#175881),(#175882,#175883,#175884)),
 .UNSPECIFIED.,.F.,.F.,.F.)
B_SPLINE_SURFACE_WITH_KNOTS((4,2,2,2,2,2,4),(3,3),(0.00807927244133089,
0.00881458117408921,0.00918223554046837,0.00954988990684753,0.0099175442732267,
0.0102851986396059,0.0110205073723642),(0.,1.),.UNSPECIFIED.)
GEOMETRIC_REPRESENTATION_ITEM()
RATIONAL_B_SPLINE_SURFACE(((1.,0.707106781186548,1.),(1.,0.705697402766896,
1.),(1.,0.704316028414221,1.),(1.,0.702287640598182,1.),(1.,0.70162085852966,
1.),(1.,0.700346303389684,1.),(1.,0.699732822392533,1.),(1.,0.69855427952325,
1.),(1.,0.697985323371657,1.),(1.,0.696930428409623,1.),(1.,0.69644149384419,
1.),(1.,0.695089684342733,1.),(1.,0.694335092820993,1.),(1.,0.693797102764879,
1.)))
REPRESENTATION_ITEM('')
SURFACE()
);
#2760=(
BOUNDED_SURFACE()
B_SPLINE_SURFACE(3,2,((#176024,#176025,#176026),(#176027,#176028,#176029),
(#176030,#176031,#176032),(#176033,#176034,#176035)),.UNSPECIFIED.,.F.,
 .F.,.F.)
B_SPLINE_SURFACE_WITH_KNOTS((4,4),(3,3),(0.0156098999423859,0.0162171358932854),
(0.,0.915625791428726),.UNSPECIFIED.)
GEOMETRIC_REPRESENTATION_ITEM()
RATIONAL_B_SPLINE_SURFACE(((1.,0.809621640719886,0.967873953213285),(1.,
0.812433937177746,0.968348523789085),(1.,0.815135819310926,0.968804462122364),
(1.,0.817729693080373,0.969242174215226)))
REPRESENTATION_ITEM('')
SURFACE()
);
#2761=(
BOUNDED_SURFACE()
B_SPLINE_SURFACE(3,2,((#176070,#176071,#176072),(#176073,#176074,#176075),
(#176076,#176077,#176078),(#176079,#176080,#176081),(#176082,#176083,#176084),
(#176085,#176086,#176087),(#176088,#176089,#176090),(#176091,#176092,#176093),
(#176094,#176095,#176096),(#176097,#176098,#176099),(#176100,#176101,#176102),
(#176103,#176104,#176105),(#176106,#176107,#176108),(#176109,#176110,#176111)),
 .UNSPECIFIED.,.F.,.F.,.F.)
B_SPLINE_SURFACE_WITH_KNOTS((4,2,2,2,2,2,4),(3,3),(0.00807902625150492,
0.00883280378349999,0.00920969254949752,0.00958658131549505,0.00996347008149258,
0.0103403588474901,0.0110941363794852),(0.,1.),.UNSPECIFIED.)
GEOMETRIC_REPRESENTATION_ITEM()
RATIONAL_B_SPLINE_SURFACE(((1.,0.707106781186548,1.),(1.,0.708503208405905,
1.),(1.,0.709864127404626,1.),(1.,0.711851747119499,1.),(1.,0.712500882329163,
1.),(1.,0.713738228851022,1.),(1.,0.714331705876986,1.),(1.,0.715467776552351,
1.),(1.,0.716012641761659,1.),(1.,0.71701515809269,1.),(1.,0.717477434704573,
1.),(1.,0.718748007011303,1.),(1.,0.719442582755427,1.),(1.,0.719919801430648,
1.)))
REPRESENTATION_ITEM('')
SURFACE()
);
#2762=(
BOUNDED_SURFACE()
B_SPLINE_SURFACE(3,2,((#176211,#176212,#176213),(#176214,#176215,#176216),
(#176217,#176218,#176219),(#176220,#176221,#176222)),.UNSPECIFIED.,.F.,
 .F.,.F.)
B_SPLINE_SURFACE_WITH_KNOTS((4,4),(3,3),(0.,0.000650589467290063),(0.,1.),
 .UNSPECIFIED.)
GEOMETRIC_REPRESENTATION_ITEM()
RATIONAL_B_SPLINE_SURFACE(((1.,0.761354724782838,1.),(1.,0.761348936155314,
1.),(1.,0.759749503531854,1.),(1.,0.756551244268667,1.)))
REPRESENTATION_ITEM('')
SURFACE()
);
#2763=(
BOUNDED_SURFACE()
B_SPLINE_SURFACE(3,2,((#176230,#176231,#176232),(#176233,#176234,#176235),
(#176236,#176237,#176238),(#176239,#176240,#176241)),.UNSPECIFIED.,.F.,
 .F.,.F.)
B_SPLINE_SURFACE_WITH_KNOTS((4,4),(3,3),(-6.51412822692206E-5,0.000716554104961429),
(-0.000128171463349183,1.),.UNSPECIFIED.)
GEOMETRIC_REPRESENTATION_ITEM()
RATIONAL_B_SPLINE_SURFACE(((1.00009698047895,0.621676789764313,1.),(1.00009906013662,
0.613563994562098,1.),(1.00010008654859,0.609559936451183,1.),(1.00009988696594,
0.610338513229391,1.)))
REPRESENTATION_ITEM('')
SURFACE()
);
#2764=(
BOUNDED_SURFACE()
B_SPLINE_SURFACE(3,2,((#176291,#176292,#176293),(#176294,#176295,#176296),
(#176297,#176298,#176299),(#176300,#176301,#176302)),.UNSPECIFIED.,.F.,
 .F.,.F.)
B_SPLINE_SURFACE_WITH_KNOTS((4,4),(3,3),(-6.51893458122614E-5,0.000717082803934875),
(-0.000140476308568739,1.),.UNSPECIFIED.)
GEOMETRIC_REPRESENTATION_ITEM()
RATIONAL_B_SPLINE_SURFACE(((1.00005469398346,0.805326663217762,1.),(1.00005450492213,
0.805999592802024,1.),(1.00005546526461,0.802581427505982,1.),(1.00005755719884,
0.795135566176566,1.)))
REPRESENTATION_ITEM('')
SURFACE()
);
#2765=(
BOUNDED_SURFACE()
B_SPLINE_SURFACE(3,2,((#176310,#176311,#176312),(#176313,#176314,#176315),
(#176316,#176317,#176318),(#176319,#176320,#176321)),.UNSPECIFIED.,.F.,
 .F.,.F.)
B_SPLINE_SURFACE_WITH_KNOTS((4,4),(3,3),(-3.51851606592903E-5,0.00068875516054279),
(-3.51851606592598E-5,1.),.UNSPECIFIED.)
GEOMETRIC_REPRESENTATION_ITEM()
RATIONAL_B_SPLINE_SURFACE(((1.00003035731885,0.568606220890069,1.),(1.00003120327315,
0.556584756681408,1.),(1.00003165553005,0.550157943671109,1.),(1.00003160738783,
0.550842070368458,1.)))
REPRESENTATION_ITEM('')
SURFACE()
);
#2766=(
BOUNDED_SURFACE()
B_SPLINE_SURFACE(3,2,((#176408,#176409,#176410),(#176411,#176412,#176413),
(#176414,#176415,#176416),(#176417,#176418,#176419),(#176420,#176421,#176422),
(#176423,#176424,#176425),(#176426,#176427,#176428),(#176429,#176430,#176431),
(#176432,#176433,#176434),(#176435,#176436,#176437)),.UNSPECIFIED.,.F.,
 .F.,.F.)
B_SPLINE_SURFACE_WITH_KNOTS((4,2,2,2,4),(3,3),(0.00131180726843869,0.00173116479138241,
0.00215052231432612,0.00256987983726984,0.00298923736021356),(0.,1.00000719536613),
 .UNSPECIFIED.)
GEOMETRIC_REPRESENTATION_ITEM()
RATIONAL_B_SPLINE_SURFACE(((1.,0.707104673712603,1.00000421497822),(1.,
0.735459277067931,1.00000380693471),(1.,0.757076784024019,1.00000349584296),
(1.,0.786069896430007,1.00000307861084),(1.,0.793429076618431,1.00000297270685),
(1.,0.793448571747574,1.0000029724263),(1.,0.78610382913614,1.00000307812252),
(1.,0.757124528684552,1.00000349515588),(1.,0.735523766261738,1.00000380600667),
(1.,0.707104673712603,1.00000421497822)))
REPRESENTATION_ITEM('')
SURFACE()
);
#2767=(
BOUNDED_SURFACE()
B_SPLINE_SURFACE(3,2,((#176476,#176477,#176478),(#176479,#176480,#176481),
(#176482,#176483,#176484),(#176485,#176486,#176487),(#176488,#176489,#176490),
(#176491,#176492,#176493),(#176494,#176495,#176496),(#176497,#176498,#176499),
(#176500,#176501,#176502),(#176503,#176504,#176505)),.UNSPECIFIED.,.F.,
 .F.,.F.)
B_SPLINE_SURFACE_WITH_KNOTS((4,2,2,2,4),(3,3),(0.00108313181642967,0.00175636478508591,
0.00242959775374216,0.0031028307223984,0.00377606369105465),(0.,1.00020946001139),
 .UNSPECIFIED.)
GEOMETRIC_REPRESENTATION_ITEM()
RATIONAL_B_SPLINE_SURFACE(((1.,0.707045431769604,1.00012272453439),(1.,
0.774791710231264,1.00009434426188),(1.,0.828921293970805,1.00007166829543),
(1.,0.903779687679842,1.00004030861543),(1.,0.92410102032017,1.0000317956023),
(1.,0.924695389732779,1.00003154660905),(1.,0.904861584947158,1.000039855387),
(1.,0.830176121522683,1.00007114262304),(1.,0.775998513536546,1.00009383870781),
(1.,0.707045431769604,1.00012272453439)))
REPRESENTATION_ITEM('')
SURFACE()
);
#2768=(
BOUNDED_SURFACE()
B_SPLINE_SURFACE(3,2,((#176567,#176568,#176569),(#176570,#176571,#176572),
(#176573,#176574,#176575),(#176576,#176577,#176578),(#176579,#176580,#176581),
(#176582,#176583,#176584),(#176585,#176586,#176587),(#176588,#176589,#176590),
(#176591,#176592,#176593),(#176594,#176595,#176596)),.UNSPECIFIED.,.F.,
 .F.,.F.)
B_SPLINE_SURFACE_WITH_KNOTS((4,2,2,2,4),(3,3),(0.00116892975483565,0.00173273620432837,
0.00229654265382108,0.0028603491033138,0.00342415555280651),(0.,1.00008736726516),
 .UNSPECIFIED.)
GEOMETRIC_REPRESENTATION_ITEM()
RATIONAL_B_SPLINE_SURFACE(((1.,0.707081191907032,1.00005118303035),(1.,
0.756727911750276,1.00004250803408),(1.,0.79532361474289,1.00003576403205),
(1.,0.847730260009984,1.0000266067815),(1.,0.861376184832611,1.00002422236723),
(1.,0.861443104052992,1.00002421067414),(1.,0.847851660205351,1.00002658556869),
(1.,0.795420207077594,1.00003574715403),(1.,0.756766547571532,1.00004250128307),
(1.,0.707081191907032,1.00005118303035)))
REPRESENTATION_ITEM('')
SURFACE()
);
#2769=(
BOUNDED_SURFACE()
B_SPLINE_SURFACE(3,2,((#176718,#176719,#176720),(#176721,#176722,#176723),
(#176724,#176725,#176726),(#176727,#176728,#176729),(#176730,#176731,#176732),
(#176733,#176734,#176735),(#176736,#176737,#176738),(#176739,#176740,#176741),
(#176742,#176743,#176744),(#176745,#176746,#176747)),.UNSPECIFIED.,.F.,
 .F.,.F.)
B_SPLINE_SURFACE_WITH_KNOTS((4,2,2,2,4),(3,3),(8.78519494496445E-16,0.392699081698725,
0.785398163397449,1.17809724509617,1.5707963267949),(0.,1.),
 .UNSPECIFIED.)
GEOMETRIC_REPRESENTATION_ITEM()
RATIONAL_B_SPLINE_SURFACE(((1.,0.754709580222768,1.),(1.,0.754714219644573,
1.),(1.,0.753512297211018,1.),(1.,0.748871927581762,1.),(1.,0.745429367161016,
1.),(1.,0.736738129073881,1.),(1.,0.73149075671205,1.),(1.,0.719894264547496,
1.),(1.,0.713550262087909,1.),(1.,0.707106781186548,1.)))
REPRESENTATION_ITEM('')
SURFACE()
);
#2770=(
BOUNDED_SURFACE()
B_SPLINE_SURFACE(3,2,((#176850,#176851,#176852),(#176853,#176854,#176855),
(#176856,#176857,#176858),(#176859,#176860,#176861),(#176862,#176863,#176864),
(#176865,#176866,#176867),(#176868,#176869,#176870),(#176871,#176872,#176873),
(#176874,#176875,#176876),(#176877,#176878,#176879)),.UNSPECIFIED.,.F.,
 .F.,.F.)
B_SPLINE_SURFACE_WITH_KNOTS((4,2,2,2,4),(3,3),(4.71238898038469,5.10508806208341,
5.49778714378214,5.89048622548086,6.28318530717959),(0.,1.),
 .UNSPECIFIED.)
GEOMETRIC_REPRESENTATION_ITEM()
RATIONAL_B_SPLINE_SURFACE(((1.,0.707106781186548,1.),(1.,0.71355026185156,
1.),(1.,0.719894264862189,1.),(1.,0.73149075639733,1.),(1.,0.73673812929671,
1.),(1.,0.745429366938189,1.),(1.,0.748871927696634,1.),(1.,0.753512297096161,
1.),(1.,0.754714219730837,1.),(1.,0.754709580222772,1.)))
REPRESENTATION_ITEM('')
SURFACE()
);
#2771=(
BOUNDED_SURFACE()
B_SPLINE_SURFACE(3,2,((#176896,#176897,#176898),(#176899,#176900,#176901),
(#176902,#176903,#176904),(#176905,#176906,#176907),(#176908,#176909,#176910),
(#176911,#176912,#176913),(#176914,#176915,#176916),(#176917,#176918,#176919),
(#176920,#176921,#176922),(#176923,#176924,#176925)),.UNSPECIFIED.,.F.,
 .F.,.F.)
B_SPLINE_SURFACE_WITH_KNOTS((4,2,2,2,4),(3,3),(0.00116892975483561,0.00173273620432837,
0.00229654265382113,0.00286034910331391,0.00342415555280667),(0.,1.00008736726517),
 .UNSPECIFIED.)
GEOMETRIC_REPRESENTATION_ITEM()
RATIONAL_B_SPLINE_SURFACE(((1.,0.707081191907034,1.00005118303036),(1.,
0.75672791175003,1.00004250803408),(1.,0.795323614743255,1.00003576403205),
(1.,0.847730260009664,1.0000266067815),(1.,0.861376184834009,1.00002422236724),
(1.,0.861443104051655,1.00002421067414),(1.,0.847851660205381,1.0000265855687),
(1.,0.795420207077597,1.00003574715403),(1.,0.756766547571556,1.00004250128307),
(1.,0.707081191907034,1.00005118303036)))
REPRESENTATION_ITEM('')
SURFACE()
);
#2772=(
BOUNDED_SURFACE()
B_SPLINE_SURFACE(2,2,((#176985,#176986,#176987),(#176988,#176989,#176990),
(#176991,#176992,#176993)),.UNSPECIFIED.,.F.,.F.,.F.)
B_SPLINE_SURFACE_WITH_KNOTS((3,3),(3,3),(-3.74064361396611E-16,1.57079632679492),
(-1.5707963267949,0.),.UNSPECIFIED.)
GEOMETRIC_REPRESENTATION_ITEM()
RATIONAL_B_SPLINE_SURFACE(((1.,0.707106781186548,1.),(0.707106781186552,
0.500000000000003,0.707106781186552),(1.,0.707106781186548,1.)))
REPRESENTATION_ITEM('')
SURFACE()
);
#2773=(
BOUNDED_SURFACE()
B_SPLINE_SURFACE(2,2,((#177001,#177002,#177003),(#177004,#177005,#177006),
(#177007,#177008,#177009)),.UNSPECIFIED.,.F.,.F.,.F.)
B_SPLINE_SURFACE_WITH_KNOTS((3,3),(3,3),(0.,1.57079632679492),(-3.14159265358979,
-1.5707963267949),.UNSPECIFIED.)
GEOMETRIC_REPRESENTATION_ITEM()
RATIONAL_B_SPLINE_SURFACE(((1.,0.707106781186548,1.),(0.707106781186552,
0.500000000000003,0.707106781186552),(1.,0.707106781186548,1.)))
REPRESENTATION_ITEM('')
SURFACE()
);
#2774=(
BOUNDED_SURFACE()
B_SPLINE_SURFACE(2,2,((#177029,#177030,#177031),(#177032,#177033,#177034),
(#177035,#177036,#177037)),.UNSPECIFIED.,.F.,.F.,.F.)
B_SPLINE_SURFACE_WITH_KNOTS((3,3),(3,3),(-3.74064361396611E-16,1.57079632679492),
(-1.5707963267949,0.),.UNSPECIFIED.)
GEOMETRIC_REPRESENTATION_ITEM()
RATIONAL_B_SPLINE_SURFACE(((1.,0.707106781186548,1.),(0.707106781186552,
0.500000000000003,0.707106781186552),(1.,0.707106781186548,1.)))
REPRESENTATION_ITEM('')
SURFACE()
);
#2775=(
BOUNDED_SURFACE()
B_SPLINE_SURFACE(2,2,((#177045,#177046,#177047),(#177048,#177049,#177050),
(#177051,#177052,#177053)),.UNSPECIFIED.,.F.,.F.,.F.)
B_SPLINE_SURFACE_WITH_KNOTS((3,3),(3,3),(0.,1.57079632679501),(-3.14159265358979,
-1.5707963267949),.UNSPECIFIED.)
GEOMETRIC_REPRESENTATION_ITEM()
RATIONAL_B_SPLINE_SURFACE(((1.,0.707106781186548,1.),(0.707106781186506,
0.49999999999997,0.707106781186506),(1.,0.707106781186548,1.)))
REPRESENTATION_ITEM('')
SURFACE()
);
#2776=(
BOUNDED_SURFACE()
B_SPLINE_SURFACE(2,2,((#177073,#177074,#177075),(#177076,#177077,#177078),
(#177079,#177080,#177081)),.UNSPECIFIED.,.F.,.F.,.F.)
B_SPLINE_SURFACE_WITH_KNOTS((3,3),(3,3),(-3.74064361396611E-16,1.57079632679501),
(-1.5707963267949,0.),.UNSPECIFIED.)
GEOMETRIC_REPRESENTATION_ITEM()
RATIONAL_B_SPLINE_SURFACE(((1.,0.707106781186548,1.),(0.707106781186506,
0.49999999999997,0.707106781186506),(1.,0.707106781186548,1.)))
REPRESENTATION_ITEM('')
SURFACE()
);
#2777=(
BOUNDED_SURFACE()
B_SPLINE_SURFACE(3,2,((#177091,#177092,#177093),(#177094,#177095,#177096),
(#177097,#177098,#177099),(#177100,#177101,#177102),(#177103,#177104,#177105),
(#177106,#177107,#177108)),.UNSPECIFIED.,.F.,.F.,.F.)
B_SPLINE_SURFACE_WITH_KNOTS((4,2,4),(3,3),(0.19058679356565,0.194723599184011,
0.198860404802373),(0.,1.),.UNSPECIFIED.)
GEOMETRIC_REPRESENTATION_ITEM()
RATIONAL_B_SPLINE_SURFACE(((1.,0.954062806827576,1.),(1.,0.95589180838713,
1.),(1.,0.957713181483215,1.),(1.,0.961295526062221,1.),(1.,0.963047831711069,
1.),(1.,0.964700553047209,1.)))
REPRESENTATION_ITEM('')
SURFACE()
);
#2778=(
BOUNDED_SURFACE()
B_SPLINE_SURFACE(3,2,((#177180,#177181,#177182),(#177183,#177184,#177185),
(#177186,#177187,#177188),(#177189,#177190,#177191),(#177192,#177193,#177194),
(#177195,#177196,#177197),(#177198,#177199,#177200),(#177201,#177202,#177203),
(#177204,#177205,#177206),(#177207,#177208,#177209)),.UNSPECIFIED.,.F.,
 .F.,.F.)
B_SPLINE_SURFACE_WITH_KNOTS((4,2,2,2,4),(3,3),(0.00166905748884283,0.00189688228523533,
0.00212470708162783,0.00235253187802032,0.00258035667441282),(0.,1.),
 .UNSPECIFIED.)
GEOMETRIC_REPRESENTATION_ITEM()
RATIONAL_B_SPLINE_SURFACE(((1.,0.727682857482998,1.),(1.,0.742747587336582,
1.),(1.,0.756565090576503,1.),(1.,0.779563382898484,1.),(1.,0.788904601358709,
1.),(1.,0.801793098601248,1.),(1.,0.805447378128131,1.),(1.,0.806422615061365,
1.),(1.,0.803776299349016,1.),(1.,0.798143461625347,1.)))
REPRESENTATION_ITEM('')
SURFACE()
);
#2779=(
BOUNDED_SURFACE()
B_SPLINE_SURFACE(3,2,((#177347,#177348,#177349),(#177350,#177351,#177352),
(#177353,#177354,#177355),(#177356,#177357,#177358)),.UNSPECIFIED.,.F.,
 .F.,.F.)
B_SPLINE_SURFACE_WITH_KNOTS((4,4),(3,3),(0.00165976994196512,0.00175987143987977),
(0.,1.),.UNSPECIFIED.)
GEOMETRIC_REPRESENTATION_ITEM()
RATIONAL_B_SPLINE_SURFACE(((1.,0.707106781186549,1.),(1.,0.714158119082749,
1.),(1.,0.721010468727715,1.),(1.,0.727682857483054,1.)))
REPRESENTATION_ITEM('')
SURFACE()
);
#2780=(
BOUNDED_SURFACE()
B_SPLINE_SURFACE(3,2,((#177385,#177386,#177387),(#177388,#177389,#177390),
(#177391,#177392,#177393),(#177394,#177395,#177396),(#177397,#177398,#177399),
(#177400,#177401,#177402),(#177403,#177404,#177405),(#177406,#177407,#177408),
(#177409,#177410,#177411),(#177412,#177413,#177414),(#177415,#177416,#177417),
(#177418,#177419,#177420)),.UNSPECIFIED.,.F.,.F.,.F.)
B_SPLINE_SURFACE_WITH_KNOTS((4,2,2,2,2,4),(3,3),(-2.00577401909819E-18,
0.000253295312002929,0.000379942968004394,0.00050659062400586,0.000759885936008791,
0.00107305843962858),(-0.000819314453937797,1.),.UNSPECIFIED.)
GEOMETRIC_REPRESENTATION_ITEM()
RATIONAL_B_SPLINE_SURFACE(((1.00062441413186,0.618941098343779,1.),(1.000636782846,
0.611392888935679,1.),(1.00064233967356,0.608001744342297,1.),(1.00063916769033,
0.609937498807523,1.),(1.00063617465599,0.611764046800477,1.),(1.0006268165417,
0.617474988578315,1.),(1.00062041650623,0.621380714544669,1.),(1.00059694010773,
0.635707569383962,1.),(1.00057586843891,0.64856689873871,1.),(1.00052425844524,
0.680062738598407,1.),(1.00049229616275,0.699568242459855,1.),(1.00046353459627,
0.717120457208093,1.)))
REPRESENTATION_ITEM('')
SURFACE()
);
#2781=(
BOUNDED_SURFACE()
B_SPLINE_SURFACE(3,2,((#177478,#177479,#177480),(#177481,#177482,#177483),
(#177484,#177485,#177486),(#177487,#177488,#177489),(#177490,#177491,#177492),
(#177493,#177494,#177495),(#177496,#177497,#177498),(#177499,#177500,#177501),
(#177502,#177503,#177504),(#177505,#177506,#177507),(#177508,#177509,#177510),
(#177511,#177512,#177513)),.UNSPECIFIED.,.F.,.F.,.F.)
B_SPLINE_SURFACE_WITH_KNOTS((4,2,2,2,2,4),(3,3),(0.,0.000250417359226946,
0.000375626038840418,0.000500834718453891,0.000751252077680836,0.00100166943690778),
(0.,1.00140468204324),.UNSPECIFIED.)
GEOMETRIC_REPRESENTATION_ITEM()
RATIONAL_B_SPLINE_SURFACE(((1.,0.706695359341495,1.00082399952386),(1.,
0.713853670046366,1.00080388922285),(1.,0.720999103056668,1.00078381509997),
(1.,0.73025084315396,1.0007578235936),(1.,0.733150182806824,1.00074967829291),
(1.,0.738287011792474,1.00073524707003),(1.,0.740523082653704,1.00072896513286),
(1.,0.746225847024098,1.00071294399145),(1.,0.748459431198593,1.00070666904028),
(1.,0.749389678141756,1.00070405563793),(1.,0.748089205673001,1.00070770913858),
(1.,0.745115248769628,1.0007160640663)))
REPRESENTATION_ITEM('')
SURFACE()
);
#2782=(
BOUNDED_SURFACE()
B_SPLINE_SURFACE(3,2,((#177610,#177611,#177612),(#177613,#177614,#177615),
(#177616,#177617,#177618),(#177619,#177620,#177621),(#177622,#177623,#177624),
(#177625,#177626,#177627)),.UNSPECIFIED.,.F.,.F.,.F.)
B_SPLINE_SURFACE_WITH_KNOTS((4,2,4),(3,3),(0.,0.00138008432392828,0.00276016864785656),
(0.,1.),.UNSPECIFIED.)
GEOMETRIC_REPRESENTATION_ITEM()
RATIONAL_B_SPLINE_SURFACE(((1.,0.889512696472458,1.),(1.,0.875621469665309,
1.),(1.,0.859481975708513,1.),(1.,0.823331923932046,1.),(1.,0.803217377248123,
1.),(1.,0.782160982635976,1.)))
REPRESENTATION_ITEM('')
SURFACE()
);
#2783=(
BOUNDED_SURFACE()
B_SPLINE_SURFACE(3,2,((#177678,#177679,#177680),(#177681,#177682,#177683),
(#177684,#177685,#177686),(#177687,#177688,#177689)),.UNSPECIFIED.,.F.,
 .F.,.F.)
B_SPLINE_SURFACE_WITH_KNOTS((4,4),(3,3),(-3.41523684332934E-18,0.000418670815451504),
(0.,1.),.UNSPECIFIED.)
GEOMETRIC_REPRESENTATION_ITEM()
RATIONAL_B_SPLINE_SURFACE(((1.,0.80178372573727,1.),(1.,0.801581038760284,
1.),(1.,0.797360979426379,1.),(1.,0.782160982635977,1.)))
REPRESENTATION_ITEM('')
SURFACE()
);
#2784=(
BOUNDED_SURFACE()
B_SPLINE_SURFACE(3,2,((#177736,#177737,#177738),(#177739,#177740,#177741),
(#177742,#177743,#177744),(#177745,#177746,#177747),(#177748,#177749,#177750),
(#177751,#177752,#177753)),.UNSPECIFIED.,.F.,.F.,.F.)
B_SPLINE_SURFACE_WITH_KNOTS((4,2,4),(3,3),(-1.97866896478604E-18,0.00038804539867497,
0.000776090797349943),(0.,1.),.UNSPECIFIED.)
GEOMETRIC_REPRESENTATION_ITEM()
RATIONAL_B_SPLINE_SURFACE(((1.,0.889512696472455,1.),(1.,0.863343118435834,
1.),(1.,0.832896241151233,1.),(1.,0.770252595987774,1.),(1.,0.738321744191135,
1.),(1.,0.707106781186616,1.)))
REPRESENTATION_ITEM('')
SURFACE()
);
#2785=(
BOUNDED_SURFACE()
B_SPLINE_SURFACE(3,2,((#177788,#177789,#177790),(#177791,#177792,#177793),
(#177794,#177795,#177796),(#177797,#177798,#177799),(#177800,#177801,#177802),
(#177803,#177804,#177805),(#177806,#177807,#177808),(#177809,#177810,#177811),
(#177812,#177813,#177814),(#177815,#177816,#177817)),.UNSPECIFIED.,.F.,
 .F.,.F.)
B_SPLINE_SURFACE_WITH_KNOTS((4,2,2,2,4),(3,3),(0.00312784824903477,0.00367780251889487,
0.00407062699736637,0.00446345147583787,0.00501340574569797),(0.,1.00073967576989),
 .UNSPECIFIED.)
GEOMETRIC_REPRESENTATION_ITEM()
RATIONAL_B_SPLINE_SURFACE(((1.,0.799013820880279,1.00029732921356),(1.,
0.805121639253135,1.00028829360304),(1.,0.800160744451582,1.00029563251041),
(1.,0.77993744364898,1.00032554988159),(1.,0.767978651035377,1.00034324113985),
(1.,0.743437812578867,1.00037954566701),(1.,0.730757029672295,1.00039830500273),
(1.,0.708822787991186,1.00043075345694),(1.,0.70267339919749,1.00043985056472),
(1.,0.710079976844615,1.00042889363267)))
REPRESENTATION_ITEM('')
SURFACE()
);
#2786=(
BOUNDED_SURFACE()
B_SPLINE_SURFACE(2,2,((#177886,#177887,#177888),(#177889,#177890,#177891),
(#177892,#177893,#177894)),.UNSPECIFIED.,.F.,.F.,.F.)
B_SPLINE_SURFACE_WITH_KNOTS((3,3),(3,3),(-1.5707963267949,0.),(-2.40432329481773,
-1.5707963267949),.UNSPECIFIED.)
GEOMETRIC_REPRESENTATION_ITEM()
RATIONAL_B_SPLINE_SURFACE(((1.,0.914403878918655,1.),(0.707106781186554,
0.64658118352667,0.707106781186554),(1.,0.914403878918655,1.)))
REPRESENTATION_ITEM('')
SURFACE()
);
#2787=(
BOUNDED_SURFACE()
B_SPLINE_SURFACE(2,2,((#177902,#177903,#177904),(#177905,#177906,#177907),
(#177908,#177909,#177910)),.UNSPECIFIED.,.F.,.F.,.F.)
B_SPLINE_SURFACE_WITH_KNOTS((3,3),(3,3),(-1.5707963267949,-1.75915766232281E-16),
(-3.14159265358979,-2.36370134837197),.UNSPECIFIED.)
GEOMETRIC_REPRESENTATION_ITEM()
RATIONAL_B_SPLINE_SURFACE(((1.,0.925309396359852,1.),(0.707106781186554,
0.654292548861688,0.707106781186554),(1.,0.925309396359852,1.)))
REPRESENTATION_ITEM('')
SURFACE()
);
#2788=(
BOUNDED_SURFACE()
B_SPLINE_SURFACE(3,2,((#177954,#177955,#177956),(#177957,#177958,#177959),
(#177960,#177961,#177962),(#177963,#177964,#177965),(#177966,#177967,#177968),
(#177969,#177970,#177971),(#177972,#177973,#177974),(#177975,#177976,#177977),
(#177978,#177979,#177980),(#177981,#177982,#177983)),.UNSPECIFIED.,.F.,
 .F.,.F.)
B_SPLINE_SURFACE_WITH_KNOTS((4,2,2,2,4),(3,3),(1.57071221042854,1.96349540849362,
2.35619449019234,2.74889357189107,3.14167676995614),(0.,1.00008411636635),
 .UNSPECIFIED.)
GEOMETRIC_REPRESENTATION_ITEM()
RATIONAL_B_SPLINE_SURFACE(((1.,0.707084736317511,1.00004927793526),(1.,
0.703049896773505,1.00004995672734),(1.,0.698980464825185,1.000050641339),
(1.,0.691398460047746,1.00005191688038),(1.,0.68788946354642,1.00005250720845),
(1.,0.682000298653236,1.00005349795876),(1.,0.679623581412379,1.00005389780039),
(1.,0.676403465575794,1.00005443952928),(1.,0.675558134885499,1.00005458174157),
(1.,0.675562922401557,1.00005458093616)))
REPRESENTATION_ITEM('')
SURFACE()
);
#2789=(
BOUNDED_SURFACE()
B_SPLINE_SURFACE(3,2,((#178188,#178189,#178190),(#178191,#178192,#178193),
(#178194,#178195,#178196),(#178197,#178198,#178199),(#178200,#178201,#178202),
(#178203,#178204,#178205),(#178206,#178207,#178208),(#178209,#178210,#178211),
(#178212,#178213,#178214),(#178215,#178216,#178217)),.UNSPECIFIED.,.F.,
 .F.,.F.)
B_SPLINE_SURFACE_WITH_KNOTS((4,2,2,2,4),(3,3),(3.1415926535898,3.53429173528852,
3.92699081698724,4.31968989868597,4.71238898038469),(0.,1.),
 .UNSPECIFIED.)
GEOMETRIC_REPRESENTATION_ITEM()
RATIONAL_B_SPLINE_SURFACE(((1.,0.73727733681012,1.),(1.,0.737280525007918,
1.),(1.,0.736509240245186,1.),(1.,0.733539335051142,1.),(1.,0.731338116837293,
1.),(1.,0.725801833007076,1.),(1.,0.722468048845319,1.),(1.,0.715136249134486,
1.),(1.,0.711141648505406,1.),(1.,0.707106781186552,1.)))
REPRESENTATION_ITEM('')
SURFACE()
);
#2790=(
BOUNDED_SURFACE()
B_SPLINE_SURFACE(3,2,((#178292,#178293,#178294),(#178295,#178296,#178297),
(#178298,#178299,#178300),(#178301,#178302,#178303),(#178304,#178305,#178306),
(#178307,#178308,#178309),(#178310,#178311,#178312),(#178313,#178314,#178315),
(#178316,#178317,#178318),(#178319,#178320,#178321)),.UNSPECIFIED.,.F.,
 .F.,.F.)
B_SPLINE_SURFACE_WITH_KNOTS((4,2,2,2,4),(3,3),(1.57071221043463,1.96349540849362,
2.35619449019234,2.74889357189107,3.14167676995005),(0.,1.00008411636026),
 .UNSPECIFIED.)
GEOMETRIC_REPRESENTATION_ITEM()
RATIONAL_B_SPLINE_SURFACE(((0.999999999999999,0.707084736319112,1.00004927793169),
(1.,0.70304989677498,1.00004995672372),(1.,0.698980464827243,1.00005064133533),
(1.,0.691398460049362,1.00005191687662),(1.,0.687889463547922,1.00005250720465),
(1.,0.682000298655582,1.00005349795488),(1.,0.679623581414333,1.00005389779649),
(1.,0.676403465577792,1.00005443952534),(1.,0.675558134887503,1.00005458173762),
(1.,0.675562922403545,1.0000545809322)))
REPRESENTATION_ITEM('')
SURFACE()
);
#2791=(
BOUNDED_SURFACE()
B_SPLINE_SURFACE(3,2,((#178536,#178537,#178538),(#178539,#178540,#178541),
(#178542,#178543,#178544),(#178545,#178546,#178547),(#178548,#178549,#178550),
(#178551,#178552,#178553),(#178554,#178555,#178556),(#178557,#178558,#178559),
(#178560,#178561,#178562),(#178563,#178564,#178565)),.UNSPECIFIED.,.F.,
 .F.,.F.)
B_SPLINE_SURFACE_WITH_KNOTS((4,2,2,2,4),(3,3),(3.1415926535898,3.53429173528852,
3.92699081698724,4.31968989868597,4.71238898038469),(0.,1.),
 .UNSPECIFIED.)
GEOMETRIC_REPRESENTATION_ITEM()
RATIONAL_B_SPLINE_SURFACE(((1.,0.73727733681012,1.),(1.,0.737280525007918,
1.),(1.,0.736509240245177,1.),(1.,0.733539335051133,1.),(1.,0.731338116836513,
1.),(1.,0.725801833007847,1.),(1.,0.722468048844965,1.),(1.,0.715136249134831,
1.),(1.,0.711141648505139,1.),(1.,0.707106781186548,1.)))
REPRESENTATION_ITEM('')
SURFACE()
);
#2792=(
BOUNDED_SURFACE()
B_SPLINE_SURFACE(3,2,((#178674,#178675,#178676),(#178677,#178678,#178679),
(#178680,#178681,#178682),(#178683,#178684,#178685),(#178686,#178687,#178688),
(#178689,#178690,#178691)),.UNSPECIFIED.,.F.,.F.,.F.)
B_SPLINE_SURFACE_WITH_KNOTS((4,2,4),(3,3),(0.00432986646256736,0.00505584518302534,
0.00578182390348332),(0.,1.),.UNSPECIFIED.)
GEOMETRIC_REPRESENTATION_ITEM()
RATIONAL_B_SPLINE_SURFACE(((1.,0.737277336810087,1.),(1.,0.750110373322841,
1.),(1.,0.762782449795825,1.),(1.,0.783852338027907,1.),(1.,0.792419881107176,
1.),(1.,0.79736306112227,1.)))
REPRESENTATION_ITEM('')
SURFACE()
);
#2793=(
BOUNDED_SURFACE()
B_SPLINE_SURFACE(3,2,((#178959,#178960,#178961),(#178962,#178963,#178964),
(#178965,#178966,#178967),(#178968,#178969,#178970),(#178971,#178972,#178973),
(#178974,#178975,#178976),(#178977,#178978,#178979),(#178980,#178981,#178982),
(#178983,#178984,#178985),(#178986,#178987,#178988)),.UNSPECIFIED.,.F.,
 .F.,.F.)
B_SPLINE_SURFACE_WITH_KNOTS((4,2,2,2,4),(3,3),(-1.77635683940025E-15,0.392699081698723,
0.785398163397447,1.17809724509617,1.5707963267949),(0.,1.),
 .UNSPECIFIED.)
GEOMETRIC_REPRESENTATION_ITEM()
RATIONAL_B_SPLINE_SURFACE(((1.,0.675590207615662,1.),(1.,0.675585785528387,
1.),(1.,0.676431027860615,1.),(1.,0.679650528045674,1.),(1.,0.682027045382935,
1.),(1.,0.687915714942327,1.),(1.,0.691424416304369,1.),(1.,0.699004971485606,
1.),(1.,0.703073130219524,1.),(1.,0.707106781186548,1.)))
REPRESENTATION_ITEM('')
SURFACE()
);
#2794=(
BOUNDED_SURFACE()
B_SPLINE_SURFACE(3,2,((#179098,#179099,#179100),(#179101,#179102,#179103),
(#179104,#179105,#179106),(#179107,#179108,#179109)),.UNSPECIFIED.,.F.,
 .F.,.F.)
B_SPLINE_SURFACE_WITH_KNOTS((4,4),(3,3),(-8.23993651088983E-18,0.000144871551798125),
(0.453761120778822,1.),.UNSPECIFIED.)
GEOMETRIC_REPRESENTATION_ITEM()
RATIONAL_B_SPLINE_SURFACE(((0.947063795072845,0.941669523342704,1.),(0.948417719357794,
0.943161414365259,1.),(0.949729094777561,0.944606420735039,1.),(0.950997479396062,
0.946004055482066,1.)))
REPRESENTATION_ITEM('')
SURFACE()
);
#2795=(
BOUNDED_SURFACE()
B_SPLINE_SURFACE(3,2,((#179111,#179112,#179113),(#179114,#179115,#179116),
(#179117,#179118,#179119),(#179120,#179121,#179122)),.UNSPECIFIED.,.F.,
 .F.,.F.)
B_SPLINE_SURFACE_WITH_KNOTS((4,4),(3,3),(-5.74627151417317E-18,0.000655078443521525),
(0.,1.),.UNSPECIFIED.)
GEOMETRIC_REPRESENTATION_ITEM()
RATIONAL_B_SPLINE_SURFACE(((1.,0.773398994756356,1.),(1.,0.76231666392952,
1.),(1.,0.750153503473797,1.),(1.,0.737277336810164,1.)))
REPRESENTATION_ITEM('')
SURFACE()
);
#2796=(
BOUNDED_SURFACE()
B_SPLINE_SURFACE(3,2,((#179189,#179190,#179191),(#179192,#179193,#179194),
(#179195,#179196,#179197),(#179198,#179199,#179200),(#179201,#179202,#179203),
(#179204,#179205,#179206),(#179207,#179208,#179209),(#179210,#179211,#179212),
(#179213,#179214,#179215),(#179216,#179217,#179218)),.UNSPECIFIED.,.F.,
 .F.,.F.)
B_SPLINE_SURFACE_WITH_KNOTS((4,2,2,2,4),(3,3),(4.71238898038469,5.10508806208342,
5.49778714378214,5.89048622548086,6.28318530717959),(0.,1.),
 .UNSPECIFIED.)
GEOMETRIC_REPRESENTATION_ITEM()
RATIONAL_B_SPLINE_SURFACE(((1.,0.707106781186545,1.),(1.,0.711141648505767,
1.),(1.,0.715136249133983,1.),(1.,0.722468048845823,1.),(1.,0.725801833007033,
1.),(1.,0.731338116837333,1.),(1.,0.73353933505153,1.),(1.,0.736509240244789,
1.),(1.,0.737280525008216,1.),(1.,0.737277336810123,1.)))
REPRESENTATION_ITEM('')
SURFACE()
);
#2797=(
BOUNDED_SURFACE()
B_SPLINE_SURFACE(3,2,((#179415,#179416,#179417),(#179418,#179419,#179420),
(#179421,#179422,#179423),(#179424,#179425,#179426),(#179427,#179428,#179429),
(#179430,#179431,#179432),(#179433,#179434,#179435),(#179436,#179437,#179438),
(#179439,#179440,#179441),(#179442,#179443,#179444)),.UNSPECIFIED.,.F.,
 .F.,.F.)
B_SPLINE_SURFACE_WITH_KNOTS((4,2,2,2,4),(3,3),(4.71238898038469,5.10508806208342,
5.49778714378214,5.89048622548086,6.28318530717959),(0.,1.),
 .UNSPECIFIED.)
GEOMETRIC_REPRESENTATION_ITEM()
RATIONAL_B_SPLINE_SURFACE(((1.,0.707106781186545,1.),(1.,0.711141648505882,
1.),(1.,0.715136249133832,1.),(1.,0.722468048845978,1.),(1.,0.725801833007229,
1.),(1.,0.731338116837136,1.),(1.,0.733539335051522,1.),(1.,0.736509240244802,
1.),(1.,0.737280525008203,1.),(1.,0.737277336810123,1.)))
REPRESENTATION_ITEM('')
SURFACE()
);
#2798=(
BOUNDED_SURFACE()
B_SPLINE_SURFACE(3,2,((#179517,#179518,#179519),(#179520,#179521,#179522),
(#179523,#179524,#179525),(#179526,#179527,#179528),(#179529,#179530,#179531),
(#179532,#179533,#179534),(#179535,#179536,#179537),(#179538,#179539,#179540),
(#179541,#179542,#179543),(#179544,#179545,#179546)),.UNSPECIFIED.,.F.,
 .F.,.F.)
B_SPLINE_SURFACE_WITH_KNOTS((4,2,2,2,4),(3,3),(-1.77635683940025E-15,0.392699081698723,
0.785398163397447,1.17809724509617,1.5707963267949),(0.,1.),
 .UNSPECIFIED.)
GEOMETRIC_REPRESENTATION_ITEM()
RATIONAL_B_SPLINE_SURFACE(((1.,0.675590207615668,1.),(1.,0.675585785528724,
1.),(1.,0.676431027860173,1.),(1.,0.679650528046127,1.),(1.,0.682027045382925,
1.),(1.,0.687915714942339,1.),(1.,0.69142441630503,1.),(1.,0.699004971484955,
1.),(1.,0.703073130220009,1.),(1.,0.70710678118655,1.)))
REPRESENTATION_ITEM('')
SURFACE()
);
#2799=(
BOUNDED_SURFACE()
B_SPLINE_SURFACE(3,2,((#179770,#179771,#179772),(#179773,#179774,#179775),
(#179776,#179777,#179778),(#179779,#179780,#179781),(#179782,#179783,#179784),
(#179785,#179786,#179787),(#179788,#179789,#179790),(#179791,#179792,#179793),
(#179794,#179795,#179796),(#179797,#179798,#179799)),.UNSPECIFIED.,.F.,
 .F.,.F.)
B_SPLINE_SURFACE_WITH_KNOTS((4,2,2,2,4),(3,3),(1.5707963267949,1.96349540849362,
2.35619449019234,2.74889357189107,3.1415926535898),(0.,1.),
 .UNSPECIFIED.)
GEOMETRIC_REPRESENTATION_ITEM()
RATIONAL_B_SPLINE_SURFACE(((1.,0.707106781186548,1.),(1.,0.711141648505595,
1.),(1.,0.715136249134216,1.),(1.,0.722468048845599,1.),(1.,0.725801833007891,
1.),(1.,0.731338116836469,1.),(1.,0.733539335051304,1.),(1.,0.73650924024502,
1.),(1.,0.737280525008041,1.),(1.,0.737277336810125,1.)))
REPRESENTATION_ITEM('')
SURFACE()
);
#2800=(
BOUNDED_SURFACE()
B_SPLINE_SURFACE(3,2,((#179872,#179873,#179874),(#179875,#179876,#179877),
(#179878,#179879,#179880),(#179881,#179882,#179883),(#179884,#179885,#179886),
(#179887,#179888,#179889),(#179890,#179891,#179892),(#179893,#179894,#179895),
(#179896,#179897,#179898),(#179899,#179900,#179901),(#179902,#179903,#179904),
(#179905,#179906,#179907)),.UNSPECIFIED.,.F.,.F.,.F.)
B_SPLINE_SURFACE_WITH_KNOTS((4,2,2,2,2,4),(3,3),(0.00373720614906648,0.00431441150266452,
0.00489161685626256,0.00518021953306157,0.00546882220986059,0.00604602756345863),
(0.,1.),.UNSPECIFIED.)
GEOMETRIC_REPRESENTATION_ITEM()
RATIONAL_B_SPLINE_SURFACE(((1.,0.702399276808564,1.),(1.,0.697901374758016,
1.),(1.,0.693446103155503,1.),(1.,0.685742881148842,1.),(1.,0.682394877642487,
1.),(1.,0.6786862147386,1.),(1.,0.677675780152448,1.),(1.,0.676083839724519,
1.),(1.,0.675500346164623,1.),(1.,0.674441428307327,1.),(1.,0.674627601820987,
1.),(1.,0.675590207615657,1.)))
REPRESENTATION_ITEM('')
SURFACE()
);
#2801=(
BOUNDED_SURFACE()
B_SPLINE_SURFACE(3,2,((#180151,#180152,#180153),(#180154,#180155,#180156),
(#180157,#180158,#180159),(#180160,#180161,#180162),(#180163,#180164,#180165),
(#180166,#180167,#180168),(#180169,#180170,#180171),(#180172,#180173,#180174),
(#180175,#180176,#180177),(#180178,#180179,#180180)),.UNSPECIFIED.,.F.,
 .F.,.F.)
B_SPLINE_SURFACE_WITH_KNOTS((4,2,2,2,4),(3,3),(1.5707122104307,1.96349540849362,
2.35619449019234,2.74889357189106,3.14167676995398),(0.,1.0000841163642),
 .UNSPECIFIED.)
GEOMETRIC_REPRESENTATION_ITEM()
RATIONAL_B_SPLINE_SURFACE(((1.,0.70708473631808,1.000049277934),(1.,0.703049896774256,
1.00004995672606),(1.,0.698980464825608,1.0000506413377),(1.,0.691398460048643,
1.00005191687905),(1.,0.687889463547443,1.00005250720711),(1.,0.682000298653572,
1.00005349795739),(1.,0.67962358141276,1.00005389779901),(1.,0.676403465576801,
1.00005443952789),(1.,0.675558134885977,1.00005458174018),(1.,0.675562922402261,
1.00005458093476)))
REPRESENTATION_ITEM('')
SURFACE()
);
#2802=(
BOUNDED_SURFACE()
B_SPLINE_SURFACE(3,2,((#180256,#180257,#180258),(#180259,#180260,#180261),
(#180262,#180263,#180264),(#180265,#180266,#180267),(#180268,#180269,#180270),
(#180271,#180272,#180273),(#180274,#180275,#180276),(#180277,#180278,#180279),
(#180280,#180281,#180282),(#180283,#180284,#180285)),.UNSPECIFIED.,.F.,
 .F.,.F.)
B_SPLINE_SURFACE_WITH_KNOTS((4,2,2,2,4),(3,3),(3.1415926535898,3.53429173528852,
3.92699081698724,4.31968989868597,4.71238898038469),(0.,1.),
 .UNSPECIFIED.)
GEOMETRIC_REPRESENTATION_ITEM()
RATIONAL_B_SPLINE_SURFACE(((1.,0.737277336810125,1.),(1.,0.737280525008216,
1.),(1.,0.736509240244793,1.),(1.,0.733539335051535,1.),(1.,0.731338116837053,
1.),(1.,0.725801833007317,1.),(1.,0.722468048845379,1.),(1.,0.715136249134436,
1.),(1.,0.711141648505436,1.),(1.,0.707106781186548,1.)))
REPRESENTATION_ITEM('')
SURFACE()
);
#2803=(
BOUNDED_SURFACE()
B_SPLINE_SURFACE(3,2,((#180499,#180500,#180501),(#180502,#180503,#180504),
(#180505,#180506,#180507),(#180508,#180509,#180510),(#180511,#180512,#180513),
(#180514,#180515,#180516),(#180517,#180518,#180519),(#180520,#180521,#180522),
(#180523,#180524,#180525),(#180526,#180527,#180528)),.UNSPECIFIED.,.F.,
 .F.,.F.)
B_SPLINE_SURFACE_WITH_KNOTS((4,2,2,2,4),(3,3),(0.,0.392699081698724,0.785398163397448,
1.17809724509617,1.5707963267949),(0.,1.),.UNSPECIFIED.)
GEOMETRIC_REPRESENTATION_ITEM()
RATIONAL_B_SPLINE_SURFACE(((1.,0.67559020761567,1.),(1.,0.675585785528568,
1.),(1.,0.676431027860386,1.),(1.,0.679650528045925,1.),(1.,0.682027045382314,
1.),(1.,0.687915714942951,1.),(1.,0.69142441630529,1.),(1.,0.69900497148469,
1.),(1.,0.703073130220208,1.),(1.,0.707106781186548,1.)))
REPRESENTATION_ITEM('')
SURFACE()
);
#2804=(
BOUNDED_SURFACE()
B_SPLINE_SURFACE(3,2,((#180669,#180670,#180671),(#180672,#180673,#180674),
(#180675,#180676,#180677),(#180678,#180679,#180680),(#180681,#180682,#180683),
(#180684,#180685,#180686)),.UNSPECIFIED.,.F.,.F.,.F.)
B_SPLINE_SURFACE_WITH_KNOTS((4,2,4),(3,3),(-0.000141606762778327,0.00070803381389838,
0.00155767439057644),(0.,1.00109719399777),.UNSPECIFIED.)
GEOMETRIC_REPRESENTATION_ITEM()
RATIONAL_B_SPLINE_SURFACE(((1.,0.802844010548984,1.0004326367365),(1.,0.797864106908113,
1.00044356457727),(1.,0.787124435107925,1.00046713158414),(1.,0.7608388846863,
1.00052481228045),(1.,0.744970654526623,1.00055963333422),(1.,0.729042216494434,
1.00059458650742)))
REPRESENTATION_ITEM('')
SURFACE()
);
#2805=(
BOUNDED_SURFACE()
B_SPLINE_SURFACE(3,2,((#180705,#180706,#180707),(#180708,#180709,#180710),
(#180711,#180712,#180713),(#180714,#180715,#180716),(#180717,#180718,#180719),
(#180720,#180721,#180722),(#180723,#180724,#180725),(#180726,#180727,#180728),
(#180729,#180730,#180731),(#180732,#180733,#180734)),.UNSPECIFIED.,.F.,
 .F.,.F.)
B_SPLINE_SURFACE_WITH_KNOTS((4,2,2,2,4),(3,3),(4.71238898038469,5.10508806208342,
5.49778714378214,5.89048622548086,6.28318530717959),(0.,1.),
 .UNSPECIFIED.)
GEOMETRIC_REPRESENTATION_ITEM()
RATIONAL_B_SPLINE_SURFACE(((1.,0.707106781186548,1.),(1.,0.711141648505921,
1.),(1.,0.715136249133786,1.),(1.,0.722468048846019,1.),(1.,0.725801833007554,
1.),(1.,0.731338116836806,1.),(1.,0.733539335051135,1.),(1.,0.736509240245178,
1.),(1.,0.737280525007913,1.),(1.,0.73727733681012,1.)))
REPRESENTATION_ITEM('')
SURFACE()
);
#2806=(
BOUNDED_SURFACE()
B_SPLINE_SURFACE(3,2,((#180946,#180947,#180948),(#180949,#180950,#180951),
(#180952,#180953,#180954),(#180955,#180956,#180957),(#180958,#180959,#180960),
(#180961,#180962,#180963),(#180964,#180965,#180966),(#180967,#180968,#180969),
(#180970,#180971,#180972),(#180973,#180974,#180975)),.UNSPECIFIED.,.F.,
 .F.,.F.)
B_SPLINE_SURFACE_WITH_KNOTS((4,2,2,2,4),(3,3),(4.71238898038469,5.10508806208341,
5.49778714378214,5.89048622548086,6.28318530717959),(0.,1.),
 .UNSPECIFIED.)
GEOMETRIC_REPRESENTATION_ITEM()
RATIONAL_B_SPLINE_SURFACE(((1.,0.707106781186548,1.),(1.,0.71114164850559,
1.),(1.,0.71513624913423,1.),(1.,0.722468048845566,1.),(1.,0.725801833007554,
1.),(1.,0.731338116836806,1.),(1.,0.733539335051299,1.),(1.,0.736509240245015,
1.),(1.,0.737280525008035,1.),(1.,0.73727733681012,1.)))
REPRESENTATION_ITEM('')
SURFACE()
);
#2807=(
BOUNDED_SURFACE()
B_SPLINE_SURFACE(3,2,((#181048,#181049,#181050),(#181051,#181052,#181053),
(#181054,#181055,#181056),(#181057,#181058,#181059),(#181060,#181061,#181062),
(#181063,#181064,#181065),(#181066,#181067,#181068),(#181069,#181070,#181071),
(#181072,#181073,#181074),(#181075,#181076,#181077)),.UNSPECIFIED.,.F.,
 .F.,.F.)
B_SPLINE_SURFACE_WITH_KNOTS((4,2,2,2,4),(3,3),(1.18015353016497E-15,0.392699081698726,
0.785398163397449,1.17809724509617,1.5707963267949),(0.,1.),
 .UNSPECIFIED.)
GEOMETRIC_REPRESENTATION_ITEM()
RATIONAL_B_SPLINE_SURFACE(((1.,0.67559020761567,1.),(1.,0.675585785528194,
1.),(1.,0.676431027860885,1.),(1.,0.679650528045421,1.),(1.,0.682027045382314,
1.),(1.,0.687915714942951,1.),(1.,0.691424416305301,1.),(1.,0.699004971484679,
1.),(1.,0.703073130220216,1.),(1.,0.707106781186548,1.)))
REPRESENTATION_ITEM('')
SURFACE()
);
#2808=(
BOUNDED_SURFACE()
B_SPLINE_SURFACE(3,2,((#181164,#181165,#181166),(#181167,#181168,#181169),
(#181170,#181171,#181172),(#181173,#181174,#181175)),.UNSPECIFIED.,.F.,
 .F.,.F.)
B_SPLINE_SURFACE_WITH_KNOTS((4,4),(3,3),(-3.67368196280255E-5,0.000690197182632251),
(-3.67368196280259E-5,1.),.UNSPECIFIED.)
GEOMETRIC_REPRESENTATION_ITEM()
RATIONAL_B_SPLINE_SURFACE(((1.00003296216371,0.551374288254589,1.),(1.0000330156919,
0.550645752157623,1.),(1.00003255073788,0.5569739268851,1.),(1.00003165550557,
0.569158328193655,1.)))
REPRESENTATION_ITEM('')
SURFACE()
);
#2809=(
BOUNDED_SURFACE()
B_SPLINE_SURFACE(3,2,((#181187,#181188,#181189),(#181190,#181191,#181192),
(#181193,#181194,#181195),(#181196,#181197,#181198)),.UNSPECIFIED.,.F.,
 .F.,.F.)
B_SPLINE_SURFACE_WITH_KNOTS((4,4),(3,3),(-6.51913040321377E-5,0.000717104344353579),
(-0.000141700954976534,1.),.UNSPECIFIED.)
GEOMETRIC_REPRESENTATION_ITEM()
RATIONAL_B_SPLINE_SURFACE(((1.00005816020197,0.794778369766663,1.),(1.00005608252674,
0.802109566767656,1.),(1.00005509894849,0.805580179391821,1.),(1.00005528841351,
0.804911641151865,1.)))
REPRESENTATION_ITEM('')
SURFACE()
);
#2810=(
BOUNDED_SURFACE()
B_SPLINE_SURFACE(3,2,((#181286,#181287,#181288),(#181289,#181290,#181291),
(#181292,#181293,#181294),(#181295,#181296,#181297)),.UNSPECIFIED.,.F.,
 .F.,.F.)
B_SPLINE_SURFACE_WITH_KNOTS((4,4),(3,3),(-6.5137241604418E-5,0.000716509657648598),
(-0.000128883529287276,1.),.UNSPECIFIED.)
GEOMETRIC_REPRESENTATION_ITEM()
RATIONAL_B_SPLINE_SURFACE(((1.00010029146477,0.610922104164585,1.),(1.00010049120256,
0.610147227047914,1.),(1.00009948511932,0.614050298485325,1.),(1.00009738307965,
0.622205101827837,1.)))
REPRESENTATION_ITEM('')
SURFACE()
);
#2811=(
BOUNDED_SURFACE()
B_SPLINE_SURFACE(3,2,((#181345,#181346,#181347),(#181348,#181349,#181350),
(#181351,#181352,#181353),(#181354,#181355,#181356)),.UNSPECIFIED.,.F.,
 .F.,.F.)
B_SPLINE_SURFACE_WITH_KNOTS((4,4),(3,3),(-6.50587846610001E-5,0.000715646631271033),
(-0.000198020186981615,1.),.UNSPECIFIED.)
GEOMETRIC_REPRESENTATION_ITEM()
RATIONAL_B_SPLINE_SURFACE(((1.00009701693625,0.755032712249884,1.),(1.00009537889841,
0.759168749755136,1.),(1.00009461137112,0.761106752395794,1.),(1.00009475863492,
0.760734912009421,1.)))
REPRESENTATION_ITEM('')
SURFACE()
);
#2812=(
BOUNDED_SURFACE()
B_SPLINE_SURFACE(3,2,((#181360,#181361,#181362),(#181363,#181364,#181365),
(#181366,#181367,#181368),(#181369,#181370,#181371),(#181372,#181373,#181374),
(#181375,#181376,#181377),(#181378,#181379,#181380),(#181381,#181382,#181383),
(#181384,#181385,#181386),(#181387,#181388,#181389),(#181390,#181391,#181392),
(#181393,#181394,#181395),(#181396,#181397,#181398),(#181399,#181400,#181401)),
 .UNSPECIFIED.,.F.,.F.,.F.)
B_SPLINE_SURFACE_WITH_KNOTS((4,2,2,2,2,2,4),(3,3),(0.00807909221698663,
0.00882982802565525,0.00920519592998956,0.00958056383432386,0.00995593173865817,
0.0103312996429925,0.0110820354516611),(0.,1.),.UNSPECIFIED.)
GEOMETRIC_REPRESENTATION_ITEM()
RATIONAL_B_SPLINE_SURFACE(((1.,0.707106781186556,1.),(1.,0.708510771074171,
1.),(1.,0.709878889431803,1.),(1.,0.711876867675041,1.),(1.,0.712529775389558,
1.),(1.,0.713774284861137,1.),(1.,0.714371256763372,1.),(1.,0.715514222535529,
1.),(1.,0.716062813357328,1.),(1.,0.717072969030255,1.),(1.,0.717538977439758,
1.),(1.,0.718820706504871,1.),(1.,0.719523481892828,1.),(1.,0.720009098745653,
1.)))
REPRESENTATION_ITEM('')
SURFACE()
);
#2813=(
BOUNDED_SURFACE()
B_SPLINE_SURFACE(3,2,((#181447,#181448,#181449),(#181450,#181451,#181452),
(#181453,#181454,#181455),(#181456,#181457,#181458)),.UNSPECIFIED.,.F.,
 .F.,.F.)
B_SPLINE_SURFACE_WITH_KNOTS((4,4),(3,3),(0.0318721040045715,0.0324798405467945),
(0.,0.915779521794752),.UNSPECIFIED.)
GEOMETRIC_REPRESENTATION_ITEM()
RATIONAL_B_SPLINE_SURFACE(((1.,0.819053335514945,0.969521170774848),(1.,
0.81649287568617,0.969089884472439),(1.,0.813824444819125,0.968640411425078),
(1.,0.811045676639188,0.968172353055207)))
REPRESENTATION_ITEM('')
SURFACE()
);
#2814=(
BOUNDED_SURFACE()
B_SPLINE_SURFACE(3,2,((#181591,#181592,#181593),(#181594,#181595,#181596),
(#181597,#181598,#181599),(#181600,#181601,#181602),(#181603,#181604,#181605),
(#181606,#181607,#181608),(#181609,#181610,#181611),(#181612,#181613,#181614),
(#181615,#181616,#181617),(#181618,#181619,#181620),(#181621,#181622,#181623),
(#181624,#181625,#181626),(#181627,#181628,#181629),(#181630,#181631,#181632)),
 .UNSPECIFIED.,.F.,.F.,.F.)
B_SPLINE_SURFACE_WITH_KNOTS((4,2,2,2,2,2,4),(3,3),(0.00807931853788568,
0.00881187542632408,0.00917815387054328,0.00954443231476248,0.00991071075898168,
0.0102769892032009,0.0110095460916393),(0.,1.),.UNSPECIFIED.)
GEOMETRIC_REPRESENTATION_ITEM()
RATIONAL_B_SPLINE_SURFACE(((1.,0.707106781186552,1.),(1.,0.705694108475444,
1.),(1.,0.704309639709031,1.),(1.,0.702276829363826,1.),(1.,0.701608277715413,
1.),(1.,0.700330266875156,1.),(1.,0.699715065357364,1.),(1.,0.698533028725346,
1.),(1.,0.697962156582885,1.),(1.,0.696902668323859,1.),(1.,0.696411414935025,
1.),(1.,0.695052392645847,1.),(1.,0.69429223033984,1.),(1.,0.69374733452232,
1.)))
REPRESENTATION_ITEM('')
SURFACE()
);
#2815=(
BOUNDED_SURFACE()
B_SPLINE_SURFACE(3,2,((#181733,#181734,#181735),(#181736,#181737,#181738),
(#181739,#181740,#181741),(#181742,#181743,#181744)),.UNSPECIFIED.,.F.,
 .F.,.F.)
B_SPLINE_SURFACE_WITH_KNOTS((4,4),(3,3),(0.,0.000650359837711272),(0.,1.),
 .UNSPECIFIED.)
GEOMETRIC_REPRESENTATION_ITEM()
RATIONAL_B_SPLINE_SURFACE(((1.,0.665108204576639,1.),(1.,0.66511166059484,
1.),(1.,0.666441892349684,1.),(1.,0.669061697655964,1.)))
REPRESENTATION_ITEM('')
SURFACE()
);
#2816=(
BOUNDED_SURFACE()
B_SPLINE_SURFACE(3,2,((#181783,#181784,#181785),(#181786,#181787,#181788),
(#181789,#181790,#181791),(#181792,#181793,#181794)),.UNSPECIFIED.,.F.,
 .F.,.F.)
B_SPLINE_SURFACE_WITH_KNOTS((4,4),(3,3),(0.,0.000650121463573334),(0.,1.),
 .UNSPECIFIED.)
GEOMETRIC_REPRESENTATION_ITEM()
RATIONAL_B_SPLINE_SURFACE(((1.,0.713284154090124,1.),(1.,0.713692564168438,
1.),(1.,0.713902215282654,1.),(1.,0.713903527556066,1.)))
REPRESENTATION_ITEM('')
SURFACE()
);
#2817=(
BOUNDED_SURFACE()
B_SPLINE_SURFACE(3,2,((#181798,#181799,#181800),(#181801,#181802,#181803),
(#181804,#181805,#181806),(#181807,#181808,#181809),(#181810,#181811,#181812),
(#181813,#181814,#181815),(#181816,#181817,#181818),(#181819,#181820,#181821),
(#181822,#181823,#181824),(#181825,#181826,#181827)),.UNSPECIFIED.,.F.,
 .F.,.F.)
B_SPLINE_SURFACE_WITH_KNOTS((4,2,2,2,4),(3,3),(0.00807567041695258,0.00870229794915108,
0.00932892548134959,0.00995555301354809,0.0105821805457466),(0.,1.),
 .UNSPECIFIED.)
GEOMETRIC_REPRESENTATION_ITEM()
RATIONAL_B_SPLINE_SURFACE(((1.,0.707106781186548,1.),(1.,0.707144476742774,
1.),(1.,0.707181156772813,1.),(1.,0.707252569458078,1.),(1.,0.707287275051322,
1.),(1.,0.707350941456054,1.),(1.,0.707380803865577,1.),(1.,0.707433415861318,
1.),(1.,0.707456236659423,1.),(1.,0.707475611987371,1.)))
REPRESENTATION_ITEM('')
SURFACE()
);
#2818=(
BOUNDED_SURFACE()
B_SPLINE_SURFACE(3,2,((#181942,#181943,#181944),(#181945,#181946,#181947),
(#181948,#181949,#181950),(#181951,#181952,#181953)),.UNSPECIFIED.,.F.,
 .F.,.F.)
B_SPLINE_SURFACE_WITH_KNOTS((4,4),(3,3),(0.0237206528291238,0.0242322821884044),
(0.,0.921037832550836),.UNSPECIFIED.)
GEOMETRIC_REPRESENTATION_ITEM()
RATIONAL_B_SPLINE_SURFACE(((1.,0.866462949751686,0.97891125015525),(1.,
0.866562397986968,0.978926955451664),(1.,0.866592995680722,0.9789317875721),
(1.,0.866554773618892,0.978925751378407)))
REPRESENTATION_ITEM('')
SURFACE()
);
#2819=(
BOUNDED_SURFACE()
B_SPLINE_SURFACE(3,2,((#182017,#182018,#182019),(#182020,#182021,#182022),
(#182023,#182024,#182025),(#182026,#182027,#182028),(#182029,#182030,#182031),
(#182032,#182033,#182034),(#182035,#182036,#182037),(#182038,#182039,#182040),
(#182041,#182042,#182043),(#182044,#182045,#182046)),.UNSPECIFIED.,.F.,
 .F.,.F.)
B_SPLINE_SURFACE_WITH_KNOTS((4,2,2,2,4),(3,3),(0.00807569195610403,0.00870260410927289,
0.00932951626244174,0.0099564284156106,0.0105833405687795),(0.,1.),
 .UNSPECIFIED.)
GEOMETRIC_REPRESENTATION_ITEM()
RATIONAL_B_SPLINE_SURFACE(((1.,0.707106781186548,1.),(1.,0.707206112905989,
1.),(1.,0.707302756119535,1.),(1.,0.707490889447615,1.),(1.,0.707582303244654,
1.),(1.,0.707749976398179,1.),(1.,0.707828611057685,1.),(1.,0.70796711497316,
1.),(1.,0.708027180199908,1.),(1.,0.708078164615097,1.)))
REPRESENTATION_ITEM('')
SURFACE()
);
#2820=(
BOUNDED_SURFACE()
B_SPLINE_SURFACE(3,2,((#182150,#182151,#182152),(#182153,#182154,#182155),
(#182156,#182157,#182158),(#182159,#182160,#182161)),.UNSPECIFIED.,.F.,
 .F.,.F.)
B_SPLINE_SURFACE_WITH_KNOTS((4,4),(3,3),(0.,0.000650124307745721),(0.,1.),
 .UNSPECIFIED.)
GEOMETRIC_REPRESENTATION_ITEM()
RATIONAL_B_SPLINE_SURFACE(((1.,0.715240287646145,1.),(1.,0.715239393380683,
1.),(1.,0.714992351911572,1.),(1.,0.71449972514277,1.)))
REPRESENTATION_ITEM('')
SURFACE()
);
#2821=(
BOUNDED_SURFACE()
B_SPLINE_SURFACE(3,2,((#182209,#182210,#182211),(#182212,#182213,#182214),
(#182215,#182216,#182217),(#182218,#182219,#182220)),.UNSPECIFIED.,.F.,
 .F.,.F.)
B_SPLINE_SURFACE_WITH_KNOTS((4,4),(3,3),(0.,0.0006503810773206),(0.,1.),
 .UNSPECIFIED.)
GEOMETRIC_REPRESENTATION_ITEM()
RATIONAL_B_SPLINE_SURFACE(((1.,0.667763418073535,1.),(1.,0.665075430476096,
1.),(1.,0.663677894706716,1.),(1.,0.663670476501713,1.)))
REPRESENTATION_ITEM('')
SURFACE()
);
#2822=(
BOUNDED_SURFACE()
B_SPLINE_SURFACE(3,2,((#182224,#182225,#182226),(#182227,#182228,#182229),
(#182230,#182231,#182232),(#182233,#182234,#182235),(#182236,#182237,#182238),
(#182239,#182240,#182241),(#182242,#182243,#182244),(#182245,#182246,#182247),
(#182248,#182249,#182250),(#182251,#182252,#182253),(#182254,#182255,#182256),
(#182257,#182258,#182259),(#182260,#182261,#182262),(#182263,#182264,#182265)),
 .UNSPECIFIED.,.F.,.F.,.F.)
B_SPLINE_SURFACE_WITH_KNOTS((4,2,2,2,2,2,4),(3,3),(0.00807922902311453,
0.00881773053780572,0.00918698129515131,0.0095562320524969,0.0099254828098425,
0.0102947335671881,0.0110332350818793),(0.,1.),.UNSPECIFIED.)
GEOMETRIC_REPRESENTATION_ITEM()
RATIONAL_B_SPLINE_SURFACE(((1.,0.707106781186548,1.),(1.,0.705699386801107,
1.),(1.,0.704319784944778,1.),(1.,0.702293838625036,1.),(1.,0.701628229397446,
1.),(1.,0.700355977320158,1.),(1.,0.699743668156969,1.),(1.,0.698567591087498,
1.),(1.,0.698000119405105,1.),(1.,0.696949115865192,1.),(1.,0.696462203809247,
1.),(1.,0.695116916536575,1.),(1.,0.694367821279467,1.),(1.,0.693837065201558,
1.)))
REPRESENTATION_ITEM('')
SURFACE()
);
#2823=(
BOUNDED_SURFACE()
B_SPLINE_SURFACE(3,2,((#182373,#182374,#182375),(#182376,#182377,#182378),
(#182379,#182380,#182381),(#182382,#182383,#182384)),.UNSPECIFIED.,.F.,
 .F.,.F.)
B_SPLINE_SURFACE_WITH_KNOTS((4,4),(3,3),(0.0154746506919765,0.0160816000283851),
(0.,0.915442911086902),.UNSPECIFIED.)
GEOMETRIC_REPRESENTATION_ITEM()
RATIONAL_B_SPLINE_SURFACE(((1.,0.807945871955147,0.967520924037568),(1.,
0.810803635237244,0.968004212325442),(1.,0.813550381031034,0.968468725982056),
(1.,0.816188583297829,0.968914883389344)))
REPRESENTATION_ITEM('')
SURFACE()
);
#2824=(
BOUNDED_SURFACE()
B_SPLINE_SURFACE(3,2,((#182419,#182420,#182421),(#182422,#182423,#182424),
(#182425,#182426,#182427),(#182428,#182429,#182430),(#182431,#182432,#182433),
(#182434,#182435,#182436),(#182437,#182438,#182439),(#182440,#182441,#182442),
(#182443,#182444,#182445),(#182446,#182447,#182448),(#182449,#182450,#182451),
(#182452,#182453,#182454),(#182455,#182456,#182457),(#182458,#182459,#182460)),
 .UNSPECIFIED.,.F.,.F.,.F.)
B_SPLINE_SURFACE_WITH_KNOTS((4,2,2,2,2,2,4),(3,3),(0.00807895877935271,
0.00883634587130868,0.00921503941728666,0.00959373296326465,0.00997242650924264,
0.0103511200552206,0.0111085071471766),(0.,1.),.UNSPECIFIED.)
GEOMETRIC_REPRESENTATION_ITEM()
RATIONAL_B_SPLINE_SURFACE(((1.,0.707106781186548,1.),(1.,0.708496200821205,
1.),(1.,0.70985049824013,1.),(1.,0.711828637936002,1.),(1.,0.712474210732742,
1.),(1.,0.71370482119381,1.),(1.,0.714294998379545,1.),(1.,0.715424510819791,
1.),(1.,0.715965704866287,1.),(1.,0.716960611510995,1.),(1.,0.71741913219781,
1.),(1.,0.71867831515119,1.),(1.,0.719364099598229,1.),(1.,0.719832136235989,
1.)))
REPRESENTATION_ITEM('')
SURFACE()
);
#2825=(
BOUNDED_SURFACE()
B_SPLINE_SURFACE(3,2,((#182582,#182583,#182584),(#182585,#182586,#182587),
(#182588,#182589,#182590),(#182591,#182592,#182593)),.UNSPECIFIED.,.F.,
 .F.,.F.)
B_SPLINE_SURFACE_WITH_KNOTS((4,4),(3,3),(0.,0.00065060314950297),(0.,1.),
 .UNSPECIFIED.)
GEOMETRIC_REPRESENTATION_ITEM()
RATIONAL_B_SPLINE_SURFACE(((1.,0.762081632339421,1.),(1.,0.762075781187422,
1.),(1.,0.760455646763466,1.),(1.,0.757216058458816,1.)))
REPRESENTATION_ITEM('')
SURFACE()
);
#2826=(
BOUNDED_SURFACE()
B_SPLINE_SURFACE(3,2,((#182605,#182606,#182607),(#182608,#182609,#182610),
(#182611,#182612,#182613),(#182614,#182615,#182616)),.UNSPECIFIED.,.F.,
 .F.,.F.)
B_SPLINE_SURFACE_WITH_KNOTS((4,4),(3,3),(-6.51439314691719E-5,0.0007165832461609),
(-0.00012692018125823,1.),.UNSPECIFIED.)
GEOMETRIC_REPRESENTATION_ITEM()
RATIONAL_B_SPLINE_SURFACE(((1.00009625164489,0.620818202688323,1.),(1.00009833294279,
0.612618963298313,1.),(1.00009936087757,0.608569430840879,1.),(1.00009916096194,
0.609356995261984,1.)))
REPRESENTATION_ITEM('')
SURFACE()
);
#2827=(
BOUNDED_SURFACE()
B_SPLINE_SURFACE(3,2,((#182759,#182760,#182761),(#182762,#182763,#182764),
(#182765,#182766,#182767),(#182768,#182769,#182770)),.UNSPECIFIED.,.F.,
 .F.,.F.)
B_SPLINE_SURFACE_WITH_KNOTS((4,4),(3,3),(-6.51926395977004E-5,0.000717119035574768),
(-0.000138815926047248,1.),.UNSPECIFIED.)
GEOMETRIC_REPRESENTATION_ITEM()
RATIONAL_B_SPLINE_SURFACE(((1.00005383408411,0.806095432842632,1.),(1.00005364581143,
0.806773570717775,1.),(1.00005460199526,0.803329499666753,1.),(1.00005668422386,
0.795829536739356,1.)))
REPRESENTATION_ITEM('')
SURFACE()
);
#2828=(
BOUNDED_SURFACE()
B_SPLINE_SURFACE(3,2,((#182776,#182777,#182778),(#182779,#182780,#182781),
(#182782,#182783,#182784),(#182785,#182786,#182787)),.UNSPECIFIED.,.F.,
 .F.,.F.)
B_SPLINE_SURFACE_WITH_KNOTS((4,4),(3,3),(0.00485453262895891,0.0055923285159134),
(0.,1.00004278948359),.UNSPECIFIED.)
GEOMETRIC_REPRESENTATION_ITEM()
RATIONAL_B_SPLINE_SURFACE(((1.,0.567949101515402,1.00003697446966),(1.,
0.55537551727941,1.00003805050401),(1.,0.548757935635794,1.00003861682981),
(1.,0.549661265383694,1.00003853952379)))
REPRESENTATION_ITEM('')
SURFACE()
);
#2829=(
BOUNDED_SURFACE()
B_SPLINE_SURFACE(3,2,((#183025,#183026,#183027),(#183028,#183029,#183030),
(#183031,#183032,#183033),(#183034,#183035,#183036),(#183037,#183038,#183039),
(#183040,#183041,#183042),(#183043,#183044,#183045),(#183046,#183047,#183048),
(#183049,#183050,#183051),(#183052,#183053,#183054)),.UNSPECIFIED.,.F.,
 .F.,.F.)
B_SPLINE_SURFACE_WITH_KNOTS((4,2,2,2,4),(3,3),(0.00807856278467327,0.00871080510931882,
0.00934304743396438,0.00997528975860994,0.0106075320832555),(0.,1.),
 .UNSPECIFIED.)
GEOMETRIC_REPRESENTATION_ITEM()
RATIONAL_B_SPLINE_SURFACE(((1.,0.707106781186548,1.),(1.,0.706030220592194,
1.),(1.,0.704978540375902,1.),(1.,0.702923837367757,1.),(1.,0.701922380471311,
1.),(1.,0.700080728636545,1.),(1.,0.699214393311896,1.),(1.,0.697689255248067,
1.),(1.,0.697026914527849,1.),(1.,0.696465765714756,1.)))
REPRESENTATION_ITEM('')
SURFACE()
);
#2830=(
BOUNDED_SURFACE()
B_SPLINE_SURFACE(3,2,((#183211,#183212,#183213),(#183214,#183215,#183216),
(#183217,#183218,#183219),(#183220,#183221,#183222)),.UNSPECIFIED.,.F.,
 .F.,.F.)
B_SPLINE_SURFACE_WITH_KNOTS((4,4),(3,3),(0.0283524505452003,0.0289409470909155),
(0.0793668899028847,1.),.UNSPECIFIED.)
GEOMETRIC_REPRESENTATION_ITEM()
RATIONAL_B_SPLINE_SURFACE(((0.978461885750617,0.864312975626627,1.),(0.978267423016933,
0.863087888352061,1.),(0.978058310717098,0.861770510916135,1.),(0.977834425305255,
0.860360064997711,1.)))
REPRESENTATION_ITEM('')
SURFACE()
);
#2831=(
BOUNDED_SURFACE()
B_SPLINE_SURFACE(3,2,((#183319,#183320,#183321),(#183322,#183323,#183324),
(#183325,#183326,#183327),(#183328,#183329,#183330),(#183331,#183332,#183333),
(#183334,#183335,#183336),(#183337,#183338,#183339),(#183340,#183341,#183342),
(#183343,#183344,#183345),(#183346,#183347,#183348),(#183349,#183350,#183351),
(#183352,#183353,#183354)),.UNSPECIFIED.,.F.,.F.,.F.)
B_SPLINE_SURFACE_WITH_KNOTS((4,2,2,2,2,4),(3,3),(0.00807907499033046,0.00872002967587247,
0.00904050701864348,0.00936098436141448,0.0100019390469565,0.0106428937324985),
(0.,1.),.UNSPECIFIED.)
GEOMETRIC_REPRESENTATION_ITEM()
RATIONAL_B_SPLINE_SURFACE(((1.,0.707106781186548,1.),(1.,0.708291653108703,
1.),(1.,0.709443749235048,1.),(1.,0.71112469687116,1.),(1.,0.711680940824733,
1.),(1.,0.712751570007901,1.),(1.,0.713267249229028,1.),(1.,0.714757432797168,
1.),(1.,0.715686917775259,1.),(1.,0.717310091250008,1.),(1.,0.718010566750711,
1.),(1.,0.718598488256614,1.)))
REPRESENTATION_ITEM('')
SURFACE()
);
#2832=(
BOUNDED_SURFACE()
B_SPLINE_SURFACE(3,2,((#183462,#183463,#183464),(#183465,#183466,#183467),
(#183468,#183469,#183470),(#183471,#183472,#183473)),.UNSPECIFIED.,.F.,
 .F.,.F.)
B_SPLINE_SURFACE_WITH_KNOTS((4,4),(3,3),(0.,0.000650274811908555),(0.,1.),
 .UNSPECIFIED.)
GEOMETRIC_REPRESENTATION_ITEM()
RATIONAL_B_SPLINE_SURFACE(((1.,0.73939111071482,1.),(1.,0.73938749716724,
1.),(1.,0.738423154307972,1.),(1.,0.736495153922513,1.)))
REPRESENTATION_ITEM('')
SURFACE()
);
#2833=(
BOUNDED_SURFACE()
B_SPLINE_SURFACE(3,2,((#183547,#183548,#183549),(#183550,#183551,#183552),
(#183553,#183554,#183555),(#183556,#183557,#183558)),.UNSPECIFIED.,.F.,
 .F.,.F.)
B_SPLINE_SURFACE_WITH_KNOTS((4,4),(3,3),(-6.5085150333794E-5,0.000715936653671951),
(-0.00015557324309298,1.),.UNSPECIFIED.)
GEOMETRIC_REPRESENTATION_ITEM()
RATIONAL_B_SPLINE_SURFACE(((1.00011117085853,0.642705723933352,1.),(1.00011304395471,
0.636685742162949,1.),(1.00011395382865,0.633761479841946,1.),(1.00011377765073,
0.634327701648564,1.)))
REPRESENTATION_ITEM('')
SURFACE()
);
#2834=(
BOUNDED_SURFACE()
B_SPLINE_SURFACE(3,2,((#183562,#183563,#183564),(#183565,#183566,#183567),
(#183568,#183569,#183570),(#183571,#183572,#183573),(#183574,#183575,#183576),
(#183577,#183578,#183579),(#183580,#183581,#183582),(#183583,#183584,#183585),
(#183586,#183587,#183588),(#183589,#183590,#183591),(#183592,#183593,#183594),
(#183595,#183596,#183597)),.UNSPECIFIED.,.F.,.F.,.F.)
B_SPLINE_SURFACE_WITH_KNOTS((4,2,2,2,2,4),(3,3),(0.00807589507756136,0.00894079878156724,
0.00980570248557312,0.010238154337576,0.010670606189579,0.0115355098935849),
(0.,1.),.UNSPECIFIED.)
GEOMETRIC_REPRESENTATION_ITEM()
RATIONAL_B_SPLINE_SURFACE(((1.,0.707106781186548,1.),(1.,0.706684802682679,
1.),(1.,0.706265611788784,1.),(1.,0.705449765784865,1.),(1.,0.705070572349072,
1.),(1.,0.704559600788765,1.),(1.,0.704402907652403,1.),(1.,0.7041166887103,
1.),(1.,0.703986299022118,1.),(1.,0.703645597188673,1.),(1.,0.703488957328521,
1.),(1.,0.703406029216022,1.)))
REPRESENTATION_ITEM('')
SURFACE()
);
#2835=(
BOUNDED_SURFACE()
B_SPLINE_SURFACE(3,2,((#183769,#183770,#183771),(#183772,#183773,#183774),
(#183775,#183776,#183777),(#183778,#183779,#183780)),.UNSPECIFIED.,.F.,
 .F.,.F.)
B_SPLINE_SURFACE_WITH_KNOTS((4,4),(3,3),(0.0370067204754696,0.0375452288399126),
(0.093403953485077,1.),.UNSPECIFIED.)
GEOMETRIC_REPRESENTATION_ITEM()
RATIONAL_B_SPLINE_SURFACE(((0.953268748425463,0.74984328911729,1.),(0.952543344408727,
0.745960134338133,1.),(0.951798218335464,0.741971405566697,1.),(0.951032530022134,
0.737872605222811,1.)))
REPRESENTATION_ITEM('')
SURFACE()
);
#2836=(
BOUNDED_SURFACE()
B_SPLINE_SURFACE(3,2,((#183865,#183866,#183867),(#183868,#183869,#183870),
(#183871,#183872,#183873),(#183874,#183875,#183876),(#183877,#183878,#183879),
(#183880,#183881,#183882),(#183883,#183884,#183885),(#183886,#183887,#183888),
(#183889,#183890,#183891),(#183892,#183893,#183894),(#183895,#183896,#183897),
(#183898,#183899,#183900),(#183901,#183902,#183903),(#183904,#183905,#183906)),
 .UNSPECIFIED.,.F.,.F.,.F.)
B_SPLINE_SURFACE_WITH_KNOTS((4,2,2,2,2,2,4),(3,3),(0.00807568025026493,
0.00898700204274496,0.00944266293898498,0.009898323835225,0.010353984731465,
0.010809645627705,0.0117209674201851),(0.,1.),.UNSPECIFIED.)
GEOMETRIC_REPRESENTATION_ITEM()
RATIONAL_B_SPLINE_SURFACE(((1.,0.707106781186546,1.),(1.,0.707214557916128,
1.),(1.,0.707322930753557,1.),(1.,0.707478596210236,1.),(1.,0.707528365558662,
1.),(1.,0.70762361150633,1.),(1.,0.70766951928712,1.),(1.,0.70775397022188,
1.),(1.,0.707792549798564,1.),(1.,0.707862266510969,1.),(1.,0.707893578069266,
1.),(1.,0.707972242595767,1.),(1.,0.70800597758526,1.),(1.,0.708018339291814,
1.)))
REPRESENTATION_ITEM('')
SURFACE()
);
#2837=(
BOUNDED_SURFACE()
B_SPLINE_SURFACE(3,2,((#184041,#184042,#184043),(#184044,#184045,#184046),
(#184047,#184048,#184049),(#184050,#184051,#184052)),.UNSPECIFIED.,.F.,
 .F.,.F.)
B_SPLINE_SURFACE_WITH_KNOTS((4,4),(3,3),(-6.51209638471711E-5,0.0007163306023189),
(-0.000173014936682415,1.),.UNSPECIFIED.)
GEOMETRIC_REPRESENTATION_ITEM()
RATIONAL_B_SPLINE_SURFACE(((1.00007384993111,0.786579319308486,1.),(1.00007366103227,
0.787125222591237,1.),(1.00007462377578,0.784342967102351,1.),(1.000076734131,
0.778244201129574,1.)))
REPRESENTATION_ITEM('')
SURFACE()
);
#2838=(
BOUNDED_SURFACE()
B_SPLINE_SURFACE(3,2,((#184058,#184059,#184060),(#184061,#184062,#184063),
(#184064,#184065,#184066),(#184067,#184068,#184069)),.UNSPECIFIED.,.F.,
 .F.,.F.)
B_SPLINE_SURFACE_WITH_KNOTS((4,4),(3,3),(-6.52563961816873E-5,0.000717820357998492),
(-7.66067673815307E-5,1.),.UNSPECIFIED.)
GEOMETRIC_REPRESENTATION_ITEM()
RATIONAL_B_SPLINE_SURFACE(((1.00006271537587,0.590666869146107,1.),(1.00006444960589,
0.579347829852736,1.),(1.0000653307431,0.573596789585195,1.),(1.00006515810741,
0.574723554882865,1.)))
REPRESENTATION_ITEM('')
SURFACE()
);
#2839=(
BOUNDED_SURFACE()
B_SPLINE_SURFACE(3,2,((#184193,#184194,#184195),(#184196,#184197,#184198),
(#184199,#184200,#184201),(#184202,#184203,#184204)),.UNSPECIFIED.,.F.,
 .F.,.F.)
B_SPLINE_SURFACE_WITH_KNOTS((4,4),(3,3),(0.,0.000921798889909707),(0.,1.),
 .UNSPECIFIED.)
GEOMETRIC_REPRESENTATION_ITEM()
RATIONAL_B_SPLINE_SURFACE(((1.,0.831289505264087,1.),(1.,0.831333394817592,
1.),(1.,0.824011622363235,1.),(1.,0.810617639934149,1.)))
REPRESENTATION_ITEM('')
SURFACE()
);
#2840=(
BOUNDED_SURFACE()
B_SPLINE_SURFACE(3,2,((#184372,#184373,#184374),(#184375,#184376,#184377),
(#184378,#184379,#184380),(#184381,#184382,#184383)),.UNSPECIFIED.,.F.,
 .F.,.F.)
B_SPLINE_SURFACE_WITH_KNOTS((4,4),(3,3),(-3.51472716647773E-5,0.000688646726988702),
(-3.51472716647773E-5,1.),.UNSPECIFIED.)
GEOMETRIC_REPRESENTATION_ITEM()
RATIONAL_B_SPLINE_SURFACE(((1.00003159713423,0.550503741378662,1.),(1.00003164632144,
0.54980401125791,1.),(1.00003120056771,0.556145239310851,1.),(1.00003034444782,
0.568324276979128,1.)))
REPRESENTATION_ITEM('')
SURFACE()
);
#2841=(
BOUNDED_SURFACE()
B_SPLINE_SURFACE(3,2,((#184396,#184397,#184398),(#184399,#184400,#184401),
(#184402,#184403,#184404),(#184405,#184406,#184407)),.UNSPECIFIED.,.F.,
 .F.,.F.)
B_SPLINE_SURFACE_WITH_KNOTS((4,4),(3,3),(-6.51938878740144E-5,0.000717132766614092),
(-0.000140422077604399,1.),.UNSPECIFIED.)
GEOMETRIC_REPRESENTATION_ITEM()
RATIONAL_B_SPLINE_SURFACE(((1.00005748506357,0.795313299193262,1.),(1.00005541449137,
0.802685972468769,1.),(1.00005443402968,0.806177096184806,1.),(1.00005462291181,
0.805504544806424,1.)))
REPRESENTATION_ITEM('')
SURFACE()
);
#2842=(
BOUNDED_SURFACE()
B_SPLINE_SURFACE(3,2,((#184496,#184497,#184498),(#184499,#184500,#184501),
(#184502,#184503,#184504),(#184505,#184506,#184507)),.UNSPECIFIED.,.F.,
 .F.,.F.)
B_SPLINE_SURFACE_WITH_KNOTS((4,4),(3,3),(-6.51392861930307E-5,0.000716532148123338),
(-0.000127892595311363,1.),.UNSPECIFIED.)
GEOMETRIC_REPRESENTATION_ITEM()
RATIONAL_B_SPLINE_SURFACE(((1.00009972016694,0.610140967503593,1.),(1.00009992021532,
0.609358872291238,1.),(1.00009891274698,0.613297600455479,1.),(1.0000968090023,
0.621522254435956,1.)))
REPRESENTATION_ITEM('')
SURFACE()
);
#2843=(
BOUNDED_SURFACE()
B_SPLINE_SURFACE(3,2,((#184567,#184568,#184569),(#184570,#184571,#184572),
(#184573,#184574,#184575),(#184576,#184577,#184578)),.UNSPECIFIED.,.F.,
 .F.,.F.)
B_SPLINE_SURFACE_WITH_KNOTS((4,4),(3,3),(-6.5059972238603E-5,0.000715659694624669),
(-0.000197643858000933,1.),.UNSPECIFIED.)
GEOMETRIC_REPRESENTATION_ITEM()
RATIONAL_B_SPLINE_SURFACE(((1.00009661013076,0.755595413549805,1.),(1.00009495673333,
0.759778183122702,1.),(1.0000941819758,0.761738166948696,1.),(1.00009433062994,
0.761362101277921,1.)))
REPRESENTATION_ITEM('')
SURFACE()
);
#2844=(
BOUNDED_SURFACE()
B_SPLINE_SURFACE(3,2,((#184582,#184583,#184584),(#184585,#184586,#184587),
(#184588,#184589,#184590),(#184591,#184592,#184593),(#184594,#184595,#184596),
(#184597,#184598,#184599),(#184600,#184601,#184602),(#184603,#184604,#184605),
(#184606,#184607,#184608),(#184609,#184610,#184611),(#184612,#184613,#184614),
(#184615,#184616,#184617)),.UNSPECIFIED.,.F.,.F.,.F.)
B_SPLINE_SURFACE_WITH_KNOTS((4,2,2,2,2,4),(3,3),(0.00807807165860127,0.00885401549830484,
0.00962995933800841,0.0100179312578602,0.010405903177712,0.0111818470174155),
(0.,1.),.UNSPECIFIED.)
GEOMETRIC_REPRESENTATION_ITEM()
RATIONAL_B_SPLINE_SURFACE(((1.,0.707106781186548,1.),(1.,0.708323960348238,
1.),(1.,0.709510365636766,1.),(1.,0.711820403892163,1.),(1.,0.712901935204825,
1.),(1.,0.714375984986412,1.),(1.,0.714843782196838,1.),(1.,0.715700614088123,
1.),(1.,0.716094239791898,1.),(1.,0.71717000694229,1.),(1.,0.717742537382462,
1.),(1.,0.718120418666571,1.)))
REPRESENTATION_ITEM('')
SURFACE()
);
#2845=(
BOUNDED_SURFACE()
B_SPLINE_SURFACE(3,2,((#184765,#184766,#184767),(#184768,#184769,#184770),
(#184771,#184772,#184773),(#184774,#184775,#184776)),.UNSPECIFIED.,.F.,
 .F.,.F.)
B_SPLINE_SURFACE_WITH_KNOTS((4,4),(3,3),(0.0316780996002149,0.032272159678108),
(0.,0.914522259344732),.UNSPECIFIED.)
GEOMETRIC_REPRESENTATION_ITEM()
RATIONAL_B_SPLINE_SURFACE(((1.,0.807106741558702,0.96702384016161),(1.,
0.804531496903973,0.966583587972169),(1.,0.801850982035351,0.966125339262643),
(1.,0.799062830164071,0.965648689417522)))
REPRESENTATION_ITEM('')
SURFACE()
);
#2846=(
BOUNDED_SURFACE()
B_SPLINE_SURFACE(3,2,((#184867,#184868,#184869),(#184870,#184871,#184872),
(#184873,#184874,#184875),(#184876,#184877,#184878),(#184879,#184880,#184881),
(#184882,#184883,#184884),(#184885,#184886,#184887),(#184888,#184889,#184890),
(#184891,#184892,#184893),(#184894,#184895,#184896),(#184897,#184898,#184899),
(#184900,#184901,#184902),(#184903,#184904,#184905),(#184906,#184907,#184908)),
 .UNSPECIFIED.,.F.,.F.,.F.)
B_SPLINE_SURFACE_WITH_KNOTS((4,2,2,2,2,2,4),(3,3),(0.00807831625971351,
0.00883535021604665,0.00921386719421322,0.00959238417237979,0.00997090115054636,
0.0103494181287129,0.0111064520850461),(0.,1.),.UNSPECIFIED.)
GEOMETRIC_REPRESENTATION_ITEM()
RATIONAL_B_SPLINE_SURFACE(((1.,0.707106781186548,1.),(1.,0.705861961062141,
1.),(1.,0.704642623504988,1.),(1.,0.702853606538468,1.),(1.,0.702268342990035,
1.),(1.,0.701150362247141,1.),(1.,0.700612993986993,1.),(1.,0.699582583564998,
1.),(1.,0.699087807793684,1.),(1.,0.698176683118393,1.),(1.,0.697755963868462,
1.),(1.,0.696598958196255,1.),(1.,0.695966377684547,1.),(1.,0.695533955710884,
1.)))
REPRESENTATION_ITEM('')
SURFACE()
);
#2847=(
BOUNDED_SURFACE()
B_SPLINE_SURFACE(3,2,((#185016,#185017,#185018),(#185019,#185020,#185021),
(#185022,#185023,#185024),(#185025,#185026,#185027)),.UNSPECIFIED.,.F.,
 .F.,.F.)
B_SPLINE_SURFACE_WITH_KNOTS((4,4),(3,3),(0.,0.000650368158908551),(0.,1.),
 .UNSPECIFIED.)
GEOMETRIC_REPRESENTATION_ITEM()
RATIONAL_B_SPLINE_SURFACE(((1.,0.66438972944168,1.),(1.,0.664393217905862,
1.),(1.,0.665747114157887,1.),(1.,0.66841287307604,1.)))
REPRESENTATION_ITEM('')
SURFACE()
);
#2848=(
BOUNDED_SURFACE()
B_SPLINE_SURFACE(3,2,((#185110,#185111,#185112),(#185113,#185114,#185115),
(#185116,#185117,#185118),(#185119,#185120,#185121)),.UNSPECIFIED.,.F.,
 .F.,.F.)
B_SPLINE_SURFACE_WITH_KNOTS((4,4),(3,3),(0.,0.000650122897330092),(0.,1.),
 .UNSPECIFIED.)
GEOMETRIC_REPRESENTATION_ITEM()
RATIONAL_B_SPLINE_SURFACE(((1.,0.713892198341303,1.),(1.,0.714340614318511,
1.),(1.,0.714570777789516,1.),(1.,0.714572220188112,1.)))
REPRESENTATION_ITEM('')
SURFACE()
);
#2849=(
BOUNDED_SURFACE()
B_SPLINE_SURFACE(3,2,((#185125,#185126,#185127),(#185128,#185129,#185130),
(#185131,#185132,#185133),(#185134,#185135,#185136),(#185137,#185138,#185139),
(#185140,#185141,#185142),(#185143,#185144,#185145),(#185146,#185147,#185148),
(#185149,#185150,#185151),(#185152,#185153,#185154),(#185155,#185156,#185157),
(#185158,#185159,#185160)),.UNSPECIFIED.,.F.,.F.,.F.)
B_SPLINE_SURFACE_WITH_KNOTS((4,2,2,2,2,4),(3,3),(0.00807567643991074,0.0087258483708248,
0.00905093433628183,0.00937602030173886,0.0100261922326529,0.010676364163567),
(0.,1.),.UNSPECIFIED.)
GEOMETRIC_REPRESENTATION_ITEM()
RATIONAL_B_SPLINE_SURFACE(((1.,0.707106781186547,1.),(1.,0.707170635637275,
1.),(1.,0.707232744268554,1.),(1.,0.70732338528182,1.),(1.,0.707353375007997,
1.),(1.,0.707410998957093,1.),(1.,0.707438747129451,1.),(1.,0.707518900645085,
1.),(1.,0.707568814651682,1.),(1.,0.707655521042551,1.),(1.,0.707692858707996,
1.),(1.,0.707723858215708,1.)))
REPRESENTATION_ITEM('')
SURFACE()
);
#2850=(
BOUNDED_SURFACE()
B_SPLINE_SURFACE(3,2,((#185275,#185276,#185277),(#185278,#185279,#185280),
(#185281,#185282,#185283),(#185284,#185285,#185286),(#185287,#185288,#185289),
(#185290,#185291,#185292),(#185293,#185294,#185295),(#185296,#185297,#185298),
(#185299,#185300,#185301),(#185302,#185303,#185304)),.UNSPECIFIED.,.F.,
 .F.,.F.)
B_SPLINE_SURFACE_WITH_KNOTS((4,2,2,2,4),(3,3),(0.00807567872552143,0.00870243807057167,
0.0093291974156219,0.00995595676067213,0.0105827161057224),(0.,1.),
 .UNSPECIFIED.)
GEOMETRIC_REPRESENTATION_ITEM()
RATIONAL_B_SPLINE_SURFACE(((1.,0.707106781186547,1.),(1.,0.707175173315664,
1.),(1.,0.707241719347897,1.),(1.,0.707371272007346,1.),(1.,0.70743422794471,
1.),(1.,0.707549712034256,1.),(1.,0.707603875852248,1.),(1.,0.707699291327501,
1.),(1.,0.707740674853624,1.),(1.,0.707775806502368,1.)))
REPRESENTATION_ITEM('')
SURFACE()
);
#2851=(
BOUNDED_SURFACE()
B_SPLINE_SURFACE(3,2,((#185425,#185426,#185427),(#185428,#185429,#185430),
(#185431,#185432,#185433),(#185434,#185435,#185436)),.UNSPECIFIED.,.F.,
 .F.,.F.)
B_SPLINE_SURFACE_WITH_KNOTS((4,4),(3,3),(-2.91650384398601E-17,0.000810744804887501),
(0.,1.),.UNSPECIFIED.)
GEOMETRIC_REPRESENTATION_ITEM()
RATIONAL_B_SPLINE_SURFACE(((1.,0.804104907750019,1.),(1.,0.778265384411316,
1.),(1.,0.743775615594857,1.),(1.,0.707106781186549,1.)))
REPRESENTATION_ITEM('')
SURFACE()
);
#2852=(
BOUNDED_SURFACE()
B_SPLINE_SURFACE(3,2,((#185472,#185473,#185474),(#185475,#185476,#185477),
(#185478,#185479,#185480),(#185481,#185482,#185483),(#185484,#185485,#185486),
(#185487,#185488,#185489),(#185490,#185491,#185492),(#185493,#185494,#185495),
(#185496,#185497,#185498),(#185499,#185500,#185501)),.UNSPECIFIED.,.F.,
 .F.,.F.)
B_SPLINE_SURFACE_WITH_KNOTS((4,2,2,2,4),(3,3),(-0.00010658318899339,0.000906588491342359,
0.00113323561417795,0.00135988273701354,0.00191976017167813),(-0.00126250237001865,
1.),.UNSPECIFIED.)
GEOMETRIC_REPRESENTATION_ITEM()
RATIONAL_B_SPLINE_SURFACE(((1.0007701286604,0.694999122897755,1.),(1.0006124677188,
0.757438982554043,1.),(1.0004932878644,0.804638836285473,1.),(1.00039728502394,
0.842659691824301,1.),(1.00038216130089,0.848649273867104,1.),(1.00035602630873,
0.858999746381121,1.),(1.00034494217433,0.863389494339642,1.),(1.00031477912816,
0.875335232776448,1.),(1.00030645813634,0.878630668891778,1.),(1.00031199678186,
0.876437150031478,1.)))
REPRESENTATION_ITEM('')
SURFACE()
);
#2853=(
BOUNDED_SURFACE()
B_SPLINE_SURFACE(3,2,((#185532,#185533,#185534),(#185535,#185536,#185537),
(#185538,#185539,#185540),(#185541,#185542,#185543),(#185544,#185545,#185546),
(#185547,#185548,#185549),(#185550,#185551,#185552),(#185553,#185554,#185555),
(#185556,#185557,#185558),(#185559,#185560,#185561)),.UNSPECIFIED.,.F.,
 .F.,.F.)
B_SPLINE_SURFACE_WITH_KNOTS((4,2,2,2,4),(3,3),(-1.86157513015761E-16,0.000442340065143073,
0.000884680130286332,0.00132702019542959,0.00176936026057285),(0.,1.),
 .UNSPECIFIED.)
GEOMETRIC_REPRESENTATION_ITEM()
RATIONAL_B_SPLINE_SURFACE(((1.,0.83292929166297,1.),(1.,0.829173169481905,
1.),(1.,0.823008202027213,1.),(1.,0.806154887727085,1.),(1.,0.795326013033949,
1.),(1.,0.768452086196073,1.),(1.,0.752322946736307,1.),(1.,0.713492386952618,
1.),(1.,0.690945244483084,1.),(1.,0.664473794614023,1.)))
REPRESENTATION_ITEM('')
SURFACE()
);
#2854=(
BOUNDED_SURFACE()
B_SPLINE_SURFACE(3,2,((#185616,#185617,#185618),(#185619,#185620,#185621),
(#185622,#185623,#185624),(#185625,#185626,#185627)),.UNSPECIFIED.,.F.,
 .F.,.F.)
B_SPLINE_SURFACE_WITH_KNOTS((4,4),(3,3),(-2.30501381870419E-16,0.000504122926429285),
(0.,1.),.UNSPECIFIED.)
GEOMETRIC_REPRESENTATION_ITEM()
RATIONAL_B_SPLINE_SURFACE(((1.,0.832929291663028,1.),(1.,0.830988393206304,
1.),(1.,0.828976922242354,1.),(1.,0.82689272482991,1.)))
REPRESENTATION_ITEM('')
SURFACE()
);
#2855=(
BOUNDED_SURFACE()
B_SPLINE_SURFACE(3,2,((#185631,#185632,#185633),(#185634,#185635,#185636),
(#185637,#185638,#185639),(#185640,#185641,#185642),(#185643,#185644,#185645),
(#185646,#185647,#185648),(#185649,#185650,#185651),(#185652,#185653,#185654)),
 .UNSPECIFIED.,.F.,.F.,.F.)
B_SPLINE_SURFACE_WITH_KNOTS((4,2,2,4),(3,3),(-0.000157492231769603,0.000393730579424047,
0.000787461158848095,0.00173241454946589),(-0.00194680660466252,1.),
 .UNSPECIFIED.)
GEOMETRIC_REPRESENTATION_ITEM()
RATIONAL_B_SPLINE_SURFACE(((1.00101966603795,0.738118302171479,1.),(1.00090725032211,
0.766990126307879,1.),(1.00082716197042,0.787559285950097,1.),(1.00072872925164,
0.812839845032754,1.),(1.0007006626831,0.820048205758201,1.),(1.00063732175048,
0.836316111484255,1.),(1.00064987188718,0.833092849177034,1.),(1.00069510349992,
0.82147597551466,1.)))
REPRESENTATION_ITEM('')
SURFACE()
);
#2856=(
BOUNDED_SURFACE()
B_SPLINE_SURFACE(3,2,((#185690,#185691,#185692),(#185693,#185694,#185695),
(#185696,#185697,#185698),(#185699,#185700,#185701),(#185702,#185703,#185704),
(#185705,#185706,#185707)),.UNSPECIFIED.,.F.,.F.,.F.)
B_SPLINE_SURFACE_WITH_KNOTS((4,2,4),(3,3),(-0.000159127492400632,0.000795637462001992,
0.00175040241640461),(-0.00149890992630704,1.),.UNSPECIFIED.)
GEOMETRIC_REPRESENTATION_ITEM()
RATIONAL_B_SPLINE_SURFACE(((1.00083523485068,0.721385909846626,1.),(1.00092263143497,
0.692232528860078,1.),(1.00101713444213,0.66070861755133,1.),(1.00114771935088,
0.617148658924304,1.),(1.00118312565315,0.605337975155434,1.),(1.0011655374311,
0.611204979483453,1.)))
REPRESENTATION_ITEM('')
SURFACE()
);
#2857=(
BOUNDED_SURFACE()
B_SPLINE_SURFACE(3,2,((#185736,#185737,#185738),(#185739,#185740,#185741),
(#185742,#185743,#185744),(#185745,#185746,#185747),(#185748,#185749,#185750),
(#185751,#185752,#185753),(#185754,#185755,#185756),(#185757,#185758,#185759),
(#185760,#185761,#185762),(#185763,#185764,#185765)),.UNSPECIFIED.,.F.,
 .F.,.F.)
B_SPLINE_SURFACE_WITH_KNOTS((4,2,2,2,4),(3,3),(-0.000159688588089931,0.000399221470224828,
0.000798442940449655,0.00119766441067448,0.00175657446898924),(0.,1.0022804026225),
 .UNSPECIFIED.)
GEOMETRIC_REPRESENTATION_ITEM()
RATIONAL_B_SPLINE_SURFACE(((1.,0.803619719160217,1.00089565221487),(1.,
0.806811279572102,1.0008810961294),(1.,0.804342659083832,1.00089235502667),
(1.,0.792184442804338,1.00094780628325),(1.,0.784707370490891,1.00098190775387),
(1.,0.766448262692597,1.00106518398849),(1.,0.75551433976755,1.00111505148151),
(1.,0.727335726940382,1.00124356864669),(1.,0.708767918151572,1.00132825280641),
(1.,0.691224111502863,1.00140826669179)))
REPRESENTATION_ITEM('')
SURFACE()
);
#2858=(
BOUNDED_SURFACE()
B_SPLINE_SURFACE(3,2,((#185822,#185823,#185824),(#185825,#185826,#185827),
(#185828,#185829,#185830),(#185831,#185832,#185833),(#185834,#185835,#185836),
(#185837,#185838,#185839),(#185840,#185841,#185842),(#185843,#185844,#185845),
(#185846,#185847,#185848),(#185849,#185850,#185851)),.UNSPECIFIED.,.F.,
 .F.,.F.)
B_SPLINE_SURFACE_WITH_KNOTS((4,2,2,2,4),(3,3),(-4.08272591082004E-15,0.000408890006701704,
0.000817780013407491,0.00122667002011328,0.00163556002681907),(0.,1.),
 .UNSPECIFIED.)
GEOMETRIC_REPRESENTATION_ITEM()
RATIONAL_B_SPLINE_SURFACE(((1.,0.707106781186878,1.),(1.,0.688891921544893,
1.),(1.,0.670532818962991,1.),(1.,0.634368444020432,1.),(1.,0.617287210907485,
1.),(1.,0.586753298958185,1.),(1.,0.573879231151052,1.),(1.,0.555793216592158,
1.),(1.,0.550823008344725,1.),(1.,0.550808342809435,1.)))
REPRESENTATION_ITEM('')
SURFACE()
);
#2859=(
BOUNDED_SURFACE()
B_SPLINE_SURFACE(3,2,((#186037,#186038,#186039),(#186040,#186041,#186042),
(#186043,#186044,#186045),(#186046,#186047,#186048),(#186049,#186050,#186051),
(#186052,#186053,#186054)),.UNSPECIFIED.,.F.,.F.,.F.)
B_SPLINE_SURFACE_WITH_KNOTS((4,2,4),(3,3),(0.0202634924775631,0.0220347355863407,
0.0238059786951184),(0.,1.),.UNSPECIFIED.)
GEOMETRIC_REPRESENTATION_ITEM()
RATIONAL_B_SPLINE_SURFACE(((1.,0.707106781186538,1.),(1.,0.681614664404396,
1.),(1.,0.655059254259685,1.),(1.,0.598852069172831,1.),(1.,0.569209502658738,
1.),(1.,0.537299608347133,1.)))
REPRESENTATION_ITEM('')
SURFACE()
);
#2860=(
BOUNDED_SURFACE()
B_SPLINE_SURFACE(3,2,((#186115,#186116,#186117),(#186118,#186119,#186120),
(#186121,#186122,#186123),(#186124,#186125,#186126),(#186127,#186128,#186129),
(#186130,#186131,#186132),(#186133,#186134,#186135),(#186136,#186137,#186138),
(#186139,#186140,#186141),(#186142,#186143,#186144),(#186145,#186146,#186147),
(#186148,#186149,#186150),(#186151,#186152,#186153),(#186154,#186155,#186156)),
 .UNSPECIFIED.,.F.,.F.,.F.)
B_SPLINE_SURFACE_WITH_KNOTS((4,2,2,2,2,2,4),(3,3),(-9.99593665452691E-5,
0.000249898416362892,0.000374847624544338,0.000499796832725785,0.000624746040907231,
0.000749695249088677,0.00109955303199673),(0.,1.00121399112233),
 .UNSPECIFIED.)
GEOMETRIC_REPRESENTATION_ITEM()
RATIONAL_B_SPLINE_SURFACE(((1.,0.68747168837863,1.00075881319157),(1.,0.683926541024849,
1.0007674207464),(1.,0.682240046418907,1.00077151552536),(1.,0.682757896742324,
1.00077025819397),(1.,0.68316009237754,1.00076928167011),(1.,0.684454083092429,
1.00076613988363),(1.,0.685335934686193,1.00076399876362),(1.,0.687573292179631,
1.00075856649935),(1.,0.688886296979987,1.000755378547),(1.,0.691863134152753,
1.0007481508392),(1.,0.693539259522199,1.00074408123657),(1.,0.700231778213878,
1.00072783192001),(1.,0.706116410220352,1.00071354413798),(1.,0.711375149613269,
1.00070077601211)))
REPRESENTATION_ITEM('')
SURFACE()
);
#2861=(
BOUNDED_SURFACE()
B_SPLINE_SURFACE(3,2,((#186234,#186235,#186236),(#186237,#186238,#186239),
(#186240,#186241,#186242),(#186243,#186244,#186245)),.UNSPECIFIED.,.F.,
 .F.,.F.)
B_SPLINE_SURFACE_WITH_KNOTS((4,4),(3,3),(-6.93889390390723E-18,0.0331958858056162),
(0.,1.),.UNSPECIFIED.)
GEOMETRIC_REPRESENTATION_ITEM()
RATIONAL_B_SPLINE_SURFACE(((1.,0.685275128444715,1.),(1.,0.687584548418076,
1.),(1.,0.689209215689052,1.),(1.,0.690549802660031,1.)))
REPRESENTATION_ITEM('')
SURFACE()
);
#2862=(
BOUNDED_SURFACE()
B_SPLINE_SURFACE(3,2,((#186258,#186259,#186260),(#186261,#186262,#186263),
(#186264,#186265,#186266),(#186267,#186268,#186269)),.UNSPECIFIED.,.F.,
 .F.,.F.)
B_SPLINE_SURFACE_WITH_KNOTS((4,4),(3,3),(0.,0.000650162698700256),(0.,1.),
 .UNSPECIFIED.)
GEOMETRIC_REPRESENTATION_ITEM()
RATIONAL_B_SPLINE_SURFACE(((1.,0.690549802660026,1.),(1.,0.689437188232559,
1.),(1.,0.688863085247593,1.),(1.,0.688859710772113,1.)))
REPRESENTATION_ITEM('')
SURFACE()
);
#2863=(
BOUNDED_SURFACE()
B_SPLINE_SURFACE(3,2,((#186361,#186362,#186363),(#186364,#186365,#186366),
(#186367,#186368,#186369),(#186370,#186371,#186372),(#186373,#186374,#186375),
(#186376,#186377,#186378)),.UNSPECIFIED.,.F.,.F.,.F.)
B_SPLINE_SURFACE_WITH_KNOTS((4,2,4),(3,3),(0.,0.785398163397448,1.5707963267949),
(0.,1.),.UNSPECIFIED.)
GEOMETRIC_REPRESENTATION_ITEM()
RATIONAL_B_SPLINE_SURFACE(((1.,0.675590207615664,1.),(1.,0.675526278181762,
1.),(1.,0.679082711196844,1.),(1.,0.690860049128418,1.),(1.,0.699025295935035,
1.),(1.,0.707106781186543,1.)))
REPRESENTATION_ITEM('')
SURFACE()
);
#2864=(
BOUNDED_SURFACE()
B_SPLINE_SURFACE(3,2,((#186392,#186393,#186394),(#186395,#186396,#186397),
(#186398,#186399,#186400),(#186401,#186402,#186403),(#186404,#186405,#186406),
(#186407,#186408,#186409)),.UNSPECIFIED.,.F.,.F.,.F.)
B_SPLINE_SURFACE_WITH_KNOTS((4,2,4),(3,3),(1.5707963267949,2.35619449019234,
3.1415926535898),(0.,1.),.UNSPECIFIED.)
GEOMETRIC_REPRESENTATION_ITEM()
RATIONAL_B_SPLINE_SURFACE(((1.,0.707106781186543,1.),(1.,0.715202981902222,
1.),(1.,0.723033691557528,1.),(1.,0.73410625828684,1.),(1.,0.737326538316928,
1.),(1.,0.737277336810125,1.)))
REPRESENTATION_ITEM('')
SURFACE()
);
#2865=(
BOUNDED_SURFACE()
B_SPLINE_SURFACE(3,2,((#186427,#186428,#186429),(#186430,#186431,#186432),
(#186433,#186434,#186435),(#186436,#186437,#186438),(#186439,#186440,#186441),
(#186442,#186443,#186444)),.UNSPECIFIED.,.F.,.F.,.F.)
B_SPLINE_SURFACE_WITH_KNOTS((4,2,4),(3,3),(0.,0.785398163397448,1.5707963267949),
(0.,1.),.UNSPECIFIED.)
GEOMETRIC_REPRESENTATION_ITEM()
RATIONAL_B_SPLINE_SURFACE(((1.,0.675590207615664,1.),(1.,0.675526278181461,
1.),(1.,0.679082711197251,1.),(1.,0.690860049128011,1.),(1.,0.699025295935341,
1.),(1.,0.707106781186543,1.)))
REPRESENTATION_ITEM('')
SURFACE()
);
#2866=(
BOUNDED_SURFACE()
B_SPLINE_SURFACE(3,2,((#186458,#186459,#186460),(#186461,#186462,#186463),
(#186464,#186465,#186466),(#186467,#186468,#186469),(#186470,#186471,#186472),
(#186473,#186474,#186475)),.UNSPECIFIED.,.F.,.F.,.F.)
B_SPLINE_SURFACE_WITH_KNOTS((4,2,4),(3,3),(4.71238898038469,5.49778714378214,
6.28318530717959),(0.,1.),.UNSPECIFIED.)
GEOMETRIC_REPRESENTATION_ITEM()
RATIONAL_B_SPLINE_SURFACE(((1.,0.707106781186538,1.),(1.,0.715202981902668,
1.),(1.,0.723033691556936,1.),(1.,0.734106258287417,1.),(1.,0.737326538316498,
1.),(1.,0.737277336810125,1.)))
REPRESENTATION_ITEM('')
SURFACE()
);
#2867=(
BOUNDED_SURFACE()
B_SPLINE_SURFACE(3,2,((#186491,#186492,#186493),(#186494,#186495,#186496),
(#186497,#186498,#186499),(#186500,#186501,#186502)),.UNSPECIFIED.,.F.,
 .F.,.F.)
B_SPLINE_SURFACE_WITH_KNOTS((4,4),(3,3),(2.22847122787663,3.14161440295379),
(0.,1.000021749364),.UNSPECIFIED.)
GEOMETRIC_REPRESENTATION_ITEM()
RATIONAL_B_SPLINE_SURFACE(((1.,0.725692460307628,1.00001193202905),(1.,
0.732974645844472,1.00001161526325),(1.,0.737323110435418,1.00001142611057),
(1.,0.737271619087494,1.00001142835038)))
REPRESENTATION_ITEM('')
SURFACE()
);
#2868=(
BOUNDED_SURFACE()
B_SPLINE_SURFACE(3,2,((#186510,#186511,#186512),(#186513,#186514,#186515),
(#186516,#186517,#186518),(#186519,#186520,#186521),(#186522,#186523,#186524),
(#186525,#186526,#186527)),.UNSPECIFIED.,.F.,.F.,.F.)
B_SPLINE_SURFACE_WITH_KNOTS((4,2,4),(3,3),(9.63948754967748E-5,0.00173129457116097,
0.00336619426682516),(0.,1.),.UNSPECIFIED.)
GEOMETRIC_REPRESENTATION_ITEM()
RATIONAL_B_SPLINE_SURFACE(((1.,0.88872394157032,1.),(1.,0.863203710383462,
1.),(1.,0.835728844788038,1.),(1.,0.775725241916869,1.),(1.,0.743211702946043,
1.),(1.,0.707106781186548,1.)))
REPRESENTATION_ITEM('')
SURFACE()
);
#2869=(
BOUNDED_SURFACE()
B_SPLINE_SURFACE(3,2,((#186551,#186552,#186553),(#186554,#186555,#186556),
(#186557,#186558,#186559),(#186560,#186561,#186562),(#186563,#186564,#186565),
(#186566,#186567,#186568)),.UNSPECIFIED.,.F.,.F.,.F.)
B_SPLINE_SURFACE_WITH_KNOTS((4,2,4),(3,3),(3.1415926535898,3.92699081698724,
4.71238898038469),(0.,1.),.UNSPECIFIED.)
GEOMETRIC_REPRESENTATION_ITEM()
RATIONAL_B_SPLINE_SURFACE(((1.,0.737277336810123,1.),(1.,0.737326538316937,
1.),(1.,0.73410625828684,1.),(1.,0.723033691557529,1.),(1.,0.715202981902217,
1.),(1.,0.707106781186543,1.)))
REPRESENTATION_ITEM('')
SURFACE()
);
#2870=(
BOUNDED_SURFACE()
B_SPLINE_SURFACE(3,2,((#186582,#186583,#186584),(#186585,#186586,#186587),
(#186588,#186589,#186590),(#186591,#186592,#186593),(#186594,#186595,#186596),
(#186597,#186598,#186599)),.UNSPECIFIED.,.F.,.F.,.F.)
B_SPLINE_SURFACE_WITH_KNOTS((4,2,4),(3,3),(4.71234651107924,5.49778714378214,
6.28322777648504),(-4.24693054514115E-5,1.),.UNSPECIFIED.)
GEOMETRIC_REPRESENTATION_ITEM()
RATIONAL_B_SPLINE_SURFACE(((1.00002487888834,0.707095653254892,1.),(1.00002556538397,
0.699013396841122,1.),(1.00002625900611,0.690847238604463,1.),(1.00002725945341,
0.679068763627425,1.),(1.00002756155034,0.675512113380383,1.),(1.00002755608648,
0.675576440559981,1.)))
REPRESENTATION_ITEM('')
SURFACE()
);
#2871=(
BOUNDED_SURFACE()
B_SPLINE_SURFACE(3,2,((#186615,#186616,#186617),(#186618,#186619,#186620),
(#186621,#186622,#186623),(#186624,#186625,#186626),(#186627,#186628,#186629),
(#186630,#186631,#186632)),.UNSPECIFIED.,.F.,.F.,.F.)
B_SPLINE_SURFACE_WITH_KNOTS((4,2,4),(3,3),(0.,0.00168309713341273,0.00336619426682545),
(0.,1.),.UNSPECIFIED.)
GEOMETRIC_REPRESENTATION_ITEM()
RATIONAL_B_SPLINE_SURFACE(((1.,0.707106781186545,1.),(1.,0.744273762477552,
1.),(1.,0.7776417896067,1.),(1.,0.83910580954319,1.),(1.,0.867185102973278,
1.),(1.,0.89321434471954,1.)))
REPRESENTATION_ITEM('')
SURFACE()
);
#2872=(
BOUNDED_SURFACE()
B_SPLINE_SURFACE(3,2,((#186656,#186657,#186658),(#186659,#186660,#186661),
(#186662,#186663,#186664),(#186665,#186666,#186667)),.UNSPECIFIED.,.F.,
 .F.,.F.)
B_SPLINE_SURFACE_WITH_KNOTS((4,4),(3,3),(3.1415926535898,3.72189740710945),
(0.,1.),.UNSPECIFIED.)
GEOMETRIC_REPRESENTATION_ITEM()
RATIONAL_B_SPLINE_SURFACE(((1.,0.737277336810124,1.),(1.,0.737285953283754,
1.),(1.,0.735586930398308,1.),(1.,0.732423362569238,1.)))
REPRESENTATION_ITEM('')
SURFACE()
);
#2873=(
BOUNDED_SURFACE()
B_SPLINE_SURFACE(3,2,((#186679,#186680,#186681),(#186682,#186683,#186684),
(#186685,#186686,#186687),(#186688,#186689,#186690),(#186691,#186692,#186693),
(#186694,#186695,#186696)),.UNSPECIFIED.,.F.,.F.,.F.)
B_SPLINE_SURFACE_WITH_KNOTS((4,2,4),(3,3),(0.,0.785398163397448,1.5707963267949),
(0.,1.),.UNSPECIFIED.)
GEOMETRIC_REPRESENTATION_ITEM()
RATIONAL_B_SPLINE_SURFACE(((1.,0.737277336810127,1.),(1.,0.737326538316762,
1.),(1.,0.734106258287074,1.),(1.,0.723033691557295,1.),(1.,0.715202981902387,
1.),(1.,0.707106781186548,1.)))
REPRESENTATION_ITEM('')
SURFACE()
);
#2874=(
BOUNDED_SURFACE()
B_SPLINE_SURFACE(3,2,((#186710,#186711,#186712),(#186713,#186714,#186715),
(#186716,#186717,#186718),(#186719,#186720,#186721),(#186722,#186723,#186724),
(#186725,#186726,#186727)),.UNSPECIFIED.,.F.,.F.,.F.)
B_SPLINE_SURFACE_WITH_KNOTS((4,2,4),(3,3),(4.7123465110751,5.49778714378214,
6.28322777648918),(-4.24693095901446E-5,1.),.UNSPECIFIED.)
GEOMETRIC_REPRESENTATION_ITEM()
RATIONAL_B_SPLINE_SURFACE(((1.00002487889076,0.707095653253807,0.999999999999999),
(1.00002556538646,0.69901339684015,1.),(1.00002625900867,0.690847238602975,
1.),(1.00002725945607,0.679068763626294,1.),(1.00002756155303,0.675512113378835,
1.),(1.00002755608917,0.675576440558639,0.999999999999999)))
REPRESENTATION_ITEM('')
SURFACE()
);
#2875=(
BOUNDED_SURFACE()
B_SPLINE_SURFACE(3,2,((#186751,#186752,#186753),(#186754,#186755,#186756),
(#186757,#186758,#186759),(#186760,#186761,#186762),(#186763,#186764,#186765),
(#186766,#186767,#186768)),.UNSPECIFIED.,.F.,.F.,.F.)
B_SPLINE_SURFACE_WITH_KNOTS((4,2,4),(3,3),(3.1415926535898,3.92699081698724,
4.71238898038469),(0.,1.),.UNSPECIFIED.)
GEOMETRIC_REPRESENTATION_ITEM()
RATIONAL_B_SPLINE_SURFACE(((1.,0.675590207615659,1.),(1.,0.675526278181249,
1.),(1.,0.679082711197525,1.),(1.,0.69086004912773,1.),(1.,0.699025295935556,
1.),(1.,0.707106781186543,1.)))
REPRESENTATION_ITEM('')
SURFACE()
);
#2876=(
BOUNDED_SURFACE()
B_SPLINE_SURFACE(3,2,((#186782,#186783,#186784),(#186785,#186786,#186787),
(#186788,#186789,#186790),(#186791,#186792,#186793),(#186794,#186795,#186796),
(#186797,#186798,#186799)),.UNSPECIFIED.,.F.,.F.,.F.)
B_SPLINE_SURFACE_WITH_KNOTS((4,2,4),(3,3),(1.5707963267949,2.35619449019234,
3.1415926535898),(0.,1.),.UNSPECIFIED.)
GEOMETRIC_REPRESENTATION_ITEM()
RATIONAL_B_SPLINE_SURFACE(((1.,0.707106781186543,1.),(1.,0.71520298190223,
1.),(1.,0.723033691557516,1.),(1.,0.734106258286857,1.),(1.,0.737326538316932,
1.),(1.,0.737277336810125,1.)))
REPRESENTATION_ITEM('')
SURFACE()
);
#2877=(
BOUNDED_SURFACE()
B_SPLINE_SURFACE(3,2,((#186815,#186816,#186817),(#186818,#186819,#186820),
(#186821,#186822,#186823),(#186824,#186825,#186826),(#186827,#186828,#186829),
(#186830,#186831,#186832)),.UNSPECIFIED.,.F.,.F.,.F.)
B_SPLINE_SURFACE_WITH_KNOTS((4,2,4),(3,3),(0.,0.00162565899344706,0.00325131798689413),
(0.,1.),.UNSPECIFIED.)
GEOMETRIC_REPRESENTATION_ITEM()
RATIONAL_B_SPLINE_SURFACE(((1.,0.893214344719539,1.),(1.,0.868075018581634,
1.),(1.,0.841018189595232,1.),(1.,0.782003386508022,1.),(1.,0.750058517040659,
1.),(1.,0.714668958264373,1.)))
REPRESENTATION_ITEM('')
SURFACE()
);
#2878=(
BOUNDED_SURFACE()
B_SPLINE_SURFACE(3,2,((#186855,#186856,#186857),(#186858,#186859,#186860),
(#186861,#186862,#186863),(#186864,#186865,#186866),(#186867,#186868,#186869),
(#186870,#186871,#186872)),.UNSPECIFIED.,.F.,.F.,.F.)
B_SPLINE_SURFACE_WITH_KNOTS((4,2,4),(3,3),(3.1415926535898,3.92699081698724,
4.71238898038469),(0.,1.),.UNSPECIFIED.)
GEOMETRIC_REPRESENTATION_ITEM()
RATIONAL_B_SPLINE_SURFACE(((1.,0.675590207615659,1.),(1.,0.675526278181242,
1.),(1.,0.679082711197541,1.),(1.,0.690860049127717,1.),(1.,0.699025295935567,
1.),(1.,0.707106781186543,1.)))
REPRESENTATION_ITEM('')
SURFACE()
);
#2879=(
BOUNDED_SURFACE()
B_SPLINE_SURFACE(3,2,((#186886,#186887,#186888),(#186889,#186890,#186891),
(#186892,#186893,#186894),(#186895,#186896,#186897),(#186898,#186899,#186900),
(#186901,#186902,#186903)),.UNSPECIFIED.,.F.,.F.,.F.)
B_SPLINE_SURFACE_WITH_KNOTS((4,2,4),(3,3),(4.71238898038469,5.49778714378214,
6.28318530717959),(0.,1.),.UNSPECIFIED.)
GEOMETRIC_REPRESENTATION_ITEM()
RATIONAL_B_SPLINE_SURFACE(((1.,0.707106781186543,1.),(1.,0.715202981902221,
1.),(1.,0.723033691557525,1.),(1.,0.734106258286841,1.),(1.,0.737326538316939,
1.),(1.,0.737277336810125,1.)))
REPRESENTATION_ITEM('')
SURFACE()
);
#2880=(
BOUNDED_SURFACE()
B_SPLINE_SURFACE(3,2,((#186917,#186918,#186919),(#186920,#186921,#186922),
(#186923,#186924,#186925),(#186926,#186927,#186928),(#186929,#186930,#186931),
(#186932,#186933,#186934)),.UNSPECIFIED.,.F.,.F.,.F.)
B_SPLINE_SURFACE_WITH_KNOTS((4,2,4),(3,3),(-3.25260651745651E-18,0.00101351621082632,
0.00202703242165263),(0.,1.),.UNSPECIFIED.)
GEOMETRIC_REPRESENTATION_ITEM()
RATIONAL_B_SPLINE_SURFACE(((1.,0.893214344719542,1.),(1.,0.912305000874927,
1.),(1.,0.927255525935639,1.),(1.,0.94789383214718,1.),(1.,0.953590869545161,
1.),(1.,0.953555223991885,1.)))
REPRESENTATION_ITEM('')
SURFACE()
);
#2881=(
BOUNDED_SURFACE()
B_SPLINE_SURFACE(3,2,((#187005,#187006,#187007),(#187008,#187009,#187010),
(#187011,#187012,#187013),(#187014,#187015,#187016),(#187017,#187018,#187019),
(#187020,#187021,#187022)),.UNSPECIFIED.,.F.,.F.,.F.)
B_SPLINE_SURFACE_WITH_KNOTS((4,2,4),(3,3),(3.1415926535898,3.92699081698724,
4.71238898038469),(0.,1.),.UNSPECIFIED.)
GEOMETRIC_REPRESENTATION_ITEM()
RATIONAL_B_SPLINE_SURFACE(((1.,0.73727733681012,1.),(1.,0.737326538316634,
1.),(1.,0.734106258287243,1.),(1.,0.723033691557116,1.),(1.,0.715202981902516,
1.),(1.,0.707106781186548,1.)))
REPRESENTATION_ITEM('')
SURFACE()
);
#2882=(
BOUNDED_SURFACE()
B_SPLINE_SURFACE(3,2,((#187036,#187037,#187038),(#187039,#187040,#187041),
(#187042,#187043,#187044),(#187045,#187046,#187047),(#187048,#187049,#187050),
(#187051,#187052,#187053)),.UNSPECIFIED.,.F.,.F.,.F.)
B_SPLINE_SURFACE_WITH_KNOTS((4,2,4),(3,3),(4.71234651106924,5.49778714378214,
6.28322777649504),(-4.24693154496904E-5,1.),.UNSPECIFIED.)
GEOMETRIC_REPRESENTATION_ITEM()
RATIONAL_B_SPLINE_SURFACE(((1.0000248788942,0.707095653252277,1.),(1.00002556538999,
0.699013396839213,1.),(1.00002625901229,0.690847238600254,1.),(1.00002725945983,
0.679068763625337,1.),(1.00002756155683,0.675512113376159,1.),(1.00002755609297,
0.675576440556743,1.)))
REPRESENTATION_ITEM('')
SURFACE()
);
#2883=(
BOUNDED_SURFACE()
B_SPLINE_SURFACE(3,2,((#187069,#187070,#187071),(#187072,#187073,#187074),
(#187075,#187076,#187077),(#187078,#187079,#187080),(#187081,#187082,#187083),
(#187084,#187085,#187086)),.UNSPECIFIED.,.F.,.F.,.F.)
B_SPLINE_SURFACE_WITH_KNOTS((4,2,4),(3,3),(0.,0.00169934430350512,0.00339868860701024),
(0.,1.),.UNSPECIFIED.)
GEOMETRIC_REPRESENTATION_ITEM()
RATIONAL_B_SPLINE_SURFACE(((1.,0.707106781186547,1.),(1.,0.74482559038907,
1.),(1.,0.778551967557851,1.),(1.,0.840511428018892,1.),(1.,0.868726285027217,
1.),(1.,0.894799245647903,1.)))
REPRESENTATION_ITEM('')
SURFACE()
);
#2884=(
BOUNDED_SURFACE()
B_SPLINE_SURFACE(3,2,((#187110,#187111,#187112),(#187113,#187114,#187115),
(#187116,#187117,#187118),(#187119,#187120,#187121),(#187122,#187123,#187124),
(#187125,#187126,#187127)),.UNSPECIFIED.,.F.,.F.,.F.)
B_SPLINE_SURFACE_WITH_KNOTS((4,2,4),(3,3),(3.1415926535898,3.72828696246945,
4.31498127134909),(0.,1.),.UNSPECIFIED.)
GEOMETRIC_REPRESENTATION_ITEM()
RATIONAL_B_SPLINE_SURFACE(((1.,0.737277336810115,1.),(1.,0.73729299178243,
1.),(1.,0.735539930277599,1.),(1.,0.729097328045697,1.),(1.,0.724411344440144,
1.),(1.,0.71893387489533,1.)))
REPRESENTATION_ITEM('')
SURFACE()
);
#2885=(
BOUNDED_SURFACE()
B_SPLINE_SURFACE(3,2,((#187175,#187176,#187177),(#187178,#187179,#187180),
(#187181,#187182,#187183),(#187184,#187185,#187186),(#187187,#187188,#187189),
(#187190,#187191,#187192)),.UNSPECIFIED.,.F.,.F.,.F.)
B_SPLINE_SURFACE_WITH_KNOTS((4,2,4),(3,3),(1.41124413247309E-15,0.78539816339745,
1.5707963267949),(0.,1.),.UNSPECIFIED.)
GEOMETRIC_REPRESENTATION_ITEM()
RATIONAL_B_SPLINE_SURFACE(((1.,0.73727733681012,1.),(1.,0.737326538316275,
1.),(1.,0.734106258287724,1.),(1.,0.723033691556635,1.),(1.,0.715202981902879,
1.),(1.,0.707106781186548,1.)))
REPRESENTATION_ITEM('')
SURFACE()
);
#2886=(
BOUNDED_SURFACE()
B_SPLINE_SURFACE(3,2,((#187206,#187207,#187208),(#187209,#187210,#187211),
(#187212,#187213,#187214),(#187215,#187216,#187217),(#187218,#187219,#187220),
(#187221,#187222,#187223)),.UNSPECIFIED.,.F.,.F.,.F.)
B_SPLINE_SURFACE_WITH_KNOTS((4,2,4),(3,3),(4.71234651107879,5.49778714378214,
6.28322777648549),(-4.24693058989126E-5,1.),.UNSPECIFIED.)
GEOMETRIC_REPRESENTATION_ITEM()
RATIONAL_B_SPLINE_SURFACE(((1.0000248788886,0.70709565325478,1.),(1.00002556538424,
0.699013396841888,1.),(1.00002625900639,0.690847238603135,1.),(1.0000272594537,
0.679068763628474,1.),(1.00002756155063,0.675512113379344,1.),(1.00002755608677,
0.675576440559839,1.)))
REPRESENTATION_ITEM('')
SURFACE()
);
#2887=(
BOUNDED_SURFACE()
B_SPLINE_SURFACE(3,2,((#187237,#187238,#187239),(#187240,#187241,#187242),
(#187243,#187244,#187245),(#187246,#187247,#187248),(#187249,#187250,#187251),
(#187252,#187253,#187254),(#187255,#187256,#187257),(#187258,#187259,#187260)),
 .UNSPECIFIED.,.F.,.F.,.F.)
B_SPLINE_SURFACE_WITH_KNOTS((4,2,2,4),(3,3),(-3.14418630020796E-18,0.000761037462531171,
0.00114155619379676,0.00152207492506235),(0.,1.),.UNSPECIFIED.)
GEOMETRIC_REPRESENTATION_ITEM()
RATIONAL_B_SPLINE_SURFACE(((1.,0.691935594449023,1.),(1.,0.657938057153071,
1.),(1.,0.623321566128117,1.),(1.,0.582569634693765,1.),(1.,0.571407182182735,
1.),(1.,0.5555307216223,1.),(1.,0.551373498869702,1.),(1.,0.551334230064852,
1.)))
REPRESENTATION_ITEM('')
SURFACE()
);
#2888=(
BOUNDED_SURFACE()
B_SPLINE_SURFACE(3,2,((#187340,#187341,#187342),(#187343,#187344,#187345),
(#187346,#187347,#187348),(#187349,#187350,#187351),(#187352,#187353,#187354),
(#187355,#187356,#187357),(#187358,#187359,#187360),(#187361,#187362,#187363),
(#187364,#187365,#187366),(#187367,#187368,#187369)),.UNSPECIFIED.,.F.,
 .F.,.F.)
B_SPLINE_SURFACE_WITH_KNOTS((4,2,2,2,4),(3,3),(-0.000159653390897044,0.000399133477242608,
0.000798266954485216,0.00119740043172782,0.00175618729986758),(-0.00202899497456342,
1.),.UNSPECIFIED.)
GEOMETRIC_REPRESENTATION_ITEM()
RATIONAL_B_SPLINE_SURFACE(((1.00079837996119,0.803257284714785,1.),(1.00078548688006,
0.806434493454874,1.),(1.00079545917955,0.803977045403331,1.),(1.00084458507115,
0.791871078604599,1.),(1.00087479655517,0.784426140493272,1.),(1.00094857178652,
0.766245900455217,1.),(1.00099274968817,0.755359254060113,1.),(1.00110658067738,
0.727308176893173,1.),(1.00118157563583,0.70882736264828,1.),(1.0012523988413,
0.691374582737139,1.)))
REPRESENTATION_ITEM('')
SURFACE()
);
#2889=(
BOUNDED_SURFACE()
B_SPLINE_SURFACE(3,2,((#187419,#187420,#187421),(#187422,#187423,#187424),
(#187425,#187426,#187427),(#187428,#187429,#187430),(#187431,#187432,#187433),
(#187434,#187435,#187436)),.UNSPECIFIED.,.F.,.F.,.F.)
B_SPLINE_SURFACE_WITH_KNOTS((4,2,4),(3,3),(-0.000140547083940185,0.000795474163050539,
0.00173149541004126),(-0.000140547083940185,1.00127446610899),
 .UNSPECIFIED.)
GEOMETRIC_REPRESENTATION_ITEM()
RATIONAL_B_SPLINE_SURFACE(((1.00007870553575,0.719646060326318,1.00071450264019),
(1.00008671779993,0.691105884499127,1.00078723937792),(1.00009529453502,
0.660555028733005,1.00086510048138),(1.00010720671514,0.618123113407254,
1.0009732413392),(1.0001104843585,0.606447946977011,1.00100299635976),(1.00010906895813,
0.611489689798581,1.00099014710727)))
REPRESENTATION_ITEM('')
SURFACE()
);
#2890=(
BOUNDED_SURFACE()
B_SPLINE_SURFACE(3,2,((#187466,#187467,#187468),(#187469,#187470,#187471),
(#187472,#187473,#187474),(#187475,#187476,#187477),(#187478,#187479,#187480),
(#187481,#187482,#187483),(#187484,#187485,#187486),(#187487,#187488,#187489)),
 .UNSPECIFIED.,.F.,.F.,.F.)
B_SPLINE_SURFACE_WITH_KNOTS((4,2,2,4),(3,3),(-0.000157666505658259,0.000394166264145648,
0.000788332528291295,0.00173433156224098),(-0.00241203109543842,1.00210445955167),
 .UNSPECIFIED.)
GEOMETRIC_REPRESENTATION_ITEM()
RATIONAL_B_SPLINE_SURFACE(((1.00126783966346,0.736629804805208,1.00110583094575),
(1.00112683188768,0.765921557145529,1.00098284160685),(1.00102615333431,
0.786835660891743,1.0008950280898),(1.00090176020874,0.812676027545364,
1.00078653032651),(1.00086612520509,0.820078539185068,1.00075544888071),
(1.00078492300801,0.836946790835935,1.00068462296716),(1.00079943453383,
0.833932290266678,1.00069728016253),(1.00085506469522,0.822376155144815,
1.00074580171913)))
REPRESENTATION_ITEM('')
SURFACE()
);
#2891=(
BOUNDED_SURFACE()
B_SPLINE_SURFACE(3,2,((#187520,#187521,#187522),(#187523,#187524,#187525),
(#187526,#187527,#187528),(#187529,#187530,#187531)),.UNSPECIFIED.,.F.,
 .F.,.F.)
B_SPLINE_SURFACE_WITH_KNOTS((4,4),(3,3),(0.,0.000504125640440226),(0.,1.),
 .UNSPECIFIED.)
GEOMETRIC_REPRESENTATION_ITEM()
RATIONAL_B_SPLINE_SURFACE(((1.,0.828190603154496,1.),(1.,0.830246482056442,
1.),(1.,0.832229943187683,1.),(1.,0.834143101464675,1.)))
REPRESENTATION_ITEM('')
SURFACE()
);
#2892=(
BOUNDED_SURFACE()
B_SPLINE_SURFACE(3,2,((#187535,#187536,#187537),(#187538,#187539,#187540),
(#187541,#187542,#187543),(#187544,#187545,#187546),(#187547,#187548,#187549),
(#187550,#187551,#187552),(#187553,#187554,#187555),(#187556,#187557,#187558),
(#187559,#187560,#187561),(#187562,#187563,#187564)),.UNSPECIFIED.,.F.,
 .F.,.F.)
B_SPLINE_SURFACE_WITH_KNOTS((4,2,2,2,4),(3,3),(-8.34022521184474E-16,0.000443043867974425,
0.000886087735949684,0.00132913160392494,0.00177217547190021),(0.,1.),
 .UNSPECIFIED.)
GEOMETRIC_REPRESENTATION_ITEM()
RATIONAL_B_SPLINE_SURFACE(((1.,0.834143101464621,1.),(1.,0.830444108750761,
1.),(1.,0.824302497883951,1.),(1.,0.80744078994961,1.),(1.,0.79657978834944,
1.),(1.,0.769588124839812,1.),(1.,0.753384767045469,1.),(1.,0.714346006222175,
1.),(1.,0.691706791956038,1.),(1.,0.665108204576645,1.)))
REPRESENTATION_ITEM('')
SURFACE()
);
#2893=(
BOUNDED_SURFACE()
B_SPLINE_SURFACE(3,2,((#187627,#187628,#187629),(#187630,#187631,#187632),
(#187633,#187634,#187635),(#187636,#187637,#187638),(#187639,#187640,#187641),
(#187642,#187643,#187644),(#187645,#187646,#187647),(#187648,#187649,#187650),
(#187651,#187652,#187653),(#187654,#187655,#187656)),.UNSPECIFIED.,.F.,
 .F.,.F.)
B_SPLINE_SURFACE_WITH_KNOTS((4,2,2,2,4),(3,3),(-0.000173686186586184,0.000907880296577857,
0.00113485037072232,0.00136182044486679,0.00198944677974189),(0.,1.00144242662926),
 .UNSPECIFIED.)
GEOMETRIC_REPRESENTATION_ITEM()
RATIONAL_B_SPLINE_SURFACE(((1.,0.681665301346584,1.00091834889271),(1.,
0.750503632449571,1.00071976040892),(1.,0.8021030753377,1.00057090358796),
(1.,0.842357054042358,1.00045477676633),(1.,0.848376815809341,1.00043741063698),
(1.,0.858788711892737,1.00040737384464),(1.,0.863209133647019,1.00039462157653),
(1.,0.876279812131844,1.00035691458712),(1.,0.879347925892028,1.00034806352914),
(1.,0.875471233314833,1.00035924721835)))
REPRESENTATION_ITEM('')
SURFACE()
);
#2894=(
BOUNDED_SURFACE()
B_SPLINE_SURFACE(3,2,((#187676,#187677,#187678),(#187679,#187680,#187681),
(#187682,#187683,#187684),(#187685,#187686,#187687)),.UNSPECIFIED.,.F.,
 .F.,.F.)
B_SPLINE_SURFACE_WITH_KNOTS((4,4),(3,3),(0.,0.000503779257761556),(0.,1.),
 .UNSPECIFIED.)
GEOMETRIC_REPRESENTATION_ITEM()
RATIONAL_B_SPLINE_SURFACE(((1.,0.877279917170998,1.),(1.,0.877311423474942,
1.),(1.,0.87728564981134,1.),(1.,0.877202574460556,1.)))
REPRESENTATION_ITEM('')
SURFACE()
);
#2895=(
BOUNDED_SURFACE()
B_SPLINE_SURFACE(3,2,((#187691,#187692,#187693),(#187694,#187695,#187696),
(#187697,#187698,#187699),(#187700,#187701,#187702),(#187703,#187704,#187705),
(#187706,#187707,#187708),(#187709,#187710,#187711),(#187712,#187713,#187714),
(#187715,#187716,#187717),(#187718,#187719,#187720)),.UNSPECIFIED.,.F.,
 .F.,.F.)
B_SPLINE_SURFACE_WITH_KNOTS((4,2,2,2,4),(3,3),(-0.000115990203183372,0.000453061765036137,
0.000906123530072295,0.00135918529510845,0.00192823726332794),(0.,1.00079444254916),
 .UNSPECIFIED.)
GEOMETRIC_REPRESENTATION_ITEM()
RATIONAL_B_SPLINE_SURFACE(((1.,0.876263374194623,1.00019660328086),(1.,
0.878805941473907,1.0001925634336),(1.,0.875602380876755,1.00019765352329),
(1.,0.86018205071516,1.0002221546561),(1.,0.849863211484357,1.00023855010598),
(1.,0.822219823797783,1.00028247227274),(1.,0.805074602369326,1.00030971405958),
(1.,0.759404065674411,1.00038227929477),(1.,0.729387016381409,1.00042997293708),
(1.,0.694075111441602,1.00048607949663)))
REPRESENTATION_ITEM('')
SURFACE()
);
#2896=(
BOUNDED_SURFACE()
B_SPLINE_SURFACE(3,2,((#187753,#187754,#187755),(#187756,#187757,#187758),
(#187759,#187760,#187761),(#187762,#187763,#187764),(#187765,#187766,#187767),
(#187768,#187769,#187770),(#187771,#187772,#187773),(#187774,#187775,#187776),
(#187777,#187778,#187779),(#187780,#187781,#187782),(#187783,#187784,#187785),
(#187786,#187787,#187788)),.UNSPECIFIED.,.F.,.F.,.F.)
B_SPLINE_SURFACE_WITH_KNOTS((4,2,2,2,2,4),(3,3),(0.,0.000440377446917856,
0.000880754893835713,0.00110094361729464,0.00132113234075357,0.00176150978767142),
(0.,1.),.UNSPECIFIED.)
GEOMETRIC_REPRESENTATION_ITEM()
RATIONAL_B_SPLINE_SURFACE(((1.,0.663670476503535,1.),(1.,0.690166095882704,
1.),(1.,0.712198476344476,1.),(1.,0.750819491395322,1.),(1.,0.766789812455876,
1.),(1.,0.786909315979615,1.),(1.,0.793060196071366,1.),(1.,0.803891824235189,
1.),(1.,0.808661939460988,1.),(1.,0.821430084171777,1.),(1.,0.827612685850937,
1.),(1.,0.831517473467322,1.)))
REPRESENTATION_ITEM('')
SURFACE()
);
#2897=(
BOUNDED_SURFACE()
B_SPLINE_SURFACE(3,2,((#187834,#187835,#187836),(#187837,#187838,#187839),
(#187840,#187841,#187842),(#187843,#187844,#187845)),.UNSPECIFIED.,.F.,
 .F.,.F.)
B_SPLINE_SURFACE_WITH_KNOTS((4,4),(3,3),(-2.62810606610486E-16,0.000504136652582459),
(0.,1.),.UNSPECIFIED.)
GEOMETRIC_REPRESENTATION_ITEM()
RATIONAL_B_SPLINE_SURFACE(((1.,0.831517473467334,1.),(1.,0.829540548856785,
1.),(1.,0.827492428459287,1.),(1.,0.825370895892945,1.)))
REPRESENTATION_ITEM('')
SURFACE()
);
#2898=(
BOUNDED_SURFACE()
B_SPLINE_SURFACE(3,2,((#187849,#187850,#187851),(#187852,#187853,#187854),
(#187855,#187856,#187857),(#187858,#187859,#187860),(#187861,#187862,#187863),
(#187864,#187865,#187866),(#187867,#187868,#187869),(#187870,#187871,#187872),
(#187873,#187874,#187875),(#187876,#187877,#187878)),.UNSPECIFIED.,.F.,
 .F.,.F.)
B_SPLINE_SURFACE_WITH_KNOTS((4,2,2,2,4),(3,3),(0.,0.00039329942356206,0.000786598847124121,
0.00117989827068618,0.00157319769424824),(0.,1.),.UNSPECIFIED.)
GEOMETRIC_REPRESENTATION_ITEM()
RATIONAL_B_SPLINE_SURFACE(((1.,0.825370895892916,1.),(1.,0.829081051796028,
1.),(1.,0.831084991111337,1.),(1.,0.831059675364535,1.),(1.,0.829021889329635,
1.),(1.,0.819977402296451,1.),(1.,0.812885056457023,1.),(1.,0.792515337687537,
1.),(1.,0.779105591645567,1.),(1.,0.762081632340355,1.)))
REPRESENTATION_ITEM('')
SURFACE()
);
#2899=(
BOUNDED_SURFACE()
B_SPLINE_SURFACE(3,2,((#187935,#187936,#187937),(#187938,#187939,#187940),
(#187941,#187942,#187943),(#187944,#187945,#187946),(#187947,#187948,#187949),
(#187950,#187951,#187952),(#187953,#187954,#187955),(#187956,#187957,#187958),
(#187959,#187960,#187961),(#187962,#187963,#187964)),.UNSPECIFIED.,.F.,
 .F.,.F.)
B_SPLINE_SURFACE_WITH_KNOTS((4,2,2,2,4),(3,3),(0.,0.000397955182835291,
0.000795910365670582,0.00119386554850587,0.00159182073134117),(0.,1.),
 .UNSPECIFIED.)
GEOMETRIC_REPRESENTATION_ITEM()
RATIONAL_B_SPLINE_SURFACE(((1.,0.60931006565052,1.),(1.,0.60928110676943,
1.),(1.,0.611992414032709,1.),(1.,0.622151576786515,1.),(1.,0.629646305612374,
1.),(1.,0.647895096091951,1.),(1.,0.658798646820943,1.),(1.,0.682038372243284,
1.),(1.,0.694657643733687,1.),(1.,0.707106781186553,1.)))
REPRESENTATION_ITEM('')
SURFACE()
);
#2900=(
BOUNDED_SURFACE()
B_SPLINE_SURFACE(3,2,((#188014,#188015,#188016),(#188017,#188018,#188019),
(#188020,#188021,#188022),(#188023,#188024,#188025),(#188026,#188027,#188028),
(#188029,#188030,#188031),(#188032,#188033,#188034),(#188035,#188036,#188037)),
 .UNSPECIFIED.,.F.,.F.,.F.)
B_SPLINE_SURFACE_WITH_KNOTS((4,2,2,4),(3,3),(0.,0.000399389907139719,0.000798779814279438,
0.00159755962855888),(0.,1.),.UNSPECIFIED.)
GEOMETRIC_REPRESENTATION_ITEM()
RATIONAL_B_SPLINE_SURFACE(((1.,0.707106781186543,1.),(1.,0.719972059607527,
1.),(1.,0.732679659198347,1.),(1.,0.756479572209125,1.),(1.,0.767365377234031,
1.),(1.,0.79501980381119,1.),(1.,0.806340389868128,1.),(1.,0.806206028026398,
1.)))
REPRESENTATION_ITEM('')
SURFACE()
);
#2901=(
BOUNDED_SURFACE()
B_SPLINE_SURFACE(3,2,((#188109,#188110,#188111),(#188112,#188113,#188114),
(#188115,#188116,#188117),(#188118,#188119,#188120),(#188121,#188122,#188123),
(#188124,#188125,#188126)),.UNSPECIFIED.,.F.,.F.,.F.)
B_SPLINE_SURFACE_WITH_KNOTS((4,2,4),(3,3),(0.,0.000635851334990063,0.00127170266998013),
(0.,1.),.UNSPECIFIED.)
GEOMETRIC_REPRESENTATION_ITEM()
RATIONAL_B_SPLINE_SURFACE(((1.,0.549598954535088,1.),(1.,0.549481216714779,
1.),(1.,0.561870616792487,1.),(1.,0.602538835999935,1.),(1.,0.629604434612806,
1.),(1.,0.65799444631184,1.)))
REPRESENTATION_ITEM('')
SURFACE()
);
#2902=(
BOUNDED_SURFACE()
B_SPLINE_SURFACE(3,2,((#188207,#188208,#188209),(#188210,#188211,#188212),
(#188213,#188214,#188215),(#188216,#188217,#188218),(#188219,#188220,#188221),
(#188222,#188223,#188224)),.UNSPECIFIED.,.F.,.F.,.F.)
B_SPLINE_SURFACE_WITH_KNOTS((4,2,4),(3,3),(0.,0.000500133683539797,0.00100026736707959),
(-0.00102329236961724,1.),.UNSPECIFIED.)
GEOMETRIC_REPRESENTATION_ITEM()
RATIONAL_B_SPLINE_SURFACE(((1.0006000441848,0.706807065790613,1.),(1.00056790491851,
0.722510918987102,1.),(1.00055014554087,0.731188486689425,1.),(1.0005372619169,
0.737483668960894,1.),(1.00054173734042,0.735296892411237,1.),(1.00054817863633,
0.732149553437697,1.)))
REPRESENTATION_ITEM('')
SURFACE()
);
#2903=(
BOUNDED_SURFACE()
B_SPLINE_SURFACE(3,2,((#188242,#188243,#188244),(#188245,#188246,#188247),
(#188248,#188249,#188250),(#188251,#188252,#188253)),.UNSPECIFIED.,.F.,
 .F.,.F.)
B_SPLINE_SURFACE_WITH_KNOTS((4,4),(3,3),(5.42101086242752E-20,0.000113625826113285),
(0.,1.),.UNSPECIFIED.)
GEOMETRIC_REPRESENTATION_ITEM()
RATIONAL_B_SPLINE_SURFACE(((1.,0.691935594449019,1.),(1.,0.697297182114951,
1.),(1.,0.702351867303478,1.),(1.,0.70710678118654,1.)))
REPRESENTATION_ITEM('')
SURFACE()
);
#2904=(
BOUNDED_SURFACE()
B_SPLINE_SURFACE(3,2,((#188263,#188264,#188265),(#188266,#188267,#188268),
(#188269,#188270,#188271),(#188272,#188273,#188274)),.UNSPECIFIED.,.F.,
 .F.,.F.)
B_SPLINE_SURFACE_WITH_KNOTS((4,4),(3,3),(-1.50704101975485E-17,0.000358861832009556),
(0.,1.),.UNSPECIFIED.)
GEOMETRIC_REPRESENTATION_ITEM()
RATIONAL_B_SPLINE_SURFACE(((1.,0.707106781186544,1.),(1.,0.693584131808955,
1.),(1.,0.67719600445086,1.),(1.,0.65799444631037,1.)))
REPRESENTATION_ITEM('')
SURFACE()
);
#2905=(
BOUNDED_SURFACE()
B_SPLINE_SURFACE(3,2,((#188288,#188289,#188290),(#188291,#188292,#188293),
(#188294,#188295,#188296),(#188297,#188298,#188299)),.UNSPECIFIED.,.F.,
 .F.,.F.)
B_SPLINE_SURFACE_WITH_KNOTS((4,4),(3,3),(0.000909429960036056,0.00157021148057203),
(0.,1.),.UNSPECIFIED.)
GEOMETRIC_REPRESENTATION_ITEM()
RATIONAL_B_SPLINE_SURFACE(((1.,0.72569894652024,1.),(1.,0.728856973451895,
1.),(1.,0.724481780670466,1.),(1.,0.707106781186543,1.)))
REPRESENTATION_ITEM('')
SURFACE()
);
#2906=(
BOUNDED_SURFACE()
B_SPLINE_SURFACE(3,2,((#188335,#188336,#188337),(#188338,#188339,#188340),
(#188341,#188342,#188343),(#188344,#188345,#188346),(#188347,#188348,#188349),
(#188350,#188351,#188352),(#188353,#188354,#188355),(#188356,#188357,#188358),
(#188359,#188360,#188361),(#188362,#188363,#188364),(#188365,#188366,#188367),
(#188368,#188369,#188370)),.UNSPECIFIED.,.F.,.F.,.F.)
B_SPLINE_SURFACE_WITH_KNOTS((4,2,2,2,2,4),(3,3),(0.,0.000471787629256711,
0.000943575258513421,0.00117946907314178,0.00141536288777013,0.00188715051702685),
(0.,1.),.UNSPECIFIED.)
GEOMETRIC_REPRESENTATION_ITEM()
RATIONAL_B_SPLINE_SURFACE(((1.,0.688859710774758,1.),(1.,0.717278497414175,
1.),(1.,0.742415568607548,1.),(1.,0.786827943379553,1.),(1.,0.806155596178757,
1.),(1.,0.829868996905786,1.),(1.,0.837032764561711,1.),(1.,0.849395444084014,
1.),(1.,0.854694123459555,1.),(1.,0.86824784980175,1.),(1.,0.873676740317143,
1.),(1.,0.875436198637081,1.)))
REPRESENTATION_ITEM('')
SURFACE()
);
#2907=(
BOUNDED_SURFACE()
B_SPLINE_SURFACE(3,2,((#188416,#188417,#188418),(#188419,#188420,#188421),
(#188422,#188423,#188424),(#188425,#188426,#188427)),.UNSPECIFIED.,.F.,
 .F.,.F.)
B_SPLINE_SURFACE_WITH_KNOTS((4,4),(3,3),(0.,0.000504208024932662),(0.,1.),
 .UNSPECIFIED.)
GEOMETRIC_REPRESENTATION_ITEM()
RATIONAL_B_SPLINE_SURFACE(((1.,0.872490094680101,1.),(1.,0.873532316568381,
1.),(1.,0.874514063294085,1.),(1.,0.875436198637085,1.)))
REPRESENTATION_ITEM('')
SURFACE()
);
#2908=(
BOUNDED_SURFACE()
B_SPLINE_SURFACE(3,2,((#188431,#188432,#188433),(#188434,#188435,#188436),
(#188437,#188438,#188439),(#188440,#188441,#188442),(#188443,#188444,#188445),
(#188446,#188447,#188448),(#188449,#188450,#188451),(#188452,#188453,#188454),
(#188455,#188456,#188457),(#188458,#188459,#188460)),.UNSPECIFIED.,.F.,
 .F.,.F.)
B_SPLINE_SURFACE_WITH_KNOTS((4,2,2,2,4),(3,3),(-9.01822866958479E-5,0.000428050429885702,
0.000856100859773762,0.00128415128966182,0.00180238400624337),(0.,1.00070975129598),
 .UNSPECIFIED.)
GEOMETRIC_REPRESENTATION_ITEM()
RATIONAL_B_SPLINE_SURFACE(((1.,0.87087120065611,1.00018329866537),(1.,0.874579814490895,
1.00017803427842),(1.,0.873810679327731,1.00017912606777),(1.,0.863911307902413,
1.00019317825117),(1.,0.856204559855697,1.000204118),(1.,0.833962775819185,
1.00023569027009),(1.,0.819525279404997,1.00025618433367),(1.,0.780375333947201,
1.00031175778272),(1.,0.754589472410923,1.00034836088001),(1.,0.723415614990647,
1.00039261225142)))
REPRESENTATION_ITEM('')
SURFACE()
);
#2909=(
BOUNDED_SURFACE()
B_SPLINE_SURFACE(3,2,((#188483,#188484,#188485),(#188486,#188487,#188488),
(#188489,#188490,#188491),(#188492,#188493,#188494),(#188495,#188496,#188497),
(#188498,#188499,#188500)),.UNSPECIFIED.,.F.,.F.,.F.)
B_SPLINE_SURFACE_WITH_KNOTS((4,2,4),(3,3),(-0.000165293417219257,0.000826467086096255,
0.0018182275894121),(-0.00110131312783401,1.00167262876028),
 .UNSPECIFIED.)
GEOMETRIC_REPRESENTATION_ITEM()
RATIONAL_B_SPLINE_SURFACE(((1.00085459808061,0.61135981365314,1.00129866887682),
(1.00075392303127,0.657143171733025,1.00114568052331),(1.00067880279221,
0.691305129694834,1.00103152590643),(1.00056376087147,0.743622019388052,
1.00085670529147),(1.00052307748563,0.762123346519561,1.00079488178847),
(1.00049052902468,0.77692520509168,1.00074542032329)))
REPRESENTATION_ITEM('')
SURFACE()
);
#2910=(
BOUNDED_SURFACE()
B_SPLINE_SURFACE(3,2,((#188515,#188516,#188517),(#188518,#188519,#188520),
(#188521,#188522,#188523),(#188524,#188525,#188526)),.UNSPECIFIED.,.F.,
 .F.,.F.)
B_SPLINE_SURFACE_WITH_KNOTS((4,4),(3,3),(2.16840434497101E-19,0.000504355062152837),
(0.,1.),.UNSPECIFIED.)
GEOMETRIC_REPRESENTATION_ITEM()
RATIONAL_B_SPLINE_SURFACE(((1.,0.759233451646319,1.),(1.,0.762871393877082,
1.),(1.,0.766403968732707,1.),(1.,0.769836971136898,1.)))
REPRESENTATION_ITEM('')
SURFACE()
);
#2911=(
BOUNDED_SURFACE()
B_SPLINE_SURFACE(3,2,((#188530,#188531,#188532),(#188533,#188534,#188535),
(#188536,#188537,#188538),(#188539,#188540,#188541),(#188542,#188543,#188544),
(#188545,#188546,#188547),(#188548,#188549,#188550),(#188551,#188552,#188553),
(#188554,#188555,#188556),(#188557,#188558,#188559)),.UNSPECIFIED.,.F.,
 .F.,.F.)
B_SPLINE_SURFACE_WITH_KNOTS((4,2,2,2,4),(3,3),(-3.25260651745651E-18,0.000393055033931551,
0.000786110067863104,0.00117916510179466,0.00157222013572621),(0.,1.),
 .UNSPECIFIED.)
GEOMETRIC_REPRESENTATION_ITEM()
RATIONAL_B_SPLINE_SURFACE(((1.,0.759233451646328,1.),(1.,0.765853834182409,
1.),(1.,0.77182063876785,1.),(1.,0.782085007421256,1.),(1.,0.786377884755709,
1.),(1.,0.792439775573655,1.),(1.,0.794229619467717,1.),(1.,0.793882695203775,
1.),(1.,0.791736824593394,1.),(1.,0.786683372191859,1.)))
REPRESENTATION_ITEM('')
SURFACE()
);
#2912=(
BOUNDED_SURFACE()
B_SPLINE_SURFACE(3,2,((#188613,#188614,#188615),(#188616,#188617,#188618),
(#188619,#188620,#188621),(#188622,#188623,#188624),(#188625,#188626,#188627),
(#188628,#188629,#188630),(#188631,#188632,#188633),(#188634,#188635,#188636),
(#188637,#188638,#188639),(#188640,#188641,#188642)),.UNSPECIFIED.,.F.,
 .F.,.F.)
B_SPLINE_SURFACE_WITH_KNOTS((4,2,2,2,4),(3,3),(0.,0.000403813407730069,
0.00080762681546014,0.00121144022319021,0.00161525363092028),(0.,1.),
 .UNSPECIFIED.)
GEOMETRIC_REPRESENTATION_ITEM()
RATIONAL_B_SPLINE_SURFACE(((1.,0.574616980402532,1.),(1.,0.574559944255782,
1.),(1.,0.578580805360036,1.),(1.,0.593205211704828,1.),(1.,0.603887596362185,
1.),(1.,0.629170763939607,1.),(1.,0.643946507952345,1.),(1.,0.674809145535283,
1.),(1.,0.691194307570675,1.),(1.,0.707106781186543,1.)))
REPRESENTATION_ITEM('')
SURFACE()
);
#2913=(
BOUNDED_SURFACE()
B_SPLINE_SURFACE(3,2,((#188695,#188696,#188697),(#188698,#188699,#188700),
(#188701,#188702,#188703),(#188704,#188705,#188706),(#188707,#188708,#188709),
(#188710,#188711,#188712)),.UNSPECIFIED.,.F.,.F.,.F.)
B_SPLINE_SURFACE_WITH_KNOTS((4,2,4),(3,3),(-0.00016234715873864,0.0008117357936932,
0.00178581874612504),(-0.00233857113343664,1.00211339902085),
 .UNSPECIFIED.)
GEOMETRIC_REPRESENTATION_ITEM()
RATIONAL_B_SPLINE_SURFACE(((1.00146568173025,0.685964966691454,1.00132425925821),
(1.00127996764077,0.725755822420716,1.00115646457449),(1.00109456509479,
0.765479927253636,1.00098895137367),(1.00083507105024,0.821078778791707,
1.00075449570444),(1.00076572018014,0.83593780469964,1.000691836445),(1.00079936494528,
0.828729121720177,1.00072223485333)))
REPRESENTATION_ITEM('')
SURFACE()
);
#2914=(
BOUNDED_SURFACE()
B_SPLINE_SURFACE(3,2,((#188743,#188744,#188745),(#188746,#188747,#188748),
(#188749,#188750,#188751),(#188752,#188753,#188754),(#188755,#188756,#188757),
(#188758,#188759,#188760),(#188761,#188762,#188763),(#188764,#188765,#188766),
(#188767,#188768,#188769),(#188770,#188771,#188772)),.UNSPECIFIED.,.F.,
 .F.,.F.)
B_SPLINE_SURFACE_WITH_KNOTS((4,2,2,2,4),(3,3),(0.,0.000408971318093432,
0.000817942636186865,0.0012269139542803,0.00163588527237373),(0.,1.),
 .UNSPECIFIED.)
GEOMETRIC_REPRESENTATION_ITEM()
RATIONAL_B_SPLINE_SURFACE(((1.,0.707106781186548,1.),(1.,0.688859876352089,
1.),(1.,0.670469148037181,1.),(1.,0.634232875326911,1.),(1.,0.617116919953528,
1.),(1.,0.586509610415134,1.),(1.,0.573603373050602,1.),(1.,0.555466576286827,
1.),(1.,0.550482231415542,1.),(1.,0.55046727607882,1.)))
REPRESENTATION_ITEM('')
SURFACE()
);
#2915=(
BOUNDED_SURFACE()
B_SPLINE_SURFACE(3,2,((#188826,#188827,#188828),(#188829,#188830,#188831),
(#188832,#188833,#188834),(#188835,#188836,#188837),(#188838,#188839,#188840),
(#188841,#188842,#188843),(#188844,#188845,#188846),(#188847,#188848,#188849),
(#188850,#188851,#188852),(#188853,#188854,#188855)),.UNSPECIFIED.,.F.,
 .F.,.F.)
B_SPLINE_SURFACE_WITH_KNOTS((4,2,2,2,4),(3,3),(-0.000159702872864176,0.000399257182160439,
0.000798514364320879,0.00119777154648132,0.00175673160150589),(-0.00203488447750748,
1.),.UNSPECIFIED.)
GEOMETRIC_REPRESENTATION_ITEM()
RATIONAL_B_SPLINE_SURFACE(((1.00079831838497,0.803841841197695,1.),(1.00078530711036,
0.807038896055489,1.),(1.00079537143545,0.804565948522982,1.),(1.00084493107595,
0.792388441387141,1.),(1.00087540891547,0.784899603603664,1.),(1.00094983349238,
0.766612428647442,1.),(1.00099439906428,0.755662035051707,1.),(1.00110925525072,
0.727440239732745,1.),(1.00118493769597,0.708843988672124,1.),(1.00125645292226,
0.691271682458585,1.)))
REPRESENTATION_ITEM('')
SURFACE()
);
#2916=(
BOUNDED_SURFACE()
B_SPLINE_SURFACE(3,2,((#188905,#188906,#188907),(#188908,#188909,#188910),
(#188911,#188912,#188913),(#188914,#188915,#188916),(#188917,#188918,#188919),
(#188920,#188921,#188922)),.UNSPECIFIED.,.F.,.F.,.F.)
B_SPLINE_SURFACE_WITH_KNOTS((4,2,4),(3,3),(-9.2024572792766E-5,0.000795696580732677,
0.00168341773425804),(0.,1.00126533647542),.UNSPECIFIED.)
GEOMETRIC_REPRESENTATION_ITEM()
RATIONAL_B_SPLINE_SURFACE(((1.,0.715289297039673,1.0007205096748),(1.,0.687888441120641,
1.0007898522797),(1.,0.659167558273284,1.00086253544105),(1.,0.618590884857398,
1.0009652217309),(1.,0.606932851144685,1.00099472440148),(1.,0.610119385799617,
1.00098666032442)))
REPRESENTATION_ITEM('')
SURFACE()
);
#2917=(
BOUNDED_SURFACE()
B_SPLINE_SURFACE(3,2,((#188952,#188953,#188954),(#188955,#188956,#188957),
(#188958,#188959,#188960),(#188961,#188962,#188963),(#188964,#188965,#188966),
(#188967,#188968,#188969),(#188970,#188971,#188972),(#188973,#188974,#188975),
(#188976,#188977,#188978),(#188979,#188980,#188981)),.UNSPECIFIED.,.F.,
 .F.,.F.)
B_SPLINE_SURFACE_WITH_KNOTS((4,2,2,2,4),(3,3),(-7.15573433840433E-18,0.000392138229924569,
0.000784276459849145,0.00117641468977372,0.00156855291969829),(0.,1.),
 .UNSPECIFIED.)
GEOMETRIC_REPRESENTATION_ITEM()
RATIONAL_B_SPLINE_SURFACE(((1.,0.761454662564716,1.),(1.,0.777350220421001,
1.),(1.,0.789525254479917,1.),(1.,0.80808932428192,1.),(1.,0.814267286660623,
1.),(1.,0.822043050215882,1.),(1.,0.823560107182087,1.),(1.,0.822913353545903,
1.),(1.,0.820747192732385,1.),(1.,0.816955285488498,1.)))
REPRESENTATION_ITEM('')
SURFACE()
);
#2918=(
BOUNDED_SURFACE()
B_SPLINE_SURFACE(3,2,((#189021,#189022,#189023),(#189024,#189025,#189026),
(#189027,#189028,#189029),(#189030,#189031,#189032)),.UNSPECIFIED.,.F.,
 .F.,.F.)
B_SPLINE_SURFACE_WITH_KNOTS((4,4),(3,3),(0.,0.000503800937603746),(0.,1.),
 .UNSPECIFIED.)
GEOMETRIC_REPRESENTATION_ITEM()
RATIONAL_B_SPLINE_SURFACE(((1.,0.816955285488328,1.),(1.,0.819071576866324,
1.),(1.,0.821113754793722,1.),(1.,0.823084066989369,1.)))
REPRESENTATION_ITEM('')
SURFACE()
);
#2919=(
BOUNDED_SURFACE()
B_SPLINE_SURFACE(3,2,((#189036,#189037,#189038),(#189039,#189040,#189041),
(#189042,#189043,#189044),(#189045,#189046,#189047),(#189048,#189049,#189050),
(#189051,#189052,#189053),(#189054,#189055,#189056),(#189057,#189058,#189059),
(#189060,#189061,#189062),(#189063,#189064,#189065)),.UNSPECIFIED.,.F.,
 .F.,.F.)
B_SPLINE_SURFACE_WITH_KNOTS((4,2,2,2,4),(3,3),(-4.62791697325438E-16,0.00043428534736775,
0.000868570694735964,0.00130285604210418,0.00173714138947239),(0.,1.),
 .UNSPECIFIED.)
GEOMETRIC_REPRESENTATION_ITEM()
RATIONAL_B_SPLINE_SURFACE(((1.,0.823084066989561,1.),(1.,0.819254444805576,
1.),(1.,0.813299508531675,1.),(1.,0.797300511206505,1.),(1.,0.787129420739965,
1.),(1.,0.761999300344554,1.),(1.,0.746886433981532,1.),(1.,0.710597168436061,
1.),(1.,0.68930848675479,1.),(1.,0.664389729441784,1.)))
REPRESENTATION_ITEM('')
SURFACE()
);
#2920=(
BOUNDED_SURFACE()
B_SPLINE_SURFACE(3,2,((#189124,#189125,#189126),(#189127,#189128,#189129),
(#189130,#189131,#189132),(#189133,#189134,#189135),(#189136,#189137,#189138),
(#189139,#189140,#189141),(#189142,#189143,#189144),(#189145,#189146,#189147)),
 .UNSPECIFIED.,.F.,.F.,.F.)
B_SPLINE_SURFACE_WITH_KNOTS((4,2,2,4),(3,3),(-2.3396834471962E-5,0.000883592517330617,
0.00132538877599593,0.00179058186913343),(0.,1.00056892075226),
 .UNSPECIFIED.)
GEOMETRIC_REPRESENTATION_ITEM()
RATIONAL_B_SPLINE_SURFACE(((1.,0.710255087975394,1.00032968378662),(1.,
0.764314513729547,1.00026817272829),(1.,0.803922650049074,1.00022310494687),
(1.,0.84311117612549,1.0001785146154),(1.,0.852411846552129,1.00016793192657),
(1.,0.865347821163161,1.00015321283775),(1.,0.86831947063463,1.00014983157165),
(1.,0.867933686036368,1.00015027053338)))
REPRESENTATION_ITEM('')
SURFACE()
);
#2921=(
BOUNDED_SURFACE()
B_SPLINE_SURFACE(3,2,((#189196,#189197,#189198),(#189199,#189200,#189201),
(#189202,#189203,#189204),(#189205,#189206,#189207)),.UNSPECIFIED.,.F.,
 .F.,.F.)
B_SPLINE_SURFACE_WITH_KNOTS((4,4),(3,3),(0.,0.00040046484477139),(0.,1.),
 .UNSPECIFIED.)
GEOMETRIC_REPRESENTATION_ITEM()
RATIONAL_B_SPLINE_SURFACE(((1.,0.707106781186548,1.),(1.,0.718332690797356,
1.),(1.,0.721890377876178,1.),(1.,0.71893387489533,1.)))
REPRESENTATION_ITEM('')
SURFACE()
);
#2922=(
BOUNDED_SURFACE()
B_SPLINE_SURFACE(3,2,((#189227,#189228,#189229),(#189230,#189231,#189232),
(#189233,#189234,#189235),(#189236,#189237,#189238)),.UNSPECIFIED.,.F.,
 .F.,.F.)
B_SPLINE_SURFACE_WITH_KNOTS((4,4),(3,3),(0.,0.000502699148463484),(0.,1.),
 .UNSPECIFIED.)
GEOMETRIC_REPRESENTATION_ITEM()
RATIONAL_B_SPLINE_SURFACE(((1.,0.868041451421792,1.),(1.,0.868099423952364,
1.),(1.,0.868099396145349,1.),(1.,0.868041451421496,1.)))
REPRESENTATION_ITEM('')
SURFACE()
);
#2923=(
BOUNDED_SURFACE()
B_SPLINE_SURFACE(3,2,((#189240,#189241,#189242),(#189243,#189244,#189245),
(#189246,#189247,#189248),(#189249,#189250,#189251)),.UNSPECIFIED.,.F.,
 .F.,.F.)
B_SPLINE_SURFACE_WITH_KNOTS((4,4),(3,3),(0.0235251249547107,0.0240364247854912),
(0.,0.920133931130292),.UNSPECIFIED.)
GEOMETRIC_REPRESENTATION_ITEM()
RATIONAL_B_SPLINE_SURFACE(((1.,0.856496456488226,0.977077872221683),(1.,
0.856565845946365,0.977088955948168),(1.,0.856565846106366,0.977088955973725),
(1.,0.85649645648538,0.977077872221228)))
REPRESENTATION_ITEM('')
SURFACE()
);
#2924=(
BOUNDED_SURFACE()
B_SPLINE_SURFACE(3,2,((#189255,#189256,#189257),(#189258,#189259,#189260),
(#189261,#189262,#189263),(#189264,#189265,#189266)),.UNSPECIFIED.,.F.,
 .F.,.F.)
B_SPLINE_SURFACE_WITH_KNOTS((4,4),(3,3),(0.0238558353156833,0.0243674807756399),
(0.,0.921037717824849),.UNSPECIFIED.)
GEOMETRIC_REPRESENTATION_ITEM()
RATIONAL_B_SPLINE_SURFACE(((1.,0.866519190723957,0.978920101345955),(1.,
0.866587888331177,0.978930950385647),(1.,0.866587880203078,0.978930949102021),
(1.,0.866519190868502,0.978920101368782)))
REPRESENTATION_ITEM('')
SURFACE()
);
#2925=(
BOUNDED_SURFACE()
B_SPLINE_SURFACE(3,2,((#189268,#189269,#189270),(#189271,#189272,#189273),
(#189274,#189275,#189276),(#189277,#189278,#189279)),.UNSPECIFIED.,.F.,
 .F.,.F.)
B_SPLINE_SURFACE_WITH_KNOTS((4,4),(3,3),(-8.67361737988404E-19,0.00050299424914367),
(0.,1.),.UNSPECIFIED.)
GEOMETRIC_REPRESENTATION_ITEM()
RATIONAL_B_SPLINE_SURFACE(((1.,0.877250029438358,1.),(1.,0.877307222991301,
1.),(1.,0.877307195652826,1.),(1.,0.877250029437921,1.)))
REPRESENTATION_ITEM('')
SURFACE()
);
#2926=(
BOUNDED_SURFACE()
B_SPLINE_SURFACE(3,2,((#189418,#189419,#189420),(#189421,#189422,#189423),
(#189424,#189425,#189426),(#189427,#189428,#189429),(#189430,#189431,#189432),
(#189433,#189434,#189435)),.UNSPECIFIED.,.F.,.F.,.F.)
B_SPLINE_SURFACE_WITH_KNOTS((4,2,4),(3,3),(0.,0.000611885440421095,0.00122377088084219),
(0.,1.),.UNSPECIFIED.)
GEOMETRIC_REPRESENTATION_ITEM()
RATIONAL_B_SPLINE_SURFACE(((1.,0.713250449154079,1.),(1.,0.672263173507019,
1.),(1.,0.648659882421647,1.),(1.,0.648739723662275,1.),(1.,0.672275262307808,
1.),(1.,0.713250449154082,1.)))
REPRESENTATION_ITEM('')
SURFACE()
);
#2927=(
BOUNDED_SURFACE()
B_SPLINE_SURFACE(3,2,((#189462,#189463,#189464),(#189465,#189466,#189467),
(#189468,#189469,#189470),(#189471,#189472,#189473),(#189474,#189475,#189476),
(#189477,#189478,#189479),(#189480,#189481,#189482),(#189483,#189484,#189485),
(#189486,#189487,#189488),(#189489,#189490,#189491)),.UNSPECIFIED.,.F.,
 .F.,.F.)
B_SPLINE_SURFACE_WITH_KNOTS((4,2,2,2,4),(3,3),(-1.10588621593521E-17,0.00061030576480229,
0.00122061152960459,0.00183091729440689,0.0024412230592092),(0.,1.),
 .UNSPECIFIED.)
GEOMETRIC_REPRESENTATION_ITEM()
RATIONAL_B_SPLINE_SURFACE(((1.,0.727552664059041,1.),(1.,0.745088511631937,
1.),(1.,0.761651043043578,1.),(1.,0.793171709476032,1.),(1.,0.808261553244041,
1.),(1.,0.836218122215552,1.),(1.,0.8491155211034,1.),(1.,0.872797166619207,
1.),(1.,0.883451618896772,1.),(1.,0.892325300547709,1.)))
REPRESENTATION_ITEM('')
SURFACE()
);
#2928=(
BOUNDED_SURFACE()
B_SPLINE_SURFACE(3,2,((#189539,#189540,#189541),(#189542,#189543,#189544),
(#189545,#189546,#189547),(#189548,#189549,#189550)),.UNSPECIFIED.,.F.,
 .F.,.F.)
B_SPLINE_SURFACE_WITH_KNOTS((4,4),(3,3),(0.,0.010514647628205),(0.,1.),
 .UNSPECIFIED.)
GEOMETRIC_REPRESENTATION_ITEM()
RATIONAL_B_SPLINE_SURFACE(((1.,0.727552664059029,1.),(1.,0.728396913847474,
1.),(1.,0.728235528042243,1.),(1.,0.727880838895167,1.)))
REPRESENTATION_ITEM('')
SURFACE()
);
#2929=(
BOUNDED_SURFACE()
B_SPLINE_SURFACE(3,2,((#189581,#189582,#189583),(#189584,#189585,#189586),
(#189587,#189588,#189589),(#189590,#189591,#189592),(#189593,#189594,#189595),
(#189596,#189597,#189598),(#189599,#189600,#189601),(#189602,#189603,#189604),
(#189605,#189606,#189607),(#189608,#189609,#189610)),.UNSPECIFIED.,.F.,
 .F.,.F.)
B_SPLINE_SURFACE_WITH_KNOTS((4,2,2,2,4),(3,3),(-0.000237785429372242,0.000594463573430658,
0.00118892714686131,0.00178339072029198,0.00261563972309489),(0.,1.00128235392051),
 .UNSPECIFIED.)
GEOMETRIC_REPRESENTATION_ITEM()
RATIONAL_B_SPLINE_SURFACE(((1.,0.922004222179873,1.00020003638294),(1.,
0.933851150468113,1.00016965247307),(1.,0.92880531270258,1.00018259357275),
(1.,0.902012680283328,1.0002513088472),(1.,0.885879697912423,1.00029268523358),
(1.,0.848390934561697,1.0003888329589),(1.,0.826950983044361,1.00044382017067),
(1.,0.770649871834025,1.00058821607204),(1.,0.734476704092988,1.00068098967898),
(1.,0.693640011354707,1.00078572386505)))
REPRESENTATION_ITEM('')
SURFACE()
);
#2930=(
BOUNDED_SURFACE()
B_SPLINE_SURFACE(3,2,((#189682,#189683,#189684),(#189685,#189686,#189687),
(#189688,#189689,#189690),(#189691,#189692,#189693),(#189694,#189695,#189696),
(#189697,#189698,#189699)),.UNSPECIFIED.,.F.,.F.,.F.)
B_SPLINE_SURFACE_WITH_KNOTS((4,2,4),(3,3),(-1.38777878078145E-17,0.0041604828508626,
0.00832096570172521),(0.,1.),.UNSPECIFIED.)
GEOMETRIC_REPRESENTATION_ITEM()
RATIONAL_B_SPLINE_SURFACE(((1.,0.928260885086434,1.),(1.,0.928493402693592,
1.),(1.,0.928615016565842,1.),(1.,0.928561249118847,1.),(1.,0.928391240061757,
1.),(1.,0.928132015153712,1.)))
REPRESENTATION_ITEM('')
SURFACE()
);
#2931=(
BOUNDED_SURFACE()
B_SPLINE_SURFACE(3,2,((#189722,#189723,#189724),(#189725,#189726,#189727),
(#189728,#189729,#189730),(#189731,#189732,#189733),(#189734,#189735,#189736),
(#189737,#189738,#189739),(#189740,#189741,#189742),(#189743,#189744,#189745),
(#189746,#189747,#189748),(#189749,#189750,#189751)),.UNSPECIFIED.,.F.,
 .F.,.F.)
B_SPLINE_SURFACE_WITH_KNOTS((4,2,2,2,4),(3,3),(-0.00023493367097703,0.000587334177442414,
0.00117466835488487,0.00176200253232733,0.00258427038074678),(0.,1.00065879078994),
 .UNSPECIFIED.)
GEOMETRIC_REPRESENTATION_ITEM()
RATIONAL_B_SPLINE_SURFACE(((1.,0.701334864614367,1.00039351568094),(1.,
0.741616670565157,1.00034044111541),(1.,0.777121913763768,1.00029366006098),
(1.,0.832030184715688,1.00022131393459),(1.,0.853267713621314,1.00019333175771),
(1.,0.889718813400979,1.00014530446007),(1.,0.905272975779917,1.00012481058223),
(1.,0.930301816583754,1.00009183304262),(1.,0.933805909408884,1.00008721611446),
(1.,0.920947462794136,1.00010415816686)))
REPRESENTATION_ITEM('')
SURFACE()
);
#2932=(
BOUNDED_SURFACE()
B_SPLINE_SURFACE(3,2,((#189820,#189821,#189822),(#189823,#189824,#189825),
(#189826,#189827,#189828),(#189829,#189830,#189831)),.UNSPECIFIED.,.F.,
 .F.,.F.)
B_SPLINE_SURFACE_WITH_KNOTS((4,4),(3,3),(0.,0.0107001581246114),(0.,1.),
 .UNSPECIFIED.)
GEOMETRIC_REPRESENTATION_ITEM()
RATIONAL_B_SPLINE_SURFACE(((1.,0.73489735095993,1.),(1.,0.734875794442845,
1.),(1.,0.734252034560147,1.),(1.,0.73129868040477,1.)))
REPRESENTATION_ITEM('')
SURFACE()
);
#2933=(
BOUNDED_SURFACE()
B_SPLINE_SURFACE(3,2,((#189843,#189844,#189845),(#189846,#189847,#189848),
(#189849,#189850,#189851),(#189852,#189853,#189854)),.UNSPECIFIED.,.F.,
 .F.,.F.)
B_SPLINE_SURFACE_WITH_KNOTS((4,4),(3,3),(0.,0.000517122404042923),(0.,1.),
 .UNSPECIFIED.)
GEOMETRIC_REPRESENTATION_ITEM()
RATIONAL_B_SPLINE_SURFACE(((1.,0.707106781186546,1.),(1.,0.731070766440982,
1.),(1.,0.753745435486364,1.),(1.,0.77196935846749,1.)))
REPRESENTATION_ITEM('')
SURFACE()
);
#2934=(
BOUNDED_SURFACE()
B_SPLINE_SURFACE(3,2,((#189866,#189867,#189868),(#189869,#189870,#189871),
(#189872,#189873,#189874),(#189875,#189876,#189877),(#189878,#189879,#189880),
(#189881,#189882,#189883)),.UNSPECIFIED.,.F.,.F.,.F.)
B_SPLINE_SURFACE_WITH_KNOTS((4,2,4),(3,3),(-2.92626166353837E-16,0.00117037761632422,
0.00247736720267303),(0.,1.00013661197002),.UNSPECIFIED.)
GEOMETRIC_REPRESENTATION_ITEM()
RATIONAL_B_SPLINE_SURFACE(((1.,0.888632222864986,1.00003042834286),(1.,
0.871230572502141,1.00003518289034),(1.,0.84777527697816,1.0000415914386),
(1.,0.791539704054847,1.0000569563434),(1.,0.757531651118529,1.00006624815762),
(1.,0.719456177971868,1.00007665128841)))
REPRESENTATION_ITEM('')
SURFACE()
);
#2935=(
BOUNDED_SURFACE()
B_SPLINE_SURFACE(3,2,((#189921,#189922,#189923),(#189924,#189925,#189926),
(#189927,#189928,#189929),(#189930,#189931,#189932),(#189933,#189934,#189935),
(#189936,#189937,#189938),(#189939,#189940,#189941),(#189942,#189943,#189944),
(#189945,#189946,#189947),(#189948,#189949,#189950),(#189951,#189952,#189953),
(#189954,#189955,#189956)),.UNSPECIFIED.,.F.,.F.,.F.)
B_SPLINE_SURFACE_WITH_KNOTS((4,2,2,2,2,4),(3,3),(-0.000229639107487331,
0.000574097768718188,0.00114819553743641,0.00143524442179553,0.00172229330615464,
0.00252603018236012),(0.,1.0004970139285),.UNSPECIFIED.)
GEOMETRIC_REPRESENTATION_ITEM()
RATIONAL_B_SPLINE_SURFACE(((1.,0.700923021341121,1.00029729084818),(1.,
0.7401895073962,1.00025825886719),(1.,0.774929246625952,1.00022372659865),
(1.,0.828726764317455,1.00017025036743),(1.,0.848866331641938,1.00015023107648),
(1.,0.875086581874444,1.00012416741733),(1.,0.883052096108772,1.00011624947429),
(1.,0.896973719729107,1.00010241099259),(1.,0.903053458090336,1.0000963675633),
(1.,0.921003114707731,1.0000785251046),(1.,0.923996083572407,1.00007555001017),
(1.,0.912082123762018,1.00008739281811)))
REPRESENTATION_ITEM('')
SURFACE()
);
#2936=(
BOUNDED_SURFACE()
B_SPLINE_SURFACE(3,2,((#190030,#190031,#190032),(#190033,#190034,#190035),
(#190036,#190037,#190038),(#190039,#190040,#190041)),.UNSPECIFIED.,.F.,
 .F.,.F.)
B_SPLINE_SURFACE_WITH_KNOTS((4,4),(3,3),(-0.00012025625334337,0.00992992973959445),
(0.,1.00012025625329),.UNSPECIFIED.)
GEOMETRIC_REPRESENTATION_ITEM()
RATIONAL_B_SPLINE_SURFACE(((1.,0.733625250090197,1.00006406645879),(1.,
0.732900523743408,1.00006424076454),(1.,0.731718785769699,1.0000645249873),
(1.,0.729605009136797,1.00006503337702)))
REPRESENTATION_ITEM('')
SURFACE()
);
#2937=(
BOUNDED_SURFACE()
B_SPLINE_SURFACE(3,2,((#190062,#190063,#190064),(#190065,#190066,#190067),
(#190068,#190069,#190070),(#190071,#190072,#190073),(#190074,#190075,#190076),
(#190077,#190078,#190079)),.UNSPECIFIED.,.F.,.F.,.F.)
B_SPLINE_SURFACE_WITH_KNOTS((4,2,4),(3,3),(-1.04083408558608E-17,0.00416021787251448,
0.00832043574502897),(0.,1.),.UNSPECIFIED.)
GEOMETRIC_REPRESENTATION_ITEM()
RATIONAL_B_SPLINE_SURFACE(((1.,0.91815876419713,1.),(1.,0.918478576988139,
1.),(1.,0.918702883828552,1.),(1.,0.918900670636956,1.),(1.,0.918880394705029,
1.),(1.,0.918792784744087,1.)))
REPRESENTATION_ITEM('')
SURFACE()
);
#2938=(
BOUNDED_SURFACE()
B_SPLINE_SURFACE(3,2,((#190115,#190116,#190117),(#190118,#190119,#190120),
(#190121,#190122,#190123),(#190124,#190125,#190126),(#190127,#190128,#190129),
(#190130,#190131,#190132)),.UNSPECIFIED.,.F.,.F.,.F.)
B_SPLINE_SURFACE_WITH_KNOTS((4,2,4),(3,3),(0.,0.00128099832444667,0.00256199664889334),
(0.,1.),.UNSPECIFIED.)
GEOMETRIC_REPRESENTATION_ITEM()
RATIONAL_B_SPLINE_SURFACE(((1.,0.901968956514557,1.),(1.,0.883369478136272,
1.),(1.,0.857628018061933,1.),(1.,0.799434735382796,1.),(1.,0.766284883168506,
1.),(1.,0.729712990977659,1.)))
REPRESENTATION_ITEM('')
SURFACE()
);
#2939=(
BOUNDED_SURFACE()
B_SPLINE_SURFACE(3,2,((#190148,#190149,#190150),(#190151,#190152,#190153),
(#190154,#190155,#190156),(#190157,#190158,#190159),(#190160,#190161,#190162),
(#190163,#190164,#190165),(#190166,#190167,#190168),(#190169,#190170,#190171),
(#190172,#190173,#190174),(#190175,#190176,#190177)),.UNSPECIFIED.,.F.,
 .F.,.F.)
B_SPLINE_SURFACE_WITH_KNOTS((4,2,2,2,4),(3,3),(-0.000230073755017583,0.000575184387543924,
0.00115036877508786,0.00172555316263179,0.0025308113051933),(0.,1.00091870395598),
 .UNSPECIFIED.)
GEOMETRIC_REPRESENTATION_ITEM()
RATIONAL_B_SPLINE_SURFACE(((1.,0.912190934045583,1.00016134107253),(1.,
0.923169507875512,1.00014116895411),(1.,0.919328473509897,1.00014822650104),
(1.,0.895550804689188,1.00019191577786),(1.,0.880755800234217,1.00021910023611),
(1.,0.845438547487969,1.00028399243573),(1.,0.825154962787659,1.00032126165474),
(1.,0.771085355509094,1.00042060957895),(1.,0.736236157458662,1.00048464177118),
(1.,0.696833914618885,1.00055703976392)))
REPRESENTATION_ITEM('')
SURFACE()
);
#2940=(
BOUNDED_SURFACE()
B_SPLINE_SURFACE(3,2,((#190247,#190248,#190249),(#190250,#190251,#190252),
(#190253,#190254,#190255),(#190256,#190257,#190258)),.UNSPECIFIED.,.F.,
 .F.,.F.)
B_SPLINE_SURFACE_WITH_KNOTS((4,4),(3,3),(-8.33055367281454E-5,0.00981269153950731),
(0.,1.00008330553673),.UNSPECIFIED.)
GEOMETRIC_REPRESENTATION_ITEM()
RATIONAL_B_SPLINE_SURFACE(((1.,0.729482986426254,1.00004507113002),(1.,
0.730583093938839,1.00004488783993),(1.,0.730289958374372,1.00004493667956),
(1.,0.729733000633497,1.00004502947488)))
REPRESENTATION_ITEM('')
SURFACE()
);
#2941=(
BOUNDED_SURFACE()
B_SPLINE_SURFACE(3,2,((#190285,#190286,#190287),(#190288,#190289,#190290),
(#190291,#190292,#190293),(#190294,#190295,#190296)),.UNSPECIFIED.,.F.,
 .F.,.F.)
B_SPLINE_SURFACE_WITH_KNOTS((4,4),(3,3),(-6.39679281766448E-18,3.42512019832298E-5),
(0.,1.),.UNSPECIFIED.)
GEOMETRIC_REPRESENTATION_ITEM()
RATIONAL_B_SPLINE_SURFACE(((1.,0.707106781186548,1.),(1.,0.70842711846827,
1.),(1.,0.709730890158149,1.),(1.,0.711017327239758,1.)))
REPRESENTATION_ITEM('')
SURFACE()
);
#2942=(
BOUNDED_SURFACE()
B_SPLINE_SURFACE(3,2,((#190308,#190309,#190310),(#190311,#190312,#190313),
(#190314,#190315,#190316),(#190317,#190318,#190319),(#190320,#190321,#190322),
(#190323,#190324,#190325),(#190326,#190327,#190328),(#190329,#190330,#190331)),
 .UNSPECIFIED.,.F.,.F.,.F.)
B_SPLINE_SURFACE_WITH_KNOTS((4,2,2,4),(3,3),(-4.40186082029115E-17,0.00128517876997136,
0.00192776815495707,0.00257035753994277),(0.,1.),.UNSPECIFIED.)
GEOMETRIC_REPRESENTATION_ITEM()
RATIONAL_B_SPLINE_SURFACE(((1.,0.729533004763577,1.),(1.,0.766429181343272,
1.),(1.,0.799163813689396,1.),(1.,0.843673470277402,1.),(1.,0.857403797497954,
1.),(1.,0.882315838156852,1.),(1.,0.8936522353954,1.),(1.,0.903015666115932,
1.)))
REPRESENTATION_ITEM('')
SURFACE()
);
#2943=(
BOUNDED_SURFACE()
B_SPLINE_SURFACE(3,2,((#190367,#190368,#190369),(#190370,#190371,#190372),
(#190373,#190374,#190375),(#190376,#190377,#190378)),.UNSPECIFIED.,.F.,
 .F.,.F.)
B_SPLINE_SURFACE_WITH_KNOTS((4,4),(3,3),(-6.61363325216158E-18,2.21589532008063E-5),
(0.,1.),.UNSPECIFIED.)
GEOMETRIC_REPRESENTATION_ITEM()
RATIONAL_B_SPLINE_SURFACE(((1.,0.707106781186552,1.),(1.,0.707961610595566,
1.),(1.,0.708809519028292,1.),(1.,0.709650295730098,1.)))
REPRESENTATION_ITEM('')
SURFACE()
);
#2944=(
BOUNDED_SURFACE()
B_SPLINE_SURFACE(3,2,((#190438,#190439,#190440),(#190441,#190442,#190443),
(#190444,#190445,#190446),(#190447,#190448,#190449)),.UNSPECIFIED.,.F.,
 .F.,.F.)
B_SPLINE_SURFACE_WITH_KNOTS((4,4),(3,3),(0.00880203782093236,0.00917783640854858),
(0.,1.),.UNSPECIFIED.)
GEOMETRIC_REPRESENTATION_ITEM()
RATIONAL_B_SPLINE_SURFACE(((1.,0.928452770819608,1.),(1.,0.928460035446427,
1.),(1.,0.928468213633899,1.),(1.,0.928477160954731,1.)))
REPRESENTATION_ITEM('')
SURFACE()
);
#2945=(
BOUNDED_SURFACE()
B_SPLINE_SURFACE(3,2,((#190455,#190456,#190457),(#190458,#190459,#190460),
(#190461,#190462,#190463),(#190464,#190465,#190466)),.UNSPECIFIED.,.F.,
 .F.,.F.)
B_SPLINE_SURFACE_WITH_KNOTS((4,4),(3,3),(0.,0.000210836370419711),(0.,1.),
 .UNSPECIFIED.)
GEOMETRIC_REPRESENTATION_ITEM()
RATIONAL_B_SPLINE_SURFACE(((1.,0.928492930368189,1.),(1.,0.928487440815482,
1.),(1.,0.928482179049582,1.),(1.,0.928477160954739,1.)))
REPRESENTATION_ITEM('')
SURFACE()
);
#2946=(
BOUNDED_SURFACE()
B_SPLINE_SURFACE(3,2,((#190475,#190476,#190477),(#190478,#190479,#190480),
(#190481,#190482,#190483),(#190484,#190485,#190486),(#190487,#190488,#190489),
(#190490,#190491,#190492),(#190493,#190494,#190495),(#190496,#190497,#190498),
(#190499,#190500,#190501),(#190502,#190503,#190504),(#190505,#190506,#190507),
(#190508,#190509,#190510)),.UNSPECIFIED.,.F.,.F.,.F.)
B_SPLINE_SURFACE_WITH_KNOTS((4,2,2,2,2,4),(3,3),(0.,0.000515857252641128,
0.00103171450528226,0.00154757175792339,0.00180550038424395,0.00206342901056451),
(0.,1.),.UNSPECIFIED.)
GEOMETRIC_REPRESENTATION_ITEM()
RATIONAL_B_SPLINE_SURFACE(((1.,0.833636261310757,1.),(1.,0.852503152936051,
1.),(1.,0.870009925957043,1.),(1.,0.902231799969848,1.),(1.,0.917257297026174,
1.),(1.,0.941890812780404,1.),(1.,0.951540383616161,1.),(1.,0.957012273115604,
1.),(1.,0.957266013039511,1.),(1.,0.954585364787499,1.),(1.,0.951691174223743,
1.),(1.,0.94762543845782,1.)))
REPRESENTATION_ITEM('')
SURFACE()
);
#2947=(
BOUNDED_SURFACE()
B_SPLINE_SURFACE(3,2,((#190538,#190539,#190540),(#190541,#190542,#190543),
(#190544,#190545,#190546),(#190547,#190548,#190549),(#190550,#190551,#190552),
(#190553,#190554,#190555),(#190556,#190557,#190558),(#190559,#190560,#190561),
(#190562,#190563,#190564),(#190565,#190566,#190567),(#190568,#190569,#190570),
(#190571,#190572,#190573)),.UNSPECIFIED.,.F.,.F.,.F.)
B_SPLINE_SURFACE_WITH_KNOTS((4,2,2,2,2,4),(3,3),(-0.000236631349860531,
0.000591578374651329,0.000887367561976994,0.00118315674930266,0.00177473512395399,
0.00260294484846585),(-0.000316350823376031,1.),.UNSPECIFIED.)
GEOMETRIC_REPRESENTATION_ITEM()
RATIONAL_B_SPLINE_SURFACE(((1.00005654889587,0.910623125196701,1.),(1.00004251824259,
0.932798906393937,1.),(1.00003076168259,0.951380429072687,1.),(1.00002821571298,
0.95540439459059,1.),(1.00002884406971,0.954411261834663,1.),(1.0000324794467,
0.94866546204241,1.),(1.00003543438326,0.943995114528206,1.),(1.00004647347567,
0.926547566441873,1.),(1.00005663693604,0.910483975614549,1.),(1.00008366922795,
0.867758795350838,1.),(1.00010211678816,0.838601987700274,1.),(1.00012218890575,
0.806877528490201,1.)))
REPRESENTATION_ITEM('')
SURFACE()
);
#2948=(
BOUNDED_SURFACE()
B_SPLINE_SURFACE(3,2,((#190623,#190624,#190625),(#190626,#190627,#190628),
(#190629,#190630,#190631),(#190632,#190633,#190634)),.UNSPECIFIED.,.F.,
 .F.,.F.)
B_SPLINE_SURFACE_WITH_KNOTS((4,4),(3,3),(-5.20417042793042E-18,0.000729297262992661),
(0.,1.),.UNSPECIFIED.)
GEOMETRIC_REPRESENTATION_ITEM()
RATIONAL_B_SPLINE_SURFACE(((1.,0.833636261310766,1.),(1.,0.833189131672253,
1.),(1.,0.83273693675361,1.),(1.,0.832279622729512,1.)))
REPRESENTATION_ITEM('')
SURFACE()
);
#2949=(
BOUNDED_SURFACE()
B_SPLINE_SURFACE(3,2,((#190640,#190641,#190642),(#190643,#190644,#190645),
(#190646,#190647,#190648),(#190649,#190650,#190651)),.UNSPECIFIED.,.F.,
 .F.,.F.)
B_SPLINE_SURFACE_WITH_KNOTS((4,4),(3,3),(-1.04083408558608E-17,0.000723082784825488),
(0.,1.),.UNSPECIFIED.)
GEOMETRIC_REPRESENTATION_ITEM()
RATIONAL_B_SPLINE_SURFACE(((1.,0.832455503270619,1.),(1.,0.832789231498785,
1.),(1.,0.833122604759493,1.),(1.,0.833454935865631,1.)))
REPRESENTATION_ITEM('')
SURFACE()
);
#2950=(
BOUNDED_SURFACE()
B_SPLINE_SURFACE(3,2,((#190657,#190658,#190659),(#190660,#190661,#190662),
(#190663,#190664,#190665),(#190666,#190667,#190668)),.UNSPECIFIED.,.F.,
 .F.,.F.)
B_SPLINE_SURFACE_WITH_KNOTS((4,4),(3,3),(-5.74122752815573E-5,0.0016458175534959),
(0.,1.0000582174393),.UNSPECIFIED.)
GEOMETRIC_REPRESENTATION_ITEM()
RATIONAL_B_SPLINE_SURFACE(((1.,0.831178243785979,1.00001965674069),(1.,
0.842029459925232,1.00001839328066),(1.,0.851208165407911,1.0000173245592),
(1.,0.858742600214373,1.0000164472882)))
REPRESENTATION_ITEM('')
SURFACE()
);
#2951=(
BOUNDED_SURFACE()
B_SPLINE_SURFACE(3,2,((#190695,#190696,#190697),(#190698,#190699,#190700),
(#190701,#190702,#190703),(#190704,#190705,#190706)),.UNSPECIFIED.,.F.,
 .F.,.F.)
B_SPLINE_SURFACE_WITH_KNOTS((4,4),(3,3),(-5.23390230695915E-5,0.00157016878280004),
(0.,1.00005233902307),.UNSPECIFIED.)
GEOMETRIC_REPRESENTATION_ITEM()
RATIONAL_B_SPLINE_SURFACE(((1.,0.857807746985037,1.00001488440722),(1.,
0.850509611749564,1.00001564836176),(1.,0.841739216144316,1.00001656642963),
(1.,0.831471023017743,1.00001764128403)))
REPRESENTATION_ITEM('')
SURFACE()
);
#2952=(
BOUNDED_SURFACE()
B_SPLINE_SURFACE(3,2,((#190733,#190734,#190735),(#190736,#190737,#190738),
(#190739,#190740,#190741),(#190742,#190743,#190744),(#190745,#190746,#190747),
(#190748,#190749,#190750),(#190751,#190752,#190753),(#190754,#190755,#190756)),
 .UNSPECIFIED.,.F.,.F.,.F.)
B_SPLINE_SURFACE_WITH_KNOTS((4,2,2,4),(3,3),(-2.40757934422131E-15,0.000787383129295151,
0.00157476625859271,0.00314953251718783),(0.,1.),.UNSPECIFIED.)
GEOMETRIC_REPRESENTATION_ITEM()
RATIONAL_B_SPLINE_SURFACE(((1.,0.989234343678173,1.),(1.,0.988443605143724,
1.),(1.,0.984599769902277,1.),(1.,0.971863446961927,1.),(1.,0.962926004132788,
1.),(1.,0.929467293227288,1.),(1.,0.898004938874792,1.),(1.,0.857972509692102,
1.)))
REPRESENTATION_ITEM('')
SURFACE()
);
#2953=(
BOUNDED_SURFACE()
B_SPLINE_SURFACE(3,2,((#190776,#190777,#190778),(#190779,#190780,#190781),
(#190782,#190783,#190784),(#190785,#190786,#190787),(#190788,#190789,#190790),
(#190791,#190792,#190793),(#190794,#190795,#190796),(#190797,#190798,#190799)),
 .UNSPECIFIED.,.F.,.F.,.F.)
B_SPLINE_SURFACE_WITH_KNOTS((4,2,2,4),(3,3),(2.16840434497101E-19,0.00157702467408662,
0.00236553701112993,0.00315404934817324),(0.,1.),.UNSPECIFIED.)
GEOMETRIC_REPRESENTATION_ITEM()
RATIONAL_B_SPLINE_SURFACE(((1.,0.857104357126295,1.),(1.,0.897186993221649,
1.),(1.,0.928714693488658,1.),(1.,0.962508133039243,1.),(1.,0.971517540750285,
1.),(1.,0.984393580256014,1.),(1.,0.988371316630897,1.),(1.,0.989172917436462,
1.)))
REPRESENTATION_ITEM('')
SURFACE()
);
#2954=(
BOUNDED_SURFACE()
B_SPLINE_SURFACE(3,2,((#190819,#190820,#190821),(#190822,#190823,#190824),
(#190825,#190826,#190827),(#190828,#190829,#190830),(#190831,#190832,#190833),
(#190834,#190835,#190836),(#190837,#190838,#190839),(#190840,#190841,#190842),
(#190843,#190844,#190845),(#190846,#190847,#190848),(#190849,#190850,#190851),
(#190852,#190853,#190854),(#190855,#190856,#190857),(#190858,#190859,#190860),
(#190861,#190862,#190863),(#190864,#190865,#190866),(#190867,#190868,#190869),
(#190870,#190871,#190872)),.UNSPECIFIED.,.F.,.F.,.F.)
B_SPLINE_SURFACE_WITH_KNOTS((4,2,2,2,2,2,2,2,4),(3,3),(-0.000508741685376785,
0.00254370842688261,0.00381556264032431,0.00445148974704516,0.00476945330040559,
0.0049284350770858,0.00500792596542591,0.00504767140959596,0.0055961585391427),
(0.,1.00567142871774),.UNSPECIFIED.)
GEOMETRIC_REPRESENTATION_ITEM()
RATIONAL_B_SPLINE_SURFACE(((1.,0.988073899798154,1.00013527605435),(1.,
0.990274117753828,1.00011031929575),(1.,0.992465877278408,1.00008545847993),
(1.,0.995553721434854,1.00005043350388),(1.,0.996459905831034,1.00004015478347),
(1.,0.997814118238599,1.00002479414519),(1.,0.998264976714179,1.00001968012178),
(1.,0.99893609089222,1.00001206776933),(1.,0.999159203039956,1.00000953704005),
(1.,0.999488994833662,1.00000579625875),(1.,0.999598301582193,1.00000455640789),
(1.,0.999757142399174,1.00000275469914),(1.,0.999809501617783,1.00000216079599),
(1.,0.999882023724343,1.00000133818808),(1.,0.999905504951442,1.00000107184386),
(1.,1.00019880923877,0.999997744935148),(1.,0.999814228249837,1.00000210718248),
(1.,0.965387876575238,1.00039260038155)))
REPRESENTATION_ITEM('')
SURFACE()
);
#2955=(
BOUNDED_SURFACE()
B_SPLINE_SURFACE(3,2,((#190912,#190913,#190914),(#190915,#190916,#190917),
(#190918,#190919,#190920),(#190921,#190922,#190923),(#190924,#190925,#190926),
(#190927,#190928,#190929),(#190930,#190931,#190932),(#190933,#190934,#190935),
(#190936,#190937,#190938),(#190939,#190940,#190941),(#190942,#190943,#190944),
(#190945,#190946,#190947),(#190948,#190949,#190950),(#190951,#190952,#190953),
(#190954,#190955,#190956),(#190957,#190958,#190959),(#190960,#190961,#190962),
(#190963,#190964,#190965)),.UNSPECIFIED.,.F.,.F.,.F.)
B_SPLINE_SURFACE_WITH_KNOTS((4,2,2,2,2,2,2,2,4),(3,3),(-7.45388993583784E-20,
4.05793239028379E-5,8.11586478056759E-5,0.000162317295611352,0.000324634591222704,
0.000649269182445408,0.00129853836489082,0.00259707672978163,0.00519415345956326),
(0.,1.),.UNSPECIFIED.)
GEOMETRIC_REPRESENTATION_ITEM()
RATIONAL_B_SPLINE_SURFACE(((1.,0.999961923064171,1.),(1.,0.999961833753432,
1.),(1.,0.999944633098586,1.),(1.,0.999904212270329,1.),(1.,0.99988023258917,
1.),(1.,0.999806855851567,1.),(1.,0.999754783512162,1.),(1.,0.999595776401296,
1.),(1.,0.999485889992571,1.),(1.,0.999156267866573,1.),(1.,0.998933623645324,
1.),(1.,0.998262897761582,1.),(1.,0.997812273447783,1.),(1.,0.996459235447427,
1.),(1.,0.995553264664008,1.),(1.,0.992828768547989,1.),(1.,0.991003554465269,
1.),(1.,0.989172917436461,1.)))
REPRESENTATION_ITEM('')
SURFACE()
);
#2956=(
BOUNDED_SURFACE()
B_SPLINE_SURFACE(3,2,((#191015,#191016,#191017),(#191018,#191019,#191020),
(#191021,#191022,#191023),(#191024,#191025,#191026),(#191027,#191028,#191029),
(#191030,#191031,#191032),(#191033,#191034,#191035),(#191036,#191037,#191038),
(#191039,#191040,#191041),(#191042,#191043,#191044),(#191045,#191046,#191047),
(#191048,#191049,#191050),(#191051,#191052,#191053),(#191054,#191055,#191056),
(#191057,#191058,#191059),(#191060,#191061,#191062),(#191063,#191064,#191065),
(#191066,#191067,#191068)),.UNSPECIFIED.,.F.,.F.,.F.)
B_SPLINE_SURFACE_WITH_KNOTS((4,2,2,2,2,2,2,2,4),(3,3),(-0.000525941938450675,
0.00262970969225337,0.00394456453838006,0.00460199196144341,0.00493070567297508,
0.00509506252874091,0.00517724095662383,0.00521833017056529,0.00578536132295742),
(0.,1.00671701195453),.UNSPECIFIED.)
GEOMETRIC_REPRESENTATION_ITEM()
RATIONAL_B_SPLINE_SURFACE(((1.,0.987652440486347,1.00016587740972),(1.,
0.989930475499347,1.00013527423289),(1.,0.992199484515042,1.00010479231153),
(1.,0.995396092253403,1.00006184900674),(1.,0.996334181463897,1.00004924669386),
(1.,0.997736167759121,1.00003041237645),(1.,0.998202686027925,1.00002414515887),
(1.,0.998897407157577,1.00001481225861),(1.,0.999128412532823,1.00001170892687),
(1.,0.999469951933241,1.0000071206784),(1.,0.999583268571811,1.00000559837997),
(1.,0.999747958495426,1.0000033859316),(1.,0.999802181877435,1.00000265749339),
(1.,0.999877976982937,1.00000163926013),(1.,0.999902135273186,1.00000131471708),
(1.,1.000210891347,0.999997166880602),(1.,0.999880980100307,1.00000159891618),
(1.,0.96165859498486,1.00051507935168)))
REPRESENTATION_ITEM('')
SURFACE()
);
#2957=(
BOUNDED_SURFACE()
B_SPLINE_SURFACE(3,2,((#191117,#191118,#191119),(#191120,#191121,#191122),
(#191123,#191124,#191125),(#191126,#191127,#191128),(#191129,#191130,#191131),
(#191132,#191133,#191134),(#191135,#191136,#191137),(#191138,#191139,#191140)),
 .UNSPECIFIED.,.F.,.F.,.F.)
B_SPLINE_SURFACE_WITH_KNOTS((4,2,2,4),(3,3),(0.,0.000786373253240854,0.0015727465064817,
0.00314549301296342),(0.,1.),.UNSPECIFIED.)
GEOMETRIC_REPRESENTATION_ITEM()
RATIONAL_B_SPLINE_SURFACE(((1.,0.988865480076014,1.),(1.,0.988061700311495,
1.),(1.,0.984209057857027,1.),(1.,0.971450599512814,1.),(1.,0.962500813802613,
1.),(1.,0.929017994266129,1.),(1.,0.897560549282588,1.),(1.,0.857509777230937,
1.)))
REPRESENTATION_ITEM('')
SURFACE()
);
#2958=(
BOUNDED_SURFACE()
B_SPLINE_SURFACE(3,2,((#191160,#191161,#191162),(#191163,#191164,#191165),
(#191166,#191167,#191168),(#191169,#191170,#191171),(#191172,#191173,#191174),
(#191175,#191176,#191177),(#191178,#191179,#191180),(#191181,#191182,#191183),
(#191184,#191185,#191186),(#191187,#191188,#191189),(#191190,#191191,#191192),
(#191193,#191194,#191195),(#191196,#191197,#191198),(#191199,#191200,#191201),
(#191202,#191203,#191204),(#191205,#191206,#191207),(#191208,#191209,#191210),
(#191211,#191212,#191213)),.UNSPECIFIED.,.F.,.F.,.F.)
B_SPLINE_SURFACE_WITH_KNOTS((4,2,2,2,2,2,2,2,4),(3,3),(-1.32137139771671E-19,
4.17669388829254E-5,8.35338777658508E-5,0.000167067755531702,0.000334135511063404,
0.000668271022126808,0.00133654204425361,0.00267308408850723,0.00534616817701446),
(0.,1.),.UNSPECIFIED.)
GEOMETRIC_REPRESENTATION_ITEM()
RATIONAL_B_SPLINE_SURFACE(((1.,0.999961923064171,1.),(1.,0.999961782802257,
1.),(1.,0.999943671528414,1.),(1.,0.999901604878771,1.),(1.,0.999876750335241,
1.),(1.,0.999800908054986,1.),(1.,0.99974715657318,1.),(1.,0.999583072363253,
1.),(1.,0.999469900307565,1.),(1.,0.999130340955253,1.),(1.,0.998901033022514,
1.),(1.,0.998210264756137,1.),(1.,0.997746391825068,1.),(1.,0.996353373847482,
1.),(1.,0.9954206326127,1.),(1.,0.992615540215937,1.),(1.,0.990736373728666,
1.),(1.,0.988851372352096,1.)))
REPRESENTATION_ITEM('')
SURFACE()
);
#2959=(
BOUNDED_SURFACE()
B_SPLINE_SURFACE(3,2,((#191260,#191261,#191262),(#191263,#191264,#191265),
(#191266,#191267,#191268),(#191269,#191270,#191271)),.UNSPECIFIED.,.F.,
 .F.,.F.)
B_SPLINE_SURFACE_WITH_KNOTS((4,4),(3,3),(-1.85521401386541E-5,0.00125436719122141),
(0.,1.00001918161636),.UNSPECIFIED.)
GEOMETRIC_REPRESENTATION_ITEM()
RATIONAL_B_SPLINE_SURFACE(((1.,0.837815237008462,1.0000062219318),(1.,0.84540513832919,
1.00000593075865),(1.,0.852052930826092,1.00000567572784),(1.,0.857765949207726,
1.00000545655799)))
REPRESENTATION_ITEM('')
SURFACE()
);
#2960=(
BOUNDED_SURFACE()
B_SPLINE_SURFACE(3,2,((#191295,#191296,#191297),(#191298,#191299,#191300),
(#191301,#191302,#191303),(#191304,#191305,#191306),(#191307,#191308,#191309),
(#191310,#191311,#191312),(#191313,#191314,#191315),(#191316,#191317,#191318)),
 .UNSPECIFIED.,.F.,.F.,.F.)
B_SPLINE_SURFACE_WITH_KNOTS((4,2,2,4),(3,3),(8.13151629364128E-20,0.00157235613934946,
0.00235853420902418,0.00314471227869891),(0.,1.),.UNSPECIFIED.)
GEOMETRIC_REPRESENTATION_ITEM()
RATIONAL_B_SPLINE_SURFACE(((1.,0.857407773863101,1.),(1.,0.897293426532578,
1.),(1.,0.928679392158714,1.),(1.,0.962320286971746,1.),(1.,0.971291611639875,
1.),(1.,0.984107082217988,1.),(1.,0.988059746314391,1.),(1.,0.988851372352099,
1.)))
REPRESENTATION_ITEM('')
SURFACE()
);
#2961=(
BOUNDED_SURFACE()
B_SPLINE_SURFACE(3,2,((#191348,#191349,#191350),(#191351,#191352,#191353),
(#191354,#191355,#191356),(#191357,#191358,#191359)),.UNSPECIFIED.,.F.,
 .F.,.F.)
B_SPLINE_SURFACE_WITH_KNOTS((4,4),(3,3),(0.,0.000753104234298227),(0.,1.),
 .UNSPECIFIED.)
GEOMETRIC_REPRESENTATION_ITEM()
RATIONAL_B_SPLINE_SURFACE(((1.,0.839275484760762,1.),(1.,0.838901603374917,
1.),(1.,0.838526082980222,1.),(1.,0.83814959787298,1.)))
REPRESENTATION_ITEM('')
SURFACE()
);
#2962=(
BOUNDED_SURFACE()
B_SPLINE_SURFACE(3,2,((#191365,#191366,#191367),(#191368,#191369,#191370),
(#191371,#191372,#191373),(#191374,#191375,#191376)),.UNSPECIFIED.,.F.,
 .F.,.F.)
B_SPLINE_SURFACE_WITH_KNOTS((4,4),(3,3),(0.,0.00121469382512386),(0.,1.),
 .UNSPECIFIED.)
GEOMETRIC_REPRESENTATION_ITEM()
RATIONAL_B_SPLINE_SURFACE(((1.,0.857407773863101,1.),(1.,0.851918824817362,
1.),(1.,0.845578741226857,1.),(1.,0.83838293312654,1.)))
REPRESENTATION_ITEM('')
SURFACE()
);
#2963=(
BOUNDED_SURFACE()
B_SPLINE_SURFACE(3,2,((#191397,#191398,#191399),(#191400,#191401,#191402),
(#191403,#191404,#191405),(#191406,#191407,#191408),(#191409,#191410,#191411),
(#191412,#191413,#191414),(#191415,#191416,#191417),(#191418,#191419,#191420),
(#191421,#191422,#191423),(#191424,#191425,#191426),(#191427,#191428,#191429),
(#191430,#191431,#191432),(#191433,#191434,#191435),(#191436,#191437,#191438)),
 .UNSPECIFIED.,.F.,.F.,.F.)
B_SPLINE_SURFACE_WITH_KNOTS((4,2,2,2,2,2,4),(3,3),(-0.000226840284413293,
0.000567100711032879,0.000850651066549369,0.00113420142206586,0.00141775177758235,
0.00170130213309884,0.00249524312854497),(-0.000282176477353801,1.00009539139101),
 .UNSPECIFIED.)
GEOMETRIC_REPRESENTATION_ITEM()
RATIONAL_B_SPLINE_SURFACE(((1.00010528003724,0.813432211160089,1.0000355838799),
(1.00008775714205,0.844484705969625,1.00002966126993),(1.00007212354181,
0.872189162633845,1.00002437722779),(1.00005392748604,0.90443457190974,
1.00001822709449),(1.0000494556467,0.912359162369374,1.00001671564561),
(1.00004150285258,0.926452386996823,1.00001402765957),(1.00003795528609,
0.932739064433654,1.00001282860813),(1.00003236888526,0.942638780270556,
1.00001094044565),(1.00003027209024,0.946354531320264,1.00001023174432),
(1.00002812425189,0.950160736773148,1.00000950579073),(1.00002807138552,
0.950254421792609,1.00000948792228),(1.00003175744819,0.943722313910005,
1.00001073378441),(1.00004241856759,0.924829639419119,1.00001433716452),
(1.00005485908397,0.902783678063587,1.00001854196775)))
REPRESENTATION_ITEM('')
SURFACE()
);
#2964=(
BOUNDED_SURFACE()
B_SPLINE_SURFACE(3,2,((#191537,#191538,#191539),(#191540,#191541,#191542),
(#191543,#191544,#191545),(#191546,#191547,#191548)),.UNSPECIFIED.,.F.,
 .F.,.F.)
B_SPLINE_SURFACE_WITH_KNOTS((4,4),(3,3),(0.,0.000758627814399393),(0.,1.),
 .UNSPECIFIED.)
GEOMETRIC_REPRESENTATION_ITEM()
RATIONAL_B_SPLINE_SURFACE(((1.,0.838382933127103,1.),(1.,0.838759998356351,
1.),(1.,0.839135655634363,1.),(1.,0.839509576764081,1.)))
REPRESENTATION_ITEM('')
SURFACE()
);
#2965=(
BOUNDED_SURFACE()
B_SPLINE_SURFACE(3,2,((#191554,#191555,#191556),(#191557,#191558,#191559),
(#191560,#191561,#191562),(#191563,#191564,#191565),(#191566,#191567,#191568),
(#191569,#191570,#191571),(#191572,#191573,#191574),(#191575,#191576,#191577),
(#191578,#191579,#191580),(#191581,#191582,#191583),(#191584,#191585,#191586),
(#191587,#191588,#191589)),.UNSPECIFIED.,.F.,.F.,.F.)
B_SPLINE_SURFACE_WITH_KNOTS((4,2,2,2,2,4),(3,3),(-0.000216256680534375,
0.000582607613633213,0.000867916290121638,0.00115322496661006,0.00172384231958692,
0.00252270661375451),(-0.000244207734780689,1.),.UNSPECIFIED.)
GEOMETRIC_REPRESENTATION_ITEM()
RATIONAL_B_SPLINE_SURFACE(((1.00004816059777,0.901394200701356,1.),(1.00003731388615,
0.923602161531115,1.),(1.00002813164864,0.942402216152368,1.),(1.00002468431679,
0.94946041162475,1.),(1.00002465107978,0.949528462309686,1.),(1.00002636666531,
0.946015908672132,1.),(1.00002810233345,0.942462237161793,1.),(1.00003527537775,
0.927775879444964,1.),(1.0000424644099,0.913056787614755,1.),(1.0000622011378,
0.872647076777095,1.),(1.00007580610643,0.844791757926684,1.),(1.00009107581698,
0.813527984557883,1.)))
REPRESENTATION_ITEM('')
SURFACE()
);
#2966=(
BOUNDED_SURFACE()
B_SPLINE_SURFACE(2,2,((#191642,#191643,#191644),(#191645,#191646,#191647),
(#191648,#191649,#191650)),.UNSPECIFIED.,.F.,.F.,.F.)
B_SPLINE_SURFACE_WITH_KNOTS((3,3),(3,3),(1.74317346290508E-16,1.57079632679495),
(-0.736541846753928,0.787072384273275),.UNSPECIFIED.)
GEOMETRIC_REPRESENTATION_ITEM()
RATIONAL_B_SPLINE_SURFACE(((1.,0.723589867251388,1.),(0.707106781186616,
0.51165530193138,0.707106781186616),(1.,0.723589867251388,1.)))
REPRESENTATION_ITEM('')
SURFACE()
);
#2967=(
BOUNDED_SURFACE()
B_SPLINE_SURFACE(2,2,((#191663,#191664,#191665),(#191666,#191667,#191668),
(#191669,#191670,#191671)),.UNSPECIFIED.,.F.,.F.,.F.)
B_SPLINE_SURFACE_WITH_KNOTS((3,3),(3,3),(-1.74317346290519E-16,1.57079632679496),
(-2.35452026931659,-0.830906038289448),.UNSPECIFIED.)
GEOMETRIC_REPRESENTATION_ITEM()
RATIONAL_B_SPLINE_SURFACE(((1.,0.72358986725141,1.),(0.707106781186587,
0.511655301931375,0.707106781186587),(1.,0.72358986725141,1.)))
REPRESENTATION_ITEM('')
SURFACE()
);
#2968=(
BOUNDED_SURFACE()
B_SPLINE_SURFACE(2,2,((#191686,#191687,#191688),(#191689,#191690,#191691),
(#191692,#191693,#191694)),.UNSPECIFIED.,.F.,.F.,.F.)
B_SPLINE_SURFACE_WITH_KNOTS((3,3),(3,3),(1.81714697791953E-16,1.57079632679495),
(-0.74383310368946,0.26549733202973),.UNSPECIFIED.)
GEOMETRIC_REPRESENTATION_ITEM()
RATIONAL_B_SPLINE_SURFACE(((1.,0.875336395469216,1.),(0.707106781186606,
0.618956301055724,0.707106781186606),(1.,0.875336395469216,1.)))
REPRESENTATION_ITEM('')
SURFACE()
);
#2969=(
BOUNDED_SURFACE()
B_SPLINE_SURFACE(2,2,((#191706,#191707,#191708),(#191709,#191710,#191711),
(#191712,#191713,#191714)),.UNSPECIFIED.,.F.,.F.,.F.)
B_SPLINE_SURFACE_WITH_KNOTS((3,3),(3,3),(-6.30291942997115E-17,1.57079632679495),
(-1.82889777036346,-0.819567334644225),.UNSPECIFIED.)
GEOMETRIC_REPRESENTATION_ITEM()
RATIONAL_B_SPLINE_SURFACE(((1.,0.875336395469206,1.),(0.707106781186601,
0.618956301055712,0.707106781186601),(1.,0.875336395469206,1.)))
REPRESENTATION_ITEM('')
SURFACE()
);
#2970=(
BOUNDED_SURFACE()
B_SPLINE_SURFACE(2,2,((#191729,#191730,#191731),(#191732,#191733,#191734),
(#191735,#191736,#191737)),.UNSPECIFIED.,.F.,.F.,.F.)
B_SPLINE_SURFACE_WITH_KNOTS((3,3),(3,3),(-1.57079632679491,1.68131336473773E-16),
(-1.83117576062825,-0.821845324909055),.UNSPECIFIED.)
GEOMETRIC_REPRESENTATION_ITEM()
RATIONAL_B_SPLINE_SURFACE(((1.,0.875336395469216,1.),(0.70710678118653,
0.618956301055656,0.70710678118653),(1.,0.875336395469216,1.)))
REPRESENTATION_ITEM('')
SURFACE()
);
#2971=(
BOUNDED_SURFACE()
B_SPLINE_SURFACE(2,2,((#191749,#191750,#191751),(#191752,#191753,#191754),
(#191755,#191756,#191757)),.UNSPECIFIED.,.F.,.F.,.F.)
B_SPLINE_SURFACE_WITH_KNOTS((3,3),(3,3),(-1.5707963267949,2.47147205475768E-16),
(-0.746111093954295,0.263219341764958),.UNSPECIFIED.)
GEOMETRIC_REPRESENTATION_ITEM()
RATIONAL_B_SPLINE_SURFACE(((1.,0.875336395469201,1.),(0.707106781186519,
0.618956301055637,0.707106781186519),(1.,0.875336395469201,1.)))
REPRESENTATION_ITEM('')
SURFACE()
);
#2972=(
BOUNDED_SURFACE()
B_SPLINE_SURFACE(2,2,((#191772,#191773,#191774),(#191775,#191776,#191777),
(#191778,#191779,#191780)),.UNSPECIFIED.,.F.,.F.,.F.)
B_SPLINE_SURFACE_WITH_KNOTS((3,3),(3,3),(-1.57079632679491,1.67905497988288E-16),
(-2.34670754812599,-0.823093317098874),.UNSPECIFIED.)
GEOMETRIC_REPRESENTATION_ITEM()
RATIONAL_B_SPLINE_SURFACE(((1.,0.723589867251417,1.),(0.70710678118653,
0.511655301931338,0.70710678118653),(1.,0.723589867251417,1.)))
REPRESENTATION_ITEM('')
SURFACE()
);
#2973=(
BOUNDED_SURFACE()
B_SPLINE_SURFACE(2,2,((#191792,#191793,#191794),(#191795,#191796,#191797),
(#191798,#191799,#191800)),.UNSPECIFIED.,.F.,.F.,.F.)
B_SPLINE_SURFACE_WITH_KNOTS((3,3),(3,3),(-1.57079632679491,2.478375474118E-16),
(-0.728729125563299,0.794885105463935),.UNSPECIFIED.)
GEOMETRIC_REPRESENTATION_ITEM()
RATIONAL_B_SPLINE_SURFACE(((1.,0.723589867251377,1.),(0.70710678118653,
0.511655301931309,0.70710678118653),(1.,0.723589867251377,1.)))
REPRESENTATION_ITEM('')
SURFACE()
);
#2974=(
BOUNDED_SURFACE()
B_SPLINE_SURFACE(3,2,((#193720,#193721,#193722),(#193723,#193724,#193725),
(#193726,#193727,#193728),(#193729,#193730,#193731),(#193732,#193733,#193734),
(#193735,#193736,#193737),(#193738,#193739,#193740),(#193741,#193742,#193743),
(#193744,#193745,#193746),(#193747,#193748,#193749),(#193750,#193751,#193752),
(#193753,#193754,#193755),(#193756,#193757,#193758),(#193759,#193760,#193761),
(#193762,#193763,#193764),(#193765,#193766,#193767),(#193768,#193769,#193770),
(#193771,#193772,#193773),(#193774,#193775,#193776),(#193777,#193778,#193779),
(#193780,#193781,#193782),(#193783,#193784,#193785),(#193786,#193787,#193788),
(#193789,#193790,#193791),(#193792,#193793,#193794),(#193795,#193796,#193797),
(#193798,#193799,#193800),(#193801,#193802,#193803),(#193804,#193805,#193806),
(#193807,#193808,#193809),(#193810,#193811,#193812),(#193813,#193814,#193815),
(#193816,#193817,#193818),(#193819,#193820,#193821),(#193822,#193823,#193824),
(#193825,#193826,#193827),(#193828,#193829,#193830),(#193831,#193832,#193833),
(#193834,#193835,#193836),(#193837,#193838,#193839),(#193840,#193841,#193842),
(#193843,#193844,#193845),(#193846,#193847,#193848),(#193849,#193850,#193851),
(#193852,#193853,#193854),(#193855,#193856,#193857),(#193858,#193859,#193860),
(#193861,#193862,#193863)),.UNSPECIFIED.,.F.,.F.,.F.)
B_SPLINE_SURFACE_WITH_KNOTS((4,2,2,2,2,2,2,2,2,2,2,2,2,2,2,2,2,2,2,2,2,
2,2,4),(3,3),(0.,0.0059149619404375,0.00739370242554688,0.00743991306570655,
0.00748612370586621,0.00757854498618555,0.00776338754682422,0.00813307266810157,
0.00887244291065625,0.011829923880875,0.0133086643659844,0.0140480346085391,
0.0140942452486987,0.0141404558888584,0.0142328771691777,0.0144177197298164,
0.0147874048510938,0.0177448858213125,0.0192236263064219,0.0199629965489765,
0.0201478391096152,0.0203326816702539,0.0207023667915313,0.02365984776175),
(-0.000128696703876237,1.),.UNSPECIFIED.)
GEOMETRIC_REPRESENTATION_ITEM()
RATIONAL_B_SPLINE_SURFACE(((1.00003576453942,0.861051066802645,1.),(1.00003300380643,
0.871776799904612,1.),(1.00003114473836,0.878999471558354,1.),(1.00002957069443,
0.885114794930814,1.),(1.0000292946172,0.886187383506178,1.),(1.00002904679648,
0.887150192641286,1.),(1.00002905930675,0.887101588964017,1.),(1.00002907039925,
0.88705849344574,1.),(1.00002907595876,0.887036894169038,1.),(1.0000290926768,
0.886971942860521,1.),(1.00002910387483,0.886928437357747,1.),(1.00002913762479,
0.886797315265569,1.),(1.00002916033256,0.886709093220405,1.),(1.00002922906338,
0.886442066884952,1.),(1.00002927569335,0.886260904621482,1.),(1.00002941790449,
0.885708399652157,1.),(1.00002951579679,0.885328077943985,1.),(1.00003001983054,
0.883369854726223,1.),(1.0000304754155,0.881599860064861,1.),(1.00003124833757,
0.878596977882908,1.),(1.00003152026012,0.877540530673196,1.),(1.00003195407994,
0.875855095812049,1.),(1.00003210266429,0.875277830252333,1.),(1.00003226456337,
0.874648835593434,1.),(1.00003223907406,0.874747864199818,1.),(1.00003222073887,
0.87481909833159,1.),(1.00003221161445,0.874854547615397,1.),(1.00003218436966,
0.874960396475737,1.),(1.00003216637769,0.875030297104221,1.),(1.00003211290697,
0.875238036387284,1.),(1.0000320779332,0.87537391310078,1.),(1.00003197496994,
0.875773936029893,1.),(1.00003190893599,0.876030484733642,1.),(1.00003133689918,
0.878252906904018,1.),(1.00003098535817,0.879618680051682,1.),(1.00003066804144,
0.880851488372246,1.),(1.00003059686398,0.881128020145932,1.),(1.00003054204845,
0.88134098415604,1.),(1.00003053232869,0.881378746411579,1.),(1.00003053090852,
0.881384263936795,1.),(1.00003053116352,0.881383273219239,1.),(1.00003053276312,
0.881377058605224,1.),(1.00003053808665,0.881356376158469,1.),(1.00003051977626,
0.881427513909725,1.),(1.00003050821747,0.881472421022649,1.),(1.00003041011411,
0.88185356269165,1.),(1.0000303659271,0.882025233799165,1.),(1.00003036612293,
0.882024472999063,1.)))
REPRESENTATION_ITEM('')
SURFACE()
);
#2975=(
BOUNDED_SURFACE()
B_SPLINE_SURFACE(3,2,((#194043,#194044,#194045),(#194046,#194047,#194048),
(#194049,#194050,#194051),(#194052,#194053,#194054)),.UNSPECIFIED.,.F.,
 .F.,.F.)
B_SPLINE_SURFACE_WITH_KNOTS((4,4),(3,3),(1.0842021724855E-19,0.000322395538615675),
(0.,1.),.UNSPECIFIED.)
GEOMETRIC_REPRESENTATION_ITEM()
RATIONAL_B_SPLINE_SURFACE(((1.,0.861068946771251,1.),(1.,0.868023491094222,
1.),(1.,0.874094710294855,1.),(1.,0.879223463974629,1.)))
REPRESENTATION_ITEM('')
SURFACE()
);
#2976=(
BOUNDED_SURFACE()
B_SPLINE_SURFACE(3,2,((#194066,#194067,#194068),(#194069,#194070,#194071),
(#194072,#194073,#194074),(#194075,#194076,#194077)),.UNSPECIFIED.,.F.,
 .F.,.F.)
B_SPLINE_SURFACE_WITH_KNOTS((4,4),(3,3),(-1.56125112837912E-17,0.00371972595076131),
(0.,1.),.UNSPECIFIED.)
GEOMETRIC_REPRESENTATION_ITEM()
RATIONAL_B_SPLINE_SURFACE(((1.,0.879223463974645,1.),(1.,0.879197541860131,
1.),(1.,0.879166735457461,1.),(1.,0.879131676488835,1.)))
REPRESENTATION_ITEM('')
SURFACE()
);
#2977=(
BOUNDED_SURFACE()
B_SPLINE_SURFACE(3,2,((#194083,#194084,#194085),(#194086,#194087,#194088),
(#194089,#194090,#194091),(#194092,#194093,#194094),(#194095,#194096,#194097),
(#194098,#194099,#194100),(#194101,#194102,#194103),(#194104,#194105,#194106),
(#194107,#194108,#194109),(#194110,#194111,#194112),(#194113,#194114,#194115),
(#194116,#194117,#194118),(#194119,#194120,#194121),(#194122,#194123,#194124),
(#194125,#194126,#194127),(#194128,#194129,#194130),(#194131,#194132,#194133),
(#194134,#194135,#194136),(#194137,#194138,#194139),(#194140,#194141,#194142),
(#194143,#194144,#194145),(#194146,#194147,#194148),(#194149,#194150,#194151),
(#194152,#194153,#194154),(#194155,#194156,#194157),(#194158,#194159,#194160)),
 .UNSPECIFIED.,.F.,.F.,.F.)
B_SPLINE_SURFACE_WITH_KNOTS((4,2,2,2,2,2,2,2,2,2,2,2,4),(3,3),(0.,0.000191440896835587,
0.00028716134525338,0.000382881793671173,0.00057432269050676,0.000670043138924553,
0.000765763587342347,0.000957204484177933,0.00114864538101352,0.00124436582943131,
0.00129222605364021,0.00134008627784911,0.00153152717468469),(0.,1.),
 .UNSPECIFIED.)
GEOMETRIC_REPRESENTATION_ITEM()
RATIONAL_B_SPLINE_SURFACE(((1.,0.879131676489345,1.),(1.,0.880626887596785,
1.),(1.,0.882841814432506,1.),(1.,0.886761296901068,1.),(1.,0.888121788557817,
1.),(1.,0.890288150019219,1.),(1.,0.891026608347966,1.),(1.,0.892657535905197,
1.),(1.,0.894092695678742,1.),(1.,0.897075330661339,1.),(1.,0.898026040345514,
1.),(1.,0.899562222232299,1.),(1.,0.900146620417538,1.),(1.,0.901818107518504,
1.),(1.,0.902658365336305,1.),(1.,0.905247057738554,1.),(1.,0.906646088930788,
1.),(1.,0.907839183414567,1.),(1.,0.908162443627513,1.),(1.,0.90858816846029,
1.),(1.,0.908692441152182,1.),(1.,0.909187146997205,1.),(1.,0.909555346803908,
1.),(1.,0.911583034137221,1.),(1.,0.912990115533129,1.),(1.,0.913476533865317,
1.)))
REPRESENTATION_ITEM('')
SURFACE()
);
#2978=(
BOUNDED_SURFACE()
B_SPLINE_SURFACE(3,2,((#194227,#194228,#194229),(#194230,#194231,#194232),
(#194233,#194234,#194235),(#194236,#194237,#194238),(#194239,#194240,#194241),
(#194242,#194243,#194244),(#194245,#194246,#194247),(#194248,#194249,#194250),
(#194251,#194252,#194253),(#194254,#194255,#194256),(#194257,#194258,#194259),
(#194260,#194261,#194262)),.UNSPECIFIED.,.F.,.F.,.F.)
B_SPLINE_SURFACE_WITH_KNOTS((4,2,2,2,2,4),(3,3),(-0.000409539429897566,
0.00646885457540742,0.0129377091508148,0.0161721364385186,0.0194065637262222,
0.0262849577315271),(0.,1.0004095394299),.UNSPECIFIED.)
GEOMETRIC_REPRESENTATION_ITEM()
RATIONAL_B_SPLINE_SURFACE(((1.,0.913179721902361,1.00007111265439),(1.,
0.914649363023394,1.00006990890242),(1.,0.916017546687799,1.0000687882521),
(1.,0.918006651041594,1.00006715901878),(1.,0.918577734918004,1.00006669125605),
(1.,0.918977605127172,1.00006636373081),(1.,0.919016659308045,1.00006633174236),
(1.,0.918937808682391,1.00006639632724),(1.,0.918820432299286,1.00006649246775),
(1.,0.918221056281877,1.00006698340398),(1.,0.917500522000491,1.00006757357837),
(0.999999999999999,0.916883429763216,1.00006807902558)))
REPRESENTATION_ITEM('')
SURFACE()
);
#2979=(
BOUNDED_SURFACE()
B_SPLINE_SURFACE(3,2,((#194367,#194368,#194369),(#194370,#194371,#194372),
(#194373,#194374,#194375),(#194376,#194377,#194378),(#194379,#194380,#194381),
(#194382,#194383,#194384),(#194385,#194386,#194387),(#194388,#194389,#194390),
(#194391,#194392,#194393),(#194394,#194395,#194396),(#194397,#194398,#194399),
(#194400,#194401,#194402),(#194403,#194404,#194405),(#194406,#194407,#194408),
(#194409,#194410,#194411),(#194412,#194413,#194414),(#194415,#194416,#194417),
(#194418,#194419,#194420),(#194421,#194422,#194423),(#194424,#194425,#194426),
(#194427,#194428,#194429),(#194430,#194431,#194432),(#194433,#194434,#194435),
(#194436,#194437,#194438),(#194439,#194440,#194441),(#194442,#194443,#194444),
(#194445,#194446,#194447),(#194448,#194449,#194450),(#194451,#194452,#194453),
(#194454,#194455,#194456),(#194457,#194458,#194459),(#194460,#194461,#194462),
(#194463,#194464,#194465),(#194466,#194467,#194468)),.UNSPECIFIED.,.F.,
 .F.,.F.)
B_SPLINE_SURFACE_WITH_KNOTS((4,2,2,2,2,2,2,2,2,2,2,2,2,2,2,2,4),(3,3),(0.,
0.000127304511784401,0.000254609023568802,0.000318261279461002,0.000381913535353202,
0.000509218047137603,0.000636522558922004,0.000763827070706405,0.000891131582490806,
0.00101843609427521,0.00114574060605961,0.00127304511784401,0.00140034962962841,
0.00152765414141281,0.00165495865319721,0.00178226316498161,0.00203687218855042),
(0.,1.),.UNSPECIFIED.)
GEOMETRIC_REPRESENTATION_ITEM()
RATIONAL_B_SPLINE_SURFACE(((1.,0.91702864701937,1.),(1.,0.916747691343526,
1.),(1.,0.916396650974015,1.),(1.,0.915391285047532,1.),(1.,0.91466902297872,
1.),(1.,0.913617961828943,1.),(1.,0.913301894872966,1.),(1.,0.91288722963512,
1.),(1.,0.912808085796895,1.),(1.,0.912445288290209,1.),(1.,0.912155502184342,
1.),(1.,0.911390085208123,1.),(1.,0.910897099188983,1.),(1.,0.909571313750726,
1.),(1.,0.908903094531974,1.),(1.,0.907795271007775,1.),(1.,0.907436030525757,
1.),(1.,0.9066073942613,1.),(1.,0.906098571567135,1.),(1.,0.904785338999927,
1.),(1.,0.903901015235201,1.),(1.,0.9022896096654,1.),(1.,0.90153583977931,
1.),(1.,0.900209640235172,1.),(1.,0.899552878447653,1.),(1.,0.897909996734079,
1.),(1.,0.896964437998137,1.),(1.,0.894976204823856,1.),(1.,0.894010134201253,
1.),(1.,0.892205555807536,1.),(1.,0.89146980148389,1.),(1.,0.88870491520376,
1.),(1.,0.885769567646591,1.),(1.,0.884000563436218,1.)))
REPRESENTATION_ITEM('')
SURFACE()
);
#2980=(
BOUNDED_SURFACE()
B_SPLINE_SURFACE(3,2,((#194555,#194556,#194557),(#194558,#194559,#194560),
(#194561,#194562,#194563),(#194564,#194565,#194566)),.UNSPECIFIED.,.F.,
 .F.,.F.)
B_SPLINE_SURFACE_WITH_KNOTS((4,4),(3,3),(0.,0.00767500517967513),(0.,1.),
 .UNSPECIFIED.)
GEOMETRIC_REPRESENTATION_ITEM()
RATIONAL_B_SPLINE_SURFACE(((1.,0.884000563436129,1.),(1.,0.883607612825216,
1.),(1.,0.883267077927119,1.),(1.,0.882986276630499,1.)))
REPRESENTATION_ITEM('')
SURFACE()
);
#2981=(
BOUNDED_SURFACE()
B_SPLINE_SURFACE(3,2,((#194572,#194573,#194574),(#194575,#194576,#194577),
(#194578,#194579,#194580),(#194581,#194582,#194583)),.UNSPECIFIED.,.F.,
 .F.,.F.)
B_SPLINE_SURFACE_WITH_KNOTS((4,4),(3,3),(-1.19804340059648E-17,0.000463834979289297),
(0.,1.),.UNSPECIFIED.)
GEOMETRIC_REPRESENTATION_ITEM()
RATIONAL_B_SPLINE_SURFACE(((1.,0.882986276630509,1.),(1.,0.873185362893501,
1.),(1.,0.861832566029531,1.),(1.,0.849056746210421,1.)))
REPRESENTATION_ITEM('')
SURFACE()
);
#2982=(
BOUNDED_SURFACE()
B_SPLINE_SURFACE(3,2,((#194595,#194596,#194597),(#194598,#194599,#194600),
(#194601,#194602,#194603),(#194604,#194605,#194606),(#194607,#194608,#194609),
(#194610,#194611,#194612),(#194613,#194614,#194615),(#194616,#194617,#194618),
(#194619,#194620,#194621),(#194622,#194623,#194624),(#194625,#194626,#194627),
(#194628,#194629,#194630),(#194631,#194632,#194633),(#194634,#194635,#194636),
(#194637,#194638,#194639),(#194640,#194641,#194642),(#194643,#194644,#194645),
(#194646,#194647,#194648),(#194649,#194650,#194651),(#194652,#194653,#194654),
(#194655,#194656,#194657),(#194658,#194659,#194660),(#194661,#194662,#194663),
(#194664,#194665,#194666),(#194667,#194668,#194669),(#194670,#194671,#194672),
(#194673,#194674,#194675),(#194676,#194677,#194678),(#194679,#194680,#194681),
(#194682,#194683,#194684),(#194685,#194686,#194687),(#194688,#194689,#194690),
(#194691,#194692,#194693),(#194694,#194695,#194696),(#194697,#194698,#194699),
(#194700,#194701,#194702),(#194703,#194704,#194705),(#194706,#194707,#194708),
(#194709,#194710,#194711),(#194712,#194713,#194714),(#194715,#194716,#194717),
(#194718,#194719,#194720),(#194721,#194722,#194723),(#194724,#194725,#194726),
(#194727,#194728,#194729),(#194730,#194731,#194732),(#194733,#194734,#194735),
(#194736,#194737,#194738),(#194739,#194740,#194741),(#194742,#194743,#194744),
(#194745,#194746,#194747),(#194748,#194749,#194750),(#194751,#194752,#194753),
(#194754,#194755,#194756),(#194757,#194758,#194759),(#194760,#194761,#194762),
(#194763,#194764,#194765),(#194766,#194767,#194768),(#194769,#194770,#194771),
(#194772,#194773,#194774),(#194775,#194776,#194777),(#194778,#194779,#194780),
(#194781,#194782,#194783),(#194784,#194785,#194786),(#194787,#194788,#194789),
(#194790,#194791,#194792),(#194793,#194794,#194795),(#194796,#194797,#194798),
(#194799,#194800,#194801),(#194802,#194803,#194804),(#194805,#194806,#194807),
(#194808,#194809,#194810),(#194811,#194812,#194813),(#194814,#194815,#194816),
(#194817,#194818,#194819),(#194820,#194821,#194822),(#194823,#194824,#194825),
(#194826,#194827,#194828),(#194829,#194830,#194831),(#194832,#194833,#194834),
(#194835,#194836,#194837),(#194838,#194839,#194840),(#194841,#194842,#194843),
(#194844,#194845,#194846),(#194847,#194848,#194849),(#194850,#194851,#194852),
(#194853,#194854,#194855),(#194856,#194857,#194858),(#194859,#194860,#194861),
(#194862,#194863,#194864),(#194865,#194866,#194867),(#194868,#194869,#194870),
(#194871,#194872,#194873),(#194874,#194875,#194876),(#194877,#194878,#194879),
(#194880,#194881,#194882),(#194883,#194884,#194885),(#194886,#194887,#194888),
(#194889,#194890,#194891),(#194892,#194893,#194894),(#194895,#194896,#194897),
(#194898,#194899,#194900),(#194901,#194902,#194903),(#194904,#194905,#194906)),
 .UNSPECIFIED.,.F.,.F.,.F.)
B_SPLINE_SURFACE_WITH_KNOTS((4,2,2,2,2,2,2,2,2,2,2,2,2,2,2,2,2,2,2,2,2,
2,2,2,2,2,2,2,2,2,2,2,2,2,2,2,2,2,2,2,2,2,2,2,2,2,2,2,2,2,2,4),(3,3),(-1.90819582357449E-17,
0.00250327328955147,0.00500654657910296,0.0062581832238787,0.00688400154626657,
0.00696222883656506,0.00704045612686354,0.00719691070746051,0.00750981986865445,
0.0100130931582059,0.0112647298029817,0.0115776389641756,0.0117340935447726,
0.0117732071899218,0.0118123208350711,0.0118905481253695,0.0125163664477574,
0.0137680030925332,0.0150196397373089,0.0175229130268604,0.0175620266720097,
0.0176011403171589,0.0176793676074573,0.0178358221880543,0.0181487313492483,
0.0187745496716362,0.0200261863164119,0.0225294596059634,0.0226076868962618,
0.0226468005414111,0.0226859141865603,0.0228423687671573,0.0231552779283512,
0.0237810962507391,0.0250327328955148,0.0275360061850663,0.0281618245074543,
0.0283182790880512,0.0283965063783497,0.0284356200234989,0.0284747336686481,
0.0287876428298421,0.0300392794746179,0.0325425527641693,0.0331683710865572,
0.0332465983768557,0.0333248256671542,0.0334812802477511,0.0337941894089451,
0.0350458260537208,0.0375490993432723,0.0401656877060997),(0.,1.00015179601854),
 .UNSPECIFIED.)
GEOMETRIC_REPRESENTATION_ITEM()
RATIONAL_B_SPLINE_SURFACE(((1.,0.849033833625475,1.00004583212598),(1.,
0.857897119742638,1.00004314130289),(1.,0.865043679059864,1.00004097166439),
(1.,0.876686517055576,1.00003743699149),(1.,0.881205024794411,1.00003606520852),
(1.,0.886414625564822,1.00003448361521),(1.,0.887881243937061,1.00003403836155),
(1.,0.889692656429651,1.00003348843114),(1.,0.890232954947349,1.00003332440081),
(1.,0.890771831880103,1.00003316080207),(1.,0.890856320713948,1.00003313515193),
(1.,0.890681329796628,1.00003318827778),(1.,0.890593656796271,1.0000332148946),
(1.,0.890330116618983,1.0000332949033),(1.,0.890153728390971,1.00003334845336),
(1.,0.889622566425299,1.00003350970991),(1.,0.889265797639508,1.00003361802207),
(1.,0.886032789860672,1.00003459953749),(1.,0.883009418597165,1.00003551740893),
(1.,0.878217284280675,1.00003697226275),(1.,0.876593412053755,1.00003746525742),
(1.,0.874525462184782,1.00003809307054),(1.,0.874110131143723,1.00003821916173),
(1.,0.873484749154558,1.00003840902273),(1.,0.873275890241246,1.00003847243063),
(1.,0.873014337068072,1.00003855183609),(1.,0.872962002442414,1.00003856772447),
(1.,0.872857285608954,1.00003859951566),(1.,0.872731930863508,1.00003863757236),
(1.,0.872890560350215,1.00003858941372),(1.,0.872995125812693,1.00003855766847),
(1.,0.873925639885731,1.00003827517181),(1.,0.874677728758358,1.00003804684362),
(1.,0.876724634752812,1.00003742541926),(1.,0.877812640553407,1.00003709510936),
(1.,0.879464189151955,1.00003659371236),(1.,0.880031794826061,1.00003642139179),
(1.,0.880962615838148,1.00003613880195),(1.,0.880576605528814,1.0000362559916),
(1.,0.879126719140342,1.00003669616556),(1.,0.879157178625721,1.00003668691831),
(1.,0.879182665775382,1.00003667918061),(1.,0.879195407511513,1.00003667531232),
(1.,0.879233627689003,1.00003666370898),(1.,0.879259101093747,1.00003665597546),
(1.,0.879335505234512,1.00003663277977),(1.,0.879386419815118,1.00003661732251),
(1.,0.879539134556379,1.00003657095953),(1.,0.879640904470776,1.00003654006299),
(1.,0.879946424969611,1.0000364473094),(1.,0.88014929469008,1.00003638571977),
(1.,0.880757599478193,1.00003620104328),(1.,0.881161368633861,1.00003607846218),
(1.,0.882351219988641,1.00003571723278),(1.,0.883116027430274,1.00003548504333),
(1.,0.883884077234136,1.00003525186953),(1.,0.883907336025334,1.00003524480835),
(1.,0.883942203551939,1.00003523422284),(1.,0.883958490107036,1.00003522927837),
(1.,0.883961132532197,1.00003522847615),(1.,0.883962211382421,1.00003522814862),
(1.,0.883966395700204,1.0000352268783),(1.,0.883965871907594,1.00003522703732),
(1.,0.883952745623932,1.00003523102235),(1.,0.883928595048457,1.00003523835428),
(1.,0.883810165971008,1.0000352743084),(1.,0.883670016928064,1.00003531685653),
(1.,0.88306386319684,1.00003550087998),(1.,0.882412138697386,1.00003569873835),
(1.,0.879709919903232,1.00003651911046),(1.,0.876914343405723,1.00003736782522),
(1.,0.871931382756172,1.00003888061239),(1.,0.870860364968084,1.00003920576487),
(1.,0.869420643269702,1.00003964285291),(1.,0.869127634755716,1.00003973180796),
(1.,0.868680339242782,1.00003986760332),(1.,0.86852994348834,1.00003991326227),
(1.,0.868302379480849,1.00003998234889),(1.,0.868226196408592,1.00004000547747),
(1.,0.868073169270762,1.00004005193529),(1.,0.86818422111107,1.00004001822083),
(1.,0.868924411953888,1.00003979350479),(1.,0.869577997769037,1.00003959508134),
(1.,0.872822984740276,1.00003860992913),(1.,0.87533860305511,1.00003784620744),
(1.,0.882672172604018,1.00003561979413),(1.,0.88727751836787,1.00003422164782),
(1.,0.892665553038707,1.0000325858834),(1.,0.893724673510805,1.00003226434286),
(1.,0.894892968317747,1.00003190965786),(1.,0.89502245580098,1.00003187034649),
(1.,0.895280775266388,1.00003179192276),(1.,0.89516331129965,1.00003182758388),
(1.,0.894880513654593,1.000031913439),(1.,0.894687925962448,1.00003197190709),
(1.,0.894097865318725,1.0000321510448),(1.,0.893688100021225,1.00003227544628),
(1.,0.891555270434203,1.00003292295636),(1.,0.889581836674106,1.00003352207513),
(1.,0.882741932058345,1.00003559861571),(1.,0.877005189271263,1.00003734024514),
(1.,0.862041840928008,1.00004188299854),(1.,0.852645436799408,1.00004473567201),
(0.999999999999999,0.840867469721541,1.00004831136903)))
REPRESENTATION_ITEM('')
SURFACE()
);
#2983=(
BOUNDED_SURFACE()
B_SPLINE_SURFACE(3,2,((#195298,#195299,#195300),(#195301,#195302,#195303),
(#195304,#195305,#195306),(#195307,#195308,#195309)),.UNSPECIFIED.,.F.,
 .F.,.F.)
B_SPLINE_SURFACE_WITH_KNOTS((4,4),(3,3),(-8.29532866279615E-6,0.00052578299168427),
(-8.29532866279615E-6,1.),.UNSPECIFIED.)
GEOMETRIC_REPRESENTATION_ITEM()
RATIONAL_B_SPLINE_SURFACE(((1.00000262679448,0.841670258828196,1.),(1.00000236409525,
0.857504425499066,1.),(1.00000212772213,0.871751788438872,1.),(1.00000191989843,
0.884278338845134,1.)))
REPRESENTATION_ITEM('')
SURFACE()
);
#2984=(
BOUNDED_SURFACE()
B_SPLINE_SURFACE(3,2,((#195321,#195322,#195323),(#195324,#195325,#195326),
(#195327,#195328,#195329),(#195330,#195331,#195332)),.UNSPECIFIED.,.F.,
 .F.,.F.)
B_SPLINE_SURFACE_WITH_KNOTS((4,4),(3,3),(1.7347234759768E-18,0.00761738954978064),
(0.,1.),.UNSPECIFIED.)
GEOMETRIC_REPRESENTATION_ITEM()
RATIONAL_B_SPLINE_SURFACE(((1.,0.883694369886725,1.),(1.,0.884057799195121,
1.),(1.,0.884477978068247,1.),(1.,0.884949126929568,1.)))
REPRESENTATION_ITEM('')
SURFACE()
);
#2985=(
BOUNDED_SURFACE()
B_SPLINE_SURFACE(3,2,((#195338,#195339,#195340),(#195341,#195342,#195343),
(#195344,#195345,#195346),(#195347,#195348,#195349),(#195350,#195351,#195352),
(#195353,#195354,#195355),(#195356,#195357,#195358),(#195359,#195360,#195361),
(#195362,#195363,#195364),(#195365,#195366,#195367),(#195368,#195369,#195370),
(#195371,#195372,#195373),(#195374,#195375,#195376),(#195377,#195378,#195379),
(#195380,#195381,#195382),(#195383,#195384,#195385),(#195386,#195387,#195388),
(#195389,#195390,#195391),(#195392,#195393,#195394),(#195395,#195396,#195397),
(#195398,#195399,#195400),(#195401,#195402,#195403),(#195404,#195405,#195406),
(#195407,#195408,#195409),(#195410,#195411,#195412),(#195413,#195414,#195415),
(#195416,#195417,#195418),(#195419,#195420,#195421),(#195422,#195423,#195424),
(#195425,#195426,#195427),(#195428,#195429,#195430),(#195431,#195432,#195433)),
 .UNSPECIFIED.,.F.,.F.,.F.)
B_SPLINE_SURFACE_WITH_KNOTS((4,2,2,2,2,2,2,2,2,2,2,2,2,2,2,4),(3,3),(0.,
0.0002498236013634,0.0003747354020451,0.0004996472027268,0.0006245590034085,
0.0007494708040902,0.0008743826047719,0.0009992944054536,0.001249118006817,
0.0013740298074987,0.0014989416081804,0.0016238534088621,0.00168630930920295,
0.0017487652095438,0.0018736770102255,0.0019985888109072),(0.,1.),
 .UNSPECIFIED.)
GEOMETRIC_REPRESENTATION_ITEM()
RATIONAL_B_SPLINE_SURFACE(((1.,0.884949126929531,1.),(1.,0.887143782528108,
1.),(1.,0.890918336240603,1.),(1.,0.894210449378273,1.),(1.,0.895128089226685,
1.),(1.,0.897367518060138,1.),(1.,0.898575478737319,1.),(1.,0.901068236159139,
1.),(1.,0.902188804939834,1.),(1.,0.904118344604245,1.),(1.,0.904836730307214,
1.),(1.,0.906457435203586,1.),(1.,0.907401903391372,1.),(1.,0.909436312125094,
1.),(1.,0.910504885825633,1.),(1.,0.912732113906766,1.),(1.,0.913182649173379,
1.),(1.,0.915295706676324,1.),(1.,0.916179642793504,1.),(1.,0.917783643221206,
1.),(1.,0.918289173478595,1.),(1.,0.919115574923275,1.),(1.,0.919419128152901,
1.),(1.,0.919791548547683,1.),(1.,0.91988587489381,1.),(1.,0.920431178830713,
1.),(1.,0.920846680282669,1.),(1.,0.922176939320294,1.),(1.,0.923013849094452,
1.),(1.,0.924153386273243,1.),(1.,0.924540045823644,1.),(1.,0.924853416885498,
1.)))
REPRESENTATION_ITEM('')
SURFACE()
);
#2986=(
BOUNDED_SURFACE()
B_SPLINE_SURFACE(3,2,((#195515,#195516,#195517),(#195518,#195519,#195520),
(#195521,#195522,#195523),(#195524,#195525,#195526),(#195527,#195528,#195529),
(#195530,#195531,#195532),(#195533,#195534,#195535),(#195536,#195537,#195538),
(#195539,#195540,#195541),(#195542,#195543,#195544),(#195545,#195546,#195547),
(#195548,#195549,#195550)),.UNSPECIFIED.,.F.,.F.,.F.)
B_SPLINE_SURFACE_WITH_KNOTS((4,2,2,2,2,4),(3,3),(-0.000625729109945204,
0.00715193125010649,0.014303862500213,0.0178798281252662,0.0214557937503195,
0.0292334541103712),(0.,1.00062572910995),.UNSPECIFIED.)
GEOMETRIC_REPRESENTATION_ITEM()
RATIONAL_B_SPLINE_SURFACE(((1.,0.924499160265099,1.00009448614649),(1.,
0.925778544860493,1.00009288505013),(1.,0.926988832520574,1.00009137042569),
(1.,0.928403005961066,1.00008960064671),(1.,0.928672278179807,1.00008926366378),
(1.,0.928396618697272,1.0000896086401),(1.,0.928197998538414,1.00008985720493),
(1.,0.927602144330102,1.00009060289158),(1.,0.927204819604613,1.00009110012687),
(1.,0.925564164183759,1.00009315333859),(1.,0.923967382217261,1.0000951516445),
(1.,0.922538732838579,1.00009693953951)))
REPRESENTATION_ITEM('')
SURFACE()
);
#2987=(
BOUNDED_SURFACE()
B_SPLINE_SURFACE(3,2,((#195664,#195665,#195666),(#195667,#195668,#195669),
(#195670,#195671,#195672),(#195673,#195674,#195675),(#195676,#195677,#195678),
(#195679,#195680,#195681),(#195682,#195683,#195684),(#195685,#195686,#195687),
(#195688,#195689,#195690),(#195691,#195692,#195693),(#195694,#195695,#195696),
(#195697,#195698,#195699),(#195700,#195701,#195702),(#195703,#195704,#195705),
(#195706,#195707,#195708),(#195709,#195710,#195711),(#195712,#195713,#195714),
(#195715,#195716,#195717),(#195718,#195719,#195720),(#195721,#195722,#195723),
(#195724,#195725,#195726),(#195727,#195728,#195729),(#195730,#195731,#195732),
(#195733,#195734,#195735),(#195736,#195737,#195738),(#195739,#195740,#195741),
(#195742,#195743,#195744),(#195745,#195746,#195747),(#195748,#195749,#195750),
(#195751,#195752,#195753),(#195754,#195755,#195756),(#195757,#195758,#195759),
(#195760,#195761,#195762),(#195763,#195764,#195765)),.UNSPECIFIED.,.F.,
 .F.,.F.)
B_SPLINE_SURFACE_WITH_KNOTS((4,2,2,2,2,2,2,2,2,2,2,2,2,2,2,2,4),(3,3),(0.,
0.000209917658866865,0.000262397073583582,0.000314876488300298,0.000419835317733731,
0.000524794147167163,0.000629752976600596,0.000839670635467461,0.000892150050184177,
0.000944629464900893,0.00104958829433433,0.00115454712376776,0.00125950595320119,
0.00136446478263462,0.00146942361206806,0.00157438244150149,0.00167934127093492),
(0.,1.),.UNSPECIFIED.)
GEOMETRIC_REPRESENTATION_ITEM()
RATIONAL_B_SPLINE_SURFACE(((1.,0.922934699314368,1.),(1.,0.922418139396395,
1.),(1.,0.921306581502972,1.),(1.,0.918237743219156,1.),(1.,0.917652150959428,
1.),(1.,0.91703035541482,1.),(1.,0.917005626549279,1.),(1.,0.916857059572335,
1.),(1.,0.916688851599089,1.),(1.,0.916103666089295,1.),(1.,0.915719829580818,
1.),(1.,0.914172806704204,1.),(1.,0.912988290535927,1.),(1.,0.910591006023012,
1.),(1.,0.910578234409646,1.),(1.,0.908859123022388,1.),(1.,0.908450616432512,
1.),(1.,0.90741169941527,1.),(1.,0.906720027731936,1.),(1.,0.904857077146999,
1.),(1.,0.903782469918774,1.),(1.,0.902111434863952,1.),(1.,0.901503491191089,
1.),(1.,0.899540977424082,1.),(1.,0.898323167261007,1.),(1.,0.895415117868645,
1.),(1.,0.894063264652639,1.),(1.,0.891702659041491,1.),(1.,0.890819635354087,
1.),(1.,0.888591057203743,1.),(1.,0.88687758303178,1.),(1.,0.883673322831122,
1.),(1.,0.882221756932481,1.),(1.,0.881068987522013,1.)))
REPRESENTATION_ITEM('')
SURFACE()
);
#2988=(
BOUNDED_SURFACE()
B_SPLINE_SURFACE(3,2,((#195852,#195853,#195854),(#195855,#195856,#195857),
(#195858,#195859,#195860),(#195861,#195862,#195863)),.UNSPECIFIED.,.F.,
 .F.,.F.)
B_SPLINE_SURFACE_WITH_KNOTS((4,4),(3,3),(-6.93889390390723E-18,0.00418923766731893),
(0.,1.),.UNSPECIFIED.)
GEOMETRIC_REPRESENTATION_ITEM()
RATIONAL_B_SPLINE_SURFACE(((1.,0.881068987521719,1.),(1.,0.880840248614593,
1.),(1.,0.880630793895676,1.),(1.,0.880439575617234,1.)))
REPRESENTATION_ITEM('')
SURFACE()
);
#2989=(
BOUNDED_SURFACE()
B_SPLINE_SURFACE(3,2,((#195869,#195870,#195871),(#195872,#195873,#195874),
(#195875,#195876,#195877),(#195878,#195879,#195880)),.UNSPECIFIED.,.F.,
 .F.,.F.)
B_SPLINE_SURFACE_WITH_KNOTS((4,4),(3,3),(-7.25197858200355E-6,0.00049505136265659),
(-7.25197858200355E-6,1.),.UNSPECIFIED.)
GEOMETRIC_REPRESENTATION_ITEM()
RATIONAL_B_SPLINE_SURFACE(((1.00000172705636,0.880925161180393,1.),(1.00000188960186,
0.86971818519116,1.),(1.00000207656143,0.856827939964767,1.),(1.00000228609307,
0.842381424617121,0.999999999999999)))
REPRESENTATION_ITEM('')
SURFACE()
);
#2990=(
BOUNDED_SURFACE()
B_SPLINE_SURFACE(3,2,((#195892,#195893,#195894),(#195895,#195896,#195897),
(#195898,#195899,#195900),(#195901,#195902,#195903)),.UNSPECIFIED.,.F.,
 .F.,.F.)
B_SPLINE_SURFACE_WITH_KNOTS((4,4),(3,3),(0.0429271655601134,0.046749382327419),
(0.,1.),.UNSPECIFIED.)
GEOMETRIC_REPRESENTATION_ITEM()
RATIONAL_B_SPLINE_SURFACE(((1.,0.922487559402275,1.),(1.,0.922290239059189,
1.),(1.,0.921950699598134,1.),(1.,0.921567721510049,1.)))
REPRESENTATION_ITEM('')
SURFACE()
);
#2991=(
BOUNDED_SURFACE()
B_SPLINE_SURFACE(3,2,((#195912,#195913,#195914),(#195915,#195916,#195917),
(#195918,#195919,#195920),(#195921,#195922,#195923)),.UNSPECIFIED.,.F.,
 .F.,.F.)
B_SPLINE_SURFACE_WITH_KNOTS((4,4),(3,3),(0.0243367909416761,0.0248833749525317),
(0.,1.),.UNSPECIFIED.)
GEOMETRIC_REPRESENTATION_ITEM()
RATIONAL_B_SPLINE_SURFACE(((1.,0.920889968635124,1.),(1.,0.921315643311136,
1.),(1.,0.921538438398832,1.),(1.,0.921567721510049,1.)))
REPRESENTATION_ITEM('')
SURFACE()
);
#2992=(
BOUNDED_SURFACE()
B_SPLINE_SURFACE(3,2,((#195929,#195930,#195931),(#195932,#195933,#195934),
(#195935,#195936,#195937),(#195938,#195939,#195940),(#195941,#195942,#195943),
(#195944,#195945,#195946),(#195947,#195948,#195949),(#195950,#195951,#195952),
(#195953,#195954,#195955),(#195956,#195957,#195958),(#195959,#195960,#195961),
(#195962,#195963,#195964),(#195965,#195966,#195967),(#195968,#195969,#195970),
(#195971,#195972,#195973),(#195974,#195975,#195976),(#195977,#195978,#195979),
(#195980,#195981,#195982),(#195983,#195984,#195985),(#195986,#195987,#195988),
(#195989,#195990,#195991),(#195992,#195993,#195994),(#195995,#195996,#195997),
(#195998,#195999,#196000),(#196001,#196002,#196003),(#196004,#196005,#196006)),
 .UNSPECIFIED.,.F.,.F.,.F.)
B_SPLINE_SURFACE_WITH_KNOTS((4,2,2,2,2,2,2,2,2,2,2,2,4),(3,3),(0.0236362382318929,
0.0238608230039569,0.023973115389989,0.0240854077760209,0.0243099925480849,
0.0245345773201489,0.0249837468642769,0.0252083316363409,0.0254329164084048,
0.0258820859525328,0.0263312554966607,0.0267804250407887,0.0272295945849166),
(0.,1.),.UNSPECIFIED.)
GEOMETRIC_REPRESENTATION_ITEM()
RATIONAL_B_SPLINE_SURFACE(((1.,0.920889968635126,1.),(1.,0.921094720125926,
1.),(1.,0.92133483228952,1.),(1.,0.921629553215121,1.),(1.,0.921717663867405,
1.),(1.,0.921866856601366,1.),(1.,0.92191190374927,1.),(1.,0.922251469700973,
1.),(1.,0.922692650412903,1.),(1.,0.923603719687576,1.),(1.,0.924055408647065,
1.),(1.,0.925181588378585,1.),(1.,0.925771557037175,1.),(1.,0.927073550275403,
1.),(1.,0.927638435549014,1.),(1.,0.92876341969282,1.),(1.,0.929280825357496,
1.),(1.,0.930786786259919,1.),(1.,0.931716896300058,1.),(1.,0.933882873767671,
1.),(1.,0.935142096438581,1.),(1.,0.937701084319509,1.),(1.,0.938925602458109,
1.),(1.,0.941308524649693,1.),(1.,0.942521337023694,1.),(1.,0.944221776843192,
1.)))
REPRESENTATION_ITEM('')
SURFACE()
);
#2993=(
BOUNDED_SURFACE()
B_SPLINE_SURFACE(3,2,((#196062,#196063,#196064),(#196065,#196066,#196067),
(#196068,#196069,#196070),(#196071,#196072,#196073),(#196074,#196075,#196076),
(#196077,#196078,#196079),(#196080,#196081,#196082),(#196083,#196084,#196085)),
 .UNSPECIFIED.,.F.,.F.,.F.)
B_SPLINE_SURFACE_WITH_KNOTS((4,2,2,4),(3,3),(0.,0.00023361260625816,0.00046722521251632,
0.000934450425032639),(0.,1.),.UNSPECIFIED.)
GEOMETRIC_REPRESENTATION_ITEM()
RATIONAL_B_SPLINE_SURFACE(((1.,0.957684062981954,1.),(1.,0.956682131117891,
1.),(1.,0.955470098743404,1.),(1.,0.953098741844667,1.),(1.,0.951960835596806,
1.),(1.,0.948724989903624,1.),(1.,0.946647027979619,1.),(1.,0.944221776843184,
1.)))
REPRESENTATION_ITEM('')
SURFACE()
);
#2994=(
BOUNDED_SURFACE()
B_SPLINE_SURFACE(3,2,((#196135,#196136,#196137),(#196138,#196139,#196140),
(#196141,#196142,#196143),(#196144,#196145,#196146)),.UNSPECIFIED.,.F.,
 .F.,.F.)
B_SPLINE_SURFACE_WITH_KNOTS((4,4),(3,3),(0.0114568846502287,0.0192019541084939),
(0.,1.),.UNSPECIFIED.)
GEOMETRIC_REPRESENTATION_ITEM()
RATIONAL_B_SPLINE_SURFACE(((1.,0.957684062981984,1.),(1.,0.957879658663776,
1.),(1.,0.958058054935734,1.),(1.,0.958218732174581,1.)))
REPRESENTATION_ITEM('')
SURFACE()
);
#2995=(
BOUNDED_SURFACE()
B_SPLINE_SURFACE(3,2,((#196162,#196163,#196164),(#196165,#196166,#196167),
(#196168,#196169,#196170),(#196171,#196172,#196173)),.UNSPECIFIED.,.F.,
 .F.,.F.)
B_SPLINE_SURFACE_WITH_KNOTS((4,4),(3,3),(0.00545299542660057,0.00564442024814154),
(0.,1.),.UNSPECIFIED.)
GEOMETRIC_REPRESENTATION_ITEM()
RATIONAL_B_SPLINE_SURFACE(((1.,0.992160193962408,1.),(1.,0.99307558921891,
1.),(1.,0.993813024865429,1.),(1.,0.994220746859028,1.)))
REPRESENTATION_ITEM('')
SURFACE()
);
#2996=(
BOUNDED_SURFACE()
B_SPLINE_SURFACE(3,2,((#196188,#196189,#196190),(#196191,#196192,#196193),
(#196194,#196195,#196196),(#196197,#196198,#196199),(#196200,#196201,#196202),
(#196203,#196204,#196205)),.UNSPECIFIED.,.F.,.F.,.F.)
B_SPLINE_SURFACE_WITH_KNOTS((4,2,4),(3,3),(-1.09829680072782E-16,0.000498949606022071,
0.000997899212044251),(0.,1.),.UNSPECIFIED.)
GEOMETRIC_REPRESENTATION_ITEM()
RATIONAL_B_SPLINE_SURFACE(((1.,0.994220746859027,1.),(1.,0.996098915568006,
1.),(1.,0.997550054459957,1.),(1.,0.99950507842482,1.),(1.,1.00000638742927,
1.),(1.,1.,1.)))
REPRESENTATION_ITEM('')
SURFACE()
);
#2997=(
BOUNDED_SURFACE()
B_SPLINE_SURFACE(3,2,((#196264,#196265,#196266),(#196267,#196268,#196269),
(#196270,#196271,#196272),(#196273,#196274,#196275),(#196276,#196277,#196278),
(#196279,#196280,#196281),(#196282,#196283,#196284),(#196285,#196286,#196287),
(#196288,#196289,#196290),(#196291,#196292,#196293),(#196294,#196295,#196296),
(#196297,#196298,#196299),(#196300,#196301,#196302),(#196303,#196304,#196305),
(#196306,#196307,#196308),(#196309,#196310,#196311),(#196312,#196313,#196314),
(#196315,#196316,#196317),(#196318,#196319,#196320),(#196321,#196322,#196323),
(#196324,#196325,#196326),(#196327,#196328,#196329),(#196330,#196331,#196332),
(#196333,#196334,#196335),(#196336,#196337,#196338),(#196339,#196340,#196341),
(#196342,#196343,#196344),(#196345,#196346,#196347),(#196348,#196349,#196350),
(#196351,#196352,#196353),(#196354,#196355,#196356),(#196357,#196358,#196359),
(#196360,#196361,#196362),(#196363,#196364,#196365),(#196366,#196367,#196368),
(#196369,#196370,#196371),(#196372,#196373,#196374),(#196375,#196376,#196377),
(#196378,#196379,#196380),(#196381,#196382,#196383),(#196384,#196385,#196386),
(#196387,#196388,#196389),(#196390,#196391,#196392),(#196393,#196394,#196395),
(#196396,#196397,#196398),(#196399,#196400,#196401),(#196402,#196403,#196404),
(#196405,#196406,#196407),(#196408,#196409,#196410),(#196411,#196412,#196413),
(#196414,#196415,#196416),(#196417,#196418,#196419),(#196420,#196421,#196422),
(#196423,#196424,#196425),(#196426,#196427,#196428),(#196429,#196430,#196431),
(#196432,#196433,#196434),(#196435,#196436,#196437),(#196438,#196439,#196440),
(#196441,#196442,#196443),(#196444,#196445,#196446),(#196447,#196448,#196449),
(#196450,#196451,#196452),(#196453,#196454,#196455),(#196456,#196457,#196458),
(#196459,#196460,#196461),(#196462,#196463,#196464),(#196465,#196466,#196467),
(#196468,#196469,#196470),(#196471,#196472,#196473),(#196474,#196475,#196476),
(#196477,#196478,#196479),(#196480,#196481,#196482),(#196483,#196484,#196485),
(#196486,#196487,#196488),(#196489,#196490,#196491),(#196492,#196493,#196494),
(#196495,#196496,#196497),(#196498,#196499,#196500),(#196501,#196502,#196503),
(#196504,#196505,#196506),(#196507,#196508,#196509),(#196510,#196511,#196512),
(#196513,#196514,#196515),(#196516,#196517,#196518),(#196519,#196520,#196521),
(#196522,#196523,#196524),(#196525,#196526,#196527),(#196528,#196529,#196530),
(#196531,#196532,#196533),(#196534,#196535,#196536),(#196537,#196538,#196539),
(#196540,#196541,#196542),(#196543,#196544,#196545),(#196546,#196547,#196548),
(#196549,#196550,#196551),(#196552,#196553,#196554),(#196555,#196556,#196557),
(#196558,#196559,#196560),(#196561,#196562,#196563),(#196564,#196565,#196566),
(#196567,#196568,#196569),(#196570,#196571,#196572),(#196573,#196574,#196575),
(#196576,#196577,#196578),(#196579,#196580,#196581),(#196582,#196583,#196584),
(#196585,#196586,#196587),(#196588,#196589,#196590),(#196591,#196592,#196593),
(#196594,#196595,#196596),(#196597,#196598,#196599),(#196600,#196601,#196602),
(#196603,#196604,#196605),(#196606,#196607,#196608),(#196609,#196610,#196611),
(#196612,#196613,#196614),(#196615,#196616,#196617),(#196618,#196619,#196620),
(#196621,#196622,#196623),(#196624,#196625,#196626),(#196627,#196628,#196629),
(#196630,#196631,#196632),(#196633,#196634,#196635),(#196636,#196637,#196638),
(#196639,#196640,#196641),(#196642,#196643,#196644),(#196645,#196646,#196647),
(#196648,#196649,#196650),(#196651,#196652,#196653),(#196654,#196655,#196656),
(#196657,#196658,#196659),(#196660,#196661,#196662),(#196663,#196664,#196665)),
 .UNSPECIFIED.,.F.,.F.,.F.)
B_SPLINE_SURFACE_WITH_KNOTS((4,2,2,2,2,2,2,2,2,2,2,2,2,2,2,2,2,2,2,2,2,
2,2,2,2,2,2,2,2,2,2,2,2,2,2,2,2,2,2,2,2,2,2,2,2,2,2,2,2,2,2,2,2,2,2,2,2,
2,2,2,2,2,2,2,2,2,4),(3,3),(0.0401209448553485,0.0422079288610133,0.0442949128666782,
0.046381896872343,0.0484688808780079,0.0526428488893376,0.0527732853896916,
0.0528385036398687,0.0529037218900457,0.0531645948907538,0.05368634089217,
0.0547298328950024,0.0568168169006673,0.0578603089034997,0.0589038009063321,
0.0599472929091645,0.0602081659098726,0.0603386024102267,0.0603712115353152,
0.0604038206604037,0.0604690389105808,0.060990784911997,0.0651647529233267,
0.0693387209346564,0.0698604669360726,0.0701213399367807,0.0701865581869577,
0.0702191673120462,0.0702517764371347,0.0703822129374888,0.0714257049403212,
0.0724691969431537,0.0735126889459861,0.0755996729516509,0.0766431649544833,
0.0771649109558996,0.0774257839566077,0.0775562204569617,0.0776214387071387,
0.0776540478322272,0.0776866569573158,0.0818606249686455,0.0860345929799752,
0.0870780849828076,0.0873389579835157,0.0874041762336927,0.0874367853587812,
0.0874530899213255,0.0874693944838697,0.0875998309842238,0.08812157698564,
0.0902085609913048,0.0943825290026346,0.0946434020033427,0.0947086202535197,
0.0947412293786082,0.0947738385036967,0.0949042750040508,0.095426021005467,
0.0964695130082994,0.0985564970139642,0.100643481019629,0.101686973022461,
0.102730465025294,0.104817449030959,0.105860941033791,0.106904433036624),
(-0.000150331225571141,1.),.UNSPECIFIED.)
GEOMETRIC_REPRESENTATION_ITEM()
RATIONAL_B_SPLINE_SURFACE(((1.00000971526928,0.967687121417261,1.),(1.00000979368702,
0.967426304860057,1.),(1.00000993438659,0.966958339653348,1.),(1.00001029017888,
0.965774978398451,1.),(1.00001050549399,0.965058842720181,1.),(1.00001098728375,
0.963456415296758,1.),(1.00001125422659,0.962568566336671,1.),(1.0000118294071,
0.960655522326197,1.),(1.00001213342102,0.959644375358026,1.),(1.00001308594142,
0.956476303020351,1.),(1.00001377412596,0.954187408806267,1.),(1.00001454155145,
0.951634960071011,1.),(1.00001456486356,0.951557424250059,1.),(1.00001459991773,
0.951440834491396,1.),(1.00001457230817,0.951532663561032,1.),(1.00001453962294,
0.951641374304724,1.),(1.00001452333201,0.951695557756684,1.),(1.00001444213708,
0.951965611176811,1.),(1.00001437801212,0.952178890092796,1.),(1.00001418818244,
0.952810261506986,1.),(1.00001406502106,0.953219894923565,1.),(1.0000137061962,
0.954413342436734,1.),(1.00001348115785,0.955161817519688,1.),(1.00001285359615,
0.957249080809413,1.),(1.00001250436141,0.958410631712903,1.),(1.00001210988278,
0.95972266329395,1.),(1.00001200110933,0.960084442603283,1.),(1.00001183261586,
0.960644850011032,1.),(1.00001177287885,0.960843534658787,1.),(1.00001170804724,
0.96105916386307,1.),(1.00001170266968,0.961077049592171,1.),(1.00001173086546,
0.960983270719707,1.),(1.00001173825265,0.960958701013246,1.),(1.00001175198371,
0.960913031660308,1.),(1.00001175700248,0.960896339292811,1.),(1.00001176383135,
0.960873626543695,1.),(1.00001176522489,0.960868991626948,1.),(1.00001176806761,
0.960859536780326,1.),(1.00001177105464,0.960849601956462,1.),(1.00001176869476,
0.960857450901041,1.),(1.00001176715196,0.96086258223084,1.),(1.00001175353863,
0.960907860010547,1.),(1.00001174336965,0.96094168192141,1.),(1.0000116681701,
0.961191794790978,1.),(1.00001171285899,0.961043160058672,1.),(1.00001196988856,
0.96018828251794,1.),(1.00001218283227,0.959480034084875,1.),(1.00001253635177,
0.958304232125271,1.),(1.00001257727477,0.958168122675296,1.),(1.00001264122898,
0.957955411672161,1.),(1.00001266294138,0.957883196469429,1.),(1.00001269058339,
0.957791259469782,1.),(1.00001269613687,0.957772788660441,1.),(1.00001270450487,
0.957744956766385,1.),(1.0000127126013,0.957718028118306,1.),(1.00001270395433,
0.957746787852822,1.),(1.00001269965221,0.9577610966519,1.),(1.00001267824887,
0.957832283944761,1.),(1.00001266146939,0.957888092294895,1.),(1.00001251358919,
0.958379940224678,1.),(1.00001240455658,0.958742581485571,1.),(1.00001223534349,
0.959305382336318,1.),(1.00001217514497,0.959505601958515,1.),(1.00001210726764,
0.959731361219486,1.),(1.00001209931732,0.959757803879631,1.),(1.00001215129706,
0.959584919863517,1.),(1.0000122874652,0.959132026118958,1.),(1.00001262675854,
0.95800354019393,1.),(1.00001276231487,0.957552681348205,1.),(1.00001299609705,
0.956775124398884,1.),(1.00001307914247,0.95649891625436,1.),(1.00001321097066,
0.956060457128587,1.),(1.0000132561197,0.955910291938057,1.),(1.00001332558918,
0.955679237196541,1.),(1.00001334903664,0.955601251202993,1.),(1.00001338463613,
0.955482847702871,1.),(1.000013396574,0.955443142455131,1.),(1.00001341458686,
0.955383231893246,1.),(1.00001342060882,0.955363202924128,1.),(1.00001343268791,
0.955323027998288,1.),(1.00001342097891,0.955361972010516,1.),(1.0000128917049,
0.957122331530358,1.),(1.00001245359404,0.958579483414712,1.),(1.00001173531401,
0.960968474900111,1.),(1.00001145207891,0.96191051170025,1.),(1.00001123165748,
0.962643630951223,1.),(1.00001119459058,0.962766915069294,1.),(1.00001115856949,
0.962886720799798,1.),(1.00001115188289,0.962908960376103,1.),(1.00001114420108,
0.962934509975404,1.),(1.00001114269855,0.962939507370241,1.),(1.00001114049609,
0.962946832741217,1.),(1.00001113977049,0.962949246077756,1.),(1.000011138695,
0.962952823156129,1.),(1.00001113833865,0.962954008361232,1.),(1.00001113763027,
0.962956364421279,1.),(1.00001113829343,0.962954158761119,1.),(1.00001114110855,
0.962944795699858,1.),(1.00001114414817,0.962934685949314,1.),(1.00001116199795,
0.962875317780209,1.),(1.00001118475773,0.962799619030819,1.),(1.00001133896015,
0.96228674347642,1.),(1.00001159320074,0.961441142056957,1.),(1.00001265659516,
0.957904303941762,1.),(1.00001376678907,0.954211811223626,1.),(1.00001513580773,
0.949658470243662,1.),(1.0000152171122,0.949388052460497,1.),(1.00001531968671,
0.949046890784209,1.),(1.00001534024882,0.948978501441861,1.),(1.00001537116238,
0.948875683285007,1.),(1.00001538147863,0.948841371541406,1.),(1.00001540213453,
0.948772670228394,1.),(1.00001538091888,0.948843233269349,1.),(1.00001534454108,
0.948964225425651,1.),(1.00001531549173,0.94906084323558,1.),(1.00001517050652,
0.949543062447052,1.),(1.0000150553548,0.949926055790804,1.),(1.00001471230728,
0.951067028082035,1.),(1.00001448692643,0.951816642300841,1.),(1.00001381880759,
0.954038798202261,1.),(1.00001338374559,0.955485809633019,1.),(1.00001253497379,
0.958308815288275,1.),(1.00001212137949,0.959684425368754,1.),(1.00001152065592,
0.961682425350425,1.),(1.00001132312401,0.962339414286871,1.),(1.00001094046962,
0.963612118576129,1.),(1.00001075510022,0.964228655148104,1.),(1.00001021993682,
0.966008602726101,1.),(1.00000989010539,0.967105618448797,1.),(1.0000094600318,
0.968536038448202,1.),(1.00000932763788,0.968976379179426,1.),(1.00000909187148,
0.969760535622473,1.),(1.00000898814038,0.970105544128433,1.),(1.0000089057079,
0.97037971365699,1.)))
REPRESENTATION_ITEM('')
SURFACE()
);
#2998=(
BOUNDED_SURFACE()
B_SPLINE_SURFACE(3,2,((#197269,#197270,#197271),(#197272,#197273,#197274),
(#197275,#197276,#197277),(#197278,#197279,#197280),(#197281,#197282,#197283),
(#197284,#197285,#197286)),.UNSPECIFIED.,.F.,.F.,.F.)
B_SPLINE_SURFACE_WITH_KNOTS((4,2,4),(3,3),(-2.65828754408143E-15,0.000518614521426172,
0.001037229042855),(0.,1.),.UNSPECIFIED.)
GEOMETRIC_REPRESENTATION_ITEM()
RATIONAL_B_SPLINE_SURFACE(((1.,0.994246489501235,1.),(1.,0.99609478928193,
1.),(1.,0.997541267372286,1.),(1.,0.999499888835022,1.),(1.,1.00000732330262,
1.),(1.,1.,1.)))
REPRESENTATION_ITEM('')
SURFACE()
);
#2999=(
BOUNDED_SURFACE()
B_SPLINE_SURFACE(3,2,((#197303,#197304,#197305),(#197306,#197307,#197308),
(#197309,#197310,#197311),(#197312,#197313,#197314)),.UNSPECIFIED.,.F.,
 .F.,.F.)
B_SPLINE_SURFACE_WITH_KNOTS((4,4),(3,3),(0.0119444722538381,0.0121107952282446),
(0.,1.00002036952005),.UNSPECIFIED.)
GEOMETRIC_REPRESENTATION_ITEM()
RATIONAL_B_SPLINE_SURFACE(((1.,0.99280936423786,1.0000002929396),(1.,0.993510643385736,
1.00000026437016),(1.,0.994041174404923,1.00000024275684),(1.,0.99432165622759,
1.00000023133027)))
REPRESENTATION_ITEM('')
SURFACE()
);
#3000=(
BOUNDED_SURFACE()
B_SPLINE_SURFACE(3,2,((#197329,#197330,#197331),(#197332,#197333,#197334),
(#197335,#197336,#197337),(#197338,#197339,#197340)),.UNSPECIFIED.,.F.,
 .F.,.F.)
B_SPLINE_SURFACE_WITH_KNOTS((4,4),(3,3),(0.0657640091385094,0.0735516090029935),
(0.,1.),.UNSPECIFIED.)
GEOMETRIC_REPRESENTATION_ITEM()
RATIONAL_B_SPLINE_SURFACE(((1.,0.958250447061442,1.),(1.,0.958411329127679,
1.),(1.,0.958554518262528,1.),(1.,0.958680046125676,1.)))
REPRESENTATION_ITEM('')
SURFACE()
);
#3001=(
BOUNDED_SURFACE()
B_SPLINE_SURFACE(3,2,((#197346,#197347,#197348),(#197349,#197350,#197351),
(#197352,#197353,#197354),(#197355,#197356,#197357),(#197358,#197359,#197360),
(#197361,#197362,#197363)),.UNSPECIFIED.,.F.,.F.,.F.)
B_SPLINE_SURFACE_WITH_KNOTS((4,2,4),(3,3),(-3.33934269125535E-17,0.000375063365810863,
0.00075012673162176),(0.,1.),.UNSPECIFIED.)
GEOMETRIC_REPRESENTATION_ITEM()
RATIONAL_B_SPLINE_SURFACE(((1.,0.949971414633671,1.),(1.,0.951436745841567,
1.),(1.,0.952767928482916,1.),(1.,0.955568668815872,1.),(1.,0.957047312721609,
1.),(1.,0.958250447045288,1.)))
REPRESENTATION_ITEM('')
SURFACE()
);
#3002=(
BOUNDED_SURFACE()
B_SPLINE_SURFACE(3,2,((#197380,#197381,#197382),(#197383,#197384,#197385),
(#197386,#197387,#197388),(#197389,#197390,#197391),(#197392,#197393,#197394),
(#197395,#197396,#197397),(#197398,#197399,#197400),(#197401,#197402,#197403),
(#197404,#197405,#197406),(#197407,#197408,#197409),(#197410,#197411,#197412),
(#197413,#197414,#197415),(#197416,#197417,#197418),(#197419,#197420,#197421),
(#197422,#197423,#197424),(#197425,#197426,#197427),(#197428,#197429,#197430),
(#197431,#197432,#197433),(#197434,#197435,#197436),(#197437,#197438,#197439),
(#197440,#197441,#197442),(#197443,#197444,#197445),(#197446,#197447,#197448),
(#197449,#197450,#197451),(#197452,#197453,#197454),(#197455,#197456,#197457)),
 .UNSPECIFIED.,.F.,.F.,.F.)
B_SPLINE_SURFACE_WITH_KNOTS((4,2,2,2,2,2,2,2,2,2,2,2,4),(3,3),(0.0241420258550515,
0.0246199912180732,0.0250868407533039,0.0255536902885345,0.0260205398237651,
0.0262539645913804,0.0264873893589957,0.0269542388942264,0.0271876636618417,
0.0274210884294571,0.0275378008132647,0.0276545131970724,0.0278990537924757),
(0.,1.00001111582779),.UNSPECIFIED.)
GEOMETRIC_REPRESENTATION_ITEM()
RATIONAL_B_SPLINE_SURFACE(((1.,0.950055426454912,1.00000111035056),(1.,
0.948849226790929,1.00000113716637),(1.,0.947384468413781,1.00000116973038),
(1.,0.945196499226927,1.00000121837255),(1.,0.944259740621461,1.00000123919825),
(1.,0.942078306513855,1.00000128769514),(1.,0.940957878707281,1.00000131260411),
(1.,0.938972382400276,1.00000135674498),(1.,0.938140754494424,1.00000137523344),
(1.,0.936869151046711,1.00000140350329),(1.,0.936440925028753,1.00000141302346),
(1.,0.93553683485142,1.00000143312289),(1.,0.935022314137583,1.00000144456153),
(1.,0.933816624278113,1.00000147136601),(1.,0.933295910820293,1.00000148294234),
(1.,0.932361200720811,1.00000150372249),(1.,0.932002008792242,1.00000151170792),
(1.,0.931284282765525,1.00000152766416),(1.,0.930932917594263,1.00000153547559),
(1.,0.930603729964699,1.00000154279397),(1.,0.930541982836373,1.00000154416671),
(1.,0.930392431492657,1.00000154749149),(1.,0.93030830454879,1.00000154936177),
(1.,0.930032458299446,1.00000155549429),(1.,0.929822127885655,1.00000156017028),
(1.,0.929675939651775,1.00000156342029)))
REPRESENTATION_ITEM('')
SURFACE()
);
#3003=(
BOUNDED_SURFACE()
B_SPLINE_SURFACE(3,2,((#197620,#197621,#197622),(#197623,#197624,#197625),
(#197626,#197627,#197628),(#197629,#197630,#197631)),.UNSPECIFIED.,.F.,
 .F.,.F.)
B_SPLINE_SURFACE_WITH_KNOTS((4,4),(3,3),(0.0249863231317726,0.0253614725245169),
(0.,1.),.UNSPECIFIED.)
GEOMETRIC_REPRESENTATION_ITEM()
RATIONAL_B_SPLINE_SURFACE(((1.,0.930070526504304,1.),(1.,0.930041043693298,
1.),(1.,0.929915461335265,1.),(1.,0.929697045866142,1.)))
REPRESENTATION_ITEM('')
SURFACE()
);
#3004=(
BOUNDED_SURFACE()
B_SPLINE_SURFACE(3,2,((#197637,#197638,#197639),(#197640,#197641,#197642),
(#197643,#197644,#197645),(#197646,#197647,#197648)),.UNSPECIFIED.,.F.,
 .F.,.F.)
B_SPLINE_SURFACE_WITH_KNOTS((4,4),(3,3),(0.0387340315057144,0.0427072915207099),
(0.,1.),.UNSPECIFIED.)
GEOMETRIC_REPRESENTATION_ITEM()
RATIONAL_B_SPLINE_SURFACE(((1.,0.930070526504304,1.),(1.,0.930612186341166,
1.),(1.,0.931191283587817,1.),(1.,0.931676951123116,1.)))
REPRESENTATION_ITEM('')
SURFACE()
);
#3005=(
BOUNDED_SURFACE()
B_SPLINE_SURFACE(3,2,((#197654,#197655,#197656),(#197657,#197658,#197659),
(#197660,#197661,#197662),(#197663,#197664,#197665)),.UNSPECIFIED.,.F.,
 .F.,.F.)
B_SPLINE_SURFACE_WITH_KNOTS((4,4),(3,3),(-0.000102945165535128,0.00102945165511774),
(0.,1.00671370076984),.UNSPECIFIED.)
GEOMETRIC_REPRESENTATION_ITEM()
RATIONAL_B_SPLINE_SURFACE(((0.999999999999999,0.997903207556182,1.00002815447409),
(1.,0.999219022833365,1.00001048649401),(1.,1.00001169204399,0.99999984300623),
(1.,1.,1.)))
REPRESENTATION_ITEM('')
SURFACE()
);
#3006=(
BOUNDED_SURFACE()
B_SPLINE_SURFACE(3,2,((#197735,#197736,#197737),(#197738,#197739,#197740),
(#197741,#197742,#197743),(#197744,#197745,#197746)),.UNSPECIFIED.,.F.,
 .F.,.F.)
B_SPLINE_SURFACE_WITH_KNOTS((4,4),(3,3),(0.0105620870905992,0.0106719618085628),
(0.,1.),.UNSPECIFIED.)
GEOMETRIC_REPRESENTATION_ITEM()
RATIONAL_B_SPLINE_SURFACE(((1.,0.997703261465162,1.),(1.,0.997980295466877,
1.),(1.,0.998184609657421,1.),(1.,0.998260562486345,1.)))
REPRESENTATION_ITEM('')
SURFACE()
);
#3007=(
BOUNDED_SURFACE()
B_SPLINE_SURFACE(3,2,((#197752,#197753,#197754),(#197755,#197756,#197757),
(#197758,#197759,#197760),(#197761,#197762,#197763)),.UNSPECIFIED.,.F.,
 .F.,.F.)
B_SPLINE_SURFACE_WITH_KNOTS((4,4),(3,3),(0.0270627267990643,0.0348275700538469),
(0.,1.),.UNSPECIFIED.)
GEOMETRIC_REPRESENTATION_ITEM()
RATIONAL_B_SPLINE_SURFACE(((1.,0.959662285900567,1.),(1.,0.959827071897822,
1.),(1.,0.959976275192286,1.),(1.,0.960109658705298,1.)))
REPRESENTATION_ITEM('')
SURFACE()
);
#3008=(
BOUNDED_SURFACE()
B_SPLINE_SURFACE(3,2,((#197769,#197770,#197771),(#197772,#197773,#197774),
(#197775,#197776,#197777),(#197778,#197779,#197780),(#197781,#197782,#197783),
(#197784,#197785,#197786),(#197787,#197788,#197789),(#197790,#197791,#197792),
(#197793,#197794,#197795),(#197796,#197797,#197798)),.UNSPECIFIED.,.F.,
 .F.,.F.)
B_SPLINE_SURFACE_WITH_KNOTS((4,2,2,2,4),(3,3),(-8.76035355368288E-17,0.000261575538067988,
0.000523151076136064,0.00078472661420414,0.00104630215227222),(0.,1.),
 .UNSPECIFIED.)
GEOMETRIC_REPRESENTATION_ITEM()
RATIONAL_B_SPLINE_SURFACE(((1.,0.941539462223513,1.),(1.,0.942944078103832,
1.),(1.,0.944666632267536,1.),(1.,0.947704870094427,1.),(1.,0.949116332566031,
1.),(1.,0.951938364158755,1.),(1.,0.953364849053626,1.),(1.,0.956562808919945,
1.),(1.,0.958303880696362,1.),(1.,0.959662285866081,1.)))
REPRESENTATION_ITEM('')
SURFACE()
);
#3009=(
BOUNDED_SURFACE()
B_SPLINE_SURFACE(3,2,((#197825,#197826,#197827),(#197828,#197829,#197830),
(#197831,#197832,#197833),(#197834,#197835,#197836),(#197837,#197838,#197839),
(#197840,#197841,#197842),(#197843,#197844,#197845),(#197846,#197847,#197848),
(#197849,#197850,#197851),(#197852,#197853,#197854),(#197855,#197856,#197857),
(#197858,#197859,#197860),(#197861,#197862,#197863),(#197864,#197865,#197866),
(#197867,#197868,#197869),(#197870,#197871,#197872),(#197873,#197874,#197875),
(#197876,#197877,#197878),(#197879,#197880,#197881),(#197882,#197883,#197884),
(#197885,#197886,#197887),(#197888,#197889,#197890),(#197891,#197892,#197893),
(#197894,#197895,#197896),(#197897,#197898,#197899),(#197900,#197901,#197902)),
 .UNSPECIFIED.,.F.,.F.,.F.)
B_SPLINE_SURFACE_WITH_KNOTS((4,2,2,2,2,2,2,2,2,2,2,2,4),(3,3),(0.0234563246751814,
0.0238865203213557,0.0243167159675301,0.0247469116137044,0.0251771072598787,
0.0253922050829658,0.0256073029060529,0.0260374985522272,0.0262525963753144,
0.0264676941984016,0.0265752431099451,0.0266827920214887,0.0268978898445759),
(0.,1.),.UNSPECIFIED.)
GEOMETRIC_REPRESENTATION_ITEM()
RATIONAL_B_SPLINE_SURFACE(((1.,0.941539462223482,1.),(1.,0.94001314415555,
1.),(1.,0.938778552928411,1.),(1.,0.936146669124993,1.),(1.,0.934687355972348,
1.),(1.,0.931881901141109,1.),(1.,0.930584405145522,1.),(1.,0.928334675540862,
1.),(1.,0.927304800261896,1.),(1.,0.925560477902519,1.),(1.,0.924898629931803,
1.),(1.,0.923648361190968,1.),(1.,0.923163635402122,1.),(1.,0.921866592945891,
1.),(1.,0.921255551609143,1.),(1.,0.919961545322548,1.),(1.,0.91942646515046,
1.),(1.,0.918406367469313,1.),(1.,0.917958926413567,1.),(1.,0.917720801012666,
1.),(1.,0.917685854938757,1.),(1.,0.917559269654572,1.),(1.,0.917489604007006,
1.),(1.,0.917284127651096,1.),(1.,0.917152514069398,1.),(1.,0.917108339181246,
1.)))
REPRESENTATION_ITEM('')
SURFACE()
);
#3010=(
BOUNDED_SURFACE()
B_SPLINE_SURFACE(3,2,((#197958,#197959,#197960),(#197961,#197962,#197963),
(#197964,#197965,#197966),(#197967,#197968,#197969)),.UNSPECIFIED.,.F.,
 .F.,.F.)
B_SPLINE_SURFACE_WITH_KNOTS((4,4),(3,3),(0.0245397910410617,0.0252336582652646),
(0.,1.),.UNSPECIFIED.)
GEOMETRIC_REPRESENTATION_ITEM()
RATIONAL_B_SPLINE_SURFACE(((1.,0.91828031569264,1.),(1.,0.918191277007662,
1.),(1.,0.917795655860169,1.),(1.,0.917108339181228,1.)))
REPRESENTATION_ITEM('')
SURFACE()
);
#3011=(
BOUNDED_SURFACE()
B_SPLINE_SURFACE(3,2,((#197984,#197985,#197986),(#197987,#197988,#197989),
(#197990,#197991,#197992),(#197993,#197994,#197995)),.UNSPECIFIED.,.F.,
 .F.,.F.)
B_SPLINE_SURFACE_WITH_KNOTS((4,4),(3,3),(0.0408577781618264,0.0446742483522374),
(0.,1.),.UNSPECIFIED.)
GEOMETRIC_REPRESENTATION_ITEM()
RATIONAL_B_SPLINE_SURFACE(((1.,0.918280315692642,1.),(1.,0.919146142525415,
1.),(1.,0.920060572994544,1.),(1.,0.920885718130539,1.)))
REPRESENTATION_ITEM('')
SURFACE()
);
#3012=(
BOUNDED_SURFACE()
B_SPLINE_SURFACE(3,2,((#198010,#198011,#198012),(#198013,#198014,#198015),
(#198016,#198017,#198018),(#198019,#198020,#198021),(#198022,#198023,#198024),
(#198025,#198026,#198027),(#198028,#198029,#198030),(#198031,#198032,#198033),
(#198034,#198035,#198036),(#198037,#198038,#198039),(#198040,#198041,#198042),
(#198043,#198044,#198045),(#198046,#198047,#198048),(#198049,#198050,#198051),
(#198052,#198053,#198054),(#198055,#198056,#198057),(#198058,#198059,#198060),
(#198061,#198062,#198063),(#198064,#198065,#198066),(#198067,#198068,#198069),
(#198070,#198071,#198072),(#198073,#198074,#198075),(#198076,#198077,#198078),
(#198079,#198080,#198081),(#198082,#198083,#198084),(#198085,#198086,#198087),
(#198088,#198089,#198090),(#198091,#198092,#198093),(#198094,#198095,#198096),
(#198097,#198098,#198099),(#198100,#198101,#198102),(#198103,#198104,#198105),
(#198106,#198107,#198108),(#198109,#198110,#198111),(#198112,#198113,#198114),
(#198115,#198116,#198117),(#198118,#198119,#198120),(#198121,#198122,#198123),
(#198124,#198125,#198126),(#198127,#198128,#198129),(#198130,#198131,#198132),
(#198133,#198134,#198135),(#198136,#198137,#198138),(#198139,#198140,#198141),
(#198142,#198143,#198144),(#198145,#198146,#198147),(#198148,#198149,#198150),
(#198151,#198152,#198153),(#198154,#198155,#198156),(#198157,#198158,#198159),
(#198160,#198161,#198162),(#198163,#198164,#198165),(#198166,#198167,#198168),
(#198169,#198170,#198171),(#198172,#198173,#198174),(#198175,#198176,#198177),
(#198178,#198179,#198180),(#198181,#198182,#198183),(#198184,#198185,#198186),
(#198187,#198188,#198189),(#198190,#198191,#198192),(#198193,#198194,#198195)),
 .UNSPECIFIED.,.F.,.F.,.F.)
B_SPLINE_SURFACE_WITH_KNOTS((4,2,2,2,2,2,2,2,2,2,2,2,2,2,2,2,2,2,2,2,2,
2,2,2,2,2,2,2,2,2,4),(3,3),(8.67361737988404E-19,0.00422017278643856,0.00435205318601475,
0.00438502328590881,0.00441799338580286,0.00448393358559096,0.00474769438474337,
0.00527521598304819,0.00633025917965783,0.00844034557287711,0.0126605183593157,
0.0137155615559253,0.0137815017557134,0.0138474419555015,0.0139793223550777,
0.0142430831542301,0.0147706047525349,0.0168806911457542,0.0211008639321928,
0.0221559071288024,0.0224196679279548,0.0224856081277429,0.0225185782276369,
0.022551548327531,0.0226834287271072,0.0232109503254121,0.0253210367186313,
0.0274311231118506,0.0284861663084603,0.0295412095050698,0.0337613822915084),
(-3.60075492201877E-5,1.),.UNSPECIFIED.)
GEOMETRIC_REPRESENTATION_ITEM()
RATIONAL_B_SPLINE_SURFACE(((1.00000292637104,0.959364479127511,1.),(1.00000292757611,
0.959347745547871,1.),(1.0000029869754,0.958522928388227,1.),(1.00000309965914,
0.956958204480126,1.),(1.00000310312445,0.956910085312184,1.),(1.00000310752022,
0.956849045791879,1.),(1.0000031057735,0.956873300638878,1.),(1.0000031039675,
0.956898378742207,1.),(1.00000310306648,0.956910890223367,1.),(1.0000031003694,
0.956948341850289,1.),(1.0000030985793,0.956973199179412,1.),(1.00000308966864,
0.957096932329961,1.),(1.00000308266768,0.957194147589323,1.),(1.00000306205115,
0.957480428238286,1.),(1.00000304882204,0.957664127258792,1.),(1.00000301070718,
0.958193389415057,1.),(1.00000298738066,0.958517300910559,1.),(1.00000292394881,
0.95939811406461,1.),(1.00000289040681,0.959863877542923,1.),(1.0000028158029,
0.960899825671287,1.),(1.00000280023093,0.961116057785621,1.),(1.00000283026338,
0.960699027834766,1.),(1.0000028387997,0.960580492677261,1.),(1.0000028506814,
0.96041550366659,1.),(1.00000285139065,0.960405655023073,1.),(1.00000285282986,
0.960385670240394,1.),(1.00000285177099,0.96040037370118,1.),(1.00000285025679,
0.960421399773948,1.),(1.000002849315,0.960434477515303,1.),(1.00000284669049,
0.960470921313707,1.),(1.00000284520862,0.960491498623802,1.),(1.00000284155124,
0.960542284905421,1.),(1.00000284016333,0.960561557334819,1.),(1.00000283831761,
0.960587186968871,1.),(1.00000285326178,0.960379672542332,1.),(1.00000294182501,
0.959149885586877,1.),(1.00000306027874,0.957505039829061,1.),(1.00000326284385,
0.954692225357289,1.),(1.00000330607674,0.954091894504147,1.),(1.00000336322261,
0.953298368221104,1.),(1.00000337481016,0.953137463832346,1.),(1.00000338949359,
0.952933570057739,1.),(1.00000339244022,0.952892653107387,1.),(1.00000339687514,
0.952831070026665,1.),(1.00000339835593,0.952810507723471,1.),(1.00000340132251,
0.952769313832698,1.),(1.00000340517493,0.952715819204016,1.),(1.00000339803007,
0.9528150326048,1.),(1.0000033923405,0.952894037921842,1.),(1.0000033640243,
0.953287236017829,1.),(1.0000033417926,0.953595944837787,1.),(1.00000323275155,
0.95511008637556,1.),(1.00000315226282,0.956227751003349,1.),(1.00000300554034,
0.95826513604973,1.),(1.00000293927507,0.959185294029097,1.),(1.0000028519299,
0.960398167032383,1.),(1.00000282483424,0.960774416805573,1.),(1.00000277506302,
0.961465538790771,1.),(1.00000275232028,0.961781343928606,1.),(1.00000265174015,
0.96317799730065,1.),(1.00000261355939,0.963708174443108,1.),(1.00000263292298,
0.963439292028068,1.)))
REPRESENTATION_ITEM('')
SURFACE()
);
#3013=(
BOUNDED_SURFACE()
B_SPLINE_SURFACE(3,2,((#198480,#198481,#198482),(#198483,#198484,#198485),
(#198486,#198487,#198488),(#198489,#198490,#198491),(#198492,#198493,#198494),
(#198495,#198496,#198497)),.UNSPECIFIED.,.F.,.F.,.F.)
B_SPLINE_SURFACE_WITH_KNOTS((4,2,4),(3,3),(-0.000109518730889342,0.000547593654446629,
0.00109518730889329),(-0.00197443491225529,1.),.UNSPECIFIED.)
GEOMETRIC_REPRESENTATION_ITEM()
RATIONAL_B_SPLINE_SURFACE(((1.00002435441833,0.993832559842802,1.),(1.00001601188437,
0.995945198226732,1.),(1.0000094741473,0.997600795233666,1.),(1.00000179564523,
0.999545276164647,1.),(0.999999971260214,1.00000727797757,1.),(1.,1.,1.)))
REPRESENTATION_ITEM('')
SURFACE()
);
#3014=(
BOUNDED_SURFACE()
B_SPLINE_SURFACE(3,2,((#198531,#198532,#198533),(#198534,#198535,#198536),
(#198537,#198538,#198539),(#198540,#198541,#198542)),.UNSPECIFIED.,.F.,
 .F.,.F.)
B_SPLINE_SURFACE_WITH_KNOTS((4,4),(3,3),(0.0169795328233838,0.0259332885708231),
(0.,1.),.UNSPECIFIED.)
GEOMETRIC_REPRESENTATION_ITEM()
RATIONAL_B_SPLINE_SURFACE(((1.,0.957225253293536,1.),(1.,0.957330219064779,
1.),(1.,0.957420194105006,1.),(1.,0.95749691742527,1.)))
REPRESENTATION_ITEM('')
SURFACE()
);
#3015=(
BOUNDED_SURFACE()
B_SPLINE_SURFACE(3,2,((#198553,#198554,#198555),(#198556,#198557,#198558),
(#198559,#198560,#198561),(#198562,#198563,#198564)),.UNSPECIFIED.,.F.,
 .F.,.F.)
B_SPLINE_SURFACE_WITH_KNOTS((4,4),(3,3),(0.00708837036243835,0.00717746991701786),
(0.,1.),.UNSPECIFIED.)
GEOMETRIC_REPRESENTATION_ITEM()
RATIONAL_B_SPLINE_SURFACE(((1.,0.994244619571122,1.),(1.,0.994515217115564,
1.),(1.,0.994723691418642,1.),(1.,0.99486030168986,1.)))
REPRESENTATION_ITEM('')
SURFACE()
);
#3016=(
BOUNDED_SURFACE()
B_SPLINE_SURFACE(3,2,((#198574,#198575,#198576),(#198577,#198578,#198579),
(#198580,#198581,#198582),(#198583,#198584,#198585),(#198586,#198587,#198588),
(#198589,#198590,#198591),(#198592,#198593,#198594),(#198595,#198596,#198597),
(#198598,#198599,#198600),(#198601,#198602,#198603)),.UNSPECIFIED.,.F.,
 .F.,.F.)
B_SPLINE_SURFACE_WITH_KNOTS((4,2,2,2,4),(3,3),(2.16840434497101E-19,0.000213802025234883,
0.000427604050469766,0.000641406075704648,0.00085520810093953),(0.,1.),
 .UNSPECIFIED.)
GEOMETRIC_REPRESENTATION_ITEM()
RATIONAL_B_SPLINE_SURFACE(((1.,0.946111573410138,1.),(1.,0.947006419495448,
1.),(1.,0.94806750540417,1.),(1.,0.949985245580726,1.),(1.,0.950885821685186,
1.),(1.,0.952671230936143,1.),(1.,0.95357069077605,1.),(1.,0.955449705779053,
1.),(1.,0.956409634187462,1.),(1.,0.957225253284162,1.)))
REPRESENTATION_ITEM('')
SURFACE()
);
#3017=(
BOUNDED_SURFACE()
B_SPLINE_SURFACE(3,2,((#198702,#198703,#198704),(#198705,#198706,#198707),
(#198708,#198709,#198710),(#198711,#198712,#198713),(#198714,#198715,#198716),
(#198717,#198718,#198719),(#198720,#198721,#198722),(#198723,#198724,#198725),
(#198726,#198727,#198728),(#198729,#198730,#198731),(#198732,#198733,#198734),
(#198735,#198736,#198737),(#198738,#198739,#198740),(#198741,#198742,#198743),
(#198744,#198745,#198746),(#198747,#198748,#198749),(#198750,#198751,#198752),
(#198753,#198754,#198755),(#198756,#198757,#198758),(#198759,#198760,#198761)),
 .UNSPECIFIED.,.F.,.F.,.F.)
B_SPLINE_SURFACE_WITH_KNOTS((4,2,2,2,2,2,2,2,2,4),(3,3),(0.0241892472826494,
0.0245055239061063,0.0248218005295631,0.0251380771530199,0.0252962154647483,
0.0254543537764767,0.0257706303999336,0.0260869070233904,0.0264031836468472,
0.0267194602703041),(0.,1.),.UNSPECIFIED.)
GEOMETRIC_REPRESENTATION_ITEM()
RATIONAL_B_SPLINE_SURFACE(((1.,0.929973550212778,1.),(1.,0.930197351202751,
1.),(1.,0.930513290387209,1.),(1.,0.930996534931652,1.),(1.,0.931814475301649,
1.),(1.,0.93305861889435,1.),(1.,0.933512667464957,1.),(1.,0.934381592790984,
1.),(1.,0.934697923125669,1.),(1.,0.935467938930732,1.),(1.,0.935923141258381,
1.),(1.,0.937089763990058,1.),(1.,0.937772194692309,1.),(1.,0.939224429356622,
1.),(1.,0.94003447069213,1.),(1.,0.941810586362858,1.),(1.,0.942756891232808,
1.),(1.,0.944448481966905,1.),(1.,0.945215424202475,1.),(1.,0.946111573410157,
1.)))
REPRESENTATION_ITEM('')
SURFACE()
);
#3018=(
BOUNDED_SURFACE()
B_SPLINE_SURFACE(3,2,((#198912,#198913,#198914),(#198915,#198916,#198917),
(#198918,#198919,#198920),(#198921,#198922,#198923)),.UNSPECIFIED.,.F.,
 .F.,.F.)
B_SPLINE_SURFACE_WITH_KNOTS((4,4),(3,3),(0.0252170418335343,0.0258229913570786),
(0.,1.),.UNSPECIFIED.)
GEOMETRIC_REPRESENTATION_ITEM()
RATIONAL_B_SPLINE_SURFACE(((1.,0.930836001346604,1.),(1.,0.9307923293152,
1.),(1.,0.930500666506043,1.),(1.,0.929973550212784,1.)))
REPRESENTATION_ITEM('')
SURFACE()
);
#3019=(
BOUNDED_SURFACE()
B_SPLINE_SURFACE(3,2,((#198929,#198930,#198931),(#198932,#198933,#198934),
(#198935,#198936,#198937),(#198938,#198939,#198940)),.UNSPECIFIED.,.F.,
 .F.,.F.)
B_SPLINE_SURFACE_WITH_KNOTS((4,4),(3,3),(0.0413352581734093,0.045313001148136),
(0.,1.),.UNSPECIFIED.)
GEOMETRIC_REPRESENTATION_ITEM()
RATIONAL_B_SPLINE_SURFACE(((1.,0.932166688794147,1.),(1.,0.93183558573748,
1.),(1.,0.931353352247314,1.),(1.,0.930836001346602,1.)))
REPRESENTATION_ITEM('')
SURFACE()
);
#3020=(
BOUNDED_SURFACE()
B_SPLINE_SURFACE(3,2,((#198949,#198950,#198951),(#198952,#198953,#198954),
(#198955,#198956,#198957),(#198958,#198959,#198960),(#198961,#198962,#198963),
(#198964,#198965,#198966)),.UNSPECIFIED.,.F.,.F.,.F.)
B_SPLINE_SURFACE_WITH_KNOTS((4,2,4),(3,3),(0.0163865690223841,0.0292596031542503,
0.0419823306135875),(0.,1.00027232565654),.UNSPECIFIED.)
GEOMETRIC_REPRESENTATION_ITEM()
RATIONAL_B_SPLINE_SURFACE(((1.,0.997741854080557,1.00000122990214),(1.,
0.997128059065537,1.0000015642064),(1.,0.996318687779106,1.00000200503153),
(1.,0.994008737908883,1.00000326314876),(1.,0.992515369868671,1.00000407651363),
(1.,0.990483423032272,1.00000518321614)))
REPRESENTATION_ITEM('')
SURFACE()
);
#3021=(
BOUNDED_SURFACE()
B_SPLINE_SURFACE(3,2,((#198996,#198997,#198998),(#198999,#199000,#199001),
(#199002,#199003,#199004),(#199005,#199006,#199007)),.UNSPECIFIED.,.F.,
 .F.,.F.)
B_SPLINE_SURFACE_WITH_KNOTS((4,4),(3,3),(0.0181935747412957,0.0490322053436587),
(0.,1.00237065770204),.UNSPECIFIED.)
GEOMETRIC_REPRESENTATION_ITEM()
RATIONAL_B_SPLINE_SURFACE(((1.,0.989924970143594,1.00004776889425),(1.,
0.991156791509079,1.00004192844064),(1.,0.991768207325747,1.00003902952541),
(1.,0.992256661054546,1.00003671361222)))
REPRESENTATION_ITEM('')
SURFACE()
);
#3022=(
BOUNDED_SURFACE()
B_SPLINE_SURFACE(3,2,((#199037,#199038,#199039),(#199040,#199041,#199042),
(#199043,#199044,#199045),(#199046,#199047,#199048)),.UNSPECIFIED.,.F.,
 .F.,.F.)
B_SPLINE_SURFACE_WITH_KNOTS((4,4),(3,3),(0.0486839608469686,0.0783506339606883),
(0.,1.00251465406579),.UNSPECIFIED.)
GEOMETRIC_REPRESENTATION_ITEM()
RATIONAL_B_SPLINE_SURFACE(((1.,0.993081781376145,1.00003479385318),(1.,
0.992621487987293,1.00003710881046),(1.,0.992054572782517,1.00003996000171),
(1.,0.990843694193378,1.00004604988325)))
REPRESENTATION_ITEM('')
SURFACE()
);
#3023=(
BOUNDED_SURFACE()
B_SPLINE_SURFACE(3,2,((#199078,#199079,#199080),(#199081,#199082,#199083),
(#199084,#199085,#199086),(#199087,#199088,#199089),(#199090,#199091,#199092),
(#199093,#199094,#199095)),.UNSPECIFIED.,.F.,.F.,.F.)
B_SPLINE_SURFACE_WITH_KNOTS((4,2,4),(3,3),(0.0166253761100808,0.0283648343214889,
0.0401042925328971),(0.,1.),.UNSPECIFIED.)
GEOMETRIC_REPRESENTATION_ITEM()
RATIONAL_B_SPLINE_SURFACE(((1.,0.99500220761949,1.),(1.,0.995241643636696,
1.),(1.,0.995238480184742,1.),(1.,0.994937803535913,1.),(1.,0.99463876407346,
1.),(1.,0.994244619571122,1.)))
REPRESENTATION_ITEM('')
SURFACE()
);
#3024=(
BOUNDED_SURFACE()
B_SPLINE_SURFACE(3,2,((#207098,#207099,#207100),(#207101,#207102,#207103),
(#207104,#207105,#207106),(#207107,#207108,#207109),(#207110,#207111,#207112),
(#207113,#207114,#207115)),.UNSPECIFIED.,.F.,.F.,.F.)
B_SPLINE_SURFACE_WITH_KNOTS((4,2,4),(3,3),(0.,0.000611885440421095,0.00122377088084219),
(0.,1.),.UNSPECIFIED.)
GEOMETRIC_REPRESENTATION_ITEM()
RATIONAL_B_SPLINE_SURFACE(((1.,0.713250449154079,1.),(1.,0.672263173507019,
1.),(1.,0.648659882421647,1.),(1.,0.648739723662275,1.),(1.,0.672275262307808,
1.),(1.,0.713250449154082,1.)))
REPRESENTATION_ITEM('')
SURFACE()
);
#3025=(
BOUNDED_SURFACE()
B_SPLINE_SURFACE(3,2,((#207212,#207213,#207214),(#207215,#207216,#207217),
(#207218,#207219,#207220),(#207221,#207222,#207223),(#207224,#207225,#207226),
(#207227,#207228,#207229),(#207230,#207231,#207232),(#207233,#207234,#207235),
(#207236,#207237,#207238),(#207239,#207240,#207241)),.UNSPECIFIED.,.F.,
 .F.,.F.)
B_SPLINE_SURFACE_WITH_KNOTS((4,2,2,2,4),(3,3),(-1.10588621593521E-17,0.00061030576480229,
0.00122061152960459,0.00183091729440689,0.0024412230592092),(0.,1.),
 .UNSPECIFIED.)
GEOMETRIC_REPRESENTATION_ITEM()
RATIONAL_B_SPLINE_SURFACE(((1.,0.727552664059041,1.),(1.,0.745088511631937,
1.),(1.,0.761651043043578,1.),(1.,0.793171709476032,1.),(1.,0.808261553243384,
1.),(1.,0.836218122216209,1.),(1.,0.849115521102991,1.),(1.,0.872797166619617,
1.),(1.,0.883451618896464,1.),(1.,0.892325300547709,1.)))
REPRESENTATION_ITEM('')
SURFACE()
);
#3026=(
BOUNDED_SURFACE()
B_SPLINE_SURFACE(3,2,((#207358,#207359,#207360),(#207361,#207362,#207363),
(#207364,#207365,#207366),(#207367,#207368,#207369)),.UNSPECIFIED.,.F.,
 .F.,.F.)
B_SPLINE_SURFACE_WITH_KNOTS((4,4),(3,3),(0.,0.010514647628205),(0.,1.),
 .UNSPECIFIED.)
GEOMETRIC_REPRESENTATION_ITEM()
RATIONAL_B_SPLINE_SURFACE(((1.,0.727552664059029,1.),(1.,0.728396913847474,
1.),(1.,0.728235528042243,1.),(1.,0.727880838895167,1.)))
REPRESENTATION_ITEM('')
SURFACE()
);
#3027=(
BOUNDED_SURFACE()
B_SPLINE_SURFACE(3,2,((#207427,#207428,#207429),(#207430,#207431,#207432),
(#207433,#207434,#207435),(#207436,#207437,#207438),(#207439,#207440,#207441),
(#207442,#207443,#207444),(#207445,#207446,#207447),(#207448,#207449,#207450),
(#207451,#207452,#207453),(#207454,#207455,#207456)),.UNSPECIFIED.,.F.,
 .F.,.F.)
B_SPLINE_SURFACE_WITH_KNOTS((4,2,2,2,4),(3,3),(-8.17201003445707E-5,0.000594463573430658,
0.00118892714686131,0.00178339072029198,0.00245957439406716),(0.,1.00071180428484),
 .UNSPECIFIED.)
GEOMETRIC_REPRESENTATION_ITEM()
RATIONAL_B_SPLINE_SURFACE(((1.,0.926970074644159,1.00010396602758),(1.,
0.931625564084532,1.00009733843292),(1.,0.925916756569445,1.00010546554022),
(1.,0.902068515312624,1.00013941610084),(1.,0.885944725818379,1.00016237006574),
(1.,0.848477324278585,1.00021570897966),(1.,0.827049589649371,1.0002462136863),
(1.,0.776935720203443,1.00031755622031),(1.,0.74806977061884,1.00035865003351),
(1.,0.716291963603933,1.0004038891919)))
REPRESENTATION_ITEM('')
SURFACE()
);
#3028=(
BOUNDED_SURFACE()
B_SPLINE_SURFACE(3,2,((#207529,#207530,#207531),(#207532,#207533,#207534),
(#207535,#207536,#207537),(#207538,#207539,#207540),(#207541,#207542,#207543),
(#207544,#207545,#207546)),.UNSPECIFIED.,.F.,.F.,.F.)
B_SPLINE_SURFACE_WITH_KNOTS((4,2,4),(3,3),(-1.38777878078145E-17,0.0041604828508626,
0.00832096570172521),(0.,1.),.UNSPECIFIED.)
GEOMETRIC_REPRESENTATION_ITEM()
RATIONAL_B_SPLINE_SURFACE(((1.,0.928260885086434,1.),(1.,0.928493402693592,
1.),(1.,0.928615016565842,1.),(1.,0.928561249118847,1.),(1.,0.928391240061757,
1.),(1.,0.928132015153712,1.)))
REPRESENTATION_ITEM('')
SURFACE()
);
#3029=(
BOUNDED_SURFACE()
B_SPLINE_SURFACE(3,2,((#207588,#207589,#207590),(#207591,#207592,#207593),
(#207594,#207595,#207596),(#207597,#207598,#207599),(#207600,#207601,#207602),
(#207603,#207604,#207605),(#207606,#207607,#207608),(#207609,#207610,#207611),
(#207612,#207613,#207614),(#207615,#207616,#207617)),.UNSPECIFIED.,.F.,
 .F.,.F.)
B_SPLINE_SURFACE_WITH_KNOTS((4,2,2,2,4),(3,3),(-0.00023493367097703,0.000587334177442414,
0.00117466835488487,0.00176200253232733,0.00258427038074678),(-0.000330771740685424,
1.),.UNSPECIFIED.)
GEOMETRIC_REPRESENTATION_ITEM()
RATIONAL_B_SPLINE_SURFACE(((1.0001975152061,0.701432767973641,1.),(1.00017087577531,
0.741701369416836,1.),(1.00014739521264,0.777194973892298,1.),(1.00011108291111,
0.832085245739731,1.),(1.00009703796778,0.853315812919012,1.),(1.00007293188498,
0.889754963915332,1.),(1.00006264550326,0.905304027592269,1.),(1.00004609326443,
0.930324663863228,1.),(1.00004377591455,0.933827608038183,1.),(1.00005227954766,
0.920973376459142,1.)))
REPRESENTATION_ITEM('')
SURFACE()
);
#3030=(
BOUNDED_SURFACE()
B_SPLINE_SURFACE(3,2,((#207749,#207750,#207751),(#207752,#207753,#207754),
(#207755,#207756,#207757),(#207758,#207759,#207760)),.UNSPECIFIED.,.F.,
 .F.,.F.)
B_SPLINE_SURFACE_WITH_KNOTS((4,4),(3,3),(0.,0.0107001581246114),(0.,1.),
 .UNSPECIFIED.)
GEOMETRIC_REPRESENTATION_ITEM()
RATIONAL_B_SPLINE_SURFACE(((1.,0.73489735095993,1.),(1.,0.734875794442845,
1.),(1.,0.734252034560147,1.),(1.,0.73129868040477,1.)))
REPRESENTATION_ITEM('')
SURFACE()
);
#3031=(
BOUNDED_SURFACE()
B_SPLINE_SURFACE(3,2,((#207783,#207784,#207785),(#207786,#207787,#207788),
(#207789,#207790,#207791),(#207792,#207793,#207794)),.UNSPECIFIED.,.F.,
 .F.,.F.)
B_SPLINE_SURFACE_WITH_KNOTS((4,4),(3,3),(0.,0.000517122404042923),(0.,1.),
 .UNSPECIFIED.)
GEOMETRIC_REPRESENTATION_ITEM()
RATIONAL_B_SPLINE_SURFACE(((1.,0.707106781186546,1.),(1.,0.731070766440982,
1.),(1.,0.753745435486364,1.),(1.,0.77196935846749,1.)))
REPRESENTATION_ITEM('')
SURFACE()
);
#3032=(
BOUNDED_SURFACE()
B_SPLINE_SURFACE(3,2,((#207836,#207837,#207838),(#207839,#207840,#207841),
(#207842,#207843,#207844),(#207845,#207846,#207847),(#207848,#207849,#207850),
(#207851,#207852,#207853)),.UNSPECIFIED.,.F.,.F.,.F.)
B_SPLINE_SURFACE_WITH_KNOTS((4,2,4),(3,3),(-2.92626166353837E-16,0.00117037761632422,
0.00234075523264872),(0.,1.),.UNSPECIFIED.)
GEOMETRIC_REPRESENTATION_ITEM()
RATIONAL_B_SPLINE_SURFACE(((1.,0.888647434958264,1.),(1.,0.871248161544161,
1.),(1.,0.84779606985727,1.),(1.,0.794668809935237,1.),(1.,0.764625718490638,
1.),(1.,0.731298680404815,1.)))
REPRESENTATION_ITEM('')
SURFACE()
);
#3033=(
BOUNDED_SURFACE()
B_SPLINE_SURFACE(3,2,((#207964,#207965,#207966),(#207967,#207968,#207969),
(#207970,#207971,#207972),(#207973,#207974,#207975),(#207976,#207977,#207978),
(#207979,#207980,#207981),(#207982,#207983,#207984),(#207985,#207986,#207987),
(#207988,#207989,#207990),(#207991,#207992,#207993),(#207994,#207995,#207996),
(#207997,#207998,#207999)),.UNSPECIFIED.,.F.,.F.,.F.)
B_SPLINE_SURFACE_WITH_KNOTS((4,2,2,2,2,4),(3,3),(-0.000229639107487331,
0.000574097768718188,0.00114819553743641,0.00143524442179553,0.00172229330615464,
0.00252603018236012),(-0.000695063111154208,1.00310110558421),
 .UNSPECIFIED.)
GEOMETRIC_REPRESENTATION_ITEM()
RATIONAL_B_SPLINE_SURFACE(((1.00041583704952,0.699935521594427,1.00185976660778),
(1.00036124087235,0.739331658718599,1.00161559368639),(1.00031293869035,
0.774186102461259,1.00139956968065),(1.00023813854648,0.82816125013087,
1.00106503765666),(1.0002101364639,0.848367314777069,1.00093980269216),
(1.00017367979131,0.874674139669543,1.00077675588718),(1.00016260452917,
0.882665954637282,1.0007272234977),(1.00014324788421,0.896633545018679,
1.00064065390999),(1.00013479460749,0.902733357609951,1.00060284794298),
(1.00010983737982,0.920742280843341,1.0004912306191),(1.00010567595172,
0.92374513197171,1.00047261927834),(1.00012224113811,0.911791834348499,
1.00054670450126)))
REPRESENTATION_ITEM('')
SURFACE()
);
#3034=(
BOUNDED_SURFACE()
B_SPLINE_SURFACE(3,2,((#208067,#208068,#208069),(#208070,#208071,#208072),
(#208073,#208074,#208075),(#208076,#208077,#208078)),.UNSPECIFIED.,.F.,
 .F.,.F.)
B_SPLINE_SURFACE_WITH_KNOTS((4,4),(3,3),(0.,0.00980967348625105),(0.,1.),
 .UNSPECIFIED.)
GEOMETRIC_REPRESENTATION_ITEM()
RATIONAL_B_SPLINE_SURFACE(((1.,0.733631070205817,1.),(1.,0.732913032274794,
1.),(1.,0.731754232439324,1.),(1.,0.729712990977684,1.)))
REPRESENTATION_ITEM('')
SURFACE()
);
#3035=(
BOUNDED_SURFACE()
B_SPLINE_SURFACE(3,2,((#208090,#208091,#208092),(#208093,#208094,#208095),
(#208096,#208097,#208098),(#208099,#208100,#208101),(#208102,#208103,#208104),
(#208105,#208106,#208107)),.UNSPECIFIED.,.F.,.F.,.F.)
B_SPLINE_SURFACE_WITH_KNOTS((4,2,4),(3,3),(-1.04083408558608E-17,0.00416021787251448,
0.00832043574502897),(0.,1.),.UNSPECIFIED.)
GEOMETRIC_REPRESENTATION_ITEM()
RATIONAL_B_SPLINE_SURFACE(((1.,0.91815876419713,1.),(1.,0.918478576988139,
1.),(1.,0.918702883828552,1.),(1.,0.918900670636956,1.),(1.,0.918880394705029,
1.),(1.,0.918792784744087,1.)))
REPRESENTATION_ITEM('')
SURFACE()
);
#3036=(
BOUNDED_SURFACE()
B_SPLINE_SURFACE(3,2,((#208140,#208141,#208142),(#208143,#208144,#208145),
(#208146,#208147,#208148),(#208149,#208150,#208151),(#208152,#208153,#208154),
(#208155,#208156,#208157)),.UNSPECIFIED.,.F.,.F.,.F.)
B_SPLINE_SURFACE_WITH_KNOTS((4,2,4),(3,3),(0.,0.00128099832444667,0.00256199664889334),
(0.,1.),.UNSPECIFIED.)
GEOMETRIC_REPRESENTATION_ITEM()
RATIONAL_B_SPLINE_SURFACE(((1.,0.901968956514557,1.),(1.,0.883369478142107,
1.),(1.,0.857628018054164,1.),(1.,0.799434735390564,1.),(1.,0.766284883162671,
1.),(1.,0.729712990977659,1.)))
REPRESENTATION_ITEM('')
SURFACE()
);
#3037=(
BOUNDED_SURFACE()
B_SPLINE_SURFACE(3,2,((#208301,#208302,#208303),(#208304,#208305,#208306),
(#208307,#208308,#208309),(#208310,#208311,#208312),(#208313,#208314,#208315),
(#208316,#208317,#208318),(#208319,#208320,#208321),(#208322,#208323,#208324),
(#208325,#208326,#208327),(#208328,#208329,#208330)),.UNSPECIFIED.,.F.,
 .F.,.F.)
B_SPLINE_SURFACE_WITH_KNOTS((4,2,2,2,4),(3,3),(-9.48676900924816E-18,0.000575184387543924,
0.00115036877508786,0.00172555316263179,0.00230073755017573),(0.,1.00079242647114),
 .UNSPECIFIED.)
GEOMETRIC_REPRESENTATION_ITEM()
RATIONAL_B_SPLINE_SURFACE(((1.,0.918093911035446,1.00012980910609),(1.,
0.92016598823334,1.00012652516844),(1.,0.91537620632456,1.00013411626839),
(1.,0.895563982165149,1.00016551573015),(1.,0.880770844269308,1.00018896067827),
(1.,0.8454580472065,1.00024492626859),(1.,0.825177021514163,1.00027706871183),
(1.,0.780124700037101,1.00034847001608),(1.,0.75591069420419,1.00038684565447),
(1.,0.729555383368477,1.00042861494639)))
REPRESENTATION_ITEM('')
SURFACE()
);
#3038=(
BOUNDED_SURFACE()
B_SPLINE_SURFACE(3,2,((#208401,#208402,#208403),(#208404,#208405,#208406),
(#208407,#208408,#208409),(#208410,#208411,#208412)),.UNSPECIFIED.,.F.,
 .F.,.F.)
B_SPLINE_SURFACE_WITH_KNOTS((4,4),(3,3),(0.,0.00972938600277916),(0.,1.),
 .UNSPECIFIED.)
GEOMETRIC_REPRESENTATION_ITEM()
RATIONAL_B_SPLINE_SURFACE(((1.,0.729533004763605,1.),(1.,0.730591519138966,
1.),(1.,0.730312610923774,1.),(1.,0.729769521153222,1.)))
REPRESENTATION_ITEM('')
SURFACE()
);
#3039=(
BOUNDED_SURFACE()
B_SPLINE_SURFACE(3,2,((#208435,#208436,#208437),(#208438,#208439,#208440),
(#208441,#208442,#208443),(#208444,#208445,#208446)),.UNSPECIFIED.,.F.,
 .F.,.F.)
B_SPLINE_SURFACE_WITH_KNOTS((4,4),(3,3),(-6.39679281766448E-18,3.42512019832298E-5),
(0.,1.),.UNSPECIFIED.)
GEOMETRIC_REPRESENTATION_ITEM()
RATIONAL_B_SPLINE_SURFACE(((1.,0.707106781186548,1.),(1.,0.70842711846827,
1.),(1.,0.709730890158149,1.),(1.,0.711017327239758,1.)))
REPRESENTATION_ITEM('')
SURFACE()
);
#3040=(
BOUNDED_SURFACE()
B_SPLINE_SURFACE(3,2,((#208458,#208459,#208460),(#208461,#208462,#208463),
(#208464,#208465,#208466),(#208467,#208468,#208469),(#208470,#208471,#208472),
(#208473,#208474,#208475),(#208476,#208477,#208478),(#208479,#208480,#208481)),
 .UNSPECIFIED.,.F.,.F.,.F.)
B_SPLINE_SURFACE_WITH_KNOTS((4,2,2,4),(3,3),(-4.40186082029115E-17,0.00128517876997136,
0.00192776815495707,0.00257035753994277),(0.,1.),.UNSPECIFIED.)
GEOMETRIC_REPRESENTATION_ITEM()
RATIONAL_B_SPLINE_SURFACE(((1.,0.729533004763577,1.),(1.,0.766429181343272,
1.),(1.,0.799163813689396,1.),(1.,0.843673470277402,1.),(1.,0.857403797499188,
1.),(1.,0.882315838155618,1.),(1.,0.893652235396326,1.),(1.,0.903015666115932,
1.)))
REPRESENTATION_ITEM('')
SURFACE()
);
#3041=(
BOUNDED_SURFACE()
B_SPLINE_SURFACE(3,2,((#208605,#208606,#208607),(#208608,#208609,#208610),
(#208611,#208612,#208613),(#208614,#208615,#208616)),.UNSPECIFIED.,.F.,
 .F.,.F.)
B_SPLINE_SURFACE_WITH_KNOTS((4,4),(3,3),(-6.61363325216158E-18,2.21589532008063E-5),
(0.,1.),.UNSPECIFIED.)
GEOMETRIC_REPRESENTATION_ITEM()
RATIONAL_B_SPLINE_SURFACE(((1.,0.707106781186552,1.),(1.,0.707961610595566,
1.),(1.,0.708809519028292,1.),(1.,0.709650295730098,1.)))
REPRESENTATION_ITEM('')
SURFACE()
);
#3042=(
BOUNDED_SURFACE()
B_SPLINE_SURFACE(3,2,((#208682,#208683,#208684),(#208685,#208686,#208687),
(#208688,#208689,#208690),(#208691,#208692,#208693)),.UNSPECIFIED.,.F.,
 .F.,.F.)
B_SPLINE_SURFACE_WITH_KNOTS((4,4),(3,3),(0.00880203782093267,0.00917783640854858),
(0.,1.),.UNSPECIFIED.)
GEOMETRIC_REPRESENTATION_ITEM()
RATIONAL_B_SPLINE_SURFACE(((1.,0.928452770819611,1.),(1.,0.928460035446405,
1.),(1.,0.928468213633922,1.),(1.,0.928477160954726,1.)))
REPRESENTATION_ITEM('')
SURFACE()
);
#3043=(
BOUNDED_SURFACE()
B_SPLINE_SURFACE(3,2,((#208699,#208700,#208701),(#208702,#208703,#208704),
(#208705,#208706,#208707),(#208708,#208709,#208710)),.UNSPECIFIED.,.F.,
 .F.,.F.)
B_SPLINE_SURFACE_WITH_KNOTS((4,4),(3,3),(0.,0.000210836370419711),(0.,1.),
 .UNSPECIFIED.)
GEOMETRIC_REPRESENTATION_ITEM()
RATIONAL_B_SPLINE_SURFACE(((1.,0.928492930368189,1.),(1.,0.928487440815482,
1.),(1.,0.928482179049582,1.),(1.,0.928477160954739,1.)))
REPRESENTATION_ITEM('')
SURFACE()
);
#3044=(
BOUNDED_SURFACE()
B_SPLINE_SURFACE(3,2,((#208719,#208720,#208721),(#208722,#208723,#208724),
(#208725,#208726,#208727),(#208728,#208729,#208730),(#208731,#208732,#208733),
(#208734,#208735,#208736),(#208737,#208738,#208739),(#208740,#208741,#208742),
(#208743,#208744,#208745),(#208746,#208747,#208748),(#208749,#208750,#208751),
(#208752,#208753,#208754)),.UNSPECIFIED.,.F.,.F.,.F.)
B_SPLINE_SURFACE_WITH_KNOTS((4,2,2,2,2,4),(3,3),(-0.000206342901056451,
0.000515857252641128,0.00103171450528226,0.00154757175792339,0.00180550038424395,
0.00226977191162085),(-0.00146001009681673,1.00056090637502),
 .UNSPECIFIED.)
GEOMETRIC_REPRESENTATION_ITEM()
RATIONAL_B_SPLINE_SURFACE(((1.00055460374899,0.809961833654899,1.00021287626228),
(1.00047293149373,0.837947301944298,1.00018152760215),(1.00039897300112,
0.863289605070118,1.00015313975317),(1.00028590192954,0.90203405847295,
1.00010973913222),(1.00024196311713,0.917089945412939,1.00009287388352),
(1.00016992773463,0.941773283793271,1.00006522419127),(1.00014170965431,
0.951442371408365,1.00005439310786),(1.00012570829839,0.956925328102896,
1.00004825122936),(1.00012496629093,0.957179581229155,1.00004796642102),
(1.00013594085639,0.953419083216919,1.00005217884201),(1.00015771831893,
0.945956910345841,1.00006053779169),(1.00018769789889,0.935684234741691,
1.0000720450001)))
REPRESENTATION_ITEM('')
SURFACE()
);
#3045=(
BOUNDED_SURFACE()
B_SPLINE_SURFACE(3,2,((#208813,#208814,#208815),(#208816,#208817,#208818),
(#208819,#208820,#208821),(#208822,#208823,#208824),(#208825,#208826,#208827),
(#208828,#208829,#208830),(#208831,#208832,#208833),(#208834,#208835,#208836),
(#208837,#208838,#208839),(#208840,#208841,#208842),(#208843,#208844,#208845),
(#208846,#208847,#208848)),.UNSPECIFIED.,.F.,.F.,.F.)
B_SPLINE_SURFACE_WITH_KNOTS((4,2,2,2,2,4),(3,3),(-0.000236631349860531,
0.000591578374651329,0.000887367561976994,0.00118315674930266,0.00177473512395399,
0.00260294484846584),(-0.00119575409929547,1.),.UNSPECIFIED.)
GEOMETRIC_REPRESENTATION_ITEM()
RATIONAL_B_SPLINE_SURFACE(((1.00021393343793,0.910544551738771,1.),(1.00016085325225,
0.932739828219605,1.),(1.00011637632197,0.951337686385449,1.),(1.00010674451532,
0.955365189471307,1.),(1.00010912168845,0.954371183627145,1.),(1.00012287489593,
0.948620332558914,1.),(1.0001340538894,0.943945879224083,1.),(1.00017581652603,
0.926482992559179,1.),(1.00021426650785,0.910405279824543,1.),(1.00031653395365,
0.86764253878067,1.),(1.00038632399849,0.838460098645234,1.),(1.0004622600014,
0.80670774966673,1.)))
REPRESENTATION_ITEM('')
SURFACE()
);
#3046=(
BOUNDED_SURFACE()
B_SPLINE_SURFACE(3,2,((#208999,#209000,#209001),(#209002,#209003,#209004),
(#209005,#209006,#209007),(#209008,#209009,#209010)),.UNSPECIFIED.,.F.,
 .F.,.F.)
B_SPLINE_SURFACE_WITH_KNOTS((4,4),(3,3),(-5.20417042793042E-18,0.000729297262992661),
(0.,1.),.UNSPECIFIED.)
GEOMETRIC_REPRESENTATION_ITEM()
RATIONAL_B_SPLINE_SURFACE(((1.,0.833636261310766,1.),(1.,0.833189131672253,
1.),(1.,0.83273693675361,1.),(1.,0.832279622729512,1.)))
REPRESENTATION_ITEM('')
SURFACE()
);
#3047=(
BOUNDED_SURFACE()
B_SPLINE_SURFACE(3,2,((#209016,#209017,#209018),(#209019,#209020,#209021),
(#209022,#209023,#209024),(#209025,#209026,#209027)),.UNSPECIFIED.,.F.,
 .F.,.F.)
B_SPLINE_SURFACE_WITH_KNOTS((4,4),(3,3),(-1.04083408558608E-17,0.000723082784825488),
(0.,1.),.UNSPECIFIED.)
GEOMETRIC_REPRESENTATION_ITEM()
RATIONAL_B_SPLINE_SURFACE(((1.,0.832455503270619,1.),(1.,0.832789231498785,
1.),(1.,0.833122604759493,1.),(1.,0.833454935865631,1.)))
REPRESENTATION_ITEM('')
SURFACE()
);
#3048=(
BOUNDED_SURFACE()
B_SPLINE_SURFACE(3,2,((#209033,#209034,#209035),(#209036,#209037,#209038),
(#209039,#209040,#209041),(#209042,#209043,#209044)),.UNSPECIFIED.,.F.,
 .F.,.F.)
B_SPLINE_SURFACE_WITH_KNOTS((4,4),(3,3),(0.,0.00158760011419447),(0.,1.),
 .UNSPECIFIED.)
GEOMETRIC_REPRESENTATION_ITEM()
RATIONAL_B_SPLINE_SURFACE(((1.,0.832279622729481,1.),(1.,0.842288514399813,
1.),(1.,0.850845187132399,1.),(1.,0.857972509692097,1.)))
REPRESENTATION_ITEM('')
SURFACE()
);
#3049=(
BOUNDED_SURFACE()
B_SPLINE_SURFACE(3,2,((#209107,#209108,#209109),(#209110,#209111,#209112),
(#209113,#209114,#209115),(#209116,#209117,#209118)),.UNSPECIFIED.,.F.,
 .F.,.F.)
B_SPLINE_SURFACE_WITH_KNOTS((4,4),(3,3),(-3.10081821330854E-17,0.00151853748946949),
(0.,1.),.UNSPECIFIED.)
GEOMETRIC_REPRESENTATION_ITEM()
RATIONAL_B_SPLINE_SURFACE(((1.,0.857104357126303,1.),(1.,0.850185325699861,
1.),(1.,0.84197601930101,1.),(1.,0.83245550327062,1.)))
REPRESENTATION_ITEM('')
SURFACE()
);
#3050=(
BOUNDED_SURFACE()
B_SPLINE_SURFACE(3,2,((#209184,#209185,#209186),(#209187,#209188,#209189),
(#209190,#209191,#209192),(#209193,#209194,#209195),(#209196,#209197,#209198),
(#209199,#209200,#209201),(#209202,#209203,#209204),(#209205,#209206,#209207)),
 .UNSPECIFIED.,.F.,.F.,.F.)
B_SPLINE_SURFACE_WITH_KNOTS((4,2,2,4),(3,3),(-0.000314953251722383,0.000787383129295151,
0.00157476625859271,0.00346448576890691),(0.,1.00393321929414),
 .UNSPECIFIED.)
GEOMETRIC_REPRESENTATION_ITEM()
RATIONAL_B_SPLINE_SURFACE(((1.,0.988639393495295,1.00008936751339),(1.,
0.99107983362604,1.00007016994098),(1.,0.987096480958425,1.00010150474011),
(1.,0.971752779728647,1.00022220502355),(1.,0.962780183976932,1.00029278739701),
(1.,0.924711164443769,1.00059225500129),(1.,0.884601626384202,1.00090777421924),
(1.,0.832272209417737,1.00131942036416)))
REPRESENTATION_ITEM('')
SURFACE()
);
#3051=(
BOUNDED_SURFACE()
B_SPLINE_SURFACE(3,2,((#209353,#209354,#209355),(#209356,#209357,#209358),
(#209359,#209360,#209361),(#209362,#209363,#209364),(#209365,#209366,#209367),
(#209368,#209369,#209370),(#209371,#209372,#209373),(#209374,#209375,#209376)),
 .UNSPECIFIED.,.F.,.F.,.F.)
B_SPLINE_SURFACE_WITH_KNOTS((4,2,2,4),(3,3),(-0.000315404934817324,0.00157702467408662,
0.00236553701112993,0.00346945428299001),(0.,1.00901231170094),
 .UNSPECIFIED.)
GEOMETRIC_REPRESENTATION_ITEM()
RATIONAL_B_SPLINE_SURFACE(((1.,0.830517951234993,1.00305485010237),(1.,
0.88317248166518,1.00210577202096),(1.,0.923525848545179,1.00137841777995),
(1.,0.962170244647943,1.00068186709361),(1.,0.971260847949517,1.0005180123926),
(1.,0.986851346814187,1.00023699952192),(1.,0.99108019029668,1.00016077621072),
(1.,0.988461418308015,1.00020797858959)))
REPRESENTATION_ITEM('')
SURFACE()
);
#3052=(
BOUNDED_SURFACE()
B_SPLINE_SURFACE(3,2,((#209509,#209510,#209511),(#209512,#209513,#209514),
(#209515,#209516,#209517),(#209518,#209519,#209520),(#209521,#209522,#209523),
(#209524,#209525,#209526),(#209527,#209528,#209529),(#209530,#209531,#209532),
(#209533,#209534,#209535),(#209536,#209537,#209538),(#209539,#209540,#209541),
(#209542,#209543,#209544),(#209545,#209546,#209547),(#209548,#209549,#209550),
(#209551,#209552,#209553),(#209554,#209555,#209556),(#209557,#209558,#209559),
(#209560,#209561,#209562)),.UNSPECIFIED.,.F.,.F.,.F.)
B_SPLINE_SURFACE_WITH_KNOTS((4,2,2,2,2,2,2,2,4),(3,3),(-0.000508741685376785,
0.00254370842688261,0.00381556264032431,0.00445148974704516,0.00476945330040559,
0.0049284350770858,0.00500792596542591,0.00504767140959596,0.0055961585391427),
(-0.00567142872297958,1.),.UNSPECIFIED.)
GEOMETRIC_REPRESENTATION_ITEM()
RATIONAL_B_SPLINE_SURFACE(((1.00013527605448,0.988073899798091,1.),(1.00011031929585,
0.990274117753778,1.),(1.00008545848001,0.992465877278369,1.),(1.00005043350393,
0.995553721434831,1.),(1.0000401547835,0.996459905831016,1.),(1.00002479414521,
0.997814118238588,1.),(1.0000196801218,0.99826497671417,1.),(1.00001206776935,
0.998936090892214,1.),(1.00000953704006,0.999159203039952,1.),(1.00000579625876,
0.999488994833659,1.),(1.00000455640789,0.999598301582191,1.),(1.00000275469915,
0.999757142399172,1.),(1.00000216079599,0.999809501617783,1.),(1.00000133818808,
0.999882023724343,1.),(1.00000107184386,0.999905504951442,1.),(0.999997744935146,
1.00019880923877,1.),(1.00000210718248,0.999814228249836,1.),(1.00039260038191,
0.965387876575058,1.)))
REPRESENTATION_ITEM('')
SURFACE()
);
#3053=(
BOUNDED_SURFACE()
B_SPLINE_SURFACE(3,2,((#209681,#209682,#209683),(#209684,#209685,#209686),
(#209687,#209688,#209689),(#209690,#209691,#209692),(#209693,#209694,#209695),
(#209696,#209697,#209698),(#209699,#209700,#209701),(#209702,#209703,#209704),
(#209705,#209706,#209707),(#209708,#209709,#209710),(#209711,#209712,#209713),
(#209714,#209715,#209716),(#209717,#209718,#209719),(#209720,#209721,#209722),
(#209723,#209724,#209725),(#209726,#209727,#209728),(#209729,#209730,#209731),
(#209732,#209733,#209734)),.UNSPECIFIED.,.F.,.F.,.F.)
B_SPLINE_SURFACE_WITH_KNOTS((4,2,2,2,2,2,2,2,4),(3,3),(-7.45388993583784E-20,
4.05793239028379E-5,8.11586478056759E-5,0.000162317295611352,0.000324634591222704,
0.000649269182445408,0.00129853836489082,0.00259707672978163,0.00519415345956326),
(0.,1.),.UNSPECIFIED.)
GEOMETRIC_REPRESENTATION_ITEM()
RATIONAL_B_SPLINE_SURFACE(((1.,0.999961923064171,1.),(1.,0.999961833753432,
1.),(1.,0.999944633098586,1.),(1.,0.999904212270329,1.),(1.,0.99988023258917,
1.),(1.,0.999806855851567,1.),(1.,0.999754783512162,1.),(1.,0.999595776401296,
1.),(1.,0.999485889992571,1.),(1.,0.999156267866573,1.),(1.,0.998933623645324,
1.),(1.,0.998262897761582,1.),(1.,0.997812273447783,1.),(1.,0.996459235447427,
1.),(1.,0.995553264664008,1.),(1.,0.992828768547989,1.),(1.,0.991003554465269,
1.),(1.,0.989172917436461,1.)))
REPRESENTATION_ITEM('')
SURFACE()
);
#3054=(
BOUNDED_SURFACE()
B_SPLINE_SURFACE(3,2,((#209860,#209861,#209862),(#209863,#209864,#209865),
(#209866,#209867,#209868),(#209869,#209870,#209871),(#209872,#209873,#209874),
(#209875,#209876,#209877),(#209878,#209879,#209880),(#209881,#209882,#209883),
(#209884,#209885,#209886),(#209887,#209888,#209889),(#209890,#209891,#209892),
(#209893,#209894,#209895),(#209896,#209897,#209898),(#209899,#209900,#209901),
(#209902,#209903,#209904),(#209905,#209906,#209907),(#209908,#209909,#209910),
(#209911,#209912,#209913)),.UNSPECIFIED.,.F.,.F.,.F.)
B_SPLINE_SURFACE_WITH_KNOTS((4,2,2,2,2,2,2,2,4),(3,3),(-0.000525941938450675,
0.00262970969225337,0.00394456453838006,0.00460199196144341,0.00493070567297508,
0.00509506252874091,0.00517724095662383,0.00521833017056529,0.00578536132295742),
(-0.00671701195452941,1.),.UNSPECIFIED.)
GEOMETRIC_REPRESENTATION_ITEM()
RATIONAL_B_SPLINE_SURFACE(((1.00016587740973,0.987652440486347,1.),(1.00013527423289,
0.989930475499347,1.),(1.00010479231153,0.992199484515042,1.),(1.00006184900674,
0.995396092253403,1.),(1.00004924669386,0.996334181463897,1.),(1.00003041237645,
0.997736167759121,1.),(1.00002414515887,0.998202686027925,1.),(1.00001481225861,
0.998897407157577,1.),(1.00001170892687,0.999128412532823,1.),(1.0000071206784,
0.999469951933241,1.),(1.00000559837997,0.999583268571811,1.),(1.0000033859316,
0.999747958495426,1.),(1.00000265749339,0.999802181877435,1.),(1.00000163926013,
0.999877976982937,1.),(1.00000131471708,0.999902135273186,1.),(0.999997166880602,
1.000210891347,1.),(1.00000159891618,0.999880980100307,1.),(1.00051507935168,
0.96165859498486,1.)))
REPRESENTATION_ITEM('')
SURFACE()
);
#3055=(
BOUNDED_SURFACE()
B_SPLINE_SURFACE(3,2,((#210041,#210042,#210043),(#210044,#210045,#210046),
(#210047,#210048,#210049),(#210050,#210051,#210052),(#210053,#210054,#210055),
(#210056,#210057,#210058),(#210059,#210060,#210061),(#210062,#210063,#210064)),
 .UNSPECIFIED.,.F.,.F.,.F.)
B_SPLINE_SURFACE_WITH_KNOTS((4,2,2,4),(3,3),(-0.000314549301296344,0.000786373253240854,
0.0015727465064817,0.00346004231425976),(0.,1.00377255784672),
 .UNSPECIFIED.)
GEOMETRIC_REPRESENTATION_ITEM()
RATIONAL_B_SPLINE_SURFACE(((1.,0.988289122120854,1.00008835992847),(1.,
0.990704624856171,1.00007013468087),(1.,0.986710803687609,1.00010026852365),
(1.,0.971342895247987,1.00021622117079),(1.,0.962359345953478,1.00028400308956),
(1.,0.924268992488747,1.00057139921325),(1.,0.884176841333546,1.00087389913212),
(1.,0.831820369843143,1.00126893476681)))
REPRESENTATION_ITEM('')
SURFACE()
);
#3056=(
BOUNDED_SURFACE()
B_SPLINE_SURFACE(3,2,((#210203,#210204,#210205),(#210206,#210207,#210208),
(#210209,#210210,#210211),(#210212,#210213,#210214),(#210215,#210216,#210217),
(#210218,#210219,#210220),(#210221,#210222,#210223),(#210224,#210225,#210226),
(#210227,#210228,#210229),(#210230,#210231,#210232),(#210233,#210234,#210235),
(#210236,#210237,#210238),(#210239,#210240,#210241),(#210242,#210243,#210244),
(#210245,#210246,#210247),(#210248,#210249,#210250),(#210251,#210252,#210253),
(#210254,#210255,#210256)),.UNSPECIFIED.,.F.,.F.,.F.)
B_SPLINE_SURFACE_WITH_KNOTS((4,2,2,2,2,2,2,2,4),(3,3),(-1.32137139771671E-19,
4.17669388829254E-5,8.35338777658508E-5,0.000167067755531702,0.000334135511063404,
0.000668271022126808,0.00133654204425361,0.00267308408850723,0.00534616817701446),
(0.,1.),.UNSPECIFIED.)
GEOMETRIC_REPRESENTATION_ITEM()
RATIONAL_B_SPLINE_SURFACE(((1.,0.999961923064171,1.),(1.,0.999961782802257,
1.),(1.,0.999943671528414,1.),(1.,0.999901604878771,1.),(1.,0.999876750335241,
1.),(1.,0.999800908054986,1.),(1.,0.99974715657318,1.),(1.,0.999583072363253,
1.),(1.,0.999469900307565,1.),(1.,0.999130340955253,1.),(1.,0.998901033022514,
1.),(1.,0.998210264756137,1.),(1.,0.997746391825068,1.),(1.,0.996353373847482,
1.),(1.,0.9954206326127,1.),(1.,0.992615540215937,1.),(1.,0.990736373728666,
1.),(1.,0.988851372352096,1.)))
REPRESENTATION_ITEM('')
SURFACE()
);
#3057=(
BOUNDED_SURFACE()
B_SPLINE_SURFACE(3,2,((#210379,#210380,#210381),(#210382,#210383,#210384),
(#210385,#210386,#210387),(#210388,#210389,#210390)),.UNSPECIFIED.,.F.,
 .F.,.F.)
B_SPLINE_SURFACE_WITH_KNOTS((4,4),(3,3),(-1.02728155843001E-17,0.0012351855748658),
(0.,1.),.UNSPECIFIED.)
GEOMETRIC_REPRESENTATION_ITEM()
RATIONAL_B_SPLINE_SURFACE(((1.,0.838149597872977,1.),(1.,0.845487721431554,
1.),(1.,0.851938880735554,1.),(1.,0.857509777230923,1.)))
REPRESENTATION_ITEM('')
SURFACE()
);
#3058=(
BOUNDED_SURFACE()
B_SPLINE_SURFACE(3,2,((#210447,#210448,#210449),(#210450,#210451,#210452),
(#210453,#210454,#210455),(#210456,#210457,#210458),(#210459,#210460,#210461),
(#210462,#210463,#210464),(#210465,#210466,#210467),(#210468,#210469,#210470)),
 .UNSPECIFIED.,.F.,.F.,.F.)
B_SPLINE_SURFACE_WITH_KNOTS((4,2,2,4),(3,3),(-0.000314471227869891,0.00157235613934946,
0.00235853420902418,0.00345918350656882),(-0.0010818761735745,1.00850572874588),
 .UNSPECIFIED.)
GEOMETRIC_REPRESENTATION_ITEM()
RATIONAL_B_SPLINE_SURFACE(((1.00036290706551,0.830850702039335,1.00287434018484),
(1.0002504422033,0.883270052049706,1.00198358245771),(1.00016420299662,
0.923465745801804,1.00130054032154),(1.0000816177724,0.961958335301367,
1.00064643889664),(1.00006218504651,0.971015838596884,1.00049252548399),
(1.00002887364119,0.986542129924704,1.00022868848542),(1.00001986509788,
0.990740970126149,1.00015733793731),(1.00002547576192,0.988125865671606,
1.00020177619341)))
REPRESENTATION_ITEM('')
SURFACE()
);
#3059=(
BOUNDED_SURFACE()
B_SPLINE_SURFACE(3,2,((#210542,#210543,#210544),(#210545,#210546,#210547),
(#210548,#210549,#210550),(#210551,#210552,#210553)),.UNSPECIFIED.,.F.,
 .F.,.F.)
B_SPLINE_SURFACE_WITH_KNOTS((4,4),(3,3),(0.,0.000753104234298227),(0.,1.),
 .UNSPECIFIED.)
GEOMETRIC_REPRESENTATION_ITEM()
RATIONAL_B_SPLINE_SURFACE(((1.,0.839275484760762,1.),(1.,0.838901603374917,
1.),(1.,0.838526082980222,1.),(1.,0.83814959787298,1.)))
REPRESENTATION_ITEM('')
SURFACE()
);
#3060=(
BOUNDED_SURFACE()
B_SPLINE_SURFACE(3,2,((#210559,#210560,#210561),(#210562,#210563,#210564),
(#210565,#210566,#210567),(#210568,#210569,#210570)),.UNSPECIFIED.,.F.,
 .F.,.F.)
B_SPLINE_SURFACE_WITH_KNOTS((4,4),(3,3),(0.,0.00121469382512386),(0.,1.),
 .UNSPECIFIED.)
GEOMETRIC_REPRESENTATION_ITEM()
RATIONAL_B_SPLINE_SURFACE(((1.,0.857407773863101,1.),(1.,0.851918824817362,
1.),(1.,0.845578741226857,1.),(1.,0.83838293312654,1.)))
REPRESENTATION_ITEM('')
SURFACE()
);
#3061=(
BOUNDED_SURFACE()
B_SPLINE_SURFACE(3,2,((#210627,#210628,#210629),(#210630,#210631,#210632),
(#210633,#210634,#210635),(#210636,#210637,#210638),(#210639,#210640,#210641),
(#210642,#210643,#210644),(#210645,#210646,#210647),(#210648,#210649,#210650),
(#210651,#210652,#210653),(#210654,#210655,#210656),(#210657,#210658,#210659),
(#210660,#210661,#210662),(#210663,#210664,#210665),(#210666,#210667,#210668)),
 .UNSPECIFIED.,.F.,.F.,.F.)
B_SPLINE_SURFACE_WITH_KNOTS((4,2,2,2,2,2,4),(3,3),(-0.000226840284413363,
0.000567100711032879,0.000850651066549369,0.00113420142206586,0.00141775177758235,
0.00170130213309884,0.00249524312854497),(-0.00170901498463875,1.00351063153609),
 .UNSPECIFIED.)
GEOMETRIC_REPRESENTATION_ITEM()
RATIONAL_B_SPLINE_SURFACE(((1.00063854299496,0.812526948435515,1.00131404403671),
(1.00053226337854,0.843730115906702,1.00109533347645),(1.00043744268712,
0.871568999916444,1.00090020399402),(1.0003270802267,0.903970870106644,
1.00067309143599),(1.00029995768986,0.911933912200606,1.00061727654478),
(1.00025172251529,0.926095519859969,1.00051801440582),(1.00023020586516,
0.932412701462029,1.00047373574954),(1.00019632330569,0.942360452621125,
1.00040400955167),(1.00018360585421,0.946094233207541,1.00037783857897),
(1.00017057881538,0.949918907100824,1.00035103051306),(1.000170258171,0.950013046697734,
1.00035037066582),(1.00019261482622,0.943449243773019,1.00039637795071),
(1.00025727649706,0.924464898400181,1.00052944382668),(1.0003327305413,
0.902311965806151,1.00068471909813)))
REPRESENTATION_ITEM('')
SURFACE()
);
#3062=(
BOUNDED_SURFACE()
B_SPLINE_SURFACE(3,2,((#210720,#210721,#210722),(#210723,#210724,#210725),
(#210726,#210727,#210728),(#210729,#210730,#210731)),.UNSPECIFIED.,.F.,
 .F.,.F.)
B_SPLINE_SURFACE_WITH_KNOTS((4,4),(3,3),(0.,0.000758627814399393),(0.,1.),
 .UNSPECIFIED.)
GEOMETRIC_REPRESENTATION_ITEM()
RATIONAL_B_SPLINE_SURFACE(((1.,0.838382933127103,1.),(1.,0.838759998356351,
1.),(1.,0.839135655634363,1.),(1.,0.839509576764081,1.)))
REPRESENTATION_ITEM('')
SURFACE()
);
#3063=(
BOUNDED_SURFACE()
B_SPLINE_SURFACE(3,2,((#210737,#210738,#210739),(#210740,#210741,#210742),
(#210743,#210744,#210745),(#210746,#210747,#210748),(#210749,#210750,#210751),
(#210752,#210753,#210754),(#210755,#210756,#210757),(#210758,#210759,#210760),
(#210761,#210762,#210763),(#210764,#210765,#210766),(#210767,#210768,#210769),
(#210770,#210771,#210772)),.UNSPECIFIED.,.F.,.F.,.F.)
B_SPLINE_SURFACE_WITH_KNOTS((4,2,2,2,2,4),(3,3),(-0.000216256680534387,
0.000582607613633213,0.000867916290121638,0.00115322496661006,0.00172384231958692,
0.00252270661375453),(-0.00157135189843493,1.00088857311935),
 .UNSPECIFIED.)
GEOMETRIC_REPRESENTATION_ITEM()
RATIONAL_B_SPLINE_SURFACE(((1.00031029998659,0.901175496173816,1.00017534981439),
(1.00024041434093,0.923432713562446,1.00013585759549),(1.00018125294539,
0.942274466099237,1.00010242562586),(1.00015904169639,0.949348316427786,
1.00008987409973),(1.00015882754949,0.949416518046249,1.00008975308581),
(1.0001698811118,0.945896173676258,1.00009599942865),(1.00018106406685,
0.942334620236191,1.00010231889103),(1.00022728017823,0.927615688644421,
1.00012843551011),(1.00027359929972,0.912863950337352,1.00015461033998),
(1.00040076355192,0.872364612049113,1.00022647056873),(1.00048842071942,
0.844447510986039,1.00027600543408),(1.00058680386245,0.813114395566315,
1.00033160152371)))
REPRESENTATION_ITEM('')
SURFACE()
);
#3064=(
BOUNDED_SURFACE()
B_SPLINE_SURFACE(2,2,((#210835,#210836,#210837),(#210838,#210839,#210840),
(#210841,#210842,#210843)),.UNSPECIFIED.,.F.,.F.,.F.)
B_SPLINE_SURFACE_WITH_KNOTS((3,3),(3,3),(1.74317346290508E-16,1.57079632679495),
(-0.787072384273275,0.736541846753928),.UNSPECIFIED.)
GEOMETRIC_REPRESENTATION_ITEM()
RATIONAL_B_SPLINE_SURFACE(((1.,0.723589867251388,1.),(0.707106781186616,
0.51165530193138,0.707106781186616),(1.,0.723589867251388,1.)))
REPRESENTATION_ITEM('')
SURFACE()
);
#3065=(
BOUNDED_SURFACE()
B_SPLINE_SURFACE(2,2,((#210856,#210857,#210858),(#210859,#210860,#210861),
(#210862,#210863,#210864)),.UNSPECIFIED.,.F.,.F.,.F.)
B_SPLINE_SURFACE_WITH_KNOTS((3,3),(3,3),(-1.74317346290519E-16,1.57079632679496),
(0.830906038289448,2.35452026931659),.UNSPECIFIED.)
GEOMETRIC_REPRESENTATION_ITEM()
RATIONAL_B_SPLINE_SURFACE(((1.,0.72358986725141,1.),(0.707106781186587,
0.511655301931375,0.707106781186587),(1.,0.72358986725141,1.)))
REPRESENTATION_ITEM('')
SURFACE()
);
#3066=(
BOUNDED_SURFACE()
B_SPLINE_SURFACE(2,2,((#210879,#210880,#210881),(#210882,#210883,#210884),
(#210885,#210886,#210887)),.UNSPECIFIED.,.F.,.F.,.F.)
B_SPLINE_SURFACE_WITH_KNOTS((3,3),(3,3),(1.81714697791953E-16,1.57079632679495),
(-0.26549733202973,0.74383310368946),.UNSPECIFIED.)
GEOMETRIC_REPRESENTATION_ITEM()
RATIONAL_B_SPLINE_SURFACE(((1.,0.875336395469216,1.),(0.707106781186606,
0.618956301055724,0.707106781186606),(1.,0.875336395469216,1.)))
REPRESENTATION_ITEM('')
SURFACE()
);
#3067=(
BOUNDED_SURFACE()
B_SPLINE_SURFACE(2,2,((#210899,#210900,#210901),(#210902,#210903,#210904),
(#210905,#210906,#210907)),.UNSPECIFIED.,.F.,.F.,.F.)
B_SPLINE_SURFACE_WITH_KNOTS((3,3),(3,3),(-6.30291942997115E-17,1.57079632679495),
(0.819567334644225,1.82889777036346),.UNSPECIFIED.)
GEOMETRIC_REPRESENTATION_ITEM()
RATIONAL_B_SPLINE_SURFACE(((1.,0.875336395469206,1.),(0.707106781186601,
0.618956301055712,0.707106781186601),(1.,0.875336395469206,1.)))
REPRESENTATION_ITEM('')
SURFACE()
);
#3068=(
BOUNDED_SURFACE()
B_SPLINE_SURFACE(2,2,((#210922,#210923,#210924),(#210925,#210926,#210927),
(#210928,#210929,#210930)),.UNSPECIFIED.,.F.,.F.,.F.)
B_SPLINE_SURFACE_WITH_KNOTS((3,3),(3,3),(-1.57079632679491,1.68131336473773E-16),
(0.821845324909055,1.83117576062825),.UNSPECIFIED.)
GEOMETRIC_REPRESENTATION_ITEM()
RATIONAL_B_SPLINE_SURFACE(((1.,0.875336395469216,1.),(0.70710678118653,
0.618956301055656,0.70710678118653),(1.,0.875336395469216,1.)))
REPRESENTATION_ITEM('')
SURFACE()
);
#3069=(
BOUNDED_SURFACE()
B_SPLINE_SURFACE(2,2,((#210942,#210943,#210944),(#210945,#210946,#210947),
(#210948,#210949,#210950)),.UNSPECIFIED.,.F.,.F.,.F.)
B_SPLINE_SURFACE_WITH_KNOTS((3,3),(3,3),(-1.5707963267949,2.47147205475768E-16),
(-0.263219341764958,0.746111093954295),.UNSPECIFIED.)
GEOMETRIC_REPRESENTATION_ITEM()
RATIONAL_B_SPLINE_SURFACE(((1.,0.875336395469201,1.),(0.707106781186519,
0.618956301055637,0.707106781186519),(1.,0.875336395469201,1.)))
REPRESENTATION_ITEM('')
SURFACE()
);
#3070=(
BOUNDED_SURFACE()
B_SPLINE_SURFACE(2,2,((#210965,#210966,#210967),(#210968,#210969,#210970),
(#210971,#210972,#210973)),.UNSPECIFIED.,.F.,.F.,.F.)
B_SPLINE_SURFACE_WITH_KNOTS((3,3),(3,3),(-1.57079632679491,1.67905497988288E-16),
(0.823093317098874,2.34670754812599),.UNSPECIFIED.)
GEOMETRIC_REPRESENTATION_ITEM()
RATIONAL_B_SPLINE_SURFACE(((1.,0.723589867251417,1.),(0.70710678118653,
0.511655301931338,0.70710678118653),(1.,0.723589867251417,1.)))
REPRESENTATION_ITEM('')
SURFACE()
);
#3071=(
BOUNDED_SURFACE()
B_SPLINE_SURFACE(2,2,((#210985,#210986,#210987),(#210988,#210989,#210990),
(#210991,#210992,#210993)),.UNSPECIFIED.,.F.,.F.,.F.)
B_SPLINE_SURFACE_WITH_KNOTS((3,3),(3,3),(-1.57079632679491,2.478375474118E-16),
(-0.794885105463935,0.728729125563299),.UNSPECIFIED.)
GEOMETRIC_REPRESENTATION_ITEM()
RATIONAL_B_SPLINE_SURFACE(((1.,0.723589867251377,1.),(0.70710678118653,
0.511655301931309,0.70710678118653),(1.,0.723589867251377,1.)))
REPRESENTATION_ITEM('')
SURFACE()
);
#3072=(
BOUNDED_SURFACE()
B_SPLINE_SURFACE(3,2,((#212943,#212944,#212945),(#212946,#212947,#212948),
(#212949,#212950,#212951),(#212952,#212953,#212954),(#212955,#212956,#212957),
(#212958,#212959,#212960),(#212961,#212962,#212963),(#212964,#212965,#212966),
(#212967,#212968,#212969),(#212970,#212971,#212972),(#212973,#212974,#212975),
(#212976,#212977,#212978),(#212979,#212980,#212981),(#212982,#212983,#212984),
(#212985,#212986,#212987),(#212988,#212989,#212990),(#212991,#212992,#212993),
(#212994,#212995,#212996),(#212997,#212998,#212999),(#213000,#213001,#213002),
(#213003,#213004,#213005),(#213006,#213007,#213008),(#213009,#213010,#213011),
(#213012,#213013,#213014),(#213015,#213016,#213017),(#213018,#213019,#213020),
(#213021,#213022,#213023),(#213024,#213025,#213026),(#213027,#213028,#213029),
(#213030,#213031,#213032),(#213033,#213034,#213035),(#213036,#213037,#213038),
(#213039,#213040,#213041),(#213042,#213043,#213044),(#213045,#213046,#213047),
(#213048,#213049,#213050),(#213051,#213052,#213053),(#213054,#213055,#213056),
(#213057,#213058,#213059),(#213060,#213061,#213062),(#213063,#213064,#213065),
(#213066,#213067,#213068),(#213069,#213070,#213071),(#213072,#213073,#213074),
(#213075,#213076,#213077),(#213078,#213079,#213080),(#213081,#213082,#213083),
(#213084,#213085,#213086)),.UNSPECIFIED.,.F.,.F.,.F.)
B_SPLINE_SURFACE_WITH_KNOTS((4,2,2,2,2,2,2,2,2,2,2,2,2,2,2,2,2,2,2,2,2,
2,2,4),(3,3),(0.,0.0059149619408077,0.00739370242600962,0.00743991306617218,
0.00748612370633474,0.00757854498665986,0.0077633875473101,0.00813307266861059,
0.00887244291121155,0.0118299238816154,0.0133086643668173,0.0140480346094183,
0.0140942452495808,0.0141404558897434,0.0142328771700685,0.0144177197307188,
0.0147874048520192,0.0177448858224231,0.019223626307625,0.019962996550226,
0.0201478391108762,0.0203326816715265,0.0207023667928269,0.0236598477632308),
(0.,1.),.UNSPECIFIED.)
GEOMETRIC_REPRESENTATION_ITEM()
RATIONAL_B_SPLINE_SURFACE(((1.,0.861068946771262,1.),(1.,0.871793299675347,
1.),(1.,0.879015041937488,1.),(1.,0.885129578373153,1.),(1.,0.886202028929654,
1.),(1.,0.887164714171582,1.),(1.,0.887116116747139,1.),(1.,0.887073026774255,
1.),(1.,0.887051430276885,1.),(1.,0.886986487326662,1.),(1.,0.886942987422201,
1.),(1.,0.886811882202044,1.),(1.,0.886723671509742,1.),(1.,0.886456679535479,
1.),(1.,0.886275540586052,1.),(1.,0.88572310670639,1.),(1.,0.885342833942064,
1.),(1.,0.883384862710688,1.),(1.,0.881615095800445,1.),(1.,0.878612600044596,
1.),(1.,0.877556288775192,1.),(1.,0.875871070793252,1.),(1.,0.875293879519929,
1.),(1.,0.874664965796897,1.),(1.,0.874763981664806,1.),(1.,0.874835206629783,
1.),(1.,0.874870651351952,1.),(1.,0.87497648659221,1.),(1.,0.875046378225363,
1.),(1.,0.875254090776843,1.),(1.,0.875389950005275,1.),(1.,0.875789921459867,
1.),(1.,0.876046437149636,1.),(1.,0.878268573346079,1.),(1.,0.879634170738163,
1.),(1.,0.880866820420691,1.),(1.,0.881143316614213,1.),(1.,0.881356253213235,
1.),(1.,0.881394010610288,1.),(1.,0.88139952742701,1.),(1.,0.881398536837081,
1.),(1.,0.881392323021745,1.),(1.,0.881371643237072,1.),(1.,0.881442771835474,
1.),(1.,0.881487673169753,1.),(1.,0.881868765786043,1.),(1.,0.882040414813943,
1.),(1.,0.88203965410677,1.)))
REPRESENTATION_ITEM('')
SURFACE()
);
#3073=(
BOUNDED_SURFACE()
B_SPLINE_SURFACE(3,2,((#213396,#213397,#213398),(#213399,#213400,#213401),
(#213402,#213403,#213404),(#213405,#213406,#213407)),.UNSPECIFIED.,.F.,
 .F.,.F.)
B_SPLINE_SURFACE_WITH_KNOTS((4,4),(3,3),(-8.16115679863473E-6,0.000330556732041574),
(-8.16118966828803E-6,1.),.UNSPECIFIED.)
GEOMETRIC_REPRESENTATION_ITEM()
RATIONAL_B_SPLINE_SURFACE(((1.0000022763522,0.860537967104879,1.),(1.00000215632319,
0.867891613986121,1.),(1.00000205218217,0.874271873585881,1.),(1.00000196504864,
0.8796101599594,1.)))
REPRESENTATION_ITEM('')
SURFACE()
);
#3074=(
BOUNDED_SURFACE()
B_SPLINE_SURFACE(3,2,((#213416,#213417,#213418),(#213419,#213420,#213421),
(#213422,#213423,#213424),(#213425,#213426,#213427)),.UNSPECIFIED.,.F.,
 .F.,.F.)
B_SPLINE_SURFACE_WITH_KNOTS((4,4),(3,3),(-1.56125112837912E-17,0.00371972595076131),
(0.,1.),.UNSPECIFIED.)
GEOMETRIC_REPRESENTATION_ITEM()
RATIONAL_B_SPLINE_SURFACE(((1.,0.879223463974645,1.),(1.,0.879197541860131,
1.),(1.,0.879166735457461,1.),(1.,0.879131676488835,1.)))
REPRESENTATION_ITEM('')
SURFACE()
);
#3075=(
BOUNDED_SURFACE()
B_SPLINE_SURFACE(3,2,((#213433,#213434,#213435),(#213436,#213437,#213438),
(#213439,#213440,#213441),(#213442,#213443,#213444),(#213445,#213446,#213447),
(#213448,#213449,#213450),(#213451,#213452,#213453),(#213454,#213455,#213456),
(#213457,#213458,#213459),(#213460,#213461,#213462),(#213463,#213464,#213465),
(#213466,#213467,#213468),(#213469,#213470,#213471),(#213472,#213473,#213474),
(#213475,#213476,#213477),(#213478,#213479,#213480),(#213481,#213482,#213483),
(#213484,#213485,#213486),(#213487,#213488,#213489),(#213490,#213491,#213492),
(#213493,#213494,#213495),(#213496,#213497,#213498),(#213499,#213500,#213501),
(#213502,#213503,#213504),(#213505,#213506,#213507),(#213508,#213509,#213510)),
 .UNSPECIFIED.,.F.,.F.,.F.)
B_SPLINE_SURFACE_WITH_KNOTS((4,2,2,2,2,2,2,2,2,2,2,2,4),(3,3),(-2.020502013395E-5,
0.000191440896835587,0.00028716134525338,0.000382881793671173,0.00057432269050676,
0.000670043138924553,0.000765763587342347,0.000957204484177933,0.00114864538101352,
0.00124436582943131,0.00129222605364021,0.00134008627784911,0.00155173219481786),
(-0.000614322987741022,1.),.UNSPECIFIED.)
GEOMETRIC_REPRESENTATION_ITEM()
RATIONAL_B_SPLINE_SURFACE(((1.00014914760104,0.878608155632912,1.),(1.00014732673166,
0.880090168686671,1.),(1.00014437340606,0.882493892513453,1.),(1.00013921574776,
0.886691731762652,1.),(1.00013754315828,0.888053059200701,1.),(1.00013487983185,
0.890220751507748,1.),(1.00013397197062,0.890959663488422,1.),(1.00013196690704,
0.892591592961943,1.),(1.00013020252052,0.894027634387128,1.),(1.00012653566681,
0.897012101670959,1.),(1.0001253668636,0.897963395397947,1.),(1.00012347828042,
0.899500520996579,1.),(1.00012275982084,0.900085278191057,1.),(1.00012070489333,
0.901757792124973,1.),(1.00011967187973,0.902598566132467,1.),(1.00011648933932,
0.905188848827967,1.),(1.00011476936931,0.906588739477223,1.),(1.00011330257804,
0.90778256690637,1.),(1.00011290516169,0.908106025705496,1.),(1.00011238177525,
0.908532012070824,1.),(1.00011225358233,0.908636348819827,1.),(1.00011164539059,
0.909131358574023,1.),(1.00011119272546,0.909499784574332,1.),(1.00010848940599,
0.911700027382186,1.),(1.0001066078168,0.913231460541444,1.),(1.00010622151568,
0.913545872609453,1.)))
REPRESENTATION_ITEM('')
SURFACE()
);
#3076=(
BOUNDED_SURFACE()
B_SPLINE_SURFACE(3,2,((#213626,#213627,#213628),(#213629,#213630,#213631),
(#213632,#213633,#213634),(#213635,#213636,#213637),(#213638,#213639,#213640),
(#213641,#213642,#213643),(#213644,#213645,#213646),(#213647,#213648,#213649),
(#213650,#213651,#213652),(#213653,#213654,#213655),(#213656,#213657,#213658),
(#213659,#213660,#213661)),.UNSPECIFIED.,.F.,.F.,.F.)
B_SPLINE_SURFACE_WITH_KNOTS((4,2,2,2,2,4),(3,3),(0.,0.00646885457540742,
0.0129377091508148,0.0161721364385186,0.0194065637262222,0.0258754183016297),
(0.,1.),.UNSPECIFIED.)
GEOMETRIC_REPRESENTATION_ITEM()
RATIONAL_B_SPLINE_SURFACE(((1.,0.913476533865333,1.),(1.,0.914845943871889,
1.),(1.,0.916112934302359,1.),(1.,0.918040216804478,1.),(1.,0.918611066895268,
1.),(1.,0.919010773408858,1.),(1.,0.919049811602052,1.),(1.,0.918970993255618,
1.),(1.,0.918853664923092,1.),(1.,0.918278797297209,1.),(1.,0.917618952389758,
1.),(1.,0.917028647019402,1.)))
REPRESENTATION_ITEM('')
SURFACE()
);
#3077=(
BOUNDED_SURFACE()
B_SPLINE_SURFACE(3,2,((#213793,#213794,#213795),(#213796,#213797,#213798),
(#213799,#213800,#213801),(#213802,#213803,#213804),(#213805,#213806,#213807),
(#213808,#213809,#213810),(#213811,#213812,#213813),(#213814,#213815,#213816),
(#213817,#213818,#213819),(#213820,#213821,#213822),(#213823,#213824,#213825),
(#213826,#213827,#213828),(#213829,#213830,#213831),(#213832,#213833,#213834),
(#213835,#213836,#213837),(#213838,#213839,#213840),(#213841,#213842,#213843),
(#213844,#213845,#213846),(#213847,#213848,#213849),(#213850,#213851,#213852),
(#213853,#213854,#213855),(#213856,#213857,#213858),(#213859,#213860,#213861),
(#213862,#213863,#213864),(#213865,#213866,#213867),(#213868,#213869,#213870),
(#213871,#213872,#213873),(#213874,#213875,#213876),(#213877,#213878,#213879),
(#213880,#213881,#213882),(#213883,#213884,#213885),(#213886,#213887,#213888),
(#213889,#213890,#213891),(#213892,#213893,#213894)),.UNSPECIFIED.,.F.,
 .F.,.F.)
B_SPLINE_SURFACE_WITH_KNOTS((4,2,2,2,2,2,2,2,2,2,2,2,2,2,2,2,4),(3,3),(0.,
0.000127304511784401,0.000254609023568802,0.000318261279461002,0.000381913535353202,
0.000509218047137603,0.000636522558922004,0.000763827070706405,0.000891131582490806,
0.00101843609427521,0.00114574060605961,0.00127304511784401,0.00140034962962841,
0.00152765414141281,0.00165495865319721,0.00178226316498161,0.00203687218855042),
(-0.000961805720933131,1.),.UNSPECIFIED.)
GEOMETRIC_REPRESENTATION_ITEM()
RATIONAL_B_SPLINE_SURFACE(((1.0001597581526,0.916948844697399,1.),(1.00016029912196,
0.916667618796779,1.),(1.00016097503671,0.916316240794633,1.),(1.00016291083017,
0.91530990790145,1.),(1.00016430151804,0.914586951156848,1.),(1.0001663252959,
0.913534879090444,1.),(1.00016693387069,0.913218508139461,1.),(1.00016773229267,
0.912803444074217,1.),(1.00016788468109,0.912724224114995,1.),(1.00016858323375,
0.912361077667592,1.),(1.00016914120577,0.91207101284379,1.),(1.00017061498675,
0.911304859685145,1.),(1.00017156421239,0.910811399509231,1.),(1.00017411696132,
0.909484338922955,1.),(1.00017540359175,0.908815477007135,1.),(1.00017753666339,
0.907706587971933,1.),(1.00017822836713,0.907347001970364,1.),(1.00017982387443,
0.906517568718808,1.),(1.00018080359298,0.906008256636064,1.),(1.00018333217183,
0.90469376099426,1.),(1.00018503490327,0.903808586681878,1.),(1.00018813760279,
0.902195631252981,1.),(1.00018958895774,0.901441136386703,1.),(1.00019214250402,
0.900113661296256,1.),(1.00019340707361,0.899456267831493,1.),(1.00019657037923,
0.897811805984888,1.),(1.00019839101625,0.896865337805144,1.),(1.00020221928284,
0.894875192336821,1.),(1.00020407941471,0.893908192541967,1.),(1.00020755406108,
0.892101878494427,1.),(1.00020897072777,0.891365416518063,1.),(1.00021429441008,
0.888597870954491,1.),(1.00021994630903,0.885659700163249,1.),(1.00022335245868,
0.883888994514506,1.)))
REPRESENTATION_ITEM('')
SURFACE()
);
#3078=(
BOUNDED_SURFACE()
B_SPLINE_SURFACE(3,2,((#214040,#214041,#214042),(#214043,#214044,#214045),
(#214046,#214047,#214048),(#214049,#214050,#214051)),.UNSPECIFIED.,.F.,
 .F.,.F.)
B_SPLINE_SURFACE_WITH_KNOTS((4,4),(3,3),(0.,0.00767500517967513),(0.,1.),
 .UNSPECIFIED.)
GEOMETRIC_REPRESENTATION_ITEM()
RATIONAL_B_SPLINE_SURFACE(((1.,0.884000563436129,1.),(1.,0.883607612825216,
1.),(1.,0.883267077927119,1.),(1.,0.882986276630499,1.)))
REPRESENTATION_ITEM('')
SURFACE()
);
#3079=(
BOUNDED_SURFACE()
B_SPLINE_SURFACE(3,2,((#214057,#214058,#214059),(#214060,#214061,#214062),
(#214063,#214064,#214065),(#214066,#214067,#214068)),.UNSPECIFIED.,.F.,
 .F.,.F.)
B_SPLINE_SURFACE_WITH_KNOTS((4,4),(3,3),(-4.63829152513897E-5,0.000510218477218229),
(-8.53868048819074E-5,1.),.UNSPECIFIED.)
GEOMETRIC_REPRESENTATION_ITEM()
RATIONAL_B_SPLINE_SURFACE(((1.00001949037752,0.885870085279226,1.),(1.0000214351582,
0.874482021962947,1.),(1.00002376476953,0.860840503630916,1.),(1.00002644118215,
0.845168218973911,1.)))
REPRESENTATION_ITEM('')
SURFACE()
);
#3080=(
BOUNDED_SURFACE()
B_SPLINE_SURFACE(3,2,((#214089,#214090,#214091),(#214092,#214093,#214094),
(#214095,#214096,#214097),(#214098,#214099,#214100),(#214101,#214102,#214103),
(#214104,#214105,#214106),(#214107,#214108,#214109),(#214110,#214111,#214112),
(#214113,#214114,#214115),(#214116,#214117,#214118),(#214119,#214120,#214121),
(#214122,#214123,#214124),(#214125,#214126,#214127),(#214128,#214129,#214130),
(#214131,#214132,#214133),(#214134,#214135,#214136),(#214137,#214138,#214139),
(#214140,#214141,#214142),(#214143,#214144,#214145),(#214146,#214147,#214148),
(#214149,#214150,#214151),(#214152,#214153,#214154),(#214155,#214156,#214157),
(#214158,#214159,#214160),(#214161,#214162,#214163),(#214164,#214165,#214166),
(#214167,#214168,#214169),(#214170,#214171,#214172),(#214173,#214174,#214175),
(#214176,#214177,#214178),(#214179,#214180,#214181),(#214182,#214183,#214184),
(#214185,#214186,#214187),(#214188,#214189,#214190),(#214191,#214192,#214193),
(#214194,#214195,#214196),(#214197,#214198,#214199),(#214200,#214201,#214202),
(#214203,#214204,#214205),(#214206,#214207,#214208),(#214209,#214210,#214211),
(#214212,#214213,#214214),(#214215,#214216,#214217),(#214218,#214219,#214220),
(#214221,#214222,#214223),(#214224,#214225,#214226),(#214227,#214228,#214229),
(#214230,#214231,#214232),(#214233,#214234,#214235),(#214236,#214237,#214238),
(#214239,#214240,#214241),(#214242,#214243,#214244),(#214245,#214246,#214247),
(#214248,#214249,#214250),(#214251,#214252,#214253),(#214254,#214255,#214256),
(#214257,#214258,#214259),(#214260,#214261,#214262),(#214263,#214264,#214265),
(#214266,#214267,#214268),(#214269,#214270,#214271),(#214272,#214273,#214274),
(#214275,#214276,#214277),(#214278,#214279,#214280),(#214281,#214282,#214283),
(#214284,#214285,#214286),(#214287,#214288,#214289),(#214290,#214291,#214292),
(#214293,#214294,#214295),(#214296,#214297,#214298),(#214299,#214300,#214301),
(#214302,#214303,#214304),(#214305,#214306,#214307),(#214308,#214309,#214310),
(#214311,#214312,#214313),(#214314,#214315,#214316),(#214317,#214318,#214319),
(#214320,#214321,#214322),(#214323,#214324,#214325),(#214326,#214327,#214328),
(#214329,#214330,#214331),(#214332,#214333,#214334),(#214335,#214336,#214337),
(#214338,#214339,#214340),(#214341,#214342,#214343),(#214344,#214345,#214346),
(#214347,#214348,#214349),(#214350,#214351,#214352),(#214353,#214354,#214355),
(#214356,#214357,#214358),(#214359,#214360,#214361),(#214362,#214363,#214364),
(#214365,#214366,#214367),(#214368,#214369,#214370),(#214371,#214372,#214373),
(#214374,#214375,#214376),(#214377,#214378,#214379),(#214380,#214381,#214382),
(#214383,#214384,#214385),(#214386,#214387,#214388),(#214389,#214390,#214391),
(#214392,#214393,#214394),(#214395,#214396,#214397),(#214398,#214399,#214400)),
 .UNSPECIFIED.,.F.,.F.,.F.)
B_SPLINE_SURFACE_WITH_KNOTS((4,2,2,2,2,2,2,2,2,2,2,2,2,2,2,2,2,2,2,2,2,
2,2,2,2,2,2,2,2,2,2,2,2,2,2,2,2,2,2,2,2,2,2,2,2,2,2,2,2,2,2,4),(3,3),(-1.90819582357449E-17,
0.00250327328955147,0.00500654657910296,0.0062581832238787,0.00688400154626657,
0.00696222883656506,0.00704045612686354,0.00719691070746051,0.00750981986865445,
0.0100130931582059,0.0112647298029817,0.0115776389641756,0.0117340935447726,
0.0117732071899218,0.0118123208350711,0.0118905481253695,0.0125163664477574,
0.0137680030925332,0.0150196397373089,0.0175229130268604,0.0175620266720097,
0.0176011403171589,0.0176793676074573,0.0178358221880543,0.0181487313492483,
0.0187745496716362,0.0200261863164119,0.0225294596059634,0.0226076868962618,
0.0226468005414111,0.0226859141865603,0.0228423687671573,0.0231552779283512,
0.0237810962507391,0.0250327328955148,0.0275360061850663,0.0281618245074543,
0.0283182790880512,0.0283965063783497,0.0284356200234989,0.0284747336686481,
0.0287876428298421,0.0300392794746179,0.0325425527641693,0.0331683710865572,
0.0332465983768557,0.0333248256671542,0.0334812802477511,0.0337941894089451,
0.0350458260537208,0.0375490993432723,0.0400523726328238),(-0.0381612915992707,
1.),.UNSPECIFIED.)
GEOMETRIC_REPRESENTATION_ITEM()
RATIONAL_B_SPLINE_SURFACE(((1.01196001158971,0.843296556687619,1.),(1.01125783435868,
0.85249668070863,1.),(1.01069166159088,0.859914835913468,1.),(1.00976927957171,
0.872000145143153,1.),(1.00941130926471,0.876690373015487,1.),(1.00899858840752,
0.882097958030137,1.),(1.00888239831572,0.883620313366265,1.),(1.00873889255595,
0.885500566284285,1.),(1.00869608841852,0.886061398159222,1.),(1.00865339690349,
0.886620754423689,1.),(1.00864670343397,0.88670845414809,1.),(1.00866056676143,
0.886526812923762,1.),(1.00866751249057,0.886435808022655,1.),(1.00868839096718,
0.886162252336477,1.),(1.00870236499396,0.885979160698443,1.),(1.00874444530519,
0.885427812598559,1.),(1.00877270964358,0.885057485269314,1.),(1.00902883862555,
0.881701611146218,1.),(1.00926835954748,0.878563340507299,1.),(1.00964800740727,
0.873589087227618,1.),(1.00977665564098,0.871903501804282,1.),(1.00994048509359,
0.869756962133522,1.),(1.00997338891691,0.869325846965062,1.),(1.01002293363291,
0.868676698129656,1.),(1.01003948008887,0.86845990179927,1.),(1.01006020114881,
0.868188408630767,1.),(1.01006434726144,0.868134085094295,1.),(1.01007264325631,
0.868025388630908,1.),(1.01008257425108,0.867895269937968,1.),(1.0100700071273,
0.868059927936344,1.),(1.01006172312451,0.868168467276088,1.),(1.00998800489105,
0.86913434435171,1.),(1.00992842205968,0.869915015404356,1.),(1.00976625976859,
0.87203971145494,1.),(1.00968006454818,0.873169065530701,1.),(1.0095492237058,
0.87488337913093,1.),(1.00950425621008,0.875472555935985,1.),(1.00943051365994,
0.876438751615483,1.),(1.00946109460324,0.876038071475825,1.),(1.00957595913498,
0.874533084001203,1.),(1.00957354603934,0.874564701060542,1.),(1.00957152686768,
0.874591156816875,1.),(1.00957051742751,0.874604382786464,1.),(1.00956748950558,
0.874644055473136,1.),(1.00956547142283,0.874670496962195,1.),(1.00955941844798,
0.874749804745048,1.),(1.00955538483576,0.874802654269464,1.),(1.0095432862966,
0.874961172740026,1.),(1.00953522376587,0.875066810290442,1.),(1.00951101947695,
0.875383941706837,1.),(1.00949494750357,0.875594521232732,1.),(1.00944675569682,
0.876225943869802,1.),(1.00941476784221,0.876645057758139,1.),(1.00932050409865,
0.877880127898698,1.),(1.00925991366249,0.878674000873372,1.),(1.00919906635626,
0.879471239432123,1.),(1.00919722372212,0.879495382144067,1.),(1.00919446140767,
0.879531574766626,1.),(1.00919317113587,0.879548480271513,1.),(1.00919296179469,
0.879551223118678,1.),(1.0091928763248,0.879552342969231,1.),(1.00919254483007,
0.879556686306683,1.),(1.00919258632655,0.879556142608002,1.),(1.00919362623178,
0.879542517476642,1.),(1.00919553951585,0.879517449089296,1.),(1.00920492183756,
0.879394519265546,1.),(1.00921602488281,0.879249044036668,1.),(1.00926404627612,
0.878619854204664,1.),(1.00931567792812,0.877943361745405,1.),(1.00952975614758,
0.875138448566535,1.),(1.00975123045612,0.872236629743661,1.),(1.01014599617449,
0.867064298019097,1.),(1.01023084555145,0.865952577563629,1.),(1.01034490480467,
0.864458141075202,1.),(1.01036811785504,0.86415399714571,1.),(1.01040355400373,
0.863689702736319,1.),(1.0104154688255,0.863533591382718,1.),(1.01043349715749,
0.863297379094865,1.),(1.01043953261861,0.863218300781946,1.),(1.0104516559068,
0.863059458042581,1.),(1.01044285803288,0.863174730266686,1.),(1.01038421780063,
0.863943051120049,1.),(1.01033243868938,0.864621475631935,1.),(1.01007536067835,
0.867989784201389,1.),(1.00987606553213,0.870601005387309,1.),(1.00929507722922,
0.878213277909576,1.),(1.00893022734244,0.882993643975501,1.),(1.00850337039391,
0.888586444043777,1.),(1.00841946355952,0.889685815040908,1.),(1.00832690759306,
0.890898509404476,1.),(1.00831664918989,0.891032917894642,1.),(1.00829618431438,
0.891301054462431,1.),(1.008305490177,0.891179126427196,1.),(1.00832789429041,
0.890885581417706,1.),(1.00834315168937,0.89068567467553,1.),(1.00838989813797,
0.890073189528329,1.),(1.00842236102569,0.889647851622424,1.),(1.00859133045236,
0.887433966562537,1.),(1.00874767204339,0.88538553496503,1.),(1.0092895506672,
0.878285688483144,1.),(1.00974403336268,0.872330928090653,1.),(1.01090323982987,
0.857142678183397,1.),(1.01160967330184,0.847886787693706,1.),(1.01248680792497,
0.836394322601919,1.)))
REPRESENTATION_ITEM('')
SURFACE()
);
#3081=(
BOUNDED_SURFACE()
B_SPLINE_SURFACE(3,2,((#214913,#214914,#214915),(#214916,#214917,#214918),
(#214919,#214920,#214921),(#214922,#214923,#214924)),.UNSPECIFIED.,.F.,
 .F.,.F.)
B_SPLINE_SURFACE_WITH_KNOTS((4,4),(3,3),(-5.17487663021493E-5,0.000569235683520745),
(-0.000120686675199996,1.00000829533119),.UNSPECIFIED.)
GEOMETRIC_REPRESENTATION_ITEM()
RATIONAL_B_SPLINE_SURFACE(((1.0000391614481,0.837754362995105,1.00000269143776),
(1.00003464486359,0.856466544625889,1.00000238102774),(1.00003064258142,
0.873047974894796,1.00000210596402),(1.00002720545249,0.887287978772295,
1.00000186974144)))
REPRESENTATION_ITEM('')
SURFACE()
);
#3082=(
BOUNDED_SURFACE()
B_SPLINE_SURFACE(3,2,((#214948,#214949,#214950),(#214951,#214952,#214953),
(#214954,#214955,#214956),(#214957,#214958,#214959)),.UNSPECIFIED.,.F.,
 .F.,.F.)
B_SPLINE_SURFACE_WITH_KNOTS((4,4),(3,3),(1.7347234759768E-18,0.00761738954978064),
(0.,1.),.UNSPECIFIED.)
GEOMETRIC_REPRESENTATION_ITEM()
RATIONAL_B_SPLINE_SURFACE(((1.,0.883694369886725,1.),(1.,0.884057799195121,
1.),(1.,0.884477978068247,1.),(1.,0.884949126929568,1.)))
REPRESENTATION_ITEM('')
SURFACE()
);
#3083=(
BOUNDED_SURFACE()
B_SPLINE_SURFACE(3,2,((#214965,#214966,#214967),(#214968,#214969,#214970),
(#214971,#214972,#214973),(#214974,#214975,#214976),(#214977,#214978,#214979),
(#214980,#214981,#214982),(#214983,#214984,#214985),(#214986,#214987,#214988),
(#214989,#214990,#214991),(#214992,#214993,#214994),(#214995,#214996,#214997),
(#214998,#214999,#215000),(#215001,#215002,#215003),(#215004,#215005,#215006),
(#215007,#215008,#215009),(#215010,#215011,#215012),(#215013,#215014,#215015),
(#215016,#215017,#215018),(#215019,#215020,#215021),(#215022,#215023,#215024),
(#215025,#215026,#215027),(#215028,#215029,#215030),(#215031,#215032,#215033),
(#215034,#215035,#215036),(#215037,#215038,#215039),(#215040,#215041,#215042),
(#215043,#215044,#215045),(#215046,#215047,#215048),(#215049,#215050,#215051),
(#215052,#215053,#215054),(#215055,#215056,#215057),(#215058,#215059,#215060)),
 .UNSPECIFIED.,.F.,.F.,.F.)
B_SPLINE_SURFACE_WITH_KNOTS((4,2,2,2,2,2,2,2,2,2,2,2,2,2,2,4),(3,3),(-4.4986094344704E-5,
0.0002498236013634,0.0003747354020451,0.0004996472027268,0.0006245590034085,
0.0007494708040902,0.0008743826047719,0.0009992944054536,0.001249118006817,
0.0013740298074987,0.0014989416081804,0.0016238534088621,0.00168630930920295,
0.0017487652095438,0.0018736770102255,0.00204357490525167),(-0.000928863206409833,
1.),.UNSPECIFIED.)
GEOMETRIC_REPRESENTATION_ITEM()
RATIONAL_B_SPLINE_SURFACE(((1.00021581603045,0.883827872090034,1.),(1.00021247367029,
0.885627039143543,1.),(1.00020356699106,0.890421436842798,1.),(1.00019671059006,
0.894112185357078,1.),(1.00019500428282,0.895030677567382,1.),(1.00019084017243,
0.897272186523882,1.),(1.00018859402754,0.89848126923129,1.),(1.0001839588648,
0.900976342083762,1.),(1.00018187522096,0.902097951719568,1.),(1.0001782873346,
0.904029283662378,1.),(1.00017695153087,0.904748336647395,1.),(1.00017393790794,
0.906370546956913,1.),(1.00017218171469,0.907315892426449,1.),(1.00016839882933,
0.90935219084759,1.),(1.00016641186784,0.910421757106923,1.),(1.00016227044416,
0.912651053978273,1.),(1.00016143269546,0.913102007730518,1.),(1.00015750356649,
0.915217027974831,1.),(1.00015585992972,0.916101785147747,1.),(1.00015287736794,
0.917707275472429,1.),(1.0001519373587,0.918213275298274,1.),(1.00015040070489,
0.91904044435685,1.),(1.00014983626223,0.919344279545902,1.),(1.00014914376439,
0.919717045868286,1.),(1.00014896836908,0.919811459830685,1.),(1.00014795440259,
0.920357270280351,1.),(1.00014718179759,0.920773157676318,1.),(1.00014470824478,
0.922104652342618,1.),(1.00014315205124,0.922942339491473,1.),(1.00014065158056,
0.924288323840175,1.),(1.00013984045591,0.924724946070919,1.),(1.00013914538674,
0.925099096520833,1.)))
REPRESENTATION_ITEM('')
SURFACE()
);
#3084=(
BOUNDED_SURFACE()
B_SPLINE_SURFACE(3,2,((#215354,#215355,#215356),(#215357,#215358,#215359),
(#215360,#215361,#215362),(#215363,#215364,#215365),(#215366,#215367,#215368),
(#215369,#215370,#215371),(#215372,#215373,#215374),(#215375,#215376,#215377),
(#215378,#215379,#215380),(#215381,#215382,#215383),(#215384,#215385,#215386),
(#215387,#215388,#215389)),.UNSPECIFIED.,.F.,.F.,.F.)
B_SPLINE_SURFACE_WITH_KNOTS((4,2,2,2,2,4),(3,3),(0.,0.00715193125010649,
0.014303862500213,0.0178798281252662,0.0214557937503195,0.028607725000426),
(0.,1.),.UNSPECIFIED.)
GEOMETRIC_REPRESENTATION_ITEM()
RATIONAL_B_SPLINE_SURFACE(((1.,0.924853416885499,1.),(1.,0.926016513677579,
1.),(1.,0.927093722943951,1.),(1.,0.928447778269084,1.),(1.,0.928716882101724,
1.),(1.,0.928441394999488,1.),(1.,0.928242899045327,1.),(1.,0.927647417447185,
1.),(1.,0.927250341183873,1.),(1.,0.92570107615163,1.),(1.,0.924268637781389,
1.),(1.,0.922934699314373,1.)))
REPRESENTATION_ITEM('')
SURFACE()
);
#3085=(
BOUNDED_SURFACE()
B_SPLINE_SURFACE(3,2,((#215533,#215534,#215535),(#215536,#215537,#215538),
(#215539,#215540,#215541),(#215542,#215543,#215544),(#215545,#215546,#215547),
(#215548,#215549,#215550),(#215551,#215552,#215553),(#215554,#215555,#215556),
(#215557,#215558,#215559),(#215560,#215561,#215562),(#215563,#215564,#215565),
(#215566,#215567,#215568),(#215569,#215570,#215571),(#215572,#215573,#215574),
(#215575,#215576,#215577),(#215578,#215579,#215580),(#215581,#215582,#215583),
(#215584,#215585,#215586),(#215587,#215588,#215589),(#215590,#215591,#215592),
(#215593,#215594,#215595),(#215596,#215597,#215598),(#215599,#215600,#215601),
(#215602,#215603,#215604),(#215605,#215606,#215607),(#215608,#215609,#215610),
(#215611,#215612,#215613),(#215614,#215615,#215616),(#215617,#215618,#215619),
(#215620,#215621,#215622),(#215623,#215624,#215625),(#215626,#215627,#215628),
(#215629,#215630,#215631),(#215632,#215633,#215634)),.UNSPECIFIED.,.F.,
 .F.,.F.)
B_SPLINE_SURFACE_WITH_KNOTS((4,2,2,2,2,2,2,2,2,2,2,2,2,2,2,2,4),(3,3),(-0.00016793412709353,
0.000209917658866865,0.000262397073583582,0.000314876488300298,0.000419835317733731,
0.000524794147167163,0.000629752976600596,0.000839670635467461,0.000892150050184177,
0.000944629464900893,0.00104958829433433,0.00115454712376776,0.00125950595320119,
0.00136446478263462,0.00146942361206806,0.00157438244150149,0.00184727539802677),
(-0.00143652655570475,1.),.UNSPECIFIED.)
GEOMETRIC_REPRESENTATION_ITEM()
RATIONAL_B_SPLINE_SURFACE(((1.00022034803097,0.923305270586211,1.),(1.00022057389735,
0.923226655130542,1.),(1.00022076421095,0.923160414238506,1.),(1.00023524475682,
0.918120289566036,1.),(1.00023692961135,0.917533856087476,1.),(1.00023871862926,
0.916911167317056,1.),(1.00023878977867,0.916886402927843,1.),(1.00023921723265,
0.916737622530491,1.),(1.00023970119732,0.916569172922025,1.),(1.00024138488156,
0.915983146777706,1.),(1.00024248924841,0.915598758877892,1.),(1.0002469403122,
0.914049513661833,1.),(1.00025034837882,0.912863295904625,1.),(1.00025724579866,
0.910462567628845,1.),(1.0002572825449,0.910449777668718,1.),(1.00026222873836,
0.9087281967323,1.),(1.00026340408549,0.908319103311859,1.),(1.00026639323709,
0.907278693862733,1.),(1.00026838330125,0.906586028574658,1.),(1.00027374334603,
0.904720401811733,1.),(1.00027683518481,0.903644250881688,1.),(1.00028164305399,
0.901970815340634,1.),(1.00028339221757,0.901361998340541,1.),(1.00028903872358,
0.899396665370392,1.),(1.00029254258302,0.898177105790678,1.),(1.00030090956553,
0.895264878908138,1.),(1.00030479909101,0.893911083719088,1.),(1.00031159097903,
0.891547087035292,1.),(1.00031413159742,0.890662794860912,1.),(1.00032054361863,
0.888431015298873,1.),(1.00032547359281,0.88671507967576,1.),(1.00034206821476,
0.880939125905835,1.),(1.00035112478508,0.877786879858916,1.),(1.00034975691482,
0.87826298322615,1.)))
REPRESENTATION_ITEM('')
SURFACE()
);
#3086=(
BOUNDED_SURFACE()
B_SPLINE_SURFACE(3,2,((#215761,#215762,#215763),(#215764,#215765,#215766),
(#215767,#215768,#215769),(#215770,#215771,#215772)),.UNSPECIFIED.,.F.,
 .F.,.F.)
B_SPLINE_SURFACE_WITH_KNOTS((4,4),(3,3),(-6.93889390390723E-18,0.00418923766731893),
(0.,1.),.UNSPECIFIED.)
GEOMETRIC_REPRESENTATION_ITEM()
RATIONAL_B_SPLINE_SURFACE(((1.,0.881068987521719,1.),(1.,0.880840248614593,
1.),(1.,0.880630793895676,1.),(1.,0.880439575617234,1.)))
REPRESENTATION_ITEM('')
SURFACE()
);
#3087=(
BOUNDED_SURFACE()
B_SPLINE_SURFACE(3,2,((#215778,#215779,#215780),(#215781,#215782,#215783),
(#215784,#215785,#215786),(#215787,#215788,#215789)),.UNSPECIFIED.,.F.,
 .F.,.F.)
B_SPLINE_SURFACE_WITH_KNOTS((4,4),(3,3),(-4.87796775942825E-5,0.000536579322482048),
(-9.19097232831942E-5,1.00000725198376),.UNSPECIFIED.)
GEOMETRIC_REPRESENTATION_ITEM()
RATIONAL_B_SPLINE_SURFACE(((1.00002138549554,0.883659476497807,1.0000016872441),
(1.00002372657649,0.870923620884117,1.00000187194756),(1.00002649051571,
0.85588734854124,1.00000209001312),(1.00002964036462,0.838751665603248,
1.00000233852567)))
REPRESENTATION_ITEM('')
SURFACE()
);
#3088=(
BOUNDED_SURFACE()
B_SPLINE_SURFACE(3,2,((#215810,#215811,#215812),(#215813,#215814,#215815),
(#215816,#215817,#215818),(#215819,#215820,#215821),(#215822,#215823,#215824),
(#215825,#215826,#215827),(#215828,#215829,#215830),(#215831,#215832,#215833),
(#215834,#215835,#215836),(#215837,#215838,#215839),(#215840,#215841,#215842),
(#215843,#215844,#215845),(#215846,#215847,#215848),(#215849,#215850,#215851),
(#215852,#215853,#215854),(#215855,#215856,#215857),(#215858,#215859,#215860),
(#215861,#215862,#215863),(#215864,#215865,#215866),(#215867,#215868,#215869),
(#215870,#215871,#215872),(#215873,#215874,#215875),(#215876,#215877,#215878),
(#215879,#215880,#215881),(#215882,#215883,#215884),(#215885,#215886,#215887),
(#215888,#215889,#215890),(#215891,#215892,#215893),(#215894,#215895,#215896),
(#215897,#215898,#215899),(#215900,#215901,#215902),(#215903,#215904,#215905),
(#215906,#215907,#215908),(#215909,#215910,#215911),(#215912,#215913,#215914),
(#215915,#215916,#215917),(#215918,#215919,#215920),(#215921,#215922,#215923),
(#215924,#215925,#215926),(#215927,#215928,#215929),(#215930,#215931,#215932),
(#215933,#215934,#215935),(#215936,#215937,#215938),(#215939,#215940,#215941),
(#215942,#215943,#215944),(#215945,#215946,#215947),(#215948,#215949,#215950),
(#215951,#215952,#215953),(#215954,#215955,#215956),(#215957,#215958,#215959),
(#215960,#215961,#215962),(#215963,#215964,#215965),(#215966,#215967,#215968),
(#215969,#215970,#215971),(#215972,#215973,#215974),(#215975,#215976,#215977),
(#215978,#215979,#215980),(#215981,#215982,#215983),(#215984,#215985,#215986),
(#215987,#215988,#215989),(#215990,#215991,#215992),(#215993,#215994,#215995),
(#215996,#215997,#215998),(#215999,#216000,#216001),(#216002,#216003,#216004),
(#216005,#216006,#216007),(#216008,#216009,#216010),(#216011,#216012,#216013),
(#216014,#216015,#216016),(#216017,#216018,#216019),(#216020,#216021,#216022),
(#216023,#216024,#216025),(#216026,#216027,#216028),(#216029,#216030,#216031),
(#216032,#216033,#216034),(#216035,#216036,#216037),(#216038,#216039,#216040),
(#216041,#216042,#216043),(#216044,#216045,#216046),(#216047,#216048,#216049),
(#216050,#216051,#216052),(#216053,#216054,#216055),(#216056,#216057,#216058),
(#216059,#216060,#216061),(#216062,#216063,#216064),(#216065,#216066,#216067),
(#216068,#216069,#216070),(#216071,#216072,#216073),(#216074,#216075,#216076),
(#216077,#216078,#216079),(#216080,#216081,#216082),(#216083,#216084,#216085),
(#216086,#216087,#216088),(#216089,#216090,#216091),(#216092,#216093,#216094),
(#216095,#216096,#216097),(#216098,#216099,#216100),(#216101,#216102,#216103),
(#216104,#216105,#216106),(#216107,#216108,#216109),(#216110,#216111,#216112),
(#216113,#216114,#216115),(#216116,#216117,#216118),(#216119,#216120,#216121)),
 .UNSPECIFIED.,.F.,.F.,.F.)
B_SPLINE_SURFACE_WITH_KNOTS((4,2,2,2,2,2,2,2,2,2,2,2,2,2,2,2,2,2,2,2,2,
2,2,2,2,2,2,2,2,2,2,2,2,2,2,2,2,2,2,2,2,2,2,2,2,2,2,2,2,2,2,4),(3,3),(-3.46944695195361E-18,
0.00252618215747139,0.00505236431494278,0.00631545539367848,0.00639439858609946,
0.00647334177852044,0.0066312281633624,0.00694700093304633,0.00757854647241417,
0.0101047286298856,0.0107362741692534,0.0110520469389373,0.0111309901313583,
0.0111704617275688,0.0112099333237793,0.0113678197086213,0.012630910787357,
0.0151570929448283,0.016420184023564,0.0170517295629319,0.0173675023326158,
0.0174464455250368,0.0174859171212473,0.0175253887174578,0.0176832751022998,
0.0189463661810354,0.0202094572597711,0.0227356394172426,0.0228145826096635,
0.022854054205874,0.0228935258020845,0.0230514121869265,0.0233671849566104,
0.0239987304959783,0.025261821574714,0.0277880037321854,0.029051094810921,
0.029208981195763,0.029287924388184,0.029366867580605,0.0296826403502888,
0.0303141858896567,0.0328403680471281,0.0341034591258638,0.0341824023182848,
0.0342218739144953,0.0342613455107057,0.0344192318955477,0.0347350046652317,
0.0353665502045995,0.0378927323620709,0.0404189145195423),(-0.00400343516766361,
1.),.UNSPECIFIED.)
GEOMETRIC_REPRESENTATION_ITEM()
RATIONAL_B_SPLINE_SURFACE(((1.00126205257496,0.842378791948742,1.),(1.00116206025281,
0.854867107353403,1.),(1.00108355000387,0.864672467707073,1.),(1.00095888244726,
0.880242540830635,1.),(1.00091226223324,0.886065067244628,1.),(1.00086179031195,
0.892368643945316,1.),(1.00084832168461,0.894050777759472,1.),(1.00083725616009,
0.89543278147101,1.),(1.00083939692912,0.89516541495365,1.),(1.0008423307566,
0.894799001192412,1.),(1.00084380125902,0.894615346111281,1.),(1.00084822302296,
0.894063099883762,1.),(1.00085118454391,0.893693227408759,1.),(1.00086010596924,
0.892579006126042,1.),(1.00086610276788,0.891830049494227,1.),(1.00088420600063,
0.889569087096759,1.),(1.00089642239576,0.888043347997252,1.),(1.00095780436928,
0.880377184946395,1.),(1.00100879881346,0.874008348928721,1.),(1.00107119105981,
0.866216010132179,1.),(1.00108365614793,0.864659211083758,1.),(1.00110223373256,
0.862339005579313,1.),(1.00110840636504,0.86156808857656,1.),(1.0011160880171,
0.860608705979043,1.),(1.00111762264437,0.860417042169444,1.),(1.0011199218686,
0.860129885748125,1.),(1.00112136395188,0.859949780012029,1.),(1.00111940556711,
0.860194368058238,1.),(1.0011184314474,0.860316028541052,1.),(1.00111358603219,
0.86092118573824,1.),(1.00110979027839,0.861395247842052,1.),(1.00107633361689,
0.86557374207204,1.),(1.00105157373995,0.868666071022459,1.),(1.00098953843601,
0.876413830301835,1.),(1.00096444592774,0.879547702492012,1.),(1.00094661068597,
0.8817751947611,1.),(1.00094402396992,0.882098256823662,1.),(1.00094525304224,
0.881944754610406,1.),(1.00094651635627,0.881786975855158,1.),(1.00094973604407,
0.881384860213925,1.),(1.00095103043371,0.881223200342202,1.),(1.00095293246182,
0.880985650833325,1.),(1.00095332707769,0.880936366175553,1.),(1.00095394048422,
0.88085975615034,1.),(1.00095414853362,0.880833772290365,1.),(1.00095457182273,
0.880780906552175,1.),(1.00095468954101,0.880766204393413,1.),(1.00095544962206,
0.880671275785742,1.),(1.0009560445374,0.880596975178003,1.),(1.00096127208582,
0.879944092315028,1.),(1.0009650012442,0.879478347496011,1.),(1.00096997719539,
0.878856887301876,1.),(1.00097130929268,0.878690518017464,1.),(1.00097096264402,
0.878733811919358,1.),(1.00096516997834,0.879457273826079,1.),(1.0009556328047,
0.880648397604047,1.),(1.00095534056217,0.880684896575533,1.),(1.0009548975107,
0.880740230488282,1.),(1.00095474904569,0.880758772690539,1.),(1.00095445058259,
0.880796048566581,1.),(1.00095424553061,0.880821658070792,1.),(1.00095323023239,
0.880948461449914,1.),(1.00095247254334,0.881043091314579,1.),(1.00095036084046,
0.881306827679129,1.),(1.00094916809947,0.881455792373385,1.),(1.00094622018284,
0.881823965768153,1.),(1.00094509490487,0.881964504820641,1.),(1.00094416392081,
0.882080777973223,1.),(1.00094679343264,0.881752371027292,1.),(1.00096430182822,
0.879565699475922,1.),(1.00098858666124,0.876532700064088,1.),(1.00104815881752,
0.869092570052193,1.),(1.00107185053063,0.866133647012636,1.),(1.00110348918137,
0.862182209133539,1.),(1.00110707459538,0.861734416942979,1.),(1.00111256022933,
0.861049301070322,1.),(1.00111440669401,0.860818691031526,1.),(1.00111813589513,
0.860352940874234,1.),(1.00112173560586,0.859903363126305,1.),(1.00111433813456,
0.860827253609506,1.),(1.00110838255543,0.861571062223461,1.),(1.00109042205054,
0.863814198947867,1.),(1.00107832275572,0.865325313066906,1.),(1.00101749555892,
0.872922188531655,1.),(1.00096720718229,0.879202841836596,1.),(1.00089304098,
0.888465662287133,1.),(1.00086839099238,0.891544266859536,1.),(1.00084316866518,
0.894694352491815,1.),(1.00084168868037,0.894879191853632,1.),(1.00083947448171,
0.895155729198434,1.),(1.00083873737851,0.895247788038785,1.),(1.00083726514029,
0.895431659908763,1.),(1.0008378809652,0.895354747846773,1.),(1.00083952894906,
0.89514892662193,1.),(1.00084089654681,0.894978123586918,1.),(1.00084514785539,
0.894447165996617,1.),(1.0008481799721,0.894068476623283,1.),(1.00085788119072,
0.892856864818009,1.),(1.000865153556,0.891948599169143,1.),(1.0009057894337,
0.886873472934737,1.),(1.00095157280583,0.881155461999917,1.),(1.00107806329298,
0.865357718081277,1.),(1.00116014641827,0.855106131398954,1.),(1.00126205257496,
0.842378791948798,1.)))
REPRESENTATION_ITEM('')
SURFACE()
);
#3089=(
BOUNDED_SURFACE()
B_SPLINE_SURFACE(3,2,((#216727,#216728,#216729),(#216730,#216731,#216732),
(#216733,#216734,#216735),(#216736,#216737,#216738)),.UNSPECIFIED.,.F.,
 .F.,.F.)
B_SPLINE_SURFACE_WITH_KNOTS((4,4),(3,3),(0.0429271655601134,0.046749382327419),
(0.,1.),.UNSPECIFIED.)
GEOMETRIC_REPRESENTATION_ITEM()
RATIONAL_B_SPLINE_SURFACE(((1.,0.922487559402275,1.),(1.,0.922290239059189,
1.),(1.,0.921950699598134,1.),(1.,0.921567721510049,1.)))
REPRESENTATION_ITEM('')
SURFACE()
);
#3090=(
BOUNDED_SURFACE()
B_SPLINE_SURFACE(3,2,((#216765,#216766,#216767),(#216768,#216769,#216770),
(#216771,#216772,#216773),(#216774,#216775,#216776)),.UNSPECIFIED.,.F.,
 .F.,.F.)
B_SPLINE_SURFACE_WITH_KNOTS((4,4),(3,3),(0.0243367909416761,0.0248833749525317),
(0.,1.),.UNSPECIFIED.)
GEOMETRIC_REPRESENTATION_ITEM()
RATIONAL_B_SPLINE_SURFACE(((1.,0.920889968635124,1.),(1.,0.921315643311137,
1.),(1.,0.921538438398832,1.),(1.,0.921567721510049,1.)))
REPRESENTATION_ITEM('')
SURFACE()
);
#3091=(
BOUNDED_SURFACE()
B_SPLINE_SURFACE(3,2,((#216782,#216783,#216784),(#216785,#216786,#216787),
(#216788,#216789,#216790),(#216791,#216792,#216793),(#216794,#216795,#216796),
(#216797,#216798,#216799),(#216800,#216801,#216802),(#216803,#216804,#216805),
(#216806,#216807,#216808),(#216809,#216810,#216811),(#216812,#216813,#216814),
(#216815,#216816,#216817),(#216818,#216819,#216820),(#216821,#216822,#216823),
(#216824,#216825,#216826),(#216827,#216828,#216829),(#216830,#216831,#216832),
(#216833,#216834,#216835),(#216836,#216837,#216838),(#216839,#216840,#216841),
(#216842,#216843,#216844),(#216845,#216846,#216847),(#216848,#216849,#216850),
(#216851,#216852,#216853),(#216854,#216855,#216856),(#216857,#216858,#216859)),
 .UNSPECIFIED.,.F.,.F.,.F.)
B_SPLINE_SURFACE_WITH_KNOTS((4,2,2,2,2,2,2,2,2,2,2,2,4),(3,3),(0.0235924208938234,
0.0238608230039568,0.0239731153899888,0.0240854077760208,0.0243099925480848,
0.0245345773201488,0.0249837468642768,0.0252083316363408,0.0254329164084048,
0.0258820859525327,0.0263312554966607,0.0267804250407887,0.0272734119229856),
(-0.000493556320524505,1.),.UNSPECIFIED.)
GEOMETRIC_REPRESENTATION_ITEM()
RATIONAL_B_SPLINE_SURFACE(((1.00007824284398,0.920735647859346,1.),(1.00007802101355,
0.920960374425325,1.),(1.00007772756555,0.921257653567913,1.),(1.00007739864045,
0.921590872985578,1.),(1.00007731162238,0.92167902712557,1.),(1.00007716427966,
0.921828293494607,1.),(1.00007711979111,0.92187336287521,1.),(1.00007678443583,
0.922213096423567,1.),(1.00007634872583,0.922654494882402,1.),(1.00007544895396,
0.92356601382016,1.),(1.00007500286602,0.924017925712546,1.),(1.0000738906511,
0.925144661281554,1.),(1.00007330799815,0.92573492111959,1.),(1.00007202214984,
0.927037556965429,1.),(1.00007146426924,0.927602721040608,1.),(1.00007035323508,
0.928728260429265,1.),(1.00006984224533,0.929245921461416,1.),(1.00006835495859,
0.930752625641717,1.),(1.00006743638207,0.931683194740616,1.),(1.00006529726307,
0.933850241244143,1.),(1.00006405365497,0.935110085410391,1.),(1.00006152639895,
0.937670336295846,1.),(1.00006031706504,0.938895458806362,1.),(1.00005784890346,
0.941395843745346,1.),(1.0000565320274,0.942729912423448,1.),(1.00005458091539,
0.944706497397475,1.)))
REPRESENTATION_ITEM('')
SURFACE()
);
#3092=(
BOUNDED_SURFACE()
B_SPLINE_SURFACE(3,2,((#217189,#217190,#217191),(#217192,#217193,#217194),
(#217195,#217196,#217197),(#217198,#217199,#217200),(#217201,#217202,#217203),
(#217204,#217205,#217206),(#217207,#217208,#217209),(#217210,#217211,#217212)),
 .UNSPECIFIED.,.F.,.F.,.F.)
B_SPLINE_SURFACE_WITH_KNOTS((4,2,2,4),(3,3),(-6.62670003357417E-5,0.000233612606258176,
0.000467225212516351,0.00100071742536861),(0.,1.00006626700034),
 .UNSPECIFIED.)
GEOMETRIC_REPRESENTATION_ITEM()
RATIONAL_B_SPLINE_SURFACE(((1.,0.958477827751749,1.0000055030996),(1.,0.957369041680115,
1.00000565005146),(1.,0.955803501995477,1.0000058575387),(1.,0.953095633837129,
1.0000062164233),(1.,0.951957652185137,1.00000636724456),(1.,0.9484156097212,
1.00000683668562),(1.,0.946055609381867,1.0000071494659),(1.,0.943163908413987,
1.0000075327146)))
REPRESENTATION_ITEM('')
SURFACE()
);
#3093=(
BOUNDED_SURFACE()
B_SPLINE_SURFACE(3,2,((#217248,#217249,#217250),(#217251,#217252,#217253),
(#217254,#217255,#217256),(#217257,#217258,#217259)),.UNSPECIFIED.,.F.,
 .F.,.F.)
B_SPLINE_SURFACE_WITH_KNOTS((4,4),(3,3),(0.0114568846502287,0.0192019541084939),
(0.,1.),.UNSPECIFIED.)
GEOMETRIC_REPRESENTATION_ITEM()
RATIONAL_B_SPLINE_SURFACE(((1.,0.957684062981984,1.),(1.,0.957879658663776,
1.),(1.,0.958058054935734,1.),(1.,0.958218732174581,1.)))
REPRESENTATION_ITEM('')
SURFACE()
);
#3094=(
BOUNDED_SURFACE()
B_SPLINE_SURFACE(3,2,((#217281,#217282,#217283),(#217284,#217285,#217286),
(#217287,#217288,#217289),(#217290,#217291,#217292)),.UNSPECIFIED.,.F.,
 .F.,.F.)
B_SPLINE_SURFACE_WITH_KNOTS((4,4),(3,3),(0.00543385294581827,0.00566356273029558),
(0.,1.0000263042412),.UNSPECIFIED.)
GEOMETRIC_REPRESENTATION_ITEM()
RATIONAL_B_SPLINE_SURFACE(((1.,0.991880174791391,1.00000042717168),(1.,
0.993019568317563,1.00000036722992),(1.,0.993924546422819,1.00000031962039),
(0.999999999999999,0.994332871227875,1.00000029813904)))
REPRESENTATION_ITEM('')
SURFACE()
);
#3095=(
BOUNDED_SURFACE()
B_SPLINE_SURFACE(3,2,((#217307,#217308,#217309),(#217310,#217311,#217312),
(#217313,#217314,#217315),(#217316,#217317,#217318),(#217319,#217320,#217321),
(#217322,#217323,#217324)),.UNSPECIFIED.,.F.,.F.,.F.)
B_SPLINE_SURFACE_WITH_KNOTS((4,2,4),(3,3),(-1.09829680072782E-16,0.000498949606022071,
0.000997899212044251),(0.,1.),.UNSPECIFIED.)
GEOMETRIC_REPRESENTATION_ITEM()
RATIONAL_B_SPLINE_SURFACE(((1.,0.994220746859027,1.),(1.,0.996098915568006,
1.),(1.,0.997550054459957,1.),(1.,0.99950507842482,1.),(1.,1.00000638742927,
1.),(1.,1.,1.)))
REPRESENTATION_ITEM('')
SURFACE()
);
#3096=(
BOUNDED_SURFACE()
B_SPLINE_SURFACE(3,2,((#217350,#217351,#217352),(#217353,#217354,#217355),
(#217356,#217357,#217358),(#217359,#217360,#217361),(#217362,#217363,#217364),
(#217365,#217366,#217367),(#217368,#217369,#217370),(#217371,#217372,#217373),
(#217374,#217375,#217376),(#217377,#217378,#217379),(#217380,#217381,#217382),
(#217383,#217384,#217385),(#217386,#217387,#217388),(#217389,#217390,#217391),
(#217392,#217393,#217394),(#217395,#217396,#217397),(#217398,#217399,#217400),
(#217401,#217402,#217403),(#217404,#217405,#217406),(#217407,#217408,#217409),
(#217410,#217411,#217412),(#217413,#217414,#217415),(#217416,#217417,#217418),
(#217419,#217420,#217421),(#217422,#217423,#217424),(#217425,#217426,#217427),
(#217428,#217429,#217430),(#217431,#217432,#217433),(#217434,#217435,#217436),
(#217437,#217438,#217439),(#217440,#217441,#217442),(#217443,#217444,#217445),
(#217446,#217447,#217448),(#217449,#217450,#217451),(#217452,#217453,#217454),
(#217455,#217456,#217457),(#217458,#217459,#217460),(#217461,#217462,#217463),
(#217464,#217465,#217466),(#217467,#217468,#217469),(#217470,#217471,#217472),
(#217473,#217474,#217475),(#217476,#217477,#217478),(#217479,#217480,#217481),
(#217482,#217483,#217484),(#217485,#217486,#217487),(#217488,#217489,#217490),
(#217491,#217492,#217493),(#217494,#217495,#217496),(#217497,#217498,#217499),
(#217500,#217501,#217502),(#217503,#217504,#217505),(#217506,#217507,#217508),
(#217509,#217510,#217511),(#217512,#217513,#217514),(#217515,#217516,#217517),
(#217518,#217519,#217520),(#217521,#217522,#217523),(#217524,#217525,#217526),
(#217527,#217528,#217529),(#217530,#217531,#217532),(#217533,#217534,#217535),
(#217536,#217537,#217538),(#217539,#217540,#217541),(#217542,#217543,#217544),
(#217545,#217546,#217547),(#217548,#217549,#217550),(#217551,#217552,#217553),
(#217554,#217555,#217556),(#217557,#217558,#217559),(#217560,#217561,#217562),
(#217563,#217564,#217565),(#217566,#217567,#217568),(#217569,#217570,#217571),
(#217572,#217573,#217574),(#217575,#217576,#217577),(#217578,#217579,#217580),
(#217581,#217582,#217583),(#217584,#217585,#217586),(#217587,#217588,#217589),
(#217590,#217591,#217592),(#217593,#217594,#217595),(#217596,#217597,#217598),
(#217599,#217600,#217601),(#217602,#217603,#217604),(#217605,#217606,#217607),
(#217608,#217609,#217610),(#217611,#217612,#217613),(#217614,#217615,#217616),
(#217617,#217618,#217619),(#217620,#217621,#217622),(#217623,#217624,#217625),
(#217626,#217627,#217628),(#217629,#217630,#217631),(#217632,#217633,#217634),
(#217635,#217636,#217637),(#217638,#217639,#217640),(#217641,#217642,#217643),
(#217644,#217645,#217646),(#217647,#217648,#217649),(#217650,#217651,#217652),
(#217653,#217654,#217655),(#217656,#217657,#217658),(#217659,#217660,#217661),
(#217662,#217663,#217664),(#217665,#217666,#217667),(#217668,#217669,#217670),
(#217671,#217672,#217673),(#217674,#217675,#217676),(#217677,#217678,#217679),
(#217680,#217681,#217682),(#217683,#217684,#217685),(#217686,#217687,#217688),
(#217689,#217690,#217691),(#217692,#217693,#217694),(#217695,#217696,#217697),
(#217698,#217699,#217700),(#217701,#217702,#217703),(#217704,#217705,#217706),
(#217707,#217708,#217709),(#217710,#217711,#217712),(#217713,#217714,#217715),
(#217716,#217717,#217718),(#217719,#217720,#217721),(#217722,#217723,#217724),
(#217725,#217726,#217727),(#217728,#217729,#217730),(#217731,#217732,#217733),
(#217734,#217735,#217736),(#217737,#217738,#217739),(#217740,#217741,#217742),
(#217743,#217744,#217745),(#217746,#217747,#217748),(#217749,#217750,#217751)),
 .UNSPECIFIED.,.F.,.F.,.F.)
B_SPLINE_SURFACE_WITH_KNOTS((4,2,2,2,2,2,2,2,2,2,2,2,2,2,2,2,2,2,2,2,2,
2,2,2,2,2,2,2,2,2,2,2,2,2,2,2,2,2,2,2,2,2,2,2,2,2,2,2,2,2,2,2,2,2,2,2,2,
2,2,2,2,2,2,2,2,2,4),(3,3),(0.0401209448553485,0.0422079288610133,0.0442949128666782,
0.046381896872343,0.0484688808780079,0.0526428488893376,0.0527732853896916,
0.0528385036398687,0.0529037218900457,0.0531645948907538,0.05368634089217,
0.0547298328950024,0.0568168169006673,0.0578603089034997,0.0589038009063321,
0.0599472929091645,0.0602081659098726,0.0603386024102267,0.0603712115353152,
0.0604038206604037,0.0604690389105808,0.060990784911997,0.0651647529233267,
0.0693387209346564,0.0698604669360726,0.0701213399367807,0.0701865581869577,
0.0702191673120462,0.0702517764371347,0.0703822129374888,0.0714257049403212,
0.0724691969431537,0.0735126889459861,0.0755996729516509,0.0766431649544833,
0.0771649109558996,0.0774257839566077,0.0775562204569617,0.0776214387071387,
0.0776540478322272,0.0776866569573158,0.0818606249686455,0.0860345929799752,
0.0870780849828076,0.0873389579835157,0.0874041762336927,0.0874367853587812,
0.0874530899213255,0.0874693944838697,0.0875998309842238,0.08812157698564,
0.0902085609913048,0.0943825290026346,0.0946434020033427,0.0947086202535197,
0.0947412293786082,0.0947738385036967,0.0949042750040508,0.095426021005467,
0.0964695130082994,0.0985564970139642,0.100643481019629,0.101686973022461,
0.102730465025294,0.104817449030959,0.105860941033791,0.106904433036624),
(0.,1.00211619801959),.UNSPECIFIED.)
GEOMETRIC_REPRESENTATION_ITEM()
RATIONAL_B_SPLINE_SURFACE(((1.,0.967623608150263,1.00013702971263),(1.,
0.967362278939665,1.00013813576134),(1.,0.966893393913631,1.00014012026847),
(1.,0.965707706678196,1.00014513856643),(1.,0.964990163383989,1.00014817549383),
(1.,0.9633845862752,1.00015497093202),(1.,0.962494992184358,1.00015873604653),
(1.,0.960578187950096,1.00016684872118),(1.,0.959565053500142,1.00017113670741),
(1.,0.956390754090381,1.00018457159966),(1.,0.954097360891505,1.00019427814795),
(1.,0.951539895136251,1.00020510235588),(1.,0.951462206912974,1.00020543116321),
(1.,0.951345387989037,1.00020592558716),(1.,0.951437397555211,1.00020553616624),
(1.,0.951546321977574,1.00020507515495),(1.,0.951600611930997,1.00020484537836),
(1.,0.951871196160378,1.00020370015874),(1.,0.95208489429128,1.00020279570362),
(1.,0.952717506711006,1.00020011823732),(1.,0.9531279452915,1.0001983810987),
(1.,0.954323738610181,1.00019332002779),(1.,0.955073684874735,1.00019014595819),
(1.,0.957165050829292,1.00018129446921),(1.,0.95832888484391,1.00017636866273),
(1.,0.959643495316587,1.00017080471058),(1.,0.96000598572915,1.00016927050759),
(1.,0.960567494657221,1.00016689397943),(1.,0.960766569834018,1.00016605141444),
(1.,0.960982622872878,1.00016513699241),(1.,0.961000543757655,1.00016506114413),
(1.,0.96090658055613,1.00016545883361),(1.,0.960881962556224,1.00016556302674),
(1.,0.960836203436817,1.00016575669745),(1.,0.960819478259316,1.00016582748503),
(1.,0.960796720866671,1.00016592380333),(1.,0.960792076839665,1.00016594345869),
(1.,0.960782603408868,1.000165983554),(1.,0.960772649057408,1.00016602568476),
(1.,0.960780513429616,1.00016599239962),(1.,0.960785654845429,1.00016597063911),
(1.,0.960831021621874,1.00016577862895),(1.,0.960864910012085,1.00016563519986),
(1.,0.961115514496332,1.00016457454243),(1.,0.960966587611861,1.00016520485999),
(1.,0.960110029748364,1.0001688301521),(1.,0.959400389202501,1.00017183363193),
(1.,0.958222276120302,1.00017681987307),(1.,0.958085899137497,1.00017739707448),
(1.,0.957872770035717,1.00017829912124),(1.,0.957800412888855,1.00017860536534),
(1.,0.95770829518048,1.00017899524397),(1.,0.957689788065446,1.00017907357341),
(1.,0.957661901465818,1.00017919160054),(1.,0.95763491988757,1.00017930579727),
(1.,0.957663736151373,1.00017918383543),(1.,0.957678073075429,1.00017912315589),
(1.,0.95774940029199,1.00017882127086),(1.,0.957805318337416,1.00017858460354),
(1.,0.958298133029376,1.00017649881659),(1.,0.958661487087527,1.00017496095832),
(1.,0.959225394163478,1.00017257428024),(1.,0.95942600733162,1.00017172520586),
(1.,0.959652210338516,1.00017076782515),(1.,0.959678704973595,1.00017065568936),
(1.,0.959505481141619,1.00017138884122),(1.,0.959051697202111,1.00017330943457),
(1.,0.957920993157528,1.00017809502189),(1.,0.957469248115843,1.00018000698582),
(1.,0.956690162824021,1.00018330438332),(1.,0.956413411772314,1.00018447570338),
(1.,0.955974090823865,1.00018633508362),(1.,0.955823630472945,1.00018697189141),
(1.,0.955592121576858,1.00018795172875),(1.,0.955513982296279,1.00018828244513),
(1.,0.955395346065634,1.00018878456064),(1.,0.955355562774398,1.00018895293929),
(1.,0.955295534454033,1.00018920700291),(1.,0.955275466116547,1.00018929194006),
(1.,0.955235212224026,1.00018946231048),(1.,0.955274232783486,1.00018929716002),
(1.,0.957038052415492,1.00018183197679),(1.,0.95849806843578,1.00017565261077),
(1.,0.960891755654296,1.00016552157847),(1.,0.961835644094202,1.00016152666877),
(1.,0.962570204344262,1.00015841771888),(1.,0.962693730785603,1.00015789490606),
(1.,0.962813772003151,1.00015738684409),(1.,0.962836055292866,1.00015729253238),
(1.,0.96286165511172,1.00015718418381),(1.,0.962866662329318,1.00015716299128),
(1.,0.962874002098797,1.00015713192647),(1.,0.962876420178934,1.00015712169219),
(1.,0.962880004288309,1.00015710652282),(1.,0.962881191823016,1.00015710149671),
(1.,0.962883552514071,1.00015709150533),(1.,0.962881342518526,1.0001571008589),
(1.,0.9628719610535,1.00015714056498),(1.,0.9628618314315,1.00015718343755),
(1.,0.96280234657013,1.00015743520104),(1.,0.962726499029366,1.00015775621787),
(1.,0.962212615381494,1.00015993117699),(1.,0.961365351871455,1.00016351713171),
(1.,0.957821561850805,1.00017851585456),(1.,0.954121811281669,1.00019417466422),
(1.,0.949559520376701,1.00021348408617),(1.,0.949288571068739,1.00021463085095),
(1.,0.948946738814693,1.00021607762043),(1.,0.948878215048348,1.00021636764015),
(1.,0.94877519479492,1.00021680366266),(1.,0.948740815609189,1.00021694916899),
(1.,0.948671979258847,1.00021724051168),(1.,0.94874268099657,1.00021694127393),
(1.,0.948863910971176,1.00021642818066),(1.,0.948960718690678,1.00021601845206),
(1.,0.949443885738123,1.00021397349776),(1.,0.949827631882834,1.0002123493321),
(1.,0.950970846836433,1.00020751079365),(1.,0.951721934475459,1.00020433189331),
(1.,0.95394845818276,1.00019490836319),(1.,0.955398313814889,1.00018877199995),
(1.,0.958226868294617,1.00017680043717),(1.,0.95960518223231,1.00017096686672),
(1.,0.961607109424986,1.000162493918),(1.,0.962265389719952,1.00015970781509),
(1.,0.963540595600696,1.00015431063877),(1.,0.96415834401959,1.00015169608281),
(1.,0.965941790209826,1.00014414783222),(1.,0.967040962196452,1.00013949570105),
(1.,0.96847419378806,1.00013342969734),(1.,0.968915400040616,1.00013156233775),
(1.,0.969701097798822,1.00012823695367),(1.,0.970046784443818,1.00012677387088),
(1.,0.970321492872041,1.00012561119602)))
REPRESENTATION_ITEM('')
SURFACE()
);
#3097=(
BOUNDED_SURFACE()
B_SPLINE_SURFACE(3,2,((#218553,#218554,#218555),(#218556,#218557,#218558),
(#218559,#218560,#218561),(#218562,#218563,#218564),(#218565,#218566,#218567),
(#218568,#218569,#218570)),.UNSPECIFIED.,.F.,.F.,.F.)
B_SPLINE_SURFACE_WITH_KNOTS((4,2,4),(3,3),(-2.65828754408143E-15,0.000518614521426172,
0.001037229042855),(0.,1.),.UNSPECIFIED.)
GEOMETRIC_REPRESENTATION_ITEM()
RATIONAL_B_SPLINE_SURFACE(((1.,0.994246489501235,1.),(1.,0.99609478928193,
1.),(1.,0.997541267372286,1.),(1.,0.999499888835022,1.),(1.,1.00000732330262,
1.),(1.,1.,1.)))
REPRESENTATION_ITEM('')
SURFACE()
);
#3098=(
BOUNDED_SURFACE()
B_SPLINE_SURFACE(3,2,((#218579,#218580,#218581),(#218582,#218583,#218584),
(#218585,#218586,#218587),(#218588,#218589,#218590)),.UNSPECIFIED.,.F.,
 .F.,.F.)
B_SPLINE_SURFACE_WITH_KNOTS((4,4),(3,3),(0.0119444722538381,0.0121107952282447),
(-2.03695309557864E-5,1.),.UNSPECIFIED.)
GEOMETRIC_REPRESENTATION_ITEM()
RATIONAL_B_SPLINE_SURFACE(((1.00000029293976,0.992809364237771,1.),(1.0000002643703,
0.993510643385671,1.),(1.00000024275696,0.994041174404857,1.),(1.0000002313304,
0.994321656227528,1.)))
REPRESENTATION_ITEM('')
SURFACE()
);
#3099=(
BOUNDED_SURFACE()
B_SPLINE_SURFACE(3,2,((#218605,#218606,#218607),(#218608,#218609,#218610),
(#218611,#218612,#218613),(#218614,#218615,#218616)),.UNSPECIFIED.,.F.,
 .F.,.F.)
B_SPLINE_SURFACE_WITH_KNOTS((4,4),(3,3),(0.0657640091385094,0.0735516090029935),
(0.,1.),.UNSPECIFIED.)
GEOMETRIC_REPRESENTATION_ITEM()
RATIONAL_B_SPLINE_SURFACE(((1.,0.958250447061442,1.),(1.,0.958411329127679,
1.),(1.,0.958554518262528,1.),(1.,0.958680046125676,1.)))
REPRESENTATION_ITEM('')
SURFACE()
);
#3100=(
BOUNDED_SURFACE()
B_SPLINE_SURFACE(3,2,((#218622,#218623,#218624),(#218625,#218626,#218627),
(#218628,#218629,#218630),(#218631,#218632,#218633),(#218634,#218635,#218636),
(#218637,#218638,#218639)),.UNSPECIFIED.,.F.,.F.,.F.)
B_SPLINE_SURFACE_WITH_KNOTS((4,2,4),(3,3),(-7.50126731622146E-5,0.000375063365810873,
0.000825139404783385),(0.,1.00007657360774),.UNSPECIFIED.)
GEOMETRIC_REPRESENTATION_ITEM()
RATIONAL_B_SPLINE_SURFACE(((1.,0.949070591842026,1.00000779969705),(1.,
0.950903281061525,1.00000751902579),(1.,0.952484216272804,1.00000727690997),
(1.,0.955845362028548,1.00000676215986),(1.,0.957638657720463,1.00000648752161),
(1.,0.95893329183817,1.000006289252)))
REPRESENTATION_ITEM('')
SURFACE()
);
#3101=(
BOUNDED_SURFACE()
B_SPLINE_SURFACE(3,2,((#218663,#218664,#218665),(#218666,#218667,#218668),
(#218669,#218670,#218671),(#218672,#218673,#218674),(#218675,#218676,#218677),
(#218678,#218679,#218680),(#218681,#218682,#218683),(#218684,#218685,#218686),
(#218687,#218688,#218689),(#218690,#218691,#218692),(#218693,#218694,#218695),
(#218696,#218697,#218698),(#218699,#218700,#218701),(#218702,#218703,#218704),
(#218705,#218706,#218707),(#218708,#218709,#218710),(#218711,#218712,#218713),
(#218714,#218715,#218716),(#218717,#218718,#218719),(#218720,#218721,#218722),
(#218723,#218724,#218725),(#218726,#218727,#218728),(#218729,#218730,#218731),
(#218732,#218733,#218734),(#218735,#218736,#218737),(#218738,#218739,#218740)),
 .UNSPECIFIED.,.F.,.F.,.F.)
B_SPLINE_SURFACE_WITH_KNOTS((4,2,2,2,2,2,2,2,2,2,2,2,4),(3,3),(0.0241531416828426,
0.0246199912180733,0.0250868407533039,0.0255536902885345,0.0260205398237651,
0.0262539645913804,0.0264873893589958,0.0269542388942264,0.0271876636618417,
0.0274210884294571,0.0275378008132647,0.0276545131970724,0.0278879379646877),
(-0.000276129488825748,1.),.UNSPECIFIED.)
GEOMETRIC_REPRESENTATION_ITEM()
RATIONAL_B_SPLINE_SURFACE(((1.00002763636452,0.949957600265961,1.),(1.00002829348857,
0.948767716395043,1.),(1.00002907932003,0.947344776267276,1.),(1.00003027374605,
0.945181975713108,1.),(1.0000307912165,0.944244968855354,1.),(1.00003199625233,
0.942062956644543,1.),(1.00003261518263,0.940942231912179,1.),(1.00003371198137,
0.938956209428044,1.),(1.00003417137706,0.938124361131481,1.),(1.00003487381759,
0.936852420695295,1.),(1.00003511037192,0.936424081193685,1.),(1.00003560979616,
0.935519751421037,1.),(1.00003589402015,0.935005094353774,1.),(1.00003656004965,
0.933799084975963,1.),(1.00003684769454,0.933278233520713,1.),(1.00003736403339,
0.93234327571486,1.),(1.00003756245292,0.931983988594581,1.),(1.00003795892861,
0.931266072365573,1.),(1.0000381530246,0.930914614077073,1.),(1.0000383348696,
0.930585339209706,1.),(1.00003836897905,0.930523575717338,1.),(1.000038451592,
0.930373984741388,1.),(1.00003849806418,0.930289835502992,1.),(1.00003864575439,
0.930022406245385,1.),(1.00003875609486,0.929822607823737,1.),(1.00003883615842,
0.929677633147427,1.)))
REPRESENTATION_ITEM('')
SURFACE()
);
#3102=(
BOUNDED_SURFACE()
B_SPLINE_SURFACE(3,2,((#219004,#219005,#219006),(#219007,#219008,#219009),
(#219010,#219011,#219012),(#219013,#219014,#219015)),.UNSPECIFIED.,.F.,
 .F.,.F.)
B_SPLINE_SURFACE_WITH_KNOTS((4,4),(3,3),(0.0249863231317726,0.0253614725245169),
(0.,1.),.UNSPECIFIED.)
GEOMETRIC_REPRESENTATION_ITEM()
RATIONAL_B_SPLINE_SURFACE(((1.,0.930070526504304,1.),(1.,0.930041043693297,
1.),(1.,0.929915461335265,1.),(1.,0.929697045866144,1.)))
REPRESENTATION_ITEM('')
SURFACE()
);
#3103=(
BOUNDED_SURFACE()
B_SPLINE_SURFACE(3,2,((#219021,#219022,#219023),(#219024,#219025,#219026),
(#219027,#219028,#219029),(#219030,#219031,#219032)),.UNSPECIFIED.,.F.,
 .F.,.F.)
B_SPLINE_SURFACE_WITH_KNOTS((4,4),(3,3),(0.0387340315057144,0.0427072915207103),
(0.,1.),.UNSPECIFIED.)
GEOMETRIC_REPRESENTATION_ITEM()
RATIONAL_B_SPLINE_SURFACE(((1.,0.930070526504304,1.),(1.,0.930612186341169,
1.),(1.,0.931191283587816,1.),(1.,0.931676951123116,1.)))
REPRESENTATION_ITEM('')
SURFACE()
);
#3104=(
BOUNDED_SURFACE()
B_SPLINE_SURFACE(3,2,((#219068,#219069,#219070),(#219071,#219072,#219073),
(#219074,#219075,#219076),(#219077,#219078,#219079),(#219080,#219081,#219082),
(#219083,#219084,#219085),(#219086,#219087,#219088),(#219089,#219090,#219091),
(#219092,#219093,#219094),(#219095,#219096,#219097),(#219098,#219099,#219100),
(#219101,#219102,#219103),(#219104,#219105,#219106),(#219107,#219108,#219109),
(#219110,#219111,#219112),(#219113,#219114,#219115),(#219116,#219117,#219118),
(#219119,#219120,#219121),(#219122,#219123,#219124),(#219125,#219126,#219127),
(#219128,#219129,#219130),(#219131,#219132,#219133),(#219134,#219135,#219136),
(#219137,#219138,#219139),(#219140,#219141,#219142),(#219143,#219144,#219145),
(#219146,#219147,#219148),(#219149,#219150,#219151),(#219152,#219153,#219154),
(#219155,#219156,#219157),(#219158,#219159,#219160),(#219161,#219162,#219163),
(#219164,#219165,#219166),(#219167,#219168,#219169),(#219170,#219171,#219172),
(#219173,#219174,#219175),(#219176,#219177,#219178),(#219179,#219180,#219181),
(#219182,#219183,#219184),(#219185,#219186,#219187),(#219188,#219189,#219190),
(#219191,#219192,#219193),(#219194,#219195,#219196),(#219197,#219198,#219199),
(#219200,#219201,#219202),(#219203,#219204,#219205),(#219206,#219207,#219208),
(#219209,#219210,#219211),(#219212,#219213,#219214),(#219215,#219216,#219217),
(#219218,#219219,#219220),(#219221,#219222,#219223),(#219224,#219225,#219226),
(#219227,#219228,#219229),(#219230,#219231,#219232),(#219233,#219234,#219235),
(#219236,#219237,#219238),(#219239,#219240,#219241),(#219242,#219243,#219244),
(#219245,#219246,#219247),(#219248,#219249,#219250),(#219251,#219252,#219253),
(#219254,#219255,#219256),(#219257,#219258,#219259),(#219260,#219261,#219262),
(#219263,#219264,#219265),(#219266,#219267,#219268),(#219269,#219270,#219271),
(#219272,#219273,#219274),(#219275,#219276,#219277),(#219278,#219279,#219280),
(#219281,#219282,#219283),(#219284,#219285,#219286),(#219287,#219288,#219289),
(#219290,#219291,#219292),(#219293,#219294,#219295),(#219296,#219297,#219298),
(#219299,#219300,#219301),(#219302,#219303,#219304),(#219305,#219306,#219307),
(#219308,#219309,#219310),(#219311,#219312,#219313),(#219314,#219315,#219316),
(#219317,#219318,#219319),(#219320,#219321,#219322),(#219323,#219324,#219325),
(#219326,#219327,#219328),(#219329,#219330,#219331),(#219332,#219333,#219334),
(#219335,#219336,#219337),(#219338,#219339,#219340),(#219341,#219342,#219343),
(#219344,#219345,#219346),(#219347,#219348,#219349),(#219350,#219351,#219352),
(#219353,#219354,#219355),(#219356,#219357,#219358),(#219359,#219360,#219361),
(#219362,#219363,#219364),(#219365,#219366,#219367),(#219368,#219369,#219370),
(#219371,#219372,#219373),(#219374,#219375,#219376),(#219377,#219378,#219379),
(#219380,#219381,#219382),(#219383,#219384,#219385),(#219386,#219387,#219388),
(#219389,#219390,#219391),(#219392,#219393,#219394),(#219395,#219396,#219397),
(#219398,#219399,#219400),(#219401,#219402,#219403),(#219404,#219405,#219406),
(#219407,#219408,#219409),(#219410,#219411,#219412),(#219413,#219414,#219415),
(#219416,#219417,#219418),(#219419,#219420,#219421),(#219422,#219423,#219424),
(#219425,#219426,#219427),(#219428,#219429,#219430),(#219431,#219432,#219433),
(#219434,#219435,#219436),(#219437,#219438,#219439),(#219440,#219441,#219442),
(#219443,#219444,#219445)),.UNSPECIFIED.,.F.,.F.,.F.)
B_SPLINE_SURFACE_WITH_KNOTS((4,2,2,2,2,2,2,2,2,2,2,2,2,2,2,2,2,2,2,2,2,
2,2,2,2,2,2,2,2,2,2,2,2,2,2,2,2,2,2,2,2,2,2,2,2,2,2,2,2,2,2,2,2,2,2,2,2,
2,2,2,2,2,4),(3,3),(-0.0208001925820885,-0.0186971148351636,-0.0165940370882388,
-0.0123878815943892,-0.0113363427209268,-0.0108105732841956,-0.0107448521046042,
-0.0106791309250128,-0.01054768856583,-0.0102848038474644,-0.00818172610053958,
-0.00397557060668997,-0.00292403173322756,-0.00279258937404477,-0.00272686819445337,
-0.00266114701486196,-0.00239826229649636,-0.00187249285976516,0.000230584887159648,
0.00443674038100926,0.00653981812793407,0.00759135700139648,0.00811712643812768,
0.00824856879731048,0.00831428997690188,0.00834715056669758,0.00838001115649328,
0.00864289587485888,0.0107459736217837,0.0117975124952461,0.0128490513687085,
0.0139005902421709,0.0149521291156333,0.0170552068625581,0.0181067457360205,
0.0181724669156119,0.0182053275054076,0.0182381880952033,0.0183696304543861,
0.0186325151727517,0.0191582846094829,0.0212613623564077,0.0254675178502573,
0.0275705955971822,0.0286221344706445,0.0291479039073758,0.0291807644971715,
0.0292136250869671,0.0292464856767628,0.0292793462665586,0.0294107886257414,
0.029673673344107,0.0338798288379566,0.0359829065848814,0.0365086760216126,
0.0367715607399782,0.036903003099161,0.0369687242787524,0.0370344454583438,
0.0380859843318062,0.0422921398256558,0.0443952175725807,0.0464982953195054),
(-0.000276885655367279,1.),.UNSPECIFIED.)
GEOMETRIC_REPRESENTATION_ITEM()
RATIONAL_B_SPLINE_SURFACE(((1.0000178221674,0.967816737606249,1.),(1.00001842741335,
0.966723784718768,1.),(1.00001902799113,0.965639261620645,1.),(1.00002019116422,
0.963538804148879,1.),(1.00002075669582,0.962517567422574,1.),(1.00002238403677,
0.959578915815827,1.),(1.00002337031455,0.957797895819759,1.),(1.00002455994145,
0.955649668060796,1.),(1.00002479580039,0.955223754076267,1.),(1.00002514701149,
0.954589537228534,1.),(1.00002526365088,0.954378909864324,1.),(1.00002539442655,
0.954142755210289,1.),(1.00002535993735,0.954205035799784,1.),(1.00002530498449,
0.954304269644752,1.),(1.00002527759341,0.95435373244978,1.),(1.00002519567715,
0.954501656806086,1.),(1.00002514140894,0.954599654306862,1.),(1.00002497963994,
0.954891776693891,1.),(1.00002487317471,0.955084031573329,1.),(1.00002392760603,
0.956791539099975,1.),(1.00002317337716,0.958153525278607,1.),(1.00002124289493,
0.961639589270802,1.),(1.00002040044771,0.963160880111278,1.),(1.00002005485079,
0.963784958886781,1.),(1.00002002036804,0.96384722781288,1.),(1.00002002020255,
0.96384752666274,1.),(1.00002002072063,0.963846591104061,1.),(1.00002002230128,
0.963843736761046,1.),(1.00002003224056,0.963825788430608,1.),(1.00002004614413,
0.963800681366758,1.),(1.0000200530961,0.963788127505428,1.),(1.00002008785585,
0.963725358348255,1.),(1.00002011566327,0.963675143731717,1.),(1.00002019904931,
0.963524565254967,1.),(1.00002025459039,0.963424269201259,1.),(1.00002053167059,
0.962923917881688,1.),(1.00002075111335,0.962527648246921,1.),(1.00002139578426,
0.961363501776867,1.),(1.00002180611404,0.960622528444111,1.),(1.00002240703783,
0.959537380513288,1.),(1.00002260586054,0.959178346540822,1.),(1.00002290466648,
0.958638762910466,1.),(1.00002300423325,0.958458965270393,1.),(1.00002315445808,
0.958187689342807,1.),(1.00002320468023,0.958096998204385,1.),(1.00002326775072,
0.957983105536474,1.),(1.00002328037942,0.957960300638801,1.),(1.00002329935517,
0.957926034231589,1.),(1.00002330568552,0.957914602889172,1.),(1.00002331518898,
0.957897441554315,1.),(1.00002331835812,0.957891718722412,1.),(1.00002332469909,
0.957880268198829,1.),(1.0000233342893,0.957862950189563,1.),(1.00002326570032,
0.957986808148111,1.),(1.00002320624477,0.958094172961626,1.),(1.00002268469492,
0.959035987448788,1.),(1.00002231597137,0.959701828289977,1.),(1.00002192048742,
0.960415993042883,1.),(1.00002181534814,0.960605853508497,1.),(1.00002165963563,
0.960887039090721,1.),(1.00002161074628,0.960975323464167,1.),(1.00002156885829,
0.961050964778899,1.),(1.00002157262121,0.961044169689148,1.),(1.00002163274295,
0.960935601880239,1.),(1.00002169236395,0.960827938305037,1.),(1.00002195462671,
0.960354344324168,1.),(1.00002223986213,0.959839266325176,1.),(1.00002282165689,
0.95878866158457,1.),(1.00002304014723,0.958394111825039,1.),(1.00002329817088,
0.957928172825059,1.),(1.00002331344442,0.957900591864297,1.),(1.00002333649845,
0.957858960912326,1.),(1.00002332375725,0.957881968962704,1.),(1.00002331736747,
0.957893507631862,1.),(1.00002331417392,0.957899274538583,1.),(1.00002329821279,
0.957928097152465,1.),(1.000023285465,0.957951117104651,1.),(1.0000232472804,
0.9580200708351,1.),(1.00002322190232,0.958065898550066,1.),(1.00002314596772,
0.958203021226092,1.),(1.00002309561029,0.958293956657091,1.),(1.00002284471333,
0.958747026277197,1.),(1.00002264663059,0.959104724004719,1.),(1.00002204771429,
0.960186246811101,1.),(1.00002164152455,0.960919744067784,1.),(1.00002099795675,
0.962081898526066,1.),(1.00002077788797,0.962479298636387,1.),(1.00002044118626,
0.963087314445631,1.),(1.00002032779168,0.963292082332173,1.),(1.00002015724606,
0.963600053539546,1.),(1.0000201003211,0.963702848610252,1.),(1.00002003985951,
0.963812030128801,1.),(1.00002003630303,0.963818452413985,1.),(1.0000200291903,
0.963831296571643,1.),(1.00002002404297,0.963840591621128,1.),(1.00002002011293,
0.963847688499234,1.),(1.00002002151763,0.963845151877356,1.),(1.0000200210696,
0.963845960940693,1.),(1.00002002088064,0.963846302169928,1.),(1.00002002011118,
0.963847691658443,1.),(1.00002002005674,0.963847789958493,1.),(1.0000200215801,
0.963845039083613,1.),(1.00002002484447,0.96383914428714,1.),(1.00002011873487,
0.963669597025071,1.),(1.00002080897953,0.962423153516154,1.),(1.00002261635824,
0.95915938980657,1.),(1.00002334790121,0.957838369809624,1.),(1.00002438902999,
0.955958299899251,1.),(1.00002460376163,0.955570537600982,1.),(1.00002493505981,
0.954972279475213,1.),(1.00002504702576,0.954770091421123,1.),(1.00002521723854,
0.954462721246432,1.),(1.00002527435347,0.954359583139847,1.),(1.00002536058752,
0.954203861714998,1.),(1.0000253934109,0.954144589270825,1.),(1.00002536300565,
0.954199495063233,1.),(1.00002534779637,0.954226959973017,1.),(1.0000250891242,
0.954694070074855,1.),(1.00002484395155,0.955136802747112,1.),(1.00002360770641,
0.95736921369098,1.),(1.00002258796812,0.959210656666961,1.),(1.00002090417295,
0.962251253288119,1.),(1.000020317103,0.963311383954806,1.),(1.00001908992458,
0.965527422225216,1.),(1.0000184437515,0.966694281295037,1.),(1.00001779951518,
0.967857642975733,1.)))
REPRESENTATION_ITEM('')
SURFACE()
);
#3105=(
BOUNDED_SURFACE()
B_SPLINE_SURFACE(3,2,((#220102,#220103,#220104),(#220105,#220106,#220107),
(#220108,#220109,#220110),(#220111,#220112,#220113)),.UNSPECIFIED.,.F.,
 .F.,.F.)
B_SPLINE_SURFACE_WITH_KNOTS((4,4),(3,3),(-0.000102945165535282,0.00102945165511775),
(0.,1.00456220410723),.UNSPECIFIED.)
GEOMETRIC_REPRESENTATION_ITEM()
RATIONAL_B_SPLINE_SURFACE(((1.,0.99790768871298,1.00001909110229),(1.,0.999220691897535,
1.00000711072525),(1.,1.00001166705636,0.999999893545015),(1.,1.,1.)))
REPRESENTATION_ITEM('')
SURFACE()
);
#3106=(
BOUNDED_SURFACE()
B_SPLINE_SURFACE(3,2,((#220117,#220118,#220119),(#220120,#220121,#220122),
(#220123,#220124,#220125),(#220126,#220127,#220128)),.UNSPECIFIED.,.F.,
 .F.,.F.)
B_SPLINE_SURFACE_WITH_KNOTS((4,4),(3,3),(0.0105620870905992,0.0106719618085628),
(0.,1.),.UNSPECIFIED.)
GEOMETRIC_REPRESENTATION_ITEM()
RATIONAL_B_SPLINE_SURFACE(((1.,0.997703261465161,1.),(1.,0.997980295466883,
1.),(1.,0.998184609657418,1.),(1.,0.998260562486346,1.)))
REPRESENTATION_ITEM('')
SURFACE()
);
#3107=(
BOUNDED_SURFACE()
B_SPLINE_SURFACE(3,2,((#220134,#220135,#220136),(#220137,#220138,#220139),
(#220140,#220141,#220142),(#220143,#220144,#220145)),.UNSPECIFIED.,.F.,
 .F.,.F.)
B_SPLINE_SURFACE_WITH_KNOTS((4,4),(3,3),(0.0270627267990834,0.0348275700538468),
(0.,1.),.UNSPECIFIED.)
GEOMETRIC_REPRESENTATION_ITEM()
RATIONAL_B_SPLINE_SURFACE(((1.,0.959662285900572,1.),(1.,0.959827071897818,
1.),(1.,0.959976275192295,1.),(1.,0.960109658705296,1.)))
REPRESENTATION_ITEM('')
SURFACE()
);
#3108=(
BOUNDED_SURFACE()
B_SPLINE_SURFACE(3,2,((#220151,#220152,#220153),(#220154,#220155,#220156),
(#220157,#220158,#220159),(#220160,#220161,#220162),(#220163,#220164,#220165),
(#220166,#220167,#220168),(#220169,#220170,#220171),(#220172,#220173,#220174),
(#220175,#220176,#220177),(#220178,#220179,#220180)),.UNSPECIFIED.,.F.,
 .F.,.F.)
B_SPLINE_SURFACE_WITH_KNOTS((4,2,2,2,4),(3,3),(-8.76035355368288E-17,0.000261575538067988,
0.000523151076136064,0.00078472661420414,0.00104630215227222),(0.,1.),
 .UNSPECIFIED.)
GEOMETRIC_REPRESENTATION_ITEM()
RATIONAL_B_SPLINE_SURFACE(((1.,0.941539462223513,1.),(1.,0.942944078103613,
1.),(1.,0.944666632267826,1.),(1.,0.947704870094144,1.),(1.,0.949116332566215,
1.),(1.,0.951938364158571,1.),(1.,0.953364849054759,1.),(1.,0.956562808918851,
1.),(1.,0.958303880697236,1.),(1.,0.959662285866025,1.)))
REPRESENTATION_ITEM('')
SURFACE()
);
#3109=(
BOUNDED_SURFACE()
B_SPLINE_SURFACE(3,2,((#220318,#220319,#220320),(#220321,#220322,#220323),
(#220324,#220325,#220326),(#220327,#220328,#220329),(#220330,#220331,#220332),
(#220333,#220334,#220335),(#220336,#220337,#220338),(#220339,#220340,#220341),
(#220342,#220343,#220344),(#220345,#220346,#220347),(#220348,#220349,#220350),
(#220351,#220352,#220353),(#220354,#220355,#220356),(#220357,#220358,#220359),
(#220360,#220361,#220362),(#220363,#220364,#220365),(#220366,#220367,#220368),
(#220369,#220370,#220371),(#220372,#220373,#220374),(#220375,#220376,#220377),
(#220378,#220379,#220380),(#220381,#220382,#220383),(#220384,#220385,#220386),
(#220387,#220388,#220389),(#220390,#220391,#220392),(#220393,#220394,#220395)),
 .UNSPECIFIED.,.F.,.F.,.F.)
B_SPLINE_SURFACE_WITH_KNOTS((4,2,2,2,2,2,2,2,2,2,2,2,4),(3,3),(0.0232773420264243,
0.0238865203213561,0.0243167159675304,0.0247469116137046,0.0251771072598788,
0.025392205082966,0.0256073029060531,0.0260374985522273,0.0262525963753145,
0.0264676941984016,0.0265752431099451,0.0266827920214887,0.0270768724933326),
(-0.000622430556160899,1.),.UNSPECIFIED.)
GEOMETRIC_REPRESENTATION_ITEM()
RATIONAL_B_SPLINE_SURFACE(((1.00007022535184,0.94358780176874,1.),(1.00007345968059,
0.940989657513307,1.),(1.00007557765372,0.939288284476128,1.),(1.00007953800459,
0.936106924857717,1.),(1.00008135577751,0.93464670339122,1.),(1.00008485035292,
0.931839502350726,1.),(1.00008646656058,0.930541198756514,1.),(1.00008926890465,
0.928290068854851,1.),(1.00009055175433,0.927259552546139,1.),(1.00009272454497,
0.925514144470467,1.),(1.00009354896659,0.924851884544549,1.),(1.00009510634629,
0.923600837597642,1.),(1.00009571013816,0.923115810099967,1.),(1.00009732578087,
0.92181796032787,1.),(1.00009808691593,0.921206538657284,1.),(1.00009969877668,
0.919911726943257,1.),(1.00010036529178,0.919376313722562,1.),(1.00010163596213,
0.918355581096937,1.),(1.00010219331079,0.917907861542757,1.),(1.00010248992835,
0.917669587924958,1.),(1.00010253345844,0.917634620099449,1.),(1.00010269113762,
0.917507956025272,1.),(1.00010277791566,0.917438247014893,1.),(1.00010317584749,
0.917118587394104,1.),(1.00010346600792,0.916885500804008,1.),(1.00010310505887,
0.917175452062668,1.)))
REPRESENTATION_ITEM('')
SURFACE()
);
#3110=(
BOUNDED_SURFACE()
B_SPLINE_SURFACE(3,2,((#220594,#220595,#220596),(#220597,#220598,#220599),
(#220600,#220601,#220602),(#220603,#220604,#220605)),.UNSPECIFIED.,.F.,
 .F.,.F.)
B_SPLINE_SURFACE_WITH_KNOTS((4,4),(3,3),(0.0245397910410617,0.0252336582652646),
(0.,1.),.UNSPECIFIED.)
GEOMETRIC_REPRESENTATION_ITEM()
RATIONAL_B_SPLINE_SURFACE(((1.,0.91828031569264,1.),(1.,0.918191277007669,
1.),(1.,0.917795655860158,1.),(1.,0.917108339181228,1.)))
REPRESENTATION_ITEM('')
SURFACE()
);
#3111=(
BOUNDED_SURFACE()
B_SPLINE_SURFACE(3,2,((#220620,#220621,#220622),(#220623,#220624,#220625),
(#220626,#220627,#220628),(#220629,#220630,#220631)),.UNSPECIFIED.,.F.,
 .F.,.F.)
B_SPLINE_SURFACE_WITH_KNOTS((4,4),(3,3),(0.0408577781618264,0.0446742483522374),
(0.,1.),.UNSPECIFIED.)
GEOMETRIC_REPRESENTATION_ITEM()
RATIONAL_B_SPLINE_SURFACE(((1.,0.918280315692642,1.),(1.,0.919146142525415,
1.),(1.,0.920060572994544,1.),(1.,0.920885718130539,1.)))
REPRESENTATION_ITEM('')
SURFACE()
);
#3112=(
BOUNDED_SURFACE()
B_SPLINE_SURFACE(3,2,((#220649,#220650,#220651),(#220652,#220653,#220654),
(#220655,#220656,#220657),(#220658,#220659,#220660),(#220661,#220662,#220663),
(#220664,#220665,#220666),(#220667,#220668,#220669),(#220670,#220671,#220672),
(#220673,#220674,#220675),(#220676,#220677,#220678),(#220679,#220680,#220681),
(#220682,#220683,#220684),(#220685,#220686,#220687),(#220688,#220689,#220690),
(#220691,#220692,#220693),(#220694,#220695,#220696),(#220697,#220698,#220699),
(#220700,#220701,#220702),(#220703,#220704,#220705),(#220706,#220707,#220708),
(#220709,#220710,#220711),(#220712,#220713,#220714),(#220715,#220716,#220717),
(#220718,#220719,#220720),(#220721,#220722,#220723),(#220724,#220725,#220726),
(#220727,#220728,#220729),(#220730,#220731,#220732),(#220733,#220734,#220735),
(#220736,#220737,#220738),(#220739,#220740,#220741),(#220742,#220743,#220744),
(#220745,#220746,#220747),(#220748,#220749,#220750),(#220751,#220752,#220753),
(#220754,#220755,#220756),(#220757,#220758,#220759),(#220760,#220761,#220762),
(#220763,#220764,#220765),(#220766,#220767,#220768),(#220769,#220770,#220771),
(#220772,#220773,#220774),(#220775,#220776,#220777),(#220778,#220779,#220780),
(#220781,#220782,#220783),(#220784,#220785,#220786),(#220787,#220788,#220789),
(#220790,#220791,#220792),(#220793,#220794,#220795),(#220796,#220797,#220798),
(#220799,#220800,#220801),(#220802,#220803,#220804),(#220805,#220806,#220807),
(#220808,#220809,#220810),(#220811,#220812,#220813),(#220814,#220815,#220816),
(#220817,#220818,#220819),(#220820,#220821,#220822),(#220823,#220824,#220825),
(#220826,#220827,#220828),(#220829,#220830,#220831),(#220832,#220833,#220834)),
 .UNSPECIFIED.,.F.,.F.,.F.)
B_SPLINE_SURFACE_WITH_KNOTS((4,2,2,2,2,2,2,2,2,2,2,2,2,2,2,2,2,2,2,2,2,
2,2,2,2,2,2,2,2,2,4),(3,3),(8.67361737988404E-19,0.00422017278643856,0.00435205318601475,
0.00438502328590881,0.00441799338580286,0.00448393358559096,0.00474769438474337,
0.00527521598304819,0.00633025917965783,0.00844034557287711,0.0126605183593157,
0.0137155615559253,0.0137815017557134,0.0138474419555015,0.0139793223550777,
0.0142430831542301,0.0147706047525349,0.0168806911457542,0.0211008639321928,
0.0221559071288024,0.0224196679279548,0.0224856081277429,0.0225185782276369,
0.022551548327531,0.0226834287271072,0.0232109503254121,0.0253210367186313,
0.0274311231118506,0.0284861663084603,0.0295412095050698,0.0337613822915084),
(0.,1.00028876552603),.UNSPECIFIED.)
GEOMETRIC_REPRESENTATION_ITEM()
RATIONAL_B_SPLINE_SURFACE(((1.,0.959354208545287,1.0000234742067),(1.,0.959337470736254,
1.0000234838733),(1.,0.958512445104999,1.00002396035123),(1.,0.95694732571469,
1.00002486425627),(1.,0.956899194384682,1.00002489205361),(1.,0.956838139436707,
1.00002492731474),(1.,0.956862400414095,1.00002491330327),(1.,0.956887484855878,
1.00002489881623),(1.,0.956899999499305,1.00002489158863),(1.,0.956937460592084,
1.00002486995369),(1.,0.956962324203891,1.00002485559418),(1.,0.957086088627733,
1.00002478411638),(1.,0.957183328458195,1.00002472795736),(1.,0.957469681464417,
1.00002456257961),(1.,0.957653426914545,1.0000244564609),(1.,0.958182822841225,
1.00002415071832),(1.,0.958506816204993,1.00002396360209),(1.,0.959387851983579,
1.00002345477657),(1.,0.959853733183088,1.00002318571571),(1.,0.960889943146176,
1.00002258727228),(1.,0.961106229913013,1.00002246235996),(1.,0.960689094558209,
1.00002270326858),(1.,0.960570529441095,1.00002277174361),(1.,0.960405498729637,
1.00002286705397),(1.,0.960395647596876,1.00002287274331),(1.,0.960375657763087,
1.00002288428806),(1.,0.960390364940156,1.00002287579421),(1.,0.960411396327207,
1.00002286364793),(1.,0.960424477373958,1.00002285609322),(1.,0.960460930383527,
1.00002283504047),(1.,0.960481512894489,1.00002282315343),(1.,0.960532312012284,
1.00002279381537),(1.,0.960551589312845,1.00002278268213),(1.,0.960577225424367,
1.00002276787648),(1.,0.960369658550149,1.00002288775279),(1.,0.959139560764285,
1.00002359817246),(1.,0.957494299277627,1.00002454836206),(1.,0.954680773867681,
1.00002617326035),(1.,0.954080291282266,1.00002652005769),(1.,0.953286564436122,
1.00002697845959),(1.,0.95312561937944,1.00002707141035),(1.,0.952921674070366,
1.0000271891951),(1.,0.952880746778416,1.00002721283189),(1.,0.952819148132629,
1.00002724840702),(1.,0.952798580632323,1.00002726028539),(1.,0.952757376329878,
1.00002728408215),(1.,0.952703868180498,1.00002731498477),(1.,0.952803106657217,
1.00002725767147),(1.,0.952882131942925,1.00002721203191),(1.,0.953275429419064,
1.0000269848904),(1.,0.953584216264606,1.00002680655641),(1.,0.955098740501949,
1.00002593187164),(1.,0.956216687617054,1.00002528622246),(1.,0.958254587609343,
1.00002410927194),(1.,0.959174978159034,1.00002357771781),(1.,0.960388157713114,
1.00002287706895),(1.,0.960764502584019,1.0000226597181),(1.,0.961455799248518,
1.00002226047281),(1.,0.961771684206244,1.00002207803944),(1.,0.963168690580858,
1.00002127122488),(1.,0.963699001724993,1.00002096495372),(1.,0.963430051350225,
1.00002112028092)))
REPRESENTATION_ITEM('')
SURFACE()
);
#3113=(
BOUNDED_SURFACE()
B_SPLINE_SURFACE(3,2,((#221269,#221270,#221271),(#221272,#221273,#221274),
(#221275,#221276,#221277),(#221278,#221279,#221280),(#221281,#221282,#221283),
(#221284,#221285,#221286)),.UNSPECIFIED.,.F.,.F.,.F.)
B_SPLINE_SURFACE_WITH_KNOTS((4,2,4),(3,3),(-3.10081821330854E-17,0.000547593654446629,
0.00109518730889329),(0.,1.),.UNSPECIFIED.)
GEOMETRIC_REPRESENTATION_ITEM()
RATIONAL_B_SPLINE_SURFACE(((1.,0.994860301689857,1.),(1.,0.996487472179808,
1.),(1.,0.997781945631374,1.),(1.,0.999546172218064,1.),(1.,1.00000726363599,
1.),(1.,1.,1.)))
REPRESENTATION_ITEM('')
SURFACE()
);
#3114=(
BOUNDED_SURFACE()
B_SPLINE_SURFACE(3,2,((#221317,#221318,#221319),(#221320,#221321,#221322),
(#221323,#221324,#221325),(#221326,#221327,#221328)),.UNSPECIFIED.,.F.,
 .F.,.F.)
B_SPLINE_SURFACE_WITH_KNOTS((4,4),(3,3),(0.0169795328233838,0.0259332885708231),
(0.,1.),.UNSPECIFIED.)
GEOMETRIC_REPRESENTATION_ITEM()
RATIONAL_B_SPLINE_SURFACE(((1.,0.957225253293536,1.),(1.,0.957330219064779,
1.),(1.,0.957420194105006,1.),(1.,0.95749691742527,1.)))
REPRESENTATION_ITEM('')
SURFACE()
);
#3115=(
BOUNDED_SURFACE()
B_SPLINE_SURFACE(3,2,((#221345,#221346,#221347),(#221348,#221349,#221350),
(#221351,#221352,#221353),(#221354,#221355,#221356)),.UNSPECIFIED.,.F.,
 .F.,.F.)
B_SPLINE_SURFACE_WITH_KNOTS((4,4),(3,3),(0.00708837036243835,0.00717746991701786),
(0.,1.),.UNSPECIFIED.)
GEOMETRIC_REPRESENTATION_ITEM()
RATIONAL_B_SPLINE_SURFACE(((1.,0.994244619571122,1.),(1.,0.99451521711556,
1.),(1.,0.994723691418652,1.),(1.,0.994860301689858,1.)))
REPRESENTATION_ITEM('')
SURFACE()
);
#3116=(
BOUNDED_SURFACE()
B_SPLINE_SURFACE(3,2,((#221366,#221367,#221368),(#221369,#221370,#221371),
(#221372,#221373,#221374),(#221375,#221376,#221377),(#221378,#221379,#221380),
(#221381,#221382,#221383),(#221384,#221385,#221386),(#221387,#221388,#221389),
(#221390,#221391,#221392),(#221393,#221394,#221395)),.UNSPECIFIED.,.F.,
 .F.,.F.)
B_SPLINE_SURFACE_WITH_KNOTS((4,2,2,2,4),(3,3),(-3.64042682515704E-5,0.000213802025234883,
0.000427604050469766,0.000641406075704648,0.000891612369191551),(-3.64042682525183E-5,
1.),.UNSPECIFIED.)
GEOMETRIC_REPRESENTATION_ITEM()
RATIONAL_B_SPLINE_SURFACE(((1.00000395581295,0.945668280974287,1.),(1.00000388505117,
0.946640169426575,1.),(1.00000379315429,0.947902341199865,1.),(1.00000364163364,
0.949983424830958,1.),(1.00000357606162,0.950884033719279,1.),(1.00000344606386,
0.95266950796714,1.),(1.00000338057312,0.953569000549728,1.),(1.00000323211214,
0.955608060593106,1.),(1.0000031500215,0.956735547071876,1.),(1.00000308511796,
0.957626974709355,1.)))
REPRESENTATION_ITEM('')
SURFACE()
);
#3117=(
BOUNDED_SURFACE()
B_SPLINE_SURFACE(3,2,((#221439,#221440,#221441),(#221442,#221443,#221444),
(#221445,#221446,#221447),(#221448,#221449,#221450),(#221451,#221452,#221453),
(#221454,#221455,#221456),(#221457,#221458,#221459),(#221460,#221461,#221462),
(#221463,#221464,#221465),(#221466,#221467,#221468),(#221469,#221470,#221471),
(#221472,#221473,#221474),(#221475,#221476,#221477),(#221478,#221479,#221480),
(#221481,#221482,#221483),(#221484,#221485,#221486),(#221487,#221488,#221489),
(#221490,#221491,#221492),(#221493,#221494,#221495),(#221496,#221497,#221498)),
 .UNSPECIFIED.,.F.,.F.,.F.)
B_SPLINE_SURFACE_WITH_KNOTS((4,2,2,2,2,2,2,2,2,4),(3,3),(0.0241832201811484,
0.0245055239061063,0.0248218005295632,0.02513807715302,0.0252962154647484,
0.0254543537764769,0.0257706303999337,0.0260869070233905,0.0264031836468474,
0.0267254873718053),(-6.02710150104311E-6,1.),.UNSPECIFIED.)
GEOMETRIC_REPRESENTATION_ITEM()
RATIONAL_B_SPLINE_SURFACE(((1.00000084427113,0.929960435071147,1.),(1.00000084156585,
0.930184862090941,1.),(1.00000083766746,0.930508267100976,1.),(1.00000083178679,
0.930996119039314,1.),(1.00000082192711,0.931814064338866,1.),(1.00000080692986,
0.933058215433481,1.),(1.00000080145663,0.933512266741312,1.),(1.00000079098237,
0.934381197300965,1.),(1.00000078716924,0.934697529544281,1.),(1.00000077788725,
0.935467549988599,1.),(1.00000077240012,0.935922755061344,1.),(1.00000075833733,
0.937089384822285,1.),(1.00000075011112,0.937771819638465,1.),(1.00000073260548,
0.939224063056665,1.),(1.00000072284102,0.940034109274095,1.),(1.00000070143123,
0.941810235649062,1.),(1.00000069002421,0.942756546224953,1.),(1.00000066943902,
0.944464265082494,1.),(1.00000066003637,0.945244295905894,1.),(1.00000064896667,
0.946162623330347,1.)))
REPRESENTATION_ITEM('')
SURFACE()
);
#3118=(
BOUNDED_SURFACE()
B_SPLINE_SURFACE(3,2,((#221813,#221814,#221815),(#221816,#221817,#221818),
(#221819,#221820,#221821),(#221822,#221823,#221824)),.UNSPECIFIED.,.F.,
 .F.,.F.)
B_SPLINE_SURFACE_WITH_KNOTS((4,4),(3,3),(0.0252170418335343,0.0258229913570787),
(0.,1.),.UNSPECIFIED.)
GEOMETRIC_REPRESENTATION_ITEM()
RATIONAL_B_SPLINE_SURFACE(((1.,0.930836001346604,1.),(1.,0.930792329315189,
1.),(1.,0.93050066650605,1.),(1.,0.929973550212784,1.)))
REPRESENTATION_ITEM('')
SURFACE()
);
#3119=(
BOUNDED_SURFACE()
B_SPLINE_SURFACE(3,2,((#221842,#221843,#221844),(#221845,#221846,#221847),
(#221848,#221849,#221850),(#221851,#221852,#221853)),.UNSPECIFIED.,.F.,
 .F.,.F.)
B_SPLINE_SURFACE_WITH_KNOTS((4,4),(3,3),(0.0413352581734094,0.0453130011481359),
(0.,1.),.UNSPECIFIED.)
GEOMETRIC_REPRESENTATION_ITEM()
RATIONAL_B_SPLINE_SURFACE(((1.,0.932166688794147,1.),(1.,0.931835585737477,
1.),(1.,0.931353352247319,1.),(1.,0.930836001346601,1.)))
REPRESENTATION_ITEM('')
SURFACE()
);
#3120=(
BOUNDED_SURFACE()
B_SPLINE_SURFACE(3,2,((#221886,#221887,#221888),(#221889,#221890,#221891),
(#221892,#221893,#221894),(#221895,#221896,#221897),(#221898,#221899,#221900),
(#221901,#221902,#221903)),.UNSPECIFIED.,.F.,.F.,.F.)
B_SPLINE_SURFACE_WITH_KNOTS((4,2,4),(3,3),(0.0166588946789198,0.0292596031542503,
0.0418603116295807),(0.,1.),.UNSPECIFIED.)
GEOMETRIC_REPRESENTATION_ITEM()
RATIONAL_B_SPLINE_SURFACE(((1.,0.997703261465172,1.),(1.,0.997094448547928,
1.),(1.,0.996295120040444,1.),(1.,0.994021377933446,1.),(1.,0.992546012713842,
1.),(1.,0.990544312570191,1.)))
REPRESENTATION_ITEM('')
SURFACE()
);
#3121=(
BOUNDED_SURFACE()
B_SPLINE_SURFACE(3,2,((#221942,#221943,#221944),(#221945,#221946,#221947),
(#221948,#221949,#221950),(#221951,#221952,#221953)),.UNSPECIFIED.,.F.,
 .F.,.F.)
B_SPLINE_SURFACE_WITH_KNOTS((4,4),(3,3),(0.0204076478587134,0.0466615476412126),
(0.,1.),.UNSPECIFIED.)
GEOMETRIC_REPRESENTATION_ITEM()
RATIONAL_B_SPLINE_SURFACE(((1.,0.990204100637796,1.),(1.,0.991176825451801,
1.),(1.,0.991726788386978,1.),(1.,0.99216019396246,1.)))
REPRESENTATION_ITEM('')
SURFACE()
);
#3122=(
BOUNDED_SURFACE()
B_SPLINE_SURFACE(3,2,((#222037,#222038,#222039),(#222040,#222041,#222042),
(#222043,#222044,#222045),(#222046,#222047,#222048)),.UNSPECIFIED.,.F.,
 .F.,.F.)
B_SPLINE_SURFACE_WITH_KNOTS((4,4),(3,3),(0.0511685324324545,0.0760142482873155),
(0.,1.),.UNSPECIFIED.)
GEOMETRIC_REPRESENTATION_ITEM()
RATIONAL_B_SPLINE_SURFACE(((1.,0.992981223849425,1.),(1.,0.992578629089082,
1.),(1.,0.992069952154663,1.),(1.,0.99114034013539,1.)))
REPRESENTATION_ITEM('')
SURFACE()
);
#3123=(
BOUNDED_SURFACE()
B_SPLINE_SURFACE(3,2,((#222119,#222120,#222121),(#222122,#222123,#222124),
(#222125,#222126,#222127),(#222128,#222129,#222130),(#222131,#222132,#222133),
(#222134,#222135,#222136)),.UNSPECIFIED.,.F.,.F.,.F.)
B_SPLINE_SURFACE_WITH_KNOTS((4,2,4),(3,3),(0.0166253761100813,0.0283648343214891,
0.0402199721685829),(-0.000115679635685861,1.),.UNSPECIFIED.)
GEOMETRIC_REPRESENTATION_ITEM()
RATIONAL_B_SPLINE_SURFACE(((1.00000115641936,0.995001629476687,1.),(1.00000110101721,
0.995241093190461,1.),(1.00000110174919,0.995237929375604,1.),(1.00000117166435,
0.994935736348517,1.),(1.00000124188212,0.994632235347241,1.),(1.00000133441707,
0.994232273186486,1.)))
REPRESENTATION_ITEM('')
SURFACE()
);
#3124=(
BOUNDED_SURFACE()
B_SPLINE_SURFACE(3,2,((#235472,#235473,#235474),(#235475,#235476,#235477),
(#235478,#235479,#235480),(#235481,#235482,#235483),(#235484,#235485,#235486),
(#235487,#235488,#235489),(#235490,#235491,#235492),(#235493,#235494,#235495),
(#235496,#235497,#235498),(#235499,#235500,#235501)),.UNSPECIFIED.,.F.,
 .F.,.F.)
B_SPLINE_SURFACE_WITH_KNOTS((4,2,2,2,4),(3,3),(4.71238898038469,5.10508806208341,
5.49778714378214,5.89048622548086,6.28318530717959),(0.,1.),
 .UNSPECIFIED.)
GEOMETRIC_REPRESENTATION_ITEM()
RATIONAL_B_SPLINE_SURFACE(((1.,0.707106781186554,1.),(1.,0.7340577581143,
1.),(1.,0.759389607022087,1.),(1.,0.804397146462884,1.),(1.,0.824065680681991,
1.),(1.,0.856126418973412,1.),(1.,0.868523258375879,1.),(1.,0.885147394261533,
1.),(1.,0.889385678509254,1.),(1.,0.889376480585547,1.)))
REPRESENTATION_ITEM('')
SURFACE()
);
#3125=(
BOUNDED_SURFACE()
B_SPLINE_SURFACE(3,2,((#235559,#235560,#235561),(#235562,#235563,#235564),
(#235565,#235566,#235567),(#235568,#235569,#235570),(#235571,#235572,#235573),
(#235574,#235575,#235576),(#235577,#235578,#235579),(#235580,#235581,#235582),
(#235583,#235584,#235585),(#235586,#235587,#235588)),.UNSPECIFIED.,.F.,
 .F.,.F.)
B_SPLINE_SURFACE_WITH_KNOTS((4,2,2,2,4),(3,3),(4.71238898038469,5.10508806208341,
5.49778714378214,5.89048622548086,6.28318530717959),(0.,1.),
 .UNSPECIFIED.)
GEOMETRIC_REPRESENTATION_ITEM()
RATIONAL_B_SPLINE_SURFACE(((1.,0.707106781186555,1.),(1.,0.7340577581143,
1.),(1.,0.759389607022087,1.),(1.,0.804397146462884,1.),(1.,0.82406568068196,
1.),(1.,0.856126418973443,1.),(1.,0.868523258375851,1.),(1.,0.885147394261561,
1.),(1.,0.889385678509233,1.),(1.,0.889376480585547,1.)))
REPRESENTATION_ITEM('')
SURFACE()
);
#3126=(
BOUNDED_SURFACE()
B_SPLINE_SURFACE(1,2,((#244439,#244440,#244441,#244442,#244443,#244444,
#244445,#244446,#244447,#244448,#244449,#244450,#244451,#244452,#244453,
#244454,#244455,#244456,#244457,#244458,#244459,#244460,#244461,#244462,
#244463,#244464,#244465,#244466,#244467,#244468,#244469,#244470,#244471,
#244472,#244473,#244474,#244475,#244476,#244477,#244478,#244479,#244480,
#244481,#244482,#244483,#244484,#244485,#244486,#244487,#244488,#244489,
#244490,#244491,#244492,#244493,#244494,#244495,#244496,#244497,#244498,
#244499,#244500,#244501,#244502,#244503,#244504,#244505,#244506,#244507,
#244508,#244509,#244510,#244511,#244512,#244513,#244514,#244515,#244516,
#244517,#244518,#244519,#244520,#244521,#244522,#244523,#244524,#244525,
#244526,#244527,#244528,#244529,#244530,#244531,#244532,#244533,#244534,
#244535,#244536,#244537,#244538,#244539,#244540,#244541,#244542,#244543,
#244544,#244545,#244546,#244547,#244548,#244549,#244550,#244551,#244552,
#244553,#244554,#244555,#244556,#244557,#244558,#244559,#244560,#244561,
#244562,#244563,#244564,#244565,#244566,#244567,#244568,#244569,#244570,
#244571,#244572,#244573,#244574,#244575,#244576,#244577,#244578,#244579,
#244580,#244581,#244582,#244583,#244584,#244585,#244586,#244587,#244588,
#244589,#244590,#244591,#244592,#244593,#244594,#244595,#244596,#244597,
#244598,#244599,#244600,#244601,#244602,#244603,#244604,#244605,#244606,
#244607,#244608,#244609,#244610,#244611,#244612,#244613,#244614,#244615,
#244616,#244617,#244618,#244619,#244620,#244621,#244622,#244623,#244624,
#244625,#244626,#244627,#244628,#244629,#244630,#244631,#244632,#244633,
#244634,#244635,#244636,#244637,#244638,#244639,#244640,#244641,#244642,
#244643,#244644,#244645,#244646,#244647,#244648,#244649,#244650,#244651,
#244652,#244653,#244654,#244655,#244656,#244657,#244658,#244659,#244660,
#244661,#244662,#244663,#244664,#244665,#244666,#244667,#244668,#244669,
#244670,#244671,#244672,#244673,#244674,#244675,#244676,#244677,#244678,
#244679,#244680,#244681,#244682,#244683,#244684,#244685,#244686,#244687,
#244688,#244689,#244690,#244691,#244692,#244693,#244694,#244695,#244696,
#244697,#244698,#244699,#244700,#244701,#244702,#244703,#244704,#244705,
#244706,#244707,#244708,#244709,#244710,#244711,#244712,#244713,#244714,
#244715),(#244716,#244717,#244718,#244719,#244720,#244721,#244722,#244723,
#244724,#244725,#244726,#244727,#244728,#244729,#244730,#244731,#244732,
#244733,#244734,#244735,#244736,#244737,#244738,#244739,#244740,#244741,
#244742,#244743,#244744,#244745,#244746,#244747,#244748,#244749,#244750,
#244751,#244752,#244753,#244754,#244755,#244756,#244757,#244758,#244759,
#244760,#244761,#244762,#244763,#244764,#244765,#244766,#244767,#244768,
#244769,#244770,#244771,#244772,#244773,#244774,#244775,#244776,#244777,
#244778,#244779,#244780,#244781,#244782,#244783,#244784,#244785,#244786,
#244787,#244788,#244789,#244790,#244791,#244792,#244793,#244794,#244795,
#244796,#244797,#244798,#244799,#244800,#244801,#244802,#244803,#244804,
#244805,#244806,#244807,#244808,#244809,#244810,#244811,#244812,#244813,
#244814,#244815,#244816,#244817,#244818,#244819,#244820,#244821,#244822,
#244823,#244824,#244825,#244826,#244827,#244828,#244829,#244830,#244831,
#244832,#244833,#244834,#244835,#244836,#244837,#244838,#244839,#244840,
#244841,#244842,#244843,#244844,#244845,#244846,#244847,#244848,#244849,
#244850,#244851,#244852,#244853,#244854,#244855,#244856,#244857,#244858,
#244859,#244860,#244861,#244862,#244863,#244864,#244865,#244866,#244867,
#244868,#244869,#244870,#244871,#244872,#244873,#244874,#244875,#244876,
#244877,#244878,#244879,#244880,#244881,#244882,#244883,#244884,#244885,
#244886,#244887,#244888,#244889,#244890,#244891,#244892,#244893,#244894,
#244895,#244896,#244897,#244898,#244899,#244900,#244901,#244902,#244903,
#244904,#244905,#244906,#244907,#244908,#244909,#244910,#244911,#244912,
#244913,#244914,#244915,#244916,#244917,#244918,#244919,#244920,#244921,
#244922,#244923,#244924,#244925,#244926,#244927,#244928,#244929,#244930,
#244931,#244932,#244933,#244934,#244935,#244936,#244937,#244938,#244939,
#244940,#244941,#244942,#244943,#244944,#244945,#244946,#244947,#244948,
#244949,#244950,#244951,#244952,#244953,#244954,#244955,#244956,#244957,
#244958,#244959,#244960,#244961,#244962,#244963,#244964,#244965,#244966,
#244967,#244968,#244969,#244970,#244971,#244972,#244973,#244974,#244975,
#244976,#244977,#244978,#244979,#244980,#244981,#244982,#244983,#244984,
#244985,#244986,#244987,#244988,#244989,#244990,#244991,#244992)),
 .UNSPECIFIED.,.F.,.F.,.F.)
B_SPLINE_SURFACE_WITH_KNOTS((2,2),(3,2,2,2,2,2,2,2,2,2,2,2,2,2,2,2,2,2,
2,2,2,2,2,2,2,2,2,2,2,2,2,2,2,2,2,2,2,2,2,2,2,2,2,2,2,2,2,2,2,2,2,2,2,2,
2,2,2,2,2,2,2,2,2,2,2,2,2,2,2,2,2,2,2,2,2,2,2,2,2,2,2,2,2,2,2,2,2,2,2,2,
2,2,2,2,2,2,2,2,2,2,2,2,2,2,2,2,2,2,2,2,2,2,2,2,2,2,2,2,2,2,2,2,2,2,2,2,
2,2,2,2,2,2,2,2,2,2,2,2,3),(0.,1.),(0.,0.0072463768115942,0.0144927536231884,
0.0217391304347826,0.0289855072463768,0.036231884057971,0.0434782608695652,
0.0507246376811594,0.0579710144927536,0.0652173913043478,0.072463768115942,
0.0797101449275362,0.0869565217391304,0.0942028985507246,0.101449275362319,
0.108695652173913,0.115942028985507,0.123188405797101,0.130434782608696,
0.13768115942029,0.144927536231884,0.152173913043478,0.159420289855073,
0.166666666666667,0.173913043478261,0.181159420289855,0.18840579710145,
0.195652173913044,0.202898550724637,0.210144927536232,0.217391304347826,
0.224637681159421,0.231884057971014,0.239130434782609,0.246376811594203,
0.253623188405797,0.260869565217392,0.268115942028985,0.275362318840579,
0.282608695652174,0.289855072463768,0.297101449275363,0.304347826086956,
0.31159420289855,0.318840579710145,0.326086956521739,0.333333333333334,
0.340579710144927,0.347826086956521,0.355072463768116,0.36231884057971,
0.369565217391304,0.376811594202899,0.384057971014493,0.391304347826087,
0.398550724637681,0.405797101449275,0.41304347826087,0.420289855072463,
0.427536231884058,0.434782608695652,0.442028985507247,0.449275362318841,
0.456521739130435,0.463768115942029,0.471014492753623,0.478260869565218,
0.485507246376812,0.492753623188406,0.5,0.507246376811594,0.514492753623188,
0.521739130434783,0.528985507246377,0.536231884057971,0.543478260869565,
0.550724637681159,0.557971014492754,0.565217391304348,0.572463768115942,
0.579710144927536,0.586956521739131,0.594202898550725,0.601449275362319,
0.608695652173913,0.615942028985507,0.623188405797101,0.630434782608696,
0.63768115942029,0.644927536231884,0.652173913043478,0.659420289855073,
0.666666666666667,0.673913043478261,0.681159420289855,0.688405797101449,
0.695652173913044,0.702898550724638,0.710144927536232,0.717391304347826,
0.72463768115942,0.731884057971015,0.739130434782609,0.746376811594203,
0.753623188405797,0.760869565217391,0.768115942028986,0.77536231884058,
0.782608695652174,0.789855072463768,0.797101449275362,0.804347826086956,
0.811594202898551,0.818840579710145,0.826086956521739,0.833333333333333,
0.840579710144928,0.847826086956522,0.855072463768116,0.86231884057971,
0.869565217391304,0.876811594202899,0.884057971014493,0.891304347826087,
0.898550724637681,0.905797101449275,0.91304347826087,0.920289855072464,
0.927536231884058,0.934782608695652,0.942028985507246,0.94927536231884,
0.956521739130435,0.963768115942029,0.971014492753623,0.978260869565217,
0.985507246376812,0.992753623188406,0.993818585798284),.UNSPECIFIED.)
GEOMETRIC_REPRESENTATION_ITEM()
RATIONAL_B_SPLINE_SURFACE(((1.,0.866025403784439,1.,0.866025403784439,1.,
0.866025403784439,1.,0.866025403784439,1.,0.866025403784439,1.,0.866025403784439,
1.,0.866025403784439,1.,0.866025403784439,1.,0.866025403784439,1.,0.866025403784439,
1.,0.866025403784439,1.,0.866025403784439,1.,0.866025403784439,1.,0.866025403784439,
1.,0.866025403784439,1.,0.866025403784439,1.,0.866025403784439,1.,0.866025403784439,
1.,0.866025403784439,1.,0.866025403784439,1.,0.866025403784439,1.,0.866025403784439,
1.,0.866025403784439,1.,0.866025403784439,1.,0.866025403784439,1.,0.866025403784439,
1.,0.866025403784439,1.,0.866025403784439,1.,0.866025403784439,1.,0.866025403784439,
1.,0.866025403784439,1.,0.866025403784439,1.,0.866025403784439,1.,0.866025403784439,
1.,0.866025403784439,1.,0.866025403784439,1.,0.866025403784439,1.,0.866025403784439,
1.,0.866025403784439,1.,0.866025403784439,1.,0.866025403784439,1.,0.866025403784439,
1.,0.866025403784439,1.,0.866025403784439,1.,0.866025403784439,1.,0.866025403784439,
1.,0.866025403784439,1.,0.866025403784439,1.,0.866025403784439,1.,0.866025403784439,
1.,0.866025403784439,1.,0.866025403784439,1.,0.866025403784439,1.,0.866025403784439,
1.,0.866025403784439,1.,0.866025403784439,1.,0.866025403784439,1.,0.866025403784439,
1.,0.866025403784439,1.,0.866025403784439,1.,0.866025403784439,1.,0.866025403784439,
1.,0.866025403784439,1.,0.866025403784439,1.,0.866025403784439,1.,0.866025403784439,
1.,0.866025403784439,1.,0.866025403784439,1.,0.866025403784439,1.,0.866025403784439,
1.,0.866025403784439,1.,0.866025403784439,1.,0.866025403784439,1.,0.866025403784439,
1.,0.866025403784439,1.,0.866025403784439,1.,0.866025403784439,1.,0.866025403784439,
1.,0.866025403784439,1.,0.866025403784439,1.,0.866025403784439,1.,0.866025403784439,
1.,0.866025403784439,1.,0.866025403784439,1.,0.866025403784439,1.,0.866025403784439,
1.,0.866025403784439,1.,0.866025403784439,1.,0.866025403784439,1.,0.866025403784439,
1.,0.866025403784439,1.,0.866025403784439,1.,0.866025403784439,1.,0.866025403784439,
1.,0.866025403784439,1.,0.866025403784439,1.,0.866025403784439,1.,0.866025403784439,
1.,0.866025403784439,1.,0.866025403784439,1.,0.866025403784439,1.,0.866025403784439,
1.,0.866025403784439,1.,0.866025403784439,1.,0.866025403784439,1.,0.866025403784439,
1.,0.866025403784439,1.,0.866025403784439,1.,0.866025403784439,1.,0.866025403784439,
1.,0.866025403784439,1.,0.866025403784439,1.,0.866025403784439,1.,0.866025403784439,
1.,0.866025403784439,1.,0.866025403784439,1.,0.866025403784439,1.,0.866025403784439,
1.,0.866025403784439,1.,0.866025403784439,1.,0.866025403784439,1.,0.866025403784439,
1.,0.866025403784439,1.,0.866025403784439,1.,0.866025403784439,1.,0.866025403784439,
1.,0.866025403784439,1.,0.866025403784439,1.,0.866025403784439,1.,0.866025403784439,
1.,0.866025403784439,1.,0.866025403784439,1.,0.866025403784439,1.,0.866025403784439,
1.,0.866025403784439,1.,0.866025403784439,1.,0.866025403784439,1.,0.98031044488126,
0.966408234404338),(1.,0.866025403784439,1.,0.866025403784439,1.,0.866025403784439,
1.,0.866025403784439,1.,0.866025403784439,1.,0.866025403784439,1.,0.866025403784439,
1.,0.866025403784439,1.,0.866025403784439,1.,0.866025403784439,1.,0.866025403784439,
1.,0.866025403784439,1.,0.866025403784439,1.,0.866025403784439,1.,0.866025403784439,
1.,0.866025403784439,1.,0.866025403784439,1.,0.866025403784439,1.,0.866025403784439,
1.,0.866025403784439,1.,0.866025403784439,1.,0.866025403784439,1.,0.866025403784439,
1.,0.866025403784439,1.,0.866025403784439,1.,0.866025403784439,1.,0.866025403784439,
1.,0.866025403784439,1.,0.866025403784439,1.,0.866025403784439,1.,0.866025403784439,
1.,0.866025403784439,1.,0.866025403784439,1.,0.866025403784439,1.,0.866025403784439,
1.,0.866025403784439,1.,0.866025403784439,1.,0.866025403784439,1.,0.866025403784439,
1.,0.866025403784439,1.,0.866025403784439,1.,0.866025403784439,1.,0.866025403784439,
1.,0.866025403784439,1.,0.866025403784439,1.,0.866025403784439,1.,0.866025403784439,
1.,0.866025403784439,1.,0.866025403784439,1.,0.866025403784439,1.,0.866025403784439,
1.,0.866025403784439,1.,0.866025403784439,1.,0.866025403784439,1.,0.866025403784439,
1.,0.866025403784439,1.,0.866025403784439,1.,0.866025403784439,1.,0.866025403784439,
1.,0.866025403784439,1.,0.866025403784439,1.,0.866025403784439,1.,0.866025403784439,
1.,0.866025403784439,1.,0.866025403784439,1.,0.866025403784439,1.,0.866025403784439,
1.,0.866025403784439,1.,0.866025403784439,1.,0.866025403784439,1.,0.866025403784439,
1.,0.866025403784439,1.,0.866025403784439,1.,0.866025403784439,1.,0.866025403784439,
1.,0.866025403784439,1.,0.866025403784439,1.,0.866025403784439,1.,0.866025403784439,
1.,0.866025403784439,1.,0.866025403784439,1.,0.866025403784439,1.,0.866025403784439,
1.,0.866025403784439,1.,0.866025403784439,1.,0.866025403784439,1.,0.866025403784439,
1.,0.866025403784439,1.,0.866025403784439,1.,0.866025403784439,1.,0.866025403784439,
1.,0.866025403784439,1.,0.866025403784439,1.,0.866025403784439,1.,0.866025403784439,
1.,0.866025403784439,1.,0.866025403784439,1.,0.866025403784439,1.,0.866025403784439,
1.,0.866025403784439,1.,0.866025403784439,1.,0.866025403784439,1.,0.866025403784439,
1.,0.866025403784439,1.,0.866025403784439,1.,0.866025403784439,1.,0.866025403784439,
1.,0.866025403784439,1.,0.866025403784439,1.,0.866025403784439,1.,0.866025403784439,
1.,0.866025403784439,1.,0.866025403784439,1.,0.866025403784439,1.,0.866025403784439,
1.,0.866025403784439,1.,0.866025403784439,1.,0.866025403784439,1.,0.866025403784439,
1.,0.866025403784439,1.,0.866025403784439,1.,0.866025403784439,1.,0.866025403784439,
1.,0.866025403784439,1.,0.866025403784439,1.,0.866025403784439,1.,0.866025403784439,
1.,0.866025403784439,1.,0.866025403784439,1.,0.866025403784439,1.,0.866025403784439,
1.,0.866025403784439,1.,0.866025403784439,1.,0.866025403784439,1.,0.866025403784439,
1.,0.866025403784439,1.,0.866025403784439,1.,0.98031044488126,0.966408234404338)))
REPRESENTATION_ITEM('')
SURFACE()
);
#3127=(
BOUNDED_SURFACE()
B_SPLINE_SURFACE(1,2,((#245436,#245437,#245438,#245439,#245440,#245441,
#245442,#245443,#245444,#245445,#245446,#245447,#245448,#245449,#245450,
#245451,#245452,#245453,#245454,#245455,#245456,#245457,#245458,#245459,
#245460,#245461,#245462,#245463,#245464,#245465,#245466,#245467,#245468,
#245469,#245470,#245471,#245472,#245473,#245474,#245475,#245476,#245477,
#245478,#245479,#245480,#245481,#245482,#245483,#245484,#245485,#245486,
#245487,#245488,#245489,#245490,#245491,#245492,#245493,#245494,#245495,
#245496,#245497,#245498,#245499,#245500,#245501,#245502,#245503,#245504,
#245505,#245506,#245507,#245508,#245509,#245510,#245511,#245512,#245513,
#245514,#245515,#245516,#245517,#245518,#245519,#245520,#245521,#245522,
#245523,#245524,#245525,#245526,#245527,#245528,#245529,#245530,#245531,
#245532,#245533,#245534,#245535,#245536,#245537,#245538,#245539,#245540,
#245541,#245542,#245543,#245544,#245545,#245546,#245547,#245548,#245549,
#245550,#245551,#245552,#245553,#245554,#245555,#245556,#245557,#245558,
#245559,#245560,#245561,#245562,#245563,#245564,#245565,#245566,#245567,
#245568,#245569,#245570,#245571,#245572,#245573,#245574,#245575,#245576,
#245577,#245578,#245579,#245580,#245581,#245582,#245583,#245584,#245585,
#245586,#245587,#245588,#245589,#245590,#245591,#245592,#245593,#245594,
#245595,#245596,#245597,#245598,#245599,#245600,#245601,#245602,#245603,
#245604,#245605,#245606,#245607,#245608,#245609,#245610,#245611,#245612,
#245613,#245614,#245615,#245616,#245617,#245618,#245619,#245620,#245621,
#245622,#245623,#245624,#245625,#245626,#245627,#245628,#245629,#245630,
#245631,#245632,#245633,#245634,#245635,#245636,#245637,#245638,#245639,
#245640,#245641,#245642,#245643,#245644,#245645,#245646,#245647,#245648,
#245649,#245650,#245651,#245652,#245653,#245654,#245655,#245656,#245657,
#245658,#245659,#245660,#245661,#245662,#245663,#245664,#245665,#245666,
#245667,#245668,#245669,#245670,#245671,#245672,#245673,#245674,#245675,
#245676,#245677,#245678,#245679,#245680,#245681,#245682,#245683,#245684,
#245685,#245686,#245687,#245688,#245689,#245690,#245691,#245692,#245693,
#245694,#245695,#245696,#245697,#245698,#245699,#245700,#245701,#245702,
#245703,#245704,#245705,#245706,#245707,#245708,#245709,#245710,#245711,
#245712),(#245713,#245714,#245715,#245716,#245717,#245718,#245719,#245720,
#245721,#245722,#245723,#245724,#245725,#245726,#245727,#245728,#245729,
#245730,#245731,#245732,#245733,#245734,#245735,#245736,#245737,#245738,
#245739,#245740,#245741,#245742,#245743,#245744,#245745,#245746,#245747,
#245748,#245749,#245750,#245751,#245752,#245753,#245754,#245755,#245756,
#245757,#245758,#245759,#245760,#245761,#245762,#245763,#245764,#245765,
#245766,#245767,#245768,#245769,#245770,#245771,#245772,#245773,#245774,
#245775,#245776,#245777,#245778,#245779,#245780,#245781,#245782,#245783,
#245784,#245785,#245786,#245787,#245788,#245789,#245790,#245791,#245792,
#245793,#245794,#245795,#245796,#245797,#245798,#245799,#245800,#245801,
#245802,#245803,#245804,#245805,#245806,#245807,#245808,#245809,#245810,
#245811,#245812,#245813,#245814,#245815,#245816,#245817,#245818,#245819,
#245820,#245821,#245822,#245823,#245824,#245825,#245826,#245827,#245828,
#245829,#245830,#245831,#245832,#245833,#245834,#245835,#245836,#245837,
#245838,#245839,#245840,#245841,#245842,#245843,#245844,#245845,#245846,
#245847,#245848,#245849,#245850,#245851,#245852,#245853,#245854,#245855,
#245856,#245857,#245858,#245859,#245860,#245861,#245862,#245863,#245864,
#245865,#245866,#245867,#245868,#245869,#245870,#245871,#245872,#245873,
#245874,#245875,#245876,#245877,#245878,#245879,#245880,#245881,#245882,
#245883,#245884,#245885,#245886,#245887,#245888,#245889,#245890,#245891,
#245892,#245893,#245894,#245895,#245896,#245897,#245898,#245899,#245900,
#245901,#245902,#245903,#245904,#245905,#245906,#245907,#245908,#245909,
#245910,#245911,#245912,#245913,#245914,#245915,#245916,#245917,#245918,
#245919,#245920,#245921,#245922,#245923,#245924,#245925,#245926,#245927,
#245928,#245929,#245930,#245931,#245932,#245933,#245934,#245935,#245936,
#245937,#245938,#245939,#245940,#245941,#245942,#245943,#245944,#245945,
#245946,#245947,#245948,#245949,#245950,#245951,#245952,#245953,#245954,
#245955,#245956,#245957,#245958,#245959,#245960,#245961,#245962,#245963,
#245964,#245965,#245966,#245967,#245968,#245969,#245970,#245971,#245972,
#245973,#245974,#245975,#245976,#245977,#245978,#245979,#245980,#245981,
#245982,#245983,#245984,#245985,#245986,#245987,#245988,#245989)),
 .UNSPECIFIED.,.F.,.F.,.F.)
B_SPLINE_SURFACE_WITH_KNOTS((2,2),(3,2,2,2,2,2,2,2,2,2,2,2,2,2,2,2,2,2,
2,2,2,2,2,2,2,2,2,2,2,2,2,2,2,2,2,2,2,2,2,2,2,2,2,2,2,2,2,2,2,2,2,2,2,2,
2,2,2,2,2,2,2,2,2,2,2,2,2,2,2,2,2,2,2,2,2,2,2,2,2,2,2,2,2,2,2,2,2,2,2,2,
2,2,2,2,2,2,2,2,2,2,2,2,2,2,2,2,2,2,2,2,2,2,2,2,2,2,2,2,2,2,2,2,2,2,2,2,
2,2,2,2,2,2,2,2,2,2,2,2,3),(0.,1.),(0.,0.0072463768115942,0.0144927536231884,
0.0217391304347826,0.0289855072463768,0.036231884057971,0.0434782608695652,
0.0507246376811594,0.0579710144927536,0.0652173913043478,0.072463768115942,
0.0797101449275362,0.0869565217391304,0.0942028985507246,0.101449275362319,
0.108695652173913,0.115942028985507,0.123188405797101,0.130434782608696,
0.13768115942029,0.144927536231884,0.152173913043478,0.159420289855073,
0.166666666666667,0.173913043478261,0.181159420289855,0.18840579710145,
0.195652173913044,0.202898550724637,0.210144927536232,0.217391304347826,
0.224637681159421,0.231884057971014,0.239130434782609,0.246376811594203,
0.253623188405797,0.260869565217392,0.268115942028985,0.275362318840579,
0.282608695652174,0.289855072463768,0.297101449275363,0.304347826086956,
0.31159420289855,0.318840579710145,0.326086956521739,0.333333333333334,
0.340579710144927,0.347826086956521,0.355072463768116,0.36231884057971,
0.369565217391304,0.376811594202899,0.384057971014493,0.391304347826087,
0.398550724637681,0.405797101449275,0.41304347826087,0.420289855072463,
0.427536231884058,0.434782608695652,0.442028985507247,0.449275362318841,
0.456521739130435,0.463768115942029,0.471014492753623,0.478260869565218,
0.485507246376812,0.492753623188406,0.5,0.507246376811594,0.514492753623188,
0.521739130434783,0.528985507246377,0.536231884057971,0.543478260869565,
0.550724637681159,0.557971014492754,0.565217391304348,0.572463768115942,
0.579710144927536,0.586956521739131,0.594202898550725,0.601449275362319,
0.608695652173913,0.615942028985507,0.623188405797101,0.630434782608696,
0.63768115942029,0.644927536231884,0.652173913043478,0.659420289855073,
0.666666666666667,0.673913043478261,0.681159420289855,0.688405797101449,
0.695652173913044,0.702898550724638,0.710144927536232,0.717391304347826,
0.72463768115942,0.731884057971015,0.739130434782609,0.746376811594203,
0.753623188405797,0.760869565217391,0.768115942028986,0.77536231884058,
0.782608695652174,0.789855072463768,0.797101449275362,0.804347826086956,
0.811594202898551,0.818840579710145,0.826086956521739,0.833333333333333,
0.840579710144928,0.847826086956522,0.855072463768116,0.86231884057971,
0.869565217391304,0.876811594202899,0.884057971014493,0.891304347826087,
0.898550724637681,0.905797101449275,0.91304347826087,0.920289855072464,
0.927536231884058,0.934782608695652,0.942028985507246,0.94927536231884,
0.956521739130435,0.963768115942029,0.971014492753623,0.978260869565217,
0.985507246376812,0.992753623188406,0.993818585798284),.UNSPECIFIED.)
GEOMETRIC_REPRESENTATION_ITEM()
RATIONAL_B_SPLINE_SURFACE(((1.,0.866025403784439,1.,0.866025403784439,1.,
0.866025403784439,1.,0.866025403784439,1.,0.866025403784439,1.,0.866025403784439,
1.,0.866025403784439,1.,0.866025403784439,1.,0.866025403784439,1.,0.866025403784439,
1.,0.866025403784439,1.,0.866025403784439,1.,0.866025403784439,1.,0.866025403784439,
1.,0.866025403784439,1.,0.866025403784439,1.,0.866025403784439,1.,0.866025403784439,
1.,0.866025403784439,1.,0.866025403784439,1.,0.866025403784439,1.,0.866025403784439,
1.,0.866025403784439,1.,0.866025403784439,1.,0.866025403784439,1.,0.866025403784439,
1.,0.866025403784439,1.,0.866025403784439,1.,0.866025403784439,1.,0.866025403784439,
1.,0.866025403784439,1.,0.866025403784439,1.,0.866025403784439,1.,0.866025403784439,
1.,0.866025403784439,1.,0.866025403784439,1.,0.866025403784439,1.,0.866025403784439,
1.,0.866025403784439,1.,0.866025403784439,1.,0.866025403784439,1.,0.866025403784439,
1.,0.866025403784439,1.,0.866025403784439,1.,0.866025403784439,1.,0.866025403784439,
1.,0.866025403784439,1.,0.866025403784439,1.,0.866025403784439,1.,0.866025403784439,
1.,0.866025403784439,1.,0.866025403784439,1.,0.866025403784439,1.,0.866025403784439,
1.,0.866025403784439,1.,0.866025403784439,1.,0.866025403784439,1.,0.866025403784439,
1.,0.866025403784439,1.,0.866025403784439,1.,0.866025403784439,1.,0.866025403784439,
1.,0.866025403784439,1.,0.866025403784439,1.,0.866025403784439,1.,0.866025403784439,
1.,0.866025403784439,1.,0.866025403784439,1.,0.866025403784439,1.,0.866025403784439,
1.,0.866025403784439,1.,0.866025403784439,1.,0.866025403784439,1.,0.866025403784439,
1.,0.866025403784439,1.,0.866025403784439,1.,0.866025403784439,1.,0.866025403784439,
1.,0.866025403784439,1.,0.866025403784439,1.,0.866025403784439,1.,0.866025403784439,
1.,0.866025403784439,1.,0.866025403784439,1.,0.866025403784439,1.,0.866025403784439,
1.,0.866025403784439,1.,0.866025403784439,1.,0.866025403784439,1.,0.866025403784439,
1.,0.866025403784439,1.,0.866025403784439,1.,0.866025403784439,1.,0.866025403784439,
1.,0.866025403784439,1.,0.866025403784439,1.,0.866025403784439,1.,0.866025403784439,
1.,0.866025403784439,1.,0.866025403784439,1.,0.866025403784439,1.,0.866025403784439,
1.,0.866025403784439,1.,0.866025403784439,1.,0.866025403784439,1.,0.866025403784439,
1.,0.866025403784439,1.,0.866025403784439,1.,0.866025403784439,1.,0.866025403784439,
1.,0.866025403784439,1.,0.866025403784439,1.,0.866025403784439,1.,0.866025403784439,
1.,0.866025403784439,1.,0.866025403784439,1.,0.866025403784439,1.,0.866025403784439,
1.,0.866025403784439,1.,0.866025403784439,1.,0.866025403784439,1.,0.866025403784439,
1.,0.866025403784439,1.,0.866025403784439,1.,0.866025403784439,1.,0.866025403784439,
1.,0.866025403784439,1.,0.866025403784439,1.,0.866025403784439,1.,0.866025403784439,
1.,0.866025403784439,1.,0.866025403784439,1.,0.866025403784439,1.,0.866025403784439,
1.,0.866025403784439,1.,0.866025403784439,1.,0.866025403784439,1.,0.98031044488126,
0.966408234404338),(1.,0.866025403784439,1.,0.866025403784439,1.,0.866025403784439,
1.,0.866025403784439,1.,0.866025403784439,1.,0.866025403784439,1.,0.866025403784439,
1.,0.866025403784439,1.,0.866025403784439,1.,0.866025403784439,1.,0.866025403784439,
1.,0.866025403784439,1.,0.866025403784439,1.,0.866025403784439,1.,0.866025403784439,
1.,0.866025403784439,1.,0.866025403784439,1.,0.866025403784439,1.,0.866025403784439,
1.,0.866025403784439,1.,0.866025403784439,1.,0.866025403784439,1.,0.866025403784439,
1.,0.866025403784439,1.,0.866025403784439,1.,0.866025403784439,1.,0.866025403784439,
1.,0.866025403784439,1.,0.866025403784439,1.,0.866025403784439,1.,0.866025403784439,
1.,0.866025403784439,1.,0.866025403784439,1.,0.866025403784439,1.,0.866025403784439,
1.,0.866025403784439,1.,0.866025403784439,1.,0.866025403784439,1.,0.866025403784439,
1.,0.866025403784439,1.,0.866025403784439,1.,0.866025403784439,1.,0.866025403784439,
1.,0.866025403784439,1.,0.866025403784439,1.,0.866025403784439,1.,0.866025403784439,
1.,0.866025403784439,1.,0.866025403784439,1.,0.866025403784439,1.,0.866025403784439,
1.,0.866025403784439,1.,0.866025403784439,1.,0.866025403784439,1.,0.866025403784439,
1.,0.866025403784439,1.,0.866025403784439,1.,0.866025403784439,1.,0.866025403784439,
1.,0.866025403784439,1.,0.866025403784439,1.,0.866025403784439,1.,0.866025403784439,
1.,0.866025403784439,1.,0.866025403784439,1.,0.866025403784439,1.,0.866025403784439,
1.,0.866025403784439,1.,0.866025403784439,1.,0.866025403784439,1.,0.866025403784439,
1.,0.866025403784439,1.,0.866025403784439,1.,0.866025403784439,1.,0.866025403784439,
1.,0.866025403784439,1.,0.866025403784439,1.,0.866025403784439,1.,0.866025403784439,
1.,0.866025403784439,1.,0.866025403784439,1.,0.866025403784439,1.,0.866025403784439,
1.,0.866025403784439,1.,0.866025403784439,1.,0.866025403784439,1.,0.866025403784439,
1.,0.866025403784439,1.,0.866025403784439,1.,0.866025403784439,1.,0.866025403784439,
1.,0.866025403784439,1.,0.866025403784439,1.,0.866025403784439,1.,0.866025403784439,
1.,0.866025403784439,1.,0.866025403784439,1.,0.866025403784439,1.,0.866025403784439,
1.,0.866025403784439,1.,0.866025403784439,1.,0.866025403784439,1.,0.866025403784439,
1.,0.866025403784439,1.,0.866025403784439,1.,0.866025403784439,1.,0.866025403784439,
1.,0.866025403784439,1.,0.866025403784439,1.,0.866025403784439,1.,0.866025403784439,
1.,0.866025403784439,1.,0.866025403784439,1.,0.866025403784439,1.,0.866025403784439,
1.,0.866025403784439,1.,0.866025403784439,1.,0.866025403784439,1.,0.866025403784439,
1.,0.866025403784439,1.,0.866025403784439,1.,0.866025403784439,1.,0.866025403784439,
1.,0.866025403784439,1.,0.866025403784439,1.,0.866025403784439,1.,0.866025403784439,
1.,0.866025403784439,1.,0.866025403784439,1.,0.866025403784439,1.,0.866025403784439,
1.,0.866025403784439,1.,0.866025403784439,1.,0.866025403784439,1.,0.866025403784439,
1.,0.866025403784439,1.,0.866025403784439,1.,0.98031044488126,0.966408234404338)))
REPRESENTATION_ITEM('')
SURFACE()
);
#3128=(
BOUNDED_SURFACE()
B_SPLINE_SURFACE(3,2,((#246021,#246022,#246023),(#246024,#246025,#246026),
(#246027,#246028,#246029),(#246030,#246031,#246032)),.UNSPECIFIED.,.F.,
 .F.,.F.)
B_SPLINE_SURFACE_WITH_KNOTS((4,4),(3,3),(0.,0.000928457009668218),(0.,0.749952265697638),
 .UNSPECIFIED.)
GEOMETRIC_REPRESENTATION_ITEM()
RATIONAL_B_SPLINE_SURFACE(((1.,0.97561107945597,0.98780321135177),(1.,0.97592437041105,
0.98795988673876),(1.,0.97623752029395,0.988116491576193),(1.,0.97655053044864,
0.988273026536181)))
REPRESENTATION_ITEM('')
SURFACE()
);
#3129=(
BOUNDED_SURFACE()
B_SPLINE_SURFACE(3,2,((#246039,#246040,#246041),(#246042,#246043,#246044),
(#246045,#246046,#246047),(#246048,#246049,#246050),(#246051,#246052,#246053),
(#246054,#246055,#246056),(#246057,#246058,#246059),(#246060,#246061,#246062),
(#246063,#246064,#246065),(#246066,#246067,#246068),(#246069,#246070,#246071),
(#246072,#246073,#246074),(#246075,#246076,#246077),(#246078,#246079,#246080)),
 .UNSPECIFIED.,.F.,.F.,.F.)
B_SPLINE_SURFACE_WITH_KNOTS((4,2,2,2,2,2,4),(3,3),(0.012210545256649,0.012913253531591,
0.0134151880136936,0.0136661552547448,0.0139171224957961,0.0141680897368473,
0.0144191053734446),(-0.00118607011455501,1.00106010974999),
 .UNSPECIFIED.)
GEOMETRIC_REPRESENTATION_ITEM()
RATIONAL_B_SPLINE_SURFACE(((1.00042223753196,0.821812523909012,1.00037734852569),
(1.00036561497319,0.845707677874531,1.00032674563643),(1.00031052998004,
0.868953967361828,1.00027751685078),(1.00022051976633,0.906938967721429,
1.00019707582205),(1.00018420004347,0.922266169259384,1.00016461732929),
(1.0001333136267,0.943740627317328,1.00011914076008),(1.00011734829418,
0.950478120060816,1.00010487273738),(1.00008857958998,0.962618733823534,
1.00007916249778),(1.00007587856666,0.967978663051886,1.00006781174835),
(1.00005828162361,0.975404707950268,1.00005208557525),(1.00005406471308,
0.977184276526349,1.00004831697381),(1.00005807698422,0.975491067339927,
1.00005190269153),(1.00006613372506,0.972091060928923,1.00005910290242),
(1.00007724141785,0.96740352939868,1.00006902971182)))
REPRESENTATION_ITEM('')
SURFACE()
);
#3130=(
BOUNDED_SURFACE()
B_SPLINE_SURFACE(3,2,((#246236,#246237,#246238),(#246239,#246240,#246241),
(#246242,#246243,#246244),(#246245,#246246,#246247)),.UNSPECIFIED.,.F.,
 .F.,.F.)
B_SPLINE_SURFACE_WITH_KNOTS((4,4),(3,3),(2.58410722075169,2.75084833243122),
(0.,1.),.UNSPECIFIED.)
GEOMETRIC_REPRESENTATION_ITEM()
RATIONAL_B_SPLINE_SURFACE(((1.,0.832178067339829,1.),(1.,0.836186490185363,
1.),(1.,0.83962897728861,1.),(1.,0.84247914424116,1.)))
REPRESENTATION_ITEM('')
SURFACE()
);
#3131=(
BOUNDED_SURFACE()
B_SPLINE_SURFACE(3,2,((#246253,#246254,#246255),(#246256,#246257,#246258),
(#246259,#246260,#246261),(#246262,#246263,#246264)),.UNSPECIFIED.,.F.,
 .F.,.F.)
B_SPLINE_SURFACE_WITH_KNOTS((4,4),(3,3),(0.,0.00132498435822727),(0.,1.),
 .UNSPECIFIED.)
GEOMETRIC_REPRESENTATION_ITEM()
RATIONAL_B_SPLINE_SURFACE(((1.,0.832178067339829,1.),(1.,0.82686356673151,
1.),(1.,0.821151298721319,1.),(1.,0.815289268529491,1.)))
REPRESENTATION_ITEM('')
SURFACE()
);
#3132=(
BOUNDED_SURFACE()
B_SPLINE_SURFACE(3,2,((#246297,#246298,#246299),(#246300,#246301,#246302),
(#246303,#246304,#246305),(#246306,#246307,#246308),(#246309,#246310,#246311),
(#246312,#246313,#246314),(#246315,#246316,#246317),(#246318,#246319,#246320),
(#246321,#246322,#246323),(#246324,#246325,#246326)),.UNSPECIFIED.,.F.,
 .F.,.F.)
B_SPLINE_SURFACE_WITH_KNOTS((4,2,2,2,4),(3,3),(-3.38271077815477E-17,0.0053077668156845,
0.00663470851960563,0.00796165022352677,0.010615533631369),(0.,1.),
 .UNSPECIFIED.)
GEOMETRIC_REPRESENTATION_ITEM()
RATIONAL_B_SPLINE_SURFACE(((1.,0.815289268529492,1.),(1.,0.819667585266128,
1.),(1.,0.820338423873395,1.),(1.,0.816466016787285,1.),(1.,0.815452764187778,
1.),(1.,0.812995487572161,1.),(1.,0.81154866816968,1.),(1.,0.806583085327115,
1.),(1.,0.802440012727956,1.),(1.,0.797521159322293,1.)))
REPRESENTATION_ITEM('')
SURFACE()
);
#3133=(
BOUNDED_SURFACE()
B_SPLINE_SURFACE(3,2,((#246443,#246444,#246445),(#246446,#246447,#246448),
(#246449,#246450,#246451),(#246452,#246453,#246454),(#246455,#246456,#246457),
(#246458,#246459,#246460)),.UNSPECIFIED.,.F.,.F.,.F.)
B_SPLINE_SURFACE_WITH_KNOTS((4,2,4),(3,3),(0.00808931143172237,0.0087165405671442,
0.00934376970256604),(0.,1.),.UNSPECIFIED.)
GEOMETRIC_REPRESENTATION_ITEM()
RATIONAL_B_SPLINE_SURFACE(((1.,0.797521159322292,1.),(1.,0.820509064499797,
1.),(1.,0.842744492243191,1.),(1.,0.885608693575932,1.),(1.,0.906523136189702,
1.),(1.,0.925255145240244,1.)))
REPRESENTATION_ITEM('')
SURFACE()
);
#3134=(
BOUNDED_SURFACE()
B_SPLINE_SURFACE(3,2,((#246523,#246524,#246525),(#246526,#246527,#246528),
(#246529,#246530,#246531),(#246532,#246533,#246534),(#246535,#246536,#246537),
(#246538,#246539,#246540),(#246541,#246542,#246543),(#246544,#246545,#246546),
(#246547,#246548,#246549),(#246550,#246551,#246552),(#246553,#246554,#246555),
(#246556,#246557,#246558),(#246559,#246560,#246561),(#246562,#246563,#246564),
(#246565,#246566,#246567),(#246568,#246569,#246570),(#246571,#246572,#246573),
(#246574,#246575,#246576),(#246577,#246578,#246579),(#246580,#246581,#246582)),
 .UNSPECIFIED.,.F.,.F.,.F.)
B_SPLINE_SURFACE_WITH_KNOTS((4,2,2,2,2,2,2,2,2,4),(3,3),(0.00111929193439265,
0.00178147539823544,0.00211256713015685,0.00227811299611754,0.00236088592909789,
0.00240227239558807,0.00242296562883316,0.00243331224545569,0.00243848555376697,
0.00244365886207824),(0.,1.),.UNSPECIFIED.)
GEOMETRIC_REPRESENTATION_ITEM()
RATIONAL_B_SPLINE_SURFACE(((1.,0.849234981733232,1.),(1.,0.870241987650574,
1.),(1.,0.895121832531114,1.),(1.,0.933989529870412,1.),(1.,0.947468186626281,
1.),(1.,0.967283733305218,1.),(1.,0.973827959689554,1.),(1.,0.983885895426172,
1.),(1.,0.987109304535727,1.),(1.,0.991867531035233,1.),(1.,0.993380275833142,
1.),(1.,0.996085964157165,1.),(1.,0.99695187264233,1.),(1.,0.99815729362421,
1.),(1.,0.998544146160859,1.),(1.,0.999082128717776,1.),(1.,0.999255712640949,
1.),(1.,0.999568658539456,1.),(1.,0.999758809035204,1.),(1.,0.99967095488344,
1.)))
REPRESENTATION_ITEM('')
SURFACE()
);
#3135=(
BOUNDED_SURFACE()
B_SPLINE_SURFACE(3,2,((#246601,#246602,#246603),(#246604,#246605,#246606),
(#246607,#246608,#246609),(#246610,#246611,#246612),(#246613,#246614,#246615),
(#246616,#246617,#246618)),.UNSPECIFIED.,.F.,.F.,.F.)
B_SPLINE_SURFACE_WITH_KNOTS((4,2,4),(3,3),(-1.368745591061E-5,0.000558644410170963,
0.00113103749536398),(0.,1.0001876508054),.UNSPECIFIED.)
GEOMETRIC_REPRESENTATION_ITEM()
RATIONAL_B_SPLINE_SURFACE(((1.,0.776510200206641,1.00008387608186),(1.,
0.780671305424827,1.00008231441237),(1.,0.789444453094105,1.00007902183592),
(1.,0.815105956743532,1.00006939103226),(1.,0.831679493744461,1.00006317095713),
(1.,0.850563496104669,1.00005608376062)))
REPRESENTATION_ITEM('')
SURFACE()
);
#3136=(
BOUNDED_SURFACE()
B_SPLINE_SURFACE(3,2,((#246676,#246677,#246678),(#246679,#246680,#246681),
(#246682,#246683,#246684),(#246685,#246686,#246687)),.UNSPECIFIED.,.F.,
 .F.,.F.)
B_SPLINE_SURFACE_WITH_KNOTS((4,4),(3,3),(0.00612686414750675,0.00733563944177598),
(0.,1.),.UNSPECIFIED.)
GEOMETRIC_REPRESENTATION_ITEM()
RATIONAL_B_SPLINE_SURFACE(((1.,0.776858520243962,1.),(1.,0.757903633195438,
1.),(1.,0.733510495431111,1.),(1.,0.707106781186548,1.)))
REPRESENTATION_ITEM('')
SURFACE()
);
#3137=(
BOUNDED_SURFACE()
B_SPLINE_SURFACE(3,2,((#246689,#246690,#246691),(#246692,#246693,#246694),
(#246695,#246696,#246697),(#246698,#246699,#246700)),.UNSPECIFIED.,.F.,
 .F.,.F.)
B_SPLINE_SURFACE_WITH_KNOTS((4,4),(3,3),(0.00603197572710737,0.00723932307207816),
(0.,1.),.UNSPECIFIED.)
GEOMETRIC_REPRESENTATION_ITEM()
RATIONAL_B_SPLINE_SURFACE(((1.,0.707106781186549,1.),(1.,0.733656875693368,
1.),(1.,0.758260023147512,1.),(1.,0.776858520243961,1.)))
REPRESENTATION_ITEM('')
SURFACE()
);
#3138=(
BOUNDED_SURFACE()
B_SPLINE_SURFACE(3,2,((#246704,#246705,#246706),(#246707,#246708,#246709),
(#246710,#246711,#246712),(#246713,#246714,#246715),(#246716,#246717,#246718),
(#246719,#246720,#246721)),.UNSPECIFIED.,.F.,.F.,.F.)
B_SPLINE_SURFACE_WITH_KNOTS((4,2,4),(3,3),(-0.000111927549594358,0.000559637745952908,
0.00123115031984094),(0.,1.00031845895621),.UNSPECIFIED.)
GEOMETRIC_REPRESENTATION_ITEM()
RATIONAL_B_SPLINE_SURFACE(((1.,0.860513397693372,1.00008884151555),(1.,
0.837277590186421,1.00010364081756),(1.,0.817467037853214,1.0001162585132),
(1.,0.787333305184159,1.0001354512273),(1.,0.777597790956806,1.0001416519507),
(1.,0.774832571355172,1.0001434131686)))
REPRESENTATION_ITEM('')
SURFACE()
);
#3139=(
BOUNDED_SURFACE()
B_SPLINE_SURFACE(3,2,((#246776,#246777,#246778),(#246779,#246780,#246781),
(#246782,#246783,#246784),(#246785,#246786,#246787),(#246788,#246789,#246790),
(#246791,#246792,#246793),(#246794,#246795,#246796),(#246797,#246798,#246799),
(#246800,#246801,#246802),(#246803,#246804,#246805),(#246806,#246807,#246808),
(#246809,#246810,#246811),(#246812,#246813,#246814),(#246815,#246816,#246817),
(#246818,#246819,#246820),(#246821,#246822,#246823),(#246824,#246825,#246826),
(#246827,#246828,#246829),(#246830,#246831,#246832),(#246833,#246834,#246835)),
 .UNSPECIFIED.,.F.,.F.,.F.)
B_SPLINE_SURFACE_WITH_KNOTS((4,2,2,2,2,2,2,2,2,4),(3,3),(0.00111929193439371,
0.00178158198025093,0.00211272700317955,0.00227829951464385,0.00236108577037601,
0.00240247889824208,0.00242317546217512,0.00243352374414164,0.0024386978851249,
0.00244387202610816),(0.,1.),.UNSPECIFIED.)
GEOMETRIC_REPRESENTATION_ITEM()
RATIONAL_B_SPLINE_SURFACE(((1.,0.849234981733213,1.),(1.,0.870241987653356,
1.),(1.,0.89512183252925,1.),(1.,0.933989529872486,1.),(1.,0.947468186625073,
1.),(1.,0.967283733305516,1.),(1.,0.973827959687474,1.),(1.,0.983885895428084,
1.),(1.,0.98710930453863,1.),(1.,0.99186753103398,1.),(1.,0.993380275830688,
1.),(1.,0.996085964157665,1.),(1.,0.99695187264221,1.),(1.,0.998157293624355,
1.),(1.,0.998544146162347,1.),(1.,0.999082128717726,1.),(1.,0.999255712642408,
1.),(1.,0.999568658539312,1.),(1.,0.999758809037123,1.),(1.,0.999670954879881,
1.)))
REPRESENTATION_ITEM('')
SURFACE()
);
#3140=(
BOUNDED_SURFACE()
B_SPLINE_SURFACE(3,2,((#246852,#246853,#246854),(#246855,#246856,#246857),
(#246858,#246859,#246860),(#246861,#246862,#246863)),.UNSPECIFIED.,.F.,
 .F.,.F.)
B_SPLINE_SURFACE_WITH_KNOTS((4,4),(3,3),(0.0408455795445267,0.042773718086462),
(0.,1.),.UNSPECIFIED.)
GEOMETRIC_REPRESENTATION_ITEM()
RATIONAL_B_SPLINE_SURFACE(((1.,0.967701496827011,1.),(1.,0.968545704393032,
1.),(1.,0.969390043334334,1.),(1.,0.970233777086396,1.)))
REPRESENTATION_ITEM('')
SURFACE()
);
#3141=(
BOUNDED_SURFACE()
B_SPLINE_SURFACE(3,2,((#246884,#246885,#246886),(#246887,#246888,#246889),
(#246890,#246891,#246892),(#246893,#246894,#246895),(#246896,#246897,#246898),
(#246899,#246900,#246901),(#246902,#246903,#246904),(#246905,#246906,#246907),
(#246908,#246909,#246910),(#246911,#246912,#246913),(#246914,#246915,#246916),
(#246917,#246918,#246919),(#246920,#246921,#246922),(#246923,#246924,#246925)),
 .UNSPECIFIED.,.F.,.F.,.F.)
B_SPLINE_SURFACE_WITH_KNOTS((4,2,2,2,2,2,4),(3,3),(0.00641476504360471,
0.00720885616391255,0.00758281066823651,0.00795676517256048,0.00833071967688444,
0.0087046741812084,0.00945258318985632),(0.,1.00004618211165),
 .UNSPECIFIED.)
GEOMETRIC_REPRESENTATION_ITEM()
RATIONAL_B_SPLINE_SURFACE(((1.,0.706895776308564,1.00002707234397),(1.,
0.708010377644408,1.00002696939468),(1.,0.709414341304934,1.00002683971867),
(1.,0.712474126198451,1.00002655710402),(1.,0.713589100039244,1.00002645412032),
(1.,0.716224859765459,1.00002621067042),(1.,0.717766798011333,1.00002606825049),
(1.,0.721310542436779,1.00002574093529),(1.,0.723318075519062,1.00002555551106),
(1.,0.727854283400673,1.00002513652774),(1.,0.730408561181452,1.00002490060386),
(1.,0.738132660070436,1.00002418717346),(1.,0.743606172212938,1.00002368161677),
(1.,0.745071384918521,1.00002354628353)))
REPRESENTATION_ITEM('')
SURFACE()
);
#3142=(
BOUNDED_SURFACE()
B_SPLINE_SURFACE(3,2,((#247118,#247119,#247120),(#247121,#247122,#247123),
(#247124,#247125,#247126),(#247127,#247128,#247129),(#247130,#247131,#247132),
(#247133,#247134,#247135),(#247136,#247137,#247138),(#247139,#247140,#247141),
(#247142,#247143,#247144),(#247145,#247146,#247147)),.UNSPECIFIED.,.F.,
 .F.,.F.)
B_SPLINE_SURFACE_WITH_KNOTS((4,2,2,2,4),(3,3),(0.,0.392699081698725,0.785398163397449,
1.17809724509617,1.5707963267949),(0.,1.),.UNSPECIFIED.)
GEOMETRIC_REPRESENTATION_ITEM()
RATIONAL_B_SPLINE_SURFACE(((1.,0.819152044288993,1.),(1.,0.819160091424011,
1.),(1.,0.816447805244711,1.),(1.,0.805887184900773,1.),(1.,0.798030050106979,
1.),(1.,0.777942514786192,1.),(1.,0.765710795400617,1.),(1.,0.738207714616384,
1.),(1.,0.722944887324406,1.),(1.,0.707106781186549,1.)))
REPRESENTATION_ITEM('')
SURFACE()
);
#3143=(
BOUNDED_SURFACE()
B_SPLINE_SURFACE(3,2,((#247249,#247250,#247251),(#247252,#247253,#247254),
(#247255,#247256,#247257),(#247258,#247259,#247260),(#247261,#247262,#247263),
(#247264,#247265,#247266),(#247267,#247268,#247269),(#247270,#247271,#247272),
(#247273,#247274,#247275),(#247276,#247277,#247278),(#247279,#247280,#247281),
(#247282,#247283,#247284),(#247285,#247286,#247287),(#247288,#247289,#247290)),
 .UNSPECIFIED.,.F.,.F.,.F.)
B_SPLINE_SURFACE_WITH_KNOTS((4,2,2,2,2,2,4),(3,3),(0.00646808747938269,
0.00724932038878676,0.00763316097925953,0.0080170015697323,0.00840084216020507,
0.00878468275067784,0.00955236393162338),(-1.35517284585259E-5,1.),
 .UNSPECIFIED.)
GEOMETRIC_REPRESENTATION_ITEM()
RATIONAL_B_SPLINE_SURFACE(((1.00000793151294,0.707361574991507,1.),(1.00000806626139,
0.7023899417983,1.),(1.00000820227477,0.697371638210326,1.),(1.00000839312539,
0.690330078134294,1.),(1.00000845317796,0.688114398442112,1.),(1.00000856755574,
0.683894354745816,1.),(1.00000862230378,0.681874389455888,1.),(1.00000872143439,
0.678216899825171,1.),(1.00000876629923,0.676561581859308,1.),(1.00000884629199,
0.673610195926044,1.),(1.00000888117563,0.672323140891743,1.),(1.00000896617579,
0.669187003750694,1.),(1.00000899882615,0.667982347216541,1.),(1.0000090031805,
0.667821690638002,1.)))
REPRESENTATION_ITEM('')
SURFACE()
);
#3144=(
BOUNDED_SURFACE()
B_SPLINE_SURFACE(3,2,((#247491,#247492,#247493),(#247494,#247495,#247496),
(#247497,#247498,#247499),(#247500,#247501,#247502),(#247503,#247504,#247505),
(#247506,#247507,#247508),(#247509,#247510,#247511),(#247512,#247513,#247514),
(#247515,#247516,#247517),(#247518,#247519,#247520)),.UNSPECIFIED.,.F.,
 .F.,.F.)
B_SPLINE_SURFACE_WITH_KNOTS((4,2,2,2,4),(3,3),(1.5707963267949,1.96585160298382,
2.36090687917273,2.75596215536165,3.15101743155057),(0.,1.),
 .UNSPECIFIED.)
GEOMETRIC_REPRESENTATION_ITEM()
RATIONAL_B_SPLINE_SURFACE(((1.,0.707106781186549,1.),(1.,0.723040087310248,
1.),(1.,0.738390656304015,1.),(1.,0.766022585770263,1.),(1.,0.778295218542395,
1.),(1.,0.7983986260281,1.),(1.,0.806230755417563,1.),(1.,0.816669539143349,
1.),(1.,0.819285194795031,1.),(1.,0.819147408352828,1.)))
REPRESENTATION_ITEM('')
SURFACE()
);
#3145=(
BOUNDED_SURFACE()
B_SPLINE_SURFACE(3,2,((#247631,#247632,#247633),(#247634,#247635,#247636),
(#247637,#247638,#247639),(#247640,#247641,#247642)),.UNSPECIFIED.,.F.,
 .F.,.F.)
B_SPLINE_SURFACE_WITH_KNOTS((4,4),(3,3),(0.,0.000561888377921629),(0.,1.),
 .UNSPECIFIED.)
GEOMETRIC_REPRESENTATION_ITEM()
RATIONAL_B_SPLINE_SURFACE(((1.,0.721830660407024,1.),(1.,0.726161642227015,
1.),(1.,0.730217605430419,1.),(1.,0.734028581001202,1.)))
REPRESENTATION_ITEM('')
SURFACE()
);
#3146=(
BOUNDED_SURFACE()
B_SPLINE_SURFACE(3,2,((#247648,#247649,#247650),(#247651,#247652,#247653),
(#247654,#247655,#247656),(#247657,#247658,#247659)),.UNSPECIFIED.,.F.,
 .F.,.F.)
B_SPLINE_SURFACE_WITH_KNOTS((4,4),(3,3),(-8.67361737988403E-18,0.0027255914917872),
(0.,1.),.UNSPECIFIED.)
GEOMETRIC_REPRESENTATION_ITEM()
RATIONAL_B_SPLINE_SURFACE(((1.,0.721830660407024,1.),(1.,0.722050915678773,
1.),(1.,0.722280885253549,1.),(1.,0.722521956262064,1.)))
REPRESENTATION_ITEM('')
SURFACE()
);
#3147=(
BOUNDED_SURFACE()
B_SPLINE_SURFACE(3,2,((#247675,#247676,#247677),(#247678,#247679,#247680),
(#247681,#247682,#247683),(#247684,#247685,#247686),(#247687,#247688,#247689),
(#247690,#247691,#247692),(#247693,#247694,#247695),(#247696,#247697,#247698),
(#247699,#247700,#247701),(#247702,#247703,#247704),(#247705,#247706,#247707),
(#247708,#247709,#247710)),.UNSPECIFIED.,.F.,.F.,.F.)
B_SPLINE_SURFACE_WITH_KNOTS((4,2,2,2,2,4),(3,3),(-2.71050543121376E-20,
0.000196917635222578,0.000295376452833867,0.000393835270445156,0.000590752905667733,
0.000787670540890311),(0.,1.),.UNSPECIFIED.)
GEOMETRIC_REPRESENTATION_ITEM()
RATIONAL_B_SPLINE_SURFACE(((1.,0.768827303401079,1.),(1.,0.768839794086584,
1.),(1.,0.767245932333086,1.),(1.,0.76267317155594,1.),(1.,0.760806266526503,
1.),(1.,0.756383065794974,1.),(1.,0.753812076955945,1.),(1.,0.745366037508728,
1.),(1.,0.738532036970522,1.),(1.,0.723650553821477,1.),(1.,0.715418707911078,
1.),(1.,0.707106781186548,1.)))
REPRESENTATION_ITEM('')
SURFACE()
);
#3148=(
BOUNDED_SURFACE()
B_SPLINE_SURFACE(3,2,((#247840,#247841,#247842),(#247843,#247844,#247845),
(#247846,#247847,#247848),(#247849,#247850,#247851)),.UNSPECIFIED.,.F.,
 .F.,.F.)
B_SPLINE_SURFACE_WITH_KNOTS((4,4),(3,3),(0.,0.00308554567306433),(0.,1.),
 .UNSPECIFIED.)
GEOMETRIC_REPRESENTATION_ITEM()
RATIONAL_B_SPLINE_SURFACE(((1.,0.722521956262063,1.),(1.,0.722249049952648,
1.),(1.,0.721990362413173,1.),(1.,0.721743903804635,1.)))
REPRESENTATION_ITEM('')
SURFACE()
);
#3149=(
BOUNDED_SURFACE()
B_SPLINE_SURFACE(3,2,((#247867,#247868,#247869),(#247870,#247871,#247872),
(#247873,#247874,#247875),(#247876,#247877,#247878),(#247879,#247880,#247881),
(#247882,#247883,#247884),(#247885,#247886,#247887),(#247888,#247889,#247890),
(#247891,#247892,#247893),(#247894,#247895,#247896),(#247897,#247898,#247899),
(#247900,#247901,#247902)),.UNSPECIFIED.,.F.,.F.,.F.)
B_SPLINE_SURFACE_WITH_KNOTS((4,2,2,2,2,4),(3,3),(0.,0.000196919474660801,
0.000295379211991202,0.000393838949321602,0.000590758423982404,0.000787677898643205),
(0.,1.),.UNSPECIFIED.)
GEOMETRIC_REPRESENTATION_ITEM()
RATIONAL_B_SPLINE_SURFACE(((1.,0.707106781186546,1.),(1.,0.715396063584809,
1.),(1.,0.723543617208936,1.),(1.,0.734788510950855,1.),(1.,0.738325118179662,
1.),(1.,0.744992206539526,1.),(1.,0.748144662339383,1.),(1.,0.756608512730963,
1.),(1.,0.761139004306969,1.),(1.,0.767215293085605,1.),(1.,0.768836106148694,
1.),(1.,0.768827303401081,1.)))
REPRESENTATION_ITEM('')
SURFACE()
);
#3150=(
BOUNDED_SURFACE()
B_SPLINE_SURFACE(3,2,((#248044,#248045,#248046),(#248047,#248048,#248049),
(#248050,#248051,#248052),(#248053,#248054,#248055)),.UNSPECIFIED.,.F.,
 .F.,.F.)
B_SPLINE_SURFACE_WITH_KNOTS((4,4),(3,3),(0.,0.00168726762248989),(0.,1.),
 .UNSPECIFIED.)
GEOMETRIC_REPRESENTATION_ITEM()
RATIONAL_B_SPLINE_SURFACE(((1.,0.788010753606719,1.),(1.,0.787995580138724,
1.),(1.,0.785892129585524,1.),(1.,0.781757935428468,1.)))
REPRESENTATION_ITEM('')
SURFACE()
);
#3151=(
BOUNDED_SURFACE()
B_SPLINE_SURFACE(3,2,((#248107,#248108,#248109),(#248110,#248111,#248112),
(#248113,#248114,#248115),(#248116,#248117,#248118),(#248119,#248120,#248121),
(#248122,#248123,#248124)),.UNSPECIFIED.,.F.,.F.,.F.)
B_SPLINE_SURFACE_WITH_KNOTS((4,2,4),(3,3),(0.,0.000492064922826377,0.000984129845652755),
(0.,1.),.UNSPECIFIED.)
GEOMETRIC_REPRESENTATION_ITEM()
RATIONAL_B_SPLINE_SURFACE(((1.,0.788010753606719,1.),(1.,0.787995463701203,
1.),(1.,0.786698704019208,1.),(1.,0.781418067371145,1.),(1.,0.777580790644453,
1.),(1.,0.772541161150265,1.)))
REPRESENTATION_ITEM('')
SURFACE()
);
#3152=(
BOUNDED_SURFACE()
B_SPLINE_SURFACE(3,2,((#248148,#248149,#248150),(#248151,#248152,#248153),
(#248154,#248155,#248156),(#248157,#248158,#248159),(#248160,#248161,#248162),
(#248163,#248164,#248165)),.UNSPECIFIED.,.F.,.F.,.F.)
B_SPLINE_SURFACE_WITH_KNOTS((4,2,4),(3,3),(1.0842021724855E-19,0.000492127602558551,
0.000984255205117102),(0.,1.),.UNSPECIFIED.)
GEOMETRIC_REPRESENTATION_ITEM()
RATIONAL_B_SPLINE_SURFACE(((1.,0.772541161150265,1.),(1.,0.7775811913717,
1.),(1.,0.781415995839735,1.),(1.,0.786696090924191,1.),(1.,0.787997416142609,
1.),(1.,0.788010753606718,1.)))
REPRESENTATION_ITEM('')
SURFACE()
);
#3153=(
BOUNDED_SURFACE()
B_SPLINE_SURFACE(3,2,((#248192,#248193,#248194),(#248195,#248196,#248197),
(#248198,#248199,#248200),(#248201,#248202,#248203)),.UNSPECIFIED.,.F.,
 .F.,.F.)
B_SPLINE_SURFACE_WITH_KNOTS((4,4),(3,3),(-3.46944695195361E-18,0.00168726762248988),
(0.,1.),.UNSPECIFIED.)
GEOMETRIC_REPRESENTATION_ITEM()
RATIONAL_B_SPLINE_SURFACE(((1.,0.781757935428468,1.),(1.,0.785892129585526,
1.),(1.,0.787995580138721,1.),(1.,0.78801075360672,1.)))
REPRESENTATION_ITEM('')
SURFACE()
);
#3154=(
BOUNDED_SURFACE()
B_SPLINE_SURFACE(3,2,((#248257,#248258,#248259),(#248260,#248261,#248262),
(#248263,#248264,#248265),(#248266,#248267,#248268),(#248269,#248270,#248271),
(#248272,#248273,#248274)),.UNSPECIFIED.,.F.,.F.,.F.)
B_SPLINE_SURFACE_WITH_KNOTS((4,2,4),(3,3),(0.,0.000492064922826383,0.000984129845652766),
(0.,1.),.UNSPECIFIED.)
GEOMETRIC_REPRESENTATION_ITEM()
RATIONAL_B_SPLINE_SURFACE(((1.,0.78801075360672,1.),(1.,0.787995463701083,
1.),(1.,0.786698704019365,1.),(1.,0.781418067370988,1.),(1.,0.777580790644572,
1.),(1.,0.772541161150265,1.)))
REPRESENTATION_ITEM('')
SURFACE()
);
#3155=(
BOUNDED_SURFACE()
B_SPLINE_SURFACE(3,2,((#248298,#248299,#248300),(#248301,#248302,#248303),
(#248304,#248305,#248306),(#248307,#248308,#248309),(#248310,#248311,#248312),
(#248313,#248314,#248315)),.UNSPECIFIED.,.F.,.F.,.F.)
B_SPLINE_SURFACE_WITH_KNOTS((4,2,4),(3,3),(0.,0.000492127602558548,0.000984255205117095),
(0.,1.),.UNSPECIFIED.)
GEOMETRIC_REPRESENTATION_ITEM()
RATIONAL_B_SPLINE_SURFACE(((1.,0.772541161150265,1.),(1.,0.777581191371582,
1.),(1.,0.781415995839892,1.),(1.,0.786696090924034,1.),(1.,0.787997416142728,
1.),(1.,0.78801075360672,1.)))
REPRESENTATION_ITEM('')
SURFACE()
);
#3156=(
BOUNDED_SURFACE()
B_SPLINE_SURFACE(3,2,((#248342,#248343,#248344),(#248345,#248346,#248347),
(#248348,#248349,#248350),(#248351,#248352,#248353)),.UNSPECIFIED.,.F.,
 .F.,.F.)
B_SPLINE_SURFACE_WITH_KNOTS((4,4),(3,3),(0.,0.00168726762248988),(0.,1.),
 .UNSPECIFIED.)
GEOMETRIC_REPRESENTATION_ITEM()
RATIONAL_B_SPLINE_SURFACE(((1.,0.78175793542847,1.),(1.,0.785892129585525,
1.),(1.,0.787995580138723,1.),(1.,0.788010753606719,1.)))
REPRESENTATION_ITEM('')
SURFACE()
);
#3157=(
BOUNDED_SURFACE()
B_SPLINE_SURFACE(3,2,((#248371,#248372,#248373),(#248374,#248375,#248376),
(#248377,#248378,#248379),(#248380,#248381,#248382)),.UNSPECIFIED.,.F.,
 .F.,.F.)
B_SPLINE_SURFACE_WITH_KNOTS((4,4),(3,3),(-0.000914415610118037,0.0178445500057952),
(0.,1.00091441561012),.UNSPECIFIED.)
GEOMETRIC_REPRESENTATION_ITEM()
RATIONAL_B_SPLINE_SURFACE(((1.,0.771817621836307,1.00041730705709),(1.,
0.77533655889149,1.00041087151514),(1.,0.779001978127809,1.00040416808201),
(1.,0.782001690466344,1.00039868211443)))
REPRESENTATION_ITEM('')
SURFACE()
);
#3158=(
BOUNDED_SURFACE()
B_SPLINE_SURFACE(3,2,((#248413,#248414,#248415),(#248416,#248417,#248418),
(#248419,#248420,#248421),(#248422,#248423,#248424)),.UNSPECIFIED.,.F.,
 .F.,.F.)
B_SPLINE_SURFACE_WITH_KNOTS((4,4),(3,3),(-0.000914415609804201,0.0178445500054813),
(0.,1.0009144156098),.UNSPECIFIED.)
GEOMETRIC_REPRESENTATION_ITEM()
RATIONAL_B_SPLINE_SURFACE(((1.,0.771817621836556,1.00041730705695),(1.,
0.77533655889162,1.000410871515),(1.,0.779001978127809,1.00040416808187),
(0.999999999999999,0.782001690466259,1.0003986821143)))
REPRESENTATION_ITEM('')
SURFACE()
);
#3159=(
BOUNDED_SURFACE()
B_SPLINE_SURFACE(3,2,((#248455,#248456,#248457),(#248458,#248459,#248460),
(#248461,#248462,#248463),(#248464,#248465,#248466)),.UNSPECIFIED.,.F.,
 .F.,.F.)
B_SPLINE_SURFACE_WITH_KNOTS((4,4),(3,3),(-0.000914415609905059,0.0178445500055823),
(0.,1.00091441560991),.UNSPECIFIED.)
GEOMETRIC_REPRESENTATION_ITEM()
RATIONAL_B_SPLINE_SURFACE(((0.999999999999999,0.782001690466286,1.00039868211434),
(1.,0.779001978127807,1.00040416808192),(1.,0.775336558891579,1.00041087151505),
(1.,0.771817621836475,1.000417307057)))
REPRESENTATION_ITEM('')
SURFACE()
);
#3160=(
BOUNDED_SURFACE()
B_SPLINE_SURFACE(3,2,((#248606,#248607,#248608),(#248609,#248610,#248611),
(#248612,#248613,#248614),(#248615,#248616,#248617)),.UNSPECIFIED.,.F.,
 .F.,.F.)
B_SPLINE_SURFACE_WITH_KNOTS((4,4),(3,3),(0.,0.00168726762248989),(0.,1.),
 .UNSPECIFIED.)
GEOMETRIC_REPRESENTATION_ITEM()
RATIONAL_B_SPLINE_SURFACE(((1.,0.788010753606719,1.),(1.,0.787995580138724,
1.),(1.,0.785892129585524,1.),(1.,0.781757935428468,1.)))
REPRESENTATION_ITEM('')
SURFACE()
);
#3161=(
BOUNDED_SURFACE()
B_SPLINE_SURFACE(3,2,((#248701,#248702,#248703),(#248704,#248705,#248706),
(#248707,#248708,#248709),(#248710,#248711,#248712),(#248713,#248714,#248715),
(#248716,#248717,#248718)),.UNSPECIFIED.,.F.,.F.,.F.)
B_SPLINE_SURFACE_WITH_KNOTS((4,2,4),(3,3),(0.,0.000492064922826377,0.000984129845652755),
(0.,1.),.UNSPECIFIED.)
GEOMETRIC_REPRESENTATION_ITEM()
RATIONAL_B_SPLINE_SURFACE(((1.,0.788010753606719,1.),(1.,0.787995463701203,
1.),(1.,0.786698704019208,1.),(1.,0.781418067371145,1.),(1.,0.777580790644453,
1.),(1.,0.772541161150265,1.)))
REPRESENTATION_ITEM('')
SURFACE()
);
#3162=(
BOUNDED_SURFACE()
B_SPLINE_SURFACE(3,2,((#248742,#248743,#248744),(#248745,#248746,#248747),
(#248748,#248749,#248750),(#248751,#248752,#248753),(#248754,#248755,#248756),
(#248757,#248758,#248759)),.UNSPECIFIED.,.F.,.F.,.F.)
B_SPLINE_SURFACE_WITH_KNOTS((4,2,4),(3,3),(1.0842021724855E-19,0.000492127602558551,
0.000984255205117102),(0.,1.),.UNSPECIFIED.)
GEOMETRIC_REPRESENTATION_ITEM()
RATIONAL_B_SPLINE_SURFACE(((1.,0.772541161150265,1.),(1.,0.7775811913717,
1.),(1.,0.781415995839735,1.),(1.,0.786696090924191,1.),(1.,0.787997416142609,
1.),(1.,0.788010753606718,1.)))
REPRESENTATION_ITEM('')
SURFACE()
);
#3163=(
BOUNDED_SURFACE()
B_SPLINE_SURFACE(3,2,((#248786,#248787,#248788),(#248789,#248790,#248791),
(#248792,#248793,#248794),(#248795,#248796,#248797)),.UNSPECIFIED.,.F.,
 .F.,.F.)
B_SPLINE_SURFACE_WITH_KNOTS((4,4),(3,3),(-3.46944695195361E-18,0.00168726762248988),
(0.,1.),.UNSPECIFIED.)
GEOMETRIC_REPRESENTATION_ITEM()
RATIONAL_B_SPLINE_SURFACE(((1.,0.781757935428468,1.),(1.,0.785892129585526,
1.),(1.,0.787995580138721,1.),(1.,0.78801075360672,1.)))
REPRESENTATION_ITEM('')
SURFACE()
);
#3164=(
BOUNDED_SURFACE()
B_SPLINE_SURFACE(3,2,((#248818,#248819,#248820),(#248821,#248822,#248823),
(#248824,#248825,#248826),(#248827,#248828,#248829)),.UNSPECIFIED.,.F.,
 .F.,.F.)
B_SPLINE_SURFACE_WITH_KNOTS((4,4),(3,3),(0.,0.00168726762248987),(0.,1.),
 .UNSPECIFIED.)
GEOMETRIC_REPRESENTATION_ITEM()
RATIONAL_B_SPLINE_SURFACE(((1.,0.78801075360672,1.),(1.,0.787995580138721,
1.),(1.,0.785892129585525,1.),(1.,0.78175793542847,1.)))
REPRESENTATION_ITEM('')
SURFACE()
);
#3165=(
BOUNDED_SURFACE()
B_SPLINE_SURFACE(3,2,((#248913,#248914,#248915),(#248916,#248917,#248918),
(#248919,#248920,#248921),(#248922,#248923,#248924),(#248925,#248926,#248927),
(#248928,#248929,#248930)),.UNSPECIFIED.,.F.,.F.,.F.)
B_SPLINE_SURFACE_WITH_KNOTS((4,2,4),(3,3),(0.,0.000492064922826383,0.000984129845652766),
(0.,1.),.UNSPECIFIED.)
GEOMETRIC_REPRESENTATION_ITEM()
RATIONAL_B_SPLINE_SURFACE(((1.,0.78801075360672,1.),(1.,0.787995463701083,
1.),(1.,0.786698704019365,1.),(1.,0.781418067370988,1.),(1.,0.777580790644572,
1.),(1.,0.772541161150265,1.)))
REPRESENTATION_ITEM('')
SURFACE()
);
#3166=(
BOUNDED_SURFACE()
B_SPLINE_SURFACE(3,2,((#248954,#248955,#248956),(#248957,#248958,#248959),
(#248960,#248961,#248962),(#248963,#248964,#248965),(#248966,#248967,#248968),
(#248969,#248970,#248971)),.UNSPECIFIED.,.F.,.F.,.F.)
B_SPLINE_SURFACE_WITH_KNOTS((4,2,4),(3,3),(0.,0.000492127602558548,0.000984255205117095),
(0.,1.),.UNSPECIFIED.)
GEOMETRIC_REPRESENTATION_ITEM()
RATIONAL_B_SPLINE_SURFACE(((1.,0.772541161150265,1.),(1.,0.777581191371582,
1.),(1.,0.781415995839892,1.),(1.,0.786696090924034,1.),(1.,0.787997416142728,
1.),(1.,0.78801075360672,1.)))
REPRESENTATION_ITEM('')
SURFACE()
);
#3167=(
BOUNDED_SURFACE()
B_SPLINE_SURFACE(3,2,((#248998,#248999,#249000),(#249001,#249002,#249003),
(#249004,#249005,#249006),(#249007,#249008,#249009)),.UNSPECIFIED.,.F.,
 .F.,.F.)
B_SPLINE_SURFACE_WITH_KNOTS((4,4),(3,3),(0.,0.00168726762248988),(0.,1.),
 .UNSPECIFIED.)
GEOMETRIC_REPRESENTATION_ITEM()
RATIONAL_B_SPLINE_SURFACE(((1.,0.78175793542847,1.),(1.,0.785892129585525,
1.),(1.,0.787995580138723,1.),(1.,0.788010753606719,1.)))
REPRESENTATION_ITEM('')
SURFACE()
);
#3168=(
BOUNDED_SURFACE()
B_SPLINE_SURFACE(3,2,((#249041,#249042,#249043),(#249044,#249045,#249046),
(#249047,#249048,#249049),(#249050,#249051,#249052)),.UNSPECIFIED.,.F.,
 .F.,.F.)
B_SPLINE_SURFACE_WITH_KNOTS((4,4),(3,3),(-1.38777878078145E-17,0.0169301343956772),
(0.,1.),.UNSPECIFIED.)
GEOMETRIC_REPRESENTATION_ITEM()
RATIONAL_B_SPLINE_SURFACE(((1.,0.772541161150265,1.),(1.,0.775725268487667,
1.),(1.,0.778996361886149,1.),(1.,0.78175793542847,1.)))
REPRESENTATION_ITEM('')
SURFACE()
);
#3169=(
BOUNDED_SURFACE()
B_SPLINE_SURFACE(3,2,((#249071,#249072,#249073),(#249074,#249075,#249076),
(#249077,#249078,#249079),(#249080,#249081,#249082)),.UNSPECIFIED.,.F.,
 .F.,.F.)
B_SPLINE_SURFACE_WITH_KNOTS((4,4),(3,3),(-6.93889390390723E-18,0.0169301343956773),
(0.,1.),.UNSPECIFIED.)
GEOMETRIC_REPRESENTATION_ITEM()
RATIONAL_B_SPLINE_SURFACE(((1.,0.781757935428468,1.),(1.,0.778996361886152,
1.),(1.,0.775725268487663,1.),(1.,0.772541161150265,1.)))
REPRESENTATION_ITEM('')
SURFACE()
);
#3170=(
BOUNDED_SURFACE()
B_SPLINE_SURFACE(3,2,((#249102,#249103,#249104),(#249105,#249106,#249107),
(#249108,#249109,#249110),(#249111,#249112,#249113)),.UNSPECIFIED.,.F.,
 .F.,.F.)
B_SPLINE_SURFACE_WITH_KNOTS((4,4),(3,3),(-6.93889390390723E-18,0.0169301343956771),
(0.,1.),.UNSPECIFIED.)
GEOMETRIC_REPRESENTATION_ITEM()
RATIONAL_B_SPLINE_SURFACE(((1.,0.772541161150265,1.),(1.,0.775725268487663,
1.),(1.,0.778996361886151,1.),(1.,0.781757935428468,1.)))
REPRESENTATION_ITEM('')
SURFACE()
);
#3171=(
BOUNDED_SURFACE()
B_SPLINE_SURFACE(3,2,((#249132,#249133,#249134),(#249135,#249136,#249137),
(#249138,#249139,#249140),(#249141,#249142,#249143)),.UNSPECIFIED.,.F.,
 .F.,.F.)
B_SPLINE_SURFACE_WITH_KNOTS((4,4),(3,3),(0.,0.0169301343956772),(0.,1.),
 .UNSPECIFIED.)
GEOMETRIC_REPRESENTATION_ITEM()
RATIONAL_B_SPLINE_SURFACE(((1.,0.781757935428468,1.),(1.,0.778996361886149,
1.),(1.,0.775725268487665,1.),(1.,0.772541161150265,1.)))
REPRESENTATION_ITEM('')
SURFACE()
);
#3172=(
BOUNDED_SURFACE()
B_SPLINE_SURFACE(3,2,((#249172,#249173,#249174),(#249175,#249176,#249177),
(#249178,#249179,#249180),(#249181,#249182,#249183)),.UNSPECIFIED.,.F.,
 .F.,.F.)
B_SPLINE_SURFACE_WITH_KNOTS((4,4),(3,3),(0.00337631140392896,0.0169301343956773),
(0.,1.),.UNSPECIFIED.)
GEOMETRIC_REPRESENTATION_ITEM()
RATIONAL_B_SPLINE_SURFACE(((1.,0.780050659744625,1.),(1.,0.777690973944284,
1.),(1.,0.775093372307372,1.),(1.,0.772541161150265,1.)))
REPRESENTATION_ITEM('')
SURFACE()
);
#3173=(
BOUNDED_SURFACE()
B_SPLINE_SURFACE(1,2,((#249602,#249603,#249604,#249605,#249606,#249607,
#249608,#249609,#249610,#249611,#249612,#249613,#249614,#249615,#249616,
#249617,#249618,#249619,#249620,#249621,#249622,#249623,#249624,#249625,
#249626,#249627,#249628,#249629,#249630,#249631,#249632,#249633,#249634,
#249635,#249636,#249637,#249638,#249639,#249640,#249641,#249642,#249643,
#249644,#249645,#249646,#249647,#249648,#249649,#249650,#249651,#249652,
#249653,#249654,#249655,#249656,#249657,#249658,#249659,#249660,#249661,
#249662,#249663,#249664,#249665,#249666,#249667,#249668,#249669,#249670,
#249671,#249672,#249673,#249674,#249675,#249676,#249677,#249678,#249679,
#249680,#249681,#249682,#249683,#249684,#249685,#249686,#249687,#249688,
#249689,#249690,#249691,#249692,#249693,#249694,#249695,#249696,#249697,
#249698,#249699,#249700,#249701,#249702,#249703,#249704,#249705,#249706,
#249707,#249708,#249709,#249710,#249711,#249712,#249713,#249714,#249715,
#249716,#249717,#249718,#249719,#249720,#249721,#249722,#249723,#249724,
#249725,#249726,#249727,#249728,#249729,#249730,#249731,#249732,#249733,
#249734,#249735,#249736,#249737,#249738,#249739,#249740,#249741,#249742,
#249743,#249744,#249745,#249746,#249747,#249748,#249749,#249750,#249751,
#249752,#249753,#249754,#249755,#249756,#249757,#249758,#249759,#249760,
#249761,#249762,#249763,#249764,#249765,#249766,#249767,#249768,#249769,
#249770,#249771,#249772,#249773,#249774,#249775,#249776,#249777,#249778,
#249779,#249780,#249781,#249782,#249783,#249784,#249785,#249786,#249787,
#249788,#249789,#249790,#249791,#249792,#249793,#249794,#249795,#249796,
#249797,#249798,#249799,#249800,#249801,#249802,#249803,#249804,#249805,
#249806,#249807,#249808,#249809,#249810,#249811,#249812,#249813,#249814,
#249815,#249816,#249817,#249818,#249819,#249820,#249821,#249822,#249823,
#249824,#249825,#249826,#249827,#249828,#249829,#249830,#249831,#249832,
#249833,#249834,#249835,#249836,#249837,#249838,#249839,#249840,#249841,
#249842,#249843,#249844,#249845,#249846,#249847,#249848,#249849,#249850,
#249851,#249852,#249853,#249854,#249855,#249856,#249857,#249858,#249859,
#249860,#249861,#249862,#249863,#249864,#249865,#249866,#249867,#249868,
#249869,#249870,#249871,#249872,#249873,#249874,#249875,#249876,#249877,
#249878),(#249879,#249880,#249881,#249882,#249883,#249884,#249885,#249886,
#249887,#249888,#249889,#249890,#249891,#249892,#249893,#249894,#249895,
#249896,#249897,#249898,#249899,#249900,#249901,#249902,#249903,#249904,
#249905,#249906,#249907,#249908,#249909,#249910,#249911,#249912,#249913,
#249914,#249915,#249916,#249917,#249918,#249919,#249920,#249921,#249922,
#249923,#249924,#249925,#249926,#249927,#249928,#249929,#249930,#249931,
#249932,#249933,#249934,#249935,#249936,#249937,#249938,#249939,#249940,
#249941,#249942,#249943,#249944,#249945,#249946,#249947,#249948,#249949,
#249950,#249951,#249952,#249953,#249954,#249955,#249956,#249957,#249958,
#249959,#249960,#249961,#249962,#249963,#249964,#249965,#249966,#249967,
#249968,#249969,#249970,#249971,#249972,#249973,#249974,#249975,#249976,
#249977,#249978,#249979,#249980,#249981,#249982,#249983,#249984,#249985,
#249986,#249987,#249988,#249989,#249990,#249991,#249992,#249993,#249994,
#249995,#249996,#249997,#249998,#249999,#250000,#250001,#250002,#250003,
#250004,#250005,#250006,#250007,#250008,#250009,#250010,#250011,#250012,
#250013,#250014,#250015,#250016,#250017,#250018,#250019,#250020,#250021,
#250022,#250023,#250024,#250025,#250026,#250027,#250028,#250029,#250030,
#250031,#250032,#250033,#250034,#250035,#250036,#250037,#250038,#250039,
#250040,#250041,#250042,#250043,#250044,#250045,#250046,#250047,#250048,
#250049,#250050,#250051,#250052,#250053,#250054,#250055,#250056,#250057,
#250058,#250059,#250060,#250061,#250062,#250063,#250064,#250065,#250066,
#250067,#250068,#250069,#250070,#250071,#250072,#250073,#250074,#250075,
#250076,#250077,#250078,#250079,#250080,#250081,#250082,#250083,#250084,
#250085,#250086,#250087,#250088,#250089,#250090,#250091,#250092,#250093,
#250094,#250095,#250096,#250097,#250098,#250099,#250100,#250101,#250102,
#250103,#250104,#250105,#250106,#250107,#250108,#250109,#250110,#250111,
#250112,#250113,#250114,#250115,#250116,#250117,#250118,#250119,#250120,
#250121,#250122,#250123,#250124,#250125,#250126,#250127,#250128,#250129,
#250130,#250131,#250132,#250133,#250134,#250135,#250136,#250137,#250138,
#250139,#250140,#250141,#250142,#250143,#250144,#250145,#250146,#250147,
#250148,#250149,#250150,#250151,#250152,#250153,#250154,#250155)),
 .UNSPECIFIED.,.F.,.F.,.F.)
B_SPLINE_SURFACE_WITH_KNOTS((2,2),(3,2,2,2,2,2,2,2,2,2,2,2,2,2,2,2,2,2,
2,2,2,2,2,2,2,2,2,2,2,2,2,2,2,2,2,2,2,2,2,2,2,2,2,2,2,2,2,2,2,2,2,2,2,2,
2,2,2,2,2,2,2,2,2,2,2,2,2,2,2,2,2,2,2,2,2,2,2,2,2,2,2,2,2,2,2,2,2,2,2,2,
2,2,2,2,2,2,2,2,2,2,2,2,2,2,2,2,2,2,2,2,2,2,2,2,2,2,2,2,2,2,2,2,2,2,2,2,
2,2,2,2,2,2,2,2,2,2,2,2,3),(0.,1.),(0.,0.0072463768115942,0.0144927536231884,
0.0217391304347826,0.0289855072463768,0.036231884057971,0.0434782608695652,
0.0507246376811594,0.0579710144927536,0.0652173913043478,0.072463768115942,
0.0797101449275362,0.0869565217391304,0.0942028985507246,0.101449275362319,
0.108695652173913,0.115942028985507,0.123188405797101,0.130434782608696,
0.13768115942029,0.144927536231884,0.152173913043478,0.159420289855073,
0.166666666666667,0.173913043478261,0.181159420289855,0.18840579710145,
0.195652173913044,0.202898550724637,0.210144927536232,0.217391304347826,
0.224637681159421,0.231884057971014,0.239130434782609,0.246376811594203,
0.253623188405797,0.260869565217392,0.268115942028985,0.275362318840579,
0.282608695652174,0.289855072463768,0.297101449275363,0.304347826086956,
0.31159420289855,0.318840579710145,0.326086956521739,0.333333333333334,
0.340579710144927,0.347826086956521,0.355072463768116,0.36231884057971,
0.369565217391304,0.376811594202899,0.384057971014493,0.391304347826087,
0.398550724637681,0.405797101449275,0.41304347826087,0.420289855072463,
0.427536231884058,0.434782608695652,0.442028985507247,0.449275362318841,
0.456521739130435,0.463768115942029,0.471014492753623,0.478260869565218,
0.485507246376812,0.492753623188406,0.5,0.507246376811594,0.514492753623188,
0.521739130434783,0.528985507246377,0.536231884057971,0.543478260869565,
0.550724637681159,0.557971014492754,0.565217391304348,0.572463768115942,
0.579710144927536,0.586956521739131,0.594202898550725,0.601449275362319,
0.608695652173913,0.615942028985507,0.623188405797101,0.630434782608696,
0.63768115942029,0.644927536231884,0.652173913043478,0.659420289855073,
0.666666666666667,0.673913043478261,0.681159420289855,0.688405797101449,
0.695652173913044,0.702898550724638,0.710144927536232,0.717391304347826,
0.72463768115942,0.731884057971015,0.739130434782609,0.746376811594203,
0.753623188405797,0.760869565217391,0.768115942028986,0.77536231884058,
0.782608695652174,0.789855072463768,0.797101449275362,0.804347826086956,
0.811594202898551,0.818840579710145,0.826086956521739,0.833333333333333,
0.840579710144928,0.847826086956522,0.855072463768116,0.86231884057971,
0.869565217391304,0.876811594202899,0.884057971014493,0.891304347826087,
0.898550724637681,0.905797101449275,0.91304347826087,0.920289855072464,
0.927536231884058,0.934782608695652,0.942028985507246,0.94927536231884,
0.956521739130435,0.963768115942029,0.971014492753623,0.978260869565217,
0.985507246376812,0.992753623188406,0.993818585798284),.UNSPECIFIED.)
GEOMETRIC_REPRESENTATION_ITEM()
RATIONAL_B_SPLINE_SURFACE(((1.,0.866025403784439,1.,0.866025403784439,1.,
0.866025403784439,1.,0.866025403784439,1.,0.866025403784439,1.,0.866025403784439,
1.,0.866025403784439,1.,0.866025403784439,1.,0.866025403784439,1.,0.866025403784439,
1.,0.866025403784439,1.,0.866025403784439,1.,0.866025403784439,1.,0.866025403784439,
1.,0.866025403784439,1.,0.866025403784439,1.,0.866025403784439,1.,0.866025403784439,
1.,0.866025403784439,1.,0.866025403784439,1.,0.866025403784439,1.,0.866025403784439,
1.,0.866025403784439,1.,0.866025403784439,1.,0.866025403784439,1.,0.866025403784439,
1.,0.866025403784439,1.,0.866025403784439,1.,0.866025403784439,1.,0.866025403784439,
1.,0.866025403784439,1.,0.866025403784439,1.,0.866025403784439,1.,0.866025403784439,
1.,0.866025403784439,1.,0.866025403784439,1.,0.866025403784439,1.,0.866025403784439,
1.,0.866025403784439,1.,0.866025403784439,1.,0.866025403784439,1.,0.866025403784439,
1.,0.866025403784439,1.,0.866025403784439,1.,0.866025403784439,1.,0.866025403784439,
1.,0.866025403784439,1.,0.866025403784439,1.,0.866025403784439,1.,0.866025403784439,
1.,0.866025403784439,1.,0.866025403784439,1.,0.866025403784439,1.,0.866025403784439,
1.,0.866025403784439,1.,0.866025403784439,1.,0.866025403784439,1.,0.866025403784439,
1.,0.866025403784439,1.,0.866025403784439,1.,0.866025403784439,1.,0.866025403784439,
1.,0.866025403784439,1.,0.866025403784439,1.,0.866025403784439,1.,0.866025403784439,
1.,0.866025403784439,1.,0.866025403784439,1.,0.866025403784439,1.,0.866025403784439,
1.,0.866025403784439,1.,0.866025403784439,1.,0.866025403784439,1.,0.866025403784439,
1.,0.866025403784439,1.,0.866025403784439,1.,0.866025403784439,1.,0.866025403784439,
1.,0.866025403784439,1.,0.866025403784439,1.,0.866025403784439,1.,0.866025403784439,
1.,0.866025403784439,1.,0.866025403784439,1.,0.866025403784439,1.,0.866025403784439,
1.,0.866025403784439,1.,0.866025403784439,1.,0.866025403784439,1.,0.866025403784439,
1.,0.866025403784439,1.,0.866025403784439,1.,0.866025403784439,1.,0.866025403784439,
1.,0.866025403784439,1.,0.866025403784439,1.,0.866025403784439,1.,0.866025403784439,
1.,0.866025403784439,1.,0.866025403784439,1.,0.866025403784439,1.,0.866025403784439,
1.,0.866025403784439,1.,0.866025403784439,1.,0.866025403784439,1.,0.866025403784439,
1.,0.866025403784439,1.,0.866025403784439,1.,0.866025403784439,1.,0.866025403784439,
1.,0.866025403784439,1.,0.866025403784439,1.,0.866025403784439,1.,0.866025403784439,
1.,0.866025403784439,1.,0.866025403784439,1.,0.866025403784439,1.,0.866025403784439,
1.,0.866025403784439,1.,0.866025403784439,1.,0.866025403784439,1.,0.866025403784439,
1.,0.866025403784439,1.,0.866025403784439,1.,0.866025403784439,1.,0.866025403784439,
1.,0.866025403784439,1.,0.866025403784439,1.,0.866025403784439,1.,0.866025403784439,
1.,0.866025403784439,1.,0.866025403784439,1.,0.866025403784439,1.,0.866025403784439,
1.,0.866025403784439,1.,0.866025403784439,1.,0.866025403784439,1.,0.98031044488126,
0.966408234404338),(1.,0.866025403784439,1.,0.866025403784439,1.,0.866025403784439,
1.,0.866025403784439,1.,0.866025403784439,1.,0.866025403784439,1.,0.866025403784439,
1.,0.866025403784439,1.,0.866025403784439,1.,0.866025403784439,1.,0.866025403784439,
1.,0.866025403784439,1.,0.866025403784439,1.,0.866025403784439,1.,0.866025403784439,
1.,0.866025403784439,1.,0.866025403784439,1.,0.866025403784439,1.,0.866025403784439,
1.,0.866025403784439,1.,0.866025403784439,1.,0.866025403784439,1.,0.866025403784439,
1.,0.866025403784439,1.,0.866025403784439,1.,0.866025403784439,1.,0.866025403784439,
1.,0.866025403784439,1.,0.866025403784439,1.,0.866025403784439,1.,0.866025403784439,
1.,0.866025403784439,1.,0.866025403784439,1.,0.866025403784439,1.,0.866025403784439,
1.,0.866025403784439,1.,0.866025403784439,1.,0.866025403784439,1.,0.866025403784439,
1.,0.866025403784439,1.,0.866025403784439,1.,0.866025403784439,1.,0.866025403784439,
1.,0.866025403784439,1.,0.866025403784439,1.,0.866025403784439,1.,0.866025403784439,
1.,0.866025403784439,1.,0.866025403784439,1.,0.866025403784439,1.,0.866025403784439,
1.,0.866025403784439,1.,0.866025403784439,1.,0.866025403784439,1.,0.866025403784439,
1.,0.866025403784439,1.,0.866025403784439,1.,0.866025403784439,1.,0.866025403784439,
1.,0.866025403784439,1.,0.866025403784439,1.,0.866025403784439,1.,0.866025403784439,
1.,0.866025403784439,1.,0.866025403784439,1.,0.866025403784439,1.,0.866025403784439,
1.,0.866025403784439,1.,0.866025403784439,1.,0.866025403784439,1.,0.866025403784439,
1.,0.866025403784439,1.,0.866025403784439,1.,0.866025403784439,1.,0.866025403784439,
1.,0.866025403784439,1.,0.866025403784439,1.,0.866025403784439,1.,0.866025403784439,
1.,0.866025403784439,1.,0.866025403784439,1.,0.866025403784439,1.,0.866025403784439,
1.,0.866025403784439,1.,0.866025403784439,1.,0.866025403784439,1.,0.866025403784439,
1.,0.866025403784439,1.,0.866025403784439,1.,0.866025403784439,1.,0.866025403784439,
1.,0.866025403784439,1.,0.866025403784439,1.,0.866025403784439,1.,0.866025403784439,
1.,0.866025403784439,1.,0.866025403784439,1.,0.866025403784439,1.,0.866025403784439,
1.,0.866025403784439,1.,0.866025403784439,1.,0.866025403784439,1.,0.866025403784439,
1.,0.866025403784439,1.,0.866025403784439,1.,0.866025403784439,1.,0.866025403784439,
1.,0.866025403784439,1.,0.866025403784439,1.,0.866025403784439,1.,0.866025403784439,
1.,0.866025403784439,1.,0.866025403784439,1.,0.866025403784439,1.,0.866025403784439,
1.,0.866025403784439,1.,0.866025403784439,1.,0.866025403784439,1.,0.866025403784439,
1.,0.866025403784439,1.,0.866025403784439,1.,0.866025403784439,1.,0.866025403784439,
1.,0.866025403784439,1.,0.866025403784439,1.,0.866025403784439,1.,0.866025403784439,
1.,0.866025403784439,1.,0.866025403784439,1.,0.866025403784439,1.,0.866025403784439,
1.,0.866025403784439,1.,0.866025403784439,1.,0.866025403784439,1.,0.866025403784439,
1.,0.866025403784439,1.,0.866025403784439,1.,0.98031044488126,0.966408234404338)))
REPRESENTATION_ITEM('')
SURFACE()
);
#3174=(
BOUNDED_SURFACE()
B_SPLINE_SURFACE(1,2,((#252065,#252066,#252067,#252068,#252069,#252070,
#252071,#252072,#252073,#252074,#252075,#252076,#252077,#252078,#252079,
#252080,#252081,#252082,#252083,#252084,#252085,#252086,#252087,#252088,
#252089,#252090,#252091,#252092,#252093,#252094,#252095,#252096,#252097,
#252098,#252099,#252100,#252101,#252102,#252103,#252104,#252105,#252106,
#252107,#252108,#252109,#252110,#252111,#252112,#252113,#252114,#252115,
#252116,#252117,#252118,#252119,#252120,#252121,#252122,#252123,#252124,
#252125,#252126,#252127,#252128,#252129,#252130,#252131,#252132,#252133,
#252134,#252135,#252136,#252137,#252138,#252139,#252140,#252141,#252142,
#252143,#252144,#252145,#252146,#252147,#252148,#252149,#252150,#252151,
#252152,#252153,#252154,#252155,#252156,#252157,#252158,#252159,#252160,
#252161,#252162,#252163,#252164,#252165,#252166,#252167,#252168,#252169,
#252170,#252171,#252172,#252173,#252174,#252175,#252176,#252177,#252178,
#252179,#252180,#252181,#252182,#252183,#252184,#252185,#252186,#252187,
#252188,#252189,#252190,#252191,#252192,#252193,#252194,#252195,#252196,
#252197,#252198,#252199,#252200,#252201,#252202,#252203,#252204,#252205,
#252206,#252207,#252208,#252209,#252210,#252211,#252212,#252213,#252214,
#252215,#252216,#252217,#252218,#252219,#252220,#252221,#252222,#252223,
#252224,#252225,#252226,#252227,#252228,#252229,#252230,#252231,#252232,
#252233,#252234,#252235,#252236,#252237,#252238,#252239,#252240,#252241,
#252242,#252243,#252244,#252245,#252246,#252247,#252248,#252249,#252250,
#252251,#252252,#252253,#252254,#252255,#252256,#252257,#252258,#252259,
#252260,#252261,#252262,#252263,#252264,#252265,#252266,#252267,#252268,
#252269,#252270,#252271,#252272,#252273,#252274,#252275,#252276,#252277,
#252278,#252279,#252280,#252281,#252282,#252283,#252284,#252285,#252286,
#252287,#252288,#252289,#252290,#252291,#252292,#252293,#252294,#252295,
#252296,#252297,#252298,#252299,#252300,#252301,#252302,#252303,#252304,
#252305,#252306,#252307,#252308,#252309,#252310,#252311,#252312,#252313,
#252314,#252315,#252316,#252317,#252318,#252319,#252320,#252321,#252322,
#252323,#252324,#252325,#252326,#252327,#252328,#252329,#252330,#252331,
#252332,#252333,#252334,#252335,#252336,#252337,#252338,#252339,#252340,
#252341),(#252342,#252343,#252344,#252345,#252346,#252347,#252348,#252349,
#252350,#252351,#252352,#252353,#252354,#252355,#252356,#252357,#252358,
#252359,#252360,#252361,#252362,#252363,#252364,#252365,#252366,#252367,
#252368,#252369,#252370,#252371,#252372,#252373,#252374,#252375,#252376,
#252377,#252378,#252379,#252380,#252381,#252382,#252383,#252384,#252385,
#252386,#252387,#252388,#252389,#252390,#252391,#252392,#252393,#252394,
#252395,#252396,#252397,#252398,#252399,#252400,#252401,#252402,#252403,
#252404,#252405,#252406,#252407,#252408,#252409,#252410,#252411,#252412,
#252413,#252414,#252415,#252416,#252417,#252418,#252419,#252420,#252421,
#252422,#252423,#252424,#252425,#252426,#252427,#252428,#252429,#252430,
#252431,#252432,#252433,#252434,#252435,#252436,#252437,#252438,#252439,
#252440,#252441,#252442,#252443,#252444,#252445,#252446,#252447,#252448,
#252449,#252450,#252451,#252452,#252453,#252454,#252455,#252456,#252457,
#252458,#252459,#252460,#252461,#252462,#252463,#252464,#252465,#252466,
#252467,#252468,#252469,#252470,#252471,#252472,#252473,#252474,#252475,
#252476,#252477,#252478,#252479,#252480,#252481,#252482,#252483,#252484,
#252485,#252486,#252487,#252488,#252489,#252490,#252491,#252492,#252493,
#252494,#252495,#252496,#252497,#252498,#252499,#252500,#252501,#252502,
#252503,#252504,#252505,#252506,#252507,#252508,#252509,#252510,#252511,
#252512,#252513,#252514,#252515,#252516,#252517,#252518,#252519,#252520,
#252521,#252522,#252523,#252524,#252525,#252526,#252527,#252528,#252529,
#252530,#252531,#252532,#252533,#252534,#252535,#252536,#252537,#252538,
#252539,#252540,#252541,#252542,#252543,#252544,#252545,#252546,#252547,
#252548,#252549,#252550,#252551,#252552,#252553,#252554,#252555,#252556,
#252557,#252558,#252559,#252560,#252561,#252562,#252563,#252564,#252565,
#252566,#252567,#252568,#252569,#252570,#252571,#252572,#252573,#252574,
#252575,#252576,#252577,#252578,#252579,#252580,#252581,#252582,#252583,
#252584,#252585,#252586,#252587,#252588,#252589,#252590,#252591,#252592,
#252593,#252594,#252595,#252596,#252597,#252598,#252599,#252600,#252601,
#252602,#252603,#252604,#252605,#252606,#252607,#252608,#252609,#252610,
#252611,#252612,#252613,#252614,#252615,#252616,#252617,#252618)),
 .UNSPECIFIED.,.F.,.F.,.F.)
B_SPLINE_SURFACE_WITH_KNOTS((2,2),(3,2,2,2,2,2,2,2,2,2,2,2,2,2,2,2,2,2,
2,2,2,2,2,2,2,2,2,2,2,2,2,2,2,2,2,2,2,2,2,2,2,2,2,2,2,2,2,2,2,2,2,2,2,2,
2,2,2,2,2,2,2,2,2,2,2,2,2,2,2,2,2,2,2,2,2,2,2,2,2,2,2,2,2,2,2,2,2,2,2,2,
2,2,2,2,2,2,2,2,2,2,2,2,2,2,2,2,2,2,2,2,2,2,2,2,2,2,2,2,2,2,2,2,2,2,2,2,
2,2,2,2,2,2,2,2,2,2,2,2,3),(0.,1.),(0.,0.0072463768115942,0.0144927536231884,
0.0217391304347826,0.0289855072463768,0.036231884057971,0.0434782608695652,
0.0507246376811594,0.0579710144927536,0.0652173913043478,0.072463768115942,
0.0797101449275362,0.0869565217391304,0.0942028985507246,0.101449275362319,
0.108695652173913,0.115942028985507,0.123188405797101,0.130434782608696,
0.13768115942029,0.144927536231884,0.152173913043478,0.159420289855073,
0.166666666666667,0.173913043478261,0.181159420289855,0.18840579710145,
0.195652173913044,0.202898550724637,0.210144927536232,0.217391304347826,
0.224637681159421,0.231884057971014,0.239130434782609,0.246376811594203,
0.253623188405797,0.260869565217392,0.268115942028985,0.275362318840579,
0.282608695652174,0.289855072463768,0.297101449275363,0.304347826086956,
0.31159420289855,0.318840579710145,0.326086956521739,0.333333333333334,
0.340579710144927,0.347826086956521,0.355072463768116,0.36231884057971,
0.369565217391304,0.376811594202899,0.384057971014493,0.391304347826087,
0.398550724637681,0.405797101449275,0.41304347826087,0.420289855072463,
0.427536231884058,0.434782608695652,0.442028985507247,0.449275362318841,
0.456521739130435,0.463768115942029,0.471014492753623,0.478260869565218,
0.485507246376812,0.492753623188406,0.5,0.507246376811594,0.514492753623188,
0.521739130434783,0.528985507246377,0.536231884057971,0.543478260869565,
0.550724637681159,0.557971014492754,0.565217391304348,0.572463768115942,
0.579710144927536,0.586956521739131,0.594202898550725,0.601449275362319,
0.608695652173913,0.615942028985507,0.623188405797101,0.630434782608696,
0.63768115942029,0.644927536231884,0.652173913043478,0.659420289855073,
0.666666666666667,0.673913043478261,0.681159420289855,0.688405797101449,
0.695652173913044,0.702898550724638,0.710144927536232,0.717391304347826,
0.72463768115942,0.731884057971015,0.739130434782609,0.746376811594203,
0.753623188405797,0.760869565217391,0.768115942028986,0.77536231884058,
0.782608695652174,0.789855072463768,0.797101449275362,0.804347826086956,
0.811594202898551,0.818840579710145,0.826086956521739,0.833333333333333,
0.840579710144928,0.847826086956522,0.855072463768116,0.86231884057971,
0.869565217391304,0.876811594202899,0.884057971014493,0.891304347826087,
0.898550724637681,0.905797101449275,0.91304347826087,0.920289855072464,
0.927536231884058,0.934782608695652,0.942028985507246,0.94927536231884,
0.956521739130435,0.963768115942029,0.971014492753623,0.978260869565217,
0.985507246376812,0.992753623188406,0.993818495192186),.UNSPECIFIED.)
GEOMETRIC_REPRESENTATION_ITEM()
RATIONAL_B_SPLINE_SURFACE(((1.,0.866025403784439,1.,0.866025403784439,1.,
0.866025403784439,1.,0.866025403784439,1.,0.866025403784439,1.,0.866025403784439,
1.,0.866025403784439,1.,0.866025403784439,1.,0.866025403784439,1.,0.866025403784439,
1.,0.866025403784439,1.,0.866025403784439,1.,0.866025403784439,1.,0.866025403784439,
1.,0.866025403784439,1.,0.866025403784439,1.,0.866025403784439,1.,0.866025403784439,
1.,0.866025403784439,1.,0.866025403784439,1.,0.866025403784439,1.,0.866025403784439,
1.,0.866025403784439,1.,0.866025403784439,1.,0.866025403784439,1.,0.866025403784439,
1.,0.866025403784439,1.,0.866025403784439,1.,0.866025403784439,1.,0.866025403784439,
1.,0.866025403784439,1.,0.866025403784439,1.,0.866025403784439,1.,0.866025403784439,
1.,0.866025403784439,1.,0.866025403784439,1.,0.866025403784439,1.,0.866025403784439,
1.,0.866025403784439,1.,0.866025403784439,1.,0.866025403784439,1.,0.866025403784439,
1.,0.866025403784439,1.,0.866025403784439,1.,0.866025403784439,1.,0.866025403784439,
1.,0.866025403784439,1.,0.866025403784439,1.,0.866025403784439,1.,0.866025403784439,
1.,0.866025403784439,1.,0.866025403784439,1.,0.866025403784439,1.,0.866025403784439,
1.,0.866025403784439,1.,0.866025403784439,1.,0.866025403784439,1.,0.866025403784439,
1.,0.866025403784439,1.,0.866025403784439,1.,0.866025403784439,1.,0.866025403784439,
1.,0.866025403784439,1.,0.866025403784439,1.,0.866025403784439,1.,0.866025403784439,
1.,0.866025403784439,1.,0.866025403784439,1.,0.866025403784439,1.,0.866025403784439,
1.,0.866025403784439,1.,0.866025403784439,1.,0.866025403784439,1.,0.866025403784439,
1.,0.866025403784439,1.,0.866025403784439,1.,0.866025403784439,1.,0.866025403784439,
1.,0.866025403784439,1.,0.866025403784439,1.,0.866025403784439,1.,0.866025403784439,
1.,0.866025403784439,1.,0.866025403784439,1.,0.866025403784439,1.,0.866025403784439,
1.,0.866025403784439,1.,0.866025403784439,1.,0.866025403784439,1.,0.866025403784439,
1.,0.866025403784439,1.,0.866025403784439,1.,0.866025403784439,1.,0.866025403784439,
1.,0.866025403784439,1.,0.866025403784439,1.,0.866025403784439,1.,0.866025403784439,
1.,0.866025403784439,1.,0.866025403784439,1.,0.866025403784439,1.,0.866025403784439,
1.,0.866025403784439,1.,0.866025403784439,1.,0.866025403784439,1.,0.866025403784439,
1.,0.866025403784439,1.,0.866025403784439,1.,0.866025403784439,1.,0.866025403784439,
1.,0.866025403784439,1.,0.866025403784439,1.,0.866025403784439,1.,0.866025403784439,
1.,0.866025403784439,1.,0.866025403784439,1.,0.866025403784439,1.,0.866025403784439,
1.,0.866025403784439,1.,0.866025403784439,1.,0.866025403784439,1.,0.866025403784439,
1.,0.866025403784439,1.,0.866025403784439,1.,0.866025403784439,1.,0.866025403784439,
1.,0.866025403784439,1.,0.866025403784439,1.,0.866025403784439,1.,0.866025403784439,
1.,0.866025403784439,1.,0.866025403784439,1.,0.866025403784439,1.,0.866025403784439,
1.,0.866025403784439,1.,0.866025403784439,1.,0.866025403784439,1.,0.980312120051573,
0.966410600022306),(1.,0.866025403784439,1.,0.866025403784439,1.,0.866025403784439,
1.,0.866025403784439,1.,0.866025403784439,1.,0.866025403784439,1.,0.866025403784439,
1.,0.866025403784439,1.,0.866025403784439,1.,0.866025403784439,1.,0.866025403784439,
1.,0.866025403784439,1.,0.866025403784439,1.,0.866025403784439,1.,0.866025403784439,
1.,0.866025403784439,1.,0.866025403784439,1.,0.866025403784439,1.,0.866025403784439,
1.,0.866025403784439,1.,0.866025403784439,1.,0.866025403784439,1.,0.866025403784439,
1.,0.866025403784439,1.,0.866025403784439,1.,0.866025403784439,1.,0.866025403784439,
1.,0.866025403784439,1.,0.866025403784439,1.,0.866025403784439,1.,0.866025403784439,
1.,0.866025403784439,1.,0.866025403784439,1.,0.866025403784439,1.,0.866025403784439,
1.,0.866025403784439,1.,0.866025403784439,1.,0.866025403784439,1.,0.866025403784439,
1.,0.866025403784439,1.,0.866025403784439,1.,0.866025403784439,1.,0.866025403784439,
1.,0.866025403784439,1.,0.866025403784439,1.,0.866025403784439,1.,0.866025403784439,
1.,0.866025403784439,1.,0.866025403784439,1.,0.866025403784439,1.,0.866025403784439,
1.,0.866025403784439,1.,0.866025403784439,1.,0.866025403784439,1.,0.866025403784439,
1.,0.866025403784439,1.,0.866025403784439,1.,0.866025403784439,1.,0.866025403784439,
1.,0.866025403784439,1.,0.866025403784439,1.,0.866025403784439,1.,0.866025403784439,
1.,0.866025403784439,1.,0.866025403784439,1.,0.866025403784439,1.,0.866025403784439,
1.,0.866025403784439,1.,0.866025403784439,1.,0.866025403784439,1.,0.866025403784439,
1.,0.866025403784439,1.,0.866025403784439,1.,0.866025403784439,1.,0.866025403784439,
1.,0.866025403784439,1.,0.866025403784439,1.,0.866025403784439,1.,0.866025403784439,
1.,0.866025403784439,1.,0.866025403784439,1.,0.866025403784439,1.,0.866025403784439,
1.,0.866025403784439,1.,0.866025403784439,1.,0.866025403784439,1.,0.866025403784439,
1.,0.866025403784439,1.,0.866025403784439,1.,0.866025403784439,1.,0.866025403784439,
1.,0.866025403784439,1.,0.866025403784439,1.,0.866025403784439,1.,0.866025403784439,
1.,0.866025403784439,1.,0.866025403784439,1.,0.866025403784439,1.,0.866025403784439,
1.,0.866025403784439,1.,0.866025403784439,1.,0.866025403784439,1.,0.866025403784439,
1.,0.866025403784439,1.,0.866025403784439,1.,0.866025403784439,1.,0.866025403784439,
1.,0.866025403784439,1.,0.866025403784439,1.,0.866025403784439,1.,0.866025403784439,
1.,0.866025403784439,1.,0.866025403784439,1.,0.866025403784439,1.,0.866025403784439,
1.,0.866025403784439,1.,0.866025403784439,1.,0.866025403784439,1.,0.866025403784439,
1.,0.866025403784439,1.,0.866025403784439,1.,0.866025403784439,1.,0.866025403784439,
1.,0.866025403784439,1.,0.866025403784439,1.,0.866025403784439,1.,0.866025403784439,
1.,0.866025403784439,1.,0.866025403784439,1.,0.866025403784439,1.,0.866025403784439,
1.,0.866025403784439,1.,0.866025403784439,1.,0.866025403784439,1.,0.866025403784439,
1.,0.866025403784439,1.,0.866025403784439,1.,0.980312120051573,0.966410600022306)))
REPRESENTATION_ITEM('')
SURFACE()
);
#3175=(
BOUNDED_SURFACE()
B_SPLINE_SURFACE(1,2,((#252619,#252620,#252621,#252622,#252623,#252624,
#252625,#252626,#252627,#252628,#252629,#252630,#252631,#252632,#252633,
#252634,#252635,#252636,#252637,#252638,#252639,#252640,#252641,#252642,
#252643,#252644,#252645,#252646,#252647,#252648,#252649,#252650,#252651,
#252652,#252653,#252654,#252655,#252656,#252657,#252658,#252659,#252660,
#252661,#252662,#252663,#252664,#252665,#252666,#252667,#252668,#252669,
#252670,#252671,#252672,#252673,#252674,#252675,#252676,#252677,#252678,
#252679,#252680,#252681,#252682,#252683,#252684,#252685,#252686,#252687,
#252688,#252689,#252690,#252691,#252692,#252693,#252694,#252695,#252696,
#252697,#252698,#252699,#252700,#252701,#252702,#252703,#252704,#252705,
#252706,#252707,#252708,#252709,#252710,#252711,#252712,#252713,#252714,
#252715,#252716,#252717,#252718,#252719,#252720,#252721,#252722,#252723,
#252724,#252725,#252726,#252727,#252728,#252729,#252730,#252731,#252732,
#252733,#252734,#252735,#252736,#252737,#252738,#252739,#252740,#252741,
#252742,#252743,#252744,#252745,#252746,#252747,#252748,#252749,#252750,
#252751,#252752,#252753,#252754,#252755,#252756,#252757,#252758,#252759,
#252760,#252761,#252762,#252763,#252764,#252765,#252766,#252767,#252768,
#252769,#252770,#252771,#252772,#252773,#252774,#252775,#252776,#252777,
#252778,#252779,#252780,#252781,#252782,#252783,#252784,#252785,#252786,
#252787,#252788,#252789,#252790,#252791,#252792,#252793,#252794,#252795,
#252796,#252797,#252798,#252799,#252800,#252801,#252802,#252803,#252804,
#252805,#252806,#252807,#252808,#252809,#252810,#252811,#252812,#252813,
#252814,#252815,#252816,#252817,#252818,#252819,#252820,#252821,#252822,
#252823,#252824,#252825,#252826,#252827,#252828,#252829,#252830,#252831,
#252832,#252833,#252834,#252835,#252836,#252837,#252838,#252839,#252840,
#252841,#252842,#252843,#252844,#252845,#252846,#252847,#252848,#252849,
#252850,#252851,#252852,#252853,#252854,#252855,#252856,#252857,#252858,
#252859,#252860,#252861,#252862,#252863,#252864,#252865,#252866,#252867,
#252868,#252869,#252870,#252871,#252872,#252873,#252874,#252875,#252876,
#252877,#252878,#252879,#252880,#252881,#252882,#252883,#252884,#252885,
#252886,#252887,#252888,#252889,#252890,#252891,#252892,#252893,#252894,
#252895),(#252896,#252897,#252898,#252899,#252900,#252901,#252902,#252903,
#252904,#252905,#252906,#252907,#252908,#252909,#252910,#252911,#252912,
#252913,#252914,#252915,#252916,#252917,#252918,#252919,#252920,#252921,
#252922,#252923,#252924,#252925,#252926,#252927,#252928,#252929,#252930,
#252931,#252932,#252933,#252934,#252935,#252936,#252937,#252938,#252939,
#252940,#252941,#252942,#252943,#252944,#252945,#252946,#252947,#252948,
#252949,#252950,#252951,#252952,#252953,#252954,#252955,#252956,#252957,
#252958,#252959,#252960,#252961,#252962,#252963,#252964,#252965,#252966,
#252967,#252968,#252969,#252970,#252971,#252972,#252973,#252974,#252975,
#252976,#252977,#252978,#252979,#252980,#252981,#252982,#252983,#252984,
#252985,#252986,#252987,#252988,#252989,#252990,#252991,#252992,#252993,
#252994,#252995,#252996,#252997,#252998,#252999,#253000,#253001,#253002,
#253003,#253004,#253005,#253006,#253007,#253008,#253009,#253010,#253011,
#253012,#253013,#253014,#253015,#253016,#253017,#253018,#253019,#253020,
#253021,#253022,#253023,#253024,#253025,#253026,#253027,#253028,#253029,
#253030,#253031,#253032,#253033,#253034,#253035,#253036,#253037,#253038,
#253039,#253040,#253041,#253042,#253043,#253044,#253045,#253046,#253047,
#253048,#253049,#253050,#253051,#253052,#253053,#253054,#253055,#253056,
#253057,#253058,#253059,#253060,#253061,#253062,#253063,#253064,#253065,
#253066,#253067,#253068,#253069,#253070,#253071,#253072,#253073,#253074,
#253075,#253076,#253077,#253078,#253079,#253080,#253081,#253082,#253083,
#253084,#253085,#253086,#253087,#253088,#253089,#253090,#253091,#253092,
#253093,#253094,#253095,#253096,#253097,#253098,#253099,#253100,#253101,
#253102,#253103,#253104,#253105,#253106,#253107,#253108,#253109,#253110,
#253111,#253112,#253113,#253114,#253115,#253116,#253117,#253118,#253119,
#253120,#253121,#253122,#253123,#253124,#253125,#253126,#253127,#253128,
#253129,#253130,#253131,#253132,#253133,#253134,#253135,#253136,#253137,
#253138,#253139,#253140,#253141,#253142,#253143,#253144,#253145,#253146,
#253147,#253148,#253149,#253150,#253151,#253152,#253153,#253154,#253155,
#253156,#253157,#253158,#253159,#253160,#253161,#253162,#253163,#253164,
#253165,#253166,#253167,#253168,#253169,#253170,#253171,#253172)),
 .UNSPECIFIED.,.F.,.F.,.F.)
B_SPLINE_SURFACE_WITH_KNOTS((2,2),(3,2,2,2,2,2,2,2,2,2,2,2,2,2,2,2,2,2,
2,2,2,2,2,2,2,2,2,2,2,2,2,2,2,2,2,2,2,2,2,2,2,2,2,2,2,2,2,2,2,2,2,2,2,2,
2,2,2,2,2,2,2,2,2,2,2,2,2,2,2,2,2,2,2,2,2,2,2,2,2,2,2,2,2,2,2,2,2,2,2,2,
2,2,2,2,2,2,2,2,2,2,2,2,2,2,2,2,2,2,2,2,2,2,2,2,2,2,2,2,2,2,2,2,2,2,2,2,
2,2,2,2,2,2,2,2,2,2,2,2,3),(0.,1.00000048160228),(0.,0.0072463768115942,
0.0144927536231884,0.0217391304347826,0.0289855072463768,0.036231884057971,
0.0434782608695652,0.0507246376811594,0.0579710144927536,0.0652173913043478,
0.072463768115942,0.0797101449275362,0.0869565217391304,0.0942028985507246,
0.101449275362319,0.108695652173913,0.115942028985507,0.123188405797101,
0.130434782608696,0.13768115942029,0.144927536231884,0.152173913043478,
0.159420289855073,0.166666666666667,0.173913043478261,0.181159420289855,
0.18840579710145,0.195652173913044,0.202898550724637,0.210144927536232,
0.217391304347826,0.224637681159421,0.231884057971014,0.239130434782609,
0.246376811594203,0.253623188405797,0.260869565217392,0.268115942028985,
0.275362318840579,0.282608695652174,0.289855072463768,0.297101449275363,
0.304347826086956,0.31159420289855,0.318840579710145,0.326086956521739,
0.333333333333334,0.340579710144927,0.347826086956521,0.355072463768116,
0.36231884057971,0.369565217391304,0.376811594202899,0.384057971014493,
0.391304347826087,0.398550724637681,0.405797101449275,0.41304347826087,
0.420289855072463,0.427536231884058,0.434782608695652,0.442028985507247,
0.449275362318841,0.456521739130435,0.463768115942029,0.471014492753623,
0.478260869565218,0.485507246376812,0.492753623188406,0.5,0.507246376811594,
0.514492753623188,0.521739130434783,0.528985507246377,0.536231884057971,
0.543478260869565,0.550724637681159,0.557971014492754,0.565217391304348,
0.572463768115942,0.579710144927536,0.586956521739131,0.594202898550725,
0.601449275362319,0.608695652173913,0.615942028985507,0.623188405797101,
0.630434782608696,0.63768115942029,0.644927536231884,0.652173913043478,
0.659420289855073,0.666666666666667,0.673913043478261,0.681159420289855,
0.688405797101449,0.695652173913044,0.702898550724638,0.710144927536232,
0.717391304347826,0.72463768115942,0.731884057971015,0.739130434782609,
0.746376811594203,0.753623188405797,0.760869565217391,0.768115942028986,
0.77536231884058,0.782608695652174,0.789855072463768,0.797101449275362,
0.804347826086956,0.811594202898551,0.818840579710145,0.826086956521739,
0.833333333333333,0.840579710144928,0.847826086956522,0.855072463768116,
0.86231884057971,0.869565217391304,0.876811594202899,0.884057971014493,
0.891304347826087,0.898550724637681,0.905797101449275,0.91304347826087,
0.920289855072464,0.927536231884058,0.934782608695652,0.942028985507246,
0.94927536231884,0.956521739130435,0.963768115942029,0.971014492753623,
0.978260869565217,0.985507246376812,0.992753623188406,0.993818495192186),
 .UNSPECIFIED.)
GEOMETRIC_REPRESENTATION_ITEM()
RATIONAL_B_SPLINE_SURFACE(((1.,0.866025403784439,1.,0.866025403784439,1.,
0.866025403784439,1.,0.866025403784439,1.,0.866025403784439,1.,0.866025403784439,
1.,0.866025403784439,1.,0.866025403784439,1.,0.866025403784439,1.,0.866025403784439,
1.,0.866025403784439,1.,0.866025403784439,1.,0.866025403784439,1.,0.866025403784439,
1.,0.866025403784439,1.,0.866025403784439,1.,0.866025403784439,1.,0.866025403784439,
1.,0.866025403784439,1.,0.866025403784439,1.,0.866025403784439,1.,0.866025403784439,
1.,0.866025403784439,1.,0.866025403784439,1.,0.866025403784439,1.,0.866025403784439,
1.,0.866025403784439,1.,0.866025403784439,1.,0.866025403784439,1.,0.866025403784439,
1.,0.866025403784439,1.,0.866025403784439,1.,0.866025403784439,1.,0.866025403784439,
1.,0.866025403784439,1.,0.866025403784439,1.,0.866025403784439,1.,0.866025403784439,
1.,0.866025403784439,1.,0.866025403784439,1.,0.866025403784439,1.,0.866025403784439,
1.,0.866025403784439,1.,0.866025403784439,1.,0.866025403784439,1.,0.866025403784439,
1.,0.866025403784439,1.,0.866025403784439,1.,0.866025403784439,1.,0.866025403784439,
1.,0.866025403784439,1.,0.866025403784439,1.,0.866025403784439,1.,0.866025403784439,
1.,0.866025403784439,1.,0.866025403784439,1.,0.866025403784439,1.,0.866025403784439,
1.,0.866025403784439,1.,0.866025403784439,1.,0.866025403784439,1.,0.866025403784439,
1.,0.866025403784439,1.,0.866025403784439,1.,0.866025403784439,1.,0.866025403784439,
1.,0.866025403784439,1.,0.866025403784439,1.,0.866025403784439,1.,0.866025403784439,
1.,0.866025403784439,1.,0.866025403784439,1.,0.866025403784439,1.,0.866025403784439,
1.,0.866025403784439,1.,0.866025403784439,1.,0.866025403784439,1.,0.866025403784439,
1.,0.866025403784439,1.,0.866025403784439,1.,0.866025403784439,1.,0.866025403784439,
1.,0.866025403784439,1.,0.866025403784439,1.,0.866025403784439,1.,0.866025403784439,
1.,0.866025403784439,1.,0.866025403784439,1.,0.866025403784439,1.,0.866025403784439,
1.,0.866025403784439,1.,0.866025403784439,1.,0.866025403784439,1.,0.866025403784439,
1.,0.866025403784439,1.,0.866025403784439,1.,0.866025403784439,1.,0.866025403784439,
1.,0.866025403784439,1.,0.866025403784439,1.,0.866025403784439,1.,0.866025403784439,
1.,0.866025403784439,1.,0.866025403784439,1.,0.866025403784439,1.,0.866025403784439,
1.,0.866025403784439,1.,0.866025403784439,1.,0.866025403784439,1.,0.866025403784439,
1.,0.866025403784439,1.,0.866025403784439,1.,0.866025403784439,1.,0.866025403784439,
1.,0.866025403784439,1.,0.866025403784439,1.,0.866025403784439,1.,0.866025403784439,
1.,0.866025403784439,1.,0.866025403784439,1.,0.866025403784439,1.,0.866025403784439,
1.,0.866025403784439,1.,0.866025403784439,1.,0.866025403784439,1.,0.866025403784439,
1.,0.866025403784439,1.,0.866025403784439,1.,0.866025403784439,1.,0.866025403784439,
1.,0.866025403784439,1.,0.866025403784439,1.,0.866025403784439,1.,0.866025403784439,
1.,0.866025403784439,1.,0.866025403784439,1.,0.866025403784439,1.,0.980312120051573,
0.966410600022306),(1.,0.866025403784439,1.,0.866025403784439,1.,0.866025403784439,
1.,0.866025403784439,1.,0.866025403784439,1.,0.866025403784439,1.,0.866025403784439,
1.,0.866025403784439,1.,0.866025403784439,1.,0.866025403784439,1.,0.866025403784439,
1.,0.866025403784439,1.,0.866025403784439,1.,0.866025403784439,1.,0.866025403784439,
1.,0.866025403784439,1.,0.866025403784439,1.,0.866025403784439,1.,0.866025403784439,
1.,0.866025403784439,1.,0.866025403784439,1.,0.866025403784439,1.,0.866025403784439,
1.,0.866025403784439,1.,0.866025403784439,1.,0.866025403784439,1.,0.866025403784439,
1.,0.866025403784439,1.,0.866025403784439,1.,0.866025403784439,1.,0.866025403784439,
1.,0.866025403784439,1.,0.866025403784439,1.,0.866025403784439,1.,0.866025403784439,
1.,0.866025403784439,1.,0.866025403784439,1.,0.866025403784439,1.,0.866025403784439,
1.,0.866025403784439,1.,0.866025403784439,1.,0.866025403784439,1.,0.866025403784439,
1.,0.866025403784439,1.,0.866025403784439,1.,0.866025403784439,1.,0.866025403784439,
1.,0.866025403784439,1.,0.866025403784439,1.,0.866025403784439,1.,0.866025403784439,
1.,0.866025403784439,1.,0.866025403784439,1.,0.866025403784439,1.,0.866025403784439,
1.,0.866025403784439,1.,0.866025403784439,1.,0.866025403784439,1.,0.866025403784439,
1.,0.866025403784439,1.,0.866025403784439,1.,0.866025403784439,1.,0.866025403784439,
1.,0.866025403784439,1.,0.866025403784439,1.,0.866025403784439,1.,0.866025403784439,
1.,0.866025403784439,1.,0.866025403784439,1.,0.866025403784439,1.,0.866025403784439,
1.,0.866025403784439,1.,0.866025403784439,1.,0.866025403784439,1.,0.866025403784439,
1.,0.866025403784439,1.,0.866025403784439,1.,0.866025403784439,1.,0.866025403784439,
1.,0.866025403784439,1.,0.866025403784439,1.,0.866025403784439,1.,0.866025403784439,
1.,0.866025403784439,1.,0.866025403784439,1.,0.866025403784439,1.,0.866025403784439,
1.,0.866025403784439,1.,0.866025403784439,1.,0.866025403784439,1.,0.866025403784439,
1.,0.866025403784439,1.,0.866025403784439,1.,0.866025403784439,1.,0.866025403784439,
1.,0.866025403784439,1.,0.866025403784439,1.,0.866025403784439,1.,0.866025403784439,
1.,0.866025403784439,1.,0.866025403784439,1.,0.866025403784439,1.,0.866025403784439,
1.,0.866025403784439,1.,0.866025403784439,1.,0.866025403784439,1.,0.866025403784439,
1.,0.866025403784439,1.,0.866025403784439,1.,0.866025403784439,1.,0.866025403784439,
1.,0.866025403784439,1.,0.866025403784439,1.,0.866025403784439,1.,0.866025403784439,
1.,0.866025403784439,1.,0.866025403784439,1.,0.866025403784439,1.,0.866025403784439,
1.,0.866025403784439,1.,0.866025403784439,1.,0.866025403784439,1.,0.866025403784439,
1.,0.866025403784439,1.,0.866025403784439,1.,0.866025403784439,1.,0.866025403784439,
1.,0.866025403784439,1.,0.866025403784439,1.,0.866025403784439,1.,0.866025403784439,
1.,0.866025403784439,1.,0.866025403784439,1.,0.866025403784439,1.,0.866025403784439,
1.,0.866025403784439,1.,0.866025403784439,1.,0.980312120051573,0.966410600022306)))
REPRESENTATION_ITEM('')
SURFACE()
);
#3176=(
BOUNDED_SURFACE()
B_SPLINE_SURFACE(1,2,((#253229,#253230,#253231,#253232,#253233,#253234,
#253235,#253236,#253237,#253238,#253239,#253240,#253241,#253242,#253243,
#253244,#253245,#253246,#253247,#253248,#253249,#253250,#253251,#253252,
#253253,#253254,#253255,#253256,#253257,#253258,#253259,#253260,#253261,
#253262,#253263,#253264,#253265,#253266,#253267,#253268,#253269,#253270,
#253271,#253272,#253273,#253274,#253275,#253276,#253277,#253278,#253279,
#253280,#253281,#253282,#253283,#253284,#253285,#253286,#253287,#253288,
#253289,#253290,#253291,#253292,#253293,#253294,#253295,#253296,#253297,
#253298,#253299,#253300,#253301,#253302,#253303,#253304,#253305,#253306,
#253307,#253308,#253309,#253310,#253311,#253312,#253313,#253314,#253315,
#253316,#253317,#253318,#253319,#253320,#253321,#253322,#253323,#253324,
#253325,#253326,#253327,#253328,#253329,#253330,#253331,#253332,#253333,
#253334,#253335,#253336,#253337,#253338,#253339,#253340,#253341,#253342,
#253343,#253344,#253345,#253346,#253347,#253348,#253349,#253350,#253351,
#253352,#253353,#253354,#253355,#253356,#253357,#253358,#253359,#253360,
#253361,#253362,#253363,#253364,#253365,#253366,#253367,#253368,#253369,
#253370,#253371,#253372,#253373,#253374,#253375,#253376,#253377,#253378,
#253379,#253380,#253381,#253382,#253383,#253384,#253385,#253386,#253387,
#253388,#253389,#253390,#253391,#253392,#253393,#253394,#253395,#253396,
#253397,#253398,#253399,#253400,#253401,#253402,#253403,#253404,#253405,
#253406,#253407,#253408,#253409,#253410,#253411,#253412,#253413,#253414,
#253415,#253416,#253417,#253418,#253419,#253420,#253421,#253422,#253423,
#253424,#253425,#253426,#253427,#253428,#253429,#253430,#253431,#253432,
#253433,#253434,#253435,#253436,#253437,#253438,#253439,#253440,#253441,
#253442,#253443,#253444,#253445,#253446,#253447,#253448,#253449,#253450,
#253451,#253452,#253453,#253454,#253455,#253456,#253457,#253458,#253459,
#253460,#253461,#253462,#253463,#253464,#253465,#253466,#253467,#253468,
#253469,#253470,#253471,#253472,#253473,#253474,#253475,#253476,#253477,
#253478,#253479,#253480,#253481,#253482,#253483,#253484,#253485,#253486,
#253487,#253488,#253489,#253490,#253491,#253492,#253493,#253494,#253495,
#253496,#253497,#253498,#253499,#253500,#253501,#253502,#253503,#253504,
#253505),(#253506,#253507,#253508,#253509,#253510,#253511,#253512,#253513,
#253514,#253515,#253516,#253517,#253518,#253519,#253520,#253521,#253522,
#253523,#253524,#253525,#253526,#253527,#253528,#253529,#253530,#253531,
#253532,#253533,#253534,#253535,#253536,#253537,#253538,#253539,#253540,
#253541,#253542,#253543,#253544,#253545,#253546,#253547,#253548,#253549,
#253550,#253551,#253552,#253553,#253554,#253555,#253556,#253557,#253558,
#253559,#253560,#253561,#253562,#253563,#253564,#253565,#253566,#253567,
#253568,#253569,#253570,#253571,#253572,#253573,#253574,#253575,#253576,
#253577,#253578,#253579,#253580,#253581,#253582,#253583,#253584,#253585,
#253586,#253587,#253588,#253589,#253590,#253591,#253592,#253593,#253594,
#253595,#253596,#253597,#253598,#253599,#253600,#253601,#253602,#253603,
#253604,#253605,#253606,#253607,#253608,#253609,#253610,#253611,#253612,
#253613,#253614,#253615,#253616,#253617,#253618,#253619,#253620,#253621,
#253622,#253623,#253624,#253625,#253626,#253627,#253628,#253629,#253630,
#253631,#253632,#253633,#253634,#253635,#253636,#253637,#253638,#253639,
#253640,#253641,#253642,#253643,#253644,#253645,#253646,#253647,#253648,
#253649,#253650,#253651,#253652,#253653,#253654,#253655,#253656,#253657,
#253658,#253659,#253660,#253661,#253662,#253663,#253664,#253665,#253666,
#253667,#253668,#253669,#253670,#253671,#253672,#253673,#253674,#253675,
#253676,#253677,#253678,#253679,#253680,#253681,#253682,#253683,#253684,
#253685,#253686,#253687,#253688,#253689,#253690,#253691,#253692,#253693,
#253694,#253695,#253696,#253697,#253698,#253699,#253700,#253701,#253702,
#253703,#253704,#253705,#253706,#253707,#253708,#253709,#253710,#253711,
#253712,#253713,#253714,#253715,#253716,#253717,#253718,#253719,#253720,
#253721,#253722,#253723,#253724,#253725,#253726,#253727,#253728,#253729,
#253730,#253731,#253732,#253733,#253734,#253735,#253736,#253737,#253738,
#253739,#253740,#253741,#253742,#253743,#253744,#253745,#253746,#253747,
#253748,#253749,#253750,#253751,#253752,#253753,#253754,#253755,#253756,
#253757,#253758,#253759,#253760,#253761,#253762,#253763,#253764,#253765,
#253766,#253767,#253768,#253769,#253770,#253771,#253772,#253773,#253774,
#253775,#253776,#253777,#253778,#253779,#253780,#253781,#253782)),
 .UNSPECIFIED.,.F.,.F.,.F.)
B_SPLINE_SURFACE_WITH_KNOTS((2,2),(3,2,2,2,2,2,2,2,2,2,2,2,2,2,2,2,2,2,
2,2,2,2,2,2,2,2,2,2,2,2,2,2,2,2,2,2,2,2,2,2,2,2,2,2,2,2,2,2,2,2,2,2,2,2,
2,2,2,2,2,2,2,2,2,2,2,2,2,2,2,2,2,2,2,2,2,2,2,2,2,2,2,2,2,2,2,2,2,2,2,2,
2,2,2,2,2,2,2,2,2,2,2,2,2,2,2,2,2,2,2,2,2,2,2,2,2,2,2,2,2,2,2,2,2,2,2,2,
2,2,2,2,2,2,2,2,2,2,2,2,3),(0.,1.),(0.,0.0072463768115942,0.0144927536231884,
0.0217391304347826,0.0289855072463768,0.036231884057971,0.0434782608695652,
0.0507246376811594,0.0579710144927536,0.0652173913043478,0.072463768115942,
0.0797101449275362,0.0869565217391304,0.0942028985507246,0.101449275362319,
0.108695652173913,0.115942028985507,0.123188405797101,0.130434782608696,
0.13768115942029,0.144927536231884,0.152173913043478,0.159420289855073,
0.166666666666667,0.173913043478261,0.181159420289855,0.18840579710145,
0.195652173913044,0.202898550724637,0.210144927536232,0.217391304347826,
0.224637681159421,0.231884057971014,0.239130434782609,0.246376811594203,
0.253623188405797,0.260869565217392,0.268115942028985,0.275362318840579,
0.282608695652174,0.289855072463768,0.297101449275363,0.304347826086956,
0.31159420289855,0.318840579710145,0.326086956521739,0.333333333333334,
0.340579710144927,0.347826086956521,0.355072463768116,0.36231884057971,
0.369565217391304,0.376811594202899,0.384057971014493,0.391304347826087,
0.398550724637681,0.405797101449275,0.41304347826087,0.420289855072463,
0.427536231884058,0.434782608695652,0.442028985507247,0.449275362318841,
0.456521739130435,0.463768115942029,0.471014492753623,0.478260869565218,
0.485507246376812,0.492753623188406,0.5,0.507246376811594,0.514492753623188,
0.521739130434783,0.528985507246377,0.536231884057971,0.543478260869565,
0.550724637681159,0.557971014492754,0.565217391304348,0.572463768115942,
0.579710144927536,0.586956521739131,0.594202898550725,0.601449275362319,
0.608695652173913,0.615942028985507,0.623188405797101,0.630434782608696,
0.63768115942029,0.644927536231884,0.652173913043478,0.659420289855073,
0.666666666666667,0.673913043478261,0.681159420289855,0.688405797101449,
0.695652173913044,0.702898550724638,0.710144927536232,0.717391304347826,
0.72463768115942,0.731884057971015,0.739130434782609,0.746376811594203,
0.753623188405797,0.760869565217391,0.768115942028986,0.77536231884058,
0.782608695652174,0.789855072463768,0.797101449275362,0.804347826086956,
0.811594202898551,0.818840579710145,0.826086956521739,0.833333333333333,
0.840579710144928,0.847826086956522,0.855072463768116,0.86231884057971,
0.869565217391304,0.876811594202899,0.884057971014493,0.891304347826087,
0.898550724637681,0.905797101449275,0.91304347826087,0.920289855072464,
0.927536231884058,0.934782608695652,0.942028985507246,0.94927536231884,
0.956521739130435,0.963768115942029,0.971014492753623,0.978260869565217,
0.985507246376812,0.992753623188406,0.993818585798284),.UNSPECIFIED.)
GEOMETRIC_REPRESENTATION_ITEM()
RATIONAL_B_SPLINE_SURFACE(((1.,0.866025403784439,1.,0.866025403784439,1.,
0.866025403784439,1.,0.866025403784439,1.,0.866025403784439,1.,0.866025403784439,
1.,0.866025403784439,1.,0.866025403784439,1.,0.866025403784439,1.,0.866025403784439,
1.,0.866025403784439,1.,0.866025403784439,1.,0.866025403784439,1.,0.866025403784439,
1.,0.866025403784439,1.,0.866025403784439,1.,0.866025403784439,1.,0.866025403784439,
1.,0.866025403784439,1.,0.866025403784439,1.,0.866025403784439,1.,0.866025403784439,
1.,0.866025403784439,1.,0.866025403784439,1.,0.866025403784439,1.,0.866025403784439,
1.,0.866025403784439,1.,0.866025403784439,1.,0.866025403784439,1.,0.866025403784439,
1.,0.866025403784439,1.,0.866025403784439,1.,0.866025403784439,1.,0.866025403784439,
1.,0.866025403784439,1.,0.866025403784439,1.,0.866025403784439,1.,0.866025403784439,
1.,0.866025403784439,1.,0.866025403784439,1.,0.866025403784439,1.,0.866025403784439,
1.,0.866025403784439,1.,0.866025403784439,1.,0.866025403784439,1.,0.866025403784439,
1.,0.866025403784439,1.,0.866025403784439,1.,0.866025403784439,1.,0.866025403784439,
1.,0.866025403784439,1.,0.866025403784439,1.,0.866025403784439,1.,0.866025403784439,
1.,0.866025403784439,1.,0.866025403784439,1.,0.866025403784439,1.,0.866025403784439,
1.,0.866025403784439,1.,0.866025403784439,1.,0.866025403784439,1.,0.866025403784439,
1.,0.866025403784439,1.,0.866025403784439,1.,0.866025403784439,1.,0.866025403784439,
1.,0.866025403784439,1.,0.866025403784439,1.,0.866025403784439,1.,0.866025403784439,
1.,0.866025403784439,1.,0.866025403784439,1.,0.866025403784439,1.,0.866025403784439,
1.,0.866025403784439,1.,0.866025403784439,1.,0.866025403784439,1.,0.866025403784439,
1.,0.866025403784439,1.,0.866025403784439,1.,0.866025403784439,1.,0.866025403784439,
1.,0.866025403784439,1.,0.866025403784439,1.,0.866025403784439,1.,0.866025403784439,
1.,0.866025403784439,1.,0.866025403784439,1.,0.866025403784439,1.,0.866025403784439,
1.,0.866025403784439,1.,0.866025403784439,1.,0.866025403784439,1.,0.866025403784439,
1.,0.866025403784439,1.,0.866025403784439,1.,0.866025403784439,1.,0.866025403784439,
1.,0.866025403784439,1.,0.866025403784439,1.,0.866025403784439,1.,0.866025403784439,
1.,0.866025403784439,1.,0.866025403784439,1.,0.866025403784439,1.,0.866025403784439,
1.,0.866025403784439,1.,0.866025403784439,1.,0.866025403784439,1.,0.866025403784439,
1.,0.866025403784439,1.,0.866025403784439,1.,0.866025403784439,1.,0.866025403784439,
1.,0.866025403784439,1.,0.866025403784439,1.,0.866025403784439,1.,0.866025403784439,
1.,0.866025403784439,1.,0.866025403784439,1.,0.866025403784439,1.,0.866025403784439,
1.,0.866025403784439,1.,0.866025403784439,1.,0.866025403784439,1.,0.866025403784439,
1.,0.866025403784439,1.,0.866025403784439,1.,0.866025403784439,1.,0.866025403784439,
1.,0.866025403784439,1.,0.866025403784439,1.,0.866025403784439,1.,0.866025403784439,
1.,0.866025403784439,1.,0.866025403784439,1.,0.866025403784439,1.,0.98031044488126,
0.966408234404338),(1.,0.866025403784439,1.,0.866025403784439,1.,0.866025403784439,
1.,0.866025403784439,1.,0.866025403784439,1.,0.866025403784439,1.,0.866025403784439,
1.,0.866025403784439,1.,0.866025403784439,1.,0.866025403784439,1.,0.866025403784439,
1.,0.866025403784439,1.,0.866025403784439,1.,0.866025403784439,1.,0.866025403784439,
1.,0.866025403784439,1.,0.866025403784439,1.,0.866025403784439,1.,0.866025403784439,
1.,0.866025403784439,1.,0.866025403784439,1.,0.866025403784439,1.,0.866025403784439,
1.,0.866025403784439,1.,0.866025403784439,1.,0.866025403784439,1.,0.866025403784439,
1.,0.866025403784439,1.,0.866025403784439,1.,0.866025403784439,1.,0.866025403784439,
1.,0.866025403784439,1.,0.866025403784439,1.,0.866025403784439,1.,0.866025403784439,
1.,0.866025403784439,1.,0.866025403784439,1.,0.866025403784439,1.,0.866025403784439,
1.,0.866025403784439,1.,0.866025403784439,1.,0.866025403784439,1.,0.866025403784439,
1.,0.866025403784439,1.,0.866025403784439,1.,0.866025403784439,1.,0.866025403784439,
1.,0.866025403784439,1.,0.866025403784439,1.,0.866025403784439,1.,0.866025403784439,
1.,0.866025403784439,1.,0.866025403784439,1.,0.866025403784439,1.,0.866025403784439,
1.,0.866025403784439,1.,0.866025403784439,1.,0.866025403784439,1.,0.866025403784439,
1.,0.866025403784439,1.,0.866025403784439,1.,0.866025403784439,1.,0.866025403784439,
1.,0.866025403784439,1.,0.866025403784439,1.,0.866025403784439,1.,0.866025403784439,
1.,0.866025403784439,1.,0.866025403784439,1.,0.866025403784439,1.,0.866025403784439,
1.,0.866025403784439,1.,0.866025403784439,1.,0.866025403784439,1.,0.866025403784439,
1.,0.866025403784439,1.,0.866025403784439,1.,0.866025403784439,1.,0.866025403784439,
1.,0.866025403784439,1.,0.866025403784439,1.,0.866025403784439,1.,0.866025403784439,
1.,0.866025403784439,1.,0.866025403784439,1.,0.866025403784439,1.,0.866025403784439,
1.,0.866025403784439,1.,0.866025403784439,1.,0.866025403784439,1.,0.866025403784439,
1.,0.866025403784439,1.,0.866025403784439,1.,0.866025403784439,1.,0.866025403784439,
1.,0.866025403784439,1.,0.866025403784439,1.,0.866025403784439,1.,0.866025403784439,
1.,0.866025403784439,1.,0.866025403784439,1.,0.866025403784439,1.,0.866025403784439,
1.,0.866025403784439,1.,0.866025403784439,1.,0.866025403784439,1.,0.866025403784439,
1.,0.866025403784439,1.,0.866025403784439,1.,0.866025403784439,1.,0.866025403784439,
1.,0.866025403784439,1.,0.866025403784439,1.,0.866025403784439,1.,0.866025403784439,
1.,0.866025403784439,1.,0.866025403784439,1.,0.866025403784439,1.,0.866025403784439,
1.,0.866025403784439,1.,0.866025403784439,1.,0.866025403784439,1.,0.866025403784439,
1.,0.866025403784439,1.,0.866025403784439,1.,0.866025403784439,1.,0.866025403784439,
1.,0.866025403784439,1.,0.866025403784439,1.,0.866025403784439,1.,0.866025403784439,
1.,0.866025403784439,1.,0.866025403784439,1.,0.866025403784439,1.,0.866025403784439,
1.,0.866025403784439,1.,0.866025403784439,1.,0.98031044488126,0.966408234404338)))
REPRESENTATION_ITEM('')
SURFACE()
);
#3177=(
BOUNDED_SURFACE()
B_SPLINE_SURFACE(1,2,((#253816,#253817,#253818,#253819,#253820,#253821,
#253822,#253823,#253824,#253825,#253826,#253827,#253828,#253829,#253830,
#253831,#253832,#253833,#253834,#253835,#253836,#253837,#253838,#253839,
#253840,#253841,#253842,#253843,#253844,#253845,#253846,#253847,#253848,
#253849,#253850,#253851,#253852,#253853,#253854,#253855,#253856,#253857,
#253858,#253859,#253860,#253861,#253862,#253863,#253864,#253865,#253866,
#253867,#253868,#253869,#253870,#253871,#253872,#253873,#253874,#253875,
#253876,#253877,#253878,#253879,#253880,#253881,#253882,#253883,#253884,
#253885,#253886,#253887,#253888,#253889,#253890,#253891,#253892,#253893,
#253894,#253895,#253896,#253897,#253898,#253899,#253900,#253901,#253902,
#253903,#253904,#253905,#253906,#253907,#253908,#253909,#253910,#253911,
#253912,#253913,#253914,#253915,#253916,#253917,#253918,#253919,#253920,
#253921,#253922,#253923,#253924,#253925,#253926,#253927,#253928,#253929,
#253930,#253931,#253932,#253933,#253934,#253935,#253936,#253937,#253938,
#253939,#253940,#253941,#253942,#253943,#253944,#253945,#253946,#253947,
#253948,#253949,#253950,#253951,#253952,#253953,#253954,#253955,#253956,
#253957,#253958,#253959,#253960,#253961,#253962,#253963,#253964,#253965,
#253966,#253967,#253968,#253969,#253970,#253971,#253972,#253973,#253974,
#253975,#253976,#253977,#253978,#253979,#253980,#253981,#253982,#253983,
#253984,#253985,#253986,#253987,#253988,#253989,#253990,#253991,#253992,
#253993,#253994,#253995,#253996,#253997,#253998,#253999,#254000,#254001,
#254002,#254003,#254004,#254005,#254006,#254007,#254008,#254009,#254010,
#254011,#254012,#254013,#254014,#254015,#254016,#254017,#254018,#254019,
#254020,#254021,#254022,#254023,#254024,#254025,#254026,#254027,#254028,
#254029,#254030,#254031,#254032,#254033,#254034,#254035,#254036,#254037,
#254038,#254039,#254040,#254041,#254042,#254043,#254044,#254045,#254046,
#254047,#254048,#254049,#254050,#254051,#254052,#254053,#254054,#254055,
#254056,#254057,#254058,#254059,#254060,#254061,#254062,#254063,#254064,
#254065,#254066,#254067,#254068,#254069,#254070,#254071,#254072,#254073,
#254074,#254075,#254076,#254077,#254078,#254079,#254080,#254081,#254082,
#254083,#254084,#254085,#254086,#254087,#254088,#254089,#254090,#254091,
#254092),(#254093,#254094,#254095,#254096,#254097,#254098,#254099,#254100,
#254101,#254102,#254103,#254104,#254105,#254106,#254107,#254108,#254109,
#254110,#254111,#254112,#254113,#254114,#254115,#254116,#254117,#254118,
#254119,#254120,#254121,#254122,#254123,#254124,#254125,#254126,#254127,
#254128,#254129,#254130,#254131,#254132,#254133,#254134,#254135,#254136,
#254137,#254138,#254139,#254140,#254141,#254142,#254143,#254144,#254145,
#254146,#254147,#254148,#254149,#254150,#254151,#254152,#254153,#254154,
#254155,#254156,#254157,#254158,#254159,#254160,#254161,#254162,#254163,
#254164,#254165,#254166,#254167,#254168,#254169,#254170,#254171,#254172,
#254173,#254174,#254175,#254176,#254177,#254178,#254179,#254180,#254181,
#254182,#254183,#254184,#254185,#254186,#254187,#254188,#254189,#254190,
#254191,#254192,#254193,#254194,#254195,#254196,#254197,#254198,#254199,
#254200,#254201,#254202,#254203,#254204,#254205,#254206,#254207,#254208,
#254209,#254210,#254211,#254212,#254213,#254214,#254215,#254216,#254217,
#254218,#254219,#254220,#254221,#254222,#254223,#254224,#254225,#254226,
#254227,#254228,#254229,#254230,#254231,#254232,#254233,#254234,#254235,
#254236,#254237,#254238,#254239,#254240,#254241,#254242,#254243,#254244,
#254245,#254246,#254247,#254248,#254249,#254250,#254251,#254252,#254253,
#254254,#254255,#254256,#254257,#254258,#254259,#254260,#254261,#254262,
#254263,#254264,#254265,#254266,#254267,#254268,#254269,#254270,#254271,
#254272,#254273,#254274,#254275,#254276,#254277,#254278,#254279,#254280,
#254281,#254282,#254283,#254284,#254285,#254286,#254287,#254288,#254289,
#254290,#254291,#254292,#254293,#254294,#254295,#254296,#254297,#254298,
#254299,#254300,#254301,#254302,#254303,#254304,#254305,#254306,#254307,
#254308,#254309,#254310,#254311,#254312,#254313,#254314,#254315,#254316,
#254317,#254318,#254319,#254320,#254321,#254322,#254323,#254324,#254325,
#254326,#254327,#254328,#254329,#254330,#254331,#254332,#254333,#254334,
#254335,#254336,#254337,#254338,#254339,#254340,#254341,#254342,#254343,
#254344,#254345,#254346,#254347,#254348,#254349,#254350,#254351,#254352,
#254353,#254354,#254355,#254356,#254357,#254358,#254359,#254360,#254361,
#254362,#254363,#254364,#254365,#254366,#254367,#254368,#254369)),
 .UNSPECIFIED.,.F.,.F.,.F.)
B_SPLINE_SURFACE_WITH_KNOTS((2,2),(3,2,2,2,2,2,2,2,2,2,2,2,2,2,2,2,2,2,
2,2,2,2,2,2,2,2,2,2,2,2,2,2,2,2,2,2,2,2,2,2,2,2,2,2,2,2,2,2,2,2,2,2,2,2,
2,2,2,2,2,2,2,2,2,2,2,2,2,2,2,2,2,2,2,2,2,2,2,2,2,2,2,2,2,2,2,2,2,2,2,2,
2,2,2,2,2,2,2,2,2,2,2,2,2,2,2,2,2,2,2,2,2,2,2,2,2,2,2,2,2,2,2,2,2,2,2,2,
2,2,2,2,2,2,2,2,2,2,2,2,3),(0.,1.),(0.,0.0072463768115942,0.0144927536231884,
0.0217391304347826,0.0289855072463768,0.036231884057971,0.0434782608695652,
0.0507246376811594,0.0579710144927536,0.0652173913043478,0.072463768115942,
0.0797101449275362,0.0869565217391304,0.0942028985507246,0.101449275362319,
0.108695652173913,0.115942028985507,0.123188405797101,0.130434782608696,
0.13768115942029,0.144927536231884,0.152173913043478,0.159420289855073,
0.166666666666667,0.173913043478261,0.181159420289855,0.18840579710145,
0.195652173913044,0.202898550724637,0.210144927536232,0.217391304347826,
0.224637681159421,0.231884057971014,0.239130434782609,0.246376811594203,
0.253623188405797,0.260869565217392,0.268115942028985,0.275362318840579,
0.282608695652174,0.289855072463768,0.297101449275363,0.304347826086956,
0.31159420289855,0.318840579710145,0.326086956521739,0.333333333333334,
0.340579710144927,0.347826086956521,0.355072463768116,0.36231884057971,
0.369565217391304,0.376811594202899,0.384057971014493,0.391304347826087,
0.398550724637681,0.405797101449275,0.41304347826087,0.420289855072463,
0.427536231884058,0.434782608695652,0.442028985507247,0.449275362318841,
0.456521739130435,0.463768115942029,0.471014492753623,0.478260869565218,
0.485507246376812,0.492753623188406,0.5,0.507246376811594,0.514492753623188,
0.521739130434783,0.528985507246377,0.536231884057971,0.543478260869565,
0.550724637681159,0.557971014492754,0.565217391304348,0.572463768115942,
0.579710144927536,0.586956521739131,0.594202898550725,0.601449275362319,
0.608695652173913,0.615942028985507,0.623188405797101,0.630434782608696,
0.63768115942029,0.644927536231884,0.652173913043478,0.659420289855073,
0.666666666666667,0.673913043478261,0.681159420289855,0.688405797101449,
0.695652173913044,0.702898550724638,0.710144927536232,0.717391304347826,
0.72463768115942,0.731884057971015,0.739130434782609,0.746376811594203,
0.753623188405797,0.760869565217391,0.768115942028986,0.77536231884058,
0.782608695652174,0.789855072463768,0.797101449275362,0.804347826086956,
0.811594202898551,0.818840579710145,0.826086956521739,0.833333333333333,
0.840579710144928,0.847826086956522,0.855072463768116,0.86231884057971,
0.869565217391304,0.876811594202899,0.884057971014493,0.891304347826087,
0.898550724637681,0.905797101449275,0.91304347826087,0.920289855072464,
0.927536231884058,0.934782608695652,0.942028985507246,0.94927536231884,
0.956521739130435,0.963768115942029,0.971014492753623,0.978260869565217,
0.985507246376812,0.992753623188406,0.993818585798284),.UNSPECIFIED.)
GEOMETRIC_REPRESENTATION_ITEM()
RATIONAL_B_SPLINE_SURFACE(((1.,0.866025403784439,1.,0.866025403784439,1.,
0.866025403784439,1.,0.866025403784439,1.,0.866025403784439,1.,0.866025403784439,
1.,0.866025403784439,1.,0.866025403784439,1.,0.866025403784439,1.,0.866025403784439,
1.,0.866025403784439,1.,0.866025403784439,1.,0.866025403784439,1.,0.866025403784439,
1.,0.866025403784439,1.,0.866025403784439,1.,0.866025403784439,1.,0.866025403784439,
1.,0.866025403784439,1.,0.866025403784439,1.,0.866025403784439,1.,0.866025403784439,
1.,0.866025403784439,1.,0.866025403784439,1.,0.866025403784439,1.,0.866025403784439,
1.,0.866025403784439,1.,0.866025403784439,1.,0.866025403784439,1.,0.866025403784439,
1.,0.866025403784439,1.,0.866025403784439,1.,0.866025403784439,1.,0.866025403784439,
1.,0.866025403784439,1.,0.866025403784439,1.,0.866025403784439,1.,0.866025403784439,
1.,0.866025403784439,1.,0.866025403784439,1.,0.866025403784439,1.,0.866025403784439,
1.,0.866025403784439,1.,0.866025403784439,1.,0.866025403784439,1.,0.866025403784439,
1.,0.866025403784439,1.,0.866025403784439,1.,0.866025403784439,1.,0.866025403784439,
1.,0.866025403784439,1.,0.866025403784439,1.,0.866025403784439,1.,0.866025403784439,
1.,0.866025403784439,1.,0.866025403784439,1.,0.866025403784439,1.,0.866025403784439,
1.,0.866025403784439,1.,0.866025403784439,1.,0.866025403784439,1.,0.866025403784439,
1.,0.866025403784439,1.,0.866025403784439,1.,0.866025403784439,1.,0.866025403784439,
1.,0.866025403784439,1.,0.866025403784439,1.,0.866025403784439,1.,0.866025403784439,
1.,0.866025403784439,1.,0.866025403784439,1.,0.866025403784439,1.,0.866025403784439,
1.,0.866025403784439,1.,0.866025403784439,1.,0.866025403784439,1.,0.866025403784439,
1.,0.866025403784439,1.,0.866025403784439,1.,0.866025403784439,1.,0.866025403784439,
1.,0.866025403784439,1.,0.866025403784439,1.,0.866025403784439,1.,0.866025403784439,
1.,0.866025403784439,1.,0.866025403784439,1.,0.866025403784439,1.,0.866025403784439,
1.,0.866025403784439,1.,0.866025403784439,1.,0.866025403784439,1.,0.866025403784439,
1.,0.866025403784439,1.,0.866025403784439,1.,0.866025403784439,1.,0.866025403784439,
1.,0.866025403784439,1.,0.866025403784439,1.,0.866025403784439,1.,0.866025403784439,
1.,0.866025403784439,1.,0.866025403784439,1.,0.866025403784439,1.,0.866025403784439,
1.,0.866025403784439,1.,0.866025403784439,1.,0.866025403784439,1.,0.866025403784439,
1.,0.866025403784439,1.,0.866025403784439,1.,0.866025403784439,1.,0.866025403784439,
1.,0.866025403784439,1.,0.866025403784439,1.,0.866025403784439,1.,0.866025403784439,
1.,0.866025403784439,1.,0.866025403784439,1.,0.866025403784439,1.,0.866025403784439,
1.,0.866025403784439,1.,0.866025403784439,1.,0.866025403784439,1.,0.866025403784439,
1.,0.866025403784439,1.,0.866025403784439,1.,0.866025403784439,1.,0.866025403784439,
1.,0.866025403784439,1.,0.866025403784439,1.,0.866025403784439,1.,0.866025403784439,
1.,0.866025403784439,1.,0.866025403784439,1.,0.866025403784439,1.,0.98031044488126,
0.966408234404338),(1.,0.866025403784439,1.,0.866025403784439,1.,0.866025403784439,
1.,0.866025403784439,1.,0.866025403784439,1.,0.866025403784439,1.,0.866025403784439,
1.,0.866025403784439,1.,0.866025403784439,1.,0.866025403784439,1.,0.866025403784439,
1.,0.866025403784439,1.,0.866025403784439,1.,0.866025403784439,1.,0.866025403784439,
1.,0.866025403784439,1.,0.866025403784439,1.,0.866025403784439,1.,0.866025403784439,
1.,0.866025403784439,1.,0.866025403784439,1.,0.866025403784439,1.,0.866025403784439,
1.,0.866025403784439,1.,0.866025403784439,1.,0.866025403784439,1.,0.866025403784439,
1.,0.866025403784439,1.,0.866025403784439,1.,0.866025403784439,1.,0.866025403784439,
1.,0.866025403784439,1.,0.866025403784439,1.,0.866025403784439,1.,0.866025403784439,
1.,0.866025403784439,1.,0.866025403784439,1.,0.866025403784439,1.,0.866025403784439,
1.,0.866025403784439,1.,0.866025403784439,1.,0.866025403784439,1.,0.866025403784439,
1.,0.866025403784439,1.,0.866025403784439,1.,0.866025403784439,1.,0.866025403784439,
1.,0.866025403784439,1.,0.866025403784439,1.,0.866025403784439,1.,0.866025403784439,
1.,0.866025403784439,1.,0.866025403784439,1.,0.866025403784439,1.,0.866025403784439,
1.,0.866025403784439,1.,0.866025403784439,1.,0.866025403784439,1.,0.866025403784439,
1.,0.866025403784439,1.,0.866025403784439,1.,0.866025403784439,1.,0.866025403784439,
1.,0.866025403784439,1.,0.866025403784439,1.,0.866025403784439,1.,0.866025403784439,
1.,0.866025403784439,1.,0.866025403784439,1.,0.866025403784439,1.,0.866025403784439,
1.,0.866025403784439,1.,0.866025403784439,1.,0.866025403784439,1.,0.866025403784439,
1.,0.866025403784439,1.,0.866025403784439,1.,0.866025403784439,1.,0.866025403784439,
1.,0.866025403784439,1.,0.866025403784439,1.,0.866025403784439,1.,0.866025403784439,
1.,0.866025403784439,1.,0.866025403784439,1.,0.866025403784439,1.,0.866025403784439,
1.,0.866025403784439,1.,0.866025403784439,1.,0.866025403784439,1.,0.866025403784439,
1.,0.866025403784439,1.,0.866025403784439,1.,0.866025403784439,1.,0.866025403784439,
1.,0.866025403784439,1.,0.866025403784439,1.,0.866025403784439,1.,0.866025403784439,
1.,0.866025403784439,1.,0.866025403784439,1.,0.866025403784439,1.,0.866025403784439,
1.,0.866025403784439,1.,0.866025403784439,1.,0.866025403784439,1.,0.866025403784439,
1.,0.866025403784439,1.,0.866025403784439,1.,0.866025403784439,1.,0.866025403784439,
1.,0.866025403784439,1.,0.866025403784439,1.,0.866025403784439,1.,0.866025403784439,
1.,0.866025403784439,1.,0.866025403784439,1.,0.866025403784439,1.,0.866025403784439,
1.,0.866025403784439,1.,0.866025403784439,1.,0.866025403784439,1.,0.866025403784439,
1.,0.866025403784439,1.,0.866025403784439,1.,0.866025403784439,1.,0.866025403784439,
1.,0.866025403784439,1.,0.866025403784439,1.,0.866025403784439,1.,0.866025403784439,
1.,0.866025403784439,1.,0.866025403784439,1.,0.866025403784439,1.,0.866025403784439,
1.,0.866025403784439,1.,0.866025403784439,1.,0.98031044488126,0.966408234404338)))
REPRESENTATION_ITEM('')
SURFACE()
);
#3178=(
BOUNDED_SURFACE()
B_SPLINE_SURFACE(1,2,((#256166,#256167,#256168,#256169,#256170,#256171,
#256172,#256173,#256174,#256175,#256176,#256177,#256178,#256179,#256180,
#256181,#256182,#256183,#256184,#256185,#256186,#256187,#256188,#256189,
#256190,#256191,#256192,#256193,#256194,#256195,#256196,#256197,#256198,
#256199,#256200,#256201,#256202,#256203,#256204,#256205,#256206,#256207,
#256208,#256209,#256210,#256211,#256212,#256213,#256214,#256215,#256216,
#256217,#256218,#256219,#256220,#256221,#256222,#256223,#256224,#256225,
#256226,#256227,#256228,#256229,#256230,#256231,#256232,#256233,#256234,
#256235,#256236,#256237,#256238,#256239,#256240,#256241,#256242,#256243,
#256244,#256245,#256246,#256247,#256248,#256249,#256250,#256251,#256252,
#256253,#256254,#256255,#256256,#256257,#256258,#256259,#256260,#256261,
#256262,#256263,#256264,#256265,#256266,#256267,#256268,#256269,#256270,
#256271,#256272,#256273,#256274,#256275,#256276,#256277,#256278,#256279,
#256280,#256281,#256282,#256283,#256284,#256285,#256286,#256287,#256288,
#256289,#256290,#256291,#256292,#256293,#256294,#256295,#256296,#256297,
#256298,#256299,#256300,#256301,#256302,#256303,#256304,#256305,#256306,
#256307,#256308,#256309,#256310,#256311,#256312,#256313,#256314,#256315,
#256316,#256317,#256318,#256319,#256320,#256321,#256322,#256323,#256324,
#256325,#256326,#256327,#256328,#256329,#256330,#256331,#256332,#256333,
#256334,#256335,#256336,#256337,#256338,#256339,#256340,#256341,#256342,
#256343,#256344,#256345,#256346,#256347,#256348,#256349,#256350,#256351,
#256352,#256353,#256354,#256355,#256356,#256357,#256358,#256359,#256360,
#256361,#256362,#256363,#256364,#256365,#256366,#256367,#256368,#256369,
#256370,#256371,#256372,#256373,#256374,#256375,#256376,#256377,#256378,
#256379,#256380,#256381,#256382,#256383,#256384,#256385,#256386,#256387,
#256388,#256389,#256390,#256391,#256392,#256393,#256394,#256395,#256396,
#256397,#256398,#256399,#256400,#256401,#256402,#256403,#256404,#256405,
#256406,#256407,#256408,#256409,#256410,#256411,#256412,#256413,#256414,
#256415,#256416,#256417,#256418,#256419,#256420,#256421,#256422,#256423,
#256424,#256425,#256426,#256427,#256428,#256429,#256430,#256431,#256432,
#256433,#256434,#256435,#256436,#256437,#256438,#256439,#256440,#256441,
#256442),(#256443,#256444,#256445,#256446,#256447,#256448,#256449,#256450,
#256451,#256452,#256453,#256454,#256455,#256456,#256457,#256458,#256459,
#256460,#256461,#256462,#256463,#256464,#256465,#256466,#256467,#256468,
#256469,#256470,#256471,#256472,#256473,#256474,#256475,#256476,#256477,
#256478,#256479,#256480,#256481,#256482,#256483,#256484,#256485,#256486,
#256487,#256488,#256489,#256490,#256491,#256492,#256493,#256494,#256495,
#256496,#256497,#256498,#256499,#256500,#256501,#256502,#256503,#256504,
#256505,#256506,#256507,#256508,#256509,#256510,#256511,#256512,#256513,
#256514,#256515,#256516,#256517,#256518,#256519,#256520,#256521,#256522,
#256523,#256524,#256525,#256526,#256527,#256528,#256529,#256530,#256531,
#256532,#256533,#256534,#256535,#256536,#256537,#256538,#256539,#256540,
#256541,#256542,#256543,#256544,#256545,#256546,#256547,#256548,#256549,
#256550,#256551,#256552,#256553,#256554,#256555,#256556,#256557,#256558,
#256559,#256560,#256561,#256562,#256563,#256564,#256565,#256566,#256567,
#256568,#256569,#256570,#256571,#256572,#256573,#256574,#256575,#256576,
#256577,#256578,#256579,#256580,#256581,#256582,#256583,#256584,#256585,
#256586,#256587,#256588,#256589,#256590,#256591,#256592,#256593,#256594,
#256595,#256596,#256597,#256598,#256599,#256600,#256601,#256602,#256603,
#256604,#256605,#256606,#256607,#256608,#256609,#256610,#256611,#256612,
#256613,#256614,#256615,#256616,#256617,#256618,#256619,#256620,#256621,
#256622,#256623,#256624,#256625,#256626,#256627,#256628,#256629,#256630,
#256631,#256632,#256633,#256634,#256635,#256636,#256637,#256638,#256639,
#256640,#256641,#256642,#256643,#256644,#256645,#256646,#256647,#256648,
#256649,#256650,#256651,#256652,#256653,#256654,#256655,#256656,#256657,
#256658,#256659,#256660,#256661,#256662,#256663,#256664,#256665,#256666,
#256667,#256668,#256669,#256670,#256671,#256672,#256673,#256674,#256675,
#256676,#256677,#256678,#256679,#256680,#256681,#256682,#256683,#256684,
#256685,#256686,#256687,#256688,#256689,#256690,#256691,#256692,#256693,
#256694,#256695,#256696,#256697,#256698,#256699,#256700,#256701,#256702,
#256703,#256704,#256705,#256706,#256707,#256708,#256709,#256710,#256711,
#256712,#256713,#256714,#256715,#256716,#256717,#256718,#256719)),
 .UNSPECIFIED.,.F.,.F.,.F.)
B_SPLINE_SURFACE_WITH_KNOTS((2,2),(3,2,2,2,2,2,2,2,2,2,2,2,2,2,2,2,2,2,
2,2,2,2,2,2,2,2,2,2,2,2,2,2,2,2,2,2,2,2,2,2,2,2,2,2,2,2,2,2,2,2,2,2,2,2,
2,2,2,2,2,2,2,2,2,2,2,2,2,2,2,2,2,2,2,2,2,2,2,2,2,2,2,2,2,2,2,2,2,2,2,2,
2,2,2,2,2,2,2,2,2,2,2,2,2,2,2,2,2,2,2,2,2,2,2,2,2,2,2,2,2,2,2,2,2,2,2,2,
2,2,2,2,2,2,2,2,2,2,2,2,3),(0.,1.),(0.,0.0072463768115942,0.0144927536231884,
0.0217391304347826,0.0289855072463768,0.036231884057971,0.0434782608695652,
0.0507246376811594,0.0579710144927536,0.0652173913043478,0.072463768115942,
0.0797101449275362,0.0869565217391304,0.0942028985507246,0.101449275362319,
0.108695652173913,0.115942028985507,0.123188405797101,0.130434782608696,
0.13768115942029,0.144927536231884,0.152173913043478,0.159420289855073,
0.166666666666667,0.173913043478261,0.181159420289855,0.18840579710145,
0.195652173913044,0.202898550724637,0.210144927536232,0.217391304347826,
0.224637681159421,0.231884057971014,0.239130434782609,0.246376811594203,
0.253623188405797,0.260869565217392,0.268115942028985,0.275362318840579,
0.282608695652174,0.289855072463768,0.297101449275363,0.304347826086956,
0.31159420289855,0.318840579710145,0.326086956521739,0.333333333333334,
0.340579710144927,0.347826086956521,0.355072463768116,0.36231884057971,
0.369565217391304,0.376811594202899,0.384057971014493,0.391304347826087,
0.398550724637681,0.405797101449275,0.41304347826087,0.420289855072463,
0.427536231884058,0.434782608695652,0.442028985507247,0.449275362318841,
0.456521739130435,0.463768115942029,0.471014492753623,0.478260869565218,
0.485507246376812,0.492753623188406,0.5,0.507246376811594,0.514492753623188,
0.521739130434783,0.528985507246377,0.536231884057971,0.543478260869565,
0.550724637681159,0.557971014492754,0.565217391304348,0.572463768115942,
0.579710144927536,0.586956521739131,0.594202898550725,0.601449275362319,
0.608695652173913,0.615942028985507,0.623188405797101,0.630434782608696,
0.63768115942029,0.644927536231884,0.652173913043478,0.659420289855073,
0.666666666666667,0.673913043478261,0.681159420289855,0.688405797101449,
0.695652173913044,0.702898550724638,0.710144927536232,0.717391304347826,
0.72463768115942,0.731884057971015,0.739130434782609,0.746376811594203,
0.753623188405797,0.760869565217391,0.768115942028986,0.77536231884058,
0.782608695652174,0.789855072463768,0.797101449275362,0.804347826086956,
0.811594202898551,0.818840579710145,0.826086956521739,0.833333333333333,
0.840579710144928,0.847826086956522,0.855072463768116,0.86231884057971,
0.869565217391304,0.876811594202899,0.884057971014493,0.891304347826087,
0.898550724637681,0.905797101449275,0.91304347826087,0.920289855072464,
0.927536231884058,0.934782608695652,0.942028985507246,0.94927536231884,
0.956521739130435,0.963768115942029,0.971014492753623,0.978260869565217,
0.985507246376812,0.992753623188406,0.993818495192186),.UNSPECIFIED.)
GEOMETRIC_REPRESENTATION_ITEM()
RATIONAL_B_SPLINE_SURFACE(((1.,0.866025403784439,1.,0.866025403784439,1.,
0.866025403784439,1.,0.866025403784439,1.,0.866025403784439,1.,0.866025403784439,
1.,0.866025403784439,1.,0.866025403784439,1.,0.866025403784439,1.,0.866025403784439,
1.,0.866025403784439,1.,0.866025403784439,1.,0.866025403784439,1.,0.866025403784439,
1.,0.866025403784439,1.,0.866025403784439,1.,0.866025403784439,1.,0.866025403784439,
1.,0.866025403784439,1.,0.866025403784439,1.,0.866025403784439,1.,0.866025403784439,
1.,0.866025403784439,1.,0.866025403784439,1.,0.866025403784439,1.,0.866025403784439,
1.,0.866025403784439,1.,0.866025403784439,1.,0.866025403784439,1.,0.866025403784439,
1.,0.866025403784439,1.,0.866025403784439,1.,0.866025403784439,1.,0.866025403784439,
1.,0.866025403784439,1.,0.866025403784439,1.,0.866025403784439,1.,0.866025403784439,
1.,0.866025403784439,1.,0.866025403784439,1.,0.866025403784439,1.,0.866025403784439,
1.,0.866025403784439,1.,0.866025403784439,1.,0.866025403784439,1.,0.866025403784439,
1.,0.866025403784439,1.,0.866025403784439,1.,0.866025403784439,1.,0.866025403784439,
1.,0.866025403784439,1.,0.866025403784439,1.,0.866025403784439,1.,0.866025403784439,
1.,0.866025403784439,1.,0.866025403784439,1.,0.866025403784439,1.,0.866025403784439,
1.,0.866025403784439,1.,0.866025403784439,1.,0.866025403784439,1.,0.866025403784439,
1.,0.866025403784439,1.,0.866025403784439,1.,0.866025403784439,1.,0.866025403784439,
1.,0.866025403784439,1.,0.866025403784439,1.,0.866025403784439,1.,0.866025403784439,
1.,0.866025403784439,1.,0.866025403784439,1.,0.866025403784439,1.,0.866025403784439,
1.,0.866025403784439,1.,0.866025403784439,1.,0.866025403784439,1.,0.866025403784439,
1.,0.866025403784439,1.,0.866025403784439,1.,0.866025403784439,1.,0.866025403784439,
1.,0.866025403784439,1.,0.866025403784439,1.,0.866025403784439,1.,0.866025403784439,
1.,0.866025403784439,1.,0.866025403784439,1.,0.866025403784439,1.,0.866025403784439,
1.,0.866025403784439,1.,0.866025403784439,1.,0.866025403784439,1.,0.866025403784439,
1.,0.866025403784439,1.,0.866025403784439,1.,0.866025403784439,1.,0.866025403784439,
1.,0.866025403784439,1.,0.866025403784439,1.,0.866025403784439,1.,0.866025403784439,
1.,0.866025403784439,1.,0.866025403784439,1.,0.866025403784439,1.,0.866025403784439,
1.,0.866025403784439,1.,0.866025403784439,1.,0.866025403784439,1.,0.866025403784439,
1.,0.866025403784439,1.,0.866025403784439,1.,0.866025403784439,1.,0.866025403784439,
1.,0.866025403784439,1.,0.866025403784439,1.,0.866025403784439,1.,0.866025403784439,
1.,0.866025403784439,1.,0.866025403784439,1.,0.866025403784439,1.,0.866025403784439,
1.,0.866025403784439,1.,0.866025403784439,1.,0.866025403784439,1.,0.866025403784439,
1.,0.866025403784439,1.,0.866025403784439,1.,0.866025403784439,1.,0.866025403784439,
1.,0.866025403784439,1.,0.866025403784439,1.,0.866025403784439,1.,0.866025403784439,
1.,0.866025403784439,1.,0.866025403784439,1.,0.866025403784439,1.,0.980312120051573,
0.966410600022306),(1.,0.866025403784439,1.,0.866025403784439,1.,0.866025403784439,
1.,0.866025403784439,1.,0.866025403784439,1.,0.866025403784439,1.,0.866025403784439,
1.,0.866025403784439,1.,0.866025403784439,1.,0.866025403784439,1.,0.866025403784439,
1.,0.866025403784439,1.,0.866025403784439,1.,0.866025403784439,1.,0.866025403784439,
1.,0.866025403784439,1.,0.866025403784439,1.,0.866025403784439,1.,0.866025403784439,
1.,0.866025403784439,1.,0.866025403784439,1.,0.866025403784439,1.,0.866025403784439,
1.,0.866025403784439,1.,0.866025403784439,1.,0.866025403784439,1.,0.866025403784439,
1.,0.866025403784439,1.,0.866025403784439,1.,0.866025403784439,1.,0.866025403784439,
1.,0.866025403784439,1.,0.866025403784439,1.,0.866025403784439,1.,0.866025403784439,
1.,0.866025403784439,1.,0.866025403784439,1.,0.866025403784439,1.,0.866025403784439,
1.,0.866025403784439,1.,0.866025403784439,1.,0.866025403784439,1.,0.866025403784439,
1.,0.866025403784439,1.,0.866025403784439,1.,0.866025403784439,1.,0.866025403784439,
1.,0.866025403784439,1.,0.866025403784439,1.,0.866025403784439,1.,0.866025403784439,
1.,0.866025403784439,1.,0.866025403784439,1.,0.866025403784439,1.,0.866025403784439,
1.,0.866025403784439,1.,0.866025403784439,1.,0.866025403784439,1.,0.866025403784439,
1.,0.866025403784439,1.,0.866025403784439,1.,0.866025403784439,1.,0.866025403784439,
1.,0.866025403784439,1.,0.866025403784439,1.,0.866025403784439,1.,0.866025403784439,
1.,0.866025403784439,1.,0.866025403784439,1.,0.866025403784439,1.,0.866025403784439,
1.,0.866025403784439,1.,0.866025403784439,1.,0.866025403784439,1.,0.866025403784439,
1.,0.866025403784439,1.,0.866025403784439,1.,0.866025403784439,1.,0.866025403784439,
1.,0.866025403784439,1.,0.866025403784439,1.,0.866025403784439,1.,0.866025403784439,
1.,0.866025403784439,1.,0.866025403784439,1.,0.866025403784439,1.,0.866025403784439,
1.,0.866025403784439,1.,0.866025403784439,1.,0.866025403784439,1.,0.866025403784439,
1.,0.866025403784439,1.,0.866025403784439,1.,0.866025403784439,1.,0.866025403784439,
1.,0.866025403784439,1.,0.866025403784439,1.,0.866025403784439,1.,0.866025403784439,
1.,0.866025403784439,1.,0.866025403784439,1.,0.866025403784439,1.,0.866025403784439,
1.,0.866025403784439,1.,0.866025403784439,1.,0.866025403784439,1.,0.866025403784439,
1.,0.866025403784439,1.,0.866025403784439,1.,0.866025403784439,1.,0.866025403784439,
1.,0.866025403784439,1.,0.866025403784439,1.,0.866025403784439,1.,0.866025403784439,
1.,0.866025403784439,1.,0.866025403784439,1.,0.866025403784439,1.,0.866025403784439,
1.,0.866025403784439,1.,0.866025403784439,1.,0.866025403784439,1.,0.866025403784439,
1.,0.866025403784439,1.,0.866025403784439,1.,0.866025403784439,1.,0.866025403784439,
1.,0.866025403784439,1.,0.866025403784439,1.,0.866025403784439,1.,0.866025403784439,
1.,0.866025403784439,1.,0.866025403784439,1.,0.866025403784439,1.,0.866025403784439,
1.,0.866025403784439,1.,0.866025403784439,1.,0.980312120051573,0.966410600022306)))
REPRESENTATION_ITEM('')
SURFACE()
);
#3179=(
BOUNDED_SURFACE()
B_SPLINE_SURFACE(1,2,((#256742,#256743,#256744,#256745,#256746,#256747,
#256748,#256749,#256750,#256751,#256752,#256753,#256754,#256755,#256756,
#256757,#256758,#256759,#256760,#256761,#256762,#256763,#256764,#256765,
#256766,#256767,#256768,#256769,#256770,#256771,#256772,#256773,#256774,
#256775,#256776,#256777,#256778,#256779,#256780,#256781,#256782,#256783,
#256784,#256785,#256786,#256787,#256788,#256789,#256790,#256791,#256792,
#256793,#256794,#256795,#256796,#256797,#256798,#256799,#256800,#256801,
#256802,#256803,#256804,#256805,#256806,#256807,#256808,#256809,#256810,
#256811,#256812,#256813,#256814,#256815,#256816,#256817,#256818,#256819,
#256820,#256821,#256822,#256823,#256824,#256825,#256826,#256827,#256828,
#256829,#256830,#256831,#256832,#256833,#256834,#256835,#256836,#256837,
#256838,#256839,#256840,#256841,#256842,#256843,#256844,#256845,#256846,
#256847,#256848,#256849,#256850,#256851,#256852,#256853,#256854,#256855,
#256856,#256857,#256858,#256859,#256860,#256861,#256862,#256863,#256864,
#256865,#256866,#256867,#256868,#256869,#256870,#256871,#256872,#256873,
#256874,#256875,#256876,#256877,#256878,#256879,#256880,#256881,#256882,
#256883,#256884,#256885,#256886,#256887,#256888,#256889,#256890,#256891,
#256892,#256893,#256894,#256895,#256896,#256897,#256898,#256899,#256900,
#256901,#256902,#256903,#256904,#256905,#256906,#256907,#256908,#256909,
#256910,#256911,#256912,#256913,#256914,#256915,#256916,#256917,#256918,
#256919,#256920,#256921,#256922,#256923,#256924,#256925,#256926,#256927,
#256928,#256929,#256930,#256931,#256932,#256933,#256934,#256935,#256936,
#256937,#256938,#256939,#256940,#256941,#256942,#256943,#256944,#256945,
#256946,#256947,#256948,#256949,#256950,#256951,#256952,#256953,#256954,
#256955,#256956,#256957,#256958,#256959,#256960,#256961,#256962,#256963,
#256964,#256965,#256966,#256967,#256968,#256969,#256970,#256971,#256972,
#256973,#256974,#256975,#256976,#256977,#256978,#256979,#256980,#256981,
#256982,#256983,#256984,#256985,#256986,#256987,#256988,#256989,#256990,
#256991,#256992,#256993,#256994,#256995,#256996,#256997,#256998,#256999,
#257000,#257001,#257002,#257003,#257004,#257005,#257006,#257007,#257008,
#257009,#257010,#257011,#257012,#257013,#257014,#257015,#257016,#257017,
#257018),(#257019,#257020,#257021,#257022,#257023,#257024,#257025,#257026,
#257027,#257028,#257029,#257030,#257031,#257032,#257033,#257034,#257035,
#257036,#257037,#257038,#257039,#257040,#257041,#257042,#257043,#257044,
#257045,#257046,#257047,#257048,#257049,#257050,#257051,#257052,#257053,
#257054,#257055,#257056,#257057,#257058,#257059,#257060,#257061,#257062,
#257063,#257064,#257065,#257066,#257067,#257068,#257069,#257070,#257071,
#257072,#257073,#257074,#257075,#257076,#257077,#257078,#257079,#257080,
#257081,#257082,#257083,#257084,#257085,#257086,#257087,#257088,#257089,
#257090,#257091,#257092,#257093,#257094,#257095,#257096,#257097,#257098,
#257099,#257100,#257101,#257102,#257103,#257104,#257105,#257106,#257107,
#257108,#257109,#257110,#257111,#257112,#257113,#257114,#257115,#257116,
#257117,#257118,#257119,#257120,#257121,#257122,#257123,#257124,#257125,
#257126,#257127,#257128,#257129,#257130,#257131,#257132,#257133,#257134,
#257135,#257136,#257137,#257138,#257139,#257140,#257141,#257142,#257143,
#257144,#257145,#257146,#257147,#257148,#257149,#257150,#257151,#257152,
#257153,#257154,#257155,#257156,#257157,#257158,#257159,#257160,#257161,
#257162,#257163,#257164,#257165,#257166,#257167,#257168,#257169,#257170,
#257171,#257172,#257173,#257174,#257175,#257176,#257177,#257178,#257179,
#257180,#257181,#257182,#257183,#257184,#257185,#257186,#257187,#257188,
#257189,#257190,#257191,#257192,#257193,#257194,#257195,#257196,#257197,
#257198,#257199,#257200,#257201,#257202,#257203,#257204,#257205,#257206,
#257207,#257208,#257209,#257210,#257211,#257212,#257213,#257214,#257215,
#257216,#257217,#257218,#257219,#257220,#257221,#257222,#257223,#257224,
#257225,#257226,#257227,#257228,#257229,#257230,#257231,#257232,#257233,
#257234,#257235,#257236,#257237,#257238,#257239,#257240,#257241,#257242,
#257243,#257244,#257245,#257246,#257247,#257248,#257249,#257250,#257251,
#257252,#257253,#257254,#257255,#257256,#257257,#257258,#257259,#257260,
#257261,#257262,#257263,#257264,#257265,#257266,#257267,#257268,#257269,
#257270,#257271,#257272,#257273,#257274,#257275,#257276,#257277,#257278,
#257279,#257280,#257281,#257282,#257283,#257284,#257285,#257286,#257287,
#257288,#257289,#257290,#257291,#257292,#257293,#257294,#257295)),
 .UNSPECIFIED.,.F.,.F.,.F.)
B_SPLINE_SURFACE_WITH_KNOTS((2,2),(3,2,2,2,2,2,2,2,2,2,2,2,2,2,2,2,2,2,
2,2,2,2,2,2,2,2,2,2,2,2,2,2,2,2,2,2,2,2,2,2,2,2,2,2,2,2,2,2,2,2,2,2,2,2,
2,2,2,2,2,2,2,2,2,2,2,2,2,2,2,2,2,2,2,2,2,2,2,2,2,2,2,2,2,2,2,2,2,2,2,2,
2,2,2,2,2,2,2,2,2,2,2,2,2,2,2,2,2,2,2,2,2,2,2,2,2,2,2,2,2,2,2,2,2,2,2,2,
2,2,2,2,2,2,2,2,2,2,2,2,3),(0.,1.00000038849803),(0.,0.0072463768115942,
0.0144927536231884,0.0217391304347826,0.0289855072463768,0.036231884057971,
0.0434782608695652,0.0507246376811594,0.0579710144927536,0.0652173913043478,
0.072463768115942,0.0797101449275362,0.0869565217391304,0.0942028985507246,
0.101449275362319,0.108695652173913,0.115942028985507,0.123188405797101,
0.130434782608696,0.13768115942029,0.144927536231884,0.152173913043478,
0.159420289855073,0.166666666666667,0.173913043478261,0.181159420289855,
0.18840579710145,0.195652173913044,0.202898550724637,0.210144927536232,
0.217391304347826,0.224637681159421,0.231884057971014,0.239130434782609,
0.246376811594203,0.253623188405797,0.260869565217392,0.268115942028985,
0.275362318840579,0.282608695652174,0.289855072463768,0.297101449275363,
0.304347826086956,0.31159420289855,0.318840579710145,0.326086956521739,
0.333333333333334,0.340579710144927,0.347826086956521,0.355072463768116,
0.36231884057971,0.369565217391304,0.376811594202899,0.384057971014493,
0.391304347826087,0.398550724637681,0.405797101449275,0.41304347826087,
0.420289855072463,0.427536231884058,0.434782608695652,0.442028985507247,
0.449275362318841,0.456521739130435,0.463768115942029,0.471014492753623,
0.478260869565218,0.485507246376812,0.492753623188406,0.5,0.507246376811594,
0.514492753623188,0.521739130434783,0.528985507246377,0.536231884057971,
0.543478260869565,0.550724637681159,0.557971014492754,0.565217391304348,
0.572463768115942,0.579710144927536,0.586956521739131,0.594202898550725,
0.601449275362319,0.608695652173913,0.615942028985507,0.623188405797101,
0.630434782608696,0.63768115942029,0.644927536231884,0.652173913043478,
0.659420289855073,0.666666666666667,0.673913043478261,0.681159420289855,
0.688405797101449,0.695652173913044,0.702898550724638,0.710144927536232,
0.717391304347826,0.72463768115942,0.731884057971015,0.739130434782609,
0.746376811594203,0.753623188405797,0.760869565217391,0.768115942028986,
0.77536231884058,0.782608695652174,0.789855072463768,0.797101449275362,
0.804347826086956,0.811594202898551,0.818840579710145,0.826086956521739,
0.833333333333333,0.840579710144928,0.847826086956522,0.855072463768116,
0.86231884057971,0.869565217391304,0.876811594202899,0.884057971014493,
0.891304347826087,0.898550724637681,0.905797101449275,0.91304347826087,
0.920289855072464,0.927536231884058,0.934782608695652,0.942028985507246,
0.94927536231884,0.956521739130435,0.963768115942029,0.971014492753623,
0.978260869565217,0.985507246376812,0.992753623188406,0.993818495192186),
 .UNSPECIFIED.)
GEOMETRIC_REPRESENTATION_ITEM()
RATIONAL_B_SPLINE_SURFACE(((1.,0.866025403784439,1.,0.866025403784439,1.,
0.866025403784439,1.,0.866025403784439,1.,0.866025403784439,1.,0.866025403784439,
1.,0.866025403784439,1.,0.866025403784439,1.,0.866025403784439,1.,0.866025403784439,
1.,0.866025403784439,1.,0.866025403784439,1.,0.866025403784439,1.,0.866025403784439,
1.,0.866025403784439,1.,0.866025403784439,1.,0.866025403784439,1.,0.866025403784439,
1.,0.866025403784439,1.,0.866025403784439,1.,0.866025403784439,1.,0.866025403784439,
1.,0.866025403784439,1.,0.866025403784439,1.,0.866025403784439,1.,0.866025403784439,
1.,0.866025403784439,1.,0.866025403784439,1.,0.866025403784439,1.,0.866025403784439,
1.,0.866025403784439,1.,0.866025403784439,1.,0.866025403784439,1.,0.866025403784439,
1.,0.866025403784439,1.,0.866025403784439,1.,0.866025403784439,1.,0.866025403784439,
1.,0.866025403784439,1.,0.866025403784439,1.,0.866025403784439,1.,0.866025403784439,
1.,0.866025403784439,1.,0.866025403784439,1.,0.866025403784439,1.,0.866025403784439,
1.,0.866025403784439,1.,0.866025403784439,1.,0.866025403784439,1.,0.866025403784439,
1.,0.866025403784439,1.,0.866025403784439,1.,0.866025403784439,1.,0.866025403784439,
1.,0.866025403784439,1.,0.866025403784439,1.,0.866025403784439,1.,0.866025403784439,
1.,0.866025403784439,1.,0.866025403784439,1.,0.866025403784439,1.,0.866025403784439,
1.,0.866025403784439,1.,0.866025403784439,1.,0.866025403784439,1.,0.866025403784439,
1.,0.866025403784439,1.,0.866025403784439,1.,0.866025403784439,1.,0.866025403784439,
1.,0.866025403784439,1.,0.866025403784439,1.,0.866025403784439,1.,0.866025403784439,
1.,0.866025403784439,1.,0.866025403784439,1.,0.866025403784439,1.,0.866025403784439,
1.,0.866025403784439,1.,0.866025403784439,1.,0.866025403784439,1.,0.866025403784439,
1.,0.866025403784439,1.,0.866025403784439,1.,0.866025403784439,1.,0.866025403784439,
1.,0.866025403784439,1.,0.866025403784439,1.,0.866025403784439,1.,0.866025403784439,
1.,0.866025403784439,1.,0.866025403784439,1.,0.866025403784439,1.,0.866025403784439,
1.,0.866025403784439,1.,0.866025403784439,1.,0.866025403784439,1.,0.866025403784439,
1.,0.866025403784439,1.,0.866025403784439,1.,0.866025403784439,1.,0.866025403784439,
1.,0.866025403784439,1.,0.866025403784439,1.,0.866025403784439,1.,0.866025403784439,
1.,0.866025403784439,1.,0.866025403784439,1.,0.866025403784439,1.,0.866025403784439,
1.,0.866025403784439,1.,0.866025403784439,1.,0.866025403784439,1.,0.866025403784439,
1.,0.866025403784439,1.,0.866025403784439,1.,0.866025403784439,1.,0.866025403784439,
1.,0.866025403784439,1.,0.866025403784439,1.,0.866025403784439,1.,0.866025403784439,
1.,0.866025403784439,1.,0.866025403784439,1.,0.866025403784439,1.,0.866025403784439,
1.,0.866025403784439,1.,0.866025403784439,1.,0.866025403784439,1.,0.866025403784439,
1.,0.866025403784439,1.,0.866025403784439,1.,0.866025403784439,1.,0.866025403784439,
1.,0.866025403784439,1.,0.866025403784439,1.,0.866025403784439,1.,0.980312120051573,
0.966410600022306),(1.,0.866025403784439,1.,0.866025403784439,1.,0.866025403784439,
1.,0.866025403784439,1.,0.866025403784439,1.,0.866025403784439,1.,0.866025403784439,
1.,0.866025403784439,1.,0.866025403784439,1.,0.866025403784439,1.,0.866025403784439,
1.,0.866025403784439,1.,0.866025403784439,1.,0.866025403784439,1.,0.866025403784439,
1.,0.866025403784439,1.,0.866025403784439,1.,0.866025403784439,1.,0.866025403784439,
1.,0.866025403784439,1.,0.866025403784439,1.,0.866025403784439,1.,0.866025403784439,
1.,0.866025403784439,1.,0.866025403784439,1.,0.866025403784439,1.,0.866025403784439,
1.,0.866025403784439,1.,0.866025403784439,1.,0.866025403784439,1.,0.866025403784439,
1.,0.866025403784439,1.,0.866025403784439,1.,0.866025403784439,1.,0.866025403784439,
1.,0.866025403784439,1.,0.866025403784439,1.,0.866025403784439,1.,0.866025403784439,
1.,0.866025403784439,1.,0.866025403784439,1.,0.866025403784439,1.,0.866025403784439,
1.,0.866025403784439,1.,0.866025403784439,1.,0.866025403784439,1.,0.866025403784439,
1.,0.866025403784439,1.,0.866025403784439,1.,0.866025403784439,1.,0.866025403784439,
1.,0.866025403784439,1.,0.866025403784439,1.,0.866025403784439,1.,0.866025403784439,
1.,0.866025403784439,1.,0.866025403784439,1.,0.866025403784439,1.,0.866025403784439,
1.,0.866025403784439,1.,0.866025403784439,1.,0.866025403784439,1.,0.866025403784439,
1.,0.866025403784439,1.,0.866025403784439,1.,0.866025403784439,1.,0.866025403784439,
1.,0.866025403784439,1.,0.866025403784439,1.,0.866025403784439,1.,0.866025403784439,
1.,0.866025403784439,1.,0.866025403784439,1.,0.866025403784439,1.,0.866025403784439,
1.,0.866025403784439,1.,0.866025403784439,1.,0.866025403784439,1.,0.866025403784439,
1.,0.866025403784439,1.,0.866025403784439,1.,0.866025403784439,1.,0.866025403784439,
1.,0.866025403784439,1.,0.866025403784439,1.,0.866025403784439,1.,0.866025403784439,
1.,0.866025403784439,1.,0.866025403784439,1.,0.866025403784439,1.,0.866025403784439,
1.,0.866025403784439,1.,0.866025403784439,1.,0.866025403784439,1.,0.866025403784439,
1.,0.866025403784439,1.,0.866025403784439,1.,0.866025403784439,1.,0.866025403784439,
1.,0.866025403784439,1.,0.866025403784439,1.,0.866025403784439,1.,0.866025403784439,
1.,0.866025403784439,1.,0.866025403784439,1.,0.866025403784439,1.,0.866025403784439,
1.,0.866025403784439,1.,0.866025403784439,1.,0.866025403784439,1.,0.866025403784439,
1.,0.866025403784439,1.,0.866025403784439,1.,0.866025403784439,1.,0.866025403784439,
1.,0.866025403784439,1.,0.866025403784439,1.,0.866025403784439,1.,0.866025403784439,
1.,0.866025403784439,1.,0.866025403784439,1.,0.866025403784439,1.,0.866025403784439,
1.,0.866025403784439,1.,0.866025403784439,1.,0.866025403784439,1.,0.866025403784439,
1.,0.866025403784439,1.,0.866025403784439,1.,0.866025403784439,1.,0.866025403784439,
1.,0.866025403784439,1.,0.866025403784439,1.,0.866025403784439,1.,0.866025403784439,
1.,0.866025403784439,1.,0.866025403784439,1.,0.980312120051573,0.966410600022306)))
REPRESENTATION_ITEM('')
SURFACE()
);
#3180=(
BOUNDED_SURFACE()
B_SPLINE_SURFACE(1,2,((#257346,#257347,#257348,#257349,#257350,#257351,
#257352,#257353,#257354,#257355,#257356,#257357,#257358,#257359,#257360,
#257361,#257362,#257363,#257364,#257365,#257366,#257367,#257368,#257369,
#257370,#257371,#257372,#257373,#257374,#257375,#257376,#257377,#257378,
#257379,#257380,#257381,#257382,#257383,#257384,#257385,#257386,#257387,
#257388,#257389,#257390,#257391,#257392,#257393,#257394,#257395,#257396,
#257397,#257398,#257399,#257400,#257401,#257402,#257403,#257404,#257405,
#257406,#257407,#257408,#257409,#257410,#257411,#257412,#257413,#257414,
#257415,#257416,#257417,#257418,#257419,#257420,#257421,#257422,#257423,
#257424,#257425,#257426,#257427,#257428,#257429,#257430,#257431,#257432,
#257433,#257434,#257435,#257436,#257437,#257438,#257439,#257440,#257441,
#257442,#257443,#257444,#257445,#257446,#257447,#257448,#257449,#257450,
#257451,#257452,#257453,#257454,#257455,#257456,#257457,#257458,#257459,
#257460,#257461,#257462,#257463,#257464,#257465,#257466,#257467,#257468,
#257469,#257470,#257471,#257472,#257473,#257474,#257475,#257476,#257477,
#257478,#257479,#257480,#257481,#257482,#257483,#257484,#257485,#257486,
#257487,#257488,#257489,#257490,#257491,#257492,#257493,#257494,#257495,
#257496,#257497,#257498,#257499,#257500,#257501,#257502,#257503,#257504,
#257505,#257506,#257507,#257508,#257509,#257510,#257511,#257512,#257513,
#257514,#257515,#257516,#257517,#257518,#257519,#257520,#257521,#257522,
#257523,#257524,#257525,#257526,#257527,#257528,#257529,#257530,#257531,
#257532,#257533,#257534,#257535,#257536,#257537,#257538,#257539,#257540,
#257541,#257542,#257543,#257544,#257545,#257546,#257547,#257548,#257549,
#257550,#257551,#257552,#257553,#257554,#257555,#257556,#257557,#257558,
#257559,#257560,#257561,#257562,#257563,#257564,#257565,#257566,#257567,
#257568,#257569,#257570,#257571,#257572,#257573,#257574,#257575,#257576,
#257577,#257578,#257579,#257580,#257581,#257582,#257583,#257584,#257585,
#257586,#257587,#257588,#257589,#257590,#257591,#257592,#257593,#257594,
#257595,#257596,#257597,#257598,#257599,#257600,#257601,#257602,#257603,
#257604,#257605,#257606,#257607,#257608,#257609,#257610,#257611,#257612,
#257613,#257614,#257615,#257616,#257617,#257618,#257619,#257620,#257621,
#257622),(#257623,#257624,#257625,#257626,#257627,#257628,#257629,#257630,
#257631,#257632,#257633,#257634,#257635,#257636,#257637,#257638,#257639,
#257640,#257641,#257642,#257643,#257644,#257645,#257646,#257647,#257648,
#257649,#257650,#257651,#257652,#257653,#257654,#257655,#257656,#257657,
#257658,#257659,#257660,#257661,#257662,#257663,#257664,#257665,#257666,
#257667,#257668,#257669,#257670,#257671,#257672,#257673,#257674,#257675,
#257676,#257677,#257678,#257679,#257680,#257681,#257682,#257683,#257684,
#257685,#257686,#257687,#257688,#257689,#257690,#257691,#257692,#257693,
#257694,#257695,#257696,#257697,#257698,#257699,#257700,#257701,#257702,
#257703,#257704,#257705,#257706,#257707,#257708,#257709,#257710,#257711,
#257712,#257713,#257714,#257715,#257716,#257717,#257718,#257719,#257720,
#257721,#257722,#257723,#257724,#257725,#257726,#257727,#257728,#257729,
#257730,#257731,#257732,#257733,#257734,#257735,#257736,#257737,#257738,
#257739,#257740,#257741,#257742,#257743,#257744,#257745,#257746,#257747,
#257748,#257749,#257750,#257751,#257752,#257753,#257754,#257755,#257756,
#257757,#257758,#257759,#257760,#257761,#257762,#257763,#257764,#257765,
#257766,#257767,#257768,#257769,#257770,#257771,#257772,#257773,#257774,
#257775,#257776,#257777,#257778,#257779,#257780,#257781,#257782,#257783,
#257784,#257785,#257786,#257787,#257788,#257789,#257790,#257791,#257792,
#257793,#257794,#257795,#257796,#257797,#257798,#257799,#257800,#257801,
#257802,#257803,#257804,#257805,#257806,#257807,#257808,#257809,#257810,
#257811,#257812,#257813,#257814,#257815,#257816,#257817,#257818,#257819,
#257820,#257821,#257822,#257823,#257824,#257825,#257826,#257827,#257828,
#257829,#257830,#257831,#257832,#257833,#257834,#257835,#257836,#257837,
#257838,#257839,#257840,#257841,#257842,#257843,#257844,#257845,#257846,
#257847,#257848,#257849,#257850,#257851,#257852,#257853,#257854,#257855,
#257856,#257857,#257858,#257859,#257860,#257861,#257862,#257863,#257864,
#257865,#257866,#257867,#257868,#257869,#257870,#257871,#257872,#257873,
#257874,#257875,#257876,#257877,#257878,#257879,#257880,#257881,#257882,
#257883,#257884,#257885,#257886,#257887,#257888,#257889,#257890,#257891,
#257892,#257893,#257894,#257895,#257896,#257897,#257898,#257899)),
 .UNSPECIFIED.,.F.,.F.,.F.)
B_SPLINE_SURFACE_WITH_KNOTS((2,2),(3,2,2,2,2,2,2,2,2,2,2,2,2,2,2,2,2,2,
2,2,2,2,2,2,2,2,2,2,2,2,2,2,2,2,2,2,2,2,2,2,2,2,2,2,2,2,2,2,2,2,2,2,2,2,
2,2,2,2,2,2,2,2,2,2,2,2,2,2,2,2,2,2,2,2,2,2,2,2,2,2,2,2,2,2,2,2,2,2,2,2,
2,2,2,2,2,2,2,2,2,2,2,2,2,2,2,2,2,2,2,2,2,2,2,2,2,2,2,2,2,2,2,2,2,2,2,2,
2,2,2,2,2,2,2,2,2,2,2,2,3),(0.,1.),(0.,0.0072463768115942,0.0144927536231884,
0.0217391304347826,0.0289855072463768,0.036231884057971,0.0434782608695652,
0.0507246376811594,0.0579710144927536,0.0652173913043478,0.072463768115942,
0.0797101449275362,0.0869565217391304,0.0942028985507246,0.101449275362319,
0.108695652173913,0.115942028985507,0.123188405797101,0.130434782608696,
0.13768115942029,0.144927536231884,0.152173913043478,0.159420289855073,
0.166666666666667,0.173913043478261,0.181159420289855,0.18840579710145,
0.195652173913044,0.202898550724637,0.210144927536232,0.217391304347826,
0.224637681159421,0.231884057971014,0.239130434782609,0.246376811594203,
0.253623188405797,0.260869565217392,0.268115942028985,0.275362318840579,
0.282608695652174,0.289855072463768,0.297101449275363,0.304347826086956,
0.31159420289855,0.318840579710145,0.326086956521739,0.333333333333334,
0.340579710144927,0.347826086956521,0.355072463768116,0.36231884057971,
0.369565217391304,0.376811594202899,0.384057971014493,0.391304347826087,
0.398550724637681,0.405797101449275,0.41304347826087,0.420289855072463,
0.427536231884058,0.434782608695652,0.442028985507247,0.449275362318841,
0.456521739130435,0.463768115942029,0.471014492753623,0.478260869565218,
0.485507246376812,0.492753623188406,0.5,0.507246376811594,0.514492753623188,
0.521739130434783,0.528985507246377,0.536231884057971,0.543478260869565,
0.550724637681159,0.557971014492754,0.565217391304348,0.572463768115942,
0.579710144927536,0.586956521739131,0.594202898550725,0.601449275362319,
0.608695652173913,0.615942028985507,0.623188405797101,0.630434782608696,
0.63768115942029,0.644927536231884,0.652173913043478,0.659420289855073,
0.666666666666667,0.673913043478261,0.681159420289855,0.688405797101449,
0.695652173913044,0.702898550724638,0.710144927536232,0.717391304347826,
0.72463768115942,0.731884057971015,0.739130434782609,0.746376811594203,
0.753623188405797,0.760869565217391,0.768115942028986,0.77536231884058,
0.782608695652174,0.789855072463768,0.797101449275362,0.804347826086956,
0.811594202898551,0.818840579710145,0.826086956521739,0.833333333333333,
0.840579710144928,0.847826086956522,0.855072463768116,0.86231884057971,
0.869565217391304,0.876811594202899,0.884057971014493,0.891304347826087,
0.898550724637681,0.905797101449275,0.91304347826087,0.920289855072464,
0.927536231884058,0.934782608695652,0.942028985507246,0.94927536231884,
0.956521739130435,0.963768115942029,0.971014492753623,0.978260869565217,
0.985507246376812,0.992753623188406,0.993818585798284),.UNSPECIFIED.)
GEOMETRIC_REPRESENTATION_ITEM()
RATIONAL_B_SPLINE_SURFACE(((1.,0.866025403784439,1.,0.866025403784439,1.,
0.866025403784439,1.,0.866025403784439,1.,0.866025403784439,1.,0.866025403784439,
1.,0.866025403784439,1.,0.866025403784439,1.,0.866025403784439,1.,0.866025403784439,
1.,0.866025403784439,1.,0.866025403784439,1.,0.866025403784439,1.,0.866025403784439,
1.,0.866025403784439,1.,0.866025403784439,1.,0.866025403784439,1.,0.866025403784439,
1.,0.866025403784439,1.,0.866025403784439,1.,0.866025403784439,1.,0.866025403784439,
1.,0.866025403784439,1.,0.866025403784439,1.,0.866025403784439,1.,0.866025403784439,
1.,0.866025403784439,1.,0.866025403784439,1.,0.866025403784439,1.,0.866025403784439,
1.,0.866025403784439,1.,0.866025403784439,1.,0.866025403784439,1.,0.866025403784439,
1.,0.866025403784439,1.,0.866025403784439,1.,0.866025403784439,1.,0.866025403784439,
1.,0.866025403784439,1.,0.866025403784439,1.,0.866025403784439,1.,0.866025403784439,
1.,0.866025403784439,1.,0.866025403784439,1.,0.866025403784439,1.,0.866025403784439,
1.,0.866025403784439,1.,0.866025403784439,1.,0.866025403784439,1.,0.866025403784439,
1.,0.866025403784439,1.,0.866025403784439,1.,0.866025403784439,1.,0.866025403784439,
1.,0.866025403784439,1.,0.866025403784439,1.,0.866025403784439,1.,0.866025403784439,
1.,0.866025403784439,1.,0.866025403784439,1.,0.866025403784439,1.,0.866025403784439,
1.,0.866025403784439,1.,0.866025403784439,1.,0.866025403784439,1.,0.866025403784439,
1.,0.866025403784439,1.,0.866025403784439,1.,0.866025403784439,1.,0.866025403784439,
1.,0.866025403784439,1.,0.866025403784439,1.,0.866025403784439,1.,0.866025403784439,
1.,0.866025403784439,1.,0.866025403784439,1.,0.866025403784439,1.,0.866025403784439,
1.,0.866025403784439,1.,0.866025403784439,1.,0.866025403784439,1.,0.866025403784439,
1.,0.866025403784439,1.,0.866025403784439,1.,0.866025403784439,1.,0.866025403784439,
1.,0.866025403784439,1.,0.866025403784439,1.,0.866025403784439,1.,0.866025403784439,
1.,0.866025403784439,1.,0.866025403784439,1.,0.866025403784439,1.,0.866025403784439,
1.,0.866025403784439,1.,0.866025403784439,1.,0.866025403784439,1.,0.866025403784439,
1.,0.866025403784439,1.,0.866025403784439,1.,0.866025403784439,1.,0.866025403784439,
1.,0.866025403784439,1.,0.866025403784439,1.,0.866025403784439,1.,0.866025403784439,
1.,0.866025403784439,1.,0.866025403784439,1.,0.866025403784439,1.,0.866025403784439,
1.,0.866025403784439,1.,0.866025403784439,1.,0.866025403784439,1.,0.866025403784439,
1.,0.866025403784439,1.,0.866025403784439,1.,0.866025403784439,1.,0.866025403784439,
1.,0.866025403784439,1.,0.866025403784439,1.,0.866025403784439,1.,0.866025403784439,
1.,0.866025403784439,1.,0.866025403784439,1.,0.866025403784439,1.,0.866025403784439,
1.,0.866025403784439,1.,0.866025403784439,1.,0.866025403784439,1.,0.866025403784439,
1.,0.866025403784439,1.,0.866025403784439,1.,0.866025403784439,1.,0.866025403784439,
1.,0.866025403784439,1.,0.866025403784439,1.,0.866025403784439,1.,0.98031044488126,
0.966408234404338),(1.,0.866025403784439,1.,0.866025403784439,1.,0.866025403784439,
1.,0.866025403784439,1.,0.866025403784439,1.,0.866025403784439,1.,0.866025403784439,
1.,0.866025403784439,1.,0.866025403784439,1.,0.866025403784439,1.,0.866025403784439,
1.,0.866025403784439,1.,0.866025403784439,1.,0.866025403784439,1.,0.866025403784439,
1.,0.866025403784439,1.,0.866025403784439,1.,0.866025403784439,1.,0.866025403784439,
1.,0.866025403784439,1.,0.866025403784439,1.,0.866025403784439,1.,0.866025403784439,
1.,0.866025403784439,1.,0.866025403784439,1.,0.866025403784439,1.,0.866025403784439,
1.,0.866025403784439,1.,0.866025403784439,1.,0.866025403784439,1.,0.866025403784439,
1.,0.866025403784439,1.,0.866025403784439,1.,0.866025403784439,1.,0.866025403784439,
1.,0.866025403784439,1.,0.866025403784439,1.,0.866025403784439,1.,0.866025403784439,
1.,0.866025403784439,1.,0.866025403784439,1.,0.866025403784439,1.,0.866025403784439,
1.,0.866025403784439,1.,0.866025403784439,1.,0.866025403784439,1.,0.866025403784439,
1.,0.866025403784439,1.,0.866025403784439,1.,0.866025403784439,1.,0.866025403784439,
1.,0.866025403784439,1.,0.866025403784439,1.,0.866025403784439,1.,0.866025403784439,
1.,0.866025403784439,1.,0.866025403784439,1.,0.866025403784439,1.,0.866025403784439,
1.,0.866025403784439,1.,0.866025403784439,1.,0.866025403784439,1.,0.866025403784439,
1.,0.866025403784439,1.,0.866025403784439,1.,0.866025403784439,1.,0.866025403784439,
1.,0.866025403784439,1.,0.866025403784439,1.,0.866025403784439,1.,0.866025403784439,
1.,0.866025403784439,1.,0.866025403784439,1.,0.866025403784439,1.,0.866025403784439,
1.,0.866025403784439,1.,0.866025403784439,1.,0.866025403784439,1.,0.866025403784439,
1.,0.866025403784439,1.,0.866025403784439,1.,0.866025403784439,1.,0.866025403784439,
1.,0.866025403784439,1.,0.866025403784439,1.,0.866025403784439,1.,0.866025403784439,
1.,0.866025403784439,1.,0.866025403784439,1.,0.866025403784439,1.,0.866025403784439,
1.,0.866025403784439,1.,0.866025403784439,1.,0.866025403784439,1.,0.866025403784439,
1.,0.866025403784439,1.,0.866025403784439,1.,0.866025403784439,1.,0.866025403784439,
1.,0.866025403784439,1.,0.866025403784439,1.,0.866025403784439,1.,0.866025403784439,
1.,0.866025403784439,1.,0.866025403784439,1.,0.866025403784439,1.,0.866025403784439,
1.,0.866025403784439,1.,0.866025403784439,1.,0.866025403784439,1.,0.866025403784439,
1.,0.866025403784439,1.,0.866025403784439,1.,0.866025403784439,1.,0.866025403784439,
1.,0.866025403784439,1.,0.866025403784439,1.,0.866025403784439,1.,0.866025403784439,
1.,0.866025403784439,1.,0.866025403784439,1.,0.866025403784439,1.,0.866025403784439,
1.,0.866025403784439,1.,0.866025403784439,1.,0.866025403784439,1.,0.866025403784439,
1.,0.866025403784439,1.,0.866025403784439,1.,0.866025403784439,1.,0.866025403784439,
1.,0.866025403784439,1.,0.866025403784439,1.,0.866025403784439,1.,0.866025403784439,
1.,0.866025403784439,1.,0.866025403784439,1.,0.98031044488126,0.966408234404338)))
REPRESENTATION_ITEM('')
SURFACE()
);
#3181=(
BOUNDED_SURFACE()
B_SPLINE_SURFACE(1,2,((#257947,#257948,#257949,#257950,#257951,#257952,
#257953,#257954,#257955,#257956,#257957,#257958,#257959,#257960,#257961,
#257962,#257963,#257964,#257965,#257966,#257967,#257968,#257969,#257970,
#257971,#257972,#257973,#257974,#257975,#257976,#257977,#257978,#257979,
#257980,#257981,#257982,#257983,#257984,#257985,#257986,#257987,#257988,
#257989,#257990,#257991,#257992,#257993,#257994,#257995,#257996,#257997,
#257998,#257999,#258000,#258001,#258002,#258003,#258004,#258005,#258006,
#258007,#258008,#258009,#258010,#258011,#258012,#258013,#258014,#258015,
#258016,#258017,#258018,#258019,#258020,#258021,#258022,#258023,#258024,
#258025,#258026,#258027,#258028,#258029,#258030,#258031,#258032,#258033,
#258034,#258035,#258036,#258037,#258038,#258039,#258040,#258041,#258042,
#258043,#258044,#258045,#258046,#258047,#258048,#258049,#258050,#258051,
#258052,#258053,#258054,#258055,#258056,#258057,#258058,#258059,#258060,
#258061,#258062,#258063,#258064,#258065,#258066,#258067,#258068,#258069,
#258070,#258071,#258072,#258073,#258074,#258075,#258076,#258077,#258078,
#258079,#258080,#258081,#258082,#258083,#258084,#258085,#258086,#258087,
#258088,#258089,#258090,#258091,#258092,#258093,#258094,#258095,#258096,
#258097,#258098,#258099,#258100,#258101,#258102,#258103,#258104,#258105,
#258106,#258107,#258108,#258109,#258110,#258111,#258112,#258113,#258114,
#258115,#258116,#258117,#258118,#258119,#258120,#258121,#258122,#258123,
#258124,#258125,#258126,#258127,#258128,#258129,#258130,#258131,#258132,
#258133,#258134,#258135,#258136,#258137,#258138,#258139,#258140,#258141,
#258142,#258143,#258144,#258145,#258146,#258147,#258148,#258149,#258150,
#258151,#258152,#258153,#258154,#258155,#258156,#258157,#258158,#258159,
#258160,#258161,#258162,#258163,#258164,#258165,#258166,#258167,#258168,
#258169,#258170,#258171,#258172,#258173,#258174,#258175,#258176,#258177,
#258178,#258179,#258180,#258181,#258182,#258183,#258184,#258185,#258186,
#258187,#258188,#258189,#258190,#258191,#258192,#258193,#258194,#258195,
#258196,#258197,#258198,#258199,#258200,#258201,#258202,#258203,#258204,
#258205,#258206,#258207,#258208,#258209,#258210,#258211,#258212,#258213,
#258214,#258215,#258216,#258217,#258218,#258219,#258220,#258221,#258222,
#258223),(#258224,#258225,#258226,#258227,#258228,#258229,#258230,#258231,
#258232,#258233,#258234,#258235,#258236,#258237,#258238,#258239,#258240,
#258241,#258242,#258243,#258244,#258245,#258246,#258247,#258248,#258249,
#258250,#258251,#258252,#258253,#258254,#258255,#258256,#258257,#258258,
#258259,#258260,#258261,#258262,#258263,#258264,#258265,#258266,#258267,
#258268,#258269,#258270,#258271,#258272,#258273,#258274,#258275,#258276,
#258277,#258278,#258279,#258280,#258281,#258282,#258283,#258284,#258285,
#258286,#258287,#258288,#258289,#258290,#258291,#258292,#258293,#258294,
#258295,#258296,#258297,#258298,#258299,#258300,#258301,#258302,#258303,
#258304,#258305,#258306,#258307,#258308,#258309,#258310,#258311,#258312,
#258313,#258314,#258315,#258316,#258317,#258318,#258319,#258320,#258321,
#258322,#258323,#258324,#258325,#258326,#258327,#258328,#258329,#258330,
#258331,#258332,#258333,#258334,#258335,#258336,#258337,#258338,#258339,
#258340,#258341,#258342,#258343,#258344,#258345,#258346,#258347,#258348,
#258349,#258350,#258351,#258352,#258353,#258354,#258355,#258356,#258357,
#258358,#258359,#258360,#258361,#258362,#258363,#258364,#258365,#258366,
#258367,#258368,#258369,#258370,#258371,#258372,#258373,#258374,#258375,
#258376,#258377,#258378,#258379,#258380,#258381,#258382,#258383,#258384,
#258385,#258386,#258387,#258388,#258389,#258390,#258391,#258392,#258393,
#258394,#258395,#258396,#258397,#258398,#258399,#258400,#258401,#258402,
#258403,#258404,#258405,#258406,#258407,#258408,#258409,#258410,#258411,
#258412,#258413,#258414,#258415,#258416,#258417,#258418,#258419,#258420,
#258421,#258422,#258423,#258424,#258425,#258426,#258427,#258428,#258429,
#258430,#258431,#258432,#258433,#258434,#258435,#258436,#258437,#258438,
#258439,#258440,#258441,#258442,#258443,#258444,#258445,#258446,#258447,
#258448,#258449,#258450,#258451,#258452,#258453,#258454,#258455,#258456,
#258457,#258458,#258459,#258460,#258461,#258462,#258463,#258464,#258465,
#258466,#258467,#258468,#258469,#258470,#258471,#258472,#258473,#258474,
#258475,#258476,#258477,#258478,#258479,#258480,#258481,#258482,#258483,
#258484,#258485,#258486,#258487,#258488,#258489,#258490,#258491,#258492,
#258493,#258494,#258495,#258496,#258497,#258498,#258499,#258500)),
 .UNSPECIFIED.,.F.,.F.,.F.)
B_SPLINE_SURFACE_WITH_KNOTS((2,2),(3,2,2,2,2,2,2,2,2,2,2,2,2,2,2,2,2,2,
2,2,2,2,2,2,2,2,2,2,2,2,2,2,2,2,2,2,2,2,2,2,2,2,2,2,2,2,2,2,2,2,2,2,2,2,
2,2,2,2,2,2,2,2,2,2,2,2,2,2,2,2,2,2,2,2,2,2,2,2,2,2,2,2,2,2,2,2,2,2,2,2,
2,2,2,2,2,2,2,2,2,2,2,2,2,2,2,2,2,2,2,2,2,2,2,2,2,2,2,2,2,2,2,2,2,2,2,2,
2,2,2,2,2,2,2,2,2,2,2,2,3),(0.,1.),(0.,0.0072463768115942,0.0144927536231884,
0.0217391304347826,0.0289855072463768,0.036231884057971,0.0434782608695652,
0.0507246376811594,0.0579710144927536,0.0652173913043478,0.072463768115942,
0.0797101449275362,0.0869565217391304,0.0942028985507246,0.101449275362319,
0.108695652173913,0.115942028985507,0.123188405797101,0.130434782608696,
0.13768115942029,0.144927536231884,0.152173913043478,0.159420289855073,
0.166666666666667,0.173913043478261,0.181159420289855,0.18840579710145,
0.195652173913044,0.202898550724637,0.210144927536232,0.217391304347826,
0.224637681159421,0.231884057971014,0.239130434782609,0.246376811594203,
0.253623188405797,0.260869565217392,0.268115942028985,0.275362318840579,
0.282608695652174,0.289855072463768,0.297101449275363,0.304347826086956,
0.31159420289855,0.318840579710145,0.326086956521739,0.333333333333334,
0.340579710144927,0.347826086956521,0.355072463768116,0.36231884057971,
0.369565217391304,0.376811594202899,0.384057971014493,0.391304347826087,
0.398550724637681,0.405797101449275,0.41304347826087,0.420289855072463,
0.427536231884058,0.434782608695652,0.442028985507247,0.449275362318841,
0.456521739130435,0.463768115942029,0.471014492753623,0.478260869565218,
0.485507246376812,0.492753623188406,0.5,0.507246376811594,0.514492753623188,
0.521739130434783,0.528985507246377,0.536231884057971,0.543478260869565,
0.550724637681159,0.557971014492754,0.565217391304348,0.572463768115942,
0.579710144927536,0.586956521739131,0.594202898550725,0.601449275362319,
0.608695652173913,0.615942028985507,0.623188405797101,0.630434782608696,
0.63768115942029,0.644927536231884,0.652173913043478,0.659420289855073,
0.666666666666667,0.673913043478261,0.681159420289855,0.688405797101449,
0.695652173913044,0.702898550724638,0.710144927536232,0.717391304347826,
0.72463768115942,0.731884057971015,0.739130434782609,0.746376811594203,
0.753623188405797,0.760869565217391,0.768115942028986,0.77536231884058,
0.782608695652174,0.789855072463768,0.797101449275362,0.804347826086956,
0.811594202898551,0.818840579710145,0.826086956521739,0.833333333333333,
0.840579710144928,0.847826086956522,0.855072463768116,0.86231884057971,
0.869565217391304,0.876811594202899,0.884057971014493,0.891304347826087,
0.898550724637681,0.905797101449275,0.91304347826087,0.920289855072464,
0.927536231884058,0.934782608695652,0.942028985507246,0.94927536231884,
0.956521739130435,0.963768115942029,0.971014492753623,0.978260869565217,
0.985507246376812,0.992753623188406,0.993818585798284),.UNSPECIFIED.)
GEOMETRIC_REPRESENTATION_ITEM()
RATIONAL_B_SPLINE_SURFACE(((1.,0.866025403784439,1.,0.866025403784439,1.,
0.866025403784439,1.,0.866025403784439,1.,0.866025403784439,1.,0.866025403784439,
1.,0.866025403784439,1.,0.866025403784439,1.,0.866025403784439,1.,0.866025403784439,
1.,0.866025403784439,1.,0.866025403784439,1.,0.866025403784439,1.,0.866025403784439,
1.,0.866025403784439,1.,0.866025403784439,1.,0.866025403784439,1.,0.866025403784439,
1.,0.866025403784439,1.,0.866025403784439,1.,0.866025403784439,1.,0.866025403784439,
1.,0.866025403784439,1.,0.866025403784439,1.,0.866025403784439,1.,0.866025403784439,
1.,0.866025403784439,1.,0.866025403784439,1.,0.866025403784439,1.,0.866025403784439,
1.,0.866025403784439,1.,0.866025403784439,1.,0.866025403784439,1.,0.866025403784439,
1.,0.866025403784439,1.,0.866025403784439,1.,0.866025403784439,1.,0.866025403784439,
1.,0.866025403784439,1.,0.866025403784439,1.,0.866025403784439,1.,0.866025403784439,
1.,0.866025403784439,1.,0.866025403784439,1.,0.866025403784439,1.,0.866025403784439,
1.,0.866025403784439,1.,0.866025403784439,1.,0.866025403784439,1.,0.866025403784439,
1.,0.866025403784439,1.,0.866025403784439,1.,0.866025403784439,1.,0.866025403784439,
1.,0.866025403784439,1.,0.866025403784439,1.,0.866025403784439,1.,0.866025403784439,
1.,0.866025403784439,1.,0.866025403784439,1.,0.866025403784439,1.,0.866025403784439,
1.,0.866025403784439,1.,0.866025403784439,1.,0.866025403784439,1.,0.866025403784439,
1.,0.866025403784439,1.,0.866025403784439,1.,0.866025403784439,1.,0.866025403784439,
1.,0.866025403784439,1.,0.866025403784439,1.,0.866025403784439,1.,0.866025403784439,
1.,0.866025403784439,1.,0.866025403784439,1.,0.866025403784439,1.,0.866025403784439,
1.,0.866025403784439,1.,0.866025403784439,1.,0.866025403784439,1.,0.866025403784439,
1.,0.866025403784439,1.,0.866025403784439,1.,0.866025403784439,1.,0.866025403784439,
1.,0.866025403784439,1.,0.866025403784439,1.,0.866025403784439,1.,0.866025403784439,
1.,0.866025403784439,1.,0.866025403784439,1.,0.866025403784439,1.,0.866025403784439,
1.,0.866025403784439,1.,0.866025403784439,1.,0.866025403784439,1.,0.866025403784439,
1.,0.866025403784439,1.,0.866025403784439,1.,0.866025403784439,1.,0.866025403784439,
1.,0.866025403784439,1.,0.866025403784439,1.,0.866025403784439,1.,0.866025403784439,
1.,0.866025403784439,1.,0.866025403784439,1.,0.866025403784439,1.,0.866025403784439,
1.,0.866025403784439,1.,0.866025403784439,1.,0.866025403784439,1.,0.866025403784439,
1.,0.866025403784439,1.,0.866025403784439,1.,0.866025403784439,1.,0.866025403784439,
1.,0.866025403784439,1.,0.866025403784439,1.,0.866025403784439,1.,0.866025403784439,
1.,0.866025403784439,1.,0.866025403784439,1.,0.866025403784439,1.,0.866025403784439,
1.,0.866025403784439,1.,0.866025403784439,1.,0.866025403784439,1.,0.866025403784439,
1.,0.866025403784439,1.,0.866025403784439,1.,0.866025403784439,1.,0.866025403784439,
1.,0.866025403784439,1.,0.866025403784439,1.,0.866025403784439,1.,0.98031044488126,
0.966408234404338),(1.,0.866025403784439,1.,0.866025403784439,1.,0.866025403784439,
1.,0.866025403784439,1.,0.866025403784439,1.,0.866025403784439,1.,0.866025403784439,
1.,0.866025403784439,1.,0.866025403784439,1.,0.866025403784439,1.,0.866025403784439,
1.,0.866025403784439,1.,0.866025403784439,1.,0.866025403784439,1.,0.866025403784439,
1.,0.866025403784439,1.,0.866025403784439,1.,0.866025403784439,1.,0.866025403784439,
1.,0.866025403784439,1.,0.866025403784439,1.,0.866025403784439,1.,0.866025403784439,
1.,0.866025403784439,1.,0.866025403784439,1.,0.866025403784439,1.,0.866025403784439,
1.,0.866025403784439,1.,0.866025403784439,1.,0.866025403784439,1.,0.866025403784439,
1.,0.866025403784439,1.,0.866025403784439,1.,0.866025403784439,1.,0.866025403784439,
1.,0.866025403784439,1.,0.866025403784439,1.,0.866025403784439,1.,0.866025403784439,
1.,0.866025403784439,1.,0.866025403784439,1.,0.866025403784439,1.,0.866025403784439,
1.,0.866025403784439,1.,0.866025403784439,1.,0.866025403784439,1.,0.866025403784439,
1.,0.866025403784439,1.,0.866025403784439,1.,0.866025403784439,1.,0.866025403784439,
1.,0.866025403784439,1.,0.866025403784439,1.,0.866025403784439,1.,0.866025403784439,
1.,0.866025403784439,1.,0.866025403784439,1.,0.866025403784439,1.,0.866025403784439,
1.,0.866025403784439,1.,0.866025403784439,1.,0.866025403784439,1.,0.866025403784439,
1.,0.866025403784439,1.,0.866025403784439,1.,0.866025403784439,1.,0.866025403784439,
1.,0.866025403784439,1.,0.866025403784439,1.,0.866025403784439,1.,0.866025403784439,
1.,0.866025403784439,1.,0.866025403784439,1.,0.866025403784439,1.,0.866025403784439,
1.,0.866025403784439,1.,0.866025403784439,1.,0.866025403784439,1.,0.866025403784439,
1.,0.866025403784439,1.,0.866025403784439,1.,0.866025403784439,1.,0.866025403784439,
1.,0.866025403784439,1.,0.866025403784439,1.,0.866025403784439,1.,0.866025403784439,
1.,0.866025403784439,1.,0.866025403784439,1.,0.866025403784439,1.,0.866025403784439,
1.,0.866025403784439,1.,0.866025403784439,1.,0.866025403784439,1.,0.866025403784439,
1.,0.866025403784439,1.,0.866025403784439,1.,0.866025403784439,1.,0.866025403784439,
1.,0.866025403784439,1.,0.866025403784439,1.,0.866025403784439,1.,0.866025403784439,
1.,0.866025403784439,1.,0.866025403784439,1.,0.866025403784439,1.,0.866025403784439,
1.,0.866025403784439,1.,0.866025403784439,1.,0.866025403784439,1.,0.866025403784439,
1.,0.866025403784439,1.,0.866025403784439,1.,0.866025403784439,1.,0.866025403784439,
1.,0.866025403784439,1.,0.866025403784439,1.,0.866025403784439,1.,0.866025403784439,
1.,0.866025403784439,1.,0.866025403784439,1.,0.866025403784439,1.,0.866025403784439,
1.,0.866025403784439,1.,0.866025403784439,1.,0.866025403784439,1.,0.866025403784439,
1.,0.866025403784439,1.,0.866025403784439,1.,0.866025403784439,1.,0.866025403784439,
1.,0.866025403784439,1.,0.866025403784439,1.,0.866025403784439,1.,0.866025403784439,
1.,0.866025403784439,1.,0.866025403784439,1.,0.98031044488126,0.966408234404338)))
REPRESENTATION_ITEM('')
SURFACE()
);
#3182=(
BOUNDED_SURFACE()
B_SPLINE_SURFACE(1,2,((#260304,#260305,#260306,#260307,#260308,#260309,
#260310,#260311,#260312,#260313,#260314,#260315,#260316,#260317,#260318,
#260319,#260320,#260321,#260322,#260323,#260324,#260325,#260326,#260327,
#260328,#260329,#260330,#260331,#260332,#260333,#260334,#260335,#260336,
#260337,#260338,#260339,#260340,#260341,#260342,#260343,#260344,#260345,
#260346,#260347,#260348,#260349,#260350,#260351,#260352,#260353,#260354,
#260355,#260356,#260357,#260358,#260359,#260360,#260361,#260362,#260363,
#260364,#260365,#260366,#260367,#260368,#260369,#260370,#260371,#260372,
#260373,#260374,#260375,#260376,#260377,#260378,#260379,#260380,#260381,
#260382,#260383,#260384,#260385,#260386,#260387,#260388,#260389,#260390,
#260391,#260392,#260393,#260394,#260395,#260396,#260397,#260398,#260399,
#260400,#260401,#260402,#260403,#260404,#260405,#260406,#260407,#260408,
#260409,#260410,#260411,#260412,#260413,#260414,#260415,#260416,#260417,
#260418,#260419,#260420,#260421,#260422,#260423,#260424,#260425,#260426,
#260427,#260428,#260429,#260430,#260431,#260432,#260433,#260434,#260435,
#260436,#260437,#260438,#260439,#260440,#260441,#260442,#260443,#260444,
#260445,#260446,#260447,#260448,#260449,#260450,#260451,#260452,#260453,
#260454,#260455,#260456,#260457,#260458,#260459,#260460,#260461,#260462,
#260463,#260464,#260465,#260466,#260467,#260468,#260469,#260470,#260471,
#260472,#260473,#260474,#260475,#260476,#260477,#260478,#260479,#260480,
#260481,#260482,#260483,#260484,#260485,#260486,#260487,#260488,#260489,
#260490,#260491,#260492,#260493,#260494,#260495,#260496,#260497,#260498,
#260499,#260500,#260501,#260502,#260503,#260504,#260505,#260506,#260507,
#260508,#260509,#260510,#260511,#260512,#260513,#260514,#260515,#260516,
#260517,#260518,#260519,#260520,#260521,#260522,#260523,#260524,#260525,
#260526,#260527,#260528,#260529,#260530,#260531,#260532,#260533,#260534,
#260535,#260536,#260537,#260538,#260539,#260540,#260541,#260542,#260543,
#260544,#260545,#260546,#260547,#260548,#260549,#260550,#260551,#260552,
#260553,#260554,#260555,#260556,#260557,#260558,#260559,#260560,#260561,
#260562,#260563,#260564,#260565,#260566,#260567,#260568,#260569,#260570,
#260571,#260572,#260573,#260574,#260575,#260576,#260577,#260578,#260579,
#260580),(#260581,#260582,#260583,#260584,#260585,#260586,#260587,#260588,
#260589,#260590,#260591,#260592,#260593,#260594,#260595,#260596,#260597,
#260598,#260599,#260600,#260601,#260602,#260603,#260604,#260605,#260606,
#260607,#260608,#260609,#260610,#260611,#260612,#260613,#260614,#260615,
#260616,#260617,#260618,#260619,#260620,#260621,#260622,#260623,#260624,
#260625,#260626,#260627,#260628,#260629,#260630,#260631,#260632,#260633,
#260634,#260635,#260636,#260637,#260638,#260639,#260640,#260641,#260642,
#260643,#260644,#260645,#260646,#260647,#260648,#260649,#260650,#260651,
#260652,#260653,#260654,#260655,#260656,#260657,#260658,#260659,#260660,
#260661,#260662,#260663,#260664,#260665,#260666,#260667,#260668,#260669,
#260670,#260671,#260672,#260673,#260674,#260675,#260676,#260677,#260678,
#260679,#260680,#260681,#260682,#260683,#260684,#260685,#260686,#260687,
#260688,#260689,#260690,#260691,#260692,#260693,#260694,#260695,#260696,
#260697,#260698,#260699,#260700,#260701,#260702,#260703,#260704,#260705,
#260706,#260707,#260708,#260709,#260710,#260711,#260712,#260713,#260714,
#260715,#260716,#260717,#260718,#260719,#260720,#260721,#260722,#260723,
#260724,#260725,#260726,#260727,#260728,#260729,#260730,#260731,#260732,
#260733,#260734,#260735,#260736,#260737,#260738,#260739,#260740,#260741,
#260742,#260743,#260744,#260745,#260746,#260747,#260748,#260749,#260750,
#260751,#260752,#260753,#260754,#260755,#260756,#260757,#260758,#260759,
#260760,#260761,#260762,#260763,#260764,#260765,#260766,#260767,#260768,
#260769,#260770,#260771,#260772,#260773,#260774,#260775,#260776,#260777,
#260778,#260779,#260780,#260781,#260782,#260783,#260784,#260785,#260786,
#260787,#260788,#260789,#260790,#260791,#260792,#260793,#260794,#260795,
#260796,#260797,#260798,#260799,#260800,#260801,#260802,#260803,#260804,
#260805,#260806,#260807,#260808,#260809,#260810,#260811,#260812,#260813,
#260814,#260815,#260816,#260817,#260818,#260819,#260820,#260821,#260822,
#260823,#260824,#260825,#260826,#260827,#260828,#260829,#260830,#260831,
#260832,#260833,#260834,#260835,#260836,#260837,#260838,#260839,#260840,
#260841,#260842,#260843,#260844,#260845,#260846,#260847,#260848,#260849,
#260850,#260851,#260852,#260853,#260854,#260855,#260856,#260857)),
 .UNSPECIFIED.,.F.,.F.,.F.)
B_SPLINE_SURFACE_WITH_KNOTS((2,2),(3,2,2,2,2,2,2,2,2,2,2,2,2,2,2,2,2,2,
2,2,2,2,2,2,2,2,2,2,2,2,2,2,2,2,2,2,2,2,2,2,2,2,2,2,2,2,2,2,2,2,2,2,2,2,
2,2,2,2,2,2,2,2,2,2,2,2,2,2,2,2,2,2,2,2,2,2,2,2,2,2,2,2,2,2,2,2,2,2,2,2,
2,2,2,2,2,2,2,2,2,2,2,2,2,2,2,2,2,2,2,2,2,2,2,2,2,2,2,2,2,2,2,2,2,2,2,2,
2,2,2,2,2,2,2,2,2,2,2,2,3),(0.,1.),(0.,0.0072463768115942,0.0144927536231884,
0.0217391304347826,0.0289855072463768,0.036231884057971,0.0434782608695652,
0.0507246376811594,0.0579710144927536,0.0652173913043478,0.072463768115942,
0.0797101449275362,0.0869565217391304,0.0942028985507246,0.101449275362319,
0.108695652173913,0.115942028985507,0.123188405797101,0.130434782608696,
0.13768115942029,0.144927536231884,0.152173913043478,0.159420289855073,
0.166666666666667,0.173913043478261,0.181159420289855,0.18840579710145,
0.195652173913044,0.202898550724637,0.210144927536232,0.217391304347826,
0.224637681159421,0.231884057971014,0.239130434782609,0.246376811594203,
0.253623188405797,0.260869565217392,0.268115942028985,0.275362318840579,
0.282608695652174,0.289855072463768,0.297101449275363,0.304347826086956,
0.31159420289855,0.318840579710145,0.326086956521739,0.333333333333334,
0.340579710144927,0.347826086956521,0.355072463768116,0.36231884057971,
0.369565217391304,0.376811594202899,0.384057971014493,0.391304347826087,
0.398550724637681,0.405797101449275,0.41304347826087,0.420289855072463,
0.427536231884058,0.434782608695652,0.442028985507247,0.449275362318841,
0.456521739130435,0.463768115942029,0.471014492753623,0.478260869565218,
0.485507246376812,0.492753623188406,0.5,0.507246376811594,0.514492753623188,
0.521739130434783,0.528985507246377,0.536231884057971,0.543478260869565,
0.550724637681159,0.557971014492754,0.565217391304348,0.572463768115942,
0.579710144927536,0.586956521739131,0.594202898550725,0.601449275362319,
0.608695652173913,0.615942028985507,0.623188405797101,0.630434782608696,
0.63768115942029,0.644927536231884,0.652173913043478,0.659420289855073,
0.666666666666667,0.673913043478261,0.681159420289855,0.688405797101449,
0.695652173913044,0.702898550724638,0.710144927536232,0.717391304347826,
0.72463768115942,0.731884057971015,0.739130434782609,0.746376811594203,
0.753623188405797,0.760869565217391,0.768115942028986,0.77536231884058,
0.782608695652174,0.789855072463768,0.797101449275362,0.804347826086956,
0.811594202898551,0.818840579710145,0.826086956521739,0.833333333333333,
0.840579710144928,0.847826086956522,0.855072463768116,0.86231884057971,
0.869565217391304,0.876811594202899,0.884057971014493,0.891304347826087,
0.898550724637681,0.905797101449275,0.91304347826087,0.920289855072464,
0.927536231884058,0.934782608695652,0.942028985507246,0.94927536231884,
0.956521739130435,0.963768115942029,0.971014492753623,0.978260869565217,
0.985507246376812,0.992753623188406,0.993818495192186),.UNSPECIFIED.)
GEOMETRIC_REPRESENTATION_ITEM()
RATIONAL_B_SPLINE_SURFACE(((1.,0.866025403784439,1.,0.866025403784439,1.,
0.866025403784439,1.,0.866025403784439,1.,0.866025403784439,1.,0.866025403784439,
1.,0.866025403784439,1.,0.866025403784439,1.,0.866025403784439,1.,0.866025403784439,
1.,0.866025403784439,1.,0.866025403784439,1.,0.866025403784439,1.,0.866025403784439,
1.,0.866025403784439,1.,0.866025403784439,1.,0.866025403784439,1.,0.866025403784439,
1.,0.866025403784439,1.,0.866025403784439,1.,0.866025403784439,1.,0.866025403784439,
1.,0.866025403784439,1.,0.866025403784439,1.,0.866025403784439,1.,0.866025403784439,
1.,0.866025403784439,1.,0.866025403784439,1.,0.866025403784439,1.,0.866025403784439,
1.,0.866025403784439,1.,0.866025403784439,1.,0.866025403784439,1.,0.866025403784439,
1.,0.866025403784439,1.,0.866025403784439,1.,0.866025403784439,1.,0.866025403784439,
1.,0.866025403784439,1.,0.866025403784439,1.,0.866025403784439,1.,0.866025403784439,
1.,0.866025403784439,1.,0.866025403784439,1.,0.866025403784439,1.,0.866025403784439,
1.,0.866025403784439,1.,0.866025403784439,1.,0.866025403784439,1.,0.866025403784439,
1.,0.866025403784439,1.,0.866025403784439,1.,0.866025403784439,1.,0.866025403784439,
1.,0.866025403784439,1.,0.866025403784439,1.,0.866025403784439,1.,0.866025403784439,
1.,0.866025403784439,1.,0.866025403784439,1.,0.866025403784439,1.,0.866025403784439,
1.,0.866025403784439,1.,0.866025403784439,1.,0.866025403784439,1.,0.866025403784439,
1.,0.866025403784439,1.,0.866025403784439,1.,0.866025403784439,1.,0.866025403784439,
1.,0.866025403784439,1.,0.866025403784439,1.,0.866025403784439,1.,0.866025403784439,
1.,0.866025403784439,1.,0.866025403784439,1.,0.866025403784439,1.,0.866025403784439,
1.,0.866025403784439,1.,0.866025403784439,1.,0.866025403784439,1.,0.866025403784439,
1.,0.866025403784439,1.,0.866025403784439,1.,0.866025403784439,1.,0.866025403784439,
1.,0.866025403784439,1.,0.866025403784439,1.,0.866025403784439,1.,0.866025403784439,
1.,0.866025403784439,1.,0.866025403784439,1.,0.866025403784439,1.,0.866025403784439,
1.,0.866025403784439,1.,0.866025403784439,1.,0.866025403784439,1.,0.866025403784439,
1.,0.866025403784439,1.,0.866025403784439,1.,0.866025403784439,1.,0.866025403784439,
1.,0.866025403784439,1.,0.866025403784439,1.,0.866025403784439,1.,0.866025403784439,
1.,0.866025403784439,1.,0.866025403784439,1.,0.866025403784439,1.,0.866025403784439,
1.,0.866025403784439,1.,0.866025403784439,1.,0.866025403784439,1.,0.866025403784439,
1.,0.866025403784439,1.,0.866025403784439,1.,0.866025403784439,1.,0.866025403784439,
1.,0.866025403784439,1.,0.866025403784439,1.,0.866025403784439,1.,0.866025403784439,
1.,0.866025403784439,1.,0.866025403784439,1.,0.866025403784439,1.,0.866025403784439,
1.,0.866025403784439,1.,0.866025403784439,1.,0.866025403784439,1.,0.866025403784439,
1.,0.866025403784439,1.,0.866025403784439,1.,0.866025403784439,1.,0.866025403784439,
1.,0.866025403784439,1.,0.866025403784439,1.,0.866025403784439,1.,0.980312120051573,
0.966410600022306),(1.,0.866025403784439,1.,0.866025403784439,1.,0.866025403784439,
1.,0.866025403784439,1.,0.866025403784439,1.,0.866025403784439,1.,0.866025403784439,
1.,0.866025403784439,1.,0.866025403784439,1.,0.866025403784439,1.,0.866025403784439,
1.,0.866025403784439,1.,0.866025403784439,1.,0.866025403784439,1.,0.866025403784439,
1.,0.866025403784439,1.,0.866025403784439,1.,0.866025403784439,1.,0.866025403784439,
1.,0.866025403784439,1.,0.866025403784439,1.,0.866025403784439,1.,0.866025403784439,
1.,0.866025403784439,1.,0.866025403784439,1.,0.866025403784439,1.,0.866025403784439,
1.,0.866025403784439,1.,0.866025403784439,1.,0.866025403784439,1.,0.866025403784439,
1.,0.866025403784439,1.,0.866025403784439,1.,0.866025403784439,1.,0.866025403784439,
1.,0.866025403784439,1.,0.866025403784439,1.,0.866025403784439,1.,0.866025403784439,
1.,0.866025403784439,1.,0.866025403784439,1.,0.866025403784439,1.,0.866025403784439,
1.,0.866025403784439,1.,0.866025403784439,1.,0.866025403784439,1.,0.866025403784439,
1.,0.866025403784439,1.,0.866025403784439,1.,0.866025403784439,1.,0.866025403784439,
1.,0.866025403784439,1.,0.866025403784439,1.,0.866025403784439,1.,0.866025403784439,
1.,0.866025403784439,1.,0.866025403784439,1.,0.866025403784439,1.,0.866025403784439,
1.,0.866025403784439,1.,0.866025403784439,1.,0.866025403784439,1.,0.866025403784439,
1.,0.866025403784439,1.,0.866025403784439,1.,0.866025403784439,1.,0.866025403784439,
1.,0.866025403784439,1.,0.866025403784439,1.,0.866025403784439,1.,0.866025403784439,
1.,0.866025403784439,1.,0.866025403784439,1.,0.866025403784439,1.,0.866025403784439,
1.,0.866025403784439,1.,0.866025403784439,1.,0.866025403784439,1.,0.866025403784439,
1.,0.866025403784439,1.,0.866025403784439,1.,0.866025403784439,1.,0.866025403784439,
1.,0.866025403784439,1.,0.866025403784439,1.,0.866025403784439,1.,0.866025403784439,
1.,0.866025403784439,1.,0.866025403784439,1.,0.866025403784439,1.,0.866025403784439,
1.,0.866025403784439,1.,0.866025403784439,1.,0.866025403784439,1.,0.866025403784439,
1.,0.866025403784439,1.,0.866025403784439,1.,0.866025403784439,1.,0.866025403784439,
1.,0.866025403784439,1.,0.866025403784439,1.,0.866025403784439,1.,0.866025403784439,
1.,0.866025403784439,1.,0.866025403784439,1.,0.866025403784439,1.,0.866025403784439,
1.,0.866025403784439,1.,0.866025403784439,1.,0.866025403784439,1.,0.866025403784439,
1.,0.866025403784439,1.,0.866025403784439,1.,0.866025403784439,1.,0.866025403784439,
1.,0.866025403784439,1.,0.866025403784439,1.,0.866025403784439,1.,0.866025403784439,
1.,0.866025403784439,1.,0.866025403784439,1.,0.866025403784439,1.,0.866025403784439,
1.,0.866025403784439,1.,0.866025403784439,1.,0.866025403784439,1.,0.866025403784439,
1.,0.866025403784439,1.,0.866025403784439,1.,0.866025403784439,1.,0.866025403784439,
1.,0.866025403784439,1.,0.866025403784439,1.,0.866025403784439,1.,0.866025403784439,
1.,0.866025403784439,1.,0.866025403784439,1.,0.980312120051573,0.966410600022306)))
REPRESENTATION_ITEM('')
SURFACE()
);
#3183=(
BOUNDED_SURFACE()
B_SPLINE_SURFACE(1,2,((#260880,#260881,#260882,#260883,#260884,#260885,
#260886,#260887,#260888,#260889,#260890,#260891,#260892,#260893,#260894,
#260895,#260896,#260897,#260898,#260899,#260900,#260901,#260902,#260903,
#260904,#260905,#260906,#260907,#260908,#260909,#260910,#260911,#260912,
#260913,#260914,#260915,#260916,#260917,#260918,#260919,#260920,#260921,
#260922,#260923,#260924,#260925,#260926,#260927,#260928,#260929,#260930,
#260931,#260932,#260933,#260934,#260935,#260936,#260937,#260938,#260939,
#260940,#260941,#260942,#260943,#260944,#260945,#260946,#260947,#260948,
#260949,#260950,#260951,#260952,#260953,#260954,#260955,#260956,#260957,
#260958,#260959,#260960,#260961,#260962,#260963,#260964,#260965,#260966,
#260967,#260968,#260969,#260970,#260971,#260972,#260973,#260974,#260975,
#260976,#260977,#260978,#260979,#260980,#260981,#260982,#260983,#260984,
#260985,#260986,#260987,#260988,#260989,#260990,#260991,#260992,#260993,
#260994,#260995,#260996,#260997,#260998,#260999,#261000,#261001,#261002,
#261003,#261004,#261005,#261006,#261007,#261008,#261009,#261010,#261011,
#261012,#261013,#261014,#261015,#261016,#261017,#261018,#261019,#261020,
#261021,#261022,#261023,#261024,#261025,#261026,#261027,#261028,#261029,
#261030,#261031,#261032,#261033,#261034,#261035,#261036,#261037,#261038,
#261039,#261040,#261041,#261042,#261043,#261044,#261045,#261046,#261047,
#261048,#261049,#261050,#261051,#261052,#261053,#261054,#261055,#261056,
#261057,#261058,#261059,#261060,#261061,#261062,#261063,#261064,#261065,
#261066,#261067,#261068,#261069,#261070,#261071,#261072,#261073,#261074,
#261075,#261076,#261077,#261078,#261079,#261080,#261081,#261082,#261083,
#261084,#261085,#261086,#261087,#261088,#261089,#261090,#261091,#261092,
#261093,#261094,#261095,#261096,#261097,#261098,#261099,#261100,#261101,
#261102,#261103,#261104,#261105,#261106,#261107,#261108,#261109,#261110,
#261111,#261112,#261113,#261114,#261115,#261116,#261117,#261118,#261119,
#261120,#261121,#261122,#261123,#261124,#261125,#261126,#261127,#261128,
#261129,#261130,#261131,#261132,#261133,#261134,#261135,#261136,#261137,
#261138,#261139,#261140,#261141,#261142,#261143,#261144,#261145,#261146,
#261147,#261148,#261149,#261150,#261151,#261152,#261153,#261154,#261155,
#261156),(#261157,#261158,#261159,#261160,#261161,#261162,#261163,#261164,
#261165,#261166,#261167,#261168,#261169,#261170,#261171,#261172,#261173,
#261174,#261175,#261176,#261177,#261178,#261179,#261180,#261181,#261182,
#261183,#261184,#261185,#261186,#261187,#261188,#261189,#261190,#261191,
#261192,#261193,#261194,#261195,#261196,#261197,#261198,#261199,#261200,
#261201,#261202,#261203,#261204,#261205,#261206,#261207,#261208,#261209,
#261210,#261211,#261212,#261213,#261214,#261215,#261216,#261217,#261218,
#261219,#261220,#261221,#261222,#261223,#261224,#261225,#261226,#261227,
#261228,#261229,#261230,#261231,#261232,#261233,#261234,#261235,#261236,
#261237,#261238,#261239,#261240,#261241,#261242,#261243,#261244,#261245,
#261246,#261247,#261248,#261249,#261250,#261251,#261252,#261253,#261254,
#261255,#261256,#261257,#261258,#261259,#261260,#261261,#261262,#261263,
#261264,#261265,#261266,#261267,#261268,#261269,#261270,#261271,#261272,
#261273,#261274,#261275,#261276,#261277,#261278,#261279,#261280,#261281,
#261282,#261283,#261284,#261285,#261286,#261287,#261288,#261289,#261290,
#261291,#261292,#261293,#261294,#261295,#261296,#261297,#261298,#261299,
#261300,#261301,#261302,#261303,#261304,#261305,#261306,#261307,#261308,
#261309,#261310,#261311,#261312,#261313,#261314,#261315,#261316,#261317,
#261318,#261319,#261320,#261321,#261322,#261323,#261324,#261325,#261326,
#261327,#261328,#261329,#261330,#261331,#261332,#261333,#261334,#261335,
#261336,#261337,#261338,#261339,#261340,#261341,#261342,#261343,#261344,
#261345,#261346,#261347,#261348,#261349,#261350,#261351,#261352,#261353,
#261354,#261355,#261356,#261357,#261358,#261359,#261360,#261361,#261362,
#261363,#261364,#261365,#261366,#261367,#261368,#261369,#261370,#261371,
#261372,#261373,#261374,#261375,#261376,#261377,#261378,#261379,#261380,
#261381,#261382,#261383,#261384,#261385,#261386,#261387,#261388,#261389,
#261390,#261391,#261392,#261393,#261394,#261395,#261396,#261397,#261398,
#261399,#261400,#261401,#261402,#261403,#261404,#261405,#261406,#261407,
#261408,#261409,#261410,#261411,#261412,#261413,#261414,#261415,#261416,
#261417,#261418,#261419,#261420,#261421,#261422,#261423,#261424,#261425,
#261426,#261427,#261428,#261429,#261430,#261431,#261432,#261433)),
 .UNSPECIFIED.,.F.,.F.,.F.)
B_SPLINE_SURFACE_WITH_KNOTS((2,2),(3,2,2,2,2,2,2,2,2,2,2,2,2,2,2,2,2,2,
2,2,2,2,2,2,2,2,2,2,2,2,2,2,2,2,2,2,2,2,2,2,2,2,2,2,2,2,2,2,2,2,2,2,2,2,
2,2,2,2,2,2,2,2,2,2,2,2,2,2,2,2,2,2,2,2,2,2,2,2,2,2,2,2,2,2,2,2,2,2,2,2,
2,2,2,2,2,2,2,2,2,2,2,2,2,2,2,2,2,2,2,2,2,2,2,2,2,2,2,2,2,2,2,2,2,2,2,2,
2,2,2,2,2,2,2,2,2,2,2,2,3),(0.,1.00000038195933),(0.,0.0072463768115942,
0.0144927536231884,0.0217391304347826,0.0289855072463768,0.036231884057971,
0.0434782608695652,0.0507246376811594,0.0579710144927536,0.0652173913043478,
0.072463768115942,0.0797101449275362,0.0869565217391304,0.0942028985507246,
0.101449275362319,0.108695652173913,0.115942028985507,0.123188405797101,
0.130434782608696,0.13768115942029,0.144927536231884,0.152173913043478,
0.159420289855073,0.166666666666667,0.173913043478261,0.181159420289855,
0.18840579710145,0.195652173913044,0.202898550724637,0.210144927536232,
0.217391304347826,0.224637681159421,0.231884057971014,0.239130434782609,
0.246376811594203,0.253623188405797,0.260869565217392,0.268115942028985,
0.275362318840579,0.282608695652174,0.289855072463768,0.297101449275363,
0.304347826086956,0.31159420289855,0.318840579710145,0.326086956521739,
0.333333333333334,0.340579710144927,0.347826086956521,0.355072463768116,
0.36231884057971,0.369565217391304,0.376811594202899,0.384057971014493,
0.391304347826087,0.398550724637681,0.405797101449275,0.41304347826087,
0.420289855072463,0.427536231884058,0.434782608695652,0.442028985507247,
0.449275362318841,0.456521739130435,0.463768115942029,0.471014492753623,
0.478260869565218,0.485507246376812,0.492753623188406,0.5,0.507246376811594,
0.514492753623188,0.521739130434783,0.528985507246377,0.536231884057971,
0.543478260869565,0.550724637681159,0.557971014492754,0.565217391304348,
0.572463768115942,0.579710144927536,0.586956521739131,0.594202898550725,
0.601449275362319,0.608695652173913,0.615942028985507,0.623188405797101,
0.630434782608696,0.63768115942029,0.644927536231884,0.652173913043478,
0.659420289855073,0.666666666666667,0.673913043478261,0.681159420289855,
0.688405797101449,0.695652173913044,0.702898550724638,0.710144927536232,
0.717391304347826,0.72463768115942,0.731884057971015,0.739130434782609,
0.746376811594203,0.753623188405797,0.760869565217391,0.768115942028986,
0.77536231884058,0.782608695652174,0.789855072463768,0.797101449275362,
0.804347826086956,0.811594202898551,0.818840579710145,0.826086956521739,
0.833333333333333,0.840579710144928,0.847826086956522,0.855072463768116,
0.86231884057971,0.869565217391304,0.876811594202899,0.884057971014493,
0.891304347826087,0.898550724637681,0.905797101449275,0.91304347826087,
0.920289855072464,0.927536231884058,0.934782608695652,0.942028985507246,
0.94927536231884,0.956521739130435,0.963768115942029,0.971014492753623,
0.978260869565217,0.985507246376812,0.992753623188406,0.993818495192186),
 .UNSPECIFIED.)
GEOMETRIC_REPRESENTATION_ITEM()
RATIONAL_B_SPLINE_SURFACE(((1.,0.866025403784439,1.,0.866025403784439,1.,
0.866025403784439,1.,0.866025403784439,1.,0.866025403784439,1.,0.866025403784439,
1.,0.866025403784439,1.,0.866025403784439,1.,0.866025403784439,1.,0.866025403784439,
1.,0.866025403784439,1.,0.866025403784439,1.,0.866025403784439,1.,0.866025403784439,
1.,0.866025403784439,1.,0.866025403784439,1.,0.866025403784439,1.,0.866025403784439,
1.,0.866025403784439,1.,0.866025403784439,1.,0.866025403784439,1.,0.866025403784439,
1.,0.866025403784439,1.,0.866025403784439,1.,0.866025403784439,1.,0.866025403784439,
1.,0.866025403784439,1.,0.866025403784439,1.,0.866025403784439,1.,0.866025403784439,
1.,0.866025403784439,1.,0.866025403784439,1.,0.866025403784439,1.,0.866025403784439,
1.,0.866025403784439,1.,0.866025403784439,1.,0.866025403784439,1.,0.866025403784439,
1.,0.866025403784439,1.,0.866025403784439,1.,0.866025403784439,1.,0.866025403784439,
1.,0.866025403784439,1.,0.866025403784439,1.,0.866025403784439,1.,0.866025403784439,
1.,0.866025403784439,1.,0.866025403784439,1.,0.866025403784439,1.,0.866025403784439,
1.,0.866025403784439,1.,0.866025403784439,1.,0.866025403784439,1.,0.866025403784439,
1.,0.866025403784439,1.,0.866025403784439,1.,0.866025403784439,1.,0.866025403784439,
1.,0.866025403784439,1.,0.866025403784439,1.,0.866025403784439,1.,0.866025403784439,
1.,0.866025403784439,1.,0.866025403784439,1.,0.866025403784439,1.,0.866025403784439,
1.,0.866025403784439,1.,0.866025403784439,1.,0.866025403784439,1.,0.866025403784439,
1.,0.866025403784439,1.,0.866025403784439,1.,0.866025403784439,1.,0.866025403784439,
1.,0.866025403784439,1.,0.866025403784439,1.,0.866025403784439,1.,0.866025403784439,
1.,0.866025403784439,1.,0.866025403784439,1.,0.866025403784439,1.,0.866025403784439,
1.,0.866025403784439,1.,0.866025403784439,1.,0.866025403784439,1.,0.866025403784439,
1.,0.866025403784439,1.,0.866025403784439,1.,0.866025403784439,1.,0.866025403784439,
1.,0.866025403784439,1.,0.866025403784439,1.,0.866025403784439,1.,0.866025403784439,
1.,0.866025403784439,1.,0.866025403784439,1.,0.866025403784439,1.,0.866025403784439,
1.,0.866025403784439,1.,0.866025403784439,1.,0.866025403784439,1.,0.866025403784439,
1.,0.866025403784439,1.,0.866025403784439,1.,0.866025403784439,1.,0.866025403784439,
1.,0.866025403784439,1.,0.866025403784439,1.,0.866025403784439,1.,0.866025403784439,
1.,0.866025403784439,1.,0.866025403784439,1.,0.866025403784439,1.,0.866025403784439,
1.,0.866025403784439,1.,0.866025403784439,1.,0.866025403784439,1.,0.866025403784439,
1.,0.866025403784439,1.,0.866025403784439,1.,0.866025403784439,1.,0.866025403784439,
1.,0.866025403784439,1.,0.866025403784439,1.,0.866025403784439,1.,0.866025403784439,
1.,0.866025403784439,1.,0.866025403784439,1.,0.866025403784439,1.,0.866025403784439,
1.,0.866025403784439,1.,0.866025403784439,1.,0.866025403784439,1.,0.866025403784439,
1.,0.866025403784439,1.,0.866025403784439,1.,0.866025403784439,1.,0.980312120051573,
0.966410600022306),(1.,0.866025403784439,1.,0.866025403784439,1.,0.866025403784439,
1.,0.866025403784439,1.,0.866025403784439,1.,0.866025403784439,1.,0.866025403784439,
1.,0.866025403784439,1.,0.866025403784439,1.,0.866025403784439,1.,0.866025403784439,
1.,0.866025403784439,1.,0.866025403784439,1.,0.866025403784439,1.,0.866025403784439,
1.,0.866025403784439,1.,0.866025403784439,1.,0.866025403784439,1.,0.866025403784439,
1.,0.866025403784439,1.,0.866025403784439,1.,0.866025403784439,1.,0.866025403784439,
1.,0.866025403784439,1.,0.866025403784439,1.,0.866025403784439,1.,0.866025403784439,
1.,0.866025403784439,1.,0.866025403784439,1.,0.866025403784439,1.,0.866025403784439,
1.,0.866025403784439,1.,0.866025403784439,1.,0.866025403784439,1.,0.866025403784439,
1.,0.866025403784439,1.,0.866025403784439,1.,0.866025403784439,1.,0.866025403784439,
1.,0.866025403784439,1.,0.866025403784439,1.,0.866025403784439,1.,0.866025403784439,
1.,0.866025403784439,1.,0.866025403784439,1.,0.866025403784439,1.,0.866025403784439,
1.,0.866025403784439,1.,0.866025403784439,1.,0.866025403784439,1.,0.866025403784439,
1.,0.866025403784439,1.,0.866025403784439,1.,0.866025403784439,1.,0.866025403784439,
1.,0.866025403784439,1.,0.866025403784439,1.,0.866025403784439,1.,0.866025403784439,
1.,0.866025403784439,1.,0.866025403784439,1.,0.866025403784439,1.,0.866025403784439,
1.,0.866025403784439,1.,0.866025403784439,1.,0.866025403784439,1.,0.866025403784439,
1.,0.866025403784439,1.,0.866025403784439,1.,0.866025403784439,1.,0.866025403784439,
1.,0.866025403784439,1.,0.866025403784439,1.,0.866025403784439,1.,0.866025403784439,
1.,0.866025403784439,1.,0.866025403784439,1.,0.866025403784439,1.,0.866025403784439,
1.,0.866025403784439,1.,0.866025403784439,1.,0.866025403784439,1.,0.866025403784439,
1.,0.866025403784439,1.,0.866025403784439,1.,0.866025403784439,1.,0.866025403784439,
1.,0.866025403784439,1.,0.866025403784439,1.,0.866025403784439,1.,0.866025403784439,
1.,0.866025403784439,1.,0.866025403784439,1.,0.866025403784439,1.,0.866025403784439,
1.,0.866025403784439,1.,0.866025403784439,1.,0.866025403784439,1.,0.866025403784439,
1.,0.866025403784439,1.,0.866025403784439,1.,0.866025403784439,1.,0.866025403784439,
1.,0.866025403784439,1.,0.866025403784439,1.,0.866025403784439,1.,0.866025403784439,
1.,0.866025403784439,1.,0.866025403784439,1.,0.866025403784439,1.,0.866025403784439,
1.,0.866025403784439,1.,0.866025403784439,1.,0.866025403784439,1.,0.866025403784439,
1.,0.866025403784439,1.,0.866025403784439,1.,0.866025403784439,1.,0.866025403784439,
1.,0.866025403784439,1.,0.866025403784439,1.,0.866025403784439,1.,0.866025403784439,
1.,0.866025403784439,1.,0.866025403784439,1.,0.866025403784439,1.,0.866025403784439,
1.,0.866025403784439,1.,0.866025403784439,1.,0.866025403784439,1.,0.866025403784439,
1.,0.866025403784439,1.,0.866025403784439,1.,0.866025403784439,1.,0.866025403784439,
1.,0.866025403784439,1.,0.866025403784439,1.,0.980312120051573,0.966410600022306)))
REPRESENTATION_ITEM('')
SURFACE()
);
#3184=(
BOUNDED_SURFACE()
B_SPLINE_SURFACE(1,2,((#261448,#261449,#261450,#261451,#261452,#261453,
#261454,#261455,#261456,#261457,#261458,#261459,#261460,#261461,#261462,
#261463,#261464,#261465,#261466,#261467,#261468,#261469,#261470,#261471,
#261472,#261473,#261474,#261475,#261476,#261477,#261478,#261479,#261480,
#261481,#261482,#261483,#261484,#261485,#261486,#261487,#261488,#261489,
#261490,#261491,#261492,#261493,#261494,#261495,#261496,#261497,#261498,
#261499,#261500,#261501,#261502,#261503,#261504,#261505,#261506,#261507,
#261508,#261509,#261510,#261511,#261512,#261513,#261514,#261515,#261516,
#261517,#261518,#261519,#261520,#261521,#261522,#261523,#261524,#261525,
#261526,#261527,#261528,#261529,#261530,#261531,#261532,#261533,#261534,
#261535,#261536,#261537,#261538,#261539,#261540,#261541,#261542,#261543,
#261544,#261545,#261546,#261547,#261548,#261549,#261550,#261551,#261552,
#261553,#261554,#261555,#261556,#261557,#261558,#261559,#261560,#261561,
#261562,#261563,#261564,#261565,#261566,#261567,#261568,#261569,#261570,
#261571,#261572,#261573,#261574,#261575,#261576,#261577,#261578,#261579,
#261580,#261581,#261582,#261583,#261584,#261585,#261586,#261587,#261588,
#261589,#261590,#261591,#261592,#261593,#261594,#261595,#261596,#261597,
#261598,#261599,#261600,#261601,#261602,#261603,#261604,#261605,#261606,
#261607,#261608,#261609,#261610,#261611,#261612,#261613,#261614,#261615,
#261616,#261617,#261618,#261619,#261620,#261621,#261622,#261623,#261624,
#261625,#261626,#261627,#261628,#261629,#261630,#261631,#261632,#261633,
#261634,#261635,#261636,#261637,#261638,#261639,#261640,#261641,#261642,
#261643,#261644,#261645,#261646,#261647,#261648,#261649,#261650,#261651,
#261652,#261653,#261654,#261655,#261656,#261657,#261658,#261659,#261660,
#261661,#261662,#261663,#261664,#261665,#261666,#261667,#261668,#261669,
#261670,#261671,#261672,#261673,#261674,#261675,#261676,#261677,#261678,
#261679,#261680,#261681,#261682,#261683,#261684,#261685,#261686,#261687,
#261688,#261689,#261690,#261691,#261692,#261693,#261694,#261695,#261696,
#261697,#261698,#261699,#261700,#261701,#261702,#261703,#261704,#261705,
#261706,#261707,#261708,#261709,#261710,#261711,#261712,#261713,#261714,
#261715,#261716,#261717,#261718,#261719,#261720,#261721,#261722,#261723,
#261724),(#261725,#261726,#261727,#261728,#261729,#261730,#261731,#261732,
#261733,#261734,#261735,#261736,#261737,#261738,#261739,#261740,#261741,
#261742,#261743,#261744,#261745,#261746,#261747,#261748,#261749,#261750,
#261751,#261752,#261753,#261754,#261755,#261756,#261757,#261758,#261759,
#261760,#261761,#261762,#261763,#261764,#261765,#261766,#261767,#261768,
#261769,#261770,#261771,#261772,#261773,#261774,#261775,#261776,#261777,
#261778,#261779,#261780,#261781,#261782,#261783,#261784,#261785,#261786,
#261787,#261788,#261789,#261790,#261791,#261792,#261793,#261794,#261795,
#261796,#261797,#261798,#261799,#261800,#261801,#261802,#261803,#261804,
#261805,#261806,#261807,#261808,#261809,#261810,#261811,#261812,#261813,
#261814,#261815,#261816,#261817,#261818,#261819,#261820,#261821,#261822,
#261823,#261824,#261825,#261826,#261827,#261828,#261829,#261830,#261831,
#261832,#261833,#261834,#261835,#261836,#261837,#261838,#261839,#261840,
#261841,#261842,#261843,#261844,#261845,#261846,#261847,#261848,#261849,
#261850,#261851,#261852,#261853,#261854,#261855,#261856,#261857,#261858,
#261859,#261860,#261861,#261862,#261863,#261864,#261865,#261866,#261867,
#261868,#261869,#261870,#261871,#261872,#261873,#261874,#261875,#261876,
#261877,#261878,#261879,#261880,#261881,#261882,#261883,#261884,#261885,
#261886,#261887,#261888,#261889,#261890,#261891,#261892,#261893,#261894,
#261895,#261896,#261897,#261898,#261899,#261900,#261901,#261902,#261903,
#261904,#261905,#261906,#261907,#261908,#261909,#261910,#261911,#261912,
#261913,#261914,#261915,#261916,#261917,#261918,#261919,#261920,#261921,
#261922,#261923,#261924,#261925,#261926,#261927,#261928,#261929,#261930,
#261931,#261932,#261933,#261934,#261935,#261936,#261937,#261938,#261939,
#261940,#261941,#261942,#261943,#261944,#261945,#261946,#261947,#261948,
#261949,#261950,#261951,#261952,#261953,#261954,#261955,#261956,#261957,
#261958,#261959,#261960,#261961,#261962,#261963,#261964,#261965,#261966,
#261967,#261968,#261969,#261970,#261971,#261972,#261973,#261974,#261975,
#261976,#261977,#261978,#261979,#261980,#261981,#261982,#261983,#261984,
#261985,#261986,#261987,#261988,#261989,#261990,#261991,#261992,#261993,
#261994,#261995,#261996,#261997,#261998,#261999,#262000,#262001)),
 .UNSPECIFIED.,.F.,.F.,.F.)
B_SPLINE_SURFACE_WITH_KNOTS((2,2),(3,2,2,2,2,2,2,2,2,2,2,2,2,2,2,2,2,2,
2,2,2,2,2,2,2,2,2,2,2,2,2,2,2,2,2,2,2,2,2,2,2,2,2,2,2,2,2,2,2,2,2,2,2,2,
2,2,2,2,2,2,2,2,2,2,2,2,2,2,2,2,2,2,2,2,2,2,2,2,2,2,2,2,2,2,2,2,2,2,2,2,
2,2,2,2,2,2,2,2,2,2,2,2,2,2,2,2,2,2,2,2,2,2,2,2,2,2,2,2,2,2,2,2,2,2,2,2,
2,2,2,2,2,2,2,2,2,2,2,2,3),(0.,1.),(0.,0.0072463768115942,0.0144927536231884,
0.0217391304347826,0.0289855072463768,0.036231884057971,0.0434782608695652,
0.0507246376811594,0.0579710144927536,0.0652173913043478,0.072463768115942,
0.0797101449275362,0.0869565217391304,0.0942028985507246,0.101449275362319,
0.108695652173913,0.115942028985507,0.123188405797101,0.130434782608696,
0.13768115942029,0.144927536231884,0.152173913043478,0.159420289855073,
0.166666666666667,0.173913043478261,0.181159420289855,0.18840579710145,
0.195652173913044,0.202898550724637,0.210144927536232,0.217391304347826,
0.224637681159421,0.231884057971014,0.239130434782609,0.246376811594203,
0.253623188405797,0.260869565217392,0.268115942028985,0.275362318840579,
0.282608695652174,0.289855072463768,0.297101449275363,0.304347826086956,
0.31159420289855,0.318840579710145,0.326086956521739,0.333333333333334,
0.340579710144927,0.347826086956521,0.355072463768116,0.36231884057971,
0.369565217391304,0.376811594202899,0.384057971014493,0.391304347826087,
0.398550724637681,0.405797101449275,0.41304347826087,0.420289855072463,
0.427536231884058,0.434782608695652,0.442028985507247,0.449275362318841,
0.456521739130435,0.463768115942029,0.471014492753623,0.478260869565218,
0.485507246376812,0.492753623188406,0.5,0.507246376811594,0.514492753623188,
0.521739130434783,0.528985507246377,0.536231884057971,0.543478260869565,
0.550724637681159,0.557971014492754,0.565217391304348,0.572463768115942,
0.579710144927536,0.586956521739131,0.594202898550725,0.601449275362319,
0.608695652173913,0.615942028985507,0.623188405797101,0.630434782608696,
0.63768115942029,0.644927536231884,0.652173913043478,0.659420289855073,
0.666666666666667,0.673913043478261,0.681159420289855,0.688405797101449,
0.695652173913044,0.702898550724638,0.710144927536232,0.717391304347826,
0.72463768115942,0.731884057971015,0.739130434782609,0.746376811594203,
0.753623188405797,0.760869565217391,0.768115942028986,0.77536231884058,
0.782608695652174,0.789855072463768,0.797101449275362,0.804347826086956,
0.811594202898551,0.818840579710145,0.826086956521739,0.833333333333333,
0.840579710144928,0.847826086956522,0.855072463768116,0.86231884057971,
0.869565217391304,0.876811594202899,0.884057971014493,0.891304347826087,
0.898550724637681,0.905797101449275,0.91304347826087,0.920289855072464,
0.927536231884058,0.934782608695652,0.942028985507246,0.94927536231884,
0.956521739130435,0.963768115942029,0.971014492753623,0.978260869565217,
0.985507246376812,0.992753623188406,0.993818585798284),.UNSPECIFIED.)
GEOMETRIC_REPRESENTATION_ITEM()
RATIONAL_B_SPLINE_SURFACE(((1.,0.866025403784439,1.,0.866025403784439,1.,
0.866025403784439,1.,0.866025403784439,1.,0.866025403784439,1.,0.866025403784439,
1.,0.866025403784439,1.,0.866025403784439,1.,0.866025403784439,1.,0.866025403784439,
1.,0.866025403784439,1.,0.866025403784439,1.,0.866025403784439,1.,0.866025403784439,
1.,0.866025403784439,1.,0.866025403784439,1.,0.866025403784439,1.,0.866025403784439,
1.,0.866025403784439,1.,0.866025403784439,1.,0.866025403784439,1.,0.866025403784439,
1.,0.866025403784439,1.,0.866025403784439,1.,0.866025403784439,1.,0.866025403784439,
1.,0.866025403784439,1.,0.866025403784439,1.,0.866025403784439,1.,0.866025403784439,
1.,0.866025403784439,1.,0.866025403784439,1.,0.866025403784439,1.,0.866025403784439,
1.,0.866025403784439,1.,0.866025403784439,1.,0.866025403784439,1.,0.866025403784439,
1.,0.866025403784439,1.,0.866025403784439,1.,0.866025403784439,1.,0.866025403784439,
1.,0.866025403784439,1.,0.866025403784439,1.,0.866025403784439,1.,0.866025403784439,
1.,0.866025403784439,1.,0.866025403784439,1.,0.866025403784439,1.,0.866025403784439,
1.,0.866025403784439,1.,0.866025403784439,1.,0.866025403784439,1.,0.866025403784439,
1.,0.866025403784439,1.,0.866025403784439,1.,0.866025403784439,1.,0.866025403784439,
1.,0.866025403784439,1.,0.866025403784439,1.,0.866025403784439,1.,0.866025403784439,
1.,0.866025403784439,1.,0.866025403784439,1.,0.866025403784439,1.,0.866025403784439,
1.,0.866025403784439,1.,0.866025403784439,1.,0.866025403784439,1.,0.866025403784439,
1.,0.866025403784439,1.,0.866025403784439,1.,0.866025403784439,1.,0.866025403784439,
1.,0.866025403784439,1.,0.866025403784439,1.,0.866025403784439,1.,0.866025403784439,
1.,0.866025403784439,1.,0.866025403784439,1.,0.866025403784439,1.,0.866025403784439,
1.,0.866025403784439,1.,0.866025403784439,1.,0.866025403784439,1.,0.866025403784439,
1.,0.866025403784439,1.,0.866025403784439,1.,0.866025403784439,1.,0.866025403784439,
1.,0.866025403784439,1.,0.866025403784439,1.,0.866025403784439,1.,0.866025403784439,
1.,0.866025403784439,1.,0.866025403784439,1.,0.866025403784439,1.,0.866025403784439,
1.,0.866025403784439,1.,0.866025403784439,1.,0.866025403784439,1.,0.866025403784439,
1.,0.866025403784439,1.,0.866025403784439,1.,0.866025403784439,1.,0.866025403784439,
1.,0.866025403784439,1.,0.866025403784439,1.,0.866025403784439,1.,0.866025403784439,
1.,0.866025403784439,1.,0.866025403784439,1.,0.866025403784439,1.,0.866025403784439,
1.,0.866025403784439,1.,0.866025403784439,1.,0.866025403784439,1.,0.866025403784439,
1.,0.866025403784439,1.,0.866025403784439,1.,0.866025403784439,1.,0.866025403784439,
1.,0.866025403784439,1.,0.866025403784439,1.,0.866025403784439,1.,0.866025403784439,
1.,0.866025403784439,1.,0.866025403784439,1.,0.866025403784439,1.,0.866025403784439,
1.,0.866025403784439,1.,0.866025403784439,1.,0.866025403784439,1.,0.866025403784439,
1.,0.866025403784439,1.,0.866025403784439,1.,0.866025403784439,1.,0.98031044488126,
0.966408234404338),(1.,0.866025403784439,1.,0.866025403784439,1.,0.866025403784439,
1.,0.866025403784439,1.,0.866025403784439,1.,0.866025403784439,1.,0.866025403784439,
1.,0.866025403784439,1.,0.866025403784439,1.,0.866025403784439,1.,0.866025403784439,
1.,0.866025403784439,1.,0.866025403784439,1.,0.866025403784439,1.,0.866025403784439,
1.,0.866025403784439,1.,0.866025403784439,1.,0.866025403784439,1.,0.866025403784439,
1.,0.866025403784439,1.,0.866025403784439,1.,0.866025403784439,1.,0.866025403784439,
1.,0.866025403784439,1.,0.866025403784439,1.,0.866025403784439,1.,0.866025403784439,
1.,0.866025403784439,1.,0.866025403784439,1.,0.866025403784439,1.,0.866025403784439,
1.,0.866025403784439,1.,0.866025403784439,1.,0.866025403784439,1.,0.866025403784439,
1.,0.866025403784439,1.,0.866025403784439,1.,0.866025403784439,1.,0.866025403784439,
1.,0.866025403784439,1.,0.866025403784439,1.,0.866025403784439,1.,0.866025403784439,
1.,0.866025403784439,1.,0.866025403784439,1.,0.866025403784439,1.,0.866025403784439,
1.,0.866025403784439,1.,0.866025403784439,1.,0.866025403784439,1.,0.866025403784439,
1.,0.866025403784439,1.,0.866025403784439,1.,0.866025403784439,1.,0.866025403784439,
1.,0.866025403784439,1.,0.866025403784439,1.,0.866025403784439,1.,0.866025403784439,
1.,0.866025403784439,1.,0.866025403784439,1.,0.866025403784439,1.,0.866025403784439,
1.,0.866025403784439,1.,0.866025403784439,1.,0.866025403784439,1.,0.866025403784439,
1.,0.866025403784439,1.,0.866025403784439,1.,0.866025403784439,1.,0.866025403784439,
1.,0.866025403784439,1.,0.866025403784439,1.,0.866025403784439,1.,0.866025403784439,
1.,0.866025403784439,1.,0.866025403784439,1.,0.866025403784439,1.,0.866025403784439,
1.,0.866025403784439,1.,0.866025403784439,1.,0.866025403784439,1.,0.866025403784439,
1.,0.866025403784439,1.,0.866025403784439,1.,0.866025403784439,1.,0.866025403784439,
1.,0.866025403784439,1.,0.866025403784439,1.,0.866025403784439,1.,0.866025403784439,
1.,0.866025403784439,1.,0.866025403784439,1.,0.866025403784439,1.,0.866025403784439,
1.,0.866025403784439,1.,0.866025403784439,1.,0.866025403784439,1.,0.866025403784439,
1.,0.866025403784439,1.,0.866025403784439,1.,0.866025403784439,1.,0.866025403784439,
1.,0.866025403784439,1.,0.866025403784439,1.,0.866025403784439,1.,0.866025403784439,
1.,0.866025403784439,1.,0.866025403784439,1.,0.866025403784439,1.,0.866025403784439,
1.,0.866025403784439,1.,0.866025403784439,1.,0.866025403784439,1.,0.866025403784439,
1.,0.866025403784439,1.,0.866025403784439,1.,0.866025403784439,1.,0.866025403784439,
1.,0.866025403784439,1.,0.866025403784439,1.,0.866025403784439,1.,0.866025403784439,
1.,0.866025403784439,1.,0.866025403784439,1.,0.866025403784439,1.,0.866025403784439,
1.,0.866025403784439,1.,0.866025403784439,1.,0.866025403784439,1.,0.866025403784439,
1.,0.866025403784439,1.,0.866025403784439,1.,0.866025403784439,1.,0.866025403784439,
1.,0.866025403784439,1.,0.866025403784439,1.,0.98031044488126,0.966408234404338)))
REPRESENTATION_ITEM('')
SURFACE()
);
#3185=(
BOUNDED_SURFACE()
B_SPLINE_SURFACE(1,2,((#262037,#262038,#262039,#262040,#262041,#262042,
#262043,#262044,#262045,#262046,#262047,#262048,#262049,#262050,#262051,
#262052,#262053,#262054,#262055,#262056,#262057,#262058,#262059,#262060,
#262061,#262062,#262063,#262064,#262065,#262066,#262067,#262068,#262069,
#262070,#262071,#262072,#262073,#262074,#262075,#262076,#262077,#262078,
#262079,#262080,#262081,#262082,#262083,#262084,#262085,#262086,#262087,
#262088,#262089,#262090,#262091,#262092,#262093,#262094,#262095,#262096,
#262097,#262098,#262099,#262100,#262101,#262102,#262103,#262104,#262105,
#262106,#262107,#262108,#262109,#262110,#262111,#262112,#262113,#262114,
#262115,#262116,#262117,#262118,#262119,#262120,#262121,#262122,#262123,
#262124,#262125,#262126,#262127,#262128,#262129,#262130,#262131,#262132,
#262133,#262134,#262135,#262136,#262137,#262138,#262139,#262140,#262141,
#262142,#262143,#262144,#262145,#262146,#262147,#262148,#262149,#262150,
#262151,#262152,#262153,#262154,#262155,#262156,#262157,#262158,#262159,
#262160,#262161,#262162,#262163,#262164,#262165,#262166,#262167,#262168,
#262169,#262170,#262171,#262172,#262173,#262174,#262175,#262176,#262177,
#262178,#262179,#262180,#262181,#262182,#262183,#262184,#262185,#262186,
#262187,#262188,#262189,#262190,#262191,#262192,#262193,#262194,#262195,
#262196,#262197,#262198,#262199,#262200,#262201,#262202,#262203,#262204,
#262205,#262206,#262207,#262208,#262209,#262210,#262211,#262212,#262213,
#262214,#262215,#262216,#262217,#262218,#262219,#262220,#262221,#262222,
#262223,#262224,#262225,#262226,#262227,#262228,#262229,#262230,#262231,
#262232,#262233,#262234,#262235,#262236,#262237,#262238,#262239,#262240,
#262241,#262242,#262243,#262244,#262245,#262246,#262247,#262248,#262249,
#262250,#262251,#262252,#262253,#262254,#262255,#262256,#262257,#262258,
#262259,#262260,#262261,#262262,#262263,#262264,#262265,#262266,#262267,
#262268,#262269,#262270,#262271,#262272,#262273,#262274,#262275,#262276,
#262277,#262278,#262279,#262280,#262281,#262282,#262283,#262284,#262285,
#262286,#262287,#262288,#262289,#262290,#262291,#262292,#262293,#262294,
#262295,#262296,#262297,#262298,#262299,#262300,#262301,#262302,#262303,
#262304,#262305,#262306,#262307,#262308,#262309,#262310,#262311,#262312,
#262313),(#262314,#262315,#262316,#262317,#262318,#262319,#262320,#262321,
#262322,#262323,#262324,#262325,#262326,#262327,#262328,#262329,#262330,
#262331,#262332,#262333,#262334,#262335,#262336,#262337,#262338,#262339,
#262340,#262341,#262342,#262343,#262344,#262345,#262346,#262347,#262348,
#262349,#262350,#262351,#262352,#262353,#262354,#262355,#262356,#262357,
#262358,#262359,#262360,#262361,#262362,#262363,#262364,#262365,#262366,
#262367,#262368,#262369,#262370,#262371,#262372,#262373,#262374,#262375,
#262376,#262377,#262378,#262379,#262380,#262381,#262382,#262383,#262384,
#262385,#262386,#262387,#262388,#262389,#262390,#262391,#262392,#262393,
#262394,#262395,#262396,#262397,#262398,#262399,#262400,#262401,#262402,
#262403,#262404,#262405,#262406,#262407,#262408,#262409,#262410,#262411,
#262412,#262413,#262414,#262415,#262416,#262417,#262418,#262419,#262420,
#262421,#262422,#262423,#262424,#262425,#262426,#262427,#262428,#262429,
#262430,#262431,#262432,#262433,#262434,#262435,#262436,#262437,#262438,
#262439,#262440,#262441,#262442,#262443,#262444,#262445,#262446,#262447,
#262448,#262449,#262450,#262451,#262452,#262453,#262454,#262455,#262456,
#262457,#262458,#262459,#262460,#262461,#262462,#262463,#262464,#262465,
#262466,#262467,#262468,#262469,#262470,#262471,#262472,#262473,#262474,
#262475,#262476,#262477,#262478,#262479,#262480,#262481,#262482,#262483,
#262484,#262485,#262486,#262487,#262488,#262489,#262490,#262491,#262492,
#262493,#262494,#262495,#262496,#262497,#262498,#262499,#262500,#262501,
#262502,#262503,#262504,#262505,#262506,#262507,#262508,#262509,#262510,
#262511,#262512,#262513,#262514,#262515,#262516,#262517,#262518,#262519,
#262520,#262521,#262522,#262523,#262524,#262525,#262526,#262527,#262528,
#262529,#262530,#262531,#262532,#262533,#262534,#262535,#262536,#262537,
#262538,#262539,#262540,#262541,#262542,#262543,#262544,#262545,#262546,
#262547,#262548,#262549,#262550,#262551,#262552,#262553,#262554,#262555,
#262556,#262557,#262558,#262559,#262560,#262561,#262562,#262563,#262564,
#262565,#262566,#262567,#262568,#262569,#262570,#262571,#262572,#262573,
#262574,#262575,#262576,#262577,#262578,#262579,#262580,#262581,#262582,
#262583,#262584,#262585,#262586,#262587,#262588,#262589,#262590)),
 .UNSPECIFIED.,.F.,.F.,.F.)
B_SPLINE_SURFACE_WITH_KNOTS((2,2),(3,2,2,2,2,2,2,2,2,2,2,2,2,2,2,2,2,2,
2,2,2,2,2,2,2,2,2,2,2,2,2,2,2,2,2,2,2,2,2,2,2,2,2,2,2,2,2,2,2,2,2,2,2,2,
2,2,2,2,2,2,2,2,2,2,2,2,2,2,2,2,2,2,2,2,2,2,2,2,2,2,2,2,2,2,2,2,2,2,2,2,
2,2,2,2,2,2,2,2,2,2,2,2,2,2,2,2,2,2,2,2,2,2,2,2,2,2,2,2,2,2,2,2,2,2,2,2,
2,2,2,2,2,2,2,2,2,2,2,2,3),(0.,1.),(0.,0.0072463768115942,0.0144927536231884,
0.0217391304347826,0.0289855072463768,0.036231884057971,0.0434782608695652,
0.0507246376811594,0.0579710144927536,0.0652173913043478,0.072463768115942,
0.0797101449275362,0.0869565217391304,0.0942028985507246,0.101449275362319,
0.108695652173913,0.115942028985507,0.123188405797101,0.130434782608696,
0.13768115942029,0.144927536231884,0.152173913043478,0.159420289855073,
0.166666666666667,0.173913043478261,0.181159420289855,0.18840579710145,
0.195652173913044,0.202898550724637,0.210144927536232,0.217391304347826,
0.224637681159421,0.231884057971014,0.239130434782609,0.246376811594203,
0.253623188405797,0.260869565217392,0.268115942028985,0.275362318840579,
0.282608695652174,0.289855072463768,0.297101449275363,0.304347826086956,
0.31159420289855,0.318840579710145,0.326086956521739,0.333333333333334,
0.340579710144927,0.347826086956521,0.355072463768116,0.36231884057971,
0.369565217391304,0.376811594202899,0.384057971014493,0.391304347826087,
0.398550724637681,0.405797101449275,0.41304347826087,0.420289855072463,
0.427536231884058,0.434782608695652,0.442028985507247,0.449275362318841,
0.456521739130435,0.463768115942029,0.471014492753623,0.478260869565218,
0.485507246376812,0.492753623188406,0.5,0.507246376811594,0.514492753623188,
0.521739130434783,0.528985507246377,0.536231884057971,0.543478260869565,
0.550724637681159,0.557971014492754,0.565217391304348,0.572463768115942,
0.579710144927536,0.586956521739131,0.594202898550725,0.601449275362319,
0.608695652173913,0.615942028985507,0.623188405797101,0.630434782608696,
0.63768115942029,0.644927536231884,0.652173913043478,0.659420289855073,
0.666666666666667,0.673913043478261,0.681159420289855,0.688405797101449,
0.695652173913044,0.702898550724638,0.710144927536232,0.717391304347826,
0.72463768115942,0.731884057971015,0.739130434782609,0.746376811594203,
0.753623188405797,0.760869565217391,0.768115942028986,0.77536231884058,
0.782608695652174,0.789855072463768,0.797101449275362,0.804347826086956,
0.811594202898551,0.818840579710145,0.826086956521739,0.833333333333333,
0.840579710144928,0.847826086956522,0.855072463768116,0.86231884057971,
0.869565217391304,0.876811594202899,0.884057971014493,0.891304347826087,
0.898550724637681,0.905797101449275,0.91304347826087,0.920289855072464,
0.927536231884058,0.934782608695652,0.942028985507246,0.94927536231884,
0.956521739130435,0.963768115942029,0.971014492753623,0.978260869565217,
0.985507246376812,0.992753623188406,0.993818585798284),.UNSPECIFIED.)
GEOMETRIC_REPRESENTATION_ITEM()
RATIONAL_B_SPLINE_SURFACE(((1.,0.866025403784439,1.,0.866025403784439,1.,
0.866025403784439,1.,0.866025403784439,1.,0.866025403784439,1.,0.866025403784439,
1.,0.866025403784439,1.,0.866025403784439,1.,0.866025403784439,1.,0.866025403784439,
1.,0.866025403784439,1.,0.866025403784439,1.,0.866025403784439,1.,0.866025403784439,
1.,0.866025403784439,1.,0.866025403784439,1.,0.866025403784439,1.,0.866025403784439,
1.,0.866025403784439,1.,0.866025403784439,1.,0.866025403784439,1.,0.866025403784439,
1.,0.866025403784439,1.,0.866025403784439,1.,0.866025403784439,1.,0.866025403784439,
1.,0.866025403784439,1.,0.866025403784439,1.,0.866025403784439,1.,0.866025403784439,
1.,0.866025403784439,1.,0.866025403784439,1.,0.866025403784439,1.,0.866025403784439,
1.,0.866025403784439,1.,0.866025403784439,1.,0.866025403784439,1.,0.866025403784439,
1.,0.866025403784439,1.,0.866025403784439,1.,0.866025403784439,1.,0.866025403784439,
1.,0.866025403784439,1.,0.866025403784439,1.,0.866025403784439,1.,0.866025403784439,
1.,0.866025403784439,1.,0.866025403784439,1.,0.866025403784439,1.,0.866025403784439,
1.,0.866025403784439,1.,0.866025403784439,1.,0.866025403784439,1.,0.866025403784439,
1.,0.866025403784439,1.,0.866025403784439,1.,0.866025403784439,1.,0.866025403784439,
1.,0.866025403784439,1.,0.866025403784439,1.,0.866025403784439,1.,0.866025403784439,
1.,0.866025403784439,1.,0.866025403784439,1.,0.866025403784439,1.,0.866025403784439,
1.,0.866025403784439,1.,0.866025403784439,1.,0.866025403784439,1.,0.866025403784439,
1.,0.866025403784439,1.,0.866025403784439,1.,0.866025403784439,1.,0.866025403784439,
1.,0.866025403784439,1.,0.866025403784439,1.,0.866025403784439,1.,0.866025403784439,
1.,0.866025403784439,1.,0.866025403784439,1.,0.866025403784439,1.,0.866025403784439,
1.,0.866025403784439,1.,0.866025403784439,1.,0.866025403784439,1.,0.866025403784439,
1.,0.866025403784439,1.,0.866025403784439,1.,0.866025403784439,1.,0.866025403784439,
1.,0.866025403784439,1.,0.866025403784439,1.,0.866025403784439,1.,0.866025403784439,
1.,0.866025403784439,1.,0.866025403784439,1.,0.866025403784439,1.,0.866025403784439,
1.,0.866025403784439,1.,0.866025403784439,1.,0.866025403784439,1.,0.866025403784439,
1.,0.866025403784439,1.,0.866025403784439,1.,0.866025403784439,1.,0.866025403784439,
1.,0.866025403784439,1.,0.866025403784439,1.,0.866025403784439,1.,0.866025403784439,
1.,0.866025403784439,1.,0.866025403784439,1.,0.866025403784439,1.,0.866025403784439,
1.,0.866025403784439,1.,0.866025403784439,1.,0.866025403784439,1.,0.866025403784439,
1.,0.866025403784439,1.,0.866025403784439,1.,0.866025403784439,1.,0.866025403784439,
1.,0.866025403784439,1.,0.866025403784439,1.,0.866025403784439,1.,0.866025403784439,
1.,0.866025403784439,1.,0.866025403784439,1.,0.866025403784439,1.,0.866025403784439,
1.,0.866025403784439,1.,0.866025403784439,1.,0.866025403784439,1.,0.866025403784439,
1.,0.866025403784439,1.,0.866025403784439,1.,0.866025403784439,1.,0.98031044488126,
0.966408234404338),(1.,0.866025403784439,1.,0.866025403784439,1.,0.866025403784439,
1.,0.866025403784439,1.,0.866025403784439,1.,0.866025403784439,1.,0.866025403784439,
1.,0.866025403784439,1.,0.866025403784439,1.,0.866025403784439,1.,0.866025403784439,
1.,0.866025403784439,1.,0.866025403784439,1.,0.866025403784439,1.,0.866025403784439,
1.,0.866025403784439,1.,0.866025403784439,1.,0.866025403784439,1.,0.866025403784439,
1.,0.866025403784439,1.,0.866025403784439,1.,0.866025403784439,1.,0.866025403784439,
1.,0.866025403784439,1.,0.866025403784439,1.,0.866025403784439,1.,0.866025403784439,
1.,0.866025403784439,1.,0.866025403784439,1.,0.866025403784439,1.,0.866025403784439,
1.,0.866025403784439,1.,0.866025403784439,1.,0.866025403784439,1.,0.866025403784439,
1.,0.866025403784439,1.,0.866025403784439,1.,0.866025403784439,1.,0.866025403784439,
1.,0.866025403784439,1.,0.866025403784439,1.,0.866025403784439,1.,0.866025403784439,
1.,0.866025403784439,1.,0.866025403784439,1.,0.866025403784439,1.,0.866025403784439,
1.,0.866025403784439,1.,0.866025403784439,1.,0.866025403784439,1.,0.866025403784439,
1.,0.866025403784439,1.,0.866025403784439,1.,0.866025403784439,1.,0.866025403784439,
1.,0.866025403784439,1.,0.866025403784439,1.,0.866025403784439,1.,0.866025403784439,
1.,0.866025403784439,1.,0.866025403784439,1.,0.866025403784439,1.,0.866025403784439,
1.,0.866025403784439,1.,0.866025403784439,1.,0.866025403784439,1.,0.866025403784439,
1.,0.866025403784439,1.,0.866025403784439,1.,0.866025403784439,1.,0.866025403784439,
1.,0.866025403784439,1.,0.866025403784439,1.,0.866025403784439,1.,0.866025403784439,
1.,0.866025403784439,1.,0.866025403784439,1.,0.866025403784439,1.,0.866025403784439,
1.,0.866025403784439,1.,0.866025403784439,1.,0.866025403784439,1.,0.866025403784439,
1.,0.866025403784439,1.,0.866025403784439,1.,0.866025403784439,1.,0.866025403784439,
1.,0.866025403784439,1.,0.866025403784439,1.,0.866025403784439,1.,0.866025403784439,
1.,0.866025403784439,1.,0.866025403784439,1.,0.866025403784439,1.,0.866025403784439,
1.,0.866025403784439,1.,0.866025403784439,1.,0.866025403784439,1.,0.866025403784439,
1.,0.866025403784439,1.,0.866025403784439,1.,0.866025403784439,1.,0.866025403784439,
1.,0.866025403784439,1.,0.866025403784439,1.,0.866025403784439,1.,0.866025403784439,
1.,0.866025403784439,1.,0.866025403784439,1.,0.866025403784439,1.,0.866025403784439,
1.,0.866025403784439,1.,0.866025403784439,1.,0.866025403784439,1.,0.866025403784439,
1.,0.866025403784439,1.,0.866025403784439,1.,0.866025403784439,1.,0.866025403784439,
1.,0.866025403784439,1.,0.866025403784439,1.,0.866025403784439,1.,0.866025403784439,
1.,0.866025403784439,1.,0.866025403784439,1.,0.866025403784439,1.,0.866025403784439,
1.,0.866025403784439,1.,0.866025403784439,1.,0.866025403784439,1.,0.866025403784439,
1.,0.866025403784439,1.,0.866025403784439,1.,0.866025403784439,1.,0.866025403784439,
1.,0.866025403784439,1.,0.866025403784439,1.,0.98031044488126,0.966408234404338)))
REPRESENTATION_ITEM('')
SURFACE()
);
#3186=(
BOUNDED_SURFACE()
B_SPLINE_SURFACE(1,2,((#264455,#264456,#264457,#264458,#264459,#264460,
#264461,#264462,#264463,#264464,#264465,#264466,#264467,#264468,#264469,
#264470,#264471,#264472,#264473,#264474,#264475,#264476,#264477,#264478,
#264479,#264480,#264481,#264482,#264483,#264484,#264485,#264486,#264487,
#264488,#264489,#264490,#264491,#264492,#264493,#264494,#264495,#264496,
#264497,#264498,#264499,#264500,#264501,#264502,#264503,#264504,#264505,
#264506,#264507,#264508,#264509,#264510,#264511,#264512,#264513,#264514,
#264515,#264516,#264517,#264518,#264519,#264520,#264521,#264522,#264523,
#264524,#264525,#264526,#264527,#264528,#264529,#264530,#264531,#264532,
#264533,#264534,#264535,#264536,#264537,#264538,#264539,#264540,#264541,
#264542,#264543,#264544,#264545,#264546,#264547,#264548,#264549,#264550,
#264551,#264552,#264553,#264554,#264555,#264556,#264557,#264558,#264559,
#264560,#264561,#264562,#264563,#264564,#264565,#264566,#264567,#264568,
#264569,#264570,#264571,#264572,#264573,#264574,#264575,#264576,#264577,
#264578,#264579,#264580,#264581,#264582,#264583,#264584,#264585,#264586,
#264587,#264588,#264589,#264590,#264591,#264592,#264593,#264594,#264595,
#264596,#264597,#264598,#264599,#264600,#264601,#264602,#264603,#264604,
#264605,#264606,#264607,#264608,#264609,#264610,#264611,#264612,#264613,
#264614,#264615,#264616,#264617,#264618,#264619,#264620,#264621,#264622,
#264623,#264624,#264625,#264626,#264627,#264628,#264629,#264630,#264631,
#264632,#264633,#264634,#264635,#264636,#264637,#264638,#264639,#264640,
#264641,#264642,#264643,#264644,#264645,#264646,#264647,#264648,#264649,
#264650,#264651,#264652,#264653,#264654,#264655,#264656,#264657,#264658,
#264659,#264660,#264661,#264662,#264663,#264664,#264665,#264666,#264667,
#264668,#264669,#264670,#264671,#264672,#264673,#264674,#264675,#264676,
#264677,#264678,#264679,#264680,#264681,#264682,#264683,#264684,#264685,
#264686,#264687,#264688,#264689,#264690,#264691,#264692,#264693,#264694,
#264695,#264696,#264697,#264698,#264699,#264700,#264701,#264702,#264703,
#264704,#264705,#264706,#264707,#264708,#264709,#264710,#264711,#264712,
#264713,#264714,#264715,#264716,#264717,#264718,#264719,#264720,#264721,
#264722,#264723,#264724,#264725,#264726,#264727,#264728,#264729,#264730,
#264731),(#264732,#264733,#264734,#264735,#264736,#264737,#264738,#264739,
#264740,#264741,#264742,#264743,#264744,#264745,#264746,#264747,#264748,
#264749,#264750,#264751,#264752,#264753,#264754,#264755,#264756,#264757,
#264758,#264759,#264760,#264761,#264762,#264763,#264764,#264765,#264766,
#264767,#264768,#264769,#264770,#264771,#264772,#264773,#264774,#264775,
#264776,#264777,#264778,#264779,#264780,#264781,#264782,#264783,#264784,
#264785,#264786,#264787,#264788,#264789,#264790,#264791,#264792,#264793,
#264794,#264795,#264796,#264797,#264798,#264799,#264800,#264801,#264802,
#264803,#264804,#264805,#264806,#264807,#264808,#264809,#264810,#264811,
#264812,#264813,#264814,#264815,#264816,#264817,#264818,#264819,#264820,
#264821,#264822,#264823,#264824,#264825,#264826,#264827,#264828,#264829,
#264830,#264831,#264832,#264833,#264834,#264835,#264836,#264837,#264838,
#264839,#264840,#264841,#264842,#264843,#264844,#264845,#264846,#264847,
#264848,#264849,#264850,#264851,#264852,#264853,#264854,#264855,#264856,
#264857,#264858,#264859,#264860,#264861,#264862,#264863,#264864,#264865,
#264866,#264867,#264868,#264869,#264870,#264871,#264872,#264873,#264874,
#264875,#264876,#264877,#264878,#264879,#264880,#264881,#264882,#264883,
#264884,#264885,#264886,#264887,#264888,#264889,#264890,#264891,#264892,
#264893,#264894,#264895,#264896,#264897,#264898,#264899,#264900,#264901,
#264902,#264903,#264904,#264905,#264906,#264907,#264908,#264909,#264910,
#264911,#264912,#264913,#264914,#264915,#264916,#264917,#264918,#264919,
#264920,#264921,#264922,#264923,#264924,#264925,#264926,#264927,#264928,
#264929,#264930,#264931,#264932,#264933,#264934,#264935,#264936,#264937,
#264938,#264939,#264940,#264941,#264942,#264943,#264944,#264945,#264946,
#264947,#264948,#264949,#264950,#264951,#264952,#264953,#264954,#264955,
#264956,#264957,#264958,#264959,#264960,#264961,#264962,#264963,#264964,
#264965,#264966,#264967,#264968,#264969,#264970,#264971,#264972,#264973,
#264974,#264975,#264976,#264977,#264978,#264979,#264980,#264981,#264982,
#264983,#264984,#264985,#264986,#264987,#264988,#264989,#264990,#264991,
#264992,#264993,#264994,#264995,#264996,#264997,#264998,#264999,#265000,
#265001,#265002,#265003,#265004,#265005,#265006,#265007,#265008)),
 .UNSPECIFIED.,.F.,.F.,.F.)
B_SPLINE_SURFACE_WITH_KNOTS((2,2),(3,2,2,2,2,2,2,2,2,2,2,2,2,2,2,2,2,2,
2,2,2,2,2,2,2,2,2,2,2,2,2,2,2,2,2,2,2,2,2,2,2,2,2,2,2,2,2,2,2,2,2,2,2,2,
2,2,2,2,2,2,2,2,2,2,2,2,2,2,2,2,2,2,2,2,2,2,2,2,2,2,2,2,2,2,2,2,2,2,2,2,
2,2,2,2,2,2,2,2,2,2,2,2,2,2,2,2,2,2,2,2,2,2,2,2,2,2,2,2,2,2,2,2,2,2,2,2,
2,2,2,2,2,2,2,2,2,2,2,2,3),(0.,1.),(0.,0.0072463768115942,0.0144927536231884,
0.0217391304347826,0.0289855072463768,0.036231884057971,0.0434782608695652,
0.0507246376811594,0.0579710144927536,0.0652173913043478,0.072463768115942,
0.0797101449275362,0.0869565217391304,0.0942028985507246,0.101449275362319,
0.108695652173913,0.115942028985507,0.123188405797101,0.130434782608696,
0.13768115942029,0.144927536231884,0.152173913043478,0.159420289855073,
0.166666666666667,0.173913043478261,0.181159420289855,0.18840579710145,
0.195652173913044,0.202898550724637,0.210144927536232,0.217391304347826,
0.224637681159421,0.231884057971014,0.239130434782609,0.246376811594203,
0.253623188405797,0.260869565217392,0.268115942028985,0.275362318840579,
0.282608695652174,0.289855072463768,0.297101449275363,0.304347826086956,
0.31159420289855,0.318840579710145,0.326086956521739,0.333333333333334,
0.340579710144927,0.347826086956521,0.355072463768116,0.36231884057971,
0.369565217391304,0.376811594202899,0.384057971014493,0.391304347826087,
0.398550724637681,0.405797101449275,0.41304347826087,0.420289855072463,
0.427536231884058,0.434782608695652,0.442028985507247,0.449275362318841,
0.456521739130435,0.463768115942029,0.471014492753623,0.478260869565218,
0.485507246376812,0.492753623188406,0.5,0.507246376811594,0.514492753623188,
0.521739130434783,0.528985507246377,0.536231884057971,0.543478260869565,
0.550724637681159,0.557971014492754,0.565217391304348,0.572463768115942,
0.579710144927536,0.586956521739131,0.594202898550725,0.601449275362319,
0.608695652173913,0.615942028985507,0.623188405797101,0.630434782608696,
0.63768115942029,0.644927536231884,0.652173913043478,0.659420289855073,
0.666666666666667,0.673913043478261,0.681159420289855,0.688405797101449,
0.695652173913044,0.702898550724638,0.710144927536232,0.717391304347826,
0.72463768115942,0.731884057971015,0.739130434782609,0.746376811594203,
0.753623188405797,0.760869565217391,0.768115942028986,0.77536231884058,
0.782608695652174,0.789855072463768,0.797101449275362,0.804347826086956,
0.811594202898551,0.818840579710145,0.826086956521739,0.833333333333333,
0.840579710144928,0.847826086956522,0.855072463768116,0.86231884057971,
0.869565217391304,0.876811594202899,0.884057971014493,0.891304347826087,
0.898550724637681,0.905797101449275,0.91304347826087,0.920289855072464,
0.927536231884058,0.934782608695652,0.942028985507246,0.94927536231884,
0.956521739130435,0.963768115942029,0.971014492753623,0.978260869565217,
0.985507246376812,0.992753623188406,0.993818495192186),.UNSPECIFIED.)
GEOMETRIC_REPRESENTATION_ITEM()
RATIONAL_B_SPLINE_SURFACE(((1.,0.866025403784439,1.,0.866025403784439,1.,
0.866025403784439,1.,0.866025403784439,1.,0.866025403784439,1.,0.866025403784439,
1.,0.866025403784439,1.,0.866025403784439,1.,0.866025403784439,1.,0.866025403784439,
1.,0.866025403784439,1.,0.866025403784439,1.,0.866025403784439,1.,0.866025403784439,
1.,0.866025403784439,1.,0.866025403784439,1.,0.866025403784439,1.,0.866025403784439,
1.,0.866025403784439,1.,0.866025403784439,1.,0.866025403784439,1.,0.866025403784439,
1.,0.866025403784439,1.,0.866025403784439,1.,0.866025403784439,1.,0.866025403784439,
1.,0.866025403784439,1.,0.866025403784439,1.,0.866025403784439,1.,0.866025403784439,
1.,0.866025403784439,1.,0.866025403784439,1.,0.866025403784439,1.,0.866025403784439,
1.,0.866025403784439,1.,0.866025403784439,1.,0.866025403784439,1.,0.866025403784439,
1.,0.866025403784439,1.,0.866025403784439,1.,0.866025403784439,1.,0.866025403784439,
1.,0.866025403784439,1.,0.866025403784439,1.,0.866025403784439,1.,0.866025403784439,
1.,0.866025403784439,1.,0.866025403784439,1.,0.866025403784439,1.,0.866025403784439,
1.,0.866025403784439,1.,0.866025403784439,1.,0.866025403784439,1.,0.866025403784439,
1.,0.866025403784439,1.,0.866025403784439,1.,0.866025403784439,1.,0.866025403784439,
1.,0.866025403784439,1.,0.866025403784439,1.,0.866025403784439,1.,0.866025403784439,
1.,0.866025403784439,1.,0.866025403784439,1.,0.866025403784439,1.,0.866025403784439,
1.,0.866025403784439,1.,0.866025403784439,1.,0.866025403784439,1.,0.866025403784439,
1.,0.866025403784439,1.,0.866025403784439,1.,0.866025403784439,1.,0.866025403784439,
1.,0.866025403784439,1.,0.866025403784439,1.,0.866025403784439,1.,0.866025403784439,
1.,0.866025403784439,1.,0.866025403784439,1.,0.866025403784439,1.,0.866025403784439,
1.,0.866025403784439,1.,0.866025403784439,1.,0.866025403784439,1.,0.866025403784439,
1.,0.866025403784439,1.,0.866025403784439,1.,0.866025403784439,1.,0.866025403784439,
1.,0.866025403784439,1.,0.866025403784439,1.,0.866025403784439,1.,0.866025403784439,
1.,0.866025403784439,1.,0.866025403784439,1.,0.866025403784439,1.,0.866025403784439,
1.,0.866025403784439,1.,0.866025403784439,1.,0.866025403784439,1.,0.866025403784439,
1.,0.866025403784439,1.,0.866025403784439,1.,0.866025403784439,1.,0.866025403784439,
1.,0.866025403784439,1.,0.866025403784439,1.,0.866025403784439,1.,0.866025403784439,
1.,0.866025403784439,1.,0.866025403784439,1.,0.866025403784439,1.,0.866025403784439,
1.,0.866025403784439,1.,0.866025403784439,1.,0.866025403784439,1.,0.866025403784439,
1.,0.866025403784439,1.,0.866025403784439,1.,0.866025403784439,1.,0.866025403784439,
1.,0.866025403784439,1.,0.866025403784439,1.,0.866025403784439,1.,0.866025403784439,
1.,0.866025403784439,1.,0.866025403784439,1.,0.866025403784439,1.,0.866025403784439,
1.,0.866025403784439,1.,0.866025403784439,1.,0.866025403784439,1.,0.866025403784439,
1.,0.866025403784439,1.,0.866025403784439,1.,0.866025403784439,1.,0.980312120051573,
0.966410600022306),(1.,0.866025403784439,1.,0.866025403784439,1.,0.866025403784439,
1.,0.866025403784439,1.,0.866025403784439,1.,0.866025403784439,1.,0.866025403784439,
1.,0.866025403784439,1.,0.866025403784439,1.,0.866025403784439,1.,0.866025403784439,
1.,0.866025403784439,1.,0.866025403784439,1.,0.866025403784439,1.,0.866025403784439,
1.,0.866025403784439,1.,0.866025403784439,1.,0.866025403784439,1.,0.866025403784439,
1.,0.866025403784439,1.,0.866025403784439,1.,0.866025403784439,1.,0.866025403784439,
1.,0.866025403784439,1.,0.866025403784439,1.,0.866025403784439,1.,0.866025403784439,
1.,0.866025403784439,1.,0.866025403784439,1.,0.866025403784439,1.,0.866025403784439,
1.,0.866025403784439,1.,0.866025403784439,1.,0.866025403784439,1.,0.866025403784439,
1.,0.866025403784439,1.,0.866025403784439,1.,0.866025403784439,1.,0.866025403784439,
1.,0.866025403784439,1.,0.866025403784439,1.,0.866025403784439,1.,0.866025403784439,
1.,0.866025403784439,1.,0.866025403784439,1.,0.866025403784439,1.,0.866025403784439,
1.,0.866025403784439,1.,0.866025403784439,1.,0.866025403784439,1.,0.866025403784439,
1.,0.866025403784439,1.,0.866025403784439,1.,0.866025403784439,1.,0.866025403784439,
1.,0.866025403784439,1.,0.866025403784439,1.,0.866025403784439,1.,0.866025403784439,
1.,0.866025403784439,1.,0.866025403784439,1.,0.866025403784439,1.,0.866025403784439,
1.,0.866025403784439,1.,0.866025403784439,1.,0.866025403784439,1.,0.866025403784439,
1.,0.866025403784439,1.,0.866025403784439,1.,0.866025403784439,1.,0.866025403784439,
1.,0.866025403784439,1.,0.866025403784439,1.,0.866025403784439,1.,0.866025403784439,
1.,0.866025403784439,1.,0.866025403784439,1.,0.866025403784439,1.,0.866025403784439,
1.,0.866025403784439,1.,0.866025403784439,1.,0.866025403784439,1.,0.866025403784439,
1.,0.866025403784439,1.,0.866025403784439,1.,0.866025403784439,1.,0.866025403784439,
1.,0.866025403784439,1.,0.866025403784439,1.,0.866025403784439,1.,0.866025403784439,
1.,0.866025403784439,1.,0.866025403784439,1.,0.866025403784439,1.,0.866025403784439,
1.,0.866025403784439,1.,0.866025403784439,1.,0.866025403784439,1.,0.866025403784439,
1.,0.866025403784439,1.,0.866025403784439,1.,0.866025403784439,1.,0.866025403784439,
1.,0.866025403784439,1.,0.866025403784439,1.,0.866025403784439,1.,0.866025403784439,
1.,0.866025403784439,1.,0.866025403784439,1.,0.866025403784439,1.,0.866025403784439,
1.,0.866025403784439,1.,0.866025403784439,1.,0.866025403784439,1.,0.866025403784439,
1.,0.866025403784439,1.,0.866025403784439,1.,0.866025403784439,1.,0.866025403784439,
1.,0.866025403784439,1.,0.866025403784439,1.,0.866025403784439,1.,0.866025403784439,
1.,0.866025403784439,1.,0.866025403784439,1.,0.866025403784439,1.,0.866025403784439,
1.,0.866025403784439,1.,0.866025403784439,1.,0.866025403784439,1.,0.866025403784439,
1.,0.866025403784439,1.,0.866025403784439,1.,0.866025403784439,1.,0.866025403784439,
1.,0.866025403784439,1.,0.866025403784439,1.,0.980312120051573,0.966410600022306)))
REPRESENTATION_ITEM('')
SURFACE()
);
#3187=(
BOUNDED_SURFACE()
B_SPLINE_SURFACE(1,2,((#265009,#265010,#265011,#265012,#265013,#265014,
#265015,#265016,#265017,#265018,#265019,#265020,#265021,#265022,#265023,
#265024,#265025,#265026,#265027,#265028,#265029,#265030,#265031,#265032,
#265033,#265034,#265035,#265036,#265037,#265038,#265039,#265040,#265041,
#265042,#265043,#265044,#265045,#265046,#265047,#265048,#265049,#265050,
#265051,#265052,#265053,#265054,#265055,#265056,#265057,#265058,#265059,
#265060,#265061,#265062,#265063,#265064,#265065,#265066,#265067,#265068,
#265069,#265070,#265071,#265072,#265073,#265074,#265075,#265076,#265077,
#265078,#265079,#265080,#265081,#265082,#265083,#265084,#265085,#265086,
#265087,#265088,#265089,#265090,#265091,#265092,#265093,#265094,#265095,
#265096,#265097,#265098,#265099,#265100,#265101,#265102,#265103,#265104,
#265105,#265106,#265107,#265108,#265109,#265110,#265111,#265112,#265113,
#265114,#265115,#265116,#265117,#265118,#265119,#265120,#265121,#265122,
#265123,#265124,#265125,#265126,#265127,#265128,#265129,#265130,#265131,
#265132,#265133,#265134,#265135,#265136,#265137,#265138,#265139,#265140,
#265141,#265142,#265143,#265144,#265145,#265146,#265147,#265148,#265149,
#265150,#265151,#265152,#265153,#265154,#265155,#265156,#265157,#265158,
#265159,#265160,#265161,#265162,#265163,#265164,#265165,#265166,#265167,
#265168,#265169,#265170,#265171,#265172,#265173,#265174,#265175,#265176,
#265177,#265178,#265179,#265180,#265181,#265182,#265183,#265184,#265185,
#265186,#265187,#265188,#265189,#265190,#265191,#265192,#265193,#265194,
#265195,#265196,#265197,#265198,#265199,#265200,#265201,#265202,#265203,
#265204,#265205,#265206,#265207,#265208,#265209,#265210,#265211,#265212,
#265213,#265214,#265215,#265216,#265217,#265218,#265219,#265220,#265221,
#265222,#265223,#265224,#265225,#265226,#265227,#265228,#265229,#265230,
#265231,#265232,#265233,#265234,#265235,#265236,#265237,#265238,#265239,
#265240,#265241,#265242,#265243,#265244,#265245,#265246,#265247,#265248,
#265249,#265250,#265251,#265252,#265253,#265254,#265255,#265256,#265257,
#265258,#265259,#265260,#265261,#265262,#265263,#265264,#265265,#265266,
#265267,#265268,#265269,#265270,#265271,#265272,#265273,#265274,#265275,
#265276,#265277,#265278,#265279,#265280,#265281,#265282,#265283,#265284,
#265285),(#265286,#265287,#265288,#265289,#265290,#265291,#265292,#265293,
#265294,#265295,#265296,#265297,#265298,#265299,#265300,#265301,#265302,
#265303,#265304,#265305,#265306,#265307,#265308,#265309,#265310,#265311,
#265312,#265313,#265314,#265315,#265316,#265317,#265318,#265319,#265320,
#265321,#265322,#265323,#265324,#265325,#265326,#265327,#265328,#265329,
#265330,#265331,#265332,#265333,#265334,#265335,#265336,#265337,#265338,
#265339,#265340,#265341,#265342,#265343,#265344,#265345,#265346,#265347,
#265348,#265349,#265350,#265351,#265352,#265353,#265354,#265355,#265356,
#265357,#265358,#265359,#265360,#265361,#265362,#265363,#265364,#265365,
#265366,#265367,#265368,#265369,#265370,#265371,#265372,#265373,#265374,
#265375,#265376,#265377,#265378,#265379,#265380,#265381,#265382,#265383,
#265384,#265385,#265386,#265387,#265388,#265389,#265390,#265391,#265392,
#265393,#265394,#265395,#265396,#265397,#265398,#265399,#265400,#265401,
#265402,#265403,#265404,#265405,#265406,#265407,#265408,#265409,#265410,
#265411,#265412,#265413,#265414,#265415,#265416,#265417,#265418,#265419,
#265420,#265421,#265422,#265423,#265424,#265425,#265426,#265427,#265428,
#265429,#265430,#265431,#265432,#265433,#265434,#265435,#265436,#265437,
#265438,#265439,#265440,#265441,#265442,#265443,#265444,#265445,#265446,
#265447,#265448,#265449,#265450,#265451,#265452,#265453,#265454,#265455,
#265456,#265457,#265458,#265459,#265460,#265461,#265462,#265463,#265464,
#265465,#265466,#265467,#265468,#265469,#265470,#265471,#265472,#265473,
#265474,#265475,#265476,#265477,#265478,#265479,#265480,#265481,#265482,
#265483,#265484,#265485,#265486,#265487,#265488,#265489,#265490,#265491,
#265492,#265493,#265494,#265495,#265496,#265497,#265498,#265499,#265500,
#265501,#265502,#265503,#265504,#265505,#265506,#265507,#265508,#265509,
#265510,#265511,#265512,#265513,#265514,#265515,#265516,#265517,#265518,
#265519,#265520,#265521,#265522,#265523,#265524,#265525,#265526,#265527,
#265528,#265529,#265530,#265531,#265532,#265533,#265534,#265535,#265536,
#265537,#265538,#265539,#265540,#265541,#265542,#265543,#265544,#265545,
#265546,#265547,#265548,#265549,#265550,#265551,#265552,#265553,#265554,
#265555,#265556,#265557,#265558,#265559,#265560,#265561,#265562)),
 .UNSPECIFIED.,.F.,.F.,.F.)
B_SPLINE_SURFACE_WITH_KNOTS((2,2),(3,2,2,2,2,2,2,2,2,2,2,2,2,2,2,2,2,2,
2,2,2,2,2,2,2,2,2,2,2,2,2,2,2,2,2,2,2,2,2,2,2,2,2,2,2,2,2,2,2,2,2,2,2,2,
2,2,2,2,2,2,2,2,2,2,2,2,2,2,2,2,2,2,2,2,2,2,2,2,2,2,2,2,2,2,2,2,2,2,2,2,
2,2,2,2,2,2,2,2,2,2,2,2,2,2,2,2,2,2,2,2,2,2,2,2,2,2,2,2,2,2,2,2,2,2,2,2,
2,2,2,2,2,2,2,2,2,2,2,2,3),(0.,1.00000035866471),(0.,0.0072463768115942,
0.0144927536231884,0.0217391304347826,0.0289855072463768,0.036231884057971,
0.0434782608695652,0.0507246376811594,0.0579710144927536,0.0652173913043478,
0.072463768115942,0.0797101449275362,0.0869565217391304,0.0942028985507246,
0.101449275362319,0.108695652173913,0.115942028985507,0.123188405797101,
0.130434782608696,0.13768115942029,0.144927536231884,0.152173913043478,
0.159420289855073,0.166666666666667,0.173913043478261,0.181159420289855,
0.18840579710145,0.195652173913044,0.202898550724637,0.210144927536232,
0.217391304347826,0.224637681159421,0.231884057971014,0.239130434782609,
0.246376811594203,0.253623188405797,0.260869565217392,0.268115942028985,
0.275362318840579,0.282608695652174,0.289855072463768,0.297101449275363,
0.304347826086956,0.31159420289855,0.318840579710145,0.326086956521739,
0.333333333333334,0.340579710144927,0.347826086956521,0.355072463768116,
0.36231884057971,0.369565217391304,0.376811594202899,0.384057971014493,
0.391304347826087,0.398550724637681,0.405797101449275,0.41304347826087,
0.420289855072463,0.427536231884058,0.434782608695652,0.442028985507247,
0.449275362318841,0.456521739130435,0.463768115942029,0.471014492753623,
0.478260869565218,0.485507246376812,0.492753623188406,0.5,0.507246376811594,
0.514492753623188,0.521739130434783,0.528985507246377,0.536231884057971,
0.543478260869565,0.550724637681159,0.557971014492754,0.565217391304348,
0.572463768115942,0.579710144927536,0.586956521739131,0.594202898550725,
0.601449275362319,0.608695652173913,0.615942028985507,0.623188405797101,
0.630434782608696,0.63768115942029,0.644927536231884,0.652173913043478,
0.659420289855073,0.666666666666667,0.673913043478261,0.681159420289855,
0.688405797101449,0.695652173913044,0.702898550724638,0.710144927536232,
0.717391304347826,0.72463768115942,0.731884057971015,0.739130434782609,
0.746376811594203,0.753623188405797,0.760869565217391,0.768115942028986,
0.77536231884058,0.782608695652174,0.789855072463768,0.797101449275362,
0.804347826086956,0.811594202898551,0.818840579710145,0.826086956521739,
0.833333333333333,0.840579710144928,0.847826086956522,0.855072463768116,
0.86231884057971,0.869565217391304,0.876811594202899,0.884057971014493,
0.891304347826087,0.898550724637681,0.905797101449275,0.91304347826087,
0.920289855072464,0.927536231884058,0.934782608695652,0.942028985507246,
0.94927536231884,0.956521739130435,0.963768115942029,0.971014492753623,
0.978260869565217,0.985507246376812,0.992753623188406,0.993818495192186),
 .UNSPECIFIED.)
GEOMETRIC_REPRESENTATION_ITEM()
RATIONAL_B_SPLINE_SURFACE(((1.,0.866025403784439,1.,0.866025403784439,1.,
0.866025403784439,1.,0.866025403784439,1.,0.866025403784439,1.,0.866025403784439,
1.,0.866025403784439,1.,0.866025403784439,1.,0.866025403784439,1.,0.866025403784439,
1.,0.866025403784439,1.,0.866025403784439,1.,0.866025403784439,1.,0.866025403784439,
1.,0.866025403784439,1.,0.866025403784439,1.,0.866025403784439,1.,0.866025403784439,
1.,0.866025403784439,1.,0.866025403784439,1.,0.866025403784439,1.,0.866025403784439,
1.,0.866025403784439,1.,0.866025403784439,1.,0.866025403784439,1.,0.866025403784439,
1.,0.866025403784439,1.,0.866025403784439,1.,0.866025403784439,1.,0.866025403784439,
1.,0.866025403784439,1.,0.866025403784439,1.,0.866025403784439,1.,0.866025403784439,
1.,0.866025403784439,1.,0.866025403784439,1.,0.866025403784439,1.,0.866025403784439,
1.,0.866025403784439,1.,0.866025403784439,1.,0.866025403784439,1.,0.866025403784439,
1.,0.866025403784439,1.,0.866025403784439,1.,0.866025403784439,1.,0.866025403784439,
1.,0.866025403784439,1.,0.866025403784439,1.,0.866025403784439,1.,0.866025403784439,
1.,0.866025403784439,1.,0.866025403784439,1.,0.866025403784439,1.,0.866025403784439,
1.,0.866025403784439,1.,0.866025403784439,1.,0.866025403784439,1.,0.866025403784439,
1.,0.866025403784439,1.,0.866025403784439,1.,0.866025403784439,1.,0.866025403784439,
1.,0.866025403784439,1.,0.866025403784439,1.,0.866025403784439,1.,0.866025403784439,
1.,0.866025403784439,1.,0.866025403784439,1.,0.866025403784439,1.,0.866025403784439,
1.,0.866025403784439,1.,0.866025403784439,1.,0.866025403784439,1.,0.866025403784439,
1.,0.866025403784439,1.,0.866025403784439,1.,0.866025403784439,1.,0.866025403784439,
1.,0.866025403784439,1.,0.866025403784439,1.,0.866025403784439,1.,0.866025403784439,
1.,0.866025403784439,1.,0.866025403784439,1.,0.866025403784439,1.,0.866025403784439,
1.,0.866025403784439,1.,0.866025403784439,1.,0.866025403784439,1.,0.866025403784439,
1.,0.866025403784439,1.,0.866025403784439,1.,0.866025403784439,1.,0.866025403784439,
1.,0.866025403784439,1.,0.866025403784439,1.,0.866025403784439,1.,0.866025403784439,
1.,0.866025403784439,1.,0.866025403784439,1.,0.866025403784439,1.,0.866025403784439,
1.,0.866025403784439,1.,0.866025403784439,1.,0.866025403784439,1.,0.866025403784439,
1.,0.866025403784439,1.,0.866025403784439,1.,0.866025403784439,1.,0.866025403784439,
1.,0.866025403784439,1.,0.866025403784439,1.,0.866025403784439,1.,0.866025403784439,
1.,0.866025403784439,1.,0.866025403784439,1.,0.866025403784439,1.,0.866025403784439,
1.,0.866025403784439,1.,0.866025403784439,1.,0.866025403784439,1.,0.866025403784439,
1.,0.866025403784439,1.,0.866025403784439,1.,0.866025403784439,1.,0.866025403784439,
1.,0.866025403784439,1.,0.866025403784439,1.,0.866025403784439,1.,0.866025403784439,
1.,0.866025403784439,1.,0.866025403784439,1.,0.866025403784439,1.,0.866025403784439,
1.,0.866025403784439,1.,0.866025403784439,1.,0.866025403784439,1.,0.980312120051573,
0.966410600022306),(1.,0.866025403784439,1.,0.866025403784439,1.,0.866025403784439,
1.,0.866025403784439,1.,0.866025403784439,1.,0.866025403784439,1.,0.866025403784439,
1.,0.866025403784439,1.,0.866025403784439,1.,0.866025403784439,1.,0.866025403784439,
1.,0.866025403784439,1.,0.866025403784439,1.,0.866025403784439,1.,0.866025403784439,
1.,0.866025403784439,1.,0.866025403784439,1.,0.866025403784439,1.,0.866025403784439,
1.,0.866025403784439,1.,0.866025403784439,1.,0.866025403784439,1.,0.866025403784439,
1.,0.866025403784439,1.,0.866025403784439,1.,0.866025403784439,1.,0.866025403784439,
1.,0.866025403784439,1.,0.866025403784439,1.,0.866025403784439,1.,0.866025403784439,
1.,0.866025403784439,1.,0.866025403784439,1.,0.866025403784439,1.,0.866025403784439,
1.,0.866025403784439,1.,0.866025403784439,1.,0.866025403784439,1.,0.866025403784439,
1.,0.866025403784439,1.,0.866025403784439,1.,0.866025403784439,1.,0.866025403784439,
1.,0.866025403784439,1.,0.866025403784439,1.,0.866025403784439,1.,0.866025403784439,
1.,0.866025403784439,1.,0.866025403784439,1.,0.866025403784439,1.,0.866025403784439,
1.,0.866025403784439,1.,0.866025403784439,1.,0.866025403784439,1.,0.866025403784439,
1.,0.866025403784439,1.,0.866025403784439,1.,0.866025403784439,1.,0.866025403784439,
1.,0.866025403784439,1.,0.866025403784439,1.,0.866025403784439,1.,0.866025403784439,
1.,0.866025403784439,1.,0.866025403784439,1.,0.866025403784439,1.,0.866025403784439,
1.,0.866025403784439,1.,0.866025403784439,1.,0.866025403784439,1.,0.866025403784439,
1.,0.866025403784439,1.,0.866025403784439,1.,0.866025403784439,1.,0.866025403784439,
1.,0.866025403784439,1.,0.866025403784439,1.,0.866025403784439,1.,0.866025403784439,
1.,0.866025403784439,1.,0.866025403784439,1.,0.866025403784439,1.,0.866025403784439,
1.,0.866025403784439,1.,0.866025403784439,1.,0.866025403784439,1.,0.866025403784439,
1.,0.866025403784439,1.,0.866025403784439,1.,0.866025403784439,1.,0.866025403784439,
1.,0.866025403784439,1.,0.866025403784439,1.,0.866025403784439,1.,0.866025403784439,
1.,0.866025403784439,1.,0.866025403784439,1.,0.866025403784439,1.,0.866025403784439,
1.,0.866025403784439,1.,0.866025403784439,1.,0.866025403784439,1.,0.866025403784439,
1.,0.866025403784439,1.,0.866025403784439,1.,0.866025403784439,1.,0.866025403784439,
1.,0.866025403784439,1.,0.866025403784439,1.,0.866025403784439,1.,0.866025403784439,
1.,0.866025403784439,1.,0.866025403784439,1.,0.866025403784439,1.,0.866025403784439,
1.,0.866025403784439,1.,0.866025403784439,1.,0.866025403784439,1.,0.866025403784439,
1.,0.866025403784439,1.,0.866025403784439,1.,0.866025403784439,1.,0.866025403784439,
1.,0.866025403784439,1.,0.866025403784439,1.,0.866025403784439,1.,0.866025403784439,
1.,0.866025403784439,1.,0.866025403784439,1.,0.866025403784439,1.,0.866025403784439,
1.,0.866025403784439,1.,0.866025403784439,1.,0.866025403784439,1.,0.866025403784439,
1.,0.866025403784439,1.,0.866025403784439,1.,0.980312120051573,0.966410600022306)))
REPRESENTATION_ITEM('')
SURFACE()
);
#3188=(
BOUNDED_SURFACE()
B_SPLINE_SURFACE(1,2,((#265569,#265570,#265571,#265572,#265573,#265574,
#265575,#265576,#265577,#265578,#265579,#265580,#265581,#265582,#265583,
#265584,#265585,#265586,#265587,#265588,#265589,#265590,#265591,#265592,
#265593,#265594,#265595,#265596,#265597,#265598,#265599,#265600,#265601,
#265602,#265603,#265604,#265605,#265606,#265607,#265608,#265609,#265610,
#265611,#265612,#265613,#265614,#265615,#265616,#265617,#265618,#265619,
#265620,#265621,#265622,#265623,#265624,#265625,#265626,#265627,#265628,
#265629,#265630,#265631,#265632,#265633,#265634,#265635,#265636,#265637,
#265638,#265639,#265640,#265641,#265642,#265643,#265644,#265645,#265646,
#265647,#265648,#265649,#265650,#265651,#265652,#265653,#265654,#265655,
#265656,#265657,#265658,#265659,#265660,#265661,#265662,#265663,#265664,
#265665,#265666,#265667,#265668,#265669,#265670,#265671,#265672,#265673,
#265674,#265675,#265676,#265677,#265678,#265679,#265680,#265681,#265682,
#265683,#265684,#265685,#265686,#265687,#265688,#265689,#265690,#265691,
#265692,#265693,#265694,#265695,#265696,#265697,#265698,#265699,#265700,
#265701,#265702,#265703,#265704,#265705,#265706,#265707,#265708,#265709,
#265710,#265711,#265712,#265713,#265714,#265715,#265716,#265717,#265718,
#265719,#265720,#265721,#265722,#265723,#265724,#265725,#265726,#265727,
#265728,#265729,#265730,#265731,#265732,#265733,#265734,#265735,#265736,
#265737,#265738,#265739,#265740,#265741,#265742,#265743,#265744,#265745,
#265746,#265747,#265748,#265749,#265750,#265751,#265752,#265753,#265754,
#265755,#265756,#265757,#265758,#265759,#265760,#265761,#265762,#265763,
#265764,#265765,#265766,#265767,#265768,#265769,#265770,#265771,#265772,
#265773,#265774,#265775,#265776,#265777,#265778,#265779,#265780,#265781,
#265782,#265783,#265784,#265785,#265786,#265787,#265788,#265789,#265790,
#265791,#265792,#265793,#265794,#265795,#265796,#265797,#265798,#265799,
#265800,#265801,#265802,#265803,#265804,#265805,#265806,#265807,#265808,
#265809,#265810,#265811,#265812,#265813,#265814,#265815,#265816,#265817,
#265818,#265819,#265820,#265821,#265822,#265823,#265824,#265825,#265826,
#265827,#265828,#265829,#265830,#265831,#265832,#265833,#265834,#265835,
#265836,#265837,#265838,#265839,#265840,#265841,#265842,#265843,#265844,
#265845),(#265846,#265847,#265848,#265849,#265850,#265851,#265852,#265853,
#265854,#265855,#265856,#265857,#265858,#265859,#265860,#265861,#265862,
#265863,#265864,#265865,#265866,#265867,#265868,#265869,#265870,#265871,
#265872,#265873,#265874,#265875,#265876,#265877,#265878,#265879,#265880,
#265881,#265882,#265883,#265884,#265885,#265886,#265887,#265888,#265889,
#265890,#265891,#265892,#265893,#265894,#265895,#265896,#265897,#265898,
#265899,#265900,#265901,#265902,#265903,#265904,#265905,#265906,#265907,
#265908,#265909,#265910,#265911,#265912,#265913,#265914,#265915,#265916,
#265917,#265918,#265919,#265920,#265921,#265922,#265923,#265924,#265925,
#265926,#265927,#265928,#265929,#265930,#265931,#265932,#265933,#265934,
#265935,#265936,#265937,#265938,#265939,#265940,#265941,#265942,#265943,
#265944,#265945,#265946,#265947,#265948,#265949,#265950,#265951,#265952,
#265953,#265954,#265955,#265956,#265957,#265958,#265959,#265960,#265961,
#265962,#265963,#265964,#265965,#265966,#265967,#265968,#265969,#265970,
#265971,#265972,#265973,#265974,#265975,#265976,#265977,#265978,#265979,
#265980,#265981,#265982,#265983,#265984,#265985,#265986,#265987,#265988,
#265989,#265990,#265991,#265992,#265993,#265994,#265995,#265996,#265997,
#265998,#265999,#266000,#266001,#266002,#266003,#266004,#266005,#266006,
#266007,#266008,#266009,#266010,#266011,#266012,#266013,#266014,#266015,
#266016,#266017,#266018,#266019,#266020,#266021,#266022,#266023,#266024,
#266025,#266026,#266027,#266028,#266029,#266030,#266031,#266032,#266033,
#266034,#266035,#266036,#266037,#266038,#266039,#266040,#266041,#266042,
#266043,#266044,#266045,#266046,#266047,#266048,#266049,#266050,#266051,
#266052,#266053,#266054,#266055,#266056,#266057,#266058,#266059,#266060,
#266061,#266062,#266063,#266064,#266065,#266066,#266067,#266068,#266069,
#266070,#266071,#266072,#266073,#266074,#266075,#266076,#266077,#266078,
#266079,#266080,#266081,#266082,#266083,#266084,#266085,#266086,#266087,
#266088,#266089,#266090,#266091,#266092,#266093,#266094,#266095,#266096,
#266097,#266098,#266099,#266100,#266101,#266102,#266103,#266104,#266105,
#266106,#266107,#266108,#266109,#266110,#266111,#266112,#266113,#266114,
#266115,#266116,#266117,#266118,#266119,#266120,#266121,#266122)),
 .UNSPECIFIED.,.F.,.F.,.F.)
B_SPLINE_SURFACE_WITH_KNOTS((2,2),(3,2,2,2,2,2,2,2,2,2,2,2,2,2,2,2,2,2,
2,2,2,2,2,2,2,2,2,2,2,2,2,2,2,2,2,2,2,2,2,2,2,2,2,2,2,2,2,2,2,2,2,2,2,2,
2,2,2,2,2,2,2,2,2,2,2,2,2,2,2,2,2,2,2,2,2,2,2,2,2,2,2,2,2,2,2,2,2,2,2,2,
2,2,2,2,2,2,2,2,2,2,2,2,2,2,2,2,2,2,2,2,2,2,2,2,2,2,2,2,2,2,2,2,2,2,2,2,
2,2,2,2,2,2,2,2,2,2,2,2,3),(0.,1.),(0.,0.0072463768115942,0.0144927536231884,
0.0217391304347826,0.0289855072463768,0.036231884057971,0.0434782608695652,
0.0507246376811594,0.0579710144927536,0.0652173913043478,0.072463768115942,
0.0797101449275362,0.0869565217391304,0.0942028985507246,0.101449275362319,
0.108695652173913,0.115942028985507,0.123188405797101,0.130434782608696,
0.13768115942029,0.144927536231884,0.152173913043478,0.159420289855073,
0.166666666666667,0.173913043478261,0.181159420289855,0.18840579710145,
0.195652173913044,0.202898550724637,0.210144927536232,0.217391304347826,
0.224637681159421,0.231884057971014,0.239130434782609,0.246376811594203,
0.253623188405797,0.260869565217392,0.268115942028985,0.275362318840579,
0.282608695652174,0.289855072463768,0.297101449275363,0.304347826086956,
0.31159420289855,0.318840579710145,0.326086956521739,0.333333333333334,
0.340579710144927,0.347826086956521,0.355072463768116,0.36231884057971,
0.369565217391304,0.376811594202899,0.384057971014493,0.391304347826087,
0.398550724637681,0.405797101449275,0.41304347826087,0.420289855072463,
0.427536231884058,0.434782608695652,0.442028985507247,0.449275362318841,
0.456521739130435,0.463768115942029,0.471014492753623,0.478260869565218,
0.485507246376812,0.492753623188406,0.5,0.507246376811594,0.514492753623188,
0.521739130434783,0.528985507246377,0.536231884057971,0.543478260869565,
0.550724637681159,0.557971014492754,0.565217391304348,0.572463768115942,
0.579710144927536,0.586956521739131,0.594202898550725,0.601449275362319,
0.608695652173913,0.615942028985507,0.623188405797101,0.630434782608696,
0.63768115942029,0.644927536231884,0.652173913043478,0.659420289855073,
0.666666666666667,0.673913043478261,0.681159420289855,0.688405797101449,
0.695652173913044,0.702898550724638,0.710144927536232,0.717391304347826,
0.72463768115942,0.731884057971015,0.739130434782609,0.746376811594203,
0.753623188405797,0.760869565217391,0.768115942028986,0.77536231884058,
0.782608695652174,0.789855072463768,0.797101449275362,0.804347826086956,
0.811594202898551,0.818840579710145,0.826086956521739,0.833333333333333,
0.840579710144928,0.847826086956522,0.855072463768116,0.86231884057971,
0.869565217391304,0.876811594202899,0.884057971014493,0.891304347826087,
0.898550724637681,0.905797101449275,0.91304347826087,0.920289855072464,
0.927536231884058,0.934782608695652,0.942028985507246,0.94927536231884,
0.956521739130435,0.963768115942029,0.971014492753623,0.978260869565217,
0.985507246376812,0.992753623188406,0.993818585798284),.UNSPECIFIED.)
GEOMETRIC_REPRESENTATION_ITEM()
RATIONAL_B_SPLINE_SURFACE(((1.,0.866025403784439,1.,0.866025403784439,1.,
0.866025403784439,1.,0.866025403784439,1.,0.866025403784439,1.,0.866025403784439,
1.,0.866025403784439,1.,0.866025403784439,1.,0.866025403784439,1.,0.866025403784439,
1.,0.866025403784439,1.,0.866025403784439,1.,0.866025403784439,1.,0.866025403784439,
1.,0.866025403784439,1.,0.866025403784439,1.,0.866025403784439,1.,0.866025403784439,
1.,0.866025403784439,1.,0.866025403784439,1.,0.866025403784439,1.,0.866025403784439,
1.,0.866025403784439,1.,0.866025403784439,1.,0.866025403784439,1.,0.866025403784439,
1.,0.866025403784439,1.,0.866025403784439,1.,0.866025403784439,1.,0.866025403784439,
1.,0.866025403784439,1.,0.866025403784439,1.,0.866025403784439,1.,0.866025403784439,
1.,0.866025403784439,1.,0.866025403784439,1.,0.866025403784439,1.,0.866025403784439,
1.,0.866025403784439,1.,0.866025403784439,1.,0.866025403784439,1.,0.866025403784439,
1.,0.866025403784439,1.,0.866025403784439,1.,0.866025403784439,1.,0.866025403784439,
1.,0.866025403784439,1.,0.866025403784439,1.,0.866025403784439,1.,0.866025403784439,
1.,0.866025403784439,1.,0.866025403784439,1.,0.866025403784439,1.,0.866025403784439,
1.,0.866025403784439,1.,0.866025403784439,1.,0.866025403784439,1.,0.866025403784439,
1.,0.866025403784439,1.,0.866025403784439,1.,0.866025403784439,1.,0.866025403784439,
1.,0.866025403784439,1.,0.866025403784439,1.,0.866025403784439,1.,0.866025403784439,
1.,0.866025403784439,1.,0.866025403784439,1.,0.866025403784439,1.,0.866025403784439,
1.,0.866025403784439,1.,0.866025403784439,1.,0.866025403784439,1.,0.866025403784439,
1.,0.866025403784439,1.,0.866025403784439,1.,0.866025403784439,1.,0.866025403784439,
1.,0.866025403784439,1.,0.866025403784439,1.,0.866025403784439,1.,0.866025403784439,
1.,0.866025403784439,1.,0.866025403784439,1.,0.866025403784439,1.,0.866025403784439,
1.,0.866025403784439,1.,0.866025403784439,1.,0.866025403784439,1.,0.866025403784439,
1.,0.866025403784439,1.,0.866025403784439,1.,0.866025403784439,1.,0.866025403784439,
1.,0.866025403784439,1.,0.866025403784439,1.,0.866025403784439,1.,0.866025403784439,
1.,0.866025403784439,1.,0.866025403784439,1.,0.866025403784439,1.,0.866025403784439,
1.,0.866025403784439,1.,0.866025403784439,1.,0.866025403784439,1.,0.866025403784439,
1.,0.866025403784439,1.,0.866025403784439,1.,0.866025403784439,1.,0.866025403784439,
1.,0.866025403784439,1.,0.866025403784439,1.,0.866025403784439,1.,0.866025403784439,
1.,0.866025403784439,1.,0.866025403784439,1.,0.866025403784439,1.,0.866025403784439,
1.,0.866025403784439,1.,0.866025403784439,1.,0.866025403784439,1.,0.866025403784439,
1.,0.866025403784439,1.,0.866025403784439,1.,0.866025403784439,1.,0.866025403784439,
1.,0.866025403784439,1.,0.866025403784439,1.,0.866025403784439,1.,0.866025403784439,
1.,0.866025403784439,1.,0.866025403784439,1.,0.866025403784439,1.,0.866025403784439,
1.,0.866025403784439,1.,0.866025403784439,1.,0.866025403784439,1.,0.98031044488126,
0.966408234404338),(1.,0.866025403784439,1.,0.866025403784439,1.,0.866025403784439,
1.,0.866025403784439,1.,0.866025403784439,1.,0.866025403784439,1.,0.866025403784439,
1.,0.866025403784439,1.,0.866025403784439,1.,0.866025403784439,1.,0.866025403784439,
1.,0.866025403784439,1.,0.866025403784439,1.,0.866025403784439,1.,0.866025403784439,
1.,0.866025403784439,1.,0.866025403784439,1.,0.866025403784439,1.,0.866025403784439,
1.,0.866025403784439,1.,0.866025403784439,1.,0.866025403784439,1.,0.866025403784439,
1.,0.866025403784439,1.,0.866025403784439,1.,0.866025403784439,1.,0.866025403784439,
1.,0.866025403784439,1.,0.866025403784439,1.,0.866025403784439,1.,0.866025403784439,
1.,0.866025403784439,1.,0.866025403784439,1.,0.866025403784439,1.,0.866025403784439,
1.,0.866025403784439,1.,0.866025403784439,1.,0.866025403784439,1.,0.866025403784439,
1.,0.866025403784439,1.,0.866025403784439,1.,0.866025403784439,1.,0.866025403784439,
1.,0.866025403784439,1.,0.866025403784439,1.,0.866025403784439,1.,0.866025403784439,
1.,0.866025403784439,1.,0.866025403784439,1.,0.866025403784439,1.,0.866025403784439,
1.,0.866025403784439,1.,0.866025403784439,1.,0.866025403784439,1.,0.866025403784439,
1.,0.866025403784439,1.,0.866025403784439,1.,0.866025403784439,1.,0.866025403784439,
1.,0.866025403784439,1.,0.866025403784439,1.,0.866025403784439,1.,0.866025403784439,
1.,0.866025403784439,1.,0.866025403784439,1.,0.866025403784439,1.,0.866025403784439,
1.,0.866025403784439,1.,0.866025403784439,1.,0.866025403784439,1.,0.866025403784439,
1.,0.866025403784439,1.,0.866025403784439,1.,0.866025403784439,1.,0.866025403784439,
1.,0.866025403784439,1.,0.866025403784439,1.,0.866025403784439,1.,0.866025403784439,
1.,0.866025403784439,1.,0.866025403784439,1.,0.866025403784439,1.,0.866025403784439,
1.,0.866025403784439,1.,0.866025403784439,1.,0.866025403784439,1.,0.866025403784439,
1.,0.866025403784439,1.,0.866025403784439,1.,0.866025403784439,1.,0.866025403784439,
1.,0.866025403784439,1.,0.866025403784439,1.,0.866025403784439,1.,0.866025403784439,
1.,0.866025403784439,1.,0.866025403784439,1.,0.866025403784439,1.,0.866025403784439,
1.,0.866025403784439,1.,0.866025403784439,1.,0.866025403784439,1.,0.866025403784439,
1.,0.866025403784439,1.,0.866025403784439,1.,0.866025403784439,1.,0.866025403784439,
1.,0.866025403784439,1.,0.866025403784439,1.,0.866025403784439,1.,0.866025403784439,
1.,0.866025403784439,1.,0.866025403784439,1.,0.866025403784439,1.,0.866025403784439,
1.,0.866025403784439,1.,0.866025403784439,1.,0.866025403784439,1.,0.866025403784439,
1.,0.866025403784439,1.,0.866025403784439,1.,0.866025403784439,1.,0.866025403784439,
1.,0.866025403784439,1.,0.866025403784439,1.,0.866025403784439,1.,0.866025403784439,
1.,0.866025403784439,1.,0.866025403784439,1.,0.866025403784439,1.,0.866025403784439,
1.,0.866025403784439,1.,0.866025403784439,1.,0.866025403784439,1.,0.866025403784439,
1.,0.866025403784439,1.,0.866025403784439,1.,0.98031044488126,0.966408234404338)))
REPRESENTATION_ITEM('')
SURFACE()
);
#3189=(
BOUNDED_SURFACE()
B_SPLINE_SURFACE(1,2,((#266133,#266134,#266135,#266136,#266137,#266138,
#266139,#266140,#266141,#266142,#266143,#266144,#266145,#266146,#266147,
#266148,#266149,#266150,#266151,#266152,#266153,#266154,#266155,#266156,
#266157,#266158,#266159,#266160,#266161,#266162,#266163,#266164,#266165,
#266166,#266167,#266168,#266169,#266170,#266171,#266172,#266173,#266174,
#266175,#266176,#266177,#266178,#266179,#266180,#266181,#266182,#266183,
#266184,#266185,#266186,#266187,#266188,#266189,#266190,#266191,#266192,
#266193,#266194,#266195,#266196,#266197,#266198,#266199,#266200,#266201,
#266202,#266203,#266204,#266205,#266206,#266207,#266208,#266209,#266210,
#266211,#266212,#266213,#266214,#266215,#266216,#266217,#266218,#266219,
#266220,#266221,#266222,#266223,#266224,#266225,#266226,#266227,#266228,
#266229,#266230,#266231,#266232,#266233,#266234,#266235,#266236,#266237,
#266238,#266239,#266240,#266241,#266242,#266243,#266244,#266245,#266246,
#266247,#266248,#266249,#266250,#266251,#266252,#266253,#266254,#266255,
#266256,#266257,#266258,#266259,#266260,#266261,#266262,#266263,#266264,
#266265,#266266,#266267,#266268,#266269,#266270,#266271,#266272,#266273,
#266274,#266275,#266276,#266277,#266278,#266279,#266280,#266281,#266282,
#266283,#266284,#266285,#266286,#266287,#266288,#266289,#266290,#266291,
#266292,#266293,#266294,#266295,#266296,#266297,#266298,#266299,#266300,
#266301,#266302,#266303,#266304,#266305,#266306,#266307,#266308,#266309,
#266310,#266311,#266312,#266313,#266314,#266315,#266316,#266317,#266318,
#266319,#266320,#266321,#266322,#266323,#266324,#266325,#266326,#266327,
#266328,#266329,#266330,#266331,#266332,#266333,#266334,#266335,#266336,
#266337,#266338,#266339,#266340,#266341,#266342,#266343,#266344,#266345,
#266346,#266347,#266348,#266349,#266350,#266351,#266352,#266353,#266354,
#266355,#266356,#266357,#266358,#266359,#266360,#266361,#266362,#266363,
#266364,#266365,#266366,#266367,#266368,#266369,#266370,#266371,#266372,
#266373,#266374,#266375,#266376,#266377,#266378,#266379,#266380,#266381,
#266382,#266383,#266384,#266385,#266386,#266387,#266388,#266389,#266390,
#266391,#266392,#266393,#266394,#266395,#266396,#266397,#266398,#266399,
#266400,#266401,#266402,#266403,#266404,#266405,#266406,#266407,#266408,
#266409),(#266410,#266411,#266412,#266413,#266414,#266415,#266416,#266417,
#266418,#266419,#266420,#266421,#266422,#266423,#266424,#266425,#266426,
#266427,#266428,#266429,#266430,#266431,#266432,#266433,#266434,#266435,
#266436,#266437,#266438,#266439,#266440,#266441,#266442,#266443,#266444,
#266445,#266446,#266447,#266448,#266449,#266450,#266451,#266452,#266453,
#266454,#266455,#266456,#266457,#266458,#266459,#266460,#266461,#266462,
#266463,#266464,#266465,#266466,#266467,#266468,#266469,#266470,#266471,
#266472,#266473,#266474,#266475,#266476,#266477,#266478,#266479,#266480,
#266481,#266482,#266483,#266484,#266485,#266486,#266487,#266488,#266489,
#266490,#266491,#266492,#266493,#266494,#266495,#266496,#266497,#266498,
#266499,#266500,#266501,#266502,#266503,#266504,#266505,#266506,#266507,
#266508,#266509,#266510,#266511,#266512,#266513,#266514,#266515,#266516,
#266517,#266518,#266519,#266520,#266521,#266522,#266523,#266524,#266525,
#266526,#266527,#266528,#266529,#266530,#266531,#266532,#266533,#266534,
#266535,#266536,#266537,#266538,#266539,#266540,#266541,#266542,#266543,
#266544,#266545,#266546,#266547,#266548,#266549,#266550,#266551,#266552,
#266553,#266554,#266555,#266556,#266557,#266558,#266559,#266560,#266561,
#266562,#266563,#266564,#266565,#266566,#266567,#266568,#266569,#266570,
#266571,#266572,#266573,#266574,#266575,#266576,#266577,#266578,#266579,
#266580,#266581,#266582,#266583,#266584,#266585,#266586,#266587,#266588,
#266589,#266590,#266591,#266592,#266593,#266594,#266595,#266596,#266597,
#266598,#266599,#266600,#266601,#266602,#266603,#266604,#266605,#266606,
#266607,#266608,#266609,#266610,#266611,#266612,#266613,#266614,#266615,
#266616,#266617,#266618,#266619,#266620,#266621,#266622,#266623,#266624,
#266625,#266626,#266627,#266628,#266629,#266630,#266631,#266632,#266633,
#266634,#266635,#266636,#266637,#266638,#266639,#266640,#266641,#266642,
#266643,#266644,#266645,#266646,#266647,#266648,#266649,#266650,#266651,
#266652,#266653,#266654,#266655,#266656,#266657,#266658,#266659,#266660,
#266661,#266662,#266663,#266664,#266665,#266666,#266667,#266668,#266669,
#266670,#266671,#266672,#266673,#266674,#266675,#266676,#266677,#266678,
#266679,#266680,#266681,#266682,#266683,#266684,#266685,#266686)),
 .UNSPECIFIED.,.F.,.F.,.F.)
B_SPLINE_SURFACE_WITH_KNOTS((2,2),(3,2,2,2,2,2,2,2,2,2,2,2,2,2,2,2,2,2,
2,2,2,2,2,2,2,2,2,2,2,2,2,2,2,2,2,2,2,2,2,2,2,2,2,2,2,2,2,2,2,2,2,2,2,2,
2,2,2,2,2,2,2,2,2,2,2,2,2,2,2,2,2,2,2,2,2,2,2,2,2,2,2,2,2,2,2,2,2,2,2,2,
2,2,2,2,2,2,2,2,2,2,2,2,2,2,2,2,2,2,2,2,2,2,2,2,2,2,2,2,2,2,2,2,2,2,2,2,
2,2,2,2,2,2,2,2,2,2,2,2,3),(0.,1.),(0.,0.0072463768115942,0.0144927536231884,
0.0217391304347826,0.0289855072463768,0.036231884057971,0.0434782608695652,
0.0507246376811594,0.0579710144927536,0.0652173913043478,0.072463768115942,
0.0797101449275362,0.0869565217391304,0.0942028985507246,0.101449275362319,
0.108695652173913,0.115942028985507,0.123188405797101,0.130434782608696,
0.13768115942029,0.144927536231884,0.152173913043478,0.159420289855073,
0.166666666666667,0.173913043478261,0.181159420289855,0.18840579710145,
0.195652173913044,0.202898550724637,0.210144927536232,0.217391304347826,
0.224637681159421,0.231884057971014,0.239130434782609,0.246376811594203,
0.253623188405797,0.260869565217392,0.268115942028985,0.275362318840579,
0.282608695652174,0.289855072463768,0.297101449275363,0.304347826086956,
0.31159420289855,0.318840579710145,0.326086956521739,0.333333333333334,
0.340579710144927,0.347826086956521,0.355072463768116,0.36231884057971,
0.369565217391304,0.376811594202899,0.384057971014493,0.391304347826087,
0.398550724637681,0.405797101449275,0.41304347826087,0.420289855072463,
0.427536231884058,0.434782608695652,0.442028985507247,0.449275362318841,
0.456521739130435,0.463768115942029,0.471014492753623,0.478260869565218,
0.485507246376812,0.492753623188406,0.5,0.507246376811594,0.514492753623188,
0.521739130434783,0.528985507246377,0.536231884057971,0.543478260869565,
0.550724637681159,0.557971014492754,0.565217391304348,0.572463768115942,
0.579710144927536,0.586956521739131,0.594202898550725,0.601449275362319,
0.608695652173913,0.615942028985507,0.623188405797101,0.630434782608696,
0.63768115942029,0.644927536231884,0.652173913043478,0.659420289855073,
0.666666666666667,0.673913043478261,0.681159420289855,0.688405797101449,
0.695652173913044,0.702898550724638,0.710144927536232,0.717391304347826,
0.72463768115942,0.731884057971015,0.739130434782609,0.746376811594203,
0.753623188405797,0.760869565217391,0.768115942028986,0.77536231884058,
0.782608695652174,0.789855072463768,0.797101449275362,0.804347826086956,
0.811594202898551,0.818840579710145,0.826086956521739,0.833333333333333,
0.840579710144928,0.847826086956522,0.855072463768116,0.86231884057971,
0.869565217391304,0.876811594202899,0.884057971014493,0.891304347826087,
0.898550724637681,0.905797101449275,0.91304347826087,0.920289855072464,
0.927536231884058,0.934782608695652,0.942028985507246,0.94927536231884,
0.956521739130435,0.963768115942029,0.971014492753623,0.978260869565217,
0.985507246376812,0.992753623188406,0.993818585798284),.UNSPECIFIED.)
GEOMETRIC_REPRESENTATION_ITEM()
RATIONAL_B_SPLINE_SURFACE(((1.,0.866025403784439,1.,0.866025403784439,1.,
0.866025403784439,1.,0.866025403784439,1.,0.866025403784439,1.,0.866025403784439,
1.,0.866025403784439,1.,0.866025403784439,1.,0.866025403784439,1.,0.866025403784439,
1.,0.866025403784439,1.,0.866025403784439,1.,0.866025403784439,1.,0.866025403784439,
1.,0.866025403784439,1.,0.866025403784439,1.,0.866025403784439,1.,0.866025403784439,
1.,0.866025403784439,1.,0.866025403784439,1.,0.866025403784439,1.,0.866025403784439,
1.,0.866025403784439,1.,0.866025403784439,1.,0.866025403784439,1.,0.866025403784439,
1.,0.866025403784439,1.,0.866025403784439,1.,0.866025403784439,1.,0.866025403784439,
1.,0.866025403784439,1.,0.866025403784439,1.,0.866025403784439,1.,0.866025403784439,
1.,0.866025403784439,1.,0.866025403784439,1.,0.866025403784439,1.,0.866025403784439,
1.,0.866025403784439,1.,0.866025403784439,1.,0.866025403784439,1.,0.866025403784439,
1.,0.866025403784439,1.,0.866025403784439,1.,0.866025403784439,1.,0.866025403784439,
1.,0.866025403784439,1.,0.866025403784439,1.,0.866025403784439,1.,0.866025403784439,
1.,0.866025403784439,1.,0.866025403784439,1.,0.866025403784439,1.,0.866025403784439,
1.,0.866025403784439,1.,0.866025403784439,1.,0.866025403784439,1.,0.866025403784439,
1.,0.866025403784439,1.,0.866025403784439,1.,0.866025403784439,1.,0.866025403784439,
1.,0.866025403784439,1.,0.866025403784439,1.,0.866025403784439,1.,0.866025403784439,
1.,0.866025403784439,1.,0.866025403784439,1.,0.866025403784439,1.,0.866025403784439,
1.,0.866025403784439,1.,0.866025403784439,1.,0.866025403784439,1.,0.866025403784439,
1.,0.866025403784439,1.,0.866025403784439,1.,0.866025403784439,1.,0.866025403784439,
1.,0.866025403784439,1.,0.866025403784439,1.,0.866025403784439,1.,0.866025403784439,
1.,0.866025403784439,1.,0.866025403784439,1.,0.866025403784439,1.,0.866025403784439,
1.,0.866025403784439,1.,0.866025403784439,1.,0.866025403784439,1.,0.866025403784439,
1.,0.866025403784439,1.,0.866025403784439,1.,0.866025403784439,1.,0.866025403784439,
1.,0.866025403784439,1.,0.866025403784439,1.,0.866025403784439,1.,0.866025403784439,
1.,0.866025403784439,1.,0.866025403784439,1.,0.866025403784439,1.,0.866025403784439,
1.,0.866025403784439,1.,0.866025403784439,1.,0.866025403784439,1.,0.866025403784439,
1.,0.866025403784439,1.,0.866025403784439,1.,0.866025403784439,1.,0.866025403784439,
1.,0.866025403784439,1.,0.866025403784439,1.,0.866025403784439,1.,0.866025403784439,
1.,0.866025403784439,1.,0.866025403784439,1.,0.866025403784439,1.,0.866025403784439,
1.,0.866025403784439,1.,0.866025403784439,1.,0.866025403784439,1.,0.866025403784439,
1.,0.866025403784439,1.,0.866025403784439,1.,0.866025403784439,1.,0.866025403784439,
1.,0.866025403784439,1.,0.866025403784439,1.,0.866025403784439,1.,0.866025403784439,
1.,0.866025403784439,1.,0.866025403784439,1.,0.866025403784439,1.,0.866025403784439,
1.,0.866025403784439,1.,0.866025403784439,1.,0.866025403784439,1.,0.98031044488126,
0.966408234404338),(1.,0.866025403784439,1.,0.866025403784439,1.,0.866025403784439,
1.,0.866025403784439,1.,0.866025403784439,1.,0.866025403784439,1.,0.866025403784439,
1.,0.866025403784439,1.,0.866025403784439,1.,0.866025403784439,1.,0.866025403784439,
1.,0.866025403784439,1.,0.866025403784439,1.,0.866025403784439,1.,0.866025403784439,
1.,0.866025403784439,1.,0.866025403784439,1.,0.866025403784439,1.,0.866025403784439,
1.,0.866025403784439,1.,0.866025403784439,1.,0.866025403784439,1.,0.866025403784439,
1.,0.866025403784439,1.,0.866025403784439,1.,0.866025403784439,1.,0.866025403784439,
1.,0.866025403784439,1.,0.866025403784439,1.,0.866025403784439,1.,0.866025403784439,
1.,0.866025403784439,1.,0.866025403784439,1.,0.866025403784439,1.,0.866025403784439,
1.,0.866025403784439,1.,0.866025403784439,1.,0.866025403784439,1.,0.866025403784439,
1.,0.866025403784439,1.,0.866025403784439,1.,0.866025403784439,1.,0.866025403784439,
1.,0.866025403784439,1.,0.866025403784439,1.,0.866025403784439,1.,0.866025403784439,
1.,0.866025403784439,1.,0.866025403784439,1.,0.866025403784439,1.,0.866025403784439,
1.,0.866025403784439,1.,0.866025403784439,1.,0.866025403784439,1.,0.866025403784439,
1.,0.866025403784439,1.,0.866025403784439,1.,0.866025403784439,1.,0.866025403784439,
1.,0.866025403784439,1.,0.866025403784439,1.,0.866025403784439,1.,0.866025403784439,
1.,0.866025403784439,1.,0.866025403784439,1.,0.866025403784439,1.,0.866025403784439,
1.,0.866025403784439,1.,0.866025403784439,1.,0.866025403784439,1.,0.866025403784439,
1.,0.866025403784439,1.,0.866025403784439,1.,0.866025403784439,1.,0.866025403784439,
1.,0.866025403784439,1.,0.866025403784439,1.,0.866025403784439,1.,0.866025403784439,
1.,0.866025403784439,1.,0.866025403784439,1.,0.866025403784439,1.,0.866025403784439,
1.,0.866025403784439,1.,0.866025403784439,1.,0.866025403784439,1.,0.866025403784439,
1.,0.866025403784439,1.,0.866025403784439,1.,0.866025403784439,1.,0.866025403784439,
1.,0.866025403784439,1.,0.866025403784439,1.,0.866025403784439,1.,0.866025403784439,
1.,0.866025403784439,1.,0.866025403784439,1.,0.866025403784439,1.,0.866025403784439,
1.,0.866025403784439,1.,0.866025403784439,1.,0.866025403784439,1.,0.866025403784439,
1.,0.866025403784439,1.,0.866025403784439,1.,0.866025403784439,1.,0.866025403784439,
1.,0.866025403784439,1.,0.866025403784439,1.,0.866025403784439,1.,0.866025403784439,
1.,0.866025403784439,1.,0.866025403784439,1.,0.866025403784439,1.,0.866025403784439,
1.,0.866025403784439,1.,0.866025403784439,1.,0.866025403784439,1.,0.866025403784439,
1.,0.866025403784439,1.,0.866025403784439,1.,0.866025403784439,1.,0.866025403784439,
1.,0.866025403784439,1.,0.866025403784439,1.,0.866025403784439,1.,0.866025403784439,
1.,0.866025403784439,1.,0.866025403784439,1.,0.866025403784439,1.,0.866025403784439,
1.,0.866025403784439,1.,0.866025403784439,1.,0.866025403784439,1.,0.866025403784439,
1.,0.866025403784439,1.,0.866025403784439,1.,0.98031044488126,0.966408234404338)))
REPRESENTATION_ITEM('')
SURFACE()
);
#3190=(
BOUNDED_SURFACE()
B_SPLINE_SURFACE(3,2,((#271081,#271082,#271083),(#271084,#271085,#271086),
(#271087,#271088,#271089),(#271090,#271091,#271092),(#271093,#271094,#271095),
(#271096,#271097,#271098),(#271099,#271100,#271101),(#271102,#271103,#271104),
(#271105,#271106,#271107),(#271108,#271109,#271110),(#271111,#271112,#271113),
(#271114,#271115,#271116),(#271117,#271118,#271119),(#271120,#271121,#271122),
(#271123,#271124,#271125),(#271126,#271127,#271128)),.UNSPECIFIED.,.F.,
 .F.,.F.)
B_SPLINE_SURFACE_WITH_KNOTS((4,2,2,2,2,2,2,4),(3,3),(0.021246894993388,
0.0219851502508119,0.0226493629442376,0.0233135756376633,0.023977788331089,
0.0246420010245147,0.0253062137179403,0.02670868166879),(-7.40425639982891E-5,
1.),.UNSPECIFIED.)
GEOMETRIC_REPRESENTATION_ITEM()
RATIONAL_B_SPLINE_SURFACE(((1.00002710501715,0.816963272991268,1.),(1.00002702241829,
0.817521052555119,1.),(1.00002733502832,0.815410036827724,1.),(1.00002846649364,
0.807769395738777,1.),(1.00002922674044,0.802635545928914,1.),(1.00003092826825,
0.791145345435121,1.),(1.00003186568695,0.784815076400909,1.),(1.00003372138338,
0.772283794894346,1.),(1.00003464066055,0.76607603331725,1.),(1.00003637793641,
0.754344430769809,1.),(1.00003719750955,0.748809957783788,1.),(1.00003871890084,
0.738536196261916,1.),(1.00003942162688,0.733790776873006,1.),(1.00004143922335,
0.720166205006836,1.),(1.00004256778357,0.712545181611092,1.),(1.00004353016739,
0.706046326330694,1.)))
REPRESENTATION_ITEM('')
SURFACE()
);
#3191=(
BOUNDED_SURFACE()
B_SPLINE_SURFACE(3,2,((#271130,#271131,#271132),(#271133,#271134,#271135),
(#271136,#271137,#271138),(#271139,#271140,#271141),(#271142,#271143,#271144),
(#271145,#271146,#271147),(#271148,#271149,#271150),(#271151,#271152,#271153),
(#271154,#271155,#271156),(#271157,#271158,#271159),(#271160,#271161,#271162),
(#271163,#271164,#271165),(#271166,#271167,#271168),(#271169,#271170,#271171),
(#271172,#271173,#271174),(#271175,#271176,#271177)),.UNSPECIFIED.,.F.,
 .F.,.F.)
B_SPLINE_SURFACE_WITH_KNOTS((4,2,2,2,2,2,2,4),(3,3),(0.0159102555591329,
0.0173176440494504,0.0179848596341063,0.0186520752187623,0.0193192908034183,
0.0199865063880743,0.0206537219727303,0.0213938948783918),(-7.2957321005512E-5,
1.),.UNSPECIFIED.)
GEOMETRIC_REPRESENTATION_ITEM()
RATIONAL_B_SPLINE_SURFACE(((1.00004288879452,0.706069288657398,1.),(1.00004194432714,
0.71254202756886,1.),(1.00004082887242,0.720186597774606,1.),(1.00003884013724,
0.733816039950407,1.),(1.00003814748,0.7385630429368,1.),(1.00003664903336,
0.748832379971001,1.),(1.00003584236797,0.754360717483753,1.),(1.00003413328098,
0.766073640691051,1.),(1.00003322932712,0.772268727405263,1.),(1.0000314042151,
0.78477680737215,1.),(1.00003048201287,0.791096956071881,1.),(1.00002880594349,
0.802583598909048,1.),(1.00002805569383,0.807725301287472,1.),(1.00002693784998,
0.815386244970287,1.),(1.00002662695858,0.817516883782438,1.),(1.00002670733337,
0.816966049480649,1.)))
REPRESENTATION_ITEM('')
SURFACE()
);
#3206=TOROIDAL_SURFACE('',#94111,2.5,0.5);
#3207=TOROIDAL_SURFACE('',#94120,2.,1.);
#3208=TOROIDAL_SURFACE('',#94128,2.,1.);
#3209=TOROIDAL_SURFACE('',#94138,57.3875000000282,1.);
#3210=TOROIDAL_SURFACE('',#94155,57.3875000000282,1.);
#3211=TOROIDAL_SURFACE('',#94165,58.8875000000282,0.5);
#3212=TOROIDAL_SURFACE('',#94172,57.3875000000282,1.);
#3213=TOROIDAL_SURFACE('',#94181,58.8875000000282,0.5);
#3214=TOROIDAL_SURFACE('',#94186,57.3875000000282,1.);
#3215=TOROIDAL_SURFACE('',#94194,58.8875000000282,0.5);
#3216=TOROIDAL_SURFACE('',#94201,57.3875000000282,1.);
#3217=TOROIDAL_SURFACE('',#94216,57.3875000000282,1.);
#3218=TOROIDAL_SURFACE('',#94233,4.5,0.5);
#3219=TOROIDAL_SURFACE('',#94256,4.5,0.5);
#3220=TOROIDAL_SURFACE('',#94265,2.,1.);
#3221=TOROIDAL_SURFACE('',#94273,2.,1.);
#3222=TOROIDAL_SURFACE('',#94281,57.3875000000282,1.);
#3223=TOROIDAL_SURFACE('',#94289,58.8875000000282,0.5);
#3224=TOROIDAL_SURFACE('',#94295,57.3875000000282,1.);
#3225=TOROIDAL_SURFACE('',#94308,57.3875000000282,1.);
#3226=TOROIDAL_SURFACE('',#94321,57.3875000000282,1.);
#3227=TOROIDAL_SURFACE('',#94334,57.3875000000282,1.);
#3228=TOROIDAL_SURFACE('',#94342,58.8875000000282,0.5);
#3229=TOROIDAL_SURFACE('',#94348,57.3875000000282,1.);
#3230=TOROIDAL_SURFACE('',#94474,1.,0.5);
#3231=TOROIDAL_SURFACE('',#94486,1.,0.5);
#3232=TOROIDAL_SURFACE('',#94492,1.,0.5);
#3233=TOROIDAL_SURFACE('',#94498,45.1752328136335,1.);
#3234=TOROIDAL_SURFACE('',#94506,1.,0.5);
#3235=TOROIDAL_SURFACE('',#94512,1.,0.5);
#3236=TOROIDAL_SURFACE('',#94518,45.1752328136335,1.);
#3237=TOROIDAL_SURFACE('',#94528,1.,0.5);
#3238=TOROIDAL_SURFACE('',#94534,1.,0.5);
#3239=TOROIDAL_SURFACE('',#94546,1.,0.5);
#3240=TOROIDAL_SURFACE('',#94552,1.,0.5);
#3241=TOROIDAL_SURFACE('',#94566,4.5,0.5);
#3242=TOROIDAL_SURFACE('',#94575,5.25,0.25);
#3243=TOROIDAL_SURFACE('',#94581,2.75,0.25);
#3244=TOROIDAL_SURFACE('',#94585,67.25,0.25);
#3245=TOROIDAL_SURFACE('',#94589,2.75,0.25);
#3246=TOROIDAL_SURFACE('',#94595,5.25,0.25);
#3247=TOROIDAL_SURFACE('',#94599,58.25,0.25);
#3248=TOROIDAL_SURFACE('',#94603,5.25,0.25);
#3249=TOROIDAL_SURFACE('',#94609,2.75,0.25);
#3250=TOROIDAL_SURFACE('',#94613,67.25,0.25);
#3251=TOROIDAL_SURFACE('',#94617,2.75,0.25);
#3252=TOROIDAL_SURFACE('',#94623,3.25,0.25);
#3253=TOROIDAL_SURFACE('',#94640,57.5,1.);
#3254=TOROIDAL_SURFACE('',#94649,59.,0.5);
#3255=TOROIDAL_SURFACE('',#94656,57.5,1.);
#3256=TOROIDAL_SURFACE('',#94671,57.5,1.);
#3257=TOROIDAL_SURFACE('',#94683,59.,0.5);
#3258=TOROIDAL_SURFACE('',#94733,59.024570260837,1.);
#3259=TOROIDAL_SURFACE('',#94888,59.024570260837,1.);
#3260=TOROIDAL_SURFACE('',#94956,59.024570260837,1.);
#3261=TOROIDAL_SURFACE('',#94973,59.024570260837,1.);
#3262=TOROIDAL_SURFACE('',#95024,59.,0.5);
#3263=TOROIDAL_SURFACE('',#95044,2.5,0.5);
#3264=TOROIDAL_SURFACE('',#95052,3.5,0.5);
#3265=TOROIDAL_SURFACE('',#95199,2.5,0.5);
#3266=TOROIDAL_SURFACE('',#95204,2.5,0.5);
#3267=TOROIDAL_SURFACE('',#95208,2.5,0.5);
#3268=TOROIDAL_SURFACE('',#95217,2.5,0.5);
#3269=TOROIDAL_SURFACE('',#95224,2.5,0.5);
#3270=TOROIDAL_SURFACE('',#95229,2.5,0.5);
#3271=TOROIDAL_SURFACE('',#95236,2.5,0.5);
#3272=TOROIDAL_SURFACE('',#95240,2.5,0.5);
#3273=TOROIDAL_SURFACE('',#95245,2.5,0.5);
#3274=TOROIDAL_SURFACE('',#95250,2.5,0.5);
#3275=TOROIDAL_SURFACE('',#95252,2.5,0.5);
#3276=TOROIDAL_SURFACE('',#95257,2.5,0.5);
#3277=TOROIDAL_SURFACE('',#95273,2.5,0.5);
#3278=TOROIDAL_SURFACE('',#95287,2.5,0.5);
#3279=TOROIDAL_SURFACE('',#95292,2.5,0.5);
#3280=TOROIDAL_SURFACE('',#95296,2.5,0.5);
#3281=TOROIDAL_SURFACE('',#95301,2.5,0.5);
#3282=TOROIDAL_SURFACE('',#95403,2.5,0.5);
#3283=TOROIDAL_SURFACE('',#95409,2.5,0.5);
#3284=TOROIDAL_SURFACE('',#95413,2.5,0.5);
#3285=TOROIDAL_SURFACE('',#95418,2.5,0.5);
#3286=TOROIDAL_SURFACE('',#95439,2.5,0.5);
#3287=TOROIDAL_SURFACE('',#95452,59.024570260837,1.);
#3288=TOROIDAL_SURFACE('',#95461,2.5,0.5);
#3289=TOROIDAL_SURFACE('',#95466,2.5,0.5);
#3290=TOROIDAL_SURFACE('',#95479,2.5,0.5);
#3291=TOROIDAL_SURFACE('',#95491,2.5,0.5);
#3292=TOROIDAL_SURFACE('',#95511,2.5,0.5);
#3293=TOROIDAL_SURFACE('',#95531,2.5,0.5);
#3294=TOROIDAL_SURFACE('',#95536,2.5,0.5);
#3295=TOROIDAL_SURFACE('',#95540,2.5,0.5);
#3296=TOROIDAL_SURFACE('',#95559,2.5,0.5);
#3297=TOROIDAL_SURFACE('',#95561,59.024570260837,1.);
#3298=TOROIDAL_SURFACE('',#95571,2.5,0.5);
#3299=TOROIDAL_SURFACE('',#95575,2.5,0.5);
#3300=TOROIDAL_SURFACE('',#95582,2.5,0.5);
#3301=TOROIDAL_SURFACE('',#95586,2.5,0.5);
#3302=TOROIDAL_SURFACE('',#95591,59.024570260837,1.);
#3303=TOROIDAL_SURFACE('',#95604,2.5,0.5);
#3304=TOROIDAL_SURFACE('',#95609,2.5,0.5);
#3305=TOROIDAL_SURFACE('',#95622,2.5,0.5);
#3306=TOROIDAL_SURFACE('',#95627,2.5,0.5);
#3307=TOROIDAL_SURFACE('',#95655,2.5,0.5);
#3308=TOROIDAL_SURFACE('',#95675,2.5,0.5);
#3309=TOROIDAL_SURFACE('',#95680,2.5,0.5);
#3310=TOROIDAL_SURFACE('',#95684,2.5,0.5);
#3311=TOROIDAL_SURFACE('',#95703,2.5,0.5);
#3312=TOROIDAL_SURFACE('',#95716,2.5,0.5);
#3313=TOROIDAL_SURFACE('',#95733,2.5,0.5);
#3314=TOROIDAL_SURFACE('',#95738,2.5,0.5);
#3315=TOROIDAL_SURFACE('',#95748,2.5,0.5);
#3316=TOROIDAL_SURFACE('',#95770,2.5,0.5);
#3317=TOROIDAL_SURFACE('',#95772,59.024570260837,1.);
#3318=TOROIDAL_SURFACE('',#95791,2.5,0.5);
#3319=TOROIDAL_SURFACE('',#95796,2.5,0.5);
#3320=TOROIDAL_SURFACE('',#95800,2.5,0.5);
#3321=TOROIDAL_SURFACE('',#95820,2.5,0.5);
#3322=TOROIDAL_SURFACE('',#95829,2.,1.);
#3323=TOROIDAL_SURFACE('',#95831,66.5,1.);
#3324=TOROIDAL_SURFACE('',#95833,2.,1.);
#3325=TOROIDAL_SURFACE('',#95848,59.,0.5);
#3326=TOROIDAL_SURFACE('',#95851,57.5,1.);
#3327=TOROIDAL_SURFACE('',#95854,59.,0.5);
#3328=TOROIDAL_SURFACE('',#95858,57.5,1.);
#3329=TOROIDAL_SURFACE('',#95863,57.5,1.);
#3330=TOROIDAL_SURFACE('',#95868,57.5,1.);
#3331=TOROIDAL_SURFACE('',#95873,57.5,1.);
#3332=TOROIDAL_SURFACE('',#95877,59.,0.5);
#3333=TOROIDAL_SURFACE('',#95880,57.5,1.);
#3334=TOROIDAL_SURFACE('',#95883,59.,0.5);
#3335=TOROIDAL_SURFACE('',#95899,2.,1.);
#3336=TOROIDAL_SURFACE('',#95901,66.5,1.);
#3337=TOROIDAL_SURFACE('',#95903,2.,1.);
#3338=TOROIDAL_SURFACE('',#95916,59.1370702608075,1.);
#3339=TOROIDAL_SURFACE('',#95957,59.1370702608075,1.);
#3340=TOROIDAL_SURFACE('',#95976,59.1370702608075,1.);
#3341=TOROIDAL_SURFACE('',#95979,59.1370702608075,1.);
#3342=TOROIDAL_SURFACE('',#95991,59.1370702608075,1.);
#3343=TOROIDAL_SURFACE('',#95998,59.1370702608075,1.);
#3344=TOROIDAL_SURFACE('',#96019,59.1370702608075,1.);
#3345=TOROIDAL_SURFACE('',#96027,59.1370702608075,1.);
#3346=TOROIDAL_SURFACE('',#96042,59.1370702608075,1.);
#3347=TOROIDAL_SURFACE('',#96046,59.1370702608075,1.);
#3348=TOROIDAL_SURFACE('',#96077,59.1370702608075,1.);
#3349=TOROIDAL_SURFACE('',#96148,59.1370702608075,1.);
#3350=TOROIDAL_SURFACE('',#96174,2.,1.);
#3351=TOROIDAL_SURFACE('',#96178,66.5,1.);
#3352=TOROIDAL_SURFACE('',#96182,2.,1.);
#3353=TOROIDAL_SURFACE('',#96206,59.,0.5);
#3354=TOROIDAL_SURFACE('',#96210,57.5,1.);
#3355=TOROIDAL_SURFACE('',#96216,59.,0.5);
#3356=TOROIDAL_SURFACE('',#96222,57.5,1.);
#3357=TOROIDAL_SURFACE('',#96231,57.5,1.);
#3358=TOROIDAL_SURFACE('',#96240,57.5,1.);
#3359=TOROIDAL_SURFACE('',#96249,57.5,1.);
#3360=TOROIDAL_SURFACE('',#96256,59.,0.5);
#3361=TOROIDAL_SURFACE('',#96260,57.5,1.);
#3362=TOROIDAL_SURFACE('',#96266,59.,0.5);
#3363=TOROIDAL_SURFACE('',#96287,2.,1.);
#3364=TOROIDAL_SURFACE('',#96291,66.5,1.);
#3365=TOROIDAL_SURFACE('',#96295,2.,1.);
#3366=TOROIDAL_SURFACE('',#96309,2.5,0.5);
#3367=TOROIDAL_SURFACE('',#96332,2.5,0.5);
#3368=TOROIDAL_SURFACE('',#96338,2.5,0.5);
#3369=TOROIDAL_SURFACE('',#96344,2.5,0.5);
#3370=TOROIDAL_SURFACE('',#96363,59.024570260837,1.);
#3371=TOROIDAL_SURFACE('',#96365,2.5,0.5);
#3372=TOROIDAL_SURFACE('',#96388,2.5,0.5);
#3373=TOROIDAL_SURFACE('',#96402,2.5,0.5);
#3374=TOROIDAL_SURFACE('',#96408,2.5,0.5);
#3375=TOROIDAL_SURFACE('',#96425,2.5,0.5);
#3376=TOROIDAL_SURFACE('',#96436,2.5,0.5);
#3377=TOROIDAL_SURFACE('',#96456,2.5,0.5);
#3378=TOROIDAL_SURFACE('',#96462,2.5,0.5);
#3379=TOROIDAL_SURFACE('',#96468,2.5,0.5);
#3380=TOROIDAL_SURFACE('',#96489,2.5,0.5);
#3381=TOROIDAL_SURFACE('',#96520,2.5,0.5);
#3382=TOROIDAL_SURFACE('',#96529,2.5,0.5);
#3383=TOROIDAL_SURFACE('',#96546,2.5,0.5);
#3384=TOROIDAL_SURFACE('',#96552,2.5,0.5);
#3385=TOROIDAL_SURFACE('',#96563,59.024570260837,1.);
#3386=TOROIDAL_SURFACE('',#96571,2.5,0.5);
#3387=TOROIDAL_SURFACE('',#96578,2.5,0.5);
#3388=TOROIDAL_SURFACE('',#96590,2.5,0.5);
#3389=TOROIDAL_SURFACE('',#96597,2.5,0.5);
#3390=TOROIDAL_SURFACE('',#96611,59.024570260837,1.);
#3391=TOROIDAL_SURFACE('',#96613,2.5,0.5);
#3392=TOROIDAL_SURFACE('',#96633,2.5,0.5);
#3393=TOROIDAL_SURFACE('',#96639,2.5,0.5);
#3394=TOROIDAL_SURFACE('',#96645,2.5,0.5);
#3395=TOROIDAL_SURFACE('',#96666,2.5,0.5);
#3396=TOROIDAL_SURFACE('',#96690,2.5,0.5);
#3397=TOROIDAL_SURFACE('',#96701,2.5,0.5);
#3398=TOROIDAL_SURFACE('',#96717,2.5,0.5);
#3399=TOROIDAL_SURFACE('',#96723,2.5,0.5);
#3400=TOROIDAL_SURFACE('',#96730,59.024570260837,1.);
#3401=TOROIDAL_SURFACE('',#96746,2.5,0.5);
#3402=TOROIDAL_SURFACE('',#96765,2.5,0.5);
#3403=TOROIDAL_SURFACE('',#96771,2.5,0.5);
#3404=TOROIDAL_SURFACE('',#96777,2.5,0.5);
#3405=TOROIDAL_SURFACE('',#96783,2.5,0.5);
#3406=TOROIDAL_SURFACE('',#96892,2.5,0.5);
#3407=TOROIDAL_SURFACE('',#96898,2.5,0.5);
#3408=TOROIDAL_SURFACE('',#96904,2.5,0.5);
#3409=TOROIDAL_SURFACE('',#96910,2.5,0.5);
#3410=TOROIDAL_SURFACE('',#96924,2.5,0.5);
#3411=TOROIDAL_SURFACE('',#96941,2.5,0.5);
#3412=TOROIDAL_SURFACE('',#96947,2.5,0.5);
#3413=TOROIDAL_SURFACE('',#96950,2.5,0.5);
#3414=TOROIDAL_SURFACE('',#96956,2.5,0.5);
#3415=TOROIDAL_SURFACE('',#96972,2.5,0.5);
#3416=TOROIDAL_SURFACE('',#96979,2.5,0.5);
#3417=TOROIDAL_SURFACE('',#96994,2.5,0.5);
#3418=TOROIDAL_SURFACE('',#97001,2.5,0.5);
#3419=TOROIDAL_SURFACE('',#97011,2.5,0.5);
#3420=TOROIDAL_SURFACE('',#97024,2.5,0.5);
#3421=TOROIDAL_SURFACE('',#97030,2.5,0.5);
#3422=TOROIDAL_SURFACE('',#97036,2.5,0.5);
#3423=TOROIDAL_SURFACE('',#97212,3.5,0.5);
#3424=TOROIDAL_SURFACE('',#97220,2.5,0.5);
#3425=TOROIDAL_SURFACE('',#97242,59.,0.5);
#3426=TOROIDAL_SURFACE('',#97277,59.024570260837,1.);
#3427=TOROIDAL_SURFACE('',#97286,59.024570260837,1.);
#3428=TOROIDAL_SURFACE('',#97323,59.024570260837,1.);
#3429=TOROIDAL_SURFACE('',#97447,59.024570260837,1.);
#3430=TOROIDAL_SURFACE('',#97490,59.,0.5);
#3431=TOROIDAL_SURFACE('',#97499,57.5,1.);
#3432=TOROIDAL_SURFACE('',#97508,57.5,1.);
#3433=TOROIDAL_SURFACE('',#97513,59.,0.5);
#3434=TOROIDAL_SURFACE('',#97518,57.5,1.);
#3435=TOROIDAL_SURFACE('',#97526,3.25,0.25);
#3436=TOROIDAL_SURFACE('',#97532,2.75,0.25);
#3437=TOROIDAL_SURFACE('',#97535,67.25,0.25);
#3438=TOROIDAL_SURFACE('',#97538,2.75,0.25);
#3439=TOROIDAL_SURFACE('',#97543,5.25,0.25);
#3440=TOROIDAL_SURFACE('',#97546,58.25,0.25);
#3441=TOROIDAL_SURFACE('',#97549,5.25,0.25);
#3442=TOROIDAL_SURFACE('',#97554,2.75,0.25);
#3443=TOROIDAL_SURFACE('',#97557,67.25,0.25);
#3444=TOROIDAL_SURFACE('',#97560,2.75,0.25);
#3445=TOROIDAL_SURFACE('',#97565,5.25,0.25);
#3446=TOROIDAL_SURFACE('',#97573,4.5,0.5);
#3447=TOROIDAL_SURFACE('',#97584,1.,0.5);
#3448=TOROIDAL_SURFACE('',#97589,1.,0.5);
#3449=TOROIDAL_SURFACE('',#97596,1.,0.5);
#3450=TOROIDAL_SURFACE('',#97601,1.,0.5);
#3451=TOROIDAL_SURFACE('',#97608,45.1752328136335,1.);
#3452=TOROIDAL_SURFACE('',#97612,1.,0.5);
#3453=TOROIDAL_SURFACE('',#97617,1.,0.5);
#3454=TOROIDAL_SURFACE('',#97621,45.1752328136335,1.);
#3455=TOROIDAL_SURFACE('',#97625,1.,0.5);
#3456=TOROIDAL_SURFACE('',#97630,1.,0.5);
#3457=TOROIDAL_SURFACE('',#97639,1.,0.5);
#3458=TOROIDAL_SURFACE('',#97753,57.3875000000282,1.);
#3459=TOROIDAL_SURFACE('',#97758,58.8875000000282,0.5);
#3460=TOROIDAL_SURFACE('',#97763,57.3875000000282,1.);
#3461=TOROIDAL_SURFACE('',#97772,57.3875000000282,1.);
#3462=TOROIDAL_SURFACE('',#97781,57.3875000000282,1.);
#3463=TOROIDAL_SURFACE('',#97790,57.3875000000282,1.);
#3464=TOROIDAL_SURFACE('',#97795,58.8875000000282,0.5);
#3465=TOROIDAL_SURFACE('',#97800,57.3875000000282,1.);
#3466=TOROIDAL_SURFACE('',#97806,2.,1.);
#3467=TOROIDAL_SURFACE('',#97811,2.,1.);
#3468=TOROIDAL_SURFACE('',#97817,4.5,0.5);
#3469=TOROIDAL_SURFACE('',#97826,4.5,0.5);
#3470=TOROIDAL_SURFACE('',#97836,57.3875000000282,1.);
#3471=TOROIDAL_SURFACE('',#97845,57.3875000000282,1.);
#3472=TOROIDAL_SURFACE('',#97850,58.8875000000282,0.5);
#3473=TOROIDAL_SURFACE('',#97855,57.3875000000282,1.);
#3474=TOROIDAL_SURFACE('',#97859,58.8875000000282,0.5);
#3475=TOROIDAL_SURFACE('',#97865,57.3875000000282,1.);
#3476=TOROIDAL_SURFACE('',#97870,58.8875000000282,0.5);
#3477=TOROIDAL_SURFACE('',#97875,57.3875000000282,1.);
#3478=TOROIDAL_SURFACE('',#97885,57.3875000000282,1.);
#3479=TOROIDAL_SURFACE('',#97894,2.,1.);
#3480=TOROIDAL_SURFACE('',#97899,2.,1.);
#3481=TOROIDAL_SURFACE('',#97905,2.5,0.5);
#3482=TOROIDAL_SURFACE('',#97917,58.25,0.25);
#3483=TOROIDAL_SURFACE('',#97921,58.25,0.25);
#3484=TOROIDAL_SURFACE('',#97925,59.,0.5);
#3485=TOROIDAL_SURFACE('',#97931,45.1752328136335,1.);
#3486=TOROIDAL_SURFACE('',#97935,57.3875000000282,1.);
#3487=TOROIDAL_SURFACE('',#97961,3.,0.25);
#3488=TOROIDAL_SURFACE('',#97983,4.01589928084081,0.5);
#3489=TOROIDAL_SURFACE('',#97995,2.,0.5);
#3490=TOROIDAL_SURFACE('',#98000,74.3,0.5);
#3491=TOROIDAL_SURFACE('',#98005,2.,0.5);
#3492=TOROIDAL_SURFACE('',#98027,2.,0.5);
#3493=TOROIDAL_SURFACE('',#98034,74.3,0.5);
#3494=TOROIDAL_SURFACE('',#98039,2.,0.5);
#3495=TOROIDAL_SURFACE('',#98042,12.0057534629026,0.5);
#3496=TOROIDAL_SURFACE('',#98047,77.6552534828746,0.5);
#3497=TOROIDAL_SURFACE('',#98051,12.0057534629026,0.5);
#3498=TOROIDAL_SURFACE('',#98055,1067.5427534629,0.5);
#3499=TOROIDAL_SURFACE('',#98059,12.0057534629025,0.5);
#3500=TOROIDAL_SURFACE('',#98063,77.6552534828746,0.5);
#3501=TOROIDAL_SURFACE('',#98067,12.0057534629026,0.5);
#3502=TOROIDAL_SURFACE('',#98090,77.6139048513169,0.5);
#3503=TOROIDAL_SURFACE('',#98095,77.6139048513167,0.5);
#3504=TOROIDAL_SURFACE('',#98115,73.05,0.75);
#3505=TOROIDAL_SURFACE('',#98129,76.3639048513167,0.75);
#3506=TOROIDAL_SURFACE('',#98142,76.3639048513169,0.75);
#3507=TOROIDAL_SURFACE('',#98155,73.05,0.75);
#3508=TOROIDAL_SURFACE('',#98171,1.2,0.45);
#3509=TOROIDAL_SURFACE('',#98178,204.945690815561,0.45);
#3510=TOROIDAL_SURFACE('',#98182,1.2,0.45);
#3511=TOROIDAL_SURFACE('',#98186,1.45,0.45);
#3512=TOROIDAL_SURFACE('',#98192,48.45,0.45);
#3513=TOROIDAL_SURFACE('',#98196,1.2,0.45);
#3514=TOROIDAL_SURFACE('',#98200,1.2,0.45);
#3515=TOROIDAL_SURFACE('',#98205,1.2,0.45);
#3516=TOROIDAL_SURFACE('',#98212,204.945690815561,0.45);
#3517=TOROIDAL_SURFACE('',#98216,1.2,0.45);
#3518=TOROIDAL_SURFACE('',#98220,1.2,0.45);
#3519=TOROIDAL_SURFACE('',#98228,1.2,0.45);
#3520=TOROIDAL_SURFACE('',#98231,1.2,0.45);
#3521=TOROIDAL_SURFACE('',#98238,204.945690815561,0.45);
#3522=TOROIDAL_SURFACE('',#98242,1.2,0.45);
#3523=TOROIDAL_SURFACE('',#98246,1.2,0.45);
#3524=TOROIDAL_SURFACE('',#98254,1.2,0.45);
#3525=TOROIDAL_SURFACE('',#98257,1.2,0.45);
#3526=TOROIDAL_SURFACE('',#98266,1.2,0.45);
#3527=TOROIDAL_SURFACE('',#98270,1.2,0.45);
#3528=TOROIDAL_SURFACE('',#98278,1.2,0.45);
#3529=TOROIDAL_SURFACE('',#98281,1.2,0.45);
#3530=TOROIDAL_SURFACE('',#98290,1.2,0.45);
#3531=TOROIDAL_SURFACE('',#98294,1.2,0.45);
#3532=TOROIDAL_SURFACE('',#98298,12.6555395526668,0.45);
#3533=TOROIDAL_SURFACE('',#98304,10.45,0.45);
#3534=TOROIDAL_SURFACE('',#98308,1.2,0.45);
#3535=TOROIDAL_SURFACE('',#98311,1.2,0.45);
#3536=TOROIDAL_SURFACE('',#98320,1.2,0.45);
#3537=TOROIDAL_SURFACE('',#98324,1.2,0.45);
#3538=TOROIDAL_SURFACE('',#98332,1.2,0.45);
#3539=TOROIDAL_SURFACE('',#98335,1.2,0.45);
#3540=TOROIDAL_SURFACE('',#98344,1.2,0.45);
#3541=TOROIDAL_SURFACE('',#98348,1.2,0.45);
#3542=TOROIDAL_SURFACE('',#98356,1.2,0.45);
#3543=TOROIDAL_SURFACE('',#98359,1.2,0.45);
#3544=TOROIDAL_SURFACE('',#98368,1.2,0.45);
#3545=TOROIDAL_SURFACE('',#98372,1.2,0.45);
#3546=TOROIDAL_SURFACE('',#98380,1.2,0.45);
#3547=TOROIDAL_SURFACE('',#98383,1.2,0.45);
#3548=TOROIDAL_SURFACE('',#98392,1.2,0.45);
#3549=TOROIDAL_SURFACE('',#98396,1.2,0.45);
#3550=TOROIDAL_SURFACE('',#98404,1.2,0.45);
#3551=TOROIDAL_SURFACE('',#98407,1.2,0.45);
#3552=TOROIDAL_SURFACE('',#98416,1.2,0.45);
#3553=TOROIDAL_SURFACE('',#98420,1.2,0.45);
#3554=TOROIDAL_SURFACE('',#98426,677.884816028482,0.45);
#3555=TOROIDAL_SURFACE('',#98430,1.2,0.45);
#3556=TOROIDAL_SURFACE('',#98433,1.2,0.45);
#3557=TOROIDAL_SURFACE('',#98442,1.2,0.45);
#3558=TOROIDAL_SURFACE('',#98446,1.2,0.45);
#3559=TOROIDAL_SURFACE('',#98452,48.45,0.45);
#3560=TOROIDAL_SURFACE('',#98456,1.2,0.45);
#3561=TOROIDAL_SURFACE('',#98460,1.45,0.45);
#3562=TOROIDAL_SURFACE('',#98464,677.884816028482,0.45);
#3563=TOROIDAL_SURFACE('',#98467,1.2,0.45);
#3564=TOROIDAL_SURFACE('',#98476,1.2,0.45);
#3565=TOROIDAL_SURFACE('',#98480,1.2,0.45);
#3566=TOROIDAL_SURFACE('',#98486,677.884816028482,0.45);
#3567=TOROIDAL_SURFACE('',#98490,1.2,0.45);
#3568=TOROIDAL_SURFACE('',#98493,1.2,0.45);
#3569=TOROIDAL_SURFACE('',#98502,1.2,0.45);
#3570=TOROIDAL_SURFACE('',#98506,1.2,0.45);
#3571=TOROIDAL_SURFACE('',#98514,1.2,0.45);
#3572=TOROIDAL_SURFACE('',#98517,1.2,0.45);
#3573=TOROIDAL_SURFACE('',#98524,11.6555395526668,0.45);
#3574=TOROIDAL_SURFACE('',#98528,1.2,0.45);
#3575=TOROIDAL_SURFACE('',#98532,10.45,0.45);
#3576=TOROIDAL_SURFACE('',#98540,1.2,0.45);
#3577=TOROIDAL_SURFACE('',#98544,1.2,0.45);
#3578=TOROIDAL_SURFACE('',#98549,1.2,0.45);
#3579=TOROIDAL_SURFACE('',#98558,1.2,0.45);
#3580=TOROIDAL_SURFACE('',#98562,10.45,0.45);
#3581=TOROIDAL_SURFACE('',#98568,11.6555395526668,0.45);
#3582=TOROIDAL_SURFACE('',#98572,1.2,0.45);
#3583=TOROIDAL_SURFACE('',#98576,1.2,0.45);
#3584=TOROIDAL_SURFACE('',#98581,1.2,0.45);
#3585=TOROIDAL_SURFACE('',#98590,1.2,0.45);
#3586=TOROIDAL_SURFACE('',#98594,1.2,0.45);
#3587=TOROIDAL_SURFACE('',#98602,1.2,0.45);
#3588=TOROIDAL_SURFACE('',#98605,1.2,0.45);
#3589=TOROIDAL_SURFACE('',#98614,1.2,0.45);
#3590=TOROIDAL_SURFACE('',#98618,1.2,0.45);
#3591=TOROIDAL_SURFACE('',#98622,677.884816028482,0.45);
#3592=TOROIDAL_SURFACE('',#98628,1.2,0.45);
#3593=TOROIDAL_SURFACE('',#98631,1.2,0.45);
#3594=TOROIDAL_SURFACE('',#98640,1.2,0.45);
#3595=TOROIDAL_SURFACE('',#98644,1.2,0.45);
#3596=TOROIDAL_SURFACE('',#98652,1.2,0.45);
#3597=TOROIDAL_SURFACE('',#98655,1.2,0.45);
#3598=TOROIDAL_SURFACE('',#98664,1.2,0.45);
#3599=TOROIDAL_SURFACE('',#98668,1.2,0.45);
#3600=TOROIDAL_SURFACE('',#98676,1.2,0.45);
#3601=TOROIDAL_SURFACE('',#98679,1.2,0.45);
#3602=TOROIDAL_SURFACE('',#98688,1.2,0.45);
#3603=TOROIDAL_SURFACE('',#98692,1.2,0.45);
#3604=TOROIDAL_SURFACE('',#98698,12.6555395526668,0.45);
#3605=TOROIDAL_SURFACE('',#98702,1.2,0.45);
#3606=TOROIDAL_SURFACE('',#98706,10.45,0.45);
#3607=TOROIDAL_SURFACE('',#98709,1.2,0.45);
#3608=TOROIDAL_SURFACE('',#98718,1.2,0.45);
#3609=TOROIDAL_SURFACE('',#98722,1.2,0.45);
#3610=TOROIDAL_SURFACE('',#98726,677.884816028482,0.45);
#3611=TOROIDAL_SURFACE('',#98732,1.2,0.45);
#3612=TOROIDAL_SURFACE('',#98735,1.2,0.45);
#3613=TOROIDAL_SURFACE('',#98744,1.2,0.45);
#3614=TOROIDAL_SURFACE('',#98748,1.2,0.45);
#3615=TOROIDAL_SURFACE('',#98752,48.45,0.45);
#3616=TOROIDAL_SURFACE('',#98758,1.45,0.45);
#3617=TOROIDAL_SURFACE('',#98762,1.2,0.45);
#3618=TOROIDAL_SURFACE('',#98766,677.884816028482,0.45);
#3619=TOROIDAL_SURFACE('',#98769,1.2,0.45);
#3620=TOROIDAL_SURFACE('',#98778,1.2,0.45);
#3621=TOROIDAL_SURFACE('',#98782,1.2,0.45);
#3622=TOROIDAL_SURFACE('',#98790,1.2,0.45);
#3623=TOROIDAL_SURFACE('',#98793,1.2,0.45);
#3624=TOROIDAL_SURFACE('',#98802,1.2,0.45);
#3625=TOROIDAL_SURFACE('',#98806,1.2,0.45);
#3626=TOROIDAL_SURFACE('',#98812,48.45,0.45);
#3627=TOROIDAL_SURFACE('',#98816,1.2,0.45);
#3628=TOROIDAL_SURFACE('',#98820,1.44999999999996,0.45);
#3629=TOROIDAL_SURFACE('',#98824,677.884816028482,0.45);
#3630=TOROIDAL_SURFACE('',#98827,1.2,0.45);
#3631=TOROIDAL_SURFACE('',#98836,1.2,0.45);
#3632=TOROIDAL_SURFACE('',#98840,1.2,0.45);
#3633=TOROIDAL_SURFACE('',#98846,677.884816028482,0.45);
#3634=TOROIDAL_SURFACE('',#98850,1.2,0.45);
#3635=TOROIDAL_SURFACE('',#98853,1.2,0.45);
#3636=TOROIDAL_SURFACE('',#98862,1.2,0.45);
#3637=TOROIDAL_SURFACE('',#98866,1.2,0.45);
#3638=TOROIDAL_SURFACE('',#98874,1.2,0.45);
#3639=TOROIDAL_SURFACE('',#98877,1.2,0.45);
#3640=TOROIDAL_SURFACE('',#98886,1.2,0.45);
#3641=TOROIDAL_SURFACE('',#98890,1.2,0.45);
#3642=TOROIDAL_SURFACE('',#98896,677.884816028482,0.45);
#3643=TOROIDAL_SURFACE('',#98900,1.2,0.45);
#3644=TOROIDAL_SURFACE('',#98903,1.2,0.45);
#3645=TOROIDAL_SURFACE('',#98912,1.2,0.45);
#3646=TOROIDAL_SURFACE('',#98916,1.2,0.45);
#3647=TOROIDAL_SURFACE('',#98924,1.2,0.45);
#3648=TOROIDAL_SURFACE('',#98927,1.2,0.45);
#3649=TOROIDAL_SURFACE('',#98934,48.45,0.45);
#3650=TOROIDAL_SURFACE('',#98938,1.2,0.45);
#3651=TOROIDAL_SURFACE('',#98942,1.2,0.45);
#3652=TOROIDAL_SURFACE('',#98947,1.2,0.45);
#3653=TOROIDAL_SURFACE('',#98954,48.45,0.45);
#3654=TOROIDAL_SURFACE('',#98958,1.2,0.45);
#3655=TOROIDAL_SURFACE('',#98962,1.2,0.45);
#3656=TOROIDAL_SURFACE('',#98967,6.44999999999992,0.45);
#3657=TOROIDAL_SURFACE('',#98972,53.45,0.45);
#3658=TOROIDAL_SURFACE('',#98976,6.45,0.45);
#3659=TOROIDAL_SURFACE('',#98980,682.884816028482,0.45);
#3660=TOROIDAL_SURFACE('',#98984,6.45,0.45);
#3661=TOROIDAL_SURFACE('',#98988,53.45,0.45);
#3662=TOROIDAL_SURFACE('',#98992,6.45,0.45);
#3663=TOROIDAL_SURFACE('',#98996,4.34999999999995,0.45);
#3664=TOROIDAL_SURFACE('',#99001,51.35,0.45);
#3665=TOROIDAL_SURFACE('',#99005,4.35,0.45);
#3666=TOROIDAL_SURFACE('',#99009,680.784816028482,0.45);
#3667=TOROIDAL_SURFACE('',#99013,4.35,0.45);
#3668=TOROIDAL_SURFACE('',#99017,51.35,0.45);
#3669=TOROIDAL_SURFACE('',#99021,4.35,0.45);
#3670=TOROIDAL_SURFACE('',#99025,1.2,0.45);
#3671=TOROIDAL_SURFACE('',#99031,1.2,0.45);
#3672=TOROIDAL_SURFACE('',#99035,11.5555395526669,0.45);
#3673=TOROIDAL_SURFACE('',#99039,1.2,0.45);
#3674=TOROIDAL_SURFACE('',#99045,1.2,0.45);
#3675=TOROIDAL_SURFACE('',#99048,1.2,0.45);
#3676=TOROIDAL_SURFACE('',#99054,1.2,0.45);
#3677=TOROIDAL_SURFACE('',#99058,11.5555395526669,0.45);
#3678=TOROIDAL_SURFACE('',#99062,1.2,0.45);
#3679=TOROIDAL_SURFACE('',#99068,1.2,0.45);
#3680=TOROIDAL_SURFACE('',#99071,1.2,0.45);
#3681=TOROIDAL_SURFACE('',#99077,1.2,0.45);
#3682=TOROIDAL_SURFACE('',#99081,11.5555395526669,0.45);
#3683=TOROIDAL_SURFACE('',#99085,1.2,0.45);
#3684=TOROIDAL_SURFACE('',#99091,1.2,0.45);
#3685=TOROIDAL_SURFACE('',#99094,1.2,0.45);
#3686=TOROIDAL_SURFACE('',#99100,1.2,0.45);
#3687=TOROIDAL_SURFACE('',#99104,11.5555395526669,0.45);
#3688=TOROIDAL_SURFACE('',#99108,1.2,0.45);
#3689=TOROIDAL_SURFACE('',#99114,1.2,0.45);
#3690=TOROIDAL_SURFACE('',#99117,12.5403589366713,1.5);
#3691=TOROIDAL_SURFACE('',#99122,78.1898589566432,1.5);
#3692=TOROIDAL_SURFACE('',#99126,12.5403589366712,1.5);
#3693=TOROIDAL_SURFACE('',#99130,1068.07735893667,1.5);
#3694=TOROIDAL_SURFACE('',#99134,12.5403589366712,1.5);
#3695=TOROIDAL_SURFACE('',#99138,78.1898589566432,1.5);
#3696=TOROIDAL_SURFACE('',#99142,12.5403589366713,1.5);
#3697=TOROIDAL_SURFACE('',#99205,17.1605488438955,4.99999999963848);
#3698=TOROIDAL_SURFACE('',#99881,4.01589928084003,0.5);
#3699=TOROIDAL_SURFACE('',#99885,4.01589928084081,0.5);
#3700=TOROIDAL_SURFACE('',#99897,2.,0.5);
#3701=TOROIDAL_SURFACE('',#99902,74.3,0.5);
#3702=TOROIDAL_SURFACE('',#99907,2.,0.5);
#3703=TOROIDAL_SURFACE('',#99929,2.,0.5);
#3704=TOROIDAL_SURFACE('',#99936,74.3,0.5);
#3705=TOROIDAL_SURFACE('',#99941,2.,0.5);
#3706=TOROIDAL_SURFACE('',#99944,232.542753462903,0.5);
#3707=TOROIDAL_SURFACE('',#99948,12.0057534629026,0.5);
#3708=TOROIDAL_SURFACE('',#99952,77.6552534828746,0.5);
#3709=TOROIDAL_SURFACE('',#99956,12.0057534629026,0.5);
#3710=TOROIDAL_SURFACE('',#99960,1067.5427534629,0.5);
#3711=TOROIDAL_SURFACE('',#99964,12.0057534629025,0.5);
#3712=TOROIDAL_SURFACE('',#99968,77.6552534828746,0.5);
#3713=TOROIDAL_SURFACE('',#99972,12.0057534629026,0.5);
#3714=TOROIDAL_SURFACE('',#99976,1067.5427534629,0.5);
#3715=TOROIDAL_SURFACE('',#99998,77.6139048513169,0.5);
#3716=TOROIDAL_SURFACE('',#100003,77.6139048513167,0.5);
#3717=TOROIDAL_SURFACE('',#100023,73.05,0.75);
#3718=TOROIDAL_SURFACE('',#100037,76.3639048513167,0.75);
#3719=TOROIDAL_SURFACE('',#100050,76.3639048513169,0.75);
#3720=TOROIDAL_SURFACE('',#100063,73.05,0.75);
#3721=TOROIDAL_SURFACE('',#100079,1.2,0.45);
#3722=TOROIDAL_SURFACE('',#100086,204.945690815561,0.45);
#3723=TOROIDAL_SURFACE('',#100090,1.2,0.45);
#3724=TOROIDAL_SURFACE('',#100094,1.45,0.45);
#3725=TOROIDAL_SURFACE('',#100100,48.45,0.45);
#3726=TOROIDAL_SURFACE('',#100104,1.2,0.45);
#3727=TOROIDAL_SURFACE('',#100108,1.2,0.45);
#3728=TOROIDAL_SURFACE('',#100113,1.2,0.45);
#3729=TOROIDAL_SURFACE('',#100120,204.945690815561,0.45);
#3730=TOROIDAL_SURFACE('',#100124,1.2,0.45);
#3731=TOROIDAL_SURFACE('',#100128,1.2,0.45);
#3732=TOROIDAL_SURFACE('',#100136,1.2,0.45);
#3733=TOROIDAL_SURFACE('',#100139,1.2,0.45);
#3734=TOROIDAL_SURFACE('',#100146,204.945690815561,0.45);
#3735=TOROIDAL_SURFACE('',#100150,1.2,0.45);
#3736=TOROIDAL_SURFACE('',#100154,1.2,0.45);
#3737=TOROIDAL_SURFACE('',#100162,1.2,0.45);
#3738=TOROIDAL_SURFACE('',#100165,1.2,0.45);
#3739=TOROIDAL_SURFACE('',#100174,1.2,0.45);
#3740=TOROIDAL_SURFACE('',#100178,1.2,0.45);
#3741=TOROIDAL_SURFACE('',#100186,1.2,0.45);
#3742=TOROIDAL_SURFACE('',#100189,1.2,0.45);
#3743=TOROIDAL_SURFACE('',#100198,1.2,0.45);
#3744=TOROIDAL_SURFACE('',#100202,1.2,0.45);
#3745=TOROIDAL_SURFACE('',#100206,12.6555395526668,0.45);
#3746=TOROIDAL_SURFACE('',#100212,10.45,0.45);
#3747=TOROIDAL_SURFACE('',#100216,1.2,0.45);
#3748=TOROIDAL_SURFACE('',#100219,1.2,0.45);
#3749=TOROIDAL_SURFACE('',#100228,1.2,0.45);
#3750=TOROIDAL_SURFACE('',#100232,1.2,0.45);
#3751=TOROIDAL_SURFACE('',#100240,1.2,0.45);
#3752=TOROIDAL_SURFACE('',#100243,1.2,0.45);
#3753=TOROIDAL_SURFACE('',#100252,1.2,0.45);
#3754=TOROIDAL_SURFACE('',#100256,1.2,0.45);
#3755=TOROIDAL_SURFACE('',#100264,1.2,0.45);
#3756=TOROIDAL_SURFACE('',#100267,1.2,0.45);
#3757=TOROIDAL_SURFACE('',#100276,1.2,0.45);
#3758=TOROIDAL_SURFACE('',#100280,1.2,0.45);
#3759=TOROIDAL_SURFACE('',#100288,1.2,0.45);
#3760=TOROIDAL_SURFACE('',#100291,1.2,0.45);
#3761=TOROIDAL_SURFACE('',#100300,1.2,0.45);
#3762=TOROIDAL_SURFACE('',#100304,1.2,0.45);
#3763=TOROIDAL_SURFACE('',#100312,1.2,0.45);
#3764=TOROIDAL_SURFACE('',#100315,1.2,0.45);
#3765=TOROIDAL_SURFACE('',#100324,1.2,0.45);
#3766=TOROIDAL_SURFACE('',#100328,1.2,0.45);
#3767=TOROIDAL_SURFACE('',#100334,677.884816028482,0.45);
#3768=TOROIDAL_SURFACE('',#100338,1.2,0.45);
#3769=TOROIDAL_SURFACE('',#100341,1.2,0.45);
#3770=TOROIDAL_SURFACE('',#100350,1.2,0.45);
#3771=TOROIDAL_SURFACE('',#100354,1.2,0.45);
#3772=TOROIDAL_SURFACE('',#100360,48.45,0.45);
#3773=TOROIDAL_SURFACE('',#100364,1.2,0.45);
#3774=TOROIDAL_SURFACE('',#100368,1.45,0.45);
#3775=TOROIDAL_SURFACE('',#100372,677.884816028482,0.45);
#3776=TOROIDAL_SURFACE('',#100375,1.2,0.45);
#3777=TOROIDAL_SURFACE('',#100384,1.2,0.45);
#3778=TOROIDAL_SURFACE('',#100388,1.2,0.45);
#3779=TOROIDAL_SURFACE('',#100394,677.884816028482,0.45);
#3780=TOROIDAL_SURFACE('',#100398,1.2,0.45);
#3781=TOROIDAL_SURFACE('',#100401,1.2,0.45);
#3782=TOROIDAL_SURFACE('',#100410,1.2,0.45);
#3783=TOROIDAL_SURFACE('',#100414,1.2,0.45);
#3784=TOROIDAL_SURFACE('',#100422,1.2,0.45);
#3785=TOROIDAL_SURFACE('',#100425,1.2,0.45);
#3786=TOROIDAL_SURFACE('',#100432,11.6555395526668,0.45);
#3787=TOROIDAL_SURFACE('',#100436,1.2,0.45);
#3788=TOROIDAL_SURFACE('',#100440,10.45,0.45);
#3789=TOROIDAL_SURFACE('',#100448,1.2,0.45);
#3790=TOROIDAL_SURFACE('',#100452,1.2,0.45);
#3791=TOROIDAL_SURFACE('',#100457,1.2,0.45);
#3792=TOROIDAL_SURFACE('',#100466,1.2,0.45);
#3793=TOROIDAL_SURFACE('',#100470,10.45,0.45);
#3794=TOROIDAL_SURFACE('',#100476,11.6555395526668,0.45);
#3795=TOROIDAL_SURFACE('',#100480,1.2,0.45);
#3796=TOROIDAL_SURFACE('',#100484,1.2,0.45);
#3797=TOROIDAL_SURFACE('',#100489,1.2,0.45);
#3798=TOROIDAL_SURFACE('',#100498,1.2,0.45);
#3799=TOROIDAL_SURFACE('',#100502,1.2,0.45);
#3800=TOROIDAL_SURFACE('',#100510,1.2,0.45);
#3801=TOROIDAL_SURFACE('',#100513,1.2,0.45);
#3802=TOROIDAL_SURFACE('',#100522,1.2,0.45);
#3803=TOROIDAL_SURFACE('',#100526,1.2,0.45);
#3804=TOROIDAL_SURFACE('',#100530,677.884816028482,0.45);
#3805=TOROIDAL_SURFACE('',#100536,1.2,0.45);
#3806=TOROIDAL_SURFACE('',#100539,1.2,0.45);
#3807=TOROIDAL_SURFACE('',#100548,1.2,0.45);
#3808=TOROIDAL_SURFACE('',#100552,1.2,0.45);
#3809=TOROIDAL_SURFACE('',#100560,1.2,0.45);
#3810=TOROIDAL_SURFACE('',#100563,1.2,0.45);
#3811=TOROIDAL_SURFACE('',#100572,1.2,0.45);
#3812=TOROIDAL_SURFACE('',#100576,1.2,0.45);
#3813=TOROIDAL_SURFACE('',#100584,1.2,0.45);
#3814=TOROIDAL_SURFACE('',#100587,1.2,0.45);
#3815=TOROIDAL_SURFACE('',#100596,1.2,0.45);
#3816=TOROIDAL_SURFACE('',#100600,1.2,0.45);
#3817=TOROIDAL_SURFACE('',#100606,12.6555395526668,0.45);
#3818=TOROIDAL_SURFACE('',#100610,1.2,0.45);
#3819=TOROIDAL_SURFACE('',#100614,10.45,0.45);
#3820=TOROIDAL_SURFACE('',#100617,1.2,0.45);
#3821=TOROIDAL_SURFACE('',#100626,1.2,0.45);
#3822=TOROIDAL_SURFACE('',#100630,1.2,0.45);
#3823=TOROIDAL_SURFACE('',#100634,677.884816028482,0.45);
#3824=TOROIDAL_SURFACE('',#100640,1.2,0.45);
#3825=TOROIDAL_SURFACE('',#100643,1.2,0.45);
#3826=TOROIDAL_SURFACE('',#100652,1.2,0.45);
#3827=TOROIDAL_SURFACE('',#100656,1.2,0.45);
#3828=TOROIDAL_SURFACE('',#100660,48.45,0.45);
#3829=TOROIDAL_SURFACE('',#100666,1.45,0.45);
#3830=TOROIDAL_SURFACE('',#100670,1.2,0.45);
#3831=TOROIDAL_SURFACE('',#100674,677.884816028482,0.45);
#3832=TOROIDAL_SURFACE('',#100677,1.2,0.45);
#3833=TOROIDAL_SURFACE('',#100686,1.2,0.45);
#3834=TOROIDAL_SURFACE('',#100690,1.2,0.45);
#3835=TOROIDAL_SURFACE('',#100698,1.2,0.45);
#3836=TOROIDAL_SURFACE('',#100701,1.2,0.45);
#3837=TOROIDAL_SURFACE('',#100710,1.2,0.45);
#3838=TOROIDAL_SURFACE('',#100714,1.2,0.45);
#3839=TOROIDAL_SURFACE('',#100720,48.45,0.45);
#3840=TOROIDAL_SURFACE('',#100724,1.2,0.45);
#3841=TOROIDAL_SURFACE('',#100728,1.44999999999996,0.45);
#3842=TOROIDAL_SURFACE('',#100732,677.884816028482,0.45);
#3843=TOROIDAL_SURFACE('',#100735,1.2,0.45);
#3844=TOROIDAL_SURFACE('',#100744,1.2,0.45);
#3845=TOROIDAL_SURFACE('',#100748,1.2,0.45);
#3846=TOROIDAL_SURFACE('',#100754,677.884816028482,0.45);
#3847=TOROIDAL_SURFACE('',#100758,1.2,0.45);
#3848=TOROIDAL_SURFACE('',#100761,1.2,0.45);
#3849=TOROIDAL_SURFACE('',#100770,1.2,0.45);
#3850=TOROIDAL_SURFACE('',#100774,1.2,0.45);
#3851=TOROIDAL_SURFACE('',#100782,1.2,0.45);
#3852=TOROIDAL_SURFACE('',#100785,1.2,0.45);
#3853=TOROIDAL_SURFACE('',#100794,1.2,0.45);
#3854=TOROIDAL_SURFACE('',#100798,1.2,0.45);
#3855=TOROIDAL_SURFACE('',#100804,677.884816028482,0.45);
#3856=TOROIDAL_SURFACE('',#100808,1.2,0.45);
#3857=TOROIDAL_SURFACE('',#100811,1.2,0.45);
#3858=TOROIDAL_SURFACE('',#100820,1.2,0.45);
#3859=TOROIDAL_SURFACE('',#100824,1.2,0.45);
#3860=TOROIDAL_SURFACE('',#100832,1.2,0.45);
#3861=TOROIDAL_SURFACE('',#100835,1.2,0.45);
#3862=TOROIDAL_SURFACE('',#100842,48.45,0.45);
#3863=TOROIDAL_SURFACE('',#100846,1.2,0.45);
#3864=TOROIDAL_SURFACE('',#100850,1.2,0.45);
#3865=TOROIDAL_SURFACE('',#100855,1.2,0.45);
#3866=TOROIDAL_SURFACE('',#100862,48.45,0.45);
#3867=TOROIDAL_SURFACE('',#100866,1.2,0.45);
#3868=TOROIDAL_SURFACE('',#100870,1.2,0.45);
#3869=TOROIDAL_SURFACE('',#100875,7.65553955266686,0.45);
#3870=TOROIDAL_SURFACE('',#100879,5.07535,0.45);
#3871=TOROIDAL_SURFACE('',#100883,682.884816028482,0.45);
#3872=TOROIDAL_SURFACE('',#100887,6.44999999999992,0.45);
#3873=TOROIDAL_SURFACE('',#100891,53.45,0.45);
#3874=TOROIDAL_SURFACE('',#100895,6.45,0.45);
#3875=TOROIDAL_SURFACE('',#100899,682.884816028482,0.45);
#3876=TOROIDAL_SURFACE('',#100903,6.45,0.45);
#3877=TOROIDAL_SURFACE('',#100907,53.45,0.45);
#3878=TOROIDAL_SURFACE('',#100911,6.45,0.45);
#3879=TOROIDAL_SURFACE('',#100915,209.945690815561,0.45);
#3880=TOROIDAL_SURFACE('',#100918,680.784816028482,0.45);
#3881=TOROIDAL_SURFACE('',#100922,4.34999999999995,0.45);
#3882=TOROIDAL_SURFACE('',#100926,51.35,0.45);
#3883=TOROIDAL_SURFACE('',#100930,4.35,0.45);
#3884=TOROIDAL_SURFACE('',#100934,680.784816028482,0.45);
#3885=TOROIDAL_SURFACE('',#100938,4.35,0.45);
#3886=TOROIDAL_SURFACE('',#100942,51.35,0.45);
#3887=TOROIDAL_SURFACE('',#100946,4.35,0.45);
#3888=TOROIDAL_SURFACE('',#100950,207.845690815561,0.45);
#3889=TOROIDAL_SURFACE('',#100953,1.2,0.45);
#3890=TOROIDAL_SURFACE('',#100959,1.2,0.45);
#3891=TOROIDAL_SURFACE('',#100963,11.5555395526669,0.45);
#3892=TOROIDAL_SURFACE('',#100967,1.2,0.45);
#3893=TOROIDAL_SURFACE('',#100973,1.2,0.45);
#3894=TOROIDAL_SURFACE('',#100976,1.2,0.45);
#3895=TOROIDAL_SURFACE('',#100982,1.2,0.45);
#3896=TOROIDAL_SURFACE('',#100986,11.5555395526669,0.45);
#3897=TOROIDAL_SURFACE('',#100990,1.2,0.45);
#3898=TOROIDAL_SURFACE('',#100996,1.2,0.45);
#3899=TOROIDAL_SURFACE('',#100999,1.2,0.45);
#3900=TOROIDAL_SURFACE('',#101005,1.2,0.45);
#3901=TOROIDAL_SURFACE('',#101009,11.5555395526669,0.45);
#3902=TOROIDAL_SURFACE('',#101013,1.2,0.45);
#3903=TOROIDAL_SURFACE('',#101019,1.2,0.45);
#3904=TOROIDAL_SURFACE('',#101022,1.2,0.45);
#3905=TOROIDAL_SURFACE('',#101028,1.2,0.45);
#3906=TOROIDAL_SURFACE('',#101032,11.5555395526669,0.45);
#3907=TOROIDAL_SURFACE('',#101036,1.2,0.45);
#3908=TOROIDAL_SURFACE('',#101042,1.2,0.45);
#3909=TOROIDAL_SURFACE('',#101045,233.077358936672,1.5);
#3910=TOROIDAL_SURFACE('',#101049,12.5403589366713,1.5);
#3911=TOROIDAL_SURFACE('',#101053,78.1898589566432,1.5);
#3912=TOROIDAL_SURFACE('',#101057,12.5403589366712,1.5);
#3913=TOROIDAL_SURFACE('',#101061,1068.07735893667,1.5);
#3914=TOROIDAL_SURFACE('',#101065,12.5403589366712,1.5);
#3915=TOROIDAL_SURFACE('',#101069,78.1898589566432,1.5);
#3916=TOROIDAL_SURFACE('',#101073,12.5403589366713,1.5);
#3917=TOROIDAL_SURFACE('',#101077,1068.07735893667,1.5);
#3918=TOROIDAL_SURFACE('',#101141,17.1621953438396,5.00000000078575);
#3919=TOROIDAL_SURFACE('',#101878,4.01589928084003,0.5);
#3920=TOROIDAL_SURFACE('',#101898,3.,0.25);
#3921=TOROIDAL_SURFACE('',#101990,3.,0.25);
#3922=TOROIDAL_SURFACE('',#102003,8.55,0.25);
#3923=TOROIDAL_SURFACE('',#102007,8.55,0.25);
#3924=TOROIDAL_SURFACE('',#102036,6.5,0.5);
#3925=TOROIDAL_SURFACE('',#102045,6.5,0.5);
#3926=TOROIDAL_SURFACE('',#102049,6.5,0.5);
#3927=TOROIDAL_SURFACE('',#102057,6.5,0.5);
#3928=TOROIDAL_SURFACE('',#102068,5.,1.);
#3929=TOROIDAL_SURFACE('',#102075,5.,1.);
#3930=TOROIDAL_SURFACE('',#102081,3.,1.);
#3931=TOROIDAL_SURFACE('',#102085,3.,1.);
#3932=TOROIDAL_SURFACE('',#102098,3.,1.);
#3933=TOROIDAL_SURFACE('',#102101,3.,1.);
#3934=TOROIDAL_SURFACE('',#102107,5.,1.);
#3935=TOROIDAL_SURFACE('',#102113,5.,1.);
#3936=TOROIDAL_SURFACE('',#102141,8.55,0.25);
#3937=TOROIDAL_SURFACE('',#102145,8.55,0.25);
#3938=TOROIDAL_SURFACE('',#102165,1.,0.5);
#3939=TOROIDAL_SURFACE('',#102171,1.,0.5);
#3940=TOROIDAL_SURFACE('',#102179,1.,0.5);
#3941=TOROIDAL_SURFACE('',#102185,1.,0.5);
#3942=TOROIDAL_SURFACE('',#102193,2.5,0.5);
#3943=TOROIDAL_SURFACE('',#102199,1.,0.5);
#3944=TOROIDAL_SURFACE('',#102205,1.,0.5);
#3945=TOROIDAL_SURFACE('',#102211,2.5,0.5);
#3946=TOROIDAL_SURFACE('',#102220,2.5,0.5);
#3947=TOROIDAL_SURFACE('',#102226,1.,0.5);
#3948=TOROIDAL_SURFACE('',#102234,2.5,0.5);
#3949=TOROIDAL_SURFACE('',#102240,1.,0.5);
#3950=TOROIDAL_SURFACE('',#102244,5.5,0.5);
#3951=TOROIDAL_SURFACE('',#102250,1.,0.5);
#3952=TOROIDAL_SURFACE('',#102256,2.5,0.5);
#3953=TOROIDAL_SURFACE('',#102265,2.5,0.5);
#3954=TOROIDAL_SURFACE('',#102271,1.,0.5);
#3955=TOROIDAL_SURFACE('',#102275,58.,0.5);
#3956=TOROIDAL_SURFACE('',#102279,1.,0.5);
#3957=TOROIDAL_SURFACE('',#102285,2.5,0.5);
#3958=TOROIDAL_SURFACE('',#102294,2.5,0.5);
#3959=TOROIDAL_SURFACE('',#102300,1.,0.5);
#3960=TOROIDAL_SURFACE('',#102304,58.,0.5);
#3961=TOROIDAL_SURFACE('',#102308,1.,0.5);
#3962=TOROIDAL_SURFACE('',#102314,2.5,0.5);
#3963=TOROIDAL_SURFACE('',#102323,2.5,0.5);
#3964=TOROIDAL_SURFACE('',#102329,1.,0.5);
#3965=TOROIDAL_SURFACE('',#102333,58.,0.5);
#3966=TOROIDAL_SURFACE('',#102337,1.,0.5);
#3967=TOROIDAL_SURFACE('',#102343,2.5,0.5);
#3968=TOROIDAL_SURFACE('',#102352,2.5,0.5);
#3969=TOROIDAL_SURFACE('',#102358,1.,0.5);
#3970=TOROIDAL_SURFACE('',#102362,58.,0.5);
#3971=TOROIDAL_SURFACE('',#102366,1.,0.5);
#3972=TOROIDAL_SURFACE('',#102372,2.5,0.5);
#3973=TOROIDAL_SURFACE('',#102381,2.5,0.5);
#3974=TOROIDAL_SURFACE('',#102387,1.,0.5);
#3975=TOROIDAL_SURFACE('',#102391,58.,0.5);
#3976=TOROIDAL_SURFACE('',#102395,1.,0.5);
#3977=TOROIDAL_SURFACE('',#102401,2.5,0.5);
#3978=TOROIDAL_SURFACE('',#102410,2.5,0.5);
#3979=TOROIDAL_SURFACE('',#102416,1.,0.5);
#3980=TOROIDAL_SURFACE('',#102420,58.,0.5);
#3981=TOROIDAL_SURFACE('',#102424,1.,0.5);
#3982=TOROIDAL_SURFACE('',#102430,2.5,0.5);
#3983=TOROIDAL_SURFACE('',#102439,2.5,0.5);
#3984=TOROIDAL_SURFACE('',#102445,1.,0.5);
#3985=TOROIDAL_SURFACE('',#102451,5.5,0.5);
#3986=TOROIDAL_SURFACE('',#102455,1.,0.5);
#3987=TOROIDAL_SURFACE('',#102461,2.5,0.5);
#3988=TOROIDAL_SURFACE('',#102470,2.5,0.5);
#3989=TOROIDAL_SURFACE('',#102476,1.,0.5);
#3990=TOROIDAL_SURFACE('',#102482,1.,0.5);
#3991=TOROIDAL_SURFACE('',#102488,2.5,0.5);
#3992=TOROIDAL_SURFACE('',#102496,1.,0.5);
#3993=TOROIDAL_SURFACE('',#102502,2.5,0.5);
#3994=TOROIDAL_SURFACE('',#102728,3.,0.25);
#3995=TOROIDAL_SURFACE('',#102752,1.75,0.75);
#3996=TOROIDAL_SURFACE('',#102759,493.060657452016,0.75);
#3997=TOROIDAL_SURFACE('',#102761,493.060657452016,0.75);
#3998=TOROIDAL_SURFACE('',#102767,1.75,0.75);
#3999=TOROIDAL_SURFACE('',#102770,1.75,0.75);
#4000=TOROIDAL_SURFACE('',#102773,1.75,0.75);
#4001=TOROIDAL_SURFACE('',#102799,1.75,0.75);
#4002=TOROIDAL_SURFACE('',#102806,493.060657452016,0.75);
#4003=TOROIDAL_SURFACE('',#102808,493.060657452016,0.75);
#4004=TOROIDAL_SURFACE('',#102814,1.75,0.75);
#4005=TOROIDAL_SURFACE('',#102817,1.75,0.75);
#4006=TOROIDAL_SURFACE('',#102820,1.75,0.75);
#4007=TOROIDAL_SURFACE('',#102838,6.25,0.75);
#4008=TOROIDAL_SURFACE('',#102845,6.25,0.75);
#4009=TOROIDAL_SURFACE('',#102863,6.25,0.75);
#4010=TOROIDAL_SURFACE('',#102870,6.25,0.75);
#4011=TOROIDAL_SURFACE('',#103086,6.75,0.25);
#4012=TOROIDAL_SURFACE('',#103090,5.89644660940673,0.25);
#4013=TOROIDAL_SURFACE('',#103095,6.75,0.25);
#4014=TOROIDAL_SURFACE('',#103212,66.,1.5);
#4015=TOROIDAL_SURFACE('',#103214,66.,1.5);
#4016=TOROIDAL_SURFACE('',#103267,56.8875000000281,1.5);
#4017=TOROIDAL_SURFACE('',#103269,54.8875000000282,1.);
#4018=TOROIDAL_SURFACE('',#103272,55.3875000000282,1.5);
#4019=TOROIDAL_SURFACE('',#103274,56.8875000000281,1.5);
#4020=TOROIDAL_SURFACE('',#103276,56.8875000000281,1.5);
#4021=TOROIDAL_SURFACE('',#103278,66.,1.5);
#4022=TOROIDAL_SURFACE('',#103280,66.,1.5);
#4023=TOROIDAL_SURFACE('',#103287,56.8875000000281,1.5);
#4127=B_SPLINE_CURVE_WITH_KNOTS('',3,(#131356,#131357,#131358,#131359,#131360,
#131361,#131362),.UNSPECIFIED.,.F.,.F.,(4,3,4),(0.,0.00021456400433525,
0.000397824826383788),.UNSPECIFIED.);
#4128=B_SPLINE_CURVE_WITH_KNOTS('',3,(#131365,#131366,#131367,#131368),
 .UNSPECIFIED.,.F.,.F.,(4,4),(0.,1.),.UNSPECIFIED.);
#4129=B_SPLINE_CURVE_WITH_KNOTS('',3,(#131379,#131380,#131381,#131382),
 .UNSPECIFIED.,.F.,.F.,(4,4),(0.,1.),.UNSPECIFIED.);
#4130=B_SPLINE_CURVE_WITH_KNOTS('',3,(#131403,#131404,#131405,#131406,#131407,
#131408,#131409,#131410,#131411,#131412),.UNSPECIFIED.,.F.,.F.,(4,3,3,4),
(0.,0.360016030384402,0.739381400890229,1.),.UNSPECIFIED.);
#4131=B_SPLINE_CURVE_WITH_KNOTS('',3,(#131429,#131430,#131431,#131432,#131433,
#131434,#131435),.UNSPECIFIED.,.F.,.F.,(4,3,4),(1.57079632679491,2.35619449019235,
3.14159265358979),.UNSPECIFIED.);
#4132=B_SPLINE_CURVE_WITH_KNOTS('',3,(#131439,#131440,#131441,#131442,#131443,
#131444,#131445),.UNSPECIFIED.,.F.,.F.,(4,3,4),(-1.77635683940025E-15,0.785398163397447,
1.57079632679489),.UNSPECIFIED.);
#4133=B_SPLINE_CURVE_WITH_KNOTS('',3,(#131451,#131452,#131453,#131454,#131455,
#131456,#131457,#131458,#131459,#131460,#131461,#131462,#131463,#131464,
#131465,#131466,#131467,#131468,#131469),.UNSPECIFIED.,.F.,.F.,(4,3,3,3,
3,3,4),(0.00047266192456923,0.000857724029065683,0.00153872216954601,0.0018499707510604,
0.00201291034255504,0.00292749448068747,0.00355315876054085),
 .UNSPECIFIED.);
#4134=B_SPLINE_CURVE_WITH_KNOTS('',3,(#131472,#131473,#131474,#131475,#131476,
#131477,#131478,#131479,#131480,#131481,#131482,#131483,#131484,#131485,
#131486,#131487,#131488,#131489,#131490,#131491,#131492,#131493,#131494,
#131495,#131496,#131497,#131498,#131499,#131500,#131501,#131502,#131503,
#131504,#131505,#131506,#131507,#131508),.UNSPECIFIED.,.F.,.F.,(4,3,3,3,
3,3,3,3,3,3,3,3,4),(1.96820403583049,2.07447029970642,2.18239924823465,
2.29295513021916,2.40448289443547,2.51591247508908,2.55489944283297,2.66627384567102,
2.77787483330248,2.88775468513439,2.99605880939301,3.10223763839193,3.14159265358979),
 .UNSPECIFIED.);
#4135=B_SPLINE_CURVE_WITH_KNOTS('',3,(#131515,#131516,#131517,#131518,#131519,
#131520,#131521),.UNSPECIFIED.,.F.,.F.,(4,3,4),(4.7123889803847,5.49778714378215,
6.28318530717959),.UNSPECIFIED.);
#4136=B_SPLINE_CURVE_WITH_KNOTS('',3,(#131525,#131526,#131527,#131528,#131529,
#131530,#131531),.UNSPECIFIED.,.F.,.F.,(4,3,4),(-1.77635683940025E-15,0.785398163397447,
1.57079632679489),.UNSPECIFIED.);
#4137=B_SPLINE_CURVE_WITH_KNOTS('',3,(#131560,#131561,#131562,#131563,#131564,
#131565,#131566,#131567,#131568,#131569,#131570,#131571,#131572,#131573,
#131574,#131575,#131576,#131577,#131578),.UNSPECIFIED.,.F.,.F.,(4,3,3,3,
3,3,4),(0.,0.000905681138571635,0.00148255506350336,0.00163490147399828,
0.00222383259525504,0.00274053607505753,0.00296511012700672),
 .UNSPECIFIED.);
#4138=B_SPLINE_CURVE_WITH_KNOTS('',3,(#131584,#131585,#131586,#131587,#131588,
#131589,#131590),.UNSPECIFIED.,.F.,.F.,(4,3,4),(4.7123889803847,5.4977871437821,
6.28318530717959),.UNSPECIFIED.);
#4139=B_SPLINE_CURVE_WITH_KNOTS('',3,(#131594,#131595,#131596,#131597,#131598,
#131599,#131600),.UNSPECIFIED.,.F.,.F.,(4,3,4),(3.1415926535898,3.92699081698724,
4.71238898038469),.UNSPECIFIED.);
#4140=B_SPLINE_CURVE_WITH_KNOTS('',3,(#131608,#131609,#131610,#131611,#131612,
#131613,#131614),.UNSPECIFIED.,.F.,.F.,(4,3,4),(4.7123889803847,5.49778714378215,
6.28318530717959),.UNSPECIFIED.);
#4141=B_SPLINE_CURVE_WITH_KNOTS('',3,(#131618,#131619,#131620,#131621,#131622,
#131623,#131624),.UNSPECIFIED.,.F.,.F.,(4,3,4),(1.23467863058848E-16,0.785398163397455,
1.57079632679491),.UNSPECIFIED.);
#4142=B_SPLINE_CURVE_WITH_KNOTS('',3,(#131660,#131661,#131662,#131663,#131664,
#131665,#131666,#131667),.UNSPECIFIED.,.F.,.F.,(4,2,2,4),(9.50038252796028E-8,
0.5,0.75,1.),.UNSPECIFIED.);
#4143=B_SPLINE_CURVE_WITH_KNOTS('',3,(#131670,#131671,#131672,#131673,#131674,
#131675,#131676,#131677),.UNSPECIFIED.,.F.,.F.,(4,2,2,4),(0.,0.25,0.5,1.),
 .UNSPECIFIED.);
#4144=B_SPLINE_CURVE_WITH_KNOTS('',3,(#131735,#131736,#131737,#131738,#131739,
#131740,#131741,#131742,#131743,#131744,#131745,#131746,#131747,#131748,
#131749,#131750,#131751,#131752,#131753,#131754,#131755,#131756,#131757,
#131758,#131759,#131760,#131761,#131762,#131763,#131764,#131765,#131766,
#131767,#131768,#131769,#131770,#131771,#131772,#131773,#131774,#131775,
#131776,#131777,#131778,#131779,#131780),.UNSPECIFIED.,.F.,.F.,(4,3,3,3,
3,3,3,3,3,3,3,3,3,3,3,4),(0.,0.000143086625661407,0.000288513574061178,
0.000426569889101407,0.000433940522460948,0.000435486060835305,0.000709558652807024,
0.000867881044921896,0.000870195056295089,0.00115300716696448,0.00130182156738284,
0.00130356397838256,0.00142320462553202,0.00154203711262815,0.00165601506682433,
0.00173576208984379),.UNSPECIFIED.);
#4145=B_SPLINE_CURVE_WITH_KNOTS('',3,(#131783,#131784,#131785,#131786,#131787,
#131788,#131789,#131790,#131791,#131792),.UNSPECIFIED.,.F.,.F.,(4,2,2,2,
4),(0.,0.25,0.5,0.75,1.),.UNSPECIFIED.);
#4146=B_SPLINE_CURVE_WITH_KNOTS('',3,(#131841,#131842,#131843,#131844,#131845,
#131846,#131847,#131848,#131849,#131850,#131851,#131852,#131853,#131854,
#131855,#131856,#131857,#131858,#131859,#131860,#131861,#131862,#131863,
#131864,#131865,#131866,#131867,#131868,#131869,#131870,#131871,#131872,
#131873,#131874,#131875,#131876,#131877),.UNSPECIFIED.,.F.,.F.,(4,3,3,3,
3,3,3,3,3,3,3,3,4),(0.,0.000202328389738336,0.000393070531576854,0.000394637415448944,
0.000657523627602419,0.000787104044603762,0.000789274830897888,0.0010065772809709,
0.00118241998772925,0.00118391224634683,0.00131758895200357,0.00145591556828473,
0.00157854966179577),.UNSPECIFIED.);
#4147=B_SPLINE_CURVE_WITH_KNOTS('',3,(#131880,#131881,#131882,#131883,#131884,
#131885,#131886,#131887,#131888,#131889),.UNSPECIFIED.,.F.,.F.,(4,2,2,2,
4),(0.,0.25,0.500000000000001,0.75,1.),.UNSPECIFIED.);
#4148=B_SPLINE_CURVE_WITH_KNOTS('',3,(#131933,#131934,#131935,#131936,#131937,
#131938),.UNSPECIFIED.,.F.,.F.,(4,2,4),(0.,0.499999999999999,1.),
 .UNSPECIFIED.);
#4149=B_SPLINE_CURVE_WITH_KNOTS('',3,(#131941,#131942,#131943,#131944,#131945,
#131946),.UNSPECIFIED.,.F.,.F.,(4,2,4),(0.,0.500000000000001,1.),
 .UNSPECIFIED.);
#4150=B_SPLINE_CURVE_WITH_KNOTS('',3,(#131984,#131985,#131986,#131987,#131988,
#131989,#131990,#131991,#131992,#131993,#131994,#131995,#131996,#131997,
#131998,#131999,#132000,#132001,#132002,#132003,#132004,#132005,#132006,
#132007,#132008,#132009,#132010,#132011,#132012,#132013,#132014,#132015,
#132016,#132017,#132018,#132019,#132020,#132021,#132022,#132023,#132024,
#132025,#132026),.UNSPECIFIED.,.F.,.F.,(4,3,3,3,3,3,3,3,3,3,3,3,3,3,4),
(0.,0.000126914134949751,0.000262536143227196,0.000398158151504642,0.000399655746142223,
0.000648709723489428,0.000797160169367613,0.000799311492284445,0.00106908297786168,
0.00119740971470135,0.00119896723842667,0.00131358784144406,0.00142842585215498,
0.00154010419706602,0.00159862298456889),.UNSPECIFIED.);
#4151=B_SPLINE_CURVE_WITH_KNOTS('',3,(#132029,#132030,#132031,#132032,#132033,
#132034,#132035,#132036,#132037,#132038,#132039,#132040,#132041,#132042,
#132043,#132044,#132045,#132046,#132047,#132048,#132049,#132050,#132051,
#132052,#132053,#132054,#132055,#132056,#132057,#132058,#132059,#132060,
#132061,#132062,#132063,#132064,#132065),.UNSPECIFIED.,.F.,.F.,(4,3,3,3,
3,3,3,3,3,3,3,3,4),(0.,0.0847666443586869,0.169627705088856,0.25,0.337926927638317,
0.426118365859893,0.499999999999999,0.587394748316425,0.674958582364191,
0.749999999999999,0.835586424041094,0.921207988122376,1.),.UNSPECIFIED.);
#4152=B_SPLINE_CURVE_WITH_KNOTS('',3,(#132119,#132120,#132121,#132122,#132123,
#132124,#132125,#132126,#132127,#132128,#132129,#132130,#132131,#132132,
#132133,#132134,#132135,#132136,#132137,#132138,#132139,#132140,#132141,
#132142,#132143,#132144,#132145,#132146,#132147,#132148,#132149,#132150,
#132151,#132152,#132153,#132154,#132155,#132156,#132157,#132158,#132159,
#132160,#132161),.UNSPECIFIED.,.F.,.F.,(4,3,3,3,3,3,3,3,3,3,3,3,3,3,4),
(0.,0.000124096840872178,0.000249826409753251,0.000377706687950382,0.000412914062840745,
0.000414565512418997,0.000703661138433462,0.00082582812568149,0.000828047391046449,
0.0011074529067618,0.00123874218852223,0.00124024370669315,0.00141015471005694,
0.00158186346550348,0.00165165625136298),.UNSPECIFIED.);
#4153=B_SPLINE_CURVE_WITH_KNOTS('',3,(#132164,#132165,#132166,#132167,#132168,
#132169,#132170,#132171,#132172,#132173),.UNSPECIFIED.,.F.,.F.,(4,2,2,2,
4),(0.,0.25,0.5,0.75,1.),.UNSPECIFIED.);
#4154=B_SPLINE_CURVE_WITH_KNOTS('',3,(#132185,#132186,#132187,#132188,#132189,
#132190,#132191,#132192,#132193,#132194,#132195,#132196,#132197,#132198,
#132199,#132200,#132201,#132202,#132203),.UNSPECIFIED.,.F.,.F.,(4,3,3,3,
3,3,4),(0.,0.163601301030445,0.331800650515222,0.5,0.666788663885585,0.833394331942792,
1.),.UNSPECIFIED.);
#4155=B_SPLINE_CURVE_WITH_KNOTS('',3,(#132211,#132212,#132213,#132214),
 .UNSPECIFIED.,.F.,.F.,(4,4),(0.,1.),.UNSPECIFIED.);
#4156=B_SPLINE_CURVE_WITH_KNOTS('',3,(#132244,#132245,#132246,#132247,#132248,
#132249),.UNSPECIFIED.,.F.,.F.,(4,2,4),(0.,0.5,1.),.UNSPECIFIED.);
#4157=B_SPLINE_CURVE_WITH_KNOTS('',3,(#132250,#132251,#132252,#132253,#132254,
#132255),.UNSPECIFIED.,.F.,.F.,(4,2,4),(0.,0.5,1.),.UNSPECIFIED.);
#4158=B_SPLINE_CURVE_WITH_KNOTS('',3,(#132295,#132296,#132297,#132298,#132299,
#132300,#132301,#132302,#132303,#132304),.UNSPECIFIED.,.F.,.F.,(4,2,2,2,
4),(0.,0.25,0.5,0.75,1.),.UNSPECIFIED.);
#4159=B_SPLINE_CURVE_WITH_KNOTS('',3,(#132305,#132306,#132307,#132308,#132309,
#132310,#132311,#132312,#132313,#132314,#132315,#132316,#132317,#132318,
#132319,#132320,#132321,#132322,#132323,#132324,#132325,#132326,#132327,
#132328,#132329,#132330,#132331,#132332,#132333,#132334,#132335,#132336,
#132337,#132338,#132339,#132340,#132341,#132342,#132343,#132344,#132345,
#132346,#132347,#132348,#132349,#132350),.UNSPECIFIED.,.F.,.F.,(4,3,3,3,
3,3,3,3,3,3,3,3,3,3,3,4),(0.,0.000126520648339663,0.000255464746612453,
0.000383289319161181,0.000402202417173518,0.000403696977019687,0.000649443966577954,
0.000805221313633907,0.000807393954039373,0.00107833188461984,0.00120950149130569,
0.00121109093105906,0.0013247333581667,0.00143856386975717,0.00154897302143399,
0.00161478790807874),.UNSPECIFIED.);
#4160=B_SPLINE_CURVE_WITH_KNOTS('',3,(#132406,#132407,#132408,#132409,#132410,
#132411,#132412,#132413,#132414,#132415),.UNSPECIFIED.,.F.,.F.,(4,2,2,2,
4),(0.,0.25,0.5,0.750000000000001,1.),.UNSPECIFIED.);
#4161=B_SPLINE_CURVE_WITH_KNOTS('',3,(#132416,#132417,#132418,#132419,#132420,
#132421,#132422,#132423,#132424,#132425,#132426,#132427,#132428,#132429,
#132430,#132431,#132432,#132433,#132434,#132435,#132436,#132437,#132438,
#132439,#132440,#132441,#132442,#132443,#132444,#132445,#132446,#132447,
#132448,#132449,#132450,#132451,#132452,#132453,#132454,#132455,#132456,
#132457,#132458),.UNSPECIFIED.,.F.,.F.,(4,3,3,3,3,3,3,3,3,3,3,3,3,3,4),
(0.,0.000133466187697127,0.000269195218942899,0.000394210955663315,0.000395766414125755,
0.000656135621800232,0.000788421911326631,0.000790581154836762,0.00102610013257283,
0.00118263286698995,0.00118412769954352,0.0013056923112994,0.00142779909867113,
0.00154775473597367,0.00157684382265327),.UNSPECIFIED.);
#4162=B_SPLINE_CURVE_WITH_KNOTS('',3,(#132497,#132498,#132499,#132500,#132501,
#132502),.UNSPECIFIED.,.F.,.F.,(4,2,4),(0.000117319100397047,0.500000000000001,
1.),.UNSPECIFIED.);
#4163=B_SPLINE_CURVE_WITH_KNOTS('',3,(#132503,#132504,#132505,#132506,#132507,
#132508),.UNSPECIFIED.,.F.,.F.,(4,2,4),(0.,0.499999999999999,1.),
 .UNSPECIFIED.);
#4164=B_SPLINE_CURVE_WITH_KNOTS('',3,(#132564,#132565,#132566,#132567,#132568,
#132569,#132570,#132571,#132572,#132573),.UNSPECIFIED.,.F.,.F.,(4,2,2,2,
4),(0.,0.25,0.5,0.75,0.999996541004657),.UNSPECIFIED.);
#4165=B_SPLINE_CURVE_WITH_KNOTS('',3,(#132574,#132575,#132576,#132577,#132578,
#132579,#132580,#132581,#132582,#132583,#132584,#132585),.UNSPECIFIED.,
 .F.,.F.,(4,2,2,2,2,4),(0.,0.000425271195884802,0.000850542391769605,0.00127581358765441,
0.00148844918559681,0.00170108478353921),.UNSPECIFIED.);
#4166=B_SPLINE_CURVE_WITH_KNOTS('',3,(#132642,#132643,#132644,#132645,#132646,
#132647,#132648,#132649,#132650,#132651,#132652,#132653),.UNSPECIFIED.,
 .F.,.F.,(4,2,2,2,2,4),(0.,0.25,0.499999999999999,0.624999999999999,0.749999999999999,
1.),.UNSPECIFIED.);
#4167=B_SPLINE_CURVE_WITH_KNOTS('',3,(#132654,#132655,#132656,#132657,#132658,
#132659,#132660,#132661,#132662,#132663,#132664,#132665,#132666,#132667,
#132668,#132669,#132670,#132671,#132672,#132673,#132674,#132675,#132676,
#132677,#132678,#132679,#132680,#132681,#132682,#132683,#132684,#132685,
#132686,#132687,#132688,#132689,#132690,#132691,#132692,#132693,#132694,
#132695,#132696),.UNSPECIFIED.,.F.,.F.,(4,3,3,3,3,3,3,3,3,3,3,3,3,3,4),
(0.,0.000155846438314328,0.000318202659849571,0.000479330525642439,0.00048138854528345,
0.000719581971214066,0.000722082817925181,0.000946156964943833,0.000960283452349071,
0.000962777090566911,0.00127358059295693,0.00144265205691353,0.00144416563585035,
0.00187401285519362,0.0019255541811338),.UNSPECIFIED.);
#4168=B_SPLINE_CURVE_WITH_KNOTS('',3,(#132719,#132720,#132721,#132722),
 .UNSPECIFIED.,.F.,.F.,(4,4),(0.,1.),.UNSPECIFIED.);
#4169=B_SPLINE_CURVE_WITH_KNOTS('',3,(#132741,#132742,#132743,#132744,#132745,
#132746,#132747,#132748,#132749,#132750),.UNSPECIFIED.,.F.,.F.,(4,3,3,4),
(0.,0.361091546871882,0.717052845282562,1.),.UNSPECIFIED.);
#4170=B_SPLINE_CURVE_WITH_KNOTS('',3,(#132760,#132761,#132762,#132763,#132764,
#132765),.UNSPECIFIED.,.F.,.F.,(4,2,4),(0.,0.5,1.),.UNSPECIFIED.);
#4171=B_SPLINE_CURVE_WITH_KNOTS('',3,(#132772,#132773,#132774,#132775,#132776,
#132777,#132778,#132779),.UNSPECIFIED.,.F.,.F.,(4,2,2,4),(0.,0.25,0.5,1.),
 .UNSPECIFIED.);
#4172=B_SPLINE_CURVE_WITH_KNOTS('',3,(#132787,#132788,#132789,#132790,#132791,
#132792,#132793,#132794,#132795,#132796,#132797,#132798,#132799,#132800,
#132801,#132802,#132803,#132804,#132805,#132806,#132807,#132808,#132809,
#132810,#132811,#132812,#132813,#132814,#132815,#132816,#132817,#132818,
#132819,#132820,#132821,#132822,#132823,#132824,#132825,#132826,#132827,
#132828,#132829),.UNSPECIFIED.,.F.,.F.,(4,3,3,3,3,3,3,3,3,3,3,3,3,3,4),
(0.,0.000127008698005028,0.000262529185195807,0.000398049672386586,0.000399547425717595,
0.000648679298355362,0.000796943972592097,0.00079909485143519,0.00106876545795233,
0.00119708559701167,0.00119864227715278,0.0013133030862701,0.00142818443762435,
0.00153991729226742,0.00159818970287038),.UNSPECIFIED.);
#4173=B_SPLINE_CURVE_WITH_KNOTS('',3,(#132833,#132834,#132835,#132836,#132837,
#132838),.UNSPECIFIED.,.F.,.F.,(4,2,4),(0.,0.500000000000001,1.),
 .UNSPECIFIED.);
#4174=B_SPLINE_CURVE_WITH_KNOTS('',3,(#132846,#132847,#132848,#132849,#132850,
#132851,#132852,#132853),.UNSPECIFIED.,.F.,.F.,(4,2,2,4),(0.,0.5,0.75,1.),
 .UNSPECIFIED.);
#4175=B_SPLINE_CURVE_WITH_KNOTS('',3,(#132857,#132858,#132859,#132860,#132861,
#132862,#132863,#132864,#132865,#132866,#132867,#132868,#132869,#132870,
#132871,#132872,#132873,#132874,#132875,#132876,#132877,#132878,#132879,
#132880,#132881,#132882,#132883,#132884,#132885,#132886,#132887,#132888,
#132889,#132890,#132891,#132892,#132893,#132894,#132895,#132896,#132897,
#132898,#132899,#132900,#132901,#132902,#132903,#132904,#132905,#132906,
#132907,#132908),.UNSPECIFIED.,.F.,.F.,(4,3,3,3,3,3,3,3,3,3,3,3,3,3,3,3,
3,4),(0.,0.00016297400035178,0.000319609377590886,0.00044215652538248,0.000443701447435103,
0.000705760117587487,0.000884313050764961,0.000886662825918404,0.00117556448144828,
0.00132646957614744,0.00132826306101653,0.0014179261914274,0.00143700870749306,
0.00151991305600227,0.0015500272930556,0.00163724702277249,0.00172192727480442,
0.00176862610152992),.UNSPECIFIED.);
#4176=B_SPLINE_CURVE_WITH_KNOTS('',3,(#132916,#132917,#132918,#132919,#132920,
#132921,#132922,#132923,#132924,#132925),.UNSPECIFIED.,.F.,.F.,(4,2,2,2,
4),(0.,0.25,0.375000000000001,0.5,1.),.UNSPECIFIED.);
#4177=B_SPLINE_CURVE_WITH_KNOTS('',3,(#132929,#132930,#132931,#132932,#132933,
#132934,#132935,#132936,#132937,#132938,#132939,#132940,#132941,#132942,
#132943,#132944,#132945,#132946,#132947,#132948,#132949,#132950),
 .UNSPECIFIED.,.F.,.F.,(4,3,3,3,3,3,3,4),(0.,0.000360666935666808,0.000449610485509243,
0.000757497233646948,0.000899220971018486,0.00134883145652773,0.00157363669928234,
0.00179844194203696),.UNSPECIFIED.);
#4178=B_SPLINE_CURVE_WITH_KNOTS('',3,(#132958,#132959,#132960,#132961,#132962,
#132963,#132964,#132965,#132966,#132967,#132968,#132969,#132970,#132971,
#132972,#132973,#132974,#132975,#132976,#132977,#132978,#132979,#132980,
#132981,#132982,#132983,#132984,#132985,#132986,#132987,#132988,#132989,
#132990,#132991,#132992,#132993,#132994,#132995,#132996,#132997,#132998,
#132999,#133000),.UNSPECIFIED.,.F.,.F.,(4,3,3,3,3,3,3,3,3,3,3,3,3,3,4),
(0.,0.000195170703378013,0.000400502314394682,0.000446304927367807,0.000448134863283483,
0.000669908621781835,0.000672202294925215,0.000876863243054838,0.000893889262421614,
0.000896269726566947,0.00123667266509072,0.00134284656974637,0.00134440458985042,
0.00167688520284659,0.0017925394531339),.UNSPECIFIED.);
#4179=B_SPLINE_CURVE_WITH_KNOTS('',3,(#133004,#133005,#133006,#133007,#133008,
#133009,#133010,#133011,#133012,#133013,#133014,#133015,#133016,#133017,
#133018,#133019,#133020,#133021,#133022,#133023,#133024,#133025,#133026,
#133027,#133028,#133029,#133030,#133031,#133032,#133033,#133034,#133035,
#133036,#133037,#133038,#133039,#133040,#133041,#133042,#133043,#133044,
#133045,#133046,#133047,#133048,#133049),.UNSPECIFIED.,.F.,.F.,(4,3,3,3,
3,3,3,3,3,3,3,3,3,3,3,4),(0.,0.000125938335250217,0.000251511263370856,
0.000372362493801517,0.000393010036481153,0.000394487267106025,0.000650087135465414,
0.000786020072962305,0.00078818046791129,0.00103122780428863,0.00117903010944346,
0.0011805925563396,0.00129302327548806,0.00140596384630442,0.00151582795231503,
0.00157204014592461),.UNSPECIFIED.);
#4180=B_SPLINE_CURVE_WITH_KNOTS('',3,(#133057,#133058,#133059,#133060,#133061,
#133062,#133063,#133064,#133065,#133066,#133067,#133068,#133069,#133070,
#133071,#133072,#133073,#133074,#133075,#133076,#133077,#133078,#133079,
#133080,#133081,#133082,#133083,#133084,#133085,#133086,#133087,#133088,
#133089,#133090,#133091,#133092,#133093,#133094,#133095,#133096,#133097,
#133098,#133099),.UNSPECIFIED.,.F.,.F.,(4,3,3,3,3,3,3,3,3,3,3,3,3,3,4),
(0.,0.000128730917859202,0.000262886260532207,0.000397041603205213,0.000398543239038962,
0.00064756610669814,0.000794935814474575,0.000797086478077925,0.00106486773330264,
0.00119408026895391,0.00119562971711689,0.00131091067532176,0.0014265060792,
0.00153915940329535,0.00159417295615585),.UNSPECIFIED.);
#4181=B_SPLINE_CURVE_WITH_KNOTS('',3,(#133103,#133104,#133105,#133106,#133107,
#133108,#133109,#133110),.UNSPECIFIED.,.F.,.F.,(4,2,2,4),(0.,0.5,0.75,1.),
 .UNSPECIFIED.);
#4182=B_SPLINE_CURVE_WITH_KNOTS('',3,(#133117,#133118,#133119,#133120,#133121,
#133122),.UNSPECIFIED.,.F.,.F.,(4,2,4),(0.,0.5,1.),.UNSPECIFIED.);
#4183=B_SPLINE_CURVE_WITH_KNOTS('',3,(#133138,#133139,#133140,#133141),
 .UNSPECIFIED.,.F.,.F.,(4,4),(0.,6.88517764864569E-5),.UNSPECIFIED.);
#4184=B_SPLINE_CURVE_WITH_KNOTS('',3,(#133167,#133168,#133169,#133170,#133171,
#133172),.UNSPECIFIED.,.F.,.F.,(4,2,4),(0.,0.5,1.),.UNSPECIFIED.);
#4185=B_SPLINE_CURVE_WITH_KNOTS('',3,(#133189,#133190,#133191,#133192,#133193,
#133194,#133195),.UNSPECIFIED.,.F.,.F.,(4,3,4),(1.5707963267949,2.35619449019235,
3.1415926535898),.UNSPECIFIED.);
#4186=B_SPLINE_CURVE_WITH_KNOTS('',3,(#133199,#133200,#133201,#133202,#133203,
#133204,#133205),.UNSPECIFIED.,.F.,.F.,(4,3,4),(1.23467863058847E-16,0.785398163397447,
1.5707963267949),.UNSPECIFIED.);
#4187=B_SPLINE_CURVE_WITH_KNOTS('',3,(#133211,#133212,#133213,#133214,#133215,
#133216,#133217,#133218,#133219,#133220,#133221,#133222,#133223,#133224,
#133225,#133226,#133227,#133228,#133229),.UNSPECIFIED.,.F.,.F.,(4,3,3,3,
3,3,4),(0.000169216231991231,0.000729993311375969,0.000968460740699438,
0.00168309612079798,0.00176770524940811,0.00279102522271593,0.00336619426682546),
 .UNSPECIFIED.);
#4188=B_SPLINE_CURVE_WITH_KNOTS('',3,(#133239,#133240,#133241,#133242,#133243,
#133244,#133245),.UNSPECIFIED.,.F.,.F.,(4,3,4),(4.71238898038469,5.49778714378214,
6.28318530717959),.UNSPECIFIED.);
#4189=B_SPLINE_CURVE_WITH_KNOTS('',3,(#133249,#133250,#133251,#133252,#133253,
#133254,#133255),.UNSPECIFIED.,.F.,.F.,(4,3,4),(1.23467863058847E-16,0.785398163397447,
1.5707963267949),.UNSPECIFIED.);
#4190=B_SPLINE_CURVE_WITH_KNOTS('',3,(#133288,#133289,#133290,#133291,#133292,
#133293,#133294),.UNSPECIFIED.,.F.,.F.,(4,3,4),(1.5707963267949,2.35619449019234,
3.14159265358979),.UNSPECIFIED.);
#4191=B_SPLINE_CURVE_WITH_KNOTS('',3,(#133298,#133299,#133300,#133301,#133302,
#133303,#133304),.UNSPECIFIED.,.F.,.F.,(4,3,4),(3.14159265358979,3.92699081698724,
4.71238898038469),.UNSPECIFIED.);
#4192=B_SPLINE_CURVE_WITH_KNOTS('',3,(#133310,#133311,#133312,#133313,#133314,
#133315,#133316,#133317,#133318,#133319,#133320,#133321,#133322,#133323,
#133324,#133325),.UNSPECIFIED.,.F.,.F.,(4,3,3,3,3,4),(0.000244714080610449,
0.00121583023103576,0.00174053473821824,0.00180545417371792,0.00292276797843844,
0.00336619426682539),.UNSPECIFIED.);
#4193=B_SPLINE_CURVE_WITH_KNOTS('',3,(#133329,#133330,#133331,#133332,#133333,
#133334,#133335),.UNSPECIFIED.,.F.,.F.,(4,3,4),(1.5707963267949,2.35619449019232,
3.14159265358979),.UNSPECIFIED.);
#4194=B_SPLINE_CURVE_WITH_KNOTS('',3,(#133339,#133340,#133341,#133342,#133343,
#133344,#133345),.UNSPECIFIED.,.F.,.F.,(4,3,4),(-1.77635683940025E-15,0.785398163397447,
1.57079632679489),.UNSPECIFIED.);
#4195=B_SPLINE_CURVE_WITH_KNOTS('',3,(#133367,#133368,#133369,#133370,#133371,
#133372),.UNSPECIFIED.,.F.,.F.,(4,2,4),(0.,0.5,1.),.UNSPECIFIED.);
#4196=B_SPLINE_CURVE_WITH_KNOTS('',3,(#133415,#133416,#133417,#133418,#133419,
#133420,#133421,#133422),.UNSPECIFIED.,.F.,.F.,(4,2,2,4),(0.,0.25,0.5,1.),
 .UNSPECIFIED.);
#4197=B_SPLINE_CURVE_WITH_KNOTS('',3,(#133459,#133460,#133461,#133462,#133463,
#133464,#133465,#133466,#133467,#133468),.UNSPECIFIED.,.F.,.F.,(4,2,2,2,
4),(0.,0.25,0.5,0.749999999999999,1.),.UNSPECIFIED.);
#4198=B_SPLINE_CURVE_WITH_KNOTS('',3,(#133517,#133518,#133519,#133520,#133521,
#133522,#133523,#133524,#133525,#133526),.UNSPECIFIED.,.F.,.F.,(4,2,2,2,
4),(0.,0.25,0.500000000000001,0.750000000000001,1.),.UNSPECIFIED.);
#4199=B_SPLINE_CURVE_WITH_KNOTS('',3,(#133580,#133581,#133582,#133583,#133584,
#133585,#133586,#133587,#133588,#133589,#133590,#133591,#133592,#133593,
#133594,#133595,#133596,#133597,#133598,#133599,#133600,#133601,#133602,
#133603,#133604,#133605,#133606,#133607,#133608,#133609,#133610,#133611,
#133612,#133613,#133614,#133615,#133616,#133617,#133618,#133619,#133620,
#133621,#133622,#133623,#133624,#133625,#133626,#133627,#133628),
 .UNSPECIFIED.,.F.,.F.,(4,3,3,3,3,3,3,3,3,3,3,3,3,3,3,3,4),(0.,0.087564719729141,
0.168782359864571,0.245864630016523,0.25,0.354535950890996,0.447075382683936,
0.5,0.555980429743289,0.611777642915431,0.625,0.691371875377358,0.750000000000001,
0.82986450531225,0.906218926800638,0.979271353598852,1.),.UNSPECIFIED.);
#4200=B_SPLINE_CURVE_WITH_KNOTS('',3,(#133677,#133678,#133679,#133680,#133681,
#133682,#133683,#133684,#133685,#133686,#133687,#133688,#133689,#133690,
#133691,#133692,#133693,#133694,#133695,#133696,#133697,#133698,#133699,
#133700,#133701,#133702,#133703,#133704,#133705,#133706,#133707,#133708,
#133709,#133710,#133711,#133712,#133713,#133714,#133715,#133716,#133717,
#133718,#133719,#133720,#133721,#133722,#133723,#133724,#133725),
 .UNSPECIFIED.,.F.,.F.,(4,3,3,3,3,3,3,3,3,3,3,3,3,3,3,3,4),(0.,0.0673211146699331,
0.134715456033185,0.202659384537495,0.25,0.322758924734933,0.396441399379554,
0.471979834578492,0.5,0.575516106875766,0.652984132469324,0.733824490565147,
0.75,0.829223437699597,0.91178455799991,0.940509163793382,1.),
 .UNSPECIFIED.);
#4201=B_SPLINE_CURVE_WITH_KNOTS('',3,(#133773,#133774,#133775,#133776,#133777,
#133778,#133779,#133780,#133781,#133782,#133783,#133784,#133785,#133786,
#133787,#133788,#133789,#133790,#133791,#133792,#133793,#133794,#133795,
#133796,#133797,#133798,#133799,#133800,#133801,#133802,#133803,#133804,
#133805,#133806,#133807,#133808,#133809,#133810,#133811,#133812,#133813,
#133814,#133815,#133816,#133817,#133818,#133819,#133820,#133821),
 .UNSPECIFIED.,.F.,.F.,(4,3,3,3,3,3,3,3,3,3,3,3,3,3,3,3,4),(0.,0.0643187684459386,
0.151144143415235,0.238358107561426,0.317473279366759,0.394527907474398,
0.469118347726267,0.5,0.567041589025861,0.624999999999999,0.679259523694771,
0.733605072096865,0.75,0.821970997330374,0.892478293684135,0.961558653299543,
1.),.UNSPECIFIED.);
#4202=B_SPLINE_CURVE_WITH_KNOTS('',3,(#133870,#133871,#133872,#133873,#133874,
#133875,#133876,#133877,#133878,#133879),.UNSPECIFIED.,.F.,.F.,(4,2,2,2,
4),(0.,0.25,0.499999999999999,0.749999999999998,1.),.UNSPECIFIED.);
#4203=B_SPLINE_CURVE_WITH_KNOTS('',3,(#133921,#133922,#133923,#133924,#133925,
#133926,#133927,#133928),.UNSPECIFIED.,.F.,.F.,(4,2,2,4),(0.,0.25,0.5,1.),
 .UNSPECIFIED.);
#4204=B_SPLINE_CURVE_WITH_KNOTS('',3,(#133965,#133966,#133967,#133968,#133969,
#133970),.UNSPECIFIED.,.F.,.F.,(4,2,4),(0.,0.499999999999999,1.),
 .UNSPECIFIED.);
#4205=B_SPLINE_CURVE_WITH_KNOTS('',3,(#134007,#134008,#134009,#134010,#134011,
#134012,#134013,#134014,#134015,#134016,#134017,#134018,#134019,#134020,
#134021,#134022,#134023,#134024,#134025,#134026,#134027,#134028,#134029,
#134030,#134031,#134032,#134033,#134034,#134035,#134036,#134037,#134038,
#134039,#134040,#134041,#134042,#134043),.UNSPECIFIED.,.F.,.F.,(4,3,3,3,
3,3,3,3,3,3,3,3,4),(0.,0.0849060387652225,0.169905587248193,0.25,0.337991601382829,
0.426246250502731,0.499999999999999,0.587308431420735,0.674783689226744,
0.749999999999999,0.835530010300542,0.921094023848129,1.),.UNSPECIFIED.);
#4206=B_SPLINE_CURVE_WITH_KNOTS('',3,(#134084,#134085,#134086,#134087,#134088,
#134089,#134090,#134091),.UNSPECIFIED.,.F.,.F.,(4,2,2,4),(0.,0.5,0.75,1.),
 .UNSPECIFIED.);
#4207=B_SPLINE_CURVE_WITH_KNOTS('',3,(#134096,#134097,#134098,#134099,#134100,
#134101,#134102,#134103,#134104,#134105),.UNSPECIFIED.,.F.,.F.,(4,2,2,2,
4),(0.,0.250000000000004,0.5,0.750000000000003,1.),.UNSPECIFIED.);
#4208=B_SPLINE_CURVE_WITH_KNOTS('',3,(#134106,#134107,#134108,#134109,#134110,
#134111,#134112,#134113,#134114,#134115),.UNSPECIFIED.,.F.,.F.,(4,2,2,2,
4),(0.,0.250000000000001,0.500000000000001,0.75,1.),.UNSPECIFIED.);
#4209=B_SPLINE_CURVE_WITH_KNOTS('',3,(#134142,#134143,#134144,#134145,#134146,
#134147),.UNSPECIFIED.,.F.,.F.,(4,2,4),(0.,0.5,1.),.UNSPECIFIED.);
#4210=B_SPLINE_CURVE_WITH_KNOTS('',3,(#134172,#134173,#134174,#134175,#134176,
#134177),.UNSPECIFIED.,.F.,.F.,(4,2,4),(0.,0.5,1.),.UNSPECIFIED.);
#4211=B_SPLINE_CURVE_WITH_KNOTS('',3,(#134185,#134186,#134187,#134188,#134189,
#134190,#134191,#134192,#134193,#134194),.UNSPECIFIED.,.F.,.F.,(4,2,2,2,
4),(0.,0.250000000000004,0.5,0.749999999999997,1.),.UNSPECIFIED.);
#4212=B_SPLINE_CURVE_WITH_KNOTS('',3,(#134215,#134216,#134217,#134218,#134219,
#134220),.UNSPECIFIED.,.F.,.F.,(4,2,4),(0.,0.5,1.),.UNSPECIFIED.);
#4213=B_SPLINE_CURVE_WITH_KNOTS('',3,(#134246,#134247,#134248,#134249,#134250,
#134251),.UNSPECIFIED.,.F.,.F.,(4,2,4),(0.,0.502999491316249,1.),
 .UNSPECIFIED.);
#4214=B_SPLINE_CURVE_WITH_KNOTS('',3,(#134252,#134253,#134254,#134255,#134256,
#134257),.UNSPECIFIED.,.F.,.F.,(4,2,4),(0.,0.5,1.),.UNSPECIFIED.);
#4215=B_SPLINE_CURVE_WITH_KNOTS('',3,(#134261,#134262,#134263,#134264,#134265,
#134266,#134267,#134268,#134269,#134270),.UNSPECIFIED.,.F.,.F.,(4,2,2,2,
4),(0.,0.25,0.5,0.75,1.),.UNSPECIFIED.);
#4216=B_SPLINE_CURVE_WITH_KNOTS('',3,(#134297,#134298,#134299,#134300,#134301,
#134302),.UNSPECIFIED.,.F.,.F.,(4,2,4),(0.,0.5,1.),.UNSPECIFIED.);
#4217=B_SPLINE_CURVE_WITH_KNOTS('',3,(#134327,#134328,#134329,#134330,#134331,
#134332),.UNSPECIFIED.,.F.,.F.,(4,2,4),(0.,0.500000000000002,1.),
 .UNSPECIFIED.);
#4218=B_SPLINE_CURVE_WITH_KNOTS('',3,(#134359,#134360,#134361,#134362,#134363,
#134364),.UNSPECIFIED.,.F.,.F.,(4,2,4),(0.,0.5,1.),.UNSPECIFIED.);
#4219=B_SPLINE_CURVE_WITH_KNOTS('',3,(#134369,#134370,#134371,#134372,#134373,
#134374,#134375,#134376,#134377,#134378),.UNSPECIFIED.,.F.,.F.,(4,2,2,2,
4),(0.,0.250000000000001,0.499999999999999,0.749999999999999,1.),
 .UNSPECIFIED.);
#4220=B_SPLINE_CURVE_WITH_KNOTS('',3,(#134379,#134380,#134381,#134382,#134383,
#134384,#134385,#134386,#134387,#134388),.UNSPECIFIED.,.F.,.F.,(4,2,2,2,
4),(0.,0.250000000000001,0.500000000000002,0.750000000000002,1.),
 .UNSPECIFIED.);
#4221=B_SPLINE_CURVE_WITH_KNOTS('',3,(#134415,#134416,#134417,#134418,#134419,
#134420),.UNSPECIFIED.,.F.,.F.,(4,2,4),(0.,0.5,1.),.UNSPECIFIED.);
#4222=B_SPLINE_CURVE_WITH_KNOTS('',3,(#134445,#134446,#134447,#134448,#134449,
#134450),.UNSPECIFIED.,.F.,.F.,(4,2,4),(0.,0.500000000000002,1.),
 .UNSPECIFIED.);
#4223=B_SPLINE_CURVE_WITH_KNOTS('',3,(#134474,#134475,#134476,#134477,#134478,
#134479),.UNSPECIFIED.,.F.,.F.,(4,2,4),(0.,0.503000256250808,1.),
 .UNSPECIFIED.);
#4224=B_SPLINE_CURVE_WITH_KNOTS('',3,(#134480,#134481,#134482,#134483,#134484,
#134485,#134486,#134487,#134488,#134489,#134490,#134491),.UNSPECIFIED.,
 .F.,.F.,(4,2,2,2,2,4),(0.,0.250000000000001,0.375000000000002,0.499999999999998,
0.750000000000001,1.),.UNSPECIFIED.);
#4225=B_SPLINE_CURVE_WITH_KNOTS('',3,(#134495,#134496,#134497,#134498,#134499,
#134500,#134501,#134502,#134503,#134504),.UNSPECIFIED.,.F.,.F.,(4,2,2,2,
4),(0.,0.25,0.5,0.75,1.),.UNSPECIFIED.);
#4226=B_SPLINE_CURVE_WITH_KNOTS('',3,(#134531,#134532,#134533,#134534,#134535,
#134536),.UNSPECIFIED.,.F.,.F.,(4,2,4),(0.,0.499999999999998,1.),
 .UNSPECIFIED.);
#4227=B_SPLINE_CURVE_WITH_KNOTS('',3,(#134561,#134562,#134563,#134564,#134565,
#134566),.UNSPECIFIED.,.F.,.F.,(4,2,4),(0.,0.500000000000002,1.),
 .UNSPECIFIED.);
#4228=B_SPLINE_CURVE_WITH_KNOTS('',3,(#134577,#134578,#134579,#134580,#134581,
#134582,#134583,#134584,#134585,#134586),.UNSPECIFIED.,.F.,.F.,(4,2,2,2,
4),(0.,0.250000000000004,0.5,0.749999999999997,1.),.UNSPECIFIED.);
#4229=B_SPLINE_CURVE_WITH_KNOTS('',3,(#134587,#134588,#134589,#134590,#134591,
#134592,#134593,#134594,#134595,#134596),.UNSPECIFIED.,.F.,.F.,(4,2,2,2,
4),(0.,0.250000000000001,0.5,0.75,1.),.UNSPECIFIED.);
#4230=B_SPLINE_CURVE_WITH_KNOTS('',3,(#134623,#134624,#134625,#134626,#134627,
#134628),.UNSPECIFIED.,.F.,.F.,(4,2,4),(0.,0.5,1.),.UNSPECIFIED.);
#4231=B_SPLINE_CURVE_WITH_KNOTS('',3,(#134653,#134654,#134655,#134656,#134657,
#134658),.UNSPECIFIED.,.F.,.F.,(4,2,4),(0.,0.5,1.),.UNSPECIFIED.);
#4232=B_SPLINE_CURVE_WITH_KNOTS('',3,(#134666,#134667,#134668,#134669,#134670,
#134671,#134672,#134673,#134674,#134675),.UNSPECIFIED.,.F.,.F.,(4,2,2,2,
4),(0.,0.250000000000004,0.5,0.749999999999997,1.),.UNSPECIFIED.);
#4233=B_SPLINE_CURVE_WITH_KNOTS('',3,(#134724,#134725,#134726,#134727,#134728,
#134729,#134730,#134731,#134732,#134733,#134734,#134735,#134736),
 .UNSPECIFIED.,.F.,.F.,(4,3,3,3,4),(0.,0.269537008270268,0.544459888994111,
0.814598147393945,1.),.UNSPECIFIED.);
#4234=B_SPLINE_CURVE_WITH_KNOTS('',3,(#134740,#134741,#134742,#134743,#134744,
#134745,#134746,#134747,#134748,#134749),.UNSPECIFIED.,.F.,.F.,(4,2,2,2,
4),(0.,0.250000000000001,0.5,0.75,1.),.UNSPECIFIED.);
#4235=B_SPLINE_CURVE_WITH_KNOTS('',3,(#134776,#134777,#134778,#134779,#134780,
#134781),.UNSPECIFIED.,.F.,.F.,(4,2,4),(0.,0.5,1.),.UNSPECIFIED.);
#4236=B_SPLINE_CURVE_WITH_KNOTS('',3,(#134806,#134807,#134808,#134809,#134810,
#134811),.UNSPECIFIED.,.F.,.F.,(4,2,4),(0.,0.499999999999998,1.),
 .UNSPECIFIED.);
#4237=B_SPLINE_CURVE_WITH_KNOTS('',3,(#134836,#134837,#134838,#134839,#134840,
#134841),.UNSPECIFIED.,.F.,.F.,(4,2,4),(0.,0.497000288786711,1.),
 .UNSPECIFIED.);
#4238=B_SPLINE_CURVE_WITH_KNOTS('',3,(#134843,#134844,#134845,#134846,#134847,
#134848),.UNSPECIFIED.,.F.,.F.,(4,2,4),(0.,0.499999999999998,1.),
 .UNSPECIFIED.);
#4239=B_SPLINE_CURVE_WITH_KNOTS('',3,(#134871,#134872,#134873,#134874,#134875,
#134876,#134877,#134878,#134879,#134880),.UNSPECIFIED.,.F.,.F.,(4,2,2,2,
4),(0.,0.250000000000001,0.499999999999998,0.749999999999999,1.),
 .UNSPECIFIED.);
#4240=B_SPLINE_CURVE_WITH_KNOTS('',3,(#134907,#134908,#134909,#134910,#134911,
#134912),.UNSPECIFIED.,.F.,.F.,(4,2,4),(0.,0.5,1.),.UNSPECIFIED.);
#4241=B_SPLINE_CURVE_WITH_KNOTS('',3,(#134937,#134938,#134939,#134940,#134941,
#134942),.UNSPECIFIED.,.F.,.F.,(4,2,4),(0.,0.5,1.),.UNSPECIFIED.);
#4242=B_SPLINE_CURVE_WITH_KNOTS('',3,(#134951,#134952,#134953,#134954,#134955,
#134956,#134957,#134958,#134959,#134960),.UNSPECIFIED.,.F.,.F.,(4,2,2,2,
4),(0.,0.249999999999998,0.499999999999999,0.749999999999999,1.),
 .UNSPECIFIED.);
#4243=B_SPLINE_CURVE_WITH_KNOTS('',3,(#134961,#134962,#134963,#134964,#134965,
#134966,#134967,#134968,#134969,#134970),.UNSPECIFIED.,.F.,.F.,(4,2,2,2,
4),(0.,0.250000000000001,0.499999999999998,0.749999999999999,1.),
 .UNSPECIFIED.);
#4244=B_SPLINE_CURVE_WITH_KNOTS('',3,(#134997,#134998,#134999,#135000,#135001,
#135002),.UNSPECIFIED.,.F.,.F.,(4,2,4),(0.,0.5,1.),.UNSPECIFIED.);
#4245=B_SPLINE_CURVE_WITH_KNOTS('',3,(#135029,#135030,#135031,#135032,#135033,
#135034),.UNSPECIFIED.,.F.,.F.,(4,2,4),(0.,0.5,1.),.UNSPECIFIED.);
#4246=B_SPLINE_CURVE_WITH_KNOTS('',3,(#135044,#135045,#135046,#135047,#135048,
#135049,#135050,#135051,#135052,#135053),.UNSPECIFIED.,.F.,.F.,(4,2,2,2,
4),(0.,0.249999999999998,0.499999999999999,0.749999999999999,1.),
 .UNSPECIFIED.);
#4247=B_SPLINE_CURVE_WITH_KNOTS('',3,(#135116,#135117,#135118,#135119),
 .UNSPECIFIED.,.F.,.F.,(4,4),(0.,1.),.UNSPECIFIED.);
#4248=B_SPLINE_CURVE_WITH_KNOTS('',3,(#135122,#135123,#135124,#135125),
 .UNSPECIFIED.,.F.,.F.,(4,4),(0.,0.0331958858056162),.UNSPECIFIED.);
#4249=B_SPLINE_CURVE_WITH_KNOTS('',3,(#135169,#135170,#135171,#135172,#135173,
#135174,#135175,#135176,#135177,#135178,#135179,#135180,#135181,#135182,
#135183,#135184,#135185,#135186,#135187,#135188,#135189,#135190,#135191,
#135192,#135193,#135194,#135195,#135196,#135197,#135198,#135199,#135200,
#135201,#135202,#135203,#135204,#135205,#135206,#135207,#135208),
 .UNSPECIFIED.,.F.,.F.,(4,3,3,3,3,3,3,3,3,3,3,3,3,4),(0.,0.250000000000401,
0.37500000000056,0.437500000000597,0.468750000000618,0.484375000000582,
0.496808957139414,0.500000000000546,0.593872927450488,0.687778494940771,
0.781121765432879,0.873618088950425,0.964138621540856,1.),.UNSPECIFIED.);
#4250=B_SPLINE_CURVE_WITH_KNOTS('',3,(#135226,#135227,#135228,#135229,#135230,
#135231),.UNSPECIFIED.,.F.,.F.,(4,2,4),(0.,0.000500369188755688,0.00100073837751138),
 .UNSPECIFIED.);
#4251=B_SPLINE_CURVE_WITH_KNOTS('',3,(#135250,#135251,#135252,#135253,#135254,
#135255),.UNSPECIFIED.,.F.,.F.,(4,2,4),(0.,0.5,1.),.UNSPECIFIED.);
#4252=B_SPLINE_CURVE_WITH_KNOTS('',3,(#135257,#135258,#135259,#135260,#135261,
#135262),.UNSPECIFIED.,.F.,.F.,(4,2,4),(0.,0.5,1.),.UNSPECIFIED.);
#4253=B_SPLINE_CURVE_WITH_KNOTS('',3,(#135264,#135265,#135266,#135267),
 .UNSPECIFIED.,.F.,.F.,(4,4),(0.,1.),.UNSPECIFIED.);
#4254=B_SPLINE_CURVE_WITH_KNOTS('',3,(#135270,#135271,#135272,#135273,#135274,
#135275,#135276,#135277,#135278,#135279),.UNSPECIFIED.,.F.,.F.,(4,2,2,2,
4),(0.,0.25,0.5,0.75,1.),.UNSPECIFIED.);
#4255=B_SPLINE_CURVE_WITH_KNOTS('',3,(#135325,#135326,#135327,#135328,#135329,
#135330,#135331,#135332,#135333,#135334,#135335,#135336),.UNSPECIFIED.,
 .F.,.F.,(4,2,2,2,2,4),(0.,0.31912132670696,0.47868199006044,0.63824265341392,
0.95736398012088,1.),.UNSPECIFIED.);
#4256=B_SPLINE_CURVE_WITH_KNOTS('',3,(#135339,#135340,#135341,#135342,#135343,
#135344,#135345,#135346,#135347,#135348,#135349,#135350,#135351,#135352,
#135353,#135354,#135355,#135356,#135357,#135358,#135359,#135360,#135361,
#135362,#135363,#135364,#135365,#135366,#135367,#135368,#135369,#135370,
#135371,#135372,#135373,#135374,#135375,#135376,#135377,#135378,#135379,
#135380,#135381),.UNSPECIFIED.,.F.,.F.,(4,3,3,3,3,3,3,3,3,3,3,3,3,3,4),
(4.80131737206195E-10,0.0725092726268684,0.144994898707486,0.21754885026403,
0.250000000000001,0.322952563145093,0.395915689830995,0.468996449355532,
0.500000000000002,0.586371586023873,0.673119802689203,0.760419685943488,
0.847982202568464,0.935943610235565,1.),.UNSPECIFIED.);
#4257=B_SPLINE_CURVE_WITH_KNOTS('',3,(#135439,#135440,#135441,#135442,#135443,
#135444),.UNSPECIFIED.,.F.,.F.,(4,2,4),(0.000562946727309309,0.00236076329038739,
0.00415857985346548),.UNSPECIFIED.);
#4258=B_SPLINE_CURVE_WITH_KNOTS('',3,(#135448,#135449,#135450,#135451,#135452,
#135453),.UNSPECIFIED.,.F.,.F.,(4,2,4),(3.44768074808928E-6,0.516296525972948,
1.),.UNSPECIFIED.);
#4259=B_SPLINE_CURVE_WITH_KNOTS('',3,(#135454,#135455,#135456,#135457,#135458,
#135459,#135460,#135461,#135462,#135463),.UNSPECIFIED.,.F.,.F.,(4,2,2,2,
4),(0.,0.250000000000004,0.500000000000003,0.750000000000001,1.),
 .UNSPECIFIED.);
#4260=B_SPLINE_CURVE_WITH_KNOTS('',3,(#135578,#135579,#135580,#135581,#135582,
#135583,#135584,#135585,#135586,#135587,#135588,#135589,#135590,#135591,
#135592,#135593,#135594,#135595,#135596,#135597,#135598,#135599,#135600,
#135601,#135602,#135603,#135604,#135605,#135606,#135607,#135608),
 .UNSPECIFIED.,.F.,.F.,(4,3,3,3,3,3,3,3,3,3,4),(0.,0.000563737664817631,
0.000564164457966258,0.00104582443004183,0.00112760220035037,0.00112832891593252,
0.00161216721523005,0.00169210723432587,0.00169249337389877,0.00210946737364631,
0.00225665783186503),.UNSPECIFIED.);
#4261=B_SPLINE_CURVE_WITH_KNOTS('',3,(#135615,#135616,#135617,#135618,#135619,
#135620,#135621,#135622,#135623,#135624),.UNSPECIFIED.,.F.,.F.,(4,2,2,2,
4),(0.,0.25,0.499999999999999,0.749999999999998,1.),.UNSPECIFIED.);
#4262=B_SPLINE_CURVE_WITH_KNOTS('',3,(#135738,#135739,#135740,#135741,#135742,
#135743,#135744,#135745,#135746,#135747,#135748,#135749,#135750,#135751,
#135752,#135753,#135754,#135755,#135756,#135757,#135758,#135759,#135760,
#135761,#135762,#135763),.UNSPECIFIED.,.F.,.F.,(4,2,2,2,2,2,2,2,2,2,2,2,
4),(0.,0.0308819193977864,0.0647401130033729,0.0887784724846976,0.122010977791757,
0.141217536873128,0.14606144500119,0.164774918181124,0.172906057212047,
0.180478634267683,0.208285706582933,0.247371596054736,0.282492401339011),
 .UNSPECIFIED.);
#4263=B_SPLINE_CURVE_WITH_KNOTS('',3,(#135772,#135773,#135774,#135775,#135776,
#135777,#135778,#135779,#135780,#135781,#135782,#135783,#135784,#135785,
#135786,#135787,#135788,#135789),.UNSPECIFIED.,.F.,.F.,(4,2,2,2,2,2,2,2,
4),(-0.2325452866513,-0.202278856490703,-0.169720566967503,-0.147070875717209,
-0.116272702466171,-0.0854925566395962,-0.062837160360675,-0.0302640152403312,
0.),.UNSPECIFIED.);
#4264=B_SPLINE_CURVE_WITH_KNOTS('',3,(#135796,#135797,#135798,#135799,#135800,
#135801,#135802,#135803),.UNSPECIFIED.,.F.,.F.,(4,2,2,4),(-0.169530887591468,
-0.138792065251541,-0.106611941486663,-0.0847654430253264),
 .UNSPECIFIED.);
#4265=B_SPLINE_CURVE_WITH_KNOTS('',3,(#135808,#135809,#135810,#135811,#135812,
#135813,#135814,#135815),.UNSPECIFIED.,.F.,.F.,(4,2,2,4),(-0.0847650334136806,
-0.0629270182290063,-0.0307530884809931,0.),.UNSPECIFIED.);
#4266=B_SPLINE_CURVE_WITH_KNOTS('',3,(#135818,#135819,#135820,#135821,#135822,
#135823,#135824,#135825,#135826,#135827,#135828,#135829,#135830,#135831,
#135832,#135833,#135834,#135835),.UNSPECIFIED.,.F.,.F.,(4,2,2,2,2,2,2,2,
4),(-0.232545286657315,-0.202278856495331,-0.169720566970565,-0.14707087571913,
-0.116272702467069,-0.0854925566400001,-0.0628371603609857,-0.030264015240477,
0.),.UNSPECIFIED.);
#4267=B_SPLINE_CURVE_WITH_KNOTS('',3,(#135870,#135871,#135872,#135873,#135874,
#135875,#135876,#135877,#135878,#135879),.UNSPECIFIED.,.F.,.F.,(4,2,2,2,
4),(0.,0.250000000000001,0.5,0.75,1.),.UNSPECIFIED.);
#4268=B_SPLINE_CURVE_WITH_KNOTS('',3,(#135882,#135883,#135884,#135885,#135886,
#135887,#135888,#135889,#135890,#135891,#135892,#135893,#135894,#135895,
#135896,#135897,#135898,#135899,#135900,#135901,#135902,#135903,#135904,
#135905,#135906,#135907,#135908,#135909,#135910,#135911,#135912,#135913,
#135914,#135915,#135916,#135917,#135918,#135919,#135920,#135921,#135922,
#135923,#135924),.UNSPECIFIED.,.F.,.F.,(4,3,3,3,3,3,3,3,3,3,3,3,3,3,4),
(0.,0.000168850029785981,0.000336050047503145,0.000405527490133943,0.000407005029304983,
0.000682198964496424,0.000811826624698267,0.000814010058609966,0.00109897545099435,
0.00121939063721614,0.00122101508791495,0.00134692436003259,0.001471310831548,
0.00159335498692783,0.00162802011721993),.UNSPECIFIED.);
#4269=B_SPLINE_CURVE_WITH_KNOTS('',3,(#135980,#135981,#135982,#135983,#135984,
#135985,#135986,#135987,#135988,#135989,#135990,#135991,#135992,#135993,
#135994,#135995,#135996,#135997,#135998,#135999,#136000,#136001,#136002,
#136003,#136004,#136005,#136006,#136007,#136008,#136009,#136010,#136011,
#136012,#136013,#136014,#136015,#136016),.UNSPECIFIED.,.F.,.F.,(4,3,3,3,
3,3,3,3,3,3,3,3,4),(0.,0.0855690909158042,0.171174585040492,0.25,0.337530389879789,
0.42495453801557,0.5,0.588221947844027,0.676235883140647,0.75,0.834877270845738,
0.919731176821254,1.),.UNSPECIFIED.);
#4270=B_SPLINE_CURVE_WITH_KNOTS('',3,(#136017,#136018,#136019,#136020,#136021,
#136022,#136023,#136024,#136025,#136026,#136027,#136028,#136029,#136030,
#136031,#136032,#136033,#136034,#136035,#136036,#136037,#136038,#136039,
#136040,#136041,#136042,#136043,#136044,#136045,#136046,#136047,#136048,
#136049,#136050,#136051,#136052,#136053,#136054,#136055,#136056,#136057,
#136058,#136059,#136060,#136061,#136062),.UNSPECIFIED.,.F.,.F.,(4,3,3,3,
3,3,3,3,3,3,3,3,3,3,3,4),(0.,0.000111620791367541,0.000225473811195175,
0.000339302579903037,0.000397521249509077,0.000399067370002251,0.00066751766164224,
0.000795042499018153,0.000797178277617397,0.00104506031877337,0.00119256374852723,
0.00119405065366288,0.00132343586690882,0.00145676043247256,0.00158159308775804,
0.0015900849980363),.UNSPECIFIED.);
#4271=B_SPLINE_CURVE_WITH_KNOTS('',3,(#136088,#136089,#136090,#136091,#136092,
#136093),.UNSPECIFIED.,.F.,.F.,(4,2,4),(0.,0.500000000000001,1.),
 .UNSPECIFIED.);
#4272=B_SPLINE_CURVE_WITH_KNOTS('',3,(#136096,#136097,#136098,#136099,#136100,
#136101),.UNSPECIFIED.,.F.,.F.,(4,2,4),(0.,0.499999999999999,1.),
 .UNSPECIFIED.);
#4273=B_SPLINE_CURVE_WITH_KNOTS('',3,(#136151,#136152,#136153,#136154,#136155,
#136156,#136157,#136158),.UNSPECIFIED.,.F.,.F.,(4,2,2,4),(0.,0.499999999999999,
0.75,1.),.UNSPECIFIED.);
#4274=B_SPLINE_CURVE_WITH_KNOTS('',3,(#136159,#136160,#136161,#136162,#136163,
#136164,#136165,#136166),.UNSPECIFIED.,.F.,.F.,(4,2,2,4),(0.,0.25,0.500000000000001,
1.),.UNSPECIFIED.);
#4275=B_SPLINE_CURVE_WITH_KNOTS('',3,(#136215,#136216,#136217,#136218,#136219,
#136220,#136221,#136222,#136223,#136224,#136225,#136226,#136227,#136228,
#136229,#136230,#136231,#136232,#136233,#136234,#136235,#136236,#136237,
#136238,#136239,#136240,#136241,#136242,#136243,#136244,#136245,#136246,
#136247,#136248,#136249,#136250,#136251,#136252,#136253,#136254,#136255,
#136256,#136257,#136258,#136259,#136260,#136261,#136262,#136263,#136264,
#136265,#136266),.UNSPECIFIED.,.F.,.F.,(4,3,3,3,3,3,3,3,3,3,3,3,3,3,3,3,
3,4),(0.,8.48627990059856E-5,0.000110154370857281,0.000197555987869132,
0.00023405941935963,0.000330463112571844,0.000419877362193068,0.000438835738394215,
0.000440617483429125,0.000729065363181661,0.00087889719586762,0.00088123496685825,
0.00114445185849832,0.00132031265264404,0.00132185245028737,0.00147439999768875,
0.00163314747063781,0.0017624699337165),.UNSPECIFIED.);
#4276=B_SPLINE_CURVE_WITH_KNOTS('',3,(#136269,#136270,#136271,#136272,#136273,
#136274,#136275,#136276,#136277,#136278),.UNSPECIFIED.,.F.,.F.,(4,2,2,2,
4),(0.,0.249999999999999,0.5,0.75,1.),.UNSPECIFIED.);
#4277=B_SPLINE_CURVE_WITH_KNOTS('',3,(#136334,#136335,#136336,#136337,#136338,
#136339,#136340,#136341,#136342,#136343,#136344,#136345,#136346,#136347,
#136348,#136349,#136350,#136351,#136352,#136353,#136354,#136355,#136356,
#136357,#136358,#136359,#136360,#136361,#136362,#136363,#136364,#136365,
#136366,#136367,#136368,#136369,#136370,#136371,#136372,#136373,#136374,
#136375,#136376,#136377,#136378,#136379,#136380,#136381,#136382),
 .UNSPECIFIED.,.F.,.F.,(4,3,3,3,3,3,3,3,3,3,3,3,3,3,3,3,4),(0.,0.0694026021440636,
0.139645419416936,0.211930659092264,0.25,0.304387057659765,0.358678892493984,
0.375,0.44229150378928,0.500000000000001,0.574699847176716,0.651271982256802,
0.731430997765807,0.813937157578756,0.900570004879131,0.937863451189354,
1.),.UNSPECIFIED.);
#4278=B_SPLINE_CURVE_WITH_KNOTS('',3,(#136383,#136384,#136385,#136386,#136387,
#136388,#136389,#136390,#136391,#136392),.UNSPECIFIED.,.F.,.F.,(4,2,2,2,
4),(0.,0.499999999999999,0.625,0.75,1.),.UNSPECIFIED.);
#4279=B_SPLINE_CURVE_WITH_KNOTS('',3,(#136398,#136399,#136400,#136401),
 .UNSPECIFIED.,.F.,.F.,(4,4),(0.,1.),.UNSPECIFIED.);
#4280=B_SPLINE_CURVE_WITH_KNOTS('',3,(#136405,#136406,#136407,#136408,#136409,
#136410),.UNSPECIFIED.,.F.,.F.,(4,2,4),(0.,0.5,1.),.UNSPECIFIED.);
#4281=B_SPLINE_CURVE_WITH_KNOTS('',3,(#136427,#136428,#136429,#136430),
 .UNSPECIFIED.,.F.,.F.,(4,4),(0.,1.),.UNSPECIFIED.);
#4282=B_SPLINE_CURVE_WITH_KNOTS('',3,(#136432,#136433,#136434,#136435),
 .UNSPECIFIED.,.F.,.F.,(4,4),(0.,1.),.UNSPECIFIED.);
#4283=B_SPLINE_CURVE_WITH_KNOTS('',3,(#136482,#136483,#136484,#136485,#136486,
#136487,#136488,#136489,#136490,#136491,#136492,#136493,#136494,#136495,
#136496,#136497,#136498,#136499,#136500,#136501,#136502,#136503,#136504,
#136505,#136506,#136507,#136508,#136509),.UNSPECIFIED.,.F.,.F.,(4,3,3,3,
3,3,3,3,3,4),(0.,0.000418680346172109,0.000626513004308685,0.000899330166364171,
0.00105990140469318,0.00112416270795522,0.00125349750883986,0.00134899524954626,
0.00159071512184879,0.00179866033272836),.UNSPECIFIED.);
#4284=B_SPLINE_CURVE_WITH_KNOTS('',3,(#136552,#136553,#136554,#136555,#136556,
#136557,#136558,#136559,#136560,#136561,#136562,#136563,#136564,#136565,
#136566,#136567,#136568,#136569,#136570,#136571,#136572,#136573,#136574,
#136575,#136576,#136577,#136578,#136579,#136580,#136581,#136582,#136583,
#136584,#136585,#136586,#136587,#136588),.UNSPECIFIED.,.F.,.F.,(4,3,3,3,
3,3,3,3,3,3,3,3,4),(0.000628504292635843,0.00064025498632194,0.000837411769726014,
0.000877277691072229,0.00100166439029042,0.00112605108950862,0.0012996740600194,
0.00158178243882745,0.00162359788638139,0.00162947384441178,0.00195921469101129,
0.00212114468325416,0.00261869148012693),.UNSPECIFIED.);
#4285=B_SPLINE_CURVE_WITH_KNOTS('',3,(#136589,#136590,#136591,#136592,#136593,
#136594,#136595,#136596,#136597,#136598,#136599,#136600),.UNSPECIFIED.,
 .F.,.F.,(4,2,2,2,2,4),(0.,0.251509454663243,0.377264181994864,0.503018909326486,
0.754528363989729,1.),.UNSPECIFIED.);
#4286=B_SPLINE_CURVE_WITH_KNOTS('',3,(#136637,#136638,#136639,#136640,#136641,
#136642,#136643),.UNSPECIFIED.,.F.,.F.,(4,3,4),(0.,0.490447172337672,1.),
 .UNSPECIFIED.);
#4287=B_SPLINE_CURVE_WITH_KNOTS('',3,(#136644,#136645,#136646,#136647,#136648,
#136649,#136650,#136651,#136652,#136653,#136654,#136655),.UNSPECIFIED.,
 .F.,.F.,(4,2,3,3,4),(0.,0.00100000000000032,0.00500000000004302,0.0210000000041071,
0.0383173498474262),.UNSPECIFIED.);
#4288=B_SPLINE_CURVE_WITH_KNOTS('',3,(#136656,#136657,#136658,#136659),
 .UNSPECIFIED.,.F.,.F.,(4,4),(0.,1.),.UNSPECIFIED.);
#4289=B_SPLINE_CURVE_WITH_KNOTS('',3,(#136677,#136678,#136679,#136680,#136681,
#136682,#136683,#136684,#136685,#136686,#136687,#136688,#136689,#136690,
#136691,#136692,#136693,#136694,#136695,#136696,#136697,#136698,#136699,
#136700,#136701,#136702,#136703,#136704,#136705,#136706,#136707,#136708,
#136709,#136710,#136711,#136712,#136713),.UNSPECIFIED.,.F.,.F.,(4,3,3,3,
3,3,3,3,3,3,3,3,4),(0.,0.000308449407263107,0.000616898814526214,0.000757033039934092,
0.00113555144207261,0.00123379762905243,0.00151396810348857,0.00181929544894823,
0.00185069644357864,0.00189260692917409,0.00221146178004248,0.00227133710209361,
0.00246759525810486),.UNSPECIFIED.);
#4290=B_SPLINE_CURVE_WITH_KNOTS('',3,(#136716,#136717,#136718,#136719,#136720,
#136721,#136722,#136723,#136724,#136725,#136726,#136727,#136728,#136729,
#136730,#136731,#136732,#136733,#136734,#136735,#136736,#136737,#136738,
#136739,#136740,#136741,#136742,#136743,#136744,#136745,#136746,#136747,
#136748,#136749,#136750,#136751,#136752),.UNSPECIFIED.,.F.,.F.,(4,3,3,3,
3,3,3,3,3,3,3,3,4),(0.00064734234469968,0.000773679728910249,0.000794515777305426,
0.00111794174210909,0.00114512410810862,0.00123603607512266,0.00151649021309283,
0.00182472980554565,0.00188790100005034,0.00225930818373534,0.00241342353596863,
0.00270777040118012,0.00300211726639161),.UNSPECIFIED.);
#4291=B_SPLINE_CURVE_WITH_KNOTS('',3,(#136761,#136762,#136763,#136764,#136765,
#136766,#136767,#136768,#136769,#136770,#136771,#136772,#136773),
 .UNSPECIFIED.,.F.,.F.,(4,3,3,3,4),(0.,0.000680510137073302,0.00109976462606963,
0.002047167230467,0.00219952925213926),.UNSPECIFIED.);
#4292=B_SPLINE_CURVE_WITH_KNOTS('',3,(#136777,#136778,#136779,#136780,#136781,
#136782,#136783,#136784,#136785,#136786,#136787,#136788,#136789),
 .UNSPECIFIED.,.F.,.F.,(4,3,3,3,4),(0.,0.000627390790128563,0.00109987581267579,
0.00205656007244151,0.00219975162535158),.UNSPECIFIED.);
#4293=B_SPLINE_CURVE_WITH_KNOTS('',3,(#136865,#136866,#136867,#136868,#136869,
#136870,#136871,#136872,#136873,#136874,#136875,#136876),.UNSPECIFIED.,
 .F.,.F.,(4,2,2,2,2,4),(0.,0.253338275236372,0.506676550472745,0.633345688090933,
0.76001482570911,1.),.UNSPECIFIED.);
#4294=B_SPLINE_CURVE_WITH_KNOTS('',3,(#136877,#136878,#136879,#136880),
 .UNSPECIFIED.,.F.,.F.,(4,4),(0.0037358385977583,0.00423610566507283),
 .UNSPECIFIED.);
#4295=B_SPLINE_CURVE_WITH_KNOTS('',3,(#136918,#136919,#136920,#136921,#136922,
#136923,#136924,#136925,#136926,#136927,#136928,#136929,#136930,#136931,
#136932,#136933,#136934,#136935,#136936,#136937,#136938,#136939,#136940,
#136941,#136942,#136943,#136944,#136945,#136946,#136947,#136948,#136949,
#136950,#136951,#136952,#136953,#136954,#136955,#136956,#136957,#136958,
#136959,#136960,#136961,#136962,#136963),.UNSPECIFIED.,.F.,.F.,(4,3,3,3,
3,3,3,3,3,3,3,3,3,3,3,4),(0.000450499470650019,0.00054011395429817,0.000798583304346381,
0.000986883024373906,0.00116741533983523,0.00137527276208873,0.00169825994125939,
0.00176385446568028,0.00188433120902044,0.00210726599697033,0.00224278914361301,
0.00241357708828729,0.00254109024997701,0.0026012470782056,0.00316630230566398,
0.00331816294739075),.UNSPECIFIED.);
#4296=B_SPLINE_CURVE_WITH_KNOTS('',3,(#136982,#136983,#136984,#136985,#136986,
#136987,#136988,#136989,#136990,#136991,#136992,#136993,#136994,#136995,
#136996,#136997,#136998,#136999,#137000,#137001,#137002,#137003,#137004,
#137005,#137006,#137007,#137008,#137009,#137010,#137011,#137012,#137013,
#137014,#137015,#137016,#137017,#137018,#137019,#137020,#137021,#137022,
#137023,#137024,#137025,#137026,#137027,#137028,#137029,#137030),
 .UNSPECIFIED.,.F.,.F.,(4,3,3,3,3,3,3,3,3,3,3,3,3,3,3,3,4),(0.,0.000568992160114069,
0.000684369961878612,0.000753736971436074,0.000939442240058873,0.00102655494281796,
0.00113065957381952,0.00136873992375731,0.00150755451437509,0.00188444398402291,
0.00205310988563609,0.00222420237610578,0.002260801563485,0.00235252174395805,
0.00254500079573646,0.00264124032162566,0.00273747984751486),
 .UNSPECIFIED.);
#4297=B_SPLINE_CURVE_WITH_KNOTS('',3,(#137038,#137039,#137040,#137041,#137042,
#137043,#137044,#137045,#137046,#137047,#137048,#137049,#137050),
 .UNSPECIFIED.,.F.,.F.,(4,3,3,3,4),(0.,0.000962747670576822,0.00119082241359643,
0.00216097007597471,0.00238164482719285),.UNSPECIFIED.);
#4298=B_SPLINE_CURVE_WITH_KNOTS('',3,(#137054,#137055,#137056,#137057,#137058,
#137059,#137060,#137061,#137062,#137063,#137064,#137065,#137066),
 .UNSPECIFIED.,.F.,.F.,(4,3,3,3,4),(0.,0.000775847435672983,0.00119114916434495,
0.00218083968926337,0.00238229832868991),.UNSPECIFIED.);
#4299=B_SPLINE_CURVE_WITH_KNOTS('',3,(#137076,#137077,#137078,#137079,#137080,
#137081),.UNSPECIFIED.,.F.,.F.,(4,2,4),(0.,0.432355968717148,1.),
 .UNSPECIFIED.);
#4300=B_SPLINE_CURVE_WITH_KNOTS('',3,(#137086,#137087,#137088,#137089),
 .UNSPECIFIED.,.F.,.F.,(4,4),(0.,1.),.UNSPECIFIED.);
#4301=B_SPLINE_CURVE_WITH_KNOTS('',3,(#137118,#137119,#137120,#137121),
 .UNSPECIFIED.,.F.,.F.,(4,4),(0.,0.0322629186945109),.UNSPECIFIED.);
#4302=B_SPLINE_CURVE_WITH_KNOTS('',3,(#137123,#137124,#137125,#137126,#137127,
#137128,#137129,#137130,#137131,#137132,#137133,#137134,#137135,#137136,
#137137,#137138),.UNSPECIFIED.,.F.,.F.,(4,3,3,3,3,4),(0.,0.000549388570662942,
0.00110809797239399,0.00147175517552831,0.00249356706682249,0.00294351035105662),
 .UNSPECIFIED.);
#4303=B_SPLINE_CURVE_WITH_KNOTS('',3,(#137142,#137143,#137144,#137145,#137146,
#137147,#137148,#137149,#137150,#137151,#137152,#137153,#137154),
 .UNSPECIFIED.,.F.,.F.,(4,3,3,3,4),(0.,0.000882415156994226,0.00147346850157273,
0.00255877694108978,0.00294693700314546),.UNSPECIFIED.);
#4304=B_SPLINE_CURVE_WITH_KNOTS('',3,(#137155,#137156,#137157,#137158),
 .UNSPECIFIED.,.F.,.F.,(4,4),(0.,0.0319950621716304),.UNSPECIFIED.);
#4305=B_SPLINE_CURVE_WITH_KNOTS('',3,(#137195,#137196,#137197,#137198),
 .UNSPECIFIED.,.F.,.F.,(4,4),(0.,0.0298008594779328),.UNSPECIFIED.);
#4306=B_SPLINE_CURVE_WITH_KNOTS('',3,(#137200,#137201,#137202,#137203,#137204,
#137205,#137206,#137207,#137208,#137209,#137210,#137211,#137212,#137213,
#137214,#137215),.UNSPECIFIED.,.F.,.F.,(4,3,3,3,3,4),(0.,0.000531847314911702,
0.00107596315612957,0.00162007899734744,0.00266000146298276,0.00324015799469487),
 .UNSPECIFIED.);
#4307=B_SPLINE_CURVE_WITH_KNOTS('',3,(#137219,#137220,#137221,#137222,#137223,
#137224,#137225,#137226,#137227,#137228,#137229,#137230,#137231),
 .UNSPECIFIED.,.F.,.F.,(4,3,3,3,4),(0.,0.000817558298561711,0.00162295210526764,
0.00275577655347827,0.00324590421053527),.UNSPECIFIED.);
#4308=B_SPLINE_CURVE_WITH_KNOTS('',3,(#137233,#137234,#137235,#137236),
 .UNSPECIFIED.,.F.,.F.,(4,4),(0.,0.0300693678107436),.UNSPECIFIED.);
#4309=B_SPLINE_CURVE_WITH_KNOTS('',3,(#137241,#137242,#137243,#137244,#137245,
#137246,#137247),.UNSPECIFIED.,.F.,.F.,(4,3,4),(6.08671444000369E-7,0.379970146635923,
1.),.UNSPECIFIED.);
#4310=B_SPLINE_CURVE_WITH_KNOTS('',3,(#137252,#137253,#137254,#137255),
 .UNSPECIFIED.,.F.,.F.,(4,4),(0.,1.),.UNSPECIFIED.);
#4311=B_SPLINE_CURVE_WITH_KNOTS('',3,(#137284,#137285,#137286,#137287),
 .UNSPECIFIED.,.F.,.F.,(4,4),(0.,0.0240963563036403),.UNSPECIFIED.);
#4312=B_SPLINE_CURVE_WITH_KNOTS('',3,(#137289,#137290,#137291,#137292,#137293,
#137294,#137295,#137296,#137297,#137298,#137299,#137300,#137301,#137302,
#137303,#137304,#137305,#137306,#137307,#137308,#137309,#137310,#137311,
#137312,#137313),.UNSPECIFIED.,.F.,.F.,(4,3,3,3,3,3,3,3,4),(0.,0.000403252952291635,
0.000810273659956253,0.000991778862067342,0.0014336523721451,0.00187173698199313,
0.00198355772413468,0.00304641612721467,0.00396711544826929),
 .UNSPECIFIED.);
#4313=B_SPLINE_CURVE_WITH_KNOTS('',3,(#137317,#137318,#137319,#137320,#137321,
#137322,#137323,#137324,#137325,#137326,#137327,#137328,#137329,#137330,
#137331,#137332,#137333,#137334,#137335),.UNSPECIFIED.,.F.,.F.,(4,3,3,3,
3,3,4),(0.,0.000606703134123721,0.00123626357061692,0.00189155006086011,
0.00198795077588647,0.00324033736596706,0.00397590155177294),
 .UNSPECIFIED.);
#4314=B_SPLINE_CURVE_WITH_KNOTS('',3,(#137336,#137337,#137338,#137339),
 .UNSPECIFIED.,.F.,.F.,(4,4),(0.,0.0238258198664154),.UNSPECIFIED.);
#4315=B_SPLINE_CURVE_WITH_KNOTS('',3,(#137346,#137347,#137348,#137349,#137350,
#137351,#137352,#137353),.UNSPECIFIED.,.F.,.F.,(4,2,2,4),(0.,0.5,0.749999999999999,
1.),.UNSPECIFIED.);
#4316=B_SPLINE_CURVE_WITH_KNOTS('',3,(#137381,#137382,#137383,#137384,#137385,
#137386,#137387,#137388,#137389,#137390,#137391,#137392,#137393,#137394,
#137395,#137396),.UNSPECIFIED.,.F.,.F.,(4,3,3,3,3,4),(0.,0.000625284942165436,
0.00128905281997377,0.00194949793575932,0.00318811191752659,0.00389899587151865),
 .UNSPECIFIED.);
#4317=B_SPLINE_CURVE_WITH_KNOTS('',3,(#137398,#137399,#137400,#137401),
 .UNSPECIFIED.,.F.,.F.,(4,4),(0.,0.024690830875569),.UNSPECIFIED.);
#4318=B_SPLINE_CURVE_WITH_KNOTS('',3,(#137419,#137420,#137421,#137422),
 .UNSPECIFIED.,.F.,.F.,(4,4),(0.,0.0278605201857756),.UNSPECIFIED.);
#4319=B_SPLINE_CURVE_WITH_KNOTS('',3,(#137424,#137425,#137426,#137427,#137428,
#137429,#137430,#137431),.UNSPECIFIED.,.F.,.F.,(4,2,2,4),(0.,0.000890496769046365,
0.00178099353809273,0.0035619870761855),.UNSPECIFIED.);
#4320=B_SPLINE_CURVE_WITH_KNOTS('',3,(#137454,#137455,#137456,#137457,#137458,
#137459),.UNSPECIFIED.,.F.,.F.,(4,2,4),(0.,0.50310275859516,1.),
 .UNSPECIFIED.);
#4321=B_SPLINE_CURVE_WITH_KNOTS('',3,(#137460,#137461,#137462,#137463),
 .UNSPECIFIED.,.F.,.F.,(4,4),(0.,1.),.UNSPECIFIED.);
#4322=B_SPLINE_CURVE_WITH_KNOTS('',3,(#137485,#137486,#137487,#137488,#137489,
#137490,#137491,#137492,#137493,#137494,#137495,#137496,#137497,#137498,
#137499,#137500,#137501,#137502,#137503,#137504,#137505,#137506,#137507,
#137508,#137509,#137510,#137511,#137512,#137513,#137514,#137515,#137516,
#137517,#137518,#137519,#137520,#137521,#137522,#137523,#137524,#137525,
#137526,#137527,#137528,#137529,#137530,#137531,#137532,#137533,#137534,
#137535,#137536,#137537,#137538,#137539,#137540,#137541,#137542,#137543,
#137544,#137545,#137546,#137547,#137548),.UNSPECIFIED.,.F.,.F.,(4,3,3,3,
3,3,3,3,3,3,3,3,3,3,3,3,3,3,3,3,3,4),(0.,0.00024394307186977,0.000489165049879305,
0.000733924827046494,0.000899069239743237,0.000911316177023075,0.00119563029973435,
0.00134860385961487,0.00136698289390588,0.00175854423315568,0.0017981384794865,
0.00182264071786975,0.00224767309935813,0.00227830273883051,0.0025704401924202,
0.00269720771922976,0.00273398747333099,0.00295810023175185,0.0031467423391014,
0.00331012937356541,0.003472902617082,0.00359627695897302),
 .UNSPECIFIED.);
#4323=B_SPLINE_CURVE_WITH_KNOTS('',3,(#137553,#137554,#137555,#137556,#137557,
#137558,#137559,#137560,#137561,#137562,#137563,#137564,#137565,#137566,
#137567,#137568,#137569,#137570,#137571,#137572,#137573,#137574,#137575,
#137576,#137577,#137578,#137579,#137580,#137581,#137582,#137583,#137584,
#137585,#137586),.UNSPECIFIED.,.F.,.F.,(4,3,3,3,3,3,3,3,3,3,3,4),(0.,0.000121613272085654,
0.000230848939029442,0.000231076761054257,0.000462001643661034,0.000462153522108514,
0.000693154344712357,0.000693230283162771,0.000767002378129216,0.00084153649830509,
0.000913992773638304,0.000924307044217028),.UNSPECIFIED.);
#4324=B_SPLINE_CURVE_WITH_KNOTS('',3,(#137588,#137589,#137590,#137591),
 .UNSPECIFIED.,.F.,.F.,(4,4),(0.,9.64176041888327E-5),.UNSPECIFIED.);
#4325=B_SPLINE_CURVE_WITH_KNOTS('',3,(#137592,#137593,#137594,#137595),
 .UNSPECIFIED.,.F.,.F.,(4,4),(0.,0.0333345873458536),.UNSPECIFIED.);
#4326=B_SPLINE_CURVE_WITH_KNOTS('',3,(#137639,#137640,#137641,#137642,#137643,
#137644,#137645,#137646,#137647,#137648,#137649,#137650,#137651,#137652),
 .UNSPECIFIED.,.F.,.F.,(4,2,2,2,2,2,4),(0.,0.222921495031895,0.352434579193248,
0.481947663354594,0.611460747515947,0.740973831677298,1.),.UNSPECIFIED.);
#4327=B_SPLINE_CURVE_WITH_KNOTS('',3,(#137667,#137668,#137669,#137670,#137671,
#137672,#137673,#137674,#137675,#137676,#137677,#137678),.UNSPECIFIED.,
 .F.,.F.,(4,2,2,2,2,4),(0.,0.251487957710783,0.502975915421567,0.628719894276953,
0.754463873132351,1.),.UNSPECIFIED.);
#4328=B_SPLINE_CURVE_WITH_KNOTS('',3,(#137717,#137718,#137719,#137720,#137721,
#137722,#137723,#137724,#137725,#137726,#137727,#137728,#137729,#137730,
#137731,#137732,#137733,#137734,#137735,#137736,#137737,#137738,#137739,
#137740,#137741,#137742,#137743,#137744,#137745,#137746,#137747,#137748,
#137749,#137750,#137751,#137752,#137753,#137754,#137755,#137756,#137757,
#137758,#137759,#137760,#137761,#137762,#137763,#137764,#137765,#137766,
#137767,#137768,#137769,#137770,#137771,#137772,#137773,#137774,#137775,
#137776,#137777),.UNSPECIFIED.,.F.,.F.,(4,3,3,3,3,3,3,3,3,3,3,3,3,3,3,3,
3,3,3,3,4),(0.000632518815593833,0.000932214526663858,0.00101585454476649,
0.00107182189614632,0.00126737972551736,0.00139919027393915,0.00150973846725992,
0.00175129113716284,0.0017825260031118,0.00194741404639006,0.00209785990015682,
0.00215891919163232,0.00222254437895217,0.00246825757120489,0.00254919746145711,
0.00271487168756755,0.00282308344954008,0.00293253319062976,0.00318749230619625,
0.00344334847758565,0.00369920464897506),.UNSPECIFIED.);
#4329=B_SPLINE_CURVE_WITH_KNOTS('',3,(#137796,#137797,#137798,#137799),
 .UNSPECIFIED.,.F.,.F.,(4,4),(3.46944695195361E-18,0.0333425790106738),
 .UNSPECIFIED.);
#4330=B_SPLINE_CURVE_WITH_KNOTS('',3,(#137800,#137801,#137802,#137803,#137804,
#137805,#137806,#137807,#137808,#137809,#137810,#137811,#137812,#137813,
#137814,#137815,#137816,#137817,#137818,#137819,#137820,#137821,#137822,
#137823,#137824,#137825,#137826,#137827,#137828,#137829,#137830,#137831,
#137832,#137833),.UNSPECIFIED.,.F.,.F.,(4,3,3,3,3,3,3,3,3,3,3,4),(0.,7.30072795026687E-5,
0.000147770013513677,0.000221881916258645,0.000252597382995535,0.00050519476599107,
0.000631493458785095,0.000757792148986605,0.000834383528242275,0.000911454457737675,
0.000985554988538247,0.00101038953198214),.UNSPECIFIED.);
#4331=B_SPLINE_CURVE_WITH_KNOTS('',3,(#137836,#137837,#137838,#137839),
 .UNSPECIFIED.,.F.,.F.,(4,4),(0.,1.),.UNSPECIFIED.);
#4332=B_SPLINE_CURVE_WITH_KNOTS('',3,(#137840,#137841,#137842,#137843),
 .UNSPECIFIED.,.F.,.F.,(4,4),(0.,1.),.UNSPECIFIED.);
#4333=B_SPLINE_CURVE_WITH_KNOTS('',3,(#137861,#137862,#137863,#137864,#137865,
#137866,#137867,#137868,#137869,#137870,#137871,#137872,#137873,#137874,
#137875,#137876,#137877,#137878,#137879,#137880,#137881,#137882,#137883,
#137884,#137885,#137886,#137887,#137888,#137889,#137890,#137891),
 .UNSPECIFIED.,.F.,.F.,(4,3,3,3,3,3,3,3,3,3,4),(0.,0.000497569400086742,
0.000640953038946951,0.00096143126389141,0.000995138800173484,0.00128203532234786,
0.00149270820026023,0.00161710055028191,0.00180479162331791,0.00192302626316565,
0.00199027760034697),.UNSPECIFIED.);
#4334=B_SPLINE_CURVE_WITH_KNOTS('',3,(#137894,#137895,#137896,#137897,#137898,
#137899),.UNSPECIFIED.,.F.,.F.,(4,2,4),(0.,0.000501785580775435,0.00100357116155087),
 .UNSPECIFIED.);
#4335=B_SPLINE_CURVE_WITH_KNOTS('',3,(#137967,#137968,#137969,#137970,#137971,
#137972,#137973,#137974,#137975,#137976),.UNSPECIFIED.,.F.,.F.,(4,2,2,2,
4),(0.,0.25149977741346,0.502999554826924,0.754499332240389,1.),
 .UNSPECIFIED.);
#4336=B_SPLINE_CURVE_WITH_KNOTS('',3,(#137977,#137978,#137979,#137980),
 .UNSPECIFIED.,.F.,.F.,(4,4),(0.0171576436379621,0.0176580988602617),
 .UNSPECIFIED.);
#4337=B_SPLINE_CURVE_WITH_KNOTS('',3,(#138012,#138013,#138014,#138015,#138016,
#138017,#138018,#138019,#138020,#138021,#138022,#138023,#138024,#138025,
#138026,#138027,#138028,#138029,#138030,#138031,#138032,#138033,#138034,
#138035,#138036,#138037,#138038,#138039),.UNSPECIFIED.,.F.,.F.,(4,3,3,3,
3,3,3,3,3,4),(0.000712605368931889,0.00092646187873443,0.00114426125513566,
0.00117428487373109,0.00139094819074949,0.00157723429047313,0.00180778147057016,
0.0020948168670341,0.00237995362541881,0.00244186321201438),
 .UNSPECIFIED.);
#4338=B_SPLINE_CURVE_WITH_KNOTS('',3,(#138083,#138084,#138085,#138086,#138087,
#138088,#138089),.UNSPECIFIED.,.F.,.F.,(4,3,4),(0.,0.014563917689728,0.029127835379456),
 .UNSPECIFIED.);
#4339=B_SPLINE_CURVE_WITH_KNOTS('',3,(#138091,#138092,#138093,#138094,#138095,
#138096,#138097,#138098,#138099,#138100,#138101,#138102,#138103,#138104,
#138105,#138106,#138107,#138108,#138109,#138110,#138111,#138112,#138113,
#138114,#138115),.UNSPECIFIED.,.F.,.F.,(4,3,3,3,3,3,3,3,4),(0.,0.000422069097418792,
0.000847931637830459,0.00104448509574678,0.00149181651230618,0.00193535496126664,
0.00208897019149356,0.00315378543073329,0.00417794038298713),
 .UNSPECIFIED.);
#4340=B_SPLINE_CURVE_WITH_KNOTS('',3,(#138119,#138120,#138121,#138122,#138123,
#138124,#138125,#138126,#138127,#138128,#138129,#138130,#138131,#138132,
#138133,#138134,#138135,#138136,#138137,#138138,#138139,#138140),
 .UNSPECIFIED.,.F.,.F.,(4,3,3,3,3,3,3,4),(0.,0.000384591749546137,0.00078374926264035,
0.00104647183020208,0.00173887398624976,0.00209294366040415,0.00337921840659428,
0.00418588732080839),.UNSPECIFIED.);
#4341=B_SPLINE_CURVE_WITH_KNOTS('',3,(#138142,#138143,#138144,#138145,#138146,
#138147,#138148),.UNSPECIFIED.,.F.,.F.,(4,3,4),(0.,0.0146992078328598,0.0293984156657196),
 .UNSPECIFIED.);
#4342=B_SPLINE_CURVE_WITH_KNOTS('',3,(#138168,#138169,#138170,#138171,#138172,
#138173,#138174),.UNSPECIFIED.,.F.,.F.,(4,3,4),(0.,0.626599975159676,0.999999250966931),
 .UNSPECIFIED.);
#4343=B_SPLINE_CURVE_WITH_KNOTS('',3,(#138181,#138182,#138183,#138184,#138185,
#138186),.UNSPECIFIED.,.F.,.F.,(4,2,4),(0.,0.5,1.),.UNSPECIFIED.);
#4344=B_SPLINE_CURVE_WITH_KNOTS('',3,(#138218,#138219,#138220,#138221,#138222,
#138223,#138224),.UNSPECIFIED.,.F.,.F.,(4,3,4),(0.,0.0178323395635859,0.0356646791271718),
 .UNSPECIFIED.);
#4345=B_SPLINE_CURVE_WITH_KNOTS('',3,(#138226,#138227,#138228,#138229,#138230,
#138231,#138232,#138233),.UNSPECIFIED.,.F.,.F.,(4,2,2,4),(0.,0.000848531500815463,
0.00169706300163092,0.00339412600326177),.UNSPECIFIED.);
#4346=B_SPLINE_CURVE_WITH_KNOTS('',3,(#138237,#138238,#138239,#138240,#138241,
#138242,#138243,#138244,#138245,#138246,#138247,#138248,#138249,#138250,
#138251,#138252),.UNSPECIFIED.,.F.,.F.,(4,3,3,3,3,4),(0.,0.000761157739919989,
0.00156083390161768,0.00170051723463269,0.00285526923553587,0.00340103446926538),
 .UNSPECIFIED.);
#4347=B_SPLINE_CURVE_WITH_KNOTS('',3,(#138253,#138254,#138255,#138256,#138257,
#138258,#138259),.UNSPECIFIED.,.F.,.F.,(4,3,4),(0.,0.0176980703187956,0.0353961406375911),
 .UNSPECIFIED.);
#4348=B_SPLINE_CURVE_WITH_KNOTS('',3,(#138289,#138290,#138291,#138292,#138293,
#138294,#138295),.UNSPECIFIED.,.F.,.F.,(4,3,4),(0.,0.0188568492058762,0.0377136984117524),
 .UNSPECIFIED.);
#4349=B_SPLINE_CURVE_WITH_KNOTS('',3,(#138297,#138298,#138299,#138300,#138301,
#138302,#138303,#138304,#138305,#138306,#138307,#138308,#138309,#138310,
#138311,#138312),.UNSPECIFIED.,.F.,.F.,(4,3,3,3,3,4),(0.,0.000540889688193241,
0.00109121002634586,0.00153442409609832,0.00256481294069221,0.00306884819219665),
 .UNSPECIFIED.);
#4350=B_SPLINE_CURVE_WITH_KNOTS('',3,(#138316,#138317,#138318,#138319,#138320,
#138321,#138322,#138323,#138324,#138325,#138326,#138327,#138328),
 .UNSPECIFIED.,.F.,.F.,(4,3,3,3,4),(2.8609792490764E-17,0.000811916222427858,
0.00153648298481487,0.00264039900673925,0.0030729659696297),
 .UNSPECIFIED.);
#4351=B_SPLINE_CURVE_WITH_KNOTS('',3,(#138330,#138331,#138332,#138333,#138334,
#138335,#138336),.UNSPECIFIED.,.F.,.F.,(4,3,4),(0.,0.018990790064314,0.0379815801286281),
 .UNSPECIFIED.);
#4352=B_SPLINE_CURVE_WITH_KNOTS('',3,(#138349,#138350,#138351,#138352,#138353,
#138354,#138355,#138356,#138357,#138358),.UNSPECIFIED.,.F.,.F.,(4,3,3,4),
(0.,0.282541552346412,0.571946461065579,0.999999565238375),
 .UNSPECIFIED.);
#4353=B_SPLINE_CURVE_WITH_KNOTS('',3,(#138359,#138360,#138361,#138362,#138363,
#138364),.UNSPECIFIED.,.F.,.F.,(4,2,4),(0.,0.500000000000001,1.),
 .UNSPECIFIED.);
#4354=B_SPLINE_CURVE_WITH_KNOTS('',3,(#138386,#138387,#138388,#138389,#138390,
#138391,#138392,#138393,#138394,#138395,#138396,#138397,#138398,#138399,
#138400,#138401,#138402,#138403,#138404,#138405,#138406,#138407,#138408,
#138409,#138410,#138411,#138412,#138413,#138414,#138415,#138416,#138417,
#138418,#138419,#138420,#138421,#138422,#138423,#138424,#138425,#138426,
#138427,#138428,#138429,#138430,#138431,#138432,#138433,#138434,#138435,
#138436,#138437),.UNSPECIFIED.,.F.,.F.,(4,3,3,3,3,3,3,3,3,3,3,3,3,3,3,3,
3,4),(0.,0.000568167570465986,0.000689873068221808,0.000757350079825038,
0.000945020241884818,0.00103480960233271,0.0011360777163446,0.00136729697222306,
0.00137974613644361,0.00151477367390368,0.00189346791975904,0.0020696192046654,
0.00221265318267551,0.00227165379781723,0.00237143867201243,0.00256546547244981,
0.0026624788726685,0.00275949227288719),.UNSPECIFIED.);
#4355=B_SPLINE_CURVE_WITH_KNOTS('',3,(#138441,#138442,#138443,#138444,#138445,
#138446,#138447,#138448,#138449,#138450,#138451,#138452,#138453,#138454,
#138455,#138456,#138457,#138458,#138459,#138460,#138461,#138462,#138463,
#138464,#138465,#138466,#138467,#138468,#138469,#138470,#138471,#138472,
#138473,#138474,#138475,#138476,#138477),.UNSPECIFIED.,.F.,.F.,(4,3,3,3,
3,3,3,3,3,3,3,3,4),(0.000467059137334316,0.000632797502959653,0.000860961305648091,
0.000897131574002758,0.00113001259983567,0.00126720169019544,0.00163753656891932,
0.00179296606233701,0.00200786773946722,0.00237820352986643,0.00245591952483837,
0.00301621129961807,0.00311887298733972),.UNSPECIFIED.);
#4356=B_SPLINE_CURVE_WITH_KNOTS('',3,(#138483,#138484,#138485,#138486),
 .UNSPECIFIED.,.F.,.F.,(4,4),(0.,0.0420570108120997),.UNSPECIFIED.);
#4357=B_SPLINE_CURVE_WITH_KNOTS('',3,(#138488,#138489,#138490,#138491,#138492,
#138493,#138494,#138495,#138496,#138497,#138498,#138499,#138500),
 .UNSPECIFIED.,.F.,.F.,(4,3,3,3,4),(0.,0.000795137544056449,0.00122134837748785,
0.00219865189863128,0.0024426967549757),.UNSPECIFIED.);
#4358=B_SPLINE_CURVE_WITH_KNOTS('',3,(#138504,#138505,#138506,#138507,#138508,
#138509,#138510,#138511,#138512,#138513,#138514,#138515,#138516),
 .UNSPECIFIED.,.F.,.F.,(4,3,3,3,4),(0.,0.00089438056074498,0.00122171954771057,
0.00222146414309878,0.00244343909542114),.UNSPECIFIED.);
#4359=B_SPLINE_CURVE_WITH_KNOTS('',3,(#138517,#138518,#138519,#138520),
 .UNSPECIFIED.,.F.,.F.,(4,4),(0.,0.0417901757617078),.UNSPECIFIED.);
#4360=B_SPLINE_CURVE_WITH_KNOTS('',3,(#138564,#138565,#138566,#138567,#138568,
#138569,#138570,#138571,#138572,#138573,#138574,#138575,#138576,#138577),
 .UNSPECIFIED.,.F.,.F.,(4,2,2,2,2,2,4),(0.,0.240255593310268,0.366879661091889,
0.493503728873512,0.620127796655135,0.746751864436756,1.),.UNSPECIFIED.);
#4361=B_SPLINE_CURVE_WITH_KNOTS('',3,(#138592,#138593,#138594,#138595,#138596,
#138597,#138598,#138599,#138600,#138601,#138602,#138603,#138604,#138605),
 .UNSPECIFIED.,.F.,.F.,(4,2,2,2,2,2,4),(0.,0.251506213404696,0.377259320107042,
0.503012426809389,0.628765533511738,0.754518640214088,1.),.UNSPECIFIED.);
#4362=B_SPLINE_CURVE_WITH_KNOTS('',3,(#138606,#138607,#138608,#138609),
 .UNSPECIFIED.,.F.,.F.,(4,4),(0.0206793054465132,0.021179777605653),
 .UNSPECIFIED.);
#4363=B_SPLINE_CURVE_WITH_KNOTS('',3,(#138653,#138654,#138655,#138656,#138657,
#138658,#138659,#138660,#138661,#138662,#138663,#138664,#138665,#138666,
#138667,#138668,#138669,#138670,#138671,#138672,#138673,#138674,#138675,
#138676,#138677,#138678,#138679,#138680,#138681,#138682,#138683,#138684,
#138685,#138686,#138687,#138688,#138689),.UNSPECIFIED.,.F.,.F.,(4,3,3,3,
3,3,3,3,3,3,3,3,4),(0.000646102271931852,0.000780355288939442,0.000794331971528649,
0.00113223030154688,0.00115328378670241,0.00123902107032975,0.00152620034295103,
0.00183193986873122,0.00189906794388762,0.00227197283133226,0.00242485866713269,
0.00272131806633342,0.00301777746553416),.UNSPECIFIED.);
#4364=B_SPLINE_CURVE_WITH_KNOTS('',3,(#138709,#138710,#138711,#138712,#138713,
#138714,#138715,#138716,#138717,#138718,#138719,#138720,#138721,#138722,
#138723,#138724,#138725,#138726,#138727,#138728,#138729,#138730,#138731,
#138732,#138733,#138734,#138735,#138736,#138737,#138738,#138739,#138740,
#138741,#138742),.UNSPECIFIED.,.F.,.F.,(4,3,3,3,3,3,3,3,3,3,3,4),(0.,0.000275770613304119,
0.000551541226608238,0.000716520337534463,0.00107478390778079,0.00110308245321648,
0.00134771653693895,0.00143334685918384,0.00165462367982471,0.00179132390797124,
0.00214954043896842,0.00220616490643295),.UNSPECIFIED.);
#4365=B_SPLINE_CURVE_WITH_KNOTS('',3,(#138750,#138751,#138752,#138753,#138754,
#138755,#138756,#138757,#138758,#138759,#138760,#138761,#138762),
 .UNSPECIFIED.,.F.,.F.,(4,3,3,3,4),(0.,0.000727903814955585,0.00111811425806593,
0.00207062545858955,0.00223622851613186),.UNSPECIFIED.);
#4366=B_SPLINE_CURVE_WITH_KNOTS('',3,(#138766,#138767,#138768,#138769,#138770,
#138771,#138772,#138773,#138774,#138775,#138776,#138777,#138778),
 .UNSPECIFIED.,.F.,.F.,(4,3,3,3,4),(0.,0.000659089694864322,0.00111822884501791,
0.00208128371043693,0.00223645769003581),.UNSPECIFIED.);
#4367=B_SPLINE_CURVE_WITH_KNOTS('',3,(#138790,#138791,#138792,#138793,#138794,
#138795),.UNSPECIFIED.,.F.,.F.,(4,2,4),(0.,0.510991543129055,1.),
 .UNSPECIFIED.);
#4368=B_SPLINE_CURVE_WITH_KNOTS('',3,(#138800,#138801,#138802,#138803),
 .UNSPECIFIED.,.F.,.F.,(4,4),(0.,1.),.UNSPECIFIED.);
#4369=B_SPLINE_CURVE_WITH_KNOTS('',3,(#138821,#138822,#138823,#138824,#138825,
#138826,#138827,#138828,#138829,#138830,#138831,#138832,#138833,#138834,
#138835,#138836,#138837,#138838,#138839,#138840,#138841,#138842,#138843,
#138844,#138845,#138846,#138847,#138848),.UNSPECIFIED.,.F.,.F.,(4,3,3,3,
3,3,3,3,3,4),(0.,0.000434392388671951,0.000626649590030437,0.000901221465792679,
0.00106184511664083,0.00112652683224085,0.00125380565733159,0.00135183219868902,
0.00158807055660419,0.00180244293158534),.UNSPECIFIED.);
#4370=B_SPLINE_CURVE_WITH_KNOTS('',3,(#138852,#138853,#138854,#138855,#138856,
#138857,#138858,#138859,#138860,#138861,#138862,#138863,#138864,#138865,
#138866,#138867,#138868,#138869,#138870,#138871,#138872,#138873,#138874,
#138875,#138876),.UNSPECIFIED.,.F.,.F.,(4,3,3,3,3,3,3,3,4),(0.000689304848361576,
0.000906283726281564,0.00111364302895385,0.00133013985168632,0.00150801684530018,
0.0017199369438561,0.00199672649963737,0.00227140074390536,0.00232672884224074),
 .UNSPECIFIED.);
#4371=B_SPLINE_CURVE_WITH_KNOTS('',3,(#138993,#138994,#138995,#138996,#138997,
#138998,#138999,#139000,#139001,#139002,#139003,#139004,#139005,#139006,
#139007,#139008,#139009,#139010,#139011,#139012,#139013,#139014,#139015,
#139016,#139017,#139018,#139019,#139020),.UNSPECIFIED.,.F.,.F.,(4,3,3,3,
3,3,3,3,3,4),(0.000653658633860215,0.000901612111390036,0.00110350292160905,
0.00119693882169381,0.00132842506548346,0.00148931670393005,0.00155334720935788,
0.0018252077501562,0.00223261138725098,0.00245303578485557),
 .UNSPECIFIED.);
#4372=B_SPLINE_CURVE_WITH_KNOTS('',3,(#139050,#139051,#139052,#139053),
 .UNSPECIFIED.,.F.,.F.,(4,4),(0.,0.0447707136167657),.UNSPECIFIED.);
#4373=B_SPLINE_CURVE_WITH_KNOTS('',3,(#139059,#139060,#139061,#139062,#139063,
#139064,#139065,#139066,#139067,#139068,#139069,#139070,#139071,#139072,
#139073,#139074,#139075,#139076,#139077,#139078,#139079,#139080,#139081,
#139082,#139083),.UNSPECIFIED.,.F.,.F.,(4,3,3,3,3,3,3,3,4),(0.,0.000275481208481522,
0.000553063545339124,0.000602887330399936,0.000809845174226025,0.00102800957885635,
0.00120532901601379,0.00142404055844574,0.00161969034845205),
 .UNSPECIFIED.);
#4374=B_SPLINE_CURVE_WITH_KNOTS('',3,(#139096,#139097,#139098,#139099),
 .UNSPECIFIED.,.F.,.F.,(4,4),(0.,1.),.UNSPECIFIED.);
#4375=B_SPLINE_CURVE_WITH_KNOTS('',3,(#139121,#139122,#139123,#139124,#139125,
#139126,#139127,#139128,#139129,#139130,#139131,#139132,#139133,#139134,
#139135,#139136,#139137,#139138,#139139,#139140,#139141,#139142,#139143,
#139144,#139145,#139146,#139147,#139148,#139149,#139150,#139151,#139152,
#139153,#139154,#139155,#139156,#139157),.UNSPECIFIED.,.F.,.F.,(4,3,3,3,
3,3,3,3,3,3,3,3,4),(0.,0.000289456070004167,0.000578912140008334,0.000732555002063411,
0.00109883518473064,0.00115782428001667,0.00146516214354768,0.001736736420025,
0.00183135727517645,0.00202619249002917,0.00217092052503125,0.00219767702911212,
0.00231564856003333),.UNSPECIFIED.);
#4376=B_SPLINE_CURVE_WITH_KNOTS('',3,(#139161,#139162,#139163,#139164,#139165,
#139166,#139167,#139168,#139169,#139170,#139171,#139172,#139173,#139174,
#139175,#139176,#139177,#139178,#139179,#139180,#139181,#139182,#139183,
#139184,#139185,#139186,#139187,#139188,#139189,#139190,#139191,#139192,
#139193,#139194,#139195,#139196,#139197),.UNSPECIFIED.,.F.,.F.,(4,3,3,3,
3,3,3,3,3,3,3,3,4),(0.000672031760609077,0.000712854075812315,0.00100252198457116,
0.00107233830279969,0.0012216976510115,0.00143188803178762,0.00171092729228739,
0.00177136354141392,0.00179176783191224,0.00215141270034081,0.00232102943181635,
0.00259586237701756,0.00287069532221878),.UNSPECIFIED.);
#4377=B_SPLINE_CURVE_WITH_KNOTS('',3,(#139208,#139209,#139210,#139211,#139212,
#139213,#139214,#139215,#139216,#139217,#139218,#139219,#139220),
 .UNSPECIFIED.,.F.,.F.,(4,3,3,3,4),(0.,0.00070198654781531,0.00111013811990961,
0.00206054695802749,0.00222027623981921),.UNSPECIFIED.);
#4378=B_SPLINE_CURVE_WITH_KNOTS('',3,(#139224,#139225,#139226,#139227,#139228,
#139229,#139230,#139231,#139232,#139233,#139234,#139235,#139236),
 .UNSPECIFIED.,.F.,.F.,(4,3,3,3,4),(0.,0.000647478258305606,0.00111023907191622,
0.002070391292413,0.00222047814383243),.UNSPECIFIED.);
#4379=B_SPLINE_CURVE_WITH_KNOTS('',3,(#139312,#139313,#139314,#139315,#139316,
#139317,#139318,#139319,#139320,#139321,#139322,#139323,#139324,#139325),
 .UNSPECIFIED.,.F.,.F.,(4,2,2,2,2,2,4),(0.,0.253127110916779,0.379690666375168,
0.506254221833555,0.632817777291944,0.759381332750333,1.),.UNSPECIFIED.);
#4380=B_SPLINE_CURVE_WITH_KNOTS('',3,(#139326,#139327,#139328,#139329),
 .UNSPECIFIED.,.F.,.F.,(4,4),(0.00436813896256353,0.00486865237729894),
 .UNSPECIFIED.);
#4381=B_SPLINE_CURVE_WITH_KNOTS('',3,(#139373,#139374,#139375,#139376,#139377,
#139378,#139379,#139380,#139381,#139382,#139383,#139384,#139385,#139386,
#139387,#139388,#139389,#139390,#139391,#139392,#139393,#139394,#139395,
#139396,#139397,#139398,#139399,#139400,#139401,#139402,#139403,#139404,
#139405,#139406,#139407,#139408,#139409),.UNSPECIFIED.,.F.,.F.,(4,3,3,3,
3,3,3,3,3,3,3,3,4),(0.000461676008985161,0.000632546215505795,0.000848081241001053,
0.00093127816033473,0.0011451568350677,0.00130839695615338,0.00168583810655035,
0.00182863766115024,0.00206327508940322,0.00244071732574779,0.00251211848723277,
0.00307037767187467,0.00319559931331531),.UNSPECIFIED.);
#4382=B_SPLINE_CURVE_WITH_KNOTS('',3,(#139428,#139429,#139430,#139431),
 .UNSPECIFIED.,.F.,.F.,(4,4),(0.,0.0419168978153696),.UNSPECIFIED.);
#4383=B_SPLINE_CURVE_WITH_KNOTS('',3,(#139433,#139434,#139435,#139436,#139437,
#139438,#139439,#139440,#139441,#139442,#139443,#139444,#139445),
 .UNSPECIFIED.,.F.,.F.,(4,3,3,3,4),(0.,0.000842979772292327,0.00121101869920095,
0.00218603126583571,0.00242203739840189),.UNSPECIFIED.);
#4384=B_SPLINE_CURVE_WITH_KNOTS('',3,(#139449,#139450,#139451,#139452,#139453,
#139454,#139455,#139456,#139457,#139458,#139459,#139460,#139461),
 .UNSPECIFIED.,.F.,.F.,(4,3,3,3,4),(0.,0.000857870627763608,0.00121135746045287,
0.00220749552005158,0.00242271492090574),.UNSPECIFIED.);
#4385=B_SPLINE_CURVE_WITH_KNOTS('',3,(#139463,#139464,#139465,#139466),
 .UNSPECIFIED.,.F.,.F.,(4,4),(0.,0.0421837023697854),.UNSPECIFIED.);
#4386=B_SPLINE_CURVE_WITH_KNOTS('',3,(#139472,#139473,#139474,#139475,#139476,
#139477,#139478,#139479,#139480,#139481,#139482,#139483,#139484,#139485,
#139486,#139487,#139488,#139489,#139490,#139491,#139492,#139493,#139494,
#139495,#139496,#139497,#139498,#139499,#139500,#139501,#139502,#139503,
#139504,#139505,#139506,#139507,#139508,#139509,#139510,#139511),
 .UNSPECIFIED.,.F.,.F.,(4,3,3,3,3,3,3,3,3,3,3,3,3,4),(0.,0.000556259975663021,
0.000647586119897307,0.000728260191095084,0.00109239125585008,0.00129517223979461,
0.00145651805257901,0.00182064826297317,0.00194275835969192,0.00212625862851252,
0.00218441767336186,0.00226655141964057,0.00244042135138774,0.00259034447958922),
 .UNSPECIFIED.);
#4387=B_SPLINE_CURVE_WITH_KNOTS('',3,(#139516,#139517,#139518,#139519,#139520,
#139521,#139522,#139523),.UNSPECIFIED.,.F.,.F.,(4,2,2,4),(0.,0.141658916901159,
0.430052386440966,1.),.UNSPECIFIED.);
#4388=B_SPLINE_CURVE_WITH_KNOTS('',3,(#139528,#139529,#139530,#139531,#139532,
#139533),.UNSPECIFIED.,.F.,.F.,(4,2,4),(0.,0.5,1.),.UNSPECIFIED.);
#4389=B_SPLINE_CURVE_WITH_KNOTS('',3,(#139563,#139564,#139565,#139566,#139567,
#139568,#139569),.UNSPECIFIED.,.F.,.F.,(4,3,4),(6.93889390390723E-18,0.0190876722191456,
0.0381753444382913),.UNSPECIFIED.);
#4390=B_SPLINE_CURVE_WITH_KNOTS('',3,(#139571,#139572,#139573,#139574,#139575,
#139576,#139577,#139578,#139579,#139580,#139581,#139582,#139583,#139584,
#139585,#139586),.UNSPECIFIED.,.F.,.F.,(4,3,3,3,3,4),(0.,0.000542853834904753,
0.0010951883108263,0.00152034213881841,0.00254894911026828,0.00304068427763681),
 .UNSPECIFIED.);
#4391=B_SPLINE_CURVE_WITH_KNOTS('',3,(#139590,#139591,#139592,#139593,#139594,
#139595,#139596,#139597,#139598,#139599,#139600,#139601,#139602),
 .UNSPECIFIED.,.F.,.F.,(4,3,3,3,4),(0.,0.000817157754010372,0.00152229638412186,
0.00262171283977742,0.00304459276824371),.UNSPECIFIED.);
#4392=B_SPLINE_CURVE_WITH_KNOTS('',3,(#139603,#139604,#139605,#139606,#139607,
#139608,#139609),.UNSPECIFIED.,.F.,.F.,(4,3,4),(0.,0.0189537577590876,0.0379075155181752),
 .UNSPECIFIED.);
#4393=B_SPLINE_CURVE_WITH_KNOTS('',3,(#139639,#139640,#139641,#139642,#139643,
#139644,#139645),.UNSPECIFIED.,.F.,.F.,(4,3,4),(0.,0.0178083890192188,0.0356167780384377),
 .UNSPECIFIED.);
#4394=B_SPLINE_CURVE_WITH_KNOTS('',3,(#139647,#139648,#139649,#139650,#139651,
#139652,#139653,#139654),.UNSPECIFIED.,.F.,.F.,(4,2,2,4),(0.,0.000841011829491348,
0.00168202365898269,0.00336404731796539),.UNSPECIFIED.);
#4395=B_SPLINE_CURVE_WITH_KNOTS('',3,(#139658,#139659,#139660,#139661,#139662,
#139663,#139664,#139665,#139666,#139667,#139668,#139669,#139670,#139671,
#139672,#139673),.UNSPECIFIED.,.F.,.F.,(4,3,3,3,3,4),(0.,0.000762418881013546,
0.00156275687157928,0.00168533471950014,0.00283547033563459,0.00337066943900028),
 .UNSPECIFIED.);
#4396=B_SPLINE_CURVE_WITH_KNOTS('',3,(#139675,#139676,#139677,#139678,#139679,
#139680,#139681),.UNSPECIFIED.,.F.,.F.,(4,3,4),(0.,0.0179426259581151,0.0358852519162302),
 .UNSPECIFIED.);
#4397=B_SPLINE_CURVE_WITH_KNOTS('',3,(#139696,#139697,#139698,#139699,#139700,
#139701,#139702),.UNSPECIFIED.,.F.,.F.,(4,3,4),(7.55544064091613E-7,0.374830472019235,
1.),.UNSPECIFIED.);
#4398=B_SPLINE_CURVE_WITH_KNOTS('',3,(#139735,#139736,#139737,#139738,#139739,
#139740,#139741),.UNSPECIFIED.,.F.,.F.,(4,3,4),(0.,0.0148367096635454,0.0296734193270908),
 .UNSPECIFIED.);
#4399=B_SPLINE_CURVE_WITH_KNOTS('',3,(#139743,#139744,#139745,#139746,#139747,
#139748,#139749,#139750,#139751,#139752,#139753,#139754,#139755,#139756,
#139757,#139758,#139759,#139760,#139761,#139762,#139763,#139764,#139765,
#139766,#139767),.UNSPECIFIED.,.F.,.F.,(4,3,3,3,3,3,3,3,4),(0.,0.000418974782549054,
0.000841777476039438,0.00103655247459,0.00148268378394067,0.00192505831514581,
0.00207310494918,0.00313777887503632,0.00414620989836001),.UNSPECIFIED.);
#4400=B_SPLINE_CURVE_WITH_KNOTS('',3,(#139771,#139772,#139773,#139774,#139775,
#139776,#139777,#139778,#139779,#139780,#139781,#139782,#139783,#139784,
#139785,#139786,#139787,#139788,#139789,#139790,#139791,#139792),
 .UNSPECIFIED.,.F.,.F.,(4,3,3,3,3,3,3,4),(1.55158384577954E-17,0.000383789572585087,
0.000781910391030218,0.00103855983331611,0.00179575082686721,0.00207711966663221,
0.00335799595905766,0.00415423933326436),.UNSPECIFIED.);
#4401=B_SPLINE_CURVE_WITH_KNOTS('',3,(#139793,#139794,#139795,#139796,#139797,
#139798,#139799),.UNSPECIFIED.,.F.,.F.,(4,3,4),(0.,0.0147014688781887,0.0294029377563774),
 .UNSPECIFIED.);
#4402=B_SPLINE_CURVE_WITH_KNOTS('',3,(#139812,#139813,#139814,#139815),
 .UNSPECIFIED.,.F.,.F.,(4,4),(0.,8.25660289862869E-5),.UNSPECIFIED.);
#4403=B_SPLINE_CURVE_WITH_KNOTS('',3,(#139920,#139921,#139922,#139923),
 .UNSPECIFIED.,.F.,.F.,(4,4),(0.,0.000203650363220012),.UNSPECIFIED.);
#4404=B_SPLINE_CURVE_WITH_KNOTS('',3,(#139925,#139926,#139927,#139928,#139929,
#139930,#139931,#139932,#139933,#139934,#139935,#139936,#139937,#139938,
#139939,#139940,#139941,#139942,#139943,#139944,#139945,#139946,#139947,
#139948,#139949),.UNSPECIFIED.,.F.,.F.,(4,3,3,3,3,3,3,3,4),(0.,7.36083385132494E-5,
0.000151188117340887,0.000234018984647725,0.000250167431468888,0.000250705751451724,
0.000332906541326753,0.0004186952522917,0.000500334862937777),
 .UNSPECIFIED.);
#4405=B_SPLINE_CURVE_WITH_KNOTS('',3,(#139951,#139952,#139953,#139954,#139955,
#139956,#139957,#139958,#139959,#139960,#139961,#139962,#139963,#139964,
#139965,#139966),.UNSPECIFIED.,.F.,.F.,(4,3,3,3,3,4),(0.,0.0014169282635678,
0.00283385652713561,0.00425078479070341,0.00538743306805026,0.00566771305427122),
 .UNSPECIFIED.);
#4406=B_SPLINE_CURVE_WITH_KNOTS('',3,(#139970,#139971,#139972,#139973,#139974,
#139975,#139976,#139977,#139978,#139979,#139980,#139981,#139982),
 .UNSPECIFIED.,.F.,.F.,(4,3,3,3,4),(6.93889390390723E-18,0.00134873564674426,
0.00269747129348853,0.00432753805226678,0.00539494258697707),
 .UNSPECIFIED.);
#4407=B_SPLINE_CURVE_WITH_KNOTS('',3,(#139984,#139985,#139986,#139987,#139988,
#139989,#139990,#139991,#139992,#139993,#139994,#139995,#139996,#139997,
#139998,#139999,#140000,#140001,#140002),.UNSPECIFIED.,.F.,.F.,(4,3,3,3,
3,3,4),(0.,0.000151278709681427,0.000175639358542286,0.000320819121628032,
0.000351502905376566,0.000527285240968795,0.000703005810753132),
 .UNSPECIFIED.);
#4408=B_SPLINE_CURVE_WITH_KNOTS('',3,(#140030,#140031,#140032,#140033,#140034,
#140035,#140036,#140037,#140038,#140039,#140040,#140041,#140042,#140043,
#140044,#140045,#140046,#140047,#140048,#140049,#140050,#140051,#140052,
#140053,#140054,#140055,#140056,#140057,#140058,#140059,#140060),
 .UNSPECIFIED.,.F.,.F.,(4,3,3,3,3,3,3,3,3,3,4),(0.,0.000563737664817591,
0.000564164457966204,0.00104582442927209,0.0011276022003503,0.00112832891593241,
0.00161216721638057,0.00169210723432567,0.00169249337389861,0.00210946737344705,
0.00225665783186482),.UNSPECIFIED.);
#4409=B_SPLINE_CURVE_WITH_KNOTS('',3,(#140097,#140098,#140099,#140100,#140101,
#140102,#140103,#140104,#140105,#140106,#140107,#140108,#140109,#140110,
#140111,#140112,#140113,#140114,#140115,#140116,#140117,#140118,#140119,
#140120,#140121,#140122,#140123,#140124,#140125,#140126,#140127,#140128,
#140129,#140130,#140131,#140132,#140133),.UNSPECIFIED.,.F.,.F.,(4,3,3,3,
3,3,3,3,3,3,3,3,4),(0.,0.000231966620805442,0.000541763265449849,0.000565419069388556,
0.000565630623675328,0.00113073622792201,0.00113126124735066,0.00146429940364797,
0.00169659085207846,0.00169689187102598,0.00198522910629736,0.00223959723149682,
0.00226252249470131),.UNSPECIFIED.);
#4410=B_SPLINE_CURVE_WITH_KNOTS('',3,(#140190,#140191,#140192,#140193,#140194,
#140195,#140196,#140197,#140198,#140199,#140200,#140201,#140202,#140203,
#140204,#140205,#140206,#140207,#140208,#140209,#140210,#140211,#140212,
#140213,#140214,#140215,#140216,#140217,#140218,#140219,#140220),
 .UNSPECIFIED.,.F.,.F.,(4,3,3,3,3,3,3,3,3,3,4),(0.,0.00011822449235466,
0.000239962463540573,0.000354016906950293,0.000486351214789361,0.000618764034589224,
0.000708033813900585,0.000911280042633104,0.00111586864905152,0.00131545298208588,
0.00141606762780121),.UNSPECIFIED.);
#4411=B_SPLINE_CURVE_WITH_KNOTS('',3,(#140233,#140234,#140235,#140236),
 .UNSPECIFIED.,.F.,.F.,(4,4),(0.,0.0203430832871546),.UNSPECIFIED.);
#4412=B_SPLINE_CURVE_WITH_KNOTS('',3,(#140238,#140239,#140240,#140241,#140242,
#140243,#140244,#140245,#140246,#140247,#140248,#140249,#140250),
 .UNSPECIFIED.,.F.,.F.,(4,3,3,3,4),(0.,0.00107468821847175,0.0021493764369435,
0.00322406465541528,0.00429875287388706),.UNSPECIFIED.);
#4413=B_SPLINE_CURVE_WITH_KNOTS('',3,(#140254,#140255,#140256,#140257,#140258,
#140259,#140260,#140261,#140262,#140263,#140264,#140265,#140266,#140267,
#140268,#140269,#140270,#140271,#140272,#140273,#140274,#140275),
 .UNSPECIFIED.,.F.,.F.,(4,3,3,3,3,3,3,4),(0.,0.000387785729070444,0.000791054588127252,
0.00107666227523054,0.00167259937147553,0.00215332455046108,0.00346243334013028,
0.00430664910092208),.UNSPECIFIED.);
#4414=B_SPLINE_CURVE_WITH_KNOTS('',3,(#140277,#140278,#140279,#140280),
 .UNSPECIFIED.,.F.,.F.,(4,4),(0.,0.0206148669995797),.UNSPECIFIED.);
#4415=B_SPLINE_CURVE_WITH_KNOTS('',3,(#140282,#140283,#140284,#140285),
 .UNSPECIFIED.,.F.,.F.,(4,4),(0.,0.000103369667661668),.UNSPECIFIED.);
#4416=B_SPLINE_CURVE_WITH_KNOTS('',3,(#140287,#140288,#140289,#140290,#140291,
#140292,#140293,#140294,#140295,#140296,#140297,#140298,#140299),
 .UNSPECIFIED.,.F.,.F.,(4,3,3,3,4),(0.,0.000379823720135543,0.000488238270882253,
0.000734566123594352,0.000976476541764506),.UNSPECIFIED.);
#4417=B_SPLINE_CURVE_WITH_KNOTS('',3,(#140308,#140309,#140310,#140311,#140312,
#140313,#140314,#140315),.UNSPECIFIED.,.F.,.F.,(4,2,2,4),(0.,0.25,0.5,1.),
 .UNSPECIFIED.);
#4418=B_SPLINE_CURVE_WITH_KNOTS('',3,(#140387,#140388,#140389,#140390,#140391,
#140392,#140393,#140394,#140395,#140396,#140397,#140398,#140399,#140400,
#140401,#140402,#140403,#140404,#140405),.UNSPECIFIED.,.F.,.F.,(4,3,3,3,
3,3,4),(0.,0.000108392306331872,0.000159419175882384,0.000279017984019056,
0.000319155213741796,0.000478738661811072,0.000638310427483592),
 .UNSPECIFIED.);
#4419=B_SPLINE_CURVE_WITH_KNOTS('',3,(#140407,#140408,#140409,#140410),
 .UNSPECIFIED.,.F.,.F.,(4,4),(0.,0.01284355850178),.UNSPECIFIED.);
#4420=B_SPLINE_CURVE_WITH_KNOTS('',3,(#140412,#140413,#140414,#140415,#140416,
#140417,#140418,#140419,#140420,#140421,#140422,#140423,#140424,#140425,
#140426,#140427),.UNSPECIFIED.,.F.,.F.,(4,3,3,3,3,4),(0.,0.00125936773350451,
0.00251873546700902,0.00377810320051352,0.00490364900521194,0.00503747093401803),
 .UNSPECIFIED.);
#4421=B_SPLINE_CURVE_WITH_KNOTS('',3,(#140431,#140432,#140433,#140434,#140435,
#140436,#140437,#140438,#140439,#140440,#140441,#140442,#140443),
 .UNSPECIFIED.,.F.,.F.,(4,3,3,3,4),(0.,0.00126095469566737,0.00252190939133473,
0.00394829824261489,0.00504381878266947),.UNSPECIFIED.);
#4422=B_SPLINE_CURVE_WITH_KNOTS('',3,(#140445,#140446,#140447,#140448),
 .UNSPECIFIED.,.F.,.F.,(4,4),(0.,0.0125680158145827),.UNSPECIFIED.);
#4423=B_SPLINE_CURVE_WITH_KNOTS('',3,(#140450,#140451,#140452,#140453,#140454,
#140455,#140456,#140457,#140458,#140459,#140460,#140461,#140462),
 .UNSPECIFIED.,.F.,.F.,(4,3,3,3,4),(0.,0.000167806452110249,0.000320197614368795,
0.000480307701132281,0.000640395228737589),.UNSPECIFIED.);
#4424=B_SPLINE_CURVE_WITH_KNOTS('',3,(#140488,#140489,#140490,#140491,#140492,
#140493,#140494,#140495,#140496,#140497,#140498,#140499,#140500,#140501,
#140502,#140503,#140504,#140505,#140506,#140507,#140508,#140509),
 .UNSPECIFIED.,.F.,.F.,(4,3,3,3,3,3,3,4),(0.,0.00011032124306843,0.00023255444160577,
0.000327443278856643,0.000415696683397808,0.000505913400363213,0.000594574640422507,
0.000654886557713287),.UNSPECIFIED.);
#4425=B_SPLINE_CURVE_WITH_KNOTS('',3,(#140511,#140512,#140513,#140514),
 .UNSPECIFIED.,.F.,.F.,(4,4),(0.,0.00876509433037234),.UNSPECIFIED.);
#4426=B_SPLINE_CURVE_WITH_KNOTS('',3,(#140516,#140517,#140518,#140519,#140520,
#140521,#140522,#140523,#140524,#140525,#140526,#140527,#140528,#140529,
#140530,#140531,#140532,#140533,#140534,#140535,#140536,#140537,#140538,
#140539,#140540),.UNSPECIFIED.,.F.,.F.,(4,3,3,3,3,3,3,3,4),(0.,0.00066897147268262,
0.00133794294536524,0.00197188997955202,0.0025968969389697,0.00267588589073048,
0.00401382883609571,0.00511764383901403,0.00535177178146096),
 .UNSPECIFIED.);
#4427=B_SPLINE_CURVE_WITH_KNOTS('',3,(#140544,#140545,#140546,#140547,#140548,
#140549,#140550,#140551,#140552,#140553,#140554,#140555,#140556,#140557,
#140558,#140559),.UNSPECIFIED.,.F.,.F.,(4,3,3,3,3,4),(0.,0.00120908655042554,
0.00133938491136683,0.00267876982273365,0.0041514377188616,0.0053575396454673),
 .UNSPECIFIED.);
#4428=B_SPLINE_CURVE_WITH_KNOTS('',3,(#140561,#140562,#140563,#140564),
 .UNSPECIFIED.,.F.,.F.,(4,4),(0.,0.00904291806877093),.UNSPECIFIED.);
#4429=B_SPLINE_CURVE_WITH_KNOTS('',3,(#140566,#140567,#140568,#140569,#140570,
#140571,#140572,#140573,#140574,#140575,#140576,#140577,#140578,#140579,
#140580,#140581),.UNSPECIFIED.,.F.,.F.,(4,3,3,3,3,4),(0.,0.00019490585199519,
0.000327981152987957,0.000444921456705669,0.000551183314035708,0.000655962305975913),
 .UNSPECIFIED.);
#4430=B_SPLINE_CURVE_WITH_KNOTS('',3,(#140697,#140698,#140699,#140700,#140701,
#140702,#140703,#140704,#140705,#140706,#140707,#140708,#140709),
 .UNSPECIFIED.,.F.,.F.,(4,3,3,3,4),(0.,0.00125486684196805,0.0025097336839361,
0.00393224022465218,0.00501946736787221),.UNSPECIFIED.);
#4431=B_SPLINE_CURVE_WITH_KNOTS('',3,(#140711,#140712,#140713,#140714),
 .UNSPECIFIED.,.F.,.F.,(4,4),(0.,0.0135233968444946),.UNSPECIFIED.);
#4432=B_SPLINE_CURVE_WITH_KNOTS('',3,(#140716,#140717,#140718,#140719,#140720,
#140721,#140722,#140723,#140724,#140725,#140726,#140727,#140728,#140729,
#140730,#140731,#140732,#140733,#140734),.UNSPECIFIED.,.F.,.F.,(4,3,3,3,
3,3,4),(0.,0.000165241084431127,0.000319189981521249,0.000429288245408173,
0.000533834104225336,0.000631975129725757,0.000638379963042499),
 .UNSPECIFIED.);
#4433=B_SPLINE_CURVE_WITH_KNOTS('',3,(#140750,#140751,#140752,#140753,#140754,
#140755,#140756,#140757,#140758,#140759,#140760,#140761,#140762,#140763,
#140764,#140765,#140766,#140767,#140768,#140769,#140770,#140771,#140772,
#140773,#140774,#140775,#140776,#140777,#140778,#140779,#140780,#140781,
#140782,#140783,#140784,#140785,#140786,#140787,#140788,#140789),
 .UNSPECIFIED.,.F.,.F.,(4,3,3,3,3,3,3,3,3,3,3,3,3,4),(0.,0.00016104755367178,
0.000326655464486219,0.00049386305290849,0.000580621437699987,0.00058187576131232,
0.0011633223004275,0.00116375152262464,0.00145467271006653,0.00145468940328081,
0.00174562728393698,0.0017460231201541,0.00204798180553722,0.00232750304524933),
 .UNSPECIFIED.);
#4434=B_SPLINE_CURVE_WITH_KNOTS('',3,(#140791,#140792,#140793,#140794,#140795,
#140796,#140797,#140798,#140799,#140800,#140801,#140802,#140803,#140804,
#140805,#140806,#140807,#140808,#140809),.UNSPECIFIED.,.F.,.F.,(4,3,3,3,
3,3,4),(0.,0.000151109125705162,0.000302236517833045,0.000386300967573319,
0.000471902393705335,0.000555234376218938,0.000604473035666092),
 .UNSPECIFIED.);
#4435=B_SPLINE_CURVE_WITH_KNOTS('',3,(#140811,#140812,#140813,#140814),
 .UNSPECIFIED.,.F.,.F.,(4,4),(0.,0.0170848224870981),.UNSPECIFIED.);
#4436=B_SPLINE_CURVE_WITH_KNOTS('',3,(#140816,#140817,#140818,#140819,#140820,
#140821,#140822,#140823,#140824,#140825,#140826,#140827,#140828),
 .UNSPECIFIED.,.F.,.F.,(4,3,3,3,4),(0.,0.00117191361843274,0.00234382723686548,
0.00351574085529822,0.00468765447373096),.UNSPECIFIED.);
#4437=B_SPLINE_CURVE_WITH_KNOTS('',3,(#140904,#140905,#140906,#140907,#140908,
#140909,#140910,#140911,#140912,#140913,#140914,#140915,#140916),
 .UNSPECIFIED.,.F.,.F.,(4,3,3,3,4),(3.1415926535898,3.53429173528852,3.92699081698724,
4.31968989868597,4.71238898038469),.UNSPECIFIED.);
#4438=B_SPLINE_CURVE_WITH_KNOTS('',3,(#140948,#140949,#140950,#140951,#140952,
#140953,#140954,#140955,#140956,#140957,#140958,#140959,#140960,#140961,
#140962,#140963,#140964,#140965,#140966),.UNSPECIFIED.,.F.,.F.,(4,3,3,3,
3,3,4),(0.,0.000168652558320961,0.000337340594483331,0.000432590797837365,
0.000530250662249296,0.000626975088861455,0.000674681188966661),
 .UNSPECIFIED.);
#4439=B_SPLINE_CURVE_WITH_KNOTS('',3,(#140973,#140974,#140975,#140976,#140977,
#140978,#140979,#140980,#140981,#140982,#140983,#140984,#140985,#140986,
#140987,#140988),.UNSPECIFIED.,.F.,.F.,(4,3,3,3,3,4),(0.,0.00159103011507281,
0.00287711962167565,0.00431567943251345,0.00538763071254621,0.00575423924335125),
 .UNSPECIFIED.);
#4440=B_SPLINE_CURVE_WITH_KNOTS('',3,(#141098,#141099,#141100,#141101,#141102,
#141103,#141104,#141105,#141106,#141107,#141108,#141109,#141110,#141111,
#141112,#141113,#141114,#141115,#141116),.UNSPECIFIED.,.F.,.F.,(4,3,3,3,
3,3,4),(0.,0.000174255415100454,0.000348555105993215,0.00044998536948759,
0.000554229835728645,0.00065771924945466,0.000697110211986431),
 .UNSPECIFIED.);
#4441=B_SPLINE_CURVE_WITH_KNOTS('',3,(#141123,#141124,#141125,#141126,#141127,
#141128,#141129,#141130,#141131,#141132,#141133,#141134,#141135,#141136,
#141137,#141138,#141139,#141140,#141141),.UNSPECIFIED.,.F.,.F.,(4,3,3,3,
3,3,4),(0.,0.00156956785490461,0.00313913570980923,0.00392391963731218,
0.00470870356471384,0.00573336346877459,0.00627827141961845),
 .UNSPECIFIED.);
#4442=B_SPLINE_CURVE_WITH_KNOTS('',3,(#141145,#141146,#141147,#141148,#141149,
#141150,#141151,#141152,#141153,#141154,#141155,#141156,#141157,#141158,
#141159,#141160),.UNSPECIFIED.,.F.,.F.,(4,3,3,3,3,4),(0.,0.00104863959930094,
0.00157050793024954,0.00314101586049909,0.00471152379074863,0.00628203172099817),
 .UNSPECIFIED.);
#4443=B_SPLINE_CURVE_WITH_KNOTS('',3,(#141167,#141168,#141169,#141170,#141171,
#141172,#141173,#141174,#141175,#141176,#141177,#141178,#141179),
 .UNSPECIFIED.,.F.,.F.,(4,3,3,3,4),(0.,0.000174780063231097,0.000349568960659906,
0.000524372653650724,0.000699137921319812),.UNSPECIFIED.);
#4444=B_SPLINE_CURVE_WITH_KNOTS('',3,(#141253,#141254,#141255,#141256,#141257,
#141258,#141259,#141260,#141261,#141262,#141263,#141264,#141265,#141266,
#141267,#141268,#141269,#141270,#141271),.UNSPECIFIED.,.F.,.F.,(4,3,3,3,
3,3,4),(0.,0.000358645716708602,0.000416788078411026,0.000833987724853057,
0.000834068655632161,0.00125109176933023,0.00166813731126432),
 .UNSPECIFIED.);
#4445=B_SPLINE_CURVE_WITH_KNOTS('',3,(#141297,#141298,#141299,#141300,#141301,
#141302,#141303,#141304,#141305,#141306,#141307,#141308,#141309,#141310,
#141311,#141312,#141313,#141314,#141315),.UNSPECIFIED.,.F.,.F.,(4,3,3,3,
3,3,4),(0.,0.000417356154990511,0.000834652124500517,0.000834737818312929,
0.0012522269622177,0.00161112215869288,0.00166930424900103),
 .UNSPECIFIED.);
#4446=B_SPLINE_CURVE_WITH_KNOTS('',3,(#141337,#141338,#141339,#141340,#141341,
#141342,#141343),.UNSPECIFIED.,.F.,.F.,(4,3,4),(0.,0.0129055642122842,0.0258111284245685),
 .UNSPECIFIED.);
#4447=B_SPLINE_CURVE_WITH_KNOTS('',3,(#141345,#141346,#141347,#141348,#141349,
#141350,#141351,#141352,#141353,#141354,#141355,#141356,#141357,#141358,
#141359,#141360),.UNSPECIFIED.,.F.,.F.,(4,3,3,3,3,4),(0.,0.00112455173535831,
0.00224910347071663,0.00337365520607496,0.00439646903553278,0.0044982069414333),
 .UNSPECIFIED.);
#4448=B_SPLINE_CURVE_WITH_KNOTS('',3,(#141364,#141365,#141366,#141367,#141368,
#141369,#141370,#141371,#141372,#141373,#141374,#141375,#141376,#141377,
#141378,#141379,#141380,#141381,#141382,#141383,#141384,#141385,#141386,
#141387,#141388),.UNSPECIFIED.,.F.,.F.,(4,3,3,3,3,3,3,3,4),(0.,0.00039368558594612,
0.000804157569269251,0.00112634951454785,0.00164227212955535,0.00217802033014988,
0.0022526990290957,0.00359217050441368,0.00450539805819141),
 .UNSPECIFIED.);
#4449=B_SPLINE_CURVE_WITH_KNOTS('',3,(#141390,#141391,#141392,#141393,#141394,
#141395,#141396),.UNSPECIFIED.,.F.,.F.,(4,3,4),(0.,0.0130414224518927,0.0260828449037854),
 .UNSPECIFIED.);
#4450=B_SPLINE_CURVE_WITH_KNOTS('',3,(#141398,#141399,#141400,#141401),
 .UNSPECIFIED.,.F.,.F.,(4,4),(0.,0.000106239733749475),.UNSPECIFIED.);
#4451=B_SPLINE_CURVE_WITH_KNOTS('',3,(#141403,#141404,#141405,#141406,#141407,
#141408,#141409,#141410,#141411,#141412,#141413,#141414,#141415),
 .UNSPECIFIED.,.F.,.F.,(4,3,3,3,4),(0.,0.000360360286282916,0.000488761174293949,
0.000765042797522198,0.000977522348587897),.UNSPECIFIED.);
#4452=B_SPLINE_CURVE_WITH_KNOTS('',3,(#141443,#141444,#141445,#141446),
 .UNSPECIFIED.,.F.,.F.,(4,4),(1.7347234759768E-18,0.000135753226310594),
 .UNSPECIFIED.);
#4453=B_SPLINE_CURVE_WITH_KNOTS('',3,(#141447,#141448,#141449,#141450),
 .UNSPECIFIED.,.F.,.F.,(4,4),(0.,1.),.UNSPECIFIED.);
#4454=B_SPLINE_CURVE_WITH_KNOTS('',3,(#141458,#141459,#141460,#141461,#141462,
#141463,#141464,#141465),.UNSPECIFIED.,.F.,.F.,(4,2,2,4),(0.,0.25,0.5,1.),
 .UNSPECIFIED.);
#4455=B_SPLINE_CURVE_WITH_KNOTS('',3,(#141537,#141538,#141539,#141540,#141541,
#141542,#141543,#141544,#141545,#141546,#141547,#141548,#141549,#141550,
#141551,#141552,#141553,#141554,#141555),.UNSPECIFIED.,.F.,.F.,(4,3,3,3,
3,3,4),(0.,0.000108634712275121,0.000159257284564384,0.000279020961387413,
0.000318828120207844,0.000478248046436964,0.000637656240415689),
 .UNSPECIFIED.);
#4456=B_SPLINE_CURVE_WITH_KNOTS('',3,(#141557,#141558,#141559,#141560),
 .UNSPECIFIED.,.F.,.F.,(4,4),(0.,0.0180689587739334),.UNSPECIFIED.);
#4457=B_SPLINE_CURVE_WITH_KNOTS('',3,(#141562,#141563,#141564,#141565,#141566,
#141567,#141568,#141569,#141570,#141571,#141572,#141573,#141574,#141575,
#141576,#141577),.UNSPECIFIED.,.F.,.F.,(4,3,3,3,3,4),(0.,0.0013179209674593,
0.00263584193491861,0.00395376290237792,0.00506352109400701,0.00527168386983722),
 .UNSPECIFIED.);
#4458=B_SPLINE_CURVE_WITH_KNOTS('',3,(#141581,#141582,#141583,#141584,#141585,
#141586,#141587,#141588,#141589,#141590,#141591,#141592,#141593,#141594,
#141595,#141596),.UNSPECIFIED.,.F.,.F.,(4,3,3,3,3,4),(0.,0.00122256915433072,
0.0013193477680122,0.00263869553602439,0.00409736884770839,0.00527739107204874),
 .UNSPECIFIED.);
#4459=B_SPLINE_CURVE_WITH_KNOTS('',3,(#141598,#141599,#141600,#141601),
 .UNSPECIFIED.,.F.,.F.,(4,4),(0.,0.0177935197894076),.UNSPECIFIED.);
#4460=B_SPLINE_CURVE_WITH_KNOTS('',3,(#141603,#141604,#141605,#141606,#141607,
#141608,#141609,#141610,#141611,#141612,#141613,#141614,#141615),
 .UNSPECIFIED.,.F.,.F.,(4,3,3,3,4),(0.,0.000166958822901273,0.000319870924789836,
0.000479817604858626,0.000639741849579673),.UNSPECIFIED.);
#4461=B_SPLINE_CURVE_WITH_KNOTS('',3,(#141641,#141642,#141643,#141644,#141645,
#141646,#141647,#141648,#141649,#141650,#141651,#141652,#141653,#141654,
#141655,#141656,#141657,#141658,#141659,#141660,#141661,#141662),
 .UNSPECIFIED.,.F.,.F.,(4,3,3,3,3,3,3,4),(0.,0.000110683358086875,0.00023326550317951,
0.000327042610606244,0.000415140332124169,0.00050518854044065,0.000593686275838932,
0.000654085221212487),.UNSPECIFIED.);
#4462=B_SPLINE_CURVE_WITH_KNOTS('',3,(#141664,#141665,#141666,#141667),
 .UNSPECIFIED.,.F.,.F.,(4,4),(0.,0.0138879247081574),.UNSPECIFIED.);
#4463=B_SPLINE_CURVE_WITH_KNOTS('',3,(#141669,#141670,#141671,#141672,#141673,
#141674,#141675,#141676,#141677,#141678,#141679,#141680,#141681,#141682,
#141683,#141684,#141685,#141686,#141687),.UNSPECIFIED.,.F.,.F.,(4,3,3,3,
3,3,4),(0.,0.00107929064721465,0.00212940062359531,0.00279822589210569,
0.00419733883815853,0.0052823468058471,0.00559645178421137),
 .UNSPECIFIED.);
#4464=B_SPLINE_CURVE_WITH_KNOTS('',3,(#141691,#141692,#141693,#141694,#141695,
#141696,#141697,#141698,#141699,#141700,#141701,#141702,#141703,#141704,
#141705,#141706),.UNSPECIFIED.,.F.,.F.,(4,3,3,3,3,4),(0.,0.00116583085678931,
0.00140039358904036,0.00280078717808072,0.0043057456358814,0.00560157435616136),
 .UNSPECIFIED.);
#4465=B_SPLINE_CURVE_WITH_KNOTS('',3,(#141708,#141709,#141710,#141711),
 .UNSPECIFIED.,.F.,.F.,(4,4),(0.,0.0141656229616797),.UNSPECIFIED.);
#4466=B_SPLINE_CURVE_WITH_KNOTS('',3,(#141713,#141714,#141715,#141716,#141717,
#141718,#141719,#141720,#141721,#141722,#141723,#141724,#141725,#141726,
#141727,#141728),.UNSPECIFIED.,.F.,.F.,(4,3,3,3,3,4),(0.,0.000193094254409061,
0.000327589980483358,0.000444218816712202,0.000550274313876603,0.000655179960966716),
 .UNSPECIFIED.);
#4467=B_SPLINE_CURVE_WITH_KNOTS('',3,(#141748,#141749,#141750,#141751,#141752,
#141753,#141754,#141755,#141756,#141757),.UNSPECIFIED.,.F.,.F.,(4,2,2,2,
4),(0.,0.25,0.5,0.750000000000001,1.),.UNSPECIFIED.);
#4468=B_SPLINE_CURVE_WITH_KNOTS('',3,(#141779,#141780,#141781,#141782,#141783,
#141784,#141785,#141786,#141787,#141788,#141789,#141790,#141791,#141792,
#141793,#141794,#141795,#141796,#141797,#141798,#141799,#141800,#141801,
#141802,#141803,#141804,#141805,#141806,#141807,#141808,#141809),
 .UNSPECIFIED.,.F.,.F.,(4,3,3,3,3,3,3,3,3,3,4),(0.,0.000166652275730451,
0.000342276073641816,0.000519944361542555,0.000694209917748529,0.000732292525246715,
0.000732496372314207,0.000946324251635485,0.00115726770428045,0.0013594228398131,
0.00146458505049343),.UNSPECIFIED.);
#4469=B_SPLINE_CURVE_WITH_KNOTS('',3,(#141814,#141815,#141816,#141817,#141818,
#141819,#141820,#141821,#141822,#141823,#141824,#141825,#141826),
 .UNSPECIFIED.,.F.,.F.,(4,3,3,3,4),(0.,0.000259173930192671,0.000518347860385342,
0.00087729776681203,0.00103669572077068),.UNSPECIFIED.);
#4470=B_SPLINE_CURVE_WITH_KNOTS('',3,(#141828,#141829,#141830,#141831),
 .UNSPECIFIED.,.F.,.F.,(4,4),(0.,0.000120540380538642),.UNSPECIFIED.);
#4471=B_SPLINE_CURVE_WITH_KNOTS('',3,(#141833,#141834,#141835,#141836,#141837,
#141838,#141839),.UNSPECIFIED.,.F.,.F.,(4,3,4),(0.,0.0128929585057523,0.0257859170115047),
 .UNSPECIFIED.);
#4472=B_SPLINE_CURVE_WITH_KNOTS('',3,(#141841,#141842,#141843,#141844,#141845,
#141846,#141847,#141848,#141849,#141850,#141851,#141852,#141853,#141854,
#141855,#141856),.UNSPECIFIED.,.F.,.F.,(4,3,3,3,3,4),(0.,0.00113243548370091,
0.00226487096740181,0.00339730645110276,0.0044193232014814,0.00452974193480371),
 .UNSPECIFIED.);
#4473=B_SPLINE_CURVE_WITH_KNOTS('',3,(#141860,#141861,#141862,#141863,#141864,
#141865,#141866,#141867,#141868,#141869,#141870,#141871,#141872,#141873,
#141874,#141875,#141876,#141877,#141878,#141879,#141880,#141881,#141882,
#141883,#141884),.UNSPECIFIED.,.F.,.F.,(4,3,3,3,3,3,3,3,4),(0.,0.00039468403092862,
0.000806360979195845,0.00113421626089741,0.00164507477301071,0.00217582874625811,
0.00226843252179482,0.00361301771688345,0.00453686504358963),
 .UNSPECIFIED.);
#4474=B_SPLINE_CURVE_WITH_KNOTS('',3,(#141886,#141887,#141888,#141889,#141890,
#141891,#141892),.UNSPECIFIED.,.F.,.F.,(4,3,4),(0.,0.0127570403976527,0.0255140807953054),
 .UNSPECIFIED.);
#4475=B_SPLINE_CURVE_WITH_KNOTS('',3,(#141961,#141962,#141963,#141964,#141965,
#141966,#141967,#141968,#141969,#141970,#141971,#141972,#141973,#141974,
#141975,#141976,#141977,#141978,#141979,#141980,#141981,#141982,#141983,
#141984,#141985,#141986,#141987,#141988,#141989,#141990,#141991),
 .UNSPECIFIED.,.F.,.F.,(4,3,3,3,3,3,3,3,3,3,4),(0.,0.000366648609662479,
0.00067395652917383,0.00118123470620554,0.00134837711191729,0.00134840211582016,
0.00202256566787594,0.00202269623773767,0.00236849530085589,0.0026591601716747,
0.00269675422383458),.UNSPECIFIED.);
#4476=B_SPLINE_CURVE_WITH_KNOTS('',3,(#141999,#142000,#142001,#142002,#142003,
#142004,#142005,#142006,#142007,#142008,#142009,#142010,#142011,#142012,
#142013,#142014,#142015,#142016,#142017,#142018,#142019,#142020,#142021,
#142022,#142023,#142024,#142025,#142026),.UNSPECIFIED.,.F.,.F.,(4,3,3,3,
3,3,3,3,3,4),(0.,0.000297352361641283,0.000685187759872983,0.000685314779244029,
0.00137061382937429,0.00137062955848806,0.00183455251927366,0.00205619372744575,
0.00244930001359206,0.00274125911697611),.UNSPECIFIED.);
#4477=B_SPLINE_CURVE_WITH_KNOTS('',3,(#142074,#142075,#142076,#142077,#142078,
#142079,#142080,#142081,#142082,#142083,#142084,#142085,#142086,#142087,
#142088,#142089,#142090,#142091,#142092),.UNSPECIFIED.,.F.,.F.,(4,3,3,3,
3,3,4),(0.,0.000175073926804946,0.000350193522739415,0.000452577371514084,
0.000557835767991038,0.000662370656289191,0.000700387045478831),
 .UNSPECIFIED.);
#4478=B_SPLINE_CURVE_WITH_KNOTS('',3,(#142099,#142100,#142101,#142102,#142103,
#142104,#142105,#142106,#142107,#142108,#142109,#142110,#142111,#142112,
#142113,#142114,#142115,#142116,#142117),.UNSPECIFIED.,.F.,.F.,(4,3,3,3,
3,3,4),(0.,0.00157595519506122,0.00315191039012244,0.00393988798770612,
0.00472786558518367,0.00575007285733746,0.00630382078024489),
 .UNSPECIFIED.);
#4479=B_SPLINE_CURVE_WITH_KNOTS('',3,(#142121,#142122,#142123,#142124,#142125,
#142126,#142127,#142128,#142129,#142130,#142131,#142132,#142133,#142134,
#142135,#142136),.UNSPECIFIED.,.F.,.F.,(4,3,3,3,3,4),(0.,0.00104430221457033,
0.00157688090361367,0.00315376180722735,0.00473064271084103,0.00630752361445471),
 .UNSPECIFIED.);
#4480=B_SPLINE_CURVE_WITH_KNOTS('',3,(#142143,#142144,#142145,#142146,#142147,
#142148,#142149,#142150,#142151,#142152,#142153,#142154,#142155),
 .UNSPECIFIED.,.F.,.F.,(4,3,3,3,4),(0.,0.000175209888250476,0.000350428553470057,
0.000525662295915621,0.000700857106940114),.UNSPECIFIED.);
#4481=B_SPLINE_CURVE_WITH_KNOTS('',3,(#142239,#142240,#142241,#142242,#142243,
#142244,#142245,#142246,#142247,#142248,#142249,#142250,#142251),
 .UNSPECIFIED.,.F.,.F.,(4,3,3,3,4),(3.1415926535898,3.53429173528852,3.92699081698725,
4.31968989868597,4.7123889803847),.UNSPECIFIED.);
#4482=B_SPLINE_CURVE_WITH_KNOTS('',3,(#142279,#142280,#142281,#142282,#142283,
#142284,#142285,#142286,#142287,#142288,#142289,#142290,#142291,#142292,
#142293,#142294,#142295,#142296,#142297,#142298,#142299,#142300),
 .UNSPECIFIED.,.F.,.F.,(4,3,3,3,3,3,3,4),(0.,0.000110166739483085,0.000232250654979584,
0.000327614165524935,0.000415934063629714,0.000506222853831995,0.000594954171387644,
0.000655228331049871),.UNSPECIFIED.);
#4483=B_SPLINE_CURVE_WITH_KNOTS('',3,(#142302,#142303,#142304,#142305),
 .UNSPECIFIED.,.F.,.F.,(4,4),(0.,0.0138038180377133),.UNSPECIFIED.);
#4484=B_SPLINE_CURVE_WITH_KNOTS('',3,(#142307,#142308,#142309,#142310,#142311,
#142312,#142313,#142314,#142315,#142316,#142317,#142318,#142319,#142320,
#142321,#142322,#142323,#142324,#142325),.UNSPECIFIED.,.F.,.F.,(4,3,3,3,
3,3,4),(0.,0.00115159118172974,0.00227058783088812,0.00281251499795634,
0.00421877249693456,0.00530146752118551,0.00562502999591277),
 .UNSPECIFIED.);
#4485=B_SPLINE_CURVE_WITH_KNOTS('',3,(#142329,#142330,#142331,#142332,#142333,
#142334,#142335,#142336,#142337,#142338,#142339,#142340,#142341,#142342,
#142343,#142344),.UNSPECIFIED.,.F.,.F.,(4,3,3,3,3,4),(0.,0.00116086488264771,
0.0014075250438046,0.0028150500876092,0.00432397808187545,0.00563010017521834),
 .UNSPECIFIED.);
#4486=B_SPLINE_CURVE_WITH_KNOTS('',3,(#142346,#142347,#142348,#142349),
 .UNSPECIFIED.,.F.,.F.,(4,4),(0.,0.0135258923233721),.UNSPECIFIED.);
#4487=B_SPLINE_CURVE_WITH_KNOTS('',3,(#142351,#142352,#142353,#142354,#142355,
#142356,#142357,#142358,#142359,#142360,#142361,#142362,#142363,#142364,
#142365,#142366),.UNSPECIFIED.,.F.,.F.,(4,3,3,3,3,4),(0.,0.000197943176920928,
0.000328605151068823,0.000446042787173481,0.000552633627937305,0.000657210302137648),
 .UNSPECIFIED.);
#4488=B_SPLINE_CURVE_WITH_KNOTS('',3,(#142434,#142435,#142436,#142437,#142438,
#142439,#142440,#142441,#142442,#142443,#142444,#142445,#142446,#142447,
#142448,#142449,#142450,#142451,#142452),.UNSPECIFIED.,.F.,.F.,(4,3,3,3,
3,3,4),(0.,0.000108019327761152,0.000159670358772899,0.000279016064561992,
0.000319662760640411,0.000479499943955603,0.000639325521280822),
 .UNSPECIFIED.);
#4489=B_SPLINE_CURVE_WITH_KNOTS('',3,(#142454,#142455,#142456,#142457),
 .UNSPECIFIED.,.F.,.F.,(4,4),(0.,0.0174508326761739),.UNSPECIFIED.);
#4490=B_SPLINE_CURVE_WITH_KNOTS('',3,(#142459,#142460,#142461,#142462,#142463,
#142464,#142465,#142466,#142467,#142468,#142469,#142470,#142471,#142472,
#142473,#142474,#142475,#142476,#142477,#142478,#142479,#142480,#142481,
#142482,#142483,#142484,#142485,#142486),.UNSPECIFIED.,.F.,.F.,(4,3,3,3,
3,3,3,3,3,4),(0.,0.000662679024145193,0.00128919539297308,0.00132535804829039,
0.00193492508883213,0.00253635637125076,0.00265071609658077,0.00397607414487116,
0.00508368314709806,0.00530143219316154),.UNSPECIFIED.);
#4491=B_SPLINE_CURVE_WITH_KNOTS('',3,(#142490,#142491,#142492,#142493,#142494,
#142495,#142496,#142497,#142498,#142499,#142500,#142501,#142502,#142503,
#142504,#142505),.UNSPECIFIED.,.F.,.F.,(4,3,3,3,3,4),(0.,0.00121734210048524,
0.00132677154899614,0.00265354309799227,0.00411654704464283,0.00530708619598447),
 .UNSPECIFIED.);
#4492=B_SPLINE_CURVE_WITH_KNOTS('',3,(#142507,#142508,#142509,#142510),
 .UNSPECIFIED.,.F.,.F.,(4,4),(0.,0.0177264565684136),.UNSPECIFIED.);
#4493=B_SPLINE_CURVE_WITH_KNOTS('',3,(#142512,#142513,#142514,#142515,#142516,
#142517,#142518,#142519,#142520,#142521,#142522,#142523,#142524),
 .UNSPECIFIED.,.F.,.F.,(4,3,3,3,4),(0.,0.000168209862999138,0.000320350766922646,
0.000480537459018473,0.000640701533845293),.UNSPECIFIED.);
#4494=B_SPLINE_CURVE_WITH_KNOTS('',3,(#142555,#142556,#142557,#142558,#142559,
#142560,#142561,#142562),.UNSPECIFIED.,.F.,.F.,(4,2,2,4),(-0.0847651026480947,
-0.0629186902711198,-0.0307386998646501,0.),.UNSPECIFIED.);
#4495=B_SPLINE_CURVE_WITH_KNOTS('',3,(#142563,#142564,#142565,#142566,#142567,
#142568,#142569,#142570),.UNSPECIFIED.,.F.,.F.,(4,2,2,4),(-0.16953083368722,
-0.138777607634066,-0.106603528596837,-0.0847654169752063),
 .UNSPECIFIED.);
#4496=B_SPLINE_CURVE_WITH_KNOTS('',3,(#142616,#142617,#142618,#142619,#142620,
#142621,#142622,#142623,#142624,#142625,#142626,#142627,#142628,#142629,
#142630,#142631,#142632,#142633,#142634,#142635,#142636,#142637,#142638,
#142639,#142640,#142641),.UNSPECIFIED.,.F.,.F.,(4,2,2,2,2,2,2,2,2,2,2,2,
4),(0.,0.035098338728144,0.0741581944022324,0.101946776653776,0.109514391089664,
0.117640234446691,0.136341904849524,0.141182675691644,0.160390411163872,
0.193626235421715,0.217667420358703,0.251529378123532,0.282413954967513),
 .UNSPECIFIED.);
#4497=B_SPLINE_CURVE_WITH_KNOTS('',3,(#142644,#142645,#142646,#142647,#142648,
#142649,#142650,#142651,#142652,#142653,#142654,#142655,#142656,#142657,
#142658,#142659,#142660,#142661),.UNSPECIFIED.,.F.,.F.,(4,2,2,2,2,2,2,2,
4),(0.,0.0302664700381103,0.0628248024585381,0.085474523550968,0.116272737380296,
0.147052923761435,0.169708349890063,0.202281537927324,0.232545593042104),
 .UNSPECIFIED.);
#4498=B_SPLINE_CURVE_WITH_KNOTS('',3,(#142711,#142712,#142713,#142714,#142715,
#142716,#142717,#142718,#142719,#142720),.UNSPECIFIED.,.F.,.F.,(4,2,2,2,
4),(0.,0.25,0.5,0.75,1.),.UNSPECIFIED.);
#4499=B_SPLINE_CURVE_WITH_KNOTS('',3,(#142742,#142743,#142744,#142745,#142746,
#142747),.UNSPECIFIED.,.F.,.F.,(4,2,4),(0.,0.5,1.),.UNSPECIFIED.);
#4500=B_SPLINE_CURVE_WITH_KNOTS('',3,(#142766,#142767,#142768,#142769),
 .UNSPECIFIED.,.F.,.F.,(4,4),(0.,1.),.UNSPECIFIED.);
#4501=B_SPLINE_CURVE_WITH_KNOTS('',3,(#142788,#142789,#142790,#142791,#142792,
#142793),.UNSPECIFIED.,.F.,.F.,(4,2,4),(0.,0.5,1.),.UNSPECIFIED.);
#4502=B_SPLINE_CURVE_WITH_KNOTS('',3,(#142942,#142943,#142944,#142945,#142946,
#142947,#142948,#142949,#142950,#142951,#142952,#142953,#142954,#142955,
#142956,#142957,#142958,#142959,#142960,#142961,#142962,#142963,#142964,
#142965,#142966,#142967,#142968,#142969),.UNSPECIFIED.,.F.,.F.,(4,3,3,3,
3,3,3,3,3,4),(0.,0.096881526972298,0.197661145229223,0.299127849036553,
0.40238568979424,0.5,0.640715041917235,0.780973931021849,0.919960936066223,
0.999999999999993),.UNSPECIFIED.);
#4503=B_SPLINE_CURVE_WITH_KNOTS('',3,(#143007,#143008,#143009,#143010,#143011,
#143012,#143013,#143014,#143015,#143016,#143017,#143018,#143019,#143020,
#143021,#143022),.UNSPECIFIED.,.F.,.F.,(4,3,3,3,3,4),(0.000681462205008639,
0.00273329612790008,0.00491895821256213,0.00671017185179961,0.00912678453081515,
0.00930288319891504),.UNSPECIFIED.);
#4504=B_SPLINE_CURVE_WITH_KNOTS('',3,(#143058,#143059,#143060,#143061,#143062,
#143063,#143064,#143065,#143066,#143067,#143068,#143069,#143070),
 .UNSPECIFIED.,.F.,.F.,(4,3,3,3,4),(0.000775072234384454,0.00360015924840977,
0.00665118856909886,0.00786282367425579,0.0104581756611108),
 .UNSPECIFIED.);
#4505=B_SPLINE_CURVE_WITH_KNOTS('',3,(#143156,#143157,#143158,#143159,#143160,
#143161,#143162,#143163,#143164,#143165),.UNSPECIFIED.,.F.,.F.,(4,2,2,2,
4),(0.,0.250000000000004,0.5,0.750000000000003,1.),.UNSPECIFIED.);
#4506=B_SPLINE_CURVE_WITH_KNOTS('',3,(#143200,#143201,#143202,#143203,#143204,
#143205,#143206,#143207,#143208,#143209,#143210,#143211,#143212),
 .UNSPECIFIED.,.F.,.F.,(4,3,3,3,4),(4.71238898038469,5.10508806208342,5.49778714378214,
5.89048622548087,6.28318530717959),.UNSPECIFIED.);
#4507=B_SPLINE_CURVE_WITH_KNOTS('',3,(#143235,#143236,#143237,#143238,#143239,
#143240,#143241,#143242,#143243,#143244,#143245,#143246,#143247),
 .UNSPECIFIED.,.F.,.F.,(4,3,3,3,4),(0.,0.00157041135329281,0.00191432655883667,
0.00304584187046407,0.00382865311767335),.UNSPECIFIED.);
#4508=B_SPLINE_CURVE_WITH_KNOTS('',3,(#143253,#143254,#143255,#143256,#143257,
#143258,#143259),.UNSPECIFIED.,.F.,.F.,(4,3,4),(4.71238898038469,5.49778714378214,
6.28318530717959),.UNSPECIFIED.);
#4509=B_SPLINE_CURVE_WITH_KNOTS('',3,(#143263,#143264,#143265,#143266,#143267,
#143268,#143269),.UNSPECIFIED.,.F.,.F.,(4,3,4),(3.1415926535898,3.92699081698724,
4.71238898038469),.UNSPECIFIED.);
#4510=B_SPLINE_CURVE_WITH_KNOTS('',3,(#143277,#143278,#143279,#143280,#143281,
#143282,#143283),.UNSPECIFIED.,.F.,.F.,(4,3,4),(4.71238898038469,5.49778714378214,
6.28318530717959),.UNSPECIFIED.);
#4511=B_SPLINE_CURVE_WITH_KNOTS('',3,(#143287,#143288,#143289,#143290,#143291,
#143292,#143293),.UNSPECIFIED.,.F.,.F.,(4,3,4),(1.23467863058847E-16,0.785398163397447,
1.5707963267949),.UNSPECIFIED.);
#4512=B_SPLINE_CURVE_WITH_KNOTS('',3,(#143299,#143300,#143301,#143302),
 .UNSPECIFIED.,.F.,.F.,(4,4),(0.,1.),.UNSPECIFIED.);
#4513=B_SPLINE_CURVE_WITH_KNOTS('',3,(#143305,#143306,#143307,#143308,#143309,
#143310),.UNSPECIFIED.,.F.,.F.,(4,2,4),(0.,0.5,1.),.UNSPECIFIED.);
#4514=B_SPLINE_CURVE_WITH_KNOTS('',3,(#143319,#143320,#143321,#143322,#143323,
#143324,#143325,#143326,#143327,#143328,#143329,#143330,#143331,#143332,
#143333,#143334,#143335,#143336,#143337,#143338,#143339,#143340,#143341,
#143342,#143343,#143344,#143345,#143346,#143347,#143348,#143349,#143350,
#143351,#143352,#143353,#143354,#143355,#143356,#143357,#143358,#143359,
#143360,#143361,#143362,#143363,#143364),.UNSPECIFIED.,.F.,.F.,(4,3,3,3,
3,3,3,3,3,3,3,3,3,3,3,4),(0.,0.000109331983970022,0.000221348099123313,
0.000333853905447977,0.000407294015799104,0.000408910815664253,0.000676681051235422,
0.000814588031598208,0.000816767951597532,0.00106247378106521,0.00122188204739731,
0.00122336180785488,0.0013543902429315,0.00149178315306396,0.00162097073973742,
0.00162917606319641),.UNSPECIFIED.);
#4515=B_SPLINE_CURVE_WITH_KNOTS('',3,(#143372,#143373,#143374,#143375,#143376,
#143377,#143378,#143379),.UNSPECIFIED.,.F.,.F.,(4,2,2,4),(0.,0.25,0.5,1.),
 .UNSPECIFIED.);
#4516=B_SPLINE_CURVE_WITH_KNOTS('',3,(#143383,#143384,#143385,#143386,#143387,
#143388),.UNSPECIFIED.,.F.,.F.,(4,2,4),(0.,0.500000000000002,1.),
 .UNSPECIFIED.);
#4517=B_SPLINE_CURVE_WITH_KNOTS('',3,(#143398,#143399,#143400,#143401,#143402,
#143403,#143404,#143405,#143406,#143407,#143408,#143409,#143410,#143411,
#143412,#143413,#143414,#143415,#143416,#143417,#143418,#143419,#143420,
#143421,#143422,#143423,#143424,#143425,#143426,#143427,#143428,#143429,
#143430,#143431,#143432,#143433,#143434,#143435,#143436,#143437,#143438,
#143439,#143440),.UNSPECIFIED.,.F.,.F.,(4,3,3,3,3,3,3,3,3,3,3,3,3,3,4),
(0.,0.000108912497168548,0.000220164732383848,0.000331071157537683,0.000392199517465978,
0.000393776648066525,0.000641215708234082,0.000785392845861507,0.000787553296133051,
0.0010345334193873,0.00117987002828322,0.00118132994419958,0.00130742143740802,
0.00144126401483706,0.0015751065922661),.UNSPECIFIED.);
#4518=B_SPLINE_CURVE_WITH_KNOTS('',3,(#143444,#143445,#143446,#143447,#143448,
#143449,#143450,#143451),.UNSPECIFIED.,.F.,.F.,(4,2,2,4),(0.,0.499999999999999,
0.749999999999998,1.),.UNSPECIFIED.);
#4519=B_SPLINE_CURVE_WITH_KNOTS('',3,(#143459,#143460,#143461,#143462,#143463,
#143464,#143465,#143466),.UNSPECIFIED.,.F.,.F.,(4,2,2,4),(0.,0.25,0.5,1.),
 .UNSPECIFIED.);
#4520=B_SPLINE_CURVE_WITH_KNOTS('',3,(#143470,#143471,#143472,#143473,#143474,
#143475,#143476,#143477,#143478,#143479,#143480,#143481,#143482,#143483,
#143484,#143485,#143486,#143487,#143488,#143489,#143490,#143491,#143492,
#143493,#143494,#143495,#143496,#143497,#143498,#143499,#143500,#143501,
#143502,#143503,#143504,#143505,#143506,#143507,#143508,#143509),
 .UNSPECIFIED.,.F.,.F.,(4,3,3,3,3,3,3,3,3,3,3,3,3,4),(0.,0.000424781762265252,
0.000463398440131748,0.000464821262797085,0.000754099901313884,0.000926796880263496,
0.000929181095996172,0.0011584961003294,0.00116090942630384,0.00139019532039531,
0.00139219601406769,0.00155797632198516,0.00171877163857689,0.00185359376052713),
 .UNSPECIFIED.);
#4521=B_SPLINE_CURVE_WITH_KNOTS('',3,(#143517,#143518,#143519,#143520,#143521,
#143522,#143523,#143524,#143525,#143526,#143527,#143528,#143529,#143530,
#143531,#143532,#143533,#143534,#143535,#143536,#143537,#143538,#143539,
#143540,#143541,#143542,#143543,#143544,#143545,#143546,#143547,#143548,
#143549,#143550,#143551,#143552,#143553,#143554,#143555,#143556,#143557,
#143558,#143559,#143560,#143561,#143562,#143563,#143564,#143565),
 .UNSPECIFIED.,.F.,.F.,(4,3,3,3,3,3,3,3,3,3,3,3,3,3,3,3,4),(0.,8.46514984579067E-5,
0.000170997186917714,0.000221020978416691,0.00025513917286035,0.0003380084618147,
0.000429234945596046,0.000448835576014519,0.000450677949086267,0.000735348747775932,
0.000898977028079799,0.000901355898172495,0.0011519668249772,0.00135049620570088,
0.00135203384725872,0.00157737282180184,0.00180271179634495),
 .UNSPECIFIED.);
#4522=B_SPLINE_CURVE_WITH_KNOTS('',3,(#143569,#143570,#143571,#143572,#143573,
#143574),.UNSPECIFIED.,.F.,.F.,(4,2,4),(0.,0.499999999999999,1.),
 .UNSPECIFIED.);
#4523=B_SPLINE_CURVE_WITH_KNOTS('',3,(#143582,#143583,#143584,#143585),
 .UNSPECIFIED.,.F.,.F.,(4,4),(0.,1.),.UNSPECIFIED.);
#4524=B_SPLINE_CURVE_WITH_KNOTS('',3,(#143587,#143588,#143589,#143590),
 .UNSPECIFIED.,.F.,.F.,(4,4),(0.,1.),.UNSPECIFIED.);
#4525=B_SPLINE_CURVE_WITH_KNOTS('',3,(#143594,#143595,#143596,#143597,#143598,
#143599,#143600,#143601,#143602,#143603,#143604,#143605,#143606,#143607,
#143608,#143609,#143610,#143611,#143612,#143613,#143614,#143615,#143616,
#143617,#143618,#143619,#143620,#143621,#143622,#143623,#143624,#143625,
#143626,#143627,#143628,#143629,#143630,#143631,#143632,#143633,#143634,
#143635,#143636,#143637,#143638,#143639),.UNSPECIFIED.,.F.,.F.,(4,3,3,3,
3,3,3,3,3,3,3,3,3,3,3,4),(0.,0.00011167181015014,0.000225567853890617,0.000339431029143606,
0.000397399329631602,0.000398944559102931,0.000667283904097484,0.000794798659263204,
0.000796933919810637,0.00104488468555027,0.00119219798889481,0.00119368499584663,
0.00132317769579387,0.00145638750716014,0.00158130618071513,0.00158959731852641),
 .UNSPECIFIED.);
#4526=B_SPLINE_CURVE_WITH_KNOTS('',3,(#143647,#143648,#143649,#143650,#143651,
#143652,#143653,#143654,#143655,#143656,#143657,#143658,#143659,#143660,
#143661,#143662,#143663,#143664,#143665,#143666,#143667,#143668,#143669,
#143670,#143671,#143672,#143673,#143674,#143675,#143676,#143677,#143678,
#143679,#143680,#143681,#143682,#143683,#143684,#143685,#143686,#143687,
#143688,#143689),.UNSPECIFIED.,.F.,.F.,(4,3,3,3,3,3,3,3,3,3,3,3,3,3,4),
(0.,0.000167563212024588,0.000333534252401052,0.000405329103688545,0.000406806783530084,
0.000681033266852063,0.000811430892222414,0.000813613567060169,0.00109814343427173,
0.00121879730292854,0.00122042035059025,0.00134667139739561,0.00147140108610396,
0.00159377061182622,0.00162722713412034),.UNSPECIFIED.);
#4527=B_SPLINE_CURVE_WITH_KNOTS('',3,(#143692,#143693,#143694,#143695),
 .UNSPECIFIED.,.F.,.F.,(4,4),(0.,1.),.UNSPECIFIED.);
#4528=B_SPLINE_CURVE_WITH_KNOTS('',3,(#143700,#143701,#143702,#143703),
 .UNSPECIFIED.,.F.,.F.,(4,4),(0.,1.),.UNSPECIFIED.);
#4529=B_SPLINE_CURVE_WITH_KNOTS('',3,(#143706,#143707,#143708,#143709,#143710,
#143711),.UNSPECIFIED.,.F.,.F.,(4,2,4),(0.,0.5,1.),.UNSPECIFIED.);
#4530=B_SPLINE_CURVE_WITH_KNOTS('',3,(#143719,#143720,#143721,#143722,#143723,
#143724,#143725),.UNSPECIFIED.,.F.,.F.,(4,3,4),(1.5707963267949,2.35619449019235,
3.1415926535898),.UNSPECIFIED.);
#4531=B_SPLINE_CURVE_WITH_KNOTS('',3,(#143729,#143730,#143731,#143732,#143733,
#143734,#143735),.UNSPECIFIED.,.F.,.F.,(4,3,4),(1.23467863058848E-16,0.785398163397447,
1.5707963267949),.UNSPECIFIED.);
#4532=B_SPLINE_CURVE_WITH_KNOTS('',3,(#143740,#143741,#143742,#143743,#143744,
#143745,#143746,#143747,#143748,#143749,#143750,#143751,#143752),
 .UNSPECIFIED.,.F.,.F.,(4,3,3,3,4),(6.93889390390723E-18,0.00113151531066751,
0.00191432655883665,0.00348473784368841,0.00382865311767331),
 .UNSPECIFIED.);
#4533=B_SPLINE_CURVE_WITH_KNOTS('',3,(#143760,#143761,#143762,#143763,#143764,
#143765,#143766),.UNSPECIFIED.,.F.,.F.,(4,3,4),(4.71238898038468,5.49778714378213,
6.28318530717959),.UNSPECIFIED.);
#4534=B_SPLINE_CURVE_WITH_KNOTS('',3,(#143770,#143771,#143772,#143773,#143774,
#143775,#143776),.UNSPECIFIED.,.F.,.F.,(4,3,4),(1.23467863058848E-16,0.785398163397447,
1.5707963267949),.UNSPECIFIED.);
#4535=B_SPLINE_CURVE_WITH_KNOTS('',3,(#143794,#143795,#143796,#143797,#143798,
#143799,#143800,#143801,#143802,#143803,#143804,#143805,#143806),
 .UNSPECIFIED.,.F.,.F.,(4,3,3,3,4),(0.,0.0015008721912107,0.00207200756106571,
0.00310801134159857,0.00414401512213143),.UNSPECIFIED.);
#4536=B_SPLINE_CURVE_WITH_KNOTS('',3,(#143812,#143813,#143814,#143815,#143816,
#143817,#143818),.UNSPECIFIED.,.F.,.F.,(4,3,4),(4.71238898038468,5.49778714378214,
6.28318530717959),.UNSPECIFIED.);
#4537=B_SPLINE_CURVE_WITH_KNOTS('',3,(#143822,#143823,#143824,#143825,#143826,
#143827,#143828),.UNSPECIFIED.,.F.,.F.,(4,3,4),(3.14159265358979,3.92699081698724,
4.71238898038469),.UNSPECIFIED.);
#4538=B_SPLINE_CURVE_WITH_KNOTS('',3,(#143836,#143837,#143838,#143839,#143840,
#143841,#143842),.UNSPECIFIED.,.F.,.F.,(4,3,4),(4.71238898038469,5.49778714378214,
6.28318530717959),.UNSPECIFIED.);
#4539=B_SPLINE_CURVE_WITH_KNOTS('',3,(#143846,#143847,#143848,#143849,#143850,
#143851,#143852),.UNSPECIFIED.,.F.,.F.,(4,3,4),(-8.88178419700125E-16,0.78539816339745,
1.5707963267949),.UNSPECIFIED.);
#4540=B_SPLINE_CURVE_WITH_KNOTS('',3,(#144008,#144009,#144010,#144011,#144012,
#144013,#144014),.UNSPECIFIED.,.F.,.F.,(4,3,4),(0.,0.619995026988033,0.999999394204749),
 .UNSPECIFIED.);
#4541=B_SPLINE_CURVE_WITH_KNOTS('',3,(#144015,#144016,#144017,#144018),
 .UNSPECIFIED.,.F.,.F.,(4,4),(0.,1.),.UNSPECIFIED.);
#4542=B_SPLINE_CURVE_WITH_KNOTS('',3,(#144062,#144063,#144064,#144065,#144066,
#144067),.UNSPECIFIED.,.F.,.F.,(4,2,4),(0.,0.567644438072849,1.),
 .UNSPECIFIED.);
#4543=B_SPLINE_CURVE_WITH_KNOTS('',3,(#144068,#144069,#144070,#144071),
 .UNSPECIFIED.,.F.,.F.,(4,4),(0.,1.),.UNSPECIFIED.);
#4544=B_SPLINE_CURVE_WITH_KNOTS('',3,(#144128,#144129,#144130,#144131,#144132,
#144133,#144134,#144135,#144136,#144137,#144138,#144139,#144140,#144141),
 .UNSPECIFIED.,.F.,.F.,(4,2,2,2,2,2,4),(0.,0.240475312512509,0.367062760427093,
0.493650208341673,0.620237656256254,0.746825104170835,1.),.UNSPECIFIED.);
#4545=B_SPLINE_CURVE_WITH_KNOTS('',3,(#144156,#144157,#144158,#144159,#144160,
#144161,#144162,#144163,#144164,#144165,#144166,#144167,#144168,#144169),
 .UNSPECIFIED.,.F.,.F.,(4,2,2,2,2,2,4),(0.,0.251505324083449,0.377257986125173,
0.503010648166897,0.628763310208625,0.75451597225035,1.),.UNSPECIFIED.);
#4546=B_SPLINE_CURVE_WITH_KNOTS('',3,(#144170,#144171,#144172,#144173),
 .UNSPECIFIED.,.F.,.F.,(4,4),(0.020578988719059,0.0210794636037261),
 .UNSPECIFIED.);
#4547=B_SPLINE_CURVE_WITH_KNOTS('',3,(#144232,#144233,#144234,#144235,#144236,
#144237,#144238,#144239,#144240,#144241,#144242,#144243),.UNSPECIFIED.,
 .F.,.F.,(4,2,3,3,4),(0.,0.00100000000000208,0.00500000000023154,0.02100000001009,
0.0385835581099273),.UNSPECIFIED.);
#4548=B_SPLINE_CURVE_WITH_KNOTS('',3,(#144245,#144246,#144247,#144248,#144249,
#144250,#144251,#144252),.UNSPECIFIED.,.F.,.F.,(4,2,2,4),(0.,0.251717747068591,
0.509550086771184,1.),.UNSPECIFIED.);
#4549=B_SPLINE_CURVE_WITH_KNOTS('',3,(#144291,#144292,#144293,#144294,#144295,
#144296),.UNSPECIFIED.,.F.,.F.,(4,2,4),(0.,0.5,1.),.UNSPECIFIED.);
#4550=B_SPLINE_CURVE_WITH_KNOTS('',3,(#144316,#144317,#144318,#144319,#144320,
#144321),.UNSPECIFIED.,.F.,.F.,(4,2,4),(0.,0.5,1.),.UNSPECIFIED.);
#4551=B_SPLINE_CURVE_WITH_KNOTS('',3,(#144405,#144406,#144407,#144408,#144409,
#144410,#144411,#144412,#144413,#144414,#144415,#144416,#144417,#144418,
#144419,#144420,#144421,#144422,#144423,#144424,#144425,#144426,#144427,
#144428,#144429),.UNSPECIFIED.,.F.,.F.,(4,3,3,3,3,3,3,3,4),(0.000524342078796179,
0.00180901876828853,0.00304673005325099,0.00340077219985262,0.00411987972637406,
0.00482370949852814,0.00550912189802027,0.00616177752105426,0.00627720230593839),
 .UNSPECIFIED.);
#4552=B_SPLINE_CURVE_WITH_KNOTS('',3,(#144430,#144431,#144432,#144433,#144434,
#144435,#144436),.UNSPECIFIED.,.F.,.F.,(4,3,4),(0.,0.500000000000002,0.999999986878769),
 .UNSPECIFIED.);
#4553=B_SPLINE_CURVE_WITH_KNOTS('',3,(#144492,#144493,#144494,#144495,#144496,
#144497,#144498,#144499,#144500,#144501,#144502,#144503,#144504,#144505,
#144506,#144507,#144508,#144509,#144510,#144511,#144512,#144513,#144514,
#144515,#144516),.UNSPECIFIED.,.F.,.F.,(4,3,3,3,3,3,3,3,4),(0.,0.141656513734972,
0.284805721555512,0.429042216431012,0.499999999999999,0.655877906767802,
0.811014022503117,0.965340744220155,1.),.UNSPECIFIED.);
#4554=B_SPLINE_CURVE_WITH_KNOTS('',3,(#144580,#144581,#144582,#144583,#144584,
#144585,#144586,#144587,#144588,#144589,#144590,#144591,#144592,#144593,
#144594,#144595,#144596,#144597,#144598,#144599,#144600,#144601,#144602,
#144603,#144604),.UNSPECIFIED.,.F.,.F.,(4,3,3,3,3,3,3,3,4),(0.,0.135948715488849,
0.27312999148841,0.411116711101826,0.5,0.651860141828472,0.802504749805492,
0.951647349185892,1.),.UNSPECIFIED.);
#4555=B_SPLINE_CURVE_WITH_KNOTS('',3,(#144627,#144628,#144629,#144630,#144631,
#144632),.UNSPECIFIED.,.F.,.F.,(4,2,4),(0.,0.5,1.),.UNSPECIFIED.);
#4556=B_SPLINE_CURVE_WITH_KNOTS('',3,(#144652,#144653,#144654,#144655,#144656,
#144657,#144658,#144659,#144660,#144661,#144662,#144663,#144664,#144665,
#144666,#144667),.UNSPECIFIED.,.F.,.F.,(4,3,3,3,3,4),(0.000601267884717356,
0.00181647811677124,0.00299735824906937,0.00382211018819771,0.00557536121785049,
0.00704295249167806),.UNSPECIFIED.);
#4557=B_SPLINE_CURVE_WITH_KNOTS('',3,(#144729,#144730,#144731,#144732,#144733,
#144734,#144735,#144736,#144737,#144738,#144739,#144740,#144741,#144742,
#144743,#144744,#144745,#144746,#144747,#144748,#144749,#144750,#144751,
#144752,#144753,#144754,#144755,#144756),.UNSPECIFIED.,.F.,.F.,(4,3,3,3,
3,3,3,3,3,4),(0.,0.113371007866148,0.229897420767909,0.347745026578629,
0.466701720784187,0.5,0.642794296332829,0.784841419789057,0.925820243963234,
0.999999999999991),.UNSPECIFIED.);
#4558=B_SPLINE_CURVE_WITH_KNOTS('',3,(#144831,#144832,#144833,#144834,#144835,
#144836,#144837,#144838,#144839,#144840,#144841,#144842,#144843,#144844,
#144845,#144846,#144847,#144848,#144849,#144850,#144851,#144852,#144853,
#144854,#144855,#144856,#144857,#144858),.UNSPECIFIED.,.F.,.F.,(4,3,3,3,
3,3,3,3,3,4),(0.,0.113914306204002,0.229749700148325,0.34594430565268,0.461668871939815,
0.5,0.63174105075801,0.760423146797041,0.884931285751174,1.),
 .UNSPECIFIED.);
#4559=B_SPLINE_CURVE_WITH_KNOTS('',3,(#144881,#144882,#144883,#144884,#144885,
#144886),.UNSPECIFIED.,.F.,.F.,(4,2,4),(1.29812701169007E-5,0.500000000000001,
1.),.UNSPECIFIED.);
#4560=B_SPLINE_CURVE_WITH_KNOTS('',3,(#144912,#144913,#144914,#144915,#144916,
#144917,#144918,#144919,#144920,#144921,#144922,#144923,#144924,#144925,
#144926,#144927),.UNSPECIFIED.,.F.,.F.,(4,3,3,3,3,4),(0.000694356721436431,
0.00259637723191676,0.00305563622484014,0.00480503978353657,0.00647539340150566,
0.00814574701947475),.UNSPECIFIED.);
#4561=B_SPLINE_CURVE_WITH_KNOTS('',3,(#144989,#144990,#144991,#144992,#144993,
#144994,#144995,#144996,#144997,#144998,#144999,#145000,#145001,#145002,
#145003,#145004,#145005,#145006,#145007,#145008,#145009,#145010,#145011,
#145012,#145013,#145014,#145015,#145016,#145017,#145018,#145019),
 .UNSPECIFIED.,.F.,.F.,(4,3,3,3,3,3,3,3,3,3,4),(0.,0.0881043395261828,0.178030981308937,
0.270574666304827,0.364321258892522,0.459368561145583,0.500000000000001,
0.64789166764264,0.797396677123148,0.945384894755191,1.),.UNSPECIFIED.);
#4562=B_SPLINE_CURVE_WITH_KNOTS('',3,(#145043,#145044,#145045,#145046,#145047,
#145048,#145049),.UNSPECIFIED.,.F.,.F.,(4,3,4),(0.,0.640590439740815,0.999999469629731),
 .UNSPECIFIED.);
#4563=B_SPLINE_CURVE_WITH_KNOTS('',3,(#145050,#145051,#145052,#145053),
 .UNSPECIFIED.,.F.,.F.,(4,4),(0.,1.),.UNSPECIFIED.);
#4564=B_SPLINE_CURVE_WITH_KNOTS('',3,(#145128,#145129,#145130,#145131,#145132,
#145133,#145134,#145135,#145136,#145137,#145138,#145139,#145140,#145141,
#145142,#145143,#145144,#145145,#145146,#145147,#145148,#145149,#145150,
#145151,#145152,#145153,#145154,#145155,#145156,#145157,#145158),
 .UNSPECIFIED.,.F.,.F.,(4,3,3,3,3,3,3,3,3,3,4),(8.28401126087789E-15,0.103891034062219,
0.209333681833554,0.314870836921643,0.419526492710104,0.5,0.61507405516711,
0.725151653805686,0.832721765547754,0.937002679485264,1.),.UNSPECIFIED.);
#4565=B_SPLINE_CURVE_WITH_KNOTS('',3,(#145272,#145273,#145274,#145275,#145276,
#145277,#145278,#145279,#145280,#145281),.UNSPECIFIED.,.F.,.F.,(4,2,2,2,
4),(0.,0.25,0.5,0.75,1.),.UNSPECIFIED.);
#4566=B_SPLINE_CURVE_WITH_KNOTS('',3,(#145320,#145321,#145322,#145323,#145324,
#145325),.UNSPECIFIED.,.F.,.F.,(4,2,4),(0.,0.5,1.),.UNSPECIFIED.);
#4567=B_SPLINE_CURVE_WITH_KNOTS('',3,(#145346,#145347,#145348,#145349,#145350,
#145351),.UNSPECIFIED.,.F.,.F.,(4,2,4),(0.,0.5,0.999999988140019),
 .UNSPECIFIED.);
#4568=B_SPLINE_CURVE_WITH_KNOTS('',3,(#145375,#145376,#145377,#145378,#145379,
#145380,#145381,#145382,#145383,#145384,#145385,#145386,#145387,#145388,
#145389,#145390,#145391,#145392,#145393,#145394,#145395,#145396,#145397,
#145398,#145399,#145400,#145401,#145402,#145403,#145404,#145405),
 .UNSPECIFIED.,.F.,.F.,(4,3,3,3,3,3,3,3,3,3,4),(0.,0.0841106566558007,0.169966621792399,
0.258433889273308,0.348104167089326,0.439210954526272,0.500000000000001,
0.653513844289969,0.813728745872899,0.971758040989338,0.999999999999993),
 .UNSPECIFIED.);
#4569=B_SPLINE_CURVE_WITH_KNOTS('',3,(#145449,#145450,#145451,#145452,#145453,
#145454,#145455,#145456,#145457,#145458,#145459,#145460,#145461,#145462,
#145463,#145464,#145465,#145466,#145467),.UNSPECIFIED.,.F.,.F.,(4,3,3,3,
3,3,4),(0.000636256268971442,0.00222779634230967,0.003876291264432,0.0056280359891258,
0.00591708699638704,0.00780896916228463,0.00825282706815076),
 .UNSPECIFIED.);
#4570=B_SPLINE_CURVE_WITH_KNOTS('',3,(#145468,#145469,#145470,#145471,#145472,
#145473,#145474,#145475,#145476,#145477,#145478,#145479,#145480,#145481,
#145482,#145483,#145484,#145485,#145486,#145487,#145488,#145489,#145490,
#145491,#145492,#145493,#145494,#145495,#145496,#145497,#145498),
 .UNSPECIFIED.,.F.,.F.,(4,3,3,3,3,3,3,3,3,3,4),(4.68648016623899E-15,0.110926165634124,
0.223711806532316,0.336827055115305,0.449445226496388,0.5,0.627102535999364,
0.751142482631481,0.87557124131574,0.993677341969705,1.),.UNSPECIFIED.);
#4571=B_SPLINE_CURVE_WITH_KNOTS('',3,(#145561,#145562,#145563,#145564,#145565,
#145566),.UNSPECIFIED.,.F.,.F.,(4,2,4),(1.4856211342407E-5,0.5,1.),
 .UNSPECIFIED.);
#4572=B_SPLINE_CURVE_WITH_KNOTS('',3,(#145587,#145588,#145589,#145590,#145591,
#145592),.UNSPECIFIED.,.F.,.F.,(4,2,4),(0.,0.500000000000001,1.),
 .UNSPECIFIED.);
#4573=B_SPLINE_CURVE_WITH_KNOTS('',3,(#145614,#145615,#145616,#145617,#145618,
#145619,#145620,#145621),.UNSPECIFIED.,.F.,.F.,(4,2,2,4),(0.,0.5,0.75,1.),
 .UNSPECIFIED.);
#4574=B_SPLINE_CURVE_WITH_KNOTS('',3,(#145666,#145667,#145668,#145669),
 .UNSPECIFIED.,.F.,.F.,(4,4),(0.,1.),.UNSPECIFIED.);
#4575=B_SPLINE_CURVE_WITH_KNOTS('',3,(#145762,#145763,#145764,#145765,#145766,
#145767,#145768,#145769,#145770,#145771,#145772,#145773,#145774,#145775,
#145776,#145777,#145778,#145779,#145780,#145781,#145782,#145783,#145784,
#145785,#145786,#145787,#145788,#145789),.UNSPECIFIED.,.F.,.F.,(4,3,3,3,
3,3,3,3,3,4),(0.,0.109785608660835,0.222741427481541,0.337045865985497,
0.452594310492733,0.500000000000001,0.64133306133531,0.781868923872316,
0.921212099227518,1.),.UNSPECIFIED.);
#4576=B_SPLINE_CURVE_WITH_KNOTS('',3,(#145815,#145816,#145817,#145818,#145819,
#145820,#145821,#145822,#145823,#145824,#145825,#145826,#145827,#145828,
#145829,#145830,#145831,#145832,#145833),.UNSPECIFIED.,.F.,.F.,(4,3,3,3,
3,3,4),(0.000544979362130299,0.00239221479430278,0.00380801466457332,0.00469824400931087,
0.00578923755784658,0.00680407029599512,0.00707104996701635),
 .UNSPECIFIED.);
#4577=B_SPLINE_CURVE_WITH_KNOTS('',3,(#145834,#145835,#145836,#145837,#145838,
#145839,#145840,#145841,#145842,#145843,#145844,#145845,#145846,#145847,
#145848,#145849,#145850,#145851,#145852,#145853,#145854,#145855,#145856,
#145857,#145858),.UNSPECIFIED.,.F.,.F.,(4,3,3,3,3,3,3,3,4),(0.,0.133858617770367,
0.268928589573922,0.404818946884987,0.5,0.650059845006746,0.798865163431494,
0.946095668638004,1.),.UNSPECIFIED.);
#4578=B_SPLINE_CURVE_WITH_KNOTS('',3,(#145915,#145916,#145917,#145918,#145919,
#145920),.UNSPECIFIED.,.F.,.F.,(4,2,4),(0.,0.5,1.),.UNSPECIFIED.);
#4579=B_SPLINE_CURVE_WITH_KNOTS('',3,(#146000,#146001,#146002,#146003,#146004,
#146005,#146006,#146007,#146008,#146009,#146010,#146011,#146012,#146013),
 .UNSPECIFIED.,.F.,.F.,(4,2,2,2,2,2,4),(0.,0.25310390433008,0.379655856495117,
0.506207808660157,0.632759760825198,0.759311712990238,1.),.UNSPECIFIED.);
#4580=B_SPLINE_CURVE_WITH_KNOTS('',3,(#146014,#146015,#146016,#146017,#146018,
#146019,#146020,#146021,#146022,#146023),.UNSPECIFIED.,.F.,.F.,(4,2,2,2,
4),(0.,0.25,0.5,0.75,1.),.UNSPECIFIED.);
#4581=B_SPLINE_CURVE_WITH_KNOTS('',3,(#146029,#146030,#146031,#146032),
 .UNSPECIFIED.,.F.,.F.,(4,4),(0.00465289315641866,0.00515351125805147),
 .UNSPECIFIED.);
#4582=B_SPLINE_CURVE_WITH_KNOTS('',3,(#146105,#146106,#146107,#146108,#146109,
#146110,#146111,#146112,#146113,#146114,#146115,#146116,#146117,#146118,
#146119,#146120,#146121,#146122,#146123,#146124,#146125,#146126,#146127,
#146128,#146129,#146130,#146131,#146132,#146133,#146134,#146135,#146136,
#146137,#146138,#146139,#146140,#146141,#146142,#146143,#146144,#146145,
#146146,#146147),.UNSPECIFIED.,.F.,.F.,(4,3,3,3,3,3,3,3,3,3,3,3,3,3,4),
(0.,0.0632636272771733,0.127512975023493,0.193161069570627,0.250000000000002,
0.323161603585242,0.398727785487939,0.478054969239045,0.500000000000001,
0.583571175025073,0.670742277688246,0.764579159679674,0.862667985480895,
0.965751654555339,1.),.UNSPECIFIED.);
#4583=B_SPLINE_CURVE_WITH_KNOTS('',3,(#146204,#146205,#146206,#146207,#146208,
#146209,#146210),.UNSPECIFIED.,.F.,.F.,(4,3,4),(0.,0.500000000000006,1.),
 .UNSPECIFIED.);
#4584=B_SPLINE_CURVE_WITH_KNOTS('',3,(#146233,#146234,#146235,#146236,#146237,
#146238,#146239,#146240,#146241,#146242,#146243,#146244,#146245,#146246,
#146247,#146248,#146249,#146250,#146251,#146252,#146253,#146254,#146255,
#146256,#146257),.UNSPECIFIED.,.F.,.F.,(4,3,3,3,3,3,3,3,4),(0.,0.140179798979954,
0.281858061384262,0.424662898949861,0.499999999999999,0.654971604573252,
0.809174109715774,0.962522009696372,1.),.UNSPECIFIED.);
#4585=B_SPLINE_CURVE_WITH_KNOTS('',3,(#146277,#146278,#146279,#146280,#146281,
#146282,#146283,#146284,#146285,#146286,#146287,#146288,#146289,#146290,
#146291,#146292,#146293,#146294,#146295,#146296,#146297,#146298),
 .UNSPECIFIED.,.F.,.F.,(4,3,3,3,3,3,3,4),(0.000499308730788156,0.00146046002319833,
0.00243695586828934,0.00338583705476887,0.00376364965220018,0.00474984309182789,
0.00578812738994236,0.00627236538267016),.UNSPECIFIED.);
#4586=B_SPLINE_CURVE_WITH_KNOTS('',3,(#146359,#146360,#146361,#146362),
 .UNSPECIFIED.,.F.,.F.,(4,4),(0.,1.),.UNSPECIFIED.);
#4587=B_SPLINE_CURVE_WITH_KNOTS('',3,(#146422,#146423,#146424,#146425,#146426,
#146427,#146428,#146429,#146430,#146431,#146432,#146433,#146434,#146435,
#146436,#146437,#146438,#146439,#146440,#146441,#146442,#146443,#146444,
#146445,#146446,#146447,#146448,#146449,#146450,#146451,#146452,#146453,
#146454,#146455,#146456,#146457,#146458,#146459,#146460,#146461,#146462,
#146463,#146464,#146465,#146466,#146467),.UNSPECIFIED.,.F.,.F.,(4,3,3,3,
3,3,3,3,3,3,3,3,3,3,3,4),(0.,0.0915750010276041,0.131325095428788,0.212675685292389,
0.290151690513043,0.365784162784195,0.439131591082695,0.5,0.56919091022333,
0.637494190722665,0.705032480811157,0.75,0.816374271265617,0.882302233429591,
0.94798000078784,1.),.UNSPECIFIED.);
#4588=B_SPLINE_CURVE_WITH_KNOTS('',3,(#146530,#146531,#146532,#146533,#146534,
#146535,#146536,#146537,#146538,#146539,#146540,#146541),.UNSPECIFIED.,
 .F.,.F.,(4,2,2,2,2,4),(0.,0.25,0.375,0.5,0.75,1.),.UNSPECIFIED.);
#4589=B_SPLINE_CURVE_WITH_KNOTS('',3,(#146574,#146575,#146576,#146577),
 .UNSPECIFIED.,.F.,.F.,(4,4),(0.,1.),.UNSPECIFIED.);
#4590=B_SPLINE_CURVE_WITH_KNOTS('',3,(#146635,#146636,#146637,#146638,#146639,
#146640,#146641,#146642,#146643,#146644,#146645,#146646,#146647,#146648,
#146649,#146650,#146651,#146652,#146653,#146654,#146655,#146656,#146657,
#146658,#146659),.UNSPECIFIED.,.F.,.F.,(4,3,3,3,3,3,3,3,4),(0.000526414844798677,
0.0016264626269863,0.00270005642798455,0.00303445478718795,0.00340650091711803,
0.00424257270328544,0.00468441200509802,0.00552307032315886,0.0062865869894374),
 .UNSPECIFIED.);
#4591=B_SPLINE_CURVE_WITH_KNOTS('',3,(#146660,#146661,#146662,#146663,#146664,
#146665,#146666),.UNSPECIFIED.,.F.,.F.,(4,3,4),(0.,0.5,1.),
 .UNSPECIFIED.);
#4592=B_SPLINE_CURVE_WITH_KNOTS('',3,(#146723,#146724,#146725,#146726,#146727,
#146728,#146729,#146730,#146731,#146732,#146733,#146734,#146735,#146736,
#146737,#146738,#146739,#146740,#146741,#146742,#146743,#146744,#146745,
#146746,#146747),.UNSPECIFIED.,.F.,.F.,(4,3,3,3,3,3,3,3,4),(0.,0.140856133935696,
0.283205124587202,0.426655231031233,0.5,0.655301545313637,0.809843231900818,
0.963548210345928,1.),.UNSPECIFIED.);
#4593=B_SPLINE_CURVE_WITH_KNOTS('',3,(#146827,#146828,#146829,#146830,#146831,
#146832,#146833,#146834,#146835,#146836,#146837,#146838,#146839,#146840),
 .UNSPECIFIED.,.F.,.F.,(4,2,2,2,2,2,4),(0.,0.251497274344898,0.377245911517345,
0.502994548689796,0.628743185862243,0.754491823034691,1.),.UNSPECIFIED.);
#4594=B_SPLINE_CURVE_WITH_KNOTS('',3,(#146841,#146842,#146843,#146844,#146845,
#146846,#146847,#146848,#146849,#146850,#146851,#146852,#146853,#146854,
#146855,#146856,#146857,#146858,#146859,#146860,#146861,#146862,#146863,
#146864,#146865,#146866,#146867,#146868,#146869,#146870,#146871,#146872,
#146873,#146874,#146875,#146876,#146877,#146878,#146879,#146880,#146881,
#146882,#146883),.UNSPECIFIED.,.F.,.F.,(4,3,3,3,3,3,3,3,3,3,3,3,3,3,4),
(0.,0.0883066236689891,0.169881016966313,0.25,0.345565144469168,0.432992430689934,
0.5,0.579720574572057,0.657499747134168,0.73321670512183,0.75,0.821556884509131,
0.891976019923854,0.961324436963321,0.999999999999875),.UNSPECIFIED.);
#4595=B_SPLINE_CURVE_WITH_KNOTS('',3,(#146889,#146890,#146891,#146892),
 .UNSPECIFIED.,.F.,.F.,(4,4),(0.0209654295165786,0.0214659702660322),
 .UNSPECIFIED.);
#4596=B_SPLINE_CURVE_WITH_KNOTS('',3,(#146951,#146952,#146953,#146954,#146955,
#146956,#146957,#146958,#146959,#146960,#146961,#146962,#146963,#146964),
 .UNSPECIFIED.,.F.,.F.,(4,2,2,2,2,2,4),(0.,0.241136840065836,0.3676140333882,
0.49409122671056,0.62056842003292,0.74704561335528,1.),.UNSPECIFIED.);
#4597=B_SPLINE_CURVE_WITH_KNOTS('',3,(#146965,#146966,#146967,#146968,#146969,
#146970),.UNSPECIFIED.,.F.,.F.,(4,2,4),(0.,0.500000000000001,1.),
 .UNSPECIFIED.);
#4598=B_SPLINE_CURVE_WITH_KNOTS('',3,(#147027,#147028,#147029,#147030,#147031,
#147032,#147033,#147034,#147035,#147036,#147037,#147038,#147039,#147040,
#147041,#147042,#147043,#147044,#147045,#147046,#147047,#147048,#147049,
#147050,#147051),.UNSPECIFIED.,.F.,.F.,(4,3,3,3,3,3,3,3,4),(6.69029905996544E-15,
0.134488788622136,0.270199226691756,0.406736460097312,0.5,0.650772475386906,
0.800288993579067,0.9482361842095,1.),.UNSPECIFIED.);
#4599=B_SPLINE_CURVE_WITH_KNOTS('',3,(#147074,#147075,#147076,#147077,#147078,
#147079),.UNSPECIFIED.,.F.,.F.,(4,2,4),(0.,0.499999999999999,1.),
 .UNSPECIFIED.);
#4600=B_SPLINE_CURVE_WITH_KNOTS('',3,(#147105,#147106,#147107,#147108,#147109,
#147110,#147111,#147112,#147113,#147114,#147115,#147116,#147117,#147118,
#147119,#147120,#147121,#147122,#147123),.UNSPECIFIED.,.F.,.F.,(4,3,3,3,
3,3,4),(0.000609719129519901,0.00229610816230499,0.00296440479617456,0.00386266882834386,
0.00506716034621366,0.00622435639369392,0.00711561852716782),
 .UNSPECIFIED.);
#4601=B_SPLINE_CURVE_WITH_KNOTS('',3,(#147192,#147193,#147194,#147195,#147196,
#147197,#147198,#147199,#147200,#147201,#147202,#147203,#147204,#147205,
#147206,#147207,#147208,#147209,#147210,#147211,#147212,#147213,#147214,
#147215,#147216,#147217,#147218,#147219),.UNSPECIFIED.,.F.,.F.,(4,3,3,3,
3,3,3,3,3,4),(0.,0.110591919110538,0.224346970330222,0.339439967219989,
0.455737261262023,0.499999999999999,0.641794484661474,0.78280483557739,
0.922640336453395,1.),.UNSPECIFIED.);
#4602=B_SPLINE_CURVE_WITH_KNOTS('',3,(#147240,#147241,#147242,#147243,#147244,
#147245),.UNSPECIFIED.,.F.,.F.,(4,2,4),(0.,0.500000000000001,1.),
 .UNSPECIFIED.);
#4603=B_SPLINE_CURVE_WITH_KNOTS('',3,(#147269,#147270,#147271,#147272),
 .UNSPECIFIED.,.F.,.F.,(4,4),(0.,1.),.UNSPECIFIED.);
#4604=B_SPLINE_CURVE_WITH_KNOTS('',3,(#147315,#147316,#147317,#147318,#147319,
#147320,#147321,#147322,#147323,#147324,#147325,#147326,#147327,#147328,
#147329,#147330,#147331,#147332,#147333,#147334,#147335,#147336,#147337,
#147338,#147339,#147340,#147341,#147342,#147343,#147344,#147345,#147346,
#147347,#147348,#147349,#147350,#147351),.UNSPECIFIED.,.F.,.F.,(4,3,3,3,
3,3,3,3,3,3,3,3,4),(0.,0.0855121196768925,0.171061973228972,0.249999999999999,
0.337442080953179,0.424780528770959,0.499999999999999,0.588285009908279,
0.676363239585974,0.75,0.835015716367125,0.920008379189467,1.),
 .UNSPECIFIED.);
#4605=B_SPLINE_CURVE_WITH_KNOTS('',3,(#147390,#147391,#147392,#147393,#147394,
#147395),.UNSPECIFIED.,.F.,.F.,(4,2,4),(0.,0.5,1.),.UNSPECIFIED.);
#4606=B_SPLINE_CURVE_WITH_KNOTS('',3,(#147416,#147417,#147418,#147419,#147420,
#147421,#147422,#147423,#147424,#147425,#147426,#147427,#147428,#147429,
#147430,#147431,#147432,#147433,#147434,#147435,#147436,#147437,#147438,
#147439,#147440,#147441,#147442,#147443),.UNSPECIFIED.,.F.,.F.,(4,3,3,3,
3,3,3,3,3,4),(0.,0.111439972739101,0.224754294220322,0.338408661878299,
0.451580972885512,0.500000000000001,0.627994499207414,0.752939260132545,
0.876469630066272,1.),.UNSPECIFIED.);
#4607=B_SPLINE_CURVE_WITH_KNOTS('',3,(#147466,#147467,#147468,#147469,#147470,
#147471,#147472),.UNSPECIFIED.,.F.,.F.,(4,3,4),(1.50276431479551E-5,0.500000000000001,
1.),.UNSPECIFIED.);
#4608=B_SPLINE_CURVE_WITH_KNOTS('',3,(#147492,#147493,#147494,#147495,#147496,
#147497,#147498,#147499,#147500,#147501,#147502,#147503,#147504,#147505,
#147506,#147507,#147508,#147509,#147510),.UNSPECIFIED.,.F.,.F.,(4,3,3,3,
3,3,4),(0.000708752105543503,0.00258350608982207,0.00304683603862546,0.00476166896123969,
0.00640184829291217,0.00796195121144225,0.00830118856937974),
 .UNSPECIFIED.);
#4609=B_SPLINE_CURVE_WITH_KNOTS('',3,(#147511,#147512,#147513,#147514,#147515,
#147516),.UNSPECIFIED.,.F.,.F.,(4,2,4),(0.,0.500000000000001,0.999999987841376),
 .UNSPECIFIED.);
#4610=B_SPLINE_CURVE_WITH_KNOTS('',3,(#147559,#147560,#147561,#147562,#147563,
#147564,#147565,#147566,#147567,#147568),.UNSPECIFIED.,.F.,.F.,(4,2,2,2,
4),(0.,0.25,0.5,0.75,1.),.UNSPECIFIED.);
#4611=B_SPLINE_CURVE_WITH_KNOTS('',3,(#147618,#147619,#147620,#147621,#147622,
#147623,#147624,#147625,#147626,#147627,#147628,#147629,#147630,#147631,
#147632,#147633,#147634,#147635,#147636,#147637,#147638,#147639,#147640,
#147641,#147642,#147643,#147644,#147645,#147646,#147647,#147648),
 .UNSPECIFIED.,.F.,.F.,(4,3,3,3,3,3,3,3,3,3,4),(0.,0.0847040358914981,0.17116589808823,
0.260240904791955,0.350519080310786,0.442212155487767,0.500000000000001,
0.652840714424581,0.811062123407797,0.96706666050884,1.),.UNSPECIFIED.);
#4612=B_SPLINE_CURVE_WITH_KNOTS('',3,(#147667,#147668,#147669,#147670,#147671,
#147672),.UNSPECIFIED.,.F.,.F.,(4,2,4),(0.,0.500000000000001,1.),
 .UNSPECIFIED.);
#4613=B_SPLINE_CURVE_WITH_KNOTS('',3,(#147687,#147688,#147689,#147690),
 .UNSPECIFIED.,.F.,.F.,(4,4),(0.000932565055856382,0.00145387661961334),
 .UNSPECIFIED.);
#4614=B_SPLINE_CURVE_WITH_KNOTS('',3,(#147692,#147693,#147694,#147695,#147696,
#147697,#147698,#147699,#147700,#147701),.UNSPECIFIED.,.F.,.F.,(4,2,2,2,
4),(0.,0.25,0.5,0.750000000000001,0.999999175968697),.UNSPECIFIED.);
#4615=B_SPLINE_CURVE_WITH_KNOTS('',3,(#147709,#147710,#147711,#147712,#147713,
#147714),.UNSPECIFIED.,.F.,.F.,(4,2,4),(0.,0.5,1.),.UNSPECIFIED.);
#4616=B_SPLINE_CURVE_WITH_KNOTS('',3,(#147750,#147751,#147752,#147753,#147754,
#147755,#147756,#147757,#147758,#147759),.UNSPECIFIED.,.F.,.F.,(4,2,2,2,
4),(0.,0.25,0.5,0.75,1.),.UNSPECIFIED.);
#4617=B_SPLINE_CURVE_WITH_KNOTS('',3,(#147767,#147768,#147769,#147770,#147771,
#147772),.UNSPECIFIED.,.F.,.F.,(4,2,4),(0.,0.499999999999999,1.),
 .UNSPECIFIED.);
#4618=B_SPLINE_CURVE_WITH_KNOTS('',3,(#147840,#147841,#147842,#147843,#147844,
#147845,#147846,#147847,#147848,#147849),.UNSPECIFIED.,.F.,.F.,(4,3,3,4),
(0.,0.499999999999717,0.749999999999858,1.),.UNSPECIFIED.);
#4619=B_SPLINE_CURVE_WITH_KNOTS('',3,(#147886,#147887,#147888,#147889,#147890,
#147891,#147892,#147893,#147894,#147895,#147896,#147897,#147898,#147899,
#147900,#147901,#147902,#147903,#147904,#147905,#147906,#147907,#147908,
#147909,#147910,#147911,#147912,#147913,#147914,#147915,#147916,#147917,
#147918,#147919,#147920,#147921,#147922,#147923,#147924,#147925,#147926,
#147927,#147928),.UNSPECIFIED.,.F.,.F.,(4,3,3,3,3,3,3,3,3,3,3,3,3,3,4),
(0.,0.0625,0.123895355591394,0.186947677795697,0.25,0.326192612901303,0.403694113418718,
0.482847078444175,0.5,0.602353575542828,0.711321847725079,0.75,0.839036507722233,
0.928336927687806,1.),.UNSPECIFIED.);
#4620=B_SPLINE_CURVE_WITH_KNOTS('',3,(#147949,#147950,#147951,#147952,#147953,
#147954),.UNSPECIFIED.,.F.,.F.,(4,2,4),(0.,0.500000000000005,1.),
 .UNSPECIFIED.);
#4621=B_SPLINE_CURVE_WITH_KNOTS('',3,(#148029,#148030,#148031,#148032,#148033,
#148034),.UNSPECIFIED.,.F.,.F.,(4,2,4),(0.,0.5,1.),.UNSPECIFIED.);
#4622=B_SPLINE_CURVE_WITH_KNOTS('',3,(#148069,#148070,#148071,#148072,#148073,
#148074,#148075,#148076,#148077,#148078),.UNSPECIFIED.,.F.,.F.,(4,2,2,2,
4),(0.,0.250000000000001,0.500000000000002,0.749999999999999,1.),
 .UNSPECIFIED.);
#4623=B_SPLINE_CURVE_WITH_KNOTS('',3,(#148165,#148166,#148167,#148168,#148169,
#148170,#148171,#148172,#148173,#148174,#148175,#148176,#148177,#148178,
#148179,#148180,#148181,#148182,#148183,#148184,#148185,#148186,#148187,
#148188,#148189,#148190,#148191,#148192,#148193,#148194,#148195),
 .UNSPECIFIED.,.F.,.F.,(4,3,3,3,3,3,3,3,3,3,4),(0.,0.0990505281004008,0.199396658312436,
0.299649788385249,0.399824894192624,0.5,0.605387357037088,0.706111159001044,
0.804538030595637,0.902269015297818,1.),.UNSPECIFIED.);
#4624=B_SPLINE_CURVE_WITH_KNOTS('',3,(#148226,#148227,#148228,#148229,#148230,
#148231,#148232,#148233),.UNSPECIFIED.,.F.,.F.,(4,2,2,4),(3.81942240222894E-5,
0.5,0.75,1.),.UNSPECIFIED.);
#4625=B_SPLINE_CURVE_WITH_KNOTS('',3,(#148258,#148259,#148260,#148261),
 .UNSPECIFIED.,.F.,.F.,(4,4),(1.85554534979779E-6,1.),.UNSPECIFIED.);
#4626=B_SPLINE_CURVE_WITH_KNOTS('',3,(#148332,#148333,#148334,#148335,#148336,
#148337,#148338,#148339,#148340,#148341),.UNSPECIFIED.,.F.,.F.,(4,3,3,4),
(0.,0.499999999999922,0.749999999999962,0.999999984042409),
 .UNSPECIFIED.);
#4627=B_SPLINE_CURVE_WITH_KNOTS('',3,(#148378,#148379,#148380,#148381,#148382,
#148383,#148384,#148385,#148386,#148387,#148388,#148389,#148390,#148391,
#148392,#148393,#148394,#148395,#148396,#148397,#148398,#148399,#148400,
#148401,#148402,#148403,#148404,#148405,#148406,#148407,#148408,#148409,
#148410,#148411,#148412,#148413,#148414,#148415,#148416,#148417),
 .UNSPECIFIED.,.F.,.F.,(4,3,3,3,3,3,3,3,3,3,3,3,3,4),(0.,0.0663260948058646,
0.133685855257027,0.202613561710615,0.25,0.331751956472141,0.41587597823607,
0.499999999999999,0.611670400716575,0.728976448656423,0.75,0.841370986237791,
0.932703732962715,1.),.UNSPECIFIED.);
#4628=B_SPLINE_CURVE_WITH_KNOTS('',3,(#148468,#148469,#148470,#148471,#148472,
#148473,#148474,#148475,#148476,#148477),.UNSPECIFIED.,.F.,.F.,(4,2,2,2,
4),(0.,0.25,0.5,0.75,1.),.UNSPECIFIED.);
#4629=B_SPLINE_CURVE_WITH_KNOTS('',3,(#148513,#148514,#148515,#148516,#148517,
#148518,#148519,#148520,#148521,#148522),.UNSPECIFIED.,.F.,.F.,(4,2,2,2,
4),(0.,0.25,0.5,0.75,1.),.UNSPECIFIED.);
#4630=B_SPLINE_CURVE_WITH_KNOTS('',3,(#148530,#148531,#148532,#148533,#148534,
#148535),.UNSPECIFIED.,.F.,.F.,(4,2,4),(0.,0.499999999999999,1.),
 .UNSPECIFIED.);
#4631=B_SPLINE_CURVE_WITH_KNOTS('',3,(#148557,#148558,#148559,#148560,#148561,
#148562),.UNSPECIFIED.,.F.,.F.,(4,2,4),(0.,0.499999999999998,1.),
 .UNSPECIFIED.);
#4632=B_SPLINE_CURVE_WITH_KNOTS('',3,(#148598,#148599,#148600,#148601,#148602,
#148603,#148604,#148605,#148606,#148607),.UNSPECIFIED.,.F.,.F.,(4,2,2,2,
4),(0.,0.250000000000001,0.500000000000002,0.750000000000002,1.),
 .UNSPECIFIED.);
#4633=B_SPLINE_CURVE_WITH_KNOTS('',3,(#148632,#148633,#148634,#148635,#148636,
#148637),.UNSPECIFIED.,.F.,.F.,(4,2,4),(0.,0.500000000000001,1.),
 .UNSPECIFIED.);
#4634=B_SPLINE_CURVE_WITH_KNOTS('',3,(#148652,#148653,#148654,#148655),
 .UNSPECIFIED.,.F.,.F.,(4,4),(0.,1.),.UNSPECIFIED.);
#4635=B_SPLINE_CURVE_WITH_KNOTS('',3,(#148682,#148683,#148684,#148685,#148686,
#148687,#148688,#148689,#148690,#148691,#148692,#148693,#148694,#148695,
#148696,#148697,#148698,#148699,#148700,#148701,#148702,#148703,#148704,
#148705,#148706,#148707,#148708,#148709,#148710,#148711,#148712,#148713,
#148714,#148715,#148716,#148717,#148718,#148719,#148720,#148721),
 .UNSPECIFIED.,.F.,.F.,(4,3,3,3,3,3,3,3,3,3,3,3,3,4),(3.23711100202308E-15,
0.0890075956720996,0.178502409862928,0.267659454900732,0.355866780049122,
0.441950412840108,0.5,0.586691146881939,0.671658526049874,0.75,0.81604551378379,
0.881127848945156,0.944594173895109,1.),.UNSPECIFIED.);
#4636=B_SPLINE_CURVE_WITH_KNOTS('',3,(#148752,#148753,#148754,#148755,#148756,
#148757,#148758,#148759),.UNSPECIFIED.,.F.,.F.,(4,2,2,4),(2.50635257585442E-5,
0.25,0.5,1.),.UNSPECIFIED.);
#4637=B_SPLINE_CURVE_WITH_KNOTS('',3,(#148773,#148774,#148775,#148776),
 .UNSPECIFIED.,.F.,.F.,(4,4),(0.,1.),.UNSPECIFIED.);
#4638=B_SPLINE_CURVE_WITH_KNOTS('',3,(#148805,#148806,#148807,#148808,#148809,
#148810,#148811,#148812),.UNSPECIFIED.,.F.,.F.,(4,2,2,4),(0.,0.5,0.75,1.),
 .UNSPECIFIED.);
#4639=B_SPLINE_CURVE_WITH_KNOTS('',3,(#148813,#148814,#148815,#148816,#148817,
#148818),.UNSPECIFIED.,.F.,.F.,(4,2,4),(0.,0.5,1.),.UNSPECIFIED.);
#4640=B_SPLINE_CURVE_WITH_KNOTS('',3,(#148856,#148857,#148858,#148859),
 .UNSPECIFIED.,.F.,.F.,(4,4),(0.,1.),.UNSPECIFIED.);
#4641=B_SPLINE_CURVE_WITH_KNOTS('',3,(#148885,#148886,#148887,#148888,#148889,
#148890,#148891,#148892,#148893,#148894,#148895,#148896,#148897,#148898,
#148899,#148900,#148901,#148902,#148903,#148904,#148905,#148906,#148907,
#148908,#148909,#148910,#148911,#148912,#148913,#148914,#148915,#148916,
#148917,#148918,#148919,#148920,#148921,#148922,#148923,#148924),
 .UNSPECIFIED.,.F.,.F.,(4,3,3,3,3,3,3,3,3,3,3,3,3,4),(0.,0.0918748454737772,
0.184355396105487,0.276688554701798,0.36816212505023,0.457673897462644,
0.5,0.589889351053675,0.678272371100533,0.75,0.820588727807885,0.890157630216019,
0.958083323445281,1.),.UNSPECIFIED.);
#4642=B_SPLINE_CURVE_WITH_KNOTS('',3,(#148964,#148965,#148966,#148967,#148968,
#148969,#148970,#148971,#148972,#148973,#148974,#148975,#148976,#148977,
#148978,#148979,#148980,#148981,#148982,#148983,#148984,#148985,#148986,
#148987,#148988,#148989,#148990,#148991,#148992,#148993,#148994,#148995,
#148996,#148997,#148998,#148999,#149000,#149001,#149002,#149003),
 .UNSPECIFIED.,.F.,.F.,(4,3,3,3,3,3,3,3,3,3,3,3,3,4),(0.,0.0714747014717626,
0.14406512628289,0.218232697883806,0.25,0.336678327359007,0.425479051500161,
0.499999999999999,0.603940978333897,0.708843934985259,0.749999999999999,
0.844822927402583,0.939528967854887,1.),.UNSPECIFIED.);
#4643=B_SPLINE_CURVE_WITH_KNOTS('',3,(#149053,#149054,#149055,#149056,#149057,
#149058,#149059,#149060),.UNSPECIFIED.,.F.,.F.,(4,2,2,4),(5.22261572021516E-9,
0.25,0.5,1.),.UNSPECIFIED.);
#4644=B_SPLINE_CURVE_WITH_KNOTS('',3,(#149074,#149075,#149076,#149077),
 .UNSPECIFIED.,.F.,.F.,(4,4),(0.,0.00407596620376747),.UNSPECIFIED.);
#4645=B_SPLINE_CURVE_WITH_KNOTS('',3,(#149106,#149107,#149108,#149109,#149110,
#149111),.UNSPECIFIED.,.F.,.F.,(4,2,4),(0.,0.5,1.),.UNSPECIFIED.);
#4646=B_SPLINE_CURVE_WITH_KNOTS('',3,(#149112,#149113,#149114,#149115,#149116,
#149117,#149118,#149119,#149120,#149121),.UNSPECIFIED.,.F.,.F.,(4,2,2,2,
4),(0.,0.25,0.5,0.75,1.),.UNSPECIFIED.);
#4647=B_SPLINE_CURVE_WITH_KNOTS('',3,(#149161,#149162,#149163,#149164,#149165,
#149166,#149167,#149168,#149169,#149170),.UNSPECIFIED.,.F.,.F.,(4,2,2,2,
4),(0.,0.249999999999998,0.499999999999999,0.749999999999999,1.),
 .UNSPECIFIED.);
#4648=B_SPLINE_CURVE_WITH_KNOTS('',3,(#149178,#149179,#149180,#149181,#149182,
#149183),.UNSPECIFIED.,.F.,.F.,(4,2,4),(0.,0.5,1.),.UNSPECIFIED.);
#4649=B_SPLINE_CURVE_WITH_KNOTS('',3,(#149239,#149240,#149241,#149242),
 .UNSPECIFIED.,.F.,.F.,(4,4),(0.,0.00425966609677044),.UNSPECIFIED.);
#4650=B_SPLINE_CURVE_WITH_KNOTS('',3,(#149275,#149276,#149277,#149278,#149279,
#149280,#149281,#149282,#149283,#149284,#149285,#149286,#149287,#149288,
#149289,#149290,#149291,#149292,#149293,#149294,#149295,#149296,#149297,
#149298,#149299,#149300,#149301,#149302,#149303,#149304,#149305,#149306,
#149307,#149308,#149309,#149310,#149311,#149312,#149313,#149314,#149315,
#149316,#149317,#149318,#149319,#149320,#149321,#149322,#149323),
 .UNSPECIFIED.,.F.,.F.,(4,3,3,3,3,3,3,3,3,3,3,3,3,3,3,3,4),(0.,0.0816151725490495,
0.165807586274525,0.25,0.328615088456192,0.405988550271647,0.481325889494902,
0.5,0.578932430016132,0.656234385435454,0.731485876446147,0.75,0.805022411038226,
0.858733068040437,0.911617182774789,0.963210525378497,1.),.UNSPECIFIED.);
#4651=B_SPLINE_CURVE_WITH_KNOTS('',3,(#149366,#149367,#149368,#149369,#149370,
#149371,#149372,#149373,#149374,#149375,#149376,#149377,#149378,#149379,
#149380,#149381,#149382,#149383,#149384,#149385,#149386,#149387,#149388,
#149389,#149390,#149391,#149392,#149393,#149394,#149395,#149396,#149397,
#149398,#149399,#149400,#149401,#149402,#149403,#149404,#149405,#149406,
#149407,#149408,#149409,#149410,#149411,#149412,#149413,#149414),
 .UNSPECIFIED.,.F.,.F.,(4,3,3,3,3,3,3,3,3,3,3,3,3,3,3,3,4),(0.,0.0510981392875666,
0.103679684270398,0.157057814696616,0.211633657635973,0.25,0.315602833834227,
0.375,0.442162015238332,0.5,0.575392432169574,0.652181332108927,0.73067248504618,
0.750000000000001,0.831704547321132,0.915852273660566,1.),.UNSPECIFIED.);
#4652=B_SPLINE_CURVE_WITH_KNOTS('',3,(#149429,#149430,#149431,#149432),
 .UNSPECIFIED.,.F.,.F.,(4,4),(0.,0.00454447370442107),.UNSPECIFIED.);
#4653=B_SPLINE_CURVE_WITH_KNOTS('',3,(#149459,#149460,#149461,#149462,#149463,
#149464,#149465,#149466),.UNSPECIFIED.,.F.,.F.,(4,2,2,4),(0.,0.5,0.75,1.),
 .UNSPECIFIED.);
#4654=B_SPLINE_CURVE_WITH_KNOTS('',3,(#149518,#149519,#149520,#149521,#149522,
#149523),.UNSPECIFIED.,.F.,.F.,(4,2,4),(0.,0.5,1.),.UNSPECIFIED.);
#4655=B_SPLINE_CURVE_WITH_KNOTS('',3,(#149558,#149559,#149560,#149561,#149562,
#149563,#149564,#149565,#149566,#149567),.UNSPECIFIED.,.F.,.F.,(4,2,2,2,
4),(0.,0.250000000000001,0.500000000000002,0.749999999999999,1.),
 .UNSPECIFIED.);
#4656=B_SPLINE_CURVE_WITH_KNOTS('',3,(#149574,#149575,#149576,#149577,#149578,
#149579,#149580,#149581,#149582,#149583),.UNSPECIFIED.,.F.,.F.,(4,3,3,4),
(0.,0.366159133847531,0.707490766021897,1.),.UNSPECIFIED.);
#4657=B_SPLINE_CURVE_WITH_KNOTS('',3,(#149587,#149588,#149589,#149590,#149591,
#149592),.UNSPECIFIED.,.F.,.F.,(4,2,4),(0.,0.5,1.),.UNSPECIFIED.);
#4658=B_SPLINE_CURVE_WITH_KNOTS('',3,(#149616,#149617,#149618,#149619,#149620,
#149621,#149622,#149623,#149624,#149625,#149626,#149627,#149628,#149629,
#149630,#149631,#149632,#149633,#149634,#149635,#149636,#149637,#149638,
#149639,#149640),.UNSPECIFIED.,.F.,.F.,(4,3,3,3,3,3,3,3,4),(0.,0.153482428046558,
0.30779152303746,0.461567879573118,0.5,0.654327083157327,0.810904002598426,
0.96838512301851,1.),.UNSPECIFIED.);
#4659=B_SPLINE_CURVE_WITH_KNOTS('',3,(#149676,#149677,#149678,#149679,#149680,
#149681),.UNSPECIFIED.,.F.,.F.,(4,2,4),(0.,0.5,1.),.UNSPECIFIED.);
#4660=B_SPLINE_CURVE_WITH_KNOTS('',3,(#149702,#149703,#149704,#149705,#149706,
#149707,#149708,#149709,#149710,#149711,#149712,#149713,#149714,#149715,
#149716,#149717,#149718,#149719,#149720,#149721,#149722,#149723,#149724,
#149725,#149726,#149727,#149728,#149729,#149730,#149731,#149732,#149733,
#149734,#149735,#149736,#149737,#149738),.UNSPECIFIED.,.F.,.F.,(4,3,3,3,
3,3,3,3,3,3,3,3,4),(0.,0.0966473935252569,0.197485545143943,0.295141620703053,
0.392110161524986,0.487415820015577,0.5,0.600531670333472,0.700398752750104,
0.794302669238309,0.886236884590961,0.975690548447645,1.),.UNSPECIFIED.);
#4661=B_SPLINE_CURVE_WITH_KNOTS('',3,(#149769,#149770,#149771,#149772,#149773,
#149774,#149775,#149776,#149777,#149778),.UNSPECIFIED.,.F.,.F.,(4,3,3,4),
(7.90081955571743E-6,0.5,0.750000000000001,1.),.UNSPECIFIED.);
#4662=B_SPLINE_CURVE_WITH_KNOTS('',3,(#149837,#149838,#149839,#149840,#149841,
#149842,#149843),.UNSPECIFIED.,.F.,.F.,(4,3,4),(4.04098200660582E-7,0.327146603495783,
1.),.UNSPECIFIED.);
#4663=B_SPLINE_CURVE_WITH_KNOTS('',3,(#149844,#149845,#149846,#149847),
 .UNSPECIFIED.,.F.,.F.,(4,4),(0.,1.),.UNSPECIFIED.);
#4664=B_SPLINE_CURVE_WITH_KNOTS('',3,(#149914,#149915,#149916,#149917,#149918,
#149919,#149920,#149921,#149922,#149923),.UNSPECIFIED.,.F.,.F.,(4,3,3,4),
(0.,0.49999999999992,0.749999999999959,0.999999993899122),.UNSPECIFIED.);
#4665=B_SPLINE_CURVE_WITH_KNOTS('',3,(#149960,#149961,#149962,#149963,#149964,
#149965,#149966,#149967,#149968,#149969),.UNSPECIFIED.,.F.,.F.,(4,2,2,2,
4),(6.1213090326977E-9,0.25,0.499999999999999,0.75,1.),.UNSPECIFIED.);
#4666=B_SPLINE_CURVE_WITH_KNOTS('',3,(#149984,#149985,#149986,#149987),
 .UNSPECIFIED.,.F.,.F.,(4,4),(0.,1.),.UNSPECIFIED.);
#4667=B_SPLINE_CURVE_WITH_KNOTS('',3,(#150020,#150021,#150022,#150023,#150024,
#150025,#150026,#150027,#150028,#150029),.UNSPECIFIED.,.F.,.F.,(4,2,2,2,
4),(0.,0.25,0.5,0.749999999999999,1.),.UNSPECIFIED.);
#4668=B_SPLINE_CURVE_WITH_KNOTS('',3,(#150065,#150066,#150067,#150068,#150069,
#150070,#150071,#150072,#150073,#150074),.UNSPECIFIED.,.F.,.F.,(4,2,2,2,
4),(0.,0.249999999999998,0.499999999999999,0.749999999999999,1.),
 .UNSPECIFIED.);
#4669=B_SPLINE_CURVE_WITH_KNOTS('',3,(#150082,#150083,#150084,#150085,#150086,
#150087),.UNSPECIFIED.,.F.,.F.,(4,2,4),(0.,0.5,1.),.UNSPECIFIED.);
#4670=B_SPLINE_CURVE_WITH_KNOTS('',3,(#150109,#150110,#150111,#150112,#150113,
#150114),.UNSPECIFIED.,.F.,.F.,(4,2,4),(0.,0.5,1.),.UNSPECIFIED.);
#4671=B_SPLINE_CURVE_WITH_KNOTS('',3,(#150150,#150151,#150152,#150153,#150154,
#150155,#150156,#150157,#150158,#150159),.UNSPECIFIED.,.F.,.F.,(4,2,2,2,
4),(0.,0.250000000000001,0.500000000000002,0.749999999999999,1.),
 .UNSPECIFIED.);
#4672=B_SPLINE_CURVE_WITH_KNOTS('',3,(#150184,#150185,#150186,#150187,#150188,
#150189),.UNSPECIFIED.,.F.,.F.,(4,2,4),(0.,0.5,1.),.UNSPECIFIED.);
#4673=B_SPLINE_CURVE_WITH_KNOTS('',3,(#150204,#150205,#150206,#150207),
 .UNSPECIFIED.,.F.,.F.,(4,4),(0.,1.),.UNSPECIFIED.);
#4674=B_SPLINE_CURVE_WITH_KNOTS('',3,(#150234,#150235,#150236,#150237,#150238,
#150239,#150240,#150241,#150242,#150243,#150244,#150245,#150246,#150247,
#150248,#150249,#150250,#150251,#150252,#150253,#150254,#150255,#150256,
#150257,#150258,#150259,#150260,#150261,#150262,#150263,#150264,#150265,
#150266,#150267,#150268,#150269,#150270,#150271,#150272,#150273),
 .UNSPECIFIED.,.F.,.F.,(4,3,3,3,3,3,3,3,3,3,3,3,3,4),(3.06013101603585E-15,
0.0868770599546466,0.174176392221001,0.261052249862412,0.346949892959567,
0.430648677455611,0.5,0.584788005264847,0.667617697597973,0.75,0.812804103608978,
0.874691742956029,0.937345871478015,1.),.UNSPECIFIED.);
#4675=B_SPLINE_CURVE_WITH_KNOTS('',3,(#150304,#150305,#150306,#150307,#150308,
#150309,#150310,#150311,#150312,#150313,#150314,#150315,#150316,#150317,
#150318,#150319,#150320,#150321,#150322,#150323,#150324,#150325,#150326,
#150327,#150328,#150329,#150330,#150331,#150332,#150333,#150334,#150335,
#150336,#150337,#150338,#150339,#150340,#150341,#150342,#150343,#150344,
#150345,#150346,#150347,#150348,#150349),.UNSPECIFIED.,.F.,.F.,(4,3,3,3,
3,3,3,3,3,3,3,3,3,3,3,4),(0.,0.0588319507752074,0.119280604150712,0.18064195969371,
0.243181726830164,0.25,0.32489127172958,0.401033799041576,0.478740210308195,
0.5,0.584292661882019,0.670546056491487,0.759159439922366,0.848371083490158,
0.937600152938783,1.),.UNSPECIFIED.);
#4676=B_SPLINE_CURVE_WITH_KNOTS('',3,(#150363,#150364,#150365,#150366),
 .UNSPECIFIED.,.F.,.F.,(4,4),(0.,1.),.UNSPECIFIED.);
#4677=B_SPLINE_CURVE_WITH_KNOTS('',3,(#150394,#150395,#150396,#150397,#150398,
#150399,#150400),.UNSPECIFIED.,.F.,.F.,(4,3,4),(0.,0.674038033463522,0.999999605243852),
 .UNSPECIFIED.);
#4678=B_SPLINE_CURVE_WITH_KNOTS('',3,(#150401,#150402,#150403,#150404),
 .UNSPECIFIED.,.F.,.F.,(4,4),(0.,1.),.UNSPECIFIED.);
#4679=B_SPLINE_CURVE_WITH_KNOTS('',3,(#150405,#150406,#150407,#150408,#150409,
#150410),.UNSPECIFIED.,.F.,.F.,(4,2,4),(0.,0.5,1.),.UNSPECIFIED.);
#4680=B_SPLINE_CURVE_WITH_KNOTS('',3,(#150477,#150478,#150479,#150480,#150481,
#150482),.UNSPECIFIED.,.F.,.F.,(4,2,4),(0.,0.499999999999999,1.),
 .UNSPECIFIED.);
#4681=B_SPLINE_CURVE_WITH_KNOTS('',3,(#150487,#150488,#150489,#150490,#150491,
#150492),.UNSPECIFIED.,.F.,.F.,(4,2,4),(0.,0.5,1.),.UNSPECIFIED.);
#4682=B_SPLINE_CURVE_WITH_KNOTS('',3,(#150543,#150544,#150545,#150546,#150547,
#150548,#150549,#150550,#150551,#150552,#150553,#150554,#150555,#150556,
#150557,#150558,#150559,#150560,#150561,#150562,#150563,#150564,#150565,
#150566,#150567,#150568,#150569,#150570,#150571,#150572,#150573,#150574,
#150575,#150576,#150577,#150578,#150579),.UNSPECIFIED.,.F.,.F.,(4,3,3,3,
3,3,3,3,3,3,3,3,4),(0.,0.096322507088443,0.197241880316332,0.294537759139576,
0.39113272840702,0.486046208564947,0.5,0.599805200905989,0.699853900679492,
0.79306779554781,0.884327816606269,0.973109138977564,1.),.UNSPECIFIED.);
#4683=B_SPLINE_CURVE_WITH_KNOTS('',3,(#150610,#150611,#150612,#150613,#150614,
#150615,#150616,#150617,#150618,#150619),.UNSPECIFIED.,.F.,.F.,(4,3,3,4),
(7.73028779751986E-6,0.499999999999999,0.75,1.),.UNSPECIFIED.);
#4684=B_SPLINE_CURVE_WITH_KNOTS('',3,(#150691,#150692,#150693,#150694,#150695,
#150696,#150697,#150698,#150699,#150700),.UNSPECIFIED.,.F.,.F.,(4,2,2,2,
4),(0.,0.250000000000004,0.5,0.750000000000003,1.),.UNSPECIFIED.);
#4685=B_SPLINE_CURVE_WITH_KNOTS('',3,(#150708,#150709,#150710,#150711,#150712,
#150713),.UNSPECIFIED.,.F.,.F.,(4,2,4),(0.,0.5,1.),.UNSPECIFIED.);
#4686=B_SPLINE_CURVE_WITH_KNOTS('',3,(#150773,#150774,#150775,#150776,#150777,
#150778),.UNSPECIFIED.,.F.,.F.,(4,2,4),(0.,0.5,1.),.UNSPECIFIED.);
#4687=B_SPLINE_CURVE_WITH_KNOTS('',3,(#150816,#150817,#150818,#150819,#150820,
#150821,#150822,#150823,#150824,#150825),.UNSPECIFIED.,.F.,.F.,(4,2,2,2,
4),(0.,0.249999999999999,0.499999999999999,0.75,1.),.UNSPECIFIED.);
#4688=B_SPLINE_CURVE_WITH_KNOTS('',3,(#150862,#150863,#150864,#150865,#150866,
#150867,#150868,#150869,#150870,#150871),.UNSPECIFIED.,.F.,.F.,(4,2,2,2,
4),(0.,0.25,0.5,0.749999999999999,1.),.UNSPECIFIED.);
#4689=B_SPLINE_CURVE_WITH_KNOTS('',3,(#150886,#150887,#150888,#150889),
 .UNSPECIFIED.,.F.,.F.,(4,4),(0.,0.0041383639263312),.UNSPECIFIED.);
#4690=B_SPLINE_CURVE_WITH_KNOTS('',3,(#150922,#150923,#150924,#150925,#150926,
#150927,#150928,#150929,#150930,#150931,#150932,#150933,#150934,#150935,
#150936,#150937,#150938,#150939,#150940,#150941,#150942,#150943,#150944,
#150945,#150946,#150947,#150948,#150949,#150950,#150951,#150952,#150953,
#150954,#150955,#150956,#150957,#150958,#150959,#150960,#150961,#150962,
#150963,#150964,#150965,#150966,#150967,#150968,#150969,#150970),
 .UNSPECIFIED.,.F.,.F.,(4,3,3,3,3,3,3,3,3,3,3,3,3,3,3,3,4),(0.,0.0814682051398938,
0.165734102569947,0.25,0.328395291585389,0.405548538423333,0.480663972186547,
0.5,0.57867163212605,0.655704680829147,0.730672357703364,0.750000000000001,
0.804753401868345,0.858198891364756,0.910821998101223,0.962154755762754,
1.),.UNSPECIFIED.);
#4691=B_SPLINE_CURVE_WITH_KNOTS('',3,(#151013,#151014,#151015,#151016,#151017,
#151018,#151019,#151020,#151021,#151022,#151023,#151024,#151025,#151026,
#151027,#151028,#151029,#151030,#151031,#151032,#151033,#151034,#151035,
#151036,#151037,#151038,#151039,#151040,#151041,#151042,#151043,#151044,
#151045,#151046,#151047,#151048,#151049,#151050,#151051,#151052,#151053,
#151054,#151055,#151056,#151057,#151058,#151059,#151060,#151061),
 .UNSPECIFIED.,.F.,.F.,(4,3,3,3,3,3,3,3,3,3,3,3,3,3,3,3,4),(0.,0.0508457726259258,
0.103170761367999,0.15628866585067,0.210605274562482,0.25,0.315356401070316,
0.375,0.441638820974095,0.5,0.575194165397271,0.651783139678669,0.730078138175237,
0.749999999999999,0.83154071027051,0.915770355135255,1.),.UNSPECIFIED.);
#4692=B_SPLINE_CURVE_WITH_KNOTS('',3,(#151076,#151077,#151078,#151079),
 .UNSPECIFIED.,.F.,.F.,(4,4),(0.,0.00385317783226068),.UNSPECIFIED.);
#4693=B_SPLINE_CURVE_WITH_KNOTS('',3,(#151105,#151106,#151107,#151108,#151109,
#151110,#151111,#151112),.UNSPECIFIED.,.F.,.F.,(4,2,2,4),(0.,0.5,0.750000000000001,
1.),.UNSPECIFIED.);
#4694=B_SPLINE_CURVE_WITH_KNOTS('',3,(#151123,#151124,#151125,#151126,#151127,
#151128),.UNSPECIFIED.,.F.,.F.,(4,2,4),(0.,0.5,1.),.UNSPECIFIED.);
#4695=B_SPLINE_CURVE_WITH_KNOTS('',3,(#151164,#151165,#151166,#151167),
 .UNSPECIFIED.,.F.,.F.,(4,4),(0.,1.),.UNSPECIFIED.);
#4696=B_SPLINE_CURVE_WITH_KNOTS('',3,(#151194,#151195,#151196,#151197,#151198,
#151199,#151200,#151201,#151202,#151203,#151204,#151205,#151206,#151207,
#151208,#151209,#151210,#151211,#151212,#151213,#151214,#151215,#151216,
#151217,#151218,#151219,#151220,#151221,#151222,#151223,#151224,#151225,
#151226,#151227,#151228,#151229,#151230,#151231,#151232,#151233,#151234,
#151235,#151236),.UNSPECIFIED.,.F.,.F.,(4,3,3,3,3,3,3,3,3,3,3,3,3,3,4),
(3.00632357117456E-15,0.0866568870700394,0.173726346313476,0.260357383779208,
0.346004233647263,0.429440823274784,0.5,0.584571854059349,0.667285927029675,
0.75,0.8125,0.874021143077118,0.937010571538559,0.996237991481499,1.),
 .UNSPECIFIED.);
#4697=B_SPLINE_CURVE_WITH_KNOTS('',3,(#151267,#151268,#151269,#151270,#151271,
#151272,#151273,#151274,#151275,#151276,#151277,#151278,#151279,#151280,
#151281,#151282,#151283,#151284,#151285,#151286,#151287,#151288,#151289,
#151290,#151291,#151292,#151293,#151294,#151295,#151296,#151297,#151298,
#151299,#151300,#151301,#151302,#151303,#151304,#151305,#151306,#151307,
#151308,#151309,#151310,#151311,#151312),.UNSPECIFIED.,.F.,.F.,(4,3,3,3,
3,3,3,3,3,3,3,3,3,3,3,4),(0.,0.0584822194913625,0.118574901578209,0.179574980246278,
0.241754287190893,0.25,0.324564021641555,0.40037551082833,0.477754744932888,
0.5,0.583489443865849,0.66889279993803,0.75661190226229,0.844919580084762,
0.933262852347954,1.),.UNSPECIFIED.);
#4698=B_SPLINE_CURVE_WITH_KNOTS('',3,(#151327,#151328,#151329,#151330),
 .UNSPECIFIED.,.F.,.F.,(4,4),(0.,1.),.UNSPECIFIED.);
#4699=B_SPLINE_CURVE_WITH_KNOTS('',3,(#151351,#151352,#151353,#151354,#151355,
#151356),.UNSPECIFIED.,.F.,.F.,(4,2,4),(0.,0.5,1.),.UNSPECIFIED.);
#4700=B_SPLINE_CURVE_WITH_KNOTS('',3,(#151392,#151393,#151394,#151395,#151396,
#151397,#151398,#151399,#151400,#151401),.UNSPECIFIED.,.F.,.F.,(4,2,2,2,
4),(0.,0.250000000000004,0.5,0.750000000000003,1.),.UNSPECIFIED.);
#4701=B_SPLINE_CURVE_WITH_KNOTS('',3,(#151409,#151410,#151411,#151412,#151413,
#151414),.UNSPECIFIED.,.F.,.F.,(4,2,4),(0.,0.499999999999998,1.),
 .UNSPECIFIED.);
#4702=B_SPLINE_CURVE_WITH_KNOTS('',3,(#151437,#151438,#151439,#151440,#151441,
#151442),.UNSPECIFIED.,.F.,.F.,(4,2,4),(0.,0.5,1.),.UNSPECIFIED.);
#4703=B_SPLINE_CURVE_WITH_KNOTS('',3,(#151480,#151481,#151482,#151483,#151484,
#151485,#151486,#151487,#151488,#151489),.UNSPECIFIED.,.F.,.F.,(4,2,2,2,
4),(0.,0.249999999999999,0.499999999999999,0.75,1.),.UNSPECIFIED.);
#4704=B_SPLINE_CURVE_WITH_KNOTS('',3,(#151520,#151521,#151522,#151523,#151524,
#151525,#151526,#151527),.UNSPECIFIED.,.F.,.F.,(4,2,2,4),(0.,0.25,0.5,1.),
 .UNSPECIFIED.);
#4705=B_SPLINE_CURVE_WITH_KNOTS('',3,(#151542,#151543,#151544,#151545),
 .UNSPECIFIED.,.F.,.F.,(4,4),(0.,1.),.UNSPECIFIED.);
#4706=B_SPLINE_CURVE_WITH_KNOTS('',3,(#151572,#151573,#151574,#151575,#151576,
#151577,#151578,#151579,#151580,#151581),.UNSPECIFIED.,.F.,.F.,(4,3,3,4),
(0.,0.49999999999996,0.749999999999982,0.99999999401614),.UNSPECIFIED.);
#4707=B_SPLINE_CURVE_WITH_KNOTS('',3,(#151611,#151612,#151613,#151614,#151615,
#151616,#151617,#151618,#151619,#151620,#151621,#151622,#151623,#151624,
#151625,#151626,#151627,#151628,#151629,#151630,#151631,#151632,#151633,
#151634,#151635,#151636,#151637,#151638,#151639,#151640,#151641,#151642,
#151643,#151644,#151645,#151646,#151647,#151648,#151649,#151650,#151651,
#151652,#151653),.UNSPECIFIED.,.F.,.F.,(4,3,3,3,3,3,3,3,3,3,3,3,3,3,4),
(0.,0.0628142014478904,0.126607829830903,0.191964238766059,0.25,0.328385271386528,
0.408052842259139,0.48922860882376,0.5,0.593627159335556,0.68989241160167,
0.789176056525988,0.889186506003656,0.988920801147075,1.),.UNSPECIFIED.);
#4708=B_SPLINE_CURVE_WITH_KNOTS('',3,(#151713,#151714,#151715,#151716,#151717,
#151718,#151719),.UNSPECIFIED.,.F.,.F.,(4,3,4),(0.,0.680762826204378,0.999999809903877),
 .UNSPECIFIED.);
#4709=B_SPLINE_CURVE_WITH_KNOTS('',3,(#151973,#151974,#151975,#151976),
 .UNSPECIFIED.,.F.,.F.,(4,4),(0.,1.),.UNSPECIFIED.);
#4710=B_SPLINE_CURVE_WITH_KNOTS('',3,(#152237,#152238,#152239,#152240,#152241,
#152242),.UNSPECIFIED.,.F.,.F.,(4,2,4),(0.,0.499999999999998,1.),
 .UNSPECIFIED.);
#4711=B_SPLINE_CURVE_WITH_KNOTS('',3,(#152351,#152352,#152353,#152354),
 .UNSPECIFIED.,.F.,.F.,(4,4),(0.,1.),.UNSPECIFIED.);
#4712=B_SPLINE_CURVE_WITH_KNOTS('',3,(#152584,#152585,#152586,#152587,#152588,
#152589,#152590,#152591),.UNSPECIFIED.,.F.,.F.,(4,2,2,4),(0.,0.25,0.500000000000001,
1.),.UNSPECIFIED.);
#4713=B_SPLINE_CURVE_WITH_KNOTS('',3,(#152619,#152620,#152621,#152622,#152623,
#152624,#152625,#152626,#152627,#152628,#152629,#152630,#152631,#152632,
#152633,#152634,#152635,#152636,#152637),.UNSPECIFIED.,.F.,.F.,(4,3,3,3,
3,3,4),(0.000623203325049932,0.00219889325760151,0.00382915155670995,0.00555512420845626,
0.00571003463709915,0.00756817415875739,0.00806753801901704),
 .UNSPECIFIED.);
#4714=B_SPLINE_CURVE_WITH_KNOTS('',3,(#152658,#152659,#152660,#152661,#152662,
#152663,#152664,#152665,#152666,#152667,#152668,#152669,#152670,#152671,
#152672,#152673),.UNSPECIFIED.,.F.,.F.,(4,3,3,3,3,4),(0.000539871559505675,
0.00223531956681298,0.00375574051851002,0.00457928549922768,0.00579560462260938,
0.00697160947751434),.UNSPECIFIED.);
#4715=B_SPLINE_CURVE_WITH_KNOTS('',3,(#152698,#152699,#152700,#152701,#152702,
#152703,#152704,#152705,#152706,#152707,#152708,#152709,#152710,#152711,
#152712,#152713,#152714,#152715,#152716,#152717,#152718,#152719,#152720,
#152721,#152722),.UNSPECIFIED.,.F.,.F.,(4,3,3,3,3,3,3,3,4),(0.00049834301207312,
0.00231282934721122,0.00337277528899485,0.00370896758807423,0.00446136300849288,
0.00522125339640802,0.00534496249690202,0.00614439986206378,0.00624720756634296),
 .UNSPECIFIED.);
#4716=B_SPLINE_CURVE_WITH_KNOTS('',3,(#152738,#152739,#152740,#152741,#152742,
#152743,#152744),.UNSPECIFIED.,.F.,.F.,(4,3,4),(7.49040536136306E-7,0.373399908132615,
1.),.UNSPECIFIED.);
#4717=B_SPLINE_CURVE_WITH_KNOTS('',3,(#152763,#152764,#152765,#152766,#152767,
#152768,#152769,#152770,#152771,#152772,#152773,#152774,#152775,#152776,
#152777,#152778,#152779,#152780,#152781),.UNSPECIFIED.,.F.,.F.,(4,3,3,3,
3,3,4),(0.000711431901436798,0.00260509764013045,0.00304924424816995,0.00478266330430852,
0.00644043866289917,0.00801739908984626,0.00833474438776835),
 .UNSPECIFIED.);
#4718=B_SPLINE_CURVE_WITH_KNOTS('',3,(#152792,#152793,#152794,#152795,#152796,
#152797),.UNSPECIFIED.,.F.,.F.,(4,2,4),(0.,0.428102325431166,1.),
 .UNSPECIFIED.);
#4719=B_SPLINE_CURVE_WITH_KNOTS('',3,(#152816,#152817,#152818,#152819,#152820,
#152821,#152822,#152823,#152824,#152825,#152826,#152827,#152828,#152829,
#152830,#152831),.UNSPECIFIED.,.F.,.F.,(4,3,3,3,3,4),(0.00061266112179062,
0.00182296639992156,0.0029850620415817,0.00388203060349254,0.00558489832474133,
0.00715140008519447),.UNSPECIFIED.);
#4720=B_SPLINE_CURVE_WITH_KNOTS('',3,(#152878,#152879,#152880,#152881,#152882,
#152883,#152884,#152885,#152886,#152887,#152888,#152889,#152890,#152891,
#152892,#152893,#152894,#152895,#152896,#152897,#152898,#152899,#152900,
#152901,#152902),.UNSPECIFIED.,.F.,.F.,(4,3,3,3,3,3,3,3,4),(0.000528035090325194,
0.0016124914159346,0.0026700115184638,0.00302714454343539,0.00341353154252654,
0.00423239659979929,0.00468651457632683,0.00549911074687934,0.0062990279947279),
 .UNSPECIFIED.);
#4721=B_SPLINE_CURVE_WITH_KNOTS('',3,(#152917,#152918,#152919,#152920,#152921,
#152922),.UNSPECIFIED.,.F.,.F.,(4,2,4),(0.,0.509180994354165,1.),
 .UNSPECIFIED.);
#4722=B_SPLINE_CURVE_WITH_KNOTS('',3,(#152941,#152942,#152943,#152944,#152945,
#152946,#152947,#152948,#152949,#152950,#152951,#152952,#152953,#152954,
#152955,#152956,#152957,#152958,#152959),.UNSPECIFIED.,.F.,.F.,(4,3,3,3,
3,3,4),(0.00049889453195992,0.00225071250487917,0.00337891514771613,0.00374149706694668,
0.00465083407571109,0.00559677886660822,0.00625893576407251),
 .UNSPECIFIED.);
#4723=B_SPLINE_CURVE_WITH_KNOTS('',3,(#152974,#152975,#152976,#152977,#152978,
#152979,#152980,#152981),.UNSPECIFIED.,.F.,.F.,(4,2,2,4),(0.,0.570298119392456,
0.858868992686398,1.),.UNSPECIFIED.);
#4724=B_SPLINE_CURVE_WITH_KNOTS('',3,(#153006,#153007,#153008,#153009,#153010,
#153011,#153012,#153013,#153014,#153015,#153016,#153017,#153018,#153019,
#153020,#153021,#153022,#153023,#153024),.UNSPECIFIED.,.F.,.F.,(4,3,3,3,
3,3,4),(0.000543628862815408,0.00167393673136798,0.00258252559983906,0.00379688806421997,
0.00467674795200451,0.00601647986746607,0.00704595220449218),
 .UNSPECIFIED.);
#4725=B_SPLINE_CURVE_WITH_KNOTS('',3,(#153034,#153035,#153036,#153037,#153038,
#153039,#153040),.UNSPECIFIED.,.F.,.F.,(4,3,4),(0.,0.625174273651469,0.99999924413068),
 .UNSPECIFIED.);
#4726=B_SPLINE_CURVE_WITH_KNOTS('',3,(#153059,#153060,#153061,#153062,#153063,
#153064,#153065,#153066,#153067,#153068,#153069,#153070,#153071,#153072,
#153073,#153074,#153075,#153076,#153077),.UNSPECIFIED.,.F.,.F.,(4,3,3,3,
3,3,4),(0.000633514536432522,0.00221236722518429,0.00384759398055232,0.00558513688102114,
0.00588295359619705,0.00776048988119671,0.00821913918141333),
 .UNSPECIFIED.);
#4727=B_SPLINE_CURVE_WITH_KNOTS('',3,(#153094,#153095,#153096,#153097),
 .UNSPECIFIED.,.F.,.F.,(4,4),(0.000856775130582955,0.0102382230284107),
 .UNSPECIFIED.);
#4728=B_SPLINE_CURVE_WITH_KNOTS('',3,(#153098,#153099,#153100,#153101),
 .UNSPECIFIED.,.F.,.F.,(4,4),(1.21683837293175E-6,1.),.UNSPECIFIED.);
#4729=B_SPLINE_CURVE_WITH_KNOTS('',3,(#153109,#153110,#153111,#153112),
 .UNSPECIFIED.,.F.,.F.,(4,4),(0.000801783579032724,0.0101814026529808),
 .UNSPECIFIED.);
#4730=B_SPLINE_CURVE_WITH_KNOTS('',3,(#153127,#153128,#153129,#153130),
 .UNSPECIFIED.,.F.,.F.,(4,4),(0.,0.999998771610134),.UNSPECIFIED.);
#4731=B_SPLINE_CURVE_WITH_KNOTS('',3,(#153158,#153159,#153160,#153161),
 .UNSPECIFIED.,.F.,.F.,(4,4),(0.,0.999998144078028),.UNSPECIFIED.);
#4732=B_SPLINE_CURVE_WITH_KNOTS('',3,(#153174,#153175,#153176,#153177),
 .UNSPECIFIED.,.F.,.F.,(4,4),(0.000716623500636008,0.00919276877023496),
 .UNSPECIFIED.);
#4733=B_SPLINE_CURVE_WITH_KNOTS('',3,(#153179,#153180,#153181,#153182),
 .UNSPECIFIED.,.F.,.F.,(4,4),(0.00078229444191847,0.00926194220748866),
 .UNSPECIFIED.);
#4734=B_SPLINE_CURVE_WITH_KNOTS('',3,(#153204,#153205,#153206,#153207),
 .UNSPECIFIED.,.F.,.F.,(4,4),(1.30575596808862E-6,1.),.UNSPECIFIED.);
#4735=B_SPLINE_CURVE_WITH_KNOTS('',3,(#153225,#153226,#153227,#153228),
 .UNSPECIFIED.,.F.,.F.,(4,4),(0.000874668174674732,0.0104577126980746),
 .UNSPECIFIED.);
#4736=B_SPLINE_CURVE_WITH_KNOTS('',3,(#153230,#153231,#153232,#153233),
 .UNSPECIFIED.,.F.,.F.,(4,4),(0.000819410081741501,0.0104007046320713),
 .UNSPECIFIED.);
#4737=B_SPLINE_CURVE_WITH_KNOTS('',3,(#153246,#153247,#153248,#153249),
 .UNSPECIFIED.,.F.,.F.,(4,4),(0.,0.999998694225143),.UNSPECIFIED.);
#4738=B_SPLINE_CURVE_WITH_KNOTS('',3,(#153259,#153260,#153261,#153262,#153263,
#153264,#153265),.UNSPECIFIED.,.F.,.F.,(4,3,4),(0.,0.672852549108075,0.999999595945834),
 .UNSPECIFIED.);
#4739=B_SPLINE_CURVE_WITH_KNOTS('',3,(#153284,#153285,#153286,#153287,#153288,
#153289,#153290,#153291,#153292,#153293,#153294,#153295,#153296),
 .UNSPECIFIED.,.F.,.F.,(4,3,3,3,4),(0.000731998639840557,0.00321503108606918,
0.00587687390150681,0.00707184840840047,0.00939432936633357),
 .UNSPECIFIED.);
#4740=B_SPLINE_CURVE_WITH_KNOTS('',3,(#153298,#153299,#153300,#153301,#153302,
#153303,#153304,#153305,#153306,#153307,#153308,#153309,#153310),
 .UNSPECIFIED.,.F.,.F.,(4,3,3,3,4),(0.000799595655510347,0.00312305020211246,
0.00581514086609625,0.00831497793887529,0.00946542910228819),
 .UNSPECIFIED.);
#4741=B_SPLINE_CURVE_WITH_KNOTS('',3,(#153353,#153354,#153355,#153356,#153357,
#153358,#153359,#153360,#153361,#153362,#153363,#153364,#153365),
 .UNSPECIFIED.,.F.,.F.,(4,3,3,3,4),(0.000734608576009405,0.00325207345695062,
0.00595173535838772,0.00710294415665481,0.0094247370890218),
 .UNSPECIFIED.);
#4742=B_SPLINE_CURVE_WITH_KNOTS('',3,(#153367,#153368,#153369,#153370,#153371,
#153372,#153373,#153374,#153375,#153376,#153377,#153378,#153379),
 .UNSPECIFIED.,.F.,.F.,(4,3,3,3,4),(0.000801891157765995,0.00312464263181538,
0.00585483490545202,0.00838933971211676,0.00949544874465978),
 .UNSPECIFIED.);
#4743=B_SPLINE_CURVE_WITH_KNOTS('',3,(#153398,#153399,#153400,#153401,#153402,
#153403,#153404),.UNSPECIFIED.,.F.,.F.,(4,3,4),(3.94809455506897E-7,0.325960924204632,
1.),.UNSPECIFIED.);
#4744=B_SPLINE_CURVE_WITH_KNOTS('',3,(#153419,#153420,#153421,#153422),
 .UNSPECIFIED.,.F.,.F.,(4,4),(1.27679595912943E-6,1.),.UNSPECIFIED.);
#4745=B_SPLINE_CURVE_WITH_KNOTS('',3,(#153435,#153436,#153437,#153438),
 .UNSPECIFIED.,.F.,.F.,(4,4),(0.000876507471789284,0.010482245256776),
 .UNSPECIFIED.);
#4746=B_SPLINE_CURVE_WITH_KNOTS('',3,(#153440,#153441,#153442,#153443),
 .UNSPECIFIED.,.F.,.F.,(4,4),(0.000821546900565006,0.0104255562384257),
 .UNSPECIFIED.);
#4747=B_SPLINE_CURVE_WITH_KNOTS('',3,(#153456,#153457,#153458,#153459),
 .UNSPECIFIED.,.F.,.F.,(4,4),(0.,0.999998701161504),.UNSPECIFIED.);
#4748=B_SPLINE_CURVE_WITH_KNOTS('',3,(#153498,#153499,#153500,#153501,#153502,
#153503,#153504,#153505,#153506,#153507,#153508,#153509,#153510,#153511,
#153512,#153513),.UNSPECIFIED.,.F.,.F.,(4,3,3,3,3,4),(0.,0.234070507545302,
0.476434331275526,0.724187361959147,0.979964419025256,0.999998630096402),
 .UNSPECIFIED.);
#4749=B_SPLINE_CURVE_WITH_KNOTS('',3,(#153515,#153516,#153517,#153518,#153519,
#153520,#153521,#153522,#153523,#153524,#153525,#153526,#153527,#153528,
#153529,#153530),.UNSPECIFIED.,.F.,.F.,(4,3,3,3,3,4),(0.,0.25,0.495026107729062,
0.747513053864531,0.982920025273709,1.),.UNSPECIFIED.);
#4750=B_SPLINE_CURVE_WITH_KNOTS('',3,(#153533,#153534,#153535,#153536),
 .UNSPECIFIED.,.F.,.F.,(4,4),(0.,0.00385317783226068),.UNSPECIFIED.);
#4751=B_SPLINE_CURVE_WITH_KNOTS('',3,(#153551,#153552,#153553,#153554),
 .UNSPECIFIED.,.F.,.F.,(4,4),(0.000821546900565006,0.0104255562384257),
 .UNSPECIFIED.);
#4752=B_SPLINE_CURVE_WITH_KNOTS('',3,(#153555,#153556,#153557,#153558,#153559,
#153560,#153561,#153562,#153563,#153564,#153565,#153566,#153567,#153568,
#153569,#153570,#153571,#153572,#153573,#153574,#153575,#153576,#153577,
#153578,#153579,#153580,#153581,#153582,#153583,#153584,#153585,#153586,
#153587,#153588,#153589,#153590,#153591,#153592,#153593,#153594,#153595,
#153596,#153597,#153598,#153599,#153600,#153601,#153602,#153603,#153604,
#153605,#153606,#153607,#153608,#153609,#153610,#153611,#153612,#153613,
#153614,#153615,#153616,#153617,#153618,#153619,#153620,#153621,#153622,
#153623,#153624,#153625,#153626,#153627,#153628,#153629,#153630,#153631,
#153632,#153633,#153634,#153635,#153636,#153637,#153638,#153639,#153640,
#153641,#153642,#153643,#153644,#153645,#153646,#153647,#153648,#153649,
#153650,#153651,#153652,#153653,#153654,#153655,#153656,#153657,#153658,
#153659,#153660,#153661,#153662,#153663,#153664,#153665,#153666,#153667,
#153668,#153669,#153670,#153671,#153672,#153673,#153674,#153675,#153676,
#153677,#153678,#153679,#153680,#153681,#153682,#153683,#153684),
 .UNSPECIFIED.,.F.,.F.,(4,3,3,3,3,3,3,3,3,3,3,3,3,3,3,3,3,3,3,3,3,3,3,3,
3,3,3,3,3,3,3,3,3,3,3,3,3,3,3,3,3,3,3,4),(0.,0.0557300906452975,0.108669123630166,
0.16220672376782,0.206103361884435,0.228051680942743,0.239025840471897,
0.244512920236474,0.247256460118762,0.247942345089334,0.248143462518013,
0.25000000000105,0.28525026953172,0.319586978968953,0.35282166185891,0.375000000001453,
0.406706302027439,0.437500000001657,0.468750000001765,0.484375000001819,
0.492187500001848,0.496093750001873,0.496600762442034,0.498046875001885,
0.499023437501879,0.499267578126878,0.499450683595627,0.500000000001873,
0.548163509889134,0.598706375701685,0.625000000001358,0.679498466368399,
0.687500000001101,0.718750000000971,0.734375000000903,0.742187500000869,
0.746093750000855,0.74894953049805,0.750000000000842,0.806399791364996,
0.865484672157621,0.926633610120571,0.991716815566447,0.999967809902464),
 .UNSPECIFIED.);
#4753=B_SPLINE_CURVE_WITH_KNOTS('',3,(#153685,#153686,#153687,#153688,#153689,
#153690,#153691,#153692,#153693,#153694,#153695,#153696,#153697,#153698,
#153699,#153700,#153701,#153702,#153703,#153704,#153705,#153706,#153707,
#153708,#153709,#153710,#153711,#153712,#153713,#153714,#153715,#153716,
#153717,#153718,#153719,#153720,#153721,#153722,#153723,#153724,#153725,
#153726,#153727,#153728,#153729,#153730,#153731,#153732,#153733,#153734,
#153735,#153736,#153737,#153738,#153739,#153740,#153741,#153742,#153743,
#153744,#153745,#153746,#153747,#153748,#153749,#153750,#153751,#153752,
#153753,#153754,#153755,#153756,#153757,#153758,#153759,#153760,#153761,
#153762,#153763,#153764,#153765,#153766,#153767,#153768,#153769,#153770,
#153771,#153772,#153773,#153774,#153775,#153776,#153777,#153778,#153779,
#153780,#153781,#153782,#153783,#153784,#153785,#153786,#153787,#153788,
#153789,#153790),.UNSPECIFIED.,.F.,.F.,(4,3,3,3,3,3,3,3,3,3,3,3,3,3,3,3,
3,3,3,3,3,3,3,3,3,3,3,3,3,3,3,3,3,3,3,4),(1.17227643855583E-8,0.0584463886983609,
0.113231413189016,0.124999999993601,0.175293985242217,0.223827131926143,
0.248046874987312,0.249999999987212,0.253226722903014,0.327396670298302,
0.374999999980813,0.387436040596127,0.422635833669734,0.44231367500128,
0.498046874974511,0.499999999974409,0.503900809428433,0.556200109021788,
0.562499999970921,0.613653614494003,0.624511718717445,0.624999999967415,
0.643506073008206,0.662090682222471,0.680808883543099,0.699860002069781,
0.718997321555854,0.738880238098642,0.749023437478302,0.749999999978387,
0.751151936740845,0.80273675767465,0.854547924236456,0.906490674366243,
0.958653924668795,1.),.UNSPECIFIED.);
#4754=B_SPLINE_CURVE_WITH_KNOTS('',3,(#153794,#153795,#153796,#153797),
 .UNSPECIFIED.,.F.,.F.,(4,4),(0.000876507471789284,0.010482245256776),
 .UNSPECIFIED.);
#4755=B_SPLINE_CURVE_WITH_KNOTS('',3,(#153814,#153815,#153816,#153817,#153818,
#153819,#153820,#153821,#153822,#153823,#153824,#153825,#153826,#153827,
#153828,#153829),.UNSPECIFIED.,.F.,.F.,(4,3,3,3,3,4),(1.34720087857547E-6,
0.250001010400659,0.492522569244812,0.729567600587388,0.959631099383557,
1.),.UNSPECIFIED.);
#4756=B_SPLINE_CURVE_WITH_KNOTS('',3,(#153830,#153831,#153832,#153833,#153834,
#153835,#153836,#153837,#153838,#153839,#153840,#153841,#153842,#153843,
#153844,#153845,#153846,#153847,#153848,#153849,#153850,#153851,#153852,
#153853,#153854,#153855,#153856,#153857,#153858,#153859,#153860,#153861,
#153862,#153863,#153864,#153865,#153866,#153867,#153868,#153869,#153870,
#153871,#153872,#153873,#153874,#153875,#153876,#153877,#153878,#153879,
#153880,#153881,#153882,#153883,#153884,#153885,#153886,#153887,#153888,
#153889,#153890,#153891,#153892,#153893,#153894,#153895,#153896,#153897,
#153898,#153899,#153900,#153901,#153902,#153903,#153904,#153905,#153906,
#153907,#153908,#153909,#153910,#153911,#153912,#153913,#153914,#153915,
#153916,#153917,#153918,#153919,#153920,#153921,#153922,#153923,#153924,
#153925,#153926,#153927,#153928,#153929,#153930,#153931,#153932,#153933,
#153934,#153935,#153936,#153937,#153938,#153939,#153940,#153941,#153942,
#153943,#153944,#153945,#153946,#153947),.UNSPECIFIED.,.F.,.F.,(4,3,3,3,
3,3,3,3,3,3,3,3,3,3,3,3,3,3,3,3,3,3,3,3,3,3,3,3,3,3,3,3,3,3,3,3,3,3,3,4),
(3.18229911605046E-5,0.0312499999998296,0.0976865037949654,0.124999999999318,
0.182154808287466,0.187499999998977,0.218749999998807,0.234374999998721,
0.242187499998673,0.246093749998648,0.249795185825512,0.249999999998623,
0.25263968832415,0.345710027577214,0.374999999997752,0.437499999997316,
0.468749999997092,0.484374999996979,0.492187499996922,0.496093749996894,
0.499023437496878,0.499999999996877,0.510199912070258,0.541121704839755,
0.562499999997224,0.593749999997398,0.624999999997572,0.656249999997749,
0.687499999997927,0.718749999998099,0.73437499999819,0.742187499998239,
0.746093749998268,0.748046874998287,0.749999999998305,0.803805944723814,
0.858633463684494,0.914040237915491,0.97030630160842,1.),.UNSPECIFIED.);
#4757=B_SPLINE_CURVE_WITH_KNOTS('',3,(#153948,#153949,#153950,#153951,#153952,
#153953,#153954,#153955,#153956,#153957,#153958,#153959,#153960,#153961,
#153962,#153963,#153964,#153965,#153966,#153967,#153968,#153969,#153970,
#153971,#153972,#153973,#153974,#153975,#153976,#153977,#153978,#153979,
#153980,#153981,#153982,#153983,#153984,#153985,#153986,#153987,#153988,
#153989,#153990,#153991,#153992,#153993,#153994,#153995,#153996,#153997,
#153998,#153999,#154000,#154001,#154002,#154003,#154004,#154005,#154006,
#154007,#154008,#154009,#154010,#154011,#154012,#154013,#154014,#154015,
#154016,#154017,#154018,#154019,#154020,#154021,#154022,#154023,#154024,
#154025,#154026,#154027,#154028,#154029,#154030,#154031,#154032,#154033,
#154034,#154035,#154036,#154037,#154038,#154039,#154040,#154041,#154042,
#154043,#154044,#154045,#154046,#154047,#154048,#154049,#154050,#154051,
#154052,#154053,#154054,#154055,#154056,#154057,#154058,#154059,#154060,
#154061,#154062,#154063,#154064,#154065),.UNSPECIFIED.,.F.,.F.,(4,3,3,3,
3,3,3,3,3,3,3,3,3,3,3,3,3,3,3,3,3,3,3,3,3,3,3,3,3,3,3,3,3,3,3,3,3,3,3,4),
(8.34701282724942E-14,0.051104738268533,0.10144538171935,0.125000000000385,
0.177843714271829,0.187500000000577,0.218750000000668,0.234375000000713,
0.242187500000736,0.246093750000747,0.249259269767851,0.250000000000758,
0.312500000000785,0.375000000000812,0.437500000000845,0.468750000000868,
0.484375000000879,0.492187500000885,0.496093750000882,0.498901284980378,
0.500000000000879,0.548101422879337,0.598678455292358,0.625000000000582,
0.678879260280721,0.713530942889026,0.730856784193179,0.739519704845255,
0.743851165171293,0.746016895334312,0.747099760415822,0.747641192956576,
0.748033970104978,0.748182625497331,0.75000000000027,0.799033416400584,
0.850056418490652,0.902463987625779,0.957816263810161,0.99999998849761),
 .UNSPECIFIED.);
#4758=B_SPLINE_CURVE_WITH_KNOTS('',3,(#154070,#154071,#154072,#154073,#154074,
#154075,#154076,#154077,#154078,#154079,#154080,#154081,#154082,#154083,
#154084,#154085),.UNSPECIFIED.,.F.,.F.,(4,3,3,3,3,4),(0.,0.230911412126844,
0.468240019037909,0.709718394074353,0.957565639068108,1.),.UNSPECIFIED.);
#4759=B_SPLINE_CURVE_WITH_KNOTS('',3,(#154086,#154087,#154088,#154089),
 .UNSPECIFIED.,.F.,.F.,(4,4),(0.,0.0041383639263312),.UNSPECIFIED.);
#4760=B_SPLINE_CURVE_WITH_KNOTS('',3,(#154094,#154095,#154096,#154097,#154098,
#154099,#154100,#154101,#154102,#154103,#154104,#154105,#154106,#154107,
#154108,#154109,#154110,#154111,#154112,#154113,#154114,#154115,#154116,
#154117,#154118,#154119,#154120,#154121,#154122,#154123,#154124,#154125,
#154126,#154127,#154128,#154129,#154130,#154131,#154132,#154133,#154134,
#154135,#154136,#154137,#154138,#154139,#154140,#154141,#154142,#154143,
#154144,#154145,#154146,#154147,#154148),.UNSPECIFIED.,.F.,.F.,(4,3,3,3,
3,3,3,3,3,3,3,3,3,3,3,3,3,3,4),(0.,0.0632048838696367,0.127921929473124,
0.195281348929666,0.249999999999537,0.321563999196289,0.374999999999306,
0.437499999999191,0.468749999999113,0.484374999999066,0.492187499999073,
0.498658068589728,0.49999999999908,0.59334512646801,0.688354285547602,0.785958734092665,
0.885147124073086,0.986657689579597,0.999999999999993),.UNSPECIFIED.);
#4761=B_SPLINE_CURVE_WITH_KNOTS('',3,(#154149,#154150,#154151,#154152,#154153,
#154154,#154155,#154156,#154157,#154158,#154159,#154160,#154161,#154162,
#154163,#154164,#154165,#154166,#154167,#154168,#154169,#154170,#154171,
#154172,#154173,#154174,#154175,#154176,#154177,#154178,#154179,#154180,
#154181,#154182,#154183,#154184,#154185,#154186,#154187,#154188,#154189,
#154190,#154191,#154192,#154193,#154194,#154195,#154196,#154197,#154198,
#154199,#154200,#154201,#154202,#154203,#154204,#154205,#154206,#154207,
#154208,#154209,#154210,#154211,#154212,#154213,#154214,#154215,#154216,
#154217,#154218,#154219,#154220,#154221,#154222,#154223,#154224,#154225,
#154226,#154227),.UNSPECIFIED.,.F.,.F.,(4,3,3,3,3,3,3,3,3,3,3,3,3,3,3,3,
3,3,3,3,3,3,3,3,3,3,4),(0.,0.0822388323866184,0.125000000000039,0.203743158983877,
0.249314582772148,0.282486317967716,0.332958488475827,0.36498976178814,
0.394097477848506,0.473638989559932,0.48437500000016,0.494250955016996,
0.50000000000016,0.522888790187838,0.595779308163083,0.625000000000112,
0.697913150166242,0.734375000000034,0.742187500000031,0.748069533718682,
0.750000000000028,0.77031774650841,0.824713583203907,0.880483079532543,
0.937161849130565,0.99522645066287,1.),.UNSPECIFIED.);
#4762=B_SPLINE_CURVE_WITH_KNOTS('',3,(#154258,#154259,#154260,#154261,#154262,
#154263,#154264,#154265,#154266,#154267,#154268,#154269,#154270),
 .UNSPECIFIED.,.F.,.F.,(4,3,3,3,4),(0.,0.264159105979835,0.53472290465884,
0.816453844755532,1.),.UNSPECIFIED.);
#4763=B_SPLINE_CURVE_WITH_KNOTS('',3,(#154275,#154276,#154277,#154278,#154279,
#154280,#154281,#154282,#154283,#154284,#154285,#154286,#154287,#154288,
#154289,#154290,#154291,#154292,#154293,#154294,#154295,#154296,#154297,
#154298,#154299,#154300,#154301,#154302,#154303,#154304,#154305,#154306,
#154307,#154308,#154309,#154310,#154311,#154312,#154313,#154314,#154315,
#154316,#154317,#154318,#154319,#154320,#154321,#154322,#154323,#154324,
#154325,#154326,#154327,#154328,#154329,#154330,#154331,#154332,#154333,
#154334,#154335,#154336,#154337,#154338,#154339,#154340,#154341,#154342,
#154343,#154344,#154345,#154346,#154347,#154348,#154349,#154350),
 .UNSPECIFIED.,.F.,.F.,(4,3,3,3,3,3,3,3,3,3,3,3,3,3,3,3,3,3,3,3,3,3,3,3,
3,4),(0.,0.0869793228874166,0.124999999999851,0.199030619385428,0.245213138173373,
0.273061238771005,0.32653577523374,0.364990790896793,0.39936394258499,0.484374999999404,
0.494494116758885,0.499999999999391,0.514138283290129,0.599085378376048,
0.62499999999927,0.68749999999923,0.71874999999921,0.7343749999992,0.742187499999195,
0.748148077780528,0.74999999999919,0.804514066320572,0.85851274981487,0.911762507617596,
0.963252162150356,1.),.UNSPECIFIED.);
#4764=B_SPLINE_CURVE_WITH_KNOTS('',3,(#154351,#154352,#154353,#154354,#154355,
#154356,#154357,#154358,#154359,#154360,#154361,#154362,#154363,#154364,
#154365,#154366,#154367),.UNSPECIFIED.,.F.,.F.,(4,2,2,2,1,1,1,2,2,4),(0.,
0.250000000000024,0.375000000000034,0.437500000000038,0.468750000000039,
0.48437500000004,0.492187500000042,0.496093750000043,0.500000000000043,
1.),.UNSPECIFIED.);
#4765=B_SPLINE_CURVE_WITH_KNOTS('',3,(#154370,#154371,#154372,#154373,#154374,
#154375,#154376,#154377,#154378,#154379,#154380,#154381,#154382,#154383,
#154384,#154385,#154386,#154387,#154388,#154389,#154390,#154391,#154392,
#154393,#154394,#154395,#154396,#154397),.UNSPECIFIED.,.F.,.F.,(4,3,3,3,
3,3,3,3,3,4),(0.,0.163940541204184,0.333114778935776,0.498046874999602,
0.499999999999603,0.50003591612275,0.639284504482635,0.781135100020726,
0.927355971067516,1.),.UNSPECIFIED.);
#4766=B_SPLINE_CURVE_WITH_KNOTS('',3,(#154399,#154400,#154401,#154402,#154403,
#154404,#154405,#154406,#154407,#154408,#154409,#154410,#154411,#154412,
#154413,#154414),.UNSPECIFIED.,.F.,.F.,(4,3,3,3,3,4),(4.19542126215829E-7,
0.2338396427201,0.339508613309501,0.56969049637124,0.786423133885641,1.),
 .UNSPECIFIED.);
#4767=B_SPLINE_CURVE_WITH_KNOTS('',3,(#154415,#154416,#154417,#154418,#154419,
#154420,#154421,#154422,#154423,#154424,#154425,#154426,#154427,#154428,
#154429,#154430,#154431,#154432,#154433),.UNSPECIFIED.,.F.,.F.,(4,3,3,3,
3,3,4),(0.,0.206475863478243,0.405461434738878,0.600838474120482,0.800419237060241,
0.988221216743423,1.),.UNSPECIFIED.);
#4768=B_SPLINE_CURVE_WITH_KNOTS('',3,(#154453,#154454,#154455,#154456,#154457,
#154458,#154459,#154460,#154461,#154462,#154463,#154464,#154465,#154466,
#154467,#154468,#154469,#154470,#154471,#154472,#154473,#154474,#154475,
#154476,#154477,#154478,#154479,#154480,#154481,#154482,#154483,#154484,
#154485,#154486,#154487,#154488,#154489,#154490,#154491,#154492,#154493,
#154494,#154495,#154496,#154497,#154498,#154499,#154500,#154501,#154502,
#154503,#154504,#154505,#154506,#154507),.UNSPECIFIED.,.F.,.F.,(4,3,3,3,
3,3,3,3,3,3,3,3,3,3,3,3,3,3,4),(0.,0.0708860635919454,0.140367818135151,
0.207849069624002,0.249999999999808,0.315086127274307,0.378502885651149,
0.437499999999646,0.46874999999961,0.484374999999591,0.492187499999582,
0.496093749999571,0.49999999999956,0.592295283092291,0.685212828844724,
0.74999999999978,0.845125224808466,0.93995821969057,1.),.UNSPECIFIED.);
#4769=B_SPLINE_CURVE_WITH_KNOTS('',3,(#154509,#154510,#154511,#154512,#154513,
#154514,#154515,#154516,#154517,#154518,#154519,#154520,#154521),
 .UNSPECIFIED.,.F.,.F.,(4,3,3,3,4),(0.000801891157765995,0.00312464263181538,
0.00585483490544955,0.00838933971206778,0.00949544874465978),
 .UNSPECIFIED.);
#4770=B_SPLINE_CURVE_WITH_KNOTS('',3,(#154522,#154523,#154524,#154525,#154526,
#154527,#154528,#154529,#154530,#154531,#154532,#154533,#154534,#154535,
#154536,#154537,#154538,#154539,#154540,#154541,#154542,#154543,#154544,
#154545,#154546,#154547,#154548,#154549,#154550,#154551,#154552,#154553,
#154554,#154555,#154556,#154557,#154558,#154559,#154560,#154561,#154562,
#154563,#154564,#154565,#154566,#154567,#154568,#154569,#154570,#154571,
#154572,#154573,#154574,#154575,#154576,#154577,#154578,#154579,#154580,
#154581,#154582,#154583,#154584,#154585,#154586,#154587,#154588,#154589,
#154590,#154591,#154592,#154593,#154594,#154595,#154596,#154597,#154598,
#154599,#154600),.UNSPECIFIED.,.F.,.F.,(4,3,3,3,3,3,3,3,3,3,3,3,3,3,3,3,
3,3,3,3,3,3,3,3,3,3,4),(0.,0.0585857549643099,0.115353783315363,0.124999999999788,
0.179827236593527,0.187499999999675,0.218749999999618,0.234374999999589,
0.242187499999581,0.246093749999577,0.249999999999573,0.340405595850071,
0.374999999999441,0.437499999999376,0.468749999999343,0.484374999999334,
0.492187499999323,0.496093749999317,0.499999999999311,0.564089078061403,
0.628856738294988,0.694923673370365,0.749999999999655,0.818394393929608,
0.887854174965178,0.959138516319878,1.),.UNSPECIFIED.);
#4771=B_SPLINE_CURVE_WITH_KNOTS('',3,(#154605,#154606,#154607,#154608,#154609,
#154610,#154611,#154612,#154613,#154614,#154615,#154616,#154617),
 .UNSPECIFIED.,.F.,.F.,(4,3,3,3,4),(0.000734608576009405,0.00325207345693861,
0.00595173535833846,0.00710294415665481,0.0094247370890218),
 .UNSPECIFIED.);
#4772=B_SPLINE_CURVE_WITH_KNOTS('',3,(#154638,#154639,#154640,#154641,#154642,
#154643,#154644,#154645,#154646,#154647,#154648,#154649,#154650,#154651,
#154652,#154653,#154654,#154655,#154656,#154657,#154658,#154659,#154660,
#154661,#154662,#154663,#154664,#154665,#154666,#154667,#154668,#154669,
#154670,#154671,#154672,#154673,#154674,#154675,#154676,#154677,#154678,
#154679,#154680,#154681,#154682,#154683,#154684,#154685,#154686,#154687,
#154688,#154689,#154690,#154691,#154692,#154693,#154694,#154695,#154696,
#154697,#154698,#154699,#154700,#154701,#154702,#154703,#154704,#154705,
#154706,#154707,#154708,#154709,#154710,#154711,#154712,#154713,#154714,
#154715,#154716,#154717,#154718,#154719,#154720,#154721,#154722),
 .UNSPECIFIED.,.F.,.F.,(4,3,3,3,3,3,3,3,3,3,3,3,3,3,3,3,3,3,3,3,3,3,3,3,
3,3,3,3,4),(0.,0.0689593679009489,0.131763023438308,0.190881511719319,0.220440755859824,
0.235220377930077,0.23891528344764,0.241686462585813,0.242263277167448,
0.248759657469872,0.25000000000033,0.33324707772351,0.37500000000042,0.406250000000441,
0.437500000000461,0.468750000000477,0.484375000000485,0.492187500000485,
0.49609375000048,0.499458273983288,0.500000000000475,0.562500000000416,
0.609375000000371,0.679687500000304,0.750000000000238,0.825469442525012,
0.875000000000119,0.957373830350825,0.999990011221892),.UNSPECIFIED.);
#4773=B_SPLINE_CURVE_WITH_KNOTS('',3,(#154724,#154725,#154726,#154727,#154728,
#154729,#154730,#154731,#154732,#154733,#154734,#154735,#154736,#154737,
#154738,#154739),.UNSPECIFIED.,.F.,.F.,(4,3,3,3,3,4),(0.,0.215215032325329,
0.443136127796081,0.660489501790431,0.894219532612502,0.999999580511107),
 .UNSPECIFIED.);
#4774=B_SPLINE_CURVE_WITH_KNOTS('',3,(#154740,#154741,#154742,#154743,#154744,
#154745,#154746,#154747,#154748,#154749,#154750,#154751,#154752,#154753,
#154754,#154755,#154756,#154757,#154758,#154759,#154760,#154761,#154762,
#154763,#154764,#154765,#154766,#154767,#154768,#154769,#154770,#154771,
#154772,#154773,#154774,#154775,#154776,#154777,#154778,#154779,#154780,
#154781,#154782,#154783,#154784,#154785,#154786,#154787,#154788,#154789,
#154790,#154791,#154792,#154793,#154794,#154795,#154796,#154797,#154798,
#154799,#154800,#154801,#154802,#154803,#154804,#154805,#154806),
 .UNSPECIFIED.,.F.,.F.,(4,3,3,3,3,3,3,3,3,3,3,3,3,3,3,3,3,3,3,3,3,3,4),
(6.92056175195316E-9,0.0702731195301449,0.124999999999889,0.18554687499984,
0.246093749999791,0.249999999999789,0.252383107672787,0.351045659631276,
0.374999999999917,0.4417236941113,0.496093750000031,0.500000000000033,0.5024909590578,
0.581475430365078,0.625000000000024,0.656250000000022,0.68750000000002,
0.723520265942537,0.750000000000016,0.812500000000012,0.859375000000009,
0.968403554298818,1.),.UNSPECIFIED.);
#4775=B_SPLINE_CURVE_WITH_KNOTS('',3,(#154855,#154856,#154857,#154858,#154859,
#154860,#154861,#154862,#154863,#154864,#154865,#154866,#154867),
 .UNSPECIFIED.,.F.,.F.,(4,3,3,3,4),(0.000799595655510347,0.00312305020211246,
0.00581514086608832,0.00831497793897699,0.00946542910228819),
 .UNSPECIFIED.);
#4776=B_SPLINE_CURVE_WITH_KNOTS('',3,(#154869,#154870,#154871,#154872,#154873,
#154874,#154875,#154876,#154877,#154878,#154879,#154880,#154881,#154882,
#154883,#154884,#154885,#154886,#154887,#154888,#154889,#154890,#154891,
#154892,#154893,#154894,#154895,#154896,#154897,#154898,#154899,#154900,
#154901,#154902,#154903,#154904,#154905,#154906,#154907,#154908,#154909,
#154910,#154911,#154912,#154913,#154914,#154915,#154916,#154917,#154918,
#154919,#154920,#154921,#154922,#154923,#154924,#154925,#154926,#154927,
#154928,#154929,#154930,#154931,#154932,#154933,#154934,#154935,#154936,
#154937,#154938,#154939,#154940,#154941,#154942,#154943,#154944),
 .UNSPECIFIED.,.F.,.F.,(4,3,3,3,3,3,3,3,3,3,3,3,3,3,3,3,3,3,3,3,3,3,3,3,
3,4),(2.00063521920002E-13,0.0591216028065502,0.117082720868845,0.125000000000246,
0.187500000000369,0.21875000000043,0.234375000000461,0.242187500000477,
0.246093750000481,0.250000000000486,0.346565173458337,0.375000000000604,
0.46785306768388,0.496093750000721,0.499268681857144,0.500000000000721,
0.552855316954113,0.562500000000631,0.609375000000563,0.666076030952446,
0.722777061904329,0.75000000000036,0.821201537843276,0.87500000000018,0.954964862982302,
0.999999992138103),.UNSPECIFIED.);
#4777=B_SPLINE_CURVE_WITH_KNOTS('',3,(#154946,#154947,#154948,#154949,#154950,
#154951,#154952,#154953,#154954,#154955,#154956,#154957,#154958,#154959,
#154960,#154961),.UNSPECIFIED.,.F.,.F.,(4,3,3,3,3,4),(4.29492375686315E-7,
0.233750383144039,0.340769128367464,0.569821997539196,0.785318576880101,
1.),.UNSPECIFIED.);
#4778=B_SPLINE_CURVE_WITH_KNOTS('',3,(#154962,#154963,#154964,#154965,#154966,
#154967,#154968,#154969,#154970,#154971,#154972,#154973,#154974,#154975,
#154976,#154977,#154978,#154979,#154980),.UNSPECIFIED.,.F.,.F.,(4,2,2,2,
1,1,1,2,2,2,4),(1.10457472515728E-5,0.249999999999914,0.374999999999875,
0.437499999999855,0.468749999999841,0.48437499999983,0.492187499999825,
0.496093749999822,0.49999999999982,0.74999999999991,1.),.UNSPECIFIED.);
#4779=B_SPLINE_CURVE_WITH_KNOTS('',3,(#154984,#154985,#154986,#154987,#154988,
#154989,#154990,#154991,#154992,#154993,#154994,#154995,#154996),
 .UNSPECIFIED.,.F.,.F.,(4,3,3,3,4),(0.000731998639840557,0.00321503108606633,
0.00587687390152188,0.00707184840840047,0.00939432936633357),
 .UNSPECIFIED.);
#4780=B_SPLINE_CURVE_WITH_KNOTS('',3,(#155019,#155020,#155021,#155022,#155023,
#155024,#155025,#155026,#155027,#155028,#155029,#155030,#155031,#155032,
#155033,#155034),.UNSPECIFIED.,.F.,.F.,(4,3,3,3,3,4),(0.,0.213825330538362,
0.440424504941056,0.659229336836956,0.892889616266567,0.999999570551571),
 .UNSPECIFIED.);
#4781=B_SPLINE_CURVE_WITH_KNOTS('',3,(#155035,#155036,#155037,#155038,#155039,
#155040,#155041,#155042,#155043,#155044,#155045,#155046,#155047,#155048,
#155049,#155050,#155051,#155052,#155053,#155054,#155055,#155056,#155057,
#155058,#155059,#155060,#155061,#155062,#155063,#155064,#155065,#155066,
#155067,#155068,#155069,#155070,#155071,#155072,#155073,#155074,#155075,
#155076,#155077,#155078,#155079,#155080,#155081,#155082,#155083,#155084,
#155085,#155086,#155087,#155088,#155089,#155090,#155091,#155092,#155093,
#155094,#155095,#155096,#155097,#155098,#155099,#155100,#155101,#155102,
#155103,#155104,#155105,#155106,#155107,#155108,#155109,#155110,#155111,
#155112,#155113,#155114,#155115,#155116,#155117,#155118,#155119,#155120,
#155121,#155122,#155123,#155124,#155125,#155126,#155127,#155128,#155129,
#155130,#155131,#155132,#155133,#155134,#155135,#155136,#155137,#155138,
#155139,#155140,#155141,#155142,#155143,#155144,#155145,#155146,#155147,
#155148,#155149),.UNSPECIFIED.,.F.,.F.,(4,3,3,3,3,3,3,3,3,3,3,3,3,3,3,3,
3,3,3,3,3,3,3,3,3,3,3,3,3,3,3,3,3,3,3,3,3,3,4),(7.04705196002291E-9,0.0707966831419206,
0.124999999999487,0.185546874999241,0.246093749998995,0.249999999998986,
0.252359143174423,0.349332373867497,0.374999999998765,0.441778173658313,
0.498046874998564,0.499999999998558,0.503193747522868,0.544115575223839,
0.562499999998729,0.59374999999881,0.609374999998851,0.617187499998871,
0.621093749998881,0.623046874998886,0.624999999998891,0.648786262364636,
0.67299328259835,0.687499999998841,0.712035681312914,0.718749999998816,
0.734374999998814,0.742187499998798,0.746093749998791,0.748046874998788,
0.749023437498787,0.749267578123787,0.749633789061286,0.749999999998785,
0.751100775325356,0.815360308562951,0.879496436852205,0.943465428441742,
1.),.UNSPECIFIED.);
#4782=B_SPLINE_CURVE_WITH_KNOTS('',3,(#155150,#155151,#155152,#155153,#155154,
#155155,#155156,#155157,#155158,#155159,#155160,#155161,#155162,#155163,
#155164,#155165,#155166,#155167,#155168,#155169,#155170,#155171,#155172,
#155173,#155174,#155175,#155176,#155177,#155178,#155179,#155180,#155181,
#155182,#155183,#155184,#155185,#155186,#155187,#155188,#155189,#155190,
#155191,#155192,#155193,#155194,#155195,#155196,#155197,#155198,#155199,
#155200,#155201,#155202,#155203,#155204,#155205,#155206,#155207,#155208,
#155209,#155210,#155211,#155212,#155213,#155214,#155215,#155216,#155217,
#155218,#155219,#155220,#155221,#155222,#155223,#155224,#155225,#155226,
#155227,#155228,#155229,#155230,#155231,#155232,#155233,#155234,#155235,
#155236,#155237),.UNSPECIFIED.,.F.,.F.,(4,3,3,3,3,3,3,3,3,3,3,3,3,3,3,3,
3,3,3,3,3,3,3,3,3,3,3,3,3,4),(0.,0.069441977607991,0.132550750715234,0.191275375357326,
0.220637687678371,0.235318843838894,0.238989132879025,0.241741849659123,
0.242574401393792,0.249103102141126,0.249999999999417,0.333593575490244,
0.374999999999471,0.406249999999485,0.437499999999498,0.468749999999512,
0.48437499999951,0.4921874999995,0.496093749999504,0.49946576207654,0.499999999999507,
0.562499999999569,0.609374999999615,0.679687499999684,0.749999999999754,
0.812499999999815,0.891008696034271,0.906249999999908,0.989050414896488,
0.999989783729688),.UNSPECIFIED.);
#4783=B_SPLINE_CURVE_WITH_KNOTS('',3,(#155242,#155243,#155244,#155245,#155246,
#155247,#155248,#155249,#155250,#155251,#155252,#155253,#155254,#155255,
#155256,#155257,#155258,#155259,#155260),.UNSPECIFIED.,.F.,.F.,(4,3,3,3,
3,3,4),(0.,0.185535625540095,0.37453758023397,0.569181963234827,0.767518059616989,
0.971532910971265,1.),.UNSPECIFIED.);
#4784=B_SPLINE_CURVE_WITH_KNOTS('',3,(#155261,#155262,#155263,#155264,#155265,
#155266,#155267,#155268,#155269,#155270,#155271,#155272,#155273,#155274,
#155275,#155276,#155277,#155278,#155279,#155280,#155281,#155282,#155283,
#155284,#155285,#155286,#155287,#155288),.UNSPECIFIED.,.F.,.F.,(4,3,3,3,
3,3,3,3,3,4),(0.,0.144905414369803,0.28628718158065,0.424070029202907,0.49804687499993,
0.4999598944088,0.499999999999929,0.669838342253323,0.834919171126662,1.),
 .UNSPECIFIED.);
#4785=B_SPLINE_CURVE_WITH_KNOTS('',3,(#155290,#155291,#155292,#155293,#155294,
#155295,#155296,#155297,#155298,#155299,#155300,#155301,#155302,#155303,
#155304,#155305),.UNSPECIFIED.,.F.,.F.,(4,2,2,2,1,1,2,2,4),(0.,0.249999999999503,
0.374999999999255,0.437499999999149,0.46874999999912,0.484374999999104,
0.492187499999097,0.499999999999091,1.),.UNSPECIFIED.);
#4786=B_SPLINE_CURVE_WITH_KNOTS('',3,(#155309,#155310,#155311,#155312,#155313,
#155314,#155315,#155316,#155317,#155318,#155319,#155320,#155321,#155322,
#155323,#155324),.UNSPECIFIED.,.F.,.F.,(4,3,3,3,3,4),(0.,0.227672506314025,
0.443584943305661,0.653737655502801,0.855842244026882,1.),.UNSPECIFIED.);
#4787=B_SPLINE_CURVE_WITH_KNOTS('',3,(#155325,#155326,#155327,#155328,#155329,
#155330,#155331,#155332,#155333,#155334,#155335,#155336,#155337,#155338,
#155339,#155340,#155341,#155342,#155343,#155344,#155345,#155346,#155347,
#155348,#155349,#155350,#155351,#155352,#155353,#155354,#155355,#155356,
#155357,#155358,#155359,#155360,#155361,#155362,#155363,#155364,#155365,
#155366,#155367),.UNSPECIFIED.,.F.,.F.,(4,3,3,3,3,3,3,3,3,3,3,3,3,3,4),
(0.,0.13007938114654,0.249999999999951,0.363303681175031,0.461966998162734,
0.496093749999904,0.499999999999904,0.500099040742567,0.58565984718958,
0.670743841464584,0.749999999999952,0.825272702193343,0.900311502331646,
0.975559281692812,1.),.UNSPECIFIED.);
#4788=B_SPLINE_CURVE_WITH_KNOTS('',3,(#155379,#155380,#155381,#155382,#155383,
#155384,#155385,#155386,#155387,#155388,#155389,#155390,#155391,#155392,
#155393,#155394,#155395,#155396,#155397,#155398,#155399,#155400,#155401,
#155402,#155403,#155404,#155405,#155406,#155407,#155408,#155409,#155410,
#155411,#155412,#155413,#155414,#155415,#155416,#155417,#155418,#155419,
#155420,#155421,#155422,#155423,#155424,#155425,#155426,#155427,#155428,
#155429,#155430,#155431,#155432,#155433,#155434,#155435,#155436,#155437,
#155438,#155439,#155440,#155441,#155442,#155443,#155444,#155445,#155446,
#155447,#155448),.UNSPECIFIED.,.F.,.F.,(4,3,3,3,3,3,3,3,3,3,3,3,3,3,3,3,
3,3,3,3,3,3,3,4),(0.,0.0468252282105052,0.0625000000000385,0.111671414475211,
0.161991880251615,0.215493244493045,0.234375000000112,0.242187500000095,
0.248559869936323,0.250000000000078,0.328196609751316,0.374999999999974,
0.432074481984959,0.469350116156201,0.478281110394449,0.484374999999853,
0.494498947188093,0.499999999999825,0.575316649815483,0.654093366024209,
0.717727187058543,0.806910800011888,0.905137785263374,1.),.UNSPECIFIED.);
#4789=B_SPLINE_CURVE_WITH_KNOTS('',3,(#155451,#155452,#155453,#155454,#155455,
#155456,#155457,#155458,#155459,#155460,#155461,#155462,#155463,#155464,
#155465,#155466,#155467,#155468,#155469,#155470,#155471,#155472,#155473,
#155474,#155475,#155476,#155477,#155478,#155479,#155480,#155481,#155482,
#155483,#155484,#155485,#155486,#155487,#155488,#155489,#155490,#155491,
#155492,#155493,#155494,#155495,#155496,#155497,#155498,#155499,#155500,
#155501,#155502,#155503,#155504,#155505,#155506,#155507,#155508,#155509,
#155510,#155511,#155512,#155513,#155514,#155515,#155516,#155517),
 .UNSPECIFIED.,.F.,.F.,(4,3,3,3,3,3,3,3,3,3,3,3,3,3,3,3,3,3,3,3,3,3,4),
(0.,0.100728557328594,0.199752664823961,0.29623824427798,0.375000000000072,
0.437500000000091,0.468750000000082,0.484375000000094,0.49448394416446,
0.500000000000106,0.581634289657116,0.660418077435017,0.687500000000417,
0.718750000000468,0.734375000000501,0.742187500000507,0.748155000660193,
0.750000000000513,0.803598400947262,0.856014092687743,0.907470928865847,
0.957106875072136,1.),.UNSPECIFIED.);
#4790=B_SPLINE_CURVE_WITH_KNOTS('',3,(#155520,#155521,#155522,#155523),
 .UNSPECIFIED.,.F.,.F.,(4,4),(0.,0.00454447370442107),.UNSPECIFIED.);
#4791=B_SPLINE_CURVE_WITH_KNOTS('',3,(#155525,#155526,#155527,#155528,#155529,
#155530,#155531,#155532,#155533,#155534,#155535,#155536,#155537,#155538,
#155539,#155540),.UNSPECIFIED.,.F.,.F.,(4,3,3,3,3,4),(0.,0.228718000314846,
0.465913558148734,0.708585998597329,0.959609200667992,0.999998621928069),
 .UNSPECIFIED.);
#4792=B_SPLINE_CURVE_WITH_KNOTS('',3,(#155541,#155542,#155543,#155544,#155545,
#155546,#155547,#155548,#155549,#155550,#155551,#155552,#155553,#155554,
#155555,#155556),.UNSPECIFIED.,.F.,.F.,(4,3,3,3,3,4),(0.,0.25,0.485591974112626,
0.71711850744027,0.943391881004635,1.),.UNSPECIFIED.);
#4793=B_SPLINE_CURVE_WITH_KNOTS('',3,(#155570,#155571,#155572,#155573,#155574,
#155575,#155576,#155577,#155578,#155579,#155580,#155581,#155582,#155583,
#155584,#155585,#155586,#155587,#155588,#155589,#155590,#155591,#155592,
#155593,#155594,#155595,#155596,#155597,#155598,#155599,#155600,#155601,
#155602,#155603,#155604,#155605,#155606,#155607,#155608,#155609,#155610,
#155611,#155612,#155613,#155614,#155615,#155616,#155617,#155618,#155619,
#155620,#155621,#155622,#155623,#155624,#155625,#155626,#155627,#155628,
#155629,#155630,#155631,#155632,#155633,#155634,#155635,#155636,#155637,
#155638,#155639,#155640,#155641,#155642,#155643,#155644,#155645,#155646,
#155647,#155648,#155649,#155650,#155651,#155652,#155653,#155654,#155655,
#155656,#155657,#155658,#155659,#155660,#155661,#155662,#155663,#155664,
#155665,#155666,#155667,#155668,#155669,#155670,#155671,#155672),
 .UNSPECIFIED.,.F.,.F.,(4,3,3,3,3,3,3,3,3,3,3,3,3,3,3,3,3,3,3,3,3,3,3,3,
3,3,3,3,3,3,3,3,3,3,4),(1.17970694753713E-8,0.0587741274153463,0.113845507635111,
0.124999999999931,0.175544805271069,0.224300881613421,0.248046874999881,
0.24999999999988,0.253204771838808,0.328016123646574,0.374999999999958,
0.387439460343596,0.422619984926577,0.442478326522261,0.498046875000016,
0.500000000000013,0.503886071361003,0.555745869040186,0.562500000000114,
0.593750000000165,0.609375000000191,0.617187500000204,0.62109375000021,
0.625000000000216,0.687500000000337,0.718750000000397,0.734375000000433,
0.742187500000451,0.746093750000454,0.750000000000456,0.751226796212957,
0.81468448368076,0.875000000000228,0.938570202129679,1.),.UNSPECIFIED.);
#4794=B_SPLINE_CURVE_WITH_KNOTS('',3,(#155674,#155675,#155676,#155677),
 .UNSPECIFIED.,.F.,.F.,(4,4),(0.000819410081741501,0.0104007046320713),
 .UNSPECIFIED.);
#4795=B_SPLINE_CURVE_WITH_KNOTS('',3,(#155678,#155679,#155680,#155681,#155682,
#155683,#155684,#155685,#155686,#155687,#155688,#155689,#155690,#155691,
#155692,#155693,#155694,#155695,#155696,#155697,#155698,#155699,#155700,
#155701,#155702,#155703,#155704,#155705,#155706,#155707,#155708,#155709,
#155710,#155711,#155712,#155713,#155714,#155715,#155716,#155717,#155718,
#155719,#155720,#155721,#155722,#155723,#155724,#155725,#155726,#155727,
#155728,#155729,#155730,#155731,#155732,#155733,#155734,#155735,#155736,
#155737,#155738,#155739,#155740,#155741,#155742,#155743,#155744,#155745,
#155746,#155747,#155748,#155749,#155750,#155751,#155752,#155753,#155754,
#155755,#155756,#155757,#155758,#155759,#155760,#155761,#155762,#155763,
#155764,#155765,#155766,#155767,#155768,#155769,#155770,#155771,#155772,
#155773,#155774,#155775,#155776,#155777,#155778,#155779,#155780,#155781,
#155782,#155783,#155784,#155785,#155786,#155787,#155788,#155789,#155790,
#155791,#155792,#155793,#155794,#155795,#155796,#155797,#155798,#155799,
#155800,#155801,#155802,#155803,#155804,#155805,#155806,#155807),
 .UNSPECIFIED.,.F.,.F.,(4,3,3,3,3,3,3,3,3,3,3,3,3,3,3,3,3,3,3,3,3,3,3,3,
3,3,3,3,3,3,3,3,3,3,3,3,3,3,3,3,3,3,3,4),(0.,0.0560216703334645,0.109196961913243,
0.163091705635906,0.206545852817787,0.228272926408728,0.239136463204198,
0.244568231601933,0.247284115800801,0.247963086850518,0.248140226278139,
0.249999999999668,0.284700972192902,0.318528987481047,0.351288118199589,
0.374999999998669,0.406284954267776,0.437499999998176,0.46874999999793,
0.484374999997806,0.492187499997762,0.496093749997764,0.496366305327242,
0.498046874997764,0.499023437497763,0.499267578122763,0.499450683591513,
0.499999999997763,0.548181491589199,0.598745345927553,0.624999999998493,
0.67952017226536,0.687499999998851,0.718749999999024,0.73437499999911,0.742187499999145,
0.746093749999162,0.748968852511644,0.74999999999918,0.806751404285961,
0.866224004565218,0.927798228713741,0.993361011423219,0.999967748998623),
 .UNSPECIFIED.);
#4796=B_SPLINE_CURVE_WITH_KNOTS('',3,(#155812,#155813,#155814,#155815),
 .UNSPECIFIED.,.F.,.F.,(4,4),(0.000874668174674732,0.0104577126980746),
 .UNSPECIFIED.);
#4797=B_SPLINE_CURVE_WITH_KNOTS('',3,(#155830,#155831,#155832,#155833,#155834,
#155835,#155836,#155837,#155838,#155839,#155840,#155841,#155842,#155843,
#155844,#155845,#155846,#155847,#155848,#155849,#155850,#155851,#155852,
#155853,#155854,#155855,#155856,#155857,#155858,#155859,#155860,#155861,
#155862,#155863,#155864,#155865,#155866,#155867,#155868,#155869,#155870,
#155871,#155872,#155873,#155874,#155875,#155876,#155877,#155878,#155879,
#155880,#155881,#155882,#155883,#155884,#155885,#155886,#155887,#155888,
#155889,#155890,#155891,#155892,#155893,#155894,#155895,#155896,#155897,
#155898,#155899,#155900,#155901,#155902,#155903,#155904,#155905,#155906,
#155907,#155908,#155909,#155910,#155911,#155912,#155913,#155914,#155915,
#155916,#155917,#155918,#155919,#155920,#155921,#155922,#155923,#155924,
#155925,#155926,#155927,#155928,#155929,#155930,#155931,#155932,#155933,
#155934,#155935,#155936,#155937,#155938,#155939,#155940,#155941,#155942,
#155943,#155944,#155945,#155946,#155947,#155948,#155949,#155950),
 .UNSPECIFIED.,.F.,.F.,(4,3,3,3,3,3,3,3,3,3,3,3,3,3,3,3,3,3,3,3,3,3,3,3,
3,3,3,3,3,3,3,3,3,3,3,3,3,3,3,3,4),(0.,0.0513261920791295,0.101891051484157,
0.125000000000127,0.178106823792157,0.187500000000194,0.218750000000228,
0.234375000000247,0.242187500000254,0.24609375000026,0.249264080962771,
0.250000000000267,0.312500000000385,0.375000000000502,0.437500000000617,
0.468750000000675,0.484375000000701,0.492187500000714,0.496093750000717,
0.498911066758421,0.500000000000721,0.548095655335943,0.598666505518088,
0.625000000000672,0.678884598604091,0.713546942576494,0.730878114562696,
0.739543700555797,0.743876493552347,0.746042890050623,0.74712608829976,
0.747667687424329,0.747967116726168,0.748168766823433,0.748209286548898,
0.750000000000624,0.79929200859889,0.850588465705387,0.903284387505033,
0.958942755428889,0.999999988259552),.UNSPECIFIED.);
#4798=B_SPLINE_CURVE_WITH_KNOTS('',3,(#155952,#155953,#155954,#155955,#155956,
#155957,#155958,#155959,#155960,#155961,#155962,#155963,#155964,#155965,
#155966,#155967),.UNSPECIFIED.,.F.,.F.,(4,3,3,3,3,4),(1.37805369294038E-6,
0.25000103354027,0.491490606329696,0.727506144562777,0.956522966635118,
1.),.UNSPECIFIED.);
#4799=B_SPLINE_CURVE_WITH_KNOTS('',3,(#155968,#155969,#155970,#155971,#155972,
#155973,#155974,#155975,#155976,#155977,#155978,#155979,#155980,#155981,
#155982,#155983,#155984,#155985,#155986,#155987,#155988,#155989,#155990,
#155991,#155992,#155993,#155994,#155995,#155996,#155997,#155998,#155999,
#156000,#156001,#156002,#156003,#156004,#156005,#156006,#156007,#156008,
#156009,#156010,#156011,#156012,#156013,#156014,#156015,#156016,#156017,
#156018,#156019,#156020,#156021,#156022,#156023,#156024,#156025,#156026,
#156027,#156028,#156029,#156030,#156031,#156032,#156033,#156034,#156035,
#156036,#156037,#156038,#156039,#156040,#156041,#156042,#156043,#156044,
#156045,#156046,#156047,#156048,#156049,#156050,#156051,#156052,#156053,
#156054,#156055,#156056,#156057,#156058,#156059,#156060,#156061,#156062,
#156063,#156064,#156065,#156066,#156067,#156068,#156069,#156070,#156071,
#156072,#156073,#156074,#156075,#156076,#156077,#156078,#156079,#156080,
#156081,#156082,#156083,#156084,#156085,#156086,#156087,#156088,#156089,
#156090,#156091,#156092,#156093,#156094,#156095,#156096,#156097,#156098,
#156099,#156100,#156101,#156102,#156103,#156104,#156105,#156106,#156107,
#156108,#156109,#156110,#156111,#156112,#156113,#156114,#156115,#156116,
#156117,#156118,#156119,#156120,#156121,#156122,#156123,#156124),
 .UNSPECIFIED.,.F.,.F.,(4,3,3,3,3,3,3,3,3,3,3,3,3,3,3,3,3,3,3,3,3,3,3,3,
3,3,3,3,3,3,3,3,3,3,3,3,3,3,3,3,3,3,3,3,3,3,3,3,3,3,3,3,4),(0.000325310152520073,
0.00195312500001419,0.00207519531251508,0.00230407714845424,0.00390625000002838,
0.00585937500004257,0.00683593750004902,0.00781250000005548,0.0156250000001289,
0.0285965136258737,0.0312500000002777,0.0468750000004264,0.0580811522582563,
0.0625000000005752,0.0937500000008728,0.109375000001022,0.117187500001095,
0.123820195931982,0.125000000001169,0.187500000001785,0.218750000002089,
0.234375000002238,0.242187500002309,0.246093750002341,0.250000000002374,
0.252616048242064,0.344815548524214,0.375000000003363,0.437500000003857,
0.468750000004101,0.484375000004223,0.492187500004284,0.496093750004315,
0.499023437504339,0.500000000004347,0.51082228289493,0.541375719978749,
0.56250000000385,0.593750000003602,0.625000000003353,0.656250000003104,
0.687500000002855,0.718750000002607,0.734375000002485,0.742187500002423,
0.746093750002393,0.748046875002378,0.750000000002362,0.804086151359939,
0.859205844316772,0.914912172240495,0.971483295233683,1.),.UNSPECIFIED.);
#4800=B_SPLINE_CURVE_WITH_KNOTS('',3,(#156148,#156149,#156150,#156151),
 .UNSPECIFIED.,.F.,.F.,(4,4),(0.,0.00425966609677044),.UNSPECIFIED.);
#4801=B_SPLINE_CURVE_WITH_KNOTS('',3,(#156154,#156155,#156156,#156157,#156158,
#156159,#156160,#156161,#156162,#156163,#156164,#156165,#156166,#156167,
#156168,#156169),.UNSPECIFIED.,.F.,.F.,(4,3,3,3,3,4),(0.,0.230186031233572,
0.466791142229912,0.707543496522388,0.954682760211977,1.),.UNSPECIFIED.);
#4802=B_SPLINE_CURVE_WITH_KNOTS('',3,(#156173,#156174,#156175,#156176,#156177,
#156178,#156179,#156180,#156181,#156182,#156183,#156184,#156185,#156186,
#156187,#156188),.UNSPECIFIED.,.F.,.F.,(4,3,3,3,3,4),(0.,0.236247566825257,
0.482337922300788,0.667935821043213,0.875614812669031,0.999999798365662),
 .UNSPECIFIED.);
#4803=B_SPLINE_CURVE_WITH_KNOTS('',3,(#156190,#156191,#156192,#156193,#156194,
#156195,#156196,#156197,#156198,#156199,#156200,#156201,#156202),
 .UNSPECIFIED.,.F.,.F.,(4,3,3,3,4),(0.,0.274763476845488,0.544290520349838,
0.806409249078579,1.),.UNSPECIFIED.);
#4804=B_SPLINE_CURVE_WITH_KNOTS('',3,(#156205,#156206,#156207,#156208),
 .UNSPECIFIED.,.F.,.F.,(4,4),(0.,0.00407596620376747),.UNSPECIFIED.);
#4805=B_SPLINE_CURVE_WITH_KNOTS('',3,(#156212,#156213,#156214,#156215,#156216,
#156217,#156218,#156219,#156220,#156221,#156222,#156223,#156224),
 .UNSPECIFIED.,.F.,.F.,(4,3,3,3,4),(0.,0.237145647143792,0.483293389898376,
0.74164604880973,0.999998707721084),.UNSPECIFIED.);
#4806=B_SPLINE_CURVE_WITH_KNOTS('',3,(#156226,#156227,#156228,#156229,#156230,
#156231,#156232,#156233,#156234,#156235),.UNSPECIFIED.,.F.,.F.,(4,3,3,4),
(0.,0.384739188680616,0.759105290249364,1.),.UNSPECIFIED.);
#4807=B_SPLINE_CURVE_WITH_KNOTS('',3,(#156279,#156280,#156281,#156282),
 .UNSPECIFIED.,.F.,.F.,(4,4),(0.00078229444191847,0.00926194220748866),
 .UNSPECIFIED.);
#4808=B_SPLINE_CURVE_WITH_KNOTS('',3,(#156284,#156285,#156286,#156287,#156288,
#156289,#156290,#156291,#156292,#156293,#156294,#156295,#156296,#156297,
#156298,#156299,#156300,#156301,#156302,#156303,#156304,#156305,#156306,
#156307,#156308,#156309,#156310,#156311,#156312,#156313,#156314,#156315,
#156316,#156317,#156318,#156319,#156320,#156321,#156322,#156323,#156324,
#156325,#156326,#156327,#156328,#156329,#156330,#156331,#156332,#156333,
#156334,#156335,#156336,#156337,#156338,#156339,#156340,#156341,#156342,
#156343,#156344,#156345,#156346,#156347,#156348,#156349,#156350,#156351,
#156352,#156353,#156354,#156355,#156356),.UNSPECIFIED.,.F.,.F.,(4,3,3,3,
3,3,3,3,3,3,3,3,3,3,3,3,3,3,3,3,3,3,3,3,4),(8.44091860321908E-14,0.0624999999999906,
0.124999999999897,0.187499999999841,0.218749999999817,0.234374999999809,
0.242187499999805,0.246093749999806,0.249999999999808,0.347890901443095,
0.37499999999986,0.469604033890482,0.496093749999897,0.499305817827702,
0.499999999999895,0.55402564985833,0.562499999999909,0.609374999999918,
0.667671420454354,0.723088971645676,0.749999999999948,0.825882492417378,
0.874999999999974,0.960462506686326,0.999999979523105),.UNSPECIFIED.);
#4809=B_SPLINE_CURVE_WITH_KNOTS('',3,(#156358,#156359,#156360,#156361,#156362,
#156363,#156364,#156365,#156366,#156367,#156368,#156369,#156370,#156371,
#156372,#156373,#156374,#156375,#156376),.UNSPECIFIED.,.F.,.F.,(4,3,3,3,
3,3,4),(1.9687011228103E-6,0.214511984278332,0.415074732621236,0.60922528181149,
0.804612640905745,0.985865888199921,1.),.UNSPECIFIED.);
#4810=B_SPLINE_CURVE_WITH_KNOTS('',3,(#156377,#156378,#156379,#156380,#156381,
#156382,#156383,#156384,#156385,#156386,#156387,#156388,#156389,#156390,
#156391,#156392,#156393,#156394,#156395,#156396,#156397,#156398,#156399,
#156400,#156401,#156402,#156403,#156404,#156405,#156406,#156407,#156408,
#156409,#156410,#156411,#156412,#156413,#156414,#156415,#156416,#156417,
#156418,#156419),.UNSPECIFIED.,.F.,.F.,(4,2,1,1,2,2,2,2,1,2,2,2,1,1,1,2,
2,2,2,1,1,1,2,2,2,4),(0.000601430764826355,0.00781249999997516,0.0117187499999639,
0.0136718749999563,0.0146484374999525,0.0156249999999487,0.0312499999999361,
0.0624999999999109,0.0937499999998857,0.109374999999876,0.124999999999867,
0.187499999999835,0.218749999999818,0.23437499999981,0.242187499999802,
0.246093749999798,0.249999999999794,0.374999999999919,0.437499999999986,
0.468750000000016,0.484375000000032,0.492187500000039,0.496093750000039,
0.500000000000038,0.750000000000019,1.),.UNSPECIFIED.);
#4811=B_SPLINE_CURVE_WITH_KNOTS('',3,(#156423,#156424,#156425,#156426),
 .UNSPECIFIED.,.F.,.F.,(4,4),(0.000716623500636008,0.00919276877023496),
 .UNSPECIFIED.);
#4812=B_SPLINE_CURVE_WITH_KNOTS('',3,(#156443,#156444,#156445,#156446,#156447,
#156448,#156449,#156450,#156451,#156452,#156453,#156454,#156455,#156456,
#156457,#156458,#156459,#156460,#156461),.UNSPECIFIED.,.F.,.F.,(4,3,3,3,
3,3,4),(0.,0.182234855225268,0.370330240564428,0.568260122897141,0.772901042897791,
0.988056605769259,0.999998030911719),.UNSPECIFIED.);
#4813=B_SPLINE_CURVE_WITH_KNOTS('',3,(#156462,#156463,#156464,#156465,#156466,
#156467,#156468,#156469,#156470,#156471,#156472,#156473,#156474,#156475,
#156476,#156477,#156478,#156479,#156480,#156481,#156482,#156483,#156484,
#156485,#156486,#156487,#156488,#156489,#156490,#156491,#156492,#156493,
#156494,#156495,#156496,#156497,#156498,#156499,#156500,#156501,#156502,
#156503,#156504,#156505,#156506,#156507,#156508,#156509,#156510,#156511,
#156512,#156513,#156514,#156515,#156516,#156517,#156518,#156519,#156520,
#156521,#156522,#156523,#156524,#156525,#156526,#156527,#156528,#156529,
#156530,#156531,#156532,#156533,#156534,#156535,#156536,#156537,#156538,
#156539,#156540,#156541,#156542,#156543,#156544,#156545,#156546,#156547,
#156548,#156549,#156550,#156551,#156552,#156553,#156554,#156555,#156556,
#156557,#156558,#156559,#156560,#156561,#156562,#156563,#156564,#156565,
#156566,#156567),.UNSPECIFIED.,.F.,.F.,(4,3,3,3,3,3,3,3,3,3,3,3,3,3,3,3,
3,3,3,3,3,3,3,3,3,3,3,3,3,3,3,3,3,3,3,4),(1.82991911842132E-8,0.0751759264972593,
0.124999999999493,0.187805693540276,0.246093749998999,0.249999999998986,
0.252178981767012,0.342801458928556,0.374999999998785,0.443052550002119,
0.498046874998592,0.499999999998585,0.503012031054894,0.54307955855884,
0.56249999999841,0.602710083228639,0.617187499998271,0.621093749998255,
0.624999999998238,0.650878840433193,0.677324037255935,0.687499999998016,
0.714364448746321,0.718749999997905,0.734374999997839,0.742187499997806,
0.746093749997789,0.748046874997766,0.74902343749777,0.749511718747773,
0.749999999997775,0.751100566896097,0.817288275153847,0.88330529692333,
0.94908639453054,1.),.UNSPECIFIED.);
#4814=B_SPLINE_CURVE_WITH_KNOTS('',3,(#156568,#156569,#156570,#156571,#156572,
#156573,#156574,#156575,#156576,#156577,#156578,#156579,#156580,#156581,
#156582,#156583,#156584,#156585,#156586,#156587,#156588,#156589,#156590,
#156591,#156592,#156593,#156594,#156595,#156596,#156597,#156598,#156599,
#156600,#156601,#156602,#156603,#156604,#156605,#156606,#156607,#156608,
#156609,#156610,#156611,#156612,#156613,#156614,#156615,#156616,#156617,
#156618,#156619,#156620,#156621,#156622,#156623,#156624,#156625,#156626,
#156627,#156628,#156629,#156630,#156631,#156632,#156633,#156634,#156635,
#156636,#156637,#156638,#156639,#156640,#156641,#156642,#156643,#156644,
#156645,#156646,#156647,#156648,#156649,#156650,#156651,#156652,#156653,
#156654,#156655),.UNSPECIFIED.,.F.,.F.,(4,3,3,3,3,3,3,3,3,3,3,3,3,3,3,3,
3,3,3,3,3,3,3,3,3,3,3,3,3,4),(0.,0.0706981254337144,0.134756746486677,0.19237837324321,
0.221189186621476,0.235594593310609,0.239195944982892,0.241896958737105,
0.242572531958201,0.249192599119759,0.249999999999742,0.335864630298422,
0.374999999999788,0.4062499999998,0.437499999999812,0.468749999999815,0.488648139108568,
0.499415549493787,0.499999999999818,0.562499999999833,0.675822191009255,
0.718749999999872,0.734374999999877,0.746329099519318,0.749999999999882,
0.833428133033808,0.874999999999941,0.906249999999956,0.953124999999978,
0.999960672072946),.UNSPECIFIED.);
#4815=B_SPLINE_CURVE_WITH_KNOTS('',3,(#156660,#156661,#156662,#156663,#156664,
#156665,#156666,#156667,#156668,#156669,#156670,#156671,#156672),
 .UNSPECIFIED.,.F.,.F.,(4,3,3,3,4),(0.,0.275945685186237,0.556684630972288,
0.845469782669404,1.),.UNSPECIFIED.);
#4816=B_SPLINE_CURVE_WITH_KNOTS('',3,(#156673,#156674,#156675,#156676,#156677,
#156678,#156679,#156680,#156681,#156682,#156683,#156684,#156685,#156686,
#156687,#156688),.UNSPECIFIED.,.F.,.F.,(4,3,3,3,3,4),(0.,0.210999634175483,
0.413457389674863,0.611835729512844,0.805917864756422,1.),.UNSPECIFIED.);
#4817=B_SPLINE_CURVE_WITH_KNOTS('',3,(#156719,#156720,#156721,#156722,#156723,
#156724,#156725,#156726,#156727,#156728,#156729,#156730,#156731,#156732,
#156733,#156734,#156735,#156736,#156737,#156738,#156739,#156740,#156741,
#156742,#156743,#156744,#156745,#156746,#156747,#156748,#156749,#156750,
#156751,#156752,#156753,#156754,#156755,#156756,#156757,#156758,#156759,
#156760,#156761,#156762,#156763,#156764,#156765,#156766,#156767,#156768,
#156769,#156770,#156771,#156772,#156773,#156774,#156775,#156776,#156777,
#156778,#156779,#156780,#156781,#156782,#156783,#156784,#156785),
 .UNSPECIFIED.,.F.,.F.,(4,3,3,3,3,3,3,3,3,3,3,3,3,3,3,3,3,3,3,3,3,3,4),
(0.,0.100713214097213,0.199722071073913,0.296192282820578,0.375000000000224,
0.437500000000288,0.468750000000316,0.48437500000034,0.494481346924202,
0.500000000000365,0.581133205728252,0.625000000000431,0.687500000000466,
0.718750000000492,0.7343750000005,0.742187500000495,0.748154667016358,0.750000000000489,
0.803589729788625,0.855998067274474,0.907448277355546,0.957078195684321,
1.),.UNSPECIFIED.);
#4818=B_SPLINE_CURVE_WITH_KNOTS('',3,(#156799,#156800,#156801,#156802,#156803,
#156804,#156805,#156806,#156807,#156808,#156809,#156810,#156811,#156812,
#156813,#156814,#156815,#156816,#156817,#156818,#156819,#156820,#156821,
#156822,#156823,#156824,#156825,#156826,#156827,#156828,#156829,#156830,
#156831,#156832,#156833,#156834,#156835,#156836,#156837,#156838,#156839,
#156840,#156841,#156842,#156843,#156844,#156845,#156846,#156847,#156848,
#156849,#156850),.UNSPECIFIED.,.F.,.F.,(4,3,3,3,3,3,3,3,3,3,3,3,3,3,3,3,
3,4),(0.,0.0915574244606729,0.18774925655722,0.264441926099368,0.370387398191383,
0.423360134237391,0.449846502260395,0.463946416685409,0.46859215699834,
0.471131668249386,0.476332870283398,0.493787055659413,0.500000000000326,
0.605248837029928,0.712774761887522,0.821859923323834,0.933891888691301,
0.999999999999318),.UNSPECIFIED.);
#4819=B_SPLINE_CURVE_WITH_KNOTS('',3,(#156865,#156866,#156867,#156868,#156869,
#156870,#156871,#156872,#156873,#156874,#156875,#156876,#156877,#156878,
#156879,#156880,#156881,#156882,#156883,#156884,#156885,#156886,#156887,
#156888,#156889,#156890,#156891,#156892,#156893,#156894,#156895,#156896,
#156897,#156898,#156899,#156900,#156901,#156902,#156903,#156904,#156905,
#156906,#156907,#156908,#156909,#156910,#156911,#156912,#156913,#156914,
#156915,#156916,#156917,#156918,#156919,#156920,#156921,#156922,#156923,
#156924,#156925,#156926,#156927,#156928,#156929,#156930,#156931,#156932,
#156933,#156934,#156935,#156936,#156937,#156938,#156939,#156940,#156941,
#156942,#156943,#156944,#156945,#156946,#156947,#156948,#156949,#156950,
#156951,#156952,#156953,#156954,#156955),.UNSPECIFIED.,.F.,.F.,(4,3,3,3,
3,3,3,3,3,3,3,3,3,3,3,3,3,3,3,3,3,3,3,3,3,3,3,3,3,3,4),(0.,0.0665803261300661,
0.124999999999229,0.185546874998862,0.241891523992033,0.246093749998496,
0.24999999999848,0.252377916984439,0.374999999997735,0.441988271863787,
0.498046874997,0.49999999999699,0.503010835744694,0.549750791226953,0.562499999997204,
0.593749999997324,0.609374999997384,0.617187499997414,0.621093749997429,
0.624999999997444,0.687499999997845,0.718749999998051,0.734374999998155,
0.742187499998214,0.746093749998243,0.749999999998272,0.751172933773213,
0.822437083828853,0.874999999999136,0.945792987000676,1.),.UNSPECIFIED.);
#4820=B_SPLINE_CURVE_WITH_KNOTS('',3,(#156957,#156958,#156959,#156960),
 .UNSPECIFIED.,.F.,.F.,(4,4),(0.000801783579032724,0.0101814026529808),
 .UNSPECIFIED.);
#4821=B_SPLINE_CURVE_WITH_KNOTS('',3,(#156961,#156962,#156963,#156964,#156965,
#156966,#156967,#156968,#156969,#156970,#156971,#156972,#156973,#156974,
#156975,#156976,#156977,#156978,#156979,#156980,#156981,#156982,#156983,
#156984,#156985,#156986,#156987,#156988,#156989,#156990,#156991,#156992,
#156993,#156994,#156995,#156996,#156997,#156998,#156999,#157000,#157001,
#157002,#157003,#157004,#157005,#157006,#157007,#157008,#157009,#157010,
#157011,#157012,#157013,#157014,#157015,#157016,#157017,#157018,#157019,
#157020,#157021,#157022,#157023,#157024,#157025,#157026,#157027,#157028,
#157029,#157030,#157031,#157032,#157033,#157034,#157035,#157036,#157037,
#157038,#157039,#157040,#157041,#157042,#157043,#157044,#157045,#157046,
#157047,#157048,#157049,#157050,#157051,#157052,#157053,#157054,#157055,
#157056,#157057,#157058,#157059,#157060,#157061,#157062,#157063,#157064,
#157065,#157066,#157067,#157068,#157069,#157070,#157071,#157072,#157073,
#157074,#157075,#157076,#157077,#157078,#157079,#157080,#157081,#157082,
#157083,#157084,#157085,#157086,#157087),.UNSPECIFIED.,.F.,.F.,(4,3,3,3,
3,3,3,3,3,3,3,3,3,3,3,3,3,3,3,3,3,3,3,3,3,3,3,3,3,3,3,3,3,3,3,3,3,3,3,3,
3,3,4),(0.,0.0575336852850224,0.11198525032856,0.167849108085092,0.208924554042927,
0.229462277021845,0.239731138511304,0.244865569256033,0.247432784628398,
0.247753686549944,0.247945857259859,0.248138049254024,0.250000000000763,
0.282925510948109,0.315143228875522,0.346441281795087,0.375000000001455,
0.406250000001632,0.437500000001809,0.468750000001998,0.484375000002073,
0.492187500002108,0.4950791904349,0.496093750002159,0.498046875002222,0.499023437502213,
0.499511718752208,0.500000000002203,0.548747958738085,0.599908063232395,
0.625000000001634,0.680103968548825,0.687500000001349,0.718750000001199,
0.734375000001116,0.742187500001066,0.746093750001048,0.749103884050622,
0.75000000000103,0.812492512889779,0.875564869958435,0.943003068446462,
0.999970051556025),.UNSPECIFIED.);
#4822=B_SPLINE_CURVE_WITH_KNOTS('',3,(#157092,#157093,#157094,#157095),
 .UNSPECIFIED.,.F.,.F.,(4,4),(0.000856775130582955,0.0102382230284107),
 .UNSPECIFIED.);
#4823=B_SPLINE_CURVE_WITH_KNOTS('',3,(#157123,#157124,#157125,#157126,#157127,
#157128,#157129,#157130,#157131,#157132),.UNSPECIFIED.,.F.,.F.,(4,3,3,4),
(0.,0.384406684848453,0.779039496016362,1.),.UNSPECIFIED.);
#4824=B_SPLINE_CURVE_WITH_KNOTS('',3,(#157133,#157134,#157135,#157136,#157137,
#157138,#157139,#157140,#157141,#157142,#157143,#157144,#157145),
 .UNSPECIFIED.,.F.,.F.,(4,3,3,3,4),(1.27819991133542E-6,0.264022670170208,
0.521486442313197,0.769264763105439,1.),.UNSPECIFIED.);
#4825=B_SPLINE_CURVE_WITH_KNOTS('',3,(#157159,#157160,#157161,#157162,#157163,
#157164,#157165,#157166,#157167,#157168,#157169,#157170,#157171,#157172,
#157173,#157174,#157175,#157176,#157177,#157178,#157179,#157180,#157181,
#157182,#157183,#157184,#157185,#157186,#157187,#157188,#157189,#157190,
#157191,#157192,#157193,#157194,#157195,#157196,#157197,#157198,#157199,
#157200,#157201,#157202,#157203,#157204,#157205,#157206,#157207,#157208,
#157209,#157210,#157211,#157212,#157213,#157214,#157215,#157216,#157217,
#157218,#157219,#157220,#157221,#157222,#157223,#157224,#157225,#157226,
#157227,#157228,#157229,#157230,#157231,#157232,#157233,#157234,#157235,
#157236,#157237,#157238,#157239,#157240,#157241,#157242,#157243,#157244,
#157245,#157246,#157247,#157248,#157249,#157250,#157251,#157252,#157253,
#157254,#157255,#157256,#157257,#157258,#157259,#157260,#157261,#157262,
#157263,#157264,#157265,#157266,#157267,#157268,#157269,#157270,#157271,
#157272,#157273,#157274,#157275,#157276),.UNSPECIFIED.,.F.,.F.,(4,3,3,3,
3,3,3,3,3,3,3,3,3,3,3,3,3,3,3,3,3,3,3,3,3,3,3,3,3,3,3,3,3,3,3,3,3,3,3,4),
(0.,0.0590683228806878,0.116947001900935,0.12500000000061,0.187500000000918,
0.218750000001069,0.234375000001147,0.242187500001189,0.246093750001211,
0.249023437501223,0.250000000001225,0.28125000000129,0.311332831951185,
0.341061141711148,0.370364786792094,0.375000000001484,0.403715310671607,
0.432254350266244,0.460813536183436,0.487361700983429,0.496093750001687,
0.49804687500169,0.499023437501685,0.499511718751682,0.500000000001679,
0.552231180312084,0.60711677393185,0.625000000001268,0.683312841681498,
0.687500000001066,0.718750000000961,0.734375000000912,0.742187500000887,
0.746093750000875,0.74924093922361,0.750000000000863,0.814480974141558,
0.880798950734992,0.951107468086681,1.),.UNSPECIFIED.);
#4826=B_SPLINE_CURVE_WITH_KNOTS('',3,(#157277,#157278,#157279,#157280),
 .UNSPECIFIED.,.F.,.F.,(4,4),(0.000932565055856382,0.00145387661961335),
 .UNSPECIFIED.);
#4827=B_SPLINE_CURVE_WITH_KNOTS('',3,(#157281,#157282,#157283,#157284,#157285,
#157286,#157287,#157288,#157289,#157290,#157291,#157292,#157293,#157294,
#157295,#157296,#157297,#157298,#157299,#157300,#157301,#157302,#157303,
#157304,#157305,#157306,#157307,#157308,#157309,#157310,#157311,#157312,
#157313,#157314,#157315,#157316,#157317,#157318,#157319,#157320,#157321,
#157322,#157323,#157324,#157325,#157326,#157327,#157328,#157329,#157330,
#157331,#157332,#157333,#157334,#157335,#157336,#157337,#157338,#157339,
#157340),.UNSPECIFIED.,.F.,.F.,(4,2,1,2,2,2,2,2,2,1,1,2,2,2,1,1,1,2,2,2,
2,1,1,1,1,2,2,2,2,2,1,1,1,1,2,2,4),(0.000325542589491421,0.00390625000006981,
0.00585937500010367,0.00683593750012059,0.00781250000013752,0.0156250000002675,
0.0312500000005256,0.0468750000007837,0.0625000000010418,0.0937500000015648,
0.109375000001826,0.117187500001961,0.125000000002096,0.187500000003154,
0.218750000003686,0.234375000003956,0.242187500004087,0.24609375000415,
0.250000000004212,0.375000000006297,0.437500000007336,0.468750000007856,
0.484375000008115,0.492187500008246,0.496093750008311,0.49902343750836,
0.500000000008378,0.625000000006009,0.687500000004824,0.718750000004232,
0.734375000003934,0.742187500003785,0.746093750003708,0.748046875003672,
0.749023437503654,0.750000000003636,1.),.UNSPECIFIED.);
#4828=B_SPLINE_CURVE_WITH_KNOTS('',3,(#157359,#157360,#157361,#157362,#157363,
#157364,#157365,#157366,#157367,#157368,#157369,#157370,#157371,#157372,
#157373,#157374,#157375,#157376,#157377),.UNSPECIFIED.,.F.,.F.,(4,3,3,3,
3,3,4),(0.000633514536432522,0.00221236722518767,0.0038475939806142,0.0055851368810824,
0.00588295359619696,0.00776048988122894,0.00821913918141333),
 .UNSPECIFIED.);
#4829=B_SPLINE_CURVE_WITH_KNOTS('',3,(#157381,#157382,#157383,#157384,#157385,
#157386,#157387,#157388,#157389,#157390,#157391,#157392,#157393,#157394,
#157395,#157396,#157397,#157398,#157399),.UNSPECIFIED.,.F.,.F.,(4,3,3,3,
3,3,4),(0.000708752105543503,0.00258350608964089,0.00304683603862555,0.00476166896126371,
0.00640184829314115,0.00796195121168144,0.00830118856937974),
 .UNSPECIFIED.);
#4830=B_SPLINE_CURVE_WITH_KNOTS('',3,(#157421,#157422,#157423,#157424,#157425,
#157426,#157427,#157428,#157429,#157430,#157431,#157432,#157433,#157434,
#157435,#157436),.UNSPECIFIED.,.F.,.F.,(4,3,3,3,3,4),(0.,0.191851125007783,
0.406480624881621,0.608561884440055,0.854526014883085,0.999999191020381),
 .UNSPECIFIED.);
#4831=B_SPLINE_CURVE_WITH_KNOTS('',3,(#157437,#157438,#157439,#157440,#157441,
#157442,#157443,#157444,#157445,#157446,#157447,#157448,#157449,#157450,
#157451,#157452,#157453,#157454,#157455,#157456,#157457,#157458,#157459,
#157460,#157461,#157462,#157463,#157464,#157465,#157466,#157467,#157468,
#157469,#157470,#157471,#157472,#157473,#157474,#157475,#157476,#157477),
 .UNSPECIFIED.,.F.,.F.,(4,2,2,1,1,1,2,2,2,2,1,1,1,1,2,2,2,2,2,1,1,1,1,2,
2,4),(1.37021161665357E-8,0.125000000001154,0.187500000001739,0.218750000002024,
0.234375000002165,0.242187500002236,0.246093750002262,0.250000000002289,
0.375000000003502,0.437500000004118,0.468750000004426,0.48437500000458,
0.492187500004649,0.496093750004684,0.498046875004701,0.500000000004718,
0.62500000000551,0.687500000005905,0.718750000006103,0.734375000006183,
0.742187500006222,0.746093750006241,0.748046875006277,0.749023437506266,
0.750000000006256,1.),.UNSPECIFIED.);
#4832=B_SPLINE_CURVE_WITH_KNOTS('',3,(#157478,#157479,#157480,#157481,#157482,
#157483,#157484,#157485,#157486,#157487,#157488,#157489,#157490,#157491,
#157492,#157493,#157494,#157495,#157496,#157497,#157498,#157499,#157500,
#157501,#157502,#157503,#157504,#157505,#157506,#157507,#157508,#157509,
#157510,#157511,#157512,#157513,#157514,#157515,#157516,#157517,#157518,
#157519,#157520,#157521,#157522,#157523,#157524,#157525,#157526,#157527,
#157528,#157529,#157530,#157531,#157532,#157533,#157534,#157535,#157536,
#157537,#157538,#157539,#157540,#157541,#157542,#157543,#157544,#157545,
#157546,#157547,#157548,#157549,#157550,#157551,#157552,#157553,#157554,
#157555,#157556,#157557,#157558,#157559,#157560,#157561,#157562,#157563,
#157564,#157565,#157566,#157567,#157568),.UNSPECIFIED.,.F.,.F.,(4,3,3,3,
3,3,3,3,3,3,3,3,3,3,3,3,3,3,3,3,3,3,3,3,3,3,3,3,3,3,4),(0.,0.0942187049135352,
0.172109352457099,0.211054676228881,0.230527338114772,0.240263669057718,
0.245131834529191,0.24584290831596,0.246288773375984,0.250000000000663,
0.310546875000763,0.368000688459125,0.430094094230093,0.49218750000106,
0.499784370190774,0.500000000001073,0.547046753073244,0.595404792786901,
0.62500000000146,0.674219419647568,0.687500000001642,0.718750000001735,
0.734375000001779,0.742187500001802,0.746093750001812,0.748046875001799,
0.750000000001786,0.824413102467963,0.901016120596062,0.980588302632023,
0.999982499870738),.UNSPECIFIED.);
#4833=B_SPLINE_CURVE_WITH_KNOTS('',3,(#157573,#157574,#157575,#157576,#157577,
#157578,#157579,#157580,#157581,#157582,#157583,#157584,#157585,#157586,
#157587,#157588,#157589,#157590,#157591,#157592,#157593,#157594,#157595,
#157596,#157597,#157598,#157599,#157600,#157601,#157602,#157603,#157604,
#157605,#157606,#157607,#157608,#157609,#157610,#157611,#157612),
 .UNSPECIFIED.,.F.,.F.,(4,3,3,3,3,3,3,3,3,3,3,3,3,4),(0.,0.152110083047855,
0.249999999999927,0.37499999999989,0.437499999999873,0.468749999999866,
0.484374999999861,0.499023437499852,0.49999999999985,0.500032662678491,
0.628278229772928,0.75903464790435,0.894326952680693,1.),.UNSPECIFIED.);
#4834=B_SPLINE_CURVE_WITH_KNOTS('',3,(#157613,#157614,#157615,#157616,#157617,
#157618,#157619,#157620,#157621,#157622,#157623,#157624,#157625,#157626,
#157627,#157628,#157629,#157630,#157631,#157632,#157633,#157634,#157635,
#157636,#157637,#157638,#157639,#157640,#157641,#157642,#157643),
 .UNSPECIFIED.,.F.,.F.,(4,3,3,3,3,3,3,3,3,3,4),(0.,0.13024412390066,0.256700429361413,
0.378760361967859,0.499023437500028,0.49997472214385,0.500000000000029,
0.659213532399644,0.814240717125258,0.964146097215223,1.),.UNSPECIFIED.);
#4835=B_SPLINE_CURVE_WITH_KNOTS('',3,(#157668,#157669,#157670,#157671,#157672,
#157673,#157674,#157675,#157676,#157677,#157678,#157679,#157680,#157681,
#157682,#157683,#157684,#157685,#157686,#157687,#157688,#157689,#157690,
#157691,#157692,#157693,#157694,#157695,#157696,#157697,#157698),
 .UNSPECIFIED.,.F.,.F.,(4,3,3,3,3,3,3,3,3,3,4),(0.,0.163914497973559,0.250000000000003,
0.312500000000004,0.347315553940031,0.375000000000005,0.500000000000005,
0.632160630087504,0.76037903141579,0.882749786044512,1.),.UNSPECIFIED.);
#4836=B_SPLINE_CURVE_WITH_KNOTS('',3,(#157702,#157703,#157704,#157705,#157706,
#157707,#157708,#157709,#157710,#157711,#157712,#157713,#157714,#157715,
#157716,#157717,#157718,#157719,#157720),.UNSPECIFIED.,.F.,.F.,(4,3,3,3,
3,3,4),(0.000609719129519901,0.00229610816233235,0.00296440479617455,0.00386266882834386,
0.00506716034621368,0.00622435639369075,0.00711561852716782),
 .UNSPECIFIED.);
#4837=B_SPLINE_CURVE_WITH_KNOTS('',3,(#157724,#157725,#157726,#157727,#157728,
#157729,#157730,#157731,#157732,#157733,#157734,#157735,#157736,#157737,
#157738,#157739,#157740,#157741,#157742),.UNSPECIFIED.,.F.,.F.,(4,3,3,3,
3,3,4),(0.000543628862815408,0.00167393673136745,0.00258252559983906,0.00379688806421983,
0.00467674795200451,0.0060164798674652,0.00704595220449218),
 .UNSPECIFIED.);
#4838=B_SPLINE_CURVE_WITH_KNOTS('',3,(#157770,#157771,#157772,#157773,#157774,
#157775,#157776,#157777,#157778,#157779,#157780,#157781,#157782,#157783,
#157784,#157785,#157786,#157787,#157788,#157789,#157790,#157791),
 .UNSPECIFIED.,.F.,.F.,(4,3,3,3,3,3,3,4),(0.,0.209978546231012,0.516853342342681,
0.55334059960295,0.677766711290302,0.809718518620088,0.850799142123614,
0.999999957313844),.UNSPECIFIED.);
#4839=B_SPLINE_CURVE_WITH_KNOTS('',3,(#157792,#157793,#157794,#157795,#157796,
#157797,#157798,#157799,#157800,#157801,#157802,#157803,#157804,#157805,
#157806,#157807,#157808,#157809,#157810,#157811,#157812,#157813,#157814,
#157815,#157816,#157817,#157818,#157819,#157820,#157821,#157822,#157823,
#157824,#157825,#157826,#157827,#157828,#157829,#157830,#157831,#157832,
#157833,#157834,#157835,#157836,#157837,#157838,#157839,#157840,#157841,
#157842,#157843,#157844,#157845,#157846,#157847,#157848,#157849,#157850,
#157851,#157852,#157853,#157854,#157855,#157856,#157857,#157858,#157859,
#157860,#157861,#157862,#157863,#157864,#157865,#157866,#157867,#157868,
#157869,#157870),.UNSPECIFIED.,.F.,.F.,(4,3,3,3,3,3,3,3,3,3,3,3,3,3,3,3,
3,3,3,3,3,3,3,3,3,3,4),(2.68021967053581E-8,0.0901737464676206,0.125000000004943,
0.187500000007436,0.218750000008682,0.234375000009306,0.242187500009617,
0.246093750009773,0.248046875009851,0.250000000009929,0.284837518478703,
0.319813158669615,0.354999270488202,0.388272574435471,0.424332270935315,
0.461189572970983,0.49804687500665,0.500000000006616,0.500285687694454,
0.569196019485871,0.625000000004962,0.700368074597989,0.750000000003308,
0.828257149063034,0.908768627880029,0.992262118086699,1.),.UNSPECIFIED.);
#4840=B_SPLINE_CURVE_WITH_KNOTS('',3,(#157871,#157872,#157873,#157874,#157875,
#157876,#157877,#157878,#157879,#157880,#157881,#157882,#157883,#157884,
#157885,#157886,#157887,#157888,#157889,#157890,#157891,#157892,#157893,
#157894,#157895,#157896,#157897,#157898,#157899,#157900,#157901,#157902,
#157903,#157904,#157905,#157906,#157907,#157908,#157909,#157910,#157911,
#157912,#157913,#157914,#157915,#157916,#157917,#157918,#157919,#157920,
#157921,#157922,#157923,#157924,#157925,#157926,#157927,#157928,#157929,
#157930,#157931,#157932,#157933,#157934),.UNSPECIFIED.,.F.,.F.,(4,3,3,3,
3,3,3,3,3,3,3,3,3,3,3,3,3,3,3,3,3,4),(0.,0.118271603684389,0.213215421513922,
0.276599705427053,0.378014263819111,0.476502100417059,0.498046875002522,
0.500000000002524,0.500226658109365,0.543785052858866,0.587308456982946,
0.625000000001855,0.668197289819432,0.71031813419112,0.734375000001243,
0.742187500001194,0.74609375000118,0.750000000001165,0.815058929541337,
0.88140492073318,0.94923986208531,0.999998612059214),.UNSPECIFIED.);
#4841=B_SPLINE_CURVE_WITH_KNOTS('',3,(#157939,#157940,#157941,#157942,#157943,
#157944,#157945,#157946,#157947,#157948,#157949,#157950,#157951,#157952,
#157953,#157954,#157955,#157956,#157957,#157958,#157959,#157960,#157961,
#157962,#157963,#157964,#157965,#157966,#157967,#157968,#157969,#157970,
#157971,#157972,#157973,#157974,#157975,#157976,#157977,#157978,#157979,
#157980,#157981),.UNSPECIFIED.,.F.,.F.,(4,3,3,3,3,3,3,3,3,3,3,3,3,3,4),
(0.,0.152629020565605,0.249999999999822,0.374999999999733,0.43749999999969,
0.468749999999669,0.484374999999659,0.492187499999655,0.49902343749965,
0.499999999999649,0.500016866394184,0.625012649795638,0.752170083217449,
0.885031771841597,1.),.UNSPECIFIED.);
#4842=B_SPLINE_CURVE_WITH_KNOTS('',3,(#157982,#157983,#157984,#157985,#157986,
#157987,#157988,#157989,#157990,#157991,#157992,#157993,#157994,#157995,
#157996,#157997),.UNSPECIFIED.,.F.,.F.,(4,2,2,1,1,1,1,2,2,4),(0.,0.249999999999634,
0.374999999999451,0.43749999999936,0.468749999999314,0.484374999999291,
0.49218749999928,0.499511718749273,0.499999999999273,1.),.UNSPECIFIED.);
#4843=B_SPLINE_CURVE_WITH_KNOTS('',3,(#158012,#158013,#158014,#158015,#158016,
#158017,#158018,#158019,#158020,#158021,#158022,#158023,#158024,#158025,
#158026,#158027,#158028,#158029,#158030,#158031,#158032,#158033,#158034,
#158035,#158036,#158037,#158038,#158039,#158040,#158041,#158042,#158043,
#158044,#158045,#158046,#158047,#158048,#158049,#158050,#158051,#158052,
#158053,#158054,#158055,#158056,#158057,#158058,#158059,#158060,#158061,
#158062,#158063,#158064,#158065,#158066,#158067,#158068,#158069,#158070,
#158071,#158072,#158073,#158074,#158075,#158076,#158077,#158078,#158079,
#158080,#158081,#158082,#158083,#158084,#158085,#158086,#158087,#158088,
#158089,#158090,#158091,#158092,#158093,#158094,#158095,#158096,#158097,
#158098,#158099,#158100,#158101,#158102,#158103,#158104,#158105,#158106,
#158107,#158108,#158109,#158110,#158111,#158112,#158113,#158114,#158115,
#158116,#158117,#158118,#158119,#158120,#158121,#158122,#158123),
 .UNSPECIFIED.,.F.,.F.,(4,3,3,3,3,3,3,3,3,3,3,3,3,3,3,3,3,3,3,3,3,3,3,3,
3,3,3,3,3,3,3,3,3,3,3,3,3,4),(0.,0.0312499999998062,0.0605342632990558,
0.0894827504846968,0.118001403536209,0.124999999999225,0.153278974298353,
0.18129948503294,0.187499999998837,0.216951734368515,0.218749999998643,
0.234374999998554,0.242187499998502,0.246093749998477,0.248046874998471,
0.249999999998465,0.251315421686666,0.287025254902491,0.323897744396542,
0.362533590707892,0.365329311803758,0.374999999998303,0.435546874998244,
0.486640465010263,0.496093749998184,0.499801280154157,0.499999999998196,
0.502837829566728,0.557028783578141,0.612188173491773,0.618785031193608,
0.707396936947145,0.740020308462563,0.749999999999098,0.808109157563208,
0.868876091672364,0.934438045836177,0.999999999999991),.UNSPECIFIED.);
#4844=B_SPLINE_CURVE_WITH_KNOTS('',3,(#158127,#158128,#158129,#158130,#158131,
#158132,#158133,#158134,#158135,#158136,#158137,#158138,#158139,#158140,
#158141,#158142,#158143,#158144,#158145,#158146,#158147,#158148,#158149,
#158150,#158151,#158152,#158153,#158154,#158155,#158156,#158157,#158158,
#158159,#158160,#158161,#158162,#158163,#158164,#158165,#158166,#158167,
#158168,#158169,#158170,#158171,#158172,#158173,#158174,#158175,#158176,
#158177,#158178,#158179,#158180,#158181,#158182,#158183,#158184,#158185,
#158186,#158187,#158188,#158189,#158190,#158191,#158192,#158193,#158194,
#158195,#158196,#158197,#158198,#158199,#158200,#158201,#158202,#158203,
#158204,#158205,#158206,#158207,#158208,#158209,#158210,#158211,#158212,
#158213,#158214,#158215,#158216,#158217,#158218,#158219,#158220,#158221,
#158222,#158223,#158224,#158225,#158226),.UNSPECIFIED.,.F.,.F.,(4,3,3,3,
3,3,3,3,3,3,3,3,3,3,3,3,3,3,3,3,3,3,3,3,3,3,3,3,3,3,3,3,3,4),(0.,0.0648910438044147,
0.128717958621191,0.191025514880074,0.250000000000982,0.31045583673544,
0.370223161889096,0.429183251024718,0.437500000001725,0.46875000000185,
0.484375000001905,0.492187500001924,0.496093750001933,0.499608596766509,
0.500000000001942,0.547658410706032,0.594339973290379,0.640919986645954,
0.687500000001529,0.718750000001471,0.734375000001432,0.742187500001413,
0.746093750001393,0.748046875001384,0.750000000001374,0.775181875051039,
0.801125965610821,0.828252261465758,0.856100708458129,0.884636130316055,
0.91411422298605,0.944011866396523,0.974420019927077,1.),.UNSPECIFIED.);
#4845=B_SPLINE_CURVE_WITH_KNOTS('',3,(#158227,#158228,#158229,#158230),
 .UNSPECIFIED.,.F.,.F.,(4,4),(0.0209654295165786,0.0214659702660322),
 .UNSPECIFIED.);
#4846=B_SPLINE_CURVE_WITH_KNOTS('',3,(#158234,#158235,#158236,#158237,#158238,
#158239,#158240,#158241,#158242,#158243,#158244,#158245,#158246,#158247,
#158248,#158249,#158250,#158251,#158252),.UNSPECIFIED.,.F.,.F.,(4,3,3,3,
3,3,4),(0.000498894531959924,0.00225071250488168,0.00337891514771613,0.00374149706694668,
0.00465083407571407,0.00559677886661334,0.00625893576407251),
 .UNSPECIFIED.);
#4847=B_SPLINE_CURVE_WITH_KNOTS('',3,(#158256,#158257,#158258,#158259,#158260,
#158261,#158262,#158263,#158264,#158265,#158266,#158267,#158268,#158269,
#158270,#158271,#158272,#158273,#158274,#158275,#158276,#158277,#158278,
#158279,#158280),.UNSPECIFIED.,.F.,.F.,(4,3,3,3,3,3,3,3,4),(0.000526414844798677,
0.00162646262698099,0.00270005642797546,0.00303445478718795,0.00340650091711803,
0.00424257270328492,0.00468441200509802,0.00552307032315888,0.0062865869894374),
 .UNSPECIFIED.);
#4848=B_SPLINE_CURVE_WITH_KNOTS('',3,(#158302,#158303,#158304,#158305,#158306,
#158307,#158308,#158309,#158310,#158311,#158312,#158313,#158314,#158315,
#158316,#158317,#158318,#158319,#158320,#158321,#158322,#158323,#158324,
#158325,#158326),.UNSPECIFIED.,.F.,.F.,(4,3,3,3,3,3,3,3,4),(7.55472550129836E-12,
0.249999999999995,0.374999999999993,0.437499999999994,0.468749999999996,
0.484374999999998,0.499999999999999,0.75,1.),.UNSPECIFIED.);
#4849=B_SPLINE_CURVE_WITH_KNOTS('',3,(#158327,#158328,#158329,#158330,#158331,
#158332,#158333,#158334,#158335,#158336,#158337,#158338,#158339,#158340,
#158341,#158342,#158343,#158344,#158345,#158346,#158347,#158348,#158349,
#158350,#158351,#158352,#158353,#158354,#158355,#158356,#158357,#158358,
#158359,#158360,#158361,#158362,#158363,#158364,#158365,#158366,#158367,
#158368,#158369,#158370,#158371,#158372,#158373,#158374,#158375,#158376,
#158377,#158378,#158379,#158380,#158381,#158382,#158383,#158384,#158385,
#158386,#158387,#158388,#158389,#158390),.UNSPECIFIED.,.F.,.F.,(4,3,3,3,
3,3,3,3,3,3,3,3,3,3,3,3,3,3,3,3,3,4),(0.,0.062499999999913,0.121268938782561,
0.124999999999826,0.182866167131341,0.187499999999739,0.221010185130871,
0.249999999999652,0.30930397539579,0.369343026326928,0.430208840841633,
0.437499999999391,0.468749999999367,0.484374999999355,0.492187499999348,
0.49609374999937,0.499999999999391,0.599290847525026,0.701894875544265,
0.806426977227526,0.914331950747426,1.),.UNSPECIFIED.);
#4850=B_SPLINE_CURVE_WITH_KNOTS('',3,(#158396,#158397,#158398,#158399,#158400,
#158401,#158402,#158403,#158404,#158405,#158406,#158407,#158408,#158409,
#158410),.UNSPECIFIED.,.F.,.F.,(4,2,2,1,1,1,2,2,4),(0.,0.250000000000126,
0.375000000000189,0.437500000000219,0.468750000000235,0.484375000000243,
0.499511718750253,0.500000000000252,1.),.UNSPECIFIED.);
#4851=B_SPLINE_CURVE_WITH_KNOTS('',3,(#158411,#158412,#158413,#158414,#158415,
#158416,#158417,#158418,#158419,#158420),.UNSPECIFIED.,.F.,.F.,(4,3,3,4),
(1.28225413371019E-15,0.448593385958983,0.838218300237572,1.),
 .UNSPECIFIED.);
#4852=B_SPLINE_CURVE_WITH_KNOTS('',3,(#158435,#158436,#158437,#158438,#158439,
#158440,#158441,#158442,#158443,#158444,#158445,#158446,#158447,#158448,
#158449,#158450,#158451,#158452,#158453,#158454,#158455,#158456,#158457,
#158458,#158459,#158460,#158461,#158462,#158463,#158464,#158465,#158466,
#158467,#158468,#158469,#158470,#158471,#158472,#158473,#158474,#158475,
#158476,#158477,#158478,#158479,#158480,#158481,#158482,#158483,#158484,
#158485,#158486,#158487,#158488,#158489,#158490,#158491,#158492,#158493,
#158494,#158495),.UNSPECIFIED.,.F.,.F.,(4,3,3,3,3,3,3,3,3,3,3,3,3,3,3,3,
3,3,3,3,4),(0.,0.0502633235240096,0.101045843377086,0.152970535449028,0.189102546852238,
0.238178111545533,0.25,0.304377708692877,0.358316326919491,0.399399448923178,
0.459255053387673,0.5,0.560867125063224,0.62437046877712,0.652851120149406,
0.729686322421556,0.75,0.830074596814701,0.910059278387214,0.989928126244262,
1.),.UNSPECIFIED.);
#4853=B_SPLINE_CURVE_WITH_KNOTS('',3,(#158499,#158500,#158501,#158502,#158503,
#158504,#158505,#158506,#158507,#158508,#158509,#158510,#158511,#158512,
#158513,#158514,#158515,#158516,#158517,#158518,#158519,#158520,#158521,
#158522,#158523,#158524,#158525,#158526,#158527,#158528,#158529,#158530,
#158531,#158532,#158533,#158534,#158535,#158536,#158537,#158538),
 .UNSPECIFIED.,.F.,.F.,(4,3,3,3,3,3,3,3,3,3,3,3,3,4),(0.,0.0800261451261139,
0.159426517805461,0.238333591819812,0.316877881690732,0.395188406678548,
0.473451575133888,0.55177676839471,0.630277038124919,0.709065913000149,
0.788573007004716,0.868542366834391,0.949461691917387,1.),.UNSPECIFIED.);
#4854=B_SPLINE_CURVE_WITH_KNOTS('',3,(#158543,#158544,#158545,#158546,#158547,
#158548,#158549,#158550,#158551,#158552,#158553,#158554,#158555,#158556,
#158557,#158558,#158559,#158560,#158561,#158562,#158563,#158564,#158565,
#158566,#158567),.UNSPECIFIED.,.F.,.F.,(4,3,3,3,3,3,3,3,4),(0.000528035090325194,
0.0016124914159284,0.00267001151846031,0.00302714454343539,0.00341353154252654,
0.00423239659979752,0.00468651457632683,0.00549911074687931,0.0062990279947279),
 .UNSPECIFIED.);
#4855=B_SPLINE_CURVE_WITH_KNOTS('',3,(#158571,#158572,#158573,#158574,#158575,
#158576,#158577,#158578,#158579,#158580,#158581,#158582,#158583,#158584,
#158585,#158586,#158587,#158588,#158589,#158590,#158591,#158592),
 .UNSPECIFIED.,.F.,.F.,(4,3,3,3,3,3,3,4),(0.000499308730788174,0.00146046002320121,
0.00243695586829252,0.00338583705476887,0.00376364965220018,0.00474984309182762,
0.00578812738994436,0.00627236538267016),.UNSPECIFIED.);
#4856=B_SPLINE_CURVE_WITH_KNOTS('',3,(#158620,#158621,#158622,#158623,#158624,
#158625,#158626,#158627,#158628,#158629,#158630,#158631,#158632,#158633,
#158634,#158635,#158636,#158637,#158638,#158639,#158640,#158641,#158642,
#158643,#158644,#158645,#158646,#158647,#158648,#158649,#158650,#158651,
#158652,#158653,#158654,#158655,#158656,#158657,#158658,#158659,#158660,
#158661,#158662),.UNSPECIFIED.,.F.,.F.,(4,3,3,3,3,3,3,3,3,3,3,3,3,3,4),
(0.,0.101173413162297,0.202391851056343,0.23209554217457,0.334240321391055,
0.431696971553665,0.49004936393671,0.499999999999992,0.562499999999993,
0.59262152003138,0.618082675029418,0.622918819150938,0.627640870459847,
0.845903088419632,1.),.UNSPECIFIED.);
#4857=B_SPLINE_CURVE_WITH_KNOTS('',3,(#158664,#158665,#158666,#158667,#158668,
#158669,#158670,#158671,#158672,#158673,#158674,#158675,#158676,#158677,
#158678,#158679,#158680,#158681,#158682,#158683,#158684,#158685,#158686,
#158687,#158688,#158689,#158690,#158691,#158692,#158693,#158694,#158695,
#158696,#158697,#158698,#158699,#158700,#158701,#158702,#158703,#158704,
#158705,#158706,#158707,#158708,#158709,#158710,#158711,#158712,#158713,
#158714,#158715,#158716,#158717,#158718,#158719,#158720,#158721,#158722,
#158723,#158724),.UNSPECIFIED.,.F.,.F.,(4,3,3,3,3,3,3,3,3,3,3,3,3,3,3,3,
3,3,3,3,4),(0.,0.107509121767451,0.212828833412304,0.315061928584091,0.374999999999339,
0.437499999999212,0.468749999999133,0.484374999999095,0.492187499999061,
0.496093749999059,0.499999999999056,0.562499999999177,0.624999999999298,
0.673320118680395,0.719243863834343,0.749999999999539,0.806482839148098,
0.864299406979082,0.922736798740935,0.98187500024349,1.),.UNSPECIFIED.);
#4858=B_SPLINE_CURVE_WITH_KNOTS('',3,(#158729,#158730,#158731,#158732,#158733,
#158734,#158735,#158736,#158737,#158738,#158739,#158740,#158741,#158742,
#158743,#158744,#158745,#158746,#158747,#158748,#158749,#158750,#158751,
#158752,#158753,#158754,#158755,#158756),.UNSPECIFIED.,.F.,.F.,(4,3,3,3,
3,3,3,3,3,4),(0.,0.249999999999957,0.374999999999935,0.437499999999924,
0.468749999999919,0.484374999999917,0.499511718749913,0.499999999999911,
0.882725836403091,1.),.UNSPECIFIED.);
#4859=B_SPLINE_CURVE_WITH_KNOTS('',3,(#158757,#158758,#158759,#158760,#158761,
#158762,#158763,#158764,#158765,#158766,#158767,#158768,#158769,#158770,
#158771,#158772),.UNSPECIFIED.,.F.,.F.,(4,2,2,1,1,1,1,2,2,4),(0.,0.249999999999903,
0.374999999999855,0.437499999999831,0.468749999999819,0.484374999999812,
0.492187499999809,0.499511718749801,0.4999999999998,1.),.UNSPECIFIED.);
#4860=B_SPLINE_CURVE_WITH_KNOTS('',3,(#158787,#158788,#158789,#158790,#158791,
#158792,#158793,#158794,#158795,#158796,#158797,#158798,#158799,#158800,
#158801,#158802,#158803,#158804,#158805,#158806,#158807,#158808,#158809,
#158810,#158811,#158812,#158813,#158814,#158815,#158816),.UNSPECIFIED.,
 .F.,.F.,(4,2,2,2,1,1,1,2,2,2,2,1,1,1,2,2,2,4),(0.,0.124999999999242,0.187499999998862,
0.218749999998682,0.2343749999986,0.242187499998551,0.246093749998534,0.248046874998532,
0.24999999999853,0.374999999998953,0.437499999999164,0.468749999999281,
0.484374999999338,0.492187499999366,0.496093749999368,0.49999999999937,
0.749999999999685,1.),.UNSPECIFIED.);
#4861=B_SPLINE_CURVE_WITH_KNOTS('',3,(#158820,#158821,#158822,#158823,#158824,
#158825,#158826,#158827,#158828,#158829,#158830,#158831,#158832,#158833,
#158834,#158835,#158836,#158837,#158838,#158839,#158840,#158841,#158842,
#158843,#158844,#158845,#158846,#158847,#158848,#158849,#158850,#158851,
#158852,#158853,#158854,#158855,#158856,#158857,#158858,#158859,#158860,
#158861,#158862,#158863,#158864,#158865,#158866,#158867,#158868,#158869,
#158870,#158871,#158872,#158873,#158874,#158875,#158876,#158877,#158878,
#158879,#158880,#158881,#158882,#158883,#158884,#158885,#158886,#158887,
#158888,#158889,#158890,#158891,#158892,#158893,#158894,#158895,#158896,
#158897,#158898,#158899,#158900,#158901,#158902,#158903,#158904,#158905,
#158906,#158907,#158908,#158909,#158910,#158911,#158912,#158913,#158914,
#158915,#158916,#158917,#158918,#158919,#158920,#158921,#158922,#158923,
#158924,#158925,#158926,#158927,#158928,#158929,#158930,#158931,#158932,
#158933,#158934,#158935,#158936,#158937,#158938,#158939,#158940,#158941,
#158942,#158943,#158944,#158945,#158946,#158947,#158948,#158949),
 .UNSPECIFIED.,.F.,.F.,(4,3,3,3,3,3,3,3,3,3,3,3,3,3,3,3,3,3,3,3,3,3,3,3,
3,3,3,3,3,3,3,3,3,3,3,3,3,3,3,3,3,3,3,4),(0.,0.0626020078314224,0.12324694439226,
0.182080107324034,0.238598266130295,0.250000000000055,0.259982465184285,
0.314824665619934,0.354767132150864,0.380835408119498,0.430687988199657,
0.463893449524915,0.480496180187545,0.488797545518859,0.492948228184517,
0.495142943523771,0.495701691310286,0.496087181651465,0.496422077430329,
0.497098910850174,0.499250141665798,0.499899244790537,0.500161408362611,
0.567469545706375,0.601123614378257,0.618828367313947,0.633430720214261,
0.634777683050139,0.671858037763955,0.690862597687715,0.729912399485414,
0.74804687500011,0.748759759105555,0.750000000000109,0.779470645992731,
0.808817315775199,0.838104849358379,0.867326644519458,0.875000000000055,
0.903673998781796,0.932886331005841,0.962446376948863,0.992551691206423,
1.),.UNSPECIFIED.);
#4862=B_SPLINE_CURVE_WITH_KNOTS('',3,(#158950,#158951,#158952,#158953),
 .UNSPECIFIED.,.F.,.F.,(4,4),(0.00465289315641866,0.00515351125805147),
 .UNSPECIFIED.);
#4863=B_SPLINE_CURVE_WITH_KNOTS('',3,(#158957,#158958,#158959,#158960,#158961,
#158962,#158963,#158964,#158965,#158966,#158967,#158968,#158969,#158970,
#158971,#158972),.UNSPECIFIED.,.F.,.F.,(4,3,3,3,3,4),(0.00061266112179062,
0.00182296639992346,0.00298506204158171,0.00388203060349254,0.00558489832474453,
0.00715140008519447),.UNSPECIFIED.);
#4864=B_SPLINE_CURVE_WITH_KNOTS('',3,(#158976,#158977,#158978,#158979,#158980,
#158981,#158982,#158983,#158984,#158985,#158986,#158987,#158988,#158989,
#158990,#158991,#158992,#158993,#158994),.UNSPECIFIED.,.F.,.F.,(4,3,3,3,
3,3,4),(0.000544979362130299,0.00239221479429946,0.00380801466457332,0.00469824400931087,
0.00578923755784715,0.00680407029599512,0.00707104996701635),
 .UNSPECIFIED.);
#4865=B_SPLINE_CURVE_WITH_KNOTS('',3,(#159016,#159017,#159018,#159019,#159020,
#159021,#159022,#159023,#159024,#159025,#159026,#159027,#159028,#159029,
#159030,#159031,#159032,#159033,#159034),.UNSPECIFIED.,.F.,.F.,(4,3,3,3,
3,3,4),(4.13078214559669E-7,0.173852294489811,0.36677856517358,0.445174356588884,
0.722587178294442,0.929452460433655,1.),.UNSPECIFIED.);
#4866=B_SPLINE_CURVE_WITH_KNOTS('',3,(#159035,#159036,#159037,#159038,#159039,
#159040,#159041,#159042,#159043,#159044,#159045,#159046,#159047,#159048,
#159049,#159050,#159051,#159052,#159053,#159054,#159055,#159056,#159057,
#159058,#159059,#159060,#159061,#159062,#159063,#159064,#159065,#159066,
#159067,#159068,#159069,#159070,#159071,#159072,#159073,#159074,#159075,
#159076,#159077,#159078,#159079,#159080,#159081,#159082,#159083,#159084,
#159085,#159086,#159087,#159088,#159089,#159090,#159091,#159092,#159093,
#159094,#159095,#159096,#159097,#159098,#159099,#159100,#159101,#159102,
#159103,#159104,#159105,#159106,#159107,#159108,#159109,#159110),
 .UNSPECIFIED.,.F.,.F.,(4,3,3,3,3,3,3,3,3,3,3,3,3,3,3,3,3,3,3,3,3,3,3,3,
3,4),(0.,0.0690701057454117,0.125000000000561,0.187500000000856,0.21875000000099,
0.23437500000107,0.242187500001099,0.246093750001112,0.250000000001125,
0.289133934492208,0.328724352958703,0.368791285218157,0.409021034277532,
0.449394661938092,0.468750000001254,0.484375000001259,0.492187500001262,
0.496093750001307,0.49804687500128,0.500000000001253,0.590549171677946,
0.683067489715376,0.778781322937074,0.876449024523388,0.977044229356509,
1.),.UNSPECIFIED.);
#4867=B_SPLINE_CURVE_WITH_KNOTS('',3,(#159111,#159112,#159113,#159114,#159115,
#159116,#159117,#159118,#159119,#159120,#159121,#159122,#159123,#159124,
#159125,#159126,#159127,#159128,#159129,#159130,#159131,#159132,#159133,
#159134,#159135,#159136,#159137,#159138,#159139,#159140,#159141,#159142,
#159143,#159144,#159145,#159146,#159147,#159148,#159149,#159150,#159151,
#159152,#159153,#159154,#159155,#159156,#159157,#159158,#159159,#159160,
#159161,#159162,#159163,#159164,#159165,#159166,#159167,#159168,#159169,
#159170,#159171,#159172,#159173,#159174,#159175,#159176,#159177,#159178,
#159179,#159180,#159181,#159182,#159183,#159184,#159185,#159186,#159187,
#159188,#159189,#159190,#159191,#159192,#159193,#159194,#159195,#159196,
#159197,#159198,#159199,#159200,#159201,#159202,#159203,#159204,#159205,
#159206,#159207,#159208,#159209,#159210),.UNSPECIFIED.,.F.,.F.,(4,3,3,3,
3,3,3,3,3,3,3,3,3,3,3,3,3,3,3,3,3,3,3,3,3,3,3,3,3,3,3,3,3,4),(0.,0.0892180981438803,
0.125000000000199,0.187500000000311,0.218750000000367,0.234375000000406,
0.242187500000414,0.246093750000407,0.2500000000004,0.318440736490326,0.384858698678957,
0.437499999999504,0.468749999999366,0.484374999999297,0.492187499999262,
0.496093749999246,0.498046874999247,0.499999999999249,0.534729265670756,
0.569880614318735,0.605480155084377,0.641236534437177,0.677123723783148,
0.68749999999937,0.718749999999408,0.734374999999456,0.742187499999477,
0.746093749999491,0.748046874999498,0.749999999999506,0.822639083758781,
0.896597809459177,0.972564265462607,1.),.UNSPECIFIED.);
#4868=B_SPLINE_CURVE_WITH_KNOTS('',3,(#159215,#159216,#159217,#159218,#159219,
#159220,#159221,#159222,#159223,#159224,#159225,#159226,#159227,#159228,
#159229,#159230),.UNSPECIFIED.,.F.,.F.,(4,2,2,1,1,1,1,2,2,4),(0.,0.250000000000162,
0.375000000000243,0.437500000000284,0.468750000000303,0.484375000000312,
0.492187500000317,0.499511718750325,0.500000000000325,1.),.UNSPECIFIED.);
#4869=B_SPLINE_CURVE_WITH_KNOTS('',3,(#159231,#159232,#159233,#159234,#159235,
#159236,#159237,#159238,#159239,#159240,#159241,#159242,#159243,#159244,
#159245,#159246),.UNSPECIFIED.,.F.,.F.,(4,2,2,1,1,1,1,2,2,4),(0.,0.249999999999989,
0.374999999999983,0.43749999999998,0.468749999999979,0.48437499999998,0.49218749999998,
0.499023437499977,0.499999999999976,1.),.UNSPECIFIED.);
#4870=B_SPLINE_CURVE_WITH_KNOTS('',3,(#159252,#159253,#159254,#159255,#159256,
#159257,#159258,#159259,#159260,#159261,#159262,#159263,#159264,#159265),
 .UNSPECIFIED.,.F.,.F.,(4,2,2,1,1,2,2,4),(0.,0.250000000000154,0.375000000000264,
0.437500000000318,0.468750000000337,0.484375000000338,0.500000000000339,
1.),.UNSPECIFIED.);
#4871=B_SPLINE_CURVE_WITH_KNOTS('',3,(#159297,#159298,#159299,#159300,#159301,
#159302,#159303,#159304,#159305,#159306,#159307,#159308,#159309,#159310,
#159311,#159312,#159313,#159314,#159315),.UNSPECIFIED.,.F.,.F.,(4,3,3,3,
3,3,4),(0.000636256268971442,0.00222779634231115,0.00387629126444982,0.00562803598926337,
0.00591708699638702,0.0078089691620698,0.00825282706815076),
 .UNSPECIFIED.);
#4872=B_SPLINE_CURVE_WITH_KNOTS('',3,(#159319,#159320,#159321,#159322,#159323,
#159324,#159325,#159326,#159327,#159328,#159329,#159330,#159331,#159332,
#159333,#159334,#159335,#159336,#159337),.UNSPECIFIED.,.F.,.F.,(4,3,3,3,
3,3,4),(0.000711431901436798,0.00260509764011623,0.00304924424816995,0.00478266330431027,
0.00644043866278196,0.00801739908969177,0.00833474438776835),
 .UNSPECIFIED.);
#4873=B_SPLINE_CURVE_WITH_KNOTS('',3,(#159359,#159360,#159361,#159362,#159363,
#159364,#159365,#159366,#159367,#159368,#159369,#159370,#159371,#159372,
#159373,#159374),.UNSPECIFIED.,.F.,.F.,(4,3,3,3,3,4),(8.01577071537318E-7,
0.262495050804752,0.389947950402742,0.611074818510006,0.806599097074307,
1.),.UNSPECIFIED.);
#4874=B_SPLINE_CURVE_WITH_KNOTS('',3,(#159375,#159376,#159377,#159378,#159379,
#159380,#159381,#159382,#159383,#159384,#159385,#159386,#159387,#159388,
#159389,#159390,#159391,#159392,#159393,#159394,#159395,#159396,#159397,
#159398,#159399,#159400,#159401,#159402,#159403,#159404,#159405,#159406,
#159407,#159408,#159409,#159410,#159411,#159412,#159413,#159414,#159415,
#159416,#159417,#159418,#159419,#159420,#159421,#159422,#159423,#159424,
#159425,#159426,#159427,#159428,#159429,#159430,#159431,#159432,#159433,
#159434,#159435,#159436,#159437,#159438,#159439,#159440,#159441,#159442,
#159443,#159444,#159445,#159446,#159447,#159448,#159449,#159450,#159451,
#159452,#159453,#159454,#159455,#159456,#159457,#159458,#159459),
 .UNSPECIFIED.,.F.,.F.,(4,3,3,3,3,3,3,3,3,3,3,3,3,3,3,3,3,3,3,3,3,3,3,3,
3,3,3,3,4),(1.71570245437392E-5,0.0625000000005735,0.125000000001147,0.18750000000171,
0.218750000001983,0.234375000002118,0.242187500002177,0.246093750002206,
0.24804687500222,0.250000000002234,0.300092256335661,0.351162113591053,
0.375000000001859,0.430234827802864,0.43750000000167,0.468750000001586,
0.484375000001535,0.4965639918839,0.500000000001485,0.500516815631294,0.55935025332849,
0.620369079944048,0.625000000001113,0.695027282812789,0.744902136073919,
0.776223206194934,0.847905243539548,0.923952621769774,1.),.UNSPECIFIED.);
#4875=B_SPLINE_CURVE_WITH_KNOTS('',3,(#159460,#159461,#159462,#159463,#159464,
#159465,#159466,#159467,#159468,#159469,#159470,#159471,#159472,#159473,
#159474,#159475,#159476,#159477,#159478,#159479,#159480,#159481,#159482,
#159483,#159484,#159485,#159486,#159487,#159488,#159489,#159490,#159491,
#159492,#159493,#159494,#159495,#159496,#159497,#159498,#159499),
 .UNSPECIFIED.,.F.,.F.,(4,2,2,1,1,1,1,2,2,2,2,2,1,1,1,2,2,2,2,1,1,1,2,2,
4),(0.,0.125000000002992,0.187500000004488,0.218750000005237,0.234375000005619,
0.242187500005819,0.246093750005911,0.249023437505987,0.250000000006018,
0.375000000004521,0.437500000003772,0.468750000003398,0.484375000003211,
0.492187500003117,0.496093750003077,0.498046875003056,0.500000000003036,
0.625000000002027,0.687500000001514,0.718750000001247,0.734375000001123,
0.742187500001071,0.746093750001047,0.750000000001022,0.999999986537213),
 .UNSPECIFIED.);
#4876=B_SPLINE_CURVE_WITH_KNOTS('',3,(#159504,#159505,#159506,#159507,#159508,
#159509,#159510,#159511,#159512,#159513,#159514,#159515,#159516,#159517,
#159518,#159519,#159520,#159521,#159522,#159523,#159524,#159525,#159526,
#159527,#159528,#159529,#159530,#159531,#159532,#159533,#159534),
 .UNSPECIFIED.,.F.,.F.,(4,3,3,3,3,3,3,3,3,3,4),(0.,0.150663464397143,0.304609114316041,
0.464152105860527,0.499023437500262,0.500000000000263,0.500022138851066,
0.6250166041383,0.749963007430494,0.880076354371466,1.),.UNSPECIFIED.);
#4877=B_SPLINE_CURVE_WITH_KNOTS('',3,(#159535,#159536,#159537,#159538,#159539,
#159540,#159541,#159542,#159543,#159544,#159545,#159546,#159547,#159548,
#159549,#159550),.UNSPECIFIED.,.F.,.F.,(4,2,2,1,1,1,1,2,2,4),(0.,0.249999999999979,
0.374999999999969,0.437499999999965,0.468749999999961,0.484374999999959,
0.492187499999957,0.499023437499959,0.499999999999959,1.),.UNSPECIFIED.);
#4878=B_SPLINE_CURVE_WITH_KNOTS('',3,(#159572,#159573,#159574,#159575,#159576,
#159577,#159578,#159579,#159580,#159581,#159582,#159583,#159584,#159585,
#159586,#159587,#159588,#159589,#159590),.UNSPECIFIED.,.F.,.F.,(4,3,3,3,
3,3,4),(0.000623203325049932,0.00219889325760342,0.00382915155667807,0.00555512420839928,
0.00571003463709915,0.00756817415875732,0.00806753801901704),
 .UNSPECIFIED.);
#4879=B_SPLINE_CURVE_WITH_KNOTS('',3,(#159594,#159595,#159596,#159597,#159598,
#159599,#159600,#159601,#159602,#159603,#159604,#159605,#159606,#159607,
#159608,#159609),.UNSPECIFIED.,.F.,.F.,(4,3,3,3,3,4),(0.000694356721436431,
0.00259637723166065,0.00305563622484018,0.00480503978353614,0.00647539340150544,
0.00814574701947475),.UNSPECIFIED.);
#4880=B_SPLINE_CURVE_WITH_KNOTS('',3,(#159623,#159624,#159625,#159626,#159627,
#159628,#159629,#159630,#159631,#159632,#159633,#159634,#159635,#159636,
#159637,#159638),.UNSPECIFIED.,.F.,.F.,(4,3,3,3,3,4),(0.000539871559505675,
0.00223531956680388,0.00375574051851002,0.00457928549922769,0.00579560462260641,
0.00697160947751436),.UNSPECIFIED.);
#4881=B_SPLINE_CURVE_WITH_KNOTS('',3,(#159642,#159643,#159644,#159645,#159646,
#159647,#159648,#159649,#159650,#159651,#159652,#159653,#159654,#159655,
#159656,#159657),.UNSPECIFIED.,.F.,.F.,(4,3,3,3,3,4),(0.000601267884717356,
0.00181647811676878,0.00299735824906937,0.00382211018819771,0.00557536121784445,
0.00704295249167806),.UNSPECIFIED.);
#4882=B_SPLINE_CURVE_WITH_KNOTS('',3,(#159662,#159663,#159664,#159665,#159666,
#159667,#159668,#159669,#159670,#159671,#159672,#159673,#159674,#159675,
#159676,#159677,#159678,#159679,#159680,#159681,#159682,#159683,#159684,
#159685,#159686),.UNSPECIFIED.,.F.,.F.,(4,3,3,3,3,3,3,3,4),(0.000498343012073112,
0.00231282934720829,0.00337277528899485,0.00370896758807423,0.00446136300849209,
0.00522125339641071,0.00534496249690202,0.00614439986206087,0.00624720756634296),
 .UNSPECIFIED.);
#4883=B_SPLINE_CURVE_WITH_KNOTS('',3,(#159690,#159691,#159692,#159693,#159694,
#159695,#159696,#159697,#159698,#159699,#159700,#159701,#159702,#159703,
#159704,#159705,#159706,#159707,#159708,#159709,#159710,#159711,#159712,
#159713,#159714),.UNSPECIFIED.,.F.,.F.,(4,3,3,3,3,3,3,3,4),(0.000524342078796179,
0.0018090187682887,0.00304673005325099,0.00340077219985262,0.00411987972637411,
0.00482370949852624,0.00550912189800533,0.00616177752105068,0.00627720230593858),
 .UNSPECIFIED.);
#4884=B_SPLINE_CURVE_WITH_KNOTS('',3,(#159726,#159727,#159728,#159729,#159730,
#159731,#159732,#159733,#159734,#159735,#159736,#159737,#159738,#159739,
#159740,#159741),.UNSPECIFIED.,.F.,.F.,(4,2,2,2,1,1,2,2,4),(0.,0.250000000000448,
0.375000000000645,0.437500000000763,0.468750000000802,0.484375000000844,
0.492187500000843,0.500000000000842,1.),.UNSPECIFIED.);
#4885=B_SPLINE_CURVE_WITH_KNOTS('',3,(#159745,#159746,#159747,#159748,#159749,
#159750,#159751,#159752,#159753,#159754,#159755,#159756,#159757),
 .UNSPECIFIED.,.F.,.F.,(4,3,3,3,4),(0.,0.282022506904398,0.55577415031973,
0.81819454057582,1.),.UNSPECIFIED.);
#4886=B_SPLINE_CURVE_WITH_KNOTS('',3,(#159758,#159759,#159760,#159761,#159762,
#159763,#159764,#159765,#159766,#159767,#159768,#159769,#159770,#159771,
#159772,#159773,#159774,#159775,#159776,#159777,#159778,#159779,#159780,
#159781,#159782,#159783,#159784,#159785,#159786,#159787,#159788,#159789,
#159790,#159791,#159792,#159793,#159794,#159795,#159796,#159797,#159798,
#159799,#159800,#159801,#159802,#159803,#159804,#159805,#159806),
 .UNSPECIFIED.,.F.,.F.,(4,3,3,3,3,3,3,3,3,3,3,3,3,3,3,3,4),(0.,0.115464076706584,
0.204631414112565,0.249999999999961,0.288081633301557,0.398618541405039,
0.498046874999928,0.499807527138215,0.499999999999929,0.569629412683859,
0.624999999999946,0.693718017752262,0.749999999999964,0.813244782606989,
0.876468684100435,0.940110360346619,1.),.UNSPECIFIED.);
#4887=B_SPLINE_CURVE_WITH_KNOTS('',3,(#159833,#159834,#159835,#159836,#159837,
#159838,#159839,#159840,#159841,#159842,#159843,#159844),.UNSPECIFIED.,
 .F.,.F.,(4,2,1,1,2,2,4),(0.,0.250000000000003,0.375000000000005,0.437500000000007,
0.468750000000007,0.500000000000006,1.),.UNSPECIFIED.);
#4888=B_SPLINE_CURVE_WITH_KNOTS('',3,(#159845,#159846,#159847,#159848,#159849,
#159850,#159851,#159852,#159853,#159854,#159855,#159856,#159857,#159858,
#159859,#159860,#159861,#159862,#159863,#159864,#159865,#159866,#159867,
#159868,#159869,#159870,#159871,#159872,#159873,#159874,#159875,#159876,
#159877,#159878,#159879,#159880,#159881,#159882,#159883,#159884,#159885,
#159886,#159887,#159888,#159889,#159890,#159891,#159892,#159893,#159894,
#159895,#159896,#159897,#159898,#159899,#159900,#159901,#159902,#159903,
#159904,#159905,#159906,#159907,#159908),.UNSPECIFIED.,.F.,.F.,(4,3,3,3,
3,3,3,3,3,3,3,3,3,3,3,3,3,3,3,3,3,4),(0.,0.06478051091971,0.124999999999183,
0.187499999998777,0.218749999998586,0.23437499999849,0.24633111659959,0.249999999998394,
0.303541233291795,0.357640266150352,0.412373093698651,0.437499999997239,
0.468749999997027,0.484374999996945,0.492187499996904,0.496093749996909,
0.499999999996914,0.597546155193341,0.698418193262823,0.801205662027104,
0.90739104893303,1.),.UNSPECIFIED.);
#4889=B_SPLINE_CURVE_WITH_KNOTS('',3,(#159930,#159931,#159932,#159933,#159934,
#159935,#159936,#159937,#159938,#159939,#159940,#159941,#159942,#159943,
#159944,#159945,#159946,#159947,#159948),.UNSPECIFIED.,.F.,.F.,(4,3,3,3,
3,3,4),(0.,0.244850538777774,0.488158489871772,0.552096889019018,0.73851462781602,
0.910728935155691,0.999999749632916),.UNSPECIFIED.);
#4890=B_SPLINE_CURVE_WITH_KNOTS('',3,(#159949,#159950,#159951,#159952,#159953,
#159954,#159955,#159956,#159957,#159958,#159959,#159960,#159961,#159962,
#159963,#159964,#159965,#159966,#159967,#159968,#159969,#159970,#159971,
#159972,#159973,#159974,#159975,#159976,#159977,#159978,#159979,#159980,
#159981,#159982,#159983,#159984,#159985,#159986,#159987,#159988,#159989,
#159990,#159991,#159992,#159993,#159994,#159995,#159996,#159997,#159998,
#159999,#160000,#160001,#160002,#160003,#160004,#160005,#160006,#160007,
#160008,#160009,#160010,#160011,#160012,#160013,#160014,#160015,#160016,
#160017,#160018,#160019,#160020,#160021,#160022,#160023,#160024,#160025,
#160026,#160027,#160028,#160029,#160030),.UNSPECIFIED.,.F.,.F.,(4,3,3,3,
3,3,3,3,3,3,3,3,3,3,3,3,3,3,3,3,3,3,3,3,3,3,3,4),(2.533555643913E-8,0.0910320813626261,
0.125000000001408,0.187500000002101,0.218750000002447,0.23437500000262,
0.242187500002707,0.24609375000275,0.248046875002772,0.250000000002794,
0.286382660441103,0.32291484838725,0.359669340739657,0.394628946654578,
0.431903778620834,0.470456940434937,0.496093750001528,0.499668058076043,
0.500000000001504,0.500264737842257,0.569725175841976,0.625000000001128,
0.700983068432055,0.750000000000752,0.82894421112137,0.910139370401911,
0.994278938005407,1.),.UNSPECIFIED.);
#4891=B_SPLINE_CURVE_WITH_KNOTS('',3,(#160031,#160032,#160033,#160034,#160035,
#160036,#160037,#160038,#160039,#160040,#160041,#160042,#160043,#160044,
#160045,#160046,#160047,#160048,#160049,#160050,#160051,#160052,#160053,
#160054,#160055,#160056,#160057,#160058,#160059,#160060,#160061,#160062,
#160063,#160064,#160065,#160066,#160067,#160068,#160069,#160070,#160071,
#160072,#160073,#160074,#160075,#160076,#160077,#160078,#160079,#160080,
#160081,#160082,#160083,#160084,#160085,#160086,#160087,#160088,#160089,
#160090,#160091,#160092,#160093,#160094,#160095,#160096,#160097,#160098,
#160099,#160100),.UNSPECIFIED.,.F.,.F.,(4,3,3,3,3,3,3,3,3,3,3,3,3,3,3,3,
3,3,3,3,3,3,3,4),(0.,0.115241963249706,0.210943191186066,0.272629228253125,
0.375456875050642,0.473607625967427,0.498046874995147,0.499999999995132,
0.500407886731958,0.537881861244917,0.575395554961941,0.612898174107899,
0.624999999996623,0.662411153773846,0.699072930188149,0.734374999997964,
0.742187499998073,0.746093749998126,0.749691223502617,0.749999999998179,
0.817036471811887,0.88546296533256,0.955529737150269,0.999991171984779),
 .UNSPECIFIED.);
#4892=B_SPLINE_CURVE_WITH_KNOTS('',3,(#160127,#160128,#160129,#160130,#160131,
#160132,#160133,#160134,#160135,#160136,#160137,#160138,#160139,#160140,
#160141,#160142),.UNSPECIFIED.,.F.,.F.,(4,3,3,3,3,4),(0.,0.200694999329658,
0.427247628482963,0.604195087233359,0.885229128579841,0.999999354109336),
 .UNSPECIFIED.);
#4893=B_SPLINE_CURVE_WITH_KNOTS('',3,(#160143,#160144,#160145,#160146,#160147,
#160148,#160149,#160150,#160151,#160152,#160153,#160154,#160155,#160156,
#160157,#160158,#160159,#160160,#160161,#160162,#160163,#160164,#160165,
#160166,#160167,#160168,#160169,#160170,#160171,#160172,#160173,#160174,
#160175,#160176,#160177,#160178,#160179,#160180,#160181,#160182,#160183,
#160184,#160185,#160186,#160187,#160188,#160189,#160190,#160191,#160192,
#160193,#160194,#160195,#160196,#160197,#160198,#160199,#160200,#160201,
#160202,#160203,#160204,#160205,#160206,#160207,#160208,#160209,#160210,
#160211,#160212,#160213,#160214,#160215,#160216,#160217,#160218,#160219,
#160220,#160221,#160222,#160223,#160224,#160225,#160226,#160227,#160228,
#160229,#160230,#160231,#160232,#160233,#160234,#160235,#160236,#160237,
#160238,#160239,#160240,#160241,#160242,#160243,#160244,#160245),
 .UNSPECIFIED.,.F.,.F.,(4,3,3,3,3,3,3,3,3,3,3,3,3,3,3,3,3,3,3,3,3,3,3,3,
3,3,3,3,3,3,3,3,3,3,4),(1.5402703012166E-8,0.125000000000293,0.208446749922841,
0.244646765557539,0.245773986165532,0.246072415283787,0.246368383987472,
0.248334622198511,0.249310060686018,0.249836852332955,0.250148121466892,
0.315972242753915,0.373760882794706,0.444714699846058,0.498046875000427,
0.500000000000431,0.500779867134539,0.53444283139843,0.562500000000715,
0.598013518121477,0.625000000000999,0.66129218269956,0.687500000001273,
0.718750000001425,0.734375000001481,0.742187500001509,0.746093750001524,
0.748046875001505,0.7485351562515,0.749267578126493,0.750000000001485,0.818372711897459,
0.888509784935343,0.961434487868489,1.),.UNSPECIFIED.);
#4894=B_SPLINE_CURVE_WITH_KNOTS('',3,(#160246,#160247,#160248,#160249,#160250,
#160251,#160252,#160253,#160254,#160255,#160256,#160257,#160258,#160259,
#160260,#160261,#160262,#160263,#160264,#160265,#160266,#160267,#160268,
#160269,#160270,#160271,#160272,#160273,#160274,#160275,#160276,#160277,
#160278,#160279,#160280,#160281,#160282,#160283,#160284,#160285,#160286,
#160287,#160288,#160289,#160290,#160291,#160292,#160293,#160294,#160295,
#160296,#160297,#160298,#160299,#160300,#160301,#160302,#160303,#160304,
#160305,#160306,#160307,#160308,#160309,#160310,#160311,#160312,#160313,
#160314,#160315,#160316,#160317,#160318,#160319,#160320,#160321,#160322,
#160323,#160324,#160325,#160326,#160327,#160328,#160329,#160330,#160331,
#160332,#160333,#160334,#160335,#160336,#160337,#160338,#160339,#160340,
#160341,#160342,#160343,#160344,#160345,#160346,#160347,#160348,#160349,
#160350,#160351,#160352,#160353,#160354),.UNSPECIFIED.,.F.,.F.,(4,3,3,3,
3,3,3,3,3,3,3,3,3,3,3,3,3,3,3,3,3,3,3,3,3,3,3,3,3,3,3,3,3,3,3,3,4),(0.,
0.0953370365995093,0.176698850256003,0.215158368973863,0.231984408412927,
0.239871614399988,0.243691979799971,0.245572315895275,0.246091243916352,
0.2463897663404,0.248249025978357,0.249171393064374,0.249740342882374,0.249997511217146,
0.250204522741881,0.310264212512982,0.368061028373041,0.428066686248988,
0.484374999998885,0.495112152105643,0.499805054424163,0.499999999998881,
0.547749307420529,0.596812594126604,0.624999999998827,0.674967800891608,
0.6874999999988,0.718749999998787,0.73437499999878,0.742187499998761,0.746093749998768,
0.748046874998789,0.749999999998811,0.825517565210902,0.903222315217755,
0.983862504053623,0.999984984351931),.UNSPECIFIED.);
#4895=B_SPLINE_CURVE_WITH_KNOTS('',3,(#160400,#160401,#160402,#160403,#160404,
#160405,#160406,#160407,#160408,#160409,#160410,#160411,#160412),
 .UNSPECIFIED.,.F.,.F.,(4,3,3,3,4),(0.,0.00150087219104035,0.00207200756106571,
0.00310801134159857,0.00414401512213143),.UNSPECIFIED.);
#4896=B_SPLINE_CURVE_WITH_KNOTS('',3,(#160416,#160417,#160418,#160419,#160420,
#160421,#160422,#160423,#160424,#160425,#160426,#160427,#160428,#160429,
#160430,#160431,#160432,#160433,#160434,#160435,#160436,#160437,#160438,
#160439,#160440,#160441,#160442,#160443,#160444,#160445,#160446,#160447,
#160448,#160449,#160450,#160451,#160452,#160453,#160454,#160455,#160456,
#160457,#160458,#160459,#160460,#160461,#160462,#160463,#160464,#160465,
#160466,#160467,#160468,#160469,#160470,#160471,#160472,#160473,#160474,
#160475,#160476,#160477,#160478,#160479,#160480,#160481,#160482,#160483,
#160484,#160485,#160486,#160487,#160488),.UNSPECIFIED.,.F.,.F.,(4,3,3,3,
3,3,3,3,3,3,3,3,3,3,3,3,3,3,3,3,3,3,3,3,4),(0.,0.0827800474306258,0.164476544804415,
0.244653694889878,0.323963103854387,0.402053885677088,0.437500000000753,
0.468750000000797,0.482808608553153,0.497325464085628,0.500000000000842,
0.563666376687189,0.625583188344086,0.687500000000982,0.718750000001013,
0.734375000001029,0.742187500001028,0.746930764484763,0.750000000001027,
0.798770062773211,0.846466169814649,0.892304506589185,0.936986645493463,
0.979989519943143,1.),.UNSPECIFIED.);
#4897=B_SPLINE_CURVE_WITH_KNOTS('',3,(#160510,#160511,#160512,#160513,#160514,
#160515,#160516,#160517,#160518,#160519,#160520,#160521,#160522,#160523,
#160524,#160525,#160526,#160527,#160528,#160529,#160530,#160531,#160532,
#160533,#160534,#160535,#160536,#160537,#160538,#160539,#160540,#160541,
#160542,#160543,#160544,#160545,#160546,#160547,#160548,#160549,#160550,
#160551,#160552,#160553,#160554,#160555,#160556,#160557,#160558,#160559,
#160560,#160561,#160562,#160563,#160564),.UNSPECIFIED.,.F.,.F.,(4,3,3,3,
3,3,3,3,3,3,3,3,3,3,3,3,3,3,4),(0.,0.104715580701354,0.210383985033992,
0.249999999999817,0.354011981377643,0.374999999999734,0.437499999999696,
0.468749999999665,0.484374999999646,0.493439254443789,0.499999999999626,
0.577747102581383,0.652041765361407,0.721927843697446,0.749999999999813,
0.814470107593342,0.877192615710051,0.938596307855025,1.),.UNSPECIFIED.);
#4898=B_SPLINE_CURVE_WITH_KNOTS('',3,(#160567,#160568,#160569,#160570,#160571,
#160572,#160573),.UNSPECIFIED.,.F.,.F.,(4,3,4),(4.71238898038468,5.49778714378214,
6.28318530717959),.UNSPECIFIED.);
#4899=B_SPLINE_CURVE_WITH_KNOTS('',3,(#160597,#160598,#160599,#160600,#160601,
#160602,#160603),.UNSPECIFIED.,.F.,.F.,(4,3,4),(3.14159265358979,3.92699081698724,
4.71238898038469),.UNSPECIFIED.);
#4900=B_SPLINE_CURVE_WITH_KNOTS('',3,(#160606,#160607,#160608,#160609,#160610,
#160611,#160612,#160613,#160614,#160615,#160616,#160617,#160618,#160619,
#160620,#160621,#160622,#160623,#160624,#160625,#160626,#160627,#160628,
#160629,#160630,#160631,#160632,#160633,#160634,#160635,#160636,#160637,
#160638,#160639,#160640,#160641,#160642,#160643,#160644,#160645,#160646,
#160647,#160648,#160649,#160650,#160651),.UNSPECIFIED.,.F.,.F.,(4,3,3,3,
3,3,3,3,3,3,3,3,3,3,3,4),(0.,0.0605468750000088,0.122426142584879,0.186284753089235,
0.245362452615264,0.322247692375512,0.398189409304048,0.475083017862261,
0.484375000000071,0.493930247608612,0.500000000000069,0.605247959003852,
0.710628641082224,0.816191187900766,0.922233554824866,1.),.UNSPECIFIED.);
#4901=B_SPLINE_CURVE_WITH_KNOTS('',3,(#160656,#160657,#160658,#160659,#160660,
#160661,#160662,#160663,#160664,#160665,#160666,#160667,#160668,#160669,
#160670,#160671,#160672,#160673,#160674,#160675,#160676,#160677,#160678,
#160679,#160680,#160681,#160682,#160683,#160684,#160685,#160686,#160687,
#160688,#160689,#160690,#160691,#160692,#160693,#160694,#160695,#160696,
#160697,#160698,#160699,#160700,#160701,#160702,#160703,#160704,#160705,
#160706,#160707,#160708,#160709,#160710,#160711,#160712,#160713,#160714,
#160715,#160716,#160717,#160718,#160719,#160720,#160721,#160722,#160723,
#160724,#160725,#160726,#160727,#160728),.UNSPECIFIED.,.F.,.F.,(4,3,3,3,
3,3,3,3,3,3,3,3,3,3,3,3,3,3,3,3,3,3,3,3,4),(0.,0.0827800472710771,0.164476544468573,
0.244653694362582,0.323963103155625,0.402053884755395,0.437500000000487,
0.468750000000525,0.482808608365209,0.497325463721906,0.500000000000563,
0.563666376083932,0.625583188042332,0.687500000000732,0.718750000000761,
0.734375000000765,0.742187500000777,0.746930764471125,0.75000000000079,
0.79877006272679,0.846466169726166,0.892304506462131,0.936986645329322,
0.979989519741638,1.),.UNSPECIFIED.);
#4902=B_SPLINE_CURVE_WITH_KNOTS('',3,(#160729,#160730,#160731,#160732,#160733,
#160734,#160735,#160736,#160737,#160738,#160739,#160740,#160741,#160742,
#160743,#160744,#160745,#160746,#160747,#160748,#160749,#160750,#160751,
#160752,#160753,#160754,#160755,#160756,#160757,#160758,#160759,#160760,
#160761,#160762,#160763,#160764,#160765,#160766,#160767,#160768,#160769,
#160770,#160771,#160772,#160773,#160774,#160775,#160776,#160777,#160778,
#160779,#160780,#160781,#160782,#160783,#160784,#160785,#160786,#160787,
#160788,#160789,#160790,#160791,#160792,#160793,#160794,#160795,#160796,
#160797,#160798),.UNSPECIFIED.,.F.,.F.,(4,3,3,3,3,3,3,3,3,3,3,3,3,3,3,3,
3,3,3,3,3,3,3,4),(0.,0.0417433063302083,0.0856783502063842,0.125000000000064,
0.172058636966678,0.221141673751301,0.242187500000112,0.247530062035886,
0.25000000000012,0.258757699077574,0.318098755622358,0.375000000000093,
0.438761223505778,0.468750000000083,0.483267071906232,0.497350908759363,
0.500000000000075,0.586409574409656,0.674221064481857,0.743171333762874,
0.750000000000038,0.839284683635661,0.929619546314489,1.),.UNSPECIFIED.);
#4903=B_SPLINE_CURVE_WITH_KNOTS('',3,(#160821,#160822,#160823,#160824,#160825,
#160826,#160827),.UNSPECIFIED.,.F.,.F.,(4,3,4),(4.71238898038469,5.49778714378214,
6.28318530717959),.UNSPECIFIED.);
#4904=B_SPLINE_CURVE_WITH_KNOTS('',3,(#160829,#160830,#160831,#160832,#160833,
#160834,#160835,#160836,#160837,#160838,#160839,#160840,#160841,#160842,
#160843,#160844,#160845,#160846,#160847,#160848,#160849,#160850,#160851,
#160852,#160853,#160854,#160855,#160856,#160857,#160858,#160859,#160860,
#160861,#160862,#160863,#160864,#160865,#160866,#160867,#160868,#160869,
#160870,#160871,#160872,#160873,#160874,#160875,#160876,#160877,#160878,
#160879,#160880,#160881,#160882,#160883),.UNSPECIFIED.,.F.,.F.,(4,3,3,3,
3,3,3,3,3,3,3,3,3,3,3,3,3,3,4),(0.,0.1047155801347,0.210383983761551,0.249999999998705,
0.354011980517942,0.374999999998113,0.437499999997821,0.468749999997671,
0.484374999997637,0.49343925441085,0.499999999997603,0.577747102421286,
0.65204176505497,0.721927843234957,0.749999999998801,0.814470107408982,
0.877192615336184,0.938596307668092,1.),.UNSPECIFIED.);
#4905=B_SPLINE_CURVE_WITH_KNOTS('',3,(#160907,#160908,#160909,#160910,#160911,
#160912,#160913),.UNSPECIFIED.,.F.,.F.,(4,3,4),(-8.88178419700125E-16,0.78539816339745,
1.5707963267949),.UNSPECIFIED.);
#4906=B_SPLINE_CURVE_WITH_KNOTS('',3,(#160916,#160917,#160918,#160919,#160920,
#160921,#160922,#160923,#160924,#160925,#160926,#160927,#160928,#160929,
#160930,#160931,#160932,#160933,#160934,#160935,#160936,#160937,#160938,
#160939,#160940,#160941,#160942,#160943,#160944,#160945,#160946,#160947,
#160948,#160949,#160950,#160951,#160952,#160953,#160954,#160955,#160956,
#160957,#160958,#160959,#160960,#160961),.UNSPECIFIED.,.F.,.F.,(4,3,3,3,
3,3,3,3,3,3,3,3,3,3,3,4),(0.,0.060546874999865,0.122426142580309,0.186284753080097,
0.245362452602329,0.322247692345566,0.398189409215696,0.475083013998846,
0.48437499999892,0.49393024760668,0.499999999998935,0.605247958974294,0.710628641027629,
0.816191187822136,0.922233554723543,1.),.UNSPECIFIED.);
#4907=B_SPLINE_CURVE_WITH_KNOTS('',3,(#160967,#160968,#160969,#160970,#160971,
#160972,#160973,#160974,#160975,#160976,#160977,#160978,#160979,#160980,
#160981,#160982,#160983,#160984,#160985,#160986,#160987,#160988,#160989,
#160990,#160991,#160992,#160993,#160994,#160995,#160996,#160997,#160998,
#160999,#161000,#161001,#161002,#161003,#161004,#161005,#161006,#161007,
#161008,#161009,#161010,#161011,#161012,#161013,#161014,#161015,#161016,
#161017,#161018,#161019,#161020,#161021,#161022,#161023,#161024,#161025,
#161026,#161027,#161028,#161029,#161030,#161031,#161032,#161033,#161034,
#161035,#161036),.UNSPECIFIED.,.F.,.F.,(4,3,3,3,3,3,3,3,3,3,3,3,3,3,3,3,
3,3,3,3,3,3,3,4),(0.,0.0417433067437773,0.085678351037766,0.125000000000076,
0.172058637390442,0.221141674281389,0.242187500000128,0.247530062059483,
0.250000000000119,0.258757699107327,0.318098756280707,0.375000000000195,
0.438761224377743,0.46875000000021,0.483267072005296,0.497350908963462,
0.500000000000197,0.586409574334292,0.67422106433992,0.743171333738989,
0.750000000000099,0.839284683557368,0.929619546162419,1.),.UNSPECIFIED.);
#4908=B_SPLINE_CURVE_WITH_KNOTS('',3,(#161079,#161080,#161081,#161082,#161083,
#161084,#161085,#161086,#161087,#161088,#161089,#161090,#161091,#161092,
#161093,#161094,#161095,#161096,#161097,#161098,#161099,#161100,#161101,
#161102,#161103,#161104,#161105,#161106,#161107,#161108,#161109,#161110,
#161111,#161112,#161113,#161114,#161115,#161116,#161117,#161118,#161119,
#161120,#161121,#161122,#161123,#161124,#161125,#161126,#161127),
 .UNSPECIFIED.,.F.,.F.,(4,3,3,3,3,3,3,3,3,3,3,3,3,3,3,3,4),(0.,0.104472515273559,
0.209822727893399,0.24999999999986,0.35418712941254,0.438820809815404,0.484374999999763,
0.493439281928252,0.49999999999974,0.577466051600214,0.651600365001254,
0.721481777027291,0.74999999999987,0.814614317509502,0.877383216253357,
0.938691608126678,1.),.UNSPECIFIED.);
#4909=B_SPLINE_CURVE_WITH_KNOTS('',3,(#161130,#161131,#161132,#161133,#161134,
#161135,#161136),.UNSPECIFIED.,.F.,.F.,(4,3,4),(1.5707963267949,2.35619449019235,
3.1415926535898),.UNSPECIFIED.);
#4910=B_SPLINE_CURVE_WITH_KNOTS('',3,(#161160,#161161,#161162,#161163,#161164,
#161165,#161166),.UNSPECIFIED.,.F.,.F.,(4,3,4),(1.23467863058848E-16,0.785398163397447,
1.5707963267949),.UNSPECIFIED.);
#4911=B_SPLINE_CURVE_WITH_KNOTS('',3,(#161169,#161170,#161171,#161172,#161173,
#161174,#161175,#161176,#161177,#161178,#161179,#161180,#161181,#161182,
#161183,#161184,#161185,#161186,#161187,#161188,#161189,#161190,#161191,
#161192,#161193,#161194,#161195,#161196,#161197,#161198,#161199,#161200,
#161201,#161202,#161203,#161204,#161205,#161206,#161207,#161208,#161209,
#161210,#161211,#161212,#161213,#161214,#161215,#161216,#161217,#161218,
#161219,#161220),.UNSPECIFIED.,.F.,.F.,(4,3,3,3,3,3,3,3,3,3,3,3,3,3,3,3,
3,4),(0.,0.0625000000000772,0.124900823545415,0.190034230928347,0.250000000000309,
0.319870182296621,0.375000000000471,0.437500000000552,0.468750000000589,
0.48437500000056,0.494074303447769,0.50000000000053,0.591975494567463,0.685251275132029,
0.780573779584712,0.877101419355448,0.975445333692385,1.),.UNSPECIFIED.);
#4912=B_SPLINE_CURVE_WITH_KNOTS('',3,(#161223,#161224,#161225,#161226,#161227,
#161228,#161229,#161230,#161231,#161232,#161233,#161234,#161235,#161236,
#161237,#161238,#161239,#161240,#161241,#161242,#161243,#161244,#161245,
#161246,#161247,#161248,#161249,#161250,#161251,#161252,#161253,#161254,
#161255,#161256,#161257,#161258,#161259,#161260,#161261,#161262,#161263,
#161264,#161265,#161266,#161267,#161268,#161269,#161270,#161271,#161272,
#161273,#161274,#161275,#161276,#161277,#161278,#161279,#161280,#161281,
#161282,#161283,#161284,#161285,#161286,#161287,#161288,#161289,#161290,
#161291,#161292,#161293,#161294,#161295,#161296,#161297,#161298),
 .UNSPECIFIED.,.F.,.F.,(4,3,3,3,3,3,3,3,3,3,3,3,3,3,3,3,3,3,3,3,3,3,3,3,
3,4),(0.,0.0427401092012923,0.0873804166631017,0.13313759505412,0.180399662455455,
0.187500000000028,0.218750000000024,0.234375000000025,0.242187500000029,
0.247546297842306,0.250000000000033,0.309158131845126,0.369865863968725,
0.375000000000126,0.437500000000172,0.46875000000019,0.483324530441297,
0.497499574224517,0.500000000000208,0.577335497435133,0.655589023587681,
0.734790128085894,0.815464874684637,0.897007690809156,0.979843823811218,
1.),.UNSPECIFIED.);
#4913=B_SPLINE_CURVE_WITH_KNOTS('',3,(#161321,#161322,#161323,#161324,#161325,
#161326,#161327,#161328,#161329,#161330,#161331,#161332,#161333),
 .UNSPECIFIED.,.F.,.F.,(4,3,3,3,4),(6.93889390390723E-18,0.00113151531066505,
0.00191432655883665,0.00348473784371938,0.00382865311767331),
 .UNSPECIFIED.);
#4914=B_SPLINE_CURVE_WITH_KNOTS('',3,(#161339,#161340,#161341,#161342,#161343,
#161344,#161345,#161346,#161347,#161348,#161349,#161350,#161351,#161352,
#161353,#161354,#161355,#161356,#161357,#161358,#161359,#161360,#161361,
#161362,#161363,#161364,#161365,#161366,#161367,#161368,#161369,#161370,
#161371,#161372,#161373,#161374,#161375,#161376,#161377,#161378,#161379,
#161380,#161381,#161382,#161383,#161384,#161385,#161386,#161387,#161388,
#161389,#161390,#161391,#161392,#161393,#161394,#161395,#161396,#161397,
#161398,#161399,#161400,#161401,#161402,#161403,#161404,#161405,#161406,
#161407,#161408),.UNSPECIFIED.,.F.,.F.,(4,3,3,3,3,3,3,3,3,3,3,3,3,3,3,3,
3,3,3,3,3,3,3,4),(0.,0.0904805863956041,0.179890948435827,0.24999999999996,
0.256840728572676,0.344945742334393,0.429509229332709,0.468749999999929,
0.482752596495082,0.497175643681866,0.499999999999926,0.56298906712764,
0.6249999999999,0.68399450346291,0.741245408299592,0.74218749999991,0.746913732826963,
0.749999999999906,0.799311389349656,0.849483542012242,0.894712088324863,
0.938468707059143,0.980197893115309,1.),.UNSPECIFIED.);
#4915=B_SPLINE_CURVE_WITH_KNOTS('',3,(#161432,#161433,#161434,#161435,#161436,
#161437,#161438),.UNSPECIFIED.,.F.,.F.,(4,3,4),(4.71238898038468,5.49778714378213,
6.28318530717959),.UNSPECIFIED.);
#4916=B_SPLINE_CURVE_WITH_KNOTS('',3,(#161440,#161441,#161442,#161443,#161444,
#161445,#161446,#161447,#161448,#161449,#161450,#161451,#161452,#161453,
#161454,#161455,#161456,#161457,#161458,#161459,#161460,#161461,#161462,
#161463,#161464,#161465,#161466,#161467,#161468,#161469,#161470,#161471,
#161472,#161473,#161474,#161475,#161476,#161477,#161478,#161479,#161480,
#161481,#161482,#161483,#161484,#161485,#161486,#161487,#161488),
 .UNSPECIFIED.,.F.,.F.,(4,3,3,3,3,3,3,3,3,3,3,3,3,3,3,3,4),(0.,0.104472515277785,
0.209822727901897,0.25000000000095,0.354187129412535,0.438820810898927,
0.484375000001802,0.493439281930502,0.500000000001818,0.577466051602124,
0.65160036500341,0.721481777029761,0.750000000000909,0.814614317510989,
0.87738321625524,0.93869160812762,1.),.UNSPECIFIED.);
#4917=B_SPLINE_CURVE_WITH_KNOTS('',3,(#161512,#161513,#161514,#161515,#161516,
#161517,#161518),.UNSPECIFIED.,.F.,.F.,(4,3,4),(1.23467863058848E-16,0.785398163397447,
1.5707963267949),.UNSPECIFIED.);
#4918=B_SPLINE_CURVE_WITH_KNOTS('',3,(#161521,#161522,#161523,#161524,#161525,
#161526,#161527,#161528,#161529,#161530,#161531,#161532,#161533,#161534,
#161535,#161536,#161537,#161538,#161539,#161540,#161541,#161542,#161543,
#161544,#161545,#161546,#161547,#161548,#161549,#161550,#161551,#161552,
#161553,#161554,#161555,#161556,#161557,#161558,#161559,#161560,#161561,
#161562,#161563,#161564,#161565,#161566,#161567,#161568,#161569,#161570,
#161571,#161572),.UNSPECIFIED.,.F.,.F.,(4,3,3,3,3,3,3,3,3,3,3,3,3,3,3,3,
3,4),(0.,0.0625000000000519,0.124900823545418,0.190034230928422,0.250000000000208,
0.319870182295419,0.375000000000326,0.437500000000372,0.468750000000392,
0.484375000000367,0.494074303447496,0.500000000000342,0.591975494567397,
0.685251275132125,0.780573779585023,0.87710141935604,0.97544533369326,1.),
 .UNSPECIFIED.);
#4919=B_SPLINE_CURVE_WITH_KNOTS('',3,(#161577,#161578,#161579,#161580,#161581,
#161582,#161583,#161584,#161585,#161586,#161587,#161588,#161589,#161590,
#161591,#161592,#161593,#161594,#161595,#161596,#161597,#161598,#161599,
#161600,#161601,#161602,#161603,#161604,#161605,#161606,#161607,#161608,
#161609,#161610,#161611,#161612,#161613,#161614,#161615,#161616,#161617,
#161618,#161619,#161620,#161621,#161622,#161623,#161624,#161625,#161626,
#161627,#161628,#161629,#161630,#161631,#161632,#161633,#161634,#161635,
#161636,#161637,#161638,#161639,#161640,#161641,#161642,#161643,#161644,
#161645,#161646),.UNSPECIFIED.,.F.,.F.,(4,3,3,3,3,3,3,3,3,3,3,3,3,3,3,3,
3,3,3,3,3,3,3,4),(0.,0.0904805863645094,0.179890948371529,0.249999999999614,
0.25684072858258,0.344945742312153,0.42950922919613,0.468749999999293,0.482752596421625,
0.497175643541116,0.499999999999244,0.562989066800544,0.624999999999167,
0.683994503499725,0.741245408316608,0.742187499999101,0.746913732804136,
0.749999999999098,0.799311389113812,0.849483541835359,0.894712087957233,
0.938468706507326,0.980197892375734,1.),.UNSPECIFIED.);
#4920=B_SPLINE_CURVE_WITH_KNOTS('',3,(#161647,#161648,#161649,#161650,#161651,
#161652,#161653,#161654,#161655,#161656,#161657,#161658,#161659,#161660,
#161661,#161662,#161663,#161664,#161665,#161666,#161667,#161668,#161669,
#161670,#161671,#161672,#161673,#161674,#161675,#161676,#161677,#161678,
#161679,#161680,#161681,#161682,#161683,#161684,#161685,#161686,#161687,
#161688,#161689,#161690,#161691,#161692,#161693,#161694,#161695,#161696,
#161697,#161698,#161699,#161700,#161701,#161702,#161703,#161704,#161705,
#161706,#161707,#161708,#161709,#161710,#161711,#161712,#161713,#161714,
#161715,#161716,#161717,#161718,#161719,#161720,#161721,#161722),
 .UNSPECIFIED.,.F.,.F.,(4,3,3,3,3,3,3,3,3,3,3,3,3,3,3,3,3,3,3,3,3,3,3,3,
3,4),(0.,0.0427401094863224,0.0873804172404971,0.133137595941066,0.180399663654732,
0.18749999999992,0.218749999999916,0.234374999999926,0.242187499999936,
0.247546297862462,0.249999999999946,0.309158132445463,0.36986586515317,
0.374999999999943,0.437499999999942,0.468749999999964,0.483324530559454,
0.497499574469254,0.499999999999985,0.577335497496591,0.655589023707543,
0.734790128260523,0.815464874927968,0.897007691098662,0.979843824141047,
1.),.UNSPECIFIED.);
#4921=B_SPLINE_CURVE_WITH_KNOTS('',3,(#161736,#161737,#161738,#161739,#161740,
#161741,#161742,#161743,#161744,#161745,#161746,#161747,#161748,#161749,
#161750,#161751,#161752,#161753,#161754,#161755,#161756,#161757,#161758,
#161759,#161760,#161761,#161762,#161763,#161764,#161765,#161766,#161767,
#161768,#161769,#161770,#161771,#161772),.UNSPECIFIED.,.F.,.F.,(4,3,3,3,
3,3,3,3,3,3,3,3,4),(1.70755612180505E-6,0.218048820966207,0.413536615724655,
0.450190577241864,0.467372121703056,0.470177992009516,0.486734929759218,
0.494754696481731,0.498886349000283,0.501099101143529,0.683464306546563,
0.847789526356529,1.),.UNSPECIFIED.);
#4922=B_SPLINE_CURVE_WITH_KNOTS('',3,(#161773,#161774,#161775,#161776,#161777,
#161778,#161779,#161780,#161781,#161782,#161783,#161784,#161785,#161786,
#161787,#161788,#161789,#161790,#161791,#161792,#161793,#161794,#161795,
#161796,#161797,#161798,#161799,#161800,#161801,#161802,#161803,#161804,
#161805,#161806),.UNSPECIFIED.,.F.,.F.,(4,3,3,3,3,3,3,3,3,3,3,4),(2.03157429207824E-5,
0.14867142041905,0.273762375268916,0.374999999999955,0.429438237983039,
0.484372693795509,0.499999999999939,0.506412229479512,0.639519611027661,
0.770764026496447,0.900223227858203,1.),.UNSPECIFIED.);
#4923=B_SPLINE_CURVE_WITH_KNOTS('',3,(#161829,#161830,#161831,#161832,#161833,
#161834,#161835,#161836,#161837,#161838,#161839,#161840,#161841,#161842),
 .UNSPECIFIED.,.F.,.F.,(4,2,2,2,2,2,4),(0.,0.250000000000022,0.375000000000029,
0.43750000000005,0.500000000000072,0.750000000000036,1.),.UNSPECIFIED.);
#4924=B_SPLINE_CURVE_WITH_KNOTS('',3,(#161845,#161846,#161847,#161848,#161849,
#161850,#161851,#161852,#161853,#161854,#161855,#161856,#161857,#161858,
#161859,#161860,#161861,#161862,#161863,#161864,#161865,#161866,#161867,
#161868,#161869,#161870,#161871,#161872),.UNSPECIFIED.,.F.,.F.,(4,3,3,3,
3,3,3,3,3,4),(0.,0.138160071953523,0.28057569199304,0.430296839593711,0.491456739356699,
0.5,0.653325725654778,0.78125,0.967247952047853,1.),.UNSPECIFIED.);
#4925=B_SPLINE_CURVE_WITH_KNOTS('',3,(#161926,#161927,#161928,#161929,#161930,
#161931,#161932,#161933,#161934,#161935,#161936,#161937,#161938,#161939,
#161940,#161941,#161942,#161943,#161944,#161945,#161946,#161947,#161948,
#161949,#161950,#161951,#161952,#161953,#161954,#161955,#161956,#161957,
#161958,#161959,#161960,#161961,#161962,#161963,#161964,#161965,#161966,
#161967,#161968,#161969,#161970,#161971,#161972,#161973,#161974,#161975,
#161976,#161977,#161978,#161979,#161980,#161981,#161982,#161983,#161984,
#161985,#161986),.UNSPECIFIED.,.F.,.F.,(4,3,3,3,3,3,3,3,3,3,3,3,3,3,3,3,
3,3,3,3,4),(0.,0.0624999999999682,0.124999999999936,0.187499999999898,0.21874999999989,
0.234374999999906,0.244323266293418,0.249999999999922,0.332208918070905,
0.37500000000021,0.437500000000337,0.468750000000369,0.484375000000366,
0.494186090879374,0.500000000000364,0.584475175928334,0.670102559384199,
0.757636314324216,0.846235385908535,0.936632476909697,1.),.UNSPECIFIED.);
#4926=B_SPLINE_CURVE_WITH_KNOTS('',3,(#161987,#161988,#161989,#161990,#161991,
#161992,#161993,#161994,#161995,#161996,#161997,#161998,#161999,#162000,
#162001,#162002,#162003,#162004,#162005,#162006,#162007,#162008,#162009,
#162010,#162011,#162012,#162013,#162014,#162015,#162016,#162017,#162018,
#162019,#162020,#162021,#162022,#162023,#162024,#162025,#162026,#162027,
#162028,#162029,#162030,#162031,#162032),.UNSPECIFIED.,.F.,.F.,(4,3,3,3,
3,3,3,3,3,3,3,3,3,3,3,4),(0.,0.000109331983970333,0.000221348099123991,
0.000333853905449093,0.000407294015799104,0.00040891081566422,0.000676681051257162,
0.000814588031598208,0.000816767951597528,0.00106247378106637,0.00122188204739731,
0.00122336180785488,0.00135439024293119,0.0014917831530638,0.00162097073973685,
0.00162917606319641),.UNSPECIFIED.);
#4927=B_SPLINE_CURVE_WITH_KNOTS('',3,(#162066,#162067,#162068,#162069,#162070,
#162071,#162072,#162073,#162074,#162075,#162076,#162077,#162078,#162079,
#162080,#162081,#162082,#162083,#162084,#162085,#162086,#162087,#162088,
#162089,#162090,#162091,#162092,#162093,#162094,#162095,#162096,#162097,
#162098,#162099,#162100,#162101,#162102,#162103,#162104,#162105,#162106,
#162107,#162108,#162109,#162110,#162111,#162112,#162113,#162114,#162115,
#162116,#162117,#162118,#162119,#162120,#162121,#162122,#162123,#162124,
#162125,#162126,#162127,#162128,#162129,#162130,#162131,#162132,#162133,
#162134,#162135,#162136,#162137,#162138),.UNSPECIFIED.,.F.,.F.,(4,3,3,3,
3,3,3,3,3,3,3,3,3,3,3,3,3,3,3,3,3,3,3,3,4),(0.,0.0886343067351491,0.17728465402347,
0.250000000000028,0.339768627519797,0.419803528705912,0.484375000000132,
0.484817009440956,0.494431768800152,0.500000000000148,0.579374625844902,
0.625000000000001,0.68749999999995,0.718749999999931,0.734374999999927,
0.74037936111593,0.74218749999993,0.747622414733742,0.749999999999932,0.797680859480093,
0.84531438956593,0.891837596509057,0.93715800399846,0.980323118936031,1.),
 .UNSPECIFIED.);
#4928=B_SPLINE_CURVE_WITH_KNOTS('',3,(#162141,#162142,#162143,#162144,#162145,
#162146,#162147,#162148,#162149,#162150),.UNSPECIFIED.,.F.,.F.,(4,2,2,2,
4),(0.,0.25,0.5,0.75,1.),.UNSPECIFIED.);
#4929=B_SPLINE_CURVE_WITH_KNOTS('',3,(#162175,#162176,#162177,#162178,#162179,
#162180,#162181,#162182,#162183,#162184,#162185,#162186,#162187,#162188,
#162189,#162190,#162191,#162192,#162193,#162194,#162195,#162196,#162197,
#162198,#162199,#162200,#162201,#162202,#162203,#162204,#162205),
 .UNSPECIFIED.,.F.,.F.,(4,3,3,3,3,3,3,3,3,3,4),(0.,0.140771014207785,0.2827542070083,
0.419250990292061,0.5,0.500558885625981,0.612546529858198,0.728431346217552,
0.844245046450148,0.956707375096577,1.),.UNSPECIFIED.);
#4930=B_SPLINE_CURVE_WITH_KNOTS('',3,(#162221,#162222,#162223,#162224,#162225,
#162226,#162227,#162228,#162229,#162230),.UNSPECIFIED.,.F.,.F.,(4,3,3,4),
(0.,0.324689572914811,0.662344786457405,1.),.UNSPECIFIED.);
#4931=B_SPLINE_CURVE_WITH_KNOTS('',3,(#162271,#162272,#162273,#162274,#162275,
#162276,#162277,#162278,#162279,#162280,#162281,#162282,#162283,#162284,
#162285,#162286,#162287,#162288,#162289,#162290,#162291,#162292,#162293,
#162294,#162295,#162296,#162297,#162298,#162299,#162300,#162301,#162302,
#162303,#162304,#162305,#162306,#162307,#162308,#162309,#162310,#162311,
#162312,#162313,#162314,#162315,#162316,#162317,#162318,#162319,#162320,
#162321,#162322,#162323,#162324,#162325,#162326,#162327,#162328,#162329,
#162330,#162331,#162332,#162333,#162334),.UNSPECIFIED.,.F.,.F.,(4,3,3,3,
3,3,3,3,3,3,3,3,3,3,3,3,3,3,3,3,3,4),(0.,0.124999999999932,0.187499999999894,
0.212470944414348,0.236430927507225,0.249999999999857,0.282985586965997,
0.374999999999872,0.415041056558414,0.454731726716648,0.49308919967899,
0.499999999999889,0.535211298208892,0.608652493243637,0.624999999999905,
0.668556878124494,0.711950889580769,0.749999999999921,0.769948319789834,
0.843818367415393,0.921909183395617,0.99999999937584),.UNSPECIFIED.);
#4932=B_SPLINE_CURVE_WITH_KNOTS('',3,(#162337,#162338,#162339,#162340,#162341,
#162342,#162343,#162344,#162345,#162346,#162347,#162348,#162349,#162350,
#162351,#162352,#162353,#162354,#162355,#162356,#162357,#162358,#162359,
#162360,#162361,#162362,#162363,#162364,#162365,#162366,#162367,#162368,
#162369,#162370,#162371,#162372,#162373,#162374,#162375,#162376,#162377,
#162378,#162379),.UNSPECIFIED.,.F.,.F.,(4,3,3,3,3,3,3,3,3,3,3,3,3,3,4),
(0.,0.000108912497168437,0.000220164732383741,0.000331071157537523,0.000392199517465982,
0.000393776648066525,0.000641215708209299,0.000785392845861483,0.000787553296133051,
0.00103453341935802,0.00117987002828324,0.00118132994419958,0.00130742143740821,
0.00144126401483716,0.0015751065922661),.UNSPECIFIED.);
#4933=B_SPLINE_CURVE_WITH_KNOTS('',3,(#162420,#162421,#162422,#162423,#162424,
#162425,#162426,#162427,#162428,#162429,#162430,#162431,#162432,#162433,
#162434,#162435,#162436,#162437,#162438,#162439,#162440,#162441,#162442,
#162443,#162444,#162445,#162446,#162447,#162448,#162449,#162450,#162451,
#162452,#162453,#162454,#162455,#162456,#162457,#162458,#162459,#162460,
#162461,#162462,#162463,#162464,#162465,#162466,#162467,#162468,#162469,
#162470,#162471,#162472,#162473,#162474,#162475,#162476,#162477,#162478,
#162479,#162480,#162481,#162482,#162483,#162484,#162485,#162486,#162487,
#162488,#162489,#162490,#162491,#162492,#162493,#162494,#162495,#162496,
#162497,#162498,#162499,#162500,#162501),.UNSPECIFIED.,.F.,.F.,(4,3,3,3,
3,3,3,3,3,3,3,3,3,3,3,3,3,3,3,3,3,3,3,3,3,3,3,4),(0.,0.0665796625644221,
0.124999999999965,0.194730242247893,0.210359162922861,0.216044757699717,
0.219049295426768,0.236001069080282,0.248594752262763,0.251421853354319,
0.320964043791546,0.391760595068546,0.437499999999978,0.46162556726757,
0.485139651704675,0.499999999999965,0.501282997982719,0.567072139505908,
0.624999999999971,0.687499999999976,0.711787277249982,0.735596853593493,
0.749999999999982,0.750995459618546,0.818462588046628,0.885485905599099,
0.951384278224423,1.),.UNSPECIFIED.);
#4934=B_SPLINE_CURVE_WITH_KNOTS('',3,(#162504,#162505,#162506,#162507,#162508,
#162509,#162510,#162511,#162512,#162513,#162514,#162515,#162516,#162517,
#162518),.UNSPECIFIED.,.F.,.F.,(4,2,2,2,1,2,2,4),(0.,0.250000000000107,
0.375000000000158,0.437500000000159,0.468750000000162,0.484375000000163,
0.500000000000164,1.),.UNSPECIFIED.);
#4935=B_SPLINE_CURVE_WITH_KNOTS('',3,(#162552,#162553,#162554,#162555,#162556,
#162557,#162558,#162559,#162560,#162561,#162562,#162563,#162564,#162565,
#162566,#162567,#162568,#162569,#162570,#162571,#162572,#162573,#162574,
#162575,#162576,#162577,#162578,#162579,#162580,#162581,#162582,#162583,
#162584,#162585,#162586,#162587,#162588,#162589,#162590,#162591,#162592,
#162593,#162594,#162595,#162596,#162597,#162598,#162599,#162600,#162601,
#162602,#162603,#162604,#162605,#162606,#162607,#162608,#162609,#162610,
#162611,#162612,#162613,#162614,#162615,#162616,#162617,#162618,#162619,
#162620,#162621,#162622,#162623,#162624,#162625,#162626,#162627),
 .UNSPECIFIED.,.F.,.F.,(4,3,3,3,3,3,3,3,3,3,3,3,3,3,3,3,3,3,3,3,3,3,3,3,
3,4),(0.,0.12499999999987,0.23628510341623,0.24999999999974,0.312499999999692,
0.374999999999645,0.4374999999996,0.468749999999579,0.484374999999532,0.493831417688319,
0.499999999999485,0.562499999999428,0.568696020518362,0.5937499999994,0.624999999999372,
0.687499999999315,0.718749999999315,0.734374999999345,0.742908936105005,
0.749999999999375,0.798369290592606,0.812499999999531,0.877723444080328,
0.929687499999824,0.995541758473931,1.),.UNSPECIFIED.);
#4936=B_SPLINE_CURVE_WITH_KNOTS('',3,(#162630,#162631,#162632,#162633,#162634,
#162635,#162636,#162637,#162638,#162639,#162640,#162641,#162642,#162643,
#162644,#162645,#162646),.UNSPECIFIED.,.F.,.F.,(4,1,1,2,2,1,1,1,2,2,4),
(0.,0.124999999999952,0.187499999999928,0.218749999999915,0.249999999999903,
0.37499999999986,0.437499999999854,0.468749999999833,0.484374999999823,
0.499999999999812,1.),.UNSPECIFIED.);
#4937=B_SPLINE_CURVE_WITH_KNOTS('',3,(#162699,#162700,#162701,#162702,#162703,
#162704,#162705,#162706,#162707,#162708,#162709,#162710,#162711,#162712,
#162713,#162714,#162715,#162716,#162717,#162718,#162719,#162720,#162721,
#162722,#162723,#162724,#162725,#162726,#162727,#162728,#162729,#162730,
#162731,#162732,#162733,#162734,#162735,#162736,#162737,#162738),
 .UNSPECIFIED.,.F.,.F.,(4,3,3,3,3,3,3,3,3,3,3,3,3,4),(0.,0.000424781762269412,
0.000463398440131748,0.000464821262797086,0.000754099901314684,0.000926796880263496,
0.000929181095996172,0.0011584961003294,0.00116090942630379,0.00139019532039531,
0.00139219601406769,0.00155797632182194,0.00171877163871738,0.00185359376052713),
 .UNSPECIFIED.);
#4938=B_SPLINE_CURVE_WITH_KNOTS('',3,(#162741,#162742,#162743,#162744,#162745,
#162746,#162747,#162748,#162749,#162750,#162751,#162752,#162753,#162754,
#162755,#162756,#162757,#162758,#162759,#162760,#162761,#162762,#162763,
#162764,#162765,#162766,#162767,#162768,#162769,#162770,#162771,#162772,
#162773,#162774,#162775,#162776,#162777,#162778,#162779,#162780,#162781,
#162782,#162783,#162784,#162785,#162786,#162787,#162788,#162789,#162790,
#162791,#162792,#162793,#162794,#162795,#162796,#162797,#162798,#162799,
#162800,#162801,#162802,#162803,#162804,#162805,#162806,#162807,#162808,
#162809,#162810,#162811,#162812,#162813,#162814,#162815,#162816,#162817,
#162818,#162819,#162820,#162821,#162822,#162823,#162824,#162825,#162826,
#162827,#162828),.UNSPECIFIED.,.F.,.F.,(4,3,3,3,3,3,3,3,3,3,3,3,3,3,3,3,
3,3,3,3,3,3,3,3,3,3,3,3,3,4),(0.,0.0471813589526015,0.062500000000042,0.111599854246627,
0.156868243243704,0.183319433108903,0.202136632240781,0.219600693186217,
0.23121412579211,0.23427767967472,0.235710755256672,0.243779701571778,0.248075229850627,
0.249694423524974,0.250682693256269,0.312508154033365,0.372068646189272,
0.386851020524303,0.43162913834518,0.437500000000381,0.468750000000386,
0.484375000000387,0.493500360972887,0.500000000000388,0.591105250217313,
0.686862723351654,0.710255118648367,0.819587104644768,0.932825248138224,
1.),.UNSPECIFIED.);
#4939=B_SPLINE_CURVE_WITH_KNOTS('',3,(#162868,#162869,#162870,#162871,#162872,
#162873,#162874,#162875,#162876,#162877,#162878,#162879,#162880,#162881,
#162882,#162883,#162884,#162885,#162886,#162887,#162888,#162889,#162890,
#162891,#162892,#162893,#162894,#162895,#162896,#162897,#162898,#162899,
#162900,#162901,#162902,#162903,#162904,#162905,#162906,#162907,#162908,
#162909,#162910,#162911,#162912,#162913,#162914,#162915,#162916,#162917,
#162918,#162919,#162920,#162921,#162922,#162923,#162924,#162925,#162926,
#162927,#162928,#162929,#162930,#162931,#162932,#162933,#162934,#162935,
#162936,#162937),.UNSPECIFIED.,.F.,.F.,(4,3,3,3,3,3,3,3,3,3,3,3,3,3,3,3,
3,3,3,3,3,3,3,4),(0.,0.0823663764173504,0.163873434652409,0.219525593901905,
0.255715741026493,0.274015070266574,0.371382535133357,0.409594292583447,
0.46875000000014,0.484375000000129,0.49436143907224,0.500000000000117,0.549262840412801,
0.624999999999946,0.687499999999886,0.718749999999881,0.732850340412289,
0.746266055559976,0.749999999999877,0.784242342539938,0.850134833448856,
0.914122650155725,0.975785622000229,1.),.UNSPECIFIED.);
#4940=B_SPLINE_CURVE_WITH_KNOTS('',3,(#162940,#162941,#162942,#162943,#162944,
#162945,#162946,#162947,#162948,#162949,#162950,#162951,#162952,#162953,
#162954,#162955,#162956,#162957,#162958,#162959,#162960,#162961,#162962,
#162963,#162964,#162965,#162966,#162967,#162968,#162969,#162970,#162971,
#162972,#162973,#162974,#162975,#162976,#162977,#162978,#162979,#162980,
#162981,#162982,#162983,#162984,#162985,#162986,#162987,#162988),
 .UNSPECIFIED.,.F.,.F.,(4,3,3,3,3,3,3,3,3,3,3,3,3,3,3,3,4),(0.,8.46514984578604E-5,
0.000170997186917751,0.000221020978418102,0.00025513917286212,0.0003380084618147,
0.000429234945598969,0.000448835576014525,0.000450677949086267,0.000735348747783541,
0.000898977028079808,0.000901355898172495,0.00115196682498163,0.00135049620570087,
0.00135203384725872,0.00157737282180184,0.00180271179634495),
 .UNSPECIFIED.);
#4941=B_SPLINE_CURVE_WITH_KNOTS('',3,(#163023,#163024,#163025,#163026,#163027,
#163028,#163029,#163030,#163031,#163032,#163033,#163034,#163035,#163036,
#163037,#163038,#163039,#163040,#163041,#163042,#163043,#163044,#163045,
#163046,#163047,#163048,#163049,#163050),.UNSPECIFIED.,.F.,.F.,(4,3,3,3,
3,3,3,3,3,4),(0.,0.125000000000083,0.187500000000098,0.250000000000114,
0.375000000000096,0.437500000000064,0.500000000000032,0.686608408121615,
0.750000000000016,1.),.UNSPECIFIED.);
#4942=B_SPLINE_CURVE_WITH_KNOTS('',3,(#163053,#163054,#163055,#163056,#163057,
#163058,#163059,#163060,#163061,#163062,#163063,#163064,#163065,#163066,
#163067,#163068,#163069,#163070,#163071,#163072,#163073,#163074,#163075,
#163076,#163077,#163078,#163079,#163080,#163081,#163082,#163083,#163084,
#163085,#163086,#163087,#163088,#163089,#163090,#163091,#163092,#163093,
#163094,#163095,#163096,#163097,#163098,#163099,#163100,#163101),
 .UNSPECIFIED.,.F.,.F.,(4,3,3,3,3,3,3,3,3,3,3,3,3,3,3,3,4),(1.05484258504493E-9,
0.191534277963448,0.259654838607526,0.331309849098388,0.397663184819074,
0.435861255746886,0.46401652053976,0.468749999999952,0.484374999999957,
0.499999999999962,0.526357797460517,0.61505709794376,0.705276548341834,
0.798422422273867,0.893550910308075,0.991493363605814,1.),.UNSPECIFIED.);
#4943=B_SPLINE_CURVE_WITH_KNOTS('',3,(#163123,#163124,#163125,#163126,#163127,
#163128),.UNSPECIFIED.,.F.,.F.,(4,2,4),(0.,0.5,1.),.UNSPECIFIED.);
#4944=B_SPLINE_CURVE_WITH_KNOTS('',3,(#163131,#163132,#163133,#163134,#163135,
#163136,#163137,#163138,#163139,#163140,#163141,#163142,#163143,#163144,
#163145,#163146,#163147,#163148,#163149,#163150,#163151,#163152,#163153,
#163154,#163155,#163156,#163157,#163158,#163159,#163160,#163161,#163162,
#163163,#163164,#163165,#163166,#163167),.UNSPECIFIED.,.F.,.F.,(4,3,3,3,
3,3,3,3,3,3,3,3,4),(0.,0.120708757094103,0.243232014226317,0.365509787471685,
0.477257340603764,0.497653150606378,0.514241701439531,0.6359369624296,0.758974043423795,
0.8125,0.90625,0.953125,1.),.UNSPECIFIED.);
#4945=B_SPLINE_CURVE_WITH_KNOTS('',3,(#163182,#163183,#163184,#163185,#163186,
#163187,#163188,#163189,#163190,#163191,#163192,#163193,#163194,#163195,
#163196,#163197,#163198,#163199,#163200,#163201,#163202,#163203,#163204,
#163205,#163206,#163207,#163208,#163209),.UNSPECIFIED.,.F.,.F.,(4,3,3,3,
3,3,3,3,3,4),(0.,0.11665693587126,0.231069038396355,0.345034028170232,0.457575140319161,
0.5,0.626037841254244,0.752522996696677,0.877297259197685,1.),
 .UNSPECIFIED.);
#4946=B_SPLINE_CURVE_WITH_KNOTS('',3,(#163247,#163248,#163249,#163250,#163251,
#163252,#163253,#163254,#163255,#163256,#163257,#163258,#163259,#163260,
#163261,#163262),.UNSPECIFIED.,.F.,.F.,(4,2,2,2,1,1,2,2,4),(0.,0.250000000000283,
0.375000000000425,0.437500000000534,0.46875000000058,0.484375000000603,
0.492187500000607,0.50000000000061,1.),.UNSPECIFIED.);
#4947=B_SPLINE_CURVE_WITH_KNOTS('',3,(#163263,#163264,#163265,#163266,#163267,
#163268,#163269,#163270,#163271,#163272,#163273,#163274,#163275,#163276,
#163277,#163278,#163279,#163280,#163281,#163282,#163283,#163284,#163285,
#163286,#163287,#163288,#163289,#163290,#163291,#163292,#163293,#163294,
#163295,#163296,#163297,#163298,#163299,#163300,#163301,#163302,#163303,
#163304,#163305,#163306,#163307,#163308),.UNSPECIFIED.,.F.,.F.,(4,3,3,3,
3,3,3,3,3,3,3,3,3,3,3,4),(0.,0.00011167181015012,0.000225567853890619,0.000339431029143628,
0.000397399329631602,0.00039894455910293,0.000667283904094347,0.000794798659263204,
0.000796933919810636,0.00104488468554081,0.00119219798889481,0.0011936849958466,
0.00132317769579385,0.00145638750716013,0.00158130618071587,0.00158959731852641),
 .UNSPECIFIED.);
#4948=B_SPLINE_CURVE_WITH_KNOTS('',3,(#163349,#163350,#163351,#163352,#163353,
#163354,#163355,#163356,#163357,#163358,#163359,#163360,#163361,#163362,
#163363,#163364,#163365,#163366,#163367,#163368,#163369,#163370,#163371,
#163372,#163373,#163374,#163375,#163376,#163377,#163378,#163379,#163380,
#163381,#163382,#163383,#163384,#163385,#163386,#163387,#163388,#163389,
#163390,#163391),.UNSPECIFIED.,.F.,.F.,(4,3,3,3,3,3,3,3,3,3,3,3,3,3,4),
(0.,0.00016756321202441,0.000333534252400233,0.000405329103688545,0.000406806783530084,
0.000681033266856812,0.00081143089222242,0.000813613567060169,0.00109814343430376,
0.00121879730292857,0.00122042035059025,0.00134667139739562,0.00147140108610384,
0.00159377061182578,0.00162722713412034),.UNSPECIFIED.);
#4949=B_SPLINE_CURVE_WITH_KNOTS('',3,(#163393,#163394,#163395,#163396,#163397,
#163398,#163399,#163400,#163401,#163402,#163403,#163404,#163405,#163406,
#163407,#163408,#163409,#163410,#163411,#163412,#163413,#163414,#163415,
#163416,#163417,#163418,#163419,#163420,#163421,#163422,#163423,#163424,
#163425,#163426,#163427,#163428,#163429,#163430,#163431,#163432,#163433,
#163434,#163435,#163436,#163437,#163438,#163439,#163440,#163441,#163442,
#163443,#163444,#163445,#163446,#163447,#163448,#163449,#163450,#163451,
#163452,#163453,#163454,#163455,#163456,#163457,#163458,#163459,#163460,
#163461,#163462),.UNSPECIFIED.,.F.,.F.,(4,3,3,3,3,3,3,3,3,3,3,3,3,3,3,3,
3,3,3,3,3,3,3,4),(0.,0.077221954709809,0.155942297777895,0.237205163639056,
0.245892449851707,0.249999999999969,0.327737648600097,0.374999999999958,
0.437499999999981,0.468749999999967,0.472685944192633,0.484374999999935,
0.492187499999947,0.497991200093118,0.499999999999958,0.61072165925943,
0.708652887979474,0.749999999999979,0.769114755462166,0.781249999999982,
0.858290325115874,0.890624999999991,0.970567820080817,1.),.UNSPECIFIED.);
#4950=B_SPLINE_CURVE_WITH_KNOTS('',3,(#163480,#163481,#163482,#163483,#163484,
#163485,#163486),.UNSPECIFIED.,.F.,.F.,(4,3,4),(0.,0.5,1.),
 .UNSPECIFIED.);
#4951=B_SPLINE_CURVE_WITH_KNOTS('',3,(#163489,#163490,#163491,#163492,#163493,
#163494,#163495,#163496,#163497,#163498,#163499,#163500,#163501,#163502,
#163503,#163504,#163505,#163506,#163507,#163508,#163509,#163510,#163511,
#163512,#163513,#163514,#163515,#163516,#163517,#163518,#163519,#163520,
#163521,#163522,#163523,#163524,#163525),.UNSPECIFIED.,.F.,.F.,(4,3,3,3,
3,3,3,3,3,3,3,3,4),(0.,0.100588965941516,0.213435253911614,0.321668078608275,
0.37500000000007,0.437500000000022,0.468749999999998,0.484374999999996,
0.492187499999995,0.499999999999994,0.684746090436115,0.879413380072057,
1.),.UNSPECIFIED.);
#4952=B_SPLINE_CURVE_WITH_KNOTS('',3,(#163539,#163540,#163541,#163542,#163543,
#163544,#163545,#163546,#163547,#163548,#163549,#163550,#163551,#163552,
#163553,#163554,#163555,#163556,#163557,#163558,#163559,#163560,#163561,
#163562,#163563,#163564,#163565,#163566,#163567,#163568,#163569,#163570,
#163571,#163572),.UNSPECIFIED.,.F.,.F.,(4,3,3,3,3,3,3,3,3,3,3,4),(0.,0.125443689754645,
0.249999999999871,0.383895651702588,0.437499999999815,0.468602955116825,
0.499115673875061,0.499999999999761,0.639475850377752,0.780204293879566,
0.923774089074692,0.999989478723035),.UNSPECIFIED.);
#4953=B_SPLINE_CURVE_WITH_KNOTS('',3,(#163574,#163575,#163576,#163577,#163578,
#163579,#163580,#163581,#163582,#163583,#163584,#163585,#163586,#163587,
#163588,#163589,#163590,#163591,#163592,#163593,#163594,#163595,#163596,
#163597,#163598,#163599,#163600,#163601,#163602,#163603,#163604,#163605,
#163606,#163607,#163608,#163609,#163610),.UNSPECIFIED.,.F.,.F.,(4,3,3,3,
3,3,3,3,3,3,3,3,4),(0.,0.118442531101612,0.242864853287292,0.378342680351954,
0.437499999999567,0.468749999999536,0.484374999999537,0.499215229757745,
0.499999999999537,0.656694403675684,0.817828302438324,0.986303070645228,
0.999999565360524),.UNSPECIFIED.);
#4954=B_SPLINE_CURVE_WITH_KNOTS('',3,(#163633,#163634,#163635,#163636,#163637,
#163638),.UNSPECIFIED.,.F.,.F.,(4,2,4),(0.,0.5,1.),.UNSPECIFIED.);
#4955=B_SPLINE_CURVE_WITH_KNOTS('',3,(#163639,#163640,#163641,#163642,#163643,
#163644,#163645,#163646,#163647,#163648,#163649,#163650),.UNSPECIFIED.,
 .F.,.F.,(4,2,2,2,2,4),(0.,0.249999999999836,0.374999999999753,0.437499999999745,
0.499999999999737,1.),.UNSPECIFIED.);
#4956=B_SPLINE_CURVE_WITH_KNOTS('',3,(#163671,#163672,#163673,#163674,#163675,
#163676,#163677,#163678,#163679,#163680,#163681,#163682,#163683),
 .UNSPECIFIED.,.F.,.F.,(4,3,3,3,4),(0.,0.00157041135329187,0.00191432655883667,
0.00304584187045998,0.00382865311767335),.UNSPECIFIED.);
#4957=B_SPLINE_CURVE_WITH_KNOTS('',3,(#163687,#163688,#163689,#163690,#163691,
#163692,#163693,#163694,#163695,#163696,#163697,#163698,#163699,#163700,
#163701,#163702,#163703,#163704,#163705,#163706,#163707,#163708,#163709,
#163710,#163711,#163712,#163713,#163714,#163715,#163716,#163717,#163718,
#163719,#163720,#163721,#163722,#163723,#163724,#163725,#163726,#163727,
#163728,#163729,#163730,#163731,#163732,#163733,#163734,#163735,#163736,
#163737,#163738,#163739,#163740,#163741,#163742,#163743,#163744,#163745,
#163746,#163747,#163748,#163749,#163750,#163751,#163752,#163753,#163754,
#163755,#163756,#163757,#163758,#163759),.UNSPECIFIED.,.F.,.F.,(4,3,3,3,
3,3,3,3,3,3,3,3,3,3,3,3,3,3,3,3,3,3,3,3,4),(0.,0.082780047467355,0.164476544882018,
0.244653695027588,0.323963104070488,0.402053886069737,0.437500000000005,
0.468750000000019,0.48280860858439,0.497325464146971,0.500000000000034,
0.563238185116385,0.624999999999974,0.687499999999944,0.718749999999934,
0.73437499999992,0.742187499999908,0.746930764488159,0.749999999999896,
0.798770062739853,0.846466169752031,0.892304506499701,0.936986645378172,
0.979989519801786,1.),.UNSPECIFIED.);
#4958=B_SPLINE_CURVE_WITH_KNOTS('',3,(#163781,#163782,#163783,#163784,#163785,
#163786,#163787,#163788,#163789,#163790,#163791,#163792,#163793,#163794,
#163795,#163796,#163797,#163798,#163799,#163800,#163801,#163802,#163803,
#163804,#163805,#163806,#163807,#163808,#163809,#163810,#163811,#163812,
#163813,#163814,#163815,#163816,#163817,#163818,#163819,#163820,#163821,
#163822,#163823,#163824,#163825,#163826,#163827,#163828,#163829,#163830,
#163831,#163832,#163833,#163834,#163835),.UNSPECIFIED.,.F.,.F.,(4,3,3,3,
3,3,3,3,3,3,3,3,3,3,3,3,3,3,4),(0.,0.104715580142832,0.210383983783548,
0.249999999999323,0.354011980528842,0.374999999999033,0.437499999998846,
0.468749999998796,0.484374999998733,0.493439254411786,0.49999999999867,
0.577747102422539,0.652041765056392,0.721927843236613,0.749999999999335,
0.814470107409843,0.877192615337485,0.938596307668742,1.),.UNSPECIFIED.);
#4959=B_SPLINE_CURVE_WITH_KNOTS('',3,(#163838,#163839,#163840,#163841,#163842,
#163843,#163844),.UNSPECIFIED.,.F.,.F.,(4,3,4),(4.71238898038469,5.49778714378214,
6.28318530717959),.UNSPECIFIED.);
#4960=B_SPLINE_CURVE_WITH_KNOTS('',3,(#163868,#163869,#163870,#163871,#163872,
#163873,#163874),.UNSPECIFIED.,.F.,.F.,(4,3,4),(3.1415926535898,3.92699081698724,
4.71238898038469),.UNSPECIFIED.);
#4961=B_SPLINE_CURVE_WITH_KNOTS('',3,(#163877,#163878,#163879,#163880,#163881,
#163882,#163883,#163884,#163885,#163886,#163887,#163888,#163889,#163890,
#163891,#163892,#163893,#163894,#163895,#163896,#163897,#163898,#163899,
#163900,#163901,#163902,#163903,#163904,#163905,#163906,#163907,#163908,
#163909,#163910,#163911,#163912,#163913,#163914,#163915,#163916,#163917,
#163918,#163919,#163920,#163921,#163922),.UNSPECIFIED.,.F.,.F.,(4,3,3,3,
3,3,3,3,3,3,3,3,3,3,3,4),(0.,0.0605468750000136,0.122426142767112,0.186284753451113,
0.245362453102209,0.322247693278209,0.398189410474041,0.475083019593307,
0.484375000000109,0.493930247632433,0.500000000000104,0.605247959968731,
0.710628642835913,0.816191190373723,0.9222335579368,1.),.UNSPECIFIED.);
#4962=B_SPLINE_CURVE_WITH_KNOTS('',3,(#163927,#163928,#163929,#163930,#163931,
#163932,#163933,#163934,#163935,#163936,#163937,#163938,#163939,#163940,
#163941,#163942,#163943,#163944,#163945,#163946,#163947,#163948,#163949,
#163950,#163951,#163952,#163953,#163954,#163955,#163956,#163957,#163958,
#163959,#163960,#163961,#163962,#163963,#163964,#163965,#163966,#163967,
#163968,#163969,#163970,#163971,#163972,#163973,#163974,#163975,#163976,
#163977,#163978,#163979,#163980,#163981,#163982,#163983,#163984,#163985,
#163986,#163987,#163988,#163989,#163990,#163991,#163992,#163993,#163994,
#163995,#163996,#163997,#163998,#163999),.UNSPECIFIED.,.F.,.F.,(4,3,3,3,
3,3,3,3,3,3,3,3,3,3,3,3,3,3,3,3,3,3,3,3,4),(0.,0.0828931975148567,0.164185746816491,
0.244579641303135,0.323662152922592,0.375000000000147,0.437500000000148,
0.468750000000125,0.482808608613976,0.497325464204033,0.500000000000102,
0.563666376881648,0.625583188440782,0.687499999999916,0.718749999999873,
0.734374999999842,0.742187499999841,0.746930764461493,0.74999999999984,
0.798770062779461,0.846466169827735,0.892304506608502,0.936986645518803,
0.979989519974505,1.),.UNSPECIFIED.);
#4963=B_SPLINE_CURVE_WITH_KNOTS('',3,(#164000,#164001,#164002,#164003,#164004,
#164005,#164006,#164007,#164008,#164009,#164010,#164011,#164012,#164013,
#164014,#164015,#164016,#164017,#164018,#164019,#164020,#164021,#164022,
#164023,#164024,#164025,#164026,#164027,#164028,#164029,#164030,#164031,
#164032,#164033,#164034,#164035,#164036,#164037,#164038,#164039,#164040,
#164041,#164042,#164043,#164044,#164045,#164046,#164047,#164048,#164049,
#164050,#164051,#164052,#164053,#164054,#164055,#164056,#164057,#164058,
#164059,#164060,#164061,#164062,#164063,#164064,#164065,#164066,#164067,
#164068,#164069),.UNSPECIFIED.,.F.,.F.,(4,3,3,3,3,3,3,3,3,3,3,3,3,3,3,3,
3,3,3,3,3,3,3,4),(0.,0.0417433064021318,0.0856783503512316,0.125000000000202,
0.172058637042935,0.221141673238027,0.242187500000332,0.247530062045159,
0.250000000000331,0.258757699094845,0.318098755992443,0.375000000000289,
0.438761223626928,0.468750000000226,0.483267071980795,0.497350908913188,
0.500000000000198,0.586409574598886,0.674221064847019,0.743171333827662,
0.750000000000099,0.839284683852181,0.929619546736012,1.),.UNSPECIFIED.);
#4964=B_SPLINE_CURVE_WITH_KNOTS('',3,(#164092,#164093,#164094,#164095,#164096,
#164097,#164098),.UNSPECIFIED.,.F.,.F.,(4,3,4),(4.71238898038469,5.49778714378214,
6.28318530717959),.UNSPECIFIED.);
#4965=B_SPLINE_CURVE_WITH_KNOTS('',3,(#164100,#164101,#164102,#164103,#164104,
#164105,#164106,#164107,#164108,#164109,#164110,#164111,#164112,#164113,
#164114,#164115,#164116,#164117,#164118,#164119,#164120,#164121,#164122,
#164123,#164124,#164125,#164126,#164127,#164128,#164129,#164130,#164131,
#164132,#164133,#164134,#164135,#164136,#164137,#164138,#164139,#164140,
#164141,#164142,#164143,#164144,#164145,#164146,#164147,#164148,#164149,
#164150,#164151,#164152,#164153,#164154),.UNSPECIFIED.,.F.,.F.,(4,3,3,3,
3,3,3,3,3,3,3,3,3,3,3,3,3,3,4),(0.,0.104715580048555,0.210383983573989,
0.250000000000528,0.354011980382662,0.375000000000741,0.43750000000089,
0.468750000000963,0.484375000000993,0.49343925440917,0.500000000001023,
0.577747102398773,0.652041765008489,0.721927843163034,0.750000000000512,
0.814470107381001,0.877192615277638,0.938596307638819,1.),.UNSPECIFIED.);
#4966=B_SPLINE_CURVE_WITH_KNOTS('',3,(#164178,#164179,#164180,#164181,#164182,
#164183,#164184),.UNSPECIFIED.,.F.,.F.,(4,3,4),(1.23467863058847E-16,0.785398163397447,
1.5707963267949),.UNSPECIFIED.);
#4967=B_SPLINE_CURVE_WITH_KNOTS('',3,(#164187,#164188,#164189,#164190,#164191,
#164192,#164193,#164194,#164195,#164196,#164197,#164198,#164199,#164200,
#164201,#164202,#164203,#164204,#164205,#164206,#164207,#164208,#164209,
#164210,#164211,#164212,#164213,#164214,#164215,#164216,#164217,#164218,
#164219,#164220,#164221,#164222,#164223,#164224,#164225,#164226,#164227,
#164228,#164229,#164230,#164231,#164232),.UNSPECIFIED.,.F.,.F.,(4,3,3,3,
3,3,3,3,3,3,3,3,3,3,3,4),(0.,0.060546874999967,0.122426142535212,0.186284752990579,
0.245362452470406,0.322247692137301,0.39818940892974,0.475083013899954,
0.484374999999736,0.493930247601759,0.499999999999743,0.605247958737039,
0.71062864059231,0.816191187206391,0.922233553949779,1.),.UNSPECIFIED.);
#4968=B_SPLINE_CURVE_WITH_KNOTS('',3,(#164238,#164239,#164240,#164241,#164242,
#164243,#164244,#164245,#164246,#164247,#164248,#164249,#164250,#164251,
#164252,#164253,#164254,#164255,#164256,#164257,#164258,#164259,#164260,
#164261,#164262,#164263,#164264,#164265,#164266,#164267,#164268,#164269,
#164270,#164271,#164272,#164273,#164274,#164275,#164276,#164277,#164278,
#164279,#164280,#164281,#164282,#164283,#164284,#164285,#164286,#164287,
#164288,#164289,#164290,#164291,#164292,#164293,#164294,#164295,#164296,
#164297,#164298,#164299,#164300,#164301,#164302,#164303,#164304,#164305,
#164306,#164307),.UNSPECIFIED.,.F.,.F.,(4,3,3,3,3,3,3,3,3,3,3,3,3,3,3,3,
3,3,3,3,3,3,3,4),(0.,0.0417041814131079,0.0849340865860686,0.13082840629655,
0.178067342047349,0.227196348247942,0.242187499999745,0.247530062045447,
0.24999999999975,0.258757699094019,0.318098755985604,0.374999999999687,
0.438761223875019,0.468749999999677,0.483267071975172,0.497350908902079,
0.499999999999685,0.586409574537516,0.674221064733702,0.74317133380861,
0.749999999999842,0.839284683789798,0.929619546616256,1.),.UNSPECIFIED.);
#4969=B_SPLINE_CURVE_WITH_KNOTS('',3,(#164333,#164334,#164335,#164336,#164337,
#164338,#164339,#164340,#164341,#164342,#164343,#164344,#164345,#164346,
#164347,#164348,#164349,#164350,#164351,#164352,#164353,#164354,#164355,
#164356,#164357,#164358,#164359,#164360,#164361,#164362,#164363,#164364,
#164365,#164366,#164367,#164368,#164369,#164370,#164371,#164372,#164373,
#164374,#164375,#164376,#164377,#164378,#164379,#164380,#164381,#164382,
#164383,#164384,#164385,#164386,#164387,#164388,#164389,#164390,#164391,
#164392,#164393,#164394,#164395,#164396,#164397,#164398,#164399,#164400,
#164401,#164402),.UNSPECIFIED.,.F.,.F.,(4,3,3,3,3,3,3,3,3,3,3,3,3,3,3,3,
3,3,3,3,3,3,3,4),(0.,0.0904805865747593,0.179890948794643,0.250000000000156,
0.256840728511668,0.344945742473561,0.429509229825221,0.468750000000257,
0.482752596547783,0.497175643783503,0.500000000000261,0.56298906728729,
0.625000000000418,0.683994503650316,0.741245408290876,0.742187500000548,
0.746913732889895,0.750000000000554,0.799311389337984,0.849483542003488,
0.894712088307748,0.938468707034261,0.980197893082773,1.),.UNSPECIFIED.);
#4970=B_SPLINE_CURVE_WITH_KNOTS('',3,(#164431,#164432,#164433,#164434,#164435,
#164436,#164437,#164438,#164439,#164440,#164441,#164442,#164443),
 .UNSPECIFIED.,.F.,.F.,(4,3,3,3,4),(0.000775072234384454,0.00360015924840042,
0.0066511885691017,0.00786282367425579,0.0104581756611108),
 .UNSPECIFIED.);
#4971=B_SPLINE_CURVE_WITH_KNOTS('',3,(#164444,#164445,#164446,#164447,#164448,
#164449,#164450,#164451,#164452,#164453,#164454,#164455,#164456,#164457,
#164458,#164459,#164460,#164461,#164462,#164463,#164464,#164465,#164466,
#164467,#164468,#164469,#164470,#164471,#164472,#164473,#164474,#164475,
#164476,#164477,#164478,#164479,#164480,#164481,#164482,#164483,#164484,
#164485,#164486,#164487,#164488,#164489,#164490,#164491,#164492,#164493,
#164494,#164495,#164496,#164497,#164498,#164499,#164500,#164501,#164502,
#164503,#164504,#164505,#164506,#164507,#164508,#164509,#164510,#164511,
#164512,#164513,#164514,#164515,#164516,#164517,#164518,#164519,#164520,
#164521,#164522,#164523,#164524,#164525,#164526,#164527,#164528,#164529,
#164530,#164531,#164532,#164533,#164534),.UNSPECIFIED.,.F.,.F.,(4,3,3,3,
3,3,3,3,3,3,3,3,3,3,3,3,3,3,3,3,3,3,3,3,3,3,3,3,3,3,4),(0.,0.0625000000000528,
0.119882029542211,0.181191318326517,0.215595659163364,0.232797829581788,
0.241398914790999,0.245699457395605,0.246075569668044,0.246422124286298,
0.250000000000211,0.328341414165092,0.37500000000021,0.406250000000209,
0.437500000000209,0.468750000000208,0.484375000000208,0.492187500000204,
0.496093750000202,0.499312791455558,0.5000000000002,0.553910651984701,0.562500000000175,
0.609375000000156,0.67005767057599,0.723432332910554,0.7500000000001,0.823678063759278,
0.87500000000005,0.96075141168338,0.999994499179906),.UNSPECIFIED.);
#4972=B_SPLINE_CURVE_WITH_KNOTS('',3,(#164535,#164536,#164537,#164538,#164539,
#164540,#164541,#164542,#164543,#164544,#164545,#164546,#164547,#164548,
#164549,#164550,#164551,#164552,#164553,#164554,#164555,#164556,#164557,
#164558,#164559,#164560,#164561,#164562,#164563,#164564,#164565,#164566,
#164567,#164568,#164569,#164570,#164571,#164572,#164573,#164574,#164575,
#164576,#164577,#164578,#164579,#164580,#164581,#164582,#164583,#164584,
#164585,#164586,#164587,#164588,#164589,#164590,#164591,#164592,#164593,
#164594,#164595,#164596,#164597,#164598,#164599,#164600,#164601,#164602,
#164603,#164604,#164605,#164606,#164607,#164608,#164609,#164610,#164611,
#164612,#164613,#164614,#164615,#164616,#164617,#164618,#164619,#164620,
#164621,#164622,#164623,#164624,#164625,#164626,#164627,#164628,#164629,
#164630,#164631,#164632,#164633,#164634,#164635,#164636,#164637,#164638,
#164639,#164640),.UNSPECIFIED.,.F.,.F.,(4,3,3,3,3,3,3,3,3,3,3,3,3,3,3,3,
3,3,3,3,3,3,3,3,3,3,3,3,3,3,3,3,3,3,3,4),(6.04008760640985E-9,0.0631615253640654,
0.125000000000745,0.181057237407362,0.234824141910246,0.246093750001476,
0.249787108631666,0.250000000001502,0.252757249528496,0.360659948060548,
0.375000000002354,0.439765134614748,0.499023437503205,0.500000000003212,
0.507860695079115,0.541007150026823,0.574249368414924,0.607699600826058,
0.625000000002433,0.659336202062174,0.691632909124592,0.726096190864088,
0.743215178935082,0.747227441764222,0.747721138167026,0.748023769356437,
0.748174988831839,0.749158680281715,0.74964860473429,0.749947616638847,
0.750081406970028,0.802195408057856,0.855320680231657,0.909014588024604,
0.963580917838172,1.),.UNSPECIFIED.);
#4973=B_SPLINE_CURVE_WITH_KNOTS('',3,(#164661,#164662,#164663,#164664,#164665,
#164666,#164667,#164668,#164669,#164670,#164671,#164672,#164673,#164674,
#164675,#164676),.UNSPECIFIED.,.F.,.F.,(4,3,3,3,3,4),(0.000681462205008639,
0.00273329612790433,0.00491895821255326,0.00671017185179961,0.00912678453082223,
0.00930288319891504),.UNSPECIFIED.);
#4974=B_SPLINE_CURVE_WITH_KNOTS('',3,(#164678,#164679,#164680,#164681,#164682,
#164683,#164684,#164685,#164686,#164687,#164688,#164689,#164690,#164691,
#164692,#164693,#164694,#164695,#164696,#164697,#164698,#164699,#164700,
#164701,#164702,#164703,#164704,#164705,#164706,#164707,#164708,#164709,
#164710,#164711,#164712,#164713,#164714,#164715,#164716,#164717,#164718,
#164719,#164720,#164721,#164722,#164723,#164724,#164725,#164726,#164727,
#164728,#164729,#164730,#164731,#164732,#164733,#164734,#164735,#164736,
#164737,#164738,#164739,#164740,#164741,#164742,#164743,#164744,#164745,
#164746,#164747,#164748,#164749,#164750,#164751,#164752,#164753,#164754,
#164755,#164756,#164757,#164758,#164759,#164760,#164761,#164762,#164763,
#164764,#164765,#164766,#164767,#164768,#164769,#164770,#164771,#164772,
#164773,#164774,#164775,#164776,#164777,#164778,#164779,#164780,#164781,
#164782,#164783),.UNSPECIFIED.,.F.,.F.,(4,3,3,3,3,3,3,3,3,3,3,3,3,3,3,3,
3,3,3,3,3,3,3,3,3,3,3,3,3,3,3,3,3,3,3,4),(0.,0.0786487036192077,0.140954525450891,
0.195477262726112,0.222738631363722,0.236369315682527,0.24318465784193,
0.246592328921631,0.247444246691557,0.247763715855279,0.24797366756617,
0.2481420722479,0.250000000001332,0.28832882578824,0.326567472140649,0.364722818248368,
0.402831690846228,0.440266729938598,0.478356316773867,0.496093750000979,
0.499612062949285,0.50000000000097,0.554876643694226,0.611930537520896,
0.625000000000741,0.684310971889722,0.687500000000626,0.718750000000563,
0.734375000000532,0.742187500000516,0.746093750000507,0.750000000000499,
0.823764329859907,0.899903185373135,0.979642186186956,0.999986903780746),
 .UNSPECIFIED.);
#4975=B_SPLINE_CURVE_WITH_KNOTS('',3,(#164785,#164786,#164787,#164788,#164789,
#164790,#164791,#164792,#164793,#164794,#164795,#164796,#164797,#164798,
#164799,#164800),.UNSPECIFIED.,.F.,.F.,(4,3,3,3,3,4),(0.,0.199145041073045,
0.413635430144668,0.625526552290449,0.851258415695788,0.999999434617583),
 .UNSPECIFIED.);
#4976=B_SPLINE_CURVE_WITH_KNOTS('',3,(#164801,#164802,#164803,#164804,#164805,
#164806,#164807,#164808,#164809,#164810,#164811,#164812,#164813,#164814,
#164815,#164816,#164817,#164818,#164819,#164820,#164821,#164822,#164823,
#164824,#164825,#164826,#164827,#164828,#164829,#164830,#164831,#164832,
#164833,#164834,#164835,#164836,#164837,#164838,#164839,#164840,#164841,
#164842,#164843,#164844,#164845,#164846,#164847,#164848,#164849,#164850,
#164851,#164852,#164853,#164854,#164855,#164856,#164857,#164858,#164859,
#164860,#164861,#164862,#164863,#164864,#164865,#164866,#164867,#164868,
#164869,#164870,#164871,#164872,#164873,#164874,#164875,#164876,#164877,
#164878,#164879,#164880,#164881,#164882,#164883,#164884,#164885,#164886,
#164887,#164888),.UNSPECIFIED.,.F.,.F.,(4,3,3,3,3,3,3,3,3,3,3,3,3,3,3,3,
3,3,3,3,3,3,3,3,3,3,3,3,3,4),(1.10570935039285E-8,0.0831077289908478,0.125000000000325,
0.192214037137834,0.246093750000652,0.250000000000664,0.251900676065446,
0.332426051101153,0.375000000000854,0.443871170179604,0.49804687500106,
0.500000000001065,0.502961890600083,0.537631002255159,0.562500000000996,
0.599948155247652,0.625000000000926,0.658190763311687,0.687500000000856,
0.718750000000822,0.734375000000804,0.742187500000796,0.746093750000792,
0.74804687500079,0.750000000000787,0.751057688908144,0.823026195316543,
0.8946442291177,0.965792345222205,1.),.UNSPECIFIED.);
#4977=B_SPLINE_CURVE_WITH_KNOTS('',3,(#164900,#164901,#164902,#164903,#164904,
#164905,#164906,#164907,#164908,#164909,#164910,#164911,#164912,#164913,
#164914,#164915,#164916,#164917,#164918,#164919,#164920,#164921,#164922,
#164923,#164924,#164925,#164926,#164927,#164928,#164929,#164930,#164931,
#164932,#164933,#164934,#164935,#164936,#164937,#164938,#164939),
 .UNSPECIFIED.,.F.,.F.,(4,3,3,3,3,3,3,3,3,3,3,3,3,4),(0.,0.125000000000011,
0.250000000000021,0.37500000000003,0.437500000000033,0.468750000000031,
0.487324584826517,0.500000000000029,0.500520266105271,0.602937076851582,
0.707582462658716,0.811875894948651,0.913121167622829,1.),.UNSPECIFIED.);
#4978=B_SPLINE_CURVE_WITH_KNOTS('',3,(#164974,#164975,#164976,#164977,#164978,
#164979,#164980,#164981,#164982,#164983,#164984,#164985,#164986,#164987,
#164988,#164989),.UNSPECIFIED.,.F.,.F.,(4,3,3,3,3,4),(0.,0.19107940674639,
0.393309555059792,0.593827441197275,0.800859069985332,1.),.UNSPECIFIED.);
#4979=B_SPLINE_CURVE_WITH_KNOTS('',3,(#164992,#164993,#164994,#164995),
 .UNSPECIFIED.,.F.,.F.,(4,4),(0.,0.0174508326761739),.UNSPECIFIED.);
#4980=B_SPLINE_CURVE_WITH_KNOTS('',3,(#165022,#165023,#165024,#165025,#165026,
#165027,#165028,#165029,#165030,#165031,#165032,#165033,#165034,#165035,
#165036,#165037,#165038,#165039,#165040,#165041,#165042,#165043,#165044,
#165045,#165046,#165047,#165048,#165049),.UNSPECIFIED.,.F.,.F.,(4,3,3,3,
3,3,3,3,3,4),(0.,0.000662679024145193,0.00128919539297031,0.00132535804829039,
0.0019349250888321,0.00253635637124923,0.00265071609658077,0.00397607414487116,
0.00508368314703509,0.00530143219316154),.UNSPECIFIED.);
#4981=B_SPLINE_CURVE_WITH_KNOTS('',3,(#165080,#165081,#165082,#165083,#165084,
#165085,#165086,#165087,#165088,#165089,#165090,#165091,#165092,#165093,
#165094,#165095),.UNSPECIFIED.,.F.,.F.,(4,3,3,3,3,4),(0.,0.00121734210059923,
0.00132677154899614,0.00265354309799227,0.00411654704464365,0.00530708619598447),
 .UNSPECIFIED.);
#4982=B_SPLINE_CURVE_WITH_KNOTS('',3,(#165110,#165111,#165112,#165113),
 .UNSPECIFIED.,.F.,.F.,(4,4),(0.,0.0177264565684136),.UNSPECIFIED.);
#4983=B_SPLINE_CURVE_WITH_KNOTS('',3,(#165140,#165141,#165142,#165143,#165144,
#165145,#165146,#165147,#165148,#165149,#165150,#165151,#165152),
 .UNSPECIFIED.,.F.,.F.,(4,3,3,3,4),(0.,0.000168209862994577,0.000320350766922646,
0.000480537459018489,0.000640701533845293),.UNSPECIFIED.);
#4984=B_SPLINE_CURVE_WITH_KNOTS('',3,(#165311,#165312,#165313,#165314,#165315,
#165316,#165317,#165318,#165319,#165320,#165321,#165322,#165323,#165324,
#165325,#165326,#165327,#165328,#165329,#165330,#165331,#165332),
 .UNSPECIFIED.,.F.,.F.,(4,3,3,3,3,3,3,4),(0.,0.000110166739482577,0.000232250654978379,
0.000327614165524935,0.000415934063629706,0.000506222853831825,0.000594954171387356,
0.000655228331049871),.UNSPECIFIED.);
#4985=B_SPLINE_CURVE_WITH_KNOTS('',3,(#165347,#165348,#165349,#165350),
 .UNSPECIFIED.,.F.,.F.,(4,4),(0.,0.0138038180377133),.UNSPECIFIED.);
#4986=B_SPLINE_CURVE_WITH_KNOTS('',3,(#165377,#165378,#165379,#165380,#165381,
#165382,#165383,#165384,#165385,#165386,#165387,#165388,#165389,#165390,
#165391,#165392,#165393,#165394,#165395),.UNSPECIFIED.,.F.,.F.,(4,3,3,3,
3,3,4),(0.,0.00115159118172271,0.00227058783087512,0.00281251499795634,
0.00421877249693456,0.00530146752106949,0.00562502999591277),
 .UNSPECIFIED.);
#4987=B_SPLINE_CURVE_WITH_KNOTS('',3,(#165426,#165427,#165428,#165429,#165430,
#165431,#165432,#165433,#165434,#165435,#165436,#165437,#165438,#165439,
#165440,#165441),.UNSPECIFIED.,.F.,.F.,(4,3,3,3,3,4),(0.,0.00116086488263883,
0.0014075250438046,0.0028150500876092,0.00432397808186733,0.00563010017521834),
 .UNSPECIFIED.);
#4988=B_SPLINE_CURVE_WITH_KNOTS('',3,(#165456,#165457,#165458,#165459),
 .UNSPECIFIED.,.F.,.F.,(4,4),(0.,0.0135258923233721),.UNSPECIFIED.);
#4989=B_SPLINE_CURVE_WITH_KNOTS('',3,(#165480,#165481,#165482,#165483,#165484,
#165485,#165486,#165487,#165488,#165489,#165490,#165491,#165492,#165493,
#165494,#165495),.UNSPECIFIED.,.F.,.F.,(4,3,3,3,3,4),(0.,0.00019794317692089,
0.000328605151068823,0.000446042787173756,0.000552633627937672,0.000657210302137648),
 .UNSPECIFIED.);
#4990=B_SPLINE_CURVE_WITH_KNOTS('',3,(#165498,#165499,#165500,#165501,#165502,
#165503,#165504,#165505,#165506,#165507,#165508,#165509,#165510,#165511,
#165512,#165513,#165514,#165515,#165516,#165517,#165518,#165519,#165520,
#165521,#165522,#165523,#165524,#165525,#165526,#165527,#165528,#165529,
#165530,#165531,#165532,#165533,#165534,#165535,#165536,#165537,#165538,
#165539,#165540,#165541,#165542,#165543,#165544,#165545,#165546,#165547,
#165548,#165549,#165550,#165551,#165552,#165553,#165554,#165555,#165556,
#165557,#165558,#165559,#165560,#165561,#165562,#165563,#165564,#165565,
#165566,#165567,#165568,#165569,#165570,#165571,#165572,#165573),
 .UNSPECIFIED.,.F.,.F.,(4,3,3,3,3,3,3,3,3,3,3,3,3,3,3,3,3,3,3,3,3,3,3,3,
3,4),(0.,0.0971694717327587,0.124999999999839,0.187499999999759,0.249999999999678,
0.337621660100129,0.374999999999518,0.437499999999443,0.468749999999418,
0.484374999999408,0.494411509442002,0.499999999999398,0.516541470396192,
0.603517981247307,0.624999999999403,0.687499999999395,0.718749999999381,
0.734374999999381,0.742187499999374,0.748133238950809,0.749999999999367,
0.804479122806833,0.85884481476214,0.912694297575866,0.965054460214556,
1.),.UNSPECIFIED.);
#4991=B_SPLINE_CURVE_WITH_KNOTS('',3,(#165583,#165584,#165585,#165586,#165587,
#165588,#165589,#165590,#165591,#165592,#165593,#165594,#165595,#165596,
#165597,#165598,#165599,#165600,#165601,#165602,#165603,#165604,#165605,
#165606,#165607,#165608,#165609,#165610,#165611,#165612,#165613,#165614,
#165615,#165616,#165617,#165618,#165619,#165620,#165621,#165622,#165623,
#165624,#165625,#165626,#165627,#165628,#165629,#165630,#165631,#165632,
#165633,#165634,#165635,#165636,#165637,#165638,#165639,#165640,#165641,
#165642,#165643,#165644,#165645,#165646,#165647,#165648,#165649,#165650,
#165651,#165652),.UNSPECIFIED.,.F.,.F.,(4,3,3,3,3,3,3,3,3,3,3,3,3,3,3,3,
3,3,3,3,3,3,3,4),(0.,0.0468928010521469,0.0624999999999663,0.11173734352247,
0.162092700602332,0.215593455071074,0.234374999999845,0.242187499999848,
0.248562191291075,0.24999999999985,0.328344811834936,0.374999999999854,
0.431665597222767,0.468940652178127,0.478556608155973,0.484374999999853,
0.494460980872878,0.499999999999851,0.57484627083378,0.653167719012279,
0.717622076559044,0.805768836993062,0.902884418496531,1.),.UNSPECIFIED.);
#4992=B_SPLINE_CURVE_WITH_KNOTS('',3,(#165696,#165697,#165698,#165699,#165700,
#165701,#165702,#165703,#165704,#165705,#165706,#165707,#165708,#165709,
#165710,#165711,#165712,#165713,#165714),.UNSPECIFIED.,.F.,.F.,(4,3,3,3,
3,3,4),(0.,0.00017507392680495,0.000350193522739415,0.000452577371514132,
0.000557835767991203,0.000662370656289507,0.000700387045478831),
 .UNSPECIFIED.);
#4993=B_SPLINE_CURVE_WITH_KNOTS('',3,(#165771,#165772,#165773,#165774,#165775,
#165776,#165777,#165778,#165779,#165780,#165781,#165782,#165783,#165784,
#165785,#165786,#165787,#165788,#165789),.UNSPECIFIED.,.F.,.F.,(4,3,3,3,
3,3,4),(0.,0.00157595519506122,0.00315191039012244,0.00393988798770612,
0.00472786558518367,0.00575007285732184,0.00630382078024489),
 .UNSPECIFIED.);
#4994=B_SPLINE_CURVE_WITH_KNOTS('',3,(#165827,#165828,#165829,#165830,#165831,
#165832,#165833,#165834,#165835,#165836,#165837,#165838,#165839,#165840,
#165841,#165842),.UNSPECIFIED.,.F.,.F.,(4,3,3,3,3,4),(0.,0.00104430221452871,
0.00157688090361367,0.00315376180722735,0.00473064271084103,0.00630752361445471),
 .UNSPECIFIED.);
#4995=B_SPLINE_CURVE_WITH_KNOTS('',3,(#165893,#165894,#165895,#165896,#165897,
#165898,#165899,#165900,#165901,#165902,#165903,#165904,#165905),
 .UNSPECIFIED.,.F.,.F.,(4,3,3,3,4),(0.,0.000175209888250467,0.000350428553470057,
0.000525662295915607,0.000700857106940114),.UNSPECIFIED.);
#4996=B_SPLINE_CURVE_WITH_KNOTS('',3,(#166018,#166019,#166020,#166021,#166022,
#166023,#166024,#166025,#166026,#166027,#166028,#166029,#166030,#166031,
#166032,#166033,#166034,#166035,#166036,#166037,#166038,#166039,#166040,
#166041,#166042,#166043,#166044,#166045),.UNSPECIFIED.,.F.,.F.,(4,3,3,3,
3,3,3,3,3,4),(0.,0.000297352361641552,0.000685187759872985,0.000685314779244029,
0.00137061382937429,0.00137062955848806,0.00183455251928066,0.00205619372744575,
0.00244930001359525,0.00274125911697611),.UNSPECIFIED.);
#4997=B_SPLINE_CURVE_WITH_KNOTS('',3,(#166048,#166049,#166050,#166051,#166052,
#166053,#166054,#166055,#166056,#166057,#166058,#166059,#166060,#166061,
#166062,#166063,#166064,#166065,#166066,#166067,#166068,#166069,#166070,
#166071,#166072,#166073),.UNSPECIFIED.,.F.,.F.,(4,2,2,2,2,2,2,2,2,2,2,2,
4),(0.,0.0308819193980004,0.0647401130039136,0.0887784724853781,0.122010977792549,
0.1412175368743,0.146061445002154,0.16477491817878,0.172906057208515,0.180478634262882,
0.208285706571513,0.24737159603407,0.282492401310004),.UNSPECIFIED.);
#4998=B_SPLINE_CURVE_WITH_KNOTS('',3,(#166151,#166152,#166153,#166154),
 .UNSPECIFIED.,.F.,.F.,(4,4),(0.,0.000120540380538642),.UNSPECIFIED.);
#4999=B_SPLINE_CURVE_WITH_KNOTS('',3,(#166175,#166176,#166177,#166178,#166179,
#166180,#166181),.UNSPECIFIED.,.F.,.F.,(4,3,4),(0.,0.0128929585057523,0.0257859170115047),
 .UNSPECIFIED.);
#5000=B_SPLINE_CURVE_WITH_KNOTS('',3,(#166208,#166209,#166210,#166211,#166212,
#166213,#166214,#166215,#166216,#166217,#166218,#166219,#166220,#166221,
#166222,#166223),.UNSPECIFIED.,.F.,.F.,(4,3,3,3,3,4),(0.,0.00113243548370091,
0.00226487096740181,0.00339730645110275,0.00441932320149626,0.0045297419348037),
 .UNSPECIFIED.);
#5001=B_SPLINE_CURVE_WITH_KNOTS('',3,(#166248,#166249,#166250,#166251,#166252,
#166253,#166254,#166255,#166256,#166257,#166258,#166259,#166260,#166261,
#166262,#166263,#166264,#166265,#166266,#166267,#166268,#166269,#166270,
#166271,#166272),.UNSPECIFIED.,.F.,.F.,(4,3,3,3,3,3,3,3,4),(0.,0.000394684030928064,
0.000806360979195566,0.00113421626089741,0.0016450747730102,0.00217582874625842,
0.00226843252179482,0.0036130177168745,0.00453686504358963),
 .UNSPECIFIED.);
#5002=B_SPLINE_CURVE_WITH_KNOTS('',3,(#166294,#166295,#166296,#166297,#166298,
#166299,#166300,#166301,#166302,#166303,#166304,#166305,#166306,#166307,
#166308,#166309,#166310,#166311,#166312,#166313,#166314,#166315,#166316,
#166317,#166318,#166319,#166320,#166321),.UNSPECIFIED.,.F.,.F.,(4,3,3,3,
3,3,3,3,3,4),(0.,0.147232559566058,0.290903059743303,0.430985431195598,
0.498046874999703,0.499959580131913,0.499999999999702,0.672084672956296,
0.838421918110885,1.),.UNSPECIFIED.);
#5003=B_SPLINE_CURVE_WITH_KNOTS('',3,(#166322,#166323,#166324,#166325,#166326,
#166327,#166328),.UNSPECIFIED.,.F.,.F.,(4,3,4),(0.,0.0127570403976527,0.0255140807953054),
 .UNSPECIFIED.);
#5004=B_SPLINE_CURVE_WITH_KNOTS('',3,(#166364,#166365,#166366,#166367,#166368,
#166369,#166370,#166371,#166372,#166373,#166374,#166375,#166376),
 .UNSPECIFIED.,.F.,.F.,(4,3,3,3,4),(0.,0.000259173930192671,0.000518347860385342,
0.000877297766812356,0.00103669572077068),.UNSPECIFIED.);
#5005=B_SPLINE_CURVE_WITH_KNOTS('',3,(#166407,#166408,#166409,#166410,#166411,
#166412,#166413,#166414,#166415,#166416,#166417,#166418,#166419,#166420,
#166421,#166422),.UNSPECIFIED.,.F.,.F.,(4,2,2,2,1,1,2,2,4),(0.,0.249999999999956,
0.374999999999936,0.437499999999936,0.468749999999936,0.484374999999931,
0.492187499999936,0.49999999999994,1.),.UNSPECIFIED.);
#5006=B_SPLINE_CURVE_WITH_KNOTS('',3,(#166423,#166424,#166425,#166426,#166427,
#166428,#166429,#166430,#166431,#166432,#166433,#166434,#166435,#166436,
#166437,#166438,#166439,#166440,#166441),.UNSPECIFIED.,.F.,.F.,(4,3,3,3,
3,3,4),(0.,0.000108019327761347,0.000159670358772896,0.000279016064561974,
0.000319662760640411,0.000479499943955599,0.000639325521280822),
 .UNSPECIFIED.);
#5007=B_SPLINE_CURVE_WITH_KNOTS('',3,(#166492,#166493,#166494,#166495,#166496,
#166497,#166498,#166499,#166500,#166501,#166502,#166503,#166504,#166505,
#166506,#166507,#166508,#166509,#166510,#166511,#166512,#166513,#166514,
#166515,#166516,#166517,#166518,#166519,#166520,#166521,#166522,#166523,
#166524,#166525,#166526,#166527,#166528,#166529,#166530,#166531,#166532,
#166533,#166534,#166535,#166536,#166537,#166538,#166539,#166540,#166541,
#166542,#166543,#166544,#166545,#166546),.UNSPECIFIED.,.F.,.F.,(4,3,3,3,
3,3,3,3,3,3,3,3,3,3,3,3,3,3,4),(0.,0.0629468896977532,0.127653253164506,
0.194231548280777,0.263838668437689,0.335209452936689,0.40915172120043,
0.437500000000475,0.4687500000005,0.484375000000496,0.492187500000494,0.498659258613318,
0.500000000000492,0.593366456738352,0.68839728589612,0.786023585231411,
0.885234101519568,0.986766500565735,1.),.UNSPECIFIED.);
#5008=B_SPLINE_CURVE_WITH_KNOTS('',3,(#166549,#166550,#166551,#166552,#166553,
#166554,#166555,#166556,#166557,#166558,#166559,#166560,#166561,#166562,
#166563,#166564,#166565,#166566,#166567,#166568,#166569,#166570),
 .UNSPECIFIED.,.F.,.F.,(4,3,3,3,3,3,3,4),(0.,0.00011068335808725,0.000233265503180217,
0.000327042610606244,0.000415140332124215,0.000505188540440904,0.000593686275839362,
0.000654085221212487),.UNSPECIFIED.);
#5009=B_SPLINE_CURVE_WITH_KNOTS('',3,(#166585,#166586,#166587,#166588),
 .UNSPECIFIED.,.F.,.F.,(4,4),(0.,0.0138879247081574),.UNSPECIFIED.);
#5010=B_SPLINE_CURVE_WITH_KNOTS('',3,(#166615,#166616,#166617,#166618,#166619,
#166620,#166621,#166622,#166623,#166624,#166625,#166626,#166627,#166628,
#166629,#166630,#166631,#166632,#166633),.UNSPECIFIED.,.F.,.F.,(4,3,3,3,
3,3,4),(0.,0.00107929064721622,0.00212940062359847,0.00279822589210569,
0.00419733883815853,0.00528234680577585,0.00559645178421137),
 .UNSPECIFIED.);
#5011=B_SPLINE_CURVE_WITH_KNOTS('',3,(#166664,#166665,#166666,#166667,#166668,
#166669,#166670,#166671,#166672,#166673,#166674,#166675,#166676,#166677,
#166678,#166679),.UNSPECIFIED.,.F.,.F.,(4,3,3,3,3,4),(0.,0.00116583085671967,
0.00140039358904036,0.00280078717808072,0.00430574563588143,0.00560157435616136),
 .UNSPECIFIED.);
#5012=B_SPLINE_CURVE_WITH_KNOTS('',3,(#166694,#166695,#166696,#166697),
 .UNSPECIFIED.,.F.,.F.,(4,4),(0.,0.0141656229616797),.UNSPECIFIED.);
#5013=B_SPLINE_CURVE_WITH_KNOTS('',3,(#166718,#166719,#166720,#166721,#166722,
#166723,#166724,#166725,#166726,#166727,#166728,#166729,#166730,#166731,
#166732,#166733),.UNSPECIFIED.,.F.,.F.,(4,3,3,3,3,4),(0.,0.000193094254403281,
0.000327589980483358,0.000444218816713235,0.000550274313879027,0.000655179960966716),
 .UNSPECIFIED.);
#5014=B_SPLINE_CURVE_WITH_KNOTS('',3,(#166893,#166894,#166895,#166896,#166897,
#166898,#166899,#166900,#166901,#166902,#166903,#166904,#166905,#166906,
#166907,#166908,#166909,#166910,#166911),.UNSPECIFIED.,.F.,.F.,(4,3,3,3,
3,3,4),(0.,0.000108634712274956,0.000159257284564388,0.000279020961387661,
0.000318828120207844,0.000478248046436968,0.000637656240415689),
 .UNSPECIFIED.);
#5015=B_SPLINE_CURVE_WITH_KNOTS('',3,(#166926,#166927,#166928,#166929),
 .UNSPECIFIED.,.F.,.F.,(4,4),(0.,0.0180689587739334),.UNSPECIFIED.);
#5016=B_SPLINE_CURVE_WITH_KNOTS('',3,(#166962,#166963,#166964,#166965,#166966,
#166967,#166968,#166969,#166970,#166971,#166972,#166973,#166974,#166975,
#166976,#166977),.UNSPECIFIED.,.F.,.F.,(4,3,3,3,3,4),(0.,0.0013179209674593,
0.00263584193491861,0.00395376290237792,0.00506352109384539,0.00527168386983722),
 .UNSPECIFIED.);
#5017=B_SPLINE_CURVE_WITH_KNOTS('',3,(#167008,#167009,#167010,#167011,#167012,
#167013,#167014,#167015,#167016,#167017,#167018,#167019,#167020,#167021,
#167022,#167023),.UNSPECIFIED.,.F.,.F.,(4,3,3,3,3,4),(0.,0.00122256915433042,
0.0013193477680122,0.00263869553602439,0.00409736884770778,0.00527739107204874),
 .UNSPECIFIED.);
#5018=B_SPLINE_CURVE_WITH_KNOTS('',3,(#167038,#167039,#167040,#167041),
 .UNSPECIFIED.,.F.,.F.,(4,4),(0.,0.0177935197894076),.UNSPECIFIED.);
#5019=B_SPLINE_CURVE_WITH_KNOTS('',3,(#167044,#167045,#167046,#167047,#167048,
#167049,#167050,#167051,#167052,#167053,#167054,#167055,#167056,#167057,
#167058,#167059,#167060,#167061,#167062),.UNSPECIFIED.,.F.,.F.,(4,3,3,3,
3,3,4),(0.,0.206413742690837,0.405311323110467,0.600590525300877,0.800295262650439,
0.987977524790166,1.),.UNSPECIFIED.);
#5020=B_SPLINE_CURVE_WITH_KNOTS('',3,(#167096,#167097,#167098,#167099,#167100,
#167101,#167102,#167103,#167104,#167105,#167106,#167107,#167108),
 .UNSPECIFIED.,.F.,.F.,(4,3,3,3,4),(0.,0.000166958822900708,0.000319870924789836,
0.000479817604858628,0.000639741849579673),.UNSPECIFIED.);
#5021=B_SPLINE_CURVE_WITH_KNOTS('',3,(#167109,#167110,#167111,#167112,#167113,
#167114,#167115,#167116,#167117,#167118,#167119,#167120,#167121,#167122,
#167123,#167124,#167125,#167126,#167127,#167128,#167129,#167130,#167131,
#167132,#167133,#167134,#167135,#167136,#167137,#167138,#167139,#167140,
#167141,#167142,#167143,#167144,#167145,#167146,#167147,#167148,#167149,
#167150,#167151,#167152,#167153,#167154,#167155,#167156,#167157,#167158,
#167159,#167160,#167161,#167162,#167163,#167164,#167165,#167166,#167167,
#167168,#167169,#167170,#167171,#167172,#167173,#167174,#167175,#167176,
#167177,#167178,#167179,#167180,#167181,#167182,#167183,#167184),
 .UNSPECIFIED.,.F.,.F.,(4,3,3,3,3,3,3,3,3,3,3,3,3,3,3,3,3,3,3,3,3,3,3,3,
3,4),(0.,0.087049194558667,0.124999999999871,0.198958822720699,0.245113667123151,
0.272917645441527,0.326518624903113,0.365109832712131,0.399526497461392,
0.484374999999516,0.49449736054903,0.499999999999496,0.513989113488382,
0.598906346294231,0.62499999999941,0.687499999999356,0.718749999999328,
0.734374999999315,0.742187499999308,0.748148548384524,0.749999999999301,
0.804506513683484,0.858475482518048,0.911683608185878,0.963118260439554,
1.),.UNSPECIFIED.);
#5022=B_SPLINE_CURVE_WITH_KNOTS('',3,(#167188,#167189,#167190,#167191,#167192,
#167193,#167194,#167195,#167196,#167197,#167198,#167199,#167200,#167201,
#167202,#167203,#167204,#167205,#167206,#167207,#167208,#167209,#167210,
#167211,#167212,#167213,#167214,#167215),.UNSPECIFIED.,.F.,.F.,(4,3,3,3,
3,3,3,3,3,4),(0.,0.164413128193527,0.334088671484012,0.498046875000089,
0.500000000000089,0.500035489066017,0.639686048889431,0.781957047690301,
0.928621019402901,1.),.UNSPECIFIED.);
#5023=B_SPLINE_CURVE_WITH_KNOTS('',3,(#167245,#167246,#167247,#167248,#167249,
#167250,#167251,#167252,#167253,#167254,#167255,#167256,#167257),
 .UNSPECIFIED.,.F.,.F.,(4,3,3,3,4),(0.,0.287427955658528,0.570428246820337,
0.848327210027682,1.),.UNSPECIFIED.);
#5024=B_SPLINE_CURVE_WITH_KNOTS('',3,(#167293,#167294,#167295,#167296,#167297,
#167298,#167299),.UNSPECIFIED.,.F.,.F.,(4,3,4),(0.,0.0129055642122842,0.0258111284245685),
 .UNSPECIFIED.);
#5025=B_SPLINE_CURVE_WITH_KNOTS('',3,(#167326,#167327,#167328,#167329,#167330,
#167331,#167332,#167333,#167334,#167335,#167336,#167337,#167338,#167339,
#167340,#167341),.UNSPECIFIED.,.F.,.F.,(4,3,3,3,3,4),(0.,0.00112455173535831,
0.00224910347071663,0.00337365520607496,0.00439646903552834,0.0044982069414333),
 .UNSPECIFIED.);
#5026=B_SPLINE_CURVE_WITH_KNOTS('',3,(#167366,#167367,#167368,#167369,#167370,
#167371,#167372,#167373,#167374,#167375,#167376,#167377,#167378,#167379,
#167380,#167381,#167382,#167383,#167384,#167385,#167386,#167387,#167388,
#167389,#167390),.UNSPECIFIED.,.F.,.F.,(4,3,3,3,3,3,3,3,4),(0.,0.000393685585946579,
0.000804157569269683,0.00112634951454785,0.00164227212955572,0.00217802033015107,
0.0022526990290957,0.0035921705044767,0.00450539805819141),
 .UNSPECIFIED.);
#5027=B_SPLINE_CURVE_WITH_KNOTS('',3,(#167411,#167412,#167413,#167414,#167415,
#167416,#167417),.UNSPECIFIED.,.F.,.F.,(4,3,4),(0.,0.0130414224518927,0.0260828449037854),
 .UNSPECIFIED.);
#5028=B_SPLINE_CURVE_WITH_KNOTS('',3,(#167432,#167433,#167434,#167435),
 .UNSPECIFIED.,.F.,.F.,(4,4),(0.,0.000106239733749475),.UNSPECIFIED.);
#5029=B_SPLINE_CURVE_WITH_KNOTS('',3,(#167456,#167457,#167458,#167459,#167460,
#167461,#167462,#167463,#167464,#167465,#167466,#167467,#167468),
 .UNSPECIFIED.,.F.,.F.,(4,3,3,3,4),(0.,0.000360360286228923,0.000488761174293949,
0.000765042797560336,0.000977522348587897),.UNSPECIFIED.);
#5030=B_SPLINE_CURVE_WITH_KNOTS('',3,(#167580,#167581,#167582,#167583,#167584,
#167585,#167586,#167587,#167588,#167589,#167590,#167591,#167592,#167593,
#167594,#167595,#167596,#167597,#167598),.UNSPECIFIED.,.F.,.F.,(4,3,3,3,
3,3,4),(0.,0.000417356154990511,0.000834652124500517,0.000834737818312929,
0.00125222696221769,0.00161112215869395,0.00166930424900103),
 .UNSPECIFIED.);
#5031=B_SPLINE_CURVE_WITH_KNOTS('',3,(#167602,#167603,#167604,#167605,#167606,
#167607,#167608,#167609),.UNSPECIFIED.,.F.,.F.,(4,2,2,4),(0.,0.0307530884815225,
0.0629270182301273,0.0847650334152431),.UNSPECIFIED.);
#5032=B_SPLINE_CURVE_WITH_KNOTS('',3,(#167610,#167611,#167612,#167613,#167614,
#167615,#167616,#167617),.UNSPECIFIED.,.F.,.F.,(4,2,2,4),(0.0847654430259031,
0.106611941487456,0.138792065252627,0.169530887592823),.UNSPECIFIED.);
#5033=B_SPLINE_CURVE_WITH_KNOTS('',3,(#167622,#167623,#167624,#167625,#167626,
#167627,#167628,#167629,#167630,#167631,#167632,#167633,#167634,#167635,
#167636,#167637,#167638,#167639,#167640,#167641,#167642,#167643,#167644,
#167645,#167646,#167647,#167648,#167649,#167650,#167651,#167652,#167653,
#167654,#167655,#167656,#167657,#167658),.UNSPECIFIED.,.F.,.F.,(4,3,3,3,
3,3,3,3,3,3,3,3,4),(0.,0.11441361461611,0.227673917164459,0.343130048663463,
0.437499999999992,0.465087007106255,0.496480388221911,0.499999999999997,
0.590811089022654,0.685064677202165,0.785221931931703,0.892701183249464,
1.),.UNSPECIFIED.);
#5034=B_SPLINE_CURVE_WITH_KNOTS('',3,(#167702,#167703,#167704,#167705,#167706,
#167707,#167708,#167709,#167710,#167711,#167712,#167713,#167714,#167715,
#167716,#167717,#167718,#167719,#167720),.UNSPECIFIED.,.F.,.F.,(4,3,3,3,
3,3,4),(0.,0.000174255415100464,0.000348555105993215,0.000449985369487469,
0.000554229835728735,0.000657719249454963,0.000697110211986431),
 .UNSPECIFIED.);
#5035=B_SPLINE_CURVE_WITH_KNOTS('',3,(#167777,#167778,#167779,#167780,#167781,
#167782,#167783,#167784,#167785,#167786,#167787,#167788,#167789,#167790,
#167791,#167792,#167793,#167794,#167795),.UNSPECIFIED.,.F.,.F.,(4,3,3,3,
3,3,4),(0.,0.00156956785490461,0.00313913570980923,0.00392391963731218,
0.00470870356471384,0.00573336346876343,0.00627827141961845),
 .UNSPECIFIED.);
#5036=B_SPLINE_CURVE_WITH_KNOTS('',3,(#167832,#167833,#167834,#167835,#167836,
#167837,#167838,#167839,#167840,#167841,#167842,#167843,#167844,#167845,
#167846,#167847),.UNSPECIFIED.,.F.,.F.,(4,3,3,3,3,4),(0.,0.00104863959929747,
0.00157050793024954,0.00314101586049909,0.00471152379074863,0.00628203172099817),
 .UNSPECIFIED.);
#5037=B_SPLINE_CURVE_WITH_KNOTS('',3,(#167899,#167900,#167901,#167902,#167903,
#167904,#167905,#167906,#167907,#167908,#167909,#167910,#167911,#167912,
#167913,#167914,#167915,#167916,#167917,#167918,#167919,#167920,#167921,
#167922,#167923,#167924,#167925,#167926,#167927,#167928,#167929,#167930,
#167931,#167932,#167933,#167934,#167935,#167936,#167937,#167938,#167939,
#167940,#167941,#167942,#167943,#167944,#167945,#167946,#167947,#167948,
#167949,#167950,#167951,#167952,#167953,#167954,#167955,#167956,#167957,
#167958,#167959,#167960,#167961,#167962,#167963,#167964,#167965,#167966,
#167967,#167968,#167969,#167970,#167971,#167972,#167973,#167974,#167975,
#167976,#167977),.UNSPECIFIED.,.F.,.F.,(4,3,3,3,3,3,3,3,3,3,3,3,3,3,3,3,
3,3,3,3,3,3,3,3,3,3,4),(0.,0.0823558144348623,0.12499999999997,0.203651427244223,
0.249243429408674,0.282302854488475,0.332820890866331,0.364919347441214,
0.394174559507633,0.47403885817937,0.484374999999898,0.494257434932484,
0.499999999999903,0.522744871728982,0.595589883701348,0.624999999999984,
0.697813020501469,0.734375000000044,0.74218750000005,0.748069745909579,
0.750000000000057,0.770214559218657,0.82461903965541,0.880397897679706,
0.937085248067258,0.995155836674171,1.),.UNSPECIFIED.);
#5038=B_SPLINE_CURVE_WITH_KNOTS('',3,(#167978,#167979,#167980,#167981,#167982,
#167983,#167984,#167985,#167986,#167987,#167988,#167989,#167990),
 .UNSPECIFIED.,.F.,.F.,(4,3,3,3,4),(0.,0.000174780063231096,0.000349568960659906,
0.00052437265365072,0.000699137921319812),.UNSPECIFIED.);
#5039=B_SPLINE_CURVE_WITH_KNOTS('',3,(#168096,#168097,#168098,#168099,#168100,
#168101,#168102,#168103,#168104,#168105,#168106,#168107,#168108,#168109,
#168110,#168111,#168112,#168113,#168114),.UNSPECIFIED.,.F.,.F.,(4,3,3,3,
3,3,4),(0.,0.000168652558320961,0.000337340594483331,0.000432590797837398,
0.000530250662249359,0.000626975088861563,0.000674681188966661),
 .UNSPECIFIED.);
#5040=B_SPLINE_CURVE_WITH_KNOTS('',3,(#168116,#168117,#168118,#168119,#168120,
#168121,#168122,#168123,#168124,#168125,#168126,#168127,#168128,#168129,
#168130,#168131,#168132,#168133,#168134,#168135,#168136,#168137,#168138,
#168139,#168140,#168141,#168142,#168143,#168144,#168145,#168146,#168147,
#168148,#168149,#168150,#168151,#168152,#168153,#168154,#168155,#168156,
#168157,#168158,#168159,#168160,#168161,#168162,#168163,#168164,#168165,
#168166,#168167,#168168,#168169,#168170,#168171,#168172,#168173,#168174,
#168175,#168176,#168177,#168178,#168179,#168180,#168181,#168182,#168183,
#168184,#168185,#168186,#168187,#168188),.UNSPECIFIED.,.F.,.F.,(4,3,3,3,
3,3,3,3,3,3,3,3,3,3,3,3,3,3,3,3,3,3,3,3,4),(0.,0.0466130745701607,0.0624999999999758,
0.110609695998509,0.161358773789719,0.214918577626033,0.218749999999909,
0.23437499999991,0.242187499999898,0.248565636806847,0.249999999999886,
0.327720997850909,0.374999999999767,0.438264832152717,0.476586654637605,
0.480754066517823,0.484374999999699,0.494592854670677,0.499999999999701,
0.578329040666612,0.660059923923264,0.720472595197765,0.817502903971575,
0.924488968621202,1.),.UNSPECIFIED.);
#5041=B_SPLINE_CURVE_WITH_KNOTS('',3,(#168232,#168233,#168234,#168235,#168236,
#168237,#168238,#168239,#168240,#168241,#168242,#168243,#168244,#168245,
#168246,#168247),.UNSPECIFIED.,.F.,.F.,(4,3,3,3,3,4),(0.,0.00159103011504873,
0.00287711962167565,0.00431567943251345,0.00538763071251274,0.00575423924335125),
 .UNSPECIFIED.);
#5042=B_SPLINE_CURVE_WITH_KNOTS('',3,(#168280,#168281,#168282,#168283,#168284,
#168285,#168286,#168287,#168288,#168289,#168290,#168291,#168292,#168293,
#168294,#168295,#168296,#168297,#168298,#168299,#168300,#168301,#168302,
#168303,#168304,#168305,#168306,#168307,#168308,#168309,#168310,#168311,
#168312,#168313,#168314,#168315,#168316,#168317,#168318,#168319,#168320,
#168321,#168322,#168323,#168324,#168325,#168326,#168327,#168328,#168329,
#168330,#168331,#168332,#168333,#168334,#168335,#168336,#168337,#168338,
#168339,#168340,#168341,#168342,#168343,#168344,#168345,#168346,#168347,
#168348,#168349,#168350,#168351,#168352,#168353,#168354,#168355,#168356,
#168357,#168358,#168359,#168360,#168361,#168362,#168363,#168364,#168365,
#168366,#168367,#168368,#168369,#168370,#168371,#168372,#168373),
 .UNSPECIFIED.,.F.,.F.,(4,3,3,3,3,3,3,3,3,3,3,3,3,3,3,3,3,3,3,3,3,3,3,3,
3,3,3,3,3,3,3,4),(0.,0.0762493613834967,0.125000000000117,0.18628438331924,
0.216926574978801,0.232247670808581,0.233849499850804,0.235177693318918,
0.243766448203366,0.247568766638362,0.249645155900695,0.250597019269575,
0.30766327935826,0.367620699912883,0.40625000000014,0.453125000000129,0.497645716780995,
0.500000000000118,0.500538290361993,0.531250000000111,0.587063744180494,
0.640625000000085,0.695312500000072,0.717781622680416,0.722656250000066,
0.736328125000062,0.750000000000059,0.812500000000044,0.87500000000003,
0.937500000000015,0.968750000000007,1.),.UNSPECIFIED.);
#5043=B_SPLINE_CURVE_WITH_KNOTS('',3,(#168377,#168378,#168379,#168380,#168381,
#168382,#168383,#168384,#168385,#168386,#168387,#168388,#168389,#168390,
#168391,#168392,#168393,#168394,#168395),.UNSPECIFIED.,.F.,.F.,(4,3,3,3,
3,3,4),(0.,0.194046007642795,0.397883063949626,0.5,0.676457301204358,0.848320696951666,
1.),.UNSPECIFIED.);
#5044=B_SPLINE_CURVE_WITH_KNOTS('',3,(#168415,#168416,#168417,#168418),
 .UNSPECIFIED.,.F.,.F.,(4,4),(0.,0.0170848224870981),.UNSPECIFIED.);
#5045=B_SPLINE_CURVE_WITH_KNOTS('',3,(#168420,#168421,#168422,#168423,#168424,
#168425,#168426,#168427,#168428,#168429,#168430,#168431,#168432,#168433,
#168434,#168435),.UNSPECIFIED.,.F.,.F.,(4,3,3,3,3,4),(0.,0.216031740979677,
0.438702468406263,0.665600341454978,0.899498011354753,1.),.UNSPECIFIED.);
#5046=B_SPLINE_CURVE_WITH_KNOTS('',3,(#168467,#168468,#168469,#168470,#168471,
#168472,#168473,#168474,#168475,#168476,#168477,#168478,#168479),
 .UNSPECIFIED.,.F.,.F.,(4,3,3,3,4),(0.,0.00117191361843274,0.00234382723686548,
0.00351574085529822,0.00468765447373096),.UNSPECIFIED.);
#5047=B_SPLINE_CURVE_WITH_KNOTS('',3,(#168542,#168543,#168544,#168545,#168546,
#168547,#168548,#168549,#168550,#168551,#168552,#168553,#168554),
 .UNSPECIFIED.,.F.,.F.,(4,3,3,3,4),(0.,0.00125486684196805,0.0025097336839361,
0.00393224022465245,0.00501946736787221),.UNSPECIFIED.);
#5048=B_SPLINE_CURVE_WITH_KNOTS('',3,(#168569,#168570,#168571,#168572),
 .UNSPECIFIED.,.F.,.F.,(4,4),(0.,0.0135233968444946),.UNSPECIFIED.);
#5049=B_SPLINE_CURVE_WITH_KNOTS('',3,(#168594,#168595,#168596,#168597,#168598,
#168599,#168600,#168601,#168602,#168603,#168604,#168605,#168606,#168607,
#168608,#168609,#168610,#168611,#168612,#168613,#168614,#168615,#168616,
#168617,#168618,#168619,#168620,#168621,#168622,#168623,#168624,#168625,
#168626,#168627,#168628,#168629,#168630,#168631,#168632,#168633,#168634,
#168635,#168636,#168637,#168638,#168639,#168640,#168641,#168642,#168643,
#168644,#168645,#168646,#168647,#168648,#168649,#168650,#168651,#168652,
#168653,#168654,#168655,#168656,#168657,#168658,#168659,#168660,#168661,
#168662,#168663,#168664,#168665,#168666,#168667,#168668,#168669),
 .UNSPECIFIED.,.F.,.F.,(4,3,3,3,3,3,3,3,3,3,3,3,3,3,3,3,3,3,3,3,3,3,3,3,
3,4),(0.,0.0971655280396629,0.125000000000066,0.221059690008173,0.250000000000131,
0.339606682262106,0.375000000000198,0.437500000000225,0.468750000000233,
0.484375000000243,0.494471091409305,0.500000000000253,0.513777078434529,
0.599578820798521,0.625000000000219,0.687500000000208,0.718750000000209,
0.734375000000208,0.742187500000215,0.748149663075622,0.750000000000222,
0.804508551754479,0.858449558770446,0.911613486215102,0.962986872288349,
1.),.UNSPECIFIED.);
#5050=B_SPLINE_CURVE_WITH_KNOTS('',3,(#168670,#168671,#168672,#168673,#168674,
#168675,#168676,#168677,#168678,#168679,#168680,#168681,#168682,#168683,
#168684,#168685,#168686,#168687,#168688),.UNSPECIFIED.,.F.,.F.,(4,3,3,3,
3,3,4),(0.,0.000165241084431759,0.000319189981521249,0.000429288245407915,
0.000533834104225207,0.000631975129725552,0.000638379963042499),
 .UNSPECIFIED.);
#5051=B_SPLINE_CURVE_WITH_KNOTS('',3,(#168734,#168735,#168736,#168737,#168738,
#168739,#168740,#168741,#168742,#168743,#168744,#168745,#168746,#168747,
#168748,#168749,#168750,#168751,#168752,#168753,#168754,#168755,#168756,
#168757,#168758,#168759,#168760,#168761,#168762,#168763,#168764,#168765,
#168766,#168767,#168768,#168769,#168770,#168771,#168772,#168773,#168774,
#168775,#168776,#168777,#168778,#168779,#168780,#168781,#168782,#168783,
#168784,#168785,#168786,#168787,#168788),.UNSPECIFIED.,.F.,.F.,(4,3,3,3,
3,3,3,3,3,3,3,3,3,3,3,3,3,3,4),(0.,0.0626986305266445,0.127141358331606,
0.194501704871004,0.263573954919851,0.335355949256235,0.37500000000041,
0.437500000000472,0.46875000000049,0.484375000000489,0.492187500000474,
0.498658321176073,0.500000000000459,0.593349888207087,0.688363929203977,
0.785973373274766,0.885166870466393,0.986682553086995,1.),.UNSPECIFIED.);
#5052=B_SPLINE_CURVE_WITH_KNOTS('',3,(#168791,#168792,#168793,#168794,#168795,
#168796,#168797,#168798,#168799,#168800,#168801,#168802,#168803,#168804,
#168805,#168806,#168807,#168808,#168809,#168810,#168811,#168812),
 .UNSPECIFIED.,.F.,.F.,(4,3,3,3,3,3,3,4),(0.,0.00011032124306877,0.000232554441606406,
0.000327443278856643,0.000415696683397815,0.000505913400363394,0.000594574640422778,
0.000654886557713287),.UNSPECIFIED.);
#5053=B_SPLINE_CURVE_WITH_KNOTS('',3,(#168827,#168828,#168829,#168830),
 .UNSPECIFIED.,.F.,.F.,(4,4),(0.,0.00876509433037234),.UNSPECIFIED.);
#5054=B_SPLINE_CURVE_WITH_KNOTS('',3,(#168857,#168858,#168859,#168860,#168861,
#168862,#168863,#168864,#168865,#168866,#168867,#168868,#168869,#168870,
#168871,#168872,#168873,#168874,#168875,#168876,#168877,#168878,#168879,
#168880,#168881),.UNSPECIFIED.,.F.,.F.,(4,3,3,3,3,3,3,3,4),(0.,0.00066897147268262,
0.00133794294536524,0.00197188997954967,0.00259689693896644,0.00267588589073048,
0.00401382883609571,0.00511764383917763,0.00535177178146096),
 .UNSPECIFIED.);
#5055=B_SPLINE_CURVE_WITH_KNOTS('',3,(#168912,#168913,#168914,#168915,#168916,
#168917,#168918,#168919,#168920,#168921,#168922,#168923,#168924,#168925,
#168926,#168927),.UNSPECIFIED.,.F.,.F.,(4,3,3,3,3,4),(0.,0.0012090865501967,
0.00133938491136683,0.00267876982273365,0.00415143771886329,0.0053575396454673),
 .UNSPECIFIED.);
#5056=B_SPLINE_CURVE_WITH_KNOTS('',3,(#168942,#168943,#168944,#168945),
 .UNSPECIFIED.,.F.,.F.,(4,4),(0.,0.00904291806877093),.UNSPECIFIED.);
#5057=B_SPLINE_CURVE_WITH_KNOTS('',3,(#168966,#168967,#168968,#168969,#168970,
#168971,#168972,#168973,#168974,#168975,#168976,#168977,#168978,#168979,
#168980,#168981),.UNSPECIFIED.,.F.,.F.,(4,3,3,3,3,4),(0.,0.00019490585198886,
0.000327981152987957,0.000444921456706714,0.000551183314037962,0.000655962305975913),
 .UNSPECIFIED.);
#5058=B_SPLINE_CURVE_WITH_KNOTS('',3,(#169141,#169142,#169143,#169144,#169145,
#169146,#169147,#169148,#169149,#169150,#169151,#169152,#169153,#169154,
#169155,#169156,#169157,#169158,#169159),.UNSPECIFIED.,.F.,.F.,(4,3,3,3,
3,3,4),(0.,0.000108392306331539,0.000159419175882383,0.000279017984019912,
0.000319155213741796,0.000478738661811073,0.000638310427483592),
 .UNSPECIFIED.);
#5059=B_SPLINE_CURVE_WITH_KNOTS('',3,(#169174,#169175,#169176,#169177),
 .UNSPECIFIED.,.F.,.F.,(4,4),(0.,0.01284355850178),.UNSPECIFIED.);
#5060=B_SPLINE_CURVE_WITH_KNOTS('',3,(#169210,#169211,#169212,#169213,#169214,
#169215,#169216,#169217,#169218,#169219,#169220,#169221,#169222,#169223,
#169224,#169225),.UNSPECIFIED.,.F.,.F.,(4,3,3,3,3,4),(0.,0.00125936773350451,
0.00251873546700902,0.00377810320051352,0.00490364900505264,0.00503747093401803),
 .UNSPECIFIED.);
#5061=B_SPLINE_CURVE_WITH_KNOTS('',3,(#169256,#169257,#169258,#169259,#169260,
#169261,#169262,#169263,#169264,#169265,#169266,#169267,#169268),
 .UNSPECIFIED.,.F.,.F.,(4,3,3,3,4),(0.,0.00126095469566737,0.00252190939133473,
0.00394829824261256,0.00504381878266947),.UNSPECIFIED.);
#5062=B_SPLINE_CURVE_WITH_KNOTS('',3,(#169283,#169284,#169285,#169286),
 .UNSPECIFIED.,.F.,.F.,(4,4),(0.,0.0125680158145827),.UNSPECIFIED.);
#5063=B_SPLINE_CURVE_WITH_KNOTS('',3,(#169289,#169290,#169291,#169292,#169293,
#169294,#169295,#169296,#169297,#169298,#169299,#169300,#169301),
 .UNSPECIFIED.,.F.,.F.,(4,3,3,3,4),(0.,0.293726063052163,0.581913693472172,
0.862643124884957,1.),.UNSPECIFIED.);
#5064=B_SPLINE_CURVE_WITH_KNOTS('',3,(#169335,#169336,#169337,#169338,#169339,
#169340,#169341,#169342,#169343,#169344,#169345,#169346,#169347),
 .UNSPECIFIED.,.F.,.F.,(4,3,3,3,4),(0.,0.000167806452105701,0.000320197614368795,
0.000480307701132286,0.000640395228737589),.UNSPECIFIED.);
#5065=B_SPLINE_CURVE_WITH_KNOTS('',3,(#169348,#169349,#169350,#169351,#169352,
#169353,#169354,#169355,#169356,#169357,#169358,#169359,#169360,#169361,
#169362,#169363,#169364,#169365,#169366,#169367,#169368,#169369,#169370,
#169371,#169372,#169373,#169374,#169375,#169376,#169377,#169378,#169379,
#169380,#169381,#169382,#169383,#169384,#169385,#169386,#169387,#169388,
#169389,#169390,#169391,#169392,#169393,#169394,#169395,#169396,#169397,
#169398,#169399,#169400,#169401,#169402,#169403,#169404,#169405,#169406,
#169407,#169408,#169409,#169410,#169411,#169412,#169413,#169414,#169415,
#169416,#169417,#169418,#169419,#169420,#169421,#169422,#169423),
 .UNSPECIFIED.,.F.,.F.,(4,3,3,3,3,3,3,3,3,3,3,3,3,3,3,3,3,3,3,3,3,3,3,3,
3,4),(0.,0.0870023380906959,0.124999999999938,0.19900805061357,0.245182333562838,
0.273016101227201,0.326530647858571,0.365028892168486,0.399414806094218,
0.484374999999772,0.494494956765455,0.499999999999771,0.514090654941682,
0.599026190945531,0.624999999999764,0.687499999999756,0.718749999999752,
0.73437499999975,0.74218749999975,0.748147972438602,0.749999999999749,0.804505950346522,
0.858489911214372,0.911721504923935,0.963189048359122,1.),.UNSPECIFIED.);
#5066=B_SPLINE_CURVE_WITH_KNOTS('',3,(#169427,#169428,#169429,#169430,#169431,
#169432,#169433,#169434,#169435,#169436,#169437,#169438,#169439,#169440,
#169441,#169442),.UNSPECIFIED.,.F.,.F.,(4,3,3,3,3,4),(0.,0.193117490837313,
0.394838118127984,0.598407779512051,0.809334151745404,1.),.UNSPECIFIED.);
#5067=B_SPLINE_CURVE_WITH_KNOTS('',3,(#169469,#169470,#169471,#169472),
 .UNSPECIFIED.,.F.,.F.,(4,4),(0.,0.0203430832871546),.UNSPECIFIED.);
#5068=B_SPLINE_CURVE_WITH_KNOTS('',3,(#169499,#169500,#169501,#169502,#169503,
#169504,#169505,#169506,#169507,#169508,#169509,#169510,#169511),
 .UNSPECIFIED.,.F.,.F.,(4,3,3,3,4),(0.,0.00107468821847175,0.0021493764369435,
0.00322406465541528,0.00429875287388706),.UNSPECIFIED.);
#5069=B_SPLINE_CURVE_WITH_KNOTS('',3,(#169536,#169537,#169538,#169539,#169540,
#169541,#169542,#169543,#169544,#169545,#169546,#169547,#169548,#169549,
#169550,#169551,#169552,#169553,#169554,#169555,#169556,#169557),
 .UNSPECIFIED.,.F.,.F.,(4,3,3,3,3,3,3,4),(0.,0.000387785729069979,0.000791054588126119,
0.00107666227523054,0.00167259937146367,0.00215332455046108,0.00346243334011356,
0.00430664910092208),.UNSPECIFIED.);
#5070=B_SPLINE_CURVE_WITH_KNOTS('',3,(#169572,#169573,#169574,#169575),
 .UNSPECIFIED.,.F.,.F.,(4,4),(0.,0.0206148669995797),.UNSPECIFIED.);
#5071=B_SPLINE_CURVE_WITH_KNOTS('',3,(#169590,#169591,#169592,#169593),
 .UNSPECIFIED.,.F.,.F.,(4,4),(0.,0.000103369667661668),.UNSPECIFIED.);
#5072=B_SPLINE_CURVE_WITH_KNOTS('',3,(#169615,#169616,#169617,#169618,#169619,
#169620,#169621,#169622,#169623,#169624,#169625,#169626,#169627,#169628,
#169629,#169630,#169631,#169632,#169633,#169634,#169635,#169636,#169637,
#169638,#169639,#169640,#169641,#169642,#169643,#169644,#169645,#169646,
#169647,#169648),.UNSPECIFIED.,.F.,.F.,(4,3,3,3,3,3,3,3,3,3,3,4),(3.96777284137604E-14,
0.124999999999938,0.249999999999836,0.379017862416308,0.468749999999687,
0.488635543023418,0.497380093045793,0.499999999999651,0.6544631322486,0.810594430460327,
0.970117896208719,0.999999999092843),.UNSPECIFIED.);
#5073=B_SPLINE_CURVE_WITH_KNOTS('',3,(#169649,#169650,#169651,#169652,#169653,
#169654,#169655,#169656,#169657,#169658,#169659,#169660,#169661),
 .UNSPECIFIED.,.F.,.F.,(4,3,3,3,4),(0.,0.000379823720134918,0.000488238270882253,
0.000734566123585685,0.000976476541764506),.UNSPECIFIED.);
#5074=B_SPLINE_CURVE_WITH_KNOTS('',3,(#169675,#169676,#169677,#169678,#169679,
#169680,#169681,#169682,#169683,#169684,#169685,#169686,#169687),
 .UNSPECIFIED.,.F.,.F.,(4,3,3,3,4),(0.,0.256134514950837,0.516016641878448,
0.782357628273516,1.),.UNSPECIFIED.);
#5075=B_SPLINE_CURVE_WITH_KNOTS('',3,(#169790,#169791,#169792,#169793,#169794,
#169795,#169796,#169797,#169798,#169799,#169800,#169801,#169802,#169803,
#169804,#169805,#169806,#169807,#169808,#169809,#169810,#169811,#169812,
#169813,#169814,#169815,#169816,#169817,#169818,#169819,#169820,#169821,
#169822,#169823,#169824,#169825,#169826),.UNSPECIFIED.,.F.,.F.,(4,3,3,3,
3,3,3,3,3,3,3,3,4),(0.,0.000231966620805271,0.000541763265450615,0.000565419069388565,
0.000565630623675328,0.00113073622792203,0.00113126124735066,0.00146429940365072,
0.00169659085207846,0.00169689187102598,0.00198522910630028,0.00223959723150185,
0.00226252249470131),.UNSPECIFIED.);
#5076=B_SPLINE_CURVE_WITH_KNOTS('',3,(#169828,#169829,#169830,#169831,#169832,
#169833,#169834,#169835,#169836,#169837,#169838,#169839,#169840,#169841,
#169842,#169843,#169844,#169845),.UNSPECIFIED.,.F.,.F.,(4,2,2,2,2,2,2,2,
4),(-0.232545286649255,-0.202278856488963,-0.169720566966038,-0.147070875715933,
-0.116272702465016,-0.0854925566385012,-0.0628371603598658,-0.0302640152400447,
0.),.UNSPECIFIED.);
#5077=B_SPLINE_CURVE_WITH_KNOTS('',3,(#169887,#169888,#169889,#169890),
 .UNSPECIFIED.,.F.,.F.,(4,4),(0.,0.000203650363220012),.UNSPECIFIED.);
#5078=B_SPLINE_CURVE_WITH_KNOTS('',3,(#169911,#169912,#169913,#169914,#169915,
#169916,#169917,#169918,#169919,#169920,#169921,#169922,#169923,#169924,
#169925,#169926,#169927,#169928,#169929,#169930,#169931,#169932,#169933,
#169934,#169935),.UNSPECIFIED.,.F.,.F.,(4,3,3,3,3,3,3,3,4),(0.,7.36083385127449E-5,
0.000151188117339882,0.000234018984645761,0.000250167431468888,0.000250705751451749,
0.000332906541327113,0.000418695252292313,0.000500334862937777),
 .UNSPECIFIED.);
#5079=B_SPLINE_CURVE_WITH_KNOTS('',3,(#169968,#169969,#169970,#169971,#169972,
#169973,#169974,#169975,#169976,#169977,#169978,#169979,#169980,#169981,
#169982,#169983),.UNSPECIFIED.,.F.,.F.,(4,3,3,3,3,4),(0.,0.0014169282635678,
0.00283385652713561,0.00425078479070341,0.00538743306816435,0.00566771305427122),
 .UNSPECIFIED.);
#5080=B_SPLINE_CURVE_WITH_KNOTS('',3,(#170013,#170014,#170015,#170016,#170017,
#170018,#170019,#170020,#170021,#170022,#170023,#170024,#170025),
 .UNSPECIFIED.,.F.,.F.,(4,3,3,3,4),(6.93889390390723E-18,0.00134873564674426,
0.00269747129348853,0.00432753805226364,0.00539494258697707),
 .UNSPECIFIED.);
#5081=B_SPLINE_CURVE_WITH_KNOTS('',3,(#170058,#170059,#170060,#170061,#170062,
#170063,#170064,#170065,#170066,#170067,#170068,#170069,#170070,#170071,
#170072,#170073,#170074,#170075,#170076),.UNSPECIFIED.,.F.,.F.,(4,3,3,3,
3,3,4),(0.,0.000151278709680665,0.000175639358542291,0.00032081912162696,
0.000351502905376566,0.000527285240968804,0.000703005810753132),
 .UNSPECIFIED.);
#5082=B_SPLINE_CURVE_WITH_KNOTS('',3,(#170079,#170080,#170081,#170082,#170083,
#170084,#170085,#170086,#170087,#170088,#170089,#170090,#170091,#170092,
#170093,#170094,#170095,#170096,#170097,#170098,#170099,#170100,#170101,
#170102,#170103),.UNSPECIFIED.,.F.,.F.,(4,2,2,2,1,2,2,2,2,1,1,2,2,4),(0.,
0.249999999999732,0.37499999999959,0.437499999999521,0.468749999999492,
0.484374999999488,0.499999999999485,0.624999999999589,0.687499999999633,
0.718749999999655,0.734374999999666,0.742187499999676,0.749999999999686,
0.999999477481404),.UNSPECIFIED.);
#5083=B_SPLINE_CURVE_WITH_KNOTS('',3,(#170195,#170196,#170197,#170198),
 .UNSPECIFIED.,.F.,.F.,(4,4),(0.,8.25660289862869E-5),.UNSPECIFIED.);
#5084=B_SPLINE_CURVE_WITH_KNOTS('',3,(#170221,#170222,#170223,#170224,#170225,
#170226,#170227),.UNSPECIFIED.,.F.,.F.,(4,3,4),(0.,0.0148367096635454,0.0296734193270908),
 .UNSPECIFIED.);
#5085=B_SPLINE_CURVE_WITH_KNOTS('',3,(#170248,#170249,#170250,#170251,#170252,
#170253,#170254,#170255,#170256,#170257,#170258,#170259,#170260,#170261,
#170262,#170263,#170264,#170265,#170266,#170267,#170268,#170269,#170270,
#170271,#170272),.UNSPECIFIED.,.F.,.F.,(4,3,3,3,3,3,3,3,4),(0.,0.000418974782548372,
0.000841777476037116,0.00103655247459,0.00148268378393581,0.0019250583151384,
0.00207310494918,0.00313777887502721,0.00414620989836001),.UNSPECIFIED.);
#5086=B_SPLINE_CURVE_WITH_KNOTS('',3,(#170298,#170299,#170300,#170301,#170302,
#170303,#170304,#170305,#170306,#170307,#170308,#170309,#170310,#170311,
#170312,#170313,#170314,#170315,#170316,#170317,#170318,#170319,#170320,
#170321,#170322,#170323,#170324,#170325,#170326,#170327,#170328,#170329,
#170330,#170331,#170332,#170333,#170334,#170335,#170336),.UNSPECIFIED.,
 .F.,.F.,(4,2,2,1,1,1,1,2,2,2,2,2,1,1,2,2,2,2,1,1,1,2,2,4),(0.,0.124999999999703,
0.187499999999554,0.218749999999476,0.234374999999437,0.242187499999421,
0.246093749999413,0.248046874999405,0.249999999999396,0.374999999999367,
0.437499999999356,0.468749999999351,0.484374999999349,0.492187499999348,
0.496093749999347,0.499999999999347,0.624999999999361,0.687499999999364,
0.718749999999365,0.734374999999367,0.742187499999368,0.746093749999375,
0.749999999999382,0.999999986192015),.UNSPECIFIED.);
#5087=B_SPLINE_CURVE_WITH_KNOTS('',3,(#170337,#170338,#170339,#170340,#170341,
#170342,#170343,#170344,#170345,#170346,#170347,#170348,#170349,#170350,
#170351,#170352,#170353,#170354,#170355,#170356,#170357,#170358),
 .UNSPECIFIED.,.F.,.F.,(4,3,3,3,3,3,3,4),(1.55158384577954E-17,0.000383789572583399,
0.000781910391026632,0.00103855983331611,0.00179575082696553,0.00207711966663221,
0.00335799595902739,0.00415423933326436),.UNSPECIFIED.);
#5088=B_SPLINE_CURVE_WITH_KNOTS('',3,(#170410,#170411,#170412,#170413,#170414,
#170415,#170416,#170417,#170418,#170419,#170420,#170421,#170422,#170423,
#170424,#170425),.UNSPECIFIED.,.F.,.F.,(4,2,2,1,1,1,1,2,2,4),(0.,0.24999999999986,
0.37499999999979,0.437499999999754,0.468749999999737,0.484374999999728,
0.492187499999723,0.49902343749972,0.499999999999719,1.),.UNSPECIFIED.);
#5089=B_SPLINE_CURVE_WITH_KNOTS('',3,(#170426,#170427,#170428,#170429,#170430,
#170431,#170432),.UNSPECIFIED.,.F.,.F.,(4,3,4),(0.,0.0147014688781887,0.0294029377563774),
 .UNSPECIFIED.);
#5090=B_SPLINE_CURVE_WITH_KNOTS('',3,(#170452,#170453,#170454,#170455,#170456,
#170457,#170458,#170459,#170460,#170461,#170462,#170463,#170464,#170465,
#170466,#170467),.UNSPECIFIED.,.F.,.F.,(4,3,3,3,3,4),(8.08667809653667E-7,
0.261781280773483,0.391444635181636,0.617402649693561,0.814980261808023,
1.),.UNSPECIFIED.);
#5091=B_SPLINE_CURVE_WITH_KNOTS('',3,(#170468,#170469,#170470,#170471,#170472,
#170473,#170474,#170475,#170476,#170477,#170478,#170479,#170480,#170481,
#170482,#170483,#170484,#170485,#170486,#170487,#170488,#170489,#170490,
#170491,#170492,#170493,#170494,#170495,#170496,#170497,#170498,#170499,
#170500,#170501,#170502,#170503,#170504,#170505,#170506,#170507,#170508,
#170509,#170510,#170511,#170512,#170513,#170514,#170515,#170516,#170517,
#170518,#170519,#170520,#170521,#170522,#170523,#170524,#170525,#170526,
#170527,#170528,#170529,#170530,#170531,#170532,#170533,#170534,#170535,
#170536,#170537,#170538,#170539,#170540,#170541,#170542,#170543,#170544,
#170545,#170546,#170547,#170548,#170549),.UNSPECIFIED.,.F.,.F.,(4,3,3,3,
3,3,3,3,3,3,3,3,3,3,3,3,3,3,3,3,3,3,3,3,3,3,3,4),(1.73784017987518E-5,0.0624999999999309,
0.124999999999862,0.187499999999794,0.21874999999976,0.234374999999738,
0.242187499999727,0.246093749999722,0.248046874999723,0.249999999999724,
0.299242278960943,0.349392080063728,0.374999999999775,0.429018671543615,
0.4374999999998,0.468749999999814,0.48437499999982,0.49577510820138,0.499999999999827,
0.500495595336202,0.562747797668036,0.62499999999987,0.696123920530156,
0.74666554161023,0.782709136401979,0.855162490063989,0.930474985780909,
1.),.UNSPECIFIED.);
#5092=B_SPLINE_CURVE_WITH_KNOTS('',3,(#170572,#170573,#170574,#170575,#170576,
#170577,#170578,#170579),.UNSPECIFIED.,.F.,.F.,(4,2,2,4),(0.,0.000841011829491348,
0.00168202365898269,0.00336404731796539),.UNSPECIFIED.);
#5093=B_SPLINE_CURVE_WITH_KNOTS('',3,(#170603,#170604,#170605,#170606,#170607,
#170608,#170609,#170610,#170611,#170612,#170613,#170614,#170615,#170616,
#170617,#170618),.UNSPECIFIED.,.F.,.F.,(4,3,3,3,3,4),(0.,0.000762418881005378,
0.00156275687156247,0.00168533471950014,0.00283547033566749,0.00337066943900028),
 .UNSPECIFIED.);
#5094=B_SPLINE_CURVE_WITH_KNOTS('',3,(#170639,#170640,#170641,#170642,#170643,
#170644,#170645),.UNSPECIFIED.,.F.,.F.,(4,3,4),(0.,0.0179426259581151,0.0358852519162302),
 .UNSPECIFIED.);
#5095=B_SPLINE_CURVE_WITH_KNOTS('',3,(#170696,#170697,#170698,#170699,#170700,
#170701,#170702,#170703,#170704,#170705,#170706,#170707,#170708,#170709,
#170710,#170711,#170712,#170713,#170714,#170715,#170716,#170717,#170718,
#170719,#170720,#170721,#170722,#170723,#170724,#170725,#170726),
 .UNSPECIFIED.,.F.,.F.,(4,3,3,3,3,3,3,3,3,3,4),(0.,0.151691911771996,0.306710028502103,
0.467372294165444,0.499023437500016,0.500000000000016,0.500021673300866,
0.625016254975649,0.750863508401593,0.881927831571319,1.),.UNSPECIFIED.);
#5096=B_SPLINE_CURVE_WITH_KNOTS('',3,(#170729,#170730,#170731,#170732,#170733,
#170734,#170735),.UNSPECIFIED.,.F.,.F.,(4,3,4),(0.,0.0178083890192188,0.0356167780384377),
 .UNSPECIFIED.);
#5097=B_SPLINE_CURVE_WITH_KNOTS('',3,(#170797,#170798,#170799,#170800,#170801,
#170802,#170803),.UNSPECIFIED.,.F.,.F.,(4,3,4),(6.93889390390723E-18,0.0190876722191456,
0.0381753444382913),.UNSPECIFIED.);
#5098=B_SPLINE_CURVE_WITH_KNOTS('',3,(#170824,#170825,#170826,#170827,#170828,
#170829,#170830,#170831,#170832,#170833,#170834,#170835,#170836,#170837,
#170838,#170839),.UNSPECIFIED.,.F.,.F.,(4,3,3,3,3,4),(0.,0.000542853834905746,
0.00109518831082765,0.00152034213881841,0.00254894911026922,0.00304068427763681),
 .UNSPECIFIED.);
#5099=B_SPLINE_CURVE_WITH_KNOTS('',3,(#170866,#170867,#170868,#170869,#170870,
#170871,#170872,#170873,#170874,#170875,#170876,#170877,#170878,#170879,
#170880,#170881,#170882,#170883,#170884,#170885,#170886,#170887,#170888,
#170889,#170890,#170891,#170892,#170893,#170894,#170895,#170896,#170897,
#170898,#170899,#170900,#170901,#170902,#170903,#170904,#170905,#170906,
#170907,#170908,#170909,#170910,#170911,#170912,#170913,#170914,#170915,
#170916,#170917,#170918,#170919,#170920,#170921,#170922,#170923,#170924,
#170925,#170926,#170927,#170928,#170929,#170930,#170931,#170932,#170933,
#170934,#170935,#170936,#170937,#170938,#170939,#170940,#170941,#170942,
#170943,#170944,#170945,#170946,#170947,#170948,#170949,#170950,#170951,
#170952,#170953,#170954,#170955,#170956,#170957,#170958,#170959,#170960,
#170961,#170962,#170963,#170964,#170965,#170966,#170967,#170968),
 .UNSPECIFIED.,.F.,.F.,(4,3,3,3,3,3,3,3,3,3,3,3,3,3,3,3,3,3,3,3,3,3,3,3,
3,3,3,3,3,3,3,3,3,3,4),(0.,0.0900245051711857,0.12500000000326,0.187500000004897,
0.218750000005709,0.234375000006121,0.242187500006326,0.246093750006424,
0.250000000006521,0.319655504681364,0.387239150766509,0.437500000011095,
0.468750000011866,0.484375000012251,0.492187500012445,0.496093750012541,
0.498046875012584,0.500000000012627,0.532507155583111,0.565381440866807,
0.598529785335568,0.631930879298941,0.66539941633402,0.698913886443443,
0.718750000017358,0.734375000017693,0.742187500017856,0.746093750017937,
0.748046875017916,0.749023437517847,0.750000000017778,0.821623578614083,
0.894552114764428,0.969478886559688,1.),.UNSPECIFIED.);
#5100=B_SPLINE_CURVE_WITH_KNOTS('',3,(#170969,#170970,#170971,#170972,#170973,
#170974,#170975,#170976,#170977,#170978,#170979,#170980,#170981),
 .UNSPECIFIED.,.F.,.F.,(4,3,3,3,4),(0.,0.000817157754010358,0.00152229638412186,
0.00262171283977965,0.00304459276824371),.UNSPECIFIED.);
#5101=B_SPLINE_CURVE_WITH_KNOTS('',3,(#171003,#171004,#171005,#171006,#171007,
#171008,#171009,#171010,#171011,#171012,#171013,#171014,#171015,#171016,
#171017,#171018),.UNSPECIFIED.,.F.,.F.,(4,2,2,1,1,1,1,2,2,4),(0.,0.249999999999946,
0.374999999999919,0.437499999999904,0.468749999999897,0.484374999999893,
0.492187499999891,0.499023437499889,0.499999999999889,1.),.UNSPECIFIED.);
#5102=B_SPLINE_CURVE_WITH_KNOTS('',3,(#171019,#171020,#171021,#171022,#171023,
#171024,#171025),.UNSPECIFIED.,.F.,.F.,(4,3,4),(0.,0.0189537577590876,0.0379075155181752),
 .UNSPECIFIED.);
#5103=B_SPLINE_CURVE_WITH_KNOTS('',3,(#171051,#171052,#171053,#171054,#171055,
#171056,#171057,#171058,#171059,#171060,#171061,#171062,#171063,#171064,
#171065,#171066,#171067,#171068,#171069,#171070,#171071,#171072),
 .UNSPECIFIED.,.F.,.F.,(4,3,3,3,3,3,3,4),(4.13152027403574E-8,0.150452793181179,
0.265782575349523,0.374279137552784,0.44848875244278,0.72424437622139,0.921304556955205,
1.),.UNSPECIFIED.);
#5104=B_SPLINE_CURVE_WITH_KNOTS('',3,(#171073,#171074,#171075,#171076,#171077,
#171078,#171079,#171080,#171081,#171082,#171083,#171084,#171085,#171086,
#171087,#171088,#171089,#171090,#171091,#171092,#171093,#171094,#171095,
#171096,#171097,#171098,#171099,#171100,#171101,#171102,#171103,#171104,
#171105,#171106,#171107,#171108,#171109,#171110,#171111,#171112,#171113,
#171114,#171115,#171116,#171117,#171118,#171119,#171120,#171121,#171122,
#171123,#171124,#171125,#171126,#171127,#171128,#171129,#171130,#171131,
#171132,#171133,#171134,#171135,#171136,#171137,#171138,#171139,#171140,
#171141,#171142,#171143,#171144,#171145,#171146,#171147,#171148,#171149,
#171150,#171151,#171152,#171153,#171154),.UNSPECIFIED.,.F.,.F.,(4,3,3,3,
3,3,3,3,3,3,3,3,3,3,3,3,3,3,3,3,3,3,3,3,3,3,3,4),(1.312206885811E-6,0.0698966901337594,
0.125000000000195,0.187500000000286,0.218750000000339,0.234375000000365,
0.242187500000377,0.246093750000384,0.250000000000391,0.290090360663461,
0.330650857430358,0.371698509928867,0.412916364884191,0.454282110705438,
0.468750000000707,0.484375000000744,0.492187500000784,0.496093750000782,
0.498046875000781,0.498535156250781,0.498901367188281,0.500000000000781,
0.590487268190957,0.682955872901068,0.77862973559014,0.876261101941014,
0.97682566140977,0.999999999999992),.UNSPECIFIED.);
#5105=B_SPLINE_CURVE_WITH_KNOTS('',3,(#171177,#171178,#171179,#171180,#171181,
#171182,#171183,#171184,#171185,#171186,#171187,#171188,#171189),
 .UNSPECIFIED.,.F.,.F.,(4,3,3,3,4),(0.,0.000842979772258894,0.00121101869920095,
0.00218603126581974,0.00242203739840189),.UNSPECIFIED.);
#5106=B_SPLINE_CURVE_WITH_KNOTS('',3,(#171214,#171215,#171216,#171217,#171218,
#171219,#171220,#171221,#171222,#171223,#171224,#171225,#171226),
 .UNSPECIFIED.,.F.,.F.,(4,3,3,3,4),(0.,0.000857870627796964,0.00121135746045287,
0.00220749552011028,0.00242271492090574),.UNSPECIFIED.);
#5107=B_SPLINE_CURVE_WITH_KNOTS('',3,(#171241,#171242,#171243,#171244),
 .UNSPECIFIED.,.F.,.F.,(4,4),(0.,0.0421837023697854),.UNSPECIFIED.);
#5108=B_SPLINE_CURVE_WITH_KNOTS('',3,(#171306,#171307,#171308,#171309,#171310,
#171311,#171312,#171313,#171314,#171315,#171316,#171317,#171318,#171319,
#171320,#171321,#171322,#171323,#171324,#171325,#171326,#171327,#171328,
#171329,#171330,#171331,#171332,#171333,#171334,#171335,#171336,#171337,
#171338,#171339,#171340,#171341,#171342,#171343,#171344,#171345),
 .UNSPECIFIED.,.F.,.F.,(4,3,3,3,3,3,3,3,3,3,3,3,3,4),(0.,0.000556259975763551,
0.000647586119897307,0.000728260191095046,0.00109239125585009,0.00129517223979461,
0.00145651805257904,0.00182064826297319,0.00194275835969192,0.00212625862851037,
0.00218441767336186,0.00226655141964057,0.00244042135138738,0.00259034447958922),
 .UNSPECIFIED.);
#5109=B_SPLINE_CURVE_WITH_KNOTS('',3,(#171360,#171361,#171362,#171363,#171364,
#171365,#171366,#171367,#171368,#171369,#171370,#171371,#171372,#171373,
#171374,#171375),.UNSPECIFIED.,.F.,.F.,(4,2,2,1,1,1,1,2,2,4),(0.,0.250000000000176,
0.375000000000264,0.437500000000308,0.46875000000033,0.484375000000341,
0.492187500000346,0.499511718750351,0.500000000000351,1.),.UNSPECIFIED.);
#5110=B_SPLINE_CURVE_WITH_KNOTS('',3,(#171378,#171379,#171380,#171381),
 .UNSPECIFIED.,.F.,.F.,(4,4),(0.,0.0419168978153696),.UNSPECIFIED.);
#5111=B_SPLINE_CURVE_WITH_KNOTS('',3,(#171390,#171391,#171392,#171393),
 .UNSPECIFIED.,.F.,.F.,(4,4),(0.00436813896256353,0.00486865237729894),
 .UNSPECIFIED.);
#5112=B_SPLINE_CURVE_WITH_KNOTS('',3,(#171443,#171444,#171445,#171446,#171447,
#171448,#171449,#171450,#171451,#171452,#171453,#171454,#171455,#171456,
#171457,#171458,#171459,#171460,#171461,#171462,#171463,#171464,#171465,
#171466,#171467,#171468,#171469,#171470,#171471,#171472,#171473,#171474,
#171475,#171476,#171477,#171478,#171479),.UNSPECIFIED.,.F.,.F.,(4,3,3,3,
3,3,3,3,3,3,3,3,4),(0.000672031760609077,0.000712854075812315,0.00100252198456931,
0.00107233830279968,0.0012216976510115,0.00143188803178761,0.00171092729228638,
0.00177136354141392,0.00179176783191222,0.00215141270034081,0.00232102943181635,
0.00259586237701756,0.00287069532221878),.UNSPECIFIED.);
#5113=B_SPLINE_CURVE_WITH_KNOTS('',3,(#171537,#171538,#171539,#171540,#171541,
#171542,#171543,#171544,#171545,#171546,#171547,#171548,#171549),
 .UNSPECIFIED.,.F.,.F.,(4,3,3,3,4),(0.,0.000701986547780456,0.00111013811990961,
0.00206054695785466,0.00222027623981923),.UNSPECIFIED.);
#5114=B_SPLINE_CURVE_WITH_KNOTS('',3,(#171574,#171575,#171576,#171577,#171578,
#171579,#171580,#171581,#171582,#171583,#171584,#171585,#171586),
 .UNSPECIFIED.,.F.,.F.,(4,3,3,3,4),(0.,0.000647478258315285,0.00111023907191622,
0.00207039129249102,0.00222047814383243),.UNSPECIFIED.);
#5115=B_SPLINE_CURVE_WITH_KNOTS('',3,(#171589,#171590,#171591,#171592,#171593,
#171594,#171595,#171596,#171597,#171598,#171599,#171600,#171601,#171602,
#171603,#171604,#171605,#171606,#171607,#171608,#171609,#171610,#171611,
#171612,#171613,#171614,#171615,#171616,#171617,#171618,#171619,#171620,
#171621,#171622,#171623,#171624,#171625,#171626,#171627,#171628,#171629,
#171630,#171631,#171632,#171633,#171634,#171635,#171636,#171637,#171638,
#171639,#171640,#171641,#171642,#171643,#171644,#171645,#171646,#171647,
#171648,#171649,#171650,#171651,#171652),.UNSPECIFIED.,.F.,.F.,(4,3,3,3,
3,3,3,3,3,3,3,3,3,3,3,3,3,3,3,3,3,4),(0.,0.137315011687963,0.249999999999215,
0.374999999998815,0.437499999998613,0.46874999999852,0.48437499999848,0.49218749999846,
0.496093749998458,0.499999999998455,0.500132617240959,0.562566308619912,
0.624999999998865,0.687499999999072,0.718749999999174,0.73987160258027,
0.749999999999276,0.805747260200159,0.863072799323141,0.921013881125668,
0.979478145917718,0.999999974089565),.UNSPECIFIED.);
#5116=B_SPLINE_CURVE_WITH_KNOTS('',3,(#171672,#171673,#171674,#171675,#171676,
#171677,#171678,#171679,#171680,#171681,#171682,#171683,#171684,#171685,
#171686,#171687),.UNSPECIFIED.,.F.,.F.,(4,2,2,1,1,1,1,2,2,4),(0.,0.249999999999879,
0.37499999999982,0.43749999999979,0.468749999999775,0.484374999999767,0.492187499999763,
0.499511718749759,0.499999999999759,1.),.UNSPECIFIED.);
#5117=B_SPLINE_CURVE_WITH_KNOTS('',3,(#171713,#171714,#171715,#171716,#171717,
#171718,#171719,#171720,#171721,#171722,#171723,#171724,#171725,#171726,
#171727,#171728,#171729,#171730,#171731,#171732,#171733,#171734,#171735,
#171736,#171737,#171738,#171739,#171740,#171741,#171742,#171743,#171744,
#171745,#171746,#171747,#171748,#171749,#171750,#171751,#171752),
 .UNSPECIFIED.,.F.,.F.,(4,3,3,3,3,3,3,3,3,3,3,3,3,4),(0.,0.179991932872247,
0.233369732025158,0.249999999999994,0.338178756215747,0.374999999999992,
0.437499999999991,0.46874999999999,0.484374999999989,0.490038899812079,
0.499999999999989,0.749999999999994,0.96759783696102,1.),.UNSPECIFIED.);
#5118=B_SPLINE_CURVE_WITH_KNOTS('',3,(#171804,#171805,#171806,#171807),
 .UNSPECIFIED.,.F.,.F.,(4,4),(0.,0.0447707136167657),.UNSPECIFIED.);
#5119=B_SPLINE_CURVE_WITH_KNOTS('',3,(#171857,#171858,#171859,#171860,#171861,
#171862,#171863,#171864,#171865,#171866,#171867,#171868,#171869,#171870,
#171871,#171872,#171873,#171874,#171875,#171876,#171877,#171878,#171879,
#171880,#171881),.UNSPECIFIED.,.F.,.F.,(4,3,3,3,3,3,3,3,4),(0.,0.000275481208481403,
0.000553063545339304,0.000602887330399936,0.000809845174226025,0.00102800957885645,
0.00120532901601379,0.00142404055844572,0.00161969034845205),
 .UNSPECIFIED.);
#5120=B_SPLINE_CURVE_WITH_KNOTS('',3,(#171896,#171897,#171898,#171899,#171900,
#171901,#171902,#171903,#171904,#171905),.UNSPECIFIED.,.F.,.F.,(4,3,3,4),
(0.,0.389160316713121,0.830817831506134,1.),.UNSPECIFIED.);
#5121=B_SPLINE_CURVE_WITH_KNOTS('',3,(#171958,#171959,#171960,#171961,#171962,
#171963,#171964,#171965,#171966,#171967,#171968,#171969,#171970,#171971,
#171972,#171973,#171974,#171975,#171976,#171977,#171978,#171979,#171980,
#171981,#171982),.UNSPECIFIED.,.F.,.F.,(4,3,3,3,3,3,3,3,4),(0.000689304848359617,
0.00090628372627929,0.00111364302895387,0.00133013985168599,0.00150801684530018,
0.00171993694385612,0.00199672649963881,0.00227140074390808,0.00232672884224074),
 .UNSPECIFIED.);
#5122=B_SPLINE_CURVE_WITH_KNOTS('',3,(#172076,#172077,#172078,#172079,#172080,
#172081,#172082,#172083,#172084,#172085,#172086,#172087,#172088,#172089,
#172090,#172091,#172092,#172093,#172094,#172095,#172096,#172097,#172098,
#172099,#172100),.UNSPECIFIED.,.F.,.F.,(4,3,3,3,3,3,3,3,4),(0.,0.374999999999775,
0.437499999999737,0.468749999999718,0.484374999999709,0.499511718749699,
0.499999999999699,0.888987273624248,1.),.UNSPECIFIED.);
#5123=B_SPLINE_CURVE_WITH_KNOTS('',3,(#172120,#172121,#172122,#172123,#172124,
#172125,#172126,#172127,#172128,#172129,#172130,#172131,#172132,#172133,
#172134,#172135,#172136,#172137,#172138,#172139,#172140,#172141,#172142,
#172143,#172144,#172145,#172146,#172147,#172148,#172149,#172150),
 .UNSPECIFIED.,.F.,.F.,(4,3,3,3,3,3,3,3,3,3,4),(0.,0.184213842299516,0.384184423243072,
0.484375000000021,0.498581836652927,0.500000000000022,0.512531515748722,
0.644734984770559,0.776535034074271,0.907370191348794,1.),.UNSPECIFIED.);
#5124=B_SPLINE_CURVE_WITH_KNOTS('',3,(#172151,#172152,#172153,#172154,#172155,
#172156,#172157,#172158,#172159,#172160,#172161,#172162,#172163,#172164,
#172165,#172166,#172167,#172168,#172169,#172170,#172171,#172172,#172173,
#172174,#172175,#172176,#172177,#172178,#172179,#172180,#172181,#172182,
#172183,#172184,#172185,#172186,#172187,#172188,#172189,#172190,#172191,
#172192,#172193,#172194,#172195,#172196,#172197,#172198,#172199,#172200,
#172201,#172202,#172203,#172204,#172205,#172206,#172207,#172208),
 .UNSPECIFIED.,.F.,.F.,(4,3,3,3,3,3,3,3,3,3,3,3,3,3,3,3,3,3,3,4),(0.,0.0625000000000331,
0.125000000000066,0.175859082344618,0.224397356720149,0.250000000000132,
0.307328937444154,0.365341671430271,0.424129973950711,0.437500000000222,
0.468750000000235,0.484375000000231,0.492187500000216,0.496093750000209,
0.500000000000202,0.59834670848804,0.700014659932125,0.803605996460746,
0.910590148948139,1.),.UNSPECIFIED.);
#5125=B_SPLINE_CURVE_WITH_KNOTS('',3,(#172231,#172232,#172233,#172234,#172235,
#172236,#172237,#172238,#172239,#172240,#172241,#172242,#172243),
 .UNSPECIFIED.,.F.,.F.,(4,3,3,3,4),(0.,0.000727903814955922,0.00111811425806593,
0.00207062545858035,0.00223622851613186),.UNSPECIFIED.);
#5126=B_SPLINE_CURVE_WITH_KNOTS('',3,(#172268,#172269,#172270,#172271,#172272,
#172273,#172274,#172275,#172276,#172277,#172278,#172279,#172280),
 .UNSPECIFIED.,.F.,.F.,(4,3,3,3,4),(0.,0.000659089694855302,0.00111822884501791,
0.002081283710365,0.00223645769003581),.UNSPECIFIED.);
#5127=B_SPLINE_CURVE_WITH_KNOTS('',3,(#172360,#172361,#172362,#172363,#172364,
#172365,#172366,#172367,#172368,#172369,#172370,#172371,#172372,#172373,
#172374,#172375,#172376,#172377,#172378,#172379,#172380,#172381,#172382,
#172383,#172384,#172385,#172386,#172387,#172388,#172389,#172390,#172391,
#172392,#172393),.UNSPECIFIED.,.F.,.F.,(4,3,3,3,3,3,3,3,3,3,3,4),(0.,0.000275770613304119,
0.000551541226608238,0.000716520337534457,0.0010747839077808,0.00110308245321648,
0.00134771653693952,0.00143334685918384,0.00165462367982471,0.00179132390797124,
0.00214954043896842,0.00220616490643295),.UNSPECIFIED.);
#5128=B_SPLINE_CURVE_WITH_KNOTS('',3,(#172408,#172409,#172410,#172411,#172412,
#172413,#172414,#172415,#172416,#172417,#172418,#172419,#172420,#172421,
#172422),.UNSPECIFIED.,.F.,.F.,(4,2,2,1,1,1,2,2,4),(0.,0.250000000000171,
0.375000000000256,0.437500000000298,0.46875000000032,0.484375000000331,
0.499511718750343,0.500000000000343,1.),.UNSPECIFIED.);
#5129=B_SPLINE_CURVE_WITH_KNOTS('',3,(#172437,#172438,#172439,#172440),
 .UNSPECIFIED.,.F.,.F.,(4,4),(0.0206793054465132,0.021179777605653),
 .UNSPECIFIED.);
#5130=B_SPLINE_CURVE_WITH_KNOTS('',3,(#172490,#172491,#172492,#172493,#172494,
#172495,#172496,#172497,#172498,#172499,#172500,#172501,#172502,#172503,
#172504,#172505,#172506,#172507,#172508,#172509,#172510,#172511,#172512,
#172513,#172514,#172515,#172516,#172517,#172518,#172519,#172520,#172521,
#172522,#172523,#172524,#172525,#172526),.UNSPECIFIED.,.F.,.F.,(4,3,3,3,
3,3,3,3,3,3,3,3,4),(0.000467059137334316,0.000632797502959653,0.00086096130564352,
0.000897131574002738,0.00113001259983567,0.00126720169019539,0.00163753656891931,
0.00179296606233701,0.00200786773946722,0.00237820352986643,0.00245591952483837,
0.0030162112996301,0.00311887298733972),.UNSPECIFIED.);
#5131=B_SPLINE_CURVE_WITH_KNOTS('',3,(#172560,#172561,#172562,#172563),
 .UNSPECIFIED.,.F.,.F.,(4,4),(0.,0.0420570108120997),.UNSPECIFIED.);
#5132=B_SPLINE_CURVE_WITH_KNOTS('',3,(#172584,#172585,#172586,#172587,#172588,
#172589,#172590,#172591,#172592,#172593,#172594,#172595,#172596),
 .UNSPECIFIED.,.F.,.F.,(4,3,3,3,4),(0.,0.000795137544078952,0.00122134837748785,
0.00219865189862556,0.00244269675497567),.UNSPECIFIED.);
#5133=B_SPLINE_CURVE_WITH_KNOTS('',3,(#172621,#172622,#172623,#172624,#172625,
#172626,#172627,#172628,#172629,#172630,#172631,#172632,#172633),
 .UNSPECIFIED.,.F.,.F.,(4,3,3,3,4),(0.,0.000894380560743248,0.00122171954771057,
0.00222146414309688,0.00244343909542114),.UNSPECIFIED.);
#5134=B_SPLINE_CURVE_WITH_KNOTS('',3,(#172636,#172637,#172638,#172639,#172640,
#172641,#172642,#172643,#172644,#172645,#172646,#172647,#172648,#172649,
#172650,#172651,#172652,#172653,#172654,#172655,#172656,#172657,#172658,
#172659,#172660,#172661,#172662,#172663,#172664,#172665,#172666,#172667,
#172668,#172669,#172670,#172671,#172672,#172673,#172674,#172675,#172676,
#172677,#172678,#172679,#172680,#172681,#172682,#172683,#172684,#172685,
#172686,#172687,#172688,#172689,#172690,#172691,#172692,#172693,#172694,
#172695,#172696,#172697,#172698,#172699),.UNSPECIFIED.,.F.,.F.,(4,3,3,3,
3,3,3,3,3,3,3,3,3,3,3,3,3,3,3,3,3,4),(0.,0.117678986907631,0.212770958931128,
0.274508663183841,0.376875434432681,0.475298330914508,0.49804687500162,
0.500000000001621,0.500228117075086,0.54311799305188,0.585976806827622,
0.62500000000116,0.667538069824397,0.709029432927037,0.73437500000076,0.742187500000732,
0.746093750000722,0.750000000000712,0.814123113213129,0.87948779349594,
0.946280975523161,0.999984983959274),.UNSPECIFIED.);
#5135=B_SPLINE_CURVE_WITH_KNOTS('',3,(#172713,#172714,#172715,#172716),
 .UNSPECIFIED.,.F.,.F.,(4,4),(0.,0.0417901757617078),.UNSPECIFIED.);
#5136=B_SPLINE_CURVE_WITH_KNOTS('',3,(#172719,#172720,#172721,#172722,#172723,
#172724,#172725,#172726,#172727,#172728,#172729,#172730,#172731,#172732,
#172733,#172734),.UNSPECIFIED.,.F.,.F.,(4,2,2,1,1,1,1,2,2,4),(0.,0.249999999999767,
0.374999999999651,0.437499999999593,0.468749999999564,0.484374999999549,
0.492187499999542,0.499511718749537,0.499999999999538,1.),.UNSPECIFIED.);
#5137=B_SPLINE_CURVE_WITH_KNOTS('',3,(#172760,#172761,#172762,#172763,#172764,
#172765,#172766,#172767,#172768,#172769,#172770,#172771,#172772,#172773,
#172774,#172775,#172776,#172777,#172778,#172779,#172780,#172781,#172782,
#172783,#172784),.UNSPECIFIED.,.F.,.F.,(4,3,3,3,3,3,3,3,4),(0.,0.234918010763658,
0.268228507342618,0.382645199292437,0.503001406327853,0.555176579325945,
0.757548181588527,0.935344993134881,0.999999537405455),.UNSPECIFIED.);
#5138=B_SPLINE_CURVE_WITH_KNOTS('',3,(#172785,#172786,#172787,#172788,#172789,
#172790,#172791,#172792,#172793,#172794,#172795,#172796,#172797,#172798,
#172799,#172800,#172801,#172802,#172803,#172804,#172805,#172806,#172807,
#172808,#172809,#172810,#172811,#172812,#172813,#172814,#172815,#172816,
#172817,#172818,#172819,#172820,#172821,#172822,#172823,#172824,#172825,
#172826,#172827,#172828,#172829,#172830,#172831,#172832,#172833,#172834,
#172835,#172836,#172837,#172838,#172839,#172840,#172841,#172842,#172843,
#172844,#172845,#172846,#172847,#172848,#172849,#172850,#172851,#172852,
#172853,#172854,#172855,#172856,#172857,#172858,#172859,#172860,#172861,
#172862,#172863),.UNSPECIFIED.,.F.,.F.,(4,3,3,3,3,3,3,3,3,3,3,3,3,3,3,3,
3,3,3,3,3,3,3,3,3,3,4),(8.70442931586916E-9,0.0902335702297538,0.125000000001714,
0.187500000002585,0.21875000000302,0.234375000003238,0.242187500003347,
0.246093750003401,0.248046875003428,0.250000000003456,0.285027994706698,
0.320202466330442,0.355598103085239,0.388926552204718,0.425197759906794,
0.462045466695683,0.498046875001628,0.500000000001617,0.500299813510911,
0.568943255332965,0.625000000001213,0.700077040250471,0.750000000000809,
0.827937432249017,0.9081222359888,0.991289142222388,1.),.UNSPECIFIED.);
#5139=B_SPLINE_CURVE_WITH_KNOTS('',3,(#172886,#172887,#172888,#172889,#172890,
#172891,#172892,#172893,#172894,#172895,#172896,#172897,#172898,#172899,
#172900,#172901),.UNSPECIFIED.,.F.,.F.,(4,3,3,3,3,4),(0.,0.000540889688193889,
0.00109121002634669,0.00153442409609832,0.00256481294069276,0.00306884819219665),
 .UNSPECIFIED.);
#5140=B_SPLINE_CURVE_WITH_KNOTS('',3,(#172925,#172926,#172927,#172928,#172929,
#172930,#172931,#172932,#172933,#172934,#172935,#172936,#172937),
 .UNSPECIFIED.,.F.,.F.,(4,3,3,3,4),(2.8609792490764E-17,0.000811916222429989,
0.00153648298481487,0.00264039900673923,0.0030729659696297),
 .UNSPECIFIED.);
#5141=B_SPLINE_CURVE_WITH_KNOTS('',3,(#172958,#172959,#172960,#172961,#172962,
#172963,#172964),.UNSPECIFIED.,.F.,.F.,(4,3,4),(0.,0.018990790064314,0.0379815801286281),
 .UNSPECIFIED.);
#5142=B_SPLINE_CURVE_WITH_KNOTS('',3,(#173011,#173012,#173013,#173014,#173015,
#173016,#173017,#173018,#173019,#173020,#173021,#173022,#173023,#173024,
#173025,#173026,#173027,#173028,#173029,#173030,#173031,#173032,#173033,
#173034,#173035,#173036,#173037,#173038,#173039,#173040,#173041,#173042,
#173043,#173044,#173045,#173046,#173047,#173048,#173049,#173050,#173051,
#173052,#173053),.UNSPECIFIED.,.F.,.F.,(4,3,3,3,3,3,3,3,3,3,3,3,3,3,4),
(0.,0.152946157858152,0.249999999999975,0.374999999999963,0.437499999999957,
0.468749999999955,0.484374999999953,0.492187499999951,0.499023437499951,
0.499999999999952,0.500017274533875,0.625012955900406,0.75266030275651,
0.885972940012859,1.),.UNSPECIFIED.);
#5143=B_SPLINE_CURVE_WITH_KNOTS('',3,(#173056,#173057,#173058,#173059,#173060,
#173061,#173062),.UNSPECIFIED.,.F.,.F.,(4,3,4),(0.,0.0188568492058762,0.0377136984117524),
 .UNSPECIFIED.);
#5144=B_SPLINE_CURVE_WITH_KNOTS('',3,(#173128,#173129,#173130,#173131,#173132,
#173133,#173134),.UNSPECIFIED.,.F.,.F.,(4,3,4),(0.,0.0178323395635859,0.0356646791271718),
 .UNSPECIFIED.);
#5145=B_SPLINE_CURVE_WITH_KNOTS('',3,(#173155,#173156,#173157,#173158,#173159,
#173160,#173161,#173162),.UNSPECIFIED.,.F.,.F.,(4,2,2,4),(0.,0.000848531500815463,
0.00169706300163092,0.00339412600326177),.UNSPECIFIED.);
#5146=B_SPLINE_CURVE_WITH_KNOTS('',3,(#173189,#173190,#173191,#173192,#173193,
#173194,#173195,#173196,#173197,#173198,#173199,#173200,#173201,#173202,
#173203,#173204,#173205,#173206,#173207,#173208,#173209,#173210,#173211,
#173212,#173213,#173214,#173215,#173216,#173217,#173218,#173219,#173220,
#173221,#173222,#173223,#173224,#173225,#173226,#173227,#173228,#173229,
#173230,#173231,#173232,#173233,#173234,#173235,#173236,#173237,#173238,
#173239,#173240,#173241,#173242,#173243,#173244,#173245,#173246,#173247,
#173248,#173249,#173250,#173251,#173252,#173253,#173254,#173255,#173256,
#173257,#173258,#173259,#173260,#173261,#173262,#173263,#173264,#173265,
#173266,#173267,#173268,#173269,#173270,#173271,#173272,#173273,#173274,
#173275,#173276,#173277,#173278,#173279,#173280,#173281,#173282,#173283,
#173284,#173285),.UNSPECIFIED.,.F.,.F.,(4,3,3,3,3,3,3,3,3,3,3,3,3,3,3,3,
3,3,3,3,3,3,3,3,3,3,3,3,3,3,3,3,4),(0.,0.0932635068722853,0.173120445513539,
0.212027264824284,0.246070731721185,0.246374889451879,0.248234265315532,
0.24923556874209,0.249694825443765,0.249937243565367,0.250147139192889,
0.308730107077419,0.365357971714009,0.424866485856754,0.484374999999498,
0.49535871603758,0.499770916189278,0.499999999999506,0.547691012729422,
0.596740786897328,0.624999999999556,0.674962700199832,0.687499999999575,
0.718749999999584,0.734374999999581,0.742187499999577,0.746093749999584,
0.748046874999589,0.749999999999594,0.824471881370616,0.901151261803454,
0.980838602588325,0.999982733045328),.UNSPECIFIED.);
#5147=B_SPLINE_CURVE_WITH_KNOTS('',3,(#173286,#173287,#173288,#173289,#173290,
#173291,#173292,#173293,#173294,#173295,#173296,#173297,#173298,#173299,
#173300,#173301),.UNSPECIFIED.,.F.,.F.,(4,3,3,3,3,4),(0.,0.000761157739917319,
0.00156083390161805,0.00170051723463269,0.00285526923554342,0.00340103446926538),
 .UNSPECIFIED.);
#5148=B_SPLINE_CURVE_WITH_KNOTS('',3,(#173323,#173324,#173325,#173326,#173327,
#173328,#173329,#173330,#173331,#173332,#173333,#173334,#173335,#173336,
#173337,#173338,#173339,#173340,#173341,#173342,#173343,#173344,#173345,
#173346,#173347,#173348,#173349,#173350,#173351,#173352,#173353),
 .UNSPECIFIED.,.F.,.F.,(4,3,3,3,3,3,3,3,3,3,4),(0.,0.131009823433625,0.258234932379081,
0.38109330009218,0.499023437500229,0.499974366980884,0.500000000000229,
0.659817335393859,0.815466379844275,0.966024828559954,1.),.UNSPECIFIED.);
#5149=B_SPLINE_CURVE_WITH_KNOTS('',3,(#173354,#173355,#173356,#173357,#173358,
#173359,#173360),.UNSPECIFIED.,.F.,.F.,(4,3,4),(0.,0.0176980703187956,0.0353961406375911),
 .UNSPECIFIED.);
#5150=B_SPLINE_CURVE_WITH_KNOTS('',3,(#173380,#173381,#173382,#173383,#173384,
#173385,#173386,#173387,#173388,#173389,#173390,#173391,#173392,#173393,
#173394,#173395),.UNSPECIFIED.,.F.,.F.,(4,3,3,3,3,4),(0.,0.192339441584989,
0.407181235959237,0.610051883739392,0.855180865457149,0.999999198430051),
 .UNSPECIFIED.);
#5151=B_SPLINE_CURVE_WITH_KNOTS('',3,(#173396,#173397,#173398,#173399,#173400,
#173401,#173402,#173403,#173404,#173405,#173406,#173407,#173408,#173409,
#173410,#173411,#173412,#173413,#173414,#173415,#173416,#173417,#173418,
#173419,#173420,#173421,#173422,#173423,#173424,#173425,#173426,#173427,
#173428,#173429,#173430,#173431,#173432,#173433,#173434,#173435,#173436,
#173437,#173438,#173439,#173440,#173441,#173442,#173443,#173444,#173445,
#173446,#173447,#173448,#173449,#173450,#173451,#173452,#173453,#173454,
#173455,#173456,#173457,#173458,#173459,#173460,#173461,#173462,#173463,
#173464,#173465,#173466,#173467,#173468,#173469,#173470,#173471,#173472,
#173473,#173474,#173475,#173476,#173477,#173478,#173479,#173480,#173481,
#173482,#173483,#173484,#173485,#173486,#173487,#173488,#173489,#173490,
#173491,#173492,#173493,#173494,#173495,#173496,#173497,#173498,#173499,
#173500,#173501),.UNSPECIFIED.,.F.,.F.,(4,3,3,3,3,3,3,3,3,3,3,3,3,3,3,3,
3,3,3,3,3,3,3,3,3,3,3,3,3,3,3,3,3,3,3,4),(0.,0.0751687560234797,0.124999999999828,
0.187499999999744,0.218749999999701,0.23437499999968,0.24218749999967,0.246093749999667,
0.249999999999665,0.306700379523328,0.362571924844633,0.417147083320517,
0.437500000000012,0.468750000000065,0.484375000000091,0.492187500000101,
0.496093750000106,0.498046875000108,0.500000000000111,0.532145122746275,
0.564912906759694,0.598491128155236,0.632424031668225,0.666766974875665,
0.68750000000056,0.718750000000641,0.734375000000671,0.742187500000699,
0.746093750000697,0.748046875000696,0.749023437500695,0.750000000000694,
0.817229294988516,0.885907714625437,0.956984553878538,1.),.UNSPECIFIED.);
#5152=B_SPLINE_CURVE_WITH_KNOTS('',3,(#173534,#173535,#173536,#173537,#173538,
#173539,#173540),.UNSPECIFIED.,.F.,.F.,(4,3,4),(0.,0.014563917689728,0.029127835379456),
 .UNSPECIFIED.);
#5153=B_SPLINE_CURVE_WITH_KNOTS('',3,(#173542,#173543,#173544,#173545,#173546,
#173547,#173548,#173549,#173550,#173551,#173552,#173553,#173554,#173555,
#173556,#173557,#173558,#173559,#173560,#173561,#173562,#173563,#173564,
#173565,#173566,#173567,#173568,#173569,#173570,#173571,#173572,#173573,
#173574,#173575,#173576,#173577,#173578,#173579,#173580,#173581),
 .UNSPECIFIED.,.F.,.F.,(4,3,3,3,3,3,3,3,3,3,3,3,3,4),(0.,0.153641825342759,
0.249999999999996,0.374999999999994,0.437499999999993,0.468749999999993,
0.484374999999993,0.49902343749999,0.499999999999989,0.500006129759065,
0.629863266340263,0.762254527670502,0.899175022789813,1.),.UNSPECIFIED.);
#5154=B_SPLINE_CURVE_WITH_KNOTS('',3,(#173601,#173602,#173603,#173604,#173605,
#173606,#173607,#173608,#173609,#173610,#173611,#173612,#173613,#173614,
#173615,#173616,#173617,#173618,#173619,#173620,#173621,#173622,#173623,
#173624,#173625),.UNSPECIFIED.,.F.,.F.,(4,3,3,3,3,3,3,3,4),(0.,0.000422069097417445,
0.000847931637827783,0.00104448509574678,0.00149181651230484,0.00193535496126402,
0.00208897019149356,0.00315378543072143,0.00417794038298713),
 .UNSPECIFIED.);
#5155=B_SPLINE_CURVE_WITH_KNOTS('',3,(#173650,#173651,#173652,#173653,#173654,
#173655,#173656,#173657,#173658,#173659,#173660,#173661,#173662,#173663,
#173664,#173665,#173666,#173667,#173668,#173669,#173670,#173671),
 .UNSPECIFIED.,.F.,.F.,(4,3,3,3,3,3,3,4),(0.,0.000384591749545137,0.00078374926263879,
0.00104647183020208,0.00173887398626118,0.00209294366040415,0.00337921840668196,
0.00418588732080839),.UNSPECIFIED.);
#5156=B_SPLINE_CURVE_WITH_KNOTS('',3,(#173692,#173693,#173694,#173695,#173696,
#173697,#173698),.UNSPECIFIED.,.F.,.F.,(4,3,4),(0.,0.0146992078328598,0.0293984156657196),
 .UNSPECIFIED.);
#5157=B_SPLINE_CURVE_WITH_KNOTS('',3,(#173764,#173765,#173766,#173767,#173768,
#173769,#173770,#173771,#173772,#173773,#173774,#173775,#173776,#173777),
 .UNSPECIFIED.,.F.,.F.,(4,2,1,1,1,1,2,2,4),(0.,0.249999999999965,0.374999999999947,
0.437499999999939,0.468749999999935,0.484374999999932,0.49902343749993,
0.49999999999993,1.),.UNSPECIFIED.);
#5158=B_SPLINE_CURVE_WITH_KNOTS('',3,(#173800,#173801,#173802,#173803),
 .UNSPECIFIED.,.F.,.F.,(4,4),(3.46944695195361E-18,0.0333425790106738),
 .UNSPECIFIED.);
#5159=B_SPLINE_CURVE_WITH_KNOTS('',3,(#173806,#173807,#173808,#173809,#173810,
#173811,#173812,#173813,#173814,#173815,#173816,#173817,#173818,#173819),
 .UNSPECIFIED.,.F.,.F.,(4,2,1,1,1,1,2,2,4),(0.,0.250000000000072,0.375000000000108,
0.437500000000126,0.468750000000135,0.484375000000139,0.499023437500143,
0.500000000000143,1.),.UNSPECIFIED.);
#5160=B_SPLINE_CURVE_WITH_KNOTS('',3,(#173839,#173840,#173841,#173842),
 .UNSPECIFIED.,.F.,.F.,(4,4),(0.,9.64176041888327E-5),.UNSPECIFIED.);
#5161=B_SPLINE_CURVE_WITH_KNOTS('',3,(#173858,#173859,#173860,#173861,#173862,
#173863,#173864,#173865,#173866,#173867,#173868,#173869,#173870,#173871,
#173872,#173873,#173874,#173875,#173876),.UNSPECIFIED.,.F.,.F.,(4,3,3,3,
3,3,4),(0.,0.190207366592191,0.372524918669027,0.545027215306253,0.713431358990858,
0.875775939334647,1.),.UNSPECIFIED.);
#5162=B_SPLINE_CURVE_WITH_KNOTS('',3,(#173877,#173878,#173879,#173880),
 .UNSPECIFIED.,.F.,.F.,(4,4),(0.,0.0333345873458536),.UNSPECIFIED.);
#5163=B_SPLINE_CURVE_WITH_KNOTS('',3,(#173897,#173898,#173899,#173900),
 .UNSPECIFIED.,.F.,.F.,(4,4),(0.,0.0278605201857756),.UNSPECIFIED.);
#5164=B_SPLINE_CURVE_WITH_KNOTS('',3,(#173903,#173904,#173905,#173906,#173907,
#173908,#173909,#173910,#173911,#173912,#173913,#173914,#173915,#173916,
#173917,#173918,#173919,#173920,#173921),.UNSPECIFIED.,.F.,.F.,(4,3,3,3,
3,3,4),(0.,0.161013821218371,0.325610113125001,0.496657244829195,0.671778199953257,
0.854525113432085,1.),.UNSPECIFIED.);
#5165=B_SPLINE_CURVE_WITH_KNOTS('',3,(#173941,#173942,#173943,#173944,#173945,
#173946,#173947,#173948),.UNSPECIFIED.,.F.,.F.,(4,2,2,4),(0.,0.000890496769046365,
0.00178099353809273,0.0035619870761855),.UNSPECIFIED.);
#5166=B_SPLINE_CURVE_WITH_KNOTS('',3,(#173951,#173952,#173953,#173954,#173955,
#173956,#173957,#173958,#173959,#173960,#173961,#173962,#173963,#173964,
#173965,#173966,#173967,#173968,#173969,#173970,#173971,#173972,#173973,
#173974,#173975,#173976,#173977,#173978,#173979,#173980,#173981,#173982,
#173983,#173984,#173985,#173986,#173987,#173988,#173989,#173990,#173991,
#173992,#173993,#173994,#173995,#173996,#173997,#173998,#173999,#174000,
#174001,#174002,#174003,#174004,#174005,#174006,#174007,#174008,#174009,
#174010,#174011,#174012,#174013,#174014,#174015,#174016,#174017,#174018,
#174019,#174020,#174021,#174022,#174023,#174024,#174025,#174026,#174027,
#174028,#174029,#174030,#174031,#174032,#174033,#174034,#174035,#174036,
#174037,#174038,#174039,#174040,#174041,#174042,#174043,#174044,#174045,
#174046,#174047,#174048,#174049,#174050,#174051,#174052,#174053),
 .UNSPECIFIED.,.F.,.F.,(4,3,3,3,3,3,3,3,3,3,3,3,3,3,3,3,3,3,3,3,3,3,3,3,
3,3,3,3,3,3,3,3,3,3,4),(1.57528194328481E-8,0.113390184051606,0.125000000000386,
0.208213799444507,0.242733949514119,0.244621770221051,0.24555830627488,
0.246025309240556,0.246288313900857,0.248148366136017,0.249993886713091,
0.250183242419508,0.305303406015141,0.358943150387979,0.415198367832281,
0.470499806007569,0.484375000001403,0.496707221246892,0.500000000001438,
0.500644507573531,0.545230766738762,0.591400861254902,0.625000000001714,
0.672876488128917,0.687500000001858,0.71875000000193,0.734375000001958,
0.742187500001965,0.746093750001959,0.748046875001948,0.750000000001936,
0.823877912198341,0.899739373902168,0.97859232774702,1.),.UNSPECIFIED.);
#5167=B_SPLINE_CURVE_WITH_KNOTS('',3,(#174109,#174110,#174111,#174112,#174113,
#174114,#174115,#174116,#174117,#174118,#174119,#174120,#174121,#174122,
#174123,#174124),.UNSPECIFIED.,.F.,.F.,(4,3,3,3,3,4),(0.,0.000625284942165368,
0.0012890528199733,0.00194949793575932,0.00318811191752231,0.00389899587151865),
 .UNSPECIFIED.);
#5168=B_SPLINE_CURVE_WITH_KNOTS('',3,(#174140,#174141,#174142,#174143,#174144,
#174145,#174146,#174147,#174148,#174149,#174150,#174151,#174152,#174153,
#174154,#174155,#174156,#174157,#174158),.UNSPECIFIED.,.F.,.F.,(4,3,3,3,
3,3,4),(0.,0.19217742618272,0.378585784323496,0.557722246321134,0.733231503446162,
0.903822311654046,1.),.UNSPECIFIED.);
#5169=B_SPLINE_CURVE_WITH_KNOTS('',3,(#174159,#174160,#174161,#174162),
 .UNSPECIFIED.,.F.,.F.,(4,4),(0.,0.024690830875569),.UNSPECIFIED.);
#5170=B_SPLINE_CURVE_WITH_KNOTS('',3,(#174190,#174191,#174192,#174193,#174194,
#174195,#174196,#174197,#174198,#174199,#174200,#174201,#174202,#174203,
#174204,#174205,#174206,#174207,#174208),.UNSPECIFIED.,.F.,.F.,(4,3,3,3,
3,3,4),(0.,0.000151109125705162,0.000302236517833045,0.000386300967573271,
0.000471902393705294,0.00055523437621895,0.000604473035666092),
 .UNSPECIFIED.);
#5171=B_SPLINE_CURVE_WITH_KNOTS('',3,(#174209,#174210,#174211,#174212,#174213,
#174214,#174215,#174216,#174217,#174218,#174219,#174220,#174221,#174222,
#174223,#174224,#174225,#174226,#174227,#174228,#174229,#174230,#174231,
#174232,#174233,#174234,#174235,#174236,#174237,#174238,#174239,#174240,
#174241,#174242,#174243,#174244,#174245,#174246,#174247,#174248,#174249,
#174250,#174251,#174252,#174253,#174254,#174255,#174256,#174257,#174258,
#174259,#174260,#174261,#174262,#174263),.UNSPECIFIED.,.F.,.F.,(4,3,3,3,
3,3,3,3,3,3,3,3,3,3,3,3,3,3,4),(0.,0.0579960117174044,0.118910654037608,
0.125000000000006,0.215056456326176,0.247031472716539,0.282964889031184,
0.361398792416325,0.433567066284115,0.476592509119368,0.485225825304686,
0.492187500000023,0.49881285509328,0.500000000000011,0.586335878991574,
0.6759254922935,0.728649541045074,0.876166749959378,1.),.UNSPECIFIED.);
#5172=B_SPLINE_CURVE_WITH_KNOTS('',3,(#174315,#174316,#174317,#174318),
 .UNSPECIFIED.,.F.,.F.,(4,4),(0.,0.0240963563036403),.UNSPECIFIED.);
#5173=B_SPLINE_CURVE_WITH_KNOTS('',3,(#174320,#174321,#174322,#174323,#174324,
#174325,#174326,#174327,#174328,#174329,#174330,#174331,#174332,#174333,
#174334,#174335,#174336,#174337,#174338),.UNSPECIFIED.,.F.,.F.,(4,3,3,3,
3,3,4),(0.,0.172866351701051,0.349384406750267,0.532176733764,0.719026799190666,
0.912787151767933,1.),.UNSPECIFIED.);
#5174=B_SPLINE_CURVE_WITH_KNOTS('',3,(#174358,#174359,#174360,#174361,#174362,
#174363,#174364,#174365,#174366,#174367,#174368,#174369,#174370,#174371,
#174372,#174373,#174374,#174375,#174376,#174377,#174378,#174379,#174380,
#174381,#174382),.UNSPECIFIED.,.F.,.F.,(4,3,3,3,3,3,3,3,4),(0.,0.000403252952291858,
0.000810273659957097,0.000991778862067342,0.00143365237214696,0.00187173698199696,
0.00198355772413468,0.00304641612723371,0.00396711544826929),
 .UNSPECIFIED.);
#5175=B_SPLINE_CURVE_WITH_KNOTS('',3,(#174407,#174408,#174409,#174410,#174411,
#174412,#174413,#174414,#174415,#174416,#174417,#174418,#174419,#174420,
#174421,#174422,#174423,#174424,#174425),.UNSPECIFIED.,.F.,.F.,(4,3,3,3,
3,3,4),(0.,0.000606703134123652,0.00123626357061655,0.00189155006086063,
0.00198795077588647,0.0032403373659691,0.00397590155177294),
 .UNSPECIFIED.);
#5176=B_SPLINE_CURVE_WITH_KNOTS('',3,(#174428,#174429,#174430,#174431,#174432,
#174433,#174434,#174435,#174436,#174437,#174438,#174439,#174440,#174441,
#174442,#174443,#174444,#174445,#174446,#174447,#174448,#174449,#174450,
#174451,#174452,#174453,#174454,#174455,#174456,#174457,#174458,#174459,
#174460,#174461,#174462,#174463,#174464,#174465,#174466),.UNSPECIFIED.,
 .F.,.F.,(4,2,2,1,1,1,1,2,2,2,2,2,1,1,2,2,2,2,1,1,1,2,2,4),(0.,0.124999999999855,
0.187499999999778,0.218749999999739,0.23437499999972,0.242187499999711,
0.246093749999706,0.248046874999704,0.249999999999701,0.374999999999798,
0.437499999999845,0.468749999999869,0.484374999999881,0.492187499999884,
0.496093749999882,0.499999999999881,0.624999999999869,0.687499999999859,
0.718749999999854,0.734374999999848,0.742187499999838,0.74609374999984,
0.749999999999841,0.999999987824138),.UNSPECIFIED.);
#5177=B_SPLINE_CURVE_WITH_KNOTS('',3,(#174480,#174481,#174482,#174483),
 .UNSPECIFIED.,.F.,.F.,(4,4),(0.,0.0238258198664154),.UNSPECIFIED.);
#5178=B_SPLINE_CURVE_WITH_KNOTS('',3,(#174486,#174487,#174488,#174489,#174490,
#174491,#174492,#174493,#174494,#174495,#174496,#174497,#174498,#174499,
#174500,#174501,#174502,#174503,#174504),.UNSPECIFIED.,.F.,.F.,(4,3,3,3,
3,3,4),(0.,0.196095667009585,0.386442595766244,0.569588535581485,0.749087760231935,
0.923761630375088,1.),.UNSPECIFIED.);
#5179=B_SPLINE_CURVE_WITH_KNOTS('',3,(#174524,#174525,#174526,#174527,#174528,
#174529,#174530,#174531,#174532,#174533,#174534,#174535,#174536,#174537,
#174538,#174539,#174540,#174541,#174542),.UNSPECIFIED.,.F.,.F.,(4,3,3,3,
3,3,4),(6.48727906844412E-7,0.345786654980507,0.395757238724258,0.59010138294459,
0.774910284816947,0.948267161783481,1.),.UNSPECIFIED.);
#5180=B_SPLINE_CURVE_WITH_KNOTS('',3,(#174543,#174544,#174545,#174546,#174547,
#174548,#174549,#174550,#174551,#174552,#174553,#174554,#174555,#174556,
#174557,#174558,#174559,#174560,#174561,#174562,#174563,#174564,#174565,
#174566,#174567,#174568,#174569,#174570,#174571,#174572,#174573,#174574,
#174575,#174576,#174577,#174578),.UNSPECIFIED.,.F.,.F.,(4,2,2,1,1,1,1,2,
2,2,2,1,2,2,2,2,2,2,1,2,4),(1.49874026637454E-5,0.124999999999844,0.187499999999766,
0.218749999999723,0.234374999999695,0.242187499999681,0.246093749999674,
0.248046874999672,0.249999999999669,0.374999999999717,0.437499999999741,
0.468749999999749,0.484374999999748,0.499999999999747,0.749999999999862,
0.812499999999884,0.828124999999901,0.83593749999991,0.843749999999918,
0.87499999999993,1.),.UNSPECIFIED.);
#5181=B_SPLINE_CURVE_WITH_KNOTS('',3,(#174611,#174612,#174613,#174614,#174615,
#174616,#174617,#174618,#174619,#174620,#174621,#174622,#174623,#174624,
#174625,#174626),.UNSPECIFIED.,.F.,.F.,(4,3,3,3,3,4),(0.,0.000531847314912768,
0.0010759631561301,0.00162007899734744,0.00266000146296125,0.00324015799469487),
 .UNSPECIFIED.);
#5182=B_SPLINE_CURVE_WITH_KNOTS('',3,(#174651,#174652,#174653,#174654,#174655,
#174656,#174657,#174658,#174659,#174660,#174661,#174662,#174663),
 .UNSPECIFIED.,.F.,.F.,(4,3,3,3,4),(0.,0.000817558298551379,0.00162295210526764,
0.00275577655351122,0.00324590421053527),.UNSPECIFIED.);
#5183=B_SPLINE_CURVE_WITH_KNOTS('',3,(#174679,#174680,#174681,#174682,#174683,
#174684,#174685,#174686,#174687,#174688,#174689,#174690,#174691,#174692,
#174693,#174694,#174695,#174696,#174697),.UNSPECIFIED.,.F.,.F.,(4,3,3,3,
3,3,4),(0.,0.185664878352089,0.364657978690721,0.534856302418504,0.701562136952496,
0.862722007449341,1.),.UNSPECIFIED.);
#5184=B_SPLINE_CURVE_WITH_KNOTS('',3,(#174698,#174699,#174700,#174701),
 .UNSPECIFIED.,.F.,.F.,(4,4),(0.,0.0300693678107436),.UNSPECIFIED.);
#5185=B_SPLINE_CURVE_WITH_KNOTS('',3,(#174715,#174716,#174717,#174718,#174719,
#174720,#174721,#174722,#174723,#174724,#174725,#174726,#174727,#174728,
#174729,#174730,#174731,#174732,#174733),.UNSPECIFIED.,.F.,.F.,(4,3,3,3,
3,3,4),(0.,0.161837694415199,0.327487306305213,0.499540509367366,0.675600434337124,
0.860932038423597,1.),.UNSPECIFIED.);
#5186=B_SPLINE_CURVE_WITH_KNOTS('',3,(#174736,#174737,#174738,#174739),
 .UNSPECIFIED.,.F.,.F.,(4,4),(0.,0.0298008594779328),.UNSPECIFIED.);
#5187=B_SPLINE_CURVE_WITH_KNOTS('',3,(#174780,#174781,#174782,#174783),
 .UNSPECIFIED.,.F.,.F.,(4,4),(0.,0.0322629186945109),.UNSPECIFIED.);
#5188=B_SPLINE_CURVE_WITH_KNOTS('',3,(#174785,#174786,#174787,#174788,#174789,
#174790,#174791,#174792,#174793,#174794,#174795,#174796,#174797,#174798,
#174799,#174800,#174801,#174802,#174803),.UNSPECIFIED.,.F.,.F.,(4,3,3,3,
3,3,4),(0.,0.159102637702074,0.329551318851037,0.5,0.684750559143937,0.882446988411837,
1.),.UNSPECIFIED.);
#5189=B_SPLINE_CURVE_WITH_KNOTS('',3,(#174823,#174824,#174825,#174826,#174827,
#174828,#174829,#174830,#174831,#174832,#174833,#174834,#174835,#174836,
#174837,#174838),.UNSPECIFIED.,.F.,.F.,(4,3,3,3,3,4),(0.,0.000549388570659784,
0.00110809797237947,0.00147175517552831,0.00249356706683659,0.0029435103510566),
 .UNSPECIFIED.);
#5190=B_SPLINE_CURVE_WITH_KNOTS('',3,(#174863,#174864,#174865,#174866,#174867,
#174868,#174869,#174870,#174871,#174872,#174873,#174874,#174875),
 .UNSPECIFIED.,.F.,.F.,(4,3,3,3,4),(0.,0.000882415156986212,0.00147346850157273,
0.00255877694109341,0.00294693700314546),.UNSPECIFIED.);
#5191=B_SPLINE_CURVE_WITH_KNOTS('',3,(#174878,#174879,#174880,#174881,#174882,
#174883,#174884,#174885,#174886,#174887,#174888,#174889,#174890,#174891,
#174892,#174893,#174894,#174895,#174896,#174897,#174898,#174899,#174900,
#174901,#174902,#174903,#174904,#174905,#174906,#174907,#174908,#174909,
#174910,#174911,#174912,#174913,#174914,#174915,#174916,#174917,#174918,
#174919,#174920,#174921,#174922,#174923,#174924,#174925,#174926,#174927,
#174928,#174929,#174930,#174931,#174932,#174933,#174934,#174935,#174936,
#174937,#174938,#174939,#174940,#174941,#174942,#174943,#174944,#174945,
#174946,#174947,#174948,#174949,#174950,#174951,#174952,#174953,#174954,
#174955,#174956,#174957,#174958,#174959,#174960,#174961,#174962,#174963,
#174964,#174965,#174966,#174967,#174968,#174969,#174970,#174971,#174972,
#174973,#174974),.UNSPECIFIED.,.F.,.F.,(4,3,3,3,3,3,3,3,3,3,3,3,3,3,3,3,
3,3,3,3,3,3,3,3,3,3,3,3,3,3,3,3,4),(0.,0.0905528058390064,0.124999999999613,
0.18749999999942,0.218749999999329,0.23437499999929,0.24218749999927,0.24609374999926,
0.24999999999925,0.319163806059011,0.386358508937325,0.437499999998957,
0.468749999998914,0.484374999998893,0.492187499998883,0.496093749998882,
0.498046874998882,0.499999999998882,0.535697174154708,0.571806572205483,
0.608542429153761,0.645244164743076,0.682070032970534,0.718749999998596,
0.734374999998572,0.742187499998564,0.746093749998559,0.748046874998577,
0.749999999998595,0.824061086681612,0.89946952859405,0.976878755501281,
1.),.UNSPECIFIED.);
#5192=B_SPLINE_CURVE_WITH_KNOTS('',3,(#174988,#174989,#174990,#174991),
 .UNSPECIFIED.,.F.,.F.,(4,4),(0.,0.0319950621716304),.UNSPECIFIED.);
#5193=B_SPLINE_CURVE_WITH_KNOTS('',3,(#174994,#174995,#174996,#174997,#174998,
#174999,#175000,#175001,#175002,#175003,#175004,#175005,#175006,#175007,
#175008,#175009,#175010,#175011,#175012),.UNSPECIFIED.,.F.,.F.,(4,3,3,3,
3,3,4),(0.,0.201044054442995,0.388350105070278,0.5,0.666356063422891,0.833178031711445,
1.),.UNSPECIFIED.);
#5194=B_SPLINE_CURVE_WITH_KNOTS('',3,(#175032,#175033,#175034,#175035,#175036,
#175037,#175038,#175039,#175040,#175041,#175042,#175043,#175044,#175045,
#175046,#175047,#175048,#175049,#175050),.UNSPECIFIED.,.F.,.F.,(4,3,3,3,
3,3,4),(2.6071439595974E-7,0.171040742442568,0.354898569694402,0.447899270646099,
0.681237843610931,0.939818966220111,1.),.UNSPECIFIED.);
#5195=B_SPLINE_CURVE_WITH_KNOTS('',3,(#175051,#175052,#175053,#175054,#175055,
#175056,#175057,#175058,#175059,#175060,#175061,#175062,#175063,#175064,
#175065,#175066,#175067,#175068,#175069,#175070,#175071,#175072,#175073,
#175074,#175075,#175076,#175077,#175078,#175079,#175080,#175081,#175082,
#175083,#175084,#175085,#175086,#175087,#175088,#175089,#175090,#175091,
#175092,#175093,#175094,#175095,#175096,#175097,#175098,#175099,#175100,
#175101,#175102,#175103,#175104,#175105,#175106,#175107,#175108,#175109,
#175110,#175111,#175112,#175113,#175114,#175115,#175116,#175117,#175118,
#175119,#175120,#175121,#175122,#175123,#175124,#175125,#175126,#175127,
#175128,#175129,#175130,#175131,#175132),.UNSPECIFIED.,.F.,.F.,(4,3,3,3,
3,3,3,3,3,3,3,3,3,3,3,3,3,3,3,3,3,3,3,3,3,3,3,4),(0.,0.0718965045218442,
0.124999999999785,0.187499999999686,0.218749999999637,0.234374999999614,
0.242187499999603,0.246093749999598,0.248046874999596,0.249999999999595,
0.284793264427814,0.319965488512714,0.355518433439908,0.391200908602362,
0.426991239961754,0.437499999999188,0.468749999999136,0.484374999999107,
0.492187499999093,0.496093749999086,0.49804687499909,0.499999999999095,
0.59050135792091,0.682969730017932,0.778626353234705,0.87622436996633,0.976719140644226,
1.),.UNSPECIFIED.);
#5196=B_SPLINE_CURVE_WITH_KNOTS('',3,(#175155,#175156,#175157,#175158,#175159,
#175160,#175161,#175162,#175163,#175164,#175165,#175166,#175167),
 .UNSPECIFIED.,.F.,.F.,(4,3,3,3,4),(0.,0.000962747670504001,0.00119082241359643,
0.00216097007606112,0.00238164482719285),.UNSPECIFIED.);
#5197=B_SPLINE_CURVE_WITH_KNOTS('',3,(#175192,#175193,#175194,#175195,#175196,
#175197,#175198,#175199,#175200,#175201,#175202,#175203,#175204),
 .UNSPECIFIED.,.F.,.F.,(4,3,3,3,4),(0.,0.000775847435696327,0.00119114916434495,
0.00218083968933889,0.00238229832868991),.UNSPECIFIED.);
#5198=B_SPLINE_CURVE_WITH_KNOTS('',3,(#175220,#175221,#175222,#175223,#175224,
#175225,#175226,#175227,#175228,#175229,#175230,#175231,#175232,#175233,
#175234,#175235),.UNSPECIFIED.,.F.,.F.,(4,2,2,1,1,1,1,2,2,4),(0.,0.250000000000137,
0.375000000000206,0.43750000000024,0.468750000000256,0.484375000000264,
0.492187500000269,0.499023437500275,0.500000000000276,1.),.UNSPECIFIED.);
#5199=B_SPLINE_CURVE_WITH_KNOTS('',3,(#175253,#175254,#175255,#175256,#175257,
#175258,#175259,#175260,#175261,#175262,#175263,#175264,#175265,#175266,
#175267),.UNSPECIFIED.,.F.,.F.,(4,2,2,1,1,1,2,2,4),(0.,0.250000000000068,
0.375000000000102,0.437500000000119,0.468750000000127,0.484375000000131,
0.499023437500133,0.500000000000132,1.),.UNSPECIFIED.);
#5200=B_SPLINE_CURVE_WITH_KNOTS('',3,(#175285,#175286,#175287,#175288),
 .UNSPECIFIED.,.F.,.F.,(4,4),(0.0037358385977583,0.00423610566507283),
 .UNSPECIFIED.);
#5201=B_SPLINE_CURVE_WITH_KNOTS('',3,(#175291,#175292,#175293,#175294),
 .UNSPECIFIED.,.F.,.F.,(4,4),(0.020578988719059,0.0210794636037261),
 .UNSPECIFIED.);
#5202=B_SPLINE_CURVE_WITH_KNOTS('',3,(#175322,#175323,#175324,#175325,#175326,
#175327,#175328,#175329,#175330,#175331,#175332,#175333,#175334,#175335),
 .UNSPECIFIED.,.F.,.F.,(4,2,1,1,1,1,2,2,4),(0.,0.249999999999876,0.374999999999813,
0.437499999999783,0.468749999999766,0.484374999999757,0.499023437499747,
0.499999999999747,1.),.UNSPECIFIED.);
#5203=B_SPLINE_CURVE_WITH_KNOTS('',3,(#175355,#175356,#175357,#175358,#175359,
#175360,#175361,#175362,#175363,#175364,#175365,#175366,#175367),
 .UNSPECIFIED.,.F.,.F.,(4,3,3,3,4),(0.,0.00068051013705706,0.00109976462606963,
0.00204716723038797,0.00219952925213926),.UNSPECIFIED.);
#5204=B_SPLINE_CURVE_WITH_KNOTS('',3,(#175392,#175393,#175394,#175395,#175396,
#175397,#175398,#175399,#175400,#175401,#175402,#175403,#175404),
 .UNSPECIFIED.,.F.,.F.,(4,3,3,3,4),(0.,0.000627390790120107,0.00109987581267579,
0.00205656007236013,0.00219975162535158),.UNSPECIFIED.);
#5205=B_SPLINE_CURVE_WITH_KNOTS('',3,(#175407,#175408,#175409,#175410,#175411,
#175412,#175413,#175414,#175415,#175416,#175417,#175418,#175419,#175420,
#175421,#175422,#175423,#175424,#175425,#175426,#175427,#175428,#175429,
#175430,#175431,#175432,#175433,#175434,#175435,#175436,#175437,#175438,
#175439,#175440,#175441,#175442,#175443,#175444,#175445,#175446,#175447,
#175448,#175449,#175450,#175451,#175452,#175453,#175454,#175455,#175456,
#175457,#175458,#175459,#175460,#175461,#175462,#175463,#175464,#175465,
#175466,#175467,#175468,#175469,#175470,#175471,#175472,#175473,#175474,
#175475,#175476),.UNSPECIFIED.,.F.,.F.,(4,3,3,3,3,3,3,3,3,3,3,3,3,3,3,3,
3,3,3,3,3,3,3,4),(0.,0.130518220707149,0.25000000000017,0.375000000000256,
0.437500000000298,0.468750000000328,0.484375000000343,0.492187500000358,
0.496093750000372,0.500000000000385,0.500118514677062,0.555615849833377,
0.610869328165162,0.625000000000319,0.67976455378678,0.687500000000294,
0.718750000000282,0.734375000000276,0.746581455128004,0.75000000000027,
0.812499999925157,0.874854647535847,0.938420259612278,0.99999999969982),
 .UNSPECIFIED.);
#5206=B_SPLINE_CURVE_WITH_KNOTS('',3,(#175496,#175497,#175498,#175499,#175500,
#175501,#175502,#175503,#175504,#175505,#175506,#175507,#175508,#175509,
#175510,#175511,#175512,#175513,#175514,#175515,#175516,#175517,#175518,
#175519,#175520,#175521,#175522,#175523,#175524,#175525,#175526,#175527,
#175528,#175529,#175530,#175531,#175532,#175533,#175534,#175535,#175536,
#175537,#175538,#175539,#175540,#175541,#175542,#175543,#175544,#175545,
#175546,#175547,#175548,#175549,#175550,#175551,#175552,#175553),
 .UNSPECIFIED.,.F.,.F.,(4,3,3,3,3,3,3,3,3,3,3,3,3,3,3,3,3,3,3,4),(0.,0.249999999999903,
0.374999999999853,0.437499999999828,0.468749999999815,0.484374999999808,
0.492431640624811,0.49639701843243,0.498364217579178,0.498854096272949,
0.498972243282005,0.499071824544578,0.499561012215921,0.499805367190425,
0.499913587130118,0.499995666848597,0.500051933987096,0.732986788196755,
0.954689120223703,1.),.UNSPECIFIED.);
#5207=B_SPLINE_CURVE_WITH_KNOTS('',3,(#175573,#175574,#175575,#175576,#175577,
#175578,#175579,#175580,#175581,#175582,#175583,#175584,#175585),
 .UNSPECIFIED.,.F.,.F.,(4,2,1,1,1,2,2,4),(0.,0.250000000000011,0.375000000000015,
0.437500000000018,0.468750000000018,0.484375000000018,0.500000000000018,
1.),.UNSPECIFIED.);
#5208=B_SPLINE_CURVE_WITH_KNOTS('',3,(#175638,#175639,#175640,#175641,#175642,
#175643,#175644,#175645,#175646,#175647,#175648,#175649),.UNSPECIFIED.,
 .F.,.F.,(4,2,3,3,4),(0.,0.00100000000000208,0.00500000000023154,0.02100000001009,
0.0385835581099273),.UNSPECIFIED.);
#5209=B_SPLINE_CURVE_WITH_KNOTS('',3,(#175667,#175668,#175669,#175670,#175671,
#175672,#175673,#175674,#175675,#175676,#175677,#175678),.UNSPECIFIED.,
 .F.,.F.,(4,2,3,3,4),(0.,0.00100000000000032,0.00500000000004302,0.0210000000041071,
0.0383173498474262),.UNSPECIFIED.);
#5210=B_SPLINE_CURVE_WITH_KNOTS('',3,(#175693,#175694,#175695,#175696,#175697,
#175698,#175699,#175700,#175701,#175702,#175703,#175704,#175705,#175706,
#175707,#175708,#175709,#175710,#175711,#175712,#175713,#175714,#175715,
#175716,#175717,#175718,#175719,#175720,#175721,#175722,#175723,#175724,
#175725,#175726,#175727,#175728,#175729,#175730,#175731,#175732,#175733,
#175734,#175735,#175736,#175737,#175738),.UNSPECIFIED.,.F.,.F.,(4,3,3,3,
3,3,3,3,3,3,3,3,3,3,3,4),(0.,0.0830546620592719,0.125000000000492,0.229571060394868,
0.250000000000983,0.348011454012246,0.375000000001503,0.437500000001736,
0.468750000001785,0.484375000001759,0.492187500001746,0.500000000001733,
0.6250000000013,0.771819373948562,0.923348618181731,1.),.UNSPECIFIED.);
#5211=B_SPLINE_CURVE_WITH_KNOTS('',3,(#175740,#175741,#175742,#175743,#175744,
#175745),.UNSPECIFIED.,.F.,.F.,(4,2,4),(0.,0.5,1.),.UNSPECIFIED.);
#5212=B_SPLINE_CURVE_WITH_KNOTS('',3,(#175759,#175760,#175761,#175762,#175763,
#175764,#175765,#175766,#175767,#175768,#175769),.UNSPECIFIED.,.F.,.F.,
(4,2,1,2,2,4),(0.,0.250000000000047,0.375000000000077,0.43750000000009,
0.500000000000103,1.),.UNSPECIFIED.);
#5213=B_SPLINE_CURVE_WITH_KNOTS('',3,(#175791,#175792,#175793,#175794,#175795,
#175796,#175797,#175798,#175799,#175800,#175801,#175802),.UNSPECIFIED.,
 .F.,.F.,(4,2,2,2,2,4),(0.,0.25000000000007,0.375000000000103,0.437500000000076,
0.500000000000049,1.),.UNSPECIFIED.);
#5214=B_SPLINE_CURVE_WITH_KNOTS('',3,(#175886,#175887,#175888,#175889,#175890,
#175891,#175892,#175893,#175894,#175895,#175896,#175897,#175898,#175899,
#175900,#175901,#175902,#175903,#175904,#175905,#175906,#175907,#175908,
#175909,#175910,#175911,#175912,#175913,#175914,#175915,#175916,#175917,
#175918,#175919,#175920,#175921,#175922),.UNSPECIFIED.,.F.,.F.,(4,3,3,3,
3,3,3,3,3,3,3,3,4),(0.00064734234469968,0.000773679728910273,0.000794515777305426,
0.00111794174211916,0.00114512410810862,0.00123603607512266,0.00151649021309282,
0.00182472980554565,0.00188790100005033,0.00225930818373536,0.00241342353596863,
0.00270777040118012,0.00300211726639161),.UNSPECIFIED.);
#5215=B_SPLINE_CURVE_WITH_KNOTS('',3,(#175924,#175925,#175926,#175927,#175928,
#175929,#175930,#175931,#175932,#175933,#175934,#175935,#175936,#175937,
#175938,#175939,#175940,#175941,#175942,#175943,#175944,#175945,#175946,
#175947,#175948,#175949,#175950,#175951,#175952,#175953,#175954,#175955,
#175956,#175957,#175958,#175959,#175960,#175961,#175962,#175963,#175964,
#175965,#175966,#175967,#175968,#175969,#175970,#175971,#175972,#175973,
#175974,#175975,#175976,#175977,#175978,#175979,#175980,#175981,#175982,
#175983,#175984,#175985,#175986,#175987,#175988,#175989,#175990,#175991,
#175992,#175993),.UNSPECIFIED.,.F.,.F.,(4,3,3,3,3,3,3,3,3,3,3,3,3,3,3,3,
3,3,3,3,3,3,3,4),(0.,0.0909637694368515,0.178799587602911,0.24999999999992,
0.269286037251739,0.320475373835143,0.406735621633324,0.46874999999988,
0.484374999999908,0.494411073072455,0.499999999999934,0.544308918389705,
0.616362009200579,0.624999999999929,0.687499999999932,0.718749999999958,
0.733555217110215,0.747697754998785,0.749999999999984,0.780356397068987,
0.849170048020548,0.916030064764027,0.980468771416945,1.),.UNSPECIFIED.);
#5216=B_SPLINE_CURVE_WITH_KNOTS('',3,(#175994,#175995,#175996,#175997,#175998,
#175999,#176000,#176001,#176002,#176003,#176004,#176005,#176006,#176007,
#176008,#176009,#176010,#176011,#176012,#176013,#176014,#176015,#176016,
#176017,#176018,#176019,#176020,#176021,#176022,#176023),.UNSPECIFIED.,
 .F.,.F.,(4,2,2,2,1,1,1,2,2,2,2,1,1,1,2,2,2,4),(0.,0.125000000000031,0.187500000000059,
0.218750000000073,0.234375000000079,0.242187500000088,0.246093750000099,
0.248046875000105,0.25000000000011,0.374999999999913,0.437499999999804,
0.468749999999764,0.484374999999732,0.492187499999724,0.496093749999717,
0.499999999999709,0.749999999999854,1.),.UNSPECIFIED.);
#5217=B_SPLINE_CURVE_WITH_KNOTS('',3,(#176038,#176039,#176040,#176041,#176042,
#176043,#176044,#176045,#176046,#176047,#176048,#176049,#176050,#176051,
#176052,#176053,#176054,#176055,#176056,#176057,#176058,#176059,#176060,
#176061,#176062,#176063,#176064,#176065,#176066,#176067,#176068,#176069),
 .UNSPECIFIED.,.F.,.F.,(4,2,2,2,1,1,1,2,2,2,2,2,1,1,1,2,2,2,4),(0.,0.249999999999737,
0.374999999999601,0.437499999999541,0.46874999999952,0.4843749999995,0.492187499999488,
0.496093749999487,0.499999999999486,0.624999999999202,0.68749999999906,
0.718749999999,0.734374999998961,0.742187499998943,0.746093749998934,0.748046874998939,
0.749999999998944,0.874999999999472,1.),.UNSPECIFIED.);
#5218=B_SPLINE_CURVE_WITH_KNOTS('',3,(#176113,#176114,#176115,#176116,#176117,
#176118,#176119,#176120,#176121,#176122,#176123,#176124,#176125,#176126,
#176127,#176128,#176129,#176130,#176131,#176132,#176133,#176134,#176135,
#176136,#176137,#176138,#176139,#176140,#176141,#176142,#176143,#176144,
#176145,#176146,#176147,#176148,#176149,#176150,#176151,#176152,#176153,
#176154,#176155,#176156,#176157,#176158,#176159,#176160,#176161),
 .UNSPECIFIED.,.F.,.F.,(4,3,3,3,3,3,3,3,3,3,3,3,3,3,3,3,4),(0.,0.0684875562747417,
0.136659016526091,0.204808625883849,0.250000000000048,0.318760027576873,
0.375000000000071,0.414532745911366,0.454363518454273,0.495640942979285,
0.500000000000095,0.584838655976972,0.66918100853855,0.753595793198019,
0.83822364534784,0.923951954929328,1.),.UNSPECIFIED.);
#5219=B_SPLINE_CURVE_WITH_KNOTS('',3,(#176162,#176163,#176164,#176165,#176166,
#176167,#176168,#176169,#176170,#176171,#176172,#176173,#176174,#176175,
#176176,#176177,#176178,#176179,#176180,#176181,#176182,#176183,#176184,
#176185,#176186,#176187,#176188,#176189,#176190,#176191,#176192,#176193,
#176194,#176195,#176196,#176197,#176198,#176199,#176200,#176201,#176202,
#176203,#176204,#176205,#176206,#176207,#176208,#176209,#176210),
 .UNSPECIFIED.,.F.,.F.,(4,3,3,3,3,3,3,3,3,3,3,3,3,3,3,3,4),(0.,0.000568992160183443,
0.000684369961878612,0.000753736971436056,0.000939442240060596,0.00102655494281796,
0.00113065957381952,0.00136873992375731,0.00150755451437507,0.00188444398402289,
0.00205310988563609,0.00222420237610578,0.00226080156348499,0.00235252174395805,
0.00254500079573646,0.00264124032162566,0.00273747984751486),
 .UNSPECIFIED.);
#5220=B_SPLINE_CURVE_WITH_KNOTS('',3,(#176251,#176252,#176253,#176254,#176255,
#176256,#176257,#176258,#176259,#176260,#176261,#176262,#176263,#176264,
#176265,#176266),.UNSPECIFIED.,.F.,.F.,(4,2,2,1,1,2,2,2,4),(0.,0.249999999999916,
0.374999999999924,0.437499999999896,0.468749999999911,0.484374999999942,
0.499999999999973,0.749999999999986,1.),.UNSPECIFIED.);
#5221=B_SPLINE_CURVE_WITH_KNOTS('',3,(#176274,#176275,#176276,#176277,#176278,
#176279,#176280,#176281,#176282,#176283,#176284,#176285,#176286,#176287,
#176288,#176289),.UNSPECIFIED.,.F.,.F.,(4,2,2,2,1,1,2,2,4),(0.,0.249999999999886,
0.374999999999848,0.437499999999797,0.46874999999974,0.484374999999751,
0.492187499999733,0.499999999999715,1.),.UNSPECIFIED.);
#5222=B_SPLINE_CURVE_WITH_KNOTS('',3,(#176330,#176331,#176332,#176333,#176334,
#176335,#176336,#176337,#176338,#176339,#176340,#176341,#176342,#176343,
#176344,#176345,#176346,#176347,#176348,#176349,#176350,#176351,#176352,
#176353,#176354,#176355,#176356,#176357,#176358,#176359,#176360,#176361,
#176362,#176363,#176364,#176365,#176366,#176367,#176368,#176369,#176370,
#176371,#176372,#176373,#176374,#176375,#176376,#176377,#176378,#176379,
#176380,#176381,#176382,#176383,#176384,#176385,#176386,#176387,#176388,
#176389,#176390,#176391,#176392,#176393,#176394,#176395,#176396,#176397,
#176398,#176399),.UNSPECIFIED.,.F.,.F.,(4,3,3,3,3,3,3,3,3,3,3,3,3,3,3,3,
3,3,3,3,3,3,3,4),(0.,0.076883980804006,0.155236173506771,0.236099575550264,
0.245845450188085,0.250000000001421,0.327307321279621,0.375000000002082,
0.437500000002376,0.468750000002516,0.472513732477007,0.484375000002586,
0.492187500002609,0.497985201456684,0.500000000002632,0.612018993597418,
0.710669180284392,0.750000000001316,0.769020159477365,0.781250000001152,
0.858443094492983,0.890625000000576,0.970594010184165,1.),.UNSPECIFIED.);
#5223=B_SPLINE_CURVE_WITH_KNOTS('',3,(#176439,#176440,#176441,#176442,#176443,
#176444,#176445,#176446),.UNSPECIFIED.,.F.,.F.,(4,2,2,4),(0.,0.0307386998643325,
0.0629186902704779,0.0847651026474671),.UNSPECIFIED.);
#5224=B_SPLINE_CURVE_WITH_KNOTS('',3,(#176447,#176448,#176449,#176450,#176451,
#176452,#176453,#176454),.UNSPECIFIED.,.F.,.F.,(4,2,2,4),(0.0847654169755104,
0.106603528597414,0.138777607634753,0.16953083368799),.UNSPECIFIED.);
#5225=B_SPLINE_CURVE_WITH_KNOTS('',3,(#176455,#176456,#176457,#176458,#176459,
#176460,#176461,#176462,#176463,#176464,#176465,#176466,#176467,#176468,
#176469,#176470,#176471,#176472,#176473),.UNSPECIFIED.,.F.,.F.,(4,3,3,3,
3,3,4),(0.,0.000358645716711148,0.000416788078411022,0.000833987724853048,
0.000834068655632161,0.00125109176933023,0.00166813731126432),
 .UNSPECIFIED.);
#5226=B_SPLINE_CURVE_WITH_KNOTS('',3,(#176506,#176507,#176508,#176509,#176510,
#176511,#176512,#176513,#176514,#176515,#176516,#176517,#176518,#176519,
#176520,#176521,#176522,#176523,#176524,#176525,#176526,#176527,#176528,
#176529,#176530,#176531),.UNSPECIFIED.,.F.,.F.,(4,2,2,2,2,2,2,2,2,2,2,2,
4),(0.,0.0350983387286775,0.0741581944032339,0.101946776655108,0.109514391091077,
0.11764023444793,0.136341904849521,0.141182675692268,0.160390411168246,
0.193626235432022,0.217667420373208,0.251529378143752,0.2824139549931),
 .UNSPECIFIED.);
#5227=B_SPLINE_CURVE_WITH_KNOTS('',3,(#176532,#176533,#176534,#176535,#176536,
#176537,#176538,#176539,#176540,#176541,#176542,#176543,#176544,#176545,
#176546,#176547,#176548,#176549,#176550,#176551,#176552,#176553,#176554,
#176555,#176556,#176557,#176558,#176559,#176560,#176561,#176562),
 .UNSPECIFIED.,.F.,.F.,(4,3,3,3,3,3,3,3,3,3,4),(0.,0.000366648609668148,
0.000673956529173827,0.00118123470619227,0.00134837711191729,0.00134840211582016,
0.00202256566787594,0.00202269623773768,0.0023684953008591,0.00265916017167732,
0.00269675422383458),.UNSPECIFIED.);
#5228=B_SPLINE_CURVE_WITH_KNOTS('',3,(#176597,#176598,#176599,#176600,#176601,
#176602,#176603,#176604,#176605,#176606,#176607,#176608,#176609,#176610,
#176611,#176612,#176613,#176614),.UNSPECIFIED.,.F.,.F.,(4,2,2,2,2,2,2,2,
4),(0.,0.0302664700381998,0.0628248024586328,0.0854745235510308,0.116272737380146,
0.147052923761063,0.169708349889542,0.202281537926532,0.232545593041181),
 .UNSPECIFIED.);
#5229=B_SPLINE_CURVE_WITH_KNOTS('',3,(#176615,#176616,#176617,#176618,#176619,
#176620,#176621,#176622,#176623,#176624,#176625,#176626,#176627,#176628,
#176629,#176630,#176631,#176632,#176633,#176634,#176635,#176636,#176637,
#176638,#176639,#176640,#176641,#176642,#176643,#176644,#176645),
 .UNSPECIFIED.,.F.,.F.,(4,3,3,3,3,3,3,3,3,3,4),(0.,0.000563737664817588,
0.000564164457966204,0.00104582442932934,0.00112760220035029,0.00112832891593241,
0.00161216721635697,0.00169210723432566,0.00169249337389861,0.00210946737344097,
0.00225665783186482),.UNSPECIFIED.);
#5230=B_SPLINE_CURVE_WITH_KNOTS('',3,(#176703,#176704,#176705,#176706,#176707,
#176708,#176709,#176710,#176711,#176712,#176713,#176714,#176715),
 .UNSPECIFIED.,.F.,.F.,(4,3,3,3,4),(4.71238898038469,5.10508806208342,5.49778714378214,
5.89048622548087,6.28318530717959),.UNSPECIFIED.);
#5231=B_SPLINE_CURVE_WITH_KNOTS('',3,(#176752,#176753,#176754,#176755,#176756,
#176757,#176758,#176759,#176760,#176761,#176762,#176763,#176764,#176765,
#176766,#176767,#176768,#176769,#176770,#176771,#176772,#176773,#176774,
#176775,#176776,#176777,#176778,#176779,#176780,#176781,#176782,#176783,
#176784,#176785,#176786,#176787,#176788,#176789,#176790,#176791,#176792,
#176793,#176794,#176795,#176796,#176797,#176798,#176799,#176800,#176801,
#176802,#176803,#176804,#176805,#176806,#176807,#176808,#176809,#176810,
#176811,#176812,#176813,#176814,#176815,#176816,#176817,#176818,#176819,
#176820,#176821,#176822,#176823,#176824,#176825,#176826,#176827,#176828,
#176829,#176830,#176831,#176832,#176833,#176834,#176835,#176836,#176837,
#176838,#176839,#176840,#176841,#176842,#176843,#176844,#176845),
 .UNSPECIFIED.,.F.,.F.,(4,3,3,3,3,3,3,3,3,3,3,3,3,3,3,3,3,3,3,3,3,3,3,3,
3,3,3,3,3,3,3,4),(0.,0.0848538873601167,0.124999999999949,0.187499999999932,
0.21134842114964,0.234943711617932,0.249999999999915,0.260068072866973,
0.318500635089809,0.374999999999881,0.433593749999855,0.485685382805016,
0.492187499999828,0.497237166982873,0.499999999999823,0.548708184837966,
0.596046174884053,0.624999999999797,0.670698621118158,0.715864692245719,
0.74124433963234,0.746093749999775,0.748046874999775,0.749999999999775,
0.787508057868778,0.824345378943297,0.860001761682919,0.874999999999888,
0.908764508078463,0.941702858531229,0.973398294005402,1.),.UNSPECIFIED.);
#5232=B_SPLINE_CURVE_WITH_KNOTS('',3,(#176928,#176929,#176930,#176931,#176932,
#176933,#176934,#176935,#176936,#176937,#176938,#176939,#176940,#176941,
#176942,#176943,#176944,#176945),.UNSPECIFIED.,.F.,.F.,(4,2,2,2,2,2,2,2,
4),(0.,0.0302664700381639,0.0628248024586889,0.0854745235512447,0.116272737380081,
0.147052923760174,0.169708349887848,0.202281537923779,0.232545593037369),
 .UNSPECIFIED.);
#5233=B_SPLINE_CURVE_WITH_KNOTS('',3,(#176946,#176947,#176948,#176949,#176950,
#176951,#176952,#176953,#176954,#176955,#176956,#176957,#176958,#176959,
#176960,#176961,#176962,#176963,#176964,#176965,#176966,#176967,#176968,
#176969,#176970,#176971,#176972,#176973,#176974,#176975,#176976),
 .UNSPECIFIED.,.F.,.F.,(4,3,3,3,3,3,3,3,3,3,4),(0.,0.000563737664817634,
0.000564164457966258,0.00104582442998829,0.00112760220035038,0.00112832891593252,
0.00161216721525258,0.00169210723432587,0.00169249337389877,0.00210946737362081,
0.00225665783186503),.UNSPECIFIED.);
#5234=B_SPLINE_CURVE_WITH_KNOTS('',3,(#177109,#177110,#177111,#177112,#177113,
#177114,#177115,#177116,#177117,#177118,#177119,#177120,#177121,#177122,
#177123,#177124,#177125,#177126,#177127,#177128,#177129,#177130,#177131,
#177132,#177133,#177134,#177135,#177136,#177137,#177138,#177139,#177140,
#177141,#177142,#177143,#177144,#177145,#177146,#177147,#177148,#177149,
#177150,#177151,#177152,#177153,#177154,#177155,#177156,#177157),
 .UNSPECIFIED.,.F.,.F.,(4,3,3,3,3,3,3,3,3,3,3,3,3,3,3,3,4),(4.25657365665928E-6,
0.0813278485490425,0.124999999999948,0.187499999999922,0.218749999999908,
0.2343749999999,0.242187499999898,0.249999999999898,0.384939308991726,0.492187499999907,
0.499607739469523,0.499999999999908,0.514870101102984,0.669487794470102,
0.749999999999954,0.879941940443589,1.),.UNSPECIFIED.);
#5235=B_SPLINE_CURVE_WITH_KNOTS('',3,(#177158,#177159,#177160,#177161,#177162,
#177163,#177164,#177165,#177166,#177167,#177168,#177169,#177170,#177171,
#177172,#177173,#177174,#177175,#177176,#177177,#177178,#177179),
 .UNSPECIFIED.,.F.,.F.,(4,3,3,3,3,3,3,4),(0.,0.197532150015397,0.462790841234246,
0.484806537167571,0.629594317573962,0.780867938240718,0.942621022464376,
1.),.UNSPECIFIED.);
#5236=B_SPLINE_CURVE_WITH_KNOTS('',3,(#177211,#177212,#177213,#177214,#177215,
#177216,#177217,#177218,#177219,#177220,#177221,#177222,#177223,#177224,
#177225,#177226,#177227,#177228,#177229,#177230,#177231,#177232,#177233,
#177234,#177235,#177236,#177237,#177238,#177239,#177240,#177241,#177242,
#177243,#177244,#177245,#177246,#177247,#177248,#177249,#177250,#177251,
#177252,#177253,#177254,#177255,#177256,#177257,#177258,#177259,#177260,
#177261,#177262,#177263,#177264,#177265,#177266,#177267,#177268,#177269,
#177270,#177271,#177272,#177273,#177274,#177275,#177276,#177277,#177278,
#177279,#177280,#177281,#177282,#177283,#177284,#177285,#177286,#177287,
#177288,#177289,#177290,#177291,#177292,#177293,#177294,#177295,#177296,
#177297,#177298,#177299,#177300,#177301,#177302,#177303,#177304,#177305,
#177306,#177307,#177308,#177309,#177310),.UNSPECIFIED.,.F.,.F.,(4,3,3,3,
3,3,3,3,3,3,3,3,3,3,3,3,3,3,3,3,3,3,3,3,3,3,3,3,3,3,3,3,3,4),(0.,0.0343791361047495,
0.0625000000001909,0.0937500000002863,0.109375000000334,0.125000000000382,
0.163294442145796,0.18750000000058,0.218750000000676,0.234375000000738,
0.241645237443817,0.242187500000769,0.246093750000772,0.248046875000773,
0.250000000000775,0.306559060440209,0.362191713414393,0.375000000000652,
0.431342405906489,0.437500000000599,0.468750000000571,0.482664534375719,
0.494988196652662,0.500000000000543,0.563130724290198,0.625155813819059,
0.6862883583218,0.747420902824542,0.750000000000271,0.801992080489307,0.854451944080758,
0.907057823204673,0.959601903223852,0.99999893160244),.UNSPECIFIED.);
#5237=B_SPLINE_CURVE_WITH_KNOTS('',3,(#177313,#177314,#177315,#177316,#177317,
#177318,#177319,#177320,#177321,#177322,#177323,#177324,#177325,#177326,
#177327,#177328,#177329,#177330,#177331,#177332,#177333,#177334,#177335,
#177336,#177337,#177338,#177339,#177340,#177341,#177342,#177343,#177344,
#177345,#177346),.UNSPECIFIED.,.F.,.F.,(4,3,3,3,3,3,3,3,3,3,3,4),(0.,0.000121613272085656,
0.000230848939029442,0.000231076761054257,0.000462001643661032,0.000462153522108514,
0.000693154344712357,0.000693230283162771,0.000767002378129274,0.000841536498305322,
0.000913992773638785,0.000924307044217028),.UNSPECIFIED.);
#5238=B_SPLINE_CURVE_WITH_KNOTS('',3,(#177422,#177423,#177424,#177425,#177426,
#177427,#177428,#177429,#177430,#177431,#177432,#177433,#177434,#177435,
#177436,#177437,#177438,#177439,#177440,#177441,#177442,#177443,#177444,
#177445,#177446,#177447,#177448,#177449,#177450,#177451,#177452,#177453,
#177454,#177455),.UNSPECIFIED.,.F.,.F.,(4,3,3,3,3,3,3,3,3,3,3,4),(0.,7.30072795026847E-5,
0.000147770013513584,0.000221881916258506,0.000252597382995535,0.00050519476599107,
0.000631493458785083,0.000757792148986605,0.000834383528241785,0.000911454457736763,
0.00098555498853702,0.00101038953198214),.UNSPECIFIED.);
#5239=B_SPLINE_CURVE_WITH_KNOTS('',3,(#177459,#177460,#177461,#177462,#177463,
#177464,#177465,#177466,#177467,#177468,#177469,#177470,#177471,#177472,
#177473,#177474,#177475,#177476),.UNSPECIFIED.,.F.,.F.,(4,2,2,2,1,1,2,2,
2,4),(0.,0.250000000000059,0.375000000000088,0.4375000000001,0.468750000000106,
0.484375000000098,0.492187500000103,0.500000000000108,0.750000000000054,
1.),.UNSPECIFIED.);
#5240=B_SPLINE_CURVE_WITH_KNOTS('',3,(#177517,#177518,#177519,#177520,#177521,
#177522,#177523,#177524,#177525,#177526,#177527,#177528,#177529,#177530,
#177531,#177532,#177533,#177534,#177535,#177536,#177537,#177538,#177539,
#177540,#177541,#177542,#177543,#177544,#177545,#177546,#177547,#177548,
#177549,#177550,#177551,#177552,#177553,#177554,#177555,#177556,#177557,
#177558,#177559,#177560,#177561,#177562,#177563,#177564,#177565,#177566,
#177567,#177568,#177569,#177570,#177571,#177572,#177573,#177574,#177575,
#177576,#177577),.UNSPECIFIED.,.F.,.F.,(4,3,3,3,3,3,3,3,3,3,3,3,3,3,3,3,
3,3,3,3,4),(0.,0.0495055255292412,0.100209542104456,0.152193164617286,0.207894873463021,
0.263458555812716,0.321344960646642,0.375000000000226,0.43750000000027,
0.46875000000028,0.484375000000273,0.492187500000252,0.497889045411213,
0.500000000000231,0.576744445667211,0.654433500550048,0.733098323656875,
0.813288233486846,0.894374265212616,0.976809019714828,0.99999999957007),
 .UNSPECIFIED.);
#5241=B_SPLINE_CURVE_WITH_KNOTS('',3,(#177580,#177581,#177582,#177583,#177584,
#177585),.UNSPECIFIED.,.F.,.F.,(4,2,4),(0.,0.000501785580775435,0.00100357116155087),
 .UNSPECIFIED.);
#5242=B_SPLINE_CURVE_WITH_KNOTS('',3,(#177600,#177601,#177602,#177603),
 .UNSPECIFIED.,.F.,.F.,(4,4),(0.0171576436379621,0.0176580988602617),
 .UNSPECIFIED.);
#5243=B_SPLINE_CURVE_WITH_KNOTS('',3,(#177632,#177633,#177634,#177635,#177636,
#177637,#177638,#177639,#177640,#177641,#177642,#177643,#177644,#177645,
#177646,#177647,#177648,#177649,#177650,#177651,#177652,#177653,#177654,
#177655,#177656,#177657,#177658,#177659,#177660,#177661,#177662,#177663,
#177664,#177665,#177666,#177667,#177668,#177669,#177670,#177671,#177672,
#177673,#177674,#177675,#177676,#177677),.UNSPECIFIED.,.F.,.F.,(4,3,3,3,
3,3,3,3,3,3,3,3,3,3,3,4),(0.,0.0785956779669218,0.160354336421304,0.24882607911666,
0.305407052180528,0.42271380724194,0.49218749999989,0.498963544975227,0.499999999999892,
0.503499840825533,0.594170920862958,0.685885083834807,0.779934809548503,
0.875859615671826,0.975510441703396,1.),.UNSPECIFIED.);
#5244=B_SPLINE_CURVE_WITH_KNOTS('',3,(#177692,#177693,#177694,#177695,#177696,
#177697,#177698,#177699,#177700,#177701,#177702,#177703,#177704,#177705,
#177706,#177707,#177708,#177709,#177710,#177711,#177712,#177713,#177714,
#177715,#177716,#177717,#177718,#177719,#177720,#177721,#177722,#177723,
#177724,#177725),.UNSPECIFIED.,.F.,.F.,(4,3,3,3,3,3,3,3,3,3,3,4),(0.,0.0625000000000025,
0.203210009066382,0.25000000000001,0.339585721546707,0.427987553177131,
0.50000000000002,0.625000000000015,0.718750000000011,0.859375000000006,
0.929687500000003,1.),.UNSPECIFIED.);
#5245=B_SPLINE_CURVE_WITH_KNOTS('',3,(#177754,#177755,#177756,#177757,#177758,
#177759,#177760,#177761,#177762,#177763,#177764,#177765,#177766,#177767,
#177768,#177769,#177770,#177771,#177772,#177773,#177774,#177775,#177776,
#177777,#177778,#177779,#177780,#177781,#177782,#177783,#177784,#177785,
#177786,#177787),.UNSPECIFIED.,.F.,.F.,(4,3,3,3,3,3,3,3,3,3,3,4),(0.,0.124999999999929,
0.245408262930441,0.357304671146824,0.468749999999767,0.487553083205154,
0.499999999999741,0.504270157601894,0.642179092659868,0.774946277671523,
0.90129593860598,1.),.UNSPECIFIED.);
#5246=B_SPLINE_CURVE_WITH_KNOTS('',3,(#177820,#177821,#177822,#177823,#177824,
#177825,#177826,#177827,#177828,#177829,#177830,#177831,#177832,#177833,
#177834,#177835),.UNSPECIFIED.,.F.,.F.,(4,2,2,2,2,2,2,4),(0.,0.249999999999971,
0.374999999999958,0.437499999999955,0.499999999999952,0.624999999999961,
0.74999999999997,1.),.UNSPECIFIED.);
#5247=B_SPLINE_CURVE_WITH_KNOTS('',3,(#177985,#177986,#177987,#177988,#177989,
#177990,#177991,#177992,#177993,#177994,#177995,#177996,#177997,#177998,
#177999,#178000,#178001,#178002,#178003,#178004,#178005,#178006,#178007,
#178008,#178009,#178010,#178011,#178012,#178013,#178014,#178015,#178016,
#178017,#178018,#178019,#178020,#178021,#178022,#178023,#178024,#178025,
#178026,#178027,#178028,#178029,#178030,#178031,#178032,#178033,#178034,
#178035,#178036,#178037,#178038,#178039,#178040,#178041,#178042,#178043,
#178044,#178045,#178046,#178047,#178048,#178049,#178050,#178051,#178052,
#178053,#178054,#178055,#178056,#178057),.UNSPECIFIED.,.F.,.F.,(4,3,3,3,
3,3,3,3,3,3,3,3,3,3,3,3,3,3,3,3,3,3,3,3,4),(0.,0.082779980612263,0.164476403995074,
0.244653469516663,0.323962788611773,0.402053471713434,0.437499999999713,
0.468749999999689,0.482808502334718,0.497325258698629,0.499999999999665,
0.563666004332427,0.625583002165994,0.687499999999561,0.718749999999545,
0.734374999999534,0.742187499999531,0.746930749075681,0.749999999999528,
0.798769943401674,0.84646594186107,0.892304179059618,0.936986222417194,
0.979989000405518,1.),.UNSPECIFIED.);
#5248=B_SPLINE_CURVE_WITH_KNOTS('',3,(#178063,#178064,#178065,#178066,#178067,
#178068,#178069,#178070,#178071,#178072,#178073,#178074,#178075,#178076,
#178077,#178078,#178079,#178080,#178081,#178082,#178083,#178084,#178085,
#178086,#178087,#178088,#178089,#178090,#178091,#178092,#178093,#178094,
#178095,#178096,#178097,#178098,#178099,#178100,#178101,#178102,#178103,
#178104,#178105,#178106,#178107,#178108,#178109,#178110,#178111,#178112,
#178113,#178114,#178115,#178116,#178117),.UNSPECIFIED.,.F.,.F.,(4,3,3,3,
3,3,3,3,3,3,3,3,3,3,3,3,3,3,4),(0.,0.104765563683224,0.210444272545764,
0.25000000000008,0.354080737998022,0.375000000000133,0.437500000000166,
0.468750000000186,0.484375000000179,0.493467332381432,0.500000000000171,
0.577628367609106,0.651921806122704,0.721921630140622,0.750000000000086,
0.814799791967406,0.877825876853573,0.938912938426786,1.),.UNSPECIFIED.);
#5249=B_SPLINE_CURVE_WITH_KNOTS('',3,(#178125,#178126,#178127,#178128,#178129,
#178130,#178131,#178132,#178133,#178134,#178135,#178136,#178137,#178138,
#178139,#178140,#178141,#178142,#178143,#178144,#178145,#178146,#178147,
#178148,#178149,#178150,#178151,#178152,#178153,#178154,#178155,#178156,
#178157,#178158,#178159,#178160,#178161,#178162,#178163,#178164,#178165,
#178166,#178167,#178168,#178169,#178170),.UNSPECIFIED.,.F.,.F.,(4,3,3,3,
3,3,3,3,3,3,3,3,3,3,3,4),(0.,0.0625000000000026,0.124542361690346,0.189407379068573,
0.25000000000001,0.320392682405879,0.396093817100428,0.473112575495438,
0.484375000000034,0.493957180840421,0.500000000000055,0.60537483706371,
0.710879749792983,0.81656475508876,0.922725793047527,1.),.UNSPECIFIED.);
#5250=B_SPLINE_CURVE_WITH_KNOTS('',3,(#178175,#178176,#178177,#178178,#178179,
#178180,#178181,#178182,#178183,#178184,#178185,#178186,#178187),
 .UNSPECIFIED.,.F.,.F.,(4,3,3,3,4),(3.1415926535898,3.53429173528852,3.92699081698725,
4.31968989868597,4.7123889803847),.UNSPECIFIED.);
#5251=B_SPLINE_CURVE_WITH_KNOTS('',3,(#178220,#178221,#178222,#178223,#178224,
#178225,#178226,#178227,#178228,#178229,#178230,#178231,#178232,#178233,
#178234,#178235,#178236,#178237,#178238,#178239,#178240,#178241,#178242,
#178243,#178244,#178245,#178246,#178247,#178248,#178249,#178250,#178251,
#178252,#178253,#178254,#178255,#178256,#178257,#178258,#178259,#178260,
#178261,#178262,#178263,#178264,#178265,#178266,#178267,#178268,#178269,
#178270,#178271,#178272,#178273,#178274,#178275,#178276,#178277,#178278,
#178279,#178280,#178281,#178282,#178283,#178284,#178285,#178286,#178287,
#178288,#178289),.UNSPECIFIED.,.F.,.F.,(4,3,3,3,3,3,3,3,3,3,3,3,3,3,3,3,
3,3,3,3,3,3,3,4),(0.,0.0418556349283318,0.085887226797697,0.125000000000002,
0.172074981291823,0.221103566867858,0.242187500000009,0.247532486206105,
0.250000000000003,0.258757700059768,0.31821086461791,0.374999999999964,
0.438770544658119,0.468749999999953,0.48328939377611,0.497396607321518,
0.499999999999955,0.586546601545785,0.674398018105785,0.743166321732782,
0.749999999999978,0.839281118802835,0.929643700148846,1.),.UNSPECIFIED.);
#5252=B_SPLINE_CURVE_WITH_KNOTS('',3,(#178335,#178336,#178337,#178338,#178339,
#178340,#178341,#178342,#178343,#178344,#178345,#178346,#178347,#178348,
#178349,#178350,#178351,#178352,#178353,#178354,#178355,#178356,#178357,
#178358,#178359,#178360,#178361,#178362,#178363,#178364,#178365,#178366,
#178367,#178368,#178369,#178370,#178371,#178372,#178373,#178374,#178375,
#178376,#178377,#178378,#178379,#178380,#178381,#178382,#178383,#178384,
#178385,#178386,#178387,#178388,#178389,#178390,#178391,#178392,#178393,
#178394,#178395,#178396,#178397,#178398,#178399,#178400,#178401,#178402,
#178403,#178404,#178405,#178406,#178407),.UNSPECIFIED.,.F.,.F.,(4,3,3,3,
3,3,3,3,3,3,3,3,3,3,3,3,3,3,3,3,3,3,3,3,4),(0.,0.082893131556343,0.164185603605923,
0.244579415150671,0.32366183441379,0.374999999999872,0.437499999999848,
0.468749999999836,0.482808502022526,0.497325258097958,0.499999999999824,
0.563666002926397,0.625583001463082,0.687499999999767,0.71874999999976,
0.734374999999749,0.742187499999748,0.746930748996793,0.749999999999748,
0.798769942118381,0.84646593941013,0.892304175537976,0.936986217868166,
0.979988994819292,1.),.UNSPECIFIED.);
#5253=B_SPLINE_CURVE_WITH_KNOTS('',3,(#178414,#178415,#178416,#178417,#178418,
#178419,#178420,#178421,#178422,#178423,#178424,#178425,#178426,#178427,
#178428,#178429,#178430,#178431,#178432,#178433,#178434,#178435,#178436,
#178437,#178438,#178439,#178440,#178441,#178442,#178443,#178444,#178445,
#178446,#178447,#178448,#178449,#178450,#178451,#178452,#178453,#178454,
#178455,#178456,#178457,#178458,#178459,#178460,#178461,#178462,#178463,
#178464,#178465,#178466,#178467,#178468),.UNSPECIFIED.,.F.,.F.,(4,3,3,3,
3,3,3,3,3,3,3,3,3,3,3,3,3,3,4),(0.,0.104765562818283,0.210444270602352,
0.249999999999833,0.354080736731079,0.374999999999737,0.437499999999706,
0.468749999999691,0.484374999999682,0.493467332336236,0.499999999999673,
0.577628367388466,0.651921805693988,0.721921629485197,0.749999999999836,
0.814799791699761,0.877825876310641,0.938912938155321,1.),.UNSPECIFIED.);
#5254=B_SPLINE_CURVE_WITH_KNOTS('',3,(#178476,#178477,#178478,#178479,#178480,
#178481,#178482,#178483,#178484,#178485,#178486,#178487,#178488,#178489,
#178490,#178491,#178492,#178493,#178494,#178495,#178496,#178497,#178498,
#178499,#178500,#178501,#178502,#178503,#178504,#178505,#178506,#178507,
#178508,#178509,#178510,#178511,#178512,#178513,#178514,#178515,#178516,
#178517,#178518,#178519,#178520,#178521),.UNSPECIFIED.,.F.,.F.,(4,3,3,3,
3,3,3,3,3,3,3,3,3,3,3,4),(0.,0.0625000000000706,0.124542361511373,0.189407378720157,
0.250000000000282,0.320392682263235,0.396093816754809,0.473112577400942,
0.48437500000048,0.493957180817966,0.500000000000473,0.605374836123673,
0.710879748053809,0.816564752616696,0.922725789936784,1.),.UNSPECIFIED.);
#5255=B_SPLINE_CURVE_WITH_KNOTS('',3,(#178568,#178569,#178570,#178571,#178572,
#178573,#178574,#178575,#178576,#178577,#178578,#178579,#178580,#178581,
#178582,#178583,#178584,#178585,#178586,#178587,#178588,#178589,#178590,
#178591,#178592,#178593,#178594,#178595,#178596,#178597,#178598,#178599,
#178600,#178601,#178602,#178603,#178604,#178605,#178606,#178607,#178608,
#178609,#178610,#178611,#178612,#178613,#178614,#178615,#178616,#178617,
#178618,#178619,#178620,#178621,#178622,#178623,#178624,#178625,#178626,
#178627,#178628,#178629,#178630,#178631,#178632,#178633,#178634,#178635,
#178636,#178637),.UNSPECIFIED.,.F.,.F.,(4,3,3,3,3,3,3,3,3,3,3,3,3,3,3,3,
3,3,3,3,3,3,3,4),(0.,0.0418556342384494,0.0858872254110088,0.12499999999993,
0.172074980585341,0.221103564965063,0.242187499999858,0.247532486136659,
0.249999999999857,0.258757699937542,0.318210861887775,0.374999999999913,
0.438770542085752,0.468749999999938,0.483289393255924,0.497396606247191,
0.499999999999944,0.586546600221947,0.674398015536128,0.74316632133627,
0.749999999999972,0.83928111752282,0.929643697667232,1.),.UNSPECIFIED.);
#5256=B_SPLINE_CURVE_WITH_KNOTS('',3,(#178643,#178644,#178645,#178646,#178647,
#178648,#178649,#178650,#178651,#178652,#178653,#178654,#178655,#178656,
#178657,#178658,#178659,#178660,#178661,#178662,#178663,#178664,#178665,
#178666,#178667,#178668,#178669,#178670,#178671,#178672,#178673),
 .UNSPECIFIED.,.F.,.F.,(4,3,3,3,3,3,3,3,3,3,4),(0.,0.000166652275730501,
0.000342276073641851,0.000519944361542677,0.000694209917748756,0.000732292525246715,
0.000732496372314203,0.000946324251635091,0.0011572677042798,0.00135942283981261,
0.00146458505049343),.UNSPECIFIED.);
#5257=B_SPLINE_CURVE_WITH_KNOTS('',3,(#178694,#178695,#178696,#178697,#178698,
#178699,#178700,#178701,#178702,#178703,#178704,#178705,#178706,#178707,
#178708,#178709,#178710,#178711,#178712,#178713,#178714,#178715,#178716,
#178717,#178718,#178719,#178720,#178721,#178722,#178723,#178724,#178725,
#178726,#178727,#178728,#178729,#178730,#178731,#178732,#178733,#178734,
#178735,#178736,#178737,#178738,#178739,#178740,#178741,#178742,#178743,
#178744,#178745,#178746,#178747,#178748,#178749,#178750,#178751,#178752,
#178753,#178754,#178755,#178756,#178757,#178758,#178759,#178760,#178761,
#178762,#178763),.UNSPECIFIED.,.F.,.F.,(4,3,3,3,3,3,3,3,3,3,3,3,3,3,3,3,
3,3,3,3,3,3,3,4),(1.89239362219216E-7,0.109656192603923,0.214471642067222,
0.250000000000101,0.350954415556579,0.44027528545044,0.48437500000021,0.494567477383746,
0.495748146752598,0.500000000000218,0.584905953245314,0.625000000000277,
0.687500000000317,0.718750000000337,0.734375000000348,0.742187500000354,
0.747999956706539,0.75000000000036,0.801011505835862,0.850758629376896,
0.899080436624542,0.945809460694209,0.990195448603225,1.),.UNSPECIFIED.);
#5258=B_SPLINE_CURVE_WITH_KNOTS('',3,(#178765,#178766,#178767,#178768,#178769,
#178770,#178771,#178772,#178773,#178774,#178775,#178776,#178777,#178778,
#178779,#178780,#178781,#178782,#178783,#178784,#178785,#178786,#178787,
#178788,#178789,#178790,#178791,#178792,#178793,#178794,#178795,#178796,
#178797,#178798,#178799,#178800,#178801,#178802,#178803,#178804,#178805,
#178806,#178807,#178808,#178809,#178810,#178811,#178812,#178813,#178814,
#178815,#178816,#178817,#178818,#178819),.UNSPECIFIED.,.F.,.F.,(4,3,3,3,
3,3,3,3,3,3,3,3,3,3,3,3,3,3,4),(3.58447939321108E-8,0.140119837080351,0.271105288786313,
0.384337543497189,0.440953670852627,0.469261734530347,0.483415766369206,
0.490492782288636,0.494031290248351,0.495800544228208,0.496350538320295,
0.497569798208066,0.499532416183815,0.499974395152803,0.500257543470681,
0.662105397139048,0.822253299281346,0.98089203121495,1.),.UNSPECIFIED.);
#5259=B_SPLINE_CURVE_WITH_KNOTS('',3,(#178837,#178838,#178839,#178840,#178841,
#178842,#178843,#178844,#178845,#178846,#178847,#178848,#178849,#178850,
#178851,#178852,#178853,#178854,#178855,#178856,#178857,#178858,#178859,
#178860,#178861,#178862,#178863,#178864,#178865,#178866,#178867,#178868,
#178869,#178870,#178871,#178872,#178873,#178874,#178875,#178876,#178877,
#178878,#178879,#178880,#178881,#178882,#178883,#178884,#178885),
 .UNSPECIFIED.,.F.,.F.,(4,3,3,3,3,3,3,3,3,3,3,3,3,3,3,3,4),(0.,0.104670426468367,
0.210224880572374,0.249999999999829,0.354199578347449,0.438725565324252,
0.484374999999684,0.493467343025674,0.499999999999679,0.577519175226156,
0.651750918301883,0.721751437166635,0.74999999999984,0.814856950659882,
0.877899885674253,0.938949942837126,1.),.UNSPECIFIED.);
#5260=B_SPLINE_CURVE_WITH_KNOTS('',3,(#178893,#178894,#178895,#178896,#178897,
#178898,#178899,#178900,#178901,#178902,#178903,#178904,#178905,#178906,
#178907,#178908,#178909,#178910,#178911,#178912,#178913,#178914,#178915,
#178916,#178917,#178918,#178919,#178920,#178921,#178922,#178923,#178924,
#178925,#178926,#178927,#178928,#178929,#178930,#178931,#178932,#178933,
#178934,#178935,#178936,#178937,#178938,#178939,#178940,#178941,#178942,
#178943,#178944),.UNSPECIFIED.,.F.,.F.,(4,3,3,3,3,3,3,3,3,3,3,3,3,3,3,3,
3,4),(0.,0.0624999999999843,0.124900823539908,0.19003423091758,0.249999999999937,
0.319870182290624,0.374999999999898,0.437499999999879,0.468749999999869,
0.484374999999867,0.494074303446313,0.499999999999866,0.591975494556334,
0.685251275110955,0.780573779554895,0.877101419317664,0.97544533364762,
1.),.UNSPECIFIED.);
#5261=B_SPLINE_CURVE_WITH_KNOTS('',3,(#178991,#178992,#178993,#178994,#178995,
#178996,#178997,#178998,#178999,#179000,#179001,#179002,#179003,#179004,
#179005,#179006,#179007,#179008,#179009,#179010,#179011,#179012,#179013,
#179014,#179015,#179016,#179017,#179018,#179019,#179020,#179021,#179022,
#179023,#179024,#179025,#179026,#179027,#179028,#179029,#179030,#179031,
#179032,#179033,#179034,#179035,#179036,#179037,#179038,#179039,#179040,
#179041,#179042,#179043,#179044,#179045,#179046,#179047,#179048,#179049,
#179050,#179051,#179052,#179053,#179054,#179055,#179056,#179057,#179058,
#179059,#179060,#179061,#179062,#179063,#179064,#179065,#179066),
 .UNSPECIFIED.,.F.,.F.,(4,3,3,3,3,3,3,3,3,3,3,3,3,3,3,3,3,3,3,3,3,3,3,3,
3,4),(0.,0.0427402135105615,0.0873806279031941,0.133137916968273,0.180400098768673,
0.187499999999966,0.218749999999969,0.234374999999968,0.242187499999964,
0.247546309647879,0.249999999999959,0.309558526821291,0.370252346988014,
0.432604522742537,0.437499999999955,0.468749999999956,0.483324625619423,
0.497499771299632,0.499999999999956,0.577335604024361,0.655589231504514,
0.734790431766,0.815465264185707,0.897008160634072,0.979844363470657,1.),
 .UNSPECIFIED.);
#5262=B_SPLINE_CURVE_WITH_KNOTS('',3,(#179073,#179074,#179075,#179076,#179077,
#179078,#179079,#179080,#179081,#179082,#179083,#179084,#179085,#179086,
#179087,#179088,#179089,#179090,#179091,#179092,#179093),.UNSPECIFIED.,
 .F.,.F.,(4,2,1,1,1,2,2,1,1,1,1,2,2,4),(0.,0.124999999999982,0.187499999999972,
0.218749999999967,0.234374999999965,0.242187499999963,0.249999999999962,
0.374999999999944,0.437499999999935,0.46874999999993,0.484374999999928,
0.492187499999928,0.499999999999928,1.),.UNSPECIFIED.);
#5263=B_SPLINE_CURVE_WITH_KNOTS('',3,(#179094,#179095,#179096,#179097),
 .UNSPECIFIED.,.F.,.F.,(4,4),(1.7347234759768E-18,0.000135753226310594),
 .UNSPECIFIED.);
#5264=B_SPLINE_CURVE_WITH_KNOTS('',3,(#179127,#179128,#179129,#179130,#179131,
#179132,#179133,#179134,#179135,#179136,#179137,#179138,#179139,#179140,
#179141,#179142,#179143,#179144,#179145,#179146,#179147,#179148,#179149,
#179150,#179151,#179152,#179153,#179154,#179155,#179156,#179157,#179158,
#179159,#179160,#179161,#179162,#179163,#179164,#179165,#179166,#179167,
#179168,#179169),.UNSPECIFIED.,.F.,.F.,(4,3,3,3,3,3,3,3,3,3,3,3,3,3,4),
(0.,0.101744188003888,0.124999999999806,0.210937499999683,0.263804240260239,
0.356835436800772,0.448994247360205,0.468749999999312,0.484374999999354,
0.488281249999364,0.492187499999375,0.499999999999396,0.720215862423713,
0.94347057076842,1.),.UNSPECIFIED.);
#5265=B_SPLINE_CURVE_WITH_KNOTS('',3,(#179220,#179221,#179222,#179223,#179224,
#179225,#179226,#179227,#179228,#179229,#179230,#179231,#179232,#179233,
#179234,#179235,#179236,#179237,#179238,#179239,#179240,#179241,#179242,
#179243,#179244,#179245,#179246,#179247,#179248,#179249,#179250,#179251,
#179252,#179253,#179254,#179255,#179256,#179257,#179258,#179259,#179260,
#179261,#179262,#179263,#179264,#179265,#179266,#179267,#179268,#179269,
#179270,#179271,#179272,#179273,#179274,#179275,#179276,#179277,#179278,
#179279,#179280,#179281,#179282,#179283,#179284,#179285,#179286,#179287,
#179288,#179289),.UNSPECIFIED.,.F.,.F.,(4,3,3,3,3,3,3,3,3,3,3,3,3,3,3,3,
3,3,3,3,3,3,3,4),(0.,0.0905130979426558,0.179924323869351,0.249999999999846,
0.256845940090264,0.344978647123152,0.429175620757808,0.468749999999701,
0.482777958801453,0.497225251801371,0.49999999999968,0.563069736113812,
0.624999999999634,0.683922647535721,0.74124546623732,0.742187499999593,
0.746915985771409,0.749999999999596,0.799322866456926,0.849492149842694,
0.894781080106962,0.938608217041727,0.980419225683544,1.),.UNSPECIFIED.);
#5266=B_SPLINE_CURVE_WITH_KNOTS('',3,(#179293,#179294,#179295,#179296,#179297,
#179298,#179299,#179300,#179301,#179302,#179303,#179304,#179305,#179306,
#179307,#179308,#179309,#179310,#179311,#179312,#179313,#179314,#179315,
#179316,#179317,#179318,#179319,#179320,#179321,#179322,#179323,#179324,
#179325,#179326,#179327,#179328,#179329,#179330,#179331,#179332,#179333,
#179334,#179335,#179336,#179337,#179338,#179339,#179340,#179341),
 .UNSPECIFIED.,.F.,.F.,(4,3,3,3,3,3,3,3,3,3,3,3,3,3,3,3,4),(0.,0.104670426730792,
0.210224881162747,0.250000000000034,0.354199578725455,0.438725566300584,
0.484375000000055,0.493467343039256,0.500000000000053,0.577519175286133,
0.65175091842001,0.721751437351517,0.750000000000026,0.814856950739285,
0.877899885834773,0.938949942917387,1.),.UNSPECIFIED.);
#5267=B_SPLINE_CURVE_WITH_KNOTS('',3,(#179349,#179350,#179351,#179352,#179353,
#179354,#179355,#179356,#179357,#179358,#179359,#179360,#179361,#179362,
#179363,#179364,#179365,#179366,#179367,#179368,#179369,#179370,#179371,
#179372,#179373,#179374,#179375,#179376,#179377,#179378,#179379,#179380,
#179381,#179382,#179383,#179384,#179385,#179386,#179387,#179388,#179389,
#179390,#179391,#179392,#179393,#179394,#179395,#179396,#179397,#179398,
#179399,#179400),.UNSPECIFIED.,.F.,.F.,(4,3,3,3,3,3,3,3,3,3,3,3,3,3,3,3,
3,4),(0.,0.0625000000000074,0.12490082348445,0.190034230807917,0.25000000000003,
0.319870182241521,0.375000000000042,0.437500000000057,0.468750000000049,
0.484375000000045,0.494074303438786,0.500000000000041,0.591975494447328,
0.685251274899277,0.780573779252049,0.877101418930033,0.975445333187664,
1.),.UNSPECIFIED.);
#5268=B_SPLINE_CURVE_WITH_KNOTS('',3,(#179446,#179447,#179448,#179449,#179450,
#179451,#179452,#179453,#179454,#179455,#179456,#179457,#179458,#179459,
#179460,#179461,#179462,#179463,#179464,#179465,#179466,#179467,#179468,
#179469,#179470,#179471,#179472,#179473,#179474,#179475,#179476,#179477,
#179478,#179479,#179480,#179481,#179482,#179483,#179484,#179485,#179486,
#179487,#179488,#179489,#179490,#179491,#179492,#179493,#179494,#179495,
#179496,#179497,#179498,#179499,#179500,#179501,#179502,#179503,#179504,
#179505,#179506,#179507,#179508,#179509,#179510,#179511,#179512,#179513,
#179514,#179515),.UNSPECIFIED.,.F.,.F.,(4,3,3,3,3,3,3,3,3,3,3,3,3,3,3,3,
3,3,3,3,3,3,3,4),(0.,0.0905130975136295,0.179924322983699,0.249999999999951,
0.256845940234234,0.344978646792586,0.429175619853906,0.468749999999914,
0.482777958649709,0.497225251507927,0.499999999999913,0.563069735586386,
0.624999999999939,0.683922647435557,0.741245466266932,0.742187499999951,
0.74691598574573,0.749999999999955,0.799322866380848,0.849492149785636,
0.894781079988712,0.938608216864493,0.980419225446453,1.),.UNSPECIFIED.);
#5269=B_SPLINE_CURVE_WITH_KNOTS('',3,(#179549,#179550,#179551,#179552,#179553,
#179554,#179555,#179556,#179557,#179558,#179559,#179560,#179561,#179562,
#179563,#179564,#179565,#179566,#179567,#179568,#179569,#179570,#179571,
#179572,#179573,#179574,#179575,#179576,#179577,#179578,#179579,#179580,
#179581,#179582,#179583,#179584,#179585,#179586,#179587,#179588,#179589,
#179590,#179591,#179592,#179593,#179594,#179595,#179596,#179597,#179598,
#179599,#179600,#179601,#179602,#179603,#179604,#179605,#179606,#179607,
#179608,#179609,#179610,#179611,#179612,#179613,#179614,#179615,#179616,
#179617,#179618,#179619,#179620,#179621,#179622,#179623,#179624),
 .UNSPECIFIED.,.F.,.F.,(4,3,3,3,3,3,3,3,3,3,3,3,3,3,3,3,3,3,3,3,3,3,3,3,
3,4),(0.,0.0430097483234137,0.0878255518128777,0.124999999999833,0.172143318494293,
0.187499999999742,0.218749999999705,0.234374999999686,0.242187499999689,
0.247546309656834,0.249999999999692,0.309158559883821,0.36986670864448,
0.374999999999702,0.43749999999971,0.468749999999719,0.483324625655138,
0.497499771373716,0.499999999999727,0.577335604004243,0.655589231465469,
0.734790431709053,0.815465264114797,0.897008160548024,0.979844363371395,
1.),.UNSPECIFIED.);
#5270=B_SPLINE_CURVE_WITH_KNOTS('',3,(#179645,#179646,#179647,#179648,#179649,
#179650,#179651,#179652,#179653,#179654,#179655,#179656,#179657,#179658,
#179659,#179660,#179661,#179662,#179663,#179664,#179665,#179666,#179667,
#179668,#179669,#179670,#179671,#179672,#179673,#179674,#179675,#179676,
#179677,#179678,#179679,#179680,#179681,#179682,#179683,#179684,#179685,
#179686,#179687,#179688,#179689,#179690,#179691,#179692,#179693,#179694,
#179695,#179696,#179697,#179698,#179699),.UNSPECIFIED.,.F.,.F.,(4,3,3,3,
3,3,3,3,3,3,3,3,3,3,3,3,3,3,4),(0.,0.104765563478566,0.210444272083717,
0.250000000000343,0.354080737693078,0.375000000000532,0.437500000000626,
0.468750000000673,0.484375000000687,0.493467332371258,0.500000000000701,
0.577628367556246,0.651921806019438,0.721921629982362,0.75000000000035,
0.814799791902674,0.877825876721737,0.938912938360868,1.),.UNSPECIFIED.);
#5271=B_SPLINE_CURVE_WITH_KNOTS('',3,(#179707,#179708,#179709,#179710,#179711,
#179712,#179713,#179714,#179715,#179716,#179717,#179718,#179719,#179720,
#179721,#179722,#179723,#179724,#179725,#179726,#179727,#179728,#179729,
#179730,#179731,#179732,#179733,#179734,#179735,#179736,#179737,#179738,
#179739,#179740,#179741,#179742,#179743,#179744,#179745,#179746,#179747,
#179748,#179749,#179750,#179751,#179752),.UNSPECIFIED.,.F.,.F.,(4,3,3,3,
3,3,3,3,3,3,3,3,3,3,3,4),(0.,0.0625000000000197,0.124542361697189,0.189407379081926,
0.250000000000079,0.320392682411276,0.396093817089821,0.473112577633271,
0.484375000000176,0.493957180841483,0.500000000000194,0.605374837099206,
0.710879749859165,0.816564755183575,0.922725793167858,1.),.UNSPECIFIED.);
#5272=B_SPLINE_CURVE_WITH_KNOTS('',3,(#179757,#179758,#179759,#179760,#179761,
#179762,#179763,#179764,#179765,#179766,#179767,#179768,#179769),
 .UNSPECIFIED.,.F.,.F.,(4,3,3,3,4),(3.1415926535898,3.53429173528852,3.92699081698724,
4.31968989868597,4.71238898038469),.UNSPECIFIED.);
#5273=B_SPLINE_CURVE_WITH_KNOTS('',3,(#179802,#179803,#179804,#179805,#179806,
#179807,#179808,#179809,#179810,#179811,#179812,#179813,#179814,#179815,
#179816,#179817,#179818,#179819,#179820,#179821,#179822,#179823,#179824,
#179825,#179826,#179827,#179828,#179829,#179830,#179831,#179832,#179833,
#179834,#179835,#179836,#179837,#179838,#179839,#179840,#179841,#179842,
#179843,#179844,#179845,#179846,#179847,#179848,#179849,#179850,#179851,
#179852,#179853,#179854,#179855,#179856,#179857,#179858,#179859,#179860,
#179861,#179862,#179863,#179864,#179865,#179866,#179867,#179868,#179869,
#179870,#179871),.UNSPECIFIED.,.F.,.F.,(4,3,3,3,3,3,3,3,3,3,3,3,3,3,3,3,
3,3,3,3,3,3,3,4),(0.,0.0418556347635635,0.0858872264664174,0.12499999999986,
0.172074981123076,0.221103566406418,0.242187499999732,0.247532486182558,
0.249999999999724,0.258757700014179,0.318210863601387,0.374999999999747,
0.438770543659797,0.468749999999766,0.483289393572595,0.497396606901275,
0.499999999999779,0.586546600897368,0.674398016851886,0.743166321541273,
0.749999999999889,0.839281118186762,0.929643698954937,1.),.UNSPECIFIED.);
#5274=B_SPLINE_CURVE_WITH_KNOTS('',3,(#179911,#179912,#179913,#179914,#179915,
#179916,#179917,#179918,#179919,#179920,#179921,#179922,#179923,#179924,
#179925,#179926,#179927,#179928,#179929,#179930,#179931,#179932,#179933,
#179934,#179935,#179936,#179937,#179938,#179939,#179940,#179941,#179942,
#179943,#179944,#179945,#179946,#179947,#179948,#179949,#179950),
 .UNSPECIFIED.,.F.,.F.,(4,3,3,3,3,3,3,3,3,3,3,3,3,4),(0.,0.000161047553671253,
0.00032665546448548,0.000493863052907836,0.000580621437699987,0.00058187576131232,
0.0011633223004275,0.00116375152262464,0.00145467271006653,0.00145468940328081,
0.00174562728393698,0.0017460231201541,0.00204798180553644,0.00232750304524933),
 .UNSPECIFIED.);
#5275=B_SPLINE_CURVE_WITH_KNOTS('',3,(#179951,#179952,#179953,#179954,#179955,
#179956,#179957,#179958,#179959,#179960,#179961,#179962,#179963,#179964,
#179965,#179966,#179967,#179968,#179969,#179970,#179971,#179972,#179973,
#179974,#179975,#179976,#179977,#179978,#179979,#179980,#179981,#179982,
#179983,#179984,#179985,#179986,#179987,#179988,#179989,#179990,#179991,
#179992,#179993,#179994,#179995,#179996,#179997,#179998,#179999,#180000,
#180001,#180002,#180003,#180004,#180005,#180006,#180007,#180008,#180009,
#180010,#180011,#180012,#180013,#180014,#180015,#180016,#180017,#180018,
#180019,#180020),.UNSPECIFIED.,.F.,.F.,(4,3,3,3,3,3,3,3,3,3,3,3,3,3,3,3,
3,3,3,3,3,3,3,4),(0.,0.0645978303967565,0.128839691720708,0.192883319322283,
0.249999999999887,0.314290451368615,0.374999999999836,0.437499999999809,
0.468749999999795,0.484374999999779,0.492187499999781,0.497804168442645,
0.499999999999782,0.555878234310221,0.609222458807199,0.661110211917442,
0.710954042038781,0.749999999999891,0.797583166200646,0.844123803798507,
0.88948355346123,0.934266047761903,0.978456173795685,1.),.UNSPECIFIED.);
#5276=B_SPLINE_CURVE_WITH_KNOTS('',3,(#180028,#180029,#180030,#180031,#180032,
#180033,#180034,#180035,#180036,#180037,#180038,#180039,#180040,#180041,
#180042,#180043,#180044,#180045,#180046,#180047,#180048,#180049,#180050,
#180051,#180052,#180053,#180054,#180055,#180056,#180057,#180058,#180059,
#180060,#180061,#180062,#180063,#180064,#180065,#180066,#180067,#180068,
#180069,#180070,#180071,#180072,#180073,#180074,#180075,#180076,#180077,
#180078,#180079,#180080,#180081,#180082),.UNSPECIFIED.,.F.,.F.,(4,3,3,3,
3,3,3,3,3,3,3,3,3,3,3,3,3,3,4),(0.,0.104765563474887,0.210444272078553,
0.250000000000062,0.35408073770077,0.375000000000105,0.437500000000124,
0.468750000000142,0.484375000000157,0.493467332370735,0.500000000000172,
0.577628367556476,0.651921806020633,0.721921629984373,0.750000000000086,
0.814799791903652,0.877825876724308,0.938912938362154,1.),.UNSPECIFIED.);
#5277=B_SPLINE_CURVE_WITH_KNOTS('',3,(#180090,#180091,#180092,#180093,#180094,
#180095,#180096,#180097,#180098,#180099,#180100,#180101,#180102,#180103,
#180104,#180105,#180106,#180107,#180108,#180109,#180110,#180111,#180112,
#180113,#180114,#180115,#180116,#180117,#180118,#180119,#180120,#180121,
#180122,#180123,#180124,#180125,#180126,#180127,#180128,#180129,#180130,
#180131,#180132,#180133,#180134,#180135),.UNSPECIFIED.,.F.,.F.,(4,3,3,3,
3,3,3,3,3,3,3,3,3,3,3,4),(0.,0.0625000000000364,0.124542361523147,0.189407378742922,
0.250000000000146,0.32039268227165,0.39609381677263,0.473112576960276,0.484375000000262,
0.493957180819043,0.500000000000255,0.605374836184627,0.710879748162737,
0.816564752767341,0.922725790120419,1.),.UNSPECIFIED.);
#5278=B_SPLINE_CURVE_WITH_KNOTS('',3,(#180183,#180184,#180185,#180186,#180187,
#180188,#180189,#180190,#180191,#180192,#180193,#180194,#180195,#180196,
#180197,#180198,#180199,#180200,#180201,#180202,#180203,#180204,#180205,
#180206,#180207,#180208,#180209,#180210,#180211,#180212,#180213,#180214,
#180215,#180216,#180217,#180218,#180219,#180220,#180221,#180222,#180223,
#180224,#180225,#180226,#180227,#180228,#180229,#180230,#180231,#180232,
#180233,#180234,#180235,#180236,#180237,#180238,#180239,#180240,#180241,
#180242,#180243,#180244,#180245,#180246,#180247,#180248,#180249,#180250,
#180251,#180252,#180253,#180254,#180255),.UNSPECIFIED.,.F.,.F.,(4,3,3,3,
3,3,3,3,3,3,3,3,3,3,3,3,3,3,3,3,3,3,3,3,4),(0.,0.0828931316413898,0.16418560379089,
0.244579415455065,0.323661834828471,0.374999999999967,0.437499999999958,
0.468749999999954,0.4828085023222,0.497325258675924,0.49999999999995,0.563237806906317,
0.624999999999955,0.687499999999966,0.718749999999971,0.734374999999977,
0.742187499999976,0.746930749059886,0.749999999999976,0.798769942866912,
0.846465940839484,0.892304177591545,0.936986220520651,0.979988998076433,
1.),.UNSPECIFIED.);
#5279=B_SPLINE_CURVE_WITH_KNOTS('',3,(#180288,#180289,#180290,#180291,#180292,
#180293,#180294,#180295,#180296,#180297,#180298,#180299,#180300,#180301,
#180302,#180303,#180304,#180305,#180306,#180307,#180308,#180309,#180310,
#180311,#180312,#180313,#180314,#180315,#180316,#180317,#180318,#180319,
#180320,#180321,#180322,#180323,#180324,#180325,#180326,#180327,#180328,
#180329,#180330,#180331,#180332,#180333,#180334,#180335,#180336,#180337,
#180338,#180339,#180340,#180341,#180342,#180343,#180344,#180345,#180346,
#180347,#180348,#180349,#180350,#180351,#180352,#180353,#180354,#180355,
#180356,#180357),.UNSPECIFIED.,.F.,.F.,(4,3,3,3,3,3,3,3,3,3,3,3,3,3,3,3,
3,3,3,3,3,3,3,4),(0.,0.0418167934441984,0.085151181427437,0.130899470147945,
0.178154905267451,0.227239765683116,0.24218750000028,0.247532486200105,
0.250000000000283,0.258757700046366,0.318210864309325,0.375000000000234,
0.438770544391353,0.468750000000198,0.483289393711794,0.497396607188351,
0.500000000000183,0.586546601298008,0.674398017630146,0.743166321661521,
0.750000000000092,0.839281118572534,0.92964369970189,1.),.UNSPECIFIED.);
#5280=B_SPLINE_CURVE_WITH_KNOTS('',3,(#180377,#180378,#180379,#180380,#180381,
#180382,#180383,#180384,#180385,#180386,#180387,#180388,#180389,#180390,
#180391,#180392,#180393,#180394,#180395,#180396,#180397,#180398,#180399,
#180400,#180401,#180402,#180403,#180404,#180405,#180406,#180407,#180408,
#180409,#180410,#180411,#180412,#180413,#180414,#180415,#180416,#180417,
#180418,#180419,#180420,#180421,#180422,#180423,#180424,#180425),
 .UNSPECIFIED.,.F.,.F.,(4,3,3,3,3,3,3,3,3,3,3,3,3,3,3,3,4),(0.,0.104670426541109,
0.210224880734563,0.249999999999775,0.354199578449117,0.438725567291639,
0.484374999999608,0.493467343029225,0.499999999999603,0.577519175242144,
0.651750918333578,0.721751437216418,0.749999999999802,0.814856950681533,
0.877899885718081,0.93894994285904,1.),.UNSPECIFIED.);
#5281=B_SPLINE_CURVE_WITH_KNOTS('',3,(#180433,#180434,#180435,#180436,#180437,
#180438,#180439,#180440,#180441,#180442,#180443,#180444,#180445,#180446,
#180447,#180448,#180449,#180450,#180451,#180452,#180453,#180454,#180455,
#180456,#180457,#180458,#180459,#180460,#180461,#180462,#180463,#180464,
#180465,#180466,#180467,#180468,#180469,#180470,#180471,#180472,#180473,
#180474,#180475,#180476,#180477,#180478,#180479,#180480,#180481,#180482,
#180483,#180484),.UNSPECIFIED.,.F.,.F.,(4,3,3,3,3,3,3,3,3,3,3,3,3,3,3,3,
3,4),(0.,0.0603576848723925,0.122428434116216,0.187494850857853,0.254338193740552,
0.324292162869377,0.37500000000018,0.4375000000002,0.468750000000182,0.484375000000177,
0.494074303427759,0.500000000000172,0.591975494289549,0.685251274592972,
0.780573778813809,0.877101418369239,0.975445332522005,1.),.UNSPECIFIED.);
#5282=B_SPLINE_CURVE_WITH_KNOTS('',3,(#180531,#180532,#180533,#180534,#180535,
#180536,#180537,#180538,#180539,#180540,#180541,#180542,#180543,#180544,
#180545,#180546,#180547,#180548,#180549,#180550,#180551,#180552,#180553,
#180554,#180555,#180556,#180557,#180558,#180559,#180560,#180561,#180562,
#180563,#180564,#180565,#180566,#180567,#180568,#180569,#180570,#180571,
#180572,#180573,#180574,#180575,#180576,#180577,#180578,#180579,#180580,
#180581,#180582,#180583,#180584,#180585,#180586,#180587,#180588,#180589,
#180590,#180591,#180592,#180593,#180594,#180595,#180596,#180597,#180598,
#180599,#180600,#180601,#180602,#180603,#180604,#180605,#180606),
 .UNSPECIFIED.,.F.,.F.,(4,3,3,3,3,3,3,3,3,3,3,3,3,3,3,3,3,3,3,3,3,3,3,3,
3,4),(0.,0.0430097487356867,0.0878255526448179,0.124999999999681,0.172143318924996,
0.187499999999521,0.218749999999441,0.234374999999418,0.242187499999425,
0.247546309684307,0.249999999999432,0.309158560680158,0.369866710216006,
0.374999999999513,0.437499999999554,0.468749999999584,0.483324625807977,
0.497499771690094,0.499999999999615,0.577335604065574,0.65558923158524,
0.734790431884213,0.815465264338645,0.897008160817874,0.979844363681157,
1.),.UNSPECIFIED.);
#5283=B_SPLINE_CURVE_WITH_KNOTS('',3,(#180612,#180613,#180614,#180615,#180616,
#180617,#180618,#180619,#180620,#180621,#180622,#180623,#180624,#180625,
#180626,#180627,#180628,#180629,#180630,#180631,#180632),.UNSPECIFIED.,
 .F.,.F.,(4,2,1,1,1,2,2,1,1,1,1,2,2,4),(0.,0.125000000000008,0.18750000000001,
0.218750000000008,0.234375000000006,0.242187500000008,0.250000000000009,
0.375000000000036,0.437500000000049,0.468750000000053,0.484375000000051,
0.492187500000049,0.500000000000047,1.),.UNSPECIFIED.);
#5284=B_SPLINE_CURVE_WITH_KNOTS('',3,(#180635,#180636,#180637,#180638,#180639,
#180640,#180641,#180642,#180643,#180644,#180645,#180646,#180647,#180648,
#180649,#180650,#180651,#180652,#180653,#180654,#180655,#180656,#180657,
#180658,#180659,#180660,#180661,#180662,#180663,#180664,#180665),
 .UNSPECIFIED.,.F.,.F.,(4,3,3,3,3,3,3,3,3,3,4),(0.,0.000118224492354554,
0.000239962463540374,0.000354016906950293,0.000486351214795248,0.000618764034602114,
0.000708033813900585,0.000911280042592202,0.00111586864896652,0.00131545298196076,
0.00141606762780121),.UNSPECIFIED.);
#5285=B_SPLINE_CURVE_WITH_KNOTS('',3,(#180688,#180689,#180690,#180691,#180692,
#180693,#180694,#180695,#180696,#180697,#180698,#180699,#180700,#180701,
#180702,#180703),.UNSPECIFIED.,.F.,.F.,(4,2,2,2,1,1,2,2,4),(0.,0.25000000000023,
0.375000000000355,0.437500000000406,0.468750000000446,0.484375000000451,
0.492187500000452,0.500000000000452,1.),.UNSPECIFIED.);
#5286=B_SPLINE_CURVE_WITH_KNOTS('',3,(#180748,#180749,#180750,#180751,#180752,
#180753,#180754,#180755,#180756,#180757,#180758,#180759,#180760,#180761,
#180762,#180763,#180764,#180765,#180766,#180767,#180768,#180769,#180770,
#180771,#180772,#180773,#180774,#180775,#180776,#180777,#180778,#180779,
#180780,#180781,#180782,#180783,#180784,#180785,#180786,#180787,#180788,
#180789,#180790,#180791,#180792,#180793,#180794,#180795,#180796,#180797,
#180798,#180799,#180800,#180801,#180802,#180803,#180804,#180805,#180806,
#180807,#180808,#180809,#180810,#180811,#180812,#180813,#180814,#180815,
#180816,#180817),.UNSPECIFIED.,.F.,.F.,(4,3,3,3,3,3,3,3,3,3,3,3,3,3,3,3,
3,3,3,3,3,3,3,4),(0.,0.0905130970652387,0.179924322055766,0.250000000000042,
0.25684594038563,0.344978646443199,0.429175619074524,0.468750000000064,
0.4827779584993,0.497225251216987,0.500000000000063,0.563069735064877,0.625,
0.683922646620614,0.741245466295442,0.742187499999971,0.746915985725626,
0.749999999999977,0.799322866332637,0.849492149749478,0.894781079909806,
0.938608216744346,0.980419225283251,1.),.UNSPECIFIED.);
#5287=B_SPLINE_CURVE_WITH_KNOTS('',3,(#180824,#180825,#180826,#180827,#180828,
#180829,#180830,#180831,#180832,#180833,#180834,#180835,#180836,#180837,
#180838,#180839,#180840,#180841,#180842,#180843,#180844,#180845,#180846,
#180847,#180848,#180849,#180850,#180851,#180852,#180853,#180854,#180855,
#180856,#180857,#180858,#180859,#180860,#180861,#180862,#180863,#180864,
#180865,#180866,#180867,#180868,#180869,#180870,#180871,#180872),
 .UNSPECIFIED.,.F.,.F.,(4,3,3,3,3,3,3,3,3,3,3,3,3,3,3,3,4),(0.,0.104670426476868,
0.210224880592324,0.250000000000098,0.354199578363952,0.438725565774003,
0.484375000000191,0.493467343026711,0.500000000000194,0.577519175228676,
0.651750918306284,0.721751437173546,0.750000000000097,0.814856950663166,
0.877899885680621,0.93894994284031,1.),.UNSPECIFIED.);
#5288=B_SPLINE_CURVE_WITH_KNOTS('',3,(#180880,#180881,#180882,#180883,#180884,
#180885,#180886,#180887,#180888,#180889,#180890,#180891,#180892,#180893,
#180894,#180895,#180896,#180897,#180898,#180899,#180900,#180901,#180902,
#180903,#180904,#180905,#180906,#180907,#180908,#180909,#180910,#180911,
#180912,#180913,#180914,#180915,#180916,#180917,#180918,#180919,#180920,
#180921,#180922,#180923,#180924,#180925,#180926,#180927,#180928,#180929,
#180930,#180931),.UNSPECIFIED.,.F.,.F.,(4,3,3,3,3,3,3,3,3,3,3,3,3,3,3,3,
3,4),(0.,0.0625000000000059,0.124900823533827,0.190034230905517,0.250000000000024,
0.319870182285393,0.375000000000043,0.43750000000004,0.468750000000034,
0.484375000000031,0.494074303445622,0.500000000000028,0.591975494544407,
0.685251275087606,0.780573779521403,0.877101419274667,0.975445333596583,
1.),.UNSPECIFIED.);
#5289=B_SPLINE_CURVE_WITH_KNOTS('',3,(#180977,#180978,#180979,#180980,#180981,
#180982,#180983,#180984,#180985,#180986,#180987,#180988,#180989,#180990,
#180991,#180992,#180993,#180994,#180995,#180996,#180997,#180998,#180999,
#181000,#181001,#181002,#181003,#181004,#181005,#181006,#181007,#181008,
#181009,#181010,#181011,#181012,#181013,#181014,#181015,#181016,#181017,
#181018,#181019,#181020,#181021,#181022,#181023,#181024,#181025,#181026,
#181027,#181028,#181029,#181030,#181031,#181032,#181033,#181034,#181035,
#181036,#181037,#181038,#181039,#181040,#181041,#181042,#181043,#181044,
#181045,#181046),.UNSPECIFIED.,.F.,.F.,(4,3,3,3,3,3,3,3,3,3,3,3,3,3,3,3,
3,3,3,3,3,3,3,4),(0.,0.0905130976711778,0.179924323296518,0.2500000000002,
0.256845940181976,0.344978646915006,0.429175619818899,0.46875000000037,
0.482777958797654,0.497225251792372,0.500000000000387,0.563069736211347,
0.625000000000415,0.683922647615147,0.741245466233434,0.742187500000435,
0.746915985752997,0.750000000000441,0.799322866751923,0.849492150063943,
0.894781080567531,0.938608217733336,0.980419226610287,1.),.UNSPECIFIED.);
#5290=B_SPLINE_CURVE_WITH_KNOTS('',3,(#181080,#181081,#181082,#181083,#181084,
#181085,#181086,#181087,#181088,#181089,#181090,#181091,#181092,#181093,
#181094,#181095,#181096,#181097,#181098,#181099,#181100,#181101,#181102,
#181103,#181104,#181105,#181106,#181107,#181108,#181109,#181110,#181111,
#181112,#181113,#181114,#181115,#181116,#181117,#181118,#181119,#181120,
#181121,#181122,#181123,#181124,#181125,#181126,#181127,#181128,#181129,
#181130,#181131,#181132,#181133,#181134,#181135,#181136,#181137,#181138,
#181139,#181140,#181141,#181142,#181143,#181144,#181145,#181146,#181147,
#181148,#181149,#181150,#181151,#181152,#181153,#181154,#181155),
 .UNSPECIFIED.,.F.,.F.,(4,3,3,3,3,3,3,3,3,3,3,3,3,3,3,3,3,3,3,3,3,3,3,3,
3,4),(0.,0.0430097489401156,0.0878255530574435,0.125000000000092,0.172143319139764,
0.187500000000139,0.21875000000016,0.234375000000171,0.242187500000173,
0.247546309687597,0.250000000000175,0.309158560547553,0.369866709953412,
0.375000000000161,0.437851735660631,0.468750000000141,0.483324625752687,
0.497499771574761,0.500000000000134,0.577335603884166,0.65558923123085,
0.734790431366338,0.81546526367158,0.897008160014305,0.979844362759134,
1.),.UNSPECIFIED.);
#5291=B_SPLINE_CURVE_WITH_KNOTS('',3,(#181204,#181205,#181206,#181207,#181208,
#181209,#181210,#181211,#181212,#181213,#181214,#181215,#181216,#181217,
#181218,#181219,#181220,#181221),.UNSPECIFIED.,.F.,.F.,(4,2,2,2,1,1,2,2,
2,4),(0.,0.249999999999941,0.374999999999907,0.437499999999891,0.468749999999884,
0.484374999999875,0.492187499999875,0.499999999999874,0.749999999999937,
1.),.UNSPECIFIED.);
#5292=B_SPLINE_CURVE_WITH_KNOTS('',3,(#181229,#181230,#181231,#181232,#181233,
#181234,#181235,#181236,#181237,#181238,#181239,#181240,#181241,#181242,
#181243,#181244,#181245,#181246,#181247,#181248,#181249,#181250,#181251,
#181252,#181253,#181254,#181255,#181256,#181257,#181258,#181259,#181260,
#181261,#181262,#181263,#181264,#181265,#181266,#181267,#181268,#181269,
#181270,#181271,#181272,#181273,#181274,#181275,#181276,#181277,#181278,
#181279,#181280),.UNSPECIFIED.,.F.,.F.,(4,3,3,3,3,3,3,3,3,3,3,3,3,3,3,3,
3,4),(0.,0.0670765920356927,0.13598231875245,0.207892462939091,0.28167954349829,
0.358370245208511,0.374999999999787,0.437499999999752,0.468749999999743,
0.484374999999756,0.49392515163699,0.499999999999768,0.589682112064697,
0.680498948238462,0.773128091633332,0.866800460343817,0.962105139368486,
1.),.UNSPECIFIED.);
#5293=B_SPLINE_CURVE_WITH_KNOTS('',3,(#181308,#181309,#181310,#181311,#181312,
#181313,#181314,#181315,#181316,#181317,#181318,#181319,#181320,#181321,
#181322,#181323,#181324,#181325,#181326,#181327,#181328,#181329,#181330,
#181331,#181332,#181333,#181334,#181335,#181336,#181337,#181338,#181339,
#181340,#181341,#181342,#181343,#181344),.UNSPECIFIED.,.F.,.F.,(4,3,3,3,
3,3,3,3,3,3,3,3,4),(0.000461676008985161,0.000632546215505795,0.00084808124100127,
0.000931278160334732,0.0011451568350677,0.00130839695615338,0.00168583810655035,
0.00182863766115024,0.00206327508940322,0.0024407173257478,0.00251211848723277,
0.00307037767189825,0.00319559931331531),.UNSPECIFIED.);
#5294=B_SPLINE_CURVE_WITH_KNOTS('',3,(#181403,#181404,#181405,#181406,#181407,
#181408,#181409,#181410,#181411,#181412,#181413,#181414,#181415,#181416),
 .UNSPECIFIED.,.F.,.F.,(4,2,2,2,2,2,4),(0.,0.249999999999991,0.374999999999987,
0.437499999999983,0.499999999999979,0.749999999999989,1.),.UNSPECIFIED.);
#5295=B_SPLINE_CURVE_WITH_KNOTS('',3,(#181417,#181418,#181419,#181420,#181421,
#181422,#181423,#181424,#181425,#181426,#181427,#181428,#181429,#181430,
#181431,#181432,#181433,#181434,#181435,#181436,#181437,#181438,#181439,
#181440,#181441,#181442,#181443,#181444,#181445,#181446),.UNSPECIFIED.,
 .F.,.F.,(4,2,2,2,1,1,1,2,2,2,2,1,1,1,2,2,2,4),(0.,0.125000000000023,0.187500000000034,
0.218750000000039,0.234375000000041,0.242187500000045,0.246093750000045,
0.248046875000043,0.250000000000041,0.374999999999938,0.437499999999886,
0.468749999999863,0.48437499999985,0.492187499999843,0.496093749999843,
0.499999999999843,0.749999999999921,1.),.UNSPECIFIED.);
#5296=B_SPLINE_CURVE_WITH_KNOTS('',3,(#181461,#181462,#181463,#181464,#181465,
#181466,#181467,#181468,#181469,#181470,#181471,#181472,#181473,#181474,
#181475,#181476,#181477,#181478,#181479,#181480,#181481,#181482,#181483,
#181484,#181485,#181486,#181487,#181488,#181489,#181490,#181491,#181492,
#181493,#181494,#181495,#181496,#181497,#181498,#181499,#181500,#181501,
#181502,#181503,#181504,#181505,#181506,#181507,#181508,#181509,#181510,
#181511,#181512,#181513,#181514,#181515,#181516,#181517,#181518,#181519,
#181520,#181521,#181522,#181523,#181524,#181525,#181526,#181527,#181528,
#181529,#181530,#181531,#181532,#181533,#181534,#181535,#181536,#181537,
#181538,#181539,#181540,#181541,#181542,#181543,#181544,#181545,#181546,
#181547,#181548,#181549,#181550,#181551,#181552,#181553,#181554,#181555,
#181556,#181557,#181558,#181559,#181560,#181561,#181562,#181563,#181564,
#181565,#181566,#181567,#181568,#181569,#181570,#181571,#181572,#181573,
#181574,#181575,#181576,#181577,#181578,#181579,#181580,#181581,#181582,
#181583,#181584,#181585,#181586,#181587,#181588,#181589,#181590),
 .UNSPECIFIED.,.F.,.F.,(4,3,3,3,3,3,3,3,3,3,3,3,3,3,3,3,3,3,3,3,3,3,3,3,
3,3,3,3,3,3,3,3,3,3,3,3,3,3,3,3,3,3,3,4),(0.,0.062499999999966,0.120656530897949,
0.176870757385599,0.230542201431043,0.249999999999864,0.259793340669136,
0.313569339020365,0.35253241852512,0.371529541832909,0.380609090930782,
0.425963310764886,0.461524220485096,0.479304675345201,0.488194902775253,
0.49264001649028,0.495270859962502,0.495839588709159,0.496320627056616,
0.497085130205306,0.499236772471531,0.499899226174417,0.5001602572298,0.567475246236759,
0.601132740740238,0.61841473872259,0.633624637649322,0.634790235243718,
0.671680165287415,0.690752079936576,0.730043729761344,0.748046874999687,
0.748752498895434,0.749999999999691,0.779220977126903,0.808330934535299,
0.837387447374634,0.86638313108366,0.874999999999846,0.903412282810721,
0.93238433174654,0.961715718964714,0.991613901781098,1.),.UNSPECIFIED.);
#5297=B_SPLINE_CURVE_WITH_KNOTS('',3,(#181634,#181635,#181636,#181637,#181638,
#181639,#181640,#181641,#181642,#181643,#181644,#181645,#181646,#181647,
#181648,#181649,#181650,#181651,#181652,#181653,#181654,#181655,#181656,
#181657,#181658,#181659,#181660,#181661,#181662,#181663,#181664,#181665,
#181666,#181667,#181668,#181669,#181670,#181671,#181672,#181673,#181674,
#181675,#181676,#181677,#181678,#181679,#181680,#181681,#181682,#181683,
#181684,#181685,#181686,#181687,#181688,#181689,#181690,#181691),
 .UNSPECIFIED.,.F.,.F.,(4,3,3,3,3,3,3,3,3,3,3,3,3,3,3,3,3,3,3,4),(0.,0.0624999999999946,
0.132935195695894,0.187179787252051,0.220234134189882,0.236211803414422,
0.26695249642912,0.339621823531675,0.395049568810745,0.445404134727815,
0.458833950506198,0.484374999999953,0.493493076075797,0.499999999999957,
0.585514487699712,0.672074572499599,0.730941551546193,0.820268275761333,
0.912558465070212,1.),.UNSPECIFIED.);
#5298=B_SPLINE_CURVE_WITH_KNOTS('',3,(#181692,#181693,#181694,#181695,#181696,
#181697,#181698,#181699,#181700,#181701,#181702,#181703,#181704,#181705,
#181706,#181707,#181708,#181709,#181710,#181711,#181712,#181713,#181714,
#181715,#181716,#181717,#181718,#181719,#181720,#181721,#181722,#181723,
#181724,#181725,#181726,#181727,#181728),.UNSPECIFIED.,.F.,.F.,(4,3,3,3,
3,3,3,3,3,3,3,3,4),(0.,0.000289456070004167,0.000578912140008334,0.000732555002063405,
0.00109883518473064,0.00115782428001667,0.00146516214354768,0.001736736420025,
0.00183135727517645,0.00202619249002917,0.00217092052503125,0.00219767702911212,
0.00231564856003333),.UNSPECIFIED.);
#5299=B_SPLINE_CURVE_WITH_KNOTS('',3,(#181755,#181756,#181757,#181758,#181759,
#181760,#181761,#181762,#181763,#181764,#181765,#181766,#181767,#181768,
#181769,#181770,#181771,#181772,#181773,#181774,#181775,#181776,#181777,
#181778,#181779,#181780,#181781,#181782),.UNSPECIFIED.,.F.,.F.,(4,3,3,3,
3,3,3,3,3,4),(0.000653658633860215,0.000901612111392076,0.00110350292160905,
0.00119693882169383,0.00132842506548346,0.00148931670393185,0.00155334720935788,
0.0018252077501562,0.00223261138725129,0.00245303578485557),
 .UNSPECIFIED.);
#5300=B_SPLINE_CURVE_WITH_KNOTS('',3,(#181829,#181830,#181831,#181832,#181833,
#181834,#181835,#181836,#181837,#181838,#181839,#181840,#181841,#181842,
#181843,#181844,#181845,#181846,#181847,#181848,#181849,#181850,#181851,
#181852,#181853,#181854,#181855,#181856,#181857,#181858,#181859,#181860,
#181861,#181862,#181863,#181864,#181865,#181866,#181867,#181868,#181869,
#181870,#181871,#181872,#181873,#181874,#181875,#181876,#181877,#181878,
#181879,#181880,#181881,#181882,#181883,#181884,#181885,#181886,#181887,
#181888,#181889,#181890,#181891,#181892,#181893,#181894,#181895,#181896,
#181897,#181898,#181899,#181900,#181901),.UNSPECIFIED.,.F.,.F.,(4,3,3,3,
3,3,3,3,3,3,3,3,3,3,3,3,3,3,3,3,3,3,3,3,4),(8.44303797994522E-15,0.135144161881906,
0.24999999999991,0.349909277361936,0.374999999999867,0.437499999999847,
0.46874999999984,0.484374999999842,0.493921148051312,0.499999999999845,
0.562216067098283,0.565498317572536,0.624999999999914,0.67538814217395,
0.683242331719054,0.687499999999947,0.718749999999953,0.73193993458769,
0.744411742542878,0.749999999999959,0.795268362209216,0.848575988791016,
0.901164076236429,0.952422125938682,1.),.UNSPECIFIED.);
#5301=B_SPLINE_CURVE_WITH_KNOTS('',3,(#181902,#181903,#181904,#181905,#181906,
#181907,#181908,#181909,#181910,#181911,#181912,#181913,#181914,#181915,
#181916,#181917,#181918,#181919,#181920,#181921,#181922,#181923,#181924,
#181925,#181926,#181927,#181928,#181929,#181930,#181931,#181932,#181933,
#181934,#181935,#181936,#181937,#181938,#181939,#181940,#181941),
 .UNSPECIFIED.,.F.,.F.,(4,3,3,3,3,3,3,3,3,3,3,3,3,4),(0.,0.0779250053195204,
0.155057508641545,0.231528329066271,0.307465716646408,0.382995817637975,
0.460121340433228,0.535227647548595,0.610339521074979,0.685565358678351,
0.764174019008763,0.840195626431609,0.920097813215804,1.),.UNSPECIFIED.);
#5302=B_SPLINE_CURVE_WITH_KNOTS('',3,(#181956,#181957,#181958,#181959,#181960,
#181961,#181962,#181963,#181964,#181965,#181966,#181967,#181968,#181969,
#181970,#181971,#181972,#181973,#181974,#181975,#181976,#181977,#181978,
#181979,#181980,#181981,#181982,#181983,#181984,#181985,#181986,#181987,
#181988,#181989,#181990,#181991,#181992,#181993,#181994,#181995,#181996,
#181997,#181998,#181999,#182000,#182001,#182002,#182003,#182004,#182005,
#182006,#182007,#182008,#182009,#182010,#182011,#182012,#182013,#182014,
#182015,#182016),.UNSPECIFIED.,.F.,.F.,(4,3,3,3,3,3,3,3,3,3,3,3,3,3,3,3,
3,3,3,3,4),(0.,0.0773791158424523,0.154909736797379,0.232737497421732,0.25,
0.333103137439076,0.348714047736977,0.408234656906365,0.465438190403892,
0.5,0.554799431810658,0.601556608085492,0.65460625822029,0.708180619658644,
0.75,0.798278525182264,0.811109335356995,0.861461000849684,0.911120449252677,
0.959993731055844,1.),.UNSPECIFIED.);
#5303=B_SPLINE_CURVE_WITH_KNOTS('',3,(#182048,#182049,#182050,#182051,#182052,
#182053,#182054,#182055,#182056,#182057,#182058,#182059,#182060,#182061,
#182062,#182063,#182064,#182065,#182066,#182067,#182068,#182069,#182070,
#182071,#182072,#182073,#182074,#182075,#182076,#182077,#182078,#182079,
#182080,#182081,#182082,#182083,#182084,#182085,#182086,#182087,#182088,
#182089,#182090,#182091,#182092,#182093,#182094,#182095,#182096,#182097,
#182098,#182099,#182100,#182101,#182102,#182103,#182104,#182105,#182106,
#182107,#182108,#182109,#182110,#182111,#182112,#182113,#182114,#182115,
#182116,#182117),.UNSPECIFIED.,.F.,.F.,(4,3,3,3,3,3,3,3,3,3,3,3,3,3,3,3,
3,3,3,3,3,3,3,4),(2.30429796095351E-13,0.0653635991916027,0.124999999999902,
0.172311751454373,0.201820164413576,0.204919298358608,0.218749999999829,
0.230991507982218,0.243867579297171,0.249999999999807,0.312499999999765,
0.374999999999722,0.435313808412958,0.437499999999674,0.468749999999655,
0.484374999999648,0.493599726240859,0.49999999999964,0.591487052058411,
0.685705265585678,0.714514960993195,0.818813520304589,0.926648756273366,
1.),.UNSPECIFIED.);
#5304=B_SPLINE_CURVE_WITH_KNOTS('',3,(#182118,#182119,#182120,#182121,#182122,
#182123,#182124,#182125,#182126,#182127,#182128,#182129,#182130,#182131,
#182132,#182133,#182134,#182135,#182136,#182137,#182138,#182139,#182140,
#182141,#182142,#182143,#182144,#182145),.UNSPECIFIED.,.F.,.F.,(4,3,3,3,
3,3,3,3,3,4),(0.,0.000434392388669906,0.000626649590030441,0.000901221465792679,
0.00106184511664208,0.00112652683224085,0.00125380565733158,0.00135183219868902,
0.00158807055660732,0.00180244293158536),.UNSPECIFIED.);
#5305=B_SPLINE_CURVE_WITH_KNOTS('',3,(#182172,#182173,#182174,#182175,#182176,
#182177,#182178,#182179,#182180,#182181,#182182,#182183,#182184,#182185,
#182186,#182187,#182188,#182189,#182190,#182191,#182192,#182193,#182194,
#182195,#182196,#182197,#182198,#182199,#182200,#182201,#182202,#182203,
#182204,#182205,#182206,#182207,#182208),.UNSPECIFIED.,.F.,.F.,(4,3,3,3,
3,3,3,3,3,3,3,3,4),(0.000646102271928282,0.000780355288939433,0.000794331971528649,
0.00113223030152275,0.00115328378670241,0.00123902107032975,0.00152620034295103,
0.00183193986873122,0.00189906794388761,0.00227197283133227,0.00242485866713269,
0.00272131806633342,0.00301777746553416),.UNSPECIFIED.);
#5306=B_SPLINE_CURVE_WITH_KNOTS('',3,(#182267,#182268,#182269,#182270,#182271,
#182272,#182273,#182274,#182275,#182276,#182277,#182278,#182279,#182280,
#182281,#182282,#182283,#182284,#182285,#182286,#182287,#182288,#182289,
#182290,#182291,#182292,#182293,#182294,#182295,#182296,#182297,#182298,
#182299,#182300,#182301,#182302,#182303,#182304,#182305,#182306,#182307,
#182308,#182309,#182310,#182311,#182312,#182313,#182314,#182315,#182316,
#182317,#182318,#182319,#182320,#182321,#182322,#182323,#182324,#182325,
#182326,#182327,#182328,#182329,#182330,#182331,#182332,#182333,#182334,
#182335,#182336,#182337,#182338,#182339,#182340,#182341,#182342),
 .UNSPECIFIED.,.F.,.F.,(4,3,3,3,3,3,3,3,3,3,3,3,3,3,3,3,3,3,3,3,3,3,3,3,
3,4),(0.,0.0747149608966636,0.149327349717458,0.224017940702021,0.249999999999885,
0.267379393754175,0.368064696876988,0.403285137580062,0.468749999999801,
0.484374999999806,0.494437622037064,0.499999999999811,0.542078850476596,
0.617551256841197,0.624999999999861,0.661231284595247,0.715848897344134,
0.718749999999887,0.734374999999892,0.748641071841499,0.749999999999896,
0.778559801946971,0.844934573565376,0.910167849387285,0.973985577236299,
1.),.UNSPECIFIED.);
#5307=B_SPLINE_CURVE_WITH_KNOTS('',3,(#182343,#182344,#182345,#182346,#182347,
#182348,#182349,#182350,#182351,#182352,#182353,#182354,#182355,#182356,
#182357,#182358,#182359,#182360,#182361,#182362,#182363,#182364,#182365,
#182366,#182367,#182368,#182369,#182370,#182371,#182372),.UNSPECIFIED.,
 .F.,.F.,(4,2,2,2,1,1,1,2,2,2,2,1,1,1,2,2,2,4),(0.,0.124999999999883,0.187499999999825,
0.218749999999798,0.234374999999784,0.242187499999776,0.246093749999774,
0.248046874999774,0.249999999999774,0.374999999999773,0.43749999999977,
0.468749999999767,0.484374999999767,0.492187499999767,0.496093749999768,
0.499999999999768,0.749999999999884,1.),.UNSPECIFIED.);
#5308=B_SPLINE_CURVE_WITH_KNOTS('',3,(#182387,#182388,#182389,#182390,#182391,
#182392,#182393,#182394,#182395,#182396,#182397,#182398,#182399,#182400,
#182401,#182402,#182403,#182404,#182405,#182406,#182407,#182408,#182409,
#182410,#182411,#182412,#182413,#182414,#182415,#182416,#182417,#182418),
 .UNSPECIFIED.,.F.,.F.,(4,2,2,2,1,1,1,2,2,2,2,2,1,1,1,2,2,2,4),(0.,0.249999999999888,
0.374999999999834,0.437499999999805,0.468749999999789,0.484374999999781,
0.492187499999776,0.496093749999774,0.499999999999773,0.624999999999617,
0.687499999999539,0.718749999999501,0.734374999999485,0.742187499999479,
0.746093749999476,0.748046874999477,0.749999999999478,0.874999999999739,
1.),.UNSPECIFIED.);
#5309=B_SPLINE_CURVE_WITH_KNOTS('',3,(#182462,#182463,#182464,#182465,#182466,
#182467,#182468,#182469,#182470,#182471,#182472,#182473,#182474,#182475,
#182476,#182477,#182478,#182479,#182480,#182481,#182482,#182483,#182484,
#182485,#182486,#182487,#182488,#182489,#182490,#182491,#182492,#182493,
#182494,#182495,#182496,#182497,#182498,#182499,#182500,#182501,#182502,
#182503,#182504,#182505,#182506,#182507,#182508,#182509,#182510,#182511,
#182512,#182513,#182514,#182515,#182516,#182517,#182518,#182519,#182520,
#182521,#182522,#182523,#182524,#182525),.UNSPECIFIED.,.F.,.F.,(4,3,3,3,
3,3,3,3,3,3,3,3,3,3,3,3,3,3,3,3,3,4),(6.93365572599307E-10,0.0799018607364408,
0.124999999999984,0.16590247381775,0.206515416690505,0.23522651337888,0.249999999999967,
0.308568145931547,0.367273300160574,0.425754288427686,0.470393849025489,
0.499999999999945,0.60399947981351,0.624999999999934,0.687499999999939,
0.711940888291548,0.72132830679594,0.746951441711128,0.749999999999944,
0.863504722177636,0.982906462376687,1.),.UNSPECIFIED.);
#5310=B_SPLINE_CURVE_WITH_KNOTS('',3,(#182526,#182527,#182528,#182529,#182530,
#182531,#182532,#182533,#182534,#182535,#182536,#182537,#182538,#182539,
#182540,#182541,#182542,#182543,#182544,#182545,#182546,#182547,#182548,
#182549,#182550,#182551,#182552,#182553,#182554,#182555,#182556,#182557,
#182558,#182559,#182560,#182561,#182562,#182563,#182564,#182565,#182566,
#182567,#182568,#182569,#182570,#182571,#182572,#182573,#182574,#182575,
#182576,#182577),.UNSPECIFIED.,.F.,.F.,(4,3,3,3,3,3,3,3,3,3,3,3,3,3,3,3,
3,4),(0.,0.000568167570453903,0.000689873068221808,0.000757350079825042,
0.000945020241885804,0.00103480960233271,0.0011360777163446,0.00136729697222071,
0.00137974613644361,0.00151477367390368,0.00189346791975904,0.0020696192046654,
0.00221265318266025,0.00227165379781724,0.00237143867201243,0.00256546547244981,
0.0026624788726685,0.00275949227288719),.UNSPECIFIED.);
#5311=B_SPLINE_CURVE_WITH_KNOTS('',3,(#182622,#182623,#182624,#182625,#182626,
#182627,#182628,#182629,#182630,#182631,#182632,#182633,#182634,#182635,
#182636,#182637,#182638,#182639,#182640,#182641,#182642,#182643,#182644,
#182645,#182646,#182647,#182648,#182649,#182650,#182651,#182652,#182653,
#182654,#182655,#182656,#182657,#182658,#182659,#182660,#182661,#182662,
#182663,#182664,#182665,#182666,#182667,#182668,#182669,#182670),
 .UNSPECIFIED.,.F.,.F.,(4,3,3,3,3,3,3,3,3,3,3,3,3,3,3,3,4),(0.,0.0948667215790916,
0.188589440506681,0.28179472025342,0.37500000000016,0.437500000000192,0.468750000000196,
0.484375000000191,0.493434737105491,0.500000000000186,0.580918025814847,
0.659023039321664,0.734520568710628,0.806482846270357,0.876608217979102,
0.944078406641015,1.),.UNSPECIFIED.);
#5312=B_SPLINE_CURVE_WITH_KNOTS('',3,(#182678,#182679,#182680,#182681,#182682,
#182683,#182684,#182685,#182686,#182687,#182688,#182689,#182690,#182691,
#182692,#182693,#182694,#182695,#182696,#182697,#182698,#182699,#182700,
#182701,#182702,#182703,#182704,#182705,#182706,#182707,#182708,#182709,
#182710,#182711,#182712,#182713,#182714,#182715,#182716,#182717,#182718,
#182719,#182720,#182721,#182722,#182723,#182724,#182725,#182726,#182727,
#182728,#182729,#182730,#182731,#182732,#182733,#182734,#182735,#182736,
#182737,#182738,#182739,#182740,#182741,#182742,#182743,#182744,#182745,
#182746,#182747,#182748,#182749,#182750,#182751,#182752,#182753),
 .UNSPECIFIED.,.F.,.F.,(4,3,3,3,3,3,3,3,3,3,3,3,3,3,3,3,3,3,3,3,3,3,3,3,
3,4),(0.,0.0421877665880278,0.0918529461680548,0.121595727119581,0.156341218045798,
0.187500000000267,0.2187500000003,0.234375000000331,0.242187500000325,0.246093750000323,
0.25000000000032,0.259656373146243,0.33431792746277,0.375000000000227,0.437500000000185,
0.48437500000018,0.494310480798385,0.500000000000185,0.515232119733451,
0.593015658117578,0.675285422265481,0.712991994452306,0.801479119446512,
0.856495997226153,0.935184420368532,1.),.UNSPECIFIED.);
#5313=B_SPLINE_CURVE_WITH_KNOTS('',3,(#182792,#182793,#182794,#182795,#182796,
#182797,#182798,#182799,#182800,#182801,#182802,#182803,#182804),
 .UNSPECIFIED.,.F.,.F.,(4,3,3,3,4),(0.,0.304005884126683,0.606187253193727,
0.905860933135587,1.),.UNSPECIFIED.);
#5314=B_SPLINE_CURVE_WITH_KNOTS('',3,(#182811,#182812,#182813,#182814,#182815,
#182816,#182817,#182818,#182819,#182820,#182821,#182822,#182823,#182824,
#182825,#182826,#182827,#182828,#182829,#182830,#182831,#182832,#182833,
#182834,#182835,#182836,#182837,#182838,#182839,#182840,#182841,#182842,
#182843,#182844,#182845,#182846,#182847,#182848,#182849,#182850,#182851,
#182852,#182853),.UNSPECIFIED.,.F.,.F.,(4,3,3,3,3,3,3,3,3,3,3,3,3,3,4),
(0.,0.114160776840688,0.232043703654348,0.249999999999881,0.374999999999845,
0.437499999999821,0.468749999999809,0.47471823218372,0.489504435425131,
0.499999999999797,0.613342917066077,0.721572740801358,0.827582465287451,
0.930897765172478,1.),.UNSPECIFIED.);
#5315=B_SPLINE_CURVE_WITH_KNOTS('',3,(#182855,#182856,#182857,#182858),
 .UNSPECIFIED.,.F.,.F.,(4,4),(0.,1.),.UNSPECIFIED.);
#5316=B_SPLINE_CURVE_WITH_KNOTS('',3,(#182866,#182867,#182868,#182869,#182870,
#182871,#182872,#182873,#182874,#182875,#182876,#182877,#182878),
 .UNSPECIFIED.,.F.,.F.,(4,3,3,3,4),(0.,0.25,0.496827497839013,0.750275035845233,
1.),.UNSPECIFIED.);
#5317=B_SPLINE_CURVE_WITH_KNOTS('',3,(#182884,#182885,#182886,#182887,#182888,
#182889,#182890,#182891,#182892,#182893,#182894,#182895,#182896,#182897,
#182898,#182899,#182900,#182901,#182902,#182903,#182904,#182905,#182906,
#182907,#182908,#182909,#182910,#182911,#182912,#182913,#182914,#182915,
#182916,#182917),.UNSPECIFIED.,.F.,.F.,(4,3,3,3,3,3,3,3,3,3,3,4),(0.,0.106653491061592,
0.219036071567704,0.250000000000003,0.334704087655355,0.420584442640105,
0.486614479419915,0.500000000000006,0.660932422463628,0.818357566951526,
0.966974096514476,1.),.UNSPECIFIED.);
#5318=B_SPLINE_CURVE_WITH_KNOTS('',3,(#182925,#182926,#182927,#182928),
 .UNSPECIFIED.,.F.,.F.,(4,4),(0.,6.88517764864569E-5),.UNSPECIFIED.);
#5319=B_SPLINE_CURVE_WITH_KNOTS('',3,(#182929,#182930,#182931,#182932,#182933,
#182934,#182935,#182936,#182937,#182938,#182939,#182940,#182941,#182942,
#182943,#182944,#182945,#182946,#182947,#182948,#182949,#182950,#182951,
#182952,#182953,#182954,#182955,#182956,#182957,#182958,#182959,#182960,
#182961,#182962,#182963,#182964,#182965,#182966,#182967,#182968,#182969,
#182970,#182971,#182972,#182973,#182974,#182975,#182976,#182977),
 .UNSPECIFIED.,.F.,.F.,(4,3,3,3,3,3,3,3,3,3,3,3,3,3,3,3,4),(0.,0.0789809457866306,
0.161285417776234,0.245599696437801,0.333230417767524,0.37499999999985,
0.437499999999833,0.46874999999983,0.484374999999829,0.49397464410552,0.499999999999828,
0.591682610550623,0.684555700018607,0.779305938640673,0.875152751961459,
0.972664363097949,1.),.UNSPECIFIED.);
#5320=B_SPLINE_CURVE_WITH_KNOTS('',3,(#182984,#182985,#182986,#182987,#182988,
#182989,#182990,#182991,#182992,#182993,#182994,#182995,#182996,#182997,
#182998,#182999,#183000,#183001,#183002,#183003,#183004,#183005,#183006,
#183007,#183008,#183009,#183010,#183011),.UNSPECIFIED.,.F.,.F.,(4,3,3,3,
3,3,3,3,3,4),(0.000712605368931889,0.000926461878734654,0.00114426125513561,
0.00117428487373109,0.00139094819074976,0.00157723429047313,0.00180778147057016,
0.00209481686703422,0.00237995362541951,0.00244186321201438),
 .UNSPECIFIED.);
#5321=B_SPLINE_CURVE_WITH_KNOTS('',3,(#183015,#183016,#183017,#183018,#183019,
#183020),.UNSPECIFIED.,.F.,.F.,(4,2,4),(0.,0.000500369188755688,0.00100073837751138),
 .UNSPECIFIED.);
#5322=B_SPLINE_CURVE_WITH_KNOTS('',3,(#183021,#183022,#183023,#183024),
 .UNSPECIFIED.,.F.,.F.,(4,4),(0.,0.0331958858056162),.UNSPECIFIED.);
#5323=B_SPLINE_CURVE_WITH_KNOTS('',3,(#183056,#183057,#183058,#183059,#183060,
#183061,#183062,#183063,#183064,#183065,#183066,#183067,#183068,#183069,
#183070,#183071,#183072,#183073,#183074,#183075,#183076,#183077,#183078,
#183079,#183080,#183081,#183082,#183083,#183084,#183085,#183086,#183087,
#183088,#183089,#183090,#183091,#183092,#183093,#183094,#183095,#183096,
#183097,#183098,#183099,#183100,#183101,#183102,#183103,#183104,#183105,
#183106,#183107,#183108,#183109,#183110,#183111,#183112,#183113,#183114,
#183115,#183116,#183117,#183118,#183119,#183120,#183121,#183122,#183123,
#183124,#183125),.UNSPECIFIED.,.F.,.F.,(4,3,3,3,3,3,3,3,3,3,3,3,3,3,3,3,
3,3,3,3,3,3,3,4),(0.,0.102857470141467,0.125000000000026,0.220263138689686,
0.250000000000052,0.284634156633098,0.375000000000079,0.4375000000001,0.468750000000111,
0.484375000000114,0.493913132672327,0.500000000000116,0.563704176814045,
0.62500000000009,0.682712478891769,0.699894434445292,0.734375000000072,
0.743077120945512,0.750000000000067,0.794106423027594,0.849243360995836,
0.903603919149664,0.957011397681897,0.999999993037464),.UNSPECIFIED.);
#5324=B_SPLINE_CURVE_WITH_KNOTS('',3,(#183126,#183127,#183128,#183129,#183130,
#183131,#183132,#183133,#183134,#183135,#183136,#183137,#183138,#183139,
#183140,#183141,#183142,#183143,#183144,#183145,#183146,#183147,#183148,
#183149,#183150,#183151,#183152,#183153,#183154,#183155,#183156,#183157,
#183158,#183159,#183160,#183161,#183162,#183163,#183164,#183165,#183166,
#183167,#183168,#183169,#183170,#183171,#183172,#183173,#183174,#183175,
#183176,#183177,#183178,#183179,#183180,#183181,#183182,#183183,#183184,
#183185,#183186,#183187,#183188,#183189,#183190,#183191,#183192,#183193,
#183194,#183195,#183196,#183197,#183198,#183199,#183200,#183201,#183202,
#183203,#183204,#183205,#183206,#183207,#183208,#183209,#183210),
 .UNSPECIFIED.,.F.,.F.,(4,3,3,3,3,3,3,3,3,3,3,3,3,3,3,3,3,3,3,3,3,3,3,3,
3,3,3,3,4),(0.,0.0312894328292875,0.0622354553383098,0.0936177276691337,
0.124999999999958,0.156249999999947,0.187499999999937,0.194792789675713,
0.202551490020127,0.203124999999931,0.218749999999926,0.242527406522679,
0.282862122212415,0.329320663124785,0.380198846483021,0.431355268401253,
0.485129013232248,0.496093749999816,0.499999999999818,0.502687086598598,
0.566609075637323,0.632182148458018,0.70053635082894,0.740544135088561,
0.749999999999909,0.823221108105435,0.897670430593762,0.974675815205079,
0.999999999970395),.UNSPECIFIED.);
#5325=B_SPLINE_CURVE_WITH_KNOTS('',3,(#183225,#183226,#183227,#183228,#183229,
#183230,#183231,#183232,#183233,#183234,#183235,#183236,#183237,#183238,
#183239,#183240,#183241,#183242,#183243,#183244,#183245,#183246,#183247,
#183248,#183249,#183250,#183251,#183252,#183253,#183254,#183255,#183256,
#183257,#183258,#183259,#183260,#183261,#183262,#183263,#183264,#183265,
#183266,#183267,#183268,#183269,#183270,#183271,#183272,#183273,#183274,
#183275,#183276,#183277,#183278,#183279,#183280,#183281,#183282,#183283,
#183284,#183285,#183286,#183287,#183288,#183289,#183290,#183291,#183292,
#183293,#183294,#183295,#183296,#183297,#183298,#183299,#183300,#183301,
#183302,#183303,#183304,#183305,#183306,#183307,#183308,#183309,#183310,
#183311,#183312,#183313,#183314,#183315,#183316,#183317,#183318),
 .UNSPECIFIED.,.F.,.F.,(4,3,3,3,3,3,3,3,3,3,3,3,3,3,3,3,3,3,3,3,3,3,3,3,
3,3,3,3,3,3,3,4),(0.,0.07198248742987,0.142766259275923,0.211951276696239,
0.250000000000095,0.317389348407017,0.383564948093474,0.437500000000164,
0.468750000000174,0.484375000000181,0.492187500000187,0.496093750000192,
0.49978162785641,0.500000000000198,0.553158315085203,0.604461352990886,
0.654731630643987,0.703470233159367,0.750000000000084,0.781250000000072,
0.78515625000007,0.788461425907795,0.789062500000069,0.796875000000065,
0.812500000000058,0.840059259163279,0.86829920100936,0.89716635807548,0.926821656402351,
0.956825743880503,0.987204115019961,1.),.UNSPECIFIED.);
#5326=B_SPLINE_CURVE_WITH_KNOTS('',3,(#183356,#183357,#183358,#183359,#183360,
#183361,#183362,#183363,#183364,#183365,#183366,#183367,#183368,#183369,
#183370,#183371,#183372,#183373,#183374,#183375,#183376,#183377,#183378,
#183379,#183380,#183381,#183382,#183383,#183384,#183385,#183386,#183387,
#183388,#183389,#183390,#183391,#183392,#183393,#183394,#183395,#183396,
#183397,#183398,#183399,#183400,#183401,#183402,#183403,#183404,#183405,
#183406,#183407,#183408,#183409,#183410,#183411,#183412,#183413,#183414,
#183415,#183416,#183417,#183418,#183419,#183420,#183421,#183422,#183423,
#183424,#183425),.UNSPECIFIED.,.F.,.F.,(4,3,3,3,3,3,3,3,3,3,3,3,3,3,3,3,
3,3,3,3,3,3,3,4),(3.27359973213996E-13,0.0857365026607216,0.124999999999915,
0.174375612862638,0.204585644336071,0.209083762348739,0.218749999999854,
0.232924773331302,0.247673015334756,0.249999999999833,0.312499999999785,
0.374999999999736,0.437499999999679,0.43884535386112,0.468749999999659,
0.484374999999656,0.493704288796288,0.499999999999654,0.59264919846013,
0.688070810914995,0.716212286393592,0.820643696798982,0.928592372305829,
0.999996088506396),.UNSPECIFIED.);
#5327=B_SPLINE_CURVE_WITH_KNOTS('',3,(#183426,#183427,#183428,#183429,#183430,
#183431,#183432,#183433,#183434,#183435,#183436,#183437,#183438,#183439,
#183440,#183441,#183442,#183443,#183444,#183445,#183446,#183447,#183448,
#183449,#183450,#183451,#183452,#183453,#183454,#183455,#183456),
 .UNSPECIFIED.,.F.,.F.,(4,3,3,3,3,3,3,3,3,3,4),(0.,0.000497569400086742,
0.000640953038946957,0.0009614312638914,0.000995138800173484,0.00128203532234786,
0.00149270820026023,0.00161710055028191,0.00180479162331784,0.00192302626316565,
0.00199027760034697),.UNSPECIFIED.);
#5328=B_SPLINE_CURVE_WITH_KNOTS('',3,(#183485,#183486,#183487,#183488,#183489,
#183490,#183491,#183492,#183493,#183494,#183495,#183496,#183497,#183498,
#183499,#183500,#183501,#183502,#183503,#183504,#183505,#183506,#183507,
#183508,#183509,#183510,#183511,#183512,#183513,#183514,#183515,#183516,
#183517,#183518,#183519,#183520,#183521,#183522,#183523,#183524,#183525,
#183526,#183527,#183528,#183529,#183530,#183531,#183532,#183533,#183534,
#183535,#183536,#183537,#183538,#183539,#183540,#183541,#183542,#183543,
#183544,#183545),.UNSPECIFIED.,.F.,.F.,(4,3,3,3,3,3,3,3,3,3,3,3,3,3,3,3,
3,3,3,3,4),(0.000632518815593833,0.000932214526658406,0.00101585454476649,
0.00107182189614633,0.00126737972551708,0.00139919027393915,0.00150973846725992,
0.00175129113716496,0.0017825260031118,0.00194741404639007,0.00209785990015683,
0.00215891919182298,0.00222254437896024,0.00246825757121381,0.00254919746145711,
0.00271487168756702,0.0028230834495401,0.00293253319062976,0.00318749230619698,
0.00344334847758602,0.00369920464897506),.UNSPECIFIED.);
#5329=B_SPLINE_CURVE_WITH_KNOTS('',3,(#183599,#183600,#183601,#183602,#183603,
#183604,#183605,#183606,#183607,#183608,#183609,#183610,#183611,#183612,
#183613,#183614,#183615,#183616,#183617,#183618,#183619,#183620,#183621,
#183622,#183623,#183624,#183625,#183626,#183627,#183628,#183629,#183630,
#183631,#183632,#183633,#183634,#183635,#183636,#183637,#183638,#183639,
#183640,#183641,#183642,#183643,#183644,#183645,#183646,#183647,#183648,
#183649,#183650,#183651,#183652,#183653,#183654,#183655,#183656,#183657,
#183658,#183659,#183660,#183661,#183662,#183663,#183664,#183665,#183666,
#183667,#183668,#183669,#183670,#183671,#183672,#183673,#183674,#183675,
#183676,#183677,#183678,#183679,#183680),.UNSPECIFIED.,.F.,.F.,(4,3,3,3,
3,3,3,3,3,3,3,3,3,3,3,3,3,3,3,3,3,3,3,3,3,3,3,4),(0.,0.0347059239069192,
0.0702944863998228,0.107079974258399,0.125000000000524,0.162191772866572,
0.187500000000781,0.218750000000929,0.234375000001002,0.242187500000992,
0.249424935941155,0.250000000000981,0.301248065768145,0.352433147510947,
0.375000000000836,0.437500000000757,0.468750000000713,0.484375000000691,
0.498608696187955,0.50000000000067,0.569611194950186,0.639357942877805,
0.709783596290922,0.750000000000335,0.822081078895063,0.895102993899266,
0.969950340120507,1.),.UNSPECIFIED.);
#5330=B_SPLINE_CURVE_WITH_KNOTS('',3,(#183681,#183682,#183683,#183684,#183685,
#183686,#183687,#183688,#183689,#183690,#183691,#183692,#183693,#183694,
#183695,#183696,#183697,#183698,#183699,#183700,#183701,#183702,#183703,
#183704,#183705,#183706,#183707,#183708,#183709,#183710,#183711,#183712,
#183713,#183714,#183715,#183716,#183717,#183718,#183719,#183720,#183721,
#183722,#183723,#183724,#183725,#183726,#183727,#183728,#183729,#183730,
#183731,#183732,#183733,#183734,#183735,#183736,#183737,#183738,#183739,
#183740,#183741,#183742,#183743,#183744,#183745,#183746,#183747,#183748,
#183749,#183750,#183751,#183752,#183753,#183754,#183755,#183756,#183757,
#183758,#183759,#183760,#183761,#183762,#183763,#183764,#183765,#183766,
#183767,#183768),.UNSPECIFIED.,.F.,.F.,(4,3,3,3,3,3,3,3,3,3,3,3,3,3,3,3,
3,3,3,3,3,3,3,3,3,3,3,3,3,4),(0.,0.0551115055721159,0.108953779567591,0.162273305591977,
0.21144363860674,0.236028805114121,0.248602245718417,0.256548955259473,
0.260613971621503,0.318507353716111,0.361927390287068,0.376413794214911,
0.423796678888208,0.471178079428924,0.492187499999938,0.497822391426295,
0.499999999999937,0.503298936899024,0.556038805749608,0.608145796234962,
0.635679690970773,0.685905062891556,0.737189132830948,0.749999999999968,
0.761847144546501,0.808861184933272,0.856645888699954,0.902952577790402,
0.951476288895201,1.),.UNSPECIFIED.);
#5331=B_SPLINE_CURVE_WITH_KNOTS('',3,(#183783,#183784,#183785,#183786,#183787,
#183788,#183789,#183790,#183791,#183792,#183793,#183794,#183795,#183796,
#183797,#183798,#183799,#183800,#183801,#183802,#183803,#183804,#183805,
#183806,#183807,#183808,#183809,#183810,#183811,#183812,#183813,#183814,
#183815,#183816,#183817,#183818,#183819,#183820,#183821,#183822,#183823,
#183824,#183825,#183826,#183827,#183828,#183829,#183830,#183831,#183832,
#183833,#183834,#183835,#183836,#183837,#183838,#183839,#183840,#183841,
#183842,#183843,#183844,#183845,#183846,#183847,#183848,#183849,#183850,
#183851,#183852,#183853,#183854,#183855,#183856,#183857,#183858,#183859,
#183860,#183861,#183862,#183863,#183864),.UNSPECIFIED.,.F.,.F.,(4,3,3,3,
3,3,3,3,3,3,3,3,3,3,3,3,3,3,3,3,3,3,3,3,3,3,3,4),(1.34985451482093E-13,
0.056751333121689,0.111716230590216,0.165601173577879,0.217745992585657,
0.250000000000001,0.300400507324752,0.350801014649504,0.389142445556312,
0.426377110084194,0.462057538976088,0.488683010340457,0.500000000000003,
0.54693009782314,0.591723632592143,0.606245868675057,0.625000000000002,
0.660743347771245,0.696577628491914,0.712544338223846,0.750000000000001,
0.811350030058359,0.866771747342932,0.875000000000001,0.911268783979688,
0.947507821305827,0.983698341291556,1.),.UNSPECIFIED.);
#5332=B_SPLINE_CURVE_WITH_KNOTS('',3,(#183908,#183909,#183910,#183911,#183912,
#183913,#183914,#183915,#183916,#183917,#183918,#183919,#183920,#183921,
#183922,#183923,#183924,#183925,#183926,#183927,#183928,#183929,#183930,
#183931,#183932,#183933,#183934,#183935,#183936,#183937,#183938,#183939,
#183940,#183941,#183942,#183943,#183944,#183945,#183946,#183947,#183948,
#183949,#183950,#183951,#183952,#183953,#183954,#183955,#183956,#183957,
#183958,#183959,#183960,#183961,#183962,#183963,#183964,#183965,#183966,
#183967,#183968,#183969,#183970,#183971),.UNSPECIFIED.,.F.,.F.,(4,3,3,3,
3,3,3,3,3,3,3,3,3,3,3,3,3,3,3,3,3,4),(8.59038016877541E-10,0.0733303750771787,
0.125000000000027,0.190074946227628,0.22888061590917,0.294022873922094,
0.36021312493933,0.430448645641966,0.484375000000101,0.493741968173762,
0.500000000000104,0.504812740617916,0.587025088775253,0.625000000000078,
0.681677197130213,0.715381499528901,0.736543530082876,0.766480294100765,
0.838951501085421,0.875000000000026,0.954886761461704,1.),.UNSPECIFIED.);
#5333=B_SPLINE_CURVE_WITH_KNOTS('',3,(#183972,#183973,#183974,#183975,#183976,
#183977,#183978,#183979,#183980,#183981,#183982,#183983,#183984,#183985,
#183986,#183987,#183988,#183989,#183990,#183991,#183992,#183993,#183994,
#183995,#183996,#183997,#183998,#183999,#184000,#184001,#184002,#184003,
#184004,#184005,#184006,#184007,#184008,#184009,#184010,#184011,#184012,
#184013,#184014,#184015,#184016,#184017,#184018,#184019,#184020,#184021,
#184022,#184023,#184024,#184025,#184026,#184027,#184028,#184029,#184030,
#184031,#184032,#184033,#184034,#184035),.UNSPECIFIED.,.F.,.F.,(4,3,3,3,
3,3,3,3,3,3,3,3,3,3,3,3,3,3,3,3,3,4),(0.,0.000243943071869819,0.000489165049879495,
0.000733924827046607,0.000899069239743237,0.000911316177023075,0.00119563029973622,
0.00134860385961487,0.00136698289390588,0.00175854423317811,0.0017981384794865,
0.00182264071786974,0.00224767309935813,0.00227830273883051,0.00257044019241884,
0.00269720771922976,0.002733987473331,0.00295810023175296,0.0031467423391014,
0.00331012937356572,0.00347290261708232,0.00359627695897302),
 .UNSPECIFIED.);
#5334=B_SPLINE_CURVE_WITH_KNOTS('',3,(#184082,#184083,#184084,#184085,#184086,
#184087,#184088,#184089,#184090,#184091,#184092,#184093,#184094,#184095,
#184096,#184097,#184098,#184099,#184100,#184101,#184102,#184103,#184104,
#184105,#184106,#184107,#184108,#184109,#184110,#184111,#184112,#184113,
#184114,#184115,#184116,#184117,#184118,#184119,#184120,#184121,#184122,
#184123,#184124,#184125,#184126,#184127,#184128,#184129,#184130,#184131,
#184132,#184133,#184134,#184135,#184136,#184137,#184138,#184139,#184140,
#184141,#184142,#184143,#184144,#184145,#184146,#184147,#184148,#184149,
#184150,#184151,#184152,#184153,#184154,#184155,#184156,#184157,#184158,
#184159,#184160,#184161,#184162,#184163),.UNSPECIFIED.,.F.,.F.,(4,3,3,3,
3,3,3,3,3,3,3,3,3,3,3,3,3,3,3,3,3,3,3,3,3,3,3,4),(0.,0.0863130095180163,
0.124999999999993,0.187499999999993,0.218749999999993,0.232144860506862,
0.247931741713982,0.249999999999992,0.333313232249592,0.37499999999993,
0.437499999999906,0.468749999999902,0.476693585153444,0.491282462856874,
0.499999999999898,0.57747845846861,0.624999999999936,0.68749999999994,0.718749999999944,
0.734374999999939,0.735025645679648,0.744357247627351,0.749999999999935,
0.812499999999951,0.87138267660412,0.927432801000241,0.979960253731857,
1.),.UNSPECIFIED.);
#5335=B_SPLINE_CURVE_WITH_KNOTS('',3,(#184171,#184172,#184173,#184174,#184175,
#184176,#184177,#184178,#184179,#184180,#184181,#184182,#184183,#184184,
#184185,#184186),.UNSPECIFIED.,.F.,.F.,(4,2,2,2,1,1,2,2,4),(0.,0.249999999999856,
0.374999999999799,0.437499999999791,0.468749999999786,0.484374999999784,
0.492187499999798,0.499999999999811,1.),.UNSPECIFIED.);
#5336=B_SPLINE_CURVE_WITH_KNOTS('',3,(#184207,#184208,#184209,#184210,#184211,
#184212,#184213,#184214,#184215,#184216,#184217,#184218,#184219,#184220,
#184221,#184222),.UNSPECIFIED.,.F.,.F.,(4,3,3,3,3,4),(0.,0.228004650890224,
0.457585570846926,0.688183484414605,0.920419006980701,1.),.UNSPECIFIED.);
#5337=B_SPLINE_CURVE_WITH_KNOTS('',3,(#184227,#184228,#184229,#184230,#184231,
#184232,#184233,#184234,#184235,#184236,#184237,#184238,#184239,#184240,
#184241,#184242,#184243,#184244,#184245,#184246,#184247,#184248,#184249,
#184250,#184251,#184252,#184253,#184254,#184255,#184256,#184257,#184258,
#184259,#184260),.UNSPECIFIED.,.F.,.F.,(4,3,3,3,3,3,3,3,3,3,3,4),(0.,0.137126090839981,
0.258934713814541,0.410851602161014,0.468750000000055,0.490339286585085,
0.500000000000056,0.513599342481747,0.6455154402161,0.774520962955583,0.899340216824067,
1.),.UNSPECIFIED.);
#5338=B_SPLINE_CURVE_WITH_KNOTS('',3,(#184261,#184262,#184263,#184264,#184265,
#184266,#184267,#184268,#184269,#184270,#184271,#184272,#184273,#184274,
#184275,#184276,#184277,#184278,#184279,#184280,#184281,#184282,#184283,
#184284,#184285,#184286,#184287,#184288,#184289,#184290,#184291),
 .UNSPECIFIED.,.F.,.F.,(4,3,3,3,3,3,3,3,3,3,4),(0.,0.0729993287143241,0.1205082445585,
0.219240574404831,0.349365992062872,0.499876044794966,0.502870118528192,
0.562504597086005,0.749896118500103,0.887412448086525,1.),.UNSPECIFIED.);
#5339=B_SPLINE_CURVE_WITH_KNOTS('',3,(#184296,#184297,#184298,#184299,#184300,
#184301,#184302,#184303,#184304,#184305,#184306,#184307,#184308,#184309,
#184310,#184311,#184312,#184313,#184314,#184315,#184316,#184317,#184318,
#184319,#184320,#184321,#184322,#184323,#184324,#184325,#184326,#184327,
#184328,#184329,#184330,#184331,#184332,#184333,#184334,#184335,#184336,
#184337,#184338,#184339,#184340,#184341,#184342,#184343,#184344,#184345,
#184346,#184347,#184348,#184349,#184350,#184351,#184352,#184353,#184354,
#184355,#184356,#184357,#184358,#184359,#184360,#184361,#184362,#184363,
#184364,#184365),.UNSPECIFIED.,.F.,.F.,(4,3,3,3,3,3,3,3,3,3,3,3,3,3,3,3,
3,3,3,3,3,3,3,4),(0.,0.0795438263529059,0.124999999999882,0.187499999999824,
0.218749999999794,0.231135975157282,0.249999999999765,0.342939196677063,
0.374999999999647,0.437499999999583,0.468749999999534,0.484374999999514,
0.492187499999508,0.498391551397716,0.499999999999502,0.527623760044591,
0.604845273664748,0.683741209693796,0.714465797142799,0.754800912699018,
0.84727383837472,0.8572328985714,0.930360007098205,1.),.UNSPECIFIED.);
#5340=B_SPLINE_CURVE_WITH_KNOTS('',3,(#184413,#184414,#184415,#184416,#184417,
#184418,#184419,#184420,#184421,#184422,#184423,#184424,#184425,#184426,
#184427,#184428,#184429,#184430),.UNSPECIFIED.,.F.,.F.,(4,2,2,2,1,1,2,2,
2,4),(0.,0.250000000000419,0.375000000000626,0.437500000000725,0.468750000000762,
0.484375000000761,0.492187500000745,0.500000000000729,0.750000000000364,
1.),.UNSPECIFIED.);
#5341=B_SPLINE_CURVE_WITH_KNOTS('',3,(#184438,#184439,#184440,#184441,#184442,
#184443,#184444,#184445,#184446,#184447,#184448,#184449,#184450,#184451,
#184452,#184453,#184454,#184455,#184456,#184457,#184458,#184459,#184460,
#184461,#184462,#184463,#184464,#184465,#184466,#184467,#184468,#184469,
#184470,#184471,#184472,#184473,#184474,#184475,#184476,#184477,#184478,
#184479,#184480,#184481,#184482,#184483,#184484,#184485,#184486,#184487,
#184488,#184489),.UNSPECIFIED.,.F.,.F.,(4,3,3,3,3,3,3,3,3,3,3,3,3,3,3,3,
3,4),(0.,0.0670799139916658,0.13599024748976,0.207907147469578,0.281702493042214,
0.358403426941099,0.374999999999999,0.437499999999991,0.468749999999991,
0.48437499999998,0.493917046584479,0.49999999999997,0.589612381791532,0.680360224688852,
0.772922373758745,0.866528534163224,0.961769826620013,1.),.UNSPECIFIED.);
#5342=B_SPLINE_CURVE_WITH_KNOTS('',3,(#184521,#184522,#184523,#184524,#184525,
#184526,#184527,#184528,#184529,#184530,#184531,#184532,#184533,#184534,
#184535,#184536,#184537,#184538,#184539,#184540,#184541,#184542,#184543,
#184544,#184545,#184546,#184547,#184548,#184549,#184550,#184551,#184552,
#184553,#184554,#184555,#184556,#184557,#184558,#184559,#184560,#184561,
#184562,#184563,#184564,#184565,#184566),.UNSPECIFIED.,.F.,.F.,(4,3,3,3,
3,3,3,3,3,3,3,3,3,3,3,4),(0.000450499470650019,0.00054011395429817,0.000798583304342707,
0.000986883024373894,0.00116741533983523,0.00137527276208874,0.00169825994125316,
0.00176385446568028,0.00188433120902044,0.00210726599696856,0.00224278914361301,
0.00241357708828738,0.00254109024997703,0.0026012470782056,0.00316630230572219,
0.00331816294739075),.UNSPECIFIED.);
#5343=B_SPLINE_CURVE_WITH_KNOTS('',3,(#184619,#184620,#184621,#184622,#184623,
#184624,#184625,#184626,#184627,#184628,#184629,#184630,#184631,#184632,
#184633,#184634,#184635,#184636,#184637,#184638,#184639,#184640,#184641,
#184642,#184643,#184644,#184645,#184646,#184647,#184648,#184649,#184650,
#184651,#184652,#184653,#184654,#184655,#184656,#184657,#184658,#184659,
#184660,#184661,#184662,#184663,#184664,#184665,#184666,#184667,#184668,
#184669,#184670,#184671,#184672,#184673,#184674,#184675,#184676,#184677,
#184678,#184679,#184680,#184681,#184682),.UNSPECIFIED.,.F.,.F.,(4,3,3,3,
3,3,3,3,3,3,3,3,3,3,3,3,3,3,3,3,3,4),(0.,0.0922518249521236,0.124999999999966,
0.187499999999968,0.21401656664708,0.239789942133961,0.24999999999997,0.275182709279866,
0.401192886020697,0.499999999999992,0.524820514521064,0.618210322834091,
0.624999999999993,0.662910196285119,0.700740355222286,0.739058341955884,
0.749999999999994,0.762750903735254,0.832354637129329,0.902472607068448,
0.972781141742723,0.999999847268213),.UNSPECIFIED.);
#5344=B_SPLINE_CURVE_WITH_KNOTS('',3,(#184683,#184684,#184685,#184686,#184687,
#184688,#184689,#184690,#184691,#184692,#184693,#184694,#184695,#184696,
#184697,#184698,#184699,#184700,#184701,#184702,#184703,#184704,#184705,
#184706,#184707,#184708,#184709,#184710,#184711,#184712,#184713,#184714,
#184715,#184716,#184717,#184718,#184719,#184720,#184721,#184722,#184723,
#184724,#184725,#184726,#184727,#184728,#184729,#184730,#184731,#184732,
#184733,#184734,#184735,#184736,#184737,#184738,#184739,#184740,#184741,
#184742,#184743,#184744,#184745,#184746,#184747,#184748,#184749,#184750,
#184751,#184752,#184753,#184754,#184755,#184756,#184757,#184758,#184759,
#184760,#184761,#184762,#184763,#184764),.UNSPECIFIED.,.F.,.F.,(4,3,3,3,
3,3,3,3,3,3,3,3,3,3,3,3,3,3,3,3,3,3,3,3,3,3,3,4),(0.,0.0569576591821558,
0.112755151148855,0.168107128830785,0.223066017844343,0.249999999999972,
0.260222583084969,0.335298290313108,0.374999999999957,0.431109645708327,
0.437499999999951,0.468749999999948,0.484374999999947,0.493293930533613,
0.499999999999946,0.507115891968341,0.561313062720312,0.611963343037344,
0.624999999999959,0.639766051419202,0.691395847196872,0.736848157965738,
0.761599820846938,0.766283550877083,0.84574998738632,0.922874993617906,
0.995168128022229,0.999999999849491),.UNSPECIFIED.);
#5345=B_SPLINE_CURVE_WITH_KNOTS('',3,(#184779,#184780,#184781,#184782,#184783,
#184784,#184785,#184786,#184787,#184788,#184789,#184790,#184791,#184792,
#184793,#184794,#184795,#184796,#184797,#184798,#184799,#184800,#184801,
#184802,#184803,#184804,#184805,#184806,#184807,#184808,#184809,#184810,
#184811,#184812,#184813,#184814,#184815,#184816,#184817,#184818,#184819,
#184820,#184821,#184822,#184823,#184824,#184825,#184826,#184827,#184828,
#184829,#184830,#184831,#184832,#184833,#184834,#184835,#184836,#184837,
#184838,#184839,#184840,#184841,#184842,#184843,#184844,#184845,#184846,
#184847,#184848,#184849,#184850,#184851,#184852,#184853,#184854,#184855,
#184856,#184857,#184858,#184859,#184860,#184861,#184862,#184863,#184864,
#184865,#184866),.UNSPECIFIED.,.F.,.F.,(4,3,3,3,3,3,3,3,3,3,3,3,3,3,3,3,
3,3,3,3,3,3,3,3,3,3,3,3,3,4),(4.79077677789156E-15,0.0625000000000102,0.119437937333093,
0.174434651404281,0.226856935996688,0.250000000000027,0.259607248156974,
0.31248276171328,0.346461802787087,0.369037373645423,0.380440843860894,
0.418757995092361,0.442888681175932,0.469986336276138,0.483535163826241,
0.485333141233566,0.495430448048758,0.497083991376344,0.50000000000005,
0.56320260393989,0.618434035218326,0.68012401263361,0.738312181743081,0.741813990048893,
0.750000000000025,0.805848380212432,0.862121697127147,0.918811408327095,
0.976432987956455,1.),.UNSPECIFIED.);
#5346=B_SPLINE_CURVE_WITH_KNOTS('',3,(#184910,#184911,#184912,#184913,#184914,
#184915,#184916,#184917,#184918,#184919,#184920,#184921,#184922,#184923,
#184924,#184925,#184926,#184927,#184928,#184929,#184930,#184931,#184932,
#184933,#184934,#184935,#184936,#184937,#184938,#184939,#184940,#184941,
#184942,#184943,#184944,#184945,#184946,#184947,#184948,#184949,#184950,
#184951,#184952,#184953,#184954,#184955,#184956,#184957,#184958,#184959,
#184960,#184961,#184962,#184963,#184964,#184965,#184966,#184967,#184968,
#184969,#184970,#184971,#184972,#184973),.UNSPECIFIED.,.F.,.F.,(4,3,3,3,
3,3,3,3,3,3,3,3,3,3,3,3,3,3,3,3,3,4),(0.,0.0691966740878807,0.125000000000041,
0.185982401655162,0.227879315918833,0.238353522132354,0.267545001222266,
0.342870914442811,0.407678156640436,0.452094475638223,0.463461622214131,
0.484375000000144,0.493645266144116,0.500000000000138,0.562500000000121,
0.649447035395343,0.713513413029987,0.736394070790565,0.750000000000069,
0.840743294607341,0.935248128666082,1.),.UNSPECIFIED.);
#5347=B_SPLINE_CURVE_WITH_KNOTS('',3,(#184974,#184975,#184976,#184977,#184978,
#184979,#184980,#184981,#184982,#184983,#184984,#184985,#184986,#184987,
#184988,#184989,#184990,#184991,#184992,#184993,#184994,#184995,#184996,
#184997,#184998,#184999,#185000,#185001,#185002,#185003,#185004,#185005,
#185006,#185007,#185008,#185009,#185010),.UNSPECIFIED.,.F.,.F.,(4,3,3,3,
3,3,3,3,3,3,3,3,4),(0.,0.000308449407263107,0.000616898814526214,0.000757033039934084,
0.00113555144207261,0.00123379762905243,0.00151396810348859,0.00181929544895182,
0.00185069644357864,0.00189260692917412,0.00221146178004545,0.00227133710209363,
0.00246759525810486),.UNSPECIFIED.);
#5348=B_SPLINE_CURVE_WITH_KNOTS('',3,(#185038,#185039,#185040,#185041,#185042,
#185043,#185044,#185045,#185046,#185047,#185048,#185049,#185050,#185051,
#185052,#185053,#185054,#185055,#185056,#185057,#185058,#185059,#185060,
#185061,#185062,#185063,#185064,#185065),.UNSPECIFIED.,.F.,.F.,(4,3,3,3,
3,3,3,3,3,4),(0.,0.000418680346171866,0.000626513004308685,0.000899330166364171,
0.00105990140469727,0.00112416270795522,0.00125349750883986,0.00134899524954626,
0.0015907151218419,0.00179866033272836),.UNSPECIFIED.);
#5349=B_SPLINE_CURVE_WITH_KNOTS('',3,(#185072,#185073,#185074,#185075,#185076,
#185077,#185078,#185079,#185080,#185081,#185082,#185083,#185084,#185085,
#185086,#185087,#185088,#185089,#185090,#185091,#185092,#185093,#185094,
#185095,#185096,#185097,#185098,#185099,#185100,#185101,#185102,#185103,
#185104,#185105,#185106,#185107,#185108),.UNSPECIFIED.,.F.,.F.,(4,3,3,3,
3,3,3,3,3,3,3,3,4),(0.000628504292635843,0.000640254986321947,0.000837411769728766,
0.000877277691072229,0.00100166439029042,0.00112605108950862,0.00129967406001939,
0.00158178243883092,0.00162359788638139,0.00162947384441178,0.00195921469101131,
0.00212114468325416,0.00261869148012693),.UNSPECIFIED.);
#5350=B_SPLINE_CURVE_WITH_KNOTS('',3,(#185162,#185163,#185164,#185165,#185166,
#185167,#185168,#185169,#185170,#185171,#185172,#185173,#185174,#185175,
#185176,#185177,#185178,#185179,#185180,#185181,#185182,#185183,#185184,
#185185,#185186,#185187,#185188,#185189,#185190,#185191,#185192,#185193,
#185194,#185195,#185196,#185197,#185198,#185199,#185200,#185201,#185202,
#185203,#185204,#185205,#185206,#185207,#185208,#185209,#185210,#185211,
#185212,#185213,#185214,#185215,#185216,#185217,#185218,#185219,#185220,
#185221,#185222,#185223,#185224,#185225),.UNSPECIFIED.,.F.,.F.,(4,3,3,3,
3,3,3,3,3,3,3,3,3,3,3,3,3,3,3,3,3,4),(1.06711334784298E-7,0.162604295707322,
0.250000000000111,0.346235688365917,0.37500000000017,0.437500000000205,
0.468750000000223,0.484375000000228,0.494029099182314,0.500000000000232,
0.562024892877923,0.625000000000202,0.686304312199343,0.718750000000151,
0.732744455805283,0.746155904384784,0.750000000000127,0.791548708438476,
0.845340878863513,0.898737355231329,0.951745167827004,1.),.UNSPECIFIED.);
#5351=B_SPLINE_CURVE_WITH_KNOTS('',3,(#185227,#185228,#185229,#185230,#185231,
#185232,#185233,#185234,#185235,#185236,#185237,#185238,#185239,#185240,
#185241,#185242,#185243,#185244,#185245,#185246,#185247,#185248,#185249,
#185250,#185251,#185252,#185253,#185254,#185255,#185256,#185257,#185258,
#185259,#185260,#185261,#185262,#185263,#185264,#185265,#185266,#185267,
#185268,#185269),.UNSPECIFIED.,.F.,.F.,(4,3,3,3,3,3,3,3,3,3,3,3,3,3,4),
(6.03724857329268E-15,0.0751859964940513,0.1495754148425,0.223294821152985,
0.29646818908788,0.369217351735024,0.441662438840354,0.51393127270104,0.586176148411227,
0.658501301088192,0.731011174783843,0.804060525502846,0.877464812066976,
0.951640239520033,1.),.UNSPECIFIED.);
#5352=B_SPLINE_CURVE_WITH_KNOTS('',3,(#185306,#185307,#185308,#185309,#185310,
#185311,#185312,#185313,#185314,#185315,#185316,#185317,#185318,#185319,
#185320,#185321,#185322,#185323,#185324,#185325,#185326,#185327,#185328,
#185329,#185330,#185331,#185332,#185333,#185334,#185335,#185336,#185337,
#185338,#185339,#185340,#185341,#185342,#185343,#185344,#185345),
 .UNSPECIFIED.,.F.,.F.,(4,3,3,3,3,3,3,3,3,3,3,3,3,4),(0.,0.0769432907447413,
0.153258768055538,0.229074002309316,0.304514589970782,0.379704601656095,
0.457241526449082,0.532396464239891,0.607701562850284,0.683265685333108,
0.762449263999828,0.839174120767956,0.919587060383972,0.999999999999988),
 .UNSPECIFIED.);
#5353=B_SPLINE_CURVE_WITH_KNOTS('',3,(#185346,#185347,#185348,#185349,#185350,
#185351,#185352,#185353,#185354,#185355,#185356,#185357,#185358,#185359,
#185360,#185361,#185362,#185363,#185364,#185365,#185366,#185367,#185368,
#185369,#185370,#185371,#185372,#185373,#185374,#185375,#185376,#185377,
#185378,#185379,#185380,#185381,#185382,#185383,#185384,#185385,#185386,
#185387,#185388,#185389,#185390,#185391,#185392,#185393,#185394,#185395,
#185396,#185397,#185398,#185399,#185400,#185401,#185402,#185403,#185404,
#185405,#185406,#185407,#185408,#185409,#185410,#185411,#185412,#185413,
#185414,#185415,#185416,#185417,#185418),.UNSPECIFIED.,.F.,.F.,(4,3,3,3,
3,3,3,3,3,3,3,3,3,3,3,3,3,3,3,3,3,3,3,3,4),(0.,0.053066835316157,0.107443152978828,
0.12499999999975,0.164971619184019,0.190888873117842,0.204943238368287,
0.218749999999565,0.230944613269073,0.243881742710735,0.249999999999505,
0.3086696401951,0.31701739205347,0.374999999999218,0.43499167648113,0.437499999999049,
0.46874999999896,0.484374999998946,0.493605897327227,0.499999999998931,
0.562499999999065,0.672531769754724,0.785034592397643,0.90313919621424,
1.),.UNSPECIFIED.);
#5354=B_SPLINE_CURVE_WITH_KNOTS('',3,(#185437,#185438,#185439,#185440,#185441,
#185442,#185443,#185444,#185445,#185446,#185447,#185448,#185449,#185450,
#185451,#185452,#185453,#185454,#185455,#185456,#185457,#185458,#185459,
#185460,#185461,#185462,#185463,#185464,#185465,#185466,#185467),
 .UNSPECIFIED.,.F.,.F.,(4,3,3,3,3,3,3,3,3,3,4),(0.,0.133384645899484,0.241711565162048,
0.265234332982687,0.367395294896058,0.446470883034051,0.501816373465676,
0.633825505921846,0.766458015306425,0.897442561934306,1.),.UNSPECIFIED.);
#5355=B_SPLINE_CURVE_WITH_KNOTS('',3,(#185505,#185506,#185507,#185508,#185509,
#185510,#185511,#185512,#185513,#185514,#185515,#185516,#185517,#185518,
#185519,#185520,#185521,#185522),.UNSPECIFIED.,.F.,.F.,(4,2,1,1,1,2,2,1,
2,2,4),(0.,0.250000000000277,0.375000000000416,0.437500000000485,0.468750000000498,
0.484375000000484,0.500000000000469,0.625000000000387,0.68750000000033,
0.750000000000273,1.),.UNSPECIFIED.);
#5356=B_SPLINE_CURVE_WITH_KNOTS('',3,(#185564,#185565,#185566,#185567,#185568,
#185569,#185570,#185571,#185572,#185573,#185574,#185575,#185576,#185577,
#185578,#185579,#185580,#185581,#185582,#185583,#185584,#185585,#185586,
#185587,#185588,#185589,#185590,#185591,#185592,#185593,#185594,#185595,
#185596,#185597,#185598,#185599,#185600,#185601,#185602,#185603,#185604,
#185605,#185606,#185607,#185608,#185609,#185610,#185611,#185612,#185613,
#185614,#185615),.UNSPECIFIED.,.F.,.F.,(4,3,3,3,3,3,3,3,3,3,3,3,3,3,3,3,
3,4),(0.,8.48627990060068E-5,0.000110154370857281,0.000197555987869283,
0.00023405941937725,0.000330463112571844,0.000419877362193912,0.000438835738394224,
0.000440617483429125,0.000729065363264048,0.000878897195867667,0.00088123496685825,
0.00114445185852502,0.00132031265264404,0.00132185245028737,0.00147439999768883,
0.00163314747063792,0.0017624699337165),.UNSPECIFIED.);
#5357=B_SPLINE_CURVE_WITH_KNOTS('',3,(#185656,#185657,#185658,#185659,#185660,
#185661,#185662,#185663,#185664,#185665,#185666,#185667,#185668,#185669,
#185670,#185671,#185672,#185673,#185674,#185675,#185676,#185677,#185678,
#185679,#185680),.UNSPECIFIED.,.F.,.F.,(4,3,3,3,3,3,3,3,4),(0.,0.124999999999963,
0.187499999999945,0.249999999999927,0.374999999999939,0.499999999999951,
0.696720148433668,0.749999999999976,1.),.UNSPECIFIED.);
#5358=B_SPLINE_CURVE_WITH_KNOTS('',3,(#185710,#185711,#185712,#185713,#185714,
#185715,#185716,#185717,#185718,#185719,#185720,#185721,#185722,#185723,
#185724,#185725,#185726,#185727,#185728,#185729,#185730,#185731),
 .UNSPECIFIED.,.F.,.F.,(4,3,3,3,3,3,3,4),(0.,0.22646738217556,0.25,0.5,
0.689823042701396,0.75,0.923487802122837,1.),.UNSPECIFIED.);
#5359=B_SPLINE_CURVE_WITH_KNOTS('',3,(#185767,#185768,#185769,#185770,#185771,
#185772,#185773,#185774,#185775,#185776,#185777,#185778,#185779,#185780,
#185781,#185782,#185783,#185784,#185785,#185786,#185787,#185788,#185789,
#185790,#185791,#185792,#185793,#185794,#185795,#185796,#185797,#185798,
#185799,#185800,#185801,#185802,#185803,#185804,#185805,#185806,#185807,
#185808,#185809,#185810,#185811,#185812),.UNSPECIFIED.,.F.,.F.,(4,3,3,3,
3,3,3,3,3,3,3,3,3,3,3,4),(0.,0.000111620791367575,0.000225473811195191,
0.000339302579903024,0.000397521249509077,0.000399067370002251,0.000667517661644283,
0.000795042499018153,0.000797178277617395,0.00104506031877655,0.00119256374852723,
0.00119405065366289,0.0013234358669085,0.0014567604324724,0.00158159308775795,
0.0015900849980363),.UNSPECIFIED.);
#5360=B_SPLINE_CURVE_WITH_KNOTS('',3,(#185852,#185853,#185854,#185855,#185856,
#185857,#185858,#185859,#185860,#185861,#185862,#185863,#185864,#185865,
#185866,#185867,#185868,#185869,#185870,#185871,#185872,#185873,#185874,
#185875,#185876,#185877,#185878,#185879,#185880,#185881,#185882,#185883,
#185884,#185885,#185886,#185887,#185888,#185889,#185890,#185891,#185892,
#185893,#185894),.UNSPECIFIED.,.F.,.F.,(4,3,3,3,3,3,3,3,3,3,3,3,3,3,4),
(0.,0.000168850029785425,0.000336050047502259,0.000405527490133955,0.000407005029304983,
0.000682198964448582,0.000811826624698246,0.000814010058609966,0.00109897545099617,
0.00121939063721615,0.00122101508791495,0.00134692436003165,0.00147131083154616,
0.00159335498692557,0.0016280201172199),.UNSPECIFIED.);
#5361=B_SPLINE_CURVE_WITH_KNOTS('',3,(#186057,#186058,#186059,#186060,#186061,
#186062),.UNSPECIFIED.,.F.,.F.,(4,2,4),(0.000562946727309309,0.00236076329038739,
0.00415857985346548),.UNSPECIFIED.);
#5362=B_SPLINE_CURVE_WITH_KNOTS('',3,(#186160,#186161,#186162,#186163,#186164,
#186165,#186166,#186167,#186168,#186169,#186170,#186171,#186172,#186173,
#186174,#186175,#186176,#186177,#186178,#186179,#186180,#186181,#186182,
#186183,#186184,#186185,#186186,#186187,#186188,#186189,#186190,#186191,
#186192,#186193,#186194,#186195,#186196,#186197,#186198,#186199,#186200,
#186201,#186202,#186203,#186204,#186205,#186206,#186207,#186208,#186209,
#186210,#186211,#186212,#186213,#186214,#186215,#186216,#186217,#186218,
#186219,#186220,#186221,#186222,#186223,#186224,#186225,#186226,#186227,
#186228,#186229,#186230,#186231,#186232),.UNSPECIFIED.,.F.,.F.,(4,3,3,3,
3,3,3,3,3,3,3,3,3,3,3,3,3,3,3,3,3,3,3,3,4),(5.59106843353732E-9,0.0443629897048473,
0.119873585712499,0.190502577283635,0.209068196859206,0.249999999999805,
0.321582585084567,0.367287555228283,0.381990119969657,0.441953706375988,
0.492187499999601,0.497575926912646,0.499999999999598,0.531254057232031,
0.585370887938339,0.637190770031103,0.685890707754348,0.723267035789511,
0.749999999999799,0.802882641837966,0.854604290016104,0.8749999999999,0.920965954037863,
0.964332381888369,1.),.UNSPECIFIED.);
#5363=B_SPLINE_CURVE_WITH_KNOTS('',3,(#186248,#186249,#186250,#186251,#186252,
#186253,#186254,#186255,#186256,#186257),.UNSPECIFIED.,.F.,.F.,(4,3,3,4),
(0.,0.371377520235629,0.776879610669599,1.),.UNSPECIFIED.);
#5364=B_SPLINE_CURVE_WITH_KNOTS('',3,(#186275,#186276,#186277,#186278,#186279,
#186280,#186281,#186282,#186283,#186284,#186285,#186286,#186287,#186288,
#186289,#186290,#186291,#186292,#186293,#186294,#186295,#186296,#186297,
#186298,#186299,#186300,#186301,#186302,#186303,#186304,#186305,#186306,
#186307,#186308,#186309,#186310,#186311),.UNSPECIFIED.,.F.,.F.,(4,3,3,3,
3,3,3,3,3,3,3,3,4),(0.,0.152151913276676,0.25000000000001,0.386714368335732,
0.437499999999995,0.463570378436081,0.490496823135862,0.499999999999993,
0.614091604002371,0.723372130571636,0.830296728032007,0.934020703510205,
1.),.UNSPECIFIED.);
#5365=B_SPLINE_CURVE_WITH_KNOTS('',3,(#186313,#186314,#186315,#186316,#186317,
#186318,#186319,#186320,#186321,#186322,#186323,#186324,#186325),
 .UNSPECIFIED.,.F.,.F.,(4,3,3,3,4),(0.,0.306533919199522,0.613513205477452,
0.921258276490977,1.),.UNSPECIFIED.);
#5366=B_SPLINE_CURVE_WITH_KNOTS('',3,(#186381,#186382,#186383,#186384,#186385,
#186386,#186387),.UNSPECIFIED.,.F.,.F.,(4,3,4),(4.7123889803847,5.4977871437821,
6.28318530717959),.UNSPECIFIED.);
#5367=B_SPLINE_CURVE_WITH_KNOTS('',3,(#186412,#186413,#186414,#186415,#186416,
#186417,#186418),.UNSPECIFIED.,.F.,.F.,(4,3,4),(3.1415926535898,3.92699081698724,
4.71238898038469),.UNSPECIFIED.);
#5368=B_SPLINE_CURVE_WITH_KNOTS('',3,(#186447,#186448,#186449,#186450,#186451,
#186452,#186453),.UNSPECIFIED.,.F.,.F.,(4,3,4),(4.7123889803847,5.49778714378215,
6.28318530717959),.UNSPECIFIED.);
#5369=B_SPLINE_CURVE_WITH_KNOTS('',3,(#186478,#186479,#186480,#186481,#186482,
#186483,#186484),.UNSPECIFIED.,.F.,.F.,(4,3,4),(1.23467863058848E-16,0.785398163397455,
1.57079632679491),.UNSPECIFIED.);
#5370=B_SPLINE_CURVE_WITH_KNOTS('',3,(#186528,#186529,#186530,#186531,#186532,
#186533,#186534,#186535,#186536,#186537,#186538,#186539,#186540,#186541,
#186542,#186543,#186544,#186545,#186546),.UNSPECIFIED.,.F.,.F.,(4,3,3,3,
3,3,4),(0.,0.000905681138562551,0.00148255506350336,0.00163490147399828,
0.00222383259525504,0.00274053607504981,0.00296511012700672),
 .UNSPECIFIED.);
#5371=B_SPLINE_CURVE_WITH_KNOTS('',3,(#186571,#186572,#186573,#186574,#186575,
#186576,#186577),.UNSPECIFIED.,.F.,.F.,(4,3,4),(1.5707963267949,2.35619449019235,
3.1415926535898),.UNSPECIFIED.);
#5372=B_SPLINE_CURVE_WITH_KNOTS('',3,(#186602,#186603,#186604,#186605,#186606,
#186607,#186608),.UNSPECIFIED.,.F.,.F.,(4,3,4),(1.23467863058847E-16,0.785398163397447,
1.5707963267949),.UNSPECIFIED.);
#5373=B_SPLINE_CURVE_WITH_KNOTS('',3,(#186633,#186634,#186635,#186636,#186637,
#186638,#186639,#186640,#186641,#186642,#186643,#186644,#186645,#186646,
#186647,#186648,#186649,#186650,#186651),.UNSPECIFIED.,.F.,.F.,(4,3,3,3,
3,3,4),(0.000169216231990766,0.000729993311367161,0.000968460740699438,
0.00168309612079798,0.00176770524940811,0.00279102522271382,0.00336619426682546),
 .UNSPECIFIED.);
#5374=B_SPLINE_CURVE_WITH_KNOTS('',3,(#186698,#186699,#186700,#186701,#186702,
#186703,#186704),.UNSPECIFIED.,.F.,.F.,(4,3,4),(4.71238898038469,5.49778714378214,
6.28318530717959),.UNSPECIFIED.);
#5375=B_SPLINE_CURVE_WITH_KNOTS('',3,(#186729,#186730,#186731,#186732,#186733,
#186734,#186735),.UNSPECIFIED.,.F.,.F.,(4,3,4),(1.23467863058847E-16,0.785398163397447,
1.5707963267949),.UNSPECIFIED.);
#5376=B_SPLINE_CURVE_WITH_KNOTS('',3,(#186771,#186772,#186773,#186774,#186775,
#186776,#186777),.UNSPECIFIED.,.F.,.F.,(4,3,4),(1.5707963267949,2.35619449019234,
3.14159265358979),.UNSPECIFIED.);
#5377=B_SPLINE_CURVE_WITH_KNOTS('',3,(#186802,#186803,#186804,#186805,#186806,
#186807,#186808),.UNSPECIFIED.,.F.,.F.,(4,3,4),(3.14159265358979,3.92699081698724,
4.71238898038469),.UNSPECIFIED.);
#5378=B_SPLINE_CURVE_WITH_KNOTS('',3,(#186834,#186835,#186836,#186837,#186838,
#186839,#186840,#186841,#186842,#186843,#186844,#186845,#186846,#186847,
#186848,#186849),.UNSPECIFIED.,.F.,.F.,(4,3,3,3,3,4),(0.000244714080610449,
0.00121583023104281,0.00174053473821824,0.00180545417371792,0.00292276797849773,
0.00336619426682539),.UNSPECIFIED.);
#5379=B_SPLINE_CURVE_WITH_KNOTS('',3,(#186874,#186875,#186876,#186877,#186878,
#186879,#186880),.UNSPECIFIED.,.F.,.F.,(4,3,4),(1.5707963267949,2.35619449019232,
3.14159265358979),.UNSPECIFIED.);
#5380=B_SPLINE_CURVE_WITH_KNOTS('',3,(#186905,#186906,#186907,#186908,#186909,
#186910,#186911),.UNSPECIFIED.,.F.,.F.,(4,3,4),(-1.77635683940025E-15,0.785398163397447,
1.57079632679489),.UNSPECIFIED.);
#5381=B_SPLINE_CURVE_WITH_KNOTS('',3,(#186937,#186938,#186939,#186940,#186941,
#186942,#186943,#186944,#186945,#186946,#186947,#186948,#186949,#186950,
#186951,#186952,#186953,#186954,#186955,#186956,#186957,#186958,#186959,
#186960,#186961,#186962,#186963,#186964,#186965,#186966,#186967,#186968,
#186969,#186970,#186971,#186972,#186973,#186974,#186975,#186976,#186977,
#186978,#186979,#186980,#186981,#186982,#186983,#186984,#186985,#186986,
#186987,#186988,#186989,#186990,#186991,#186992,#186993,#186994),
 .UNSPECIFIED.,.F.,.F.,(4,3,3,3,3,3,3,3,3,3,3,3,3,3,3,3,3,3,3,4),(0.,0.0574313460779371,
0.117800031813472,0.183766052524469,0.218749999999997,0.234374999999995,
0.242187499999999,0.250000000000002,0.336658026235113,0.375000000000007,
0.466327390959677,0.484375000000006,0.496043375977593,0.500000000000006,
0.502720832074079,0.59984784615854,0.7048612171632,0.815201166331238,0.93528875928782,
1.),.UNSPECIFIED.);
#5382=B_SPLINE_CURVE_WITH_KNOTS('',3,(#187025,#187026,#187027,#187028,#187029,
#187030,#187031),.UNSPECIFIED.,.F.,.F.,(4,3,4),(1.57079632679491,2.35619449019235,
3.14159265358979),.UNSPECIFIED.);
#5383=B_SPLINE_CURVE_WITH_KNOTS('',3,(#187056,#187057,#187058,#187059,#187060,
#187061,#187062),.UNSPECIFIED.,.F.,.F.,(4,3,4),(-1.77635683940025E-15,0.785398163397447,
1.57079632679489),.UNSPECIFIED.);
#5384=B_SPLINE_CURVE_WITH_KNOTS('',3,(#187087,#187088,#187089,#187090,#187091,
#187092,#187093,#187094,#187095,#187096,#187097,#187098,#187099,#187100,
#187101,#187102,#187103,#187104,#187105),.UNSPECIFIED.,.F.,.F.,(4,3,3,3,
3,3,4),(0.00047266192456923,0.000857724029065683,0.00153872216956474,0.0018499707510604,
0.00201291034255504,0.00292749448069884,0.00355315876054085),
 .UNSPECIFIED.);
#5385=B_SPLINE_CURVE_WITH_KNOTS('',3,(#187130,#187131,#187132,#187133,#187134,
#187135,#187136,#187137,#187138,#187139,#187140,#187141,#187142,#187143,
#187144,#187145,#187146,#187147,#187148,#187149,#187150,#187151,#187152,
#187153,#187154,#187155,#187156,#187157,#187158,#187159,#187160,#187161,
#187162,#187163,#187164,#187165,#187166),.UNSPECIFIED.,.F.,.F.,(4,3,3,3,
3,3,3,3,3,3,3,3,4),(1.96820403583049,2.07447029970642,2.18239924823465,
2.29295513021916,2.40448289443547,2.51591247508908,2.55489944283297,2.66627384567102,
2.77787483330248,2.88775468513439,2.99605880939301,3.10223763839193,3.14159265358979),
 .UNSPECIFIED.);
#5386=B_SPLINE_CURVE_WITH_KNOTS('',3,(#187195,#187196,#187197,#187198,#187199,
#187200,#187201),.UNSPECIFIED.,.F.,.F.,(4,3,4),(4.7123889803847,5.49778714378215,
6.28318530717959),.UNSPECIFIED.);
#5387=B_SPLINE_CURVE_WITH_KNOTS('',3,(#187226,#187227,#187228,#187229,#187230,
#187231,#187232),.UNSPECIFIED.,.F.,.F.,(4,3,4),(-1.77635683940025E-15,0.785398163397447,
1.57079632679489),.UNSPECIFIED.);
#5388=B_SPLINE_CURVE_WITH_KNOTS('',3,(#187264,#187265,#187266,#187267,#187268,
#187269,#187270,#187271,#187272,#187273,#187274,#187275,#187276,#187277,
#187278,#187279,#187280,#187281,#187282,#187283,#187284,#187285,#187286,
#187287,#187288,#187289,#187290,#187291,#187292,#187293,#187294,#187295,
#187296,#187297,#187298,#187299,#187300,#187301,#187302,#187303,#187304,
#187305,#187306,#187307,#187308,#187309,#187310,#187311,#187312,#187313,
#187314,#187315,#187316,#187317,#187318,#187319,#187320,#187321,#187322,
#187323,#187324,#187325,#187326,#187327,#187328,#187329,#187330),
 .UNSPECIFIED.,.F.,.F.,(4,3,3,3,3,3,3,3,3,3,3,3,3,3,3,3,3,3,3,3,3,3,4),
(0.,0.103658513321288,0.125,0.169018534161299,0.213461877707459,0.250000000000001,
0.250951766798841,0.335698253700407,0.375000000000001,0.416829400350235,
0.459227774972107,0.500000000000001,0.501310898730185,0.571535494191993,
0.625000000000002,0.672446050926232,0.687500000000002,0.735320212679162,
0.750000000000002,0.819805912927389,0.890142978787528,0.960075009265078,
1.),.UNSPECIFIED.);
#5389=B_SPLINE_CURVE_WITH_KNOTS('',3,(#187371,#187372,#187373,#187374,#187375,
#187376,#187377,#187378,#187379,#187380,#187381,#187382,#187383,#187384,
#187385,#187386,#187387,#187388,#187389,#187390,#187391,#187392,#187393,
#187394,#187395,#187396,#187397,#187398,#187399,#187400,#187401,#187402,
#187403,#187404,#187405,#187406,#187407,#187408,#187409,#187410,#187411,
#187412,#187413),.UNSPECIFIED.,.F.,.F.,(4,3,3,3,3,3,3,3,3,3,3,3,3,3,4),
(0.,0.000127008698005063,0.000262529185195825,0.000398049672386588,0.000399547425717595,
0.00064867929835264,0.000796943972592095,0.00079909485143519,0.00106876545795213,
0.00119708559701166,0.00119864227715278,0.00131330308627002,0.00142818443762419,
0.00153991729226719,0.00159818970287038),.UNSPECIFIED.);
#5390=B_SPLINE_CURVE_WITH_KNOTS('',3,(#187438,#187439,#187440,#187441,#187442,
#187443,#187444,#187445,#187446,#187447,#187448,#187449,#187450,#187451,
#187452,#187453,#187454,#187455,#187456),.UNSPECIFIED.,.F.,.F.,(4,3,3,3,
3,3,4),(0.,0.176003355398739,0.25,0.442266421325595,0.5,0.75,1.),
 .UNSPECIFIED.);
#5391=B_SPLINE_CURVE_WITH_KNOTS('',3,(#187492,#187493,#187494,#187495,#187496,
#187497,#187498,#187499,#187500,#187501,#187502,#187503,#187504,#187505,
#187506,#187507,#187508,#187509,#187510,#187511,#187512,#187513,#187514,
#187515,#187516,#187517,#187518,#187519),.UNSPECIFIED.,.F.,.F.,(4,3,3,3,
3,3,3,3,3,4),(0.,0.231192918218893,0.249999999999998,0.374999999999998,
0.499999999999999,0.624999999999999,0.687499999999999,0.749999999999999,
0.943972933317676,1.),.UNSPECIFIED.);
#5392=B_SPLINE_CURVE_WITH_KNOTS('',3,(#187567,#187568,#187569,#187570,#187571,
#187572,#187573,#187574,#187575,#187576,#187577,#187578,#187579,#187580,
#187581,#187582,#187583,#187584,#187585,#187586,#187587,#187588,#187589,
#187590,#187591,#187592,#187593,#187594,#187595,#187596,#187597,#187598,
#187599,#187600,#187601,#187602,#187603,#187604,#187605,#187606,#187607,
#187608,#187609,#187610,#187611,#187612,#187613,#187614,#187615,#187616,
#187617,#187618),.UNSPECIFIED.,.F.,.F.,(4,3,3,3,3,3,3,3,3,3,3,3,3,3,3,3,
3,4),(0.,0.000162974000351715,0.000319609377590832,0.00044215652538248,
0.000443701447435103,0.000705760117587417,0.000884313050764961,0.000886662825918405,
0.00117556448146201,0.00132646957614744,0.00132826306101653,0.00141792619142879,
0.00143700870749306,0.00151991305600227,0.00155002729305631,0.00163724702277407,
0.0017219272748049,0.00176862610152992),.UNSPECIFIED.);
#5393=B_SPLINE_CURVE_WITH_KNOTS('',3,(#187659,#187660,#187661,#187662,#187663,
#187664,#187665,#187666,#187667,#187668,#187669,#187670,#187671,#187672,
#187673,#187674,#187675),.UNSPECIFIED.,.F.,.F.,(4,1,1,2,2,1,1,1,2,2,4),
(0.,0.125000000000005,0.187500000000007,0.218750000000008,0.250000000000009,
0.375000000000011,0.437500000000013,0.46875000000001,0.484375000000014,
0.500000000000017,1.),.UNSPECIFIED.);
#5394=B_SPLINE_CURVE_WITH_KNOTS('',3,(#187723,#187724,#187725,#187726,#187727,
#187728,#187729,#187730,#187731,#187732,#187733,#187734,#187735,#187736,
#187737,#187738,#187739,#187740,#187741,#187742,#187743,#187744),
 .UNSPECIFIED.,.F.,.F.,(4,3,3,3,3,3,3,4),(0.,0.000360666935666808,0.000449610485509243,
0.000757497233646948,0.000899220971018486,0.00134883145652773,0.00157363669928234,
0.00179844194203696),.UNSPECIFIED.);
#5395=B_SPLINE_CURVE_WITH_KNOTS('',3,(#187791,#187792,#187793,#187794,#187795,
#187796,#187797,#187798,#187799,#187800,#187801,#187802,#187803,#187804,
#187805,#187806,#187807,#187808,#187809,#187810,#187811,#187812,#187813,
#187814,#187815,#187816,#187817,#187818,#187819,#187820,#187821,#187822,
#187823,#187824,#187825,#187826,#187827,#187828,#187829,#187830,#187831,
#187832,#187833),.UNSPECIFIED.,.F.,.F.,(4,3,3,3,3,3,3,3,3,3,3,3,3,3,4),
(0.,0.000195170703352208,0.000400502314359219,0.000446304927367807,0.000448134863283483,
0.000669908621781837,0.000672202294925215,0.000876863243061371,0.000893889262421621,
0.000896269726566947,0.00123667266508701,0.00134284656974638,0.00134440458985042,
0.00167688520284754,0.0017925394531339),.UNSPECIFIED.);
#5396=B_SPLINE_CURVE_WITH_KNOTS('',3,(#187881,#187882,#187883,#187884,#187885,
#187886,#187887,#187888,#187889,#187890,#187891,#187892,#187893,#187894,
#187895,#187896,#187897,#187898,#187899,#187900,#187901,#187902,#187903,
#187904,#187905,#187906,#187907,#187908,#187909,#187910,#187911,#187912,
#187913,#187914,#187915,#187916,#187917,#187918,#187919,#187920,#187921,
#187922,#187923,#187924,#187925,#187926),.UNSPECIFIED.,.F.,.F.,(4,3,3,3,
3,3,3,3,3,3,3,3,3,3,3,4),(0.,0.000125938335250352,0.000251511263371068,
0.000372362493801798,0.000393010036481153,0.000394487267106017,0.000650087135459798,
0.000786020072962305,0.000788180467911298,0.00103122780428417,0.00117903010944346,
0.00118059255633961,0.00129302327548811,0.00140596384630459,0.00151582795231526,
0.00157204014592461),.UNSPECIFIED.);
#5397=B_SPLINE_CURVE_WITH_KNOTS('',3,(#187966,#187967,#187968,#187969,#187970,
#187971,#187972,#187973,#187974,#187975,#187976,#187977,#187978,#187979,
#187980,#187981,#187982,#187983,#187984,#187985,#187986,#187987,#187988,
#187989,#187990,#187991,#187992,#187993,#187994,#187995,#187996,#187997,
#187998,#187999,#188000,#188001,#188002,#188003,#188004,#188005,#188006,
#188007,#188008),.UNSPECIFIED.,.F.,.F.,(4,3,3,3,3,3,3,3,3,3,3,3,3,3,4),
(0.,0.00012873091785914,0.000262886260532174,0.000397041603205207,0.000398543239038962,
0.000647566106702508,0.00079493581447458,0.000797086478077925,0.0010648677332478,
0.0011940802689539,0.00119562971711689,0.00131091067532157,0.00142650607919961,
0.00153915940329476,0.00159417295615585),.UNSPECIFIED.);
#5398=B_SPLINE_CURVE_WITH_KNOTS('',3,(#188039,#188040,#188041,#188042,#188043,
#188044,#188045,#188046,#188047,#188048,#188049,#188050,#188051,#188052,
#188053,#188054,#188055,#188056,#188057,#188058,#188059,#188060,#188061,
#188062,#188063,#188064,#188065,#188066,#188067,#188068,#188069,#188070,
#188071,#188072,#188073,#188074,#188075,#188076,#188077,#188078,#188079,
#188080,#188081,#188082,#188083,#188084,#188085,#188086,#188087,#188088,
#188089,#188090,#188091,#188092,#188093,#188094,#188095,#188096,#188097,
#188098,#188099),.UNSPECIFIED.,.F.,.F.,(4,3,3,3,3,3,3,3,3,3,3,3,3,3,3,3,
3,3,3,3,4),(0.,0.0625,0.139972153586169,0.15625,0.203125,0.25,0.3125,0.373286324414759,
0.43664316220738,0.496400222194438,0.5,0.501338831661234,0.571965089366115,
0.643232621636668,0.714229744959872,0.75,0.750926094557218,0.816401548475787,
0.88227904244363,0.947752342475233,1.),.UNSPECIFIED.);
#5399=B_SPLINE_CURVE_WITH_KNOTS('',3,(#188129,#188130,#188131,#188132,#188133,
#188134,#188135,#188136,#188137,#188138,#188139,#188140,#188141,#188142,
#188143,#188144,#188145,#188146,#188147,#188148,#188149,#188150,#188151,
#188152,#188153,#188154,#188155,#188156,#188157,#188158,#188159,#188160,
#188161,#188162,#188163,#188164,#188165,#188166,#188167,#188168,#188169,
#188170,#188171,#188172,#188173,#188174,#188175,#188176,#188177,#188178,
#188179,#188180),.UNSPECIFIED.,.F.,.F.,(4,3,3,3,3,3,3,3,3,3,3,3,3,3,3,3,
3,4),(0.,0.0644560924807926,0.128938108510493,0.192301428483669,0.25,0.31621626382761,
0.382182203805898,0.446812923850572,0.49888213793019,0.5,0.564513527455447,
0.629270711991716,0.693229549254467,0.75,0.825671875473234,0.901486212188946,
0.976405679522825,1.),.UNSPECIFIED.);
#5400=B_SPLINE_CURVE_WITH_KNOTS('',3,(#188227,#188228,#188229,#188230,#188231,
#188232,#188233,#188234,#188235,#188236,#188237),.UNSPECIFIED.,.F.,.F.,
(4,2,1,2,2,4),(0.,0.250000000000002,0.375000000000004,0.437500000000004,
0.500000000000005,1.),.UNSPECIFIED.);
#5401=B_SPLINE_CURVE_WITH_KNOTS('',3,(#188277,#188278,#188279,#188280,#188281,
#188282,#188283),.UNSPECIFIED.,.F.,.F.,(4,3,4),(0.,0.000214564004336314,
0.000397824826383788),.UNSPECIFIED.);
#5402=B_SPLINE_CURVE_WITH_KNOTS('',3,(#188300,#188301,#188302,#188303,#188304,
#188305,#188306,#188307,#188308,#188309,#188310,#188311,#188312,#188313,
#188314,#188315,#188316,#188317,#188318,#188319,#188320,#188321,#188322,
#188323,#188324,#188325,#188326,#188327,#188328,#188329,#188330),
 .UNSPECIFIED.,.F.,.F.,(4,3,3,3,3,3,3,3,3,3,4),(0.,0.148641184291234,0.250000000000006,
0.345102558943317,0.426964739075402,0.498594146690977,0.519796210982841,
0.671896501503741,0.824299079636482,0.974619845594587,1.),.UNSPECIFIED.);
#5403=B_SPLINE_CURVE_WITH_KNOTS('',3,(#188372,#188373,#188374,#188375,#188376,
#188377,#188378,#188379,#188380,#188381,#188382,#188383,#188384,#188385,
#188386,#188387,#188388,#188389,#188390,#188391,#188392,#188393,#188394,
#188395,#188396,#188397,#188398,#188399,#188400,#188401,#188402,#188403,
#188404,#188405,#188406,#188407,#188408,#188409,#188410,#188411,#188412,
#188413,#188414),.UNSPECIFIED.,.F.,.F.,(4,3,3,3,3,3,3,3,3,3,3,3,3,3,4),
(0.,0.00015584643830928,0.000318202659845265,0.000479330525642436,0.00048138854528345,
0.000719581971214055,0.000722082817925181,0.000946156964932637,0.000960283452349063,
0.000962777090566911,0.0012735805929567,0.00144265205691352,0.00144416563585035,
0.00187401285515416,0.0019255541811338),.UNSPECIFIED.);
#5404=B_SPLINE_CURVE_WITH_KNOTS('',3,(#188462,#188463,#188464,#188465,#188466,
#188467,#188468,#188469,#188470,#188471,#188472,#188473),.UNSPECIFIED.,
 .F.,.F.,(4,2,2,2,2,4),(0.,0.000425271195884802,0.000850542391769605,0.00127581358765441,
0.00148844918559681,0.00170108478353921),.UNSPECIFIED.);
#5405=B_SPLINE_CURVE_WITH_KNOTS('',3,(#188502,#188503,#188504,#188505,#188506,
#188507,#188508,#188509,#188510,#188511,#188512,#188513),.UNSPECIFIED.,
 .F.,.F.,(4,2,2,2,2,4),(0.,0.125,0.25,0.5,0.75,1.),.UNSPECIFIED.);
#5406=B_SPLINE_CURVE_WITH_KNOTS('',3,(#188561,#188562,#188563,#188564,#188565,
#188566,#188567,#188568,#188569,#188570,#188571,#188572,#188573,#188574,
#188575,#188576,#188577,#188578,#188579,#188580,#188581,#188582,#188583,
#188584,#188585,#188586,#188587,#188588,#188589,#188590,#188591,#188592,
#188593,#188594,#188595,#188596,#188597,#188598,#188599,#188600,#188601,
#188602,#188603),.UNSPECIFIED.,.F.,.F.,(4,3,3,3,3,3,3,3,3,3,3,3,3,3,4),
(0.,0.000133466187697468,0.000269195218943483,0.000394210955663315,0.000395766414125746,
0.000656135621812108,0.000788421911326631,0.000790581154836762,0.00102610013258057,
0.00118263286698995,0.00118412769954352,0.00130569231129943,0.00142779909867114,
0.00154775473597367,0.00157684382265327),.UNSPECIFIED.);
#5407=B_SPLINE_CURVE_WITH_KNOTS('',3,(#188644,#188645,#188646,#188647,#188648,
#188649,#188650,#188651,#188652,#188653,#188654,#188655,#188656,#188657,
#188658,#188659,#188660,#188661,#188662,#188663,#188664,#188665,#188666,
#188667,#188668,#188669,#188670,#188671,#188672,#188673,#188674,#188675,
#188676,#188677,#188678,#188679,#188680,#188681,#188682,#188683,#188684,
#188685,#188686,#188687,#188688,#188689),.UNSPECIFIED.,.F.,.F.,(4,3,3,3,
3,3,3,3,3,3,3,3,3,3,3,4),(0.,0.000126520648339655,0.000255464746612705,
0.000383289319161563,0.000402202417173513,0.000403696977019687,0.000649443966573114,
0.000805221313633904,0.000807393954039373,0.00107833188460959,0.00120950149130568,
0.00121109093105906,0.00132473335816662,0.00143856386975698,0.00154897302143375,
0.00161478790807874),.UNSPECIFIED.);
#5408=B_SPLINE_CURVE_WITH_KNOTS('',3,(#188714,#188715,#188716,#188717,#188718,
#188719,#188720,#188721,#188722,#188723,#188724,#188725,#188726,#188727),
 .UNSPECIFIED.,.F.,.F.,(4,2,2,2,2,2,4),(0.,0.124999999999998,0.249999999999996,
0.374999999999994,0.499999999999992,0.749999999999996,1.),.UNSPECIFIED.);
#5409=B_SPLINE_CURVE_WITH_KNOTS('',3,(#188775,#188776,#188777,#188778,#188779,
#188780,#188781,#188782,#188783,#188784,#188785,#188786,#188787,#188788,
#188789,#188790,#188791,#188792,#188793,#188794,#188795,#188796,#188797,
#188798,#188799,#188800,#188801,#188802,#188803,#188804,#188805,#188806,
#188807,#188808,#188809,#188810,#188811,#188812,#188813,#188814,#188815,
#188816,#188817),.UNSPECIFIED.,.F.,.F.,(4,3,3,3,3,3,3,3,3,3,3,3,3,3,4),
(0.,0.000124096840872279,0.000249826409753379,0.000377706687950511,0.000412914062840745,
0.000414565512418999,0.000703661138430754,0.00082582812568149,0.000828047391046449,
0.00110745290673328,0.00123874218852223,0.00124024370669316,0.00141015471005652,
0.00158186346550297,0.00165165625136298),.UNSPECIFIED.);
#5410=B_SPLINE_CURVE_WITH_KNOTS('',3,(#188858,#188859,#188860,#188861,#188862,
#188863,#188864,#188865,#188866,#188867,#188868,#188869,#188870,#188871,
#188872,#188873,#188874,#188875,#188876,#188877,#188878,#188879,#188880,
#188881,#188882,#188883,#188884,#188885,#188886,#188887,#188888,#188889,
#188890,#188891,#188892,#188893,#188894,#188895,#188896,#188897,#188898,
#188899,#188900),.UNSPECIFIED.,.F.,.F.,(4,3,3,3,3,3,3,3,3,3,3,3,3,3,4),
(0.,0.000126914134949833,0.000262536143227239,0.000398158151504644,0.000399655746142223,
0.000648709723487763,0.000797160169367609,0.000799311492284445,0.00106908297786263,
0.00119740971470136,0.00119896723842667,0.00131358784144415,0.00142842585215519,
0.0015401041970663,0.00159862298456889),.UNSPECIFIED.);
#5411=B_SPLINE_CURVE_WITH_KNOTS('',3,(#188925,#188926,#188927,#188928,#188929,
#188930,#188931,#188932,#188933,#188934,#188935,#188936,#188937,#188938,
#188939,#188940,#188941,#188942,#188943),.UNSPECIFIED.,.F.,.F.,(4,3,3,3,
3,3,4),(0.,0.175945370266497,0.249999999999999,0.442549347776631,0.499999999999999,
0.749999999999998,1.),.UNSPECIFIED.);
#5412=B_SPLINE_CURVE_WITH_KNOTS('',3,(#188984,#188985,#188986,#188987,#188988,
#188989,#188990,#188991,#188992,#188993,#188994,#188995,#188996,#188997,
#188998,#188999,#189000,#189001,#189002,#189003,#189004,#189005,#189006,
#189007,#189008,#189009,#189010,#189011,#189012,#189013,#189014,#189015,
#189016,#189017,#189018,#189019,#189020),.UNSPECIFIED.,.F.,.F.,(4,3,3,3,
3,3,3,3,3,3,3,3,4),(0.,0.000202328389737709,0.00039307053157685,0.000394637415448944,
0.000657523627630533,0.000787104044603751,0.000789274830897888,0.00100657728096933,
0.00118241998772925,0.00118391224634683,0.00131758895200345,0.00145591556828444,
0.00157854966179577),.UNSPECIFIED.);
#5413=B_SPLINE_CURVE_WITH_KNOTS('',3,(#189070,#189071,#189072,#189073,#189074,
#189075,#189076,#189077,#189078,#189079,#189080,#189081,#189082,#189083,
#189084,#189085,#189086,#189087,#189088,#189089,#189090,#189091,#189092,
#189093,#189094,#189095,#189096,#189097,#189098,#189099,#189100,#189101,
#189102,#189103,#189104,#189105,#189106,#189107,#189108,#189109,#189110,
#189111,#189112,#189113,#189114,#189115),.UNSPECIFIED.,.F.,.F.,(4,3,3,3,
3,3,3,3,3,3,3,3,3,3,3,4),(0.,0.00014308662566148,0.000288513574061214,0.00042656988910148,
0.000433940522460948,0.000435486060835305,0.000709558652808421,0.000867881044921896,
0.000870195056295086,0.00115300716696084,0.00130182156738284,0.00130356397838256,
0.00142320462553198,0.00154203711262811,0.00165601506682426,0.00173576208984379),
 .UNSPECIFIED.);
#5414=B_SPLINE_CURVE_WITH_KNOTS('',3,(#189149,#189150,#189151,#189152,#189153,
#189154,#189155,#189156,#189157,#189158,#189159,#189160,#189161,#189162,
#189163),.UNSPECIFIED.,.F.,.F.,(4,1,2,2,1,1,2,2,4),(0.,0.124999999999991,
0.187499999999987,0.249999999999983,0.374999999999974,0.437499999999969,
0.468749999999972,0.499999999999974,1.),.UNSPECIFIED.);
#5415=B_SPLINE_CURVE_WITH_KNOTS('',3,(#189210,#189211,#189212,#189213,#189214,
#189215,#189216,#189217,#189218,#189219,#189220,#189221,#189222),
 .UNSPECIFIED.,.F.,.F.,(4,3,3,3,4),(0.,0.306929728150734,0.616198997155632,
0.925384154814288,1.),.UNSPECIFIED.);
#5416=B_SPLINE_CURVE_WITH_KNOTS('',3,(#189440,#189441,#189442,#189443,#189444,
#189445),.UNSPECIFIED.,.F.,.F.,(4,2,4),(0.,0.5,1.),.UNSPECIFIED.);
#5417=B_SPLINE_CURVE_WITH_KNOTS('',3,(#189496,#189497,#189498,#189499,#189500,
#189501,#189502,#189503,#189504,#189505,#189506,#189507,#189508,#189509,
#189510,#189511,#189512,#189513,#189514,#189515,#189516,#189517,#189518,
#189519,#189520,#189521,#189522,#189523,#189524,#189525,#189526),
 .UNSPECIFIED.,.F.,.F.,(4,3,3,3,3,3,3,3,3,3,4),(2.72268262058649E-15,0.000200725121679123,
0.000415654200899631,0.000612812743333638,0.000613704338138227,0.00122637007266604,
0.00122740867627373,0.00180004332072134,0.0018404606068653,0.00184111301440923,
0.00245481735254474),.UNSPECIFIED.);
#5418=B_SPLINE_CURVE_WITH_KNOTS('',3,(#189529,#189530,#189531,#189532,#189533,
#189534,#189535,#189536,#189537,#189538),.UNSPECIFIED.,.F.,.F.,(4,2,2,2,
4),(0.,0.25,0.5,0.749999999999999,1.),.UNSPECIFIED.);
#5419=B_SPLINE_CURVE_WITH_KNOTS('',3,(#189554,#189555,#189556,#189557),
 .UNSPECIFIED.,.F.,.F.,(4,4),(0.,0.0105146476282051),.UNSPECIFIED.);
#5420=B_SPLINE_CURVE_WITH_KNOTS('',3,(#189558,#189559,#189560,#189561,#189562,
#189563,#189564,#189565,#189566,#189567,#189568,#189569,#189570,#189571,
#189572,#189573,#189574,#189575,#189576),.UNSPECIFIED.,.F.,.F.,(4,3,3,3,
3,3,4),(0.,0.213104637861165,0.407982689360979,0.589084311419952,0.696008383904322,
0.866070542392472,1.),.UNSPECIFIED.);
#5421=B_SPLINE_CURVE_WITH_KNOTS('',3,(#189614,#189615,#189616,#189617,#189618,
#189619,#189620,#189621,#189622,#189623,#189624,#189625,#189626,#189627,
#189628,#189629,#189630,#189631,#189632,#189633,#189634,#189635,#189636,
#189637,#189638,#189639,#189640,#189641,#189642,#189643,#189644,#189645,
#189646,#189647,#189648,#189649,#189650,#189651,#189652,#189653,#189654,
#189655,#189656,#189657,#189658,#189659,#189660,#189661,#189662,#189663,
#189664,#189665),.UNSPECIFIED.,.F.,.F.,(4,3,3,3,3,3,3,3,3,3,3,3,3,3,3,3,
3,4),(0.,0.0577449572001592,0.115760673898661,0.173966397974882,0.232612154939909,
0.25,0.317701909767158,0.387380567559864,0.460298498604314,0.5,0.576716836363912,
0.655971198986622,0.738743908648322,0.750000000000001,0.828430140854719,
0.908165239695145,0.988685556276332,0.999999999999989),.UNSPECIFIED.);
#5422=B_SPLINE_CURVE_WITH_KNOTS('',3,(#189666,#189667,#189668,#189669,#189670,
#189671,#189672,#189673,#189674,#189675),.UNSPECIFIED.,.F.,.F.,(4,2,2,2,
4),(0.,0.249999999999999,0.5,0.75,1.),.UNSPECIFIED.);
#5423=B_SPLINE_CURVE_WITH_KNOTS('',3,(#189703,#189704,#189705,#189706,#189707,
#189708,#189709),.UNSPECIFIED.,.F.,.F.,(4,3,4),(9.81307786677359E-18,0.00416048285086259,
0.00832096570172518),.UNSPECIFIED.);
#5424=B_SPLINE_CURVE_WITH_KNOTS('',3,(#189710,#189711,#189712,#189713,#189714,
#189715),.UNSPECIFIED.,.F.,.F.,(4,2,4),(0.,0.5,1.),.UNSPECIFIED.);
#5425=B_SPLINE_CURVE_WITH_KNOTS('',3,(#189755,#189756,#189757,#189758,#189759,
#189760,#189761,#189762,#189763,#189764,#189765,#189766,#189767,#189768,
#189769,#189770,#189771,#189772,#189773,#189774,#189775,#189776,#189777,
#189778,#189779,#189780,#189781,#189782,#189783,#189784,#189785,#189786,
#189787,#189788,#189789,#189790,#189791,#189792,#189793,#189794,#189795,
#189796,#189797,#189798,#189799,#189800,#189801,#189802,#189803),
 .UNSPECIFIED.,.F.,.F.,(4,3,3,3,3,3,3,3,3,3,3,3,3,3,3,3,4),(1.38012332775335E-14,
0.0812387813843933,0.165619390692197,0.244281834991246,0.25,0.337320583840223,
0.420544762023585,0.5,0.571921750742126,0.641679642600622,0.708356570658027,
0.75,0.8125,0.872346811049028,0.931984514842584,0.991450954272749,1.),
 .UNSPECIFIED.);
#5426=B_SPLINE_CURVE_WITH_KNOTS('',3,(#189804,#189805,#189806,#189807,#189808,
#189809,#189810,#189811,#189812,#189813),.UNSPECIFIED.,.F.,.F.,(4,2,2,2,
4),(0.,0.25,0.5,0.75,1.),.UNSPECIFIED.);
#5427=B_SPLINE_CURVE_WITH_KNOTS('',3,(#189835,#189836,#189837,#189838),
 .UNSPECIFIED.,.F.,.F.,(4,4),(0.,0.0107001581246114),.UNSPECIFIED.);
#5428=B_SPLINE_CURVE_WITH_KNOTS('',3,(#189839,#189840,#189841,#189842),
 .UNSPECIFIED.,.F.,.F.,(4,4),(0.,1.),.UNSPECIFIED.);
#5429=B_SPLINE_CURVE_WITH_KNOTS('',3,(#189858,#189859,#189860,#189861),
 .UNSPECIFIED.,.F.,.F.,(4,4),(0.,1.),.UNSPECIFIED.);
#5430=B_SPLINE_CURVE_WITH_KNOTS('',3,(#189862,#189863,#189864,#189865),
 .UNSPECIFIED.,.F.,.F.,(4,4),(0.,1.),.UNSPECIFIED.);
#5431=B_SPLINE_CURVE_WITH_KNOTS('',3,(#189888,#189889,#189890,#189891,#189892,
#189893,#189894,#189895,#189896,#189897,#189898,#189899,#189900,#189901,
#189902,#189903,#189904,#189905,#189906,#189907,#189908,#189909,#189910,
#189911,#189912),.UNSPECIFIED.,.F.,.F.,(4,3,3,3,3,3,3,3,4),(0.,0.122312447861915,
0.247147624918063,0.375895981289337,0.424647071101479,0.558508838421222,
0.69921940889293,0.849609704446465,1.),.UNSPECIFIED.);
#5432=B_SPLINE_CURVE_WITH_KNOTS('',3,(#189913,#189914,#189915,#189916,#189917,
#189918),.UNSPECIFIED.,.F.,.F.,(4,2,4),(0.,0.5,1.),.UNSPECIFIED.);
#5433=B_SPLINE_CURVE_WITH_KNOTS('',3,(#189961,#189962,#189963,#189964,#189965,
#189966,#189967,#189968,#189969,#189970,#189971,#189972),.UNSPECIFIED.,
 .F.,.F.,(4,2,2,2,2,4),(0.,0.249999999999999,0.375,0.500000000000001,0.75,
1.),.UNSPECIFIED.);
#5434=B_SPLINE_CURVE_WITH_KNOTS('',3,(#189975,#189976,#189977,#189978,#189979,
#189980,#189981,#189982,#189983,#189984,#189985,#189986,#189987,#189988,
#189989,#189990,#189991,#189992,#189993,#189994,#189995,#189996,#189997,
#189998,#189999,#190000,#190001,#190002,#190003,#190004,#190005,#190006,
#190007,#190008,#190009,#190010,#190011,#190012,#190013,#190014,#190015,
#190016,#190017,#190018,#190019,#190020,#190021,#190022,#190023,#190024,
#190025,#190026,#190027,#190028,#190029),.UNSPECIFIED.,.F.,.F.,(4,3,3,3,
3,3,3,3,3,3,3,3,3,3,3,3,3,3,4),(0.,0.0789176820769353,0.157127159397805,
0.233367179050978,0.25,0.325562808086822,0.399246594459274,0.469841989659592,
0.499999999999999,0.577528901441685,0.625,0.678393373561975,0.731135413249808,
0.750000000000001,0.806829802933232,0.863252623549527,0.919502567920812,
0.975672037690016,1.),.UNSPECIFIED.);
#5435=B_SPLINE_CURVE_WITH_KNOTS('',3,(#190045,#190046,#190047,#190048),
 .UNSPECIFIED.,.F.,.F.,(4,4),(4.04603565571183E-17,0.00980967348625103),
 .UNSPECIFIED.);
#5436=B_SPLINE_CURVE_WITH_KNOTS('',3,(#190049,#190050,#190051,#190052,#190053,
#190054,#190055,#190056,#190057,#190058,#190059,#190060,#190061),
 .UNSPECIFIED.,.F.,.F.,(4,3,3,3,4),(0.,0.268855438291974,0.55495113409128,
0.863752202872325,1.),.UNSPECIFIED.);
#5437=B_SPLINE_CURVE_WITH_KNOTS('',3,(#190083,#190084,#190085,#190086,#190087,
#190088,#190089,#190090,#190091,#190092,#190093,#190094,#190095,#190096,
#190097,#190098,#190099,#190100,#190101,#190102,#190103,#190104,#190105,
#190106,#190107),.UNSPECIFIED.,.F.,.F.,(4,3,3,3,3,3,3,3,4),(0.,0.152876067585667,
0.30639781432929,0.373021274914802,0.5,0.656092103689984,0.810004975183274,
0.95906628874972,1.),.UNSPECIFIED.);
#5438=B_SPLINE_CURVE_WITH_KNOTS('',3,(#190108,#190109,#190110,#190111,#190112,
#190113,#190114),.UNSPECIFIED.,.F.,.F.,(4,3,4),(0.,0.00416021787251447,
0.00832043574502893),.UNSPECIFIED.);
#5439=B_SPLINE_CURVE_WITH_KNOTS('',3,(#190136,#190137,#190138,#190139,#190140,
#190141),.UNSPECIFIED.,.F.,.F.,(4,2,4),(0.,0.5,1.),.UNSPECIFIED.);
#5440=B_SPLINE_CURVE_WITH_KNOTS('',3,(#190142,#190143,#190144,#190145,#190146,
#190147),.UNSPECIFIED.,.F.,.F.,(4,2,4),(0.,0.5,1.),.UNSPECIFIED.);
#5441=B_SPLINE_CURVE_WITH_KNOTS('',3,(#190181,#190182,#190183,#190184,#190185,
#190186,#190187,#190188,#190189,#190190),.UNSPECIFIED.,.F.,.F.,(4,2,2,2,
4),(0.,0.249999999999999,0.499999999999999,0.75,1.),.UNSPECIFIED.);
#5442=B_SPLINE_CURVE_WITH_KNOTS('',3,(#190191,#190192,#190193,#190194,#190195,
#190196,#190197,#190198,#190199,#190200,#190201,#190202,#190203,#190204,
#190205,#190206,#190207,#190208,#190209,#190210,#190211,#190212,#190213,
#190214,#190215,#190216,#190217,#190218,#190219,#190220,#190221,#190222,
#190223,#190224,#190225,#190226,#190227,#190228,#190229,#190230,#190231,
#190232,#190233,#190234,#190235,#190236,#190237,#190238,#190239,#190240,
#190241,#190242),.UNSPECIFIED.,.F.,.F.,(4,3,3,3,3,3,3,3,3,3,3,3,3,3,3,3,
3,4),(0.,0.0582415495970998,0.116663503047352,0.175224355996429,0.234148749404122,
0.25,0.322580824057758,0.396872773529455,0.473813539319455,0.500000000000001,
0.572660400761366,0.647461247395867,0.725045015722337,0.750000000000002,
0.826854309093119,0.904998593137059,0.98393508435569,1.),.UNSPECIFIED.);
#5443=B_SPLINE_CURVE_WITH_KNOTS('',3,(#190262,#190263,#190264,#190265,#190266,
#190267,#190268,#190269,#190270,#190271,#190272,#190273,#190274,#190275,
#190276,#190277,#190278,#190279,#190280),.UNSPECIFIED.,.F.,.F.,(4,3,3,3,
3,3,4),(0.,0.195941169472998,0.290434549960185,0.500144896478958,0.700717460267629,
0.890960745354147,1.),.UNSPECIFIED.);
#5444=B_SPLINE_CURVE_WITH_KNOTS('',3,(#190281,#190282,#190283,#190284),
 .UNSPECIFIED.,.F.,.F.,(4,4),(0.,0.00972938600277915),.UNSPECIFIED.);
#5445=B_SPLINE_CURVE_WITH_KNOTS('',3,(#190300,#190301,#190302,#190303),
 .UNSPECIFIED.,.F.,.F.,(4,4),(0.,2.59869381596583E-5),.UNSPECIFIED.);
#5446=B_SPLINE_CURVE_WITH_KNOTS('',3,(#190304,#190305,#190306,#190307),
 .UNSPECIFIED.,.F.,.F.,(4,4),(0.,3.23803390124219E-5),.UNSPECIFIED.);
#5447=B_SPLINE_CURVE_WITH_KNOTS('',3,(#190335,#190336,#190337,#190338,#190339,
#190340,#190341,#190342),.UNSPECIFIED.,.F.,.F.,(4,2,2,4),(0.,0.249999999999999,
0.5,1.),.UNSPECIFIED.);
#5448=B_SPLINE_CURVE_WITH_KNOTS('',3,(#190343,#190344,#190345,#190346,#190347,
#190348,#190349,#190350),.UNSPECIFIED.,.F.,.F.,(4,2,2,4),(0.,0.5,0.750000000000001,
1.),.UNSPECIFIED.);
#5449=B_SPLINE_CURVE_WITH_KNOTS('',3,(#190382,#190383,#190384,#190385),
 .UNSPECIFIED.,.F.,.F.,(4,4),(6.93889390390723E-18,2.09370149851292E-5),
 .UNSPECIFIED.);
#5450=B_SPLINE_CURVE_WITH_KNOTS('',3,(#190386,#190387,#190388,#190389),
 .UNSPECIFIED.,.F.,.F.,(4,4),(0.,1.68205588696557E-5),.UNSPECIFIED.);
#5451=B_SPLINE_CURVE_WITH_KNOTS('',3,(#190471,#190472,#190473,#190474),
 .UNSPECIFIED.,.F.,.F.,(4,4),(0.,0.000210836370419721),.UNSPECIFIED.);
#5452=B_SPLINE_CURVE_WITH_KNOTS('',3,(#190512,#190513,#190514,#190515,#190516,
#190517,#190518,#190519,#190520,#190521,#190522,#190523),.UNSPECIFIED.,
 .F.,.F.,(4,2,2,2,2,4),(0.,0.125,0.249999999999999,0.5,0.75,1.),
 .UNSPECIFIED.);
#5453=B_SPLINE_CURVE_WITH_KNOTS('',3,(#190526,#190527,#190528,#190529,#190530,
#190531,#190532,#190533,#190534,#190535,#190536,#190537),.UNSPECIFIED.,
 .F.,.F.,(4,2,2,2,2,4),(0.,0.25,0.500000000000001,0.750000000000001,0.875,
1.),.UNSPECIFIED.);
#5454=B_SPLINE_CURVE_WITH_KNOTS('',3,(#190577,#190578,#190579,#190580,#190581,
#190582,#190583,#190584,#190585,#190586,#190587,#190588,#190589,#190590,
#190591,#190592,#190593,#190594,#190595,#190596,#190597,#190598,#190599,
#190600,#190601,#190602,#190603,#190604,#190605,#190606,#190607,#190608,
#190609,#190610),.UNSPECIFIED.,.F.,.F.,(4,3,3,3,3,3,3,3,3,3,3,4),(0.,0.146910620412476,
0.25,0.391211209956079,0.5,0.583892307870227,0.625,0.706893805446917,0.75,
0.85002508516687,0.938030549136298,1.),.UNSPECIFIED.);
#5455=B_SPLINE_CURVE_WITH_KNOTS('',3,(#190611,#190612,#190613,#190614,#190615,
#190616,#190617,#190618,#190619,#190620,#190621,#190622),.UNSPECIFIED.,
 .F.,.F.,(4,2,2,2,2,4),(0.,0.25,0.375,0.5,0.75,1.),.UNSPECIFIED.);
#5456=B_SPLINE_CURVE_WITH_KNOTS('',3,(#190672,#190673,#190674,#190675,#190676,
#190677,#190678,#190679,#190680,#190681),.UNSPECIFIED.,.F.,.F.,(4,3,3,4),
(6.93889390390723E-18,0.000636015601018232,0.00129844965740646,0.00158760011419448),
 .UNSPECIFIED.);
#5457=B_SPLINE_CURVE_WITH_KNOTS('',3,(#190682,#190683,#190684,#190685,#190686,
#190687,#190688,#190689,#190690,#190691,#190692,#190693,#190694),
 .UNSPECIFIED.,.F.,.F.,(4,3,3,3,4),(0.,0.25669998202569,0.50808588571949,
0.754042942859745,1.),.UNSPECIFIED.);
#5458=B_SPLINE_CURVE_WITH_KNOTS('',3,(#190710,#190711,#190712,#190713,#190714,
#190715,#190716,#190717,#190718,#190719,#190720,#190721,#190722),
 .UNSPECIFIED.,.F.,.F.,(4,3,3,3,4),(0.,0.253266620399936,0.51240411680184,
0.78046435058956,1.),.UNSPECIFIED.);
#5459=B_SPLINE_CURVE_WITH_KNOTS('',3,(#190723,#190724,#190725,#190726,#190727,
#190728,#190729,#190730,#190731,#190732),.UNSPECIFIED.,.F.,.F.,(4,3,3,4),
(0.,0.000679723972679124,0.00133201311756995,0.0015185374894695),
 .UNSPECIFIED.);
#5460=B_SPLINE_CURVE_WITH_KNOTS('',3,(#190760,#190761,#190762,#190763,#190764,
#190765,#190766,#190767),.UNSPECIFIED.,.F.,.F.,(4,2,2,4),(0.,0.25,0.5,1.),
 .UNSPECIFIED.);
#5461=B_SPLINE_CURVE_WITH_KNOTS('',3,(#190768,#190769,#190770,#190771,#190772,
#190773,#190774,#190775),.UNSPECIFIED.,.F.,.F.,(4,2,2,4),(5.09829085353129E-9,
0.5,0.75,1.),.UNSPECIFIED.);
#5462=B_SPLINE_CURVE_WITH_KNOTS('',3,(#190803,#190804,#190805,#190806,#190807,
#190808,#190809,#190810),.UNSPECIFIED.,.F.,.F.,(4,2,2,4),(0.,0.25,0.5,0.999999992626662),
 .UNSPECIFIED.);
#5463=B_SPLINE_CURVE_WITH_KNOTS('',3,(#190811,#190812,#190813,#190814,#190815,
#190816,#190817,#190818),.UNSPECIFIED.,.F.,.F.,(4,2,2,4),(0.,0.5,0.75,1.),
 .UNSPECIFIED.);
#5464=B_SPLINE_CURVE_WITH_KNOTS('',3,(#190876,#190877,#190878,#190879,#190880,
#190881,#190882,#190883,#190884,#190885,#190886,#190887,#190888,#190889,
#190890,#190891,#190892,#190893),.UNSPECIFIED.,.F.,.F.,(4,2,2,2,2,2,2,2,
4),(0.,0.00781250000000114,0.0156250000000006,0.0312500000000013,0.0625000000000006,
0.125,0.250000000000001,0.5,1.),.UNSPECIFIED.);
#5465=B_SPLINE_CURVE_WITH_KNOTS('',3,(#190894,#190895,#190896,#190897,#190898,
#190899,#190900,#190901,#190902,#190903,#190904,#190905,#190906,#190907,
#190908,#190909,#190910,#190911),.UNSPECIFIED.,.F.,.F.,(4,2,2,2,2,2,2,2,
4),(9.19004041809617E-16,0.00254332115550819,0.00381498173326183,0.00445081202213868,
0.00476872716657715,0.00492768473879635,0.00500716352490594,0.00504690291796077,
0.0050866423110156),.UNSPECIFIED.);
#5466=B_SPLINE_CURVE_WITH_KNOTS('',3,(#190969,#190970,#190971,#190972,#190973,
#190974,#190975,#190976,#190977,#190978,#190979,#190980,#190981,#190982,
#190983,#190984,#190985,#190986,#190987,#190988,#190989,#190990,#190991,
#190992,#190993),.UNSPECIFIED.,.F.,.F.,(4,3,3,3,3,3,3,3,4),(0.,4.03932117393399E-5,
8.08651294214249E-5,0.000161907626915798,0.000324108918069935,0.000648595245071396,
0.00129766017874913,0.00259586603175177,0.00519236941687791),
 .UNSPECIFIED.);
#5467=B_SPLINE_CURVE_WITH_KNOTS('',3,(#190994,#190995,#190996,#190997,#190998,
#190999,#191000,#191001,#191002,#191003,#191004,#191005,#191006,#191007,
#191008,#191009,#191010,#191011),.UNSPECIFIED.,.F.,.F.,(4,2,2,2,2,2,2,2,
4),(0.,0.5,0.75,0.875,0.9375,0.96875,0.984375,0.9921875,1.),
 .UNSPECIFIED.);
#5468=B_SPLINE_CURVE_WITH_KNOTS('',3,(#191073,#191074,#191075,#191076,#191077,
#191078,#191079,#191080,#191081,#191082,#191083,#191084,#191085,#191086,
#191087,#191088,#191089,#191090),.UNSPECIFIED.,.F.,.F.,(4,2,2,2,2,2,2,2,
4),(0.,0.00262931855771754,0.00394397783657636,0.00460130747600577,0.00492997229572051,
0.00509430470557792,0.00517647091050667,0.00521755401297108,0.00525863711543548),
 .UNSPECIFIED.);
#5469=B_SPLINE_CURVE_WITH_KNOTS('',3,(#191093,#191094,#191095,#191096,#191097,
#191098,#191099,#191100,#191101,#191102,#191103,#191104,#191105,#191106,
#191107,#191108,#191109,#191110),.UNSPECIFIED.,.F.,.F.,(4,2,2,2,2,2,2,2,
4),(0.,0.00781250000000008,0.0156250000000003,0.0312500000000008,0.0624999999999995,
0.124999999999999,0.250000000000001,0.5,1.),.UNSPECIFIED.);
#5470=B_SPLINE_CURVE_WITH_KNOTS('',3,(#191144,#191145,#191146,#191147,#191148,
#191149,#191150,#191151),.UNSPECIFIED.,.F.,.F.,(4,2,2,4),(6.90105437428163E-9,
0.500000000000001,0.75,1.),.UNSPECIFIED.);
#5471=B_SPLINE_CURVE_WITH_KNOTS('',3,(#191152,#191153,#191154,#191155,#191156,
#191157,#191158,#191159),.UNSPECIFIED.,.F.,.F.,(4,2,2,4),(0.,0.25,0.499999999999999,
1.),.UNSPECIFIED.);
#5472=B_SPLINE_CURVE_WITH_KNOTS('',3,(#191217,#191218,#191219,#191220,#191221,
#191222,#191223,#191224,#191225,#191226,#191227,#191228,#191229,#191230,
#191231,#191232,#191233,#191234),.UNSPECIFIED.,.F.,.F.,(4,2,2,2,2,2,2,2,
4),(0.,0.5,0.75,0.875,0.9375,0.96875,0.984375,0.9921875,1.),
 .UNSPECIFIED.);
#5473=B_SPLINE_CURVE_WITH_KNOTS('',3,(#191235,#191236,#191237,#191238,#191239,
#191240,#191241,#191242,#191243,#191244,#191245,#191246,#191247,#191248,
#191249,#191250,#191251,#191252,#191253,#191254,#191255,#191256,#191257,
#191258,#191259),.UNSPECIFIED.,.F.,.F.,(4,3,3,3,3,3,3,3,4),(4.9065389333868E-17,
4.15775196007892E-5,8.32361282030658E-5,0.000166653476908059,0.000333604410320719,
0.000667590055213201,0.00133565310169655,0.00267185549873087,0.0053443518360984),
 .UNSPECIFIED.);
#5474=B_SPLINE_CURVE_WITH_KNOTS('',3,(#191275,#191276,#191277,#191278,#191279,
#191280,#191281,#191282,#191283,#191284,#191285,#191286,#191287),
 .UNSPECIFIED.,.F.,.F.,(4,3,3,3,4),(0.,0.327766562741204,0.663883281370602,
0.973924754667621,1.),.UNSPECIFIED.);
#5475=B_SPLINE_CURVE_WITH_KNOTS('',3,(#191288,#191289,#191290,#191291,#191292,
#191293,#191294),.UNSPECIFIED.,.F.,.F.,(4,3,4),(0.,0.000722422580495128,
0.00123518557486524),.UNSPECIFIED.);
#5476=B_SPLINE_CURVE_WITH_KNOTS('',3,(#191323,#191324,#191325,#191326),
 .UNSPECIFIED.,.F.,.F.,(4,4),(0.,1.),.UNSPECIFIED.);
#5477=B_SPLINE_CURVE_WITH_KNOTS('',3,(#191327,#191328,#191329,#191330,#191331,
#191332,#191333,#191334,#191335,#191336,#191337,#191338,#191339),
 .UNSPECIFIED.,.F.,.F.,(4,3,3,3,4),(3.67744356508555E-9,0.288281482145314,
0.499999999999999,0.644141111476281,1.),.UNSPECIFIED.);
#5478=B_SPLINE_CURVE_WITH_KNOTS('',3,(#191340,#191341,#191342,#191343,#191344,
#191345,#191346,#191347),.UNSPECIFIED.,.F.,.F.,(4,2,2,4),(0.,0.25,0.499999999999999,
1.),.UNSPECIFIED.);
#5479=B_SPLINE_CURVE_WITH_KNOTS('',3,(#191380,#191381,#191382,#191383,#191384,
#191385,#191386),.UNSPECIFIED.,.F.,.F.,(4,3,4),(0.,0.000727844608945735,
0.00121469382512387),.UNSPECIFIED.);
#5480=B_SPLINE_CURVE_WITH_KNOTS('',3,(#191387,#191388,#191389,#191390,#191391,
#191392,#191393,#191394,#191395,#191396),.UNSPECIFIED.,.F.,.F.,(4,3,3,4),
(0.,0.318581264575039,0.659290632287519,1.),.UNSPECIFIED.);
#5481=B_SPLINE_CURVE_WITH_KNOTS('',3,(#191439,#191440,#191441,#191442,#191443,
#191444,#191445,#191446,#191447,#191448,#191449,#191450,#191451,#191452,
#191453,#191454,#191455,#191456,#191457,#191458,#191459,#191460,#191461,
#191462,#191463,#191464,#191465,#191466,#191467,#191468,#191469,#191470,
#191471,#191472,#191473,#191474,#191475),.UNSPECIFIED.,.F.,.F.,(4,3,3,3,
3,3,3,3,3,3,3,3,4),(0.,0.0917080761850634,0.193847311803682,0.25,0.338811353118771,
0.375,0.45988080137128,0.5,0.608296703387408,0.625,0.75,0.923180341345264,
1.),.UNSPECIFIED.);
#5482=B_SPLINE_CURVE_WITH_KNOTS('',3,(#191476,#191477,#191478,#191479,#191480,
#191481,#191482,#191483,#191484,#191485,#191486,#191487,#191488,#191489,
#191490,#191491,#191492,#191493,#191494,#191495,#191496,#191497,#191498,
#191499,#191500,#191501,#191502,#191503,#191504,#191505,#191506,#191507,
#191508,#191509,#191510,#191511,#191512,#191513,#191514,#191515,#191516,
#191517,#191518,#191519,#191520,#191521,#191522,#191523,#191524,#191525,
#191526,#191527,#191528,#191529,#191530,#191531,#191532,#191533,#191534,
#191535,#191536),.UNSPECIFIED.,.F.,.F.,(4,3,3,3,3,3,3,3,3,3,3,3,3,3,3,3,
3,3,3,3,4),(0.,0.0735852225213234,0.145541216767293,0.214668449408842,0.25,
0.325070225880086,0.375,0.4375,0.496212771549303,0.5,0.548323841680636,
0.595853929305818,0.625,0.667359798109466,0.709665698884139,0.75,0.80690825694747,
0.864567180132038,0.92279287238488,0.982204606290843,1.),.UNSPECIFIED.);
#5483=B_SPLINE_CURVE_WITH_KNOTS('',3,(#191590,#191591,#191592,#191593,#191594,
#191595,#191596,#191597,#191598,#191599,#191600,#191601),.UNSPECIFIED.,
 .F.,.F.,(4,2,2,2,2,4),(0.,0.25,0.375,0.499999999999999,0.75,1.),
 .UNSPECIFIED.);
#5484=B_SPLINE_CURVE_WITH_KNOTS('',3,(#191602,#191603,#191604,#191605,#191606,
#191607,#191608,#191609,#191610,#191611,#191612,#191613,#191614,#191615,
#191616,#191617,#191618,#191619,#191620,#191621,#191622,#191623,#191624,
#191625,#191626,#191627,#191628,#191629,#191630,#191631,#191632,#191633,
#191634,#191635),.UNSPECIFIED.,.F.,.F.,(4,3,3,3,3,3,3,3,3,3,3,4),(0.,0.159857018254139,
0.25,0.393133814716374,0.500000000000001,0.586072065778788,0.625,0.711030211262596,
0.75,0.860251075790316,0.958533798021047,1.),.UNSPECIFIED.);
#5485=B_SPLINE_CURVE_WITH_KNOTS('',3,(#193430,#193431,#193432,#193433,#193434,
#193435,#193436,#193437,#193438,#193439),.UNSPECIFIED.,.F.,.F.,(4,2,2,2,
4),(-0.0951055308727295,-0.0757879150760358,-0.0421208524807574,0.,0.00038304003494894),
 .UNSPECIFIED.);
#5486=B_SPLINE_CURVE_WITH_KNOTS('',3,(#193474,#193475,#193476,#193477,#193478,
#193479,#193480,#193481,#193482,#193483),.UNSPECIFIED.,.F.,.F.,(4,2,2,2,
4),(-0.324953678743299,-0.324570638701253,-0.28244978588071,-0.248782723015611,
-0.229465107064107),.UNSPECIFIED.);
#5487=B_SPLINE_CURVE_WITH_KNOTS('',3,(#193493,#193494,#193495,#193496,#193497,
#193498,#193499,#193500,#193501,#193502),.UNSPECIFIED.,.F.,.F.,(4,2,2,2,
4),(-0.0951055274869706,-0.0757879123768078,-0.0421208509780448,-1.08246744900953E-15,
0.000383040004758421),.UNSPECIFIED.);
#5488=B_SPLINE_CURVE_WITH_KNOTS('',3,(#193537,#193538,#193539,#193540,#193541,
#193542,#193543,#193544,#193545,#193546),.UNSPECIFIED.,.F.,.F.,(4,2,2,2,
4),(-0.324953682197493,-0.324570642147117,-0.282449788877878,-0.248782725655785,
-0.229465109499444),.UNSPECIFIED.);
#5489=B_SPLINE_CURVE_WITH_KNOTS('',3,(#193556,#193557,#193558,#193559,#193560,
#193561,#193562,#193563,#193564,#193565),.UNSPECIFIED.,.F.,.F.,(4,2,2,2,
4),(-0.0951055284907788,-0.0757879131770604,-0.0421208514235227,0.,0.000383040013518366),
 .UNSPECIFIED.);
#5490=B_SPLINE_CURVE_WITH_KNOTS('',3,(#193600,#193601,#193602,#193603,#193604,
#193605,#193606,#193607,#193608,#193609),.UNSPECIFIED.,.F.,.F.,(4,2,2,2,
4),(-0.324953664307694,-0.324570624303572,-0.282449773358066,-0.248782711984591,
-0.22946509688894),.UNSPECIFIED.);
#5491=B_SPLINE_CURVE_WITH_KNOTS('',3,(#193615,#193616,#193617,#193618,#193619,
#193620,#193621,#193622,#193623,#193624),.UNSPECIFIED.,.F.,.F.,(4,2,2,2,
4),(-0.0003830399169838,0.,0.042120846642674,0.0757879045921621,0.095105517723294),
 .UNSPECIFIED.);
#5492=B_SPLINE_CURVE_WITH_KNOTS('',3,(#193663,#193664,#193665,#193666,#193667,
#193668,#193669,#193670,#193671,#193672),.UNSPECIFIED.,.F.,.F.,(4,2,2,2,
4),(-0.324953631774432,-0.324570591855723,-0.28244974513484,-0.248782687123421,
-0.229465073956758),.UNSPECIFIED.);
#5493=B_SPLINE_CURVE_WITH_KNOTS('',3,(#193866,#193867,#193868,#193869,#193870,
#193871,#193872,#193873,#193874,#193875,#193876,#193877,#193878,#193879,
#193880,#193881,#193882,#193883,#193884,#193885,#193886,#193887),
 .UNSPECIFIED.,.F.,.F.,(4,2,1,1,2,2,2,2,2,2,2,4),(0.,0.0156250000000012,
0.0312500000000023,0.0625000000000033,0.125000000000004,0.250000000000003,
0.500000000000002,0.750000000000001,0.875,0.9375,0.96875,1.),
 .UNSPECIFIED.);
#5494=B_SPLINE_CURVE_WITH_KNOTS('',3,(#193889,#193890,#193891,#193892,#193893,
#193894,#193895,#193896,#193897,#193898,#193899,#193900,#193901,#193902,
#193903,#193904,#193905,#193906,#193907,#193908,#193909,#193910,#193911,
#193912,#193913,#193914),.UNSPECIFIED.,.F.,.F.,(4,2,2,2,2,2,2,2,2,2,2,2,
4),(0.,0.00459330644835038,0.0094020344365217,0.0190194904128667,0.0382544023655542,
0.0767242262709338,0.384482817513955,0.538362113135469,0.61530176094622,
0.634536672898912,0.653771584851599,0.692241408756977,1.),.UNSPECIFIED.);
#5495=B_SPLINE_CURVE_WITH_KNOTS('',3,(#193918,#193919,#193920,#193921,#193922,
#193923,#193924,#193925,#193926,#193927,#193928,#193929,#193930,#193931,
#193932,#193933,#193934,#193935,#193936,#193937,#193938,#193939,#193940,
#193941,#193942,#193943,#193944,#193945,#193946,#193947,#193948,#193949,
#193950,#193951,#193952,#193953,#193954,#193955,#193956,#193957,#193958,
#193959,#193960,#193961,#193962,#193963,#193964,#193965,#193966,#193967,
#193968,#193969,#193970,#193971,#193972,#193973,#193974,#193975,#193976,
#193977,#193978,#193979,#193980,#193981,#193982,#193983,#193984,#193985,
#193986,#193987,#193988,#193989,#193990,#193991,#193992,#193993,#193994,
#193995,#193996,#193997,#193998,#193999,#194000,#194001,#194002,#194003,
#194004,#194005,#194006,#194007,#194008,#194009,#194010,#194011,#194012,
#194013,#194014,#194015,#194016,#194017,#194018,#194019,#194020,#194021,
#194022,#194023,#194024,#194025,#194026,#194027,#194028,#194029),
 .UNSPECIFIED.,.F.,.F.,(4,3,3,3,3,3,3,3,3,3,3,3,3,3,3,3,3,3,3,3,3,3,3,3,
3,3,3,3,3,3,3,3,3,3,3,3,3,4),(4.87707812168843E-13,0.00106872162737289,
0.00213668903088859,0.00293590036890479,0.0029378487127682,0.00330316625056856,
0.00348679919079069,0.00367043213192709,0.00367231089096026,0.00440496389379973,
0.0044067730691523,0.00587402741748767,0.0058756974255364,0.00881215446495341,
0.00881354613830458,0.00917942034579961,0.00936305328639039,0.00945486975663566,
0.00950077799173426,0.00954668622681246,0.00954800831649663,0.0102812179886621,
0.0102824704946887,0.0117502815123831,0.0117513948510728,0.0146884085598291,
0.0146892435638409,0.0154229402826017,0.015790206158568,0.0159738391130884,
0.0160656555960944,0.0161115638392354,0.016157472083545,0.016158167920225,
0.0176265356072484,0.0176270922766091,0.0205649409893773,0.0235027897021455),
 .UNSPECIFIED.);
#5496=B_SPLINE_CURVE_WITH_KNOTS('',3,(#194032,#194033,#194034,#194035,#194036,
#194037,#194038,#194039,#194040,#194041,#194042),.UNSPECIFIED.,.F.,.F.,
(4,1,2,2,2,4),(0.,0.500000000000001,0.750000000000002,0.875000000000003,
0.984375000000001,1.),.UNSPECIFIED.);
#5497=B_SPLINE_CURVE_WITH_KNOTS('',3,(#194058,#194059,#194060,#194061),
 .UNSPECIFIED.,.F.,.F.,(4,4),(0.,1.),.UNSPECIFIED.);
#5498=B_SPLINE_CURVE_WITH_KNOTS('',3,(#194062,#194063,#194064,#194065),
 .UNSPECIFIED.,.F.,.F.,(4,4),(0.,0.000322395538615397),.UNSPECIFIED.);
#5499=B_SPLINE_CURVE_WITH_KNOTS('',3,(#194164,#194165,#194166,#194167,#194168,
#194169,#194170,#194171,#194172,#194173,#194174,#194175,#194176,#194177,
#194178,#194179,#194180,#194181,#194182,#194183,#194184,#194185,#194186,
#194187,#194188,#194189),.UNSPECIFIED.,.F.,.F.,(4,2,2,2,2,2,2,2,2,2,2,2,
4),(0.,0.125000000000001,0.156250000000001,0.187500000000002,0.250000000000001,
0.375000000000001,0.5,0.562500000000001,0.625,0.75,0.8125,0.875,1.),
 .UNSPECIFIED.);
#5500=B_SPLINE_CURVE_WITH_KNOTS('',3,(#194190,#194191,#194192,#194193,#194194,
#194195,#194196,#194197,#194198,#194199,#194200,#194201,#194202,#194203,
#194204,#194205,#194206,#194207,#194208,#194209,#194210,#194211,#194212,
#194213,#194214,#194215,#194216,#194217,#194218,#194219,#194220,#194221,
#194222,#194223,#194224,#194225,#194226),.UNSPECIFIED.,.F.,.F.,(4,3,3,3,
3,3,3,3,3,3,3,3,4),(0.,0.000191440270420746,0.000287160692730017,0.000382881236840892,
0.000574322481675384,0.000670043078002301,0.00076576358733981,0.000957204470373581,
0.00114864534416313,0.00124436578623716,0.00129222601008214,0.00134008623637552,
0.00153152717467962),.UNSPECIFIED.);
#5501=B_SPLINE_CURVE_WITH_KNOTS('',3,(#194266,#194267,#194268,#194269,#194270,
#194271,#194272,#194273,#194274,#194275,#194276,#194277,#194278,#194279,
#194280,#194281,#194282,#194283,#194284,#194285,#194286,#194287,#194288,
#194289,#194290,#194291,#194292,#194293,#194294,#194295,#194296,#194297,
#194298,#194299,#194300,#194301,#194302,#194303,#194304,#194305,#194306,
#194307,#194308,#194309,#194310,#194311,#194312,#194313,#194314,#194315,
#194316,#194317,#194318,#194319,#194320,#194321,#194322,#194323,#194324,
#194325,#194326,#194327,#194328,#194329,#194330,#194331,#194332,#194333,
#194334,#194335,#194336,#194337,#194338,#194339,#194340,#194341,#194342,
#194343,#194344,#194345,#194346,#194347),.UNSPECIFIED.,.F.,.F.,(4,3,3,3,
3,3,3,3,3,3,3,3,3,3,3,3,3,3,3,3,3,3,3,3,3,3,3,4),(0.,0.0401050357347157,
0.0812206026238641,0.123882732875838,0.167390541414787,0.212077250701923,
0.238079056359111,0.25,0.292319902552325,0.336625084595829,0.374999999999999,
0.420046787969305,0.466533956719877,0.495505970383118,0.5,0.545041357418745,
0.590377250465255,0.63449200813962,0.677383348177903,0.718184700217024,
0.75,0.756613713052315,0.8004091838459,0.84325569019173,0.884513955801954,
0.924879177580128,0.963805079356448,1.),.UNSPECIFIED.);
#5502=B_SPLINE_CURVE_WITH_KNOTS('',3,(#194348,#194349,#194350,#194351,#194352,
#194353,#194354,#194355,#194356,#194357,#194358,#194359,#194360,#194361,
#194362,#194363,#194364,#194365,#194366),.UNSPECIFIED.,.F.,.F.,(4,3,3,3,
3,3,4),(0.,0.00503761689939749,0.00646885457540687,0.0129377091508137,0.0161721364385172,
0.0194065637262206,0.0258754183016275),.UNSPECIFIED.);
#5503=B_SPLINE_CURVE_WITH_KNOTS('',3,(#194472,#194473,#194474,#194475,#194476,
#194477,#194478,#194479,#194480,#194481,#194482,#194483,#194484,#194485,
#194486,#194487,#194488,#194489,#194490,#194491,#194492,#194493,#194494,
#194495,#194496,#194497,#194498,#194499,#194500,#194501,#194502,#194503,
#194504,#194505),.UNSPECIFIED.,.F.,.F.,(4,2,2,2,2,2,2,2,2,2,2,2,2,2,2,2,
4),(0.,0.125000000000002,0.187500000000001,0.250000000000001,0.3125,0.375,
0.4375,0.500000000000001,0.5625,0.625,0.6875,0.75,0.8125,0.84375,0.875,
0.9375,1.),.UNSPECIFIED.);
#5504=B_SPLINE_CURVE_WITH_KNOTS('',3,(#194506,#194507,#194508,#194509,#194510,
#194511,#194512,#194513,#194514,#194515,#194516,#194517,#194518,#194519,
#194520,#194521,#194522,#194523,#194524,#194525,#194526,#194527,#194528,
#194529,#194530,#194531,#194532,#194533,#194534,#194535,#194536,#194537,
#194538,#194539,#194540,#194541,#194542,#194543,#194544,#194545,#194546,
#194547,#194548,#194549,#194550,#194551,#194552,#194553,#194554),
 .UNSPECIFIED.,.F.,.F.,(4,3,3,3,3,3,3,3,3,3,3,3,3,3,3,3,4),(0.,0.000127303360486361,
0.000254607331807631,0.000318259502487228,0.000381911773022019,0.000509216543183179,
0.000636521501341121,0.000763826506543775,0.000891131417838548,0.00101843609427484,
0.00114573874978534,0.00127303875321421,0.00140033769575051,0.00152763716845166,
0.00165493876244132,0.00178224406910835,0.00203687218854967),
 .UNSPECIFIED.);
#5505=B_SPLINE_CURVE_WITH_KNOTS('',3,(#194587,#194588,#194589,#194590),
 .UNSPECIFIED.,.F.,.F.,(4,4),(0.,1.),.UNSPECIFIED.);
#5506=B_SPLINE_CURVE_WITH_KNOTS('',3,(#194591,#194592,#194593,#194594),
 .UNSPECIFIED.,.F.,.F.,(4,4),(6.93889390390723E-18,0.000463834979289304),
 .UNSPECIFIED.);
#5507=B_SPLINE_CURVE_WITH_KNOTS('',3,(#194911,#194912,#194913,#194914,#194915,
#194916,#194917,#194918,#194919,#194920,#194921,#194922,#194923,#194924,
#194925,#194926,#194927,#194928,#194929,#194930,#194931,#194932,#194933,
#194934,#194935,#194936,#194937,#194938,#194939,#194940,#194941,#194942,
#194943,#194944,#194945,#194946,#194947,#194948,#194949,#194950,#194951,
#194952,#194953,#194954,#194955,#194956,#194957,#194958,#194959,#194960,
#194961,#194962),.UNSPECIFIED.,.F.,.F.,(4,3,3,3,3,3,3,3,3,3,3,3,3,3,3,3,
3,4),(0.,0.118561059956462,0.193296673546538,0.311563674713324,0.428677054200604,
0.467557845905428,0.500000000000002,0.618691112431543,0.730136570084834,
0.737382224863085,0.750000000000003,0.860639773248037,0.875000000000003,
0.937500000000003,0.968750000000002,0.984375000000001,0.995689543360724,
1.),.UNSPECIFIED.);
#5508=B_SPLINE_CURVE_WITH_KNOTS('',3,(#194964,#194965,#194966,#194967,#194968,
#194969,#194970,#194971,#194972,#194973,#194974,#194975,#194976,#194977,
#194978,#194979,#194980,#194981,#194982,#194983,#194984,#194985,#194986,
#194987,#194988,#194989,#194990,#194991,#194992,#194993,#194994,#194995,
#194996,#194997,#194998,#194999,#195000,#195001,#195002,#195003),
 .UNSPECIFIED.,.F.,.F.,(4,3,3,3,3,3,3,3,3,3,3,3,3,4),(0.,0.00505175093915313,
0.015625000000001,0.0212638638717959,0.031250000000002,0.0625000000000022,
0.125000000000002,0.150960766387526,0.66974837608655,0.929142180936068,
0.937500000000002,0.984375000000001,0.993990629527285,1.),.UNSPECIFIED.);
#5509=B_SPLINE_CURVE_WITH_KNOTS('',3,(#195005,#195006,#195007,#195008,#195009,
#195010,#195011,#195012,#195013,#195014,#195015,#195016,#195017,#195018,
#195019,#195020,#195021,#195022,#195023,#195024,#195025,#195026,#195027,
#195028,#195029,#195030,#195031,#195032,#195033,#195034,#195035,#195036,
#195037,#195038,#195039,#195040,#195041,#195042,#195043,#195044,#195045,
#195046,#195047,#195048),.UNSPECIFIED.,.F.,.F.,(4,2,2,2,2,2,2,2,2,2,2,2,
2,2,2,2,2,2,2,2,2,4),(1.21542793577394E-6,0.000926751404419985,0.0045096865781495,
0.0116755569256177,0.0260072976205485,0.0833342604002824,0.312642111519209,
0.427296037078671,0.484622999858401,0.513286481248267,0.527618221943199,
0.531201157116932,0.534784092290667,0.54194996263813,0.771257813757056,
0.885911739316519,0.943238702096252,0.971902183486115,0.986233924181051,
0.993399794528514,0.996982729702248,1.),.UNSPECIFIED.);
#5510=B_SPLINE_CURVE_WITH_KNOTS('',3,(#195050,#195051,#195052,#195053,#195054,
#195055,#195056,#195057,#195058,#195059,#195060,#195061,#195062,#195063,
#195064,#195065),.UNSPECIFIED.,.F.,.F.,(4,2,2,2,2,2,2,4),(0.,0.00107945262646427,
0.438665331950596,0.65745827161266,0.876251211274724,0.985647681105758,
0.999322239834636,1.),.UNSPECIFIED.);
#5511=B_SPLINE_CURVE_WITH_KNOTS('',3,(#195067,#195068,#195069,#195070,#195071,
#195072,#195073,#195074,#195075,#195076,#195077,#195078,#195079,#195080,
#195081,#195082,#195083,#195084,#195085,#195086,#195087,#195088,#195089,
#195090,#195091,#195092,#195093,#195094,#195095,#195096,#195097,#195098,
#195099,#195100,#195101,#195102,#195103,#195104,#195105,#195106,#195107,
#195108,#195109,#195110,#195111,#195112,#195113,#195114,#195115,#195116,
#195117,#195118,#195119,#195120,#195121,#195122,#195123,#195124,#195125,
#195126,#195127),.UNSPECIFIED.,.F.,.F.,(4,3,3,3,3,3,3,3,3,3,3,3,3,3,3,3,
3,3,3,3,4),(0.,0.00781249999999971,0.0156249999999994,0.0312499999999994,
0.0624999999999994,0.124999999999999,0.249129116160185,0.249999999999999,
0.350754550530283,0.451829475765032,0.497596952377019,0.499999999999999,
0.653289414190925,0.74797126632589,0.749999999999999,0.875,0.9375,0.96875,
0.984375,0.996876914777217,0.999999999247695),.UNSPECIFIED.);
#5512=B_SPLINE_CURVE_WITH_KNOTS('',3,(#195128,#195129,#195130,#195131,#195132,
#195133,#195134,#195135,#195136,#195137,#195138,#195139,#195140,#195141,
#195142,#195143),.UNSPECIFIED.,.F.,.F.,(4,3,3,3,3,4),(0.,0.00802457780095953,
0.0982041616372357,0.278563329309788,0.639281664654894,1.),
 .UNSPECIFIED.);
#5513=B_SPLINE_CURVE_WITH_KNOTS('',3,(#195144,#195145,#195146,#195147,#195148,
#195149,#195150,#195151,#195152,#195153,#195154,#195155,#195156,#195157,
#195158,#195159,#195160,#195161,#195162,#195163,#195164,#195165,#195166,
#195167,#195168,#195169,#195170,#195171,#195172,#195173,#195174,#195175,
#195176,#195177,#195178,#195179,#195180,#195181,#195182,#195183,#195184,
#195185,#195186,#195187,#195188,#195189,#195190,#195191,#195192,#195193,
#195194,#195195,#195196,#195197,#195198,#195199,#195200,#195201,#195202,
#195203,#195204,#195205,#195206,#195207,#195208,#195209,#195210,#195211,
#195212,#195213,#195214,#195215,#195216,#195217,#195218,#195219,#195220,
#195221,#195222,#195223,#195224,#195225,#195226,#195227,#195228,#195229,
#195230,#195231,#195232,#195233,#195234,#195235,#195236,#195237,#195238,
#195239,#195240,#195241,#195242,#195243,#195244,#195245,#195246,#195247,
#195248,#195249,#195250,#195251,#195252,#195253,#195254,#195255,#195256,
#195257,#195258,#195259,#195260,#195261,#195262,#195263,#195264,#195265,
#195266,#195267,#195268,#195269,#195270,#195271,#195272,#195273,#195274,
#195275,#195276,#195277,#195278,#195279,#195280,#195281,#195282,#195283,
#195284,#195285,#195286,#195287,#195288,#195289,#195290,#195291,#195292,
#195293,#195294,#195295,#195296,#195297),.UNSPECIFIED.,.F.,.F.,(4,3,3,3,
3,3,3,3,3,3,3,3,3,3,3,3,3,3,3,3,3,3,3,3,3,3,3,3,3,3,3,3,3,3,3,3,3,3,3,3,
3,3,3,3,3,3,3,3,3,3,3,4),(1.04083408558608E-17,0.00250327328955152,0.00500654657910303,
0.00625818322387879,0.00688400154626667,0.00696222883656844,0.00704045612686793,
0.00719691070746254,0.00750981986865454,0.010013093158206,0.0112647298029818,
0.011577638964179,0.0117340935447715,0.0117732071899202,0.0118123208350694,
0.0118905481253697,0.0125163664477576,0.0137680030925333,0.015019639737309,
0.0175229130268605,0.0175620266720094,0.0176011403171581,0.0176793676074551,
0.0178358221880486,0.0181487313492361,0.0187745496716364,0.0200261863164121,
0.0225294596059636,0.0226076868962739,0.022646800541427,0.0226859141865788,
0.0228423687671764,0.0231552779283514,0.0237810962507394,0.0250327328955151,
0.0275360061850667,0.0281618245074545,0.0283182790880578,0.028396506378356,
0.0284356200235045,0.0284747336686529,0.0287876428298423,0.0300392794746181,
0.0325425527641696,0.0331683710865575,0.0332465983768559,0.0333248256671528,
0.033481280247746,0.0337941894089454,0.0350458260537211,0.0375490993432726,
0.0400523726328241),.UNSPECIFIED.);
#5514=B_SPLINE_CURVE_WITH_KNOTS('',3,(#195313,#195314,#195315,#195316),
 .UNSPECIFIED.,.F.,.F.,(4,4),(0.,1.),.UNSPECIFIED.);
#5515=B_SPLINE_CURVE_WITH_KNOTS('',3,(#195317,#195318,#195319,#195320),
 .UNSPECIFIED.,.F.,.F.,(4,4),(0.,0.000517487663021482),.UNSPECIFIED.);
#5516=B_SPLINE_CURVE_WITH_KNOTS('',3,(#195437,#195438,#195439,#195440,#195441,
#195442,#195443,#195444,#195445,#195446,#195447,#195448,#195449,#195450,
#195451,#195452,#195453,#195454,#195455,#195456,#195457,#195458,#195459,
#195460,#195461,#195462,#195463,#195464,#195465,#195466,#195467,#195468),
 .UNSPECIFIED.,.F.,.F.,(4,2,2,2,2,2,2,2,2,2,2,2,2,2,2,4),(0.,0.0625000000000002,
0.125,0.15625,0.1875,0.25,0.3125,0.375,0.5,0.5625,0.625,0.6875,0.75,0.8125,
0.875,1.),.UNSPECIFIED.);
#5517=B_SPLINE_CURVE_WITH_KNOTS('',3,(#195469,#195470,#195471,#195472,#195473,
#195474,#195475,#195476,#195477,#195478,#195479,#195480,#195481,#195482,
#195483,#195484,#195485,#195486,#195487,#195488,#195489,#195490,#195491,
#195492,#195493,#195494,#195495,#195496,#195497,#195498,#195499,#195500,
#195501,#195502,#195503,#195504,#195505,#195506,#195507,#195508,#195509,
#195510,#195511,#195512,#195513,#195514),.UNSPECIFIED.,.F.,.F.,(4,3,3,3,
3,3,3,3,3,3,3,3,3,3,3,4),(6.93889390390723E-18,0.000249844530040023,0.000374757201987746,
0.000499665804996624,0.00062457208312752,0.000749477780116716,0.000874384639619363,
0.000999294405453595,0.00124911879765638,0.00137403129062446,0.00149894371772633,
0.0016238558811297,0.0016863118021229,0.00174876758300643,0.00187367862553572,
0.00199858881090719),.UNSPECIFIED.);
#5518=B_SPLINE_CURVE_WITH_KNOTS('',3,(#195554,#195555,#195556,#195557,#195558,
#195559,#195560,#195561,#195562,#195563,#195564,#195565,#195566,#195567,
#195568,#195569,#195570,#195571,#195572,#195573,#195574,#195575,#195576,
#195577,#195578,#195579,#195580,#195581,#195582,#195583,#195584,#195585,
#195586,#195587,#195588,#195589,#195590,#195591,#195592,#195593,#195594,
#195595,#195596,#195597,#195598,#195599,#195600,#195601,#195602,#195603,
#195604,#195605,#195606,#195607,#195608,#195609,#195610,#195611,#195612,
#195613,#195614,#195615,#195616,#195617,#195618,#195619,#195620,#195621,
#195622,#195623,#195624,#195625,#195626,#195627,#195628,#195629,#195630,
#195631,#195632,#195633,#195634,#195635,#195636,#195637,#195638,#195639,
#195640,#195641),.UNSPECIFIED.,.F.,.F.,(4,3,3,3,3,3,3,3,3,3,3,3,3,3,3,3,
3,3,3,3,3,3,3,3,3,3,3,3,3,4),(0.,0.0368559176034455,0.0746437033404335,
0.113370738808261,0.153426274720315,0.196061576008915,0.238696877297516,
0.249999999999999,0.291411119211606,0.334741693441388,0.374999999999999,
0.416196373054901,0.458658881793208,0.497478515250967,0.499999999999999,
0.541479495018386,0.583190607592968,0.624892955694726,0.664441000977951,
0.702841807290668,0.739636661690415,0.75,0.759103064710313,0.799902601459033,
0.839924725486378,0.879943544114783,0.917760112553561,0.954791160548494,
0.990723248093471,1.),.UNSPECIFIED.);
#5519=B_SPLINE_CURVE_WITH_KNOTS('',3,(#195642,#195643,#195644,#195645,#195646,
#195647,#195648,#195649,#195650,#195651,#195652,#195653,#195654,#195655,
#195656,#195657,#195658,#195659,#195660,#195661,#195662,#195663),
 .UNSPECIFIED.,.F.,.F.,(4,3,3,3,3,3,3,4),(9.81307786677359E-18,0.00542754419072061,
0.00715193125010651,0.014303862500213,0.0178798281252662,0.0214557937503195,
0.0280312223938407,0.028607725000426),.UNSPECIFIED.);
#5520=B_SPLINE_CURVE_WITH_KNOTS('',3,(#195769,#195770,#195771,#195772,#195773,
#195774,#195775,#195776,#195777,#195778,#195779,#195780,#195781,#195782,
#195783,#195784,#195785,#195786,#195787,#195788,#195789,#195790,#195791,
#195792,#195793,#195794,#195795,#195796,#195797,#195798,#195799,#195800,
#195801,#195802),.UNSPECIFIED.,.F.,.F.,(4,2,2,2,2,2,2,2,2,2,2,2,2,2,2,2,
4),(0.,0.0624999999999985,0.124999999999999,0.187499999999999,0.25,0.312499999999998,
0.374999999999999,0.4375,0.46875,0.499999999999999,0.624999999999999,0.6875,
0.75,0.8125,0.84375,0.875,1.),.UNSPECIFIED.);
#5521=B_SPLINE_CURVE_WITH_KNOTS('',3,(#195803,#195804,#195805,#195806,#195807,
#195808,#195809,#195810,#195811,#195812,#195813,#195814,#195815,#195816,
#195817,#195818,#195819,#195820,#195821,#195822,#195823,#195824,#195825,
#195826,#195827,#195828,#195829,#195830,#195831,#195832,#195833,#195834,
#195835,#195836,#195837,#195838,#195839,#195840,#195841,#195842,#195843,
#195844,#195845,#195846,#195847,#195848,#195849,#195850,#195851),
 .UNSPECIFIED.,.F.,.F.,(4,3,3,3,3,3,3,3,3,3,3,3,3,3,3,3,4),(0.,0.000209907523070278,
0.000262386427442229,0.000314865930148693,0.000419826308247615,0.000524787812645559,
0.000629749598530388,0.000839670635464471,0.000892150044011657,0.000944629442448278,
0.00104958821836654,0.00115454698196066,0.00125950575196963,0.00136446454713245,
0.00146942338618815,0.00157438228787588,0.00167934127092895),
 .UNSPECIFIED.);
#5522=B_SPLINE_CURVE_WITH_KNOTS('',3,(#195884,#195885,#195886,#195887),
 .UNSPECIFIED.,.F.,.F.,(4,4),(0.,0.999999715020008),.UNSPECIFIED.);
#5523=B_SPLINE_CURVE_WITH_KNOTS('',3,(#195888,#195889,#195890,#195891),
 .UNSPECIFIED.,.F.,.F.,(4,4),(3.46944695195361E-18,0.000487799384074577),
 .UNSPECIFIED.);
#5524=B_SPLINE_CURVE_WITH_KNOTS('',3,(#196010,#196011,#196012,#196013,#196014,
#196015,#196016,#196017,#196018,#196019,#196020,#196021,#196022,#196023,
#196024,#196025,#196026,#196027,#196028,#196029,#196030,#196031,#196032,
#196033,#196034,#196035),.UNSPECIFIED.,.F.,.F.,(4,2,2,2,2,2,2,2,2,2,2,2,
4),(0.,0.124999999999997,0.249999999999993,0.374999999999989,0.499999999999999,
0.562499999999991,0.624999999999996,0.749999999999993,0.812499999999998,
0.87499999999999,0.906249999999992,0.937499999999995,1.),.UNSPECIFIED.);
#5525=B_SPLINE_CURVE_WITH_KNOTS('',3,(#196036,#196037,#196038,#196039,#196040,
#196041,#196042,#196043,#196044,#196045,#196046,#196047,#196048,#196049,
#196050,#196051,#196052,#196053,#196054,#196055,#196056,#196057,#196058,
#196059,#196060,#196061),.UNSPECIFIED.,.F.,.F.,(4,2,2,2,2,2,2,2,2,2,2,2,
4),(0.,0.0625000000000051,0.0937500000000081,0.12500000000001,0.187500000000002,
0.250000000000007,0.375000000000004,0.437500000000009,0.500000000000001,
0.625000000000011,0.750000000000007,0.875000000000003,1.),.UNSPECIFIED.);
#5526=B_SPLINE_CURVE_WITH_KNOTS('',3,(#196089,#196090,#196091,#196092,#196093,
#196094,#196095,#196096,#196097,#196098,#196099,#196100,#196101,#196102,
#196103,#196104,#196105,#196106,#196107,#196108,#196109,#196110,#196111,
#196112,#196113,#196114,#196115,#196116,#196117,#196118,#196119,#196120,
#196121),.UNSPECIFIED.,.F.,.F.,(4,2,2,2,2,2,2,2,2,2,2,2,2,2,2,1,4),(0.,
0.125000000000071,0.156250000000092,0.187500000000113,0.250000000000138,
0.312500000000162,0.343750000000175,0.359375000000185,0.375000000000194,
0.406250000000208,0.437500000000221,0.500000000000248,0.562500000000275,
0.570312500000275,0.578125000000274,0.625000000000249,1.),.UNSPECIFIED.);
#5527=B_SPLINE_CURVE_WITH_KNOTS('',3,(#196122,#196123,#196124,#196125,#196126,
#196127,#196128,#196129,#196130,#196131,#196132,#196133,#196134),
 .UNSPECIFIED.,.F.,.F.,(4,3,3,3,4),(6.93889390390723E-18,0.000381255515696972,
0.000469255885429327,0.000705402670132244,0.000942818873534133),
 .UNSPECIFIED.);
#5528=B_SPLINE_CURVE_WITH_KNOTS('',3,(#196149,#196150,#196151,#196152,#196153,
#196154),.UNSPECIFIED.,.F.,.F.,(4,2,4),(0.,0.5,0.999992304477323),
 .UNSPECIFIED.);
#5529=B_SPLINE_CURVE_WITH_KNOTS('',3,(#196156,#196157,#196158,#196159),
 .UNSPECIFIED.,.F.,.F.,(4,4),(0.,1.),.UNSPECIFIED.);
#5530=B_SPLINE_CURVE_WITH_KNOTS('',3,(#196176,#196177,#196178,#196179,#196180,
#196181,#196182,#196183,#196184,#196185),.UNSPECIFIED.,.F.,.F.,(4,3,3,4),
(0.,7.57680559097057E-5,0.000160273670968369,0.000194799519911097),
 .UNSPECIFIED.);
#5531=B_SPLINE_CURVE_WITH_KNOTS('',3,(#196206,#196207,#196208,#196209,#196210,
#196211,#196212,#196213,#196214,#196215,#196216,#196217,#196218,#196219,
#196220,#196221,#196222,#196223,#196224,#196225,#196226,#196227,#196228,
#196229,#196230,#196231,#196232,#196233,#196234,#196235,#196236,#196237,
#196238,#196239,#196240,#196241,#196242,#196243,#196244,#196245,#196246,
#196247,#196248,#196249,#196250,#196251,#196252,#196253,#196254,#196255,
#196256,#196257,#196258,#196259,#196260,#196261,#196262,#196263),
 .UNSPECIFIED.,.F.,.F.,(4,3,3,3,3,3,3,3,3,3,3,3,3,3,3,3,3,3,3,4),(7.10667107881632E-12,
0.0777967911957834,0.155397709641609,0.232815426199448,0.25000000000003,
0.333850548679027,0.389419000752951,0.437500000000041,0.466951073723059,
0.496142061056067,0.500000000000037,0.500265459427049,0.567807557951046,
0.636514506183817,0.707974454992009,0.750000000000018,0.8217273781834,0.894665117182011,
0.968437096835554,0.999990298090105),.UNSPECIFIED.);
#5532=B_SPLINE_CURVE_WITH_KNOTS('',3,(#196668,#196669,#196670,#196671,#196672,
#196673,#196674,#196675,#196676,#196677,#196678,#196679,#196680,#196681,
#196682,#196683,#196684,#196685,#196686,#196687,#196688,#196689,#196690,
#196691,#196692),.UNSPECIFIED.,.F.,.F.,(4,3,3,3,3,3,3,3,4),(2.28823383841608E-11,
0.128993498150867,0.259210238149049,0.390210937649005,0.500000000000001,
0.625000000000001,0.745864344071094,0.872932172035547,1.),.UNSPECIFIED.);
#5533=B_SPLINE_CURVE_WITH_KNOTS('',3,(#196694,#196695,#196696,#196697,#196698,
#196699,#196700,#196701,#196702,#196703,#196704,#196705,#196706,#196707,
#196708,#196709,#196710,#196711,#196712,#196713,#196714,#196715,#196716,
#196717,#196718,#196719,#196720,#196721,#196722,#196723,#196724,#196725,
#196726,#196727,#196728,#196729,#196730,#196731,#196732,#196733,#196734,
#196735,#196736),.UNSPECIFIED.,.F.,.F.,(4,3,3,3,3,3,3,3,3,3,3,3,3,3,4),
(0.,0.125,0.137817678947238,0.307927954228248,0.478038229509258,0.64814850479027,
0.874999999999999,0.968749999999999,0.984374999999999,0.988369053825107,
0.9921875,0.99609375,0.9970703125,0.99853515625,0.999999999623881),
 .UNSPECIFIED.);
#5534=B_SPLINE_CURVE_WITH_KNOTS('',3,(#196738,#196739,#196740,#196741,#196742,
#196743,#196744,#196745,#196746,#196747,#196748,#196749,#196750,#196751,
#196752,#196753,#196754,#196755,#196756,#196757,#196758,#196759,#196760,
#196761,#196762,#196763,#196764,#196765),.UNSPECIFIED.,.F.,.F.,(4,2,2,2,
2,2,2,2,2,2,2,2,2,4),(0.,0.0069548877073492,0.0155193349966718,0.0497771241539778,
0.11829270246859,0.255323859097813,0.529386172356271,0.666417328985494,
0.803448485614717,0.94047964224394,0.974737431401246,0.991866325979906,
0.996148549624567,1.),.UNSPECIFIED.);
#5535=B_SPLINE_CURVE_WITH_KNOTS('',3,(#196767,#196768,#196769,#196770,#196771,
#196772,#196773,#196774,#196775,#196776,#196777,#196778,#196779,#196780,
#196781,#196782,#196783,#196784,#196785,#196786),.UNSPECIFIED.,.F.,.F.,
(4,2,2,2,2,2,2,2,2,4),(0.,0.000334191767478362,0.00697844754728855,0.0601324937857085,
0.485364863693081,0.910597233600454,0.963751279838875,0.990328302958084,
0.996972558737885,1.),.UNSPECIFIED.);
#5536=B_SPLINE_CURVE_WITH_KNOTS('',3,(#196788,#196789,#196790,#196791,#196792,
#196793,#196794,#196795,#196796,#196797,#196798,#196799,#196800,#196801,
#196802,#196803,#196804,#196805,#196806,#196807,#196808,#196809,#196810,
#196811,#196812,#196813,#196814,#196815,#196816),.UNSPECIFIED.,.F.,.F.,
(4,2,2,2,2,2,2,2,2,2,2,2,1,2,4),(0.,0.000388754147012465,0.0047713452534302,
0.0223017096791179,0.162544625084547,0.302787540489991,0.44303045589542,
0.72351628670628,0.863759202111711,0.933880659814438,0.968941388665797,
0.986471753091468,0.995236935304305,0.999619526410721,1.),.UNSPECIFIED.);
#5537=B_SPLINE_CURVE_WITH_KNOTS('',3,(#196818,#196819,#196820,#196821,#196822,
#196823,#196824,#196825,#196826,#196827,#196828,#196829,#196830,#196831,
#196832,#196833,#196834,#196835,#196836,#196837,#196838,#196839,#196840,
#196841,#196842),.UNSPECIFIED.,.F.,.F.,(4,2,1,1,1,2,2,2,2,2,2,1,1,2,4),
(0.,0.00390625000000159,0.0312500000000058,0.0625000000000054,0.125000000000005,
0.250000000000003,0.500000000000001,0.749999999999999,0.874999999999999,
0.937499999999999,0.968749999999998,0.984374999999997,0.992187499999998,
0.996093749999999,1.),.UNSPECIFIED.);
#5538=B_SPLINE_CURVE_WITH_KNOTS('',3,(#196844,#196845,#196846,#196847,#196848,
#196849,#196850,#196851,#196852,#196853,#196854,#196855,#196856,#196857,
#196858,#196859,#196860,#196861,#196862,#196863,#196864,#196865,#196866,
#196867),.UNSPECIFIED.,.F.,.F.,(4,2,1,1,1,1,2,2,2,1,2,2,1,2,4),(0.,0.00390624999999841,
0.00781249999999682,0.015624999999997,0.0312499999999974,0.062499999999997,
0.124999999999999,0.25,0.500000000000001,0.750000000000002,0.937500000000003,
0.968750000000002,0.984375000000001,0.9921875,0.99999999134495),
 .UNSPECIFIED.);
#5539=B_SPLINE_CURVE_WITH_KNOTS('',3,(#196868,#196869,#196870,#196871,#196872,
#196873,#196874,#196875,#196876,#196877,#196878,#196879,#196880,#196881,
#196882,#196883,#196884,#196885,#196886,#196887,#196888,#196889,#196890,
#196891,#196892,#196893,#196894,#196895,#196896,#196897,#196898,#196899,
#196900,#196901,#196902,#196903,#196904,#196905,#196906,#196907,#196908,
#196909,#196910,#196911,#196912,#196913,#196914,#196915,#196916),
 .UNSPECIFIED.,.F.,.F.,(4,3,3,3,3,3,3,3,3,3,3,3,3,3,3,3,4),(1.60377085177131E-7,
0.00257403723325268,0.00390624999999833,0.00781249999999667,0.0136608742270577,
0.0156249999999971,0.0312499999999979,0.0580082231262107,0.146702920920664,
0.324092316509571,0.501481712098478,0.590176409892927,0.678871107687397,
0.8562605032763,0.875000000000001,0.944955187638308,1.),.UNSPECIFIED.);
#5540=B_SPLINE_CURVE_WITH_KNOTS('',3,(#196917,#196918,#196919,#196920,#196921,
#196922,#196923,#196924,#196925,#196926,#196927,#196928,#196929,#196930,
#196931,#196932,#196933,#196934,#196935,#196936,#196937,#196938,#196939,
#196940,#196941,#196942,#196943,#196944,#196945,#196946,#196947,#196948,
#196949,#196950,#196951,#196952,#196953,#196954,#196955,#196956,#196957,
#196958,#196959,#196960,#196961,#196962,#196963,#196964,#196965,#196966,
#196967,#196968,#196969,#196970,#196971,#196972,#196973,#196974,#196975,
#196976,#196977,#196978,#196979,#196980,#196981,#196982,#196983,#196984,
#196985,#196986,#196987,#196988,#196989,#196990,#196991,#196992,#196993,
#196994,#196995,#196996,#196997,#196998,#196999,#197000,#197001,#197002,
#197003,#197004,#197005,#197006,#197007,#197008,#197009,#197010,#197011,
#197012,#197013,#197014,#197015,#197016,#197017,#197018,#197019,#197020,
#197021,#197022,#197023,#197024,#197025,#197026,#197027,#197028,#197029,
#197030,#197031,#197032,#197033,#197034,#197035,#197036,#197037,#197038,
#197039,#197040,#197041,#197042,#197043,#197044,#197045,#197046,#197047,
#197048,#197049,#197050,#197051,#197052,#197053,#197054,#197055,#197056,
#197057,#197058,#197059,#197060,#197061,#197062,#197063,#197064,#197065,
#197066,#197067,#197068,#197069,#197070,#197071,#197072,#197073,#197074,
#197075,#197076,#197077,#197078,#197079,#197080,#197081,#197082,#197083,
#197084,#197085,#197086,#197087,#197088,#197089,#197090,#197091,#197092,
#197093,#197094,#197095,#197096,#197097,#197098,#197099,#197100,#197101,
#197102,#197103,#197104,#197105,#197106,#197107,#197108,#197109,#197110,
#197111,#197112,#197113,#197114,#197115,#197116,#197117,#197118,#197119,
#197120,#197121,#197122,#197123,#197124,#197125,#197126,#197127,#197128,
#197129,#197130,#197131,#197132,#197133,#197134,#197135,#197136,#197137,
#197138,#197139,#197140,#197141,#197142,#197143,#197144,#197145,#197146,
#197147,#197148,#197149,#197150,#197151,#197152,#197153,#197154,#197155,
#197156,#197157,#197158,#197159,#197160,#197161,#197162,#197163,#197164,
#197165,#197166,#197167,#197168,#197169,#197170,#197171,#197172,#197173,
#197174,#197175,#197176,#197177,#197178,#197179,#197180,#197181,#197182,
#197183,#197184,#197185,#197186,#197187,#197188,#197189,#197190,#197191,
#197192,#197193,#197194,#197195,#197196,#197197,#197198,#197199,#197200,
#197201,#197202,#197203,#197204,#197205,#197206,#197207,#197208,#197209,
#197210,#197211,#197212,#197213,#197214,#197215,#197216,#197217,#197218,
#197219,#197220,#197221,#197222,#197223,#197224,#197225,#197226,#197227,
#197228,#197229,#197230,#197231,#197232,#197233,#197234,#197235,#197236,
#197237,#197238,#197239,#197240,#197241,#197242,#197243,#197244,#197245,
#197246,#197247,#197248,#197249,#197250,#197251,#197252,#197253,#197254,
#197255,#197256,#197257,#197258,#197259,#197260,#197261,#197262,#197263,
#197264,#197265,#197266,#197267,#197268),.UNSPECIFIED.,.F.,.F.,(4,3,3,3,
3,3,3,3,3,3,3,3,3,3,3,3,3,3,3,3,3,3,3,3,3,3,3,3,3,3,3,3,3,3,3,3,3,3,3,3,
3,3,3,3,3,3,3,3,3,3,3,3,3,3,3,3,3,3,3,3,3,3,3,3,3,3,3,3,3,3,3,3,3,3,3,3,
3,3,3,3,3,3,3,3,3,3,3,3,3,3,3,3,3,3,3,3,3,3,3,3,3,3,3,3,3,3,3,3,3,3,3,3,
3,3,3,3,3,4),(0.,0.000458642979612002,0.00148039975907437,0.00155548413886127,
0.00215808125410714,0.00351929604547634,0.00375138748260762,0.00431616250821427,
0.00485043313466948,0.00595000606436429,0.00647424376232141,0.00814921412206644,
0.00863232501642855,0.0103483019189537,0.0107904062705357,0.0114478221282345,
0.0118694468975892,0.0119975520112361,0.0121349909920248,0.0121693507398585,
0.0122037104862784,0.0122724299699395,0.012408967211116,0.0125473080812304,
0.0129484875246428,0.0164016794277588,0.0169452741711578,0.0172646500328571,
0.0191441895986679,0.0194227312869643,0.0196939101106087,0.0198313397462589,
0.0198485184451409,0.0198656971433598,0.019900054538499,0.0199622516004911,
0.0199687693285922,0.0202436289341201,0.0205017719140178,0.0213430827748702,
0.0215808125410714,0.0236608084713611,0.0257408044016508,0.0258969750492855,
0.027059011742913,0.0280550563033925,0.0289136017549235,0.0291340969304461,
0.0301383324656715,0.0301726862499191,0.0302070399948121,0.0302131375574996,
0.0302757474855599,0.0304131631667517,0.0306879973674717,0.0312376772927355,
0.0323370846027418,0.0345293000657137,0.0345360999801471,0.0356083406927672,
0.0356357138934573,0.0366115735239252,0.0366873813198207,0.036735364064563,
0.0376935360434091,0.0377664219468742,0.037834874245495,0.03797230394085,
0.0380066611974582,0.0380410184323685,0.0381097329274824,0.038305942260401,
0.0383845939060418,0.0388454625739277,0.0389343227662998,0.0416287480698856,
0.0431616250821419,0.0433319227699236,0.0455053529354623,0.0474777875903559,
0.0477291370890009,0.0480173079038827,0.0482787598919225,0.0483474623355813,
0.048381813564519,0.0484161648055658,0.0485535700013955,0.0485568282174095,
0.0488283820820523,0.049635868844463,0.0499276530066707,0.0510269469116911,
0.05179395009857,0.0521261923582727,0.054324468909372,0.0554235143696246,
0.0559730160990559,0.056110112606784,0.0562477622140428,0.0563164484206554,
0.0563851344750846,0.0565225060213207,0.0566496329203107,0.0571891532338374,
0.0582681938608909,0.0599454964430044,0.0604262751149979,0.0609187453906406,
0.0623709320634497,0.0625843563691049,0.0631171315120633,0.0647424376232119,
0.065315179230263,0.0669005188773189,0.0675129021160854,0.0679795595043724,
0.068863383040997,0.0690586001314259),.UNSPECIFIED.);
#5541=B_SPLINE_CURVE_WITH_KNOTS('',3,(#197289,#197290,#197291,#197292,#197293,
#197294,#197295,#197296,#197297,#197298,#197299,#197300,#197301,#197302),
 .UNSPECIFIED.,.F.,.F.,(4,2,2,1,1,2,2,4),(0.,0.249999999999831,0.374999999999745,
0.437499999999717,0.468749999999702,0.484374999999696,0.49999999999969,
0.999968793306949),.UNSPECIFIED.);
#5542=B_SPLINE_CURVE_WITH_KNOTS('',3,(#197318,#197319,#197320,#197321,#197322,
#197323,#197324),.UNSPECIFIED.,.F.,.F.,(4,3,4),(3.39934988877629E-17,8.80333896086783E-5,
0.000139297820505393),.UNSPECIFIED.);
#5543=B_SPLINE_CURVE_WITH_KNOTS('',3,(#197325,#197326,#197327,#197328),
 .UNSPECIFIED.,.F.,.F.,(4,4),(1.05519109601004E-16,0.000332772401868219),
 .UNSPECIFIED.);
#5544=B_SPLINE_CURVE_WITH_KNOTS('',3,(#197367,#197368,#197369,#197370,#197371,
#197372),.UNSPECIFIED.,.F.,.F.,(4,2,4),(0.,0.5,1.),.UNSPECIFIED.);
#5545=B_SPLINE_CURVE_WITH_KNOTS('',3,(#197373,#197374,#197375,#197376,#197377,
#197378,#197379),.UNSPECIFIED.,.F.,.F.,(4,3,4),(0.,0.000376539260809641,
0.00075440118473929),.UNSPECIFIED.);
#5546=B_SPLINE_CURVE_WITH_KNOTS('',3,(#197461,#197462,#197463,#197464,#197465,
#197466,#197467,#197468,#197469,#197470,#197471,#197472,#197473,#197474,
#197475,#197476,#197477,#197478,#197479,#197480,#197481,#197482,#197483,
#197484,#197485,#197486,#197487,#197488,#197489,#197490,#197491,#197492,
#197493,#197494,#197495,#197496,#197497,#197498,#197499,#197500,#197501,
#197502,#197503,#197504,#197505,#197506,#197507,#197508,#197509,#197510,
#197511,#197512,#197513,#197514,#197515,#197516,#197517,#197518,#197519,
#197520,#197521,#197522,#197523,#197524,#197525,#197526,#197527,#197528,
#197529,#197530,#197531,#197532,#197533,#197534,#197535,#197536,#197537,
#197538,#197539,#197540,#197541,#197542,#197543,#197544,#197545,#197546,
#197547,#197548,#197549,#197550,#197551,#197552,#197553,#197554,#197555,
#197556,#197557,#197558,#197559,#197560,#197561,#197562,#197563,#197564,
#197565,#197566,#197567,#197568,#197569,#197570,#197571,#197572,#197573,
#197574,#197575,#197576,#197577,#197578,#197579,#197580,#197581,#197582,
#197583,#197584,#197585,#197586,#197587,#197588,#197589,#197590,#197591,
#197592,#197593),.UNSPECIFIED.,.F.,.F.,(4,3,3,3,3,3,3,3,3,3,3,3,3,3,3,3,
3,3,3,3,3,3,3,3,3,3,3,3,3,3,3,3,3,3,3,3,3,3,3,3,3,3,3,3,4),(0.,0.0202204421099624,
0.0395451483058804,0.0582377862400879,0.0624999999999951,0.0875613665156572,
0.0937499999999927,0.105792877064545,0.119535285750553,0.124999999999989,
0.143266369710153,0.160852989255863,0.177878328056101,0.187499999999999,
0.216630220683948,0.233848186590877,0.249999999999994,0.270617506030971,
0.292475272788992,0.316626262912307,0.342458186784713,0.370975671115348,
0.374999999999997,0.399246099196213,0.403095241035769,0.429234253193885,
0.437499999999992,0.476973357033904,0.5,0.544412193223352,0.580280434548985,
0.62499999999999,0.668486704216791,0.711205001631657,0.749999999999993,
0.753891896102902,0.789218995972688,0.826185861752328,0.861325504709182,
0.874999999999997,0.910862553258451,0.928894079945525,0.964447039972762,
0.99809894552016,1.),.UNSPECIFIED.);
#5547=B_SPLINE_CURVE_WITH_KNOTS('',3,(#197594,#197595,#197596,#197597,#197598,
#197599,#197600,#197601,#197602,#197603,#197604,#197605,#197606,#197607,
#197608,#197609,#197610,#197611,#197612,#197613,#197614,#197615,#197616,
#197617,#197618,#197619),.UNSPECIFIED.,.F.,.F.,(4,2,2,2,2,2,2,2,2,2,2,2,
4),(0.,0.125000000000003,0.250000000000007,0.37500000000001,0.5,0.562500000000008,
0.625000000000003,0.750000000000007,0.812500000000001,0.875000000000011,
0.906250000000007,0.937500000000005,1.),.UNSPECIFIED.);
#5548=B_SPLINE_CURVE_WITH_KNOTS('',3,(#197650,#197651,#197652,#197653),
 .UNSPECIFIED.,.F.,.F.,(4,4),(0.,1.),.UNSPECIFIED.);
#5549=B_SPLINE_CURVE_WITH_KNOTS('',3,(#197670,#197671,#197672,#197673,#197674,
#197675,#197676,#197677,#197678,#197679,#197680,#197681,#197682,#197683,
#197684,#197685,#197686,#197687,#197688),.UNSPECIFIED.,.F.,.F.,(4,3,3,3,
3,3,4),(0.,0.185533700348248,0.389150275261186,0.586067466801276,0.777142226369554,
0.956993746407619,1.),.UNSPECIFIED.);
#5550=B_SPLINE_CURVE_WITH_KNOTS('',3,(#197689,#197690,#197691,#197692,#197693,
#197694,#197695,#197696,#197697,#197698,#197699,#197700,#197701,#197702,
#197703,#197704,#197705,#197706,#197707,#197708,#197709,#197710,#197711,
#197712,#197713,#197714,#197715,#197716,#197717,#197718,#197719,#197720,
#197721,#197722,#197723,#197724,#197725,#197726,#197727,#197728,#197729,
#197730,#197731,#197732,#197733,#197734),.UNSPECIFIED.,.F.,.F.,(4,3,3,3,
3,3,3,3,3,3,3,3,3,3,3,4),(3.82465140600628E-12,0.080165926001864,0.159888411076935,
0.238758088141874,0.25,0.3272825015128,0.40328844376453,0.47787089026108,
0.550149874260245,0.621091964466054,0.689969931524664,0.75,0.815939883785364,
0.880799348024208,0.944115505909337,1.),.UNSPECIFIED.);
#5551=B_SPLINE_CURVE_WITH_KNOTS('',3,(#197802,#197803,#197804,#197805,#197806,
#197807,#197808,#197809,#197810,#197811),.UNSPECIFIED.,.F.,.F.,(4,2,2,2,
4),(0.,0.25,0.5,0.75,1.),.UNSPECIFIED.);
#5552=B_SPLINE_CURVE_WITH_KNOTS('',3,(#197812,#197813,#197814,#197815,#197816,
#197817,#197818,#197819,#197820,#197821,#197822,#197823,#197824),
 .UNSPECIFIED.,.F.,.F.,(4,3,3,3,4),(0.,0.000262347006055043,0.000525082323798981,
0.000788127838504804,0.00105144790336124),.UNSPECIFIED.);
#5553=B_SPLINE_CURVE_WITH_KNOTS('',3,(#197906,#197907,#197908,#197909,#197910,
#197911,#197912,#197913,#197914,#197915,#197916,#197917,#197918,#197919,
#197920,#197921,#197922,#197923,#197924,#197925,#197926,#197927,#197928,
#197929,#197930,#197931),.UNSPECIFIED.,.F.,.F.,(4,2,2,2,2,2,2,2,2,2,2,2,
4),(0.,0.0624999999999995,0.0937500000000063,0.124999999999998,0.187499999999997,
0.249999999999997,0.374999999999995,0.437499999999993,0.499999999999993,
0.624999999999991,0.749999999999989,0.874999999999988,1.),.UNSPECIFIED.);
#5554=B_SPLINE_CURVE_WITH_KNOTS('',3,(#197932,#197933,#197934,#197935,#197936,
#197937,#197938,#197939,#197940,#197941,#197942,#197943,#197944,#197945,
#197946,#197947,#197948,#197949,#197950,#197951,#197952,#197953,#197954,
#197955,#197956,#197957),.UNSPECIFIED.,.F.,.F.,(4,2,2,2,2,2,2,2,2,2,2,2,
4),(0.,0.125000000000012,0.250000000000011,0.375000000000009,0.500000000000007,
0.562500000000007,0.625000000000005,0.750000000000003,0.812500000000003,
0.875000000000002,0.906249999999994,0.937500000000001,1.),.UNSPECIFIED.);
#5555=B_SPLINE_CURVE_WITH_KNOTS('',3,(#197973,#197974,#197975,#197976,#197977,
#197978,#197979,#197980,#197981,#197982),.UNSPECIFIED.,.F.,.F.,(4,3,3,4),
(0.,0.000342739114726225,0.000689887212155792,0.000728014676542687),
 .UNSPECIFIED.);
#5556=B_SPLINE_CURVE_WITH_KNOTS('',3,(#197997,#197998,#197999,#198000),
 .UNSPECIFIED.,.F.,.F.,(4,4),(0.,1.),.UNSPECIFIED.);
#5557=B_SPLINE_CURVE_WITH_KNOTS('',3,(#198198,#198199,#198200,#198201,#198202,
#198203,#198204,#198205,#198206,#198207,#198208,#198209,#198210,#198211,
#198212,#198213,#198214,#198215,#198216,#198217,#198218,#198219,#198220),
 .UNSPECIFIED.,.F.,.F.,(4,2,1,2,2,2,2,2,2,2,2,4),(0.,0.00283826710419251,
0.00633276476528107,0.0133217600874583,0.0412777413761679,0.0971897039535873,
0.209013629108426,0.432661479418103,0.879957180037457,0.991781105192296,
0.998770100514473,0.99999981607236),.UNSPECIFIED.);
#5558=B_SPLINE_CURVE_WITH_KNOTS('',3,(#198222,#198223,#198224,#198225,#198226,
#198227,#198228,#198229,#198230,#198231,#198232,#198233,#198234,#198235,
#198236,#198237,#198238,#198239,#198240,#198241,#198242,#198243,#198244,
#198245,#198246,#198247,#198248,#198249,#198250,#198251,#198252,#198253,
#198254,#198255),.UNSPECIFIED.,.F.,.F.,(4,3,3,3,3,3,3,3,3,3,3,4),(0.,0.00620530037449982,
0.0212662809590181,0.0513882421280549,0.11163216446613,0.352607853818434,
0.834559232523038,0.955047077199191,0.985169038368228,0.992699528660487,
0.996464773806616,1.),.UNSPECIFIED.);
#5559=B_SPLINE_CURVE_WITH_KNOTS('',3,(#198257,#198258,#198259,#198260,#198261,
#198262,#198263,#198264,#198265,#198266,#198267,#198268,#198269,#198270,
#198271,#198272,#198273,#198274),.UNSPECIFIED.,.F.,.F.,(4,2,2,2,2,2,2,2,
4),(1.98733438466738E-7,0.000182929632426367,0.0121606367275007,0.0600714651078031,
0.251714778628998,0.443358092150197,0.539179748910797,0.635001405671392,
1.),.UNSPECIFIED.);
#5560=B_SPLINE_CURVE_WITH_KNOTS('',3,(#198276,#198277,#198278,#198279,#198280,
#198281,#198282,#198283,#198284,#198285,#198286,#198287,#198288,#198289,
#198290,#198291,#198292,#198293,#198294,#198295,#198296,#198297,#198298,
#198299,#198300,#198301,#198302,#198303),.UNSPECIFIED.,.F.,.F.,(4,3,3,3,
3,3,3,3,3,4),(0.,0.117306771483226,0.234396839308952,0.351440364191732,
0.468658786203015,0.5,0.625,0.748613077229995,0.874306538614997,1.),
 .UNSPECIFIED.);
#5561=B_SPLINE_CURVE_WITH_KNOTS('',3,(#198304,#198305,#198306,#198307,#198308,
#198309,#198310,#198311,#198312,#198313,#198314,#198315,#198316,#198317,
#198318,#198319,#198320,#198321,#198322,#198323,#198324,#198325,#198326,
#198327,#198328,#198329,#198330,#198331,#198332,#198333,#198334,#198335,
#198336,#198337,#198338,#198339,#198340,#198341,#198342,#198343,#198344,
#198345,#198346,#198347,#198348,#198349,#198350,#198351,#198352,#198353,
#198354,#198355,#198356,#198357,#198358,#198359,#198360,#198361,#198362,
#198363,#198364,#198365,#198366,#198367,#198368,#198369,#198370,#198371,
#198372,#198373,#198374,#198375,#198376,#198377,#198378,#198379,#198380,
#198381,#198382,#198383,#198384,#198385,#198386,#198387,#198388,#198389,
#198390,#198391,#198392,#198393,#198394,#198395,#198396,#198397,#198398,
#198399,#198400,#198401,#198402,#198403,#198404,#198405,#198406,#198407,
#198408,#198409,#198410,#198411,#198412,#198413,#198414,#198415,#198416,
#198417,#198418,#198419,#198420,#198421,#198422,#198423,#198424,#198425,
#198426,#198427,#198428,#198429,#198430,#198431,#198432,#198433,#198434,
#198435,#198436,#198437,#198438,#198439,#198440,#198441,#198442,#198443,
#198444,#198445,#198446,#198447,#198448,#198449,#198450,#198451,#198452,
#198453,#198454,#198455,#198456,#198457,#198458,#198459,#198460,#198461,
#198462,#198463,#198464,#198465,#198466,#198467,#198468,#198469),
 .UNSPECIFIED.,.F.,.F.,(4,3,3,3,3,3,3,3,3,3,3,3,3,3,3,3,3,3,3,3,3,3,3,3,
3,3,3,3,3,3,3,3,3,3,3,3,3,3,3,3,3,3,3,3,3,3,3,3,3,3,3,3,3,3,3,4),(3.0340749909216E-15,
0.00129418773529668,0.00218682165402767,0.00327794725358747,0.00398945644969675,
0.00437364330805532,0.00509766529618652,0.00620616680139718,0.0079538318987134,
0.00842283797271616,0.00874728661611061,0.0106381507815725,0.0109341082701383,
0.0111918496720615,0.011330267843016,0.0113648723663157,0.0113994769397398,
0.0114686863527641,0.0114808136836452,0.0117455395577677,0.0120275190971521,
0.0128530198691994,0.0131209299241659,0.0165925219296371,0.0172816770907989,
0.0174945732322213,0.0194950733089173,0.019681394886249,0.0200483162030301,
0.0202281002997558,0.0203249209658281,0.0204632190439244,0.0205323676346262,
0.0206015162605049,0.0207748057132628,0.0217079731878835,0.0218682165402766,
0.0241483525471447,0.026134520310489,0.0262418598483319,0.0275481788415811,
0.0283480821017152,0.0284286815023595,0.0293305776083927,0.0294547291211144,
0.0295220923293734,0.0300079248057878,0.0300687977428803,0.0302844849745068,
0.0303536218586848,0.0303881901705513,0.0304227584828617,0.0305610330454479,
0.0306155031563872,0.0335427501364283,0.0349891464644424),.UNSPECIFIED.);
#5562=B_SPLINE_CURVE_WITH_KNOTS('',3,(#198470,#198471,#198472,#198473,#198474,
#198475,#198476,#198477,#198478,#198479),.UNSPECIFIED.,.F.,.F.,(4,2,2,2,
4),(4.18095462764722E-18,0.00255445063423646,0.00383167595135469,0.00447028860991381,
0.00510890126847292),.UNSPECIFIED.);
#5563=B_SPLINE_CURVE_WITH_KNOTS('',3,(#198499,#198500,#198501,#198502,#198503,
#198504,#198505,#198506,#198507,#198508,#198509,#198510,#198511,#198512,
#198513,#198514,#198515,#198516,#198517,#198518,#198519,#198520,#198521,
#198522,#198523,#198524,#198525,#198526,#198527,#198528,#198529),
 .UNSPECIFIED.,.F.,.F.,(4,3,3,3,3,3,3,3,3,3,4),(0.,0.124999999999992,0.249999999999984,
0.374999999999976,0.426911475280936,0.479016552299178,0.499999999999968,
0.624999999999976,0.749774040198044,0.874887020099022,1.),.UNSPECIFIED.);
#5564=B_SPLINE_CURVE_WITH_KNOTS('',3,(#198566,#198567,#198568,#198569,#198570,
#198571,#198572),.UNSPECIFIED.,.F.,.F.,(4,3,4),(0.,5.20100073045258E-5,
8.99378298105574E-5),.UNSPECIFIED.);
#5565=B_SPLINE_CURVE_WITH_KNOTS('',3,(#198607,#198608,#198609,#198610,#198611,
#198612,#198613,#198614,#198615,#198616,#198617,#198618,#198619),
 .UNSPECIFIED.,.F.,.F.,(4,3,3,3,4),(1.38777878078145E-17,0.000218644279498117,
0.000437193341875465,0.000655638180355839,0.000873969830693171),
 .UNSPECIFIED.);
#5566=B_SPLINE_CURVE_WITH_KNOTS('',3,(#198620,#198621,#198622,#198623,#198624,
#198625,#198626,#198627,#198628,#198629,#198630,#198631,#198632,#198633,
#198634,#198635,#198636,#198637,#198638,#198639,#198640,#198641,#198642,
#198643,#198644,#198645,#198646,#198647,#198648,#198649,#198650,#198651,
#198652,#198653,#198654,#198655,#198656,#198657,#198658,#198659,#198660,
#198661,#198662,#198663,#198664,#198665,#198666,#198667,#198668,#198669,
#198670,#198671,#198672,#198673,#198674,#198675,#198676,#198677,#198678,
#198679,#198680,#198681,#198682,#198683,#198684,#198685,#198686,#198687,
#198688,#198689,#198690,#198691,#198692,#198693,#198694,#198695,#198696,
#198697,#198698,#198699,#198700,#198701),.UNSPECIFIED.,.F.,.F.,(4,3,3,3,
3,3,3,3,3,3,3,3,3,3,3,3,3,3,3,3,3,3,3,3,3,3,3,4),(0.,0.0518784908944668,
0.0929898358507259,0.12499999999993,0.159020278629369,0.187499999999899,
0.234066953854059,0.249999999999868,0.258856206327037,0.281249999999866,
0.289062499999863,0.296874999999861,0.312499999999857,0.345889511569537,
0.374999999999793,0.406249999999761,0.421874999999748,0.427424553674678,
0.429687499999741,0.437499999999734,0.496169719132871,0.49999999999976,
0.531650206071813,0.562499999999787,0.578124999999789,0.749999999999881,
0.75959960473149,1.),.UNSPECIFIED.);
#5567=B_SPLINE_CURVE_WITH_KNOTS('',3,(#198785,#198786,#198787,#198788,#198789,
#198790,#198791,#198792,#198793,#198794,#198795,#198796,#198797,#198798,
#198799,#198800,#198801,#198802,#198803,#198804,#198805,#198806,#198807,
#198808,#198809,#198810,#198811,#198812,#198813,#198814,#198815,#198816,
#198817,#198818,#198819,#198820,#198821,#198822,#198823,#198824,#198825,
#198826,#198827,#198828,#198829,#198830,#198831,#198832,#198833,#198834,
#198835,#198836,#198837,#198838,#198839,#198840,#198841,#198842,#198843,
#198844,#198845,#198846,#198847,#198848,#198849,#198850,#198851,#198852,
#198853,#198854,#198855,#198856,#198857,#198858,#198859,#198860,#198861,
#198862,#198863,#198864,#198865,#198866,#198867,#198868,#198869,#198870,
#198871,#198872,#198873,#198874,#198875,#198876,#198877,#198878,#198879,
#198880,#198881,#198882,#198883,#198884,#198885,#198886,#198887,#198888,
#198889,#198890,#198891,#198892,#198893,#198894,#198895,#198896,#198897,
#198898,#198899,#198900,#198901,#198902,#198903,#198904,#198905,#198906,
#198907,#198908,#198909,#198910,#198911),.UNSPECIFIED.,.F.,.F.,(4,3,3,3,
3,3,3,3,3,3,3,3,3,3,3,3,3,3,3,3,3,3,3,3,3,3,3,3,3,3,3,3,3,3,3,3,3,3,3,3,
3,3,4),(0.,0.00781250000000299,0.0148064814531594,0.015625000000006,0.031250000000012,
0.0502697957749594,0.0625000000000225,0.0828125223056203,0.0864099718511293,
0.107941083662414,0.130513449180188,0.15512947215691,0.18135251250197,0.21073819198987,
0.21360810907109,0.250000000000073,0.281250000000074,0.305550632363911,
0.312500000000075,0.35152559275442,0.390681933501771,0.429805112351713,
0.44018428138064,0.46498154374185,0.487905034853124,0.509922052039041,0.530846691221498,
0.539373330825481,0.551742955240353,0.562500000000056,0.570312500000056,
0.574429310563791,0.578125000000056,0.57886137870164,0.593750000000054,
0.625000000000051,0.638851379824668,0.725746931047932,0.759003379547896,
0.82678271683287,0.879385809313665,0.93750000000001,1.),.UNSPECIFIED.);
#5568=B_SPLINE_CURVE_WITH_KNOTS('',3,(#198945,#198946,#198947,#198948),
 .UNSPECIFIED.,.F.,.F.,(4,4),(0.,0.999997872858114),.UNSPECIFIED.);
#5569=B_SPLINE_CURVE_WITH_KNOTS('',3,(#198967,#198968,#198969,#198970,#198971,
#198972,#198973,#198974,#198975,#198976,#198977,#198978,#198979,#198980,
#198981,#198982,#198983,#198984,#198985,#198986,#198987,#198988),
 .UNSPECIFIED.,.F.,.F.,(4,3,3,3,3,3,3,4),(0.,0.163501572963403,0.330250786373319,
0.496999999783234,0.657493800287202,0.817444914178316,0.976787577632667,
1.),.UNSPECIFIED.);
#5570=B_SPLINE_CURVE_WITH_KNOTS('',3,(#198989,#198990,#198991,#198992,#198993,
#198994,#198995),.UNSPECIFIED.,.F.,.F.,(4,3,4),(0.00166725821467356,0.0142672384485507,
0.0264527075460118),.UNSPECIFIED.);
#5571=B_SPLINE_CURVE_WITH_KNOTS('',3,(#199008,#199009,#199010,#199011),
 .UNSPECIFIED.,.F.,.F.,(4,4),(0.,1.),.UNSPECIFIED.);
#5572=B_SPLINE_CURVE_WITH_KNOTS('',3,(#199012,#199013,#199014,#199015,#199016,
#199017,#199018,#199019,#199020,#199021,#199022,#199023,#199024,#199025,
#199026,#199027,#199028,#199029,#199030,#199031,#199032,#199033,#199034,
#199035,#199036),.UNSPECIFIED.,.F.,.F.,(4,3,3,3,3,3,3,3,4),(0.,0.136592041997272,
0.273213474352422,0.40987042422622,0.546568921813974,0.683339210013659,
0.820155615618192,0.957042445426518,1.),.UNSPECIFIED.);
#5573=B_SPLINE_CURVE_WITH_KNOTS('',3,(#199049,#199050,#199051,#199052,#199053,
#199054,#199055,#199056,#199057,#199058,#199059,#199060,#199061,#199062,
#199063,#199064,#199065,#199066,#199067,#199068,#199069,#199070,#199071,
#199072,#199073),.UNSPECIFIED.,.F.,.F.,(4,3,3,3,3,3,3,3,4),(1.1294748534261E-15,
0.138879076413939,0.277696122602223,0.416455864927007,0.562341898695256,
0.700986033244264,0.839599984102251,0.978180893530377,1.),.UNSPECIFIED.);
#5574=B_SPLINE_CURVE_WITH_KNOTS('',3,(#199074,#199075,#199076,#199077),
 .UNSPECIFIED.,.F.,.F.,(4,4),(0.,1.),.UNSPECIFIED.);
#5575=B_SPLINE_CURVE_WITH_KNOTS('',3,(#199102,#199103,#199104,#199105,#199106,
#199107),.UNSPECIFIED.,.F.,.F.,(4,2,4),(0.,0.502999982291435,1.),
 .UNSPECIFIED.);
#5576=B_SPLINE_CURVE_WITH_KNOTS('',3,(#200138,#200139,#200140,#200141,#200142,
#200143),.UNSPECIFIED.,.F.,.F.,(4,2,4),(-0.478433280045229,-0.243107720536295,
-3.73666282285079E-6),.UNSPECIFIED.);
#5577=B_SPLINE_CURVE_WITH_KNOTS('',3,(#200146,#200147,#200148,#200149,#200150,
#200151),.UNSPECIFIED.,.F.,.F.,(4,2,4),(-0.11270920227521,-0.0563552908536106,
-1.55324366682301E-6),.UNSPECIFIED.);
#5578=B_SPLINE_CURVE_WITH_KNOTS('',3,(#200158,#200159,#200160,#200161,#200162,
#200163),.UNSPECIFIED.,.F.,.F.,(4,2,4),(-0.0955355300118146,-0.0477684952643569,
-2.39971101840152E-6),.UNSPECIFIED.);
#5579=B_SPLINE_CURVE_WITH_KNOTS('',3,(#200167,#200168,#200169,#200170,#200171,
#200172),.UNSPECIFIED.,.F.,.F.,(4,2,4),(-0.0524683090000949,-0.0262347766775936,
-1.35358985086397E-6),.UNSPECIFIED.);
#5580=B_SPLINE_CURVE_WITH_KNOTS('',3,(#200184,#200185,#200186,#200187,#200188,
#200189),.UNSPECIFIED.,.F.,.F.,(4,2,4),(-0.253936238094734,-0.126979219567194,
-2.10375784686121E-6),.UNSPECIFIED.);
#5581=B_SPLINE_CURVE_WITH_KNOTS('',3,(#200197,#200198,#200199,#200200,#200201,
#200202),.UNSPECIFIED.,.F.,.F.,(4,2,4),(-0.258394873018348,-0.130229816210363,
-7.22354834947758E-7),.UNSPECIFIED.);
#5582=B_SPLINE_CURVE_WITH_KNOTS('',3,(#200216,#200217,#200218,#200219,#200220,
#200221),.UNSPECIFIED.,.F.,.F.,(4,2,4),(-0.228463041876464,-0.114227664573105,
-1.02920038175703E-6),.UNSPECIFIED.);
#5583=B_SPLINE_CURVE_WITH_KNOTS('',3,(#200235,#200236,#200237,#200238,#200239,
#200240),.UNSPECIFIED.,.F.,.F.,(4,2,4),(-0.227406176455065,-0.113706766455299,
-2.53502892005267E-6),.UNSPECIFIED.);
#5584=B_SPLINE_CURVE_WITH_KNOTS('',3,(#200277,#200278,#200279,#200280,#200281,
#200282),.UNSPECIFIED.,.F.,.F.,(4,2,4),(0.000194400838126528,0.116630356892709,
0.234421206579217),.UNSPECIFIED.);
#5585=B_SPLINE_CURVE_WITH_KNOTS('',3,(#200663,#200664,#200665,#200666,#200667,
#200668,#200669,#200670,#200671,#200672,#200673,#200674,#200675,#200676,
#200677,#200678,#200679,#200680,#200681,#200682),.UNSPECIFIED.,.F.,.F.,
(4,2,2,2,2,2,2,2,2,4),(0.,0.017536475393927,0.0219930830442672,0.0365274377738634,
0.070751261917734,0.0870574187505271,0.108664084129225,0.116991567530894,
0.121015033558203,0.127334633238972),.UNSPECIFIED.);
#5586=B_SPLINE_CURVE_WITH_KNOTS('',3,(#200684,#200685,#200686,#200687),
 .UNSPECIFIED.,.F.,.F.,(4,4),(0.0542180481640577,0.969015107905792),
 .UNSPECIFIED.);
#5587=B_SPLINE_CURVE_WITH_KNOTS('',3,(#200689,#200690,#200691,#200692,#200693,
#200694),.UNSPECIFIED.,.F.,.F.,(4,2,4),(4.76787336209101E-6,0.023593931008308,
0.0467878966544116),.UNSPECIFIED.);
#5588=B_SPLINE_CURVE_WITH_KNOTS('',3,(#200696,#200697,#200698,#200699,#200700,
#200701,#200702,#200703,#200704,#200705,#200706,#200707,#200708,#200709,
#200710,#200711,#200712,#200713,#200714,#200715,#200716,#200717),
 .UNSPECIFIED.,.F.,.F.,(4,2,2,2,2,2,2,2,2,2,4),(-0.555900774455164,-0.502035745496051,
-0.442390038983038,-0.424393273850783,-0.278932745293561,-0.233572033726155,
-0.156253627001661,-0.103501888368127,-0.0719169619346684,-0.032299277465137,
-2.45584905744778E-8),.UNSPECIFIED.);
#5589=B_SPLINE_CURVE_WITH_KNOTS('',3,(#200718,#200719,#200720,#200721,#200722,
#200723),.UNSPECIFIED.,.F.,.F.,(4,2,4),(0.,0.499006624679324,1.),
 .UNSPECIFIED.);
#5590=B_SPLINE_CURVE_WITH_KNOTS('',3,(#201285,#201286,#201287,#201288,#201289,
#201290,#201291,#201292,#201293,#201294,#201295,#201296,#201297,#201298,
#201299,#201300,#201301,#201302,#201303,#201304,#201305,#201306,#201307,
#201308),.UNSPECIFIED.,.F.,.F.,(4,2,2,2,2,2,2,2,2,2,2,4),(2.76063624704878E-7,
0.0103153193883155,0.0162903958553272,0.030872917071823,0.0697465314854658,
0.105053549140273,0.131809427696887,0.166538084415886,0.179730168174984,
0.220760236727318,0.242652969759649,0.273632513734802),.UNSPECIFIED.);
#5591=B_SPLINE_CURVE_WITH_KNOTS('',3,(#201310,#201311,#201312,#201313,#201314,
#201315,#201316,#201317,#201318,#201319),.UNSPECIFIED.,.F.,.F.,(4,2,2,2,
4),(0.,0.121284653603274,0.248608377129924,0.503255824183223,1.),
 .UNSPECIFIED.);
#5592=B_SPLINE_CURVE_WITH_KNOTS('',3,(#201321,#201322,#201323,#201324,#201325,
#201326,#201327,#201328,#201329,#201330,#201331,#201332,#201333,#201334,
#201335,#201336,#201337,#201338,#201339,#201340,#201341,#201342,#201343,
#201344),.UNSPECIFIED.,.F.,.F.,(4,2,2,2,2,2,2,2,2,2,2,4),(-0.542815827090465,
-0.505700033297898,-0.491406398135943,-0.426347230473485,-0.367919935175952,
-0.332652097482442,-0.313415302389993,-0.269024583259606,-0.128804589688154,
-0.09423657526446,-0.0693837256095411,-9.80508876202713E-7),
 .UNSPECIFIED.);
#5593=B_SPLINE_CURVE_WITH_KNOTS('',3,(#201346,#201347,#201348,#201349,#201350,
#201351,#201352,#201353,#201354,#201355),.UNSPECIFIED.,.F.,.F.,(4,2,2,2,
4),(-0.0740026973086748,-0.0369819514200437,-0.0179638246492492,-0.00888021376129463,
-1.00929457245466E-6),.UNSPECIFIED.);
#5594=B_SPLINE_CURVE_WITH_KNOTS('',3,(#201356,#201357,#201358,#201359),
 .UNSPECIFIED.,.F.,.F.,(4,4),(0.0559227492896294,0.969509810868811),
 .UNSPECIFIED.);
#5595=B_SPLINE_CURVE_WITH_KNOTS('',3,(#201726,#201727,#201728,#201729,#201730,
#201731,#201732,#201733,#201734,#201735,#201736,#201737,#201738,#201739,
#201740,#201741,#201742,#201743),.UNSPECIFIED.,.F.,.F.,(4,2,2,2,2,2,2,2,
4),(0.,0.02720791312337,0.0372043347179621,0.0718760780183553,0.0851663596652269,
0.0954636286661527,0.105386974740314,0.122140097830235,0.143001526856776),
 .UNSPECIFIED.);
#5596=B_SPLINE_CURVE_WITH_KNOTS('',3,(#201745,#201746,#201747,#201748,#201749,
#201750,#201751,#201752,#201753,#201754,#201755,#201756,#201757),
 .UNSPECIFIED.,.F.,.F.,(4,3,3,3,4),(2.3630439517094E-9,0.205079086868114,
0.455501131081411,0.728640752439003,1.),.UNSPECIFIED.);
#5597=B_SPLINE_CURVE_WITH_KNOTS('',3,(#201759,#201760,#201761,#201762,#201763,
#201764),.UNSPECIFIED.,.F.,.F.,(4,2,4),(1.40358012628945E-6,0.0217472883131899,
0.0430970546722853),.UNSPECIFIED.);
#5598=B_SPLINE_CURVE_WITH_KNOTS('',3,(#201766,#201767,#201768,#201769,#201770,
#201771,#201772,#201773,#201774,#201775,#201776,#201777,#201778,#201779,
#201780,#201781,#201782,#201783,#201784,#201785,#201786,#201787,#201788,
#201789),.UNSPECIFIED.,.F.,.F.,(4,2,2,2,2,2,2,2,2,2,2,4),(-0.412088451451376,
-0.372529944186826,-0.32964743775779,-0.299376123190801,-0.259218195736909,
-0.205822994030569,-0.172572535791612,-0.116278410061126,-0.0779939860474743,
-0.0546435191146628,-0.0247676692703238,-1.32710811784342E-8),
 .UNSPECIFIED.);
#5599=B_SPLINE_CURVE_WITH_KNOTS('',3,(#201790,#201791,#201792,#201793,#201794,
#201795),.UNSPECIFIED.,.F.,.F.,(4,2,4),(0.,0.49886621310506,1.),
 .UNSPECIFIED.);
#5600=B_SPLINE_CURVE_WITH_KNOTS('',3,(#202318,#202319,#202320,#202321,#202322,
#202323,#202324,#202325,#202326,#202327,#202328,#202329,#202330,#202331,
#202332,#202333),.UNSPECIFIED.,.F.,.F.,(4,2,2,2,2,2,2,4),(9.90112058791825E-7,
0.0138330094252819,0.0228535045364718,0.0434251080287075,0.0559716654418013,
0.0911264005088734,0.114270201886057,0.155254267708859),.UNSPECIFIED.);
#5601=B_SPLINE_CURVE_WITH_KNOTS('',3,(#202335,#202336,#202337,#202338,#202339,
#202340,#202341),.UNSPECIFIED.,.F.,.F.,(4,3,4),(1.19928029072876E-8,0.499701190314832,
0.999999995466719),.UNSPECIFIED.);
#5602=B_SPLINE_CURVE_WITH_KNOTS('',3,(#202343,#202344,#202345,#202346,#202347,
#202348,#202349,#202350,#202351,#202352,#202353,#202354,#202355,#202356,
#202357,#202358,#202359,#202360,#202361,#202362,#202363,#202364,#202365,
#202366,#202367,#202368),.UNSPECIFIED.,.F.,.F.,(4,2,2,2,2,2,2,2,2,2,2,2,
4),(-0.557432688185859,-0.539947613481655,-0.522228990190384,-0.481224242184197,
-0.449055525828226,-0.397089859289312,-0.32199400192039,-0.278105986122691,
-0.204825331566453,-0.177237377052104,-0.128621503496169,-0.0603607907826898,
-9.84241908086325E-7),.UNSPECIFIED.);
#5603=B_SPLINE_CURVE_WITH_KNOTS('',3,(#202370,#202371,#202372,#202373,#202374,
#202375,#202376,#202377),.UNSPECIFIED.,.F.,.F.,(4,2,2,4),(-0.0542958923388243,
-0.0270296190498593,-0.0132206493661975,-1.0001819469588E-6),
 .UNSPECIFIED.);
#5604=B_SPLINE_CURVE_WITH_KNOTS('',3,(#202378,#202379,#202380,#202381),
 .UNSPECIFIED.,.F.,.F.,(4,4),(0.0408435581858421,0.955362835047561),
 .UNSPECIFIED.);
#5605=B_SPLINE_CURVE_WITH_KNOTS('',3,(#202388,#202389,#202390,#202391,#202392,
#202393),.UNSPECIFIED.,.F.,.F.,(4,2,4),(-0.0363835945027032,-0.0181194609557856,
-1.32631589895571E-6),.UNSPECIFIED.);
#5606=B_SPLINE_CURVE_WITH_KNOTS('',3,(#202396,#202397,#202398,#202399,#202400,
#202401,#202402,#202403),.UNSPECIFIED.,.F.,.F.,(4,2,2,4),(-0.501368889131238,
-0.378312632595403,-0.251119784430402,-9.99947370461385E-7),
 .UNSPECIFIED.);
#5607=B_SPLINE_CURVE_WITH_KNOTS('',3,(#202405,#202406,#202407,#202408,#202409,
#202410),.UNSPECIFIED.,.F.,.F.,(4,2,4),(-0.50276667251833,-0.250728203604819,
-1.64858791458983E-6),.UNSPECIFIED.);
#5608=B_SPLINE_CURVE_WITH_KNOTS('',3,(#202429,#202430,#202431,#202432,#202433,
#202434,#202435,#202436),.UNSPECIFIED.,.F.,.F.,(4,2,2,4),(-0.519837304219326,
-0.24805813049356,-0.122424589346183,-1.86609418195765E-6),
 .UNSPECIFIED.);
#5609=B_SPLINE_CURVE_WITH_KNOTS('',3,(#202440,#202441,#202442,#202443,#202444,
#202445,#202446,#202447),.UNSPECIFIED.,.F.,.F.,(4,2,2,4),(-0.517963944857837,
-0.397262600557783,-0.272934034479511,-1.00033364894634E-6),
 .UNSPECIFIED.);
#5610=B_SPLINE_CURVE_WITH_KNOTS('',3,(#202515,#202516,#202517,#202518,#202519,
#202520),.UNSPECIFIED.,.F.,.F.,(4,2,4),(2.38553191273868E-5,0.38451969589073,
0.769032294646552),.UNSPECIFIED.);
#5611=B_SPLINE_CURVE_WITH_KNOTS('',3,(#202522,#202523,#202524,#202525,#202526,
#202527),.UNSPECIFIED.,.F.,.F.,(4,2,4),(1.50356860986035E-5,1.25241012483363,
2.53999779295726),.UNSPECIFIED.);
#5612=B_SPLINE_CURVE_WITH_KNOTS('',3,(#202528,#202529,#202530,#202531,#202532,
#202533),.UNSPECIFIED.,.F.,.F.,(4,2,4),(-0.779389334694245,-0.389697685223124,
-5.55355428311088E-10),.UNSPECIFIED.);
#5613=B_SPLINE_CURVE_WITH_KNOTS('',3,(#202551,#202552,#202553,#202554,#202555,
#202556),.UNSPECIFIED.,.F.,.F.,(4,2,4),(-0.78359241345728,-0.391796250396355,
-5.76655713470621E-6),.UNSPECIFIED.);
#5614=B_SPLINE_CURVE_WITH_KNOTS('',3,(#202558,#202559,#202560,#202561,#202562,
#202563),.UNSPECIFIED.,.F.,.F.,(4,2,4),(5.52446895573059E-7,1.19166141028964,
2.34466320735633),.UNSPECIFIED.);
#5615=B_SPLINE_CURVE_WITH_KNOTS('',3,(#202564,#202565,#202566,#202567,#202568,
#202569),.UNSPECIFIED.,.F.,.F.,(4,2,4),(7.27550329604178E-10,0.387014349072472,
0.774020170091024),.UNSPECIFIED.);
#5616=B_SPLINE_CURVE_WITH_KNOTS('',3,(#202571,#202572,#202573,#202574,#202575,
#202576,#202577,#202578,#202579,#202580,#202581,#202582,#202583,#202584,
#202585,#202586,#202587,#202588,#202589,#202590,#202591,#202592,#202593,
#202594,#202595,#202596,#202597,#202598,#202599,#202600,#202601,#202602,
#202603,#202604,#202605,#202606,#202607,#202608,#202609,#202610,#202611,
#202612,#202613,#202614,#202615,#202616,#202617,#202618,#202619,#202620,
#202621,#202622,#202623,#202624,#202625,#202626,#202627,#202628,#202629,
#202630,#202631,#202632,#202633,#202634,#202635,#202636,#202637,#202638,
#202639,#202640,#202641,#202642,#202643,#202644,#202645,#202646,#202647,
#202648,#202649,#202650,#202651,#202652,#202653,#202654,#202655,#202656,
#202657,#202658,#202659,#202660,#202661,#202662,#202663,#202664,#202665,
#202666,#202667,#202668,#202669,#202670,#202671,#202672,#202673,#202674,
#202675,#202676,#202677,#202678,#202679,#202680,#202681,#202682,#202683,
#202684,#202685,#202686,#202687,#202688,#202689,#202690,#202691,#202692,
#202693,#202694,#202695,#202696,#202697,#202698,#202699,#202700,#202701,
#202702,#202703,#202704,#202705,#202706,#202707,#202708,#202709,#202710,
#202711,#202712,#202713,#202714,#202715,#202716,#202717,#202718,#202719,
#202720,#202721,#202722,#202723,#202724,#202725,#202726,#202727,#202728,
#202729,#202730,#202731,#202732,#202733,#202734,#202735,#202736,#202737,
#202738,#202739,#202740,#202741,#202742,#202743,#202744,#202745,#202746,
#202747,#202748,#202749,#202750,#202751),.UNSPECIFIED.,.F.,.F.,(4,3,3,3,
3,3,3,3,3,3,3,3,3,3,3,3,3,3,3,3,3,3,3,3,3,3,3,3,3,3,3,3,3,3,3,3,3,3,3,3,
3,3,3,3,3,3,3,3,3,3,3,3,3,3,3,3,3,3,3,3,4),(-24.3791246898611,-21.9390511734847,
-21.587247653096,-20.9141411659479,-20.6749811972056,-20.3837713733337,
-20.3467231118568,-20.3139855512779,-20.2510876320262,-20.1280178699515,
-19.6785227528667,-18.0213957458283,-17.1910657827344,-16.6732915992545,
-16.606389804286,-16.5376226319807,-16.3841689273798,-16.0983915481674,
-15.4288562409009,-14.0828994997063,-13.0642722748157,-12.5402964114879,
-12.2266745209215,-12.1849575357879,-12.1642539264969,-12.1461887234912,
-12.0737332692285,-11.929579766766,-11.3129407028397,-10.16778088186,-9.03949592610626,
-8.47302954415004,-8.41915480146032,-8.2767480703946,-8.20384374683888,
-8.16718304435154,-8.12582623258736,-7.79810494513167,-7.2698798002026,
-6.31526529078602,-4.47499777521626,-4.24042728411652,-4.11506543944821,
-4.0830927553645,-4.06936168313156,-4.05586885160344,-4.00154868216668,
-3.56567492147755,-2.85831957756782,-2.36821257735992,-1.74323718478967,
-1.44214112090375,-1.36520157105012,-1.33001001266006,-1.31371874445417,
-1.30574819406026,-1.29669997244628,-1.1739315159141,-0.840135585432776,
-0.462288295934132,0.),.UNSPECIFIED.);
#5617=B_SPLINE_CURVE_WITH_KNOTS('',3,(#202772,#202773,#202774,#202775,#202776,
#202777,#202778,#202779,#202780,#202781,#202782,#202783,#202784,#202785,
#202786,#202787,#202788,#202789,#202790,#202791,#202792,#202793,#202794,
#202795,#202796,#202797,#202798,#202799,#202800,#202801,#202802,#202803,
#202804,#202805,#202806,#202807,#202808,#202809,#202810,#202811,#202812,
#202813,#202814,#202815,#202816,#202817,#202818,#202819,#202820,#202821,
#202822,#202823,#202824,#202825,#202826,#202827,#202828,#202829,#202830,
#202831,#202832,#202833,#202834,#202835,#202836,#202837,#202838,#202839,
#202840,#202841,#202842,#202843,#202844,#202845,#202846,#202847),
 .UNSPECIFIED.,.F.,.F.,(4,3,3,3,3,3,3,3,3,3,3,3,3,3,3,3,3,3,3,3,3,3,3,3,
3,4),(6.34981825321816E-8,0.0989503026875498,0.125000000000009,0.187500000000015,
0.218750000000019,0.234375000000023,0.242187500000026,0.248046875000028,
0.250000000000029,0.359531791882742,0.375000000000205,0.437500000000292,
0.468750000000336,0.484375000000357,0.492187500000366,0.498046875000372,
0.500000000000373,0.625000000000412,0.687500000000433,0.718750000000443,
0.734375000000447,0.742187500000449,0.74804687500045,0.750000000000449,
0.888290218203772,1.),.UNSPECIFIED.);
#5618=B_SPLINE_CURVE_WITH_KNOTS('',3,(#202848,#202849,#202850,#202851,#202852,
#202853),.UNSPECIFIED.,.F.,.F.,(4,2,4),(-0.920999101727438,-0.460499463349185,
0.),.UNSPECIFIED.);
#5619=B_SPLINE_CURVE_WITH_KNOTS('',3,(#202857,#202858,#202859,#202860,#202861,
#202862),.UNSPECIFIED.,.F.,.F.,(4,2,4),(8.97768736117609E-5,0.0361831683940628,
0.072357762392722),.UNSPECIFIED.);
#5620=B_SPLINE_CURVE_WITH_KNOTS('',3,(#202863,#202864,#202865,#202866,#202867,
#202868,#202869,#202870,#202871,#202872,#202873,#202874,#202875,#202876,
#202877,#202878),.UNSPECIFIED.,.F.,.F.,(4,2,2,2,2,2,2,4),(0.,0.0840900735190167,
0.170079589631641,0.345597941878049,0.709772911470069,1.47183879031424,
2.24214841760652,3.28470623629705),.UNSPECIFIED.);
#5621=B_SPLINE_CURVE_WITH_KNOTS('',3,(#202882,#202883,#202884,#202885,#202886,
#202887),.UNSPECIFIED.,.F.,.F.,(4,2,4),(1.16230659145506E-5,0.0315626968355423,
0.0631239559511615),.UNSPECIFIED.);
#5622=B_SPLINE_CURVE_WITH_KNOTS('',3,(#202906,#202907,#202908,#202909,#202910,
#202911,#202912,#202913,#202914,#202915,#202916,#202917,#202918,#202919,
#202920,#202921,#202922,#202923,#202924,#202925,#202926,#202927,#202928,
#202929,#202930,#202931,#202932,#202933,#202934,#202935,#202936,#202937,
#202938,#202939,#202940,#202941,#202942,#202943,#202944,#202945),
 .UNSPECIFIED.,.F.,.F.,(4,3,3,3,3,3,3,3,3,3,3,3,3,4),(1.46398934889516E-7,
0.132682753700099,0.250000000000049,0.375000000000075,0.437500000000089,
0.468750000000096,0.484375000000098,0.492187500000101,0.499511718750102,
0.500000000000101,0.629789774175571,0.756495566402389,0.878945558600266,
1.),.UNSPECIFIED.);
#5623=B_SPLINE_CURVE_WITH_KNOTS('',3,(#202946,#202947,#202948,#202949,#202950,
#202951),.UNSPECIFIED.,.F.,.F.,(4,2,4),(-0.78909387311141,-0.394547649846113,
-2.83084323799167E-6),.UNSPECIFIED.);
#5624=B_SPLINE_CURVE_WITH_KNOTS('',3,(#202954,#202955,#202956,#202957,#202958,
#202959),.UNSPECIFIED.,.F.,.F.,(4,2,4),(-0.144999030706854,-0.0722850858966769,
-1.08948736717993E-6),.UNSPECIFIED.);
#5625=B_SPLINE_CURVE_WITH_KNOTS('',3,(#202961,#202962,#202963,#202964,#202965,
#202966),.UNSPECIFIED.,.F.,.F.,(4,2,4),(-0.145062519279745,-0.0717246702272529,
-2.04904239573723E-6),.UNSPECIFIED.);
#5626=B_SPLINE_CURVE_WITH_KNOTS('',3,(#203165,#203166,#203167,#203168,#203169,
#203170,#203171,#203172,#203173,#203174,#203175,#203176,#203177,#203178),
 .UNSPECIFIED.,.F.,.F.,(4,2,2,2,2,2,4),(-1.33017036243567,-1.18625647343036,
-1.01397324567186,-0.691555155250063,-0.300153323254672,-0.150122339964719,
-3.71851020656187E-6),.UNSPECIFIED.);
#5627=B_SPLINE_CURVE_WITH_KNOTS('',3,(#203179,#203180,#203181,#203182,#203183,
#203184,#203185,#203186,#203187,#203188,#203189,#203190,#203191,#203192,
#203193,#203194),.UNSPECIFIED.,.F.,.F.,(4,2,2,2,2,2,2,4),(0.,0.0775932728882868,
0.156868688544549,0.318279132560059,0.651367894554687,1.34248027769519,
2.03705495700613,2.68811868112204),.UNSPECIFIED.);
#5628=B_SPLINE_CURVE_WITH_KNOTS('',3,(#203195,#203196,#203197,#203198,#203199,
#203200,#203201,#203202,#203203,#203204,#203205,#203206,#203207,#203208),
 .UNSPECIFIED.,.F.,.F.,(4,2,2,2,2,2,4),(4.21885373736936E-6,0.150120351661493,
0.335800964668187,0.716383852778975,1.16414712511149,1.32805324237018,1.49332401797822),
 .UNSPECIFIED.);
#5629=B_SPLINE_CURVE_WITH_KNOTS('',3,(#203210,#203211,#203212,#203213,#203214,
#203215),.UNSPECIFIED.,.F.,.F.,(4,2,4),(-0.288938372418224,-0.144350861152813,
-2.02154080876134E-6),.UNSPECIFIED.);
#5630=B_SPLINE_CURVE_WITH_KNOTS('',3,(#203217,#203218,#203219,#203220,#203221,
#203222),.UNSPECIFIED.,.F.,.F.,(4,2,4),(-0.106301599642394,-0.0531518973430255,
0.),.UNSPECIFIED.);
#5631=B_SPLINE_CURVE_WITH_KNOTS('',3,(#203223,#203224,#203225,#203226,#203227,
#203228),.UNSPECIFIED.,.F.,.F.,(4,2,4),(-0.0594936343766405,-0.0297474281548696,
-1.17962743812669E-6),.UNSPECIFIED.);
#5632=B_SPLINE_CURVE_WITH_KNOTS('',3,(#203231,#203232,#203233,#203234,#203235,
#203236),.UNSPECIFIED.,.F.,.F.,(4,2,4),(0.,0.0596783514028972,0.119718248687109),
 .UNSPECIFIED.);
#5633=B_SPLINE_CURVE_WITH_KNOTS('',3,(#203239,#203240,#203241,#203242,#203243,
#203244),.UNSPECIFIED.,.F.,.F.,(4,2,4),(1.76072677471803E-6,0.0155815452526277,
0.031165071681481),.UNSPECIFIED.);
#5634=B_SPLINE_CURVE_WITH_KNOTS('',3,(#203526,#203527,#203528,#203529,#203530,
#203531,#203532,#203533,#203534,#203535,#203536,#203537,#203538,#203539,
#203540,#203541),.UNSPECIFIED.,.F.,.F.,(4,2,2,2,2,2,2,4),(-1.38384890716764,
-1.29505750437121,-1.20010459148349,-1.01223063363571,-0.713348009009054,
-0.327085141772229,-0.164588178759744,-3.61030969499539E-6),
 .UNSPECIFIED.);
#5635=B_SPLINE_CURVE_WITH_KNOTS('',3,(#203542,#203543,#203544,#203545,#203546,
#203547,#203548,#203549,#203550,#203551,#203552,#203553,#203554,#203555,
#203556,#203557),.UNSPECIFIED.,.F.,.F.,(4,2,2,2,2,2,2,4),(9.99999998611766E-7,
0.0993759126941353,0.203266326829571,0.419074165587955,0.737922963129613,
1.15644233100818,1.36237389456797,1.52406811373926),.UNSPECIFIED.);
#5636=B_SPLINE_CURVE_WITH_KNOTS('',3,(#203558,#203559,#203560,#203561),
 .UNSPECIFIED.,.F.,.F.,(4,4),(0.,1.),.UNSPECIFIED.);
#5637=B_SPLINE_CURVE_WITH_KNOTS('',3,(#203566,#203567,#203568,#203569,#203570,
#203571),.UNSPECIFIED.,.F.,.F.,(4,2,4),(9.87884185704088E-7,0.256849336223313,
0.514256161629985),.UNSPECIFIED.);
#5638=B_SPLINE_CURVE_WITH_KNOTS('',3,(#203573,#203574,#203575,#203576,#203577,
#203578),.UNSPECIFIED.,.F.,.F.,(4,2,4),(0.,0.0346991781454662,0.069353995647711),
 .UNSPECIFIED.);
#5639=B_SPLINE_CURVE_WITH_KNOTS('',3,(#203581,#203582,#203583,#203584,#203585,
#203586),.UNSPECIFIED.,.F.,.F.,(4,2,4),(0.,0.0363145822537585,0.0726180231601224),
 .UNSPECIFIED.);
#5640=B_SPLINE_CURVE_WITH_KNOTS('',3,(#203591,#203592,#203593,#203594,#203595,
#203596),.UNSPECIFIED.,.F.,.F.,(4,2,4),(4.78770270599075E-8,0.128060743206973,
0.256048544261365),.UNSPECIFIED.);
#5641=B_SPLINE_CURVE_WITH_KNOTS('',3,(#203601,#203602,#203603,#203604,#203605,
#203606),.UNSPECIFIED.,.F.,.F.,(4,2,4),(4.98277165604429E-5,0.167649620755388,
0.334882293597469),.UNSPECIFIED.);
#5642=B_SPLINE_CURVE_WITH_KNOTS('',3,(#203611,#203612,#203613,#203614,#203615,
#203616),.UNSPECIFIED.,.F.,.F.,(4,2,4),(3.03081736350241E-7,0.129774103732234,
0.259677566733192),.UNSPECIFIED.);
#5643=B_SPLINE_CURVE_WITH_KNOTS('',3,(#203620,#203621,#203622,#203623,#203624,
#203625),.UNSPECIFIED.,.F.,.F.,(4,2,4),(1.63384903984051E-6,0.172602040902318,
0.345633561259572),.UNSPECIFIED.);
#5644=B_SPLINE_CURVE_WITH_KNOTS('',3,(#203633,#203634,#203635,#203636,#203637,
#203638,#203639,#203640),.UNSPECIFIED.,.F.,.F.,(4,2,2,4),(4.10708027676161E-7,
0.142324182994593,0.242655243240103,0.336291803605073),.UNSPECIFIED.);
#5645=B_SPLINE_CURVE_WITH_KNOTS('',3,(#203643,#203644,#203645,#203646,#203647,
#203648,#203649,#203650),.UNSPECIFIED.,.F.,.F.,(4,2,2,4),(-0.233723723416541,
-0.134753236172302,-0.0639786247876465,0.),.UNSPECIFIED.);
#5646=B_SPLINE_CURVE_WITH_KNOTS('',3,(#203655,#203656,#203657,#203658,#203659,
#203660,#203661,#203662),.UNSPECIFIED.,.F.,.F.,(4,2,2,4),(-0.212938364160185,
-0.137840855028458,-0.114290139265485,-2.81167466484031E-6),
 .UNSPECIFIED.);
#5647=B_SPLINE_CURVE_WITH_KNOTS('',3,(#203663,#203664,#203665,#203666,#203667,
#203668),.UNSPECIFIED.,.F.,.F.,(4,2,4),(-0.274300204892665,-0.138756656361396,
0.),.UNSPECIFIED.);
#5648=B_SPLINE_CURVE_WITH_KNOTS('',3,(#203672,#203673,#203674,#203675,#203676,
#203677),.UNSPECIFIED.,.F.,.F.,(4,2,4),(-0.234582769559139,-0.113404422883209,
0.),.UNSPECIFIED.);
#5649=B_SPLINE_CURVE_WITH_KNOTS('',3,(#203682,#203683,#203684,#203685,#203686,
#203687),.UNSPECIFIED.,.F.,.F.,(4,2,4),(-0.333867148600103,-0.169761706315603,
-1.67365979304573E-6),.UNSPECIFIED.);
#5650=B_SPLINE_CURVE_WITH_KNOTS('',3,(#203688,#203689,#203690,#203691,#203692,
#203693,#203694,#203695,#203696,#203697),.UNSPECIFIED.,.F.,.F.,(4,2,2,2,
4),(-0.26114851459812,-0.219345918382166,-0.211987678333995,-0.164711934999612,
-1.00032645433914E-6),.UNSPECIFIED.);
#5651=B_SPLINE_CURVE_WITH_KNOTS('',3,(#203699,#203700,#203701,#203702,#203703,
#203704,#203705,#203706,#203707,#203708,#203709,#203710,#203711,#203712,
#203713,#203714,#203715,#203716,#203717,#203718),.UNSPECIFIED.,.F.,.F.,
(4,2,2,2,2,2,2,2,2,4),(-0.673428088960982,-0.645968473599191,-0.63864640624558,
-0.636802786602354,-0.632872979199508,-0.569476839505419,-0.344878488981366,
-0.18144254201973,-0.0902078250720447,0.),.UNSPECIFIED.);
#5652=B_SPLINE_CURVE_WITH_KNOTS('',3,(#203720,#203721,#203722,#203723,#203724,
#203725),.UNSPECIFIED.,.F.,.F.,(4,2,4),(3.82662946478662E-7,0.114173063341795,
0.229641536291977),.UNSPECIFIED.);
#5653=B_SPLINE_CURVE_WITH_KNOTS('',3,(#204832,#204833,#204834,#204835,#204836,
#204837),.UNSPECIFIED.,.F.,.F.,(4,2,4),(0.,0.130029291827762,0.259524252867855),
 .UNSPECIFIED.);
#5654=B_SPLINE_CURVE_WITH_KNOTS('',3,(#204838,#204839,#204840,#204841),
 .UNSPECIFIED.,.F.,.F.,(4,4),(-2.59791985233575E-6,0.),.UNSPECIFIED.);
#5655=B_SPLINE_CURVE_WITH_KNOTS('',3,(#204843,#204844,#204845,#204846),
 .UNSPECIFIED.,.F.,.F.,(4,4),(-5.76565361003733E-6,0.),.UNSPECIFIED.);
#5656=B_SPLINE_CURVE_WITH_KNOTS('',3,(#204847,#204848,#204849,#204850,#204851,
#204852),.UNSPECIFIED.,.F.,.F.,(4,2,4),(9.99590034037455E-7,0.121785421623563,
0.24403732646739),.UNSPECIFIED.);
#5657=B_SPLINE_CURVE_WITH_KNOTS('',3,(#204853,#204854,#204855,#204856,#204857,
#204858),.UNSPECIFIED.,.F.,.F.,(4,2,4),(1.60537344364761E-6,0.13325159691034,
0.266722953368679),.UNSPECIFIED.);
#5658=B_SPLINE_CURVE_WITH_KNOTS('',3,(#204859,#204860,#204861,#204862,#204863,
#204864),.UNSPECIFIED.,.F.,.F.,(4,2,4),(7.42837984032087E-6,0.13590839804954,
0.271773150673492),.UNSPECIFIED.);
#5659=B_SPLINE_CURVE_WITH_KNOTS('',3,(#205145,#205146,#205147,#205148),
 .UNSPECIFIED.,.F.,.F.,(4,4),(0.0216968151072032,0.926937308587682),
 .UNSPECIFIED.);
#5660=B_SPLINE_CURVE_WITH_KNOTS('',3,(#205249,#205250,#205251,#205252),
 .UNSPECIFIED.,.F.,.F.,(4,4),(0.0222286199771242,0.926269849314919),
 .UNSPECIFIED.);
#5661=B_SPLINE_CURVE_WITH_KNOTS('',3,(#205330,#205331,#205332,#205333),
 .UNSPECIFIED.,.F.,.F.,(4,4),(0.0248339691417604,0.928145544482466),
 .UNSPECIFIED.);
#5662=B_SPLINE_CURVE_WITH_KNOTS('',3,(#205455,#205456,#205457,#205458),
 .UNSPECIFIED.,.F.,.F.,(4,4),(0.0238586497886119,0.928715545244436),
 .UNSPECIFIED.);
#5663=B_SPLINE_CURVE_WITH_KNOTS('',3,(#207120,#207121,#207122,#207123,#207124,
#207125,#207126,#207127,#207128,#207129,#207130,#207131,#207132,#207133,
#207134,#207135,#207136,#207137,#207138,#207139,#207140,#207141,#207142,
#207143,#207144,#207145,#207146,#207147,#207148,#207149,#207150,#207151,
#207152,#207153,#207154,#207155,#207156,#207157,#207158,#207159,#207160,
#207161,#207162,#207163,#207164,#207165,#207166,#207167,#207168,#207169,
#207170,#207171),.UNSPECIFIED.,.F.,.F.,(4,3,3,3,3,3,3,3,3,3,3,3,3,3,3,3,
3,4),(0.,0.0806048268663761,0.158714022235957,0.232021283797936,0.25,0.324001677230945,
0.401282678539864,0.48204973327551,0.5,0.500003584331971,0.580215606076185,
0.657617727195775,0.729959718881743,0.75,0.823833465567288,0.901157686681193,
0.982168573173414,1.),.UNSPECIFIED.);
#5664=B_SPLINE_CURVE_WITH_KNOTS('',3,(#207174,#207175,#207176,#207177,#207178,
#207179,#207180,#207181,#207182,#207183,#207184,#207185,#207186,#207187,
#207188,#207189,#207190,#207191,#207192,#207193,#207194,#207195,#207196,
#207197,#207198),.UNSPECIFIED.,.F.,.F.,(4,3,3,3,3,3,3,3,4),(0.,0.153526582008217,
0.311669465590391,0.422907894812392,0.494875521969546,0.500438042996234,
0.723275285884918,0.95807330633445,1.),.UNSPECIFIED.);
#5665=B_SPLINE_CURVE_WITH_KNOTS('',3,(#207246,#207247,#207248,#207249,#207250,
#207251,#207252,#207253,#207254,#207255,#207256,#207257,#207258,#207259,
#207260,#207261,#207262,#207263,#207264,#207265,#207266,#207267,#207268,
#207269,#207270,#207271,#207272,#207273,#207274,#207275,#207276,#207277,
#207278,#207279,#207280,#207281,#207282,#207283,#207284,#207285,#207286,
#207287,#207288,#207289,#207290,#207291,#207292,#207293,#207294,#207295,
#207296,#207297,#207298,#207299,#207300,#207301,#207302,#207303,#207304,
#207305,#207306,#207307,#207308,#207309,#207310,#207311,#207312,#207313,
#207314,#207315,#207316,#207317,#207318,#207319,#207320,#207321,#207322,
#207323,#207324),.UNSPECIFIED.,.F.,.F.,(4,3,3,3,3,3,3,3,3,3,3,3,3,3,3,3,
3,3,3,3,3,3,3,3,3,3,4),(0.,0.114629667334485,0.125000000000061,0.206386555414009,
0.242187500000125,0.249216553086816,0.250000000000131,0.255775387823804,
0.323300862474338,0.375000000000178,0.461187437204239,0.468750000000189,
0.484375000000195,0.494659013330622,0.500000000000202,0.509467435940447,
0.588597252522088,0.625000000000096,0.705669214159792,0.734375000000023,
0.744075465277332,0.750000000000004,0.758228559601408,0.826291788767228,
0.897548314370709,0.974137440758978,1.),.UNSPECIFIED.);
#5666=B_SPLINE_CURVE_WITH_KNOTS('',3,(#207327,#207328,#207329,#207330,#207331,
#207332,#207333,#207334,#207335,#207336,#207337,#207338,#207339,#207340,
#207341,#207342,#207343,#207344,#207345,#207346,#207347,#207348,#207349,
#207350,#207351,#207352,#207353,#207354,#207355,#207356,#207357),
 .UNSPECIFIED.,.F.,.F.,(4,3,3,3,3,3,3,3,3,3,4),(2.72268262058649E-15,0.000200725121439935,
0.000415654200400088,0.00061281274333361,0.000613704338138227,0.00122637007266609,
0.00122740867627373,0.00180004332875768,0.00184046060686526,0.00184111301440923,
0.00245481735254474),.UNSPECIFIED.);
#5667=B_SPLINE_CURVE_WITH_KNOTS('',3,(#207373,#207374,#207375,#207376,#207377,
#207378,#207379,#207380,#207381,#207382,#207383,#207384,#207385,#207386,
#207387,#207388,#207389,#207390,#207391,#207392,#207393,#207394,#207395,
#207396,#207397,#207398,#207399,#207400,#207401,#207402,#207403,#207404,
#207405,#207406,#207407,#207408,#207409,#207410,#207411,#207412,#207413,
#207414,#207415,#207416,#207417,#207418),.UNSPECIFIED.,.F.,.F.,(4,3,3,3,
3,3,3,3,3,3,3,3,3,3,3,4),(0.,0.25,0.4375,0.47265625,0.4891357421875,0.49312686920166,
0.49519146587179,0.495762776265408,0.496086078670549,0.496404892001326,
0.498372060391946,0.499351802461493,0.499918280627807,0.500154192246593,
0.796879510224575,1.),.UNSPECIFIED.);
#5668=B_SPLINE_CURVE_WITH_KNOTS('',3,(#207419,#207420,#207421,#207422),
 .UNSPECIFIED.,.F.,.F.,(4,4),(0.,0.0105146476282051),.UNSPECIFIED.);
#5669=B_SPLINE_CURVE_WITH_KNOTS('',3,(#207460,#207461,#207462,#207463,#207464,
#207465,#207466,#207467,#207468,#207469,#207470,#207471,#207472,#207473,
#207474,#207475,#207476,#207477,#207478,#207479,#207480,#207481,#207482,
#207483,#207484,#207485,#207486,#207487,#207488),.UNSPECIFIED.,.F.,.F.,
(4,1,1,2,2,2,1,1,2,2,2,1,2,2,2,2,4),(0.,0.125000000000098,0.187500000000144,
0.218750000000156,0.250000000000167,0.37500000000017,0.437500000000172,
0.468750000000185,0.484375000000191,0.500000000000197,0.625000000000202,
0.687500000000194,0.718750000000179,0.750000000000163,0.812500000000127,
0.875000000000091,1.),.UNSPECIFIED.);
#5670=B_SPLINE_CURVE_WITH_KNOTS('',3,(#207489,#207490,#207491,#207492,#207493,
#207494,#207495,#207496,#207497,#207498,#207499,#207500,#207501,#207502,
#207503,#207504,#207505,#207506,#207507,#207508,#207509,#207510,#207511,
#207512,#207513,#207514,#207515,#207516,#207517,#207518,#207519,#207520,
#207521,#207522),.UNSPECIFIED.,.F.,.F.,(4,2,2,1,1,2,2,2,2,1,1,2,2,2,2,1,
1,2,2,4),(0.,0.124999999999803,0.187499999999708,0.218749999999656,0.234374999999626,
0.242187499999614,0.249999999999602,0.374999999999714,0.437499999999765,
0.468749999999791,0.484374999999798,0.492187499999795,0.499999999999793,
0.624999999999634,0.687499999999566,0.71874999999953,0.734374999999508,
0.742187499999501,0.749999999999494,1.),.UNSPECIFIED.);
#5671=B_SPLINE_CURVE_WITH_KNOTS('',3,(#207550,#207551,#207552,#207553,#207554,
#207555,#207556,#207557,#207558,#207559,#207560,#207561,#207562,#207563,
#207564,#207565,#207566,#207567,#207568,#207569,#207570,#207571,#207572,
#207573,#207574),.UNSPECIFIED.,.F.,.F.,(4,3,3,3,3,3,3,3,4),(0.,0.169713712399116,
0.334856856199558,0.5,0.507353484491204,0.653685075739568,0.800970657233946,
0.950008965085336,1.),.UNSPECIFIED.);
#5672=B_SPLINE_CURVE_WITH_KNOTS('',3,(#207575,#207576,#207577,#207578,#207579,
#207580,#207581),.UNSPECIFIED.,.F.,.F.,(4,3,4),(9.81307786677359E-18,0.00416048285086259,
0.00832096570172518),.UNSPECIFIED.);
#5673=B_SPLINE_CURVE_WITH_KNOTS('',3,(#207621,#207622,#207623,#207624,#207625,
#207626,#207627,#207628,#207629,#207630,#207631,#207632,#207633,#207634,
#207635,#207636,#207637,#207638,#207639,#207640,#207641,#207642,#207643,
#207644,#207645,#207646,#207647,#207648,#207649,#207650,#207651,#207652,
#207653,#207654,#207655,#207656,#207657,#207658,#207659,#207660,#207661,
#207662,#207663,#207664,#207665,#207666,#207667,#207668,#207669,#207670,
#207671,#207672,#207673,#207674,#207675,#207676,#207677,#207678,#207679,
#207680,#207681,#207682,#207683,#207684,#207685,#207686,#207687,#207688,
#207689,#207690,#207691,#207692,#207693,#207694,#207695,#207696,#207697,
#207698,#207699,#207700,#207701,#207702,#207703,#207704,#207705,#207706,
#207707,#207708),.UNSPECIFIED.,.F.,.F.,(4,3,3,3,3,3,3,3,3,3,3,3,3,3,3,3,
3,3,3,3,3,3,3,3,3,3,3,3,3,4),(0.,0.0425126216922903,0.0624999999999267,
0.0846170699876459,0.09374999999989,0.109374999999872,0.124999999999853,
0.165041622176756,0.18749999999978,0.218749999999743,0.231263054308858,
0.244025736157331,0.249115753962458,0.249999999999707,0.312499999999637,
0.367366877870503,0.420962374636525,0.47656605752872,0.484374999999499,
0.493186960475905,0.499012025841205,0.499999999999505,0.56249999999956,
0.627138290432272,0.689890516986081,0.718749999999689,0.734644169494065,
0.749415530119711,0.749999999999721,1.),.UNSPECIFIED.);
#5674=B_SPLINE_CURVE_WITH_KNOTS('',3,(#207709,#207710,#207711,#207712,#207713,
#207714,#207715,#207716,#207717,#207718,#207719,#207720,#207721,#207722,
#207723,#207724,#207725,#207726,#207727,#207728,#207729,#207730,#207731,
#207732,#207733,#207734,#207735,#207736,#207737,#207738,#207739,#207740,
#207741,#207742),.UNSPECIFIED.,.F.,.F.,(4,2,2,1,1,2,2,2,2,1,1,2,2,2,2,1,
1,2,2,4),(0.,0.125000000000029,0.187500000000059,0.21875000000007,0.234375000000061,
0.242187500000052,0.250000000000042,0.374999999999973,0.437499999999958,
0.468749999999966,0.484374999999972,0.492187499999981,0.499999999999989,
0.625000000000122,0.687500000000187,0.718750000000232,0.734375000000254,
0.742187500000259,0.750000000000263,1.),.UNSPECIFIED.);
#5675=B_SPLINE_CURVE_WITH_KNOTS('',3,(#207764,#207765,#207766,#207767,#207768,
#207769,#207770,#207771,#207772,#207773,#207774,#207775,#207776,#207777,
#207778),.UNSPECIFIED.,.F.,.F.,(4,2,1,1,1,1,1,2,2,4),(0.,0.250000000000044,
0.375000000000067,0.437500000000079,0.468750000000085,0.484375000000087,
0.492187500000093,0.496093750000094,0.500000000000094,1.),.UNSPECIFIED.);
#5676=B_SPLINE_CURVE_WITH_KNOTS('',3,(#207779,#207780,#207781,#207782),
 .UNSPECIFIED.,.F.,.F.,(4,4),(0.,0.0107001581246114),.UNSPECIFIED.);
#5677=B_SPLINE_CURVE_WITH_KNOTS('',3,(#207798,#207799,#207800,#207801,#207802,
#207803,#207804,#207805,#207806,#207807,#207808,#207809,#207810,#207811,
#207812,#207813,#207814,#207815,#207816,#207817,#207818,#207819,#207820,
#207821,#207822,#207823,#207824,#207825,#207826,#207827,#207828,#207829,
#207830,#207831),.UNSPECIFIED.,.F.,.F.,(4,3,3,3,3,3,3,3,3,3,3,4),(0.,0.22396800402836,
0.249999999999856,0.374999999999772,0.43749999999973,0.468749999999695,
0.492663034070687,0.49999999999966,0.671520232782927,0.835760116391464,
0.986566865590623,1.),.UNSPECIFIED.);
#5678=B_SPLINE_CURVE_WITH_KNOTS('',3,(#207832,#207833,#207834,#207835),
 .UNSPECIFIED.,.F.,.F.,(4,4),(0.,1.),.UNSPECIFIED.);
#5679=B_SPLINE_CURVE_WITH_KNOTS('',3,(#207856,#207857,#207858,#207859,#207860,
#207861,#207862,#207863,#207864,#207865,#207866,#207867,#207868,#207869,
#207870,#207871,#207872,#207873,#207874,#207875,#207876,#207877,#207878,
#207879,#207880,#207881,#207882,#207883,#207884,#207885,#207886,#207887,
#207888,#207889,#207890,#207891,#207892,#207893,#207894,#207895,#207896,
#207897,#207898,#207899,#207900,#207901,#207902,#207903,#207904),
 .UNSPECIFIED.,.F.,.F.,(4,3,3,3,3,3,3,3,3,3,3,3,3,3,3,3,4),(0.,0.110193348836804,
0.226300572156345,0.347525286078198,0.468750000000051,0.486260581590066,
0.500000000000042,0.50052681277108,0.578360302839722,0.625000000000001,
0.687499999999979,0.71874999999998,0.735487941433878,0.749999999999982,
0.836356690732367,0.924217807330732,1.),.UNSPECIFIED.);
#5680=B_SPLINE_CURVE_WITH_KNOTS('',3,(#207906,#207907,#207908,#207909,#207910,
#207911,#207912,#207913,#207914,#207915,#207916,#207917,#207918,#207919,
#207920,#207921,#207922,#207923,#207924,#207925,#207926,#207927,#207928,
#207929,#207930,#207931,#207932,#207933,#207934,#207935,#207936,#207937,
#207938,#207939,#207940,#207941,#207942,#207943,#207944,#207945,#207946,
#207947,#207948,#207949,#207950,#207951,#207952,#207953,#207954,#207955,
#207956,#207957,#207958,#207959,#207960),.UNSPECIFIED.,.F.,.F.,(4,3,3,3,
3,3,3,3,3,3,3,3,3,3,3,3,3,3,4),(2.53418446955826E-6,0.0998044898858354,
0.193933366124132,0.269558082684436,0.348527825145383,0.397466750068292,
0.42749756760633,0.457698304529386,0.478849152264081,0.489424576131429,
0.492068432098266,0.492601765237038,0.499268082446897,0.499999999998776,
0.616033678583699,0.725387395575726,0.830726652989945,0.930602413285796,
1.),.UNSPECIFIED.);
#5681=B_SPLINE_CURVE_WITH_KNOTS('',3,(#208004,#208005,#208006,#208007,#208008,
#208009,#208010,#208011,#208012,#208013,#208014,#208015,#208016,#208017,
#208018,#208019,#208020,#208021,#208022,#208023,#208024,#208025,#208026,
#208027,#208028,#208029,#208030,#208031,#208032,#208033,#208034,#208035,
#208036,#208037),.UNSPECIFIED.,.F.,.F.,(4,2,2,1,1,2,2,2,2,1,1,2,2,2,2,1,
1,2,2,4),(0.,0.124999999999678,0.187499999999503,0.21874999999941,0.23437499999937,
0.242187499999368,0.249999999999367,0.374999999999121,0.437499999999018,
0.468749999998965,0.484374999998937,0.49218749999893,0.499999999998922,
0.624999999999086,0.687499999999163,0.718749999999202,0.734374999999215,
0.742187499999228,0.749999999999241,1.),.UNSPECIFIED.);
#5682=B_SPLINE_CURVE_WITH_KNOTS('',3,(#208040,#208041,#208042,#208043,#208044,
#208045,#208046,#208047,#208048,#208049,#208050,#208051,#208052,#208053,
#208054,#208055,#208056,#208057,#208058,#208059,#208060,#208061,#208062,
#208063,#208064,#208065,#208066),.UNSPECIFIED.,.F.,.F.,(4,2,1,1,2,2,2,1,
1,2,2,2,1,2,2,4),(0.,0.124999999999879,0.187499999999819,0.218749999999792,
0.23437499999979,0.249999999999788,0.3749999999998,0.437499999999805,0.468749999999808,
0.484374999999806,0.499999999999804,0.62499999999983,0.68749999999983,0.718749999999846,
0.749999999999862,1.),.UNSPECIFIED.);
#5683=B_SPLINE_CURVE_WITH_KNOTS('',3,(#208082,#208083,#208084,#208085),
 .UNSPECIFIED.,.F.,.F.,(4,4),(0.,1.),.UNSPECIFIED.);
#5684=B_SPLINE_CURVE_WITH_KNOTS('',3,(#208086,#208087,#208088,#208089),
 .UNSPECIFIED.,.F.,.F.,(4,4),(4.04603565571183E-17,0.00980967348625103),
 .UNSPECIFIED.);
#5685=B_SPLINE_CURVE_WITH_KNOTS('',3,(#208111,#208112,#208113,#208114,#208115,
#208116,#208117),.UNSPECIFIED.,.F.,.F.,(4,3,4),(0.,0.00416021787251447,
0.00832043574502893),.UNSPECIFIED.);
#5686=B_SPLINE_CURVE_WITH_KNOTS('',3,(#208118,#208119,#208120,#208121,#208122,
#208123,#208124,#208125,#208126,#208127,#208128,#208129,#208130,#208131,
#208132,#208133,#208134,#208135,#208136,#208137,#208138,#208139),
 .UNSPECIFIED.,.F.,.F.,(4,3,3,3,3,3,3,4),(0.,0.174023413314913,0.343412686965267,
0.51280196061562,0.661616188253227,0.810426910260397,0.959545980295111,
1.),.UNSPECIFIED.);
#5687=B_SPLINE_CURVE_WITH_KNOTS('',3,(#208161,#208162,#208163,#208164,#208165,
#208166,#208167,#208168,#208169,#208170,#208171,#208172,#208173,#208174,
#208175,#208176,#208177,#208178,#208179,#208180,#208181,#208182,#208183,
#208184,#208185,#208186,#208187,#208188,#208189,#208190,#208191,#208192,
#208193,#208194,#208195,#208196,#208197,#208198,#208199,#208200,#208201,
#208202,#208203,#208204,#208205,#208206,#208207,#208208,#208209,#208210,
#208211,#208212,#208213,#208214,#208215,#208216,#208217,#208218),
 .UNSPECIFIED.,.F.,.F.,(4,3,3,3,3,3,3,3,3,3,3,3,3,3,3,3,3,3,3,4),(0.,0.0969945238812358,
0.200908355313719,0.288417201918382,0.395108792074533,0.484375000000186,
0.496161411879799,0.500000000000187,0.500467577071174,0.574698071762265,
0.625000000000102,0.687500000000059,0.718750000000036,0.734375000000025,
0.74523453307188,0.750000000000014,0.812500000000011,0.900353222249502,
0.989751398368336,1.),.UNSPECIFIED.);
#5688=B_SPLINE_CURVE_WITH_KNOTS('',3,(#208219,#208220,#208221,#208222,#208223,
#208224,#208225,#208226,#208227,#208228,#208229,#208230,#208231,#208232,
#208233,#208234,#208235,#208236,#208237,#208238,#208239,#208240,#208241,
#208242,#208243,#208244,#208245,#208246,#208247,#208248,#208249,#208250,
#208251,#208252,#208253,#208254,#208255,#208256,#208257,#208258,#208259,
#208260,#208261,#208262,#208263,#208264,#208265,#208266,#208267,#208268,
#208269,#208270,#208271,#208272,#208273,#208274,#208275,#208276,#208277,
#208278,#208279,#208280,#208281,#208282,#208283,#208284,#208285,#208286,
#208287,#208288,#208289,#208290,#208291,#208292,#208293,#208294,#208295,
#208296,#208297,#208298,#208299,#208300),.UNSPECIFIED.,.F.,.F.,(4,3,3,3,
3,3,3,3,3,3,3,3,3,3,3,3,3,3,3,3,3,3,3,3,3,3,3,4),(0.,0.0771005613023838,
0.125000000000185,0.216511745445919,0.286309253196597,0.356488197815171,
0.423767589799145,0.45981549070489,0.484747979915122,0.491046981783119,
0.491844143094684,0.492573845881986,0.496712163198199,0.49871666064824,
0.499810910719285,0.50025674181692,0.594269001722782,0.625000000000811,
0.687500000000829,0.718750000000836,0.734375000000824,0.742187500000821,
0.748946705574376,0.750000000000817,0.8270954483746,0.901599505899295,0.972126634077241,
1.),.UNSPECIFIED.);
#5689=B_SPLINE_CURVE_WITH_KNOTS('',3,(#208334,#208335,#208336,#208337,#208338,
#208339,#208340,#208341,#208342,#208343,#208344,#208345,#208346,#208347,
#208348,#208349,#208350,#208351,#208352,#208353,#208354,#208355,#208356,
#208357,#208358,#208359,#208360,#208361,#208362,#208363,#208364,#208365,
#208366,#208367),.UNSPECIFIED.,.F.,.F.,(4,2,2,1,1,2,2,2,2,1,1,2,2,2,2,1,
1,2,2,4),(0.,0.124999999999397,0.187499999999094,0.218749999998944,0.234374999998861,
0.242187499998828,0.249999999998795,0.374999999998407,0.437499999998207,
0.468749999998112,0.484374999998075,0.492187499998049,0.499999999998023,
0.624999999998236,0.687499999998338,0.718749999998405,0.734374999998451,
0.742187499998474,0.749999999998497,1.),.UNSPECIFIED.);
#5690=B_SPLINE_CURVE_WITH_KNOTS('',3,(#208368,#208369,#208370,#208371,#208372,
#208373,#208374,#208375,#208376,#208377,#208378,#208379,#208380,#208381,
#208382,#208383,#208384,#208385,#208386,#208387,#208388,#208389,#208390,
#208391,#208392,#208393,#208394,#208395,#208396),.UNSPECIFIED.,.F.,.F.,
(4,1,1,2,2,2,1,1,2,2,2,1,2,2,2,2,4),(0.,0.124999999999937,0.187499999999906,
0.218749999999893,0.24999999999988,0.374999999999836,0.437499999999826,
0.468749999999805,0.484374999999804,0.499999999999802,0.624999999999829,
0.687499999999847,0.718749999999856,0.749999999999865,0.812499999999898,
0.87499999999993,1.),.UNSPECIFIED.);
#5691=B_SPLINE_CURVE_WITH_KNOTS('',3,(#208416,#208417,#208418,#208419),
 .UNSPECIFIED.,.F.,.F.,(4,4),(0.,0.00972938600277915),.UNSPECIFIED.);
#5692=B_SPLINE_CURVE_WITH_KNOTS('',3,(#208420,#208421,#208422,#208423,#208424,
#208425,#208426,#208427,#208428,#208429,#208430,#208431,#208432,#208433,
#208434),.UNSPECIFIED.,.F.,.F.,(4,2,2,1,1,1,2,2,4),(0.,0.250000000000011,
0.375000000000019,0.437500000000025,0.468750000000028,0.484375000000027,
0.492187500000026,0.500000000000025,1.),.UNSPECIFIED.);
#5693=B_SPLINE_CURVE_WITH_KNOTS('',3,(#208450,#208451,#208452,#208453),
 .UNSPECIFIED.,.F.,.F.,(4,4),(0.,3.23803390124219E-5),.UNSPECIFIED.);
#5694=B_SPLINE_CURVE_WITH_KNOTS('',3,(#208454,#208455,#208456,#208457),
 .UNSPECIFIED.,.F.,.F.,(4,4),(0.,2.59869381596583E-5),.UNSPECIFIED.);
#5695=B_SPLINE_CURVE_WITH_KNOTS('',3,(#208485,#208486,#208487,#208488,#208489,
#208490,#208491,#208492,#208493,#208494,#208495,#208496,#208497,#208498,
#208499,#208500,#208501,#208502,#208503,#208504,#208505,#208506,#208507,
#208508,#208509,#208510,#208511,#208512,#208513,#208514,#208515,#208516,
#208517,#208518,#208519,#208520,#208521,#208522,#208523,#208524,#208525,
#208526,#208527,#208528,#208529,#208530),.UNSPECIFIED.,.F.,.F.,(4,3,3,3,
3,3,3,3,3,3,3,3,3,3,3,4),(0.,0.0906629207478083,0.188650654775597,0.249999999999092,
0.373046874998603,0.467058712523105,0.496093749998114,0.499999999998105,
0.508669898665942,0.586164263608202,0.66828506364852,0.733205222480325,
0.795419535562799,0.860569483442956,0.930284741721478,1.),.UNSPECIFIED.);
#5696=B_SPLINE_CURVE_WITH_KNOTS('',3,(#208531,#208532,#208533,#208534,#208535,
#208536,#208537,#208538,#208539,#208540,#208541,#208542,#208543,#208544,
#208545,#208546,#208547,#208548,#208549,#208550,#208551,#208552,#208553,
#208554,#208555,#208556,#208557,#208558,#208559,#208560,#208561,#208562,
#208563,#208564,#208565,#208566,#208567,#208568,#208569,#208570,#208571,
#208572,#208573,#208574,#208575,#208576,#208577,#208578,#208579,#208580,
#208581,#208582,#208583,#208584,#208585,#208586,#208587,#208588),
 .UNSPECIFIED.,.F.,.F.,(4,3,3,3,3,3,3,3,3,3,3,3,3,3,3,3,3,3,3,4),(0.,0.0689082811774419,
0.137184580919919,0.20664499924701,0.234374999999953,0.244741122741839,
0.249594660540849,0.249999999999948,0.361641502564665,0.374999999999894,
0.437499999999878,0.468749999999856,0.484374999999857,0.495706414317134,
0.499537692650688,0.499999999999857,0.638127812197921,0.774660191713116,
0.909042522090822,1.),.UNSPECIFIED.);
#5697=B_SPLINE_CURVE_WITH_KNOTS('',3,(#208620,#208621,#208622,#208623),
 .UNSPECIFIED.,.F.,.F.,(4,4),(0.,1.68205588696557E-5),.UNSPECIFIED.);
#5698=B_SPLINE_CURVE_WITH_KNOTS('',3,(#208624,#208625,#208626,#208627),
 .UNSPECIFIED.,.F.,.F.,(4,4),(6.93889390390723E-18,2.09370149851292E-5),
 .UNSPECIFIED.);
#5699=B_SPLINE_CURVE_WITH_KNOTS('',3,(#208714,#208715,#208716,#208717),
 .UNSPECIFIED.,.F.,.F.,(4,4),(0.,0.000210836370419721),.UNSPECIFIED.);
#5700=B_SPLINE_CURVE_WITH_KNOTS('',3,(#208756,#208757,#208758,#208759,#208760,
#208761,#208762,#208763,#208764,#208765,#208766,#208767,#208768,#208769,
#208770,#208771,#208772,#208773,#208774,#208775,#208776,#208777,#208778,
#208779,#208780,#208781,#208782,#208783,#208784,#208785,#208786,#208787),
 .UNSPECIFIED.,.F.,.F.,(4,2,2,1,2,2,1,2,2,1,1,2,2,2,1,1,2,2,4),(0.,0.0624999999999714,
0.124999999999943,0.187499999999914,0.218749999999901,0.249999999999887,
0.312499999999844,0.343749999999822,0.3749999999998,0.437499999999771,0.468749999999757,
0.484374999999755,0.499999999999754,0.624999999999732,0.687499999999739,
0.718749999999749,0.734374999999755,0.74999999999976,1.),.UNSPECIFIED.);
#5701=B_SPLINE_CURVE_WITH_KNOTS('',3,(#208789,#208790,#208791,#208792,#208793,
#208794,#208795,#208796,#208797,#208798,#208799,#208800,#208801,#208802,
#208803,#208804,#208805,#208806,#208807,#208808,#208809,#208810,#208811),
 .UNSPECIFIED.,.F.,.F.,(4,2,2,1,1,1,2,2,2,1,1,2,2,4),(0.,0.25000000000007,
0.375000000000092,0.437500000000124,0.468750000000127,0.484375000000116,
0.492187500000111,0.500000000000106,0.625000000000092,0.687500000000093,
0.718750000000093,0.734375000000072,0.750000000000051,1.),.UNSPECIFIED.);
#5702=B_SPLINE_CURVE_WITH_KNOTS('',3,(#208852,#208853,#208854,#208855,#208856,
#208857,#208858,#208859,#208860,#208861,#208862,#208863,#208864,#208865,
#208866,#208867,#208868),.UNSPECIFIED.,.F.,.F.,(4,2,2,2,1,1,1,2,2,4),(0.,
0.250000000001027,0.375000000001554,0.437500000001813,0.468750000001952,
0.48437500000201,0.492187500002025,0.496093750002033,0.50000000000204,1.),
 .UNSPECIFIED.);
#5703=B_SPLINE_CURVE_WITH_KNOTS('',3,(#208869,#208870,#208871,#208872,#208873,
#208874,#208875,#208876,#208877,#208878,#208879,#208880,#208881,#208882,
#208883,#208884,#208885,#208886,#208887,#208888,#208889,#208890,#208891,
#208892,#208893,#208894,#208895,#208896,#208897,#208898,#208899,#208900,
#208901,#208902,#208903,#208904,#208905,#208906,#208907,#208908,#208909,
#208910,#208911,#208912,#208913,#208914,#208915,#208916,#208917,#208918,
#208919,#208920,#208921,#208922,#208923,#208924,#208925,#208926,#208927,
#208928,#208929,#208930,#208931,#208932,#208933,#208934,#208935,#208936,
#208937,#208938,#208939,#208940,#208941,#208942,#208943,#208944,#208945,
#208946,#208947,#208948,#208949,#208950,#208951,#208952,#208953,#208954,
#208955,#208956,#208957,#208958,#208959,#208960,#208961,#208962,#208963,
#208964,#208965,#208966,#208967,#208968,#208969,#208970,#208971,#208972,
#208973,#208974,#208975,#208976,#208977,#208978,#208979,#208980,#208981,
#208982,#208983,#208984,#208985,#208986,#208987,#208988,#208989,#208990,
#208991,#208992,#208993,#208994,#208995,#208996,#208997,#208998),
 .UNSPECIFIED.,.F.,.F.,(4,3,3,3,3,3,3,3,3,3,3,3,3,3,3,3,3,3,3,3,3,3,3,3,
3,3,3,3,3,3,3,3,3,3,3,3,3,3,3,3,3,3,3,4),(0.,0.0823270774102905,0.125000000000094,
0.187500000000141,0.218750000000155,0.234375000000162,0.243570804458758,
0.25000000000017,0.250186396125238,0.295692350820031,0.346719906813076,
0.375000000000246,0.457188321893283,0.468750000000302,0.484375000000294,
0.492442181687317,0.500000000000287,0.50058849156398,0.537417390281148,
0.562500000000271,0.593750000000251,0.606558538060083,0.61892440865582,
0.625000000000231,0.625785934282743,0.656250000000211,0.680095796146748,
0.687004607525639,0.69277546770298,0.70312500000018,0.726562500000165,0.732421875000161,
0.75000000000015,0.750800803251414,0.792958838704499,0.81250000000011,0.843750000000093,
0.855813090863169,0.868300478426156,0.875000000000077,0.916195051773411,
0.958097525886705,0.997217794971731,1.),.UNSPECIFIED.);
#5704=B_SPLINE_CURVE_WITH_KNOTS('',3,(#209048,#209049,#209050,#209051,#209052,
#209053,#209054,#209055,#209056,#209057,#209058,#209059,#209060,#209061,
#209062,#209063,#209064,#209065,#209066,#209067,#209068,#209069,#209070,
#209071,#209072,#209073,#209074,#209075,#209076,#209077,#209078,#209079,
#209080,#209081,#209082,#209083,#209084,#209085,#209086,#209087,#209088,
#209089,#209090,#209091,#209092,#209093,#209094,#209095,#209096),
 .UNSPECIFIED.,.F.,.F.,(4,3,3,3,3,3,3,3,3,3,3,3,3,3,3,3,4),(0.,0.0467203140673268,
0.093322248216158,0.125000000000416,0.171247762433252,0.187500000000625,
0.218750000000742,0.234375000000792,0.242187500000816,0.246093750000817,
0.250000000000818,0.375000000000667,0.437500000000608,0.478869108686064,
0.50000000000055,0.75000000000027,0.999999999999991),.UNSPECIFIED.);
#5705=B_SPLINE_CURVE_WITH_KNOTS('',3,(#209097,#209098,#209099,#209100,#209101,
#209102,#209103,#209104,#209105,#209106),.UNSPECIFIED.,.F.,.F.,(4,3,3,4),
(6.93889390390723E-18,0.000636015601019443,0.00129844965740935,0.00158760011419448),
 .UNSPECIFIED.);
#5706=B_SPLINE_CURVE_WITH_KNOTS('',3,(#209122,#209123,#209124,#209125,#209126,
#209127,#209128,#209129,#209130,#209131),.UNSPECIFIED.,.F.,.F.,(4,3,3,4),
(0.,0.000679723972684053,0.00133201311757647,0.0015185374894695),
 .UNSPECIFIED.);
#5707=B_SPLINE_CURVE_WITH_KNOTS('',3,(#209132,#209133,#209134,#209135,#209136,
#209137,#209138,#209139,#209140,#209141,#209142,#209143,#209144,#209145,
#209146,#209147,#209148,#209149,#209150,#209151,#209152,#209153,#209154,
#209155,#209156,#209157,#209158,#209159,#209160,#209161,#209162,#209163,
#209164,#209165,#209166,#209167,#209168,#209169,#209170,#209171,#209172,
#209173,#209174,#209175,#209176,#209177,#209178,#209179,#209180,#209181,
#209182,#209183),.UNSPECIFIED.,.F.,.F.,(4,3,3,3,3,3,3,3,3,3,3,3,3,3,3,3,
3,4),(1.7719643363079E-14,0.249999999999962,0.374999999999965,0.437499999999957,
0.479463228974921,0.49999999999995,0.624999999999912,0.687499999999895,
0.718749999999885,0.734374999999887,0.746093749999895,0.749999999999911,
0.796573030417351,0.843551162119774,0.89092801606667,0.938447913903747,
0.986074086976133,1.),.UNSPECIFIED.);
#5708=B_SPLINE_CURVE_WITH_KNOTS('',3,(#209211,#209212,#209213,#209214,#209215,
#209216,#209217,#209218,#209219,#209220,#209221,#209222,#209223,#209224,
#209225,#209226,#209227,#209228,#209229,#209230,#209231,#209232,#209233,
#209234,#209235,#209236,#209237,#209238,#209239,#209240,#209241,#209242,
#209243,#209244,#209245,#209246,#209247,#209248,#209249,#209250,#209251,
#209252),.UNSPECIFIED.,.F.,.F.,(4,2,1,1,1,1,2,2,2,2,1,1,2,2,2,2,1,1,1,2,
2,2,2,2,1,4),(7.98944320809248E-8,0.125000000000703,0.187500000001066,0.218750000001238,
0.234375000001325,0.242187500001355,0.248046875001389,0.250000000001407,
0.375000000001313,0.437500000001265,0.468750000001242,0.48437500000123,
0.492187500001225,0.500000000001219,0.625000000001405,0.687500000001511,
0.718750000001579,0.734375000001613,0.742187500001628,0.746093750001613,
0.750000000001599,0.875000000000742,0.906250000000527,0.921875000000435,
0.937500000000343,1.),.UNSPECIFIED.);
#5709=B_SPLINE_CURVE_WITH_KNOTS('',3,(#209253,#209254,#209255,#209256,#209257,
#209258,#209259,#209260,#209261,#209262,#209263,#209264,#209265,#209266,
#209267,#209268,#209269,#209270,#209271,#209272,#209273,#209274,#209275,
#209276,#209277,#209278,#209279,#209280,#209281,#209282,#209283,#209284,
#209285,#209286,#209287,#209288,#209289,#209290,#209291,#209292,#209293,
#209294,#209295,#209296,#209297,#209298,#209299,#209300,#209301,#209302,
#209303,#209304,#209305,#209306,#209307,#209308,#209309,#209310,#209311,
#209312,#209313,#209314,#209315,#209316,#209317,#209318,#209319,#209320,
#209321,#209322,#209323,#209324,#209325,#209326,#209327,#209328,#209329,
#209330,#209331,#209332,#209333,#209334,#209335,#209336,#209337,#209338,
#209339,#209340,#209341,#209342,#209343,#209344,#209345,#209346,#209347,
#209348,#209349,#209350,#209351,#209352),.UNSPECIFIED.,.F.,.F.,(4,3,3,3,
3,3,3,3,3,3,3,3,3,3,3,3,3,3,3,3,3,3,3,3,3,3,3,3,3,3,3,3,3,4),(0.,0.0156249999999717,
0.0624999999998867,0.09374999999983,0.109374999999802,0.117187499999775,
0.123461617059797,0.124999999999748,0.140624999999709,0.181612062947922,
0.18749999999959,0.21874999999951,0.234374999999459,0.242187499999445,0.248785718386343,
0.249999999999431,0.259946689298152,0.26562499999941,0.322561688284792,
0.374999999999263,0.429126579721212,0.437499999999179,0.468749999999148,
0.484374999999132,0.492187499999136,0.49999999999914,0.510027340931445,
0.608514426712397,0.624999999999355,0.713539679447043,0.74999999999957,
0.857165949068296,0.962181280863057,1.),.UNSPECIFIED.);
#5710=B_SPLINE_CURVE_WITH_KNOTS('',3,(#209380,#209381,#209382,#209383,#209384,
#209385,#209386,#209387,#209388,#209389,#209390,#209391,#209392,#209393,
#209394,#209395,#209396,#209397,#209398,#209399,#209400,#209401,#209402,
#209403,#209404,#209405,#209406,#209407,#209408,#209409,#209410,#209411,
#209412,#209413,#209414,#209415,#209416,#209417,#209418,#209419,#209420,
#209421,#209422,#209423,#209424,#209425,#209426,#209427,#209428,#209429,
#209430,#209431,#209432,#209433,#209434,#209435,#209436,#209437,#209438,
#209439,#209440,#209441,#209442,#209443,#209444,#209445,#209446,#209447,
#209448,#209449,#209450,#209451,#209452,#209453,#209454,#209455,#209456,
#209457,#209458,#209459,#209460,#209461,#209462,#209463,#209464,#209465,
#209466,#209467,#209468,#209469,#209470,#209471,#209472,#209473),
 .UNSPECIFIED.,.F.,.F.,(4,3,3,3,3,3,3,3,3,3,3,3,3,3,3,3,3,3,3,3,3,3,3,3,
3,3,3,3,3,3,3,4),(0.,0.110965913270212,0.227650776136299,0.249999999999794,
0.376459127159745,0.484374999999595,0.489891538603025,0.499999999999583,
0.551168547591977,0.562499999999553,0.617114766859165,0.624999999999523,
0.681846022228115,0.687499999999481,0.718749999999474,0.734374999999471,
0.739546449428334,0.742187499999469,0.748939833770959,0.749999999999468,
0.791295688660075,0.81249999999959,0.843749999999639,0.859374999999662,
0.867187499999687,0.873635825536526,0.874999999999712,0.920254653271175,
0.937499999999856,0.968749999999928,0.984374999999964,1.),.UNSPECIFIED.);
#5711=B_SPLINE_CURVE_WITH_KNOTS('',3,(#209474,#209475,#209476,#209477,#209478,
#209479,#209480,#209481,#209482,#209483,#209484,#209485,#209486,#209487,
#209488,#209489,#209490,#209491,#209492,#209493,#209494,#209495,#209496,
#209497,#209498,#209499,#209500,#209501,#209502,#209503,#209504,#209505,
#209506,#209507,#209508),.UNSPECIFIED.,.F.,.F.,(4,2,2,1,1,1,2,2,2,2,1,2,
2,2,2,1,1,1,2,2,4),(0.,0.125000000000223,0.187500000000349,0.218750000000401,
0.234375000000438,0.242187500000456,0.246093750000454,0.250000000000453,
0.375000000000397,0.437500000000356,0.468750000000339,0.48437500000034,
0.500000000000341,0.625000000000326,0.687500000000331,0.718750000000338,
0.734375000000342,0.74218750000035,0.746093750000347,0.750000000000345,
0.999999939294813),.UNSPECIFIED.);
#5712=B_SPLINE_CURVE_WITH_KNOTS('',3,(#209566,#209567,#209568,#209569,#209570,
#209571,#209572,#209573,#209574,#209575,#209576,#209577,#209578,#209579,
#209580,#209581,#209582,#209583),.UNSPECIFIED.,.F.,.F.,(4,2,2,2,2,2,2,2,
4),(9.19004041809617E-16,0.00254332115550819,0.00381498173326183,0.00445081202213868,
0.00476872716657715,0.00492768473879635,0.00500716352490594,0.00504690291796077,
0.0050866423110156),.UNSPECIFIED.);
#5713=B_SPLINE_CURVE_WITH_KNOTS('',3,(#209584,#209585,#209586,#209587,#209588,
#209589,#209590,#209591,#209592,#209593,#209594,#209595,#209596,#209597,
#209598,#209599,#209600,#209601,#209602,#209603,#209604,#209605,#209606,
#209607,#209608,#209609,#209610,#209611,#209612,#209613,#209614,#209615,
#209616,#209617,#209618,#209619,#209620,#209621,#209622,#209623,#209624,
#209625,#209626,#209627,#209628,#209629,#209630,#209631,#209632,#209633,
#209634,#209635,#209636,#209637,#209638,#209639,#209640,#209641,#209642,
#209643,#209644,#209645,#209646,#209647,#209648,#209649,#209650,#209651,
#209652,#209653,#209654,#209655,#209656,#209657,#209658,#209659,#209660,
#209661,#209662,#209663,#209664,#209665,#209666,#209667,#209668,#209669,
#209670,#209671,#209672,#209673,#209674,#209675,#209676,#209677,#209678,
#209679,#209680),.UNSPECIFIED.,.F.,.F.,(4,3,3,3,3,3,3,3,3,3,3,3,3,3,3,3,
3,3,3,3,3,3,3,3,3,3,3,3,3,3,3,3,4),(0.,0.0138775285159946,0.0263638591569942,
0.0379447519617947,0.0486412646310953,0.0508344497447169,0.0653856475986571,
0.0787319799100734,0.0858260410294844,0.105561629787405,0.123439328425312,
0.138689316605115,0.165941329943547,0.19093791381173,0.214525800517685,
0.215934497679913,0.252600765134276,0.286679270362538,0.318148735572388,
0.326400669130735,0.374710481742207,0.419592700784505,0.460839040374595,
0.482156546551197,0.54530149924857,0.603918811955974,0.657495913758009,
0.699491765232357,0.780512945753581,0.855736405104934,0.927868202552467,
0.994072321442603,1.),.UNSPECIFIED.);
#5714=B_SPLINE_CURVE_WITH_KNOTS('',3,(#209738,#209739,#209740,#209741,#209742,
#209743,#209744,#209745,#209746,#209747,#209748,#209749,#209750,#209751,
#209752,#209753,#209754,#209755,#209756,#209757,#209758,#209759,#209760,
#209761,#209762,#209763,#209764,#209765,#209766,#209767,#209768,#209769,
#209770,#209771,#209772,#209773,#209774,#209775,#209776,#209777,#209778,
#209779,#209780,#209781,#209782,#209783,#209784,#209785,#209786,#209787,
#209788,#209789,#209790,#209791,#209792,#209793,#209794,#209795,#209796,
#209797,#209798,#209799,#209800,#209801,#209802,#209803,#209804,#209805,
#209806,#209807,#209808,#209809,#209810,#209811,#209812,#209813,#209814,
#209815,#209816,#209817,#209818,#209819,#209820,#209821,#209822,#209823,
#209824,#209825,#209826,#209827,#209828,#209829,#209830,#209831),
 .UNSPECIFIED.,.F.,.F.,(4,3,3,3,3,3,3,3,3,3,3,3,3,3,3,3,3,3,3,3,3,3,3,3,
3,3,3,3,3,3,3,4),(0.,0.0660388479518842,0.137757862277712,0.213874090227569,
0.300378565075664,0.354680588111974,0.411594223257197,0.47485576477693,
0.517586657220905,0.559251985910025,0.603199515032552,0.651841152392032,
0.673245241820224,0.705425371021804,0.739431720776586,0.776992864370152,
0.783656785143308,0.807195660453429,0.832000104243301,0.859138712389666,
0.86089437271487,0.878999038648541,0.898863662967972,0.91379488830539,0.926782431890997,
0.940841839198321,0.948858179523771,0.959313204820475,0.970816466407867,
0.983181220337405,0.997538681807663,1.),.UNSPECIFIED.);
#5715=B_SPLINE_CURVE_WITH_KNOTS('',3,(#209832,#209833,#209834,#209835,#209836,
#209837,#209838,#209839,#209840,#209841,#209842,#209843,#209844,#209845,
#209846,#209847,#209848,#209849,#209850,#209851,#209852,#209853,#209854,
#209855,#209856),.UNSPECIFIED.,.F.,.F.,(4,3,3,3,3,3,3,3,4),(0.,4.03932117393399E-5,
8.08651294214249E-5,0.000161907626915798,0.000324108918069935,0.000648595245071396,
0.00129766017874913,0.00259586603175174,0.00519236941687791),
 .UNSPECIFIED.);
#5716=B_SPLINE_CURVE_WITH_KNOTS('',3,(#209918,#209919,#209920,#209921,#209922,
#209923,#209924,#209925,#209926,#209927,#209928,#209929,#209930,#209931,
#209932,#209933,#209934,#209935,#209936,#209937,#209938,#209939,#209940,
#209941,#209942,#209943,#209944,#209945,#209946,#209947,#209948,#209949,
#209950,#209951,#209952,#209953,#209954,#209955,#209956,#209957,#209958,
#209959,#209960,#209961,#209962,#209963,#209964,#209965,#209966,#209967,
#209968,#209969,#209970,#209971,#209972,#209973,#209974,#209975,#209976,
#209977,#209978,#209979,#209980,#209981,#209982,#209983,#209984,#209985,
#209986,#209987,#209988,#209989,#209990,#209991,#209992,#209993,#209994,
#209995,#209996,#209997,#209998,#209999,#210000,#210001,#210002,#210003,
#210004,#210005,#210006,#210007,#210008,#210009,#210010,#210011,#210012,
#210013,#210014),.UNSPECIFIED.,.F.,.F.,(4,3,3,3,3,3,3,3,3,3,3,3,3,3,3,3,
3,3,3,3,3,3,3,3,3,3,3,3,3,3,3,3,4),(0.,0.0135707811258087,0.0257973618116296,
0.0371444834848967,0.0476053919484337,0.0512894550931262,0.0663694894719871,
0.0801408578431507,0.0863831089251375,0.106233188646732,0.124191482070428,
0.139294493982615,0.166374253731966,0.191446547086697,0.214889264756252,
0.216518840441428,0.253015854179144,0.286946529617756,0.318281048146731,
0.326893697308868,0.37512471145545,0.419927206528289,0.461095796836194,
0.482498445678343,0.545340922048112,0.603700223197135,0.657049883728935,
0.699650410399617,0.780317183144115,0.85523809456008,0.92761904728004,0.993565053861809,
1.),.UNSPECIFIED.);
#5717=B_SPLINE_CURVE_WITH_KNOTS('',3,(#210017,#210018,#210019,#210020,#210021,
#210022,#210023,#210024,#210025,#210026,#210027,#210028,#210029,#210030,
#210031,#210032,#210033,#210034),.UNSPECIFIED.,.F.,.F.,(4,2,2,2,2,2,2,2,
4),(0.,0.00262931855771754,0.00394397783657636,0.00460130747600577,0.00492997229572051,
0.00509430470557792,0.00517647091050667,0.00521755401297108,0.00525863711543548),
 .UNSPECIFIED.);
#5718=B_SPLINE_CURVE_WITH_KNOTS('',3,(#210068,#210069,#210070,#210071,#210072,
#210073,#210074,#210075,#210076,#210077,#210078,#210079,#210080,#210081,
#210082,#210083,#210084,#210085,#210086,#210087,#210088,#210089,#210090,
#210091,#210092,#210093,#210094,#210095,#210096,#210097,#210098,#210099,
#210100,#210101,#210102,#210103,#210104,#210105,#210106,#210107,#210108,
#210109,#210110,#210111,#210112,#210113,#210114,#210115,#210116,#210117,
#210118,#210119,#210120,#210121,#210122,#210123,#210124,#210125,#210126,
#210127,#210128,#210129,#210130,#210131,#210132,#210133,#210134,#210135,
#210136,#210137,#210138,#210139,#210140,#210141,#210142,#210143,#210144,
#210145,#210146,#210147,#210148,#210149,#210150,#210151,#210152,#210153,
#210154,#210155,#210156,#210157,#210158,#210159,#210160,#210161,#210162,
#210163,#210164,#210165,#210166,#210167),.UNSPECIFIED.,.F.,.F.,(4,3,3,3,
3,3,3,3,3,3,3,3,3,3,3,3,3,3,3,3,3,3,3,3,3,3,3,3,3,3,3,3,3,4),(0.,0.0156250000000012,
0.0625000000000047,0.0937500000000208,0.109375000000029,0.117187500000046,
0.123521240792477,0.125000000000063,0.140625000000092,0.182242701318326,
0.187500000000178,0.218750000000236,0.234375000000265,0.242187500000279,
0.248811697549323,0.250000000000293,0.259894607749493,0.265625000000329,
0.322815512042762,0.375000000000577,0.429301576080171,0.437500000000718,
0.468750000000776,0.484375000000792,0.492187500000788,0.500000000000784,
0.510043502713035,0.612883296558313,0.625000000000588,0.717261013975742,
0.750000000000392,0.857991169889234,0.963554025874452,1.),.UNSPECIFIED.);
#5719=B_SPLINE_CURVE_WITH_KNOTS('',3,(#210168,#210169,#210170,#210171,#210172,
#210173,#210174,#210175,#210176,#210177,#210178,#210179,#210180,#210181,
#210182,#210183,#210184,#210185,#210186,#210187,#210188,#210189,#210190,
#210191,#210192,#210193,#210194,#210195,#210196,#210197,#210198,#210199,
#210200,#210201,#210202),.UNSPECIFIED.,.F.,.F.,(4,2,1,1,1,1,2,2,2,2,1,1,
2,2,2,2,1,1,1,2,2,4),(1.1089353930245E-7,0.125000000000895,0.187500000001354,
0.218750000001597,0.23437500000172,0.242187500001771,0.248046875001825,
0.250000000001843,0.375000000001895,0.437500000001909,0.468750000001917,
0.484375000001913,0.492187500001903,0.500000000001893,0.62500000000167,
0.687500000001546,0.718750000001486,0.734375000001438,0.742187500001393,
0.74609375000137,0.750000000001347,1.),.UNSPECIFIED.);
#5720=B_SPLINE_CURVE_WITH_KNOTS('',3,(#210260,#210261,#210262,#210263,#210264,
#210265,#210266,#210267,#210268,#210269,#210270,#210271,#210272,#210273,
#210274,#210275,#210276,#210277,#210278,#210279,#210280,#210281,#210282,
#210283,#210284),.UNSPECIFIED.,.F.,.F.,(4,3,3,3,3,3,3,3,4),(4.9065389333868E-17,
4.15775196007892E-5,8.32361282030658E-5,0.000166653476908059,0.000333604410320719,
0.000667590055213201,0.00133565310169655,0.00267185549873086,0.0053443518360984),
 .UNSPECIFIED.);
#5721=B_SPLINE_CURVE_WITH_KNOTS('',3,(#210285,#210286,#210287,#210288,#210289,
#210290,#210291,#210292,#210293,#210294,#210295,#210296,#210297,#210298,
#210299,#210300,#210301,#210302,#210303,#210304,#210305,#210306,#210307,
#210308,#210309,#210310,#210311,#210312,#210313,#210314,#210315,#210316,
#210317,#210318,#210319,#210320,#210321,#210322,#210323,#210324,#210325,
#210326,#210327,#210328,#210329,#210330,#210331,#210332,#210333,#210334,
#210335,#210336,#210337,#210338,#210339,#210340,#210341,#210342,#210343,
#210344,#210345,#210346,#210347,#210348,#210349,#210350,#210351,#210352,
#210353,#210354,#210355,#210356,#210357,#210358,#210359,#210360,#210361,
#210362,#210363,#210364,#210365,#210366,#210367,#210368,#210369,#210370,
#210371,#210372,#210373,#210374,#210375,#210376,#210377,#210378),
 .UNSPECIFIED.,.F.,.F.,(4,3,3,3,3,3,3,3,3,3,3,3,3,3,3,3,3,3,3,3,3,3,3,3,
3,3,3,3,3,3,3,4),(0.,0.065834090762222,0.137306570430488,0.213134649886981,
0.300236631091948,0.354496304796746,0.411178610110194,0.474156885636163,
0.517275325911139,0.558829344637946,0.602654437698862,0.65115886647553,
0.672792203999343,0.70485168831114,0.73872438206961,0.776133779531016,0.783116707833807,
0.806639447972133,0.831430832553541,0.858566765699478,0.860332482558115,
0.8783845180258,0.898197506292583,0.913275454353936,0.926158161133152,0.940105356609658,
0.948432049893693,0.958705571236069,0.970008019291287,0.982144963325018,
0.996260037816924,1.),.UNSPECIFIED.);
#5722=B_SPLINE_CURVE_WITH_KNOTS('',3,(#210394,#210395,#210396,#210397,#210398,
#210399,#210400),.UNSPECIFIED.,.F.,.F.,(4,3,4),(0.,0.000722422580495111,
0.00123518557486524),.UNSPECIFIED.);
#5723=B_SPLINE_CURVE_WITH_KNOTS('',3,(#210401,#210402,#210403,#210404,#210405,
#210406,#210407,#210408,#210409,#210410,#210411,#210412,#210413,#210414,
#210415,#210416,#210417,#210418,#210419,#210420,#210421,#210422,#210423,
#210424,#210425,#210426,#210427,#210428,#210429,#210430,#210431,#210432,
#210433,#210434,#210435,#210436,#210437,#210438,#210439,#210440,#210441,
#210442,#210443,#210444,#210445,#210446),.UNSPECIFIED.,.F.,.F.,(4,3,3,3,
3,3,3,3,3,3,3,3,3,3,3,4),(0.,0.052742842989654,0.105378129680294,0.125000000000152,
0.177350919706812,0.187500000000203,0.218750000000212,0.234375000000214,
0.242187500000217,0.246093750000209,0.2500000000002,0.375000000000174,0.445646917646005,
0.500000000000147,0.806305246709664,1.),.UNSPECIFIED.);
#5724=B_SPLINE_CURVE_WITH_KNOTS('',3,(#210474,#210475,#210476,#210477,#210478,
#210479,#210480,#210481,#210482,#210483,#210484,#210485,#210486,#210487,
#210488,#210489,#210490,#210491,#210492,#210493,#210494,#210495,#210496,
#210497,#210498,#210499,#210500,#210501,#210502,#210503,#210504,#210505,
#210506,#210507,#210508),.UNSPECIFIED.,.F.,.F.,(4,2,2,1,1,1,2,2,2,2,1,2,
2,2,2,1,1,1,2,2,4),(0.,0.124999999999531,0.18749999999931,0.218749999999199,
0.234374999999143,0.242187499999117,0.246093749999103,0.24999999999909,
0.374999999999434,0.437499999999608,0.468749999999694,0.484374999999727,
0.49999999999976,0.624999999999942,0.687500000000033,0.718750000000096,
0.734375000000149,0.742187500000195,0.746093750000197,0.7500000000002,0.999999975394086),
 .UNSPECIFIED.);
#5725=B_SPLINE_CURVE_WITH_KNOTS('',3,(#210510,#210511,#210512,#210513,#210514,
#210515,#210516,#210517,#210518,#210519,#210520,#210521,#210522,#210523,
#210524,#210525,#210526,#210527,#210528),.UNSPECIFIED.,.F.,.F.,(4,2,2,2,
1,2,2,2,2,4),(6.19941202265524E-9,0.249999999999908,0.374999999999861,0.406249999999859,
0.437499999999856,0.499999999999882,0.624999999999895,0.687499999999901,
0.749999999999908,1.),.UNSPECIFIED.);
#5726=B_SPLINE_CURVE_WITH_KNOTS('',3,(#210529,#210530,#210531,#210532,#210533,
#210534,#210535,#210536,#210537,#210538,#210539,#210540,#210541),
 .UNSPECIFIED.,.F.,.F.,(4,3,3,3,4),(0.,0.350293314944234,0.5,0.75,1.),
 .UNSPECIFIED.);
#5727=B_SPLINE_CURVE_WITH_KNOTS('',3,(#210574,#210575,#210576,#210577,#210578,
#210579,#210580,#210581,#210582,#210583,#210584,#210585,#210586,#210587,
#210588,#210589,#210590,#210591,#210592,#210593,#210594,#210595,#210596,
#210597,#210598,#210599,#210600,#210601,#210602,#210603,#210604,#210605,
#210606,#210607,#210608,#210609,#210610,#210611,#210612,#210613,#210614,
#210615,#210616,#210617,#210618,#210619),.UNSPECIFIED.,.F.,.F.,(4,3,3,3,
3,3,3,3,3,3,3,3,3,3,3,4),(0.,0.249999999999783,0.374999999999653,0.445711246785852,
0.499999999999523,0.624999999999394,0.687499999999349,0.718749999999327,
0.734374999999336,0.746093749999319,0.749999999999331,0.802225425262499,
0.854956889811044,0.907864634104767,0.960922572191772,1.),.UNSPECIFIED.);
#5728=B_SPLINE_CURVE_WITH_KNOTS('',3,(#210620,#210621,#210622,#210623,#210624,
#210625,#210626),.UNSPECIFIED.,.F.,.F.,(4,3,4),(0.,0.000727844608904283,
0.00121469382512387),.UNSPECIFIED.);
#5729=B_SPLINE_CURVE_WITH_KNOTS('',3,(#210669,#210670,#210671,#210672,#210673,
#210674,#210675,#210676,#210677,#210678,#210679,#210680,#210681,#210682,
#210683,#210684,#210685,#210686,#210687,#210688,#210689,#210690,#210691,
#210692,#210693,#210694,#210695),.UNSPECIFIED.,.F.,.F.,(4,2,1,2,2,2,1,1,
2,2,2,1,1,2,2,4),(0.,0.124999999999888,0.187499999999837,0.218749999999819,
0.249999999999801,0.374999999999777,0.437499999999764,0.468749999999755,
0.48437499999975,0.499999999999746,0.6249999999998,0.687499999999827,0.718749999999827,
0.734374999999829,0.749999999999832,1.),.UNSPECIFIED.);
#5730=B_SPLINE_CURVE_WITH_KNOTS('',3,(#210696,#210697,#210698,#210699,#210700,
#210701,#210702,#210703,#210704,#210705,#210706,#210707,#210708,#210709,
#210710,#210711,#210712,#210713,#210714,#210715,#210716,#210717,#210718,
#210719),.UNSPECIFIED.,.F.,.F.,(4,2,2,1,1,1,1,2,2,2,2,2,2,4),(0.,0.250000000000058,
0.375000000000071,0.437500000000069,0.468750000000072,0.484375000000074,
0.492187500000075,0.49609375000008,0.500000000000086,0.62500000000011,0.687500000000122,
0.718750000000128,0.750000000000135,1.),.UNSPECIFIED.);
#5731=B_SPLINE_CURVE_WITH_KNOTS('',3,(#210773,#210774,#210775,#210776,#210777,
#210778,#210779,#210780,#210781,#210782,#210783,#210784,#210785,#210786,
#210787,#210788,#210789,#210790,#210791,#210792,#210793,#210794,#210795),
 .UNSPECIFIED.,.F.,.F.,(4,2,2,2,2,2,2,1,1,1,2,2,4),(0.,0.125000000000141,
0.187500000000215,0.218750000000266,0.250000000000316,0.375000000000535,
0.43750000000064,0.468750000000692,0.484375000000707,0.492187500000705,
0.496093750000704,0.500000000000703,1.),.UNSPECIFIED.);
#5732=B_SPLINE_CURVE_WITH_KNOTS('',3,(#210796,#210797,#210798,#210799,#210800,
#210801,#210802,#210803,#210804,#210805,#210806,#210807,#210808,#210809,
#210810,#210811,#210812,#210813,#210814,#210815,#210816,#210817,#210818,
#210819,#210820,#210821,#210822,#210823,#210824,#210825,#210826,#210827,
#210828),.UNSPECIFIED.,.F.,.F.,(4,2,1,1,2,2,2,1,1,2,2,2,2,2,2,1,2,2,4),
(0.,0.125000000000212,0.187500000000329,0.218750000000376,0.234375000000397,
0.250000000000419,0.375000000000466,0.437500000000487,0.468750000000496,
0.484375000000501,0.500000000000505,0.562500000000444,0.625000000000383,
0.687500000000321,0.75000000000026,0.812500000000199,0.84375000000017,0.87500000000014,
1.),.UNSPECIFIED.);
#5733=B_SPLINE_CURVE_WITH_KNOTS('',3,(#212647,#212648,#212649,#212650,#212651,
#212652,#212653,#212654,#212655,#212656),.UNSPECIFIED.,.F.,.F.,(4,2,2,2,
4),(0.229465105224976,0.24878272102183,0.282449783617402,0.324570636098563,
0.324953676133515),.UNSPECIFIED.);
#5734=B_SPLINE_CURVE_WITH_KNOTS('',3,(#212691,#212692,#212693,#212694,#212695,
#212696,#212697,#212698,#212699,#212700),.UNSPECIFIED.,.F.,.F.,(4,2,2,2,
4),(-0.000383040042044683,0.,0.0421208528204372,0.0757879156854754,0.0951055316369486),
 .UNSPECIFIED.);
#5735=B_SPLINE_CURVE_WITH_KNOTS('',3,(#212710,#212711,#212712,#212713,#212714,
#212715,#212716,#212717,#212718,#212719),.UNSPECIFIED.,.F.,.F.,(4,2,2,2,
4),(0.229465097061585,0.248782712171685,0.282449773570366,0.324570624548349,
0.324953664553108),.UNSPECIFIED.);
#5736=B_SPLINE_CURVE_WITH_KNOTS('',3,(#212754,#212755,#212756,#212757,#212758,
#212759,#212760,#212761,#212762,#212763),.UNSPECIFIED.,.F.,.F.,(4,2,2,2,
4),(-0.000383040050378712,1.21072856601456E-15,0.0421208532697368,0.0757879164922472,
0.0951055326488294),.UNSPECIFIED.);
#5737=B_SPLINE_CURVE_WITH_KNOTS('',3,(#212773,#212774,#212775,#212776,#212777,
#212778,#212779,#212780,#212781,#212782),.UNSPECIFIED.,.F.,.F.,(4,2,2,2,
4),(0.229465099488756,0.248782714803057,0.282449776557603,0.324570627982376,
0.324953667995646),.UNSPECIFIED.);
#5738=B_SPLINE_CURVE_WITH_KNOTS('',3,(#212817,#212818,#212819,#212820,#212821,
#212822,#212823,#212824,#212825,#212826),.UNSPECIFIED.,.F.,.F.,(4,2,2,2,
4),(-0.000383039996431936,0.,0.0421208505751745,0.0757879116535588,0.095105526579897),
 .UNSPECIFIED.);
#5739=B_SPLINE_CURVE_WITH_KNOTS('',3,(#212832,#212833,#212834,#212835,#212836,
#212837,#212838,#212839,#212840,#212841),.UNSPECIFIED.,.F.,.F.,(4,2,2,2,
4),(0.229465073530738,0.248782686661591,0.282449744610596,0.324570591252679,
0.324953631169658),.UNSPECIFIED.);
#5740=B_SPLINE_CURVE_WITH_KNOTS('',3,(#212880,#212881,#212882,#212883,#212884,
#212885,#212886,#212887,#212888,#212889),.UNSPECIFIED.,.F.,.F.,(4,2,2,2,
4),(-0.000383039917846548,0.,0.042120846689148,0.075787904675495,0.0951055178277825),
 .UNSPECIFIED.);
#5741=B_SPLINE_CURVE_WITH_KNOTS('',3,(#213089,#213090,#213091,#213092,#213093,
#213094,#213095,#213096,#213097,#213098,#213099,#213100,#213101,#213102,
#213103,#213104,#213105,#213106,#213107,#213108,#213109,#213110,#213111,
#213112,#213113,#213114,#213115,#213116,#213117,#213118,#213119,#213120,
#213121,#213122,#213123,#213124,#213125,#213126,#213127,#213128,#213129,
#213130,#213131,#213132,#213133,#213134,#213135,#213136,#213137,#213138,
#213139,#213140),.UNSPECIFIED.,.F.,.F.,(4,3,3,3,3,3,3,3,3,3,3,3,3,3,3,3,
3,4),(0.,0.00570218474091234,0.0124164787169346,0.0258456091874862,0.052708361918506,
0.106470460366992,0.214291739632625,0.317553434342842,0.421799620076628,
0.5,0.590995103774971,0.656293369359574,0.748411394066377,0.839734838233114,
0.885082497885734,0.97491039354239,0.999679933047398,1.),.UNSPECIFIED.);
#5742=B_SPLINE_CURVE_WITH_KNOTS('',3,(#213142,#213143,#213144,#213145,#213146,
#213147,#213148,#213149,#213150,#213151,#213152,#213153,#213154,#213155,
#213156,#213157,#213158,#213159,#213160,#213161,#213162,#213163,#213164,
#213165,#213166,#213167,#213168,#213169,#213170,#213171,#213172,#213173,
#213174,#213175),.UNSPECIFIED.,.F.,.F.,(4,3,3,3,3,3,3,3,3,3,3,4),(0.,0.137478057277644,
0.273420104059381,0.407374454225706,0.5,0.620341176999436,0.739318733841433,
0.80587229841711,0.896219091184997,0.9990234375,0.999068147311954,1.),
 .UNSPECIFIED.);
#5743=B_SPLINE_CURVE_WITH_KNOTS('',3,(#213178,#213179,#213180,#213181,#213182,
#213183,#213184,#213185,#213186,#213187,#213188,#213189,#213190,#213191,
#213192,#213193,#213194,#213195,#213196,#213197,#213198,#213199,#213200,
#213201,#213202,#213203,#213204,#213205,#213206,#213207,#213208,#213209,
#213210,#213211,#213212,#213213,#213214,#213215,#213216,#213217,#213218,
#213219,#213220,#213221,#213222,#213223,#213224,#213225,#213226,#213227,
#213228,#213229,#213230,#213231,#213232,#213233,#213234,#213235,#213236,
#213237,#213238,#213239,#213240,#213241,#213242,#213243,#213244,#213245,
#213246,#213247,#213248,#213249,#213250,#213251,#213252,#213253,#213254,
#213255,#213256,#213257,#213258,#213259,#213260,#213261,#213262,#213263,
#213264,#213265,#213266,#213267,#213268,#213269,#213270,#213271,#213272,
#213273,#213274,#213275,#213276,#213277,#213278,#213279,#213280,#213281,
#213282,#213283,#213284,#213285,#213286,#213287,#213288,#213289),
 .UNSPECIFIED.,.F.,.F.,(4,3,3,3,3,3,3,3,3,3,3,3,3,3,3,3,3,3,3,3,3,3,3,3,
3,3,3,3,3,3,3,3,3,3,3,3,3,4),(0.,0.00106872167482631,0.00213668912630082,
0.00293590036761761,0.0029378487127682,0.00330316624931786,0.00348679918954151,
0.00367043213068583,0.00367231089096026,0.0044049638926048,0.0044067730691523,
0.00587402741638414,0.0058756974255364,0.0088121544640339,0.00881354613830458,
0.00917942034489251,0.00936305328548731,0.00945486975574288,0.00950077799084981,
0.00954668622593886,0.00954800831649663,0.0102812179878345,0.0102824704946887,
0.0117502815116473,0.0117513948510728,0.0146884085592774,0.0146892435638409,
0.0154229402821364,0.0157902061581132,0.0159738391126328,0.0160656555956372,
0.0161115638387771,0.0161574720830854,0.016158167920225,0.0176265356068806,
0.0176270922766091,0.0205649409893773,0.0235027897021455),.UNSPECIFIED.);
#5744=B_SPLINE_CURVE_WITH_KNOTS('',3,(#213290,#213291,#213292,#213293,#213294,
#213295,#213296,#213297,#213298,#213299,#213300,#213301,#213302,#213303,
#213304,#213305,#213306,#213307,#213308,#213309,#213310,#213311,#213312,
#213313,#213314,#213315,#213316,#213317,#213318,#213319,#213320,#213321,
#213322,#213323,#213324,#213325,#213326,#213327,#213328,#213329,#213330,
#213331,#213332,#213333,#213334,#213335,#213336,#213337,#213338,#213339,
#213340,#213341,#213342,#213343,#213344,#213345,#213346,#213347,#213348,
#213349,#213350,#213351,#213352,#213353,#213354,#213355,#213356,#213357,
#213358,#213359,#213360,#213361,#213362,#213363,#213364,#213365,#213366,
#213367,#213368,#213369,#213370,#213371,#213372,#213373,#213374,#213375,
#213376,#213377,#213378,#213379,#213380,#213381,#213382,#213383,#213384,
#213385,#213386,#213387,#213388,#213389,#213390,#213391,#213392,#213393,
#213394,#213395),.UNSPECIFIED.,.F.,.F.,(4,3,3,3,3,3,3,3,3,3,3,3,3,3,3,3,
3,3,3,3,3,3,3,3,3,3,3,3,3,3,3,3,3,3,3,4),(7.33112690889359E-11,0.00447014585407084,
0.00914986570716556,0.0185087890749796,0.0372224668762703,0.0746163803537859,
0.148246793986367,0.203469604210804,0.244886711879131,0.255815311626838,
0.330322389164154,0.369138034884112,0.375000000000005,0.437500000000005,
0.468750000000006,0.484375000000006,0.492187500000006,0.499138724547647,
0.500000000000006,0.516108728237381,0.555120919008716,0.593622058561214,
0.612985630693563,0.623334726960567,0.625000000000005,0.631597432104248,
0.632529868687029,0.65830781467943,0.674061695699477,0.70060922959337,0.727034623063786,
0.750000000000003,0.819699069590602,0.888646808802703,0.956324027361056,
1.),.UNSPECIFIED.);
#5745=B_SPLINE_CURVE_WITH_KNOTS('',3,(#213411,#213412,#213413,#213414),
 .UNSPECIFIED.,.F.,.F.,(4,4),(0.,0.000322395538615397),.UNSPECIFIED.);
#5746=B_SPLINE_CURVE_WITH_KNOTS('',3,(#213514,#213515,#213516,#213517,#213518,
#213519,#213520,#213521,#213522,#213523,#213524,#213525,#213526,#213527,
#213528,#213529,#213530,#213531,#213532,#213533,#213534,#213535,#213536,
#213537,#213538,#213539,#213540,#213541,#213542,#213543,#213544,#213545,
#213546,#213547,#213548,#213549,#213550),.UNSPECIFIED.,.F.,.F.,(4,3,3,3,
3,3,3,3,3,3,3,3,4),(0.,0.000191440270420746,0.000287160692730018,0.000382881236840893,
0.000574322481675385,0.000670043078002303,0.00076576358733981,0.000957204470373583,
0.00114864534416313,0.00124436578623717,0.00129222601008214,0.00134008623637552,
0.00153152717467962),.UNSPECIFIED.);
#5747=B_SPLINE_CURVE_WITH_KNOTS('',3,(#213551,#213552,#213553,#213554,#213555,
#213556,#213557,#213558,#213559,#213560,#213561,#213562,#213563,#213564,
#213565,#213566,#213567,#213568,#213569,#213570,#213571,#213572,#213573,
#213574,#213575,#213576,#213577,#213578,#213579,#213580,#213581,#213582,
#213583,#213584,#213585,#213586,#213587,#213588,#213589,#213590,#213591,
#213592,#213593,#213594,#213595,#213596,#213597,#213598,#213599,#213600,
#213601,#213602,#213603,#213604,#213605,#213606,#213607,#213608,#213609,
#213610,#213611,#213612,#213613,#213614,#213615,#213616,#213617,#213618,
#213619,#213620,#213621,#213622,#213623,#213624,#213625),.UNSPECIFIED.,
 .F.,.F.,(4,2,2,2,1,2,2,2,2,2,1,1,1,2,2,2,2,2,2,1,2,2,2,1,1,2,2,2,2,1,1,
2,2,2,2,1,1,2,2,2,2,2,4),(0.,0.0624999999999565,0.0937499999999354,0.109374999999925,
0.117187499999921,0.121093749999922,0.124999999999922,0.156250000000006,
0.171875000000048,0.18750000000009,0.218750000000164,0.2343750000002,0.242187500000218,
0.246093750000224,0.25000000000023,0.281250000000224,0.312500000000217,
0.34375000000021,0.35937500000021,0.367187500000206,0.371093750000201,0.375000000000196,
0.437500000000105,0.468750000000063,0.484375000000042,0.492187500000031,
0.50000000000002,0.562499999999868,0.593749999999794,0.609374999999759,
0.617187499999741,0.621093749999737,0.624999999999734,0.687499999999692,
0.718749999999674,0.734374999999663,0.742187499999661,0.746093749999661,
0.74999999999966,0.812499999999755,0.843749999999799,0.874999999999842,
1.),.UNSPECIFIED.);
#5748=B_SPLINE_CURVE_WITH_KNOTS('',3,(#213665,#213666,#213667,#213668,#213669,
#213670,#213671,#213672,#213673,#213674,#213675,#213676,#213677,#213678,
#213679,#213680,#213681,#213682,#213683),.UNSPECIFIED.,.F.,.F.,(4,3,3,3,
3,3,4),(0.,0.00503761689941682,0.00646885457540687,0.0129377091508137,0.0161721364385172,
0.0194065637262206,0.0258754183016275),.UNSPECIFIED.);
#5749=B_SPLINE_CURVE_WITH_KNOTS('',3,(#213684,#213685,#213686,#213687,#213688,
#213689,#213690,#213691,#213692,#213693,#213694,#213695,#213696,#213697,
#213698,#213699,#213700,#213701,#213702,#213703,#213704,#213705,#213706,
#213707,#213708,#213709,#213710,#213711,#213712,#213713,#213714,#213715,
#213716,#213717,#213718,#213719,#213720,#213721,#213722,#213723,#213724,
#213725,#213726,#213727,#213728,#213729,#213730,#213731,#213732,#213733,
#213734,#213735,#213736,#213737,#213738,#213739,#213740,#213741,#213742,
#213743,#213744,#213745,#213746,#213747,#213748,#213749,#213750,#213751,
#213752,#213753,#213754,#213755,#213756,#213757,#213758,#213759,#213760,
#213761,#213762,#213763,#213764,#213765,#213766,#213767,#213768,#213769,
#213770,#213771,#213772,#213773,#213774,#213775,#213776,#213777,#213778,
#213779,#213780,#213781,#213782,#213783,#213784,#213785,#213786,#213787,
#213788,#213789,#213790,#213791,#213792),.UNSPECIFIED.,.F.,.F.,(4,3,3,3,
3,3,3,3,3,3,3,3,3,3,3,3,3,3,3,3,3,3,3,3,3,3,3,3,3,3,3,3,3,3,3,3,4),(0.,
0.0624999999999447,0.124999999999889,0.187011718749834,0.218110068264968,
0.241135819705506,0.249023437499779,0.249999999999779,0.251447098061137,
0.292027665321456,0.333513832660559,0.372044971928076,0.374999999999662,
0.38487225586242,0.437499999999604,0.468749999999575,0.48437499999956,0.492187499999552,
0.496093749999549,0.498046874999547,0.499023437499547,0.499511718749547,
0.499999999999547,0.501761858639276,0.563380929319468,0.62499999999966,
0.675786892642834,0.723600741712145,0.749999999999773,0.778068207596557,
0.822278116509677,0.86523298278097,0.874999999999887,0.912812998100895,
0.950228509081889,0.987192663426709,1.),.UNSPECIFIED.);
#5750=B_SPLINE_CURVE_WITH_KNOTS('',3,(#213898,#213899,#213900,#213901,#213902,
#213903,#213904,#213905,#213906,#213907,#213908,#213909,#213910,#213911,
#213912,#213913,#213914,#213915,#213916,#213917,#213918,#213919,#213920,
#213921,#213922,#213923,#213924,#213925,#213926,#213927,#213928,#213929,
#213930,#213931,#213932,#213933,#213934,#213935,#213936,#213937,#213938,
#213939,#213940,#213941,#213942,#213943,#213944,#213945,#213946),
 .UNSPECIFIED.,.F.,.F.,(4,3,3,3,3,3,3,3,3,3,3,3,3,3,3,3,4),(0.,0.000127303360486361,
0.000254607331807631,0.000318259502487228,0.000381911773022019,0.000509216543183179,
0.000636521501341121,0.000763826506543775,0.000891131417838548,0.00101843609427484,
0.00114573874978534,0.00127303875321421,0.00140033769575051,0.00152763716845166,
0.00165493876244132,0.00178224406910835,0.00203687218854967),
 .UNSPECIFIED.);
#5751=B_SPLINE_CURVE_WITH_KNOTS('',3,(#213947,#213948,#213949,#213950,#213951,
#213952,#213953,#213954,#213955,#213956,#213957,#213958,#213959,#213960,
#213961,#213962,#213963,#213964,#213965,#213966,#213967,#213968,#213969,
#213970,#213971,#213972,#213973,#213974,#213975,#213976,#213977,#213978,
#213979,#213980,#213981,#213982,#213983,#213984,#213985,#213986,#213987,
#213988,#213989,#213990,#213991,#213992,#213993,#213994,#213995,#213996,
#213997,#213998,#213999,#214000,#214001,#214002,#214003,#214004,#214005,
#214006,#214007,#214008,#214009,#214010,#214011,#214012,#214013,#214014,
#214015,#214016,#214017,#214018,#214019,#214020,#214021,#214022,#214023,
#214024,#214025,#214026,#214027,#214028,#214029,#214030,#214031,#214032,
#214033,#214034,#214035,#214036,#214037,#214038,#214039),.UNSPECIFIED.,
 .F.,.F.,(4,2,2,2,1,1,2,2,2,2,2,2,2,2,2,2,2,2,1,1,1,2,2,1,2,2,2,1,2,2,2,
2,1,2,2,2,2,1,1,2,2,2,2,1,1,2,2,2,2,1,2,2,4),(0.,0.0624999999999063,0.0937499999998621,
0.109374999999839,0.117187499999827,0.121093749999825,0.123046874999823,
0.124999999999822,0.187499999999776,0.218749999999753,0.24999999999973,
0.31249999999968,0.320312499999672,0.328124999999663,0.343749999999657,
0.374999999999638,0.390624999999631,0.394531249999628,0.398437499999625,
0.406249999999626,0.437499999999632,0.468749999999639,0.484374999999646,
0.492187499999651,0.496093749999649,0.499999999999647,0.531249999999644,
0.546874999999642,0.554687499999642,0.562499999999642,0.593749999999643,
0.609374999999644,0.617187499999646,0.621093749999647,0.624999999999648,
0.687499999999675,0.718749999999691,0.734374999999699,0.742187499999701,
0.748046874999702,0.749999999999703,0.781249999999769,0.796874999999803,
0.804687499999818,0.808593749999826,0.810546874999831,0.812499999999835,
0.843749999999876,0.859374999999898,0.867187499999907,0.871093749999913,
0.874999999999919,1.),.UNSPECIFIED.);
#5752=B_SPLINE_CURVE_WITH_KNOTS('',3,(#214072,#214073,#214074,#214075),
 .UNSPECIFIED.,.F.,.F.,(4,4),(6.93889390390723E-18,0.000463834979289304),
 .UNSPECIFIED.);
#5753=B_SPLINE_CURVE_WITH_KNOTS('',3,(#214076,#214077,#214078,#214079,#214080,
#214081,#214082,#214083,#214084,#214085,#214086,#214087,#214088),
 .UNSPECIFIED.,.F.,.F.,(4,3,3,3,4),(3.53293614125829E-14,0.25717577121601,
0.517057560954111,0.782215252408013,1.),.UNSPECIFIED.);
#5754=B_SPLINE_CURVE_WITH_KNOTS('',3,(#214404,#214405,#214406,#214407,#214408,
#214409,#214410,#214411,#214412,#214413,#214414,#214415,#214416,#214417,
#214418,#214419,#214420,#214421,#214422,#214423,#214424,#214425,#214426,
#214427,#214428,#214429,#214430,#214431,#214432,#214433,#214434,#214435,
#214436,#214437,#214438,#214439,#214440,#214441,#214442,#214443,#214444,
#214445,#214446,#214447,#214448,#214449,#214450,#214451,#214452,#214453,
#214454,#214455,#214456,#214457,#214458,#214459,#214460,#214461,#214462,
#214463,#214464,#214465,#214466,#214467,#214468,#214469,#214470,#214471,
#214472,#214473,#214474,#214475,#214476,#214477,#214478,#214479,#214480,
#214481,#214482,#214483,#214484,#214485,#214486,#214487,#214488,#214489,
#214490,#214491,#214492,#214493,#214494,#214495,#214496,#214497,#214498,
#214499,#214500,#214501,#214502,#214503,#214504,#214505,#214506,#214507,
#214508,#214509,#214510,#214511,#214512,#214513,#214514,#214515,#214516,
#214517,#214518,#214519,#214520,#214521,#214522,#214523,#214524,#214525,
#214526,#214527,#214528,#214529,#214530,#214531,#214532,#214533,#214534,
#214535,#214536,#214537,#214538,#214539,#214540,#214541,#214542,#214543,
#214544,#214545,#214546,#214547,#214548,#214549,#214550,#214551,#214552,
#214553,#214554,#214555,#214556,#214557),.UNSPECIFIED.,.F.,.F.,(4,3,3,3,
3,3,3,3,3,3,3,3,3,3,3,3,3,3,3,3,3,3,3,3,3,3,3,3,3,3,3,3,3,3,3,3,3,3,3,3,
3,3,3,3,3,3,3,3,3,3,3,4),(1.04083408558608E-17,0.00250327328955152,0.00500654657910303,
0.00625818322387879,0.00688400154626667,0.00696222883656844,0.00704045612686793,
0.00719691070746254,0.00750981986865454,0.010013093158206,0.0112647298029818,
0.011577638964179,0.0117340935447715,0.0117732071899202,0.0118123208350694,
0.0118905481253697,0.0125163664477576,0.0137680030925333,0.015019639737309,
0.0175229130268605,0.0175620266720094,0.0176011403171581,0.0176793676074551,
0.0178358221880486,0.0181487313492361,0.0187745496716364,0.0200261863164121,
0.0225294596059636,0.0226076868962739,0.022646800541427,0.0226859141865788,
0.0228423687671764,0.0231552779283514,0.0237810962507394,0.0250327328955151,
0.0275360061850667,0.0281618245074545,0.0283182790880578,0.028396506378356,
0.0284356200235045,0.0284747336686529,0.0287876428298423,0.0300392794746181,
0.0325425527641696,0.0331683710865575,0.0332465983768559,0.0333248256671528,
0.033481280247746,0.0337941894089454,0.0350458260537211,0.0375490993432726,
0.0400523726328241),.UNSPECIFIED.);
#5755=B_SPLINE_CURVE_WITH_KNOTS('',3,(#214559,#214560,#214561,#214562,#214563,
#214564,#214565,#214566,#214567,#214568,#214569,#214570,#214571,#214572,
#214573,#214574,#214575,#214576,#214577,#214578,#214579,#214580,#214581,
#214582,#214583,#214584,#214585,#214586,#214587,#214588,#214589,#214590,
#214591,#214592),.UNSPECIFIED.,.F.,.F.,(4,3,3,3,3,3,3,3,3,3,3,4),(3.16237554060526E-11,
0.00769621628560935,0.0942246885002856,0.188514052913123,0.268067768599901,
0.366694922218767,0.467383535651208,0.5,0.624300582161452,0.746194067844642,
0.873097033922321,1.),.UNSPECIFIED.);
#5756=B_SPLINE_CURVE_WITH_KNOTS('',3,(#214594,#214595,#214596,#214597,#214598,
#214599),.UNSPECIFIED.,.F.,.F.,(4,2,4),(0.,0.5,1.),.UNSPECIFIED.);
#5757=B_SPLINE_CURVE_WITH_KNOTS('',3,(#214601,#214602,#214603,#214604,#214605,
#214606,#214607,#214608,#214609,#214610,#214611,#214612,#214613,#214614,
#214615,#214616,#214617,#214618,#214619,#214620,#214621,#214622,#214623,
#214624,#214625),.UNSPECIFIED.,.F.,.F.,(4,3,3,3,3,3,3,3,4),(3.07872546239425E-8,
0.205970371403195,0.247195775727949,0.449140217199346,0.496232918574816,
0.695053534951905,0.747153201208519,0.943375398914435,1.),.UNSPECIFIED.);
#5758=B_SPLINE_CURVE_WITH_KNOTS('',3,(#214627,#214628,#214629,#214630,#214631,
#214632,#214633,#214634,#214635,#214636,#214637,#214638,#214639,#214640,
#214641,#214642,#214643,#214644,#214645,#214646,#214647,#214648,#214649,
#214650,#214651,#214652,#214653,#214654,#214655,#214656,#214657,#214658,
#214659,#214660,#214661,#214662,#214663,#214664,#214665,#214666,#214667,
#214668,#214669,#214670,#214671,#214672,#214673,#214674,#214675,#214676,
#214677,#214678,#214679,#214680,#214681,#214682,#214683,#214684,#214685,
#214686,#214687,#214688,#214689,#214690,#214691,#214692,#214693,#214694,
#214695,#214696,#214697,#214698,#214699,#214700,#214701,#214702,#214703,
#214704,#214705,#214706,#214707,#214708,#214709,#214710,#214711,#214712,
#214713,#214714,#214715,#214716,#214717,#214718,#214719,#214720,#214721,
#214722,#214723,#214724,#214725,#214726,#214727,#214728,#214729,#214730,
#214731,#214732,#214733,#214734,#214735,#214736,#214737,#214738,#214739,
#214740,#214741,#214742,#214743,#214744,#214745,#214746,#214747,#214748,
#214749,#214750,#214751,#214752,#214753,#214754,#214755,#214756,#214757,
#214758,#214759,#214760,#214761,#214762,#214763,#214764,#214765,#214766,
#214767,#214768,#214769,#214770,#214771,#214772,#214773,#214774,#214775,
#214776,#214777,#214778,#214779,#214780,#214781,#214782,#214783,#214784,
#214785,#214786,#214787,#214788,#214789,#214790,#214791,#214792,#214793,
#214794,#214795,#214796,#214797,#214798,#214799,#214800,#214801),
 .UNSPECIFIED.,.F.,.F.,(4,3,3,3,3,3,3,3,3,3,3,3,3,3,3,3,3,3,3,3,3,3,3,3,
3,3,3,3,3,3,3,3,3,3,3,3,3,3,3,3,3,3,3,3,3,3,3,3,3,3,3,3,3,3,3,3,3,3,4),
(5.11034703543556E-8,0.000873397419564922,0.0042500144715355,0.0110025729195959,
0.0245010336941165,0.0640615231347867,0.0782432330913535,0.117418545504279,
0.124999999999962,0.187499999999943,0.234374999999928,0.244074093365877,
0.249999999999923,0.28691180927552,0.312499999999901,0.343749999999891,
0.359374999999886,0.367187499999884,0.371093749999882,0.373046874999882,
0.374999999999882,0.389263941687661,0.421832640387145,0.437499999999877,
0.438011301743273,0.465579486605632,0.468749999999874,0.480420548010491,
0.484293531293508,0.484374999999873,0.485520093773314,0.486781273444035,
0.488347437529155,0.488715417527697,0.49104828189574,0.492091101543253,
0.492494932064152,0.498046874999872,0.498383440689722,0.499999999999872,
0.54381309779903,0.587574177420254,0.624999999999904,0.672300987356324,
0.720762729405673,0.749999999999936,0.780535590518307,0.800739932311164,
0.828389269516647,0.854590150943252,0.874999999999968,0.904680252492238,
0.936356112347426,0.952858265257535,0.97669791610675,0.988587589368534,
0.994528743976525,0.997498877793861,0.99999999333144),.UNSPECIFIED.);
#5759=B_SPLINE_CURVE_WITH_KNOTS('',3,(#214803,#214804,#214805,#214806,#214807,
#214808,#214809,#214810,#214811,#214812,#214813,#214814,#214815,#214816,
#214817,#214818,#214819,#214820,#214821,#214822,#214823,#214824,#214825,
#214826,#214827,#214828,#214829,#214830,#214831,#214832,#214833,#214834,
#214835,#214836,#214837,#214838,#214839,#214840,#214841,#214842,#214843,
#214844,#214845),.UNSPECIFIED.,.F.,.F.,(4,3,3,3,3,3,3,3,3,3,3,3,3,3,4),
(0.,0.00521624725809631,0.0219557443112584,0.127779125462104,0.155680996700394,
0.266876415174393,0.378071833648393,0.5,0.652665472244447,0.678222244348951,
0.841762036962165,0.931561558766766,0.972431017039262,0.994218849932195,
1.),.UNSPECIFIED.);
#5760=B_SPLINE_CURVE_WITH_KNOTS('',3,(#214846,#214847,#214848,#214849,#214850,
#214851,#214852,#214853,#214854,#214855,#214856,#214857,#214858,#214859,
#214860,#214861,#214862,#214863,#214864,#214865,#214866,#214867,#214868,
#214869,#214870,#214871,#214872,#214873,#214874,#214875,#214876,#214877,
#214878,#214879,#214880,#214881,#214882,#214883,#214884,#214885,#214886,
#214887,#214888,#214889,#214890,#214891,#214892,#214893,#214894,#214895,
#214896,#214897,#214898,#214899,#214900,#214901,#214902,#214903,#214904,
#214905,#214906,#214907,#214908,#214909,#214910,#214911,#214912),
 .UNSPECIFIED.,.F.,.F.,(4,3,3,3,3,3,3,3,3,3,3,3,3,3,3,3,3,3,3,3,3,3,4),
(0.,0.127017155003427,0.250000000000004,0.364050961127173,0.373592405032721,
0.375000000000005,0.437500000000007,0.468750000000006,0.484375000000006,
0.492187500000006,0.500000000000006,0.61402579368828,0.725538073484568,
0.742827926521692,0.853717851291447,0.92478861938177,0.969729339656795,
0.975,0.985309039289484,0.992130828740079,0.99375,0.997042240357058,1.),
 .UNSPECIFIED.);
#5761=B_SPLINE_CURVE_WITH_KNOTS('',3,(#214928,#214929,#214930,#214931),
 .UNSPECIFIED.,.F.,.F.,(4,4),(0.,0.000517487663021482),.UNSPECIFIED.);
#5762=B_SPLINE_CURVE_WITH_KNOTS('',3,(#214932,#214933,#214934,#214935,#214936,
#214937,#214938,#214939,#214940,#214941,#214942,#214943,#214944,#214945,
#214946,#214947),.UNSPECIFIED.,.F.,.F.,(4,3,3,3,3,4),(0.,0.25,0.492721003519506,
0.732246481544643,0.967977404015073,1.),.UNSPECIFIED.);
#5763=B_SPLINE_CURVE_WITH_KNOTS('',3,(#215064,#215065,#215066,#215067,#215068,
#215069,#215070,#215071,#215072,#215073,#215074,#215075,#215076,#215077,
#215078,#215079,#215080,#215081,#215082,#215083,#215084,#215085,#215086,
#215087,#215088,#215089,#215090,#215091,#215092,#215093,#215094,#215095,
#215096,#215097,#215098,#215099,#215100,#215101,#215102,#215103,#215104,
#215105,#215106,#215107,#215108,#215109),.UNSPECIFIED.,.F.,.F.,(4,3,3,3,
3,3,3,3,3,3,3,3,3,3,3,4),(6.93889390390723E-18,0.000249844530040024,0.000374757201987747,
0.000499665804996625,0.000624572083127522,0.000749477780116718,0.000874384639619365,
0.000999294405453595,0.00124911879765639,0.00137403129062446,0.00149894371772633,
0.0016238558811297,0.00168631180212291,0.00174876758300643,0.00187367862553572,
0.00199858881090719),.UNSPECIFIED.);
#5764=B_SPLINE_CURVE_WITH_KNOTS('',3,(#215110,#215111,#215112,#215113,#215114,
#215115,#215116,#215117,#215118,#215119,#215120,#215121,#215122,#215123,
#215124,#215125,#215126,#215127,#215128,#215129,#215130,#215131,#215132,
#215133,#215134,#215135,#215136,#215137,#215138,#215139,#215140,#215141,
#215142,#215143,#215144,#215145,#215146,#215147,#215148,#215149,#215150,
#215151,#215152,#215153,#215154,#215155,#215156,#215157,#215158,#215159,
#215160,#215161,#215162,#215163,#215164,#215165,#215166,#215167,#215168,
#215169,#215170,#215171,#215172,#215173,#215174,#215175,#215176,#215177,
#215178,#215179,#215180,#215181,#215182,#215183,#215184,#215185,#215186,
#215187,#215188,#215189,#215190,#215191,#215192,#215193,#215194,#215195,
#215196,#215197,#215198,#215199,#215200,#215201,#215202,#215203,#215204,
#215205,#215206,#215207,#215208,#215209,#215210,#215211,#215212,#215213,
#215214,#215215,#215216,#215217,#215218,#215219,#215220,#215221,#215222,
#215223,#215224,#215225,#215226,#215227,#215228,#215229,#215230,#215231,
#215232,#215233,#215234,#215235,#215236,#215237,#215238,#215239,#215240,
#215241,#215242,#215243,#215244,#215245,#215246,#215247,#215248,#215249,
#215250,#215251,#215252,#215253,#215254,#215255,#215256,#215257,#215258,
#215259,#215260,#215261,#215262,#215263,#215264,#215265,#215266,#215267,
#215268,#215269,#215270,#215271,#215272,#215273,#215274,#215275,#215276,
#215277,#215278,#215279,#215280,#215281,#215282,#215283,#215284,#215285,
#215286,#215287,#215288,#215289,#215290,#215291,#215292,#215293,#215294,
#215295,#215296,#215297,#215298,#215299,#215300,#215301,#215302,#215303,
#215304,#215305,#215306,#215307,#215308,#215309,#215310,#215311,#215312,
#215313,#215314,#215315,#215316,#215317,#215318,#215319,#215320,#215321,
#215322,#215323,#215324,#215325,#215326,#215327,#215328,#215329,#215330,
#215331,#215332,#215333,#215334,#215335,#215336,#215337,#215338,#215339,
#215340,#215341,#215342,#215343,#215344,#215345,#215346,#215347,#215348,
#215349,#215350,#215351,#215352,#215353),.UNSPECIFIED.,.F.,.F.,(4,3,3,3,
3,3,3,3,3,3,3,3,3,3,3,3,3,3,3,3,3,3,3,3,3,3,3,3,3,3,3,3,3,3,3,3,3,3,3,3,
3,3,3,3,3,3,3,3,3,3,3,3,3,3,3,3,3,3,3,3,3,3,3,3,3,3,3,3,3,3,3,3,3,3,3,3,
3,3,3,3,3,4),(0.,0.0176762168154105,0.0369288430396893,0.0625000000000662,
0.0804000847057079,0.0937500000001003,0.108534387348399,0.109375000000121,
0.117187500000132,0.121093750000141,0.123592830383238,0.125000000000149,
0.140625000000149,0.155299847822507,0.156250000000149,0.169812069115432,
0.171875000000153,0.175781156354155,0.179687500000153,0.186769743781012,
0.187500000000153,0.218750000000149,0.234375000000148,0.242187500000148,
0.246093750000152,0.249721061039022,0.250000000000157,0.267171415929118,
0.283690610775299,0.299270948687442,0.30601050866871,0.31250000000016,0.32812500000016,
0.344367416171609,0.362170588585856,0.375000000000162,0.396143546472783,
0.406250000000162,0.421425997586886,0.421875000000158,0.429687500000155,
0.436857136050967,0.437500000000152,0.464627815166797,0.468750000000132,
0.484375000000125,0.496966596898197,0.500000000000118,0.522165361571699,
0.530572459240834,0.531250000000112,0.548581690940993,0.562500000000106,
0.5837268904211,0.593750000000099,0.609375000000098,0.617187500000094,0.624043972239538,
0.62500000000009,0.631234248578734,0.687500000000071,0.718750000000065,
0.734375000000063,0.740976426461612,0.750000000000061,0.812500000000059,
0.843750000000054,0.85937500000005,0.860151897939662,0.867187500000048,
0.871093750000046,0.873046875000039,0.875000000000032,0.894490298314019,
0.912568234704668,0.928964010240284,0.937500000000016,0.953125000000012,
0.967043443278746,0.98046419054641,0.993247432378915,1.),.UNSPECIFIED.);
#5765=B_SPLINE_CURVE_WITH_KNOTS('',3,(#215393,#215394,#215395,#215396,#215397,
#215398,#215399,#215400,#215401,#215402,#215403,#215404,#215405,#215406,
#215407,#215408,#215409,#215410,#215411,#215412,#215413,#215414),
 .UNSPECIFIED.,.F.,.F.,(4,3,3,3,3,3,3,4),(9.81307786677359E-18,0.00542754419074161,
0.00715193125010651,0.014303862500213,0.0178798281252662,0.0214557937503195,
0.0280312223938665,0.028607725000426),.UNSPECIFIED.);
#5766=B_SPLINE_CURVE_WITH_KNOTS('',3,(#215415,#215416,#215417,#215418,#215419,
#215420,#215421,#215422,#215423,#215424,#215425,#215426,#215427,#215428,
#215429,#215430,#215431,#215432,#215433,#215434,#215435,#215436,#215437,
#215438,#215439,#215440,#215441,#215442,#215443,#215444,#215445,#215446,
#215447,#215448,#215449,#215450,#215451,#215452,#215453,#215454,#215455,
#215456,#215457,#215458,#215459,#215460,#215461,#215462,#215463,#215464,
#215465,#215466,#215467,#215468,#215469,#215470,#215471,#215472,#215473,
#215474,#215475,#215476,#215477,#215478,#215479,#215480,#215481,#215482,
#215483,#215484,#215485,#215486,#215487,#215488,#215489,#215490,#215491,
#215492,#215493,#215494,#215495,#215496,#215497,#215498,#215499,#215500,
#215501,#215502,#215503,#215504,#215505,#215506,#215507,#215508,#215509,
#215510,#215511,#215512,#215513,#215514,#215515,#215516,#215517,#215518,
#215519,#215520,#215521,#215522,#215523,#215524,#215525,#215526,#215527,
#215528,#215529,#215530,#215531,#215532),.UNSPECIFIED.,.F.,.F.,(4,3,3,3,
3,3,3,3,3,3,3,3,3,3,3,3,3,3,3,3,3,3,3,3,3,3,3,3,3,3,3,3,3,3,3,3,3,3,3,4),
(0.,0.0588562399508839,0.116099365452458,0.125000000000124,0.180790191521428,
0.215150955135839,0.237429157520627,0.24951171875025,0.25000000000025,0.251302670656806,
0.285017840611363,0.317872441773445,0.349454566382291,0.375000000000254,
0.388817631691855,0.426956164769927,0.437500000000256,0.468750000000257,
0.484375000000258,0.492187500000258,0.496093750000257,0.498046875000257,
0.499023437500257,0.499755859375256,0.500000000000256,0.501787124098895,
0.555536630444185,0.612771063976521,0.625000000000192,0.671073302300544,
0.71439559262535,0.750000000000128,0.779782388171214,0.819625737711521,
0.858392751693001,0.875000000000064,0.909733146934382,0.944132077001742,
0.978130950313487,1.),.UNSPECIFIED.);
#5767=B_SPLINE_CURVE_WITH_KNOTS('',3,(#215638,#215639,#215640,#215641,#215642,
#215643,#215644,#215645,#215646,#215647,#215648,#215649,#215650,#215651,
#215652,#215653,#215654,#215655,#215656,#215657,#215658,#215659,#215660,
#215661,#215662,#215663,#215664,#215665,#215666,#215667,#215668,#215669,
#215670,#215671,#215672,#215673,#215674,#215675,#215676,#215677,#215678,
#215679,#215680,#215681,#215682,#215683,#215684,#215685,#215686),
 .UNSPECIFIED.,.F.,.F.,(4,3,3,3,3,3,3,3,3,3,3,3,3,3,3,3,4),(0.,0.000209907523070278,
0.000262386427442229,0.000314865930148693,0.000419826308247615,0.000524787812645559,
0.000629749598530388,0.000839670635464471,0.000892150044011657,0.000944629442448278,
0.00104958821836654,0.00115454698196066,0.00125950575196963,0.00136446454713245,
0.00146942338618816,0.00157438228787588,0.00167934127092895),
 .UNSPECIFIED.);
#5768=B_SPLINE_CURVE_WITH_KNOTS('',3,(#215687,#215688,#215689,#215690,#215691,
#215692,#215693,#215694,#215695,#215696,#215697,#215698,#215699,#215700,
#215701,#215702,#215703,#215704,#215705,#215706,#215707,#215708,#215709,
#215710,#215711,#215712,#215713,#215714,#215715,#215716,#215717,#215718,
#215719,#215720,#215721,#215722,#215723,#215724,#215725,#215726,#215727,
#215728,#215729,#215730,#215731,#215732,#215733,#215734,#215735,#215736,
#215737,#215738,#215739,#215740,#215741,#215742,#215743,#215744,#215745,
#215746,#215747,#215748,#215749,#215750,#215751,#215752,#215753,#215754,
#215755,#215756,#215757,#215758,#215759,#215760),.UNSPECIFIED.,.F.,.F.,
(4,2,2,2,2,2,2,1,2,2,2,2,1,1,2,2,2,2,2,1,1,2,2,2,2,1,2,2,2,2,2,2,2,2,2,
2,2,2,2,4),(0.,0.0625000000001367,0.125000000000273,0.18750000000041,0.250000000000547,
0.281250000000612,0.289062500000624,0.296875000000636,0.31250000000065,
0.375000000000693,0.390625000000707,0.398437500000714,0.406250000000721,
0.437500000000757,0.468750000000793,0.484375000000813,0.492187500000822,
0.500000000000831,0.531250000000825,0.546875000000818,0.554687500000816,
0.558593750000814,0.562500000000813,0.593750000000799,0.609375000000795,
0.617187500000788,0.621093750000784,0.62500000000078,0.656250000000682,
0.67187500000064,0.679687500000624,0.687500000000607,0.718750000000543,
0.734375000000509,0.742187500000493,0.750000000000478,0.812500000000359,
0.875000000000239,0.93750000000012,1.),.UNSPECIFIED.);
#5769=B_SPLINE_CURVE_WITH_KNOTS('',3,(#215793,#215794,#215795,#215796),
 .UNSPECIFIED.,.F.,.F.,(4,4),(3.46944695195361E-18,0.000487799384074577),
 .UNSPECIFIED.);
#5770=B_SPLINE_CURVE_WITH_KNOTS('',3,(#215797,#215798,#215799,#215800,#215801,
#215802,#215803,#215804,#215805,#215806,#215807,#215808,#215809),
 .UNSPECIFIED.,.F.,.F.,(4,3,3,3,4),(0.,0.252285837043446,0.507554797966739,
0.768599643387901,1.),.UNSPECIFIED.);
#5771=B_SPLINE_CURVE_WITH_KNOTS('',3,(#216124,#216125,#216126,#216127,#216128,
#216129,#216130,#216131,#216132,#216133,#216134,#216135,#216136,#216137,
#216138,#216139,#216140,#216141,#216142,#216143,#216144,#216145,#216146,
#216147,#216148,#216149,#216150,#216151,#216152,#216153,#216154,#216155,
#216156,#216157,#216158,#216159,#216160,#216161,#216162,#216163,#216164,
#216165,#216166,#216167,#216168,#216169,#216170,#216171,#216172,#216173,
#216174,#216175,#216176,#216177,#216178,#216179,#216180,#216181,#216182,
#216183,#216184,#216185,#216186,#216187,#216188,#216189,#216190,#216191,
#216192,#216193,#216194,#216195,#216196,#216197,#216198,#216199,#216200,
#216201,#216202,#216203,#216204,#216205,#216206,#216207,#216208,#216209,
#216210,#216211,#216212,#216213,#216214,#216215,#216216,#216217,#216218,
#216219,#216220,#216221,#216222,#216223),.UNSPECIFIED.,.F.,.F.,(4,3,3,3,
3,3,3,3,3,3,3,3,3,3,3,3,3,3,3,3,3,3,3,3,3,3,3,3,3,3,3,3,3,4),(0.,0.0779136589103248,
0.0882485852908278,0.162928798217767,0.173223837107886,0.187500000000003,
0.218750000000004,0.234375000000004,0.242187500000003,0.246093750000003,
0.248046875000003,0.250000000000003,0.256564631049091,0.29210193516486,
0.326726692869407,0.343750000000017,0.344829642597288,0.359375000000018,
0.36718750000002,0.37109375000002,0.374620536182301,0.375000000000021,0.424706860044605,
0.474200684446832,0.500000000000017,0.503570887679342,0.596730160309364,
0.66791097260569,0.718750000000011,0.736275753263558,0.750000000000009,
0.834360354991451,0.983724571879412,0.999998925899605),.UNSPECIFIED.);
#5772=B_SPLINE_CURVE_WITH_KNOTS('',3,(#216225,#216226,#216227,#216228,#216229,
#216230,#216231,#216232,#216233,#216234,#216235,#216236,#216237,#216238,
#216239,#216240,#216241,#216242,#216243,#216244,#216245,#216246,#216247,
#216248,#216249,#216250,#216251,#216252,#216253,#216254,#216255,#216256,
#216257,#216258,#216259,#216260,#216261,#216262,#216263,#216264,#216265,
#216266,#216267,#216268,#216269,#216270),.UNSPECIFIED.,.F.,.F.,(4,3,3,3,
3,3,3,3,3,3,3,3,3,3,3,4),(0.,0.00545528971435915,0.280220483963937,0.288806896284233,
0.293100102444383,0.297393308604534,0.314566133245131,0.348911782526331,
0.417603081088726,0.554985678213514,0.829750872463092,0.967133469587875,
0.984306294228478,0.992892706548774,0.996446353274387,0.999999999838516),
 .UNSPECIFIED.);
#5773=B_SPLINE_CURVE_WITH_KNOTS('',3,(#216272,#216273,#216274,#216275,#216276,
#216277,#216278,#216279,#216280,#216281,#216282,#216283,#216284,#216285,
#216286,#216287,#216288,#216289,#216290,#216291,#216292),.UNSPECIFIED.,
 .F.,.F.,(4,2,1,1,2,2,2,2,1,1,1,2,4),(0.,0.0156250000000005,0.0312500000000011,
0.0625000000000017,0.125000000000002,0.250000000000001,0.5,0.749999999999998,
0.874999999999998,0.937499999999999,0.968749999999999,0.984375,1.),
 .UNSPECIFIED.);
#5774=B_SPLINE_CURVE_WITH_KNOTS('',3,(#216293,#216294,#216295,#216296,#216297,
#216298,#216299,#216300,#216301,#216302,#216303,#216304,#216305,#216306,
#216307,#216308,#216309,#216310,#216311,#216312,#216313,#216314,#216315,
#216316,#216317,#216318,#216319,#216320,#216321,#216322,#216323),
 .UNSPECIFIED.,.F.,.F.,(4,3,3,3,3,3,3,3,3,3,4),(0.,0.00474675381323911,
0.00781250000000027,0.0156250000000005,0.030266067385407,0.0625000000000007,
0.0813046945943531,0.125,0.18338195186464,0.591690975932319,1.),
 .UNSPECIFIED.);
#5775=B_SPLINE_CURVE_WITH_KNOTS('',3,(#216324,#216325,#216326,#216327,#216328,
#216329,#216330,#216331,#216332,#216333,#216334,#216335,#216336,#216337,
#216338,#216339,#216340,#216341,#216342,#216343,#216344,#216345,#216346,
#216347,#216348,#216349,#216350,#216351,#216352,#216353,#216354,#216355,
#216356,#216357,#216358,#216359,#216360,#216361,#216362,#216363,#216364,
#216365,#216366,#216367,#216368,#216369,#216370,#216371,#216372,#216373,
#216374,#216375,#216376,#216377,#216378,#216379,#216380,#216381,#216382,
#216383,#216384,#216385,#216386,#216387,#216388,#216389,#216390,#216391,
#216392,#216393,#216394,#216395,#216396,#216397,#216398,#216399,#216400,
#216401,#216402,#216403,#216404,#216405,#216406,#216407,#216408,#216409,
#216410,#216411,#216412,#216413,#216414,#216415,#216416,#216417,#216418,
#216419,#216420,#216421,#216422,#216423,#216424,#216425,#216426,#216427,
#216428,#216429,#216430,#216431,#216432,#216433,#216434,#216435,#216436,
#216437,#216438,#216439,#216440,#216441,#216442,#216443,#216444,#216445,
#216446,#216447,#216448,#216449,#216450,#216451,#216452,#216453,#216454,
#216455,#216456,#216457,#216458,#216459,#216460,#216461,#216462,#216463,
#216464,#216465,#216466,#216467,#216468,#216469,#216470,#216471,#216472,
#216473,#216474,#216475,#216476,#216477,#216478,#216479,#216480,#216481,
#216482,#216483,#216484,#216485,#216486,#216487,#216488,#216489,#216490,
#216491,#216492,#216493,#216494,#216495,#216496,#216497,#216498,#216499,
#216500,#216501,#216502,#216503,#216504,#216505,#216506,#216507,#216508,
#216509,#216510,#216511,#216512,#216513,#216514,#216515,#216516,#216517,
#216518,#216519,#216520,#216521,#216522,#216523,#216524,#216525,#216526,
#216527,#216528,#216529,#216530,#216531,#216532,#216533,#216534,#216535,
#216536,#216537,#216538,#216539,#216540,#216541,#216542,#216543,#216544,
#216545,#216546,#216547,#216548,#216549,#216550,#216551,#216552,#216553,
#216554,#216555,#216556,#216557,#216558,#216559,#216560,#216561,#216562,
#216563,#216564,#216565,#216566,#216567,#216568,#216569,#216570,#216571,
#216572,#216573,#216574,#216575,#216576,#216577,#216578,#216579,#216580,
#216581,#216582,#216583,#216584,#216585,#216586,#216587,#216588,#216589,
#216590,#216591,#216592,#216593,#216594,#216595,#216596,#216597,#216598,
#216599,#216600,#216601,#216602,#216603),.UNSPECIFIED.,.F.,.F.,(4,3,3,3,
3,3,3,3,3,3,3,3,3,3,3,3,3,3,3,3,3,3,3,3,3,3,3,3,3,3,3,3,3,3,3,3,3,3,3,3,
3,3,3,3,3,3,3,3,3,3,3,3,3,3,3,3,3,3,3,3,3,3,3,3,3,3,3,3,3,3,3,3,3,3,3,3,
3,3,3,3,3,3,3,3,3,3,3,3,3,3,3,3,3,4),(3.46944695195361E-18,0.00251321548397822,
0.00252618216605191,0.00431652351870221,0.00502643096795645,0.0050523631196123,
0.00628303870994556,0.00631545541643819,0.00639439869545078,0.00647334192364792,
0.00663122827834575,0.00691134258094011,0.0069470009329515,0.00753964645193465,
0.00757854646468453,0.0100528619359129,0.0101047288113934,0.0106811658069074,
0.0107362741734552,0.0109953177424047,0.0110520469397126,0.0111309901351074,
0.0111704617311478,0.0112099333265805,0.011309469677902,0.0113678197142864,
0.0125660774198911,0.0126309107307065,0.0149188987799849,0.0150792929038693,
0.0151570929628482,0.0163359006458585,0.0164201840296525,0.016964204516853,
0.0170517295614678,0.0172783564523502,0.0173675023312846,0.0174464455249122,
0.0174859171210369,0.017525388716906,0.0175925083878475,0.0176832737054695,
0.0182566011601652,0.0188331435913378,0.018943209217914,0.0195351789828337,
0.0201057238718258,0.0201875071813319,0.0211909991553901,0.0221894422408006,
0.0226189393558041,0.0226772058573312,0.0227557547052305,0.0227950386486702,
0.0228343240121577,0.0229330912913013,0.0229914102955462,0.0232472432267986,
0.0233051459757238,0.0238755470977931,0.0239316652744055,0.0251321548397822,
0.0251846404969728,0.0276453703237604,0.0276905921486432,0.0289019780657495,
0.0289435691951432,0.0291001957684129,0.0291785065739474,0.0292568164041345,
0.029530281936744,0.0295700559705409,0.0301585858077386,0.0301965438884586,
0.0326718012917168,0.0327024956320061,0.0339284090337059,0.0339554719475575,
0.0340337845090096,0.0340729398943169,0.0341120949376171,0.0342425609692031,
0.0342687153965129,0.0345567129047004,0.0345819593578056,0.035185016775695,
0.0352084472800867,0.0376982322596731,0.0377143994811302,0.0383006441491539,
0.0388957484754305,0.0394801741002239,0.0400377689422836,0.0402114477436513),
 .UNSPECIFIED.);
#5776=B_SPLINE_CURVE_WITH_KNOTS('',3,(#216605,#216606,#216607,#216608,#216609,
#216610,#216611,#216612,#216613,#216614,#216615,#216616,#216617,#216618,
#216619,#216620,#216621,#216622,#216623,#216624,#216625,#216626,#216627,
#216628,#216629,#216630,#216631,#216632,#216633,#216634,#216635,#216636,
#216637,#216638,#216639,#216640,#216641,#216642,#216643,#216644,#216645,
#216646,#216647,#216648,#216649,#216650,#216651,#216652,#216653),
 .UNSPECIFIED.,.F.,.F.,(4,3,3,3,3,3,3,3,3,3,3,3,3,3,3,3,4),(0.,0.00265415439005135,
0.102720312462561,0.20133059727198,0.249999999999989,0.353342179378799,
0.374999999999984,0.43749999999998,0.468749999999978,0.484374999999978,
0.496753448869959,0.499999999999978,0.601051550778275,0.702354920594771,
0.804823358871256,0.909563908684595,1.),.UNSPECIFIED.);
#5777=B_SPLINE_CURVE_WITH_KNOTS('',3,(#216654,#216655,#216656,#216657,#216658,
#216659,#216660,#216661,#216662,#216663,#216664,#216665,#216666,#216667,
#216668,#216669,#216670,#216671,#216672,#216673,#216674,#216675,#216676,
#216677,#216678,#216679,#216680,#216681,#216682,#216683,#216684,#216685,
#216686,#216687,#216688,#216689,#216690,#216691,#216692,#216693,#216694,
#216695,#216696,#216697,#216698,#216699,#216700,#216701,#216702,#216703,
#216704,#216705,#216706,#216707,#216708,#216709,#216710,#216711,#216712,
#216713,#216714,#216715,#216716,#216717,#216718,#216719,#216720,#216721,
#216722,#216723,#216724,#216725,#216726),.UNSPECIFIED.,.F.,.F.,(4,3,3,3,
3,3,3,3,3,3,3,3,3,3,3,3,3,3,3,3,3,3,3,3,4),(4.05198363567377E-7,0.00787298863610522,
0.0273567818531982,0.0781878140360392,0.104285438977262,0.154412767520936,
0.203500430496265,0.24678211002478,0.250000000000018,0.33637967744521,0.375000000000026,
0.43750000000003,0.468750000000032,0.484375000000032,0.492187500000033,
0.496093750000033,0.500000000000032,0.647718153766782,0.745632761495269,
0.874942760220384,0.939328417322223,0.971461269619396,0.974303379404863,
0.987472851275835,1.),.UNSPECIFIED.);
#5778=B_SPLINE_CURVE_WITH_KNOTS('',3,(#216740,#216741,#216742,#216743,#216744,
#216745,#216746,#216747,#216748,#216749,#216750,#216751,#216752,#216753,
#216754,#216755,#216756,#216757,#216758,#216759,#216760,#216761),
 .UNSPECIFIED.,.F.,.F.,(4,3,3,3,3,3,3,4),(0.,0.176890528384024,0.345636984164273,
0.509227738123205,0.660395309268134,0.806605995633615,0.946450892839879,
1.),.UNSPECIFIED.);
#5779=B_SPLINE_CURVE_WITH_KNOTS('',3,(#216863,#216864,#216865,#216866,#216867,
#216868,#216869,#216870,#216871,#216872,#216873,#216874,#216875,#216876,
#216877,#216878,#216879,#216880,#216881,#216882,#216883,#216884,#216885,
#216886,#216887,#216888,#216889,#216890,#216891,#216892,#216893,#216894,
#216895,#216896,#216897,#216898,#216899,#216900,#216901,#216902,#216903,
#216904,#216905,#216906,#216907,#216908,#216909,#216910,#216911,#216912,
#216913,#216914,#216915,#216916,#216917,#216918,#216919,#216920,#216921,
#216922,#216923,#216924,#216925,#216926,#216927,#216928,#216929,#216930,
#216931,#216932,#216933,#216934,#216935,#216936,#216937,#216938,#216939,
#216940,#216941),.UNSPECIFIED.,.F.,.F.,(4,3,3,3,3,3,3,3,3,3,3,3,3,3,3,3,
3,3,3,3,3,3,3,3,3,3,4),(0.,0.0699362617129251,0.103904228120223,0.124999999999995,
0.137268630045529,0.20235451817345,0.249999999999989,0.265485387458136,
0.326032873596611,0.374999999999986,0.38653728259255,0.43428842418918,0.437499999999984,
0.444547027425897,0.473935618526858,0.492187499999978,0.498537282033062,
0.499999999999977,0.500942948294706,0.592037747362571,0.625127000188452,
0.717273178183023,0.749301981791401,0.840484550520233,0.87405473528525,
0.964870050196674,1.),.UNSPECIFIED.);
#5780=B_SPLINE_CURVE_WITH_KNOTS('',3,(#216942,#216943,#216944,#216945,#216946,
#216947,#216948,#216949,#216950,#216951,#216952,#216953,#216954,#216955,
#216956,#216957,#216958,#216959,#216960,#216961,#216962,#216963,#216964,
#216965,#216966,#216967,#216968,#216969,#216970,#216971,#216972,#216973,
#216974,#216975,#216976,#216977,#216978,#216979,#216980,#216981,#216982,
#216983,#216984,#216985,#216986,#216987,#216988,#216989,#216990,#216991,
#216992,#216993,#216994,#216995,#216996,#216997,#216998,#216999,#217000,
#217001,#217002,#217003,#217004,#217005,#217006,#217007,#217008,#217009,
#217010,#217011,#217012,#217013,#217014,#217015,#217016,#217017,#217018,
#217019,#217020,#217021,#217022,#217023,#217024,#217025,#217026,#217027,
#217028,#217029,#217030,#217031,#217032,#217033,#217034,#217035,#217036,
#217037,#217038,#217039,#217040,#217041,#217042,#217043,#217044,#217045,
#217046,#217047,#217048,#217049,#217050,#217051,#217052,#217053,#217054,
#217055,#217056,#217057,#217058,#217059,#217060,#217061,#217062,#217063,
#217064,#217065,#217066,#217067,#217068,#217069,#217070,#217071,#217072,
#217073,#217074,#217075,#217076,#217077,#217078,#217079,#217080,#217081,
#217082,#217083,#217084,#217085,#217086,#217087,#217088,#217089,#217090,
#217091,#217092,#217093,#217094,#217095,#217096,#217097,#217098,#217099,
#217100,#217101,#217102,#217103,#217104,#217105,#217106,#217107,#217108,
#217109,#217110,#217111,#217112,#217113,#217114,#217115,#217116,#217117,
#217118,#217119,#217120,#217121,#217122,#217123,#217124,#217125,#217126,
#217127,#217128,#217129,#217130,#217131,#217132,#217133,#217134,#217135,
#217136,#217137,#217138,#217139,#217140,#217141,#217142,#217143,#217144,
#217145,#217146,#217147,#217148,#217149,#217150,#217151,#217152,#217153,
#217154,#217155,#217156,#217157,#217158,#217159,#217160,#217161,#217162,
#217163,#217164,#217165,#217166,#217167,#217168,#217169,#217170,#217171,
#217172,#217173,#217174,#217175,#217176,#217177,#217178,#217179,#217180,
#217181,#217182,#217183,#217184,#217185,#217186,#217187,#217188),
 .UNSPECIFIED.,.F.,.F.,(4,3,3,3,3,3,3,3,3,3,3,3,3,3,3,3,3,3,3,3,3,3,3,3,
3,3,3,3,3,3,3,3,3,3,3,3,3,3,3,3,3,3,3,3,3,3,3,3,3,3,3,3,3,3,3,3,3,3,3,3,
3,3,3,3,3,3,3,3,3,3,3,3,3,3,3,3,3,3,3,3,3,3,4),(0.,0.0137545866432384,0.0492401835094905,
0.0625000000000268,0.0937500000000405,0.109375000000047,0.11718750000005,
0.123875958867671,0.125000000000053,0.174156395228104,0.20291116071406,
0.218750000000069,0.234375000000071,0.242187500000073,0.246093750000075,
0.250000000000078,0.281848408221954,0.312500000000087,0.34375000000009,
0.35937500000009,0.367187500000089,0.371093750000089,0.375000000000089,
0.397346070709233,0.437500000000074,0.468750000000068,0.484375000000062,
0.498046875000063,0.500000000000065,0.52073830350297,0.531250000000054,
0.54687500000005,0.554687500000049,0.558593750000048,0.560546875000049,
0.562500000000049,0.577571866921682,0.581137214692785,0.593750000000042,
0.608462325772321,0.609375000000036,0.617187500000037,0.621093750000035,
0.623046875000043,0.62402343750004,0.625000000000037,0.666535878910816,
0.687499999999788,0.718749999999663,0.7343749999996,0.74218749999957,0.749023437499547,
0.749999999999541,0.760356549744039,0.770430402015572,0.780504254287105,
0.792502672640471,0.796874999999502,0.804687499999497,0.808593749999494,
0.810546874999492,0.812115977136946,0.81249999999949,0.828352802307223,
0.843749999999467,0.859374999999458,0.867187499999452,0.871093749999448,
0.87384301473899,0.874999999999443,0.898739986678005,0.90624999999941,0.921874999999392,
0.929687499999384,0.93359374999938,0.936523437499377,0.937499999999376,
0.947583425348786,0.958066165670755,0.969573174789762,0.984786587394881,
0.995666532359992,1.),.UNSPECIFIED.);
#5781=B_SPLINE_CURVE_WITH_KNOTS('',3,(#217216,#217217,#217218,#217219,#217220,
#217221,#217222,#217223,#217224,#217225,#217226,#217227,#217228),
 .UNSPECIFIED.,.F.,.F.,(4,3,3,3,4),(6.93889390390723E-18,0.000381255516945798,
0.000469255885454269,0.000705402670155963,0.000942818873534133),
 .UNSPECIFIED.);
#5782=B_SPLINE_CURVE_WITH_KNOTS('',3,(#217229,#217230,#217231,#217232,#217233,
#217234,#217235,#217236,#217237,#217238,#217239,#217240,#217241,#217242,
#217243,#217244,#217245,#217246,#217247),.UNSPECIFIED.,.F.,.F.,(4,2,2,1,
1,1,2,2,2,2,4),(0.,0.124999999999029,0.187499999998545,0.21874999999831,
0.234374999998192,0.242187499998133,0.246093749998135,0.249999999998136,
0.374999999998442,0.499999999998747,1.),.UNSPECIFIED.);
#5783=B_SPLINE_CURVE_WITH_KNOTS('',3,(#217262,#217263,#217264,#217265,#217266,
#217267,#217268,#217269,#217270,#217271,#217272,#217273,#217274,#217275,
#217276),.UNSPECIFIED.,.F.,.F.,(4,2,2,1,1,1,2,2,4),(0.,0.250000000000346,
0.375000000000519,0.437500000000606,0.468750000000651,0.484375000000672,
0.492187500000683,0.500000000000693,0.99998999934417),.UNSPECIFIED.);
#5784=B_SPLINE_CURVE_WITH_KNOTS('',3,(#217295,#217296,#217297,#217298,#217299,
#217300,#217301,#217302,#217303,#217304),.UNSPECIFIED.,.F.,.F.,(4,3,3,4),
(1.04998151009522E-15,7.57680534135841E-5,0.000160273665463363,0.000194799519911097),
 .UNSPECIFIED.);
#5785=B_SPLINE_CURVE_WITH_KNOTS('',3,(#217325,#217326,#217327,#217328,#217329,
#217330,#217331,#217332,#217333,#217334,#217335,#217336,#217337,#217338,
#217339,#217340,#217341,#217342,#217343,#217344,#217345,#217346,#217347,
#217348,#217349),.UNSPECIFIED.,.F.,.F.,(4,3,3,3,3,3,3,3,4),(1.42699696935763E-12,
0.134118179434847,0.269533840744077,0.405806590660504,0.5,0.627124388053351,
0.754010818070997,0.880892917577905,1.),.UNSPECIFIED.);
#5786=B_SPLINE_CURVE_WITH_KNOTS('',3,(#217754,#217755,#217756,#217757,#217758,
#217759,#217760,#217761,#217762,#217763,#217764,#217765,#217766,#217767,
#217768,#217769,#217770,#217771,#217772,#217773,#217774,#217775,#217776,
#217777,#217778,#217779,#217780,#217781,#217782,#217783,#217784,#217785,
#217786,#217787,#217788,#217789,#217790,#217791,#217792,#217793,#217794,
#217795,#217796,#217797,#217798,#217799,#217800,#217801,#217802,#217803,
#217804,#217805),.UNSPECIFIED.,.F.,.F.,(4,3,3,3,3,3,3,3,3,3,3,3,3,3,3,3,
3,4),(4.34856172578496E-12,0.0825964622752124,0.166298231137607,0.250000000000002,
0.34372743266562,0.401376017787723,0.468749999999996,0.486596533951206,
0.499999999999986,0.500286464469699,0.562714848352273,0.625720242594846,
0.691315601603277,0.749999999999993,0.81758269229801,0.886453217052764,
0.956347341619819,0.999958634704665),.UNSPECIFIED.);
#5787=B_SPLINE_CURVE_WITH_KNOTS('',3,(#217806,#217807,#217808,#217809,#217810,
#217811,#217812,#217813,#217814,#217815,#217816,#217817,#217818,#217819,
#217820,#217821,#217822,#217823,#217824,#217825,#217826,#217827,#217828,
#217829,#217830,#217831,#217832,#217833,#217834,#217835,#217836,#217837,
#217838,#217839,#217840,#217841,#217842,#217843,#217844,#217845,#217846,
#217847,#217848,#217849,#217850,#217851,#217852,#217853,#217854,#217855,
#217856,#217857,#217858,#217859,#217860,#217861,#217862,#217863,#217864,
#217865,#217866,#217867,#217868,#217869,#217870,#217871,#217872,#217873,
#217874,#217875,#217876,#217877,#217878,#217879,#217880,#217881,#217882,
#217883,#217884,#217885,#217886,#217887,#217888,#217889,#217890,#217891,
#217892,#217893,#217894,#217895,#217896,#217897,#217898,#217899,#217900,
#217901,#217902,#217903,#217904,#217905,#217906,#217907,#217908,#217909,
#217910,#217911,#217912,#217913,#217914,#217915,#217916,#217917,#217918,
#217919,#217920,#217921,#217922,#217923,#217924,#217925,#217926,#217927,
#217928,#217929,#217930,#217931,#217932,#217933,#217934,#217935,#217936,
#217937,#217938,#217939,#217940,#217941,#217942,#217943,#217944,#217945,
#217946,#217947,#217948,#217949,#217950,#217951,#217952,#217953,#217954,
#217955,#217956,#217957,#217958,#217959,#217960,#217961,#217962,#217963,
#217964,#217965,#217966,#217967,#217968,#217969,#217970,#217971,#217972,
#217973,#217974,#217975,#217976,#217977,#217978,#217979,#217980,#217981,
#217982,#217983,#217984,#217985,#217986,#217987,#217988,#217989,#217990,
#217991,#217992,#217993,#217994,#217995,#217996,#217997,#217998,#217999,
#218000,#218001,#218002,#218003,#218004,#218005,#218006,#218007,#218008,
#218009,#218010,#218011,#218012,#218013,#218014,#218015,#218016,#218017,
#218018,#218019,#218020,#218021,#218022,#218023,#218024,#218025,#218026,
#218027,#218028,#218029,#218030,#218031,#218032,#218033,#218034,#218035,
#218036,#218037,#218038,#218039,#218040,#218041,#218042,#218043,#218044,
#218045,#218046,#218047,#218048,#218049,#218050,#218051,#218052,#218053,
#218054,#218055,#218056,#218057,#218058,#218059,#218060,#218061,#218062,
#218063,#218064,#218065,#218066,#218067,#218068,#218069,#218070,#218071,
#218072,#218073,#218074,#218075,#218076,#218077,#218078,#218079,#218080,
#218081,#218082,#218083,#218084,#218085,#218086,#218087,#218088,#218089,
#218090,#218091,#218092,#218093,#218094,#218095,#218096,#218097,#218098,
#218099,#218100,#218101,#218102,#218103,#218104,#218105,#218106,#218107,
#218108,#218109,#218110,#218111,#218112,#218113,#218114,#218115,#218116,
#218117,#218118,#218119,#218120,#218121,#218122,#218123,#218124,#218125,
#218126,#218127,#218128,#218129,#218130,#218131,#218132,#218133,#218134,
#218135,#218136,#218137,#218138,#218139,#218140,#218141,#218142,#218143,
#218144,#218145,#218146,#218147,#218148,#218149,#218150,#218151,#218152,
#218153,#218154,#218155,#218156,#218157),.UNSPECIFIED.,.F.,.F.,(4,3,3,3,
3,3,3,3,3,3,3,3,3,3,3,3,3,3,3,3,3,3,3,3,3,3,3,3,3,3,3,3,3,3,3,3,3,3,3,3,
3,3,3,3,3,3,3,3,3,3,3,3,3,3,3,3,3,3,3,3,3,3,3,3,3,3,3,3,3,3,3,3,3,3,3,3,
3,3,3,3,3,3,3,3,3,3,3,3,3,3,3,3,3,3,3,3,3,3,3,3,3,3,3,3,3,3,3,3,3,3,3,3,
3,3,3,3,3,4),(7.6340784608749E-10,0.000458642979624075,0.00148039977483381,
0.00155548413886924,0.00215808125410714,0.00351929599465174,0.00375138748261493,
0.00431616250821427,0.00485043313467506,0.00595000606436421,0.00647424376232141,
0.00814921412208154,0.00863232501642855,0.0103483019189587,0.0107904062705357,
0.0114478221282486,0.0118694468975892,0.011997552011241,0.0121349909920189,
0.0121693507398505,0.0122037104862686,0.0122724299699281,0.012408967211116,
0.0125473080812288,0.0129484875246428,0.0164016813619231,0.0169452741711653,
0.0172646500328571,0.019144189598669,0.0194227312869643,0.0196939101106168,
0.0198313397462725,0.0198485184451541,0.0198656971433723,0.0199000545385089,
0.0199622516004911,0.019968769328592,0.0202436289341077,0.0205017719140178,
0.0213430827748677,0.0215808125410714,0.023660808471361,0.0257408044016506,
0.0258969750492855,0.0270590117429158,0.0280550563033925,0.0289136017549253,
0.0291340969304461,0.0301383324656715,0.030172686249919,0.0302070399948121,
0.0302131375574996,0.0302757474855599,0.0304131631667517,0.0306879973674717,
0.0312376772927354,0.0323370846027418,0.0345293000657137,0.0345360999801471,
0.0356083406927672,0.0356357138934573,0.0366115735239226,0.0366873813198207,
0.036735364064563,0.0376935360434175,0.0377664219468742,0.037834874245495,
0.03797230394085,0.0380066611974582,0.0380410184323685,0.0381097329274824,
0.038305942260401,0.0383845939060418,0.0388454625739277,0.0389343227662998,
0.0416287480698926,0.0431616250821419,0.0433319227699236,0.0455053529354617,
0.0474777875903559,0.0477291370889975,0.0480173079038827,0.0482787598919197,
0.0483474623355832,0.0483818135645227,0.0484161648055707,0.0485535700013951,
0.0485568282174095,0.048828382082034,0.049635868844463,0.0499276530066721,
0.0510269469117059,0.05179395009857,0.0521261923582703,0.0543244689093608,
0.0554235143696222,0.0559730160990558,0.056110112606784,0.0562477622140428,
0.0563164484206554,0.0563851344750846,0.0565225060213207,0.0566496329203107,
0.0571891532338374,0.0582681938608909,0.0599454964430095,0.0604262751149979,
0.06091874539064,0.0623709320756,0.0625843563691049,0.0631171315120619,
0.0647424376232119,0.0653151792302629,0.0669005188773189,0.0675129021160856,
0.0679795595043724,0.0688633830386992,0.0690586001314259),.UNSPECIFIED.);
#5788=B_SPLINE_CURVE_WITH_KNOTS('',3,(#218159,#218160,#218161,#218162,#218163,
#218164,#218165,#218166,#218167,#218168,#218169,#218170,#218171,#218172,
#218173,#218174,#218175,#218176,#218177,#218178,#218179,#218180,#218181,
#218182,#218183,#218184,#218185,#218186,#218187,#218188,#218189,#218190,
#218191,#218192,#218193,#218194,#218195,#218196,#218197,#218198,#218199,
#218200,#218201,#218202,#218203,#218204,#218205,#218206,#218207,#218208,
#218209,#218210,#218211,#218212,#218213,#218214,#218215,#218216,#218217,
#218218,#218219,#218220,#218221,#218222,#218223,#218224,#218225,#218226,
#218227,#218228,#218229,#218230,#218231,#218232,#218233,#218234,#218235,
#218236,#218237),.UNSPECIFIED.,.F.,.F.,(4,3,3,3,3,3,3,3,3,3,3,3,3,3,3,3,
3,3,3,3,3,3,3,3,3,3,4),(4.77884326448819E-11,0.00202028309269962,0.0039176051110123,
0.00783365280887212,0.0156653625435356,0.0313274786564338,0.0626484630366808,
0.125294063429656,0.188446065875006,0.250307838177388,0.302395984903941,
0.3779647184045,0.445740485537048,0.499645843896646,0.561681656144702,0.577853278825029,
0.622127447016507,0.680957127046811,0.738153985517249,0.79371261558945,
0.822603609701943,0.847641311410194,0.899965028869779,0.938213647190648,
0.950728580880526,0.981074031663759,1.),.UNSPECIFIED.);
#5789=B_SPLINE_CURVE_WITH_KNOTS('',3,(#218239,#218240,#218241,#218242,#218243,
#218244,#218245,#218246,#218247,#218248,#218249,#218250,#218251,#218252,
#218253,#218254,#218255,#218256,#218257,#218258,#218259,#218260,#218261,
#218262,#218263,#218264,#218265,#218266,#218267,#218268,#218269,#218270,
#218271,#218272,#218273,#218274,#218275,#218276,#218277,#218278,#218279,
#218280,#218281,#218282,#218283,#218284,#218285,#218286,#218287,#218288,
#218289,#218290,#218291,#218292,#218293,#218294,#218295,#218296,#218297,
#218298,#218299,#218300,#218301,#218302,#218303,#218304,#218305),
 .UNSPECIFIED.,.F.,.F.,(4,3,3,3,3,3,3,3,3,3,3,3,3,3,3,3,3,3,3,3,3,3,4),
(0.,0.0312499999999975,0.0468749999999962,0.0546874999999938,0.0585937499999938,
0.0624999999999939,0.0977910955042792,0.124999999999995,0.187499999999997,
0.218749999999998,0.237790831202695,0.25,0.375000000000006,0.437500000000008,
0.46875000000001,0.482748988899476,0.484375000000011,0.492187500000011,
0.500000000000012,0.6282098955093,0.740654930187649,0.870327465093825,1.),
 .UNSPECIFIED.);
#5790=B_SPLINE_CURVE_WITH_KNOTS('',3,(#218307,#218308,#218309,#218310,#218311,
#218312,#218313,#218314,#218315,#218316,#218317,#218318,#218319,#218320,
#218321,#218322,#218323,#218324,#218325,#218326,#218327,#218328,#218329,
#218330,#218331,#218332,#218333,#218334,#218335,#218336,#218337,#218338,
#218339,#218340,#218341,#218342,#218343,#218344),.UNSPECIFIED.,.F.,.F.,
(4,1,1,2,2,2,1,1,2,2,2,2,2,1,2,2,2,1,1,1,2,2,4),(0.,0.00390625000009151,
0.00585937500013782,0.00732421875017266,0.00781250000018431,0.0117187500001906,
0.0136718750001931,0.0146484375001943,0.0151367187501945,0.0156250000001947,
0.0312500000001926,0.0625000000001896,0.12500000000018,0.187500000000171,
0.218750000000165,0.250000000000159,0.375000000000137,0.437500000000125,
0.46875000000012,0.484375000000117,0.492187500000115,0.500000000000114,
1.),.UNSPECIFIED.);
#5791=B_SPLINE_CURVE_WITH_KNOTS('',3,(#218346,#218347,#218348,#218349,#218350,
#218351,#218352,#218353,#218354,#218355,#218356,#218357,#218358,#218359,
#218360,#218361,#218362,#218363,#218364,#218365,#218366,#218367,#218368,
#218369,#218370,#218371,#218372,#218373,#218374,#218375,#218376,#218377),
 .UNSPECIFIED.,.F.,.F.,(4,2,1,1,1,2,2,2,2,2,2,1,2,2,2,2,2,4),(0.,0.0156250000000023,
0.0234375000000034,0.0273437500000047,0.0292968750000052,0.0302734375000052,
0.0312500000000052,0.0625000000000046,0.125000000000005,0.250000000000005,
0.375000000000005,0.437500000000005,0.468750000000005,0.500000000000005,
0.625000000000004,0.687500000000004,0.750000000000003,1.),.UNSPECIFIED.);
#5792=B_SPLINE_CURVE_WITH_KNOTS('',3,(#218379,#218380,#218381,#218382,#218383,
#218384,#218385,#218386,#218387,#218388,#218389,#218390,#218391,#218392,
#218393,#218394,#218395,#218396,#218397,#218398,#218399,#218400,#218401,
#218402,#218403,#218404,#218405,#218406,#218407,#218408,#218409,#218410,
#218411,#218412,#218413,#218414,#218415,#218416,#218417,#218418,#218419,
#218420,#218421,#218422,#218423,#218424,#218425,#218426,#218427,#218428,
#218429,#218430,#218431,#218432,#218433,#218434,#218435,#218436,#218437,
#218438,#218439,#218440,#218441,#218442,#218443,#218444,#218445,#218446,
#218447,#218448,#218449,#218450,#218451,#218452,#218453,#218454,#218455,
#218456,#218457,#218458,#218459,#218460,#218461,#218462,#218463,#218464,
#218465,#218466,#218467,#218468,#218469,#218470,#218471,#218472,#218473,
#218474,#218475,#218476,#218477,#218478,#218479,#218480,#218481,#218482,
#218483,#218484,#218485,#218486,#218487,#218488,#218489,#218490,#218491,
#218492,#218493,#218494,#218495,#218496,#218497,#218498,#218499,#218500,
#218501,#218502),.UNSPECIFIED.,.F.,.F.,(4,3,3,3,3,3,3,3,3,3,3,3,3,3,3,3,
3,3,3,3,3,3,3,3,3,3,3,3,3,3,3,3,3,3,3,3,3,3,3,3,3,4),(0.,0.00032758361939681,
0.00676055619332624,0.0229628150776129,0.039310820342462,0.0564454475397725,
0.0583030570676846,0.0625000000000044,0.0683593750000044,0.0698013305664106,
0.0702138167440786,0.0705630656159106,0.0762964552156621,0.0777123116125716,
0.0786023886535299,0.0929693901461635,0.0960501440206557,0.117390760019365,
0.122790494671226,0.125341744964798,0.175764617567141,0.187228865205509,
0.191986365790403,0.222675570066603,0.249528623808278,0.252764358890674,
0.336698626740585,0.421722401430846,0.437500000000002,0.468750000000002,
0.482174841649079,0.500000000000002,0.589596724551366,0.6784245448769,0.766897797949448,
0.854958523913957,0.909319437118939,0.963183385534347,0.967483243263316,
0.990177312386673,0.99692531213621,0.999999948688291),.UNSPECIFIED.);
#5793=B_SPLINE_CURVE_WITH_KNOTS('',3,(#218504,#218505,#218506,#218507,#218508,
#218509,#218510,#218511,#218512,#218513,#218514,#218515,#218516,#218517,
#218518,#218519,#218520,#218521,#218522,#218523,#218524,#218525,#218526,
#218527,#218528,#218529,#218530,#218531,#218532,#218533,#218534,#218535,
#218536),.UNSPECIFIED.,.F.,.F.,(4,2,2,2,1,2,2,2,2,1,1,2,2,2,1,1,2,2,4),
(0.,0.0312499999999877,0.0351562499999857,0.0371093749999851,0.0390624999999845,
0.0468749999999845,0.0624999999999847,0.0937499999999842,0.124999999999984,
0.187499999999982,0.218749999999982,0.234374999999983,0.249999999999983,
0.374999999999987,0.437499999999989,0.46874999999999,0.48437499999999,0.49999999999999,
0.999999981795557),.UNSPECIFIED.);
#5794=B_SPLINE_CURVE_WITH_KNOTS('',3,(#218537,#218538,#218539,#218540,#218541,
#218542,#218543,#218544,#218545,#218546,#218547,#218548,#218549,#218550,
#218551,#218552),.UNSPECIFIED.,.F.,.F.,(4,2,2,1,1,1,1,2,2,4),(0.,0.249999999999993,
0.37499999999999,0.437499999999989,0.468749999999988,0.484374999999988,
0.492187499999988,0.498046874999989,0.499999999999989,1.),.UNSPECIFIED.);
#5795=B_SPLINE_CURVE_WITH_KNOTS('',3,(#218573,#218574,#218575,#218576,#218577,
#218578),.UNSPECIFIED.,.F.,.F.,(4,2,4),(0.,0.500000000000001,0.999968221947089),
 .UNSPECIFIED.);
#5796=B_SPLINE_CURVE_WITH_KNOTS('',3,(#218594,#218595,#218596,#218597),
 .UNSPECIFIED.,.F.,.F.,(4,4),(1.05519109601004E-16,0.000332772401868219),
 .UNSPECIFIED.);
#5797=B_SPLINE_CURVE_WITH_KNOTS('',3,(#218598,#218599,#218600,#218601,#218602,
#218603,#218604),.UNSPECIFIED.,.F.,.F.,(4,3,4),(3.39934988877629E-17,8.80333921656039E-5,
0.000139297820483867),.UNSPECIFIED.);
#5798=B_SPLINE_CURVE_WITH_KNOTS('',3,(#218643,#218644,#218645,#218646,#218647,
#218648,#218649),.UNSPECIFIED.,.F.,.F.,(4,3,4),(0.,0.00037653926080856,
0.00075440118473929),.UNSPECIFIED.);
#5799=B_SPLINE_CURVE_WITH_KNOTS('',3,(#218650,#218651,#218652,#218653,#218654,
#218655,#218656,#218657,#218658,#218659,#218660,#218661,#218662),
 .UNSPECIFIED.,.F.,.F.,(4,2,2,1,2,2,4),(0.,0.249999999999973,0.374999999999955,
0.437499999999942,0.468749999999936,0.49999999999993,1.),.UNSPECIFIED.);
#5800=B_SPLINE_CURVE_WITH_KNOTS('',3,(#218744,#218745,#218746,#218747,#218748,
#218749,#218750,#218751,#218752,#218753,#218754,#218755,#218756,#218757,
#218758,#218759,#218760,#218761,#218762,#218763,#218764,#218765,#218766,
#218767,#218768,#218769,#218770,#218771,#218772,#218773,#218774,#218775,
#218776,#218777,#218778,#218779,#218780,#218781,#218782,#218783,#218784,
#218785,#218786,#218787,#218788,#218789,#218790,#218791,#218792,#218793,
#218794,#218795,#218796,#218797,#218798,#218799,#218800,#218801,#218802,
#218803,#218804,#218805,#218806,#218807,#218808,#218809,#218810,#218811,
#218812,#218813,#218814,#218815,#218816,#218817,#218818,#218819,#218820,
#218821,#218822),.UNSPECIFIED.,.F.,.F.,(4,3,3,3,3,3,3,3,3,3,3,3,3,3,3,3,
3,3,3,3,3,3,3,3,3,3,4),(0.,0.0844654919461902,0.122470941342419,0.207003614964972,
0.245798182809739,0.249999999999935,0.333296210281669,0.370668428198448,
0.374999999999902,0.441433008969332,0.496093749999876,0.497619617625721,
0.499999999999877,0.547503235522682,0.553623071983059,0.610885110373799,
0.702888851910236,0.730748815474926,0.749999999999938,0.793828402446633,
0.855095787109683,0.859466281586824,0.874999999999969,0.893379318442533,
0.928115077845369,0.972989979546055,0.999999999999993),.UNSPECIFIED.);
#5801=B_SPLINE_CURVE_WITH_KNOTS('',3,(#218823,#218824,#218825,#218826,#218827,
#218828,#218829,#218830,#218831,#218832,#218833,#218834,#218835,#218836,
#218837,#218838,#218839,#218840,#218841,#218842,#218843,#218844,#218845,
#218846,#218847,#218848,#218849,#218850,#218851,#218852,#218853,#218854,
#218855,#218856,#218857,#218858,#218859,#218860,#218861,#218862,#218863,
#218864,#218865,#218866,#218867,#218868,#218869,#218870,#218871,#218872,
#218873,#218874,#218875,#218876,#218877,#218878,#218879,#218880,#218881,
#218882,#218883,#218884,#218885,#218886,#218887,#218888,#218889,#218890,
#218891,#218892,#218893,#218894,#218895,#218896,#218897,#218898,#218899,
#218900,#218901,#218902,#218903,#218904,#218905,#218906,#218907,#218908,
#218909,#218910,#218911,#218912,#218913,#218914,#218915,#218916,#218917,
#218918,#218919,#218920,#218921,#218922,#218923,#218924,#218925,#218926,
#218927,#218928,#218929,#218930,#218931,#218932,#218933,#218934,#218935,
#218936,#218937,#218938,#218939,#218940,#218941,#218942,#218943,#218944,
#218945,#218946,#218947,#218948,#218949,#218950,#218951,#218952,#218953,
#218954,#218955,#218956,#218957,#218958,#218959,#218960,#218961,#218962,
#218963,#218964,#218965,#218966,#218967,#218968,#218969,#218970,#218971,
#218972,#218973,#218974,#218975,#218976,#218977,#218978,#218979,#218980,
#218981,#218982,#218983,#218984,#218985,#218986,#218987,#218988,#218989,
#218990,#218991,#218992,#218993,#218994,#218995,#218996,#218997,#218998,
#218999,#219000,#219001,#219002,#219003),.UNSPECIFIED.,.F.,.F.,(4,3,3,3,
3,3,3,3,3,3,3,3,3,3,3,3,3,3,3,3,3,3,3,3,3,3,3,3,3,3,3,3,3,3,3,3,3,3,3,3,
3,3,3,3,3,3,3,3,3,3,3,3,3,3,3,3,3,3,3,3,4),(0.,0.00666408113292331,0.0129639075512711,
0.0156250000000025,0.021368878326581,0.0234375000000028,0.027343750000003,
0.0312500000000032,0.0412694451432147,0.0468750000000061,0.0568048710303721,
0.0625000000000091,0.0766768025718624,0.090160869705112,0.0937500000000153,
0.0971456960406208,0.0989180593347306,0.101562500000017,0.109375000000019,
0.12500000000002,0.144362575322191,0.16321779851779,0.181421980887489,0.187500000000014,
0.195312500000014,0.199218750000013,0.201823967502558,0.203125000000012,
0.218750000000006,0.228153442731374,0.249999999999999,0.312499999999983,
0.343749999999977,0.348147427493963,0.351562499999975,0.359374999999974,
0.37499999999998,0.391144204108983,0.401883223401621,0.406249999999994,
0.421875000000003,0.430859737207603,0.437500000000011,0.457620056656504,
0.468750000000032,0.484375000000043,0.492187500000048,0.496093750000049,
0.50000000000005,0.550509377734149,0.579051287512532,0.636233117757933,
0.692439018597193,0.747357765783153,0.764210507176442,0.80695746796269,
0.849189186907056,0.890619527408069,0.930878773987873,0.975556510704755,
1.),.UNSPECIFIED.);
#5802=B_SPLINE_CURVE_WITH_KNOTS('',3,(#219033,#219034,#219035,#219036,#219037,
#219038,#219039,#219040,#219041,#219042,#219043,#219044,#219045,#219046,
#219047,#219048,#219049,#219050,#219051,#219052,#219053,#219054,#219055,
#219056,#219057,#219058,#219059,#219060,#219061,#219062,#219063,#219064,
#219065,#219066),.UNSPECIFIED.,.F.,.F.,(4,3,3,3,3,3,3,3,3,3,3,4),(0.,0.0896986624636303,
0.182830915896643,0.281579891583428,0.383870416571602,0.490905478463475,
0.5,0.612068495674318,0.726057759562033,0.839966626268522,0.953108020681144,
1.),.UNSPECIFIED.);
#5803=B_SPLINE_CURVE_WITH_KNOTS('',3,(#219448,#219449,#219450,#219451,#219452,
#219453,#219454,#219455,#219456,#219457,#219458,#219459,#219460,#219461),
 .UNSPECIFIED.,.F.,.F.,(4,2,2,1,1,2,2,4),(0.,0.249999999999997,0.374999999999996,
0.437499999999996,0.468749999999995,0.484374999999995,0.499999999999994,
1.),.UNSPECIFIED.);
#5804=B_SPLINE_CURVE_WITH_KNOTS('',3,(#219463,#219464,#219465,#219466,#219467,
#219468,#219469,#219470,#219471,#219472,#219473,#219474,#219475,#219476,
#219477,#219478),.UNSPECIFIED.,.F.,.F.,(4,2,2,1,1,1,1,2,2,4),(0.,0.24999999999999,
0.374999999999987,0.437499999999985,0.468749999999984,0.484374999999982,
0.492187499999983,0.496093749999983,0.499999999999983,1.),.UNSPECIFIED.);
#5805=B_SPLINE_CURVE_WITH_KNOTS('',3,(#219480,#219481,#219482,#219483,#219484,
#219485),.UNSPECIFIED.,.F.,.F.,(4,2,4),(0.,0.5,0.999993881110035),
 .UNSPECIFIED.);
#5806=B_SPLINE_CURVE_WITH_KNOTS('',3,(#219486,#219487,#219488,#219489,#219490,
#219491,#219492,#219493,#219494,#219495,#219496,#219497,#219498,#219499,
#219500,#219501,#219502,#219503,#219504,#219505,#219506,#219507,#219508,
#219509,#219510,#219511,#219512,#219513,#219514,#219515,#219516,#219517,
#219518,#219519,#219520,#219521,#219522,#219523,#219524,#219525,#219526,
#219527,#219528,#219529,#219530,#219531,#219532,#219533,#219534,#219535,
#219536,#219537,#219538,#219539,#219540,#219541,#219542,#219543,#219544,
#219545,#219546,#219547,#219548,#219549,#219550,#219551,#219552,#219553,
#219554,#219555,#219556,#219557,#219558,#219559,#219560,#219561,#219562,
#219563,#219564,#219565,#219566,#219567,#219568,#219569,#219570,#219571,
#219572,#219573,#219574,#219575,#219576,#219577,#219578,#219579,#219580,
#219581,#219582,#219583,#219584,#219585,#219586,#219587,#219588,#219589,
#219590,#219591,#219592,#219593,#219594,#219595,#219596,#219597,#219598,
#219599,#219600,#219601,#219602,#219603,#219604,#219605,#219606,#219607,
#219608,#219609,#219610,#219611,#219612,#219613,#219614,#219615,#219616,
#219617,#219618,#219619,#219620,#219621,#219622,#219623,#219624,#219625,
#219626,#219627,#219628,#219629,#219630,#219631,#219632,#219633,#219634,
#219635,#219636,#219637,#219638,#219639,#219640,#219641,#219642,#219643,
#219644,#219645,#219646,#219647,#219648,#219649,#219650,#219651,#219652,
#219653,#219654,#219655,#219656,#219657,#219658,#219659,#219660,#219661,
#219662,#219663,#219664,#219665,#219666,#219667,#219668,#219669,#219670,
#219671,#219672,#219673,#219674,#219675,#219676,#219677,#219678,#219679,
#219680,#219681,#219682,#219683,#219684,#219685,#219686,#219687,#219688,
#219689,#219690,#219691,#219692,#219693,#219694,#219695,#219696,#219697,
#219698,#219699,#219700,#219701,#219702,#219703,#219704,#219705,#219706,
#219707,#219708,#219709,#219710,#219711,#219712,#219713,#219714,#219715,
#219716,#219717,#219718,#219719,#219720,#219721,#219722,#219723,#219724,
#219725,#219726,#219727,#219728,#219729,#219730,#219731,#219732,#219733,
#219734,#219735,#219736,#219737,#219738,#219739,#219740,#219741,#219742,
#219743,#219744,#219745,#219746,#219747,#219748,#219749,#219750,#219751,
#219752,#219753,#219754,#219755,#219756,#219757,#219758,#219759,#219760,
#219761,#219762,#219763,#219764,#219765,#219766,#219767,#219768,#219769,
#219770,#219771,#219772,#219773,#219774,#219775,#219776,#219777,#219778,
#219779,#219780,#219781,#219782,#219783,#219784,#219785,#219786,#219787,
#219788,#219789,#219790,#219791,#219792,#219793,#219794,#219795,#219796,
#219797,#219798,#219799,#219800,#219801,#219802,#219803,#219804,#219805,
#219806,#219807,#219808,#219809,#219810,#219811,#219812,#219813,#219814,
#219815,#219816,#219817,#219818,#219819,#219820,#219821,#219822,#219823,
#219824,#219825),.UNSPECIFIED.,.F.,.F.,(4,3,3,3,3,3,3,3,3,3,3,3,3,3,3,3,
3,3,3,3,3,3,3,3,3,3,3,3,3,3,3,3,3,3,3,3,3,3,3,3,3,3,3,3,3,3,3,3,3,3,3,3,
3,3,3,3,3,3,3,3,3,3,3,3,3,3,3,3,3,3,3,3,3,3,3,3,3,3,3,3,3,3,3,3,3,3,3,3,
3,3,3,3,3,3,3,3,3,3,3,3,3,3,3,3,3,3,3,3,3,3,3,3,3,4),(-0.0339772660920509,
-0.0325203430581518,-0.032386048693209,-0.0318780990992314,-0.0306598615635381,
-0.0302573909015708,-0.0297789321064117,-0.0276581536141349,-0.0259928474480018,
-0.0255805981207726,-0.0249267022358351,-0.0245310146243628,-0.0243936296904867,
-0.024326995626826,-0.0242603615617803,-0.024127093428565,-0.023860557156862,
-0.0234814311279529,-0.0217282650368408,-0.0213822641351333,-0.0190428209661952,
-0.0174636751340817,-0.0171839301494941,-0.0166591384012892,-0.016397507911909,
-0.0162642461309164,-0.0161976136106437,-0.0161343466530843,-0.0161309799318905,
-0.0158644424540839,-0.0153313628316309,-0.0150847631566745,-0.013198990770689,
-0.0129855961638549,-0.0106966589063659,-0.00893402822640652,-0.00878726217821559,
-0.0071484990754369,-0.00680141898440107,-0.00668809518539594,-0.00573515795867427,
-0.00563851168898612,-0.00520205258212156,-0.00511371994078121,-0.00506876286241163,
-0.00500210501706407,-0.00496877348718764,-0.00493544103430002,-0.00466882155644317,
-0.0045889281925763,-0.00312096876785597,-0.00254453035286046,-0.00248976119975661,
-0.00148840346537639,-0.000436339145097795,-0.000390594206936927,0.00046358534986054,
0.000613822975248156,0.00141916260425755,0.00166725247387988,0.00170857278588276,
0.00317162738240526,0.00379103467916695,0.00380773977870245,0.00463539969377852,
0.00485732327511229,0.00485907394948943,0.00492583309157905,0.00495921266595899,
0.00499259224328974,0.00512611059303194,0.00539314760000376,0.00590690677152213,
0.00592722382056531,0.00800607376434179,0.00806356257284219,0.0111178351121071,
0.0122044077499811,0.0123363966390162,0.0143035747428008,0.0144728977439664,
0.0153531582392106,0.0155411644433074,0.0158779499874155,0.0160752947519555,
0.0161086774948306,0.016142060232708,0.0161754429719895,0.0162088257190771,
0.0163423569135267,0.0164027417356204,0.0166094212137446,0.0187054832686268,
0.0206010757212598,0.0208827465629589,0.0227002427140795,0.0230196099239667,
0.0235538292510131,0.0237498262104893,0.0238209047714043,0.0239544298768528,
0.0240211910330551,0.0240879522750274,0.0242746179586943,0.0247994097068993,
0.0251563789301884,0.0273038426614853,0.0289977436925387,0.0294352127171892,
0.0310969106853584,0.0315785446359996,0.0322002513430661,0.0327863759675397,
0.033196077678178),.UNSPECIFIED.);
#5807=B_SPLINE_CURVE_WITH_KNOTS('',3,(#219827,#219828,#219829,#219830,#219831,
#219832,#219833,#219834,#219835,#219836,#219837,#219838,#219839,#219840),
 .UNSPECIFIED.,.F.,.F.,(4,2,2,2,2,2,4),(0.,0.177361653110089,0.396250772308705,
0.834029010705937,0.943473570305246,0.9981958501049,1.),.UNSPECIFIED.);
#5808=B_SPLINE_CURVE_WITH_KNOTS('',3,(#219842,#219843,#219844,#219845,#219846,
#219847,#219848,#219849,#219850,#219851,#219852,#219853,#219854,#219855,
#219856,#219857,#219858,#219859,#219860,#219861,#219862,#219863,#219864,
#219865,#219866),.UNSPECIFIED.,.F.,.F.,(4,2,1,1,2,1,2,2,2,2,2,2,2,4),(0.,
0.00781250000000103,0.0156250000000021,0.0312500000000029,0.0625000000000033,
0.125000000000004,0.250000000000004,0.500000000000004,0.750000000000003,
0.875000000000004,0.968750000000004,0.984375000000003,0.992187500000002,
1.),.UNSPECIFIED.);
#5809=B_SPLINE_CURVE_WITH_KNOTS('',3,(#219868,#219869,#219870,#219871,#219872,
#219873,#219874,#219875,#219876,#219877,#219878,#219879,#219880,#219881,
#219882,#219883,#219884,#219885,#219886,#219887,#219888,#219889,#219890,
#219891,#219892,#219893,#219894,#219895,#219896,#219897,#219898,#219899,
#219900,#219901,#219902,#219903,#219904,#219905,#219906,#219907,#219908,
#219909,#219910,#219911,#219912,#219913,#219914,#219915,#219916,#219917,
#219918,#219919,#219920,#219921,#219922,#219923,#219924,#219925,#219926,
#219927,#219928,#219929,#219930,#219931),.UNSPECIFIED.,.F.,.F.,(4,3,3,3,
3,3,3,3,3,3,3,3,3,3,3,3,3,3,3,3,3,4),(0.,0.00477412889230797,0.00781250000000079,
0.0106654879371521,0.0156250000000016,0.0312500000000015,0.0342309236257492,
0.0625000000000014,0.0813617964285784,0.26988528574785,0.646932264386396,
0.835455753705669,0.929717498365307,0.96875,0.976848370695126,0.984375,
0.988631089346493,0.9921875,0.994522449578665,0.99609375,0.997468127244565,
1.),.UNSPECIFIED.);
#5810=B_SPLINE_CURVE_WITH_KNOTS('',3,(#219933,#219934,#219935,#219936,#219937,
#219938,#219939,#219940,#219941,#219942,#219943,#219944,#219945,#219946,
#219947,#219948,#219949,#219950,#219951,#219952,#219953,#219954,#219955,
#219956,#219957,#219958,#219959,#219960,#219961,#219962,#219963,#219964,
#219965,#219966),.UNSPECIFIED.,.F.,.F.,(4,3,3,3,3,3,3,3,3,3,3,4),(0.,0.000940021348058807,
0.0156250000000013,0.0312500000000026,0.0544722738485389,0.0625000000000029,
0.125000000000003,0.48273015832635,0.69685910820713,0.750000000000001,0.910988091716797,
1.),.UNSPECIFIED.);
#5811=B_SPLINE_CURVE_WITH_KNOTS('',3,(#219968,#219969,#219970,#219971,#219972,
#219973,#219974,#219975,#219976,#219977,#219978,#219979,#219980,#219981,
#219982,#219983,#219984,#219985,#219986,#219987,#219988,#219989,#219990,
#219991,#219992,#219993,#219994,#219995,#219996,#219997,#219998,#219999,
#220000,#220001,#220002,#220003,#220004,#220005,#220006,#220007),
 .UNSPECIFIED.,.F.,.F.,(4,3,3,3,3,3,3,3,3,3,3,3,3,4),(0.,0.000267216601111374,
0.0131577248626226,0.120048731344561,0.225313165495544,0.329701106959535,
0.433524683977464,0.5,0.648342485904365,0.664128121681686,0.771050593343276,
0.877973065004865,0.967295544654949,0.999999999999711),.UNSPECIFIED.);
#5812=B_SPLINE_CURVE_WITH_KNOTS('',3,(#220008,#220009,#220010,#220011,#220012,
#220013,#220014,#220015,#220016,#220017,#220018,#220019,#220020,#220021,
#220022,#220023,#220024,#220025,#220026,#220027,#220028,#220029,#220030,
#220031,#220032,#220033,#220034,#220035,#220036,#220037,#220038,#220039,
#220040,#220041,#220042,#220043,#220044,#220045,#220046,#220047,#220048,
#220049,#220050,#220051,#220052,#220053,#220054,#220055,#220056,#220057,
#220058,#220059,#220060,#220061,#220062,#220063,#220064,#220065,#220066,
#220067,#220068,#220069,#220070,#220071,#220072,#220073,#220074,#220075,
#220076,#220077,#220078,#220079,#220080,#220081,#220082,#220083,#220084,
#220085,#220086,#220087,#220088,#220089,#220090,#220091,#220092,#220093,
#220094,#220095,#220096,#220097,#220098,#220099,#220100,#220101),
 .UNSPECIFIED.,.F.,.F.,(4,3,3,3,3,3,3,3,3,3,3,3,3,3,3,3,3,3,3,3,3,3,3,3,
3,3,3,3,3,3,3,4),(0.,2.26241632322562E-6,0.00248004559774673,0.0035223755445969,
0.00701329037683304,0.0422709661520407,0.0597479664257431,0.0938229732817104,
0.12793820187041,0.155552859161154,0.190169805986124,0.22547721974652,0.25,
0.330973628752631,0.342469754057526,0.375,0.4375,0.46875,0.484375,0.4921875,
0.5,0.591257092400212,0.683349188310747,0.719815403392367,0.815155205598429,
0.910495007804491,0.9582618981018,0.962510291841565,0.982178193347656,0.994141900010685,
0.997133062479398,0.999999999936109),.UNSPECIFIED.);
#5813=B_SPLINE_CURVE_WITH_KNOTS('',3,(#220184,#220185,#220186,#220187,#220188,
#220189,#220190,#220191,#220192,#220193,#220194,#220195,#220196),
 .UNSPECIFIED.,.F.,.F.,(4,3,3,3,4),(0.,0.000262347006043535,0.00052508232379868,
0.000788127838510806,0.00105144790336124),.UNSPECIFIED.);
#5814=B_SPLINE_CURVE_WITH_KNOTS('',3,(#220197,#220198,#220199,#220200,#220201,
#220202,#220203,#220204,#220205,#220206,#220207,#220208,#220209,#220210,
#220211,#220212,#220213,#220214,#220215,#220216,#220217,#220218,#220219,
#220220,#220221,#220222,#220223,#220224,#220225,#220226,#220227,#220228,
#220229,#220230,#220231,#220232,#220233,#220234,#220235,#220236,#220237,
#220238,#220239,#220240,#220241,#220242,#220243,#220244,#220245,#220246,
#220247,#220248,#220249,#220250,#220251,#220252,#220253,#220254,#220255,
#220256,#220257,#220258,#220259,#220260,#220261,#220262,#220263,#220264,
#220265,#220266,#220267,#220268,#220269,#220270,#220271,#220272,#220273,
#220274,#220275,#220276,#220277,#220278,#220279,#220280,#220281,#220282,
#220283,#220284,#220285,#220286,#220287,#220288,#220289,#220290,#220291,
#220292,#220293,#220294,#220295,#220296,#220297,#220298,#220299,#220300,
#220301,#220302,#220303,#220304,#220305,#220306,#220307,#220308,#220309,
#220310,#220311,#220312,#220313,#220314,#220315,#220316,#220317),
 .UNSPECIFIED.,.F.,.F.,(4,3,3,3,3,3,3,3,3,3,3,3,3,3,3,3,3,3,3,3,3,3,3,3,
3,3,3,3,3,3,3,3,3,3,3,3,3,3,3,3,4),(0.,0.0481141113853886,0.0922200232969331,
0.124999999999905,0.164962385534248,0.187499999999854,0.218749999999828,
0.234374999999811,0.236646032545267,0.249999999999793,0.318804263020611,
0.374999999999725,0.437499999999693,0.466954438082284,0.46874999999968,
0.484374999999679,0.498424907910557,0.499999999999678,0.562499999999683,
0.620664099512309,0.624999999999687,0.687499999999698,0.718749999999709,
0.721406653442237,0.734374999999714,0.742187499999717,0.746337890624721,
0.748348236083708,0.749380988230567,0.749974461597412,0.750497174889094,
0.790225960908271,0.832612980454062,0.853806490226957,0.859104867670181,
0.860293591729929,0.874999999999853,0.902852200787948,0.935747746931192,
0.975590086367635,1.),.UNSPECIFIED.);
#5815=B_SPLINE_CURVE_WITH_KNOTS('',3,(#220399,#220400,#220401,#220402,#220403,
#220404,#220405,#220406,#220407,#220408,#220409,#220410,#220411,#220412,
#220413,#220414,#220415,#220416,#220417,#220418,#220419,#220420,#220421,
#220422,#220423,#220424,#220425,#220426,#220427,#220428,#220429,#220430,
#220431,#220432,#220433,#220434,#220435,#220436,#220437,#220438,#220439,
#220440,#220441,#220442,#220443,#220444,#220445,#220446,#220447,#220448,
#220449,#220450,#220451,#220452,#220453,#220454,#220455,#220456,#220457,
#220458,#220459,#220460,#220461,#220462,#220463,#220464,#220465,#220466,
#220467,#220468,#220469,#220470,#220471,#220472,#220473,#220474,#220475,
#220476,#220477,#220478,#220479,#220480,#220481,#220482,#220483,#220484,
#220485,#220486,#220487,#220488,#220489,#220490,#220491,#220492,#220493,
#220494,#220495,#220496,#220497,#220498,#220499,#220500,#220501,#220502,
#220503,#220504,#220505,#220506,#220507,#220508,#220509,#220510,#220511,
#220512,#220513),.UNSPECIFIED.,.F.,.F.,(4,3,3,3,3,3,3,3,3,3,3,3,3,3,3,3,
3,3,3,3,3,3,3,3,3,3,3,3,3,3,3,3,3,3,3,3,3,3,4),(0.,0.125000000000075,0.129138910233674,
0.187500000000111,0.218750000000129,0.234375000000138,0.245584641133974,
0.248410569305501,0.250000000000148,0.336537419726474,0.371504451325829,
0.375000000000245,0.437500000000291,0.468750000000316,0.484375000000329,
0.492187500000333,0.496093750000332,0.498211359913546,0.500000000000331,
0.55551957851444,0.603575446450059,0.615889256785246,0.625000000000302,
0.687500000000288,0.718750000000278,0.734375000000271,0.742187500000269,
0.746093750000268,0.748046875000267,0.748826280767137,0.750000000000266,
0.794921440761665,0.80172102164972,0.840711183572136,0.859490017116372,
0.890874071151793,0.924376073377366,0.980784458226199,1.),.UNSPECIFIED.);
#5816=B_SPLINE_CURVE_WITH_KNOTS('',3,(#220514,#220515,#220516,#220517,#220518,
#220519,#220520,#220521,#220522,#220523,#220524,#220525,#220526,#220527,
#220528,#220529,#220530,#220531,#220532,#220533,#220534,#220535,#220536,
#220537,#220538,#220539,#220540,#220541,#220542,#220543,#220544,#220545,
#220546,#220547,#220548,#220549,#220550,#220551,#220552,#220553,#220554,
#220555,#220556,#220557,#220558,#220559,#220560,#220561,#220562,#220563,
#220564,#220565,#220566,#220567,#220568,#220569,#220570,#220571,#220572,
#220573,#220574,#220575,#220576,#220577,#220578,#220579,#220580,#220581,
#220582,#220583,#220584,#220585,#220586,#220587,#220588,#220589,#220590,
#220591,#220592,#220593),.UNSPECIFIED.,.F.,.F.,(4,2,2,2,1,2,2,2,2,2,2,2,
1,1,2,2,1,1,1,2,2,2,2,1,2,2,2,2,1,1,2,2,2,2,2,1,1,2,2,2,2,2,1,2,2,4),(0.,
0.062500000000062,0.0937500000000954,0.10937500000011,0.117187500000119,
0.123046875000124,0.125000000000124,0.156250000000161,0.171875000000177,
0.187500000000193,0.218750000000225,0.234375000000241,0.242187500000252,
0.246093750000255,0.248046875000261,0.250000000000266,0.312500000000522,
0.343750000000647,0.35937500000071,0.373046875000764,0.37500000000077,0.406250000000778,
0.421875000000782,0.429687500000782,0.433593750000785,0.437500000000788,
0.46875000000079,0.484375000000792,0.492187500000789,0.496093750000792,
0.498046875000789,0.500000000000786,0.625000000000577,0.640625000000551,
0.644531250000544,0.648437500000537,0.656250000000529,0.687500000000512,
0.750000000000475,0.781250000000457,0.785156250000452,0.789062500000447,
0.796875000000434,0.812500000000401,0.875000000000267,1.),.UNSPECIFIED.);
#5817=B_SPLINE_CURVE_WITH_KNOTS('',3,(#220610,#220611,#220612,#220613,#220614,
#220615,#220616,#220617,#220618,#220619),.UNSPECIFIED.,.F.,.F.,(4,3,3,4),
(0.,0.000342739116435002,0.000689887215256671,0.000728014676542687),
 .UNSPECIFIED.);
#5818=B_SPLINE_CURVE_WITH_KNOTS('',3,(#220633,#220634,#220635,#220636,#220637,
#220638,#220639,#220640,#220641,#220642),.UNSPECIFIED.,.F.,.F.,(4,3,3,4),
(0.,0.331792271676137,0.665896135838068,1.),.UNSPECIFIED.);
#5819=B_SPLINE_CURVE_WITH_KNOTS('',3,(#220837,#220838,#220839,#220840,#220841,
#220842,#220843,#220844,#220845,#220846,#220847,#220848,#220849,#220850,
#220851,#220852,#220853,#220854,#220855,#220856,#220857,#220858,#220859,
#220860,#220861,#220862,#220863,#220864,#220865,#220866,#220867,#220868,
#220869,#220870),.UNSPECIFIED.,.F.,.F.,(4,1,1,2,2,2,1,1,2,2,2,2,2,2,2,1,
1,2,2,4),(0.,0.00781250000002213,0.0117187500000346,0.0146484375000462,
0.0156250000000499,0.0234375000000586,0.027343750000063,0.029296875000065,
0.030273437500066,0.0312500000000671,0.0625000000000648,0.12500000000006,
0.187500000000056,0.250000000000051,0.375000000000042,0.437500000000038,
0.468750000000035,0.484375000000034,0.500000000000032,0.999999868413402),
 .UNSPECIFIED.);
#5820=B_SPLINE_CURVE_WITH_KNOTS('',3,(#220871,#220872,#220873,#220874,#220875,
#220876,#220877,#220878,#220879,#220880),.UNSPECIFIED.,.F.,.F.,(4,2,2,2,
4),(4.18095462764722E-18,0.00255445063423646,0.00383167595135469,0.00447028860991381,
0.00510890126847292),.UNSPECIFIED.);
#5821=B_SPLINE_CURVE_WITH_KNOTS('',3,(#220882,#220883,#220884,#220885,#220886,
#220887,#220888,#220889,#220890,#220891,#220892,#220893,#220894,#220895,
#220896,#220897,#220898,#220899,#220900,#220901,#220902,#220903,#220904,
#220905,#220906,#220907,#220908,#220909,#220910,#220911,#220912,#220913,
#220914,#220915,#220916,#220917,#220918,#220919,#220920,#220921,#220922,
#220923,#220924,#220925,#220926,#220927,#220928,#220929,#220930,#220931,
#220932,#220933,#220934,#220935,#220936,#220937,#220938,#220939,#220940,
#220941,#220942,#220943,#220944,#220945,#220946,#220947,#220948,#220949,
#220950,#220951,#220952,#220953,#220954,#220955,#220956,#220957,#220958,
#220959,#220960,#220961,#220962,#220963,#220964,#220965,#220966,#220967,
#220968,#220969,#220970,#220971,#220972,#220973,#220974,#220975,#220976,
#220977,#220978,#220979,#220980,#220981,#220982,#220983,#220984,#220985,
#220986,#220987,#220988,#220989,#220990,#220991,#220992,#220993,#220994,
#220995,#220996,#220997,#220998,#220999,#221000,#221001,#221002,#221003,
#221004,#221005,#221006,#221007,#221008,#221009,#221010,#221011,#221012,
#221013,#221014,#221015,#221016,#221017,#221018,#221019,#221020,#221021,
#221022,#221023,#221024,#221025,#221026,#221027,#221028,#221029,#221030,
#221031,#221032,#221033,#221034,#221035,#221036,#221037,#221038,#221039,
#221040,#221041,#221042,#221043,#221044,#221045,#221046,#221047),
 .UNSPECIFIED.,.F.,.F.,(4,3,3,3,3,3,3,3,3,3,3,3,3,3,3,3,3,3,3,3,3,3,3,3,
3,3,3,3,3,3,3,3,3,3,3,3,3,3,3,3,3,3,3,3,3,3,3,3,3,3,3,3,3,3,3,4),(3.84474371945078E-15,
0.00129418777048261,0.00218682165402767,0.00327794728486691,0.00398945644969312,
0.00437364330805532,0.0050976652962974,0.00620616680151919,0.00795383201123593,
0.00842283797271545,0.00874728661611061,0.0106381507815742,0.0109341082701383,
0.0111918496720621,0.0113302678430169,0.0113648723663165,0.0113994769397404,
0.0114686863527641,0.0114808136836452,0.0117455395577679,0.0120275190971521,
0.0128530198691882,0.0131209299241659,0.0165925164204044,0.0172816770907965,
0.0174945732322213,0.019495073308936,0.019681394886249,0.0200483162030429,
0.0202281002997558,0.0203249209658382,0.0204632190439302,0.0205323676346298,
0.0206015162605072,0.0207748057132628,0.0217079731878734,0.0218682165402766,
0.0241483517759356,0.0261345203104882,0.0262418598483319,0.0275481788415872,
0.0283480821017152,0.0284286815023595,0.0293305775946609,0.0294547291211152,
0.0295220923293734,0.0300079248057894,0.0300687977428803,0.0302844849745231,
0.0303536218586976,0.0303881901705619,0.0304227584828701,0.0305610330454487,
0.0306155031563872,0.0335427501364484,0.0349891464644424),.UNSPECIFIED.);
#5822=B_SPLINE_CURVE_WITH_KNOTS('',3,(#221049,#221050,#221051,#221052,#221053,
#221054,#221055,#221056,#221057,#221058,#221059,#221060,#221061,#221062,
#221063,#221064,#221065,#221066,#221067,#221068,#221069,#221070,#221071,
#221072,#221073,#221074,#221075,#221076,#221077,#221078,#221079,#221080,
#221081,#221082,#221083,#221084,#221085,#221086,#221087,#221088,#221089,
#221090,#221091,#221092,#221093,#221094,#221095,#221096,#221097,#221098,
#221099,#221100,#221101,#221102,#221103,#221104,#221105,#221106,#221107,
#221108,#221109,#221110,#221111,#221112),.UNSPECIFIED.,.F.,.F.,(4,3,3,3,
3,3,3,3,3,3,3,3,3,3,3,3,3,3,3,3,3,4),(3.94435119578486E-14,0.0661070715252713,
0.131240897937816,0.140624999999884,0.187499999999846,0.249999999999794,
0.308921024725339,0.365490856280017,0.374999999999676,0.428753346904277,
0.437499999999626,0.46874999999959,0.484374999999562,0.492187499999558,
0.4984488684236,0.499662271028205,0.499999999999553,0.664758583825297,0.749999999999777,
0.838636570956166,0.926879967465366,0.999999999865913),.UNSPECIFIED.);
#5823=B_SPLINE_CURVE_WITH_KNOTS('',3,(#221114,#221115,#221116,#221117,#221118,
#221119,#221120,#221121,#221122,#221123,#221124,#221125,#221126,#221127,
#221128,#221129,#221130,#221131,#221132,#221133,#221134,#221135,#221136,
#221137,#221138,#221139,#221140,#221141,#221142,#221143,#221144,#221145,
#221146,#221147,#221148,#221149,#221150,#221151,#221152,#221153,#221154,
#221155,#221156),.UNSPECIFIED.,.F.,.F.,(4,1,1,2,2,2,1,1,2,2,2,2,2,2,1,1,
1,2,2,2,1,1,1,1,2,2,4),(0.,0.00390624999994919,0.00585937499992379,0.00732421874990716,
0.00781249999990194,0.0117187499999027,0.013671874999902,0.0146484374999016,
0.0151367187499008,0.0156249999998999,0.0312499999998973,0.0624999999998953,
0.0937499999998933,0.124999999999891,0.187499999999888,0.218749999999886,
0.234374999999886,0.242187499999887,0.249999999999888,0.374999999999892,
0.437499999999895,0.468749999999897,0.484374999999897,0.492187499999897,
0.496093749999898,0.499999999999899,1.),.UNSPECIFIED.);
#5824=B_SPLINE_CURVE_WITH_KNOTS('',3,(#221157,#221158,#221159,#221160,#221161,
#221162,#221163,#221164,#221165,#221166,#221167,#221168,#221169,#221170,
#221171,#221172,#221173,#221174,#221175,#221176,#221177,#221178,#221179,
#221180,#221181,#221182,#221183,#221184,#221185,#221186,#221187,#221188,
#221189,#221190,#221191,#221192,#221193,#221194,#221195,#221196,#221197,
#221198,#221199,#221200,#221201,#221202,#221203,#221204,#221205,#221206,
#221207,#221208,#221209,#221210,#221211,#221212,#221213,#221214,#221215,
#221216,#221217,#221218,#221219,#221220,#221221,#221222,#221223,#221224,
#221225,#221226,#221227,#221228,#221229,#221230,#221231,#221232,#221233,
#221234,#221235,#221236,#221237,#221238,#221239,#221240,#221241,#221242,
#221243,#221244,#221245,#221246,#221247,#221248,#221249,#221250,#221251,
#221252,#221253,#221254,#221255,#221256,#221257,#221258,#221259,#221260,
#221261,#221262,#221263,#221264,#221265,#221266,#221267,#221268),
 .UNSPECIFIED.,.F.,.F.,(4,3,3,3,3,3,3,3,3,3,3,3,3,3,3,3,3,3,3,3,3,3,3,3,
3,3,3,3,3,3,3,3,3,3,3,3,3,4),(0.,0.00282254399121512,0.00586614516938873,
0.00651606421840167,0.0228133545141081,0.0388819768075745,0.054179413201791,
0.0625000000000008,0.0703124999999999,0.0762984211550201,0.078124999999999,
0.0937499999999989,0.113221577872514,0.124999999999998,0.187499999999997,
0.221409998208068,0.238251470487989,0.249614071096417,0.253335824028494,
0.356141776447435,0.396642919128224,0.448321459564108,0.47416072978205,
0.480620547336536,0.483496454516943,0.485164620119042,0.496996851944816,
0.499999999999993,0.641721524748589,0.788214551204109,0.838614676791042,
0.924794957777326,0.953285960601031,0.956447955489975,0.985643664365405,
0.992933726435535,0.996578250210837,0.999999904445776),.UNSPECIFIED.);
#5825=B_SPLINE_CURVE_WITH_KNOTS('',3,(#221288,#221289,#221290,#221291,#221292,
#221293,#221294,#221295,#221296,#221297,#221298,#221299,#221300,#221301,
#221302,#221303,#221304,#221305,#221306,#221307,#221308,#221309,#221310,
#221311,#221312,#221313,#221314,#221315),.UNSPECIFIED.,.F.,.F.,(4,3,3,3,
3,3,3,3,3,4),(0.,0.117448719031058,0.23465352743689,0.35179443705116,0.469085047802828,
0.5,0.625,0.748726478170368,0.874363239085184,1.),.UNSPECIFIED.);
#5826=B_SPLINE_CURVE_WITH_KNOTS('',3,(#221331,#221332,#221333,#221334,#221335,
#221336,#221337,#221338,#221339,#221340),.UNSPECIFIED.,.F.,.F.,(4,3,3,4),
(0.,0.406538901690834,0.808488591965978,0.999999999958054),
 .UNSPECIFIED.);
#5827=B_SPLINE_CURVE_WITH_KNOTS('',3,(#221359,#221360,#221361,#221362,#221363,
#221364,#221365),.UNSPECIFIED.,.F.,.F.,(4,3,4),(0.,5.20100074843796E-5,
8.9937829810603E-5),.UNSPECIFIED.);
#5828=B_SPLINE_CURVE_WITH_KNOTS('',3,(#221399,#221400,#221401,#221402,#221403,
#221404,#221405,#221406,#221407,#221408,#221409,#221410,#221411,#221412,
#221413,#221414,#221415,#221416,#221417,#221418,#221419,#221420,#221421,
#221422,#221423,#221424,#221425),.UNSPECIFIED.,.F.,.F.,(4,2,2,1,1,2,2,2,
2,2,2,1,2,2,4),(0.,0.125000000000187,0.187500000000272,0.218750000000309,
0.234375000000323,0.242187500000315,0.250000000000307,0.375000000000268,
0.437500000000258,0.500000000000248,0.62500000000022,0.687500000000207,
0.718750000000191,0.750000000000176,1.),.UNSPECIFIED.);
#5829=B_SPLINE_CURVE_WITH_KNOTS('',3,(#221426,#221427,#221428,#221429,#221430,
#221431,#221432,#221433,#221434,#221435,#221436,#221437,#221438),
 .UNSPECIFIED.,.F.,.F.,(4,3,3,3,4),(1.38777878078145E-17,0.000218644279510345,
0.000437193341879142,0.000655638180349197,0.000873969830693171),
 .UNSPECIFIED.);
#5830=B_SPLINE_CURVE_WITH_KNOTS('',3,(#221502,#221503,#221504,#221505,#221506,
#221507,#221508,#221509,#221510,#221511,#221512,#221513,#221514,#221515,
#221516,#221517,#221518,#221519,#221520,#221521,#221522,#221523,#221524,
#221525,#221526,#221527,#221528,#221529,#221530,#221531,#221532,#221533,
#221534,#221535,#221536,#221537,#221538,#221539,#221540,#221541,#221542,
#221543,#221544,#221545,#221546,#221547,#221548,#221549,#221550,#221551,
#221552,#221553,#221554,#221555,#221556,#221557,#221558,#221559,#221560,
#221561,#221562,#221563,#221564,#221565,#221566,#221567,#221568,#221569,
#221570,#221571,#221572,#221573,#221574,#221575,#221576,#221577,#221578,
#221579,#221580,#221581,#221582,#221583,#221584,#221585,#221586,#221587,
#221588,#221589,#221590,#221591,#221592,#221593,#221594,#221595,#221596,
#221597,#221598,#221599,#221600,#221601,#221602,#221603,#221604,#221605,
#221606,#221607,#221608,#221609,#221610,#221611,#221612,#221613,#221614,
#221615,#221616,#221617,#221618,#221619,#221620,#221621,#221622,#221623,
#221624,#221625,#221626,#221627,#221628,#221629,#221630,#221631,#221632,
#221633,#221634,#221635,#221636,#221637,#221638,#221639,#221640,#221641,
#221642,#221643,#221644,#221645,#221646,#221647,#221648,#221649,#221650,
#221651,#221652,#221653,#221654,#221655,#221656,#221657,#221658,#221659,
#221660,#221661,#221662,#221663,#221664,#221665,#221666,#221667,#221668,
#221669,#221670,#221671,#221672,#221673,#221674,#221675,#221676,#221677,
#221678,#221679,#221680,#221681,#221682,#221683,#221684,#221685,#221686,
#221687,#221688,#221689,#221690,#221691,#221692,#221693,#221694,#221695,
#221696,#221697,#221698,#221699,#221700,#221701,#221702,#221703,#221704,
#221705,#221706,#221707,#221708,#221709,#221710,#221711,#221712,#221713,
#221714,#221715,#221716,#221717,#221718,#221719,#221720,#221721,#221722,
#221723,#221724,#221725,#221726,#221727,#221728,#221729,#221730,#221731,
#221732,#221733,#221734,#221735,#221736,#221737,#221738,#221739,#221740,
#221741,#221742,#221743,#221744,#221745,#221746,#221747,#221748),
 .UNSPECIFIED.,.F.,.F.,(4,3,3,3,3,3,3,3,3,3,3,3,3,3,3,3,3,3,3,3,3,3,3,3,
3,3,3,3,3,3,3,3,3,3,3,3,3,3,3,3,3,3,3,3,3,3,3,3,3,3,3,3,3,3,3,3,3,3,3,3,
3,3,3,3,3,3,3,3,3,3,3,3,3,3,3,3,3,3,3,3,3,3,4),(0.,0.0312499999999464,0.0468749999999195,
0.0546874999999061,0.0585937499999004,0.0624999999998947,0.0816944959084324,
0.0937499999998461,0.109374999999822,0.117187499999809,0.1210937499998,
0.123046874999798,0.124999999999796,0.151338478147273,0.187499999999701,
0.218749999999654,0.234374999999631,0.246093749999614,0.24999999999961,
0.283734989216096,0.312499999999641,0.343749999999659,0.359374999999667,
0.359919964895214,0.367187499999673,0.371093749999678,0.374999999999682,
0.39459606244507,0.416671189759111,0.437499999999733,0.463193895153147,
0.468749999999759,0.484374999999766,0.49218749999977,0.496093749999766,
0.498046874999753,0.49999999999974,0.534110585575294,0.558950115148432,
0.562499999999334,0.593749999999131,0.609374999999031,0.617187499998981,
0.621093749998958,0.623046874998947,0.624999999998935,0.64207191973391,
0.656249999998824,0.671874999998769,0.679687499998743,0.68496404906836,
0.687499999998717,0.711490137633078,0.718749999998614,0.734374999998562,
0.742187499998539,0.74609374999853,0.746669664934028,0.749686729299358,
0.749999999998521,0.769789557229922,0.790340500844122,0.812121449595702,
0.834784976813535,0.860334536496689,0.874999999998234,0.888476593882743,
0.90624999999816,0.921874999998121,0.929687499998103,0.935546874998086,
0.937252953214231,0.937499999998081,0.945466322826954,0.953124999998562,
0.960937499998805,0.964843749998927,0.966796874998987,0.968405695614136,
0.968749999999048,0.982751356553703,0.997765223026701,1.),.UNSPECIFIED.);
#5831=B_SPLINE_CURVE_WITH_KNOTS('',3,(#221749,#221750,#221751,#221752,#221753,
#221754,#221755,#221756,#221757,#221758,#221759,#221760,#221761,#221762,
#221763,#221764,#221765,#221766,#221767,#221768,#221769,#221770,#221771,
#221772,#221773,#221774,#221775,#221776,#221777,#221778,#221779,#221780,
#221781,#221782,#221783,#221784,#221785,#221786,#221787,#221788,#221789,
#221790,#221791,#221792,#221793,#221794,#221795,#221796,#221797,#221798,
#221799,#221800,#221801,#221802,#221803,#221804,#221805,#221806,#221807,
#221808,#221809,#221810,#221811,#221812),.UNSPECIFIED.,.F.,.F.,(4,3,3,3,
3,3,3,3,3,3,3,3,3,3,3,3,3,3,3,3,3,4),(0.,0.104472712536878,0.143833362593174,
0.221616793428957,0.249999999999996,0.272765207700177,0.364018417806752,
0.374999999999994,0.390898624571728,0.437499999999996,0.446744971466346,
0.468749999999998,0.484375,0.492187500000001,0.499298442314967,0.500000000000002,
0.500701252711277,0.623020578288952,0.746999029313984,0.855597812446925,
0.872653871556337,1.),.UNSPECIFIED.);
#5832=B_SPLINE_CURVE_WITH_KNOTS('',3,(#221828,#221829,#221830,#221831,#221832,
#221833,#221834,#221835,#221836,#221837,#221838,#221839,#221840),
 .UNSPECIFIED.,.F.,.F.,(4,3,3,3,4),(0.,0.378104296523149,0.5,0.866163286535829,
1.),.UNSPECIFIED.);
#5833=B_SPLINE_CURVE_WITH_KNOTS('',3,(#221854,#221855,#221856,#221857,#221858,
#221859,#221860,#221861,#221862,#221863,#221864,#221865,#221866),
 .UNSPECIFIED.,.F.,.F.,(4,3,3,3,4),(0.,0.230076523236993,0.47903074115821,
0.750119827238623,0.999997761900286),.UNSPECIFIED.);
#5834=B_SPLINE_CURVE_WITH_KNOTS('',3,(#221867,#221868,#221869,#221870,#221871,
#221872,#221873,#221874,#221875,#221876,#221877,#221878,#221879,#221880,
#221881,#221882,#221883,#221884,#221885),.UNSPECIFIED.,.F.,.F.,(4,3,3,3,
3,3,4),(0.,0.188673283403314,0.369161567333252,0.538899468433716,0.703430166255707,
0.860489953582614,1.),.UNSPECIFIED.);
#5835=B_SPLINE_CURVE_WITH_KNOTS('',3,(#221904,#221905,#221906,#221907,#221908,
#221909,#221910,#221911,#221912,#221913,#221914,#221915,#221916,#221917,
#221918,#221919,#221920,#221921,#221922,#221923,#221924,#221925,#221926,
#221927,#221928,#221929,#221930,#221931,#221932,#221933,#221934),
 .UNSPECIFIED.,.F.,.F.,(4,3,3,3,3,3,3,3,3,3,4),(0.,0.20570874903028,0.249999999999735,
0.442981918132296,0.497264694230287,0.499023437499477,0.499999999999478,
0.649996181070983,0.79237661029201,0.925792371617293,1.),.UNSPECIFIED.);
#5836=B_SPLINE_CURVE_WITH_KNOTS('',3,(#221935,#221936,#221937,#221938,#221939,
#221940,#221941),.UNSPECIFIED.,.F.,.F.,(4,3,4),(0.00166725821467356,0.014267238448545,
0.0264527075460118),.UNSPECIFIED.);
#5837=B_SPLINE_CURVE_WITH_KNOTS('',3,(#221954,#221955,#221956,#221957,#221958,
#221959,#221960,#221961,#221962,#221963,#221964,#221965,#221966,#221967,
#221968,#221969,#221970,#221971,#221972,#221973,#221974,#221975,#221976,
#221977,#221978,#221979,#221980,#221981,#221982,#221983,#221984,#221985,
#221986,#221987,#221988,#221989,#221990,#221991,#221992,#221993,#221994,
#221995,#221996,#221997,#221998,#221999,#222000,#222001,#222002,#222003,
#222004,#222005,#222006,#222007,#222008),.UNSPECIFIED.,.F.,.F.,(4,3,3,3,
3,3,3,3,3,3,3,3,3,3,3,3,3,3,4),(0.,0.214315851661325,0.249999999999893,
0.37499999999984,0.45312499999986,0.487304687499869,0.495315551757683,0.49728697538363,
0.498268836759834,0.498758808598935,0.499018361648366,0.499101930796815,
0.499591089067522,0.499835429356063,0.499982229064921,0.500040936858297,
0.750020468429149,0.975872543910639,1.),.UNSPECIFIED.);
#5838=B_SPLINE_CURVE_WITH_KNOTS('',3,(#222009,#222010,#222011,#222012,#222013,
#222014,#222015,#222016,#222017,#222018,#222019,#222020,#222021,#222022,
#222023,#222024,#222025,#222026,#222027,#222028,#222029,#222030,#222031,
#222032,#222033,#222034,#222035,#222036),.UNSPECIFIED.,.F.,.F.,(4,3,3,3,
3,3,3,3,3,4),(0.,0.24999999999984,0.37499999999976,0.437499999999719,0.468749999999699,
0.48437499999969,0.499023437499683,0.499999999999684,0.76071527755839,1.),
 .UNSPECIFIED.);
#5839=B_SPLINE_CURVE_WITH_KNOTS('',3,(#222049,#222050,#222051,#222052,#222053,
#222054,#222055,#222056,#222057,#222058,#222059,#222060,#222061,#222062,
#222063),.UNSPECIFIED.,.F.,.F.,(4,2,2,1,1,1,2,2,4),(0.,0.250000000000125,
0.375000000000188,0.437500000000219,0.468750000000234,0.484375000000242,
0.499023437500251,0.500000000000251,1.),.UNSPECIFIED.);
#5840=B_SPLINE_CURVE_WITH_KNOTS('',3,(#222064,#222065,#222066,#222067,#222068,
#222069,#222070,#222071,#222072,#222073,#222074,#222075,#222076,#222077,
#222078,#222079,#222080,#222081,#222082,#222083,#222084,#222085,#222086,
#222087,#222088,#222089,#222090,#222091,#222092,#222093,#222094,#222095,
#222096,#222097,#222098,#222099,#222100,#222101,#222102,#222103,#222104,
#222105,#222106,#222107,#222108,#222109,#222110,#222111,#222112,#222113,
#222114,#222115,#222116,#222117,#222118),.UNSPECIFIED.,.F.,.F.,(4,3,3,3,
3,3,3,3,3,3,3,3,3,3,3,3,3,3,4),(0.,0.234963913086287,0.250000000000182,
0.375000000000272,0.453125000000238,0.487304687500223,0.495315551758032,
0.497286975383978,0.498268836760181,0.498758808599282,0.499021790751283,
0.499105006360904,0.499594161628129,0.499838500416397,0.499987953667902,
0.50004752798089,0.724683195181892,0.965177174746084,1.),.UNSPECIFIED.);
#5841=B_SPLINE_CURVE_WITH_KNOTS('',3,(#222137,#222138,#222139,#222140,#222141,
#222142,#222143,#222144,#222145,#222146,#222147,#222148,#222149,#222150,
#222151,#222152,#222153,#222154,#222155,#222156,#222157,#222158,#222159,
#222160,#222161,#222162,#222163,#222164,#222165,#222166,#222167,#222168,
#222169,#222170,#222171),.UNSPECIFIED.,.F.,.F.,(4,2,2,1,1,1,2,2,2,1,1,1,
1,2,2,2,1,1,1,1,2,2,4),(0.,0.124999999999923,0.187499999999883,0.218749999999863,
0.234374999999853,0.242187499999848,0.248046874999843,0.24999999999984,
0.374999999999744,0.437499999999695,0.46874999999967,0.484374999999657,
0.492187499999651,0.498046874999649,0.49999999999965,0.624999999999703,
0.687499999999729,0.718749999999742,0.734374999999749,0.742187499999752,
0.748046874999756,0.749999999999758,1.),.UNSPECIFIED.);
#5842=B_SPLINE_CURVE_WITH_KNOTS('',3,(#222172,#222173,#222174,#222175,#222176,
#222177,#222178,#222179,#222180,#222181,#222182,#222183,#222184,#222185,
#222186,#222187),.UNSPECIFIED.,.F.,.F.,(4,2,2,1,1,1,1,2,2,4),(0.,0.249999999999839,
0.374999999999757,0.437499999999716,0.468749999999695,0.484374999999687,
0.492187499999682,0.499023437499678,0.499999999999678,1.),.UNSPECIFIED.);
#5843=B_SPLINE_CURVE_WITH_KNOTS('',3,(#223329,#223330,#223331,#223332,#223333,
#223334),.UNSPECIFIED.,.F.,.F.,(4,2,4),(4.10724833792282E-6,0.241237590782085,
0.483186237929456),.UNSPECIFIED.);
#5844=B_SPLINE_CURVE_WITH_KNOTS('',3,(#223348,#223349,#223350,#223351,#223352,
#223353),.UNSPECIFIED.,.F.,.F.,(4,2,4),(0.,0.0477670349008267,0.0955331274490537),
 .UNSPECIFIED.);
#5845=B_SPLINE_CURVE_WITH_KNOTS('',3,(#223356,#223357,#223358,#223359,#223360,
#223361),.UNSPECIFIED.,.F.,.F.,(4,2,4),(1.13358908630587E-6,0.0262346930665884,
0.0524681434362511),.UNSPECIFIED.);
#5846=B_SPLINE_CURVE_WITH_KNOTS('',3,(#223370,#223371,#223372,#223373,#223374,
#223375),.UNSPECIFIED.,.F.,.F.,(4,2,4),(9.82188160298338E-7,0.126873328128178,
0.25376575794151),.UNSPECIFIED.);
#5847=B_SPLINE_CURVE_WITH_KNOTS('',3,(#223389,#223390,#223391,#223392,#223393,
#223394),.UNSPECIFIED.,.F.,.F.,(4,2,4),(2.15646689644485E-6,0.125624403775893,
0.258424816795553),.UNSPECIFIED.);
#5848=B_SPLINE_CURVE_WITH_KNOTS('',3,(#223408,#223409,#223410,#223411,#223412,
#223413),.UNSPECIFIED.,.F.,.F.,(4,2,4),(2.32100271924243E-6,0.114258712352594,
0.228506360165928),.UNSPECIFIED.);
#5849=B_SPLINE_CURVE_WITH_KNOTS('',3,(#223421,#223422,#223423,#223424,#223425,
#223426),.UNSPECIFIED.,.F.,.F.,(4,2,4),(1.02478977306241E-6,0.113688459278625,
0.227380714685831),.UNSPECIFIED.);
#5850=B_SPLINE_CURVE_WITH_KNOTS('',3,(#224660,#224661,#224662,#224663,#224664,
#224665,#224666,#224667,#224668,#224669,#224670,#224671,#224672,#224673),
 .UNSPECIFIED.,.F.,.F.,(4,2,2,2,2,2,4),(2.93038070849918E-6,0.0527238910564628,
0.0983357876907069,0.104035629430328,0.107433622421913,0.173175220318963,
0.608688061649262),.UNSPECIFIED.);
#5851=B_SPLINE_CURVE_WITH_KNOTS('',3,(#224675,#224676,#224677,#224678,#224679,
#224680),.UNSPECIFIED.,.F.,.F.,(4,2,4),(-0.352164527632873,-0.175885968938167,
0.),.UNSPECIFIED.);
#5852=B_SPLINE_CURVE_WITH_KNOTS('',3,(#224682,#224683,#224684,#224685,#224686,
#224687,#224688,#224689,#224690,#224691,#224692,#224693,#224694,#224695),
 .UNSPECIFIED.,.F.,.F.,(4,2,2,2,2,2,4),(-0.146050691310393,-0.133401168786229,
-0.122457304257569,-0.121089707324725,-0.120274395422017,-0.104500136704916,
-1.85098674576232E-6),.UNSPECIFIED.);
#5853=B_SPLINE_CURVE_WITH_KNOTS('',3,(#224696,#224697,#224698,#224699,#224700,
#224701),.UNSPECIFIED.,.F.,.F.,(4,2,4),(1.20017331883328E-7,0.235767253078328,
0.473063078352785),.UNSPECIFIED.);
#5854=B_SPLINE_CURVE_WITH_KNOTS('',3,(#224703,#224704,#224705,#224706,#224707,
#224708,#224709,#224710,#224711,#224712,#224713,#224714,#224715,#224716,
#224717,#224718,#224719,#224720,#224721,#224722,#224723,#224724,#224725,
#224726,#224727,#224728,#224729,#224730,#224731,#224732,#224733,#224734,
#224735,#224736,#224737,#224738,#224739,#224740,#224741,#224742,#224743,
#224744,#224745,#224746,#224747,#224748,#224749,#224750,#224751,#224752,
#224753,#224754,#224755,#224756,#224757,#224758,#224759,#224760,#224761,
#224762,#224763,#224764,#224765,#224766,#224767,#224768,#224769,#224770,
#224771,#224772,#224773,#224774,#224775,#224776,#224777,#224778,#224779,
#224780,#224781,#224782,#224783,#224784,#224785,#224786,#224787,#224788,
#224789,#224790,#224791,#224792,#224793,#224794,#224795,#224796,#224797,
#224798,#224799,#224800,#224801,#224802,#224803,#224804,#224805,#224806,
#224807,#224808,#224809,#224810,#224811,#224812,#224813,#224814,#224815,
#224816,#224817,#224818,#224819,#224820,#224821,#224822,#224823,#224824,
#224825,#224826,#224827,#224828,#224829,#224830,#224831,#224832,#224833,
#224834,#224835,#224836,#224837,#224838,#224839,#224840,#224841,#224842,
#224843,#224844,#224845,#224846,#224847,#224848,#224849,#224850,#224851,
#224852,#224853,#224854,#224855,#224856,#224857,#224858,#224859,#224860,
#224861,#224862,#224863,#224864,#224865,#224866,#224867,#224868,#224869,
#224870,#224871,#224872,#224873,#224874,#224875,#224876,#224877,#224878,
#224879,#224880,#224881,#224882,#224883,#224884,#224885,#224886,#224887,
#224888,#224889,#224890,#224891,#224892,#224893,#224894,#224895,#224896,
#224897,#224898),.UNSPECIFIED.,.F.,.F.,(4,3,3,3,3,3,3,3,3,3,3,3,3,3,3,3,
3,3,3,3,3,3,3,3,3,3,3,3,3,3,3,3,3,3,3,3,3,3,3,3,3,3,3,3,3,3,3,3,3,3,3,3,
3,3,3,3,3,3,3,3,3,3,3,3,3,4),(1.78689916273263E-6,0.349245406790117,0.705619403193492,
0.847493897628981,1.09071672564526,1.11694270883417,1.13031122083896,1.14453449936953,
1.20207522753681,1.31684392925775,1.54514481618978,2.44434146799478,4.19003111005039,
4.62046391575794,4.834341084108,4.93927480926269,4.96407578134244,4.99172316125023,
5.04802388301726,6.11997279598932,8.51952615505129,9.48378467016358,9.76391566762591,
10.5357861585198,10.5621467631509,10.5882563452092,10.6358557074836,10.7311025900593,
10.9200281613937,11.2796932852465,12.4465964798207,13.553746576423,14.6336841515732,
15.5822098205818,15.7876476637103,16.1401718470435,16.3220955100764,16.4133639203428,
16.4589226555197,16.4839070143489,16.5091312288925,17.2592565921019,18.2148053264092,
18.4712765951995,20.7885640811388,21.9649409448773,22.0549091144489,22.1009150614603,
22.1430542625552,22.312830378863,22.6646547127049,23.3174872351635,23.9964420606342,
24.6435854565312,25.0185833917038,25.8245931816792,26.0254191587144,26.1198119705167,
26.1655357658906,26.1768238193963,26.1882756857331,26.2133954469193,26.5759403027651,
27.3712415078498,27.6069804389702,28.3229150078202),.UNSPECIFIED.);
#5855=B_SPLINE_CURVE_WITH_KNOTS('',3,(#224900,#224901,#224902,#224903,#224904,
#224905,#224906,#224907,#224908,#224909,#224910,#224911,#224912,#224913,
#224914,#224915,#224916,#224917,#224918,#224919,#224920,#224921,#224922,
#224923,#224924,#224925,#224926,#224927,#224928,#224929,#224930,#224931,
#224932,#224933,#224934,#224935,#224936,#224937,#224938,#224939),
 .UNSPECIFIED.,.F.,.F.,(4,3,3,3,3,3,3,3,3,3,3,3,3,4),(1.49278976973505E-7,
0.141377231663466,0.249999999999955,0.374999999999933,0.437499999999923,
0.468749999999918,0.484374999999916,0.492187499999915,0.499023437499913,
0.499999999999912,0.518810985931556,0.696449207513925,0.858128319650762,
1.),.UNSPECIFIED.);
#5856=B_SPLINE_CURVE_WITH_KNOTS('',3,(#224941,#224942,#224943,#224944,#224945,
#224946),.UNSPECIFIED.,.F.,.F.,(4,2,4),(-0.0631146096128023,-0.0315634825964837,
-2.17021022817649E-6),.UNSPECIFIED.);
#5857=B_SPLINE_CURVE_WITH_KNOTS('',3,(#224948,#224949,#224950,#224951,#224952,
#224953,#224954,#224955,#224956,#224957,#224958,#224959,#224960,#224961,
#224962,#224963,#224964,#224965,#224966,#224967),.UNSPECIFIED.,.F.,.F.,
(4,2,2,2,2,2,2,2,2,4),(9.54272002648276E-7,0.039668729271524,0.0502460852682275,
0.0529093523368603,0.0585862970221902,0.150167472119632,0.47461910179334,
0.71071638044721,0.842512773974448,0.972825733893553),.UNSPECIFIED.);
#5858=B_SPLINE_CURVE_WITH_KNOTS('',3,(#224969,#224970,#224971,#224972,#224973,
#224974),.UNSPECIFIED.,.F.,.F.,(4,2,4),(-0.348032286208327,-0.174233719491681,
-1.04624545273724E-6),.UNSPECIFIED.);
#5859=B_SPLINE_CURVE_WITH_KNOTS('',3,(#224976,#224977,#224978,#224979,#224980,
#224981),.UNSPECIFIED.,.F.,.F.,(4,2,4),(-0.181030043604558,-0.0910312711858393,
-1.10663912709387E-5),.UNSPECIFIED.);
#5860=B_SPLINE_CURVE_WITH_KNOTS('',3,(#224982,#224983,#224984,#224985,#224986,
#224987),.UNSPECIFIED.,.F.,.F.,(4,2,4),(-0.472029599120786,-0.236764162407715,
0.),.UNSPECIFIED.);
#5861=B_SPLINE_CURVE_WITH_KNOTS('',3,(#225594,#225595,#225596,#225597,#225598,
#225599),.UNSPECIFIED.,.F.,.F.,(4,2,4),(-0.0726217219155311,-0.0363071423916649,
-3.64731715070445E-6),.UNSPECIFIED.);
#5862=B_SPLINE_CURVE_WITH_KNOTS('',3,(#225601,#225602,#225603,#225604,#225605,
#225606,#225607,#225608,#225609,#225610,#225611,#225612,#225613,#225614,
#225615,#225616,#225617,#225618,#225619,#225620,#225621,#225622,#225623,
#225624,#225625,#225626,#225627,#225628,#225629,#225630,#225631,#225632,
#225633,#225634,#225635,#225636,#225637,#225638,#225639,#225640,#225641,
#225642,#225643,#225644,#225645,#225646,#225647,#225648,#225649,#225650,
#225651,#225652,#225653,#225654,#225655,#225656,#225657,#225658,#225659,
#225660,#225661),.UNSPECIFIED.,.F.,.F.,(4,3,3,3,3,3,3,3,3,3,3,3,3,3,3,3,
3,3,3,3,4),(6.55221773018224E-8,0.198533780132414,0.249999999999826,0.374999999999739,
0.437499999999696,0.468749999999675,0.484374999999665,0.492187499999661,
0.499023437499656,0.499999999999657,0.608653468230123,0.624999999999709,
0.687499999999737,0.71874999999975,0.734374999999758,0.742187499999761,
0.748046874999763,0.749999999999764,0.857427266285853,0.964048886395737,
1.),.UNSPECIFIED.);
#5863=B_SPLINE_CURVE_WITH_KNOTS('',3,(#225662,#225663,#225664,#225665,#225666,
#225667,#225668,#225669,#225670,#225671,#225672,#225673,#225674,#225675,
#225676,#225677,#225678,#225679,#225680,#225681,#225682,#225683,#225684,
#225685,#225686,#225687,#225688,#225689,#225690,#225691,#225692,#225693,
#225694,#225695,#225696,#225697,#225698,#225699,#225700,#225701,#225702,
#225703,#225704,#225705,#225706,#225707,#225708,#225709,#225710,#225711,
#225712,#225713,#225714,#225715,#225716,#225717,#225718,#225719,#225720,
#225721,#225722,#225723,#225724,#225725,#225726,#225727,#225728,#225729,
#225730,#225731,#225732,#225733,#225734,#225735,#225736,#225737,#225738,
#225739,#225740,#225741,#225742,#225743,#225744,#225745,#225746,#225747,
#225748,#225749,#225750,#225751,#225752,#225753,#225754,#225755,#225756,
#225757,#225758,#225759,#225760,#225761,#225762,#225763,#225764,#225765,
#225766,#225767,#225768,#225769,#225770,#225771,#225772,#225773,#225774,
#225775,#225776,#225777,#225778,#225779,#225780,#225781,#225782,#225783,
#225784,#225785,#225786,#225787,#225788,#225789,#225790,#225791,#225792,
#225793,#225794,#225795,#225796,#225797,#225798,#225799,#225800,#225801,
#225802,#225803,#225804,#225805,#225806,#225807,#225808,#225809,#225810,
#225811,#225812,#225813,#225814,#225815,#225816,#225817,#225818,#225819,
#225820,#225821,#225822,#225823,#225824,#225825,#225826,#225827,#225828,
#225829,#225830,#225831,#225832,#225833),.UNSPECIFIED.,.F.,.F.,(4,3,3,3,
3,3,3,3,3,3,3,3,3,3,3,3,3,3,3,3,3,3,3,3,3,3,3,3,3,3,3,3,3,3,3,3,3,3,3,3,
3,3,3,3,3,3,3,3,3,3,3,3,3,3,3,3,3,4),(-10.0118009515725,-9.380144348375,
-9.28193689793529,-9.22251029152007,-9.19147789919078,-9.17779037797217,
-9.16464451434807,-9.13017042783428,-8.99160305605499,-8.68736646402747,
-8.52180373132443,-8.41041892963837,-8.3758072763443,-8.35673588517422,
-8.35173647900018,-8.34601909497381,-8.33358519993068,-8.21883901831532,
-7.28686586998718,-7.16008381787202,-6.80650500239442,-6.50180850406331,
-6.46109833741843,-6.44123587433924,-6.42379799474065,-6.35522340568956,
-6.22668897461121,-5.92002477860756,-5.3247417048503,-4.86206937746766,
-4.42610453669277,-4.30346091911995,-4.23870089998684,-4.22228697144672,
-4.20361062602334,-4.16537895898503,-3.87762847487079,-3.76886371593885,
-3.42827377469716,-2.92395744537593,-2.56497067190565,-2.45214102185328,
-2.43752731019248,-2.43051889000834,-2.42424270775226,-2.39905523317864,
-2.3485592868193,-2.15607432218952,-1.86312912747339,-1.70318514070286,
-1.39379233399322,-1.14178495836116,-1.12409212545336,-1.10568452874485,
-1.06389214424081,-0.982911261414093,-0.846211153564692,-6.66741710329381E-6),
 .UNSPECIFIED.);
#5864=B_SPLINE_CURVE_WITH_KNOTS('',3,(#225834,#225835,#225836,#225837,#225838,
#225839,#225840,#225841,#225842,#225843,#225844,#225845,#225846,#225847,
#225848,#225849,#225850,#225851,#225852,#225853,#225854,#225855,#225856,
#225857,#225858,#225859,#225860,#225861),.UNSPECIFIED.,.F.,.F.,(4,3,3,3,
3,3,3,3,3,4),(2.47031549411892E-5,0.330322577512475,0.531914497354827,0.575033270917861,
0.692616065858012,0.756752965780754,0.790033944881865,0.804313961995532,
0.818107734326963,0.901208376257383),.UNSPECIFIED.);
#5865=B_SPLINE_CURVE_WITH_KNOTS('',3,(#225863,#225864,#225865,#225866,#225867,
#225868,#225869,#225870,#225871,#225872),.UNSPECIFIED.,.F.,.F.,(4,2,2,2,
4),(1.01154219413529E-6,0.197911925947378,0.383079900974823,0.578872967472904,
0.753869196345672),.UNSPECIFIED.);
#5866=B_SPLINE_CURVE_WITH_KNOTS('',3,(#225874,#225875,#225876,#225877,#225878,
#225879),.UNSPECIFIED.,.F.,.F.,(4,2,4),(-0.52032371085874,-0.260164299656232,
-1.26885779850293E-6),.UNSPECIFIED.);
#5867=B_SPLINE_CURVE_WITH_KNOTS('',3,(#225881,#225882,#225883,#225884,#225885,
#225886,#225887,#225888,#225889,#225890),.UNSPECIFIED.,.F.,.F.,(4,2,2,2,
4),(-0.808794323077665,-0.596464192824083,-0.397805427063807,-0.187747447983837,
-1.59820013576218E-6),.UNSPECIFIED.);
#5868=B_SPLINE_CURVE_WITH_KNOTS('',3,(#225892,#225893,#225894,#225895,#225896,
#225897),.UNSPECIFIED.,.F.,.F.,(4,2,4),(-0.512833689847384,-0.262850347931808,
-2.73829768859812E-8),.UNSPECIFIED.);
#5869=B_SPLINE_CURVE_WITH_KNOTS('',3,(#225898,#225899,#225900,#225901,#225902,
#225903,#225904,#225905,#225906,#225907,#225908,#225909,#225910,#225911,
#225912,#225913,#225914,#225915,#225916,#225917,#225918,#225919,#225920,
#225921,#225922),.UNSPECIFIED.,.F.,.F.,(4,3,3,3,3,3,3,3,4),(-0.582199554717882,
-0.346112236555124,-0.210722915399725,-0.134760117007276,-0.0933253284297944,
-0.0718245964311411,-0.0625992031160378,-0.0536879216367247,-1.96467184541608E-6),
 .UNSPECIFIED.);
#5870=B_SPLINE_CURVE_WITH_KNOTS('',3,(#225965,#225966,#225967,#225968,#225969,
#225970),.UNSPECIFIED.,.F.,.F.,(4,2,4),(-0.234147853965519,-0.114087724688498,
0.),.UNSPECIFIED.);
#5871=B_SPLINE_CURVE_WITH_KNOTS('',3,(#226350,#226351,#226352,#226353,#226354,
#226355,#226356,#226357,#226358,#226359,#226360,#226361,#226362,#226363,
#226364,#226365,#226366,#226367,#226368,#226369),.UNSPECIFIED.,.F.,.F.,
(4,2,2,2,2,2,2,2,2,4),(-0.238232821898405,-0.205423492378447,-0.197085539277143,
-0.169892934987575,-0.105862923175614,-0.0753554195472226,-0.0349310916978768,
-0.0193510418585195,-0.0118234613898232,0.),.UNSPECIFIED.);
#5872=B_SPLINE_CURVE_WITH_KNOTS('',3,(#226371,#226372,#226373,#226374,#226375,
#226376,#226377,#226378,#226379,#226380,#226381,#226382,#226383),
 .UNSPECIFIED.,.F.,.F.,(4,3,3,3,4),(0.,0.248409226325233,0.499006625537372,
0.502852684896152,1.),.UNSPECIFIED.);
#5873=B_SPLINE_CURVE_WITH_KNOTS('',3,(#226385,#226386,#226387,#226388,#226389,
#226390,#226391,#226392,#226393,#226394,#226395,#226396,#226397,#226398,
#226399,#226400,#226401,#226402,#226403,#226404,#226405,#226406),
 .UNSPECIFIED.,.F.,.F.,(4,2,2,2,2,2,2,2,2,2,4),(4.11923473698837E-6,0.0532044237289185,
0.112114067677964,0.129888742302041,0.273554203521723,0.318355137795804,
0.394719390871768,0.446820142683063,0.478015292941828,0.517144072378212,
0.549044733910222),.UNSPECIFIED.);
#5874=B_SPLINE_CURVE_WITH_KNOTS('',3,(#226408,#226409,#226410,#226411,#226412,
#226413),.UNSPECIFIED.,.F.,.F.,(4,2,4),(-0.0469583750615504,-0.0233153845128203,
0.),.UNSPECIFIED.);
#5875=B_SPLINE_CURVE_WITH_KNOTS('',3,(#226414,#226415,#226416,#226417),
 .UNSPECIFIED.,.F.,.F.,(4,4),(0.0542180481640577,0.969015107905792),
 .UNSPECIFIED.);
#5876=B_SPLINE_CURVE_WITH_KNOTS('',3,(#226979,#226980,#226981,#226982,#226983,
#226984,#226985,#226986,#226987,#226988,#226989,#226990,#226991,#226992,
#226993,#226994,#226995,#226996,#226997,#226998,#226999,#227000),
 .UNSPECIFIED.,.F.,.F.,(4,2,2,2,2,2,2,2,2,2,4),(-0.0469823194624915,-0.0448779513354515,
-0.043871616538125,-0.0417699201921335,-0.0365670119809625,-0.0349794965192584,
-0.029838901311014,-0.0234761972380763,-0.0131803115290423,-0.00771050065983768,
-9.96545261977566E-7),.UNSPECIFIED.);
#5877=B_SPLINE_CURVE_WITH_KNOTS('',3,(#227002,#227003,#227004,#227005),
 .UNSPECIFIED.,.F.,.F.,(4,4),(0.0559227492896307,0.969509810868812),
 .UNSPECIFIED.);
#5878=B_SPLINE_CURVE_WITH_KNOTS('',3,(#227007,#227008,#227009,#227010,#227011,
#227012,#227013,#227014,#227015,#227016),.UNSPECIFIED.,.F.,.F.,(4,2,2,2,
4),(1.01948866288982E-6,0.0265245583807015,0.039717133035126,0.0460199136553313,
0.0521877159679606),.UNSPECIFIED.);
#5879=B_SPLINE_CURVE_WITH_KNOTS('',3,(#227018,#227019,#227020,#227021,#227022,
#227023,#227024,#227025,#227026,#227027,#227028,#227029,#227030,#227031,
#227032,#227033,#227034,#227035,#227036,#227037,#227038,#227039,#227040,
#227041),.UNSPECIFIED.,.F.,.F.,(4,2,2,2,2,2,2,2,2,2,2,4),(8.74098857277626E-8,
0.0345413375471952,0.0478434921558638,0.108389819035251,0.162764294558867,
0.195585772394031,0.213488203760146,0.254799752738697,0.385293361542727,
0.417463559505062,0.440592486828372,0.505162485488175),.UNSPECIFIED.);
#5880=B_SPLINE_CURVE_WITH_KNOTS('',3,(#227042,#227043,#227044,#227045,#227046,
#227047,#227048,#227049,#227050,#227051,#227052,#227053,#227054),
 .UNSPECIFIED.,.F.,.F.,(4,3,3,3,4),(0.,0.121286618183145,0.248611887968643,
0.503260702170736,1.),.UNSPECIFIED.);
#5881=B_SPLINE_CURVE_WITH_KNOTS('',3,(#227421,#227422,#227423,#227424,#227425,
#227426,#227427,#227428,#227429,#227430,#227431,#227432,#227433,#227434,
#227435,#227436,#227437,#227438,#227439,#227440),.UNSPECIFIED.,.F.,.F.,
(4,2,2,2,2,2,2,2,2,4),(-0.115918278885804,-0.0892169661896314,-0.0795730255112448,
-0.0500602494615251,-0.0402734344922609,-0.0327836602742112,-0.0258163526316461,
-0.0148454000357724,-0.00934050276061678,0.),.UNSPECIFIED.);
#5882=B_SPLINE_CURVE_WITH_KNOTS('',3,(#227442,#227443,#227444,#227445,#227446,
#227447,#227448,#227449,#227450,#227451,#227452,#227453,#227454),
 .UNSPECIFIED.,.F.,.F.,(4,3,3,3,4),(0.,0.248207134125547,0.498866213704792,
0.502443591376185,1.),.UNSPECIFIED.);
#5883=B_SPLINE_CURVE_WITH_KNOTS('',3,(#227456,#227457,#227458,#227459,#227460,
#227461,#227462,#227463,#227464,#227465,#227466,#227467,#227468,#227469,
#227470,#227471,#227472,#227473,#227474,#227475,#227476,#227477,#227478,
#227479),.UNSPECIFIED.,.F.,.F.,(4,2,2,2,2,2,2,2,2,2,2,4),(1.34129012567919E-6,
0.0388365429884076,0.0809349663735409,0.110652786603789,0.150076448441442,
0.202495348256536,0.235137840136492,0.290402658704084,0.327987073052442,
0.350910589522497,0.380240175864255,0.404554968880074),.UNSPECIFIED.);
#5884=B_SPLINE_CURVE_WITH_KNOTS('',3,(#227481,#227482,#227483,#227484,#227485,
#227486),.UNSPECIFIED.,.F.,.F.,(4,2,4),(-0.0432556987863833,-0.0214374711513382,
0.),.UNSPECIFIED.);
#5885=B_SPLINE_CURVE_WITH_KNOTS('',3,(#227487,#227488,#227489,#227490),
 .UNSPECIFIED.,.F.,.F.,(4,4),(0.,1.),.UNSPECIFIED.);
#5886=B_SPLINE_CURVE_WITH_KNOTS('',3,(#228013,#228014,#228015,#228016,#228017,
#228018,#228019,#228020,#228021,#228022,#228023,#228024,#228025,#228026,
#228027,#228028),.UNSPECIFIED.,.F.,.F.,(4,2,2,2,2,2,2,4),(-0.0532039057008744,
-0.0485064898699985,-0.0454445922183713,-0.0383797315059074,-0.0340621721264607,
-0.0219073807078276,-0.0140093117094523,-9.96369002963238E-7),
 .UNSPECIFIED.);
#5887=B_SPLINE_CURVE_WITH_KNOTS('',3,(#228030,#228031,#228032,#228033),
 .UNSPECIFIED.,.F.,.F.,(4,4),(0.0408435581858526,0.955362835047561),
 .UNSPECIFIED.);
#5888=B_SPLINE_CURVE_WITH_KNOTS('',3,(#228035,#228036,#228037,#228038,#228039,
#228040,#228041,#228042),.UNSPECIFIED.,.F.,.F.,(4,2,2,4),(1.01576402050443E-6,
0.0186922722070423,0.028158435435005,0.0372206145737922),.UNSPECIFIED.);
#5889=B_SPLINE_CURVE_WITH_KNOTS('',3,(#228044,#228045,#228046,#228047,#228048,
#228049,#228050,#228051,#228052,#228053,#228054,#228055,#228056,#228057,
#228058,#228059,#228060,#228061,#228062,#228063,#228064,#228065,#228066,
#228067,#228068,#228069),.UNSPECIFIED.,.F.,.F.,(4,2,2,2,2,2,2,2,2,2,2,2,
4),(1.00349669506866E-6,0.0149902028524071,0.0301796168541512,0.0653312244747095,
0.0929080820335093,0.137456013888724,0.20183246394693,0.239455773090012,
0.30227612781367,0.325926095178214,0.367602393520655,0.426119367916936,
0.477863235121803),.UNSPECIFIED.);
#5890=B_SPLINE_CURVE_WITH_KNOTS('',3,(#228070,#228071,#228072,#228073,#228074,
#228075),.UNSPECIFIED.,.F.,.F.,(4,2,4),(1.21996442589897E-8,0.499703627209769,
0.999999992717194),.UNSPECIFIED.);
#5891=B_SPLINE_CURVE_WITH_KNOTS('',3,(#228082,#228083,#228084,#228085,#228086,
#228087),.UNSPECIFIED.,.F.,.F.,(4,2,4),(1.00005279208342E-6,0.0180894029160134,
0.0360332116186634),.UNSPECIFIED.);
#5892=B_SPLINE_CURVE_WITH_KNOTS('',3,(#228090,#228091,#228092,#228093,#228094,
#228095,#228096,#228097),.UNSPECIFIED.,.F.,.F.,(4,2,2,4),(1.68023398205945E-6,
0.123369994045964,0.250885389419846,0.502640983753045),.UNSPECIFIED.);
#5893=B_SPLINE_CURVE_WITH_KNOTS('',3,(#228102,#228103,#228104,#228105,#228106,
#228107),.UNSPECIFIED.,.F.,.F.,(4,2,4),(9.99995512679503E-7,0.251122560205324,
0.500936979469621),.UNSPECIFIED.);
#5894=B_SPLINE_CURVE_WITH_KNOTS('',3,(#228122,#228123,#228124,#228125,#228126,
#228127),.UNSPECIFIED.,.F.,.F.,(4,2,4),(1.74474206022349E-6,0.259610843491103,
0.519873535593903),.UNSPECIFIED.);
#5895=B_SPLINE_CURVE_WITH_KNOTS('',3,(#228132,#228133,#228134,#228135,#228136,
#228137,#228138,#228139),.UNSPECIFIED.,.F.,.F.,(4,2,2,4),(9.99996049876919E-7,
0.25935475971615,0.390604083523162,0.518299611782085),.UNSPECIFIED.);
#5896=B_SPLINE_CURVE_WITH_KNOTS('',3,(#228147,#228148,#228149,#228150,#228151,
#228152),.UNSPECIFIED.,.F.,.F.,(4,2,4),(5.20898920908954E-7,0.394546120022865,
0.789090255646932),.UNSPECIFIED.);
#5897=B_SPLINE_CURVE_WITH_KNOTS('',3,(#228224,#228225,#228226,#228227,#228228,
#228229),.UNSPECIFIED.,.F.,.F.,(4,2,4),(-0.768987117999718,-0.384501938178755,
-6.39808872548997E-10),.UNSPECIFIED.);
#5898=B_SPLINE_CURVE_WITH_KNOTS('',3,(#228231,#228232,#228233,#228234,#228235,
#228236),.UNSPECIFIED.,.F.,.F.,(4,2,4),(7.16885188820924E-6,0.389700990930307,
0.77940084823311),.UNSPECIFIED.);
#5899=B_SPLINE_CURVE_WITH_KNOTS('',3,(#228237,#228238,#228239,#228240,#228241,
#228242),.UNSPECIFIED.,.F.,.F.,(4,2,4),(-2.50574735670183,-1.27023285791173,
-1.26197706507014E-7),.UNSPECIFIED.);
#5900=B_SPLINE_CURVE_WITH_KNOTS('',3,(#228260,#228261,#228262,#228263,#228264,
#228265),.UNSPECIFIED.,.F.,.F.,(4,2,4),(5.46905462932057E-7,0.391794447842365,
0.783582614970145),.UNSPECIFIED.);
#5901=B_SPLINE_CURVE_WITH_KNOTS('',3,(#228267,#228268,#228269,#228270,#228271,
#228272),.UNSPECIFIED.,.F.,.F.,(4,2,4),(-0.774055471160218,-0.387030382163849,
-1.38207304385376E-5),.UNSPECIFIED.);
#5902=B_SPLINE_CURVE_WITH_KNOTS('',3,(#228273,#228274,#228275,#228276,#228277,
#228278),.UNSPECIFIED.,.F.,.F.,(4,2,4),(-2.41443710174894,-1.18731782863127,
-8.04546614600221E-6),.UNSPECIFIED.);
#5903=B_SPLINE_CURVE_WITH_KNOTS('',3,(#228280,#228281,#228282,#228283,#228284,
#228285,#228286,#228287,#228288,#228289,#228290,#228291,#228292,#228293,
#228294,#228295,#228296,#228297,#228298,#228299,#228300,#228301,#228302,
#228303,#228304,#228305,#228306,#228307,#228308,#228309,#228310,#228311,
#228312,#228313,#228314,#228315,#228316,#228317,#228318,#228319,#228320,
#228321,#228322,#228323,#228324,#228325,#228326,#228327,#228328,#228329,
#228330,#228331,#228332,#228333,#228334,#228335,#228336,#228337,#228338,
#228339,#228340,#228341,#228342,#228343,#228344,#228345,#228346,#228347,
#228348,#228349,#228350,#228351,#228352,#228353,#228354,#228355,#228356,
#228357,#228358,#228359,#228360,#228361,#228362,#228363,#228364,#228365,
#228366,#228367,#228368,#228369,#228370,#228371,#228372,#228373,#228374,
#228375,#228376,#228377,#228378,#228379,#228380,#228381,#228382,#228383,
#228384,#228385,#228386,#228387,#228388,#228389,#228390,#228391,#228392,
#228393,#228394,#228395,#228396,#228397,#228398,#228399,#228400,#228401,
#228402,#228403,#228404,#228405,#228406,#228407,#228408,#228409,#228410,
#228411,#228412,#228413,#228414,#228415,#228416,#228417,#228418,#228419,
#228420,#228421,#228422,#228423,#228424,#228425,#228426,#228427,#228428,
#228429,#228430,#228431,#228432,#228433,#228434,#228435,#228436,#228437,
#228438,#228439,#228440,#228441,#228442,#228443,#228444,#228445,#228446,
#228447,#228448,#228449,#228450,#228451,#228452,#228453,#228454,#228455,
#228456,#228457,#228458,#228459,#228460),.UNSPECIFIED.,.F.,.F.,(4,3,3,3,
3,3,3,3,3,3,3,3,3,3,3,3,3,3,3,3,3,3,3,3,3,3,3,3,3,3,3,3,3,3,3,3,3,3,3,3,
3,3,3,3,3,3,3,3,3,3,3,3,3,3,3,3,3,3,3,3,4),(0.,0.101652515081683,0.840095270426277,
0.951350449593331,1.11460256910622,1.20222962321025,1.21337770183555,1.22322866068737,
1.24215508047792,1.27918762477272,1.41444382060503,1.91308482137222,2.16293686170842,
2.31873870184034,2.3388699155934,2.35956243431462,2.40573771750418,2.49173011142808,
2.50522275730167,2.72512517847504,3.09820563685861,3.40471762826703,3.56238559688252,
3.65675659727303,3.66930952721422,3.67553938673372,3.68097533151684,3.70277767984807,
3.74615446777659,3.93440481248742,4.2762919621573,4.4629569057448,4.80246566838423,
4.84531684069589,4.86725425690884,4.87828571635999,4.89073026763831,4.98934387426452,
5.14829048116897,5.43554060290253,5.98928985210521,6.05987373854709,6.09759598641818,
6.10721678864328,6.11134856344036,6.11540864995827,6.1317539654039,6.26291140079336,
6.47575952606869,6.58219308214426,6.81129554606021,6.90189743840945,6.92504908218588,
6.935638466,6.94054062150879,6.9429390153616,6.94566168795314,6.98260356735261,
7.08304507613446,7.15822821963323,7.33584769615335),.UNSPECIFIED.);
#5904=B_SPLINE_CURVE_WITH_KNOTS('',3,(#228478,#228479,#228480,#228481,#228482,
#228483),.UNSPECIFIED.,.F.,.F.,(4,2,4),(2.70771998432966E-6,0.460501033060921,
0.921000224556805),.UNSPECIFIED.);
#5905=B_SPLINE_CURVE_WITH_KNOTS('',3,(#228490,#228491,#228492,#228493,#228494,
#228495,#228496,#228497,#228498,#228499,#228500,#228501,#228502,#228503,
#228504,#228505),.UNSPECIFIED.,.F.,.F.,(4,2,2,2,2,2,2,4),(-0.982605045330243,
-0.957450000265146,-0.931726665878099,-0.879221227191873,-0.770280103416555,
-0.542311900866116,-0.311877616829005,-1.70255117412049E-6),
 .UNSPECIFIED.);
#5906=B_SPLINE_CURVE_WITH_KNOTS('',3,(#228506,#228507,#228508,#228509,#228510,
#228511),.UNSPECIFIED.,.F.,.F.,(4,2,4),(-0.0722680566464597,-0.0361746296017969,
0.),.UNSPECIFIED.);
#5907=B_SPLINE_CURVE_WITH_KNOTS('',3,(#228530,#228531,#228532,#228533,#228534,
#228535),.UNSPECIFIED.,.F.,.F.,(4,2,4),(1.77148721322176E-6,0.0720279028463182,
0.144150482966194),.UNSPECIFIED.);
#5908=B_SPLINE_CURVE_WITH_KNOTS('',3,(#228538,#228539,#228540,#228541,#228542,
#228543),.UNSPECIFIED.,.F.,.F.,(4,2,4),(2.79355861066373E-6,0.0720991492051481,
0.143966171702797),.UNSPECIFIED.);
#5909=B_SPLINE_CURVE_WITH_KNOTS('',3,(#228741,#228742,#228743,#228744,#228745,
#228746,#228747,#228748,#228749,#228750,#228751,#228752,#228753,#228754),
 .UNSPECIFIED.,.F.,.F.,(4,2,2,2,2,2,4),(8.79576979640004E-7,0.161091039185441,
0.353936447289158,0.714835470723924,1.15295148424327,1.32088879345487,1.48892420048076),
 .UNSPECIFIED.);
#5910=B_SPLINE_CURVE_WITH_KNOTS('',3,(#228756,#228757,#228758,#228759,#228760,
#228761),.UNSPECIFIED.,.F.,.F.,(4,2,4),(1.48538090247618E-6,0.0297476815236481,
0.059493920780927),.UNSPECIFIED.);
#5911=B_SPLINE_CURVE_WITH_KNOTS('',3,(#228763,#228764,#228765,#228766,#228767,
#228768),.UNSPECIFIED.,.F.,.F.,(4,2,4),(2.90466498097714E-6,0.053152581148337,
0.106304452166784),.UNSPECIFIED.);
#5912=B_SPLINE_CURVE_WITH_KNOTS('',3,(#228769,#228770,#228771,#228772,#228773,
#228774),.UNSPECIFIED.,.F.,.F.,(4,2,4),(5.00463248281416E-6,0.14458386001298,
0.288882060685716),.UNSPECIFIED.);
#5913=B_SPLINE_CURVE_WITH_KNOTS('',3,(#228775,#228776,#228777,#228778,#228779,
#228780,#228781,#228782,#228783,#228784,#228785,#228786,#228787,#228788),
 .UNSPECIFIED.,.F.,.F.,(4,2,2,2,2,2,4),(-1.33002773489275,-1.19632686097329,
-1.0309504969832,-0.691984499274297,-0.293184319134546,-0.147201401084202,
-3.05059735880904E-6),.UNSPECIFIED.);
#5914=B_SPLINE_CURVE_WITH_KNOTS('',3,(#228789,#228790,#228791,#228792,#228793,
#228794,#228795,#228796,#228797,#228798,#228799,#228800,#228801,#228802,
#228803,#228804),.UNSPECIFIED.,.F.,.F.,(4,2,2,2,2,2,2,4),(-2.53746494961163,
-2.46422033767662,-2.38938785749608,-2.23702354943545,-1.92260251519736,
-1.27022304439062,-0.614575319391794,-8.39797342777615E-9),
 .UNSPECIFIED.);
#5915=B_SPLINE_CURVE_WITH_KNOTS('',3,(#228807,#228808,#228809,#228810,#228811,
#228812),.UNSPECIFIED.,.F.,.F.,(4,2,4),(-0.0311640358773885,-0.0155842549001969,
-7.32013339722184E-7),.UNSPECIFIED.);
#5916=B_SPLINE_CURVE_WITH_KNOTS('',3,(#228815,#228816,#228817,#228818,#228819,
#228820),.UNSPECIFIED.,.F.,.F.,(4,2,4),(-0.118814653628038,-0.0594775620868716,
-8.25559444165143E-6),.UNSPECIFIED.);
#5917=B_SPLINE_CURVE_WITH_KNOTS('',3,(#229102,#229103,#229104,#229105,#229106,
#229107,#229108,#229109,#229110,#229111,#229112,#229113,#229114,#229115,
#229116,#229117),.UNSPECIFIED.,.F.,.F.,(4,2,2,2,2,2,2,4),(1.31319461189347E-5,
0.0969398305739712,0.200592571707003,0.40568002081205,0.731947033912492,
1.15360029034027,1.33098563964491,1.51064986605988),.UNSPECIFIED.);
#5918=B_SPLINE_CURVE_WITH_KNOTS('',3,(#229118,#229119,#229120,#229121),
 .UNSPECIFIED.,.F.,.F.,(4,4),(0.,1.),.UNSPECIFIED.);
#5919=B_SPLINE_CURVE_WITH_KNOTS('',3,(#229122,#229123,#229124,#229125,#229126,
#229127,#229128,#229129,#229130,#229131,#229132,#229133,#229134,#229135,
#229136,#229137),.UNSPECIFIED.,.F.,.F.,(4,2,2,2,2,2,2,4),(1.00000001008263E-6,
0.147548369920231,0.335441273894288,0.717509453274639,1.00870782358177,
1.20577091648481,1.30068851548524,1.39147288337523),.UNSPECIFIED.);
#5920=B_SPLINE_CURVE_WITH_KNOTS('',3,(#229141,#229142,#229143,#229144,#229145,
#229146),.UNSPECIFIED.,.F.,.F.,(4,2,4),(-0.0694028841990137,-0.0347037380359889,
-4.89524744334324E-5),.UNSPECIFIED.);
#5921=B_SPLINE_CURVE_WITH_KNOTS('',3,(#229151,#229152,#229153,#229154,#229155,
#229156),.UNSPECIFIED.,.F.,.F.,(4,2,4),(-0.256260280232773,-0.128094391485911,
-2.91397728446885E-7),.UNSPECIFIED.);
#5922=B_SPLINE_CURVE_WITH_KNOTS('',3,(#229161,#229162,#229163,#229164,#229165,
#229166),.UNSPECIFIED.,.F.,.F.,(4,2,4),(-0.335038423290503,-0.16756094841115,
-4.64089220713822E-5),.UNSPECIFIED.);
#5923=B_SPLINE_CURVE_WITH_KNOTS('',3,(#229171,#229172,#229173,#229174,#229175,
#229176),.UNSPECIFIED.,.F.,.F.,(4,2,4),(-0.259482172087391,-0.12980603886175,
-3.40862289005539E-7),.UNSPECIFIED.);
#5924=B_SPLINE_CURVE_WITH_KNOTS('',3,(#229186,#229187,#229188,#229189,#229190,
#229191,#229192,#229193),.UNSPECIFIED.,.F.,.F.,(4,2,2,4),(-0.240357308665275,
-0.138634339792356,-0.0669247924035088,0.),.UNSPECIFIED.);
#5925=B_SPLINE_CURVE_WITH_KNOTS('',3,(#229195,#229196,#229197,#229198,#229199,
#229200,#229201,#229202),.UNSPECIFIED.,.F.,.F.,(4,2,2,4),(4.59252772077989E-7,
0.137071464030345,0.235092069952917,0.323700448386457),.UNSPECIFIED.);
#5926=B_SPLINE_CURVE_WITH_KNOTS('',3,(#229208,#229209,#229210,#229211,#229212,
#229213),.UNSPECIFIED.,.F.,.F.,(4,2,4),(1.6862576013651E-6,0.176160467008657,
0.356495154469502),.UNSPECIFIED.);
#5927=B_SPLINE_CURVE_WITH_KNOTS('',3,(#229214,#229215,#229216,#229217,#229218,
#229219,#229220,#229221),.UNSPECIFIED.,.F.,.F.,(4,2,2,4),(1.58031091229498E-6,
0.158410018331858,0.208087193257185,0.449161461367469),.UNSPECIFIED.);
#5928=B_SPLINE_CURVE_WITH_KNOTS('',3,(#229224,#229225,#229226,#229227,#229228,
#229229),.UNSPECIFIED.,.F.,.F.,(4,2,4),(0.000426112405584672,0.120709745014509,
0.235106063097469),.UNSPECIFIED.);
#5929=B_SPLINE_CURVE_WITH_KNOTS('',3,(#229235,#229236,#229237,#229238,#229239,
#229240,#229241,#229242,#229243,#229244),.UNSPECIFIED.,.F.,.F.,(4,2,2,2,
4),(2.26014760912018E-6,0.103733355677681,0.121992468029059,0.239304910920547,
0.648027032476922),.UNSPECIFIED.);
#5930=B_SPLINE_CURVE_WITH_KNOTS('',3,(#229245,#229246,#229247,#229248,#229249,
#229250),.UNSPECIFIED.,.F.,.F.,(4,2,4),(0.,0.135475174046834,0.275618423023284),
 .UNSPECIFIED.);
#5931=B_SPLINE_CURVE_WITH_KNOTS('',3,(#230358,#230359,#230360,#230361,#230362,
#230363),.UNSPECIFIED.,.F.,.F.,(4,2,4),(-0.259382230541658,-0.131398743270302,
-4.17832249355321E-7),.UNSPECIFIED.);
#5932=B_SPLINE_CURVE_WITH_KNOTS('',3,(#230364,#230365,#230366,#230367,#230368,
#230369),.UNSPECIFIED.,.F.,.F.,(4,2,4),(-0.27137277077401,-0.135669107685874,
-1.55628221640116E-6),.UNSPECIFIED.);
#5933=B_SPLINE_CURVE_WITH_KNOTS('',3,(#230370,#230371,#230372,#230373,#230374,
#230375),.UNSPECIFIED.,.F.,.F.,(4,2,4),(-0.267093811957073,-0.133661308819734,
-7.086251292861E-6),.UNSPECIFIED.);
#5934=B_SPLINE_CURVE_WITH_KNOTS('',3,(#230377,#230378,#230379,#230380,#230381,
#230382),.UNSPECIFIED.,.F.,.F.,(4,2,4),(-0.24460605653258,-0.120778493079658,
0.),.UNSPECIFIED.);
#5935=B_SPLINE_CURVE_WITH_KNOTS('',3,(#230383,#230384,#230385,#230386),
 .UNSPECIFIED.,.F.,.F.,(4,4),(-5.76565965941832E-6,0.),.UNSPECIFIED.);
#5936=B_SPLINE_CURVE_WITH_KNOTS('',3,(#230387,#230388,#230389,#230390),
 .UNSPECIFIED.,.F.,.F.,(4,4),(0.,2.59792363940038E-6),.UNSPECIFIED.);
#5937=B_SPLINE_CURVE_WITH_KNOTS('',3,(#230914,#230915,#230916,#230917),
 .UNSPECIFIED.,.F.,.F.,(4,4),(0.0216968151072032,0.926937308587682),
 .UNSPECIFIED.);
#5938=B_SPLINE_CURVE_WITH_KNOTS('',3,(#231018,#231019,#231020,#231021),
 .UNSPECIFIED.,.F.,.F.,(4,4),(0.0222286199771242,0.926269849314919),
 .UNSPECIFIED.);
#5939=B_SPLINE_CURVE_WITH_KNOTS('',3,(#231099,#231100,#231101,#231102),
 .UNSPECIFIED.,.F.,.F.,(4,4),(0.0248339691417604,0.928145544482466),
 .UNSPECIFIED.);
#5940=B_SPLINE_CURVE_WITH_KNOTS('',3,(#231224,#231225,#231226,#231227),
 .UNSPECIFIED.,.F.,.F.,(4,4),(0.0238586497886119,0.928715545244436),
 .UNSPECIFIED.);
#5941=B_SPLINE_CURVE_WITH_KNOTS('',3,(#233265,#233266,#233267,#233268,#233269,
#233270,#233271,#233272,#233273,#233274,#233275,#233276,#233277,#233278,
#233279,#233280,#233281,#233282),.UNSPECIFIED.,.F.,.F.,(4,2,2,2,2,2,2,2,
4),(0.250531060456585,0.281923860175215,0.313316659893845,0.343787122861574,
0.374257585829303,0.404728048797032,0.435198511764761,0.466591311483391,
0.497984111202021),.UNSPECIFIED.);
#5942=B_SPLINE_CURVE_WITH_KNOTS('',3,(#233285,#233286,#233287,#233288,#233289,
#233290,#233291,#233292,#233293,#233294,#233295,#233296,#233297,#233298,
#233299,#233300,#233301,#233302),.UNSPECIFIED.,.F.,.F.,(4,2,2,2,2,2,2,2,
4),(-0.497984111202022,-0.466591311483392,-0.435198511764761,-0.404728048797032,
-0.374257585829303,-0.343787122861574,-0.313316659893845,-0.281923860175215,
-0.250531060456585),.UNSPECIFIED.);
#5943=B_SPLINE_CURVE_WITH_KNOTS('',3,(#233577,#233578,#233579,#233580,#233581,
#233582,#233583,#233584,#233585,#233586,#233587,#233588,#233589,#233590,
#233591,#233592,#233593,#233594),.UNSPECIFIED.,.F.,.F.,(4,2,2,2,2,2,2,2,
4),(0.250531060456585,0.281923860175215,0.313316659893845,0.343787122861574,
0.374257585829303,0.404728048797032,0.435198511764761,0.466591311483391,
0.497984111202021),.UNSPECIFIED.);
#5944=B_SPLINE_CURVE_WITH_KNOTS('',3,(#233597,#233598,#233599,#233600,#233601,
#233602,#233603,#233604,#233605,#233606,#233607,#233608,#233609,#233610,
#233611,#233612,#233613,#233614),.UNSPECIFIED.,.F.,.F.,(4,2,2,2,2,2,2,2,
4),(-0.497984111202022,-0.466591311483392,-0.435198511764761,-0.404728048797032,
-0.374257585829303,-0.343787122861574,-0.313316659893845,-0.281923860175215,
-0.250531060456585),.UNSPECIFIED.);
#5945=B_SPLINE_CURVE_WITH_KNOTS('',3,(#233663,#233664,#233665,#233666,#233667,
#233668,#233669,#233670,#233671,#233672),.UNSPECIFIED.,.F.,.F.,(4,2,2,2,
4),(-0.151069834593804,-0.13224008360155,-0.113410332609297,-0.0944672174322318,
-0.0755241022551671),.UNSPECIFIED.);
#5946=B_SPLINE_CURVE_WITH_KNOTS('',3,(#233695,#233696,#233697,#233698,#233699,
#233700,#233701,#233702,#233703,#233704),.UNSPECIFIED.,.F.,.F.,(4,2,2,2,
4),(-0.22769072019282,-0.20856051537961,-0.1894303105664,-0.170609998467856,
-0.151789686369312),.UNSPECIFIED.);
#5947=B_SPLINE_CURVE_WITH_KNOTS('',3,(#233737,#233738,#233739,#233740,#233741,
#233742,#233743,#233744,#233745,#233746),.UNSPECIFIED.,.F.,.F.,(4,2,2,2,
4),(-0.226527604643677,-0.207600143540642,-0.188672682437608,-0.16984222009878,
-0.151011757759953),.UNSPECIFIED.);
#5948=B_SPLINE_CURVE_WITH_KNOTS('',3,(#233836,#233837,#233838,#233839,#233840,
#233841,#233842,#233843,#233844,#233845),.UNSPECIFIED.,.F.,.F.,(4,2,2,2,
4),(-0.150991595557356,-0.132160886570981,-0.113330177584607,-0.0944081585608019,
-0.0754861395369968),.UNSPECIFIED.);
#5949=B_SPLINE_CURVE_WITH_KNOTS('',3,(#234376,#234377,#234378,#234379,#234380,
#234381,#234382,#234383,#234384,#234385),.UNSPECIFIED.,.F.,.F.,(4,2,2,2,
4),(-0.226530961978678,-0.207602903031429,-0.188674844084179,-0.169844408864107,
-0.151013973644034),.UNSPECIFIED.);
#5950=B_SPLINE_CURVE_WITH_KNOTS('',3,(#235141,#235142,#235143,#235144),
 .UNSPECIFIED.,.F.,.F.,(4,4),(0.463715801913011,0.551217064825118),
 .UNSPECIFIED.);
#5951=B_SPLINE_CURVE_WITH_KNOTS('',3,(#235155,#235156,#235157,#235158,#235159,
#235160),.UNSPECIFIED.,.F.,.F.,(4,2,4),(3.73929755316747,4.16560560244743,
4.26808174572346),.UNSPECIFIED.);
#5952=B_SPLINE_CURVE_WITH_KNOTS('',3,(#235166,#235167,#235168,#235169,#235170,
#235171),.UNSPECIFIED.,.F.,.F.,(4,2,4),(0.414971574747897,0.517447718023913,
0.943755767303881),.UNSPECIFIED.);
#5953=B_SPLINE_CURVE_WITH_KNOTS('',3,(#235181,#235182,#235183,#235184),
 .UNSPECIFIED.,.F.,.F.,(4,4),(0.,0.0875012629120985),.UNSPECIFIED.);
#5954=B_SPLINE_CURVE_WITH_KNOTS('',3,(#235191,#235192,#235193,#235194,#235195,
#235196),.UNSPECIFIED.,.F.,.F.,(4,2,4),(0.,0.0957509671557199,0.156185454533133),
 .UNSPECIFIED.);
#5955=B_SPLINE_CURVE_WITH_KNOTS('',3,(#235200,#235201,#235202,#235203),
 .UNSPECIFIED.,.F.,.F.,(4,4),(0.460964693240806,0.551217064825115),
 .UNSPECIFIED.);
#5956=B_SPLINE_CURVE_WITH_KNOTS('',3,(#235223,#235224,#235225,#235226,#235227,
#235228,#235229,#235230,#235231,#235232),.UNSPECIFIED.,.F.,.F.,(4,2,2,2,
4),(0.,0.250000000000004,0.5,0.750000000000003,1.),.UNSPECIFIED.);
#5957=B_SPLINE_CURVE_WITH_KNOTS('',3,(#235286,#235287,#235288,#235289),
 .UNSPECIFIED.,.F.,.F.,(4,4),(0.,0.087501262912106),.UNSPECIFIED.);
#5958=B_SPLINE_CURVE_WITH_KNOTS('',3,(#235299,#235300,#235301,#235302,#235303,
#235304),.UNSPECIFIED.,.F.,.F.,(4,2,4),(0.414971574747878,0.517447718023913,
0.943755767303879),.UNSPECIFIED.);
#5959=B_SPLINE_CURVE_WITH_KNOTS('',3,(#235311,#235312,#235313,#235314,#235315,
#235316),.UNSPECIFIED.,.F.,.F.,(4,2,4),(3.73945461705751,4.16576266633748,
4.2682388096135),.UNSPECIFIED.);
#5960=B_SPLINE_CURVE_WITH_KNOTS('',3,(#235324,#235325,#235326,#235327),
 .UNSPECIFIED.,.F.,.F.,(4,4),(0.463715801913015,0.551217064825115),
 .UNSPECIFIED.);
#5961=B_SPLINE_CURVE_WITH_KNOTS('',3,(#235336,#235337,#235338,#235339,#235340,
#235341),.UNSPECIFIED.,.F.,.F.,(4,2,4),(0.395031610291999,0.455466097669405,
0.551217064825116),.UNSPECIFIED.);
#5962=B_SPLINE_CURVE_WITH_KNOTS('',3,(#235347,#235348,#235349,#235350),
 .UNSPECIFIED.,.F.,.F.,(4,4),(0.,0.0902523715843086),.UNSPECIFIED.);
#5963=B_SPLINE_CURVE_WITH_KNOTS('',3,(#235368,#235369,#235370,#235371,#235372,
#235373,#235374,#235375,#235376,#235377,#235378,#235379,#235380,#235381,
#235382,#235383,#235384,#235385,#235386,#235387,#235388,#235389,#235390,
#235391,#235392,#235393,#235394,#235395,#235396,#235397,#235398,#235399,
#235400,#235401,#235402,#235403,#235404,#235405,#235406,#235407,#235408,
#235409,#235410,#235411,#235412,#235413,#235414,#235415,#235416,#235417,
#235418,#235419,#235420,#235421,#235422,#235423,#235424,#235425,#235426,
#235427,#235428,#235429,#235430,#235431,#235432,#235433,#235434,#235435,
#235436,#235437,#235438,#235439,#235440,#235441,#235442,#235443),
 .UNSPECIFIED.,.F.,.F.,(4,3,3,3,3,3,3,3,3,3,3,3,3,3,3,3,3,3,3,3,3,3,3,3,
3,4),(0.,0.0631673587290824,0.126547835356396,0.189564804454163,0.250000000000068,
0.260069163320057,0.344083184009803,0.375000000000095,0.460278096077198,
0.468750000000068,0.482531787683698,0.496942193289613,0.500000000000047,
0.566043536818633,0.624999999999914,0.692784513998588,0.741244196317371,
0.742187499999759,0.747855634183151,0.749999999999754,0.807209377839192,
0.858244761980869,0.906405690497173,0.953202845248587,0.996323746112527,
1.),.UNSPECIFIED.);
#5964=B_SPLINE_CURVE_WITH_KNOTS('',3,(#235643,#235644,#235645,#235646,#235647,
#235648,#235649,#235650,#235651,#235652,#235653,#235654,#235655,#235656,
#235657,#235658,#235659,#235660,#235661,#235662),.UNSPECIFIED.,.F.,.F.,
(4,2,2,2,2,2,2,2,2,4),(-23.538612912682,-23.492751629174,-23.4452708186545,
-23.3654723554788,-23.2889368147367,-23.2112691912892,-23.1318212040186,
-23.0559652009404,-22.9774384343871,-22.9093233420168),.UNSPECIFIED.);
#5965=B_SPLINE_CURVE_WITH_KNOTS('',3,(#235665,#235666,#235667,#235668,#235669,
#235670,#235671,#235672,#235673,#235674,#235675,#235676,#235677,#235678,
#235679,#235680,#235681,#235682,#235683,#235684,#235685,#235686,#235687,
#235688,#235689,#235690,#235691,#235692),.UNSPECIFIED.,.F.,.F.,(4,2,2,2,
2,2,2,2,2,2,2,2,2,4),(-0.919201423751235,-0.863947826486626,-0.784692530174886,
-0.708354325422247,-0.628658366861542,-0.550251814512154,-0.473954549019739,
-0.393359509391264,-0.315854735569516,-0.238120045391477,-0.158534522064103,
-0.0819365090807384,-0.0416788465054895,-9.999999992516E-7),
 .UNSPECIFIED.);
#5966=B_SPLINE_CURVE_WITH_KNOTS('',3,(#235697,#235698,#235699,#235700,#235701,
#235702,#235703,#235704,#235705,#235706,#235707,#235708,#235709,#235710,
#235711,#235712,#235713,#235714,#235715,#235716,#235717,#235718,#235719,
#235720,#235721,#235722,#235723,#235724,#235725,#235726,#235727,#235728,
#235729,#235730,#235731,#235732),.UNSPECIFIED.,.F.,.F.,(4,2,2,2,2,2,2,2,
2,2,2,2,2,2,2,2,2,4),(-22.9093233420168,-22.8980081380999,-22.8214383480908,
-22.7418667046431,-22.6649521723812,-22.5874864184619,-22.5080154533073,
-22.4321155129901,-22.3537860381917,-22.2735454894312,-22.1971278635793,
-22.1177268304184,-22.0403427308672,-21.9630230720725,-21.883490552651,
-21.8074370746856,-21.729248955998,-21.6498054932123),.UNSPECIFIED.);
#5967=B_SPLINE_CURVE_WITH_KNOTS('',3,(#235733,#235734,#235735,#235736,#235737,
#235738,#235739,#235740,#235741,#235742,#235743,#235744,#235745,#235746,
#235747,#235748,#235749,#235750,#235751,#235752,#235753,#235754,#235755,
#235756,#235757,#235758,#235759,#235760,#235761,#235762,#235763,#235764,
#235765,#235766,#235767,#235768),.UNSPECIFIED.,.F.,.F.,(4,2,2,2,2,2,2,2,
2,2,2,2,2,2,2,2,2,4),(-2.18087056096665,-2.11334107330462,-2.03463289979668,
-1.95862454259661,-1.87902018720997,-1.80117228584085,-1.72452337235938,
-1.64453746915212,-1.56758510758694,-1.48881063002582,-1.4098497250647,
-1.33374220758123,-1.25411458432869,-1.17600877123226,-1.09960383018546,
-1.01933486542919,-0.942126422073293,-0.919201423751235),.UNSPECIFIED.);
#5968=B_SPLINE_CURVE_WITH_KNOTS('',3,(#235773,#235774,#235775,#235776,#235777,
#235778,#235779,#235780,#235781,#235782,#235783,#235784,#235785,#235786,
#235787,#235788,#235789,#235790,#235791,#235792,#235793,#235794,#235795,
#235796,#235797,#235798,#235799,#235800,#235801,#235802,#235803,#235804,
#235805,#235806,#235807,#235808,#235809,#235810),.UNSPECIFIED.,.F.,.F.,
(4,2,2,2,2,2,2,2,2,2,2,2,2,2,2,2,2,2,4),(-21.6498054932123,-21.6497464036347,
-21.5734775119496,-21.4942444230556,-21.4161627634651,-21.3389785571066,
-21.2587331926262,-21.1823927786933,-21.1043114670783,-21.0247306584986,
-20.9486563934726,-20.8697210600931,-20.7910568722386,-20.714132461226,
-20.6341741471182,-20.5576019018695,-20.4797824951719,-20.4002288768587,
-20.3887331680916),.UNSPECIFIED.);
#5969=B_SPLINE_CURVE_WITH_KNOTS('',3,(#235811,#235812,#235813,#235814,#235815,
#235816,#235817,#235818,#235819,#235820,#235821,#235822,#235823,#235824,
#235825,#235826,#235827,#235828,#235829,#235830,#235831,#235832,#235833,
#235834,#235835,#235836,#235837,#235838,#235839,#235840,#235841,#235842,
#235843,#235844,#235845,#235846),.UNSPECIFIED.,.F.,.F.,(4,2,2,2,2,2,2,2,
2,2,2,2,2,2,2,2,2,4),(-3.44277235542014,-3.36378726174833,-3.28543153234955,
-3.20925143282931,-3.1295715636847,-3.05208541691551,-2.97460818332899,
-2.89503370211843,-2.81845045220135,-2.73815053652911,-2.65964627644047,
-2.58360826692366,-2.50398561017137,-2.42634623254457,-2.34933057724823,
-2.26957822067693,-2.19283610748922,-2.18087056096665),.UNSPECIFIED.);
#5970=B_SPLINE_CURVE_WITH_KNOTS('',3,(#235851,#235852,#235853,#235854,#235855,
#235856,#235857,#235858,#235859,#235860,#235861,#235862,#235863,#235864,
#235865,#235866,#235867,#235868,#235869,#235870,#235871,#235872,#235873,
#235874,#235875,#235876,#235877,#235878,#235879,#235880,#235881,#235882,
#235883,#235884,#235885,#235886),.UNSPECIFIED.,.F.,.F.,(4,2,2,2,2,2,2,2,
2,2,2,2,2,2,2,2,2,4),(-20.3887331680916,-20.324265763245,-20.2455870739102,
-20.1662125920531,-20.0895026903313,-20.0097825331845,-19.93285402267,-19.8552477503529,
-19.7756794908763,-19.6996979335461,-19.6212277463401,-19.5410546843959,
-19.464508413356,-19.3849712910484,-19.3075886648593,-19.2301407428766,
-19.150518751006,-19.1278936731383),.UNSPECIFIED.);
#5971=B_SPLINE_CURVE_WITH_KNOTS('',3,(#235887,#235888,#235889,#235890,#235891,
#235892,#235893,#235894,#235895,#235896,#235897,#235898,#235899,#235900,
#235901,#235902,#235903,#235904,#235905,#235906,#235907,#235908,#235909,
#235910,#235911,#235912,#235913,#235914,#235915,#235916,#235917,#235918,
#235919,#235920,#235921,#235922,#235923,#235924),.UNSPECIFIED.,.F.,.F.,
(4,2,2,2,2,2,2,2,2,2,2,2,2,2,2,2,2,2,4),(-4.7060737882392,-4.69519937299706,
-4.61551026078769,-4.53753270632772,-4.46086272369519,-4.380739889656,-4.30365892107839,
-4.22493237909333,-4.14583270082916,-4.06960942142222,-3.9898882750686,
-3.91164341996169,-3.83519103093889,-3.7547756928784,-3.67742986449246,
-3.5992709523531,-3.51986889045247,-3.44343853969079,-3.44277235542014),
 .UNSPECIFIED.);
#5972=B_SPLINE_CURVE_WITH_KNOTS('',3,(#235929,#235930,#235931,#235932,#235933,
#235934,#235935,#235936,#235937,#235938,#235939,#235940,#235941,#235942,
#235943,#235944,#235945,#235946,#235947,#235948,#235949,#235950,#235951,
#235952,#235953,#235954,#235955,#235956,#235957,#235958,#235959,#235960,
#235961,#235962,#235963,#235964),.UNSPECIFIED.,.F.,.F.,(4,2,2,2,2,2,2,2,
2,2,2,2,2,2,2,2,2,4),(-19.1278936731383,-19.0744044534855,-18.996087951931,
-18.9164933593102,-18.8401028125983,-18.7607411272415,-18.6826906925281,
-18.6053864788049,-18.5250128810173,-18.4486382082739,-18.3704354020229,
-18.2907776589607,-18.214602649211,-18.1355462654448,-18.0569413086003,
-17.9799052983999,-17.8998277847766,-17.8656348671598),.UNSPECIFIED.);
#5973=B_SPLINE_CURVE_WITH_KNOTS('',3,(#235965,#235966,#235967,#235968,#235969,
#235970,#235971,#235972,#235973,#235974,#235975,#235976,#235977,#235978,
#235979,#235980,#235981,#235982,#235983,#235984,#235985,#235986,#235987,
#235988,#235989,#235990,#235991,#235992,#235993,#235994,#235995,#235996,
#235997,#235998,#235999,#236000),.UNSPECIFIED.,.F.,.F.,(4,2,2,2,2,2,2,2,
2,2,2,2,2,2,2,2,2,4),(-5.96899237092104,-5.94689777629729,-5.86714879464217,
-5.78955527581653,-5.71209524525375,-5.63240631532895,-5.55571520757411,
-5.47549701610858,-5.39687374256572,-5.3207715990157,-5.2410722589028,-5.16331386417817,
-5.08629968512605,-5.00642109254712,-4.92956024459656,-4.85013448804389,
-4.77129673291419,-4.7060737882392),.UNSPECIFIED.);
#5974=B_SPLINE_CURVE_WITH_KNOTS('',3,(#236005,#236006,#236007,#236008,#236009,
#236010,#236011,#236012,#236013,#236014,#236015,#236016,#236017,#236018,
#236019,#236020,#236021,#236022,#236023,#236024,#236025,#236026,#236027,
#236028,#236029,#236030,#236031,#236032,#236033,#236034,#236035,#236036,
#236037,#236038,#236039,#236040),.UNSPECIFIED.,.F.,.F.,(4,2,2,2,2,2,2,2,
2,2,2,2,2,2,2,2,2,4),(-17.8656348671598,-17.8232472448269,-17.7453153279261,
-17.6656933743908,-17.5896555747679,-17.5108646186686,-17.43157097449,-17.3547589518092,
-17.2749298588699,-17.1980155426997,-17.1203069744517,-17.0406782951708,
-16.9646465413014,-16.886074223839,-16.8059950689099,-16.7293571613581,
-16.6497224659435,-16.6038873599052),.UNSPECIFIED.);
#5975=B_SPLINE_CURVE_WITH_KNOTS('',3,(#236041,#236042,#236043,#236044,#236045,
#236046,#236047,#236048,#236049,#236050,#236051,#236052,#236053,#236054,
#236055,#236056,#236057,#236058,#236059,#236060,#236061,#236062,#236063,
#236064,#236065,#236066,#236067,#236068,#236069,#236070,#236071,#236072,
#236073,#236074,#236075,#236076),.UNSPECIFIED.,.F.,.F.,(4,2,2,2,2,2,2,2,
2,2,2,2,2,2,2,2,2,4),(-7.23318841533112,-7.19957470382814,-7.11935355932711,
-7.0421810608984,-6.96352897163342,-6.88432908237977,-6.80802291954084,
-6.72824482451805,-6.64989908822763,-6.57342887176945,-6.49290657182504,
-6.41546114839076,-6.33734862206539,-6.25783914264643,-6.18130749664818,
-6.10158446177322,-6.02312142516336,-5.96899237092104),.UNSPECIFIED.);
#5976=B_SPLINE_CURVE_WITH_KNOTS('',3,(#236081,#236082,#236083,#236084,#236085,
#236086,#236087,#236088,#236089,#236090,#236091,#236092,#236093,#236094,
#236095,#236096,#236097,#236098,#236099,#236100,#236101,#236102,#236103,
#236104,#236105,#236106,#236107,#236108,#236109,#236110,#236111,#236112,
#236113,#236114,#236115,#236116),.UNSPECIFIED.,.F.,.F.,(4,2,2,2,2,2,2,2,
2,2,2,2,2,2,2,2,2,4),(-16.6038873599052,-16.5723700238927,-16.4948310453186,
-16.4151560532357,-16.3390120605727,-16.2606047195213,-16.1809544208964,
-16.1044785091047,-16.0250259669085,-15.9470346001031,-15.8696467819783,
-15.789182869367,-15.7128037003227,-15.6345161629282,-15.554817361204,-15.4785735840658,
-15.3994333255414,-15.3409628745653),.UNSPECIFIED.);
#5977=B_SPLINE_CURVE_WITH_KNOTS('',3,(#236117,#236118,#236119,#236120,#236121,
#236122,#236123,#236124,#236125,#236126,#236127,#236128,#236129,#236130,
#236131,#236132,#236133,#236134,#236135,#236136,#236137,#236138,#236139,
#236140,#236141,#236142,#236143,#236144,#236145,#236146,#236147,#236148,
#236149,#236150,#236151,#236152),.UNSPECIFIED.,.F.,.F.,(4,2,2,2,2,2,2,2,
2,2,2,2,2,2,2,2,2,4),(-8.49672659742791,-8.45141042511854,-8.37164403540904,
-8.29488064960835,-8.2147729910192,-8.13606764451279,-8.05993239453284,
-7.98019242317436,-7.90235158161355,-7.82536795780181,-7.74540092188602,
-7.66845766152962,-7.58912849400417,-7.51019892410252,-7.43404417168783,
-7.3543066092219,-7.27623678020524,-7.23318841533112),.UNSPECIFIED.);
#5978=B_SPLINE_CURVE_WITH_KNOTS('',3,(#236157,#236158,#236159,#236160,#236161,
#236162,#236163,#236164,#236165,#236166,#236167,#236168,#236169,#236170,
#236171,#236172,#236173,#236174,#236175,#236176,#236177,#236178,#236179,
#236180,#236181,#236182,#236183,#236184,#236185,#236186,#236187,#236188,
#236189,#236190,#236191,#236192),.UNSPECIFIED.,.F.,.F.,(4,2,2,2,2,2,2,2,
2,2,2,2,2,2,2,2,2,4),(-15.3409628745653,-15.3209156696805,-15.2438038964523,
-15.1636444677601,-15.0870850956638,-15.0090768059695,-14.9294222582231,
-14.8533408497659,-14.7744741587621,-14.6952904569345,-14.6184115554974,
-14.5385101569848,-14.4616398790464,-14.3838645152729,-14.3042110278374,
-14.2281598966633,-14.149521329459,-14.0787866057879),.UNSPECIFIED.);
#5979=B_SPLINE_CURVE_WITH_KNOTS('',3,(#236193,#236194,#236195,#236196,#236197,
#236198,#236199,#236200,#236201,#236202,#236203,#236204,#236205,#236206,
#236207,#236208,#236209,#236210,#236211,#236212,#236213,#236214,#236215,
#236216,#236217,#236218,#236219,#236220,#236221,#236222,#236223,#236224,
#236225,#236226,#236227,#236228),.UNSPECIFIED.,.F.,.F.,(4,2,2,2,2,2,2,2,
2,2,2,2,2,2,2,2,2,4),(-9.76130517536905,-9.70340846015941,-9.62414431736556,
-9.54778645507806,-9.46798686882107,-9.38957577756636,-9.31311791274687,
-9.23252523276213,-9.15501539013617,-9.0769787310619,-8.99739820703599,
-8.92080027718151,-8.84104113619735,-8.7625069471703,-8.6862708056307,-8.60648851823689,
-8.52882343306893,-8.49672659742791),.UNSPECIFIED.);
#5980=B_SPLINE_CURVE_WITH_KNOTS('',3,(#236233,#236234,#236235,#236236,#236237,
#236238,#236239,#236240,#236241,#236242,#236243,#236244,#236245,#236246,
#236247,#236248,#236249,#236250,#236251,#236252,#236253,#236254,#236255,
#236256,#236257,#236258,#236259,#236260,#236261,#236262,#236263,#236264,
#236265,#236266,#236267,#236268,#236269,#236270),.UNSPECIFIED.,.F.,.F.,
(4,2,2,2,2,2,2,2,2,2,2,2,2,2,2,2,2,2,4),(-14.0787866057879,-14.0695668038531,
-13.9928719303782,-13.9131756726274,-13.8358841817083,-13.7582890624203,
-13.6785965537892,-13.6024539769723,-13.5239910721253,-13.4443203751484,
-13.3677933054043,-13.2882854129754,-13.2103839518074,-13.129881596516,
-13.0524588825429,-12.9745208657521,-12.8950294193056,-12.8185173950185,
-12.815698709465),.UNSPECIFIED.);
#5981=B_SPLINE_CURVE_WITH_KNOTS('',3,(#236271,#236272,#236273,#236274,#236275,
#236276,#236277,#236278,#236279,#236280,#236281,#236282,#236283,#236284,
#236285,#236286,#236287,#236288,#236289,#236290,#236291,#236292,#236293,
#236294,#236295,#236296,#236297,#236298,#236299,#236300,#236301,#236302,
#236303,#236304,#236305,#236306),.UNSPECIFIED.,.F.,.F.,(4,2,2,2,2,2,2,2,
2,2,2,2,2,2,2,2,2,4),(-11.0249860124619,-10.9547951692771,-10.8760427721033,
-10.7999052685861,-10.7201601701575,-10.6422715072435,-10.56534947872,-10.4853296583778,
-10.4083383410507,-10.3291372920938,-10.2501513951993,-10.1739699629713,
-10.0942194333807,-10.0160924019212,-9.93946853215564,-9.85918519782063,
-9.78195594007543,-9.76130517536905),.UNSPECIFIED.);
#5982=B_SPLINE_CURVE_WITH_KNOTS('',3,(#236311,#236312,#236313,#236314,#236315,
#236316,#236317,#236318,#236319,#236320,#236321,#236322,#236323,#236324,
#236325,#236326,#236327,#236328,#236329,#236330,#236331,#236332,#236333,
#236334,#236335,#236336,#236337,#236338,#236339,#236340,#236341,#236342,
#236343,#236344,#236345,#236346),.UNSPECIFIED.,.F.,.F.,(4,2,2,2,2,2,2,2,
2,2,2,2,2,2,2,2,2,4),(-12.815698709465,-12.7388502838186,-12.6604039289512,
-12.5842573753116,-12.5045673723298,-12.426989055931,-12.3496716860682,
-12.2699941073719,-12.1933163681172,-12.1133125021989,-12.0346943554925,
-11.958646940508,-11.8789986323752,-11.8012439329055,-11.7243541098449,
-11.6444752807082,-11.5676171032067,-11.5534578894946),.UNSPECIFIED.);
#5983=B_SPLINE_CURVE_WITH_KNOTS('',3,(#236347,#236348,#236349,#236350,#236351,
#236352,#236353,#236354,#236355,#236356,#236357,#236358,#236359,#236360,
#236361,#236362,#236363,#236364,#236365,#236366,#236367,#236368,#236369,
#236370,#236371,#236372,#236373,#236374,#236375,#236376,#236377,#236378,
#236379,#236380,#236381,#236382,#236383,#236384),.UNSPECIFIED.,.F.,.F.,
(4,2,2,2,2,2,2,2,2,2,2,2,2,2,2,2,2,2,4),(-12.2894458654892,-12.2877187485206,
-12.2079332513791,-12.1294910114847,-12.053076894753,-11.9724489486166,
-11.8949085570648,-11.816980570571,-11.7373638662537,-11.6607332796557,
-11.5809733408869,-11.5024026205688,-11.4261854709585,-11.3464053946431,
-11.2687029874123,-11.1913692300601,-11.1115606273989,-11.0347589397308,
-11.0249860124619),.UNSPECIFIED.);
#5984=B_SPLINE_CURVE_WITH_KNOTS('',3,(#236389,#236390,#236391,#236392,#236393,
#236394,#236395,#236396,#236397,#236398,#236399,#236400,#236401,#236402,
#236403,#236404,#236405,#236406,#236407,#236408,#236409,#236410,#236411,
#236412,#236413,#236414,#236415,#236416,#236417,#236418,#236419,#236420,
#236421,#236422,#236423,#236424),.UNSPECIFIED.,.F.,.F.,(4,2,2,2,2,2,2,2,
2,2,2,2,2,2,2,2,2,4),(-11.5534578894946,-11.4883896521,-11.4095468044081,
-11.3334780090213,-11.2538314964982,-11.1758473301944,-11.09927687961,-11.0191434895105,
-10.9420556489546,-10.8635026982174,-10.7843892130607,-10.7081672155377,
-10.6284795542192,-10.5502191518199,-10.47383832356,-10.3934034755595,-10.3160424178526,
-10.2909000381992),.UNSPECIFIED.);
#5985=B_SPLINE_CURVE_WITH_KNOTS('',3,(#236425,#236426,#236427,#236428,#236429,
#236430,#236431,#236432,#236433,#236434,#236435,#236436,#236437,#236438,
#236439,#236440,#236441,#236442,#236443,#236444,#236445,#236446,#236447,
#236448,#236449,#236450,#236451,#236452,#236453,#236454,#236455,#236456,
#236457,#236458,#236459,#236460),.UNSPECIFIED.,.F.,.F.,(4,2,2,2,2,2,2,2,
2,2,2,2,2,2,2,2,2,4),(-13.5529028614626,-13.5366310611161,-13.4596134279343,
-13.3795630232731,-13.3027330821113,-13.2248185416059,-13.1450960915604,
-13.0689795559661,-12.9899718253951,-12.9137942828532,-12.8340666894434,
-12.7559164845886,-12.6793631199568,-12.599052526635,-12.5218002367153,
-12.4433917233644,-12.3640980140278,-12.2894458654892),.UNSPECIFIED.);
#5986=B_SPLINE_CURVE_WITH_KNOTS('',3,(#236465,#236466,#236467,#236468,#236469,
#236470,#236471,#236472,#236473,#236474,#236475,#236476,#236477,#236478,
#236479,#236480,#236481,#236482,#236483,#236484,#236485,#236486,#236487,
#236488,#236489,#236490,#236491,#236492,#236493,#236494,#236495,#236496,
#236497,#236498,#236499,#236500),.UNSPECIFIED.,.F.,.F.,(4,2,2,2,2,2,2,2,
2,2,2,2,2,2,2,2,2,4),(-10.2909000381992,-10.2380261799054,-10.1586029228117,
-10.082154433658,-10.0025206211922,-9.92414258171931,-9.84800606350118,
-9.76834654803807,-9.69083698889078,-9.61347022104288,-9.53386720169178,
-9.45725895014511,-9.37714223779883,-9.29860326982443,-9.22258650707221,
-9.14297599529373,-9.06530087798291,-9.02890583393059),.UNSPECIFIED.);
#5987=B_SPLINE_CURVE_WITH_KNOTS('',3,(#236501,#236502,#236503,#236504,#236505,
#236506,#236507,#236508,#236509,#236510,#236511,#236512,#236513,#236514,
#236515,#236516,#236517,#236518,#236519,#236520,#236521,#236522,#236523,
#236524,#236525,#236526,#236527,#236528,#236529,#236530,#236531,#236532,
#236533,#236534,#236535,#236536),.UNSPECIFIED.,.F.,.F.,(4,2,2,2,2,2,2,2,
2,2,2,2,2,2,2,2,2,4),(-14.8171068447876,-14.7898947256491,-14.7123410728569,
-14.6316990445303,-14.5552778459057,-14.4768221679673,-14.3970268053498,
-14.3206350511274,-14.2413279210765,-14.1629199795842,-14.0856550865695,
-14.0053311123276,-13.9287728850427,-13.8506099370316,-13.7708732308644,
-13.6946853232978,-13.6156648455926,-13.5529028614626),.UNSPECIFIED.);
#5988=B_SPLINE_CURVE_WITH_KNOTS('',3,(#236541,#236542,#236543,#236544,#236545,
#236546,#236547,#236548,#236549,#236550,#236551,#236552,#236553,#236554,
#236555,#236556,#236557,#236558,#236559,#236560,#236561,#236562,#236563,
#236564,#236565,#236566,#236567,#236568,#236569,#236570,#236571,#236572,
#236573,#236574,#236575,#236576),.UNSPECIFIED.,.F.,.F.,(4,2,2,2,2,2,2,2,
2,2,2,2,2,2,2,2,2,4),(-9.02890583393059,-8.98837818038564,-8.9085848357724,
-8.83180622648821,-8.75247998524822,-8.67372599849014,-8.5977120980958,
-8.51811118370627,-8.44021636866933,-8.36363570047745,-8.28359760205359,
-8.20659839258143,-8.12796884716024,-8.04895256139842,-7.97281085546684,
-7.89317727237044,-7.81501477128926,-7.76734335477425),.UNSPECIFIED.);
#5989=B_SPLINE_CURVE_WITH_KNOTS('',3,(#236577,#236578,#236579,#236580,#236581,
#236582,#236583,#236584,#236585,#236586,#236587,#236588,#236589,#236590,
#236591,#236592,#236593,#236594,#236595,#236596,#236597,#236598,#236599,
#236600,#236601,#236602,#236603,#236604,#236605,#236606,#236607,#236608,
#236609,#236610,#236611,#236612),.UNSPECIFIED.,.F.,.F.,(4,2,2,2,2,2,2,2,
2,2,2,2,2,2,2,2,2,4),(-16.0812642602168,-16.0427033691111,-15.9648000015417,
-15.8850434578948,-15.8088951087731,-15.7301279517022,-15.6501648691772,
-15.5733494034149,-15.4935262820714,-15.4161882581257,-15.3384720230956,
-15.2586811009834,-15.1824548683918,-15.1038702650408,-15.0240992276322,
-14.9474553393011,-14.8678246263304,-14.8171068447876),.UNSPECIFIED.);
#5990=B_SPLINE_CURVE_WITH_KNOTS('',3,(#236617,#236618,#236619,#236620,#236621,
#236622,#236623,#236624,#236625,#236626,#236627,#236628,#236629,#236630,
#236631,#236632,#236633,#236634,#236635,#236636,#236637,#236638,#236639,
#236640,#236641,#236642,#236643,#236644,#236645,#236646,#236647,#236648,
#236649,#236650,#236651,#236652),.UNSPECIFIED.,.F.,.F.,(4,2,2,2,2,2,2,2,
2,2,2,2,2,2,2,2,2,4),(-7.76734335477425,-7.73864941116114,-7.65831844901966,
-7.58105403612982,-7.50298926113532,-7.42367035955319,-7.34732022310147,
-7.26775524759053,-7.18948146926026,-7.11338601140779,-7.0337926806513,
-6.95638747398355,-6.87900125726489,-6.79950955808733,-6.7230061602176,
-6.64280571406996,-6.56438262228941,-6.50606900159132),.UNSPECIFIED.);
#5991=B_SPLINE_CURVE_WITH_KNOTS('',3,(#236653,#236654,#236655,#236656,#236657,
#236658,#236659,#236660,#236661,#236662,#236663,#236664,#236665,#236666,
#236667,#236668,#236669,#236670,#236671,#236672,#236673,#236674,#236675,
#236676,#236677,#236678,#236679,#236680,#236681,#236682,#236683,#236684,
#236685,#236686,#236687,#236688),.UNSPECIFIED.,.F.,.F.,(4,2,2,2,2,2,2,2,
2,2,2,2,2,2,2,2,2,4),(-17.3455030680058,-17.2955931490807,-17.2171658662611,
-17.137353476371,-17.060980682749,-16.9817003234495,-16.9031503849096,-16.8259057966854,
-16.7456062623404,-16.6689747781945,-16.5908322516153,-16.5110696292502,
-16.4348753299627,-16.3558738930773,-16.2766722752647,-16.1996663634789,
-16.1196311389729,-16.0812642602168),.UNSPECIFIED.);
#5992=B_SPLINE_CURVE_WITH_KNOTS('',3,(#236693,#236694,#236695,#236696,#236697,
#236698,#236699,#236700,#236701,#236702,#236703,#236704,#236705,#236706,
#236707,#236708,#236709,#236710,#236711,#236712,#236713,#236714,#236715,
#236716,#236717,#236718,#236719,#236720,#236721,#236722,#236723,#236724,
#236725,#236726,#236727,#236728),.UNSPECIFIED.,.F.,.F.,(4,2,2,2,2,2,2,2,
2,2,2,2,2,2,2,2,2,4),(-6.50606900159132,-6.48842746165265,-6.40889066737013,
-6.33133145822056,-6.25440506460236,-6.17473473444485,-6.09807176978359,
-6.01867433671648,-5.94004670161983,-5.86411917020774,-5.78460000677712,
-5.70683164491114,-5.6302697856161,-5.55036530368567,-5.47349152610902,
-5.39481215007952,-5.31593132099885,-5.24598146676954),.UNSPECIFIED.);
#5993=B_SPLINE_CURVE_WITH_KNOTS('',3,(#236729,#236730,#236731,#236732,#236733,
#236734,#236735,#236736,#236737,#236738,#236739,#236740,#236741,#236742,
#236743,#236744,#236745,#236746,#236747,#236748,#236749,#236750,#236751,
#236752,#236753,#236754,#236755,#236756,#236757,#236758,#236759,#236760,
#236761,#236762,#236763,#236764),.UNSPECIFIED.,.F.,.F.,(4,2,2,2,2,2,2,2,
2,2,2,2,2,2,2,2,2,4),(-18.6099778127053,-18.5493148479147,-18.4705919470025,
-18.390482017717,-18.3137021311011,-18.2339184021079,-18.1564983637494,
-18.0788167044097,-17.999020658113,-17.9227728263697,-17.8442219756113,
-17.7644488433926,-17.6878349083277,-17.6082375764479,-17.5301961468915,
-17.4526703162838,-17.3720607330546,-17.3455030680058),.UNSPECIFIED.);
#5994=B_SPLINE_CURVE_WITH_KNOTS('',3,(#236769,#236770,#236771,#236772,#236773,
#236774,#236775,#236776,#236777,#236778,#236779,#236780,#236781,#236782,
#236783,#236784,#236785,#236786,#236787,#236788,#236789,#236790,#236791,
#236792,#236793,#236794,#236795,#236796,#236797,#236798,#236799,#236800,
#236801,#236802,#236803,#236804,#236805,#236806),.UNSPECIFIED.,.F.,.F.,
(4,2,2,2,2,2,2,2,2,2,2,2,2,2,2,2,2,2,4),(-5.24598146676954,-5.23990258087749,
-5.16035947250977,-5.08233272728431,-5.00601244460324,-4.92582445436964,
-4.84869417225652,-4.77060768728586,-4.69143207223894,-4.61517073377482,
-4.53555851063403,-4.45723061749692,-4.38101556066038,-4.30132492142305,
-4.22386755581104,-4.14629439014171,-4.06675367644276,-3.99020072545403,
-3.98436239557673),.UNSPECIFIED.);
#5995=B_SPLINE_CURVE_WITH_KNOTS('',3,(#236807,#236808,#236809,#236810,#236811,
#236812,#236813,#236814,#236815,#236816,#236817,#236818,#236819,#236820,
#236821,#236822,#236823,#236824,#236825,#236826,#236827,#236828,#236829,
#236830,#236831,#236832,#236833,#236834,#236835,#236836,#236837,#236838,
#236839,#236840,#236841,#236842),.UNSPECIFIED.,.F.,.F.,(4,2,2,2,2,2,2,2,
2,2,2,2,2,2,2,2,2,4),(-19.8737805950392,-19.8012842880796,-19.7220653407672,
-19.6434081509384,-19.5662175651196,-19.4859773616869,-19.4093051239936,
-19.3312170184939,-19.2514644782548,-19.175294381749,-19.0963464545443,
-19.0170139310546,-18.9400533385336,-18.8600680614421,-18.7830760907932,
-18.7052177840403,-18.6254634676243,-18.6099778127053),.UNSPECIFIED.);
#5996=B_SPLINE_CURVE_WITH_KNOTS('',3,(#236847,#236848,#236849,#236850,#236851,
#236852,#236853,#236854,#236855,#236856,#236857,#236858,#236859,#236860,
#236861,#236862,#236863,#236864,#236865,#236866,#236867,#236868,#236869,
#236870,#236871,#236872,#236873,#236874,#236875,#236876,#236877,#236878,
#236879,#236880,#236881,#236882),.UNSPECIFIED.,.F.,.F.,(4,2,2,2,2,2,2,2,
2,2,2,2,2,2,2,2,2,4),(-3.98436239557673,-3.91058816835304,-3.8320914425044,
-3.75604716698683,-3.67642092649783,-3.5987893352205,-3.52175035472291,
-3.44200702890818,-3.36527291528161,-3.28573643693738,-3.20703850423459,
-3.13103018768841,-3.05142431534688,-2.97358691830964,-2.89692041149797,
-2.81694626637145,-2.74000442254937,-2.72287955455984),.UNSPECIFIED.);
#5997=B_SPLINE_CURVE_WITH_KNOTS('',3,(#236883,#236884,#236885,#236886,#236887,
#236888,#236889,#236890,#236891,#236892,#236893,#236894,#236895,#236896,
#236897,#236898,#236899,#236900,#236901,#236902,#236903,#236904,#236905,
#236906,#236907,#236908,#236909,#236910,#236911,#236912,#236913,#236914,
#236915,#236916,#236917,#236918,#236919,#236920),.UNSPECIFIED.,.F.,.F.,
(4,2,2,2,2,2,2,2,2,2,2,2,2,2,2,2,2,2,4),(-21.1380887072673,-21.1301824628563,
-21.0534720598587,-20.973762889165,-20.8962932999746,-20.8186803921204,
-20.7389147745979,-20.6626769042768,-20.5841943615403,-20.5044544735613,
-20.427904062833,-20.348374912106,-20.2702550696609,-20.1927908814288,-20.1122487957223,
-20.0357663606382,-19.9574016283348,-19.8776078608383,-19.8737805950392),
 .UNSPECIFIED.);
#5998=B_SPLINE_CURVE_WITH_KNOTS('',3,(#236925,#236926,#236927,#236928,#236929,
#236930,#236931,#236932,#236933,#236934,#236935,#236936,#236937,#236938,
#236939,#236940,#236941,#236942,#236943,#236944,#236945,#236946,#236947,
#236948,#236949,#236950,#236951,#236952,#236953,#236954,#236955,#236956,
#236957,#236958,#236959,#236960),.UNSPECIFIED.,.F.,.F.,(4,2,2,2,2,2,2,2,
2,2,2,2,2,2,2,2,2,4),(-2.72287955455984,-2.6611939409923,-2.58224561704119,
-2.50614498809059,-2.42651807456794,-2.34842515143559,-2.27200938659411,
-2.19175457142759,-2.11455886794221,-2.03635146652478,-1.95711065417433,
-1.88078587379711,-1.80109296697817,-1.7227012773198,-1.64640027132008,
-1.56582136420733,-1.48833119993793,-1.4603242851032),.UNSPECIFIED.);
#5999=B_SPLINE_CURVE_WITH_KNOTS('',3,(#236961,#236962,#236963,#236964,#236965,
#236966,#236967,#236968,#236969,#236970,#236971,#236972,#236973,#236974,
#236975,#236976,#236977,#236978,#236979,#236980,#236981,#236982,#236983,
#236984,#236985,#236986,#236987,#236988,#236989,#236990,#236991,#236992,
#236993,#236994,#236995,#236996),.UNSPECIFIED.,.F.,.F.,(4,2,2,2,2,2,2,2,
2,2,2,2,2,2,2,2,2,4),(-22.4011363767123,-22.3825091502153,-22.3054072138646,
-22.2252623253679,-22.1485797733878,-22.0705810376521,-21.9908740563847,
-21.9147588411359,-21.8358997915956,-21.7564682633744,-21.6795872469303,
-21.5996874662663,-21.522662492958,-21.4448837755089,-21.3651672061648,
-21.2890491931534,-21.2104054765067,-21.1380887072673),.UNSPECIFIED.);
#6000=B_SPLINE_CURVE_WITH_KNOTS('',3,(#237002,#237003,#237004,#237005,#237006,
#237007,#237008,#237009),.UNSPECIFIED.,.F.,.F.,(4,2,2,4),(-0.790626080807867,
-0.749696276559816,-0.708676254523423,-0.640412608621221),.UNSPECIFIED.);
#6001=B_SPLINE_CURVE_WITH_KNOTS('',3,(#237011,#237012,#237013,#237014,#237015,
#237016),.UNSPECIFIED.,.F.,.F.,(4,2,4),(0.,0.0243519941209903,0.0487062313865143),
 .UNSPECIFIED.);
#6002=B_SPLINE_CURVE_WITH_KNOTS('',3,(#237017,#237018,#237019,#237020,#237021,
#237022,#237023,#237024),.UNSPECIFIED.,.F.,.F.,(4,2,2,4),(-0.197604024225048,
-0.160169062454954,-0.0801828347949093,-1.0183968231669E-6),
 .UNSPECIFIED.);
#6003=B_SPLINE_CURVE_WITH_KNOTS('',3,(#237030,#237031,#237032,#237033,#237034,
#237035,#237036,#237037,#237038,#237039,#237040,#237041),.UNSPECIFIED.,
 .F.,.F.,(4,2,2,2,2,4),(-23.5722065003637,-23.497693055354,-23.4210054488723,
-23.342379146909,-23.2652626317729,-23.2565691746208),.UNSPECIFIED.);
#6004=B_SPLINE_CURVE_WITH_KNOTS('',3,(#237044,#237045,#237046,#237047,#237048,
#237049,#237050,#237051,#237052,#237053,#237054,#237055,#237056,#237057,
#237058,#237059,#237060,#237061),.UNSPECIFIED.,.F.,.F.,(4,2,2,2,2,2,2,2,
4),(-0.602752842964723,-0.541077168469372,-0.464578035407547,-0.384478668278887,
-0.307424763205198,-0.228970812045174,-0.149889767174645,-0.0750970133704404,
-9.99999999695689E-7),.UNSPECIFIED.);
#6005=B_SPLINE_CURVE_WITH_KNOTS('',3,(#237066,#237067,#237068,#237069,#237070,
#237071,#237072,#237073,#237074,#237075,#237076,#237077,#237078,#237079,
#237080,#237081,#237082,#237083,#237084,#237085,#237086,#237087,#237088,
#237089,#237090,#237091,#237092,#237093,#237094,#237095,#237096,#237097,
#237098,#237099,#237100,#237101),.UNSPECIFIED.,.F.,.F.,(4,2,2,2,2,2,2,2,
2,2,2,2,2,2,2,2,2,4),(-23.2565691746208,-23.1851002816822,-23.1084754817438,
-23.0304622347963,-22.9507738401723,-22.8746683922162,-22.7957957470848,
-22.7164884410324,-22.6395993516767,-22.5596891465343,-22.4827386348412,
-22.4049524313817,-22.3252601513637,-22.2491695959833,-22.1705192500891,
-22.090431095132,-22.0137198994339,-21.993829988038),.UNSPECIFIED.);
#6006=B_SPLINE_CURVE_WITH_KNOTS('',3,(#237102,#237103,#237104,#237105,#237106,
#237107,#237108,#237109,#237110,#237111,#237112,#237113,#237114,#237115,
#237116,#237117,#237118,#237119,#237120,#237121,#237122,#237123,#237124,
#237125,#237126,#237127,#237128,#237129,#237130,#237131,#237132,#237133,
#237134,#237135,#237136,#237137),.UNSPECIFIED.,.F.,.F.,(4,2,2,2,2,2,2,2,
2,2,2,2,2,2,2,2,2,4),(-1.86395731614265,-1.79131469143525,-1.71408508177727,
-1.63444898401876,-1.55781207307748,-1.47792338108508,-1.39934401643668,
-1.32335141532464,-1.24375914507094,-1.16604229617437,-1.08923305708754,
-1.00939166539875,-0.932570581095492,-0.853451657054535,-0.774644071183091,
-0.698620497957606,-0.619026937738768,-0.602752842964723),.UNSPECIFIED.);
#6007=B_SPLINE_CURVE_WITH_KNOTS('',3,(#237142,#237143,#237144,#237145,#237146,
#237147,#237148,#237149,#237150,#237151,#237152,#237153,#237154,#237155,
#237156,#237157,#237158,#237159,#237160,#237161,#237162,#237163,#237164,
#237165,#237166,#237167,#237168,#237169,#237170,#237171,#237172,#237173,
#237174,#237175,#237176,#237177),.UNSPECIFIED.,.F.,.F.,(4,2,2,2,2,2,2,2,
2,2,2,2,2,2,2,2,2,4),(-21.993829988038,-21.9340081905832,-21.8566253226136,
-21.7790127559565,-21.6992767985655,-21.6230814628004,-21.5446001511914,
-21.4648878735189,-21.3883409400274,-21.308813815213,-21.2308021377538,
-21.1533434094453,-21.0728045264707,-20.9963828996738,-20.9180235568831,
-20.8382680744993,-20.7619585762964,-20.7299620242508),.UNSPECIFIED.);
#6008=B_SPLINE_CURVE_WITH_KNOTS('',3,(#237178,#237179,#237180,#237181,#237182,
#237183,#237184,#237185,#237186,#237187,#237188,#237189,#237190,#237191,
#237192,#237193,#237194,#237195,#237196,#237197,#237198,#237199,#237200,
#237201,#237202,#237203,#237204,#237205,#237206,#237207,#237208,#237209,
#237210,#237211,#237212,#237213,#237214,#237215),.UNSPECIFIED.,.F.,.F.,
(4,2,2,2,2,2,2,2,2,2,2,2,2,2,2,2,2,2,4),(-3.12604785474054,-3.11916406014114,
-3.04206941199171,-2.96373543201984,-2.88460664086586,-2.80838290395217,
-2.72874018594438,-2.65046210727937,-2.57416915143261,-2.49371165741852,
-2.41633340568906,-2.33849516052129,-2.25904746070068,-2.18257839052104,
-2.10296905145572,-2.02456552352352,-1.94848217127368,-1.86885112563732,
-1.86395731614265),.UNSPECIFIED.);
#6009=B_SPLINE_CURVE_WITH_KNOTS('',3,(#237220,#237221,#237222,#237223,#237224,
#237225,#237226,#237227,#237228,#237229,#237230,#237231,#237232,#237233,
#237234,#237235,#237236,#237237,#237238,#237239,#237240,#237241,#237242,
#237243,#237244,#237245,#237246,#237247,#237248,#237249,#237250,#237251,
#237252,#237253,#237254,#237255),.UNSPECIFIED.,.F.,.F.,(4,2,2,2,2,2,2,2,
2,2,2,2,2,2,2,2,2,4),(-20.7299620242508,-20.6827463946196,-20.6042186226985,
-20.5270388935432,-20.4468076578971,-20.3702151620859,-20.2921382009833,
-20.2124301153876,-20.1362922046833,-20.0573566378915,-19.9781710469159,
-19.9012274967379,-19.8212578690367,-19.7443628476554,-19.6665223661209,
-19.5868182062698,-19.5107195193131,-19.4668934640671),.UNSPECIFIED.);
#6010=B_SPLINE_CURVE_WITH_KNOTS('',3,(#237256,#237257,#237258,#237259,#237260,
#237261,#237262,#237263,#237264,#237265,#237266,#237267,#237268,#237269,
#237270,#237271,#237272,#237273,#237274,#237275,#237276,#237277,#237278,
#237279,#237280,#237281,#237282,#237283,#237284,#237285,#237286,#237287,
#237288,#237289,#237290,#237291),.UNSPECIFIED.,.F.,.F.,(4,2,2,2,2,2,2,2,
2,2,2,2,2,2,2,2,2,4),(-4.38713111494036,-4.36896197353506,-4.2923027086423,
-4.21257525484536,-4.13396520723424,-4.05798513071122,-3.97840472490161,
-3.90065622254177,-3.82392384525069,-3.74404628396318,-3.66719317659379,
-3.58821871314422,-3.50937129947931,-3.43333555020512,-3.35374592435993,
-3.27575513813943,-3.19930900911089,-3.12604785474054),.UNSPECIFIED.);
#6011=B_SPLINE_CURVE_WITH_KNOTS('',3,(#237296,#237297,#237298,#237299,#237300,
#237301,#237302,#237303,#237304,#237305,#237306,#237307,#237308,#237309,
#237310,#237311,#237312,#237313,#237314,#237315,#237316,#237317,#237318,
#237319,#237320,#237321,#237322,#237323,#237324,#237325,#237326,#237327,
#237328,#237329,#237330,#237331),.UNSPECIFIED.,.F.,.F.,(4,2,2,2,2,2,2,2,
2,2,2,2,2,2,2,2,2,4),(-19.4668934640671,-19.4320155876266,-19.3520645278124,
-19.2753086679126,-19.1955481533192,-19.1182381534648,-19.0405818480038,
-18.9608413232741,-18.8846589211247,-18.8061345868867,-18.7264147794134,
-18.6498288754341,-18.5702590313714,-18.4923494476519,-18.4148538038223,
-18.3342730653254,-18.2578890735217,-18.2031408914352),.UNSPECIFIED.);
#6012=B_SPLINE_CURVE_WITH_KNOTS('',3,(#237332,#237333,#237334,#237335,#237336,
#237337,#237338,#237339,#237340,#237341,#237342,#237343,#237344,#237345,
#237346,#237347,#237348,#237349,#237350,#237351,#237352,#237353,#237354,
#237355,#237356,#237357,#237358,#237359,#237360,#237361,#237362,#237363,
#237364,#237365,#237366,#237367),.UNSPECIFIED.,.F.,.F.,(4,2,2,2,2,2,2,2,
2,2,2,2,2,2,2,2,2,4),(-5.64892676185118,-5.6188978192691,-5.54266696049746,
-5.46305555514589,-5.38476245669672,-5.30852869070133,-5.22805245343415,
-5.15065962464527,-5.07294679429705,-4.99347930984184,-4.91699341878228,
-4.83740023522811,-4.75897645240369,-4.68292735856954,-4.60331559595368,
-4.52575792609574,-4.44862376378175,-4.38713111494036),.UNSPECIFIED.);
#6013=B_SPLINE_CURVE_WITH_KNOTS('',3,(#237372,#237373,#237374,#237375,#237376,
#237377,#237378,#237379,#237380,#237381,#237382,#237383,#237384,#237385,
#237386,#237387,#237388,#237389,#237390,#237391,#237392,#237393,#237394,
#237395,#237396,#237397,#237398,#237399,#237400,#237401,#237402,#237403,
#237404,#237405,#237406,#237407),.UNSPECIFIED.,.F.,.F.,(4,2,2,2,2,2,2,2,
2,2,2,2,2,2,2,2,2,4),(-18.2031408914352,-18.179492152848,-18.0997439313982,
-18.0234073251507,-17.9441590506585,-17.8657632814858,-17.7885541573198,
-17.7082890833817,-17.631760730409,-17.5536541757552,-17.4739621076796,
-17.3978222587249,-17.3188583449362,-17.2398298963329,-17.1628655277294,
-17.0828713188359,-17.0060645825577,-16.9401280371148),.UNSPECIFIED.);
#6014=B_SPLINE_CURVE_WITH_KNOTS('',3,(#237408,#237409,#237410,#237411,#237412,
#237413,#237414,#237415,#237416,#237417,#237418,#237419,#237420,#237421,
#237422,#237423,#237424,#237425,#237426,#237427,#237428,#237429,#237430,
#237431,#237432,#237433,#237434,#237435,#237436,#237437,#237438,#237439,
#237440,#237441,#237442,#237443),.UNSPECIFIED.,.F.,.F.,(4,2,2,2,2,2,2,2,
2,2,2,2,2,2,2,2,2,4),(-6.90946184483317,-6.86760642961369,-6.7916708400602,
-6.7121392179253,-6.63439293140309,-6.55777252826709,-6.47789349608262,
-6.40104193860036,-6.32225111214459,-6.24339822683304,-6.16738099587715,
-6.08783178147495,-6.00983394361517,-5.93347443663795,-5.85331874214117,
-5.77621703982064,-5.69803979876399,-5.64892676185118),.UNSPECIFIED.);
#6015=B_SPLINE_CURVE_WITH_KNOTS('',3,(#237448,#237449,#237450,#237451,#237452,
#237453,#237454,#237455,#237456,#237457,#237458,#237459,#237460,#237461,
#237462,#237463,#237464,#237465,#237466,#237467,#237468,#237469,#237470,
#237471,#237472,#237473,#237474,#237475,#237476,#237477,#237478,#237479,
#237480,#237481,#237482,#237483),.UNSPECIFIED.,.F.,.F.,(4,2,2,2,2,2,2,2,
2,2,2,2,2,2,2,2,2,4),(-16.9401280371148,-16.9282037503213,-16.8485236627961,
-16.7724481057347,-16.6937249444493,-16.6139486511616,-16.537181650428,
-16.4574070398215,-16.3802047121582,-16.3025384902836,-16.222829570132,
-16.1466925369983,-16.0681594104423,-15.9884679751763,-15.9118764226213,
-15.8322983428692,-15.7545270051868,-15.6771758708029),.UNSPECIFIED.);
#6016=B_SPLINE_CURVE_WITH_KNOTS('',3,(#237484,#237485,#237486,#237487,#237488,
#237489,#237490,#237491,#237492,#237493,#237494,#237495,#237496,#237497,
#237498,#237499,#237500,#237501,#237502,#237503,#237504,#237505,#237506,
#237507,#237508,#237509,#237510,#237511,#237512,#237513,#237514,#237515,
#237516,#237517,#237518,#237519),.UNSPECIFIED.,.F.,.F.,(4,2,2,2,2,2,2,2,
2,2,2,2,2,2,2,2,2,4),(-8.17021312579191,-8.11747034451843,-8.04133415108175,
-7.96171687108957,-7.88431742195717,-7.80684514073046,-7.72736245062139,
-7.65086608992251,-7.5705299105957,-7.49212030099125,-7.41613911530324,
-7.33658395835915,-7.25903903962238,-7.18203779924169,-7.10238510837754,
-7.02573715227108,-6.94621282645275,-6.90946184483317),.UNSPECIFIED.);
#6017=B_SPLINE_CURVE_WITH_KNOTS('',3,(#237524,#237525,#237526,#237527,#237528,
#237529,#237530,#237531,#237532,#237533,#237534,#237535,#237536,#237537,
#237538,#237539,#237540,#237541,#237542,#237543,#237544,#237545,#237546,
#237547,#237548,#237549,#237550,#237551,#237552,#237553,#237554,#237555,
#237556,#237557,#237558,#237559,#237560,#237561),.UNSPECIFIED.,.F.,.F.,
(4,2,2,2,2,2,2,2,2,2,2,2,2,2,2,2,2,2,4),(-15.6771758708029,-15.6770280684428,
-15.5964402318874,-15.5201268390809,-15.4417262916037,-15.3620219047567,
-15.2856882575655,-15.2064383814064,-15.1282131561966,-15.0510083229075,
-14.9707442012106,-14.8943145632693,-14.81621240392,-14.7365735239284,-14.6604627016941,
-14.5815049486408,-14.5026750732159,-14.4257236808457,-14.4146492123929),
 .UNSPECIFIED.);
#6018=B_SPLINE_CURVE_WITH_KNOTS('',3,(#237562,#237563,#237564,#237565,#237566,
#237567,#237568,#237569,#237570,#237571,#237572,#237573,#237574,#237575,
#237576,#237577,#237578,#237579,#237580,#237581,#237582,#237583,#237584,
#237585,#237586,#237587,#237588,#237589,#237590,#237591,#237592,#237593,
#237594,#237595,#237596,#237597),.UNSPECIFIED.,.F.,.F.,(4,2,2,2,2,2,2,2,
2,2,2,2,2,2,2,2,2,4),(-9.42971000722909,-9.3658882895704,-9.28942247658091,
-9.20958233406318,-9.1327714201309,-9.05421232368468,-8.97539387085022,
-8.8994311344934,-8.81996532926532,-8.74199974137761,-8.66576704950347,
-8.58564082857867,-8.50857101307976,-8.43059536142831,-8.35148004581058,
-8.27527702862697,-8.19573923437247,-8.17021312579191),.UNSPECIFIED.);
#6019=B_SPLINE_CURVE_WITH_KNOTS('',3,(#237602,#237603,#237604,#237605,#237606,
#237607,#237608,#237609,#237610,#237611,#237612,#237613,#237614,#237615,
#237616,#237617,#237618,#237619,#237620,#237621,#237622,#237623,#237624,
#237625,#237626,#237627,#237628,#237629,#237630,#237631,#237632,#237633,
#237634,#237635,#237636,#237637),.UNSPECIFIED.,.F.,.F.,(4,2,2,2,2,2,2,2,
2,2,2,2,2,2,2,2,2,4),(-14.4146492123929,-14.3457397794975,-14.2690579791201,
-14.1912108935331,-14.1115926026985,-14.0355727044255,-13.9568648986143,
-13.8773078146962,-13.7976881026888,-13.7198092566215,-13.643166601816,
-13.5631476297004,-13.4861645139395,-13.4074202264935,-13.3284254156655,
-13.2522917794569,-13.1726458279891,-13.1529000929986),.UNSPECIFIED.);
#6020=B_SPLINE_CURVE_WITH_KNOTS('',3,(#237638,#237639,#237640,#237641,#237642,
#237643,#237644,#237645,#237646,#237647,#237648,#237649,#237650,#237651,
#237652,#237653,#237654,#237655,#237656,#237657,#237658,#237659,#237660,
#237661,#237662,#237663,#237664,#237665,#237666,#237667,#237668,#237669,
#237670,#237671,#237672,#237673),.UNSPECIFIED.,.F.,.F.,(4,2,2,2,2,2,2,2,
2,2,2,2,2,2,2,2,2,4),(-10.6886668367708,-10.6141171329505,-10.5368397267788,
-10.4574188227709,-10.3809842606412,-10.3009163157618,-10.2225611611604,
-10.1466878558215,-10.0672335555996,-9.98974112954057,-9.91291816909027,
-9.83331520225674,-9.75671789916803,-9.677448188703,-9.59888546489566,-9.52303209351768,
-9.44359290672304,-9.42971000722909),.UNSPECIFIED.);
#6021=B_SPLINE_CURVE_WITH_KNOTS('',3,(#237678,#237679,#237680,#237681,#237682,
#237683,#237684,#237685,#237686,#237687,#237688,#237689,#237690,#237691,
#237692,#237693,#237694,#237695,#237696,#237697,#237698,#237699,#237700,
#237701,#237702,#237703,#237704,#237705,#237706,#237707,#237708,#237709,
#237710,#237711,#237712,#237713),.UNSPECIFIED.,.F.,.F.,(4,2,2,2,2,2,2,2,
2,2,2,2,2,2,2,2,2,4),(-13.1529000929986,-13.0945058791895,-13.0180982140432,
-12.9377929757886,-12.8605508001914,-12.7823927291035,-12.7031007650497,
-12.626727585356,-12.5470099608498,-12.4685664186318,-12.3922568723288,
-12.3124597685296,-12.234887676826,-12.1572356575688,-12.0775759124685,
-12.0009090277532,-11.9203829768641,-11.8894930626961),.UNSPECIFIED.);
#6022=B_SPLINE_CURVE_WITH_KNOTS('',3,(#237714,#237715,#237716,#237717,#237718,
#237719,#237720,#237721,#237722,#237723,#237724,#237725,#237726,#237727,
#237728,#237729,#237730,#237731,#237732,#237733,#237734,#237735,#237736,
#237737,#237738,#237739,#237740,#237741,#237742,#237743,#237744,#237745,
#237746,#237747,#237748,#237749,#237750,#237751),.UNSPECIFIED.,.F.,.F.,
(4,2,2,2,2,2,2,2,2,2,2,2,2,2,2,2,2,2,4),(-11.949044188699,-11.9399073283772,
-11.8629827014429,-11.7844811604486,-11.7055394645275,-11.6294741132395,
-11.5499292488032,-11.4718399984583,-11.3955712959968,-11.3153146061308,
-11.2381226360676,-11.1601765604512,-11.0809304220309,-11.004650968641,
-10.9251700697058,-10.8469676740098,-10.7709605586456,-10.6914521379874,
-10.6886668367708),.UNSPECIFIED.);
#6023=B_SPLINE_CURVE_WITH_KNOTS('',3,(#237756,#237757,#237758,#237759,#237760,
#237761,#237762,#237763,#237764,#237765,#237766,#237767,#237768,#237769,
#237770,#237771,#237772,#237773,#237774,#237775,#237776,#237777,#237778,
#237779,#237780,#237781,#237782,#237783,#237784,#237785,#237786,#237787,
#237788,#237789,#237790,#237791),.UNSPECIFIED.,.F.,.F.,(4,2,2,2,2,2,2,2,
2,2,2,2,2,2,2,2,2,4),(-11.8894930626961,-11.8417990530921,-11.7656459491589,
-11.6859115275326,-11.6081942888121,-11.5310151799915,-11.4511857098612,
-11.3743674966686,-11.294655740804,-11.2158751815502,-11.1397691168386,
-11.0600587262734,-10.9821402628285,-10.9053440481854,-10.8252883261443,
-10.7482666060734,-10.6692911183768,-10.6263497039737),.UNSPECIFIED.);
#6024=B_SPLINE_CURVE_WITH_KNOTS('',3,(#237792,#237793,#237794,#237795,#237796,
#237797,#237798,#237799,#237800,#237801,#237802,#237803,#237804,#237805,
#237806,#237807,#237808,#237809,#237810,#237811,#237812,#237813,#237814,
#237815,#237816,#237817,#237818,#237819,#237820,#237821,#237822,#237823,
#237824,#237825,#237826,#237827),.UNSPECIFIED.,.F.,.F.,(4,2,2,2,2,2,2,2,
2,2,2,2,2,2,2,2,2,4),(-13.2089732113637,-13.188699892793,-13.1121716476065,
-13.0321957518606,-12.9537363504872,-12.8778110294063,-12.7982941966592,
-12.7206973807655,-12.643886836538,-12.5641727738037,-12.4874712705778,
-12.4082806472394,-12.3296035017028,-12.2536736195776,-12.1741639788225,
-12.0963447205716,-12.0198688686453,-11.949044188699),.UNSPECIFIED.);
#6025=B_SPLINE_CURVE_WITH_KNOTS('',3,(#237832,#237833,#237834,#237835,#237836,
#237837,#237838,#237839,#237840,#237841,#237842,#237843,#237844,#237845,
#237846,#237847,#237848,#237849,#237850,#237851,#237852,#237853,#237854,
#237855,#237856,#237857,#237858,#237859,#237860,#237861,#237862,#237863,
#237864,#237865,#237866,#237867),.UNSPECIFIED.,.F.,.F.,(4,2,2,2,2,2,2,2,
2,2,2,2,2,2,2,2,2,4),(-10.6263497039737,-10.590264032485,-10.5140776179666,
-10.4343500724478,-10.3561800171732,-10.2796467264391,-10.1993142464524,
-10.1220423076596,-10.0436833142805,-9.96436692329861,-9.88796784593152,
-9.80817848973431,-9.72971296377646,-9.65330724382957,-9.57265395682767,
-9.49509066675103,-9.41719889463007,-9.36205618767461),.UNSPECIFIED.);
#6026=B_SPLINE_CURVE_WITH_KNOTS('',3,(#237868,#237869,#237870,#237871,#237872,
#237873,#237874,#237875,#237876,#237877,#237878,#237879,#237880,#237881,
#237882,#237883,#237884,#237885,#237886,#237887,#237888,#237889,#237890,
#237891,#237892,#237893,#237894,#237895,#237896,#237897,#237898,#237899,
#237900,#237901,#237902,#237903),.UNSPECIFIED.,.F.,.F.,(4,2,2,2,2,2,2,2,
2,2,2,2,2,2,2,2,2,4),(-14.4685414185229,-14.4371861006538,-14.3570666160918,
-14.2806911965607,-14.201333110894,-14.1240417499958,-14.046765531488,-13.9672936809693,
-13.8913078705452,-13.8131641808844,-13.73372132699,-13.6574971431671,-13.5783096732641,
-13.5003327647789,-13.4231949969096,-13.3429966170248,-13.2667342522707,
-13.2089732113637),.UNSPECIFIED.);
#6027=B_SPLINE_CURVE_WITH_KNOTS('',3,(#237908,#237909,#237910,#237911,#237912,
#237913,#237914,#237915,#237916,#237917,#237918,#237919,#237920,#237921,
#237922,#237923,#237924,#237925,#237926,#237927,#237928,#237929,#237930,
#237931,#237932,#237933,#237934,#237935,#237936,#237937,#237938,#237939,
#237940,#237941,#237942,#237943),.UNSPECIFIED.,.F.,.F.,(4,2,2,2,2,2,2,2,
2,2,2,2,2,2,2,2,2,4),(-9.36205618767461,-9.33755664571965,-9.26090242145497,
-9.18113217965199,-9.10253596259969,-9.02631670802215,-8.94652766712044,
-8.86879953456162,-8.79148939019274,-8.71165272718738,-8.63482504688624,
-8.55491220288934,-8.47612988204783,-8.3999810243187,-8.32022382374916,
-8.24230500962556,-8.16539861414471,-8.09802537957356),.UNSPECIFIED.);
#6028=B_SPLINE_CURVE_WITH_KNOTS('',3,(#237944,#237945,#237946,#237947,#237948,
#237949,#237950,#237951,#237952,#237953,#237954,#237955,#237956,#237957,
#237958,#237959,#237960,#237961,#237962,#237963,#237964,#237965,#237966,
#237967,#237968,#237969,#237970,#237971,#237972,#237973,#237974,#237975,
#237976,#237977,#237978,#237979),.UNSPECIFIED.,.F.,.F.,(4,2,2,2,2,2,2,2,
2,2,2,2,2,2,2,2,2,4),(-15.7266574265448,-15.6832398993101,-15.6046482364568,
-15.5279086562263,-15.4481445412296,-15.371686569013,-15.2940538243071,
-15.2146602981345,-15.1388543838039,-15.0603634600351,-14.9810490749452,
-14.9045172989487,-14.8249840679432,-14.7481560310107,-14.6707292209604,
-14.5913158937944,-14.515475679086,-14.4685414185229),.UNSPECIFIED.);
#6029=B_SPLINE_CURVE_WITH_KNOTS('',3,(#237984,#237985,#237986,#237987,#237988,
#237989,#237990,#237991,#237992,#237993,#237994,#237995,#237996,#237997,
#237998,#237999,#238000,#238001,#238002,#238003,#238004,#238005,#238006,
#238007,#238008,#238009,#238010,#238011,#238012,#238013,#238014,#238015,
#238016,#238017,#238018,#238019),.UNSPECIFIED.,.F.,.F.,(4,2,2,2,2,2,2,2,
2,2,2,2,2,2,2,2,2,4),(-8.09802537957356,-8.08534627872566,-8.00832485868984,
-7.92916764555054,-7.8501479341364,-7.7739446603837,-7.69417866279333,-7.61601753652654,
-7.53939934799904,-7.45907954203661,-7.38181651819004,-7.30330259097503,
-7.22400130531918,-7.14761101036681,-7.06779228564878,-6.98934367034265,
-6.91288045049293,-6.83360317581237),.UNSPECIFIED.);
#6030=B_SPLINE_CURVE_WITH_KNOTS('',3,(#238020,#238021,#238022,#238023,#238024,
#238025,#238026,#238027,#238028,#238029,#238030,#238031,#238032,#238033,
#238034,#238035,#238036,#238037,#238038,#238039,#238040,#238041,#238042,
#238043,#238044,#238045,#238046,#238047,#238048,#238049,#238050,#238051,
#238052,#238053,#238054,#238055),.UNSPECIFIED.,.F.,.F.,(4,2,2,2,2,2,2,2,
2,2,2,2,2,2,2,2,2,4),(-16.9860676137287,-16.9305459155631,-16.8530028103589,
-16.775715329367,-16.6953469507869,-16.6192500471932,-16.5410633784241,
-16.4615818946196,-16.3854570106574,-16.3064235736138,-16.2284315885244,
-16.1514382709984,-16.0713936373972,-15.9951840612662,-15.9172958763925,
-15.8378808126566,-15.7619811309377,-15.7266574265448),.UNSPECIFIED.);
#6031=B_SPLINE_CURVE_WITH_KNOTS('',3,(#238060,#238061,#238062,#238063,#238064,
#238065,#238066,#238067,#238068,#238069,#238070,#238071,#238072,#238073,
#238074,#238075,#238076,#238077,#238078,#238079,#238080,#238081,#238082,
#238083,#238084,#238085,#238086,#238087,#238088,#238089,#238090,#238091,
#238092,#238093,#238094,#238095,#238096,#238097),.UNSPECIFIED.,.F.,.F.,
(4,2,2,2,2,2,2,2,2,2,2,2,2,2,2,2,2,2,4),(-6.83360317581237,-6.83224784905331,
-6.75470100800845,-6.67668555636461,-6.5970650214824,-6.52042947802374,
-6.4406450177057,-6.36207097203192,-6.28581916926094,-6.2060127908259,-6.12830778993307,
-6.05090391849408,-5.9710949013656,-5.8942914568354,-5.81421912317929,-5.73546942914718,
-5.65930973552131,-5.57954261838186,-5.56913783942761),.UNSPECIFIED.);
#6032=B_SPLINE_CURVE_WITH_KNOTS('',3,(#238098,#238099,#238100,#238101,#238102,
#238103,#238104,#238105,#238106,#238107,#238108,#238109,#238110,#238111,
#238112,#238113,#238114,#238115,#238116,#238117,#238118,#238119,#238120,
#238121,#238122,#238123,#238124,#238125,#238126,#238127,#238128,#238129,
#238130,#238131,#238132,#238133),.UNSPECIFIED.,.F.,.F.,(4,2,2,2,2,2,2,2,
2,2,2,2,2,2,2,2,2,4),(-18.2453522235663,-18.1776525209244,-18.1010656003546,
-18.0234153086571,-17.9439557986802,-17.8680906548125,-17.7895805206712,
-17.7100420811292,-17.6334836692764,-17.5539255287679,-17.476946377409,
-17.3994913336737,-17.3200039291733,-17.2440800453835,-17.1657605948636,
-17.0862902489563,-17.0099074139525,-16.9860676137287),.UNSPECIFIED.);
#6033=B_SPLINE_CURVE_WITH_KNOTS('',3,(#238138,#238139,#238140,#238141,#238142,
#238143,#238144,#238145,#238146,#238147,#238148,#238149,#238150,#238151,
#238152,#238153,#238154,#238155,#238156,#238157,#238158,#238159,#238160,
#238161,#238162,#238163,#238164,#238165,#238166,#238167,#238168,#238169,
#238170,#238171,#238172,#238173),.UNSPECIFIED.,.F.,.F.,(4,2,2,2,2,2,2,2,
2,2,2,2,2,2,2,2,2,4),(-5.56913783942761,-5.50165737991348,-5.42467576492216,
-5.34466158022702,-5.26767409052678,-5.1883740752882,-5.10939616535199,
-5.03320676482875,-4.95343878279698,-4.87532052203619,-4.79865084377856,
-4.71837849729253,-4.64115802239225,-4.56252559337156,-4.48327392493462,
-4.40692255332495,-4.32711046819931,-4.30497396562869),.UNSPECIFIED.);
#6034=B_SPLINE_CURVE_WITH_KNOTS('',3,(#238174,#238175,#238176,#238177,#238178,
#238179,#238180,#238181,#238182,#238183,#238184,#238185,#238186,#238187,
#238188,#238189,#238190,#238191,#238192,#238193,#238194,#238195,#238196,
#238197,#238198,#238199,#238200,#238201,#238202,#238203,#238204,#238205,
#238206,#238207,#238208,#238209),.UNSPECIFIED.,.F.,.F.,(4,2,2,2,2,2,2,2,
2,2,2,2,2,2,2,2,2,4),(-19.5051615199427,-19.4256178472367,-19.3494467260214,
-19.2712598891341,-19.1917305088467,-19.1155993348017,-19.0365636442837,
-18.958396927912,-18.8813955586696,-18.8013460874971,-18.7250340151242,
-18.6471376406698,-18.5676652621586,-18.4917331427441,-18.412981897987,
-18.334187158106,-18.2574308338498,-18.2453522235663),.UNSPECIFIED.);
#6035=B_SPLINE_CURVE_WITH_KNOTS('',3,(#238214,#238215,#238216,#238217,#238218,
#238219,#238220,#238221,#238222,#238223,#238224,#238225,#238226,#238227,
#238228,#238229,#238230,#238231,#238232,#238233,#238234,#238235,#238236,
#238237,#238238,#238239,#238240,#238241,#238242,#238243,#238244,#238245,
#238246,#238247,#238248,#238249),.UNSPECIFIED.,.F.,.F.,(4,2,2,2,2,2,2,2,
2,2,2,2,2,2,2,2,2,4),(-4.30497396562869,-4.24871276630561,-4.17222419819763,
-4.09164713925734,-4.01415041814135,-3.93604575143311,-3.85648152440021,
-3.77989805921464,-3.70013491408271,-3.62161738401807,-3.54536495412576,
-3.46557701007066,-3.38792909310605,-3.31046498954944,-3.23071851119358,
-3.15397297029016,-3.07377666013053,-3.0404377993062),.UNSPECIFIED.);
#6036=B_SPLINE_CURVE_WITH_KNOTS('',3,(#238250,#238251,#238252,#238253,#238254,
#238255,#238256,#238257,#238258,#238259,#238260,#238261,#238262,#238263,
#238264,#238265,#238266,#238267,#238268,#238269,#238270,#238271,#238272,
#238273,#238274,#238275,#238276,#238277,#238278,#238279,#238280,#238281,
#238282,#238283,#238284,#238285,#238286,#238287),.UNSPECIFIED.,.F.,.F.,
(4,2,2,2,2,2,2,2,2,2,2,2,2,2,2,2,2,2,4),(-20.7651480509305,-20.7542372169798,
-20.6747496324084,-20.5988578946382,-20.5203631373555,-20.4406458485752,
-20.364094824007,-20.2845468918017,-20.2074562622594,-20.1300073492215,
-20.0504843172495,-19.9745114843353,-19.896196995271,-19.8166942811889,
-19.7403133680385,-19.6609562476344,-19.5832709603124,-19.5059830142488,
-19.5051615199427),.UNSPECIFIED.);
#6037=B_SPLINE_CURVE_WITH_KNOTS('',3,(#238292,#238293,#238294,#238295,#238296,
#238297,#238298,#238299,#238300,#238301,#238302,#238303,#238304,#238305,
#238306,#238307,#238308,#238309,#238310,#238311,#238312,#238313,#238314,
#238315,#238316,#238317,#238318,#238319,#238320,#238321,#238322,#238323,
#238324,#238325,#238326,#238327),.UNSPECIFIED.,.F.,.F.,(4,2,2,2,2,2,2,2,
2,2,2,2,2,2,2,2,2,4),(-3.0404377993062,-2.99509419358038,-2.91895468092827,
-2.83921330030169,-2.7613958259546,-2.68437088706612,-2.60443001067381,
-2.52751036167285,-2.44810103283402,-2.3691998612149,-2.29305490552806,
-2.21332045711987,-2.13527956318884,-2.05858944660127,-1.9784000437842,
-1.90125631748013,-1.82253721525056,-1.77693741255607),.UNSPECIFIED.);
#6038=B_SPLINE_CURVE_WITH_KNOTS('',3,(#238328,#238329,#238330,#238331,#238332,
#238333,#238334,#238335,#238336,#238337,#238338,#238339,#238340,#238341,
#238342,#238343,#238344,#238345,#238346,#238347,#238348,#238349,#238350,
#238351,#238352,#238353,#238354,#238355,#238356,#238357,#238358,#238359,
#238360,#238361,#238362,#238363),.UNSPECIFIED.,.F.,.F.,(4,2,2,2,2,2,2,2,
2,2,2,2,2,2,2,2,2,4),(-22.0249622838298,-22.0023547571536,-21.922814161715,
-21.8467066862456,-21.7677031731419,-21.6894008143267,-21.6124250410366,
-21.5324054689352,-21.4560257497192,-21.3781551357414,-21.29866276063,-21.2227291775328,
-21.1440023962923,-21.0650466736007,-20.9883073940863,-20.9085497524053,
-20.8318709630664,-20.7651480509305),.UNSPECIFIED.);
#6039=B_SPLINE_CURVE_WITH_KNOTS('',3,(#238369,#238370,#238371,#238372,#238373,
#238374,#238375,#238376,#238377,#238378,#238379,#238380,#238381,#238382,
#238383,#238384),.UNSPECIFIED.,.F.,.F.,(4,2,2,2,2,2,2,4),(0.324863770283186,
0.395667134570481,0.472791225099944,0.552555445808509,0.629311039769859,
0.708734538016899,0.749777571670018,0.790730601234904),.UNSPECIFIED.);
#6040=B_SPLINE_CURVE_WITH_KNOTS('',3,(#238386,#238387,#238388,#238389,#238390,
#238391),.UNSPECIFIED.,.F.,.F.,(4,2,4),(1.00022081805299E-6,0.0243479089776584,
0.0486953353237867),.UNSPECIFIED.);
#6041=B_SPLINE_CURVE_WITH_KNOTS('',3,(#238392,#238393,#238394,#238395,#238396,
#238397,#238398,#238399,#238400,#238401,#238402,#238403,#238404,#238405,
#238406,#238407,#238408,#238409),.UNSPECIFIED.,.F.,.F.,(4,2,2,2,2,2,2,2,
4),(-0.513010840582583,-0.491707909785119,-0.415055184345757,-0.334765707541337,
-0.256186603725737,-0.180098289337284,-0.100418478920529,-0.0495366954217494,
-1.00000008074197E-6),.UNSPECIFIED.);
#6042=B_SPLINE_CURVE_WITH_KNOTS('',3,(#238419,#238420,#238421,#238422,#238423,
#238424),.UNSPECIFIED.,.F.,.F.,(4,2,4),(-0.0520203312674702,-0.0267861740298943,
-1.0000000459226E-6),.UNSPECIFIED.);
#6043=B_SPLINE_CURVE_WITH_KNOTS('',3,(#238441,#238442,#238443,#238444,#238445,
#238446,#238447,#238448,#238449,#238450,#238451,#238452),.UNSPECIFIED.,
 .F.,.F.,(4,2,2,2,2,4),(-0.179361978655781,-0.134721706620385,-0.0896676871854849,
-0.0448235819521571,-0.0392550189488239,-1.00000011879486E-6),
 .UNSPECIFIED.);
#6044=B_SPLINE_CURVE_WITH_KNOTS('',3,(#238969,#238970,#238971,#238972,#238973,
#238974,#238975,#238976,#238977,#238978,#238979,#238980,#238981,#238982,
#238983,#238984,#238985,#238986,#238987,#238988,#238989,#238990,#238991,
#238992,#238993,#238994,#238995,#238996),.UNSPECIFIED.,.F.,.F.,(4,2,2,2,
2,2,2,2,2,2,2,2,2,4),(22.6236748723828,22.6407093081193,22.7173617942293,
22.7968830932907,22.8754944544741,22.9514332474403,23.0309680597223,23.1087193135484,
23.1853402255204,23.2652245118562,23.3420810027936,23.4208695790923,23.4959114338434,
23.5687658403324),.UNSPECIFIED.);
#6045=B_SPLINE_CURVE_WITH_KNOTS('',3,(#238999,#239000,#239001,#239002,#239003,
#239004,#239005,#239006,#239007,#239008,#239009,#239010,#239011,#239012,
#239013,#239014,#239015,#239016,#239017,#239018,#239019,#239020,#239021,
#239022,#239023,#239024,#239025,#239026,#239027,#239028,#239029,#239030,
#239031,#239032,#239033,#239034),.UNSPECIFIED.,.F.,.F.,(4,2,2,2,2,2,2,2,
2,2,2,2,2,2,2,2,2,4),(9.99999999717517E-7,0.0462547190314567,0.0908553254087972,
0.167757479715614,0.247681226172906,0.324646289047548,0.40244572157152,
0.482152132491632,0.558256242839576,0.636919981793369,0.717024322840535,
0.793748683042598,0.873474040064272,0.950871759823262,1.02849766570582,
1.10824785849813,1.18445704254395,1.23484507369462),.UNSPECIFIED.);
#6046=B_SPLINE_CURVE_WITH_KNOTS('',3,(#239039,#239040,#239041,#239042,#239043,
#239044,#239045,#239046,#239047,#239048,#239049,#239050,#239051,#239052,
#239053,#239054,#239055,#239056,#239057,#239058,#239059,#239060,#239061,
#239062,#239063,#239064,#239065,#239066,#239067,#239068,#239069,#239070,
#239071,#239072,#239073,#239074),.UNSPECIFIED.,.F.,.F.,(4,2,2,2,2,2,2,2,
2,2,2,2,2,2,2,2,2,4),(21.3625688139077,21.3913787543729,21.4677304856353,
21.5473202777439,21.625593224373,21.7017308865875,21.7813507414309,21.8587542522225,
21.9362256297425,22.0157126587402,22.0922131081633,22.1725458477689,22.2509599885555,
22.3269434172786,22.4065014473729,22.4840508988643,22.5610518004103,22.6236748723828),
 .UNSPECIFIED.);
#6047=B_SPLINE_CURVE_WITH_KNOTS('',3,(#239075,#239076,#239077,#239078,#239079,
#239080,#239081,#239082,#239083,#239084,#239085,#239086,#239087,#239088,
#239089,#239090,#239091,#239092,#239093,#239094,#239095,#239096,#239097,
#239098,#239099,#239100,#239101,#239102,#239103,#239104,#239105,#239106,
#239107,#239108,#239109,#239110),.UNSPECIFIED.,.F.,.F.,(4,2,2,2,2,2,2,2,
2,2,2,2,2,2,2,2,2,4),(1.23484507369462,1.26295188142383,1.34267841695845,
1.41923862457627,1.49877951130816,1.57680660074797,1.65427879563786,1.73483163550077,
1.81126754077481,1.88964050402294,1.96941044583165,2.04573335376308,2.12495932843831,
2.20350299174566,2.28069623673453,2.36094148010891,2.43754863000376,2.49897999942429),
 .UNSPECIFIED.);
#6048=B_SPLINE_CURVE_WITH_KNOTS('',3,(#239115,#239116,#239117,#239118,#239119,
#239120,#239121,#239122,#239123,#239124,#239125,#239126,#239127,#239128,
#239129,#239130,#239131,#239132,#239133,#239134,#239135,#239136,#239137,
#239138,#239139,#239140,#239141,#239142,#239143,#239144,#239145,#239146,
#239147,#239148,#239149,#239150),.UNSPECIFIED.,.F.,.F.,(4,2,2,2,2,2,2,2,
2,2,2,2,2,2,2,2,2,4),(20.1001536081644,20.1407906125954,20.2168374619708,
20.2964789771982,20.3743832097966,20.4510415586,20.5310869382233,20.6080951883912,
20.6868495520353,20.765870747754,20.8420282128573,20.9216967326681,20.9998629340078,
21.0762885379599,21.1566210589077,21.2338891810234,21.3120596620606,21.3625688139077),
 .UNSPECIFIED.);
#6049=B_SPLINE_CURVE_WITH_KNOTS('',3,(#239151,#239152,#239153,#239154,#239155,
#239156,#239157,#239158,#239159,#239160,#239161,#239162,#239163,#239164,
#239165,#239166,#239167,#239168,#239169,#239170,#239171,#239172,#239173,
#239174,#239175,#239176,#239177,#239178,#239179,#239180,#239181,#239182,
#239183,#239184,#239185,#239186),.UNSPECIFIED.,.F.,.F.,(4,2,2,2,2,2,2,2,
2,2,2,2,2,2,2,2,2,4),(2.49897999942429,2.51563926655626,2.59536191643896,
2.67151353631666,2.7504629491092,2.82966487001291,2.90662200693993,2.98660571779551,
3.06351576270205,3.14136999944524,3.22108882729151,3.29720154164607,3.37591939849584,
3.45588714541026,3.53265668598561,3.61243138446563,3.68975672333244,3.76219964214866),
 .UNSPECIFIED.);
#6050=B_SPLINE_CURVE_WITH_KNOTS('',3,(#239191,#239192,#239193,#239194,#239195,
#239196,#239197,#239198,#239199,#239200,#239201,#239202,#239203,#239204,
#239205,#239206,#239207,#239208,#239209,#239210,#239211,#239212,#239213,
#239214,#239215,#239216,#239217,#239218,#239219,#239220,#239221,#239222,
#239223,#239224,#239225,#239226),.UNSPECIFIED.,.F.,.F.,(4,2,2,2,2,2,2,2,
2,2,2,2,2,2,2,2,2,4),(18.8378147773619,18.8895407867648,18.9657401122406,
19.045450464741,19.1229833437424,19.2004539326094,19.2800782003355,19.3567083962423,
19.4369741709152,19.5155301835049,19.5915961112866,19.6712524836123,19.7489436039846,
19.8259591767686,19.905766394743,19.9825601373105,20.0620261236383,20.1001536081644),
 .UNSPECIFIED.);
#6051=B_SPLINE_CURVE_WITH_KNOTS('',3,(#239227,#239228,#239229,#239230,#239231,
#239232,#239233,#239234,#239235,#239236,#239237,#239238,#239239,#239240,
#239241,#239242,#239243,#239244,#239245,#239246,#239247,#239248,#239249,
#239250,#239251,#239252,#239253,#239254,#239255,#239256,#239257,#239258,
#239259,#239260,#239261,#239262,#239263,#239264),.UNSPECIFIED.,.F.,.F.,
(4,2,2,2,2,2,2,2,2,2,2,2,2,2,2,2,2,2,4),(3.76219964214866,3.76742688845616,
3.84718218555019,3.92337891552651,4.00191728040496,4.08165181563963,4.15825144289695,
4.23783551467587,4.31576094089768,4.39327050359559,4.47386566806185,4.55026435353068,
4.62867535147353,4.7084385050342,4.78478892495954,4.86405145560046,4.94246356555156,
5.01968665557928,5.02622452893907),.UNSPECIFIED.);
#6052=B_SPLINE_CURVE_WITH_KNOTS('',3,(#239269,#239270,#239271,#239272,#239273,
#239274,#239275,#239276,#239277,#239278,#239279,#239280,#239281,#239282,
#239283,#239284,#239285,#239286,#239287,#239288,#239289,#239290,#239291,
#239292,#239293,#239294,#239295,#239296,#239297,#239298,#239299,#239300,
#239301,#239302,#239303,#239304),.UNSPECIFIED.,.F.,.F.,(4,2,2,2,2,2,2,2,
2,2,2,2,2,2,2,2,2,4),(17.5740980330669,17.6369933046161,17.7136606695414,
17.7938263393176,17.8709472323695,17.9496429457457,18.0287862833124,18.1050454201912,
18.1847918646659,18.2630806427599,18.3395412734652,18.4200031485925,18.4973923493336,
18.5755322223201,18.6549810287802,18.7314554867318,18.811138344041,18.8378147773619),
 .UNSPECIFIED.);
#6053=B_SPLINE_CURVE_WITH_KNOTS('',3,(#239305,#239306,#239307,#239308,#239309,
#239310,#239311,#239312,#239313,#239314,#239315,#239316,#239317,#239318,
#239319,#239320,#239321,#239322,#239323,#239324,#239325,#239326,#239327,
#239328,#239329,#239330,#239331,#239332,#239333,#239334,#239335,#239336,
#239337,#239338,#239339,#239340),.UNSPECIFIED.,.F.,.F.,(4,2,2,2,2,2,2,2,
2,2,2,2,2,2,2,2,2,4),(5.02622452893907,5.09996620350271,5.17650963611587,
5.25463032028455,5.33433742926195,5.4104913933453,5.48946961334628,5.56851486802525,
5.64549327134522,5.7255020272037,5.80232422478868,5.88019926400631,5.95989449979103,
6.03598450046676,6.11472204449212,6.19451553182695,6.27129665989664,6.28915126608589),
 .UNSPECIFIED.);
#6054=B_SPLINE_CURVE_WITH_KNOTS('',3,(#239345,#239346,#239347,#239348,#239349,
#239350,#239351,#239352,#239353,#239354,#239355,#239356,#239357,#239358,
#239359,#239360,#239361,#239362,#239363,#239364,#239365,#239366,#239367,
#239368,#239369,#239370,#239371,#239372,#239373,#239374,#239375,#239376,
#239377,#239378,#239379,#239380),.UNSPECIFIED.,.F.,.F.,(4,2,2,2,2,2,2,2,
2,2,2,2,2,2,2,2,2,4),(16.3109364258552,16.3847150284939,16.4621561301153,
16.541878995712,16.6186018112264,16.698774275327,16.777433447177,16.8535503932859,
16.9332681431273,17.0110625795403,17.088064655456,17.1679818672716,17.2448787446325,
17.3242644681819,17.4031422854142,17.4792646858285,17.5589755096573,17.5740980330669),
 .UNSPECIFIED.);
#6055=B_SPLINE_CURVE_WITH_KNOTS('',3,(#239381,#239382,#239383,#239384,#239385,
#239386,#239387,#239388,#239389,#239390,#239391,#239392,#239393,#239394,
#239395,#239396,#239397,#239398,#239399,#239400,#239401,#239402,#239403,
#239404,#239405,#239406,#239407,#239408,#239409,#239410,#239411,#239412,
#239413,#239414,#239415,#239416),.UNSPECIFIED.,.F.,.F.,(4,2,2,2,2,2,2,2,
2,2,2,2,2,2,2,2,2,4),(6.28915126608589,6.35108591673579,6.42830404984285,
6.50598458202569,6.58570875809415,6.66186055160458,6.74040816495516,6.82011480794906,
6.896720527872,6.9763132947808,7.05410096033775,7.13161426404932,7.21221698959725,
7.28854551609797,7.3669605933149,7.44668040181184,7.52302826097822,7.55270818716772),
 .UNSPECIFIED.);
#6056=B_SPLINE_CURVE_WITH_KNOTS('',3,(#239421,#239422,#239423,#239424,#239425,
#239426,#239427,#239428,#239429,#239430,#239431,#239432,#239433,#239434,
#239435,#239436,#239437,#239438,#239439,#239440,#239441,#239442,#239443,
#239444,#239445,#239446,#239447,#239448,#239449,#239450,#239451,#239452,
#239453,#239454,#239455,#239456,#239457,#239458),.UNSPECIFIED.,.F.,.F.,
(4,2,2,2,2,2,2,2,2,2,2,2,2,2,2,2,2,2,4),(15.0466193961525,15.0546599548629,
15.1318575552455,15.210466605289,15.2896948007098,15.3660235527781,15.4458119759886,
15.5241864587444,15.600652332661,15.6812055287019,15.7586792974288,15.8367607569033,
15.9163014218172,15.9928622064941,16.0726017119744,16.1510959904507,16.2273258093889,
16.3070901049585,16.3109364258552),.UNSPECIFIED.);
#6057=B_SPLINE_CURVE_WITH_KNOTS('',3,(#239459,#239460,#239461,#239462,#239463,
#239464,#239465,#239466,#239467,#239468,#239469,#239470,#239471,#239472,
#239473,#239474,#239475,#239476,#239477,#239478,#239479,#239480,#239481,
#239482,#239483,#239484,#239485,#239486,#239487,#239488,#239489,#239490,
#239491,#239492,#239493,#239494),.UNSPECIFIED.,.F.,.F.,(4,2,2,2,2,2,2,2,
2,2,2,2,2,2,2,2,2,4),(7.55270818716772,7.60229285314904,7.68053493798863,
7.75775418641584,7.8380332458771,7.91447842599388,7.9925951681434,8.07224958728399,
8.14837493544016,8.22734745510189,8.30619469613861,8.38316057429433,8.46315948803179,
8.53985724263922,8.61771899026031,8.69735293570344,8.77338771037036,8.81490714031691),
 .UNSPECIFIED.);
#6058=B_SPLINE_CURVE_WITH_KNOTS('',3,(#239499,#239500,#239501,#239502,#239503,
#239504,#239505,#239506,#239507,#239508,#239509,#239510,#239511,#239512,
#239513,#239514,#239515,#239516,#239517,#239518,#239519,#239520,#239521,
#239522,#239523,#239524,#239525,#239526,#239527,#239528,#239529,#239530,
#239531,#239532,#239533,#239534),.UNSPECIFIED.,.F.,.F.,(4,2,2,2,2,2,2,2,
2,2,2,2,2,2,2,2,2,4),(13.7830271212104,13.8023150783772,13.8790957622896,
13.9591442691831,14.0378706299548,14.1140077346993,14.1937511946023,14.2716133566261,
14.3485721051306,14.4285625845395,14.505527264209,14.584803690052,14.6637582039623,
14.7399250197211,14.8196693484089,14.8977644685878,14.9744113852441,15.0466193961525),
 .UNSPECIFIED.);
#6059=B_SPLINE_CURVE_WITH_KNOTS('',3,(#239535,#239536,#239537,#239538,#239539,
#239540,#239541,#239542,#239543,#239544,#239545,#239546,#239547,#239548,
#239549,#239550,#239551,#239552,#239553,#239554,#239555,#239556,#239557,
#239558,#239559,#239560,#239561,#239562,#239563,#239564,#239565,#239566,
#239567,#239568,#239569,#239570),.UNSPECIFIED.,.F.,.F.,(4,2,2,2,2,2,2,2,
2,2,2,2,2,2,2,2,2,4),(8.81490714031691,8.85211036064628,8.9316852408578,
9.008443970894,9.08821269376554,9.16528452273819,9.24294109920656,9.32259595371586,
9.39866832476149,9.47719040174472,9.55683132445173,9.63340918913478,9.71297561297174,
9.79058398860146,9.86806671460512,9.94545247074768,10.0232994383367,10.07726006159),
 .UNSPECIFIED.);
#6060=B_SPLINE_CURVE_WITH_KNOTS('',3,(#239575,#239576,#239577,#239578,#239579,
#239580,#239581,#239582,#239583,#239584,#239585,#239586,#239587,#239588,
#239589,#239590,#239591,#239592,#239593,#239594,#239595,#239596,#239597,
#239598,#239599,#239600,#239601,#239602,#239603,#239604,#239605,#239606,
#239607,#239608,#239609,#239610),.UNSPECIFIED.,.F.,.F.,(4,2,2,2,2,2,2,2,
2,2,2,2,2,2,2,2,2,4),(12.5184563203764,12.5497802836604,12.6261479314363,
12.7059429734401,12.7843683363411,12.8608088529379,12.9414175563509,13.0189414121536,
13.0969336657911,13.1765306033314,13.2531434329733,13.3329042286112,13.4114549875406,
13.4876841628844,13.5674668685525,13.6451488408897,13.7225297112902,13.7830271212104),
 .UNSPECIFIED.);
#6061=B_SPLINE_CURVE_WITH_KNOTS('',3,(#239611,#239612,#239613,#239614,#239615,
#239616,#239617,#239618,#239619,#239620,#239621,#239622,#239623,#239624,
#239625,#239626,#239627,#239628,#239629,#239630,#239631,#239632,#239633,
#239634,#239635,#239636,#239637,#239638,#239639,#239640,#239641,#239642,
#239643,#239644,#239645,#239646),.UNSPECIFIED.,.F.,.F.,(4,2,2,2,2,2,2,2,
2,2,2,2,2,2,2,2,2,4),(10.07726006159,10.1027548027335,10.1792312683471,
10.2588485858205,10.3372596705821,10.4133508147372,10.4929898662385,10.5705337636431,
10.6477717871671,10.7274155175606,10.8040597932003,10.8839577096872,10.9625445602035,
11.0385447654803,11.1181449759676,11.1958692177396,11.2726866802344,11.3388557888326),
 .UNSPECIFIED.);
#6062=B_SPLINE_CURVE_WITH_KNOTS('',3,(#239651,#239652,#239653,#239654,#239655,
#239656,#239657,#239658,#239659,#239660,#239661,#239662,#239663,#239664,
#239665,#239666,#239667,#239668,#239669,#239670,#239671,#239672,#239673,
#239674,#239675,#239676,#239677,#239678,#239679,#239680,#239681,#239682,
#239683,#239684,#239685,#239686),.UNSPECIFIED.,.F.,.F.,(4,2,2,2,2,2,2,2,
2,2,2,2,2,2,2,2,2,4),(11.2548510467115,11.2980233086365,11.3741495640617,
11.4538830912037,11.5317788009478,11.6086623347247,11.6886909350883,11.7656895172056,
11.8448231642113,11.923819448896,12.0000001175665,12.0797424434144,12.1578803983245,
12.2344758235014,12.3147718199753,12.3920119387833,12.4705025041557,12.5184563203764),
 .UNSPECIFIED.);
#6063=B_SPLINE_CURVE_WITH_KNOTS('',3,(#239687,#239688,#239689,#239690,#239691,
#239692,#239693,#239694,#239695,#239696,#239697,#239698,#239699,#239700,
#239701,#239702,#239703,#239704,#239705,#239706,#239707,#239708,#239709,
#239710,#239711,#239712,#239713,#239714,#239715,#239716,#239717,#239718,
#239719,#239720,#239721,#239722),.UNSPECIFIED.,.F.,.F.,(4,2,2,2,2,2,2,2,
2,2,2,2,2,2,2,2,2,4),(11.3388557888326,11.3525356361157,11.4293640214325,
11.5084919604289,11.5873069769148,11.6633379518827,11.7429393865072,11.8208965953283,
11.8974038509132,11.9775108617879,12.0545721457777,12.1330349777865,12.2121235451364,
12.288317305646,12.3679631434665,12.4461995842588,12.5225273003769,12.6005934315007),
 .UNSPECIFIED.);
#6064=B_SPLINE_CURVE_WITH_KNOTS('',3,(#239727,#239728,#239729,#239730,#239731,
#239732,#239733,#239734,#239735,#239736,#239737,#239738,#239739,#239740,
#239741,#239742,#239743,#239744,#239745,#239746,#239747,#239748,#239749,
#239750,#239751,#239752,#239753,#239754,#239755,#239756,#239757,#239758,
#239759,#239760,#239761,#239762),.UNSPECIFIED.,.F.,.F.,(4,2,2,2,2,2,2,2,
2,2,2,2,2,2,2,2,2,4),(9.99071847554691,10.0448123826062,10.1211953987327,
10.2018247631317,10.2793650452417,10.3572336365993,10.4368522634336,10.513483750659,
10.5932303128834,10.6718032184567,10.7479998379628,10.8277651919765,10.9054702711791,
10.9827574236387,11.0625704099994,11.1393753047155,11.2192643489391,11.2548510467115),
 .UNSPECIFIED.);
#6065=B_SPLINE_CURVE_WITH_KNOTS('',3,(#239763,#239764,#239765,#239766,#239767,
#239768,#239769,#239770,#239771,#239772,#239773,#239774,#239775,#239776,
#239777,#239778,#239779,#239780,#239781,#239782,#239783,#239784,#239785,
#239786,#239787,#239788,#239789,#239790,#239791,#239792,#239793,#239794,
#239795,#239796,#239797,#239798,#239799,#239800),.UNSPECIFIED.,.F.,.F.,
(4,2,2,2,2,2,2,2,2,2,2,2,2,2,2,2,2,2,4),(12.6005934315007,12.602938763315,
12.6802760682319,12.7582135669689,12.8376143514832,12.9140404005903,12.9936380748357,
13.0719943611852,13.1480875810128,13.2277098734604,13.3051983880356,13.3824979963671,
13.4620809471436,13.5386690096921,13.6186921682012,13.6972135502531,13.7731950393595,
13.8527712040441,13.8621232120524),.UNSPECIFIED.);
#6066=B_SPLINE_CURVE_WITH_KNOTS('',3,(#239805,#239806,#239807,#239808,#239809,
#239810,#239811,#239812,#239813,#239814,#239815,#239816,#239817,#239818,
#239819,#239820,#239821,#239822,#239823,#239824,#239825,#239826,#239827,
#239828,#239829,#239830,#239831,#239832,#239833,#239834,#239835,#239836,
#239837,#239838,#239839,#239840),.UNSPECIFIED.,.F.,.F.,(4,2,2,2,2,2,2,2,
2,2,2,2,2,2,2,2,2,4),(8.72728889099367,8.79501613456367,8.87186385542684,
8.94976017855893,9.02947910082415,9.10559165966755,9.18435078087881,9.26417432599307,
9.34097681421297,9.42078815997437,9.49803277374631,9.57573497112963,9.65548316171832,
9.73165848498506,9.8102280573935,9.88660446939589,9.96637013208894,9.99071847554691),
 .UNSPECIFIED.);
#6067=B_SPLINE_CURVE_WITH_KNOTS('',3,(#239841,#239842,#239843,#239844,#239845,
#239846,#239847,#239848,#239849,#239850,#239851,#239852,#239853,#239854,
#239855,#239856,#239857,#239858,#239859,#239860,#239861,#239862,#239863,
#239864,#239865,#239866,#239867,#239868,#239869,#239870,#239871,#239872,
#239873,#239874,#239875,#239876),.UNSPECIFIED.,.F.,.F.,(4,2,2,2,2,2,2,2,
2,2,2,2,2,2,2,2,2,4),(13.8621232120524,13.9304294236307,14.0072915450429,
14.0870689942372,14.1638312685282,14.243069734594,14.3218098137758,14.3977978550319,
14.4773674628283,14.5552490882758,14.6317781328063,14.7118040439196,14.7887903475489,
14.8673410523001,14.9463465581447,15.0224722538337,15.1020778057827,15.1231092357584),
 .UNSPECIFIED.);
#6068=B_SPLINE_CURVE_WITH_KNOTS('',3,(#239881,#239882,#239883,#239884,#239885,
#239886,#239887,#239888,#239889,#239890,#239891,#239892,#239893,#239894,
#239895,#239896,#239897,#239898,#239899,#239900,#239901,#239902,#239903,
#239904,#239905,#239906,#239907,#239908,#239909,#239910,#239911,#239912,
#239913,#239914,#239915,#239916),.UNSPECIFIED.,.F.,.F.,(4,2,2,2,2,2,2,2,
2,2,2,2,2,2,2,2,2,4),(7.46340241241562,7.54301805341094,7.61943998793248,
7.69787170413151,7.77765784819711,7.85402877837828,7.93331233352954,8.0117522463032,
8.08899605949032,8.16929701121815,8.24586485699811,8.32400650944155,8.40373696570717,
8.47991244175215,8.55891192768175,8.63798625095867,8.71498566581844,8.72728889099367),
 .UNSPECIFIED.);
#6069=B_SPLINE_CURVE_WITH_KNOTS('',3,(#239917,#239918,#239919,#239920,#239921,
#239922,#239923,#239924,#239925,#239926,#239927,#239928,#239929,#239930,
#239931,#239932,#239933,#239934,#239935,#239936,#239937,#239938,#239939,
#239940,#239941,#239942,#239943,#239944,#239945,#239946,#239947,#239948,
#239949,#239950,#239951,#239952),.UNSPECIFIED.,.F.,.F.,(4,2,2,2,2,2,2,2,
2,2,2,2,2,2,2,2,2,4),(15.1231092357584,15.1802303202402,15.2565541765279,
15.3368761555168,15.4141306527047,15.4921277966692,15.5714385512177,15.6477800297023,
15.7273227850391,15.8055890541803,15.881653251365,15.9612233321017,16.0386216052047,
16.1159520022845,16.1954382244697,16.2719354612956,16.3520530655929,16.3842164827505),
 .UNSPECIFIED.);
#6070=B_SPLINE_CURVE_WITH_KNOTS('',3,(#239957,#239958,#239959,#239960,#239961,
#239962,#239963,#239964,#239965,#239966,#239967,#239968,#239969,#239970,
#239971,#239972,#239973,#239974,#239975,#239976,#239977,#239978,#239979,
#239980,#239981,#239982,#239983,#239984,#239985,#239986,#239987,#239988,
#239989,#239990,#239991,#239992,#239993,#239994),.UNSPECIFIED.,.F.,.F.,
(4,2,2,2,2,2,2,2,2,2,2,2,2,2,2,2,2,2,4),(6.19938299209805,6.21014794327352,
6.28988894821445,6.36602291168288,6.44476091855524,6.5247570910379,6.60154659665179,
6.68134194060473,6.75869227209202,6.83638269450315,6.9161604845104,6.9923793783196,
7.07093827717526,7.1506951720957,7.22731494863593,7.30691986016907,7.38487167598359,
7.46240172944621,7.46340241241562),.UNSPECIFIED.);
#6071=B_SPLINE_CURVE_WITH_KNOTS('',3,(#239995,#239996,#239997,#239998,#239999,
#240000,#240001,#240002,#240003,#240004,#240005,#240006,#240007,#240008,
#240009,#240010,#240011,#240012,#240013,#240014,#240015,#240016,#240017,
#240018,#240019,#240020,#240021,#240022,#240023,#240024,#240025,#240026,
#240027,#240028,#240029,#240030),.UNSPECIFIED.,.F.,.F.,(4,2,2,2,2,2,2,2,
2,2,2,2,2,2,2,2,2,4),(16.3842164827505,16.4304731640843,16.5064051428445,
16.5859216865821,16.6634784492848,16.7403553652435,16.820024748001,16.8966857350638,
16.9760055552314,17.054634238895,17.1305483096494,17.2100503919758,17.2878203704037,
17.364341733933,17.4442493394675,17.5211249001405,17.5997353506844,17.6440450612851),
 .UNSPECIFIED.);
#6072=B_SPLINE_CURVE_WITH_KNOTS('',3,(#240035,#240036,#240037,#240038,#240039,
#240040,#240041,#240042,#240043,#240044,#240045,#240046,#240047,#240048,
#240049,#240050,#240051,#240052,#240053,#240054,#240055,#240056,#240057,
#240058,#240059,#240060,#240061,#240062,#240063,#240064,#240065,#240066,
#240067,#240068,#240069,#240070),.UNSPECIFIED.,.F.,.F.,(4,2,2,2,2,2,2,2,
2,2,2,2,2,2,2,2,2,4),(4.93557907506006,4.95807649474067,5.03786794568686,
5.11421010640617,5.1934556653646,5.27202569037795,5.34923825762195,5.42950345425129,
5.50613366843463,5.58424385977541,5.66398836103944,5.74016022249727,5.81912946818321,
5.89835892633256,5.97533567811949,6.05533965656332,6.13227383133234,6.19938299209805),
 .UNSPECIFIED.);
#6073=B_SPLINE_CURVE_WITH_KNOTS('',3,(#240071,#240072,#240073,#240074,#240075,
#240076,#240077,#240078,#240079,#240080,#240081,#240082,#240083,#240084,
#240085,#240086,#240087,#240088,#240089,#240090,#240091,#240092,#240093,
#240094,#240095,#240096,#240097,#240098,#240099,#240100,#240101,#240102,
#240103,#240104,#240105,#240106),.UNSPECIFIED.,.F.,.F.,(4,2,2,2,2,2,2,2,
2,2,2,2,2,2,2,2,2,4),(17.6440450612851,17.6786207001756,17.7546464114692,
17.8341758503396,17.91220775608,17.9884979989117,18.068692661484,18.145828028411,
18.2238569341798,18.3030400062917,18.3792607066525,18.4587122680853,18.5368510646172,
18.6128551439165,18.6923365995457,18.7696075127427,18.8469399687415,18.9040360682104),
 .UNSPECIFIED.);
#6074=B_SPLINE_CURVE_WITH_KNOTS('',3,(#240111,#240112,#240113,#240114,#240115,
#240116,#240117,#240118,#240119,#240120,#240121,#240122,#240123,#240124,
#240125,#240126,#240127,#240128,#240129,#240130,#240131,#240132,#240133,
#240134,#240135,#240136,#240137,#240138,#240139,#240140,#240141,#240142,
#240143,#240144,#240145,#240146),.UNSPECIFIED.,.F.,.F.,(4,2,2,2,2,2,2,2,
2,2,2,2,2,2,2,2,2,4),(3.6713151088133,3.7050232003142,3.78515463088442,
3.86189760876706,3.94164221384685,4.01906364102073,4.0967084462536,4.17647971918973,
4.25270981752711,4.33122379458765,4.41097122102382,4.48755018224877,4.56711046192888,
4.64516256671576,4.7226538463442,4.80322638839784,4.87968423324783,4.93557907506006),
 .UNSPECIFIED.);
#6075=B_SPLINE_CURVE_WITH_KNOTS('',3,(#240147,#240148,#240149,#240150,#240151,
#240152,#240153,#240154,#240155,#240156,#240157,#240158,#240159,#240160,
#240161,#240162,#240163,#240164,#240165,#240166,#240167,#240168,#240169,
#240170,#240171,#240172,#240173,#240174,#240175,#240176,#240177,#240178,
#240179,#240180,#240181,#240182),.UNSPECIFIED.,.F.,.F.,(4,2,2,2,2,2,2,2,
2,2,2,2,2,2,2,2,2,4),(18.9040360682104,18.9262910406328,19.0026605322289,
19.0828460907298,19.1611264225512,19.2369775122534,19.3163976259115,19.3938148083998,
19.4706783340212,19.5502001780755,19.6267219868126,19.706098068117,19.7845758100659,
19.8603835447724,19.9397808781415,20.0174000463419,20.0938853198427,20.1622975463945),
 .UNSPECIFIED.);
#6076=B_SPLINE_CURVE_WITH_KNOTS('',3,(#240187,#240188,#240189,#240190,#240191,
#240192,#240193,#240194,#240195,#240196,#240197,#240198,#240199,#240200,
#240201,#240202,#240203,#240204,#240205,#240206,#240207,#240208,#240209,
#240210,#240211,#240212,#240213,#240214,#240215,#240216,#240217,#240218,
#240219,#240220,#240221,#240222),.UNSPECIFIED.,.F.,.F.,(4,2,2,2,2,2,2,2,
2,2,2,2,2,2,2,2,2,4),(2.40800177534909,2.45399201896089,2.53265891076704,
2.60980635838972,2.69000068997139,2.76666154078788,2.84470609564807,2.9244289591419,
3.0005666709432,3.07947104951592,3.15882048506469,3.23574089239875,3.31568349328153,
3.39267145052468,3.47048938577085,3.55021656235879,3.62634069975032,3.6713151088133),
 .UNSPECIFIED.);
#6077=B_SPLINE_CURVE_WITH_KNOTS('',3,(#240223,#240224,#240225,#240226,#240227,
#240228,#240229,#240230,#240231,#240232,#240233,#240234,#240235,#240236,
#240237,#240238,#240239,#240240,#240241,#240242,#240243,#240244,#240245,
#240246,#240247,#240248,#240249,#240250,#240251,#240252,#240253,#240254,
#240255,#240256,#240257,#240258),.UNSPECIFIED.,.F.,.F.,(4,2,2,2,2,2,2,2,
2,2,2,2,2,2,2,2,2,4),(20.1622975463945,20.1736340848943,20.2503600390948,
20.3290056748752,20.4077303181208,20.4836219336482,20.5630375985878,20.6409087371531,
20.7171358811133,20.7971616872148,20.8741381490283,20.9521737072777,21.0311876618635,
21.1072948695045,21.1867734591295,21.2649400887203,21.3410441964928,21.4212632201289),
 .UNSPECIFIED.);
#6078=B_SPLINE_CURVE_WITH_KNOTS('',3,(#240264,#240265,#240266,#240267,#240268,
#240269),.UNSPECIFIED.,.F.,.F.,(4,2,4),(22.6805778338202,22.7225346851399,
22.7746249205198),.UNSPECIFIED.);
#6079=B_SPLINE_CURVE_WITH_KNOTS('',3,(#240271,#240272,#240273,#240274,#240275,
#240276,#240277,#240278,#240279,#240280),.UNSPECIFIED.,.F.,.F.,(4,2,2,2,
4),(0.,0.0529987112262313,0.105968001362697,0.158971646797024,0.21203675183673),
 .UNSPECIFIED.);
#6080=B_SPLINE_CURVE_WITH_KNOTS('',3,(#240282,#240283,#240284,#240285,#240286,
#240287,#240288,#240289,#240290,#240291,#240292,#240293,#240294,#240295,
#240296,#240297,#240298,#240299,#240300,#240301,#240302,#240303,#240304,
#240305,#240306,#240307),.UNSPECIFIED.,.F.,.F.,(4,2,2,2,2,2,2,2,2,2,2,2,
4),(-0.790728037067121,-0.749775115806686,-0.708732159090347,-0.62930879973315,
-0.552553327511713,-0.472789234158408,-0.395665227958601,-0.31556998695274,
-0.238516351993173,-0.159861788318521,-0.080788503022024,-0.0396943940909934,
-9.95303702788775E-7),.UNSPECIFIED.);
#6081=B_SPLINE_CURVE_WITH_KNOTS('',3,(#240310,#240311,#240312,#240313,#240314,
#240315,#240316,#240317,#240318,#240319,#240320,#240321,#240322,#240323,
#240324,#240325,#240326,#240327,#240328,#240329,#240330,#240331,#240332,
#240333,#240334,#240335,#240336,#240337,#240338,#240339,#240340,#240341,
#240342,#240343),.UNSPECIFIED.,.F.,.F.,(4,2,2,2,2,2,2,2,2,2,2,2,2,2,2,2,
4),(1.00510724934941E-6,0.0525834672969985,0.106573631372961,0.186239291839903,
0.262311996105734,0.341115594311459,0.42055455516659,0.497383903920253,
0.577229073521196,0.654240311296405,0.731967090606045,0.811644918579921,
0.887728407406906,0.966320033313811,1.04655454272418,1.12321674093992,1.14417183100891),
 .UNSPECIFIED.);
#6082=B_SPLINE_CURVE_WITH_KNOTS('',3,(#240353,#240354,#240355,#240356,#240357,
#240358,#240359,#240360,#240361,#240362,#240363,#240364,#240365,#240366,
#240367,#240368),.UNSPECIFIED.,.F.,.F.,(4,3,3,3,3,4),(0.,0.144328413863221,
0.303472318230778,0.628464617347887,0.963059075130798,1.),.UNSPECIFIED.);
#6083=B_SPLINE_CURVE_WITH_KNOTS('',3,(#240385,#240386,#240387,#240388,#240389,
#240390,#240391,#240392,#240393,#240394,#240395,#240396),.UNSPECIFIED.,
 .F.,.F.,(4,2,2,2,2,4),(1.00000010121019E-6,0.0446394239019562,0.0896993921078784,
0.134509378723331,0.140080640396739,0.179359231239673),.UNSPECIFIED.);
#6084=B_SPLINE_CURVE_WITH_KNOTS('',3,(#240914,#240915,#240916,#240917,#240918,
#240919,#240920,#240921,#240922,#240923),.UNSPECIFIED.,.F.,.F.,(4,2,2,2,
4),(9.99999999774313E-7,0.0674884200460847,0.133887544817669,0.212371065462948,
0.287372916582337),.UNSPECIFIED.);
#6085=B_SPLINE_CURVE_WITH_KNOTS('',3,(#240928,#240929,#240930,#240931,#240932,
#240933,#240934,#240935,#240936,#240937,#240938,#240939,#240940,#240941,
#240942,#240943,#240944,#240945,#240946,#240947,#240948,#240949,#240950,
#240951,#240952,#240953,#240954,#240955,#240956,#240957,#240958,#240959,
#240960,#240961,#240962,#240963),.UNSPECIFIED.,.F.,.F.,(4,2,2,2,2,2,2,2,
2,2,2,2,2,2,2,2,2,4),(22.2691796383917,22.2806866530766,22.3601873799206,
22.4379542915872,22.5144766103392,22.5943809263863,22.671253438802,22.7498674627958,
22.8287494305076,22.9047725585822,22.9843003162939,23.062328811022,23.1386190219282,
23.2188100493447,23.2959420465468,23.3739734639397,23.4527575968905,23.5294112994357),
 .UNSPECIFIED.);
#6086=B_SPLINE_CURVE_WITH_KNOTS('',3,(#240964,#240965,#240966,#240967,#240968,
#240969,#240970,#240971,#240972,#240973,#240974,#240975,#240976,#240977,
#240978,#240979,#240980,#240981,#240982,#240983,#240984,#240985,#240986,
#240987,#240988,#240989,#240990,#240991,#240992,#240993,#240994,#240995,
#240996,#240997,#240998,#240999,#241000,#241001),.UNSPECIFIED.,.F.,.F.,
(4,2,2,2,2,2,2,2,2,2,2,2,2,2,2,2,2,2,4),(0.287372916582337,0.292012075113482,
0.368555506568093,0.448083595544,0.52580567198518,0.603255911016295,0.683793119295233,
0.760058356770533,0.838409640892086,0.918063811525401,0.994349480776281,
1.07354955396753,1.15172514075825,1.22888144004619,1.30909511453487,1.38547644460694,
1.46352950583805,1.54311818413994,1.54965533150543),.UNSPECIFIED.);
#6087=B_SPLINE_CURVE_WITH_KNOTS('',3,(#241006,#241007,#241008,#241009,#241010,
#241011,#241012,#241013,#241014,#241015,#241016,#241017,#241018,#241019,
#241020,#241021,#241022,#241023,#241024,#241025,#241026,#241027,#241028,
#241029,#241030,#241031,#241032,#241033,#241034,#241035,#241036,#241037,
#241038,#241039,#241040,#241041),.UNSPECIFIED.,.F.,.F.,(4,2,2,2,2,2,2,2,
2,2,2,2,2,2,2,2,2,4),(21.0091763975789,21.0318031777429,21.1113724869712,
21.1887685156285,21.2661013080159,21.3455850694411,21.4220800230878,21.5022024880104,
21.580619931206,21.6565512470235,21.7360667361565,21.8136208238973,21.8904995412877,
21.970166027991,22.0468243300758,22.1261485322222,22.2047741711635,22.2691796383917),
 .UNSPECIFIED.);
#6088=B_SPLINE_CURVE_WITH_KNOTS('',3,(#241042,#241043,#241044,#241045,#241046,
#241047,#241048,#241049,#241050,#241051,#241052,#241053,#241054,#241055,
#241056,#241057,#241058,#241059,#241060,#241061,#241062,#241063,#241064,
#241065,#241066,#241067,#241068,#241069,#241070,#241071,#241072,#241073,
#241074,#241075,#241076,#241077),.UNSPECIFIED.,.F.,.F.,(4,2,2,2,2,2,2,2,
2,2,2,2,2,2,2,2,2,4),(1.54965533150543,1.6191810954755,1.69808920760654,
1.77686898372047,1.85377197718216,1.93370558140581,2.01033884039764,2.08813696215977,
2.1677050397341,2.24367700877286,2.32233530521275,2.40184177204162,2.47853762445349,
2.55824105027393,2.63524770661228,2.71284064966069,2.79242948533891,2.81051496707889),
 .UNSPECIFIED.);
#6089=B_SPLINE_CURVE_WITH_KNOTS('',3,(#241082,#241083,#241084,#241085,#241086,
#241087,#241088,#241089,#241090,#241091,#241092,#241093,#241094,#241095,
#241096,#241097,#241098,#241099,#241100,#241101,#241102,#241103,#241104,
#241105,#241106,#241107,#241108,#241109,#241110,#241111,#241112,#241113,
#241114,#241115,#241116,#241117),.UNSPECIFIED.,.F.,.F.,(4,2,2,2,2,2,2,2,
2,2,2,2,2,2,2,2,2,4),(19.7477505345541,19.7819394034219,19.8619634678305,
19.9389481080936,20.0175033641031,20.0965069290084,20.1726312691743,20.2522365031935,
20.3303870326243,20.4067119579603,20.4870317747689,20.5642843143553,20.6422849545906,
20.7215935067328,20.7979329433488,20.8774748285065,20.9557388752909,21.0091763975789),
 .UNSPECIFIED.);
#6090=B_SPLINE_CURVE_WITH_KNOTS('',3,(#241118,#241119,#241120,#241121,#241122,
#241123,#241124,#241125,#241126,#241127,#241128,#241129,#241130,#241131,
#241132,#241133,#241134,#241135,#241136,#241137,#241138,#241139,#241140,
#241141,#241142,#241143,#241144,#241145,#241146,#241147,#241148,#241149,
#241150,#241151,#241152,#241153),.UNSPECIFIED.,.F.,.F.,(4,2,2,2,2,2,2,2,
2,2,2,2,2,2,2,2,2,4),(2.81051496707889,2.86843861292801,2.94689632536739,
3.02721101822537,3.1037514070629,3.18328064150779,3.26075337113605,3.33819671505569,
3.41784506617566,3.49400238700364,3.57231522265173,3.65193423432565,3.72832380273608,
3.80768284665575,3.88584597194112,3.96315144920267,4.04352381654236,4.07266414291054),
 .UNSPECIFIED.);
#6091=B_SPLINE_CURVE_WITH_KNOTS('',3,(#241158,#241159,#241160,#241161,#241162,
#241163,#241164,#241165,#241166,#241167,#241168,#241169,#241170,#241171,
#241172,#241173,#241174,#241175,#241176,#241177,#241178,#241179,#241180,
#241181,#241182,#241183,#241184,#241185,#241186,#241187,#241188,#241189,
#241190,#241191,#241192,#241193),.UNSPECIFIED.,.F.,.F.,(4,2,2,2,2,2,2,2,
2,2,2,2,2,2,2,2,2,4),(18.4868313729185,18.5326534242109,18.6122352945202,
18.6888224014101,18.7688514808402,18.8473715865055,18.9233535675701,19.002930020034,
19.0805869298598,19.1574519297428,19.2372278940146,19.3139888393418,19.3932326930507,
19.4719711381632,19.5479587690643,19.6275283739101,19.7054083287184,19.7477505345541),
 .UNSPECIFIED.);
#6092=B_SPLINE_CURVE_WITH_KNOTS('',3,(#241194,#241195,#241196,#241197,#241198,
#241199,#241200,#241201,#241202,#241203,#241204,#241205,#241206,#241207,
#241208,#241209,#241210,#241211,#241212,#241213,#241214,#241215,#241216,
#241217,#241218,#241219,#241220,#241221,#241222,#241223,#241224,#241225,
#241226,#241227,#241228,#241229),.UNSPECIFIED.,.F.,.F.,(4,2,2,2,2,2,2,2,
2,2,2,2,2,2,2,2,2,4),(4.07266414291054,4.11996124283415,4.19816525237173,
4.27785857376779,4.35404733303679,4.43310623910865,4.51184517608608,4.58888829036109,
4.6689708373675,4.74563347273896,4.82357284926374,4.90323666539291,4.97930718285682,
5.05810677448008,5.13755120139774,5.2143770041859,5.29421835227979,5.33520243665533),
 .UNSPECIFIED.);
#6093=B_SPLINE_CURVE_WITH_KNOTS('',3,(#241234,#241235,#241236,#241237,#241238,
#241239,#241240,#241241,#241242,#241243,#241244,#241245,#241246,#241247,
#241248,#241249,#241250,#241251,#241252,#241253,#241254,#241255,#241256,
#241257,#241258,#241259,#241260,#241261,#241262,#241263,#241264,#241265,
#241266,#241267,#241268,#241269),.UNSPECIFIED.,.F.,.F.,(4,2,2,2,2,2,2,2,
2,2,2,2,2,2,2,2,2,4),(17.2247319659337,17.283183116068,17.3622710832688,
17.438464650737,17.518111489222,17.5963472698658,17.6726771747172,17.7530878399949,
17.8304244991097,17.9083665824597,17.9877665213978,18.0641918344984,18.1437899655652,
18.222145378313,18.2982398577519,18.3778627113094,18.4553503172739,18.4868313729185),
 .UNSPECIFIED.);
#6094=B_SPLINE_CURVE_WITH_KNOTS('',3,(#241270,#241271,#241272,#241273,#241274,
#241275,#241276,#241277,#241278,#241279,#241280,#241281,#241282,#241283,
#241284,#241285,#241286,#241287,#241288,#241289,#241290,#241291,#241292,
#241293,#241294,#241295,#241296,#241297,#241298,#241299,#241300,#241301,
#241302,#241303,#241304,#241305),.UNSPECIFIED.,.F.,.F.,(4,2,2,2,2,2,2,2,
2,2,2,2,2,2,2,2,2,4),(5.33520243665533,5.37123175487558,5.44895499788664,
5.52863136770331,5.60471386189317,5.68330197566796,5.76354258712913,5.84020175081883,
5.91985679742295,5.99732069529608,6.07488238510482,6.15461057457674,6.23082057603543,
6.30925179094805,6.38895324573563,6.46545480897963,6.54493239908358,6.59826968210442),
 .UNSPECIFIED.);
#6095=B_SPLINE_CURVE_WITH_KNOTS('',3,(#241310,#241311,#241312,#241313,#241314,
#241315,#241316,#241317,#241318,#241319,#241320,#241321,#241322,#241323,
#241324,#241325,#241326,#241327,#241328,#241329,#241330,#241331,#241332,
#241333,#241334,#241335,#241336,#241337,#241338,#241339,#241340,#241341,
#241342,#241343,#241344,#241345),.UNSPECIFIED.,.F.,.F.,(4,2,2,2,2,2,2,2,
2,2,2,2,2,2,2,2,2,4),(15.9633759832345,16.0340829053594,16.1126697840488,
16.1886716274734,16.2682734445992,16.3459976665135,16.4228191552351,16.5026679549044,
16.5794962911535,16.6586307779,16.7374454828078,16.8134771903943,16.893079940854,
16.9710367863344,17.0475471941891,17.1276537050312,17.2047146217245,17.2247319659337),
 .UNSPECIFIED.);
#6096=B_SPLINE_CURVE_WITH_KNOTS('',3,(#241346,#241347,#241348,#241349,#241350,
#241351,#241352,#241353,#241354,#241355,#241356,#241357,#241358,#241359,
#241360,#241361,#241362,#241363,#241364,#241365,#241366,#241367,#241368,
#241369,#241370,#241371,#241372,#241373,#241374,#241375,#241376,#241377,
#241378,#241379,#241380,#241381),.UNSPECIFIED.,.F.,.F.,(4,2,2,2,2,2,2,2,
2,2,2,2,2,2,2,2,2,4),(6.59826968210442,6.62305723184909,6.70047303463833,
6.78096354367303,6.85742750785752,6.93574323524729,7.01550404527384,7.09178510173153,
7.17095517546818,7.24962779957794,7.32677300079539,7.40696484447098,7.48362817734374,
7.5616704738598,7.64139323350021,7.71753027422718,7.79643244085222,7.86199738742149),
 .UNSPECIFIED.);
#6097=B_SPLINE_CURVE_WITH_KNOTS('',3,(#241386,#241387,#241388,#241389,#241390,
#241391,#241392,#241393,#241394,#241395,#241396,#241397,#241398,#241399,
#241400,#241401,#241402,#241403,#241404,#241405,#241406,#241407,#241408,
#241409,#241410,#241411,#241412,#241413,#241414,#241415,#241416,#241417,
#241418,#241419,#241420,#241421,#241422,#241423),.UNSPECIFIED.,.F.,.F.,
(4,2,2,2,2,2,2,2,2,2,2,2,2,2,2,2,2,2,4),(14.701099149603,14.7034557678201,
14.7831089134017,14.8613951944832,14.9376995229283,15.0181652998994,15.0955516706383,
15.1734044319978,15.2528602486155,15.3293372297621,15.4089563152068,15.4873678151406,
15.5634613867607,15.6431023180422,15.7206465816924,15.7978892940474,15.8775332564797,
15.9541778414377,15.9633759832345),.UNSPECIFIED.);
#6098=B_SPLINE_CURVE_WITH_KNOTS('',3,(#241424,#241425,#241426,#241427,#241428,
#241429,#241430,#241431,#241432,#241433,#241434,#241435,#241436,#241437,
#241438,#241439,#241440,#241441,#241442,#241443,#241444,#241445,#241446,
#241447,#241448,#241449,#241450,#241451,#241452,#241453,#241454,#241455,
#241456,#241457,#241458,#241459),.UNSPECIFIED.,.F.,.F.,(4,2,2,2,2,2,2,2,
2,2,2,2,2,2,2,2,2,4),(7.86199738742149,7.87578870684037,7.95270729700455,
8.03264787424434,8.10963942101754,8.18745556104782,8.26718301070552,8.34330764872676,
8.42198839637052,8.50212736795937,8.57886900849719,8.6586121098341,8.73603794343607,
8.81368146932958,8.89345336931947,8.96968497119851,9.04819771303439,9.12550391178119),
 .UNSPECIFIED.);
#6099=B_SPLINE_CURVE_WITH_KNOTS('',3,(#241464,#241465,#241466,#241467,#241468,
#241469,#241470,#241471,#241472,#241473,#241474,#241475,#241476,#241477,
#241478,#241479,#241480,#241481,#241482,#241483,#241484,#241485,#241486,
#241487,#241488,#241489,#241490,#241491,#241492,#241493,#241494,#241495,
#241496,#241497,#241498,#241499),.UNSPECIFIED.,.F.,.F.,(4,2,2,2,2,2,2,2,
2,2,2,2,2,2,2,2,2,4),(13.4396934393828,13.4536847447015,13.5332763419421,
13.6110337656732,13.6877798940162,13.7676664530154,13.8445283476067,13.9235200048667,
14.0023761148105,14.0784213926254,14.1580218413539,14.236021157819,14.3124798944769,
14.3926334525682,14.4697365270538,14.5480864601419,14.6272236300065,14.701099149603),
 .UNSPECIFIED.);
#6100=B_SPLINE_CURVE_WITH_KNOTS('',3,(#241500,#241501,#241502,#241503,#241504,
#241505,#241506,#241507,#241508,#241509,#241510,#241511,#241512,#241513,
#241514,#241515,#241516,#241517,#241518,#241519,#241520,#241521,#241522,
#241523,#241524,#241525,#241526,#241527,#241528,#241529,#241530,#241531,
#241532,#241533,#241534,#241535,#241536,#241537),.UNSPECIFIED.,.F.,.F.,
(4,2,2,2,2,2,2,2,2,2,2,2,2,2,2,2,2,2,4),(9.12550391178119,9.12794562854735,
9.20452353347352,9.28408260990182,9.36214053189483,9.43963086875648,9.52020226565107,
9.59666281547,9.67505411358347,9.75177793909778,9.83235205988809,9.91099486481556,
9.98720176193357,10.0669933113407,10.1447688600247,10.221998524202,10.3018881334216,
10.378764057835,10.3900588862096),.UNSPECIFIED.);
#6101=B_SPLINE_CURVE_WITH_KNOTS('',3,(#241542,#241543,#241544,#241545,#241546,
#241547,#241548,#241549,#241550,#241551,#241552,#241553,#241554,#241555,
#241556,#241557,#241558,#241559,#241560,#241561,#241562,#241563,#241564,
#241565,#241566,#241567,#241568,#241569,#241570,#241571,#241572,#241573,
#241574,#241575,#241576,#241577),.UNSPECIFIED.,.F.,.F.,(4,2,2,2,2,2,2,2,
2,2,2,2,2,2,2,2,2,4),(12.1779611485506,12.2029615970869,12.2834477046188,
12.3608501882395,12.4385791971972,12.5180563732016,12.5945516971524,12.6741562699566,
12.7525895879676,12.8286503860145,12.9082736895974,12.9858407333286,13.0629895967305,
13.1426608362597,13.2193293058411,13.2990748665947,13.3776939963258,13.4396934393828),
 .UNSPECIFIED.);
#6102=B_SPLINE_CURVE_WITH_KNOTS('',3,(#241578,#241579,#241580,#241581,#241582,
#241583,#241584,#241585,#241586,#241587,#241588,#241589,#241590,#241591,
#241592,#241593,#241594,#241595,#241596,#241597,#241598,#241599,#241600,
#241601,#241602,#241603,#241604,#241605,#241606,#241607,#241608,#241609,
#241610,#241611,#241612,#241613),.UNSPECIFIED.,.F.,.F.,(4,2,2,2,2,2,2,2,
2,2,2,2,2,2,2,2,2,4),(10.3900588862096,10.4585239664231,10.5373641952025,
10.613525477726,10.6932934610687,10.7712710279127,10.8481188279578,10.9282355033061,
11.0053156823111,11.0843400095939,11.163427504345,11.2396707996032,11.3194564691121,
11.3976863806327,11.4742726349846,11.5546668407259,11.6319979505454,11.6542522257011),
 .UNSPECIFIED.);
#6103=B_SPLINE_CURVE_WITH_KNOTS('',3,(#241618,#241619,#241620,#241621,#241622,
#241623,#241624,#241625,#241626,#241627,#241628,#241629,#241630,#241631,
#241632,#241633,#241634,#241635,#241636,#241637,#241638,#241639,#241640,
#241641,#241642,#241643,#241644,#241645,#241646,#241647,#241648,#241649,
#241650,#241651,#241652,#241653),.UNSPECIFIED.,.F.,.F.,(4,2,2,2,2,2,2,2,
2,2,2,2,2,2,2,2,2,4),(10.9168245999786,10.9535273517243,11.0334169764488,
11.1102788663099,11.1890887960723,11.26795195487,11.3439801294688,11.4235418699849,
11.5015497913461,11.5779234924823,11.6580893856383,11.7352010537127,11.8133960223397,
11.8925479562904,11.968788588237,12.048412096038,12.1267149477204,12.1779611485506),
 .UNSPECIFIED.);
#6104=B_SPLINE_CURVE_WITH_KNOTS('',3,(#241654,#241655,#241656,#241657,#241658,
#241659,#241660,#241661,#241662,#241663,#241664,#241665,#241666,#241667,
#241668,#241669,#241670,#241671,#241672,#241673,#241674,#241675,#241676,
#241677,#241678,#241679,#241680,#241681,#241682,#241683,#241684,#241685,
#241686,#241687,#241688,#241689),.UNSPECIFIED.,.F.,.F.,(4,2,2,2,2,2,2,2,
2,2,2,2,2,2,2,2,2,4),(11.6542522257011,11.710407002519,11.7897844888648,
11.8662421728206,11.9460902634938,12.0246163526226,12.1010766272691,12.1817923681703,
12.2594155071029,12.3373589223573,12.4170629140417,12.4937764276779,12.5736063166663,
12.6522635035179,12.7285386772514,12.8083871849551,12.886175686978,12.9197561116359),
 .UNSPECIFIED.);
#6105=B_SPLINE_CURVE_WITH_KNOTS('',3,(#241694,#241695,#241696,#241697,#241698,
#241699,#241700,#241701,#241702,#241703,#241704,#241705,#241706,#241707,
#241708,#241709,#241710,#241711,#241712,#241713,#241714,#241715,#241716,
#241717,#241718,#241719,#241720,#241721,#241722,#241723,#241724,#241725,
#241726,#241727,#241728,#241729),.UNSPECIFIED.,.F.,.F.,(4,2,2,2,2,2,2,2,
2,2,2,2,2,2,2,2,2,4),(9.65613189117811,9.70510400601994,9.78456788722448,
9.86104801334814,9.94060117886638,10.0190219155385,10.0950163875207,10.1745848390524,
10.2521407022053,10.329158445023,10.4088221904792,10.4854809063298,10.5650253891295,
10.6436424495944,10.7195901998136,10.7991347429344,10.8768915098314,10.9168245999786),
 .UNSPECIFIED.);
#6106=B_SPLINE_CURVE_WITH_KNOTS('',3,(#241730,#241731,#241732,#241733,#241734,
#241735,#241736,#241737,#241738,#241739,#241740,#241741,#241742,#241743,
#241744,#241745,#241746,#241747,#241748,#241749,#241750,#241751,#241752,
#241753,#241754,#241755,#241756,#241757,#241758,#241759,#241760,#241761,
#241762,#241763,#241764,#241765),.UNSPECIFIED.,.F.,.F.,(4,2,2,2,2,2,2,2,
2,2,2,2,2,2,2,2,2,4),(12.9197561116359,12.9635388590835,13.0434377626046,
13.1203251920892,13.2002890507829,13.2791331064625,13.3553391645683,13.4351562582792,
13.5131362104416,13.5900964960459,13.6702118626848,13.7472937576194,13.8265024709751,
13.9055846424562,13.9818466592195,14.0616730390502,14.1398960400751,14.1845909974411),
 .UNSPECIFIED.);
#6107=B_SPLINE_CURVE_WITH_KNOTS('',3,(#241770,#241771,#241772,#241773,#241774,
#241775,#241776,#241777,#241778,#241779,#241780,#241781,#241782,#241783,
#241784,#241785,#241786,#241787,#241788,#241789,#241790,#241791,#241792,
#241793,#241794,#241795,#241796,#241797,#241798,#241799,#241800,#241801,
#241802,#241803,#241804,#241805),.UNSPECIFIED.,.F.,.F.,(4,2,2,2,2,2,2,2,
2,2,2,2,2,2,2,2,2,4),(8.39571461391817,8.45407111577228,8.53244461553089,
8.6125792647267,8.6890336707027,8.76847463807125,8.84580191678438,8.92315742029522,
9.00269660548283,9.07873856353393,9.15696198687568,9.23647302573939,9.31277379135651,
9.39204156144936,9.47004475002984,9.54725898117665,9.62753801892365,9.65613189117811),
 .UNSPECIFIED.);
#6108=B_SPLINE_CURVE_WITH_KNOTS('',3,(#241806,#241807,#241808,#241809,#241810,
#241811,#241812,#241813,#241814,#241815,#241816,#241817,#241818,#241819,
#241820,#241821,#241822,#241823,#241824,#241825,#241826,#241827,#241828,
#241829,#241830,#241831,#241832,#241833,#241834,#241835,#241836,#241837,
#241838,#241839,#241840,#241841),.UNSPECIFIED.,.F.,.F.,(4,2,2,2,2,2,2,2,
2,2,2,2,2,2,2,2,2,4),(14.1845909974411,14.2165693414243,14.2969529355151,
14.3742771308546,14.4528435761911,14.5322079993234,14.6086586834019,14.6885383554083,
14.7670495417927,14.8435693412187,14.9242664485727,15.0018751272443,15.0799445063026,
15.1596288186321,15.2363256200211,15.3161718844887,15.3948089191141,15.4504769545923),
 .UNSPECIFIED.);
#6109=B_SPLINE_CURVE_WITH_KNOTS('',3,(#241846,#241847,#241848,#241849,#241850,
#241851,#241852,#241853,#241854,#241855,#241856,#241857,#241858,#241859,
#241860,#241861,#241862,#241863,#241864,#241865,#241866,#241867,#241868,
#241869,#241870,#241871,#241872,#241873,#241874,#241875,#241876,#241877,
#241878,#241879,#241880,#241881),.UNSPECIFIED.,.F.,.F.,(4,2,2,2,2,2,2,2,
2,2,2,2,2,2,2,2,2,4),(7.13646531059583,7.20645785952193,7.28529023825674,
7.36390735835512,7.44073341990602,7.52058854397155,7.59709484904002,7.67481490273967,
7.75428113144242,7.83015861471465,7.90873729764548,7.98807040244311,8.06468506885083,
8.14430541451292,8.2211743405915,8.29868460094256,8.37816785133338,8.39571461391817),
 .UNSPECIFIED.);
#6110=B_SPLINE_CURVE_WITH_KNOTS('',3,(#241882,#241883,#241884,#241885,#241886,
#241887,#241888,#241889,#241890,#241891,#241892,#241893,#241894,#241895,
#241896,#241897,#241898,#241899,#241900,#241901,#241902,#241903,#241904,
#241905,#241906,#241907,#241908,#241909,#241910,#241911,#241912,#241913,
#241914,#241915,#241916,#241917),.UNSPECIFIED.,.F.,.F.,(4,2,2,2,2,2,2,2,
2,2,2,2,2,2,2,2,2,4),(15.4504769545923,15.4711186088728,15.5509866302239,
15.6287539943615,15.7062130664185,15.7860863660806,15.8629515346015,15.9430772952779,
16.0218907399634,16.0981095094446,16.1779386748971,16.2558870405988,16.3329245748492,
16.4130038296978,16.4900537660969,16.5694075427569,16.6484499320012,16.7154590663106),
 .UNSPECIFIED.);
#6111=B_SPLINE_CURVE_WITH_KNOTS('',3,(#241922,#241923,#241924,#241925,#241926,
#241927,#241928,#241929,#241930,#241931,#241932,#241933,#241934,#241935,
#241936,#241937,#241938,#241939,#241940,#241941,#241942,#241943,#241944,
#241945,#241946,#241947,#241948,#241949,#241950,#241951,#241952,#241953,
#241954,#241955,#241956,#241957,#241958,#241959),.UNSPECIFIED.,.F.,.F.,
(4,2,2,2,2,2,2,2,2,2,2,2,2,2,2,2,2,2,4),(5.87566374904269,5.88157874395125,
5.95808562271841,6.03757865154077,6.11509465883298,6.19250524853729,6.2721444610133,
6.34830821943425,6.42658870612222,6.50614928028767,6.58236422400605,6.66149176274634,
6.73951849537886,6.81660152826874,6.89674065773059,6.97300750773828,7.05098645673024,
7.13047725888505,7.13646531059583),.UNSPECIFIED.);
#6112=B_SPLINE_CURVE_WITH_KNOTS('',3,(#241960,#241961,#241962,#241963,#241964,
#241965,#241966,#241967,#241968,#241969,#241970,#241971,#241972,#241973,
#241974,#241975,#241976,#241977,#241978,#241979,#241980,#241981,#241982,
#241983,#241984,#241985,#241986,#241987,#241988,#241989,#241990,#241991,
#241992,#241993,#241994,#241995,#241996,#241997),.UNSPECIFIED.,.F.,.F.,
(4,2,2,2,2,2,2,2,2,2,2,2,2,2,2,2,2,2,4),(16.7154590663106,16.7246998818893,
16.8045303784101,16.8827125049289,16.9594392487068,17.0397774247768,17.1170610444518,
17.195748111439,17.2750649428163,17.3514784766028,17.4313536164282,17.509815885501,
17.5863629146892,17.6670065264203,17.744567061855,17.8227276640817,17.9023577000694,
17.9790043840932,17.9812155694434),.UNSPECIFIED.);
#6113=B_SPLINE_CURVE_WITH_KNOTS('',3,(#242002,#242003,#242004,#242005,#242006,
#242007,#242008,#242009,#242010,#242011,#242012,#242013,#242014,#242015,
#242016,#242017,#242018,#242019,#242020,#242021,#242022,#242023,#242024,
#242025,#242026,#242027,#242028,#242029,#242030,#242031,#242032,#242033,
#242034,#242035,#242036,#242037),.UNSPECIFIED.,.F.,.F.,(4,2,2,2,2,2,2,2,
2,2,2,2,2,2,2,2,2,4),(4.61497841375817,4.63217000394447,4.70906659679136,
4.78899393182726,4.86560768946728,4.94339927105396,5.02295495299878,5.09891572879304,
5.17756723650798,5.2570426907455,5.33373099645916,5.41342691260482,5.49041135868395,
5.56799652190477,5.64757199748644,5.72356699798226,5.80201668627962,5.87566374904269),
 .UNSPECIFIED.);
#6114=B_SPLINE_CURVE_WITH_KNOTS('',3,(#242038,#242039,#242040,#242041,#242042,
#242043,#242044,#242045,#242046,#242047,#242048,#242049,#242050,#242051,
#242052,#242053,#242054,#242055,#242056,#242057,#242058,#242059,#242060,
#242061,#242062,#242063,#242064,#242065,#242066,#242067,#242068,#242069,
#242070,#242071,#242072,#242073),.UNSPECIFIED.,.F.,.F.,(4,2,2,2,2,2,2,2,
2,2,2,2,2,2,2,2,2,4),(17.9812155694434,18.0588314147492,18.1374139506599,
18.2137261374055,18.2935778201302,18.3712900944934,18.4488113528749,18.5286241637414,
18.6054334063077,18.6856852076825,18.7644334583262,18.8406338650887,18.9204393841381,
18.9983219952603,19.0754047258784,19.1554127395687,19.2323968287287,19.2459664568064),
 .UNSPECIFIED.);
#6115=B_SPLINE_CURVE_WITH_KNOTS('',3,(#242078,#242079,#242080,#242081,#242082,
#242083,#242084,#242085,#242086,#242087,#242088,#242089,#242090,#242091,
#242092,#242093,#242094,#242095,#242096,#242097,#242098,#242099,#242100,
#242101,#242102,#242103,#242104,#242105,#242106,#242107,#242108,#242109,
#242110,#242111,#242112,#242113),.UNSPECIFIED.,.F.,.F.,(4,2,2,2,2,2,2,2,
2,2,2,2,2,2,2,2,2,4),(3.35320138787495,3.3812638703186,3.45870958005293,
3.53924251659103,3.61549479037889,3.6938415306858,3.77348545760913,3.84976616653828,
3.92896139623998,4.00711204191994,4.08426294194264,4.164471424109,4.24083643470692,
4.31888403362048,4.39846134862252,4.47451624184274,4.55341862304842,4.61497841375817),
 .UNSPECIFIED.);
#6116=B_SPLINE_CURVE_WITH_KNOTS('',3,(#242114,#242115,#242116,#242117,#242118,
#242119,#242120,#242121,#242122,#242123,#242124,#242125,#242126,#242127,
#242128,#242129,#242130,#242131,#242132,#242133,#242134,#242135,#242136,
#242137,#242138,#242139,#242140,#242141,#242142,#242143,#242144,#242145,
#242146,#242147,#242148,#242149),.UNSPECIFIED.,.F.,.F.,(4,2,2,2,2,2,2,2,
2,2,2,2,2,2,2,2,2,4),(19.2459664568064,19.311861864962,19.3908295702844,
19.4670368686963,19.5468359152358,19.6249427044891,19.7016916993731,19.7819490198206,
19.8591579029915,19.9379334922596,20.0171674984929,20.0935131839074,20.1733483901513,
20.2517269610892,20.3282705175368,20.4088248715252,20.4863028260136,20.5108796016852),
 .UNSPECIFIED.);
#6117=B_SPLINE_CURVE_WITH_KNOTS('',3,(#242154,#242155,#242156,#242157,#242158,
#242159,#242160,#242161,#242162,#242163,#242164,#242165,#242166,#242167,
#242168,#242169,#242170,#242171,#242172,#242173,#242174,#242175,#242176,
#242177,#242178,#242179,#242180,#242181,#242182,#242183,#242184,#242185,
#242186,#242187,#242188,#242189),.UNSPECIFIED.,.F.,.F.,(4,2,2,2,2,2,2,2,
2,2,2,2,2,2,2,2,2,4),(2.09124089524434,2.1306490107864,2.20845837087744,
2.28808039431898,2.36410071092841,2.44277166696175,2.52247191422365,2.59918710644569,
2.67890818519645,2.75604429529321,2.83365794816793,2.91330787937623,2.98938692491842,
3.06786674749038,3.14749960455273,3.2240388295728,3.30356283068734,3.35320138787495),
 .UNSPECIFIED.);
#6118=B_SPLINE_CURVE_WITH_KNOTS('',3,(#242190,#242191,#242192,#242193,#242194,
#242195,#242196,#242197,#242198,#242199,#242200,#242201,#242202,#242203,
#242204,#242205,#242206,#242207,#242208,#242209,#242210,#242211,#242212,
#242213,#242214,#242215,#242216,#242217,#242218,#242219,#242220,#242221,
#242222,#242223,#242224,#242225),.UNSPECIFIED.,.F.,.F.,(4,2,2,2,2,2,2,2,
2,2,2,2,2,2,2,2,2,4),(20.5108796016852,20.5645236332566,20.644063861161,
20.720626194123,20.8003986187961,20.878891356537,20.9551748472087,21.0349746409647,
21.1125968876481,21.190149416361,21.2698657094522,21.346584335433,21.4269312331983,
21.5055783974057,21.5817295613149,21.6614757641737,21.7392571101579,21.7750720110093),
 .UNSPECIFIED.);
#6119=B_SPLINE_CURVE_WITH_KNOTS('',3,(#242231,#242232,#242233,#242234,#242235,
#242236,#242237,#242238,#242239,#242240,#242241,#242242,#242243,#242244,
#242245,#242246,#242247,#242248,#242249,#242250,#242251,#242252,#242253,
#242254,#242255,#242256),.UNSPECIFIED.,.F.,.F.,(4,2,2,2,2,2,2,2,2,2,2,2,
4),(0.00950822744729325,0.0410482442676837,0.0835736901067871,0.162757220120456,
0.241102173023232,0.318248671367356,0.398448377125879,0.474921972698114,
0.552965181657624,0.632596307645776,0.708676431490648,0.749696686020115,
0.790626617481797),.UNSPECIFIED.);
#6120=B_SPLINE_CURVE_WITH_KNOTS('',3,(#242258,#242259,#242260,#242261,#242262,
#242263),.UNSPECIFIED.,.F.,.F.,(4,2,4),(9.99824055476731E-7,0.0243498221505662,
0.0486954662228403),.UNSPECIFIED.);
#6121=B_SPLINE_CURVE_WITH_KNOTS('',3,(#242264,#242265,#242266,#242267,#242268,
#242269,#242270,#242271,#242272,#242273,#242274,#242275,#242276,#242277,
#242278,#242279,#242280,#242281,#242282,#242283,#242284,#242285,#242286,
#242287,#242288,#242289),.UNSPECIFIED.,.F.,.F.,(4,2,2,2,2,2,2,2,2,2,2,2,
4),(1.00000007505208E-6,0.0481217371548365,0.0975555807269073,0.177241325850779,
0.253369517923901,0.331844467981179,0.411509871161699,0.488047266994232,
0.567566980440415,0.645410620509902,0.722856893712002,0.803386711797282,
0.828975078082139),.UNSPECIFIED.);
#6122=B_SPLINE_CURVE_WITH_KNOTS('',3,(#242299,#242300,#242301,#242302,#242303,
#242304),.UNSPECIFIED.,.F.,.F.,(4,2,4),(1.00000004082002E-6,0.0254438039575916,
0.0520246360988654),.UNSPECIFIED.);
#6123=B_SPLINE_CURVE_WITH_KNOTS('',3,(#242321,#242322,#242323,#242324,#242325,
#242326,#242327,#242328,#242329,#242330,#242331,#242332),.UNSPECIFIED.,
 .F.,.F.,(4,2,2,2,2,4),(1.00000007766482E-6,0.0445461052973873,0.0896481038803835,
0.134464834369227,0.140040820732742,0.179234915771338),.UNSPECIFIED.);
#6124=B_SPLINE_CURVE_WITH_KNOTS('',3,(#242853,#242854,#242855,#242856,#242857,
#242858),.UNSPECIFIED.,.F.,.F.,(4,2,4),(-0.052023619808277,-0.0259934271027802,
-1.00000004377848E-6),.UNSPECIFIED.);
#6125=B_SPLINE_CURVE_WITH_KNOTS('',3,(#242875,#242876,#242877,#242878,#242879,
#242880,#242881,#242882,#242883,#242884,#242885,#242886),.UNSPECIFIED.,
 .F.,.F.,(4,2,2,2,2,4),(-0.17929919968084,-0.134583984746606,-0.0896249144840832,
-0.0448429285044394,-0.0392636416192798,-1.00000009822798E-6),
 .UNSPECIFIED.);
#6126=B_SPLINE_CURVE_WITH_KNOTS('',3,(#243428,#243429,#243430,#243431,#243432,
#243433,#243434,#243435,#243436,#243437,#243438,#243439,#243440,#243441,
#243442,#243443,#243444,#243445,#243446,#243447,#243448,#243449,#243450,
#243451,#243452,#243453,#243454,#243455,#243456,#243457,#243458,#243459,
#243460,#243461,#243462,#243463,#243464,#243465,#243466,#243467),
 .UNSPECIFIED.,.F.,.F.,(4,3,3,3,3,3,3,3,3,3,3,3,3,4),(1.96246868729215E-28,
0.000438443356248491,0.00067092441681323,0.00110918484354966,0.00134856915744274,
0.00189097627470433,0.00203013834973696,0.00270986824049021,0.00271266901570489,
0.00339379571613445,0.00406480236073532,0.00407250537600557,0.00481439427282875,
0.00541973648098043),.UNSPECIFIED.);
#6127=B_SPLINE_CURVE_WITH_KNOTS('',3,(#243475,#243476,#243477,#243478,#243479,
#243480,#243481,#243482,#243483,#243484,#243485,#243486,#243487,#243488,
#243489,#243490,#243491,#243492,#243493,#243494,#243495,#243496,#243497,
#243498,#243499,#243500,#243501,#243502,#243503,#243504,#243505,#243506,
#243507,#243508,#243509,#243510,#243511,#243512,#243513,#243514,#243515,
#243516,#243517),.UNSPECIFIED.,.F.,.F.,(4,3,3,3,3,3,3,3,3,3,3,3,3,3,4),
(0.,0.000627149038362586,0.0012879482962516,0.00134802948058203,0.00135592142842901,
0.00202680625468173,0.00270776094006554,0.00271184285685801,0.00338988085637128,
0.0039809874146687,0.00407131269878862,0.00454781218229871,0.00474992819159083,
0.00522421399683384,0.00542368571371602),.UNSPECIFIED.);
#6128=B_SPLINE_CURVE_WITH_KNOTS('',3,(#243560,#243561,#243562,#243563,#243564,
#243565,#243566,#243567,#243568,#243569,#243570,#243571,#243572,#243573),
 .UNSPECIFIED.,.F.,.F.,(4,2,2,2,2,2,4),(-0.31539760291967,-0.309659972902578,
-0.305224290839027,-0.30075945665783,-0.294897994554676,-0.282601216297714,
-0.259650109440469),.UNSPECIFIED.);
#6129=B_SPLINE_CURVE_WITH_KNOTS('',3,(#243577,#243578,#243579,#243580,#243581,
#243582),.UNSPECIFIED.,.F.,.F.,(4,2,4),(0.,0.000518432414188003,0.00103686532124488),
 .UNSPECIFIED.);
#6130=B_SPLINE_CURVE_WITH_KNOTS('',3,(#243584,#243585,#243586,#243587,#243588,
#243589),.UNSPECIFIED.,.F.,.F.,(4,2,4),(0.,0.0400464786590225,0.088560968632653),
 .UNSPECIFIED.);
#6131=B_SPLINE_CURVE_WITH_KNOTS('',3,(#243591,#243592,#243593,#243594,#243595,
#243596,#243597,#243598,#243599,#243600,#243601,#243602,#243603,#243604,
#243605,#243606,#243607,#243608,#243609,#243610,#243611,#243612,#243613,
#243614,#243615,#243616,#243617,#243618,#243619,#243620,#243621,#243622,
#243623,#243624,#243625,#243626,#243627,#243628,#243629,#243630,#243631,
#243632,#243633,#243634,#243635,#243636,#243637,#243638,#243639,#243640,
#243641,#243642,#243643,#243644,#243645,#243646,#243647,#243648,#243649,
#243650,#243651,#243652,#243653,#243654,#243655,#243656,#243657,#243658,
#243659,#243660,#243661,#243662,#243663,#243664,#243665,#243666,#243667,
#243668,#243669,#243670,#243671,#243672,#243673,#243674,#243675,#243676,
#243677,#243678,#243679,#243680,#243681,#243682,#243683,#243684,#243685,
#243686,#243687,#243688,#243689,#243690,#243691,#243692,#243693,#243694,
#243695,#243696,#243697,#243698,#243699,#243700,#243701,#243702,#243703,
#243704,#243705,#243706,#243707,#243708,#243709,#243710,#243711,#243712,
#243713,#243714,#243715,#243716,#243717,#243718,#243719,#243720,#243721,
#243722,#243723),.UNSPECIFIED.,.F.,.F.,(4,3,3,3,3,3,3,3,3,3,3,3,3,3,3,3,
3,3,3,3,3,3,3,3,3,3,3,3,3,3,3,3,3,3,3,3,3,3,3,3,3,3,3,3,4),(1.45587086745827E-6,
0.00205325642694755,0.00478261105644799,0.00781250000000508,0.00957936860333274,
0.0129445313449779,0.0156250000000102,0.0181089234731001,0.0234375000000152,
0.0286242003934857,0.0312500000000203,0.0384097547368286,0.0468750000000305,
0.05811776116225,0.0625000000000406,0.0751447560520765,0.0892613199263578,
0.0937500000000388,0.10683528115677,0.121344253798209,0.125000000000037,
0.145340107425858,0.151594249264444,0.170677873925115,0.187500000000033,
0.21121939936984,0.235769851684623,0.25000000000003,0.293640925185931,0.375000000000023,
0.437500000000023,0.465862845666036,0.49410987334067,0.500000000000023,
0.556532034001133,0.625000000000014,0.674164735985126,0.7249035415464,0.750000000000004,
0.8125,0.838218536984945,0.864879862610272,0.874999999999995,0.939619921550813,
1.),.UNSPECIFIED.);
#6132=B_SPLINE_CURVE_WITH_KNOTS('',3,(#243731,#243732,#243733,#243734,#243735,
#243736,#243737,#243738,#243739,#243740,#243741,#243742,#243743,#243744,
#243745,#243746,#243747,#243748,#243749,#243750,#243751,#243752,#243753,
#243754,#243755,#243756,#243757,#243758,#243759,#243760,#243761,#243762,
#243763,#243764,#243765,#243766,#243767,#243768,#243769,#243770,#243771,
#243772,#243773,#243774,#243775,#243776,#243777,#243778,#243779,#243780,
#243781,#243782,#243783,#243784,#243785,#243786,#243787,#243788,#243789,
#243790,#243791,#243792,#243793,#243794,#243795,#243796,#243797,#243798,
#243799,#243800),.UNSPECIFIED.,.F.,.F.,(4,3,3,3,3,3,3,3,3,3,3,3,3,3,3,3,
3,3,3,3,3,3,3,4),(0.,0.0625000000000169,0.125000000000034,0.250000000000057,
0.37500000000008,0.437500000000086,0.500000000000093,0.625000000000091,
0.687500000000086,0.750000000000081,0.781250000000077,0.812500000000074,
0.84375000000007,0.859375000000062,0.875000000000054,0.906250000000033,
0.921875000000018,0.937500000000004,0.953124999999989,0.960937499999993,
0.968749999999996,0.9765625,0.984375000000003,0.999999989277624),
 .UNSPECIFIED.);
#6133=B_SPLINE_CURVE_WITH_KNOTS('',3,(#243802,#243803,#243804,#243805,#243806,
#243807),.UNSPECIFIED.,.F.,.F.,(4,2,4),(0.,0.0364844625194263,0.0729123026181721),
 .UNSPECIFIED.);
#6134=B_SPLINE_CURVE_WITH_KNOTS('',3,(#243809,#243810,#243811,#243812,#243813,
#243814),.UNSPECIFIED.,.F.,.F.,(4,2,4),(0.,0.000518419907319716,0.00103683901965123),
 .UNSPECIFIED.);
#6135=B_SPLINE_CURVE_WITH_KNOTS('',3,(#243818,#243819,#243820,#243821,#243822,
#243823,#243824,#243825,#243826,#243827,#243828,#243829,#243830,#243831),
 .UNSPECIFIED.,.F.,.F.,(4,2,2,2,2,2,4),(-0.0557474934792282,-0.0327963866219729,
-0.020499608365005,-0.0146381462618493,-0.0101733120806503,-0.00573763001709685,
-1.87350135405495E-15),.UNSPECIFIED.);
#6136=B_SPLINE_CURVE_WITH_KNOTS('',3,(#243868,#243869,#243870,#243871,#243872,
#243873,#243874,#243875,#243876,#243877,#243878,#243879,#243880,#243881,
#243882,#243883,#243884,#243885),.UNSPECIFIED.,.F.,.F.,(4,2,2,2,2,2,2,2,
4),(-3.75036220066221,-3.57763083092397,-3.34575392115624,-3.06826697792209,
-2.79078003468794,-2.45898956740662,-2.29309433376597,-2.21014671694564,
-2.12719910012531),.UNSPECIFIED.);
#6137=B_SPLINE_CURVE_WITH_KNOTS('',3,(#243887,#243888,#243889,#243890,#243891,
#243892,#243893,#243894,#243895,#243896,#243897,#243898,#243899,#243900,
#243901,#243902,#243903,#243904),.UNSPECIFIED.,.F.,.F.,(4,2,2,2,2,2,2,2,
4),(-2.12719910012531,-2.0512596972242,-1.97532029432308,-1.82344148852086,
-1.51968387691641,-1.21823046919714,-0.916777061477878,-0.68747239865552,
-0.512363412091961),.UNSPECIFIED.);
#6138=B_SPLINE_CURVE_WITH_KNOTS('',3,(#244376,#244377,#244378,#244379,#244380,
#244381,#244382,#244383,#244384,#244385,#244386,#244387,#244388,#244389,
#244390,#244391,#244392,#244393,#244394,#244395,#244396,#244397,#244398,
#244399,#244400,#244401,#244402,#244403,#244404,#244405,#244406,#244407,
#244408,#244409,#244410,#244411,#244412,#244413,#244414,#244415,#244416,
#244417,#244418,#244419,#244420,#244421,#244422,#244423,#244424),
 .UNSPECIFIED.,.F.,.F.,(4,3,3,3,3,3,3,3,3,3,3,3,3,3,3,3,4),(0.670958968253536,
0.671875,0.6796875,0.6875,0.69140625,0.6953125,0.703125,0.71875,0.734375,
0.7421875,0.75,0.7578125,0.765625,0.7734375,0.78125,0.7890625,0.795736939319615),
 .UNSPECIFIED.);
#6139=B_SPLINE_CURVE_WITH_KNOTS('',3,(#244425,#244426,#244427,#244428,#244429,
#244430,#244431,#244432,#244433,#244434,#244435,#244436,#244437,#244438),
 .UNSPECIFIED.,.F.,.F.,(4,2,2,2,2,2,4),(9.86350491042899E-7,0.0393479876408068,
0.0757501092296844,0.0769070276303121,0.0792997502710887,0.115445556288863,
0.157977332025505),.UNSPECIFIED.);
#6140=B_SPLINE_CURVE_WITH_KNOTS('',3,(#244993,#244994,#244995,#244996,#244997,
#244998,#244999,#245000,#245001,#245002,#245003,#245004,#245005,#245006,
#245007,#245008,#245009,#245010,#245011,#245012,#245013,#245014,#245015,
#245016,#245017,#245018,#245019,#245020,#245021,#245022,#245023),
 .UNSPECIFIED.,.F.,.F.,(4,3,3,3,3,3,3,3,3,3,4),(0.106516886763067,0.107092942250384,
0.107670887972796,0.108254131185161,0.10884090238149,0.109435073327893,
0.109760614783791,0.110353705997288,0.110941670818037,0.111523726510257,
0.112049065484215),.UNSPECIFIED.);
#6141=B_SPLINE_CURVE_WITH_KNOTS('',3,(#245376,#245377,#245378,#245379,#245380,
#245381,#245382,#245383,#245384,#245385,#245386,#245387,#245388,#245389,
#245390,#245391,#245392,#245393,#245394,#245395,#245396,#245397,#245398,
#245399,#245400,#245401,#245402,#245403,#245404,#245405,#245406,#245407,
#245408,#245409,#245410,#245411,#245412,#245413,#245414,#245415,#245416,
#245417,#245418,#245419,#245420,#245421),.UNSPECIFIED.,.F.,.F.,(4,3,3,3,
3,3,3,3,3,3,3,3,3,3,3,4),(0.610561088386796,0.61718750038455,0.625,0.6328125,
0.640625,0.6484375,0.65625,0.671874995282168,0.679687492655973,0.6875,0.69140625,
0.6953125,0.703125,0.71875,0.734375,0.735482731103291),.UNSPECIFIED.);
#6142=B_SPLINE_CURVE_WITH_KNOTS('',3,(#245422,#245423,#245424,#245425,#245426,
#245427,#245428,#245429,#245430,#245431,#245432,#245433,#245434,#245435),
 .UNSPECIFIED.,.F.,.F.,(4,2,2,2,2,2,4),(-0.159353996056155,-0.120185717626862,
-0.0828817665727692,-0.0817045553496745,-0.0792736925960643,-0.0432511430807235,
-1.00011724153364E-6),.UNSPECIFIED.);
#6143=B_SPLINE_CURVE_WITH_KNOTS('',3,(#245990,#245991,#245992,#245993,#245994,
#245995,#245996,#245997,#245998,#245999,#246000,#246001,#246002,#246003,
#246004,#246005,#246006,#246007,#246008,#246009,#246010,#246011,#246012,
#246013,#246014,#246015,#246016,#246017,#246018,#246019,#246020),
 .UNSPECIFIED.,.F.,.F.,(4,3,3,3,3,3,3,3,3,3,4),(0.106516884683353,0.107092939699245,
0.107670885152251,0.108254128432155,0.108840899894406,0.10943507143996,
0.109760614783791,0.110353692948115,0.110941647902085,0.111523698461363,
0.112049172840853),.UNSPECIFIED.);
#6144=B_SPLINE_CURVE_WITH_KNOTS('',3,(#246084,#246085,#246086,#246087,#246088,
#246089,#246090,#246091,#246092,#246093,#246094,#246095,#246096,#246097,
#246098,#246099,#246100,#246101,#246102,#246103,#246104,#246105,#246106,
#246107,#246108,#246109,#246110,#246111,#246112,#246113,#246114,#246115,
#246116,#246117,#246118,#246119,#246120,#246121,#246122,#246123,#246124,
#246125,#246126,#246127,#246128,#246129,#246130,#246131,#246132,#246133,
#246134,#246135,#246136,#246137,#246138,#246139,#246140,#246141,#246142,
#246143,#246144,#246145,#246146,#246147,#246148,#246149,#246150,#246151,
#246152,#246153,#246154,#246155,#246156,#246157,#246158,#246159,#246160,
#246161,#246162,#246163,#246164,#246165,#246166,#246167,#246168,#246169,
#246170,#246171,#246172,#246173,#246174),.UNSPECIFIED.,.F.,.F.,(4,3,3,3,
3,3,3,3,3,3,3,3,3,3,3,3,3,3,3,3,3,3,3,3,3,3,3,3,3,3,4),(4.21395407591397E-15,
0.0513337499264628,0.102587935188955,0.125000000000031,0.176343801200056,
0.187500000000046,0.218750000000049,0.234375000000048,0.244041897155707,
0.250000000000047,0.309672654416341,0.369105698372573,0.428395485970964,
0.43750000000001,0.468750000000009,0.484375000000006,0.492187500000005,
0.497814922027182,0.500000000000003,0.573415958268157,0.625000000000011,
0.687500000000019,0.718750000000022,0.734375000000019,0.742187500000021,
0.748509676604922,0.750000000000022,0.831491304930903,0.915745652465452,
0.995687255361179,1.),.UNSPECIFIED.);
#6145=B_SPLINE_CURVE_WITH_KNOTS('',3,(#246176,#246177,#246178,#246179,#246180,
#246181,#246182,#246183,#246184,#246185,#246186,#246187,#246188,#246189,
#246190,#246191,#246192,#246193,#246194,#246195,#246196,#246197,#246198,
#246199,#246200,#246201),.UNSPECIFIED.,.F.,.F.,(4,2,2,2,2,2,2,2,2,2,2,2,
4),(-0.0336607847350189,-0.0252529472090739,-0.0183080555179268,-0.0146735416284525,
-0.0131510496302063,-0.0124740531690606,-0.0121414421254511,-0.0119752048891003,
-0.0118919360214624,-0.0118502431729518,-0.00873986850434003,-0.00356796757225184,
0.),.UNSPECIFIED.);
#6146=B_SPLINE_CURVE_WITH_KNOTS('',3,(#246203,#246204,#246205,#246206,#246207,
#246208,#246209,#246210,#246211,#246212),.UNSPECIFIED.,.F.,.F.,(4,3,3,4),
(1.23506593368833E-9,0.383469765022769,0.771748903020239,0.999982570836687),
 .UNSPECIFIED.);
#6147=B_SPLINE_CURVE_WITH_KNOTS('',3,(#246213,#246214,#246215,#246216,#246217,
#246218,#246219,#246220,#246221,#246222,#246223,#246224,#246225,#246226,
#246227,#246228,#246229,#246230,#246231,#246232,#246233,#246234,#246235),
 .UNSPECIFIED.,.F.,.F.,(4,2,1,1,1,1,2,2,2,1,1,1,2,2,4),(0.,0.250000000000111,
0.375000000000166,0.437500000000193,0.468750000000216,0.484375000000238,
0.49218750000024,0.500000000000242,0.62500000000017,0.687500000000123,0.718750000000091,
0.734375000000072,0.742187500000063,0.750000000000053,1.),.UNSPECIFIED.);
#6148=B_SPLINE_CURVE_WITH_KNOTS('',3,(#246268,#246269,#246270,#246271,#246272,
#246273,#246274,#246275,#246276,#246277,#246278,#246279,#246280,#246281,
#246282,#246283),.UNSPECIFIED.,.F.,.F.,(4,3,3,3,3,4),(0.,0.205474320931334,
0.405512720698626,0.603462068588223,0.801731034294112,1.),.UNSPECIFIED.);
#6149=B_SPLINE_CURVE_WITH_KNOTS('',3,(#246284,#246285,#246286,#246287,#246288,
#246289,#246290,#246291,#246292,#246293,#246294,#246295,#246296),
 .UNSPECIFIED.,.F.,.F.,(4,3,3,3,4),(0.,0.313781217437814,0.626723184051377,
0.938079360646063,1.),.UNSPECIFIED.);
#6150=B_SPLINE_CURVE_WITH_KNOTS('',3,(#246330,#246331,#246332,#246333,#246334,
#246335,#246336,#246337,#246338,#246339,#246340,#246341,#246342,#246343,
#246344,#246345,#246346,#246347,#246348,#246349,#246350,#246351,#246352,
#246353,#246354,#246355,#246356,#246357,#246358,#246359,#246360,#246361,
#246362,#246363,#246364,#246365,#246366,#246367,#246368,#246369,#246370,
#246371,#246372,#246373,#246374,#246375,#246376,#246377,#246378,#246379,
#246380,#246381,#246382,#246383,#246384),.UNSPECIFIED.,.F.,.F.,(4,3,3,3,
3,3,3,3,3,3,3,3,3,3,3,3,3,3,4),(0.,0.138504284258626,0.25,0.374999999999999,
0.437499999999998,0.470325698801164,0.499999999999997,0.500138551474872,
0.549028602637725,0.597465662805955,0.624999999999997,0.62596050941851,
0.681158301184605,0.718749999999996,0.736589248328212,0.749999999999997,
0.750154530180252,0.886556322996174,1.),.UNSPECIFIED.);
#6151=B_SPLINE_CURVE_WITH_KNOTS('',3,(#246385,#246386,#246387,#246388,#246389,
#246390,#246391,#246392,#246393,#246394,#246395,#246396,#246397,#246398,
#246399,#246400,#246401,#246402,#246403,#246404,#246405,#246406,#246407,
#246408,#246409,#246410,#246411,#246412,#246413,#246414,#246415,#246416,
#246417,#246418,#246419,#246420,#246421,#246422,#246423,#246424,#246425,
#246426,#246427,#246428,#246429,#246430,#246431,#246432,#246433,#246434,
#246435,#246436,#246437,#246438,#246439,#246440,#246441,#246442),
 .UNSPECIFIED.,.F.,.F.,(4,3,3,3,3,3,3,3,3,3,3,3,3,3,3,3,3,3,3,4),(0.,0.080558140948196,
0.16278162914552,0.245005117342845,0.286012425338604,0.360319101235246,
0.37102880065776,0.381960157756901,0.431472826356726,0.484375000000007,
0.495385439719595,0.500000000000006,0.500151948917147,0.581487373177427,
0.662653965760947,0.74699047432071,0.828040801997895,0.909144794487731,
0.990409652328597,1.),.UNSPECIFIED.);
#6152=B_SPLINE_CURVE_WITH_KNOTS('',3,(#246463,#246464,#246465,#246466,#246467,
#246468),.UNSPECIFIED.,.F.,.F.,(4,2,4),(-0.00572418575854378,-0.00286323169356134,
0.),.UNSPECIFIED.);
#6153=B_SPLINE_CURVE_WITH_KNOTS('',3,(#246469,#246470,#246471,#246472,#246473,
#246474,#246475,#246476,#246477,#246478,#246479,#246480,#246481,#246482,
#246483,#246484,#246485,#246486,#246487,#246488,#246489,#246490,#246491,
#246492,#246493,#246494,#246495,#246496,#246497,#246498,#246499),
 .UNSPECIFIED.,.F.,.F.,(4,3,3,3,3,3,3,3,3,3,4),(0.,0.11761557917262,0.239211453690796,
0.368222332867088,0.442407161882584,0.537154674978954,0.634968309816214,
0.73831066301708,0.845453355624249,0.959390767423322,0.999998837624099),
 .UNSPECIFIED.);
#6154=B_SPLINE_CURVE_WITH_KNOTS('',3,(#246501,#246502,#246503,#246504,#246505,
#246506,#246507,#246508,#246509,#246510,#246511,#246512,#246513,#246514,
#246515,#246516),.UNSPECIFIED.,.F.,.F.,(4,3,3,3,3,4),(0.,0.160379797404396,
0.25,0.526438124442171,0.791916875509661,1.),.UNSPECIFIED.);
#6155=B_SPLINE_CURVE_WITH_KNOTS('',3,(#246517,#246518,#246519,#246520,#246521,
#246522),.UNSPECIFIED.,.F.,.F.,(4,2,4),(-0.0615356806447155,-0.0307265379384587,
0.),.UNSPECIFIED.);
#6156=B_SPLINE_CURVE_WITH_KNOTS('',3,(#246584,#246585,#246586,#246587,#246588,
#246589,#246590,#246591,#246592,#246593,#246594,#246595,#246596,#246597,
#246598,#246599),.UNSPECIFIED.,.F.,.F.,(4,2,2,2,2,2,2,4),(3.3017407839461E-5,
0.249999999999985,0.374999999999977,0.437499999999978,0.468749999999975,
0.499999999999972,0.749999999999986,0.999999937134297),.UNSPECIFIED.);
#6157=B_SPLINE_CURVE_WITH_KNOTS('',3,(#246621,#246622,#246623,#246624,#246625,
#246626,#246627,#246628,#246629,#246630,#246631,#246632,#246633,#246634,
#246635,#246636,#246637,#246638,#246639,#246640,#246641,#246642,#246643,
#246644,#246645,#246646,#246647,#246648,#246649,#246650,#246651,#246652,
#246653,#246654,#246655,#246656,#246657,#246658,#246659,#246660,#246661,
#246662,#246663,#246664,#246665,#246666,#246667,#246668,#246669,#246670,
#246671,#246672,#246673,#246674,#246675),.UNSPECIFIED.,.F.,.F.,(4,3,3,3,
3,3,3,3,3,3,3,3,3,3,3,3,3,3,4),(0.,0.136293856989282,0.250000000000071,
0.375000000000084,0.437500000000081,0.472971764724835,0.500000000000077,
0.625000000000053,0.679526483168007,0.734502976449291,0.750000000000029,
0.815145744893402,0.875000000000005,0.901444261501065,0.92472577106741,
0.937500000000002,0.96396693827555,0.990694659952347,1.),.UNSPECIFIED.);
#6158=B_SPLINE_CURVE_WITH_KNOTS('',3,(#246724,#246725,#246726,#246727,#246728,
#246729,#246730,#246731,#246732,#246733,#246734,#246735,#246736,#246737,
#246738,#246739,#246740,#246741,#246742,#246743,#246744,#246745,#246746,
#246747,#246748,#246749,#246750,#246751,#246752,#246753,#246754,#246755,
#246756,#246757,#246758,#246759,#246760,#246761,#246762,#246763,#246764,
#246765,#246766,#246767,#246768,#246769,#246770,#246771,#246772,#246773,
#246774,#246775),.UNSPECIFIED.,.F.,.F.,(4,3,3,3,3,3,3,3,3,3,3,3,3,3,3,3,
3,4),(0.,0.0264122776644583,0.0525704699845341,0.0624999999999952,0.0830347144030536,
0.106647415780136,0.12499999999999,0.180884076821772,0.236293420895041,
0.249999999999977,0.374999999999964,0.437499999999959,0.473333285050837,
0.499999999999955,0.633762556066951,0.768082693942593,0.904334277462089,
1.),.UNSPECIFIED.);
#6159=B_SPLINE_CURVE_WITH_KNOTS('',3,(#246836,#246837,#246838,#246839,#246840,
#246841,#246842,#246843,#246844,#246845,#246846,#246847,#246848,#246849,
#246850,#246851),.UNSPECIFIED.,.F.,.F.,(4,2,2,2,2,2,2,4),(4.71302443996447E-8,
0.249999999999948,0.374999999999924,0.437499999999912,0.46874999999991,
0.499999999999908,0.749999999999954,0.999999958685833),.UNSPECIFIED.);
#6160=B_SPLINE_CURVE_WITH_KNOTS('',3,(#246865,#246866,#246867,#246868),
 .UNSPECIFIED.,.F.,.F.,(4,4),(0.000150513941758003,0.00194200748227624),
 .UNSPECIFIED.);
#6161=B_SPLINE_CURVE_WITH_KNOTS('',3,(#246870,#246871,#246872,#246873,#246874,
#246875),.UNSPECIFIED.,.F.,.F.,(4,2,4),(2.80044314047858E-9,0.0954464079467005,
0.190095771623502),.UNSPECIFIED.);
#6162=B_SPLINE_CURVE_WITH_KNOTS('',3,(#246878,#246879,#246880,#246881,#246882,
#246883),.UNSPECIFIED.,.F.,.F.,(4,2,4),(-0.050445736393907,-0.0244802048333361,
-5.52363958843116E-7),.UNSPECIFIED.);
#6163=B_SPLINE_CURVE_WITH_KNOTS('',3,(#246930,#246931,#246932,#246933,#246934,
#246935,#246936,#246937,#246938,#246939,#246940,#246941,#246942,#246943,
#246944,#246945,#246946,#246947,#246948,#246949,#246950,#246951,#246952,
#246953,#246954,#246955,#246956,#246957,#246958,#246959,#246960,#246961,
#246962,#246963,#246964,#246965,#246966,#246967,#246968,#246969,#246970,
#246971,#246972,#246973,#246974,#246975,#246976,#246977,#246978,#246979,
#246980,#246981,#246982,#246983,#246984,#246985,#246986,#246987,#246988,
#246989,#246990,#246991,#246992,#246993,#246994,#246995,#246996,#246997,
#246998,#246999,#247000,#247001,#247002,#247003,#247004,#247005,#247006,
#247007,#247008,#247009,#247010,#247011,#247012,#247013,#247014,#247015,
#247016,#247017,#247018,#247019,#247020,#247021,#247022,#247023,#247024,
#247025,#247026),.UNSPECIFIED.,.F.,.F.,(4,3,3,3,3,3,3,3,3,3,3,3,3,3,3,3,
3,3,3,3,3,3,3,3,3,3,3,3,3,3,3,3,4),(4.90643966544258E-10,0.0484929148260123,
0.0624999999999239,0.0937499999998868,0.109374999999871,0.117187499999864,
0.121917492028509,0.124999999999858,0.156249999999857,0.187499999999855,
0.215117790312726,0.234374999999851,0.242144940602164,0.246418240190107,
0.249999999999851,0.292416118246735,0.337195875190666,0.361094236029373,
0.374999999999876,0.419241773384761,0.465335153524285,0.497676368738863,
0.499999999999902,0.555006865257746,0.61025570631107,0.63852067128082,0.718028377305788,
0.749999999999951,0.765547908324208,0.826638203583669,0.887847641427647,
0.949089724737531,1.),.UNSPECIFIED.);
#6164=B_SPLINE_CURVE_WITH_KNOTS('',3,(#247027,#247028,#247029,#247030,#247031,
#247032,#247033,#247034,#247035,#247036,#247037,#247038,#247039,#247040,
#247041,#247042,#247043,#247044,#247045,#247046,#247047,#247048,#247049,
#247050,#247051,#247052,#247053,#247054,#247055,#247056,#247057,#247058,
#247059,#247060,#247061,#247062,#247063,#247064,#247065,#247066,#247067,
#247068,#247069,#247070,#247071,#247072,#247073,#247074,#247075,#247076,
#247077,#247078,#247079,#247080,#247081,#247082,#247083,#247084,#247085,
#247086,#247087,#247088,#247089,#247090,#247091,#247092,#247093,#247094,
#247095,#247096,#247097,#247098,#247099,#247100,#247101,#247102,#247103,
#247104,#247105,#247106,#247107,#247108),.UNSPECIFIED.,.F.,.F.,(4,3,3,3,
3,3,3,3,3,3,3,3,3,3,3,3,3,3,3,3,3,3,3,3,3,3,3,4),(0.,0.0707256112310334,
0.143494179479758,0.17045670394154,0.244355170384741,0.249999999999997,
0.326199977717216,0.374999999999996,0.415486708305964,0.437499999999992,
0.46874999999999,0.484950527153161,0.499999999999987,0.572299455137252,
0.624999999999996,0.635472223482649,0.687500000000006,0.718750000000013,
0.734375000000019,0.742187500000023,0.748402724993224,0.750000000000026,
0.802194690059772,0.851646017502705,0.898368266629995,0.944112234320723,
0.990046607588191,0.999999999831502),.UNSPECIFIED.);
#6165=B_SPLINE_CURVE_WITH_KNOTS('',3,(#247148,#247149,#247150,#247151,#247152,
#247153,#247154,#247155,#247156,#247157,#247158,#247159,#247160,#247161,
#247162,#247163,#247164,#247165,#247166,#247167,#247168,#247169,#247170,
#247171,#247172,#247173,#247174,#247175),.UNSPECIFIED.,.F.,.F.,(4,3,3,3,
3,3,3,3,3,4),(0.838474295473316,0.930058057517816,1.02271627966907,1.11634472529987,
1.17837075498859,1.27647714794017,1.37034540944472,1.46344152971751,1.55490687474701,
1.5707963267949),.UNSPECIFIED.);
#6166=B_SPLINE_CURVE_WITH_KNOTS('',3,(#247176,#247177,#247178,#247179,#247180,
#247181,#247182,#247183,#247184,#247185,#247186,#247187,#247188,#247189,
#247190,#247191,#247192,#247193,#247194,#247195,#247196,#247197,#247198,
#247199,#247200,#247201,#247202,#247203,#247204,#247205,#247206,#247207,
#247208,#247209,#247210,#247211,#247212,#247213,#247214,#247215,#247216,
#247217,#247218,#247219,#247220,#247221,#247222,#247223,#247224,#247225,
#247226,#247227,#247228,#247229,#247230,#247231,#247232,#247233,#247234,
#247235,#247236,#247237,#247238,#247239,#247240,#247241,#247242,#247243,
#247244,#247245,#247246,#247247,#247248),.UNSPECIFIED.,.F.,.F.,(4,3,3,3,
3,3,3,3,3,3,3,3,3,3,3,3,3,3,3,3,3,3,3,3,4),(0.,0.0401919312141592,0.0819963404705172,
0.129529840467209,0.176267374973055,0.225909382758087,0.242187499999802,
0.246093749999801,0.249999999999799,0.25875764645275,0.316878823226282,
0.374999999999814,0.43851508519816,0.484374999999833,0.493696347244718,
0.499999999999837,0.573948265789786,0.624999999999878,0.666613401443068,
0.708142799438681,0.739741591291496,0.74999999999992,0.858692239174755,
0.96742933190215,1.),.UNSPECIFIED.);
#6167=B_SPLINE_CURVE_WITH_KNOTS('',3,(#247292,#247293,#247294,#247295,#247296,
#247297,#247298,#247299,#247300,#247301,#247302,#247303,#247304,#247305,
#247306,#247307,#247308,#247309,#247310,#247311,#247312,#247313,#247314,
#247315,#247316,#247317,#247318,#247319,#247320,#247321,#247322,#247323,
#247324,#247325,#247326,#247327,#247328,#247329,#247330,#247331,#247332,
#247333,#247334,#247335,#247336,#247337,#247338,#247339,#247340,#247341,
#247342,#247343,#247344,#247345,#247346,#247347,#247348,#247349,#247350,
#247351,#247352,#247353,#247354,#247355,#247356,#247357,#247358,#247359,
#247360,#247361,#247362,#247363,#247364,#247365,#247366,#247367),
 .UNSPECIFIED.,.F.,.F.,(4,3,3,3,3,3,3,3,3,3,3,3,3,3,3,3,3,3,3,3,3,3,3,3,
3,4),(0.,0.0556216394818239,0.114786080727818,0.125000000000148,0.170750843532883,
0.187500000000216,0.218750000000247,0.234375000000262,0.242187500000269,
0.250000000000276,0.307005920394933,0.367744726360799,0.375000000000249,
0.400758159320508,0.437500000000244,0.468750000000244,0.484375000000236,
0.492187500000229,0.500000000000223,0.579547472665855,0.63240430891721,
0.709879787609452,0.79182759636595,0.881990335411978,0.905051170989505,
0.999999999999986),.UNSPECIFIED.);
#6168=B_SPLINE_CURVE_WITH_KNOTS('',3,(#247369,#247370,#247371,#247372,#247373,
#247374,#247375,#247376,#247377,#247378,#247379,#247380,#247381,#247382,
#247383,#247384,#247385,#247386,#247387,#247388,#247389,#247390,#247391,
#247392,#247393,#247394,#247395,#247396,#247397,#247398,#247399,#247400,
#247401,#247402,#247403,#247404,#247405,#247406,#247407,#247408,#247409,
#247410,#247411,#247412,#247413,#247414,#247415,#247416,#247417,#247418,
#247419,#247420,#247421,#247422,#247423,#247424,#247425,#247426,#247427,
#247428,#247429,#247430,#247431,#247432,#247433,#247434,#247435,#247436,
#247437,#247438,#247439,#247440,#247441,#247442,#247443,#247444,#247445,
#247446,#247447,#247448,#247449,#247450,#247451,#247452,#247453,#247454,
#247455,#247456,#247457,#247458,#247459,#247460,#247461,#247462,#247463,
#247464,#247465,#247466,#247467,#247468,#247469,#247470,#247471,#247472,
#247473,#247474),.UNSPECIFIED.,.F.,.F.,(4,3,3,3,3,3,3,3,3,3,3,3,3,3,3,3,
3,3,3,3,3,3,3,3,3,3,3,3,3,3,3,3,3,3,3,4),(0.,0.031249999999987,0.0609011661437237,
0.0900742302575725,0.116500739893332,0.139847180987321,0.167385385740464,
0.19228716190139,0.216441510703671,0.233220755351783,0.241610377675839,
0.245805188837868,0.246124074157174,0.248829591534349,0.249999999999896,
0.25307350048546,0.303563924576077,0.356881390395021,0.368339324261443,
0.374999999999939,0.417741125365788,0.437499999999959,0.468749999999971,
0.484374999999979,0.493079053533789,0.499999999999986,0.505683401295463,
0.580643685324135,0.624064275299452,0.690096059492877,0.745168072966554,
0.749999999999993,0.820916344647453,0.892677383913134,0.965739469496175,
1.),.UNSPECIFIED.);
#6169=B_SPLINE_CURVE_WITH_KNOTS('',3,(#247479,#247480,#247481,#247482,#247483,
#247484),.UNSPECIFIED.,.F.,.F.,(4,2,4),(-0.0269664855274713,-0.0134828803856389,
-9.31064075733457E-8),.UNSPECIFIED.);
#6170=B_SPLINE_CURVE_WITH_KNOTS('',3,(#247521,#247522,#247523,#247524,#247525,
#247526,#247527,#247528,#247529,#247530,#247531,#247532,#247533,#247534,
#247535,#247536,#247537,#247538,#247539,#247540,#247541,#247542,#247543,
#247544,#247545,#247546,#247547,#247548,#247549,#247550,#247551,#247552,
#247553,#247554,#247555,#247556,#247557,#247558,#247559,#247560,#247561,
#247562,#247563,#247564,#247565,#247566,#247567,#247568,#247569,#247570,
#247571,#247572,#247573,#247574,#247575,#247576,#247577,#247578,#247579,
#247580,#247581,#247582,#247583,#247584,#247585,#247586,#247587,#247588,
#247589,#247590,#247591,#247592,#247593,#247594,#247595,#247596,#247597,
#247598,#247599,#247600,#247601,#247602),.UNSPECIFIED.,.F.,.F.,(4,3,3,3,
3,3,3,3,3,3,3,3,3,3,3,3,3,3,3,3,3,3,3,3,3,3,3,4),(2.56487959041513E-5,0.0937141008831449,
0.125000000000051,0.167506357101888,0.209606233741686,0.250000000000101,
0.255551994916339,0.331355837399193,0.375000000000152,0.446289040401504,
0.484375000000202,0.493412876541942,0.496956676406121,0.500000000000213,
0.562500000000231,0.625000000000249,0.685483798309844,0.739929054069917,
0.742187500000292,0.746093750000291,0.749589802703738,0.750000000000291,
0.799105712593443,0.846444987881696,0.890808069977353,0.933559317031731,
0.974096720592753,1.),.UNSPECIFIED.);
#6171=B_SPLINE_CURVE_WITH_KNOTS('',3,(#247603,#247604,#247605,#247606,#247607,
#247608,#247609,#247610,#247611,#247612,#247613,#247614,#247615,#247616,
#247617,#247618,#247619,#247620,#247621,#247622,#247623,#247624,#247625,
#247626,#247627,#247628,#247629,#247630),.UNSPECIFIED.,.F.,.F.,(4,3,3,3,
3,3,3,3,3,4),(1.5707963267949,1.66216581219747,1.7554915464119,1.8494444653613,
1.94323589460212,1.96555277811107,2.05915766062388,2.15220658922426,2.24364798476046,
2.30311835811648),.UNSPECIFIED.);
#6172=B_SPLINE_CURVE_WITH_KNOTS('',3,(#247713,#247714,#247715,#247716,#247717,
#247718,#247719,#247720,#247721,#247722,#247723,#247724,#247725,#247726,
#247727,#247728,#247729,#247730,#247731,#247732,#247733,#247734,#247735,
#247736,#247737,#247738,#247739,#247740,#247741,#247742,#247743,#247744,
#247745,#247746,#247747,#247748,#247749,#247750,#247751,#247752,#247753,
#247754,#247755,#247756,#247757,#247758,#247759,#247760,#247761,#247762,
#247763,#247764,#247765,#247766,#247767,#247768,#247769,#247770,#247771,
#247772,#247773,#247774,#247775,#247776,#247777,#247778,#247779,#247780,
#247781,#247782,#247783,#247784,#247785,#247786,#247787,#247788,#247789,
#247790,#247791,#247792,#247793,#247794,#247795,#247796,#247797,#247798,
#247799,#247800),.UNSPECIFIED.,.F.,.F.,(4,3,3,3,3,3,3,3,3,3,3,3,3,3,3,3,
3,3,3,3,3,3,3,3,3,3,3,3,3,4),(0.,0.0794481524643703,0.156768214864146,0.231339825995753,
0.249999999999803,0.259044933609346,0.317022466804525,0.374999999999703,
0.382132705216096,0.432682584624564,0.437499999999653,0.468749999999628,
0.484374999999614,0.492187499999605,0.496093749999601,0.499514900518553,
0.499999999999598,0.503507170613991,0.558938703049898,0.610863177296971,
0.66100706983879,0.708568267760028,0.749999999999799,0.792248812129508,
0.812499999999849,0.859374999999887,0.902003267191604,0.943270081246986,
0.982693916806458,1.),.UNSPECIFIED.);
#6173=B_SPLINE_CURVE_WITH_KNOTS('',3,(#247801,#247802,#247803,#247804,#247805,
#247806,#247807,#247808,#247809,#247810,#247811,#247812,#247813,#247814,
#247815,#247816,#247817,#247818,#247819,#247820,#247821,#247822,#247823,
#247824,#247825,#247826,#247827,#247828,#247829,#247830,#247831,#247832,
#247833,#247834,#247835,#247836,#247837),.UNSPECIFIED.,.F.,.F.,(4,3,3,3,
3,3,3,3,3,3,3,3,4),(0.,0.000111500026751792,0.000198033010607759,0.000314017729824417,
0.000396641361730405,0.000472439313739977,0.000496099573318823,0.000572015964014575,
0.000578662087025262,0.000595420430124543,0.000632317246134149,0.000714137978067164,
0.00079328272346081),.UNSPECIFIED.);
#6174=B_SPLINE_CURVE_WITH_KNOTS('',3,(#247905,#247906,#247907,#247908,#247909,
#247910,#247911,#247912,#247913,#247914,#247915,#247916,#247917,#247918,
#247919,#247920,#247921,#247922,#247923,#247924,#247925,#247926,#247927,
#247928,#247929,#247930,#247931,#247932,#247933,#247934,#247935,#247936,
#247937,#247938,#247939,#247940,#247941),.UNSPECIFIED.,.F.,.F.,(4,3,3,3,
3,3,3,3,3,3,3,3,4),(0.,8.15311101657598E-5,0.000163591288741779,0.00017635437994511,
0.00019860108990148,0.000231640871620125,0.000308214802536355,0.000385145785492459,
0.000397500346645172,0.000497039263014267,0.000596687155864874,0.000699642509595148,
0.000795000693290343),.UNSPECIFIED.);
#6175=B_SPLINE_CURVE_WITH_KNOTS('',3,(#247942,#247943,#247944,#247945,#247946,
#247947,#247948,#247949,#247950,#247951,#247952,#247953,#247954,#247955,
#247956,#247957,#247958,#247959,#247960),.UNSPECIFIED.,.F.,.F.,(4,2,2,2,
1,1,1,2,2,2,4),(0.,0.249999999999961,0.374999999999946,0.437499999999938,
0.468749999999932,0.484374999999921,0.492187499999909,0.49609374999991,
0.49999999999991,0.749999999999955,1.),.UNSPECIFIED.);
#6176=B_SPLINE_CURVE_WITH_KNOTS('',3,(#247980,#247981,#247982,#247983,#247984,
#247985,#247986,#247987,#247988,#247989,#247990,#247991,#247992,#247993,
#247994,#247995),.UNSPECIFIED.,.F.,.F.,(4,3,3,3,3,4),(0.,0.211457556634167,
0.425375488930141,0.639024931200921,0.850118550185379,1.),.UNSPECIFIED.);
#6177=B_SPLINE_CURVE_WITH_KNOTS('',3,(#248004,#248005,#248006,#248007,#248008,
#248009,#248010,#248011,#248012,#248013,#248014,#248015,#248016,#248017,
#248018,#248019),.UNSPECIFIED.,.F.,.F.,(4,3,3,3,3,4),(0.,0.211457556638465,
0.42537548893837,0.639024931212968,0.850118550201083,1.),.UNSPECIFIED.);
#6178=B_SPLINE_CURVE_WITH_KNOTS('',3,(#248028,#248029,#248030,#248031,#248032,
#248033,#248034,#248035,#248036,#248037,#248038,#248039,#248040,#248041,
#248042,#248043),.UNSPECIFIED.,.F.,.F.,(4,3,3,3,3,4),(0.,0.210153564503388,
0.423721788860115,0.637632960030634,0.849873129905918,1.),.UNSPECIFIED.);
#6179=B_SPLINE_CURVE_WITH_KNOTS('',3,(#248060,#248061,#248062,#248063,#248064,
#248065,#248066,#248067,#248068,#248069,#248070,#248071,#248072),
 .UNSPECIFIED.,.F.,.F.,(4,3,3,3,4),(0.,0.000473404920692545,0.000946160257514461,
0.0014172553414947,0.00169753871027588),.UNSPECIFIED.);
#6180=B_SPLINE_CURVE_WITH_KNOTS('',3,(#248081,#248082,#248083,#248084,#248085,
#248086),.UNSPECIFIED.,.F.,.F.,(4,2,4),(0.,0.5,1.),.UNSPECIFIED.);
#6181=B_SPLINE_CURVE_WITH_KNOTS('',3,(#248103,#248104,#248105,#248106),
 .UNSPECIFIED.,.F.,.F.,(4,4),(0.,0.0169301343956772),.UNSPECIFIED.);
#6182=B_SPLINE_CURVE_WITH_KNOTS('',3,(#248129,#248130,#248131,#248132,#248133,
#248134,#248135,#248136,#248137,#248138,#248139,#248140,#248141,#248142,
#248143,#248144),.UNSPECIFIED.,.F.,.F.,(4,3,3,3,3,4),(0.,0.000357599365643427,
0.000494441238575043,0.000494698486827334,0.000823483292681039,0.000988882477150085),
 .UNSPECIFIED.);
#6183=B_SPLINE_CURVE_WITH_KNOTS('',3,(#248170,#248171,#248172,#248173,#248174,
#248175,#248176,#248177,#248178,#248179,#248180,#248181,#248182,#248183,
#248184,#248185),.UNSPECIFIED.,.F.,.F.,(4,3,3,3,3,4),(0.,0.000351072004839477,
0.000494230507537995,0.000494489082053731,0.000752353626049509,0.000988978164107462),
 .UNSPECIFIED.);
#6184=B_SPLINE_CURVE_WITH_KNOTS('',3,(#248188,#248189,#248190,#248191),
 .UNSPECIFIED.,.F.,.F.,(4,4),(0.,0.0169301343956772),.UNSPECIFIED.);
#6185=B_SPLINE_CURVE_WITH_KNOTS('',3,(#248208,#248209,#248210,#248211,#248212,
#248213,#248214,#248215,#248216,#248217,#248218,#248219,#248220),
 .UNSPECIFIED.,.F.,.F.,(4,3,3,3,4),(0.,0.000471266058852581,0.000943667138230186,
0.00141714356512851,0.00169753871027587),.UNSPECIFIED.);
#6186=B_SPLINE_CURVE_WITH_KNOTS('',3,(#248229,#248230,#248231,#248232,#248233,
#248234),.UNSPECIFIED.,.F.,.F.,(4,2,4),(0.,0.499999999999999,1.),
 .UNSPECIFIED.);
#6187=B_SPLINE_CURVE_WITH_KNOTS('',3,(#248250,#248251,#248252,#248253),
 .UNSPECIFIED.,.F.,.F.,(4,4),(0.00345714931441652,0.0169301343956773),
 .UNSPECIFIED.);
#6188=B_SPLINE_CURVE_WITH_KNOTS('',3,(#248279,#248280,#248281,#248282,#248283,
#248284,#248285,#248286,#248287,#248288,#248289,#248290,#248291,#248292,
#248293,#248294),.UNSPECIFIED.,.F.,.F.,(4,3,3,3,3,4),(0.,0.000357599364445761,
0.000494441238575047,0.000494698486827312,0.000823483291488249,0.000988882477150094),
 .UNSPECIFIED.);
#6189=B_SPLINE_CURVE_WITH_KNOTS('',3,(#248320,#248321,#248322,#248323,#248324,
#248325,#248326,#248327,#248328,#248329,#248330,#248331,#248332,#248333,
#248334,#248335),.UNSPECIFIED.,.F.,.F.,(4,3,3,3,3,4),(0.,0.000351072006453831,
0.000494230507538011,0.000494489082053725,0.000752353626509348,0.00098897816410745),
 .UNSPECIFIED.);
#6190=B_SPLINE_CURVE_WITH_KNOTS('',3,(#248338,#248339,#248340,#248341),
 .UNSPECIFIED.,.F.,.F.,(4,4),(0.,0.0169301343956772),.UNSPECIFIED.);
#6191=B_SPLINE_CURVE_WITH_KNOTS('',3,(#248358,#248359,#248360,#248361,#248362,
#248363,#248364,#248365,#248366,#248367,#248368,#248369,#248370),
 .UNSPECIFIED.,.F.,.F.,(4,3,3,3,4),(0.,0.000471266059312478,0.000943667139110938,
0.00141714356637207,0.00169753871027587),.UNSPECIFIED.);
#6192=B_SPLINE_CURVE_WITH_KNOTS('',3,(#248383,#248384,#248385,#248386,#248387,
#248388,#248389,#248390,#248391,#248392,#248393,#248394,#248395,#248396,
#248397,#248398,#248399,#248400,#248401,#248402,#248403,#248404,#248405,
#248406,#248407,#248408,#248409,#248410),.UNSPECIFIED.,.F.,.F.,(4,3,3,3,
3,3,3,3,3,4),(0.,0.109615221367934,0.221368175865868,0.334395344060503,
0.448689930122853,0.564253205982057,0.681798912079819,0.800474133367955,
0.92099033968873,1.),.UNSPECIFIED.);
#6193=B_SPLINE_CURVE_WITH_KNOTS('',3,(#248425,#248426,#248427,#248428,#248429,
#248430,#248431,#248432,#248433,#248434,#248435,#248436,#248437,#248438,
#248439,#248440,#248441,#248442,#248443,#248444,#248445,#248446,#248447,
#248448,#248449,#248450,#248451,#248452),.UNSPECIFIED.,.F.,.F.,(4,3,3,3,
3,3,3,3,3,4),(0.,0.109615221365806,0.221368175853348,0.334395344045476,
0.448689930098025,0.564253205940007,0.681798912032425,0.800474133326316,
0.920990339655845,1.),.UNSPECIFIED.);
#6194=B_SPLINE_CURVE_WITH_KNOTS('',3,(#248467,#248468,#248469,#248470,#248471,
#248472,#248473,#248474,#248475,#248476,#248477,#248478,#248479,#248480,
#248481,#248482,#248483,#248484,#248485,#248486,#248487,#248488,#248489,
#248490,#248491,#248492,#248493,#248494),.UNSPECIFIED.,.F.,.F.,(4,3,3,3,
3,3,3,3,3,4),(0.,0.125,0.243735787420882,0.361132522922663,0.477221946749902,
0.592021254917456,0.704884640467779,0.816636758371523,0.926654827500873,
1.),.UNSPECIFIED.);
#6195=B_SPLINE_CURVE_WITH_KNOTS('',3,(#248500,#248501,#248502,#248503,#248504,
#248505,#248506,#248507,#248508,#248509,#248510,#248511,#248512,#248513,
#248514,#248515,#248516,#248517,#248518),.UNSPECIFIED.,.F.,.F.,(4,3,3,3,
3,3,4),(0.,0.193537780414673,0.395153335311005,0.588509404331274,0.782367954940123,
0.977488548866527,1.),.UNSPECIFIED.);
#6196=B_SPLINE_CURVE_WITH_KNOTS('',3,(#248527,#248528,#248529,#248530,#248531,
#248532,#248533,#248534,#248535,#248536,#248537,#248538,#248539,#248540,
#248541,#248542,#248543,#248544,#248545),.UNSPECIFIED.,.F.,.F.,(4,3,3,3,
3,3,4),(0.,0.194999919104645,0.396249939328484,0.589433349910318,0.782576073903087,
0.976165346307675,1.),.UNSPECIFIED.);
#6197=B_SPLINE_CURVE_WITH_KNOTS('',3,(#248554,#248555,#248556,#248557,#248558,
#248559,#248560,#248561,#248562,#248563,#248564,#248565,#248566,#248567,
#248568,#248569,#248570,#248571,#248572),.UNSPECIFIED.,.F.,.F.,(4,3,3,3,
3,3,4),(0.,0.193537780417685,0.395153335313264,0.588509404336086,0.78236795494766,
0.977488548876437,1.),.UNSPECIFIED.);
#6198=B_SPLINE_CURVE_WITH_KNOTS('',3,(#248581,#248582,#248583,#248584,#248585,
#248586,#248587,#248588,#248589,#248590,#248591,#248592,#248593,#248594,
#248595,#248596,#248597,#248598,#248599),.UNSPECIFIED.,.F.,.F.,(4,3,3,3,
3,3,4),(0.,0.194999919126221,0.396249939344666,0.589433349950878,0.782576073968802,
0.976165346399302,1.),.UNSPECIFIED.);
#6199=B_SPLINE_CURVE_WITH_KNOTS('',3,(#248621,#248622,#248623,#248624,#248625,
#248626,#248627,#248628,#248629,#248630,#248631,#248632,#248633),
 .UNSPECIFIED.,.F.,.F.,(4,3,3,3,4),(0.,0.000473404920692537,0.000946160257514427,
0.00141725534149459,0.00169753871027588),.UNSPECIFIED.);
#6200=B_SPLINE_CURVE_WITH_KNOTS('',3,(#248640,#248641,#248642,#248643,#248644,
#248645,#248646,#248647,#248648,#248649,#248650,#248651,#248652,#248653,
#248654,#248655,#248656,#248657,#248658,#248659,#248660,#248661),
 .UNSPECIFIED.,.F.,.F.,(4,3,3,3,3,3,3,4),(0.,0.151764361358548,0.302277176656851,
0.451566165387974,0.599064031232558,0.745556092124806,0.890528328351801,
1.),.UNSPECIFIED.);
#6201=B_SPLINE_CURVE_WITH_KNOTS('',3,(#248670,#248671,#248672,#248673,#248674,
#248675,#248676,#248677,#248678,#248679,#248680,#248681,#248682,#248683,
#248684,#248685,#248686,#248687,#248688,#248689,#248690,#248691),
 .UNSPECIFIED.,.F.,.F.,(4,3,3,3,3,3,3,4),(0.,0.14495178916051,0.291012358970586,
0.438205967951544,0.587224233824978,0.737255355597419,0.888962473623652,
1.),.UNSPECIFIED.);
#6202=B_SPLINE_CURVE_WITH_KNOTS('',3,(#248696,#248697,#248698,#248699),
 .UNSPECIFIED.,.F.,.F.,(4,4),(0.,0.0169301343956772),.UNSPECIFIED.);
#6203=B_SPLINE_CURVE_WITH_KNOTS('',3,(#248722,#248723,#248724,#248725,#248726,
#248727,#248728,#248729,#248730,#248731,#248732,#248733,#248734,#248735,
#248736,#248737),.UNSPECIFIED.,.F.,.F.,(4,3,3,3,3,4),(0.,0.000357599365646066,
0.000494441238575043,0.000494698486827332,0.000823483292682126,0.000988882477150085),
 .UNSPECIFIED.);
#6204=B_SPLINE_CURVE_WITH_KNOTS('',3,(#248763,#248764,#248765,#248766,#248767,
#248768,#248769,#248770,#248771,#248772,#248773,#248774,#248775,#248776,
#248777,#248778),.UNSPECIFIED.,.F.,.F.,(4,3,3,3,3,4),(0.,0.000351072004843104,
0.000494230507537992,0.000494489082053731,0.00075235362604859,0.000988978164107462),
 .UNSPECIFIED.);
#6205=B_SPLINE_CURVE_WITH_KNOTS('',3,(#248781,#248782,#248783,#248784),
 .UNSPECIFIED.,.F.,.F.,(4,4),(0.,0.0169301343956772),.UNSPECIFIED.);
#6206=B_SPLINE_CURVE_WITH_KNOTS('',3,(#248801,#248802,#248803,#248804,#248805,
#248806,#248807,#248808,#248809,#248810,#248811,#248812,#248813),
 .UNSPECIFIED.,.F.,.F.,(4,3,3,3,4),(0.,0.000471266058852855,0.000943667138229705,
0.00141714356512824,0.00169753871027587),.UNSPECIFIED.);
#6207=B_SPLINE_CURVE_WITH_KNOTS('',3,(#248833,#248834,#248835,#248836,#248837,
#248838,#248839,#248840,#248841,#248842,#248843,#248844,#248845),
 .UNSPECIFIED.,.F.,.F.,(4,3,3,3,4),(0.,0.000473404921390372,0.000946160258865428,
0.00141725534343648,0.00169753871027587),.UNSPECIFIED.);
#6208=B_SPLINE_CURVE_WITH_KNOTS('',3,(#248852,#248853,#248854,#248855,#248856,
#248857,#248858,#248859,#248860,#248861,#248862,#248863,#248864,#248865,
#248866,#248867,#248868,#248869,#248870,#248871,#248872,#248873),
 .UNSPECIFIED.,.F.,.F.,(4,3,3,3,3,3,3,4),(0.,0.151764361358931,0.302277176656673,
0.451566165387056,0.599064031230457,0.74555609212193,0.890528328348514,
1.),.UNSPECIFIED.);
#6209=B_SPLINE_CURVE_WITH_KNOTS('',3,(#248882,#248883,#248884,#248885,#248886,
#248887,#248888,#248889,#248890,#248891,#248892,#248893,#248894,#248895,
#248896,#248897,#248898,#248899,#248900,#248901,#248902,#248903),
 .UNSPECIFIED.,.F.,.F.,(4,3,3,3,3,3,3,4),(0.,0.144951789160898,0.291012358971132,
0.438205967951823,0.587224233825539,0.737255355598683,0.888962473625554,
1.),.UNSPECIFIED.);
#6210=B_SPLINE_CURVE_WITH_KNOTS('',3,(#248908,#248909,#248910,#248911),
 .UNSPECIFIED.,.F.,.F.,(4,4),(0.,0.0169301343956773),.UNSPECIFIED.);
#6211=B_SPLINE_CURVE_WITH_KNOTS('',3,(#248934,#248935,#248936,#248937,#248938,
#248939,#248940,#248941,#248942,#248943,#248944,#248945,#248946,#248947,
#248948,#248949),.UNSPECIFIED.,.F.,.F.,(4,3,3,3,3,4),(0.,0.000357599364441133,
0.000494441238575047,0.000494698486827317,0.000823483291485574,0.000988882477150094),
 .UNSPECIFIED.);
#6212=B_SPLINE_CURVE_WITH_KNOTS('',3,(#248975,#248976,#248977,#248978,#248979,
#248980,#248981,#248982,#248983,#248984,#248985,#248986,#248987,#248988,
#248989,#248990),.UNSPECIFIED.,.F.,.F.,(4,3,3,3,3,4),(0.,0.000351072006454456,
0.000494230507538008,0.000494489082053725,0.000752353626508291,0.00098897816410745),
 .UNSPECIFIED.);
#6213=B_SPLINE_CURVE_WITH_KNOTS('',3,(#248993,#248994,#248995,#248996),
 .UNSPECIFIED.,.F.,.F.,(4,4),(0.,0.0169301343956772),.UNSPECIFIED.);
#6214=B_SPLINE_CURVE_WITH_KNOTS('',3,(#249013,#249014,#249015,#249016,#249017,
#249018,#249019,#249020,#249021,#249022,#249023,#249024,#249025),
 .UNSPECIFIED.,.F.,.F.,(4,3,3,3,4),(0.,0.000471266059312478,0.000943667139110938,
0.00141714356637207,0.00169753871027587),.UNSPECIFIED.);
#6215=B_SPLINE_CURVE_WITH_KNOTS('',3,(#249053,#249054,#249055,#249056,#249057,
#249058,#249059,#249060,#249061,#249062,#249063,#249064,#249065,#249066,
#249067,#249068),.UNSPECIFIED.,.F.,.F.,(4,3,3,3,3,4),(0.,0.203691748333807,
0.402768811250355,0.498651532784128,0.778653969973165,1.),.UNSPECIFIED.);
#6216=B_SPLINE_CURVE_WITH_KNOTS('',3,(#249083,#249084,#249085,#249086,#249087,
#249088,#249089,#249090,#249091,#249092,#249093,#249094,#249095,#249096,
#249097,#249098,#249099,#249100,#249101),.UNSPECIFIED.,.F.,.F.,(4,3,3,3,
3,3,4),(0.,0.25440556101236,0.44080417075927,0.527162630963832,0.750951239011533,
0.954610616175962,1.),.UNSPECIFIED.);
#6217=B_SPLINE_CURVE_WITH_KNOTS('',3,(#249114,#249115,#249116,#249117,#249118,
#249119,#249120,#249121,#249122,#249123,#249124,#249125,#249126,#249127,
#249128,#249129),.UNSPECIFIED.,.F.,.F.,(4,3,3,3,3,4),(0.,0.203691748342557,
0.402768811256918,0.498651532789133,0.778653969972626,1.),.UNSPECIFIED.);
#6218=B_SPLINE_CURVE_WITH_KNOTS('',3,(#249144,#249145,#249146,#249147,#249148,
#249149,#249150,#249151,#249152,#249153,#249154,#249155,#249156,#249157,
#249158,#249159,#249160,#249161,#249162),.UNSPECIFIED.,.F.,.F.,(4,3,3,3,
3,3,4),(0.,0.254405561026845,0.440804170770133,0.527162630968293,0.750951238968695,
0.954610616116233,1.),.UNSPECIFIED.);
#6219=B_SPLINE_CURVE_WITH_KNOTS('',3,(#249184,#249185,#249186,#249187),
 .UNSPECIFIED.,.F.,.F.,(4,4),(0.,1.),.UNSPECIFIED.);
#6220=B_SPLINE_CURVE_WITH_KNOTS('',3,(#249548,#249549,#249550,#249551,#249552,
#249553,#249554,#249555,#249556,#249557,#249558,#249559,#249560,#249561,
#249562,#249563,#249564,#249565,#249566,#249567,#249568,#249569,#249570,
#249571,#249572,#249573,#249574,#249575,#249576,#249577,#249578,#249579,
#249580,#249581,#249582,#249583,#249584,#249585,#249586,#249587),
 .UNSPECIFIED.,.F.,.F.,(4,3,3,3,3,3,3,3,3,3,3,3,3,4),(0.595270229260643,
0.601562499850747,0.609375000000292,0.617187498808339,0.624999995264159,
0.632812500000061,0.636718750000023,0.640624999999984,0.65624999999983,
0.671874999999676,0.687499999999522,0.703124999999369,0.718749999999215,
0.720233735124377),.UNSPECIFIED.);
#6221=B_SPLINE_CURVE_WITH_KNOTS('',3,(#249588,#249589,#249590,#249591,#249592,
#249593,#249594,#249595,#249596,#249597,#249598,#249599,#249600,#249601),
 .UNSPECIFIED.,.F.,.F.,(4,2,2,2,2,2,4),(-0.159234538760931,-0.11979722499102,
-0.0828045251107409,-0.0816375126728872,-0.0792258592190679,-0.0429042526546323,
-1.00001016328255E-6),.UNSPECIFIED.);
#6222=B_SPLINE_CURVE_WITH_KNOTS('',3,(#250156,#250157,#250158,#250159,#250160,
#250161,#250162,#250163,#250164,#250165,#250166,#250167,#250168,#250169,
#250170,#250171,#250172,#250173,#250174,#250175,#250176,#250177,#250178,
#250179,#250180,#250181,#250182,#250183,#250184,#250185,#250186),
 .UNSPECIFIED.,.F.,.F.,(4,3,3,3,3,3,3,3,3,3,4),(0.881769399096963,0.882351628344185,
0.882937092487587,0.883530275652419,0.884057971014493,0.884652700978261,
0.885241428493491,0.88582365002593,0.886402716932186,0.886978997726707,
0.887301779570027),.UNSPECIFIED.);
#6223=B_SPLINE_CURVE_WITH_KNOTS('',3,(#250189,#250190,#250191,#250192,#250193,
#250194,#250195,#250196,#250197,#250198,#250199,#250200,#250201,#250202,
#250203,#250204,#250205,#250206,#250207,#250208,#250209,#250210,#250211,
#250212,#250213,#250214,#250215,#250216,#250217,#250218,#250219),
 .UNSPECIFIED.,.F.,.F.,(4,3,3,3,3,3,3,3,3,3,4),(0.,0.0937364629817202,0.20846275873661,
0.322150628458144,0.434851188691642,0.546612363950819,0.657479176507349,
0.767494003890456,0.876696808412568,0.985125342372657,1.),.UNSPECIFIED.);
#6224=B_SPLINE_CURVE_WITH_KNOTS('',3,(#250221,#250222,#250223,#250224,#250225,
#250226,#250227,#250228,#250229,#250230,#250231,#250232,#250233,#250234,
#250235,#250236,#250237,#250238,#250239,#250240,#250241,#250242,#250243,
#250244,#250245,#250246,#250247,#250248,#250249,#250250,#250251,#250252,
#250253,#250254,#250255,#250256,#250257,#250258,#250259,#250260,#250261,
#250262,#250263,#250264,#250265,#250266,#250267,#250268,#250269,#250270,
#250271,#250272,#250273,#250274,#250275,#250276,#250277,#250278,#250279,
#250280,#250281,#250282,#250283,#250284),.UNSPECIFIED.,.F.,.F.,(4,3,3,3,
3,3,3,3,3,3,3,3,3,3,3,3,3,3,3,3,3,4),(0.146962374419461,0.147547046336026,
0.148127472789239,0.148704825740929,0.149280291284793,0.149855398739328,
0.150431147356518,0.151008540254158,0.151591055410951,0.152176891110784,
0.152770353285494,0.153238785047258,0.15383405187594,0.154422885444334,
0.155004864618472,0.155583500875027,0.156159817034624,0.156734823245514,
0.157310355761555,0.157886625174272,0.15846634810946,0.158932774246921),
 .UNSPECIFIED.);
#6225=B_SPLINE_CURVE_WITH_KNOTS('',3,(#250285,#250286,#250287,#250288,#250289,
#250290,#250291,#250292,#250293,#250294,#250295,#250296,#250297,#250298,
#250299,#250300,#250301,#250302,#250303,#250304,#250305,#250306,#250307,
#250308,#250309,#250310,#250311,#250312,#250313,#250314,#250315,#250316,
#250317,#250318,#250319,#250320,#250321),.UNSPECIFIED.,.F.,.F.,(4,3,3,3,
3,3,3,3,3,3,3,3,4),(0.,0.00148484200664636,0.0905231864990854,0.181211845999667,
0.273638712259328,0.367899711438529,0.562354567719848,0.662791026196378,
0.765550077502759,0.863546828921589,0.870788292842745,0.978680556821164,
1.),.UNSPECIFIED.);
#6226=B_SPLINE_CURVE_WITH_KNOTS('',3,(#250680,#250681,#250682,#250683,#250684,
#250685,#250686,#250687,#250688,#250689,#250690,#250691,#250692,#250693,
#250694,#250695,#250696,#250697,#250698,#250699,#250700,#250701,#250702,
#250703),.UNSPECIFIED.,.F.,.F.,(4,2,2,2,2,2,2,2,2,2,2,4),(-0.191299715244794,
-0.157661652097922,-0.125069220643887,-0.10269082405758,-0.102057729196898,
-0.10142671334636,-0.10017288684426,-0.0988724155437573,-0.0962033280839491,
-0.0705045556846333,-0.0201379948223164,0.),.UNSPECIFIED.);
#6227=B_SPLINE_CURVE_WITH_KNOTS('',3,(#251066,#251067,#251068,#251069,#251070,
#251071,#251072,#251073,#251074,#251075,#251076,#251077,#251078,#251079,
#251080,#251081,#251082,#251083,#251084,#251085,#251086,#251087,#251088,
#251089,#251090,#251091,#251092,#251093,#251094,#251095),.UNSPECIFIED.,
 .F.,.F.,(4,2,2,1,1,1,2,2,2,2,2,1,2,2,2,2,4),(0.,0.00781249999999989,0.015625,
0.0234375,0.03125,0.046875,0.0546875,0.0625,0.06640625,0.0703125,0.078125,
0.09375,0.109375,0.1171875,0.121093749999999,0.125,0.13856539019169),
 .UNSPECIFIED.);
#6228=B_SPLINE_CURVE_WITH_KNOTS('',3,(#251096,#251097,#251098,#251099,#251100,
#251101,#251102,#251103,#251104,#251105),.UNSPECIFIED.,.F.,.F.,(4,2,2,2,
4),(-0.173949783400974,-0.127702308831258,-0.0869385908804911,-0.0411391376925877,
-1.00000012467905E-6),.UNSPECIFIED.);
#6229=B_SPLINE_CURVE_WITH_KNOTS('',3,(#251468,#251469,#251470,#251471,#251472,
#251473,#251474,#251475,#251476,#251477,#251478,#251479,#251480,#251481,
#251482,#251483,#251484,#251485),.UNSPECIFIED.,.F.,.F.,(4,2,2,2,2,2,2,2,
4),(-0.333980240161851,-0.278002895178562,-0.207048595661841,-0.167393086348014,
-0.160091762120317,-0.159200052079505,-0.128005285823074,-0.0810446390995098,
-9.65957239584814E-7),.UNSPECIFIED.);
#6230=B_SPLINE_CURVE_WITH_KNOTS('',3,(#251486,#251487,#251488,#251489,#251490,
#251491,#251492,#251493,#251494,#251495,#251496,#251497,#251498,#251499,
#251500,#251501,#251502,#251503,#251504,#251505,#251506,#251507,#251508,
#251509,#251510,#251511,#251512,#251513,#251514,#251515,#251516,#251517,
#251518,#251519,#251520,#251521,#251522,#251523,#251524,#251525,#251526,
#251527,#251528,#251529,#251530,#251531,#251532,#251533,#251534),
 .UNSPECIFIED.,.F.,.F.,(4,3,3,3,3,3,3,3,3,3,3,3,3,3,3,3,4),(0.790138930296763,
0.792968750000001,0.796875,0.8125,0.828125,0.8359375,0.84375,0.8515625,
0.859375,0.875,0.890625,0.89453125,0.8984375,0.90625,0.9140625,0.921875,
0.932216014912642),.UNSPECIFIED.);
#6231=B_SPLINE_CURVE_WITH_KNOTS('',3,(#251535,#251536,#251537,#251538,#251539,
#251540,#251541,#251542,#251543,#251544,#251545,#251546,#251547,#251548,
#251549,#251550,#251551,#251552,#251553,#251554,#251555,#251556,#251557,
#251558,#251559,#251560),.UNSPECIFIED.,.F.,.F.,(4,2,2,2,2,2,2,2,2,2,2,2,
4),(-0.866661855593407,-0.708970781836436,-0.558780900260934,-0.401558682989752,
-0.298232076935225,-0.215863746327597,-0.199487234948257,-0.19136087774753,
-0.187332094114913,-0.185319962216916,-0.124545068875862,-0.062491088958267,
-1.00000010871959E-6),.UNSPECIFIED.);
#6232=B_SPLINE_CURVE_WITH_KNOTS('',3,(#252016,#252017,#252018,#252019,#252020,
#252021,#252022,#252023,#252024,#252025,#252026,#252027,#252028,#252029,
#252030,#252031,#252032,#252033,#252034,#252035),.UNSPECIFIED.,.F.,.F.,
(4,2,2,2,2,2,2,2,2,4),(-0.737343996452552,-0.644050018112871,-0.549473453853603,
-0.457744561332403,-0.36907523507599,-0.280277933358412,-0.193344737919196,
-0.105307046015033,-0.0528181412185139,0.),.UNSPECIFIED.);
#6233=B_SPLINE_CURVE_WITH_KNOTS('',3,(#253173,#253174,#253175,#253176,#253177,
#253178),.UNSPECIFIED.,.F.,.F.,(4,2,4),(-0.0951753096986671,-0.0475925862889819,
-1.05240395974435E-6),.UNSPECIFIED.);
#6234=B_SPLINE_CURVE_WITH_KNOTS('',3,(#253179,#253180,#253181,#253182,#253183,
#253184,#253185,#253186,#253187,#253188,#253189,#253190,#253191,#253192),
 .UNSPECIFIED.,.F.,.F.,(4,2,2,2,2,2,4),(0.,0.0445367209370214,0.0852877077239505,
0.158230060143529,0.214173442983221,0.243463509223617,0.271164771184466),
 .UNSPECIFIED.);
#6235=B_SPLINE_CURVE_WITH_KNOTS('',3,(#253193,#253194,#253195,#253196,#253197,
#253198,#253199,#253200,#253201,#253202,#253203,#253204,#253205,#253206,
#253207,#253208,#253209,#253210,#253211,#253212,#253213,#253214,#253215,
#253216,#253217,#253218,#253219,#253220,#253221,#253222,#253223,#253224,
#253225,#253226,#253227,#253228),.UNSPECIFIED.,.F.,.F.,(4,2,2,2,2,2,2,2,
2,2,2,2,2,2,2,2,2,4),(-1.4603242851032,-1.41057592975987,-1.33100660979353,
-1.25442360789161,-1.1747428461744,-1.09621833622064,-1.02009237475002,
-0.940394301350014,-0.862736537925816,-0.785548626949009,-0.705782504629548,
-0.62902379887815,-0.549265680452016,-0.470550628024444,-0.394484973247153,
-0.314815339999637,-0.236962458486878,-0.197604024225048),.UNSPECIFIED.);
#6236=B_SPLINE_CURVE_WITH_KNOTS('',3,(#253784,#253785,#253786,#253787,#253788,
#253789,#253790,#253791,#253792,#253793,#253794,#253795,#253796,#253797,
#253798,#253799,#253800,#253801,#253802,#253803,#253804,#253805),
 .UNSPECIFIED.,.F.,.F.,(4,2,2,2,2,2,2,2,2,2,4),(-0.640412608621221,-0.632596141832508,
-0.552965143807485,-0.474922049306285,-0.398448588061734,-0.318248999100166,
-0.241102613874202,-0.162757814574324,-0.0835743992560574,-0.0410491015749916,
-9.99999716144728E-7),.UNSPECIFIED.);
#6237=B_SPLINE_CURVE_WITH_KNOTS('',3,(#253806,#253807,#253808,#253809,#253810,
#253811,#253812,#253813,#253814,#253815),.UNSPECIFIED.,.F.,.F.,(4,2,2,2,
4),(-0.240375949776406,-0.18190588491853,-0.119969355086001,-0.0632948344662496,
-1.01531671729965E-6),.UNSPECIFIED.);
#6238=B_SPLINE_CURVE_WITH_KNOTS('',3,(#254370,#254371,#254372,#254373,#254374,
#254375,#254376,#254377,#254378,#254379,#254380,#254381,#254382,#254383),
 .UNSPECIFIED.,.F.,.F.,(4,2,2,2,2,2,4),(0.,0.0475788933783159,0.0933534150844901,
0.157993829184702,0.243152490202414,0.307867924694747,0.372920208810498),
 .UNSPECIFIED.);
#6239=B_SPLINE_CURVE_WITH_KNOTS('',3,(#254384,#254385,#254386,#254387,#254388,
#254389),.UNSPECIFIED.,.F.,.F.,(4,2,4),(-0.0551872851809273,-0.0258550695504278,
0.),.UNSPECIFIED.);
#6240=B_SPLINE_CURVE_WITH_KNOTS('',3,(#254390,#254391,#254392,#254393,#254394,
#254395,#254396,#254397,#254398,#254399,#254400,#254401,#254402,#254403),
 .UNSPECIFIED.,.F.,.F.,(4,2,2,2,2,2,4),(-22.8114091378978,-22.7546556945913,
-22.6963478192231,-22.6166081018008,-22.5403648384663,-22.4612431166947,
-22.4011363767123),.UNSPECIFIED.);
#6241=B_SPLINE_CURVE_WITH_KNOTS('',3,(#254407,#254408,#254409,#254410,#254411,
#254412,#254413,#254414,#254415,#254416,#254417,#254418,#254419,#254420,
#254421,#254422,#254423,#254424,#254425,#254426,#254427,#254428,#254429,
#254430,#254431,#254432,#254433,#254434,#254435,#254436,#254437,#254438,
#254439,#254440,#254441,#254442,#254443,#254444,#254445,#254446,#254447,
#254448,#254449,#254450,#254451,#254452,#254453,#254454,#254455,#254456,
#254457,#254458,#254459,#254460,#254461,#254462,#254463,#254464,#254465,
#254466,#254467,#254468,#254469,#254470,#254471,#254472,#254473,#254474,
#254475,#254476,#254477,#254478,#254479,#254480,#254481,#254482,#254483,
#254484,#254485,#254486,#254487,#254488,#254489,#254490,#254491,#254492,
#254493,#254494,#254495,#254496,#254497,#254498,#254499,#254500,#254501,
#254502,#254503),.UNSPECIFIED.,.F.,.F.,(4,3,3,3,3,3,3,3,3,3,3,3,3,3,3,3,
3,3,3,3,3,3,3,3,3,3,3,3,3,3,3,3,4),(0.585665352728702,0.58593750000017,
0.593750000000174,0.601562500000179,0.609375000000184,0.617187500000188,
0.625000000000193,0.632812500000197,0.636718750000199,0.640625000000202,
0.656250000000211,0.67187500000022,0.687500000000229,0.703125000000238,
0.718750000000247,0.726562500000251,0.734375000000256,0.742187500000261,
0.750000000000265,0.75781250000027,0.765625000000274,0.773437500000279,
0.781250000000283,0.789062500000288,0.79296875000029,0.796875000000292,
0.812500000000301,0.82812500000031,0.835937500000315,0.84375000000032,0.851562500000324,
0.859375000000329,0.860346605686114),.UNSPECIFIED.);
#6242=B_SPLINE_CURVE_WITH_KNOTS('',3,(#254504,#254505,#254506,#254507,#254508,
#254509,#254510,#254511,#254512,#254513,#254514,#254515,#254516,#254517,
#254518,#254519,#254520,#254521,#254522,#254523,#254524,#254525,#254526,
#254527,#254528,#254529,#254530,#254531,#254532,#254533,#254534,#254535,
#254536,#254537,#254538,#254539,#254540,#254541,#254542,#254543,#254544,
#254545,#254546,#254547,#254548,#254549,#254550,#254551,#254552,#254553,
#254554,#254555,#254556,#254557,#254558,#254559,#254560,#254561,#254562,
#254563,#254564,#254565,#254566,#254567),.UNSPECIFIED.,.F.,.F.,(4,3,3,3,
3,3,3,3,3,3,3,3,3,3,3,3,3,3,3,3,3,4),(0.146962376116165,0.147547047946169,
0.148127474319873,0.148704827199106,0.149280292681386,0.149855400081028,
0.150431148650181,0.151008541506803,0.151591056632366,0.152176892307433,
0.15277035446366,0.153238785047258,0.153834051806347,0.154422885335194,
0.155004864512828,0.155583500799316,0.156159817014816,0.156734823307263,
0.15731035594623,0.15788662550386,0.158466348626833,0.158932777953849),
 .UNSPECIFIED.);
#6243=B_SPLINE_CURVE_WITH_KNOTS('',3,(#254926,#254927,#254928,#254929,#254930,
#254931,#254932,#254933,#254934,#254935,#254936,#254937,#254938,#254939,
#254940,#254941,#254942,#254943,#254944,#254945,#254946,#254947),
 .UNSPECIFIED.,.F.,.F.,(4,2,2,2,2,2,2,2,2,2,4),(0.,0.0414487749299163,0.0701930279287442,
0.0896240078608044,0.090185540254589,0.0913147136737188,0.0936095790942993,
0.0959463008528485,0.118254097601967,0.162358043499866,0.197736906325247),
 .UNSPECIFIED.);
#6244=B_SPLINE_CURVE_WITH_KNOTS('',3,(#255307,#255308,#255309,#255310,#255311,
#255312,#255313,#255314,#255315,#255316,#255317,#255318,#255319,#255320,
#255321,#255322,#255323,#255324,#255325,#255326,#255327,#255328,#255329,
#255330,#255331,#255332,#255333,#255334,#255335,#255336,#255337,#255338,
#255339,#255340,#255341),.UNSPECIFIED.,.F.,.F.,(4,1,2,2,2,1,1,2,2,2,2,2,
2,2,2,2,2,1,1,4),(0.594033433120655,0.609374999999978,0.617187499999968,
0.624999999999957,0.632812499999947,0.640624999999936,0.656249999999915,
0.664062499999905,0.671874999999895,0.675781249999889,0.679687499999884,
0.687499999999874,0.703124999999853,0.718749999999832,0.722656249999827,
0.726562499999822,0.734374999999811,0.74999999999979,0.75781249999978,0.762507688533689),
 .UNSPECIFIED.);
#6245=B_SPLINE_CURVE_WITH_KNOTS('',3,(#255342,#255343,#255344,#255345,#255346,
#255347,#255348,#255349,#255350,#255351),.UNSPECIFIED.,.F.,.F.,(4,2,2,2,
4),(9.46482055419996E-7,0.0627301013079089,0.114566930226501,0.175834122904311,
0.228935107620853),.UNSPECIFIED.);
#6246=B_SPLINE_CURVE_WITH_KNOTS('',3,(#255352,#255353,#255354,#255355,#255356,
#255357),.UNSPECIFIED.,.F.,.F.,(4,2,4),(0.,0.0475563832059397,0.0951278725828074),
 .UNSPECIFIED.);
#6247=B_SPLINE_CURVE_WITH_KNOTS('',3,(#255720,#255721,#255722,#255723,#255724,
#255725),.UNSPECIFIED.,.F.,.F.,(4,2,4),(9.97452242539264E-7,0.0364245031687067,
0.072772555381456),.UNSPECIFIED.);
#6248=B_SPLINE_CURVE_WITH_KNOTS('',3,(#255961,#255962,#255963,#255964,#255965,
#255966,#255967,#255968,#255969,#255970,#255971,#255972,#255973,#255974,
#255975,#255976,#255977,#255978,#255979,#255980,#255981,#255982,#255983,
#255984,#255985,#255986,#255987,#255988,#255989,#255990,#255991,#255992,
#255993,#255994,#255995,#255996,#255997,#255998,#255999,#256000,#256001,
#256002,#256003,#256004,#256005,#256006,#256007,#256008,#256009,#256010,
#256011,#256012,#256013,#256014,#256015,#256016,#256017,#256018,#256019,
#256020,#256021,#256022,#256023,#256024,#256025,#256026,#256027,#256028,
#256029,#256030,#256031,#256032,#256033,#256034,#256035,#256036,#256037,
#256038,#256039,#256040,#256041,#256042,#256043,#256044,#256045,#256046,
#256047,#256048,#256049,#256050,#256051,#256052,#256053,#256054,#256055,
#256056,#256057,#256058,#256059,#256060,#256061,#256062,#256063,#256064,
#256065,#256066,#256067,#256068,#256069,#256070,#256071,#256072,#256073,
#256074,#256075,#256076),.UNSPECIFIED.,.F.,.F.,(4,2,2,2,2,2,2,2,2,2,2,2,
2,2,2,2,2,2,2,2,2,2,2,2,2,2,2,2,2,2,2,2,2,2,2,2,2,2,2,2,2,2,2,2,2,2,2,2,
2,2,2,2,2,2,2,2,2,4),(0.5,0.5078125,0.515625,0.53125,0.546875,0.5546875,
0.5625,0.5703125,0.578125,0.59375,0.6015625,0.609375,0.6171875,0.625,0.6328125,
0.640625,0.65625,0.6640625,0.671875,0.67578125,0.6796875,0.6875,0.703125,
0.71875,0.72265625,0.7265625,0.734375,0.7421875,0.75,0.7578125,0.765625,
0.7734375,0.78125,0.7890625,0.796875,0.8125,0.8203125,0.828125,0.8359375,
0.84375,0.859375,0.875,0.87890625,0.8828125,0.890625,0.8984375,0.90625,
0.921875,0.9296875,0.93359375,0.9375,0.9453125,0.953125,0.96875,0.9765625,
0.984375,0.9921875,1.),.UNSPECIFIED.);
#6249=B_SPLINE_CURVE_WITH_KNOTS('',3,(#256080,#256081,#256082,#256083,#256084,
#256085,#256086,#256087,#256088,#256089,#256090,#256091,#256092,#256093,
#256094,#256095,#256096,#256097,#256098),.UNSPECIFIED.,.F.,.F.,(4,2,2,2,
2,1,1,1,2,2,4),(0.928243302054433,0.9296875,0.933593749999999,0.9375,0.9453125,
0.953125,0.96875,0.9765625,0.984375,0.9921875,1.),.UNSPECIFIED.);
#6250=B_SPLINE_CURVE_WITH_KNOTS('',3,(#256099,#256100,#256101,#256102,#256103,
#256104,#256105,#256106,#256107,#256108,#256109,#256110,#256111,#256112,
#256113,#256114,#256115,#256116,#256117,#256118,#256119,#256120,#256121,
#256122,#256123,#256124,#256125,#256126,#256127,#256128,#256129,#256130,
#256131,#256132,#256133,#256134,#256135,#256136,#256137,#256138),
 .UNSPECIFIED.,.F.,.F.,(4,2,2,2,2,2,2,2,2,2,2,2,2,2,2,2,2,2,2,4),(0.0717572711999334,
0.0781250000000086,0.0937500000000291,0.101562500000039,0.10937500000005,
0.11718750000006,0.121093750000065,0.12500000000007,0.140625000000091,0.156250000000111,
0.164062500000122,0.171875000000132,0.179687500000142,0.187500000000153,
0.203125000000174,0.210937500000184,0.218750000000194,0.226562500000205,
0.234375000000214,0.237493805076694),.UNSPECIFIED.);
#6251=B_SPLINE_CURVE_WITH_KNOTS('',3,(#256720,#256721,#256722,#256723,#256724,
#256725,#256726,#256727,#256728,#256729,#256730,#256731,#256732,#256733,
#256734,#256735,#256736,#256737,#256738,#256739,#256740,#256741),
 .UNSPECIFIED.,.F.,.F.,(4,2,2,2,2,2,2,2,2,2,4),(9.08424390484079E-7,0.0696685016542001,
0.132515655806531,0.167139005391392,0.173548401015734,0.174327936224742,
0.175107609363997,0.202506476161798,0.243347745195621,0.326904360471616,
0.335458527233704),.UNSPECIFIED.);
#6252=B_SPLINE_CURVE_WITH_KNOTS('',3,(#257296,#257297,#257298,#257299,#257300,
#257301,#257302,#257303,#257304,#257305,#257306,#257307,#257308,#257309),
 .UNSPECIFIED.,.F.,.F.,(4,2,2,2,2,2,4),(0.,0.0445367209381238,0.0852877077272262,
0.158230060150209,0.214173442992252,0.243463509233813,0.271164771195753),
 .UNSPECIFIED.);
#6253=B_SPLINE_CURVE_WITH_KNOTS('',3,(#257310,#257311,#257312,#257313,#257314,
#257315,#257316,#257317,#257318,#257319,#257320,#257321,#257322,#257323,
#257324,#257325,#257326,#257327,#257328,#257329,#257330,#257331,#257332,
#257333,#257334,#257335,#257336,#257337,#257338,#257339,#257340,#257341,
#257342,#257343,#257344,#257345),.UNSPECIFIED.,.F.,.F.,(4,2,2,2,2,2,2,2,
2,2,2,2,2,2,2,2,2,4),(-1.77693741255607,-1.74337044899102,-1.66708872982112,
-1.58731865470844,-1.50900670182408,-1.43252339445671,-1.35203770301058,
-1.27462559370405,-1.19646251166751,-1.11699018971931,-1.04049309552052,
-0.96078663431139,-0.882360986508158,-0.806139075597756,-0.726405109641131,
-0.648849283597101,-0.571355699778421,-0.513010840582583),.UNSPECIFIED.);
#6254=B_SPLINE_CURVE_WITH_KNOTS('',3,(#257900,#257901,#257902,#257903,#257904,
#257905,#257906,#257907,#257908,#257909,#257910,#257911,#257912,#257913),
 .UNSPECIFIED.,.F.,.F.,(4,2,2,2,2,2,4),(9.99999933537955E-7,0.0396954777717048,
0.0807907164979224,0.159863856633394,0.238518326425717,0.315571821712752,
0.324863770283186),.UNSPECIFIED.);
#6255=B_SPLINE_CURVE_WITH_KNOTS('',3,(#257915,#257916,#257917,#257918,#257919,
#257920),.UNSPECIFIED.,.F.,.F.,(4,2,4),(0.,0.0473068317072604,0.0914569630334385),
 .UNSPECIFIED.);
#6256=B_SPLINE_CURVE_WITH_KNOTS('',3,(#257921,#257922,#257923,#257924,#257925,
#257926,#257927,#257928,#257929,#257930,#257931,#257932,#257933,#257934,
#257935,#257936,#257937,#257938,#257939,#257940,#257941,#257942,#257943,
#257944,#257945,#257946),.UNSPECIFIED.,.F.,.F.,(4,2,2,2,2,2,2,2,2,2,2,2,
4),(1.00000010012831E-6,0.0641700687511304,0.1509137744414,0.264210362010751,
0.330507922832673,0.332373878134189,0.334242797798112,0.338007256168076,
0.415092030263758,0.550891681219715,0.683444154698735,0.793447320497175,
0.915560088311105),.UNSPECIFIED.);
#6257=B_SPLINE_CURVE_WITH_KNOTS('',3,(#258501,#258502,#258503,#258504,#258505,
#258506,#258507,#258508,#258509,#258510,#258511,#258512,#258513,#258514),
 .UNSPECIFIED.,.F.,.F.,(4,2,2,2,2,2,4),(0.,0.0475788933774115,0.0933534150825772,
0.157993829182703,0.243152490201031,0.307867924694816,0.372920208811896),
 .UNSPECIFIED.);
#6258=B_SPLINE_CURVE_WITH_KNOTS('',3,(#258515,#258516,#258517,#258518,#258519,
#258520,#258521,#258522,#258523,#258524,#258525,#258526,#258527,#258528,
#258529,#258530,#258531,#258532,#258533,#258534,#258535,#258536),
 .UNSPECIFIED.,.F.,.F.,(4,2,2,2,2,2,2,2,2,2,4),(-22.7495119090184,-22.6891751763705,
-22.6272563246175,-22.5477571954083,-22.4714114519975,-22.3920931070546,
-22.3143022160145,-22.2370473604176,-22.1567200784823,-22.0805078797818,
-22.0249622838298),.UNSPECIFIED.);
#6259=B_SPLINE_CURVE_WITH_KNOTS('',3,(#258539,#258540,#258541,#258542,#258543,
#258544,#258545,#258546,#258547,#258548,#258549,#258550,#258551,#258552,
#258553,#258554,#258555,#258556,#258557,#258558),.UNSPECIFIED.,.F.,.F.,
(4,2,2,2,2,2,2,2,2,4),(0.600895783241409,0.601562500000476,0.609375000000422,
0.617187500000369,0.625000000000315,0.632812500000261,0.640625000000208,
0.648437500000154,0.6562500000001,0.670958963198009),.UNSPECIFIED.);
#6260=B_SPLINE_CURVE_WITH_KNOTS('',3,(#258560,#258561,#258562,#258563,#258564,
#258565,#258566,#258567,#258568,#258569,#258570,#258571,#258572,#258573,
#258574,#258575,#258576,#258577,#258578,#258579,#258580,#258581,#258582,
#258583,#258584,#258585,#258586,#258587,#258588,#258589,#258590,#258591,
#258592,#258593,#258594,#258595,#258596,#258597,#258598,#258599,#258600,
#258601,#258602,#258603,#258604,#258605,#258606,#258607,#258608,#258609,
#258610,#258611,#258612,#258613,#258614,#258615,#258616,#258617,#258618,
#258619,#258620,#258621,#258622,#258623),.UNSPECIFIED.,.F.,.F.,(4,3,3,3,
3,3,3,3,3,3,3,3,3,3,3,3,3,3,3,3,3,4),(0.146962336060241,0.147547010031667,
0.148127438310315,0.148704792860876,0.149280259664182,0.149855368171419,
0.150431117633161,0.151008511164717,0.151591026661658,0.15217686251404,
0.152770324644434,0.153238785047258,0.153834050607704,0.15442288381429,
0.155004863907804,0.155583501870188,0.156159820503461,0.156734829941232,
0.157310366903482,0.157886641401883,0.158466370708173,0.158932909601972),
 .UNSPECIFIED.);
#6261=B_SPLINE_CURVE_WITH_KNOTS('',3,(#258624,#258625,#258626,#258627,#258628,
#258629,#258630,#258631,#258632,#258633,#258634,#258635,#258636,#258637,
#258638,#258639,#258640,#258641,#258642,#258643,#258644,#258645,#258646,
#258647,#258648,#258649,#258650,#258651),.UNSPECIFIED.,.F.,.F.,(4,3,3,3,
3,3,3,3,3,4),(0.795736943641777,0.796875,0.8046875,0.8125,0.828124999999984,
0.835937499999979,0.843749999999974,0.851562499999969,0.859374999999964,
0.87563910993131),.UNSPECIFIED.);
#6262=B_SPLINE_CURVE_WITH_KNOTS('',3,(#258653,#258654,#258655,#258656,#258657,
#258658,#258659,#258660,#258661,#258662,#258663,#258664,#258665,#258666,
#258667,#258668,#258669,#258670,#258671,#258672,#258673,#258674,#258675,
#258676,#258677,#258678,#258679,#258680,#258681,#258682,#258683,#258684,
#258685,#258686,#258687,#258688),.UNSPECIFIED.,.F.,.F.,(4,2,2,2,2,2,2,2,
2,2,2,2,2,2,2,2,2,4),(0.828975078082139,0.879713519041278,0.958060620508997,
1.03775275544132,1.11403993721078,1.19323762107853,1.27156359459928,1.34872275498068,
1.42893628260974,1.50540420656939,1.58346020570364,1.66309517102489,1.73918274620376,
1.81809535814628,1.89705049108488,1.9739640560586,2.05390581774317,2.09124089524434),
 .UNSPECIFIED.);
#6263=B_SPLINE_CURVE_WITH_KNOTS('',3,(#258690,#258691,#258692,#258693,#258694,
#258695,#258696,#258697,#258698,#258699,#258700,#258701,#258702,#258703,
#258704,#258705,#258706,#258707,#258708,#258709,#258710,#258711,#258712,
#258713,#258714,#258715,#258716,#258717,#258718,#258719),.UNSPECIFIED.,
 .F.,.F.,(4,2,2,2,2,2,2,2,2,2,2,2,2,2,4),(21.7750720110093,21.8163550216855,
21.8962550811618,21.9731379982383,22.0526849055576,22.1315413187615,22.2076747786694,
22.2874065086602,22.3654017492244,22.4421433496673,22.5222824581149,22.5993806961363,
22.6782164764829,22.7484162072171,22.8170734816833),.UNSPECIFIED.);
#6264=B_SPLINE_CURVE_WITH_KNOTS('',3,(#258721,#258722,#258723,#258724,#258725,
#258726,#258727,#258728,#258729,#258730,#258731,#258732,#258733,#258734,
#258735,#258736,#258737,#258738,#258739,#258740,#258741,#258742,#258743,
#258744,#258745,#258746,#258747,#258748,#258749,#258750,#258751,#258752,
#258753,#258754,#258755,#258756,#258757,#258758,#258759,#258760,#258761,
#258762),.UNSPECIFIED.,.F.,.F.,(4,2,2,2,2,2,2,2,2,2,2,2,2,2,2,2,2,2,2,2,
4),(0.087011959968012,0.0937500000000087,0.101562500000008,0.109375000000007,
0.117187500000007,0.125000000000006,0.132812500000006,0.140625000000005,
0.156250000000003,0.164062500000003,0.171875000000002,0.175781250000002,
0.1796875,0.1875,0.203125,0.21875,0.2265625,0.234374999999998,0.242187499999997,
0.249999999999997,0.252776195245581),.UNSPECIFIED.);
#6265=B_SPLINE_CURVE_WITH_KNOTS('',3,(#258763,#258764,#258765,#258766),
 .UNSPECIFIED.,.F.,.F.,(4,4),(1.00000019201407E-6,0.00950822744729325),
 .UNSPECIFIED.);
#6266=B_SPLINE_CURVE_WITH_KNOTS('',3,(#259117,#259118,#259119,#259120,#259121,
#259122,#259123,#259124,#259125,#259126,#259127,#259128,#259129,#259130,
#259131,#259132,#259133,#259134,#259135,#259136,#259137,#259138),
 .UNSPECIFIED.,.F.,.F.,(4,2,2,2,2,2,2,2,2,2,4),(0.,0.0407060625625224,0.0695287735504407,
0.0890141598140192,0.0901238371088544,0.0912415302284534,0.0935209638282502,
0.0958498997334589,0.118224510663079,0.161531293622999,0.199451543342295),
 .UNSPECIFIED.);
#6267=B_SPLINE_CURVE_WITH_KNOTS('',3,(#259489,#259490,#259491,#259492,#259493,
#259494,#259495,#259496,#259497,#259498,#259499,#259500,#259501,#259502,
#259503,#259504,#259505,#259506,#259507,#259508,#259509,#259510,#259511,
#259512,#259513,#259514,#259515,#259516,#259517,#259518,#259519),
 .UNSPECIFIED.,.F.,.F.,(4,1,1,2,2,2,2,1,2,2,2,1,1,2,2,2,1,1,4),(0.578748721371666,
0.59375,0.6015625,0.609375,0.6171875,0.625,0.640625,0.65625,0.6640625,0.671875,
0.6796875,0.6875,0.703125,0.7109375,0.71875,0.7265625,0.734375,0.7421875,
0.747223819417002),.UNSPECIFIED.);
#6268=B_SPLINE_CURVE_WITH_KNOTS('',3,(#259520,#259521,#259522,#259523,#259524,
#259525,#259526,#259527,#259528,#259529),.UNSPECIFIED.,.F.,.F.,(4,2,2,2,
4),(1.0000844347723E-6,0.0627354187718775,0.114609893887245,0.175887326420162,
0.228995408318134),.UNSPECIFIED.);
#6269=B_SPLINE_CURVE_WITH_KNOTS('',3,(#259530,#259531,#259532,#259533,#259534,
#259535),.UNSPECIFIED.,.F.,.F.,(4,2,4),(0.,0.0474595169994712,0.0948138149984923),
 .UNSPECIFIED.);
#6270=B_SPLINE_CURVE_WITH_KNOTS('',3,(#259890,#259891,#259892,#259893,#259894,
#259895),.UNSPECIFIED.,.F.,.F.,(4,2,4),(1.03839813943911E-6,0.0231962182546486,
0.0535038699466261),.UNSPECIFIED.);
#6271=B_SPLINE_CURVE_WITH_KNOTS('',3,(#260127,#260128,#260129,#260130,#260131,
#260132,#260133,#260134,#260135,#260136,#260137,#260138,#260139,#260140,
#260141,#260142,#260143,#260144,#260145,#260146,#260147,#260148,#260149,
#260150,#260151,#260152,#260153,#260154,#260155,#260156,#260157,#260158,
#260159,#260160,#260161,#260162,#260163,#260164,#260165,#260166,#260167,
#260168,#260169,#260170,#260171,#260172,#260173,#260174,#260175,#260176,
#260177,#260178,#260179,#260180,#260181,#260182,#260183,#260184,#260185,
#260186,#260187,#260188,#260189,#260190,#260191,#260192,#260193,#260194,
#260195,#260196,#260197,#260198,#260199,#260200,#260201,#260202,#260203,
#260204,#260205,#260206,#260207,#260208,#260209,#260210,#260211,#260212,
#260213,#260214,#260215,#260216,#260217,#260218,#260219,#260220,#260221,
#260222,#260223,#260224,#260225,#260226,#260227,#260228,#260229,#260230,
#260231,#260232,#260233,#260234,#260235,#260236,#260237,#260238,#260239,
#260240),.UNSPECIFIED.,.F.,.F.,(4,2,2,2,2,2,2,2,2,2,2,2,2,2,2,2,2,2,2,2,
2,2,2,2,2,2,2,2,2,2,2,2,2,2,2,2,2,2,2,2,2,2,2,2,2,2,2,2,2,2,2,2,2,2,2,2,
4),(0.5,0.5078125,0.515625,0.53125,0.546875,0.5546875,0.5625,0.56640625,
0.5703125,0.578125,0.59375,0.6015625,0.609375,0.6171875,0.625,0.640625,
0.65625,0.6640625,0.671875,0.6796875,0.6875,0.703125,0.7109375,0.71875,
0.7265625,0.734375,0.7421875,0.75,0.7578125,0.765625,0.7734375,0.78125,
0.796875,0.8125,0.8203125,0.82421875,0.828125,0.8359375,0.84375,0.859375,
0.8671875,0.875,0.8828125,0.890625,0.8984375,0.90625,0.921875,0.9296875,
0.93359375,0.9375,0.9453125,0.953125,0.96875,0.984375,0.98828125,0.9921875,
1.),.UNSPECIFIED.);
#6272=B_SPLINE_CURVE_WITH_KNOTS('',3,(#260243,#260244,#260245,#260246,#260247,
#260248,#260249,#260250,#260251,#260252,#260253,#260254,#260255,#260256,
#260257,#260258,#260259,#260260,#260261,#260262,#260263,#260264,#260265,
#260266,#260267,#260268,#260269,#260270,#260271,#260272,#260273,#260274,
#260275,#260276),.UNSPECIFIED.,.F.,.F.,(4,3,3,3,3,3,3,3,3,3,3,4),(0.912988518764536,
0.921875,0.9296875,0.933593749999993,0.9375,0.945312519622535,0.953125,
0.96875,0.984375,0.988281249999999,0.9921875,1.),.UNSPECIFIED.);
#6273=B_SPLINE_CURVE_WITH_KNOTS('',3,(#260858,#260859,#260860,#260861,#260862,
#260863,#260864,#260865,#260866,#260867,#260868,#260869,#260870,#260871,
#260872,#260873,#260874,#260875,#260876,#260877,#260878,#260879),
 .UNSPECIFIED.,.F.,.F.,(4,2,2,2,2,2,2,2,2,2,4),(9.99997572121511E-7,0.0698852730817763,
0.132684785041426,0.167356797468204,0.173651470712272,0.174417517076423,
0.175184206163386,0.202554827937819,0.242523180847451,0.332118763813277,
0.335590797498318),.UNSPECIFIED.);
#6274=B_SPLINE_CURVE_WITH_KNOTS('',3,(#261434,#261435,#261436,#261437,#261438,
#261439,#261440,#261441,#261442,#261443,#261444,#261445,#261446,#261447),
 .UNSPECIFIED.,.F.,.F.,(4,2,2,2,2,2,4),(0.,0.0445367209372115,0.0852877077244626,
0.158230060144531,0.214173442984663,0.243463509225319,0.271164771186406),
 .UNSPECIFIED.);
#6275=B_SPLINE_CURVE_WITH_KNOTS('',3,(#262003,#262004,#262005,#262006,#262007,
#262008),.UNSPECIFIED.,.F.,.F.,(4,2,4),(1.00000011194028E-6,0.057300026554469,
0.11061517160577),.UNSPECIFIED.);
#6276=B_SPLINE_CURVE_WITH_KNOTS('',3,(#262009,#262010,#262011,#262012,#262013,
#262014,#262015,#262016,#262017,#262018,#262019,#262020,#262021,#262022,
#262023,#262024,#262025,#262026,#262027,#262028,#262029,#262030,#262031,
#262032,#262033,#262034,#262035,#262036),.UNSPECIFIED.,.F.,.F.,(4,2,2,2,
2,2,2,2,2,2,2,2,2,4),(1.00000011188427E-6,0.0832221019749246,0.173855357223232,
0.285282254196699,0.350899698372918,0.352769583200478,0.356527952715664,
0.364166049206607,0.380007478352134,0.401208730960821,0.52557169063662,
0.65515458631013,0.741483348095175,0.817065929829985),.UNSPECIFIED.);
#6277=B_SPLINE_CURVE_WITH_KNOTS('',3,(#262591,#262592,#262593,#262594,#262595,
#262596,#262597,#262598,#262599,#262600,#262601,#262602,#262603,#262604),
 .UNSPECIFIED.,.F.,.F.,(4,2,2,2,2,2,4),(0.,0.0475788933775829,0.0933534150829525,
0.157993829183029,0.243152490201361,0.307867924693099,0.372920208808051),
 .UNSPECIFIED.);
#6278=B_SPLINE_CURVE_WITH_KNOTS('',3,(#262607,#262608,#262609,#262610,#262611,
#262612,#262613,#262614),.UNSPECIFIED.,.F.,.F.,(4,2,2,4),(-0.102619939297055,
-0.0761483982920385,-0.0380341424800056,-1.07959900090539E-6),
 .UNSPECIFIED.);
#6279=B_SPLINE_CURVE_WITH_KNOTS('',3,(#262616,#262617,#262618,#262619,#262620,
#262621,#262622,#262623,#262624,#262625,#262626,#262627,#262628,#262629,
#262630,#262631,#262632,#262633,#262634,#262635,#262636,#262637,#262638,
#262639,#262640,#262641,#262642,#262643),.UNSPECIFIED.,.F.,.F.,(4,3,3,3,
3,3,3,3,3,4),(5.74832516592867E-8,0.100019677399835,0.215425485139183,0.32964672174934,
0.44270341057891,0.554615368045972,0.665402183763977,0.775083203425616,
0.88367751419001,0.99999990291026),.UNSPECIFIED.);
#6280=B_SPLINE_CURVE_WITH_KNOTS('',3,(#262644,#262645,#262646,#262647,#262648,
#262649,#262650,#262651,#262652,#262653,#262654,#262655,#262656,#262657),
 .UNSPECIFIED.,.F.,.F.,(4,2,2,2,2,2,4),(9.94972903414894E-7,0.0412659037688975,
0.0833228578270448,0.163008146711966,0.239131811149326,0.317616589247055,
0.349058981567732),.UNSPECIFIED.);
#6281=B_SPLINE_CURVE_WITH_KNOTS('',3,(#262659,#262660,#262661,#262662,#262663,
#262664,#262665,#262666,#262667,#262668,#262669,#262670,#262671,#262672,
#262673,#262674,#262675,#262676,#262677,#262678,#262679,#262680,#262681,
#262682,#262683,#262684,#262685,#262686,#262687,#262688,#262689,#262690,
#262691,#262692,#262693,#262694),.UNSPECIFIED.,.F.,.F.,(4,2,2,2,2,2,2,2,
2,2,2,2,2,2,2,2,2,4),(1.14417183100891,1.20287505491137,1.28033601080281,
1.35790068856985,1.4376299732138,1.51383997385877,1.59227414974943,1.67197682977705,
1.74848112168798,1.82796165173032,1.90608212512207,1.98350055193403,2.06399395345673,
2.14045668174614,2.21877507056622,2.29853639318799,2.37481934054265,2.40800177534909),
 .UNSPECIFIED.);
#6282=B_SPLINE_CURVE_WITH_KNOTS('',3,(#262695,#262696,#262697,#262698,#262699,
#262700,#262701,#262702,#262703,#262704,#262705,#262706,#262707,#262708,
#262709,#262710,#262711,#262712,#262713,#262714,#262715,#262716,#262717,
#262718,#262719,#262720,#262721,#262722,#262723,#262724,#262725,#262726,
#262727,#262728,#262729,#262730,#262731,#262732),.UNSPECIFIED.,.F.,.F.,
(4,2,2,2,2,2,2,2,2,2,2,2,2,2,2,2,2,2,4),(21.4212632201289,21.4213907374562,
21.4986585247935,21.5762333053668,21.6555728240449,21.7319353477459,21.8113971171506,
21.8896946695694,21.9656166308523,22.0450966603124,22.122529601833,22.1995293602665,
22.2790633827883,22.3555994802065,22.4351823980347,22.513666830597,22.5895218629738,
22.6689712527135,22.6805778338202),.UNSPECIFIED.);
#6283=B_SPLINE_CURVE_WITH_KNOTS('',3,(#263083,#263084,#263085,#263086,#263087,
#263088,#263089,#263090,#263091,#263092,#263093,#263094,#263095,#263096,
#263097,#263098,#263099,#263100,#263101,#263102,#263103,#263104,#263105,
#263106),.UNSPECIFIED.,.F.,.F.,(4,2,2,2,2,2,2,2,2,2,2,4),(-0.166809588212098,
-0.148843254996767,-0.125453562572242,-0.102931760276549,-0.102285580484546,
-0.101637831913971,-0.100331074316472,-0.099014130685927,-0.0963279314427469,
-0.0707416722561485,-0.0202992977557707,0.),.UNSPECIFIED.);
#6284=B_SPLINE_CURVE_WITH_KNOTS('',3,(#263460,#263461,#263462,#263463,#263464,
#263465,#263466,#263467,#263468,#263469,#263470,#263471,#263472,#263473,
#263474,#263475,#263476,#263477,#263478,#263479,#263480,#263481,#263482,
#263483,#263484,#263485,#263486,#263487,#263488,#263489,#263490),
 .UNSPECIFIED.,.F.,.F.,(4,2,2,2,2,1,2,2,2,2,2,1,2,2,2,1,4),(0.,0.00781249999998982,
0.0117187499999848,0.0156249999999797,0.0312499999999596,0.0468749999999394,
0.0624999999999192,0.0664062499999142,0.0703124999999091,0.0781249999998989,
0.0937499999998787,0.101562499999869,0.117187499999848,0.124999999999838,
0.132812499999828,0.140624999999818,0.153862286619807),.UNSPECIFIED.);
#6285=B_SPLINE_CURVE_WITH_KNOTS('',3,(#263491,#263492,#263493,#263494,#263495,
#263496,#263497,#263498,#263499,#263500),.UNSPECIFIED.,.F.,.F.,(4,2,2,2,
4),(-0.103716212520426,-0.0778648817986832,-0.0553429806067814,-0.0297234386418945,
-9.99979852549906E-7),.UNSPECIFIED.);
#6286=B_SPLINE_CURVE_WITH_KNOTS('',3,(#263855,#263856,#263857,#263858,#263859,
#263860,#263861,#263862,#263863,#263864,#263865,#263866,#263867,#263868,
#263869,#263870,#263871,#263872,#263873,#263874),.UNSPECIFIED.,.F.,.F.,
(4,2,2,2,2,2,2,2,2,4),(-0.286833505370044,-0.256117950648564,-0.206802564626801,
-0.16737932509528,-0.16372205833922,-0.160109502717139,-0.159218025502164,
-0.1276378189132,-0.0816572572313796,-9.901146603708E-7),.UNSPECIFIED.);
#6287=B_SPLINE_CURVE_WITH_KNOTS('',3,(#263875,#263876,#263877,#263878,#263879,
#263880,#263881,#263882,#263883,#263884,#263885,#263886,#263887,#263888,
#263889,#263890,#263891,#263892,#263893,#263894,#263895,#263896,#263897),
 .UNSPECIFIED.,.F.,.F.,(4,1,1,2,2,2,2,1,2,2,1,1,1,1,4),(0.805330004638041,
0.8125,0.828125,0.8359375,0.84375,0.8515625,0.859375,0.875,0.890625,0.8984375,
0.90625,0.9140625,0.921875,0.9375,0.947453465595126),.UNSPECIFIED.);
#6288=B_SPLINE_CURVE_WITH_KNOTS('',3,(#263898,#263899,#263900,#263901,#263902,
#263903,#263904,#263905,#263906,#263907,#263908,#263909,#263910,#263911,
#263912,#263913,#263914,#263915,#263916,#263917,#263918,#263919,#263920,
#263921,#263922,#263923,#263924,#263925),.UNSPECIFIED.,.F.,.F.,(4,2,2,2,
2,2,2,2,2,2,2,2,2,4),(-0.57555153577955,-0.481403152518014,-0.391518410394815,
-0.304012543115108,-0.248875154314629,-0.20331457493217,-0.193640973353304,
-0.192462380537007,-0.191871804250229,-0.172674099621673,-0.162424596047124,
-0.0875987710768544,-0.0434789311703104,-1.00000008174117E-6),
 .UNSPECIFIED.);
#6289=B_SPLINE_CURVE_WITH_KNOTS('',3,(#264377,#264378,#264379,#264380,#264381,
#264382,#264383,#264384,#264385,#264386,#264387,#264388,#264389,#264390,
#264391,#264392,#264393,#264394,#264395,#264396),.UNSPECIFIED.,.F.,.F.,
(4,2,2,2,2,2,2,2,2,4),(-0.737111713840115,-0.641804134708795,-0.547885152214752,
-0.45702238184443,-0.368891693747479,-0.280602623811107,-0.193827199088049,
-0.105057099212705,-0.0527008074164365,0.),.UNSPECIFIED.);
#6290=B_SPLINE_CURVE_WITH_KNOTS('',3,(#264400,#264401,#264402,#264403,#264404,
#264405,#264406,#264407,#264408,#264409,#264410,#264411,#264412,#264413),
 .UNSPECIFIED.,.F.,.F.,(4,2,2,2,2,2,4),(0.,0.0475788933774156,0.0933534150825965,
0.157993829182779,0.243152490201106,0.307867924695236,0.372920208812621),
 .UNSPECIFIED.);
#6291=B_SPLINE_CURVE_WITH_KNOTS('',3,(#264414,#264415,#264416,#264417,#264418,
#264419,#264420,#264421,#264422,#264423,#264424,#264425,#264426,#264427),
 .UNSPECIFIED.,.F.,.F.,(4,2,2,2,2,2,4),(0.,0.0445367209371377,0.0852877077243032,
0.158230060144259,0.214173442984407,0.243463509225075,0.271164771186191),
 .UNSPECIFIED.);
#6292=B_SPLINE_CURVE_WITH_KNOTS('',3,(#265563,#265564,#265565,#265566,#265567,
#265568),.UNSPECIFIED.,.F.,.F.,(4,2,4),(-0.0951503607589064,-0.0475879046034892,
-1.01889197450439E-6),.UNSPECIFIED.);
#6293=B_SPLINE_CURVE_WITH_KNOTS('',3,(#266123,#266124,#266125,#266126,#266127,
#266128,#266129,#266130,#266131,#266132),.UNSPECIFIED.,.F.,.F.,(4,2,2,2,
4),(-0.222459738018975,-0.168926717083018,-0.11127636113476,-0.0584376614951339,
-9.93245333813508E-7),.UNSPECIFIED.);
#6294=B_SPLINE_CURVE_WITH_KNOTS('',3,(#266687,#266688,#266689,#266690,#266691,
#266692),.UNSPECIFIED.,.F.,.F.,(4,2,4),(-0.0369392618720219,-0.0184680082272592,
0.),.UNSPECIFIED.);
#6295=B_SPLINE_CURVE_WITH_KNOTS('',3,(#266695,#266696,#266697,#266698,#266699,
#266700,#266701,#266702,#266703,#266704),.UNSPECIFIED.,.F.,.F.,(4,2,2,2,
4),(2.44533830141617E-8,0.0529928666678925,0.105880759966484,0.158840335145018,
0.211973983367163),.UNSPECIFIED.);
#6296=B_SPLINE_CURVE_WITH_KNOTS('',3,(#266706,#266707,#266708,#266709,#266710,
#266711,#266712,#266713,#266714,#266715,#266716,#266717,#266718,#266719,
#266720,#266721,#266722,#266723,#266724,#266725,#266726,#266727,#266728,
#266729,#266730,#266731,#266732,#266733,#266734,#266735,#266736,#266737,
#266738,#266739,#266740,#266741,#266742,#266743,#266744,#266745,#266746,
#266747,#266748,#266749,#266750,#266751,#266752,#266753,#266754,#266755,
#266756,#266757,#266758,#266759,#266760,#266761,#266762,#266763,#266764,
#266765,#266766,#266767,#266768,#266769,#266770,#266771,#266772,#266773,
#266774,#266775,#266776,#266777,#266778,#266779,#266780,#266781,#266782,
#266783,#266784,#266785,#266786,#266787,#266788,#266789,#266790,#266791,
#266792,#266793,#266794,#266795,#266796,#266797,#266798,#266799,#266800,
#266801,#266802,#266803,#266804,#266805,#266806,#266807,#266808,#266809,
#266810,#266811,#266812,#266813,#266814,#266815,#266816,#266817),
 .UNSPECIFIED.,.F.,.F.,(4,2,2,2,2,2,2,2,2,2,2,2,2,2,2,2,2,2,2,2,2,2,2,2,
2,2,2,2,2,2,2,2,2,2,2,2,2,2,2,2,2,2,2,2,2,2,2,2,2,2,2,2,2,2,2,4),(0.,0.0078125,
0.015625,0.03125,0.046875,0.0625,0.078125,0.0859375,0.09375,0.1015625,0.109375,
0.1171875,0.125,0.140625,0.1484375,0.15625,0.1640625,0.171875,0.1875,0.1953125,
0.203125,0.2109375,0.21875,0.2265625,0.234375,0.2421875,0.25,0.2578125,
0.265625,0.28125,0.296875,0.3046875,0.30859375,0.3125,0.3203125,0.328125,
0.34375,0.3515625,0.359375,0.3671875,0.375,0.3828125,0.390625,0.3984375,
0.40625,0.4140625,0.421875,0.4296875,0.4375,0.453125,0.4609375,0.46875,
0.4765625,0.484375,0.4921875,0.5),.UNSPECIFIED.);
#6297=B_SPLINE_CURVE_WITH_KNOTS('',3,(#266818,#266819,#266820,#266821,#266822,
#266823,#266824,#266825,#266826,#266827,#266828,#266829,#266830,#266831,
#266832,#266833,#266834,#266835,#266836,#266837),.UNSPECIFIED.,.F.,.F.,
(4,2,2,2,2,2,2,2,2,4),(-0.737771146043194,-0.6422087309344,-0.548787649635823,
-0.457895273356038,-0.369025600510949,-0.28011278264437,-0.191911802745247,
-0.102744293435205,-0.0513522263156295,0.),.UNSPECIFIED.);
#6298=B_SPLINE_CURVE_WITH_KNOTS('',3,(#266838,#266839,#266840,#266841,#266842,
#266843,#266844,#266845,#266846,#266847,#266848,#266849,#266850,#266851,
#266852,#266853,#266854,#266855,#266856,#266857),.UNSPECIFIED.,.F.,.F.,
(4,2,2,2,2,2,2,2,2,4),(-0.738072505252876,-0.643967634208436,-0.550034248922507,
-0.458427614573009,-0.369107138036355,-0.279727670045679,-0.191507430126554,
-0.102692762879055,-0.0513175343902644,0.),.UNSPECIFIED.);
#6299=B_SPLINE_CURVE_WITH_KNOTS('',3,(#266858,#266859,#266860,#266861,#266862,
#266863,#266864,#266865,#266866,#266867,#266868,#266869,#266870,#266871,
#266872,#266873,#266874,#266875,#266876,#266877,#266878,#266879,#266880,
#266881,#266882,#266883,#266884,#266885,#266886,#266887,#266888,#266889,
#266890,#266891,#266892,#266893,#266894,#266895,#266896,#266897,#266898,
#266899,#266900,#266901,#266902,#266903,#266904,#266905,#266906,#266907,
#266908,#266909,#266910,#266911,#266912,#266913,#266914,#266915,#266916,
#266917,#266918,#266919,#266920,#266921,#266922,#266923,#266924,#266925,
#266926,#266927,#266928,#266929,#266930,#266931,#266932,#266933,#266934,
#266935,#266936,#266937,#266938,#266939,#266940,#266941,#266942,#266943,
#266944,#266945,#266946,#266947,#266948,#266949,#266950,#266951,#266952,
#266953,#266954,#266955,#266956,#266957,#266958,#266959,#266960,#266961,
#266962,#266963,#266964,#266965,#266966,#266967,#266968,#266969),
 .UNSPECIFIED.,.F.,.F.,(4,2,2,2,2,2,2,2,2,2,2,2,2,2,2,2,2,2,2,2,2,2,2,2,
2,2,2,2,2,2,2,2,2,2,2,2,2,2,2,2,2,2,2,2,2,2,2,2,2,2,2,2,2,2,2,4),(0.,0.0078125,
0.015625,0.03125,0.0390625,0.046875,0.0546875,0.0625,0.078125,0.0859375,
0.09375,0.1015625,0.10546875,0.109375,0.125,0.140625,0.1484375,0.15625,
0.1640625,0.171875,0.1875,0.203125,0.20703125,0.2109375,0.21875,0.2265625,
0.234375,0.2421875,0.25,0.2578125,0.265625,0.2734375,0.28125,0.296875,0.3125,
0.328125,0.34375,0.359375,0.36328125,0.3671875,0.375,0.3828125,0.390625,
0.3984375,0.40625,0.4140625,0.421875,0.4296875,0.4375,0.453125,0.4609375,
0.46875,0.4765625,0.484375,0.4921875,0.5),.UNSPECIFIED.);
#6300=B_SPLINE_CURVE_WITH_KNOTS('',3,(#267419,#267420,#267421,#267422,#267423,
#267424,#267425,#267426,#267427,#267428,#267429,#267430,#267431,#267432,
#267433,#267434,#267435,#267436,#267437,#267438,#267439,#267440,#267441,
#267442,#267443,#267444,#267445,#267446,#267447,#267448,#267449,#267450,
#267451,#267452,#267453,#267454,#267455,#267456,#267457,#267458,#267459,
#267460,#267461,#267462,#267463,#267464,#267465,#267466,#267467,#267468,
#267469,#267470,#267471,#267472,#267473,#267474,#267475,#267476,#267477,
#267478,#267479),.UNSPECIFIED.,.F.,.F.,(4,3,3,3,3,3,3,3,3,3,3,3,3,3,3,3,
3,3,3,3,4),(0.31954923250906,0.3203125,0.328125,0.3359375,0.34375,0.359375,
0.375,0.3828125,0.390625,0.3984375,0.40625,0.421875,0.4296875,0.43359375,
0.4375,0.4453125,0.453125,0.46875,0.484375,0.4921875,0.5),.UNSPECIFIED.);
#6301=B_SPLINE_CURVE_WITH_KNOTS('',3,(#268404,#268405,#268406,#268407,#268408,
#268409,#268410,#268411,#268412,#268413,#268414,#268415,#268416,#268417,
#268418,#268419,#268420,#268421,#268422,#268423),.UNSPECIFIED.,.F.,.F.,
(4,1,2,2,2,1,1,1,2,2,2,4),(0.399104234309458,0.406249999999556,0.414062499999593,
0.42187499999963,0.429687499999667,0.437499999999704,0.453124999999778,
0.460937499999815,0.468749999999852,0.476562499999889,0.484374999999926,
0.5),.UNSPECIFIED.);
#6302=B_SPLINE_CURVE_WITH_KNOTS('',3,(#268424,#268425,#268426,#268427,#268428,
#268429,#268430,#268431,#268432,#268433,#268434,#268435,#268436,#268437,
#268438,#268439),.UNSPECIFIED.,.F.,.F.,(4,1,1,2,1,1,1,1,2,2,4),(0.,0.0156250000000065,
0.031250000000013,0.0468750000000195,0.062500000000026,0.0781250000000325,
0.0859375000000357,0.0937500000000389,0.101562500000042,0.109375000000045,
0.12436089589415),.UNSPECIFIED.);
#6303=B_SPLINE_CURVE_WITH_KNOTS('',3,(#269365,#269366,#269367,#269368,#269369,
#269370,#269371,#269372,#269373,#269374,#269375,#269376,#269377,#269378,
#269379,#269380,#269381,#269382,#269383,#269384,#269385,#269386,#269387,
#269388,#269389,#269390,#269391,#269392,#269393,#269394,#269395),
 .UNSPECIFIED.,.F.,.F.,(4,3,3,3,3,3,3,3,3,3,4),(0.414335116362591,0.421874999999847,
0.429687494127349,0.437499994567745,0.453124999999908,0.460937499999924,
0.468749999999939,0.476562499999954,0.484374999999969,0.492187500000011,
0.5),.UNSPECIFIED.);
#6304=B_SPLINE_CURVE_WITH_KNOTS('',3,(#269396,#269397,#269398,#269399,#269400,
#269401,#269402,#269403,#269404,#269405,#269406,#269407,#269408,#269409,
#269410,#269411,#269412,#269413,#269414,#269415,#269416,#269417,#269418,
#269419,#269420,#269421,#269422,#269423,#269424,#269425,#269426,#269427,
#269428,#269429,#269430,#269431,#269432,#269433,#269434,#269435,#269436,
#269437,#269438,#269439,#269440,#269441),.UNSPECIFIED.,.F.,.F.,(4,3,3,3,
3,3,3,3,3,3,3,3,3,3,3,4),(0.,0.00781249973784698,0.0156249998843613,0.0312499999999252,
0.0390624999999065,0.0468749999998878,0.0546874999998691,0.0624999999998504,
0.0781249961571057,0.0859374423201947,0.0937499720252506,0.101562499999757,
0.105468749999748,0.109374999999738,0.124999992316058,0.139651873775064),
 .UNSPECIFIED.);
#6305=B_SPLINE_CURVE_WITH_KNOTS('',3,(#270291,#270292,#270293,#270294,#270295,
#270296,#270297,#270298,#270299,#270300,#270301,#270302,#270303,#270304,
#270305,#270306,#270307,#270308,#270309,#270310,#270311,#270312,#270313,
#270314,#270315,#270316,#270317,#270318,#270319,#270320,#270321,#270322,
#270323,#270324,#270325,#270326,#270327,#270328,#270329,#270330,#270331,
#270332,#270333,#270334,#270335,#270336,#270337,#270338,#270339,#270340,
#270341,#270342,#270343,#270344,#270345,#270346,#270347,#270348,#270349,
#270350,#270351,#270352,#270353,#270354,#270355,#270356,#270357),
 .UNSPECIFIED.,.F.,.F.,(4,3,3,3,3,3,3,3,3,3,3,3,3,3,3,3,3,3,3,3,3,3,4),
(0.304282083218851,0.3125,0.3203125,0.32421875,0.328125,0.3359375,0.34374999988077,
0.359375,0.3671875,0.375,0.3828125,0.390625,0.39843756172038,0.40625,0.421875,
0.4296875,0.4375,0.4453125,0.453125,0.46875,0.484375,0.4921875,0.5),
 .UNSPECIFIED.);
#6929=CONICAL_SURFACE('',#94083,1.47499999999998,0.785398163397455);
#6930=CONICAL_SURFACE('',#94094,1.47499999999998,0.785398163397455);
#6931=CONICAL_SURFACE('',#94695,58.3875000000295,0.436332312998583);
#6932=CONICAL_SURFACE('',#94706,58.3875000000295,0.436332312998583);
#6933=CONICAL_SURFACE('',#94724,58.3875000000295,0.436332312998583);
#6934=CONICAL_SURFACE('',#94752,58.3875000000295,0.436332312998583);
#6935=CONICAL_SURFACE('',#94763,58.3875000000295,0.436332312998583);
#6936=CONICAL_SURFACE('',#94786,58.3875000000295,0.436332312998583);
#6937=CONICAL_SURFACE('',#94804,58.3875000000295,0.436332312998583);
#6938=CONICAL_SURFACE('',#94815,58.3875000000295,0.436332312998583);
#6939=CONICAL_SURFACE('',#94831,58.3875000000295,0.436332312998583);
#6940=CONICAL_SURFACE('',#94842,58.3875000000295,0.436332312998583);
#6941=CONICAL_SURFACE('',#94860,58.3875000000295,0.436332312998583);
#6942=CONICAL_SURFACE('',#95152,58.5,0.436332312998583);
#6943=CONICAL_SURFACE('',#95160,58.5,0.436332312998583);
#6944=CONICAL_SURFACE('',#95165,58.5,0.436332312998583);
#6945=CONICAL_SURFACE('',#95230,58.3875000000295,0.436332312998583);
#6946=CONICAL_SURFACE('',#95513,58.3875000000295,0.436332312998583);
#6947=CONICAL_SURFACE('',#95657,58.3875000000295,0.436332312998583);
#6948=CONICAL_SURFACE('',#95705,58.3875000000295,0.436332312998583);
#6949=CONICAL_SURFACE('',#95927,58.5,0.436332312998583);
#6950=CONICAL_SURFACE('',#95934,58.5,0.436332312998583);
#6951=CONICAL_SURFACE('',#95936,58.5,0.436332312998583);
#6952=CONICAL_SURFACE('',#95938,58.5,0.436332312998583);
#6953=CONICAL_SURFACE('',#95940,58.5,0.436332312998583);
#6954=CONICAL_SURFACE('',#95946,58.5,0.436332312998583);
#6955=CONICAL_SURFACE('',#95950,58.3875000000295,0.436332312998583);
#6956=CONICAL_SURFACE('',#95961,58.5,0.436332312998583);
#6957=CONICAL_SURFACE('',#95967,58.5,0.436332312998583);
#6958=CONICAL_SURFACE('',#95968,58.3875000000295,0.436332312998583);
#6959=CONICAL_SURFACE('',#95969,58.3875000000295,0.436332312998583);
#6960=CONICAL_SURFACE('',#95974,58.5,0.436332312998583);
#6961=CONICAL_SURFACE('',#95982,58.5,0.436332312998583);
#6962=CONICAL_SURFACE('',#95989,58.5,0.436332312998583);
#6963=CONICAL_SURFACE('',#96000,58.5,0.436332312998583);
#6964=CONICAL_SURFACE('',#96002,58.3875000000295,0.436332312998583);
#6965=CONICAL_SURFACE('',#96014,58.3875000000295,0.436332312998583);
#6966=CONICAL_SURFACE('',#96017,58.5,0.436332312998583);
#6967=CONICAL_SURFACE('',#96030,58.5,0.436332312998583);
#6968=CONICAL_SURFACE('',#96040,58.5,0.436332312998583);
#6969=CONICAL_SURFACE('',#96048,58.5,0.436332312998583);
#6970=CONICAL_SURFACE('',#96055,58.3875000000295,0.436332312998583);
#6971=CONICAL_SURFACE('',#96057,58.3875000000295,0.436332312998583);
#6972=CONICAL_SURFACE('',#96059,58.5,0.436332312998583);
#6973=CONICAL_SURFACE('',#96069,58.5,0.436332312998583);
#6974=CONICAL_SURFACE('',#96087,58.3875000000295,0.436332312998583);
#6975=CONICAL_SURFACE('',#96095,58.5,0.436332312998583);
#6976=CONICAL_SURFACE('',#96106,58.5,0.436332312998583);
#6977=CONICAL_SURFACE('',#96111,58.5,0.436332312998583);
#6978=CONICAL_SURFACE('',#96117,58.5,0.436332312998583);
#6979=CONICAL_SURFACE('',#96121,58.5,0.436332312998583);
#6980=CONICAL_SURFACE('',#96135,58.5,0.436332312998583);
#6981=CONICAL_SURFACE('',#96434,58.3875000000295,0.436332312998583);
#6982=CONICAL_SURFACE('',#96487,58.3875000000295,0.436332312998583);
#6983=CONICAL_SURFACE('',#96664,58.3875000000295,0.436332312998583);
#6984=CONICAL_SURFACE('',#96992,58.3875000000295,0.436332312998583);
#6985=CONICAL_SURFACE('',#97086,58.5,0.436332312998583);
#6986=CONICAL_SURFACE('',#97095,58.5,0.436332312998583);
#6987=CONICAL_SURFACE('',#97107,58.5,0.436332312998583);
#6988=CONICAL_SURFACE('',#97339,58.3875000000295,0.436332312998583);
#6989=CONICAL_SURFACE('',#97353,58.3875000000295,0.436332312998583);
#6990=CONICAL_SURFACE('',#97364,58.3875000000295,0.436332312998583);
#6991=CONICAL_SURFACE('',#97375,58.3875000000295,0.436332312998583);
#6992=CONICAL_SURFACE('',#97386,58.3875000000295,0.436332312998583);
#6993=CONICAL_SURFACE('',#97400,58.3875000000295,0.436332312998583);
#6994=CONICAL_SURFACE('',#97422,58.3875000000295,0.436332312998583);
#6995=CONICAL_SURFACE('',#97434,58.3875000000295,0.436332312998583);
#6996=CONICAL_SURFACE('',#97454,58.3875000000295,0.436332312998583);
#6997=CONICAL_SURFACE('',#97469,58.3875000000295,0.436332312998583);
#6998=CONICAL_SURFACE('',#97481,58.3875000000295,0.436332312998583);
#6999=CONICAL_SURFACE('',#97933,58.3875000000295,0.436332312998583);
#7000=CONICAL_SURFACE('',#97948,2.,1.0471975511966);
#7001=CONICAL_SURFACE('',#97949,1.73205080756888,0.78539816339745);
#7002=CONICAL_SURFACE('',#97951,1.73205080756888,0.78539816339745);
#7003=CONICAL_SURFACE('',#97953,1.73205080756888,0.78539816339745);
#7004=CONICAL_SURFACE('',#97955,1.73205080756888,0.78539816339745);
#7005=CONICAL_SURFACE('',#97957,1.73205080756888,0.78539816339745);
#7006=CONICAL_SURFACE('',#97959,1.73205080756888,0.78539816339745);
#7007=CONICAL_SURFACE('',#97970,1.47499999999998,0.785398163397455);
#7008=CONICAL_SURFACE('',#99631,9.01478559345382,0.0174532925199415);
#7009=CONICAL_SURFACE('',#99633,74.6642856134258,0.0174532925199415);
#7010=CONICAL_SURFACE('',#99635,9.01478559345372,0.0174532925199415);
#7011=CONICAL_SURFACE('',#99638,9.01478559345379,0.0174532925199415);
#7012=CONICAL_SURFACE('',#99641,74.6642856134258,0.0174532925199415);
#7013=CONICAL_SURFACE('',#99643,9.01478559345383,0.0174532925199415);
#7014=CONICAL_SURFACE('',#99646,1067.50038076211,0.0174532925199415);
#7015=CONICAL_SURFACE('',#99649,11.963380762109,0.0174532925199415);
#7016=CONICAL_SURFACE('',#99652,77.6128807820809,0.0174532925199415);
#7017=CONICAL_SURFACE('',#99655,11.963380762109,0.0174532925199415);
#7018=CONICAL_SURFACE('',#99658,11.963380762109,0.0174532925199415);
#7019=CONICAL_SURFACE('',#99661,77.6128807820809,0.0174532925199415);
#7020=CONICAL_SURFACE('',#99664,11.963380762109,0.0174532925199415);
#7021=CONICAL_SURFACE('',#99667,1064.55178559345,0.0174532925199415);
#7022=CONICAL_SURFACE('',#99703,5.84961923789098,0.0174532925199415);
#7023=CONICAL_SURFACE('',#99705,5.84961923789177,0.0174532925199415);
#7024=CONICAL_SURFACE('',#99722,3.35,0.0174532925199415);
#7025=CONICAL_SURFACE('',#99727,3.35000000000079,0.0174532925199415);
#7026=CONICAL_SURFACE('',#99771,11.5144048313448,0.0174532925199415);
#7027=CONICAL_SURFACE('',#99772,77.1639048513167,0.0174532925199415);
#7028=CONICAL_SURFACE('',#99773,11.5144048313447,0.0174532925199415);
#7029=CONICAL_SURFACE('',#99774,11.5144048313448,0.0174532925199415);
#7030=CONICAL_SURFACE('',#99775,77.1639048513167,0.0174532925199415);
#7031=CONICAL_SURFACE('',#99776,11.5144048313448,0.0174532925199415);
#7032=CONICAL_SURFACE('',#99777,1070.,0.0174532925199415);
#7033=CONICAL_SURFACE('',#99779,14.463,0.0174532925199415);
#7034=CONICAL_SURFACE('',#99781,80.1125000199719,0.0174532925199415);
#7035=CONICAL_SURFACE('',#99783,14.463,0.0174532925199415);
#7036=CONICAL_SURFACE('',#99785,14.463,0.0174532925199415);
#7037=CONICAL_SURFACE('',#99787,80.1125000199719,0.0174532925199415);
#7038=CONICAL_SURFACE('',#99789,14.463,0.0174532925199415);
#7039=CONICAL_SURFACE('',#99791,1067.05140483134,0.0174532925199415);
#7040=CONICAL_SURFACE('',#101623,9.01478559345382,0.0174532925199415);
#7041=CONICAL_SURFACE('',#101625,74.6642856134258,0.0174532925199415);
#7042=CONICAL_SURFACE('',#101627,9.01478559345372,0.0174532925199415);
#7043=CONICAL_SURFACE('',#101630,9.01478559345379,0.0174532925199415);
#7044=CONICAL_SURFACE('',#101633,74.6642856134258,0.0174532925199415);
#7045=CONICAL_SURFACE('',#101635,9.01478559345383,0.0174532925199415);
#7046=CONICAL_SURFACE('',#101638,1064.55178559345,0.0174532925199415);
#7047=CONICAL_SURFACE('',#101652,1067.50038076211,0.0174532925199415);
#7048=CONICAL_SURFACE('',#101654,11.963380762109,0.0174532925199415);
#7049=CONICAL_SURFACE('',#101656,77.6128807820809,0.0174532925199415);
#7050=CONICAL_SURFACE('',#101658,11.963380762109,0.0174532925199415);
#7051=CONICAL_SURFACE('',#101660,232.500380762109,0.0174532925199415);
#7052=CONICAL_SURFACE('',#101662,1067.50038076211,0.0174532925199415);
#7053=CONICAL_SURFACE('',#101664,11.963380762109,0.0174532925199415);
#7054=CONICAL_SURFACE('',#101666,77.6128807820809,0.0174532925199415);
#7055=CONICAL_SURFACE('',#101668,11.963380762109,0.0174532925199415);
#7056=CONICAL_SURFACE('',#101670,1064.55178559345,0.0174532925199415);
#7057=CONICAL_SURFACE('',#101672,229.551785593454,0.0174532925199415);
#7058=CONICAL_SURFACE('',#101706,5.84961923789098,0.0174532925199415);
#7059=CONICAL_SURFACE('',#101708,5.84961923789177,0.0174532925199415);
#7060=CONICAL_SURFACE('',#101718,3.35,0.0174532925199415);
#7061=CONICAL_SURFACE('',#101721,3.35000000000079,0.0174532925199415);
#7062=CONICAL_SURFACE('',#101774,11.5144048313448,0.0174532925199415);
#7063=CONICAL_SURFACE('',#101775,77.1639048513167,0.0174532925199415);
#7064=CONICAL_SURFACE('',#101776,11.5144048313447,0.0174532925199415);
#7065=CONICAL_SURFACE('',#101777,11.5144048313448,0.0174532925199415);
#7066=CONICAL_SURFACE('',#101778,77.1639048513167,0.0174532925199415);
#7067=CONICAL_SURFACE('',#101779,11.5144048313448,0.0174532925199415);
#7068=CONICAL_SURFACE('',#101780,1067.05140483134,0.0174532925199415);
#7069=CONICAL_SURFACE('',#101792,1070.,0.0174532925199415);
#7070=CONICAL_SURFACE('',#101793,14.463,0.0174532925199415);
#7071=CONICAL_SURFACE('',#101794,80.1125000199719,0.0174532925199415);
#7072=CONICAL_SURFACE('',#101795,14.463,0.0174532925199415);
#7073=CONICAL_SURFACE('',#101796,235.,0.0174532925199415);
#7074=CONICAL_SURFACE('',#101797,1070.,0.0174532925199415);
#7075=CONICAL_SURFACE('',#101798,14.463,0.0174532925199415);
#7076=CONICAL_SURFACE('',#101799,80.1125000199719,0.0174532925199415);
#7077=CONICAL_SURFACE('',#101800,14.463,0.0174532925199415);
#7078=CONICAL_SURFACE('',#101801,1067.05140483134,0.0174532925199415);
#7079=CONICAL_SURFACE('',#101802,232.051404831345,0.0174532925199415);
#7080=CONICAL_SURFACE('',#101885,2.,1.0471975511966);
#7081=CONICAL_SURFACE('',#101886,1.73205080756888,0.78539816339745);
#7082=CONICAL_SURFACE('',#101888,1.73205080756888,0.78539816339745);
#7083=CONICAL_SURFACE('',#101890,1.73205080756888,0.78539816339745);
#7084=CONICAL_SURFACE('',#101892,1.73205080756888,0.78539816339745);
#7085=CONICAL_SURFACE('',#101894,1.73205080756888,0.78539816339745);
#7086=CONICAL_SURFACE('',#101896,1.73205080756888,0.78539816339745);
#7087=CONICAL_SURFACE('',#101914,5.,0.78539816339745);
#7088=CONICAL_SURFACE('',#101915,5.,0.78539816339745);
#7089=CONICAL_SURFACE('',#101916,5.,0.78539816339745);
#7090=CONICAL_SURFACE('',#101917,5.,0.78539816339745);
#7091=CONICAL_SURFACE('',#101918,5.,0.78539816339745);
#7092=CONICAL_SURFACE('',#101919,5.,0.78539816339745);
#7093=CONICAL_SURFACE('',#101927,5.,1.0471975511966);
#7094=CONICAL_SURFACE('',#101928,5.,1.0471975511966);
#7095=CONICAL_SURFACE('',#101929,5.,1.0471975511966);
#7096=CONICAL_SURFACE('',#101930,5.,1.0471975511966);
#7097=CONICAL_SURFACE('',#101931,5.,1.0471975511966);
#7098=CONICAL_SURFACE('',#101932,5.,1.0471975511966);
#7099=CONICAL_SURFACE('',#101946,5.,0.78539816339745);
#7100=CONICAL_SURFACE('',#101947,5.,0.78539816339745);
#7101=CONICAL_SURFACE('',#101948,5.,0.78539816339745);
#7102=CONICAL_SURFACE('',#101949,5.,0.78539816339745);
#7103=CONICAL_SURFACE('',#101950,5.,0.78539816339745);
#7104=CONICAL_SURFACE('',#101951,5.,0.78539816339745);
#7105=CONICAL_SURFACE('',#101959,5.,1.0471975511966);
#7106=CONICAL_SURFACE('',#101960,5.,1.0471975511966);
#7107=CONICAL_SURFACE('',#101961,5.,1.0471975511966);
#7108=CONICAL_SURFACE('',#101962,5.,1.0471975511966);
#7109=CONICAL_SURFACE('',#101963,5.,1.0471975511966);
#7110=CONICAL_SURFACE('',#101964,5.,1.0471975511966);
#7111=CONICAL_SURFACE('',#101977,2.,1.0471975511966);
#7112=CONICAL_SURFACE('',#101978,1.73205080756888,0.78539816339745);
#7113=CONICAL_SURFACE('',#101980,1.73205080756888,0.78539816339745);
#7114=CONICAL_SURFACE('',#101982,1.73205080756888,0.78539816339745);
#7115=CONICAL_SURFACE('',#101984,1.73205080756888,0.78539816339745);
#7116=CONICAL_SURFACE('',#101986,1.73205080756888,0.78539816339745);
#7117=CONICAL_SURFACE('',#101988,1.73205080756888,0.78539816339745);
#7118=CONICAL_SURFACE('',#102016,0.750000000000001,0.0436332312998574);
#7119=CONICAL_SURFACE('',#102018,0.750000000000001,0.0436332312998574);
#7120=CONICAL_SURFACE('',#102025,1.47499999999998,0.785398163397455);
#7121=CONICAL_SURFACE('',#102154,0.750000000000001,0.0436332312998574);
#7122=CONICAL_SURFACE('',#102156,0.750000000000001,0.0436332312998574);
#7123=CONICAL_SURFACE('',#102652,5.,0.78539816339745);
#7124=CONICAL_SURFACE('',#102653,5.,0.78539816339745);
#7125=CONICAL_SURFACE('',#102654,5.,0.78539816339745);
#7126=CONICAL_SURFACE('',#102655,5.,0.78539816339745);
#7127=CONICAL_SURFACE('',#102656,5.,0.78539816339745);
#7128=CONICAL_SURFACE('',#102657,5.,0.78539816339745);
#7129=CONICAL_SURFACE('',#102665,5.,1.0471975511966);
#7130=CONICAL_SURFACE('',#102666,5.,1.0471975511966);
#7131=CONICAL_SURFACE('',#102667,5.,1.0471975511966);
#7132=CONICAL_SURFACE('',#102668,5.,1.0471975511966);
#7133=CONICAL_SURFACE('',#102669,5.,1.0471975511966);
#7134=CONICAL_SURFACE('',#102670,5.,1.0471975511966);
#7135=CONICAL_SURFACE('',#102684,5.,0.78539816339745);
#7136=CONICAL_SURFACE('',#102685,5.,0.78539816339745);
#7137=CONICAL_SURFACE('',#102686,5.,0.78539816339745);
#7138=CONICAL_SURFACE('',#102687,5.,0.78539816339745);
#7139=CONICAL_SURFACE('',#102688,5.,0.78539816339745);
#7140=CONICAL_SURFACE('',#102689,5.,0.78539816339745);
#7141=CONICAL_SURFACE('',#102697,5.,1.0471975511966);
#7142=CONICAL_SURFACE('',#102698,5.,1.0471975511966);
#7143=CONICAL_SURFACE('',#102699,5.,1.0471975511966);
#7144=CONICAL_SURFACE('',#102700,5.,1.0471975511966);
#7145=CONICAL_SURFACE('',#102701,5.,1.0471975511966);
#7146=CONICAL_SURFACE('',#102702,5.,1.0471975511966);
#7147=CONICAL_SURFACE('',#102715,2.,1.0471975511966);
#7148=CONICAL_SURFACE('',#102716,1.73205080756888,0.78539816339745);
#7149=CONICAL_SURFACE('',#102718,1.73205080756888,0.78539816339745);
#7150=CONICAL_SURFACE('',#102720,1.73205080756888,0.78539816339745);
#7151=CONICAL_SURFACE('',#102722,1.73205080756888,0.78539816339745);
#7152=CONICAL_SURFACE('',#102724,1.73205080756888,0.78539816339745);
#7153=CONICAL_SURFACE('',#102726,1.73205080756888,0.78539816339745);
#7154=CONICAL_SURFACE('',#103107,3.,1.0471975511966);
#7155=CONICAL_SURFACE('',#103108,2.88675134594813,0.78539816339745);
#7156=CONICAL_SURFACE('',#103110,2.88675134594813,0.78539816339745);
#7157=CONICAL_SURFACE('',#103112,2.88675134594813,0.78539816339745);
#7158=CONICAL_SURFACE('',#103114,2.88675134594813,0.78539816339745);
#7159=CONICAL_SURFACE('',#103116,2.88675134594813,0.78539816339745);
#7160=CONICAL_SURFACE('',#103118,2.88675134594813,0.78539816339745);
#7161=CONICAL_SURFACE('',#103120,6.,0.785398163397452);
#7162=CONICAL_SURFACE('',#103308,58.3875000000282,1.3264502315157);
#7224=SHAPE_REPRESENTATION_RELATIONSHIP('SRR','None',#310896,#7241);
#7241=ADVANCED_BREP_SHAPE_REPRESENTATION('',(#7326,#7327,#7328,#7329,#7330,
#7331,#7332,#7333,#7334,#7335,#7336,#7337,#7338,#7339,#7340,#7341,#7342,
#7343,#7344,#7345),#310605);
#7258=STYLED_ITEM('',(#311005),#7326);
#7259=STYLED_ITEM('',(#311005),#7327);
#7260=STYLED_ITEM('',(#311005),#7328);
#7261=STYLED_ITEM('',(#311005),#7329);
#7262=STYLED_ITEM('',(#311005),#7330);
#7263=STYLED_ITEM('',(#311005),#7331);
#7264=STYLED_ITEM('',(#311005),#7332);
#7265=STYLED_ITEM('',(#311005),#7333);
#7266=STYLED_ITEM('',(#311005),#7334);
#7267=STYLED_ITEM('',(#311005),#7335);
#7268=STYLED_ITEM('',(#311005),#7336);
#7269=STYLED_ITEM('',(#311005),#7337);
#7270=STYLED_ITEM('',(#311005),#7338);
#7271=STYLED_ITEM('',(#311005),#7339);
#7272=STYLED_ITEM('',(#311005),#7340);
#7273=STYLED_ITEM('',(#311005),#7341);
#7274=STYLED_ITEM('',(#311005),#7342);
#7275=STYLED_ITEM('',(#311005),#7343);
#7276=STYLED_ITEM('',(#311005),#7344);
#7277=STYLED_ITEM('',(#311005),#7345);
#7326=MANIFOLD_SOLID_BREP('Body1',#93708);
#7327=MANIFOLD_SOLID_BREP('Body2',#93709);
#7328=MANIFOLD_SOLID_BREP('Body3',#93710);
#7329=MANIFOLD_SOLID_BREP('Body4',#93711);
#7330=MANIFOLD_SOLID_BREP('Body5',#93712);
#7331=MANIFOLD_SOLID_BREP('Body6',#93713);
#7332=MANIFOLD_SOLID_BREP('Body7',#93714);
#7333=MANIFOLD_SOLID_BREP('Body8',#93715);
#7334=MANIFOLD_SOLID_BREP('Body9',#93716);
#7335=MANIFOLD_SOLID_BREP('Body10',#93717);
#7336=MANIFOLD_SOLID_BREP('Body11',#93718);
#7337=MANIFOLD_SOLID_BREP('Body12',#93719);
#7338=MANIFOLD_SOLID_BREP('Body13',#93720);
#7339=MANIFOLD_SOLID_BREP('Body14',#93721);
#7340=MANIFOLD_SOLID_BREP('Body15',#93722);
#7341=MANIFOLD_SOLID_BREP('Body16',#93723);
#7342=MANIFOLD_SOLID_BREP('Body17',#93724);
#7343=MANIFOLD_SOLID_BREP('Body18',#93725);
#7344=MANIFOLD_SOLID_BREP('Body19',#93726);
#7345=MANIFOLD_SOLID_BREP('Body20',#93727);
#7439=FACE_BOUND('',#14531,.T.);
#7440=FACE_BOUND('',#14538,.T.);
#7441=FACE_BOUND('',#14957,.T.);
#7442=FACE_BOUND('',#14967,.T.);
#7443=FACE_BOUND('',#16361,.T.);
#7444=FACE_BOUND('',#16371,.T.);
#7445=FACE_BOUND('',#16795,.T.);
#7446=FACE_BOUND('',#16796,.T.);
#7447=FACE_BOUND('',#16797,.T.);
#7448=FACE_BOUND('',#16798,.T.);
#7449=FACE_BOUND('',#16811,.T.);
#7450=FACE_BOUND('',#16812,.T.);
#7451=FACE_BOUND('',#16813,.T.);
#7452=FACE_BOUND('',#16814,.T.);
#7453=FACE_BOUND('',#16831,.T.);
#7454=FACE_BOUND('',#16837,.T.);
#7455=FACE_BOUND('',#17565,.T.);
#7456=FACE_BOUND('',#18280,.T.);
#7457=FACE_BOUND('',#18352,.T.);
#7458=FACE_BOUND('',#18353,.T.);
#7459=FACE_BOUND('',#18354,.T.);
#7460=FACE_BOUND('',#18355,.T.);
#7461=FACE_BOUND('',#18356,.T.);
#7462=FACE_BOUND('',#18357,.T.);
#7463=FACE_BOUND('',#18358,.T.);
#7464=FACE_BOUND('',#18359,.T.);
#7465=FACE_BOUND('',#18360,.T.);
#7466=FACE_BOUND('',#18361,.T.);
#7467=FACE_BOUND('',#18362,.T.);
#7468=FACE_BOUND('',#18363,.T.);
#7469=FACE_BOUND('',#18364,.T.);
#7470=FACE_BOUND('',#18365,.T.);
#7471=FACE_BOUND('',#18366,.T.);
#7472=FACE_BOUND('',#18367,.T.);
#7473=FACE_BOUND('',#18368,.T.);
#7474=FACE_BOUND('',#18369,.T.);
#7475=FACE_BOUND('',#18370,.T.);
#7476=FACE_BOUND('',#18371,.T.);
#7477=FACE_BOUND('',#18372,.T.);
#7478=FACE_BOUND('',#18373,.T.);
#7479=FACE_BOUND('',#18374,.T.);
#7480=FACE_BOUND('',#18375,.T.);
#7481=FACE_BOUND('',#18376,.T.);
#7482=FACE_BOUND('',#18377,.T.);
#7483=FACE_BOUND('',#18378,.T.);
#7484=FACE_BOUND('',#18379,.T.);
#7485=FACE_BOUND('',#18380,.T.);
#7486=FACE_BOUND('',#18381,.T.);
#7487=FACE_BOUND('',#18382,.T.);
#7488=FACE_BOUND('',#18383,.T.);
#7489=FACE_BOUND('',#18384,.T.);
#7490=FACE_BOUND('',#18385,.T.);
#7491=FACE_BOUND('',#18386,.T.);
#7492=FACE_BOUND('',#18387,.T.);
#7493=FACE_BOUND('',#18388,.T.);
#7494=FACE_BOUND('',#18389,.T.);
#7495=FACE_BOUND('',#18390,.T.);
#7496=FACE_BOUND('',#18391,.T.);
#7497=FACE_BOUND('',#18392,.T.);
#7498=FACE_BOUND('',#18393,.T.);
#7499=FACE_BOUND('',#18394,.T.);
#7500=FACE_BOUND('',#18395,.T.);
#7501=FACE_BOUND('',#18396,.T.);
#7502=FACE_BOUND('',#18397,.T.);
#7503=FACE_BOUND('',#18398,.T.);
#7504=FACE_BOUND('',#18399,.T.);
#7505=FACE_BOUND('',#18400,.T.);
#7506=FACE_BOUND('',#18401,.T.);
#7507=FACE_BOUND('',#18402,.T.);
#7508=FACE_BOUND('',#18403,.T.);
#7509=FACE_BOUND('',#18404,.T.);
#7510=FACE_BOUND('',#18405,.T.);
#7511=FACE_BOUND('',#18406,.T.);
#7512=FACE_BOUND('',#18407,.T.);
#7513=FACE_BOUND('',#18408,.T.);
#7514=FACE_BOUND('',#18409,.T.);
#7515=FACE_BOUND('',#18410,.T.);
#7516=FACE_BOUND('',#18411,.T.);
#7517=FACE_BOUND('',#18412,.T.);
#7518=FACE_BOUND('',#18413,.T.);
#7519=FACE_BOUND('',#18414,.T.);
#7520=FACE_BOUND('',#18415,.T.);
#7521=FACE_BOUND('',#18416,.T.);
#7522=FACE_BOUND('',#18417,.T.);
#7523=FACE_BOUND('',#18418,.T.);
#7524=FACE_BOUND('',#18419,.T.);
#7525=FACE_BOUND('',#18461,.T.);
#7526=FACE_BOUND('',#18513,.T.);
#7527=FACE_BOUND('',#18531,.T.);
#7528=FACE_BOUND('',#18532,.T.);
#7529=FACE_BOUND('',#18533,.T.);
#7530=FACE_BOUND('',#18534,.T.);
#7531=FACE_BOUND('',#18535,.T.);
#7532=FACE_BOUND('',#18536,.T.);
#7533=FACE_BOUND('',#18537,.T.);
#7534=FACE_BOUND('',#18538,.T.);
#7535=FACE_BOUND('',#18539,.T.);
#7536=FACE_BOUND('',#18540,.T.);
#7537=FACE_BOUND('',#18541,.T.);
#7538=FACE_BOUND('',#18542,.T.);
#7539=FACE_BOUND('',#18543,.T.);
#7540=FACE_BOUND('',#18544,.T.);
#7541=FACE_BOUND('',#18545,.T.);
#7542=FACE_BOUND('',#18546,.T.);
#7543=FACE_BOUND('',#18547,.T.);
#7544=FACE_BOUND('',#18548,.T.);
#7545=FACE_BOUND('',#18549,.T.);
#7546=FACE_BOUND('',#18550,.T.);
#7547=FACE_BOUND('',#18551,.T.);
#7548=FACE_BOUND('',#18552,.T.);
#7549=FACE_BOUND('',#18553,.T.);
#7550=FACE_BOUND('',#18554,.T.);
#7551=FACE_BOUND('',#18555,.T.);
#7552=FACE_BOUND('',#18556,.T.);
#7553=FACE_BOUND('',#18557,.T.);
#7554=FACE_BOUND('',#18558,.T.);
#7555=FACE_BOUND('',#18559,.T.);
#7556=FACE_BOUND('',#18560,.T.);
#7557=FACE_BOUND('',#18561,.T.);
#7558=FACE_BOUND('',#18562,.T.);
#7559=FACE_BOUND('',#18563,.T.);
#7560=FACE_BOUND('',#18564,.T.);
#7561=FACE_BOUND('',#18565,.T.);
#7562=FACE_BOUND('',#18566,.T.);
#7563=FACE_BOUND('',#18567,.T.);
#7564=FACE_BOUND('',#18568,.T.);
#7565=FACE_BOUND('',#18569,.T.);
#7566=FACE_BOUND('',#18570,.T.);
#7567=FACE_BOUND('',#18571,.T.);
#7568=FACE_BOUND('',#18572,.T.);
#7569=FACE_BOUND('',#18573,.T.);
#7570=FACE_BOUND('',#18574,.T.);
#7571=FACE_BOUND('',#18575,.T.);
#7572=FACE_BOUND('',#18576,.T.);
#7573=FACE_BOUND('',#18577,.T.);
#7574=FACE_BOUND('',#18578,.T.);
#7575=FACE_BOUND('',#18579,.T.);
#7576=FACE_BOUND('',#18580,.T.);
#7577=FACE_BOUND('',#18581,.T.);
#7578=FACE_BOUND('',#18582,.T.);
#7579=FACE_BOUND('',#18583,.T.);
#7580=FACE_BOUND('',#18584,.T.);
#7581=FACE_BOUND('',#18585,.T.);
#7582=FACE_BOUND('',#18586,.T.);
#7583=FACE_BOUND('',#18587,.T.);
#7584=FACE_BOUND('',#18588,.T.);
#7585=FACE_BOUND('',#18589,.T.);
#7586=FACE_BOUND('',#18590,.T.);
#7587=FACE_BOUND('',#18591,.T.);
#7588=FACE_BOUND('',#18602,.T.);
#7589=FACE_BOUND('',#18624,.T.);
#7590=FACE_BOUND('',#18626,.T.);
#7591=FACE_BOUND('',#18642,.T.);
#7592=FACE_BOUND('',#18668,.T.);
#7593=FACE_BOUND('',#18736,.T.);
#7594=FACE_BOUND('',#18794,.T.);
#7595=FACE_BOUND('',#18797,.T.);
#7596=FACE_BOUND('',#18809,.T.);
#7597=FACE_BOUND('',#18814,.T.);
#7598=FACE_BOUND('',#18829,.T.);
#7599=FACE_BOUND('',#18830,.T.);
#7600=FACE_BOUND('',#18848,.T.);
#7601=FACE_BOUND('',#18849,.T.);
#7602=FACE_BOUND('',#18860,.T.);
#7603=FACE_BOUND('',#18868,.T.);
#7604=FACE_BOUND('',#18880,.T.);
#7605=FACE_BOUND('',#19146,.T.);
#7606=FACE_BOUND('',#19370,.T.);
#7607=FACE_BOUND('',#19371,.T.);
#7608=FACE_BOUND('',#19372,.T.);
#7609=FACE_BOUND('',#19374,.T.);
#7610=FACE_BOUND('',#19379,.T.);
#7611=FACE_BOUND('',#19384,.T.);
#7612=FACE_BOUND('',#19389,.T.);
#7613=FACE_BOUND('',#19411,.T.);
#7614=FACE_BOUND('',#19557,.T.);
#7615=FACE_BOUND('',#19558,.T.);
#7616=FACE_BOUND('',#19559,.T.);
#7617=FACE_BOUND('',#19560,.T.);
#7618=FACE_BOUND('',#19569,.T.);
#7619=FACE_BOUND('',#19570,.T.);
#7620=FACE_BOUND('',#19571,.T.);
#7621=FACE_BOUND('',#19572,.T.);
#7726=PLANE('',#94086);
#7727=PLANE('',#94089);
#7728=PLANE('',#94093);
#7729=PLANE('',#94097);
#7730=PLANE('',#94100);
#7731=PLANE('',#94104);
#7732=PLANE('',#94119);
#7733=PLANE('',#94127);
#7734=PLANE('',#94132);
#7735=PLANE('',#94263);
#7736=PLANE('',#94272);
#7737=PLANE('',#94277);
#7738=PLANE('',#94458);
#7739=PLANE('',#94463);
#7740=PLANE('',#94466);
#7741=PLANE('',#94563);
#7742=PLANE('',#94691);
#7743=PLANE('',#94698);
#7744=PLANE('',#94704);
#7745=PLANE('',#94709);
#7746=PLANE('',#94715);
#7747=PLANE('',#94720);
#7748=PLANE('',#94727);
#7749=PLANE('',#94738);
#7750=PLANE('',#94744);
#7751=PLANE('',#94747);
#7752=PLANE('',#94755);
#7753=PLANE('',#94762);
#7754=PLANE('',#94766);
#7755=PLANE('',#94769);
#7756=PLANE('',#94772);
#7757=PLANE('',#94777);
#7758=PLANE('',#94780);
#7759=PLANE('',#94789);
#7760=PLANE('',#94795);
#7761=PLANE('',#94800);
#7762=PLANE('',#94807);
#7763=PLANE('',#94813);
#7764=PLANE('',#94818);
#7765=PLANE('',#94827);
#7766=PLANE('',#94834);
#7767=PLANE('',#94840);
#7768=PLANE('',#94845);
#7769=PLANE('',#94851);
#7770=PLANE('',#94856);
#7771=PLANE('',#94863);
#7772=PLANE('',#94867);
#7773=PLANE('',#94871);
#7774=PLANE('',#94876);
#7775=PLANE('',#94879);
#7776=PLANE('',#94884);
#7777=PLANE('',#94892);
#7778=PLANE('',#94894);
#7779=PLANE('',#94899);
#7780=PLANE('',#94902);
#7781=PLANE('',#94905);
#7782=PLANE('',#94909);
#7783=PLANE('',#94914);
#7784=PLANE('',#94917);
#7785=PLANE('',#94922);
#7786=PLANE('',#94926);
#7787=PLANE('',#94929);
#7788=PLANE('',#94932);
#7789=PLANE('',#94936);
#7790=PLANE('',#94941);
#7791=PLANE('',#94945);
#7792=PLANE('',#94949);
#7793=PLANE('',#94960);
#7794=PLANE('',#94962);
#7795=PLANE('',#94967);
#7796=PLANE('',#94970);
#7797=PLANE('',#94978);
#7798=PLANE('',#94983);
#7799=PLANE('',#94988);
#7800=PLANE('',#94991);
#7801=PLANE('',#94995);
#7802=PLANE('',#94998);
#7803=PLANE('',#95003);
#7804=PLANE('',#95007);
#7805=PLANE('',#95010);
#7806=PLANE('',#95016);
#7807=PLANE('',#95035);
#7808=PLANE('',#95048);
#7809=PLANE('',#95058);
#7810=PLANE('',#95063);
#7811=PLANE('',#95069);
#7812=PLANE('',#95073);
#7813=PLANE('',#95077);
#7814=PLANE('',#95081);
#7815=PLANE('',#95085);
#7816=PLANE('',#95098);
#7817=PLANE('',#95105);
#7818=PLANE('',#95124);
#7819=PLANE('',#95131);
#7820=PLANE('',#95134);
#7821=PLANE('',#95140);
#7822=PLANE('',#95144);
#7823=PLANE('',#95148);
#7824=PLANE('',#95156);
#7825=PLANE('',#95173);
#7826=PLANE('',#95187);
#7827=PLANE('',#95325);
#7828=PLANE('',#95352);
#7829=PLANE('',#95380);
#7830=PLANE('',#95822);
#7831=PLANE('',#95825);
#7832=PLANE('',#95920);
#7833=PLANE('',#95921);
#7834=PLANE('',#95922);
#7835=PLANE('',#95923);
#7836=PLANE('',#95924);
#7837=PLANE('',#95925);
#7838=PLANE('',#95926);
#7839=PLANE('',#95928);
#7840=PLANE('',#95930);
#7841=PLANE('',#95932);
#7842=PLANE('',#95935);
#7843=PLANE('',#95937);
#7844=PLANE('',#95939);
#7845=PLANE('',#95941);
#7846=PLANE('',#95944);
#7847=PLANE('',#95945);
#7848=PLANE('',#95947);
#7849=PLANE('',#95948);
#7850=PLANE('',#95951);
#7851=PLANE('',#95953);
#7852=PLANE('',#95954);
#7853=PLANE('',#95960);
#7854=PLANE('',#95962);
#7855=PLANE('',#95963);
#7856=PLANE('',#95964);
#7857=PLANE('',#95966);
#7858=PLANE('',#95970);
#7859=PLANE('',#95972);
#7860=PLANE('',#95973);
#7861=PLANE('',#95978);
#7862=PLANE('',#95983);
#7863=PLANE('',#95984);
#7864=PLANE('',#95985);
#7865=PLANE('',#95987);
#7866=PLANE('',#95988);
#7867=PLANE('',#95993);
#7868=PLANE('',#95995);
#7869=PLANE('',#95996);
#7870=PLANE('',#96001);
#7871=PLANE('',#96003);
#7872=PLANE('',#96005);
#7873=PLANE('',#96006);
#7874=PLANE('',#96007);
#7875=PLANE('',#96009);
#7876=PLANE('',#96013);
#7877=PLANE('',#96016);
#7878=PLANE('',#96021);
#7879=PLANE('',#96022);
#7880=PLANE('',#96026);
#7881=PLANE('',#96031);
#7882=PLANE('',#96032);
#7883=PLANE('',#96036);
#7884=PLANE('',#96037);
#7885=PLANE('',#96039);
#7886=PLANE('',#96044);
#7887=PLANE('',#96049);
#7888=PLANE('',#96050);
#7889=PLANE('',#96054);
#7890=PLANE('',#96061);
#7891=PLANE('',#96065);
#7892=PLANE('',#96066);
#7893=PLANE('',#96068);
#7894=PLANE('',#96075);
#7895=PLANE('',#96081);
#7896=PLANE('',#96082);
#7897=PLANE('',#96086);
#7898=PLANE('',#96092);
#7899=PLANE('',#96094);
#7900=PLANE('',#96097);
#7901=PLANE('',#96099);
#7902=PLANE('',#96105);
#7903=PLANE('',#96109);
#7904=PLANE('',#96115);
#7905=PLANE('',#96120);
#7906=PLANE('',#96125);
#7907=PLANE('',#96129);
#7908=PLANE('',#96134);
#7909=PLANE('',#96137);
#7910=PLANE('',#96139);
#7911=PLANE('',#96140);
#7912=PLANE('',#96141);
#7913=PLANE('',#96142);
#7914=PLANE('',#96143);
#7915=PLANE('',#96144);
#7916=PLANE('',#96304);
#7917=PLANE('',#96307);
#7918=PLANE('',#96808);
#7919=PLANE('',#96838);
#7920=PLANE('',#96869);
#7921=PLANE('',#97056);
#7922=PLANE('',#97077);
#7923=PLANE('',#97101);
#7924=PLANE('',#97113);
#7925=PLANE('',#97115);
#7926=PLANE('',#97117);
#7927=PLANE('',#97119);
#7928=PLANE('',#97122);
#7929=PLANE('',#97129);
#7930=PLANE('',#97136);
#7931=PLANE('',#97143);
#7932=PLANE('',#97158);
#7933=PLANE('',#97164);
#7934=PLANE('',#97170);
#7935=PLANE('',#97176);
#7936=PLANE('',#97182);
#7937=PLANE('',#97191);
#7938=PLANE('',#97203);
#7939=PLANE('',#97217);
#7940=PLANE('',#97231);
#7941=PLANE('',#97251);
#7942=PLANE('',#97257);
#7943=PLANE('',#97259);
#7944=PLANE('',#97263);
#7945=PLANE('',#97265);
#7946=PLANE('',#97267);
#7947=PLANE('',#97269);
#7948=PLANE('',#97271);
#7949=PLANE('',#97273);
#7950=PLANE('',#97275);
#7951=PLANE('',#97278);
#7952=PLANE('',#97280);
#7953=PLANE('',#97282);
#7954=PLANE('',#97284);
#7955=PLANE('',#97290);
#7956=PLANE('',#97291);
#7957=PLANE('',#97294);
#7958=PLANE('',#97296);
#7959=PLANE('',#97299);
#7960=PLANE('',#97300);
#7961=PLANE('',#97302);
#7962=PLANE('',#97304);
#7963=PLANE('',#97307);
#7964=PLANE('',#97309);
#7965=PLANE('',#97311);
#7966=PLANE('',#97314);
#7967=PLANE('',#97315);
#7968=PLANE('',#97317);
#7969=PLANE('',#97319);
#7970=PLANE('',#97321);
#7971=PLANE('',#97324);
#7972=PLANE('',#97327);
#7973=PLANE('',#97329);
#7974=PLANE('',#97331);
#7975=PLANE('',#97334);
#7976=PLANE('',#97335);
#7977=PLANE('',#97341);
#7978=PLANE('',#97346);
#7979=PLANE('',#97349);
#7980=PLANE('',#97355);
#7981=PLANE('',#97360);
#7982=PLANE('',#97366);
#7983=PLANE('',#97371);
#7984=PLANE('',#97377);
#7985=PLANE('',#97382);
#7986=PLANE('',#97388);
#7987=PLANE('',#97393);
#7988=PLANE('',#97396);
#7989=PLANE('',#97404);
#7990=PLANE('',#97406);
#7991=PLANE('',#97412);
#7992=PLANE('',#97415);
#7993=PLANE('',#97418);
#7994=PLANE('',#97425);
#7995=PLANE('',#97430);
#7996=PLANE('',#97439);
#7997=PLANE('',#97441);
#7998=PLANE('',#97444);
#7999=PLANE('',#97450);
#8000=PLANE('',#97456);
#8001=PLANE('',#97461);
#8002=PLANE('',#97464);
#8003=PLANE('',#97471);
#8004=PLANE('',#97476);
#8005=PLANE('',#97483);
#8006=PLANE('',#97578);
#8007=PLANE('',#97647);
#8008=PLANE('',#97650);
#8009=PLANE('',#97653);
#8010=PLANE('',#97805);
#8011=PLANE('',#97808);
#8012=PLANE('',#97813);
#8013=PLANE('',#97893);
#8014=PLANE('',#97896);
#8015=PLANE('',#97901);
#8016=PLANE('',#97911);
#8017=PLANE('',#97919);
#8018=PLANE('',#97927);
#8019=PLANE('',#97928);
#8020=PLANE('',#97929);
#8021=PLANE('',#97941);
#8022=PLANE('',#97942);
#8023=PLANE('',#97943);
#8024=PLANE('',#97944);
#8025=PLANE('',#97945);
#8026=PLANE('',#97946);
#8027=PLANE('',#97947);
#8028=PLANE('',#97966);
#8029=PLANE('',#97968);
#8030=PLANE('',#97973);
#8031=PLANE('',#97976);
#8032=PLANE('',#97980);
#8033=PLANE('',#99502);
#8034=PLANE('',#99503);
#8035=PLANE('',#99510);
#8036=PLANE('',#99511);
#8037=PLANE('',#99516);
#8038=PLANE('',#99517);
#8039=PLANE('',#99518);
#8040=PLANE('',#99519);
#8041=PLANE('',#99520);
#8042=PLANE('',#99521);
#8043=PLANE('',#99522);
#8044=PLANE('',#99523);
#8045=PLANE('',#99524);
#8046=PLANE('',#99525);
#8047=PLANE('',#99526);
#8048=PLANE('',#99527);
#8049=PLANE('',#99528);
#8050=PLANE('',#99529);
#8051=PLANE('',#99530);
#8052=PLANE('',#99531);
#8053=PLANE('',#99532);
#8054=PLANE('',#99533);
#8055=PLANE('',#99534);
#8056=PLANE('',#99535);
#8057=PLANE('',#99536);
#8058=PLANE('',#99537);
#8059=PLANE('',#99538);
#8060=PLANE('',#99539);
#8061=PLANE('',#99540);
#8062=PLANE('',#99541);
#8063=PLANE('',#99542);
#8064=PLANE('',#99543);
#8065=PLANE('',#99544);
#8066=PLANE('',#99545);
#8067=PLANE('',#99546);
#8068=PLANE('',#99547);
#8069=PLANE('',#99548);
#8070=PLANE('',#99549);
#8071=PLANE('',#99550);
#8072=PLANE('',#99551);
#8073=PLANE('',#99552);
#8074=PLANE('',#99553);
#8075=PLANE('',#99554);
#8076=PLANE('',#99555);
#8077=PLANE('',#99556);
#8078=PLANE('',#99557);
#8079=PLANE('',#99558);
#8080=PLANE('',#99559);
#8081=PLANE('',#99560);
#8082=PLANE('',#99561);
#8083=PLANE('',#99562);
#8084=PLANE('',#99563);
#8085=PLANE('',#99564);
#8086=PLANE('',#99565);
#8087=PLANE('',#99566);
#8088=PLANE('',#99567);
#8089=PLANE('',#99568);
#8090=PLANE('',#99569);
#8091=PLANE('',#99570);
#8092=PLANE('',#99571);
#8093=PLANE('',#99572);
#8094=PLANE('',#99594);
#8095=PLANE('',#99596);
#8096=PLANE('',#99597);
#8097=PLANE('',#99599);
#8098=PLANE('',#99600);
#8099=PLANE('',#99601);
#8100=PLANE('',#99605);
#8101=PLANE('',#99606);
#8102=PLANE('',#99670);
#8103=PLANE('',#99674);
#8104=PLANE('',#99676);
#8105=PLANE('',#99678);
#8106=PLANE('',#99680);
#8107=PLANE('',#99682);
#8108=PLANE('',#99684);
#8109=PLANE('',#99686);
#8110=PLANE('',#99688);
#8111=PLANE('',#99690);
#8112=PLANE('',#99702);
#8113=PLANE('',#99704);
#8114=PLANE('',#99720);
#8115=PLANE('',#99725);
#8116=PLANE('',#99728);
#8117=PLANE('',#99729);
#8118=PLANE('',#99730);
#8119=PLANE('',#99732);
#8120=PLANE('',#99734);
#8121=PLANE('',#99735);
#8122=PLANE('',#99737);
#8123=PLANE('',#99738);
#8124=PLANE('',#99740);
#8125=PLANE('',#99741);
#8126=PLANE('',#99792);
#8127=PLANE('',#99793);
#8128=PLANE('',#99804);
#8129=PLANE('',#99805);
#8130=PLANE('',#99806);
#8131=PLANE('',#99807);
#8132=PLANE('',#99808);
#8133=PLANE('',#99809);
#8134=PLANE('',#99810);
#8135=PLANE('',#99811);
#8136=PLANE('',#99812);
#8137=PLANE('',#99813);
#8138=PLANE('',#99821);
#8139=PLANE('',#99822);
#8140=PLANE('',#99823);
#8141=PLANE('',#99824);
#8142=PLANE('',#99825);
#8143=PLANE('',#99826);
#8144=PLANE('',#99827);
#8145=PLANE('',#99828);
#8146=PLANE('',#99829);
#8147=PLANE('',#99830);
#8148=PLANE('',#99831);
#8149=PLANE('',#99832);
#8150=PLANE('',#99833);
#8151=PLANE('',#99834);
#8152=PLANE('',#99851);
#8153=PLANE('',#99852);
#8154=PLANE('',#99853);
#8155=PLANE('',#99854);
#8156=PLANE('',#99855);
#8157=PLANE('',#99856);
#8158=PLANE('',#99857);
#8159=PLANE('',#99858);
#8160=PLANE('',#99859);
#8161=PLANE('',#99860);
#8162=PLANE('',#99861);
#8163=PLANE('',#99862);
#8164=PLANE('',#99863);
#8165=PLANE('',#99864);
#8166=PLANE('',#99865);
#8167=PLANE('',#99866);
#8168=PLANE('',#99867);
#8169=PLANE('',#99868);
#8170=PLANE('',#99869);
#8171=PLANE('',#99870);
#8172=PLANE('',#99871);
#8173=PLANE('',#99872);
#8174=PLANE('',#99873);
#8175=PLANE('',#99874);
#8176=PLANE('',#99875);
#8177=PLANE('',#99876);
#8178=PLANE('',#99877);
#8179=PLANE('',#99878);
#8180=PLANE('',#101430);
#8181=PLANE('',#101433);
#8182=PLANE('',#101458);
#8183=PLANE('',#101459);
#8184=PLANE('',#101466);
#8185=PLANE('',#101467);
#8186=PLANE('',#101472);
#8187=PLANE('',#101473);
#8188=PLANE('',#101474);
#8189=PLANE('',#101475);
#8190=PLANE('',#101476);
#8191=PLANE('',#101477);
#8192=PLANE('',#101478);
#8193=PLANE('',#101479);
#8194=PLANE('',#101480);
#8195=PLANE('',#101481);
#8196=PLANE('',#101482);
#8197=PLANE('',#101483);
#8198=PLANE('',#101484);
#8199=PLANE('',#101485);
#8200=PLANE('',#101486);
#8201=PLANE('',#101487);
#8202=PLANE('',#101488);
#8203=PLANE('',#101489);
#8204=PLANE('',#101490);
#8205=PLANE('',#101491);
#8206=PLANE('',#101492);
#8207=PLANE('',#101493);
#8208=PLANE('',#101494);
#8209=PLANE('',#101495);
#8210=PLANE('',#101496);
#8211=PLANE('',#101497);
#8212=PLANE('',#101498);
#8213=PLANE('',#101499);
#8214=PLANE('',#101500);
#8215=PLANE('',#101501);
#8216=PLANE('',#101502);
#8217=PLANE('',#101503);
#8218=PLANE('',#101504);
#8219=PLANE('',#101505);
#8220=PLANE('',#101506);
#8221=PLANE('',#101507);
#8222=PLANE('',#101508);
#8223=PLANE('',#101509);
#8224=PLANE('',#101510);
#8225=PLANE('',#101511);
#8226=PLANE('',#101512);
#8227=PLANE('',#101513);
#8228=PLANE('',#101514);
#8229=PLANE('',#101515);
#8230=PLANE('',#101516);
#8231=PLANE('',#101517);
#8232=PLANE('',#101518);
#8233=PLANE('',#101519);
#8234=PLANE('',#101520);
#8235=PLANE('',#101521);
#8236=PLANE('',#101522);
#8237=PLANE('',#101523);
#8238=PLANE('',#101524);
#8239=PLANE('',#101525);
#8240=PLANE('',#101526);
#8241=PLANE('',#101527);
#8242=PLANE('',#101528);
#8243=PLANE('',#101529);
#8244=PLANE('',#101578);
#8245=PLANE('',#101580);
#8246=PLANE('',#101581);
#8247=PLANE('',#101583);
#8248=PLANE('',#101584);
#8249=PLANE('',#101585);
#8250=PLANE('',#101589);
#8251=PLANE('',#101590);
#8252=PLANE('',#101640);
#8253=PLANE('',#101673);
#8254=PLANE('',#101677);
#8255=PLANE('',#101679);
#8256=PLANE('',#101681);
#8257=PLANE('',#101682);
#8258=PLANE('',#101683);
#8259=PLANE('',#101684);
#8260=PLANE('',#101686);
#8261=PLANE('',#101688);
#8262=PLANE('',#101690);
#8263=PLANE('',#101691);
#8264=PLANE('',#101693);
#8265=PLANE('',#101705);
#8266=PLANE('',#101707);
#8267=PLANE('',#101716);
#8268=PLANE('',#101719);
#8269=PLANE('',#101722);
#8270=PLANE('',#101723);
#8271=PLANE('',#101724);
#8272=PLANE('',#101726);
#8273=PLANE('',#101727);
#8274=PLANE('',#101728);
#8275=PLANE('',#101730);
#8276=PLANE('',#101731);
#8277=PLANE('',#101733);
#8278=PLANE('',#101734);
#8279=PLANE('',#101736);
#8280=PLANE('',#101755);
#8281=PLANE('',#101781);
#8282=PLANE('',#101791);
#8283=PLANE('',#101803);
#8284=PLANE('',#101804);
#8285=PLANE('',#101805);
#8286=PLANE('',#101811);
#8287=PLANE('',#101812);
#8288=PLANE('',#101813);
#8289=PLANE('',#101814);
#8290=PLANE('',#101815);
#8291=PLANE('',#101816);
#8292=PLANE('',#101817);
#8293=PLANE('',#101818);
#8294=PLANE('',#101819);
#8295=PLANE('',#101820);
#8296=PLANE('',#101827);
#8297=PLANE('',#101828);
#8298=PLANE('',#101829);
#8299=PLANE('',#101830);
#8300=PLANE('',#101831);
#8301=PLANE('',#101832);
#8302=PLANE('',#101833);
#8303=PLANE('',#101834);
#8304=PLANE('',#101835);
#8305=PLANE('',#101836);
#8306=PLANE('',#101837);
#8307=PLANE('',#101838);
#8308=PLANE('',#101839);
#8309=PLANE('',#101840);
#8310=PLANE('',#101841);
#8311=PLANE('',#101850);
#8312=PLANE('',#101851);
#8313=PLANE('',#101852);
#8314=PLANE('',#101853);
#8315=PLANE('',#101854);
#8316=PLANE('',#101855);
#8317=PLANE('',#101856);
#8318=PLANE('',#101857);
#8319=PLANE('',#101858);
#8320=PLANE('',#101859);
#8321=PLANE('',#101860);
#8322=PLANE('',#101861);
#8323=PLANE('',#101862);
#8324=PLANE('',#101863);
#8325=PLANE('',#101864);
#8326=PLANE('',#101865);
#8327=PLANE('',#101866);
#8328=PLANE('',#101867);
#8329=PLANE('',#101868);
#8330=PLANE('',#101869);
#8331=PLANE('',#101870);
#8332=PLANE('',#101871);
#8333=PLANE('',#101872);
#8334=PLANE('',#101873);
#8335=PLANE('',#101874);
#8336=PLANE('',#101875);
#8337=PLANE('',#101876);
#8338=PLANE('',#101877);
#8339=PLANE('',#101879);
#8340=PLANE('',#101880);
#8341=PLANE('',#101881);
#8342=PLANE('',#101882);
#8343=PLANE('',#101883);
#8344=PLANE('',#101884);
#8345=PLANE('',#101903);
#8346=PLANE('',#101905);
#8347=PLANE('',#101907);
#8348=PLANE('',#101920);
#8349=PLANE('',#101933);
#8350=PLANE('',#101934);
#8351=PLANE('',#101935);
#8352=PLANE('',#101936);
#8353=PLANE('',#101937);
#8354=PLANE('',#101938);
#8355=PLANE('',#101939);
#8356=PLANE('',#101952);
#8357=PLANE('',#101965);
#8358=PLANE('',#101966);
#8359=PLANE('',#101967);
#8360=PLANE('',#101968);
#8361=PLANE('',#101969);
#8362=PLANE('',#101970);
#8363=PLANE('',#101971);
#8364=PLANE('',#101972);
#8365=PLANE('',#101973);
#8366=PLANE('',#101974);
#8367=PLANE('',#101975);
#8368=PLANE('',#101976);
#8369=PLANE('',#101995);
#8370=PLANE('',#101997);
#8371=PLANE('',#102012);
#8372=PLANE('',#102015);
#8373=PLANE('',#102017);
#8374=PLANE('',#102019);
#8375=PLANE('',#102024);
#8376=PLANE('',#102028);
#8377=PLANE('',#102031);
#8378=PLANE('',#102035);
#8379=PLANE('',#102060);
#8380=PLANE('',#102065);
#8381=PLANE('',#102116);
#8382=PLANE('',#102124);
#8383=PLANE('',#102126);
#8384=PLANE('',#102128);
#8385=PLANE('',#102130);
#8386=PLANE('',#102131);
#8387=PLANE('',#102132);
#8388=PLANE('',#102135);
#8389=PLANE('',#102136);
#8390=PLANE('',#102150);
#8391=PLANE('',#102153);
#8392=PLANE('',#102155);
#8393=PLANE('',#102157);
#8394=PLANE('',#102162);
#8395=PLANE('',#102560);
#8396=PLANE('',#102564);
#8397=PLANE('',#102567);
#8398=PLANE('',#102568);
#8399=PLANE('',#102569);
#8400=PLANE('',#102570);
#8401=PLANE('',#102571);
#8402=PLANE('',#102572);
#8403=PLANE('',#102573);
#8404=PLANE('',#102574);
#8405=PLANE('',#102575);
#8406=PLANE('',#102576);
#8407=PLANE('',#102577);
#8408=PLANE('',#102578);
#8409=PLANE('',#102579);
#8410=PLANE('',#102580);
#8411=PLANE('',#102584);
#8412=PLANE('',#102585);
#8413=PLANE('',#102586);
#8414=PLANE('',#102590);
#8415=PLANE('',#102591);
#8416=PLANE('',#102592);
#8417=PLANE('',#102596);
#8418=PLANE('',#102597);
#8419=PLANE('',#102598);
#8420=PLANE('',#102602);
#8421=PLANE('',#102603);
#8422=PLANE('',#102604);
#8423=PLANE('',#102606);
#8424=PLANE('',#102609);
#8425=PLANE('',#102612);
#8426=PLANE('',#102613);
#8427=PLANE('',#102618);
#8428=PLANE('',#102619);
#8429=PLANE('',#102621);
#8430=PLANE('',#102623);
#8431=PLANE('',#102625);
#8432=PLANE('',#102627);
#8433=PLANE('',#102630);
#8434=PLANE('',#102632);
#8435=PLANE('',#102634);
#8436=PLANE('',#102635);
#8437=PLANE('',#102636);
#8438=PLANE('',#102637);
#8439=PLANE('',#102638);
#8440=PLANE('',#102639);
#8441=PLANE('',#102641);
#8442=PLANE('',#102642);
#8443=PLANE('',#102643);
#8444=PLANE('',#102645);
#8445=PLANE('',#102658);
#8446=PLANE('',#102671);
#8447=PLANE('',#102672);
#8448=PLANE('',#102673);
#8449=PLANE('',#102674);
#8450=PLANE('',#102675);
#8451=PLANE('',#102676);
#8452=PLANE('',#102677);
#8453=PLANE('',#102690);
#8454=PLANE('',#102703);
#8455=PLANE('',#102704);
#8456=PLANE('',#102705);
#8457=PLANE('',#102706);
#8458=PLANE('',#102707);
#8459=PLANE('',#102708);
#8460=PLANE('',#102709);
#8461=PLANE('',#102710);
#8462=PLANE('',#102711);
#8463=PLANE('',#102712);
#8464=PLANE('',#102713);
#8465=PLANE('',#102714);
#8466=PLANE('',#102733);
#8467=PLANE('',#102735);
#8468=PLANE('',#102781);
#8469=PLANE('',#102782);
#8470=PLANE('',#102783);
#8471=PLANE('',#102828);
#8472=PLANE('',#102829);
#8473=PLANE('',#102830);
#8474=PLANE('',#102831);
#8475=PLANE('',#102832);
#8476=PLANE('',#102854);
#8477=PLANE('',#102875);
#8478=PLANE('',#102876);
#8479=PLANE('',#102877);
#8480=PLANE('',#103040);
#8481=PLANE('',#103041);
#8482=PLANE('',#103044);
#8483=PLANE('',#103045);
#8484=PLANE('',#103046);
#8485=PLANE('',#103047);
#8486=PLANE('',#103048);
#8487=PLANE('',#103049);
#8488=PLANE('',#103056);
#8489=PLANE('',#103062);
#8490=PLANE('',#103063);
#8491=PLANE('',#103069);
#8492=PLANE('',#103070);
#8493=PLANE('',#103076);
#8494=PLANE('',#103077);
#8495=PLANE('',#103085);
#8496=PLANE('',#103101);
#8497=PLANE('',#103102);
#8498=PLANE('',#103103);
#8499=PLANE('',#103104);
#8500=PLANE('',#103105);
#8501=PLANE('',#103106);
#8502=PLANE('',#103121);
#8503=PLANE('',#103168);
#8504=PLANE('',#103171);
#8505=PLANE('',#103172);
#8506=PLANE('',#103173);
#8507=PLANE('',#103186);
#8508=PLANE('',#103194);
#8509=PLANE('',#103201);
#8510=PLANE('',#103209);
#8511=PLANE('',#103233);
#8512=PLANE('',#103241);
#8513=PLANE('',#103253);
#8514=PLANE('',#103261);
#8515=PLANE('',#103304);
#8516=PLANE('',#103310);
#8517=PLANE('',#103311);
#8740=FACE_OUTER_BOUND('',#14527,.T.);
#8741=FACE_OUTER_BOUND('',#14528,.T.);
#8742=FACE_OUTER_BOUND('',#14529,.T.);
#8743=FACE_OUTER_BOUND('',#14530,.T.);
#8744=FACE_OUTER_BOUND('',#14532,.T.);
#8745=FACE_OUTER_BOUND('',#14533,.T.);
#8746=FACE_OUTER_BOUND('',#14534,.T.);
#8747=FACE_OUTER_BOUND('',#14535,.T.);
#8748=FACE_OUTER_BOUND('',#14536,.T.);
#8749=FACE_OUTER_BOUND('',#14537,.T.);
#8750=FACE_OUTER_BOUND('',#14539,.T.);
#8751=FACE_OUTER_BOUND('',#14540,.T.);
#8752=FACE_OUTER_BOUND('',#14541,.T.);
#8753=FACE_OUTER_BOUND('',#14542,.T.);
#8754=FACE_OUTER_BOUND('',#14543,.T.);
#8755=FACE_OUTER_BOUND('',#14544,.T.);
#8756=FACE_OUTER_BOUND('',#14545,.T.);
#8757=FACE_OUTER_BOUND('',#14546,.T.);
#8758=FACE_OUTER_BOUND('',#14547,.T.);
#8759=FACE_OUTER_BOUND('',#14548,.T.);
#8760=FACE_OUTER_BOUND('',#14549,.T.);
#8761=FACE_OUTER_BOUND('',#14550,.T.);
#8762=FACE_OUTER_BOUND('',#14551,.T.);
#8763=FACE_OUTER_BOUND('',#14552,.T.);
#8764=FACE_OUTER_BOUND('',#14553,.T.);
#8765=FACE_OUTER_BOUND('',#14554,.T.);
#8766=FACE_OUTER_BOUND('',#14555,.T.);
#8767=FACE_OUTER_BOUND('',#14556,.T.);
#8768=FACE_OUTER_BOUND('',#14557,.T.);
#8769=FACE_OUTER_BOUND('',#14558,.T.);
#8770=FACE_OUTER_BOUND('',#14559,.T.);
#8771=FACE_OUTER_BOUND('',#14560,.T.);
#8772=FACE_OUTER_BOUND('',#14561,.T.);
#8773=FACE_OUTER_BOUND('',#14562,.T.);
#8774=FACE_OUTER_BOUND('',#14563,.T.);
#8775=FACE_OUTER_BOUND('',#14564,.T.);
#8776=FACE_OUTER_BOUND('',#14565,.T.);
#8777=FACE_OUTER_BOUND('',#14566,.T.);
#8778=FACE_OUTER_BOUND('',#14567,.T.);
#8779=FACE_OUTER_BOUND('',#14568,.T.);
#8780=FACE_OUTER_BOUND('',#14569,.T.);
#8781=FACE_OUTER_BOUND('',#14570,.T.);
#8782=FACE_OUTER_BOUND('',#14571,.T.);
#8783=FACE_OUTER_BOUND('',#14572,.T.);
#8784=FACE_OUTER_BOUND('',#14573,.T.);
#8785=FACE_OUTER_BOUND('',#14574,.T.);
#8786=FACE_OUTER_BOUND('',#14575,.T.);
#8787=FACE_OUTER_BOUND('',#14576,.T.);
#8788=FACE_OUTER_BOUND('',#14577,.T.);
#8789=FACE_OUTER_BOUND('',#14578,.T.);
#8790=FACE_OUTER_BOUND('',#14579,.T.);
#8791=FACE_OUTER_BOUND('',#14580,.T.);
#8792=FACE_OUTER_BOUND('',#14581,.T.);
#8793=FACE_OUTER_BOUND('',#14582,.T.);
#8794=FACE_OUTER_BOUND('',#14583,.T.);
#8795=FACE_OUTER_BOUND('',#14584,.T.);
#8796=FACE_OUTER_BOUND('',#14585,.T.);
#8797=FACE_OUTER_BOUND('',#14586,.T.);
#8798=FACE_OUTER_BOUND('',#14587,.T.);
#8799=FACE_OUTER_BOUND('',#14588,.T.);
#8800=FACE_OUTER_BOUND('',#14589,.T.);
#8801=FACE_OUTER_BOUND('',#14590,.T.);
#8802=FACE_OUTER_BOUND('',#14591,.T.);
#8803=FACE_OUTER_BOUND('',#14592,.T.);
#8804=FACE_OUTER_BOUND('',#14593,.T.);
#8805=FACE_OUTER_BOUND('',#14594,.T.);
#8806=FACE_OUTER_BOUND('',#14595,.T.);
#8807=FACE_OUTER_BOUND('',#14596,.T.);
#8808=FACE_OUTER_BOUND('',#14597,.T.);
#8809=FACE_OUTER_BOUND('',#14598,.T.);
#8810=FACE_OUTER_BOUND('',#14599,.T.);
#8811=FACE_OUTER_BOUND('',#14600,.T.);
#8812=FACE_OUTER_BOUND('',#14601,.T.);
#8813=FACE_OUTER_BOUND('',#14602,.T.);
#8814=FACE_OUTER_BOUND('',#14603,.T.);
#8815=FACE_OUTER_BOUND('',#14604,.T.);
#8816=FACE_OUTER_BOUND('',#14605,.T.);
#8817=FACE_OUTER_BOUND('',#14606,.T.);
#8818=FACE_OUTER_BOUND('',#14607,.T.);
#8819=FACE_OUTER_BOUND('',#14608,.T.);
#8820=FACE_OUTER_BOUND('',#14609,.T.);
#8821=FACE_OUTER_BOUND('',#14610,.T.);
#8822=FACE_OUTER_BOUND('',#14611,.T.);
#8823=FACE_OUTER_BOUND('',#14612,.T.);
#8824=FACE_OUTER_BOUND('',#14613,.T.);
#8825=FACE_OUTER_BOUND('',#14614,.T.);
#8826=FACE_OUTER_BOUND('',#14615,.T.);
#8827=FACE_OUTER_BOUND('',#14616,.T.);
#8828=FACE_OUTER_BOUND('',#14617,.T.);
#8829=FACE_OUTER_BOUND('',#14618,.T.);
#8830=FACE_OUTER_BOUND('',#14619,.T.);
#8831=FACE_OUTER_BOUND('',#14620,.T.);
#8832=FACE_OUTER_BOUND('',#14621,.T.);
#8833=FACE_OUTER_BOUND('',#14622,.T.);
#8834=FACE_OUTER_BOUND('',#14623,.T.);
#8835=FACE_OUTER_BOUND('',#14624,.T.);
#8836=FACE_OUTER_BOUND('',#14625,.T.);
#8837=FACE_OUTER_BOUND('',#14626,.T.);
#8838=FACE_OUTER_BOUND('',#14627,.T.);
#8839=FACE_OUTER_BOUND('',#14628,.T.);
#8840=FACE_OUTER_BOUND('',#14629,.T.);
#8841=FACE_OUTER_BOUND('',#14630,.T.);
#8842=FACE_OUTER_BOUND('',#14631,.T.);
#8843=FACE_OUTER_BOUND('',#14632,.T.);
#8844=FACE_OUTER_BOUND('',#14633,.T.);
#8845=FACE_OUTER_BOUND('',#14634,.T.);
#8846=FACE_OUTER_BOUND('',#14635,.T.);
#8847=FACE_OUTER_BOUND('',#14636,.T.);
#8848=FACE_OUTER_BOUND('',#14637,.T.);
#8849=FACE_OUTER_BOUND('',#14638,.T.);
#8850=FACE_OUTER_BOUND('',#14639,.T.);
#8851=FACE_OUTER_BOUND('',#14640,.T.);
#8852=FACE_OUTER_BOUND('',#14641,.T.);
#8853=FACE_OUTER_BOUND('',#14642,.T.);
#8854=FACE_OUTER_BOUND('',#14643,.T.);
#8855=FACE_OUTER_BOUND('',#14644,.T.);
#8856=FACE_OUTER_BOUND('',#14645,.T.);
#8857=FACE_OUTER_BOUND('',#14646,.T.);
#8858=FACE_OUTER_BOUND('',#14647,.T.);
#8859=FACE_OUTER_BOUND('',#14648,.T.);
#8860=FACE_OUTER_BOUND('',#14649,.T.);
#8861=FACE_OUTER_BOUND('',#14650,.T.);
#8862=FACE_OUTER_BOUND('',#14651,.T.);
#8863=FACE_OUTER_BOUND('',#14652,.T.);
#8864=FACE_OUTER_BOUND('',#14653,.T.);
#8865=FACE_OUTER_BOUND('',#14654,.T.);
#8866=FACE_OUTER_BOUND('',#14655,.T.);
#8867=FACE_OUTER_BOUND('',#14656,.T.);
#8868=FACE_OUTER_BOUND('',#14657,.T.);
#8869=FACE_OUTER_BOUND('',#14658,.T.);
#8870=FACE_OUTER_BOUND('',#14659,.T.);
#8871=FACE_OUTER_BOUND('',#14660,.T.);
#8872=FACE_OUTER_BOUND('',#14661,.T.);
#8873=FACE_OUTER_BOUND('',#14662,.T.);
#8874=FACE_OUTER_BOUND('',#14663,.T.);
#8875=FACE_OUTER_BOUND('',#14664,.T.);
#8876=FACE_OUTER_BOUND('',#14665,.T.);
#8877=FACE_OUTER_BOUND('',#14666,.T.);
#8878=FACE_OUTER_BOUND('',#14667,.T.);
#8879=FACE_OUTER_BOUND('',#14668,.T.);
#8880=FACE_OUTER_BOUND('',#14669,.T.);
#8881=FACE_OUTER_BOUND('',#14670,.T.);
#8882=FACE_OUTER_BOUND('',#14671,.T.);
#8883=FACE_OUTER_BOUND('',#14672,.T.);
#8884=FACE_OUTER_BOUND('',#14673,.T.);
#8885=FACE_OUTER_BOUND('',#14674,.T.);
#8886=FACE_OUTER_BOUND('',#14675,.T.);
#8887=FACE_OUTER_BOUND('',#14676,.T.);
#8888=FACE_OUTER_BOUND('',#14677,.T.);
#8889=FACE_OUTER_BOUND('',#14678,.T.);
#8890=FACE_OUTER_BOUND('',#14679,.T.);
#8891=FACE_OUTER_BOUND('',#14680,.T.);
#8892=FACE_OUTER_BOUND('',#14681,.T.);
#8893=FACE_OUTER_BOUND('',#14682,.T.);
#8894=FACE_OUTER_BOUND('',#14683,.T.);
#8895=FACE_OUTER_BOUND('',#14684,.T.);
#8896=FACE_OUTER_BOUND('',#14685,.T.);
#8897=FACE_OUTER_BOUND('',#14686,.T.);
#8898=FACE_OUTER_BOUND('',#14687,.T.);
#8899=FACE_OUTER_BOUND('',#14688,.T.);
#8900=FACE_OUTER_BOUND('',#14689,.T.);
#8901=FACE_OUTER_BOUND('',#14690,.T.);
#8902=FACE_OUTER_BOUND('',#14691,.T.);
#8903=FACE_OUTER_BOUND('',#14692,.T.);
#8904=FACE_OUTER_BOUND('',#14693,.T.);
#8905=FACE_OUTER_BOUND('',#14694,.T.);
#8906=FACE_OUTER_BOUND('',#14695,.T.);
#8907=FACE_OUTER_BOUND('',#14696,.T.);
#8908=FACE_OUTER_BOUND('',#14697,.T.);
#8909=FACE_OUTER_BOUND('',#14698,.T.);
#8910=FACE_OUTER_BOUND('',#14699,.T.);
#8911=FACE_OUTER_BOUND('',#14700,.T.);
#8912=FACE_OUTER_BOUND('',#14701,.T.);
#8913=FACE_OUTER_BOUND('',#14702,.T.);
#8914=FACE_OUTER_BOUND('',#14703,.T.);
#8915=FACE_OUTER_BOUND('',#14704,.T.);
#8916=FACE_OUTER_BOUND('',#14705,.T.);
#8917=FACE_OUTER_BOUND('',#14706,.T.);
#8918=FACE_OUTER_BOUND('',#14707,.T.);
#8919=FACE_OUTER_BOUND('',#14708,.T.);
#8920=FACE_OUTER_BOUND('',#14709,.T.);
#8921=FACE_OUTER_BOUND('',#14710,.T.);
#8922=FACE_OUTER_BOUND('',#14711,.T.);
#8923=FACE_OUTER_BOUND('',#14712,.T.);
#8924=FACE_OUTER_BOUND('',#14713,.T.);
#8925=FACE_OUTER_BOUND('',#14714,.T.);
#8926=FACE_OUTER_BOUND('',#14715,.T.);
#8927=FACE_OUTER_BOUND('',#14716,.T.);
#8928=FACE_OUTER_BOUND('',#14717,.T.);
#8929=FACE_OUTER_BOUND('',#14718,.T.);
#8930=FACE_OUTER_BOUND('',#14719,.T.);
#8931=FACE_OUTER_BOUND('',#14720,.T.);
#8932=FACE_OUTER_BOUND('',#14721,.T.);
#8933=FACE_OUTER_BOUND('',#14722,.T.);
#8934=FACE_OUTER_BOUND('',#14723,.T.);
#8935=FACE_OUTER_BOUND('',#14724,.T.);
#8936=FACE_OUTER_BOUND('',#14725,.T.);
#8937=FACE_OUTER_BOUND('',#14726,.T.);
#8938=FACE_OUTER_BOUND('',#14727,.T.);
#8939=FACE_OUTER_BOUND('',#14728,.T.);
#8940=FACE_OUTER_BOUND('',#14729,.T.);
#8941=FACE_OUTER_BOUND('',#14730,.T.);
#8942=FACE_OUTER_BOUND('',#14731,.T.);
#8943=FACE_OUTER_BOUND('',#14732,.T.);
#8944=FACE_OUTER_BOUND('',#14733,.T.);
#8945=FACE_OUTER_BOUND('',#14734,.T.);
#8946=FACE_OUTER_BOUND('',#14735,.T.);
#8947=FACE_OUTER_BOUND('',#14736,.T.);
#8948=FACE_OUTER_BOUND('',#14737,.T.);
#8949=FACE_OUTER_BOUND('',#14738,.T.);
#8950=FACE_OUTER_BOUND('',#14739,.T.);
#8951=FACE_OUTER_BOUND('',#14740,.T.);
#8952=FACE_OUTER_BOUND('',#14741,.T.);
#8953=FACE_OUTER_BOUND('',#14742,.T.);
#8954=FACE_OUTER_BOUND('',#14743,.T.);
#8955=FACE_OUTER_BOUND('',#14744,.T.);
#8956=FACE_OUTER_BOUND('',#14745,.T.);
#8957=FACE_OUTER_BOUND('',#14746,.T.);
#8958=FACE_OUTER_BOUND('',#14747,.T.);
#8959=FACE_OUTER_BOUND('',#14748,.T.);
#8960=FACE_OUTER_BOUND('',#14749,.T.);
#8961=FACE_OUTER_BOUND('',#14750,.T.);
#8962=FACE_OUTER_BOUND('',#14751,.T.);
#8963=FACE_OUTER_BOUND('',#14752,.T.);
#8964=FACE_OUTER_BOUND('',#14753,.T.);
#8965=FACE_OUTER_BOUND('',#14754,.T.);
#8966=FACE_OUTER_BOUND('',#14755,.T.);
#8967=FACE_OUTER_BOUND('',#14756,.T.);
#8968=FACE_OUTER_BOUND('',#14757,.T.);
#8969=FACE_OUTER_BOUND('',#14758,.T.);
#8970=FACE_OUTER_BOUND('',#14759,.T.);
#8971=FACE_OUTER_BOUND('',#14760,.T.);
#8972=FACE_OUTER_BOUND('',#14761,.T.);
#8973=FACE_OUTER_BOUND('',#14762,.T.);
#8974=FACE_OUTER_BOUND('',#14763,.T.);
#8975=FACE_OUTER_BOUND('',#14764,.T.);
#8976=FACE_OUTER_BOUND('',#14765,.T.);
#8977=FACE_OUTER_BOUND('',#14766,.T.);
#8978=FACE_OUTER_BOUND('',#14767,.T.);
#8979=FACE_OUTER_BOUND('',#14768,.T.);
#8980=FACE_OUTER_BOUND('',#14769,.T.);
#8981=FACE_OUTER_BOUND('',#14770,.T.);
#8982=FACE_OUTER_BOUND('',#14771,.T.);
#8983=FACE_OUTER_BOUND('',#14772,.T.);
#8984=FACE_OUTER_BOUND('',#14773,.T.);
#8985=FACE_OUTER_BOUND('',#14774,.T.);
#8986=FACE_OUTER_BOUND('',#14775,.T.);
#8987=FACE_OUTER_BOUND('',#14776,.T.);
#8988=FACE_OUTER_BOUND('',#14777,.T.);
#8989=FACE_OUTER_BOUND('',#14778,.T.);
#8990=FACE_OUTER_BOUND('',#14779,.T.);
#8991=FACE_OUTER_BOUND('',#14780,.T.);
#8992=FACE_OUTER_BOUND('',#14781,.T.);
#8993=FACE_OUTER_BOUND('',#14782,.T.);
#8994=FACE_OUTER_BOUND('',#14783,.T.);
#8995=FACE_OUTER_BOUND('',#14784,.T.);
#8996=FACE_OUTER_BOUND('',#14785,.T.);
#8997=FACE_OUTER_BOUND('',#14786,.T.);
#8998=FACE_OUTER_BOUND('',#14787,.T.);
#8999=FACE_OUTER_BOUND('',#14788,.T.);
#9000=FACE_OUTER_BOUND('',#14789,.T.);
#9001=FACE_OUTER_BOUND('',#14790,.T.);
#9002=FACE_OUTER_BOUND('',#14791,.T.);
#9003=FACE_OUTER_BOUND('',#14792,.T.);
#9004=FACE_OUTER_BOUND('',#14793,.T.);
#9005=FACE_OUTER_BOUND('',#14794,.T.);
#9006=FACE_OUTER_BOUND('',#14795,.T.);
#9007=FACE_OUTER_BOUND('',#14796,.T.);
#9008=FACE_OUTER_BOUND('',#14797,.T.);
#9009=FACE_OUTER_BOUND('',#14798,.T.);
#9010=FACE_OUTER_BOUND('',#14799,.T.);
#9011=FACE_OUTER_BOUND('',#14800,.T.);
#9012=FACE_OUTER_BOUND('',#14801,.T.);
#9013=FACE_OUTER_BOUND('',#14802,.T.);
#9014=FACE_OUTER_BOUND('',#14803,.T.);
#9015=FACE_OUTER_BOUND('',#14804,.T.);
#9016=FACE_OUTER_BOUND('',#14805,.T.);
#9017=FACE_OUTER_BOUND('',#14806,.T.);
#9018=FACE_OUTER_BOUND('',#14807,.T.);
#9019=FACE_OUTER_BOUND('',#14808,.T.);
#9020=FACE_OUTER_BOUND('',#14809,.T.);
#9021=FACE_OUTER_BOUND('',#14810,.T.);
#9022=FACE_OUTER_BOUND('',#14811,.T.);
#9023=FACE_OUTER_BOUND('',#14812,.T.);
#9024=FACE_OUTER_BOUND('',#14813,.T.);
#9025=FACE_OUTER_BOUND('',#14814,.T.);
#9026=FACE_OUTER_BOUND('',#14815,.T.);
#9027=FACE_OUTER_BOUND('',#14816,.T.);
#9028=FACE_OUTER_BOUND('',#14817,.T.);
#9029=FACE_OUTER_BOUND('',#14818,.T.);
#9030=FACE_OUTER_BOUND('',#14819,.T.);
#9031=FACE_OUTER_BOUND('',#14820,.T.);
#9032=FACE_OUTER_BOUND('',#14821,.T.);
#9033=FACE_OUTER_BOUND('',#14822,.T.);
#9034=FACE_OUTER_BOUND('',#14823,.T.);
#9035=FACE_OUTER_BOUND('',#14824,.T.);
#9036=FACE_OUTER_BOUND('',#14825,.T.);
#9037=FACE_OUTER_BOUND('',#14826,.T.);
#9038=FACE_OUTER_BOUND('',#14827,.T.);
#9039=FACE_OUTER_BOUND('',#14828,.T.);
#9040=FACE_OUTER_BOUND('',#14829,.T.);
#9041=FACE_OUTER_BOUND('',#14830,.T.);
#9042=FACE_OUTER_BOUND('',#14831,.T.);
#9043=FACE_OUTER_BOUND('',#14832,.T.);
#9044=FACE_OUTER_BOUND('',#14833,.T.);
#9045=FACE_OUTER_BOUND('',#14834,.T.);
#9046=FACE_OUTER_BOUND('',#14835,.T.);
#9047=FACE_OUTER_BOUND('',#14836,.T.);
#9048=FACE_OUTER_BOUND('',#14837,.T.);
#9049=FACE_OUTER_BOUND('',#14838,.T.);
#9050=FACE_OUTER_BOUND('',#14839,.T.);
#9051=FACE_OUTER_BOUND('',#14840,.T.);
#9052=FACE_OUTER_BOUND('',#14841,.T.);
#9053=FACE_OUTER_BOUND('',#14842,.T.);
#9054=FACE_OUTER_BOUND('',#14843,.T.);
#9055=FACE_OUTER_BOUND('',#14844,.T.);
#9056=FACE_OUTER_BOUND('',#14845,.T.);
#9057=FACE_OUTER_BOUND('',#14846,.T.);
#9058=FACE_OUTER_BOUND('',#14847,.T.);
#9059=FACE_OUTER_BOUND('',#14848,.T.);
#9060=FACE_OUTER_BOUND('',#14849,.T.);
#9061=FACE_OUTER_BOUND('',#14850,.T.);
#9062=FACE_OUTER_BOUND('',#14851,.T.);
#9063=FACE_OUTER_BOUND('',#14852,.T.);
#9064=FACE_OUTER_BOUND('',#14853,.T.);
#9065=FACE_OUTER_BOUND('',#14854,.T.);
#9066=FACE_OUTER_BOUND('',#14855,.T.);
#9067=FACE_OUTER_BOUND('',#14856,.T.);
#9068=FACE_OUTER_BOUND('',#14857,.T.);
#9069=FACE_OUTER_BOUND('',#14858,.T.);
#9070=FACE_OUTER_BOUND('',#14859,.T.);
#9071=FACE_OUTER_BOUND('',#14860,.T.);
#9072=FACE_OUTER_BOUND('',#14861,.T.);
#9073=FACE_OUTER_BOUND('',#14862,.T.);
#9074=FACE_OUTER_BOUND('',#14863,.T.);
#9075=FACE_OUTER_BOUND('',#14864,.T.);
#9076=FACE_OUTER_BOUND('',#14865,.T.);
#9077=FACE_OUTER_BOUND('',#14866,.T.);
#9078=FACE_OUTER_BOUND('',#14867,.T.);
#9079=FACE_OUTER_BOUND('',#14868,.T.);
#9080=FACE_OUTER_BOUND('',#14869,.T.);
#9081=FACE_OUTER_BOUND('',#14870,.T.);
#9082=FACE_OUTER_BOUND('',#14871,.T.);
#9083=FACE_OUTER_BOUND('',#14872,.T.);
#9084=FACE_OUTER_BOUND('',#14873,.T.);
#9085=FACE_OUTER_BOUND('',#14874,.T.);
#9086=FACE_OUTER_BOUND('',#14875,.T.);
#9087=FACE_OUTER_BOUND('',#14876,.T.);
#9088=FACE_OUTER_BOUND('',#14877,.T.);
#9089=FACE_OUTER_BOUND('',#14878,.T.);
#9090=FACE_OUTER_BOUND('',#14879,.T.);
#9091=FACE_OUTER_BOUND('',#14880,.T.);
#9092=FACE_OUTER_BOUND('',#14881,.T.);
#9093=FACE_OUTER_BOUND('',#14882,.T.);
#9094=FACE_OUTER_BOUND('',#14883,.T.);
#9095=FACE_OUTER_BOUND('',#14884,.T.);
#9096=FACE_OUTER_BOUND('',#14885,.T.);
#9097=FACE_OUTER_BOUND('',#14886,.T.);
#9098=FACE_OUTER_BOUND('',#14887,.T.);
#9099=FACE_OUTER_BOUND('',#14888,.T.);
#9100=FACE_OUTER_BOUND('',#14889,.T.);
#9101=FACE_OUTER_BOUND('',#14890,.T.);
#9102=FACE_OUTER_BOUND('',#14891,.T.);
#9103=FACE_OUTER_BOUND('',#14892,.T.);
#9104=FACE_OUTER_BOUND('',#14893,.T.);
#9105=FACE_OUTER_BOUND('',#14894,.T.);
#9106=FACE_OUTER_BOUND('',#14895,.T.);
#9107=FACE_OUTER_BOUND('',#14896,.T.);
#9108=FACE_OUTER_BOUND('',#14897,.T.);
#9109=FACE_OUTER_BOUND('',#14898,.T.);
#9110=FACE_OUTER_BOUND('',#14899,.T.);
#9111=FACE_OUTER_BOUND('',#14900,.T.);
#9112=FACE_OUTER_BOUND('',#14901,.T.);
#9113=FACE_OUTER_BOUND('',#14902,.T.);
#9114=FACE_OUTER_BOUND('',#14903,.T.);
#9115=FACE_OUTER_BOUND('',#14904,.T.);
#9116=FACE_OUTER_BOUND('',#14905,.T.);
#9117=FACE_OUTER_BOUND('',#14906,.T.);
#9118=FACE_OUTER_BOUND('',#14907,.T.);
#9119=FACE_OUTER_BOUND('',#14908,.T.);
#9120=FACE_OUTER_BOUND('',#14909,.T.);
#9121=FACE_OUTER_BOUND('',#14910,.T.);
#9122=FACE_OUTER_BOUND('',#14911,.T.);
#9123=FACE_OUTER_BOUND('',#14912,.T.);
#9124=FACE_OUTER_BOUND('',#14913,.T.);
#9125=FACE_OUTER_BOUND('',#14914,.T.);
#9126=FACE_OUTER_BOUND('',#14915,.T.);
#9127=FACE_OUTER_BOUND('',#14916,.T.);
#9128=FACE_OUTER_BOUND('',#14917,.T.);
#9129=FACE_OUTER_BOUND('',#14918,.T.);
#9130=FACE_OUTER_BOUND('',#14919,.T.);
#9131=FACE_OUTER_BOUND('',#14920,.T.);
#9132=FACE_OUTER_BOUND('',#14921,.T.);
#9133=FACE_OUTER_BOUND('',#14922,.T.);
#9134=FACE_OUTER_BOUND('',#14923,.T.);
#9135=FACE_OUTER_BOUND('',#14924,.T.);
#9136=FACE_OUTER_BOUND('',#14925,.T.);
#9137=FACE_OUTER_BOUND('',#14926,.T.);
#9138=FACE_OUTER_BOUND('',#14927,.T.);
#9139=FACE_OUTER_BOUND('',#14928,.T.);
#9140=FACE_OUTER_BOUND('',#14929,.T.);
#9141=FACE_OUTER_BOUND('',#14930,.T.);
#9142=FACE_OUTER_BOUND('',#14931,.T.);
#9143=FACE_OUTER_BOUND('',#14932,.T.);
#9144=FACE_OUTER_BOUND('',#14933,.T.);
#9145=FACE_OUTER_BOUND('',#14934,.T.);
#9146=FACE_OUTER_BOUND('',#14935,.T.);
#9147=FACE_OUTER_BOUND('',#14936,.T.);
#9148=FACE_OUTER_BOUND('',#14937,.T.);
#9149=FACE_OUTER_BOUND('',#14938,.T.);
#9150=FACE_OUTER_BOUND('',#14939,.T.);
#9151=FACE_OUTER_BOUND('',#14940,.T.);
#9152=FACE_OUTER_BOUND('',#14941,.T.);
#9153=FACE_OUTER_BOUND('',#14942,.T.);
#9154=FACE_OUTER_BOUND('',#14943,.T.);
#9155=FACE_OUTER_BOUND('',#14944,.T.);
#9156=FACE_OUTER_BOUND('',#14945,.T.);
#9157=FACE_OUTER_BOUND('',#14946,.T.);
#9158=FACE_OUTER_BOUND('',#14947,.T.);
#9159=FACE_OUTER_BOUND('',#14948,.T.);
#9160=FACE_OUTER_BOUND('',#14949,.T.);
#9161=FACE_OUTER_BOUND('',#14950,.T.);
#9162=FACE_OUTER_BOUND('',#14951,.T.);
#9163=FACE_OUTER_BOUND('',#14952,.T.);
#9164=FACE_OUTER_BOUND('',#14953,.T.);
#9165=FACE_OUTER_BOUND('',#14954,.T.);
#9166=FACE_OUTER_BOUND('',#14955,.T.);
#9167=FACE_OUTER_BOUND('',#14956,.T.);
#9168=FACE_OUTER_BOUND('',#14958,.T.);
#9169=FACE_OUTER_BOUND('',#14959,.T.);
#9170=FACE_OUTER_BOUND('',#14960,.T.);
#9171=FACE_OUTER_BOUND('',#14961,.T.);
#9172=FACE_OUTER_BOUND('',#14962,.T.);
#9173=FACE_OUTER_BOUND('',#14963,.T.);
#9174=FACE_OUTER_BOUND('',#14964,.T.);
#9175=FACE_OUTER_BOUND('',#14965,.T.);
#9176=FACE_OUTER_BOUND('',#14966,.T.);
#9177=FACE_OUTER_BOUND('',#14968,.T.);
#9178=FACE_OUTER_BOUND('',#14969,.T.);
#9179=FACE_OUTER_BOUND('',#14970,.T.);
#9180=FACE_OUTER_BOUND('',#14971,.T.);
#9181=FACE_OUTER_BOUND('',#14972,.T.);
#9182=FACE_OUTER_BOUND('',#14973,.T.);
#9183=FACE_OUTER_BOUND('',#14974,.T.);
#9184=FACE_OUTER_BOUND('',#14975,.T.);
#9185=FACE_OUTER_BOUND('',#14976,.T.);
#9186=FACE_OUTER_BOUND('',#14977,.T.);
#9187=FACE_OUTER_BOUND('',#14978,.T.);
#9188=FACE_OUTER_BOUND('',#14979,.T.);
#9189=FACE_OUTER_BOUND('',#14980,.T.);
#9190=FACE_OUTER_BOUND('',#14981,.T.);
#9191=FACE_OUTER_BOUND('',#14982,.T.);
#9192=FACE_OUTER_BOUND('',#14983,.T.);
#9193=FACE_OUTER_BOUND('',#14984,.T.);
#9194=FACE_OUTER_BOUND('',#14985,.T.);
#9195=FACE_OUTER_BOUND('',#14986,.T.);
#9196=FACE_OUTER_BOUND('',#14987,.T.);
#9197=FACE_OUTER_BOUND('',#14988,.T.);
#9198=FACE_OUTER_BOUND('',#14989,.T.);
#9199=FACE_OUTER_BOUND('',#14990,.T.);
#9200=FACE_OUTER_BOUND('',#14991,.T.);
#9201=FACE_OUTER_BOUND('',#14992,.T.);
#9202=FACE_OUTER_BOUND('',#14993,.T.);
#9203=FACE_OUTER_BOUND('',#14994,.T.);
#9204=FACE_OUTER_BOUND('',#14995,.T.);
#9205=FACE_OUTER_BOUND('',#14996,.T.);
#9206=FACE_OUTER_BOUND('',#14997,.T.);
#9207=FACE_OUTER_BOUND('',#14998,.T.);
#9208=FACE_OUTER_BOUND('',#14999,.T.);
#9209=FACE_OUTER_BOUND('',#15000,.T.);
#9210=FACE_OUTER_BOUND('',#15001,.T.);
#9211=FACE_OUTER_BOUND('',#15002,.T.);
#9212=FACE_OUTER_BOUND('',#15003,.T.);
#9213=FACE_OUTER_BOUND('',#15004,.T.);
#9214=FACE_OUTER_BOUND('',#15005,.T.);
#9215=FACE_OUTER_BOUND('',#15006,.T.);
#9216=FACE_OUTER_BOUND('',#15007,.T.);
#9217=FACE_OUTER_BOUND('',#15008,.T.);
#9218=FACE_OUTER_BOUND('',#15009,.T.);
#9219=FACE_OUTER_BOUND('',#15010,.T.);
#9220=FACE_OUTER_BOUND('',#15011,.T.);
#9221=FACE_OUTER_BOUND('',#15012,.T.);
#9222=FACE_OUTER_BOUND('',#15013,.T.);
#9223=FACE_OUTER_BOUND('',#15014,.T.);
#9224=FACE_OUTER_BOUND('',#15015,.T.);
#9225=FACE_OUTER_BOUND('',#15016,.T.);
#9226=FACE_OUTER_BOUND('',#15017,.T.);
#9227=FACE_OUTER_BOUND('',#15018,.T.);
#9228=FACE_OUTER_BOUND('',#15019,.T.);
#9229=FACE_OUTER_BOUND('',#15020,.T.);
#9230=FACE_OUTER_BOUND('',#15021,.T.);
#9231=FACE_OUTER_BOUND('',#15022,.T.);
#9232=FACE_OUTER_BOUND('',#15023,.T.);
#9233=FACE_OUTER_BOUND('',#15024,.T.);
#9234=FACE_OUTER_BOUND('',#15025,.T.);
#9235=FACE_OUTER_BOUND('',#15026,.T.);
#9236=FACE_OUTER_BOUND('',#15027,.T.);
#9237=FACE_OUTER_BOUND('',#15028,.T.);
#9238=FACE_OUTER_BOUND('',#15029,.T.);
#9239=FACE_OUTER_BOUND('',#15030,.T.);
#9240=FACE_OUTER_BOUND('',#15031,.T.);
#9241=FACE_OUTER_BOUND('',#15032,.T.);
#9242=FACE_OUTER_BOUND('',#15033,.T.);
#9243=FACE_OUTER_BOUND('',#15034,.T.);
#9244=FACE_OUTER_BOUND('',#15035,.T.);
#9245=FACE_OUTER_BOUND('',#15036,.T.);
#9246=FACE_OUTER_BOUND('',#15037,.T.);
#9247=FACE_OUTER_BOUND('',#15038,.T.);
#9248=FACE_OUTER_BOUND('',#15039,.T.);
#9249=FACE_OUTER_BOUND('',#15040,.T.);
#9250=FACE_OUTER_BOUND('',#15041,.T.);
#9251=FACE_OUTER_BOUND('',#15042,.T.);
#9252=FACE_OUTER_BOUND('',#15043,.T.);
#9253=FACE_OUTER_BOUND('',#15044,.T.);
#9254=FACE_OUTER_BOUND('',#15045,.T.);
#9255=FACE_OUTER_BOUND('',#15046,.T.);
#9256=FACE_OUTER_BOUND('',#15047,.T.);
#9257=FACE_OUTER_BOUND('',#15048,.T.);
#9258=FACE_OUTER_BOUND('',#15049,.T.);
#9259=FACE_OUTER_BOUND('',#15050,.T.);
#9260=FACE_OUTER_BOUND('',#15051,.T.);
#9261=FACE_OUTER_BOUND('',#15052,.T.);
#9262=FACE_OUTER_BOUND('',#15053,.T.);
#9263=FACE_OUTER_BOUND('',#15054,.T.);
#9264=FACE_OUTER_BOUND('',#15055,.T.);
#9265=FACE_OUTER_BOUND('',#15056,.T.);
#9266=FACE_OUTER_BOUND('',#15057,.T.);
#9267=FACE_OUTER_BOUND('',#15058,.T.);
#9268=FACE_OUTER_BOUND('',#15059,.T.);
#9269=FACE_OUTER_BOUND('',#15060,.T.);
#9270=FACE_OUTER_BOUND('',#15061,.T.);
#9271=FACE_OUTER_BOUND('',#15062,.T.);
#9272=FACE_OUTER_BOUND('',#15063,.T.);
#9273=FACE_OUTER_BOUND('',#15064,.T.);
#9274=FACE_OUTER_BOUND('',#15065,.T.);
#9275=FACE_OUTER_BOUND('',#15066,.T.);
#9276=FACE_OUTER_BOUND('',#15067,.T.);
#9277=FACE_OUTER_BOUND('',#15068,.T.);
#9278=FACE_OUTER_BOUND('',#15069,.T.);
#9279=FACE_OUTER_BOUND('',#15070,.T.);
#9280=FACE_OUTER_BOUND('',#15071,.T.);
#9281=FACE_OUTER_BOUND('',#15072,.T.);
#9282=FACE_OUTER_BOUND('',#15073,.T.);
#9283=FACE_OUTER_BOUND('',#15074,.T.);
#9284=FACE_OUTER_BOUND('',#15075,.T.);
#9285=FACE_OUTER_BOUND('',#15076,.T.);
#9286=FACE_OUTER_BOUND('',#15077,.T.);
#9287=FACE_OUTER_BOUND('',#15078,.T.);
#9288=FACE_OUTER_BOUND('',#15079,.T.);
#9289=FACE_OUTER_BOUND('',#15080,.T.);
#9290=FACE_OUTER_BOUND('',#15081,.T.);
#9291=FACE_OUTER_BOUND('',#15082,.T.);
#9292=FACE_OUTER_BOUND('',#15083,.T.);
#9293=FACE_OUTER_BOUND('',#15084,.T.);
#9294=FACE_OUTER_BOUND('',#15085,.T.);
#9295=FACE_OUTER_BOUND('',#15086,.T.);
#9296=FACE_OUTER_BOUND('',#15087,.T.);
#9297=FACE_OUTER_BOUND('',#15088,.T.);
#9298=FACE_OUTER_BOUND('',#15089,.T.);
#9299=FACE_OUTER_BOUND('',#15090,.T.);
#9300=FACE_OUTER_BOUND('',#15091,.T.);
#9301=FACE_OUTER_BOUND('',#15092,.T.);
#9302=FACE_OUTER_BOUND('',#15093,.T.);
#9303=FACE_OUTER_BOUND('',#15094,.T.);
#9304=FACE_OUTER_BOUND('',#15095,.T.);
#9305=FACE_OUTER_BOUND('',#15096,.T.);
#9306=FACE_OUTER_BOUND('',#15097,.T.);
#9307=FACE_OUTER_BOUND('',#15098,.T.);
#9308=FACE_OUTER_BOUND('',#15099,.T.);
#9309=FACE_OUTER_BOUND('',#15100,.T.);
#9310=FACE_OUTER_BOUND('',#15101,.T.);
#9311=FACE_OUTER_BOUND('',#15102,.T.);
#9312=FACE_OUTER_BOUND('',#15103,.T.);
#9313=FACE_OUTER_BOUND('',#15104,.T.);
#9314=FACE_OUTER_BOUND('',#15105,.T.);
#9315=FACE_OUTER_BOUND('',#15106,.T.);
#9316=FACE_OUTER_BOUND('',#15107,.T.);
#9317=FACE_OUTER_BOUND('',#15108,.T.);
#9318=FACE_OUTER_BOUND('',#15109,.T.);
#9319=FACE_OUTER_BOUND('',#15110,.T.);
#9320=FACE_OUTER_BOUND('',#15111,.T.);
#9321=FACE_OUTER_BOUND('',#15112,.T.);
#9322=FACE_OUTER_BOUND('',#15113,.T.);
#9323=FACE_OUTER_BOUND('',#15114,.T.);
#9324=FACE_OUTER_BOUND('',#15115,.T.);
#9325=FACE_OUTER_BOUND('',#15116,.T.);
#9326=FACE_OUTER_BOUND('',#15117,.T.);
#9327=FACE_OUTER_BOUND('',#15118,.T.);
#9328=FACE_OUTER_BOUND('',#15119,.T.);
#9329=FACE_OUTER_BOUND('',#15120,.T.);
#9330=FACE_OUTER_BOUND('',#15121,.T.);
#9331=FACE_OUTER_BOUND('',#15122,.T.);
#9332=FACE_OUTER_BOUND('',#15123,.T.);
#9333=FACE_OUTER_BOUND('',#15124,.T.);
#9334=FACE_OUTER_BOUND('',#15125,.T.);
#9335=FACE_OUTER_BOUND('',#15126,.T.);
#9336=FACE_OUTER_BOUND('',#15127,.T.);
#9337=FACE_OUTER_BOUND('',#15128,.T.);
#9338=FACE_OUTER_BOUND('',#15129,.T.);
#9339=FACE_OUTER_BOUND('',#15130,.T.);
#9340=FACE_OUTER_BOUND('',#15131,.T.);
#9341=FACE_OUTER_BOUND('',#15132,.T.);
#9342=FACE_OUTER_BOUND('',#15133,.T.);
#9343=FACE_OUTER_BOUND('',#15134,.T.);
#9344=FACE_OUTER_BOUND('',#15135,.T.);
#9345=FACE_OUTER_BOUND('',#15136,.T.);
#9346=FACE_OUTER_BOUND('',#15137,.T.);
#9347=FACE_OUTER_BOUND('',#15138,.T.);
#9348=FACE_OUTER_BOUND('',#15139,.T.);
#9349=FACE_OUTER_BOUND('',#15140,.T.);
#9350=FACE_OUTER_BOUND('',#15141,.T.);
#9351=FACE_OUTER_BOUND('',#15142,.T.);
#9352=FACE_OUTER_BOUND('',#15143,.T.);
#9353=FACE_OUTER_BOUND('',#15144,.T.);
#9354=FACE_OUTER_BOUND('',#15145,.T.);
#9355=FACE_OUTER_BOUND('',#15146,.T.);
#9356=FACE_OUTER_BOUND('',#15147,.T.);
#9357=FACE_OUTER_BOUND('',#15148,.T.);
#9358=FACE_OUTER_BOUND('',#15149,.T.);
#9359=FACE_OUTER_BOUND('',#15150,.T.);
#9360=FACE_OUTER_BOUND('',#15151,.T.);
#9361=FACE_OUTER_BOUND('',#15152,.T.);
#9362=FACE_OUTER_BOUND('',#15153,.T.);
#9363=FACE_OUTER_BOUND('',#15154,.T.);
#9364=FACE_OUTER_BOUND('',#15155,.T.);
#9365=FACE_OUTER_BOUND('',#15156,.T.);
#9366=FACE_OUTER_BOUND('',#15157,.T.);
#9367=FACE_OUTER_BOUND('',#15158,.T.);
#9368=FACE_OUTER_BOUND('',#15159,.T.);
#9369=FACE_OUTER_BOUND('',#15160,.T.);
#9370=FACE_OUTER_BOUND('',#15161,.T.);
#9371=FACE_OUTER_BOUND('',#15162,.T.);
#9372=FACE_OUTER_BOUND('',#15163,.T.);
#9373=FACE_OUTER_BOUND('',#15164,.T.);
#9374=FACE_OUTER_BOUND('',#15165,.T.);
#9375=FACE_OUTER_BOUND('',#15166,.T.);
#9376=FACE_OUTER_BOUND('',#15167,.T.);
#9377=FACE_OUTER_BOUND('',#15168,.T.);
#9378=FACE_OUTER_BOUND('',#15169,.T.);
#9379=FACE_OUTER_BOUND('',#15170,.T.);
#9380=FACE_OUTER_BOUND('',#15171,.T.);
#9381=FACE_OUTER_BOUND('',#15172,.T.);
#9382=FACE_OUTER_BOUND('',#15173,.T.);
#9383=FACE_OUTER_BOUND('',#15174,.T.);
#9384=FACE_OUTER_BOUND('',#15175,.T.);
#9385=FACE_OUTER_BOUND('',#15176,.T.);
#9386=FACE_OUTER_BOUND('',#15177,.T.);
#9387=FACE_OUTER_BOUND('',#15178,.T.);
#9388=FACE_OUTER_BOUND('',#15179,.T.);
#9389=FACE_OUTER_BOUND('',#15180,.T.);
#9390=FACE_OUTER_BOUND('',#15181,.T.);
#9391=FACE_OUTER_BOUND('',#15182,.T.);
#9392=FACE_OUTER_BOUND('',#15183,.T.);
#9393=FACE_OUTER_BOUND('',#15184,.T.);
#9394=FACE_OUTER_BOUND('',#15185,.T.);
#9395=FACE_OUTER_BOUND('',#15186,.T.);
#9396=FACE_OUTER_BOUND('',#15187,.T.);
#9397=FACE_OUTER_BOUND('',#15188,.T.);
#9398=FACE_OUTER_BOUND('',#15189,.T.);
#9399=FACE_OUTER_BOUND('',#15190,.T.);
#9400=FACE_OUTER_BOUND('',#15191,.T.);
#9401=FACE_OUTER_BOUND('',#15192,.T.);
#9402=FACE_OUTER_BOUND('',#15193,.T.);
#9403=FACE_OUTER_BOUND('',#15194,.T.);
#9404=FACE_OUTER_BOUND('',#15195,.T.);
#9405=FACE_OUTER_BOUND('',#15196,.T.);
#9406=FACE_OUTER_BOUND('',#15197,.T.);
#9407=FACE_OUTER_BOUND('',#15198,.T.);
#9408=FACE_OUTER_BOUND('',#15199,.T.);
#9409=FACE_OUTER_BOUND('',#15200,.T.);
#9410=FACE_OUTER_BOUND('',#15201,.T.);
#9411=FACE_OUTER_BOUND('',#15202,.T.);
#9412=FACE_OUTER_BOUND('',#15203,.T.);
#9413=FACE_OUTER_BOUND('',#15204,.T.);
#9414=FACE_OUTER_BOUND('',#15205,.T.);
#9415=FACE_OUTER_BOUND('',#15206,.T.);
#9416=FACE_OUTER_BOUND('',#15207,.T.);
#9417=FACE_OUTER_BOUND('',#15208,.T.);
#9418=FACE_OUTER_BOUND('',#15209,.T.);
#9419=FACE_OUTER_BOUND('',#15210,.T.);
#9420=FACE_OUTER_BOUND('',#15211,.T.);
#9421=FACE_OUTER_BOUND('',#15212,.T.);
#9422=FACE_OUTER_BOUND('',#15213,.T.);
#9423=FACE_OUTER_BOUND('',#15214,.T.);
#9424=FACE_OUTER_BOUND('',#15215,.T.);
#9425=FACE_OUTER_BOUND('',#15216,.T.);
#9426=FACE_OUTER_BOUND('',#15217,.T.);
#9427=FACE_OUTER_BOUND('',#15218,.T.);
#9428=FACE_OUTER_BOUND('',#15219,.T.);
#9429=FACE_OUTER_BOUND('',#15220,.T.);
#9430=FACE_OUTER_BOUND('',#15221,.T.);
#9431=FACE_OUTER_BOUND('',#15222,.T.);
#9432=FACE_OUTER_BOUND('',#15223,.T.);
#9433=FACE_OUTER_BOUND('',#15224,.T.);
#9434=FACE_OUTER_BOUND('',#15225,.T.);
#9435=FACE_OUTER_BOUND('',#15226,.T.);
#9436=FACE_OUTER_BOUND('',#15227,.T.);
#9437=FACE_OUTER_BOUND('',#15228,.T.);
#9438=FACE_OUTER_BOUND('',#15229,.T.);
#9439=FACE_OUTER_BOUND('',#15230,.T.);
#9440=FACE_OUTER_BOUND('',#15231,.T.);
#9441=FACE_OUTER_BOUND('',#15232,.T.);
#9442=FACE_OUTER_BOUND('',#15233,.T.);
#9443=FACE_OUTER_BOUND('',#15234,.T.);
#9444=FACE_OUTER_BOUND('',#15235,.T.);
#9445=FACE_OUTER_BOUND('',#15236,.T.);
#9446=FACE_OUTER_BOUND('',#15237,.T.);
#9447=FACE_OUTER_BOUND('',#15238,.T.);
#9448=FACE_OUTER_BOUND('',#15239,.T.);
#9449=FACE_OUTER_BOUND('',#15240,.T.);
#9450=FACE_OUTER_BOUND('',#15241,.T.);
#9451=FACE_OUTER_BOUND('',#15242,.T.);
#9452=FACE_OUTER_BOUND('',#15243,.T.);
#9453=FACE_OUTER_BOUND('',#15244,.T.);
#9454=FACE_OUTER_BOUND('',#15245,.T.);
#9455=FACE_OUTER_BOUND('',#15246,.T.);
#9456=FACE_OUTER_BOUND('',#15247,.T.);
#9457=FACE_OUTER_BOUND('',#15248,.T.);
#9458=FACE_OUTER_BOUND('',#15249,.T.);
#9459=FACE_OUTER_BOUND('',#15250,.T.);
#9460=FACE_OUTER_BOUND('',#15251,.T.);
#9461=FACE_OUTER_BOUND('',#15252,.T.);
#9462=FACE_OUTER_BOUND('',#15253,.T.);
#9463=FACE_OUTER_BOUND('',#15254,.T.);
#9464=FACE_OUTER_BOUND('',#15255,.T.);
#9465=FACE_OUTER_BOUND('',#15256,.T.);
#9466=FACE_OUTER_BOUND('',#15257,.T.);
#9467=FACE_OUTER_BOUND('',#15258,.T.);
#9468=FACE_OUTER_BOUND('',#15259,.T.);
#9469=FACE_OUTER_BOUND('',#15260,.T.);
#9470=FACE_OUTER_BOUND('',#15261,.T.);
#9471=FACE_OUTER_BOUND('',#15262,.T.);
#9472=FACE_OUTER_BOUND('',#15263,.T.);
#9473=FACE_OUTER_BOUND('',#15264,.T.);
#9474=FACE_OUTER_BOUND('',#15265,.T.);
#9475=FACE_OUTER_BOUND('',#15266,.T.);
#9476=FACE_OUTER_BOUND('',#15267,.T.);
#9477=FACE_OUTER_BOUND('',#15268,.T.);
#9478=FACE_OUTER_BOUND('',#15269,.T.);
#9479=FACE_OUTER_BOUND('',#15270,.T.);
#9480=FACE_OUTER_BOUND('',#15271,.T.);
#9481=FACE_OUTER_BOUND('',#15272,.T.);
#9482=FACE_OUTER_BOUND('',#15273,.T.);
#9483=FACE_OUTER_BOUND('',#15274,.T.);
#9484=FACE_OUTER_BOUND('',#15275,.T.);
#9485=FACE_OUTER_BOUND('',#15276,.T.);
#9486=FACE_OUTER_BOUND('',#15277,.T.);
#9487=FACE_OUTER_BOUND('',#15278,.T.);
#9488=FACE_OUTER_BOUND('',#15279,.T.);
#9489=FACE_OUTER_BOUND('',#15280,.T.);
#9490=FACE_OUTER_BOUND('',#15281,.T.);
#9491=FACE_OUTER_BOUND('',#15282,.T.);
#9492=FACE_OUTER_BOUND('',#15283,.T.);
#9493=FACE_OUTER_BOUND('',#15284,.T.);
#9494=FACE_OUTER_BOUND('',#15285,.T.);
#9495=FACE_OUTER_BOUND('',#15286,.T.);
#9496=FACE_OUTER_BOUND('',#15287,.T.);
#9497=FACE_OUTER_BOUND('',#15288,.T.);
#9498=FACE_OUTER_BOUND('',#15289,.T.);
#9499=FACE_OUTER_BOUND('',#15290,.T.);
#9500=FACE_OUTER_BOUND('',#15291,.T.);
#9501=FACE_OUTER_BOUND('',#15292,.T.);
#9502=FACE_OUTER_BOUND('',#15293,.T.);
#9503=FACE_OUTER_BOUND('',#15294,.T.);
#9504=FACE_OUTER_BOUND('',#15295,.T.);
#9505=FACE_OUTER_BOUND('',#15296,.T.);
#9506=FACE_OUTER_BOUND('',#15297,.T.);
#9507=FACE_OUTER_BOUND('',#15298,.T.);
#9508=FACE_OUTER_BOUND('',#15299,.T.);
#9509=FACE_OUTER_BOUND('',#15300,.T.);
#9510=FACE_OUTER_BOUND('',#15301,.T.);
#9511=FACE_OUTER_BOUND('',#15302,.T.);
#9512=FACE_OUTER_BOUND('',#15303,.T.);
#9513=FACE_OUTER_BOUND('',#15304,.T.);
#9514=FACE_OUTER_BOUND('',#15305,.T.);
#9515=FACE_OUTER_BOUND('',#15306,.T.);
#9516=FACE_OUTER_BOUND('',#15307,.T.);
#9517=FACE_OUTER_BOUND('',#15308,.T.);
#9518=FACE_OUTER_BOUND('',#15309,.T.);
#9519=FACE_OUTER_BOUND('',#15310,.T.);
#9520=FACE_OUTER_BOUND('',#15311,.T.);
#9521=FACE_OUTER_BOUND('',#15312,.T.);
#9522=FACE_OUTER_BOUND('',#15313,.T.);
#9523=FACE_OUTER_BOUND('',#15314,.T.);
#9524=FACE_OUTER_BOUND('',#15315,.T.);
#9525=FACE_OUTER_BOUND('',#15316,.T.);
#9526=FACE_OUTER_BOUND('',#15317,.T.);
#9527=FACE_OUTER_BOUND('',#15318,.T.);
#9528=FACE_OUTER_BOUND('',#15319,.T.);
#9529=FACE_OUTER_BOUND('',#15320,.T.);
#9530=FACE_OUTER_BOUND('',#15321,.T.);
#9531=FACE_OUTER_BOUND('',#15322,.T.);
#9532=FACE_OUTER_BOUND('',#15323,.T.);
#9533=FACE_OUTER_BOUND('',#15324,.T.);
#9534=FACE_OUTER_BOUND('',#15325,.T.);
#9535=FACE_OUTER_BOUND('',#15326,.T.);
#9536=FACE_OUTER_BOUND('',#15327,.T.);
#9537=FACE_OUTER_BOUND('',#15328,.T.);
#9538=FACE_OUTER_BOUND('',#15329,.T.);
#9539=FACE_OUTER_BOUND('',#15330,.T.);
#9540=FACE_OUTER_BOUND('',#15331,.T.);
#9541=FACE_OUTER_BOUND('',#15332,.T.);
#9542=FACE_OUTER_BOUND('',#15333,.T.);
#9543=FACE_OUTER_BOUND('',#15334,.T.);
#9544=FACE_OUTER_BOUND('',#15335,.T.);
#9545=FACE_OUTER_BOUND('',#15336,.T.);
#9546=FACE_OUTER_BOUND('',#15337,.T.);
#9547=FACE_OUTER_BOUND('',#15338,.T.);
#9548=FACE_OUTER_BOUND('',#15339,.T.);
#9549=FACE_OUTER_BOUND('',#15340,.T.);
#9550=FACE_OUTER_BOUND('',#15341,.T.);
#9551=FACE_OUTER_BOUND('',#15342,.T.);
#9552=FACE_OUTER_BOUND('',#15343,.T.);
#9553=FACE_OUTER_BOUND('',#15344,.T.);
#9554=FACE_OUTER_BOUND('',#15345,.T.);
#9555=FACE_OUTER_BOUND('',#15346,.T.);
#9556=FACE_OUTER_BOUND('',#15347,.T.);
#9557=FACE_OUTER_BOUND('',#15348,.T.);
#9558=FACE_OUTER_BOUND('',#15349,.T.);
#9559=FACE_OUTER_BOUND('',#15350,.T.);
#9560=FACE_OUTER_BOUND('',#15351,.T.);
#9561=FACE_OUTER_BOUND('',#15352,.T.);
#9562=FACE_OUTER_BOUND('',#15353,.T.);
#9563=FACE_OUTER_BOUND('',#15354,.T.);
#9564=FACE_OUTER_BOUND('',#15355,.T.);
#9565=FACE_OUTER_BOUND('',#15356,.T.);
#9566=FACE_OUTER_BOUND('',#15357,.T.);
#9567=FACE_OUTER_BOUND('',#15358,.T.);
#9568=FACE_OUTER_BOUND('',#15359,.T.);
#9569=FACE_OUTER_BOUND('',#15360,.T.);
#9570=FACE_OUTER_BOUND('',#15361,.T.);
#9571=FACE_OUTER_BOUND('',#15362,.T.);
#9572=FACE_OUTER_BOUND('',#15363,.T.);
#9573=FACE_OUTER_BOUND('',#15364,.T.);
#9574=FACE_OUTER_BOUND('',#15365,.T.);
#9575=FACE_OUTER_BOUND('',#15366,.T.);
#9576=FACE_OUTER_BOUND('',#15367,.T.);
#9577=FACE_OUTER_BOUND('',#15368,.T.);
#9578=FACE_OUTER_BOUND('',#15369,.T.);
#9579=FACE_OUTER_BOUND('',#15370,.T.);
#9580=FACE_OUTER_BOUND('',#15371,.T.);
#9581=FACE_OUTER_BOUND('',#15372,.T.);
#9582=FACE_OUTER_BOUND('',#15373,.T.);
#9583=FACE_OUTER_BOUND('',#15374,.T.);
#9584=FACE_OUTER_BOUND('',#15375,.T.);
#9585=FACE_OUTER_BOUND('',#15376,.T.);
#9586=FACE_OUTER_BOUND('',#15377,.T.);
#9587=FACE_OUTER_BOUND('',#15378,.T.);
#9588=FACE_OUTER_BOUND('',#15379,.T.);
#9589=FACE_OUTER_BOUND('',#15380,.T.);
#9590=FACE_OUTER_BOUND('',#15381,.T.);
#9591=FACE_OUTER_BOUND('',#15382,.T.);
#9592=FACE_OUTER_BOUND('',#15383,.T.);
#9593=FACE_OUTER_BOUND('',#15384,.T.);
#9594=FACE_OUTER_BOUND('',#15385,.T.);
#9595=FACE_OUTER_BOUND('',#15386,.T.);
#9596=FACE_OUTER_BOUND('',#15387,.T.);
#9597=FACE_OUTER_BOUND('',#15388,.T.);
#9598=FACE_OUTER_BOUND('',#15389,.T.);
#9599=FACE_OUTER_BOUND('',#15390,.T.);
#9600=FACE_OUTER_BOUND('',#15391,.T.);
#9601=FACE_OUTER_BOUND('',#15392,.T.);
#9602=FACE_OUTER_BOUND('',#15393,.T.);
#9603=FACE_OUTER_BOUND('',#15394,.T.);
#9604=FACE_OUTER_BOUND('',#15395,.T.);
#9605=FACE_OUTER_BOUND('',#15396,.T.);
#9606=FACE_OUTER_BOUND('',#15397,.T.);
#9607=FACE_OUTER_BOUND('',#15398,.T.);
#9608=FACE_OUTER_BOUND('',#15399,.T.);
#9609=FACE_OUTER_BOUND('',#15400,.T.);
#9610=FACE_OUTER_BOUND('',#15401,.T.);
#9611=FACE_OUTER_BOUND('',#15402,.T.);
#9612=FACE_OUTER_BOUND('',#15403,.T.);
#9613=FACE_OUTER_BOUND('',#15404,.T.);
#9614=FACE_OUTER_BOUND('',#15405,.T.);
#9615=FACE_OUTER_BOUND('',#15406,.T.);
#9616=FACE_OUTER_BOUND('',#15407,.T.);
#9617=FACE_OUTER_BOUND('',#15408,.T.);
#9618=FACE_OUTER_BOUND('',#15409,.T.);
#9619=FACE_OUTER_BOUND('',#15410,.T.);
#9620=FACE_OUTER_BOUND('',#15411,.T.);
#9621=FACE_OUTER_BOUND('',#15412,.T.);
#9622=FACE_OUTER_BOUND('',#15413,.T.);
#9623=FACE_OUTER_BOUND('',#15414,.T.);
#9624=FACE_OUTER_BOUND('',#15415,.T.);
#9625=FACE_OUTER_BOUND('',#15416,.T.);
#9626=FACE_OUTER_BOUND('',#15417,.T.);
#9627=FACE_OUTER_BOUND('',#15418,.T.);
#9628=FACE_OUTER_BOUND('',#15419,.T.);
#9629=FACE_OUTER_BOUND('',#15420,.T.);
#9630=FACE_OUTER_BOUND('',#15421,.T.);
#9631=FACE_OUTER_BOUND('',#15422,.T.);
#9632=FACE_OUTER_BOUND('',#15423,.T.);
#9633=FACE_OUTER_BOUND('',#15424,.T.);
#9634=FACE_OUTER_BOUND('',#15425,.T.);
#9635=FACE_OUTER_BOUND('',#15426,.T.);
#9636=FACE_OUTER_BOUND('',#15427,.T.);
#9637=FACE_OUTER_BOUND('',#15428,.T.);
#9638=FACE_OUTER_BOUND('',#15429,.T.);
#9639=FACE_OUTER_BOUND('',#15430,.T.);
#9640=FACE_OUTER_BOUND('',#15431,.T.);
#9641=FACE_OUTER_BOUND('',#15432,.T.);
#9642=FACE_OUTER_BOUND('',#15433,.T.);
#9643=FACE_OUTER_BOUND('',#15434,.T.);
#9644=FACE_OUTER_BOUND('',#15435,.T.);
#9645=FACE_OUTER_BOUND('',#15436,.T.);
#9646=FACE_OUTER_BOUND('',#15437,.T.);
#9647=FACE_OUTER_BOUND('',#15438,.T.);
#9648=FACE_OUTER_BOUND('',#15439,.T.);
#9649=FACE_OUTER_BOUND('',#15440,.T.);
#9650=FACE_OUTER_BOUND('',#15441,.T.);
#9651=FACE_OUTER_BOUND('',#15442,.T.);
#9652=FACE_OUTER_BOUND('',#15443,.T.);
#9653=FACE_OUTER_BOUND('',#15444,.T.);
#9654=FACE_OUTER_BOUND('',#15445,.T.);
#9655=FACE_OUTER_BOUND('',#15446,.T.);
#9656=FACE_OUTER_BOUND('',#15447,.T.);
#9657=FACE_OUTER_BOUND('',#15448,.T.);
#9658=FACE_OUTER_BOUND('',#15449,.T.);
#9659=FACE_OUTER_BOUND('',#15450,.T.);
#9660=FACE_OUTER_BOUND('',#15451,.T.);
#9661=FACE_OUTER_BOUND('',#15452,.T.);
#9662=FACE_OUTER_BOUND('',#15453,.T.);
#9663=FACE_OUTER_BOUND('',#15454,.T.);
#9664=FACE_OUTER_BOUND('',#15455,.T.);
#9665=FACE_OUTER_BOUND('',#15456,.T.);
#9666=FACE_OUTER_BOUND('',#15457,.T.);
#9667=FACE_OUTER_BOUND('',#15458,.T.);
#9668=FACE_OUTER_BOUND('',#15459,.T.);
#9669=FACE_OUTER_BOUND('',#15460,.T.);
#9670=FACE_OUTER_BOUND('',#15461,.T.);
#9671=FACE_OUTER_BOUND('',#15462,.T.);
#9672=FACE_OUTER_BOUND('',#15463,.T.);
#9673=FACE_OUTER_BOUND('',#15464,.T.);
#9674=FACE_OUTER_BOUND('',#15465,.T.);
#9675=FACE_OUTER_BOUND('',#15466,.T.);
#9676=FACE_OUTER_BOUND('',#15467,.T.);
#9677=FACE_OUTER_BOUND('',#15468,.T.);
#9678=FACE_OUTER_BOUND('',#15469,.T.);
#9679=FACE_OUTER_BOUND('',#15470,.T.);
#9680=FACE_OUTER_BOUND('',#15471,.T.);
#9681=FACE_OUTER_BOUND('',#15472,.T.);
#9682=FACE_OUTER_BOUND('',#15473,.T.);
#9683=FACE_OUTER_BOUND('',#15474,.T.);
#9684=FACE_OUTER_BOUND('',#15475,.T.);
#9685=FACE_OUTER_BOUND('',#15476,.T.);
#9686=FACE_OUTER_BOUND('',#15477,.T.);
#9687=FACE_OUTER_BOUND('',#15478,.T.);
#9688=FACE_OUTER_BOUND('',#15479,.T.);
#9689=FACE_OUTER_BOUND('',#15480,.T.);
#9690=FACE_OUTER_BOUND('',#15481,.T.);
#9691=FACE_OUTER_BOUND('',#15482,.T.);
#9692=FACE_OUTER_BOUND('',#15483,.T.);
#9693=FACE_OUTER_BOUND('',#15484,.T.);
#9694=FACE_OUTER_BOUND('',#15485,.T.);
#9695=FACE_OUTER_BOUND('',#15486,.T.);
#9696=FACE_OUTER_BOUND('',#15487,.T.);
#9697=FACE_OUTER_BOUND('',#15488,.T.);
#9698=FACE_OUTER_BOUND('',#15489,.T.);
#9699=FACE_OUTER_BOUND('',#15490,.T.);
#9700=FACE_OUTER_BOUND('',#15491,.T.);
#9701=FACE_OUTER_BOUND('',#15492,.T.);
#9702=FACE_OUTER_BOUND('',#15493,.T.);
#9703=FACE_OUTER_BOUND('',#15494,.T.);
#9704=FACE_OUTER_BOUND('',#15495,.T.);
#9705=FACE_OUTER_BOUND('',#15496,.T.);
#9706=FACE_OUTER_BOUND('',#15497,.T.);
#9707=FACE_OUTER_BOUND('',#15498,.T.);
#9708=FACE_OUTER_BOUND('',#15499,.T.);
#9709=FACE_OUTER_BOUND('',#15500,.T.);
#9710=FACE_OUTER_BOUND('',#15501,.T.);
#9711=FACE_OUTER_BOUND('',#15502,.T.);
#9712=FACE_OUTER_BOUND('',#15503,.T.);
#9713=FACE_OUTER_BOUND('',#15504,.T.);
#9714=FACE_OUTER_BOUND('',#15505,.T.);
#9715=FACE_OUTER_BOUND('',#15506,.T.);
#9716=FACE_OUTER_BOUND('',#15507,.T.);
#9717=FACE_OUTER_BOUND('',#15508,.T.);
#9718=FACE_OUTER_BOUND('',#15509,.T.);
#9719=FACE_OUTER_BOUND('',#15510,.T.);
#9720=FACE_OUTER_BOUND('',#15511,.T.);
#9721=FACE_OUTER_BOUND('',#15512,.T.);
#9722=FACE_OUTER_BOUND('',#15513,.T.);
#9723=FACE_OUTER_BOUND('',#15514,.T.);
#9724=FACE_OUTER_BOUND('',#15515,.T.);
#9725=FACE_OUTER_BOUND('',#15516,.T.);
#9726=FACE_OUTER_BOUND('',#15517,.T.);
#9727=FACE_OUTER_BOUND('',#15518,.T.);
#9728=FACE_OUTER_BOUND('',#15519,.T.);
#9729=FACE_OUTER_BOUND('',#15520,.T.);
#9730=FACE_OUTER_BOUND('',#15521,.T.);
#9731=FACE_OUTER_BOUND('',#15522,.T.);
#9732=FACE_OUTER_BOUND('',#15523,.T.);
#9733=FACE_OUTER_BOUND('',#15524,.T.);
#9734=FACE_OUTER_BOUND('',#15525,.T.);
#9735=FACE_OUTER_BOUND('',#15526,.T.);
#9736=FACE_OUTER_BOUND('',#15527,.T.);
#9737=FACE_OUTER_BOUND('',#15528,.T.);
#9738=FACE_OUTER_BOUND('',#15529,.T.);
#9739=FACE_OUTER_BOUND('',#15530,.T.);
#9740=FACE_OUTER_BOUND('',#15531,.T.);
#9741=FACE_OUTER_BOUND('',#15532,.T.);
#9742=FACE_OUTER_BOUND('',#15533,.T.);
#9743=FACE_OUTER_BOUND('',#15534,.T.);
#9744=FACE_OUTER_BOUND('',#15535,.T.);
#9745=FACE_OUTER_BOUND('',#15536,.T.);
#9746=FACE_OUTER_BOUND('',#15537,.T.);
#9747=FACE_OUTER_BOUND('',#15538,.T.);
#9748=FACE_OUTER_BOUND('',#15539,.T.);
#9749=FACE_OUTER_BOUND('',#15540,.T.);
#9750=FACE_OUTER_BOUND('',#15541,.T.);
#9751=FACE_OUTER_BOUND('',#15542,.T.);
#9752=FACE_OUTER_BOUND('',#15543,.T.);
#9753=FACE_OUTER_BOUND('',#15544,.T.);
#9754=FACE_OUTER_BOUND('',#15545,.T.);
#9755=FACE_OUTER_BOUND('',#15546,.T.);
#9756=FACE_OUTER_BOUND('',#15547,.T.);
#9757=FACE_OUTER_BOUND('',#15548,.T.);
#9758=FACE_OUTER_BOUND('',#15549,.T.);
#9759=FACE_OUTER_BOUND('',#15550,.T.);
#9760=FACE_OUTER_BOUND('',#15551,.T.);
#9761=FACE_OUTER_BOUND('',#15552,.T.);
#9762=FACE_OUTER_BOUND('',#15553,.T.);
#9763=FACE_OUTER_BOUND('',#15554,.T.);
#9764=FACE_OUTER_BOUND('',#15555,.T.);
#9765=FACE_OUTER_BOUND('',#15556,.T.);
#9766=FACE_OUTER_BOUND('',#15557,.T.);
#9767=FACE_OUTER_BOUND('',#15558,.T.);
#9768=FACE_OUTER_BOUND('',#15559,.T.);
#9769=FACE_OUTER_BOUND('',#15560,.T.);
#9770=FACE_OUTER_BOUND('',#15561,.T.);
#9771=FACE_OUTER_BOUND('',#15562,.T.);
#9772=FACE_OUTER_BOUND('',#15563,.T.);
#9773=FACE_OUTER_BOUND('',#15564,.T.);
#9774=FACE_OUTER_BOUND('',#15565,.T.);
#9775=FACE_OUTER_BOUND('',#15566,.T.);
#9776=FACE_OUTER_BOUND('',#15567,.T.);
#9777=FACE_OUTER_BOUND('',#15568,.T.);
#9778=FACE_OUTER_BOUND('',#15569,.T.);
#9779=FACE_OUTER_BOUND('',#15570,.T.);
#9780=FACE_OUTER_BOUND('',#15571,.T.);
#9781=FACE_OUTER_BOUND('',#15572,.T.);
#9782=FACE_OUTER_BOUND('',#15573,.T.);
#9783=FACE_OUTER_BOUND('',#15574,.T.);
#9784=FACE_OUTER_BOUND('',#15575,.T.);
#9785=FACE_OUTER_BOUND('',#15576,.T.);
#9786=FACE_OUTER_BOUND('',#15577,.T.);
#9787=FACE_OUTER_BOUND('',#15578,.T.);
#9788=FACE_OUTER_BOUND('',#15579,.T.);
#9789=FACE_OUTER_BOUND('',#15580,.T.);
#9790=FACE_OUTER_BOUND('',#15581,.T.);
#9791=FACE_OUTER_BOUND('',#15582,.T.);
#9792=FACE_OUTER_BOUND('',#15583,.T.);
#9793=FACE_OUTER_BOUND('',#15584,.T.);
#9794=FACE_OUTER_BOUND('',#15585,.T.);
#9795=FACE_OUTER_BOUND('',#15586,.T.);
#9796=FACE_OUTER_BOUND('',#15587,.T.);
#9797=FACE_OUTER_BOUND('',#15588,.T.);
#9798=FACE_OUTER_BOUND('',#15589,.T.);
#9799=FACE_OUTER_BOUND('',#15590,.T.);
#9800=FACE_OUTER_BOUND('',#15591,.T.);
#9801=FACE_OUTER_BOUND('',#15592,.T.);
#9802=FACE_OUTER_BOUND('',#15593,.T.);
#9803=FACE_OUTER_BOUND('',#15594,.T.);
#9804=FACE_OUTER_BOUND('',#15595,.T.);
#9805=FACE_OUTER_BOUND('',#15596,.T.);
#9806=FACE_OUTER_BOUND('',#15597,.T.);
#9807=FACE_OUTER_BOUND('',#15598,.T.);
#9808=FACE_OUTER_BOUND('',#15599,.T.);
#9809=FACE_OUTER_BOUND('',#15600,.T.);
#9810=FACE_OUTER_BOUND('',#15601,.T.);
#9811=FACE_OUTER_BOUND('',#15602,.T.);
#9812=FACE_OUTER_BOUND('',#15603,.T.);
#9813=FACE_OUTER_BOUND('',#15604,.T.);
#9814=FACE_OUTER_BOUND('',#15605,.T.);
#9815=FACE_OUTER_BOUND('',#15606,.T.);
#9816=FACE_OUTER_BOUND('',#15607,.T.);
#9817=FACE_OUTER_BOUND('',#15608,.T.);
#9818=FACE_OUTER_BOUND('',#15609,.T.);
#9819=FACE_OUTER_BOUND('',#15610,.T.);
#9820=FACE_OUTER_BOUND('',#15611,.T.);
#9821=FACE_OUTER_BOUND('',#15612,.T.);
#9822=FACE_OUTER_BOUND('',#15613,.T.);
#9823=FACE_OUTER_BOUND('',#15614,.T.);
#9824=FACE_OUTER_BOUND('',#15615,.T.);
#9825=FACE_OUTER_BOUND('',#15616,.T.);
#9826=FACE_OUTER_BOUND('',#15617,.T.);
#9827=FACE_OUTER_BOUND('',#15618,.T.);
#9828=FACE_OUTER_BOUND('',#15619,.T.);
#9829=FACE_OUTER_BOUND('',#15620,.T.);
#9830=FACE_OUTER_BOUND('',#15621,.T.);
#9831=FACE_OUTER_BOUND('',#15622,.T.);
#9832=FACE_OUTER_BOUND('',#15623,.T.);
#9833=FACE_OUTER_BOUND('',#15624,.T.);
#9834=FACE_OUTER_BOUND('',#15625,.T.);
#9835=FACE_OUTER_BOUND('',#15626,.T.);
#9836=FACE_OUTER_BOUND('',#15627,.T.);
#9837=FACE_OUTER_BOUND('',#15628,.T.);
#9838=FACE_OUTER_BOUND('',#15629,.T.);
#9839=FACE_OUTER_BOUND('',#15630,.T.);
#9840=FACE_OUTER_BOUND('',#15631,.T.);
#9841=FACE_OUTER_BOUND('',#15632,.T.);
#9842=FACE_OUTER_BOUND('',#15633,.T.);
#9843=FACE_OUTER_BOUND('',#15634,.T.);
#9844=FACE_OUTER_BOUND('',#15635,.T.);
#9845=FACE_OUTER_BOUND('',#15636,.T.);
#9846=FACE_OUTER_BOUND('',#15637,.T.);
#9847=FACE_OUTER_BOUND('',#15638,.T.);
#9848=FACE_OUTER_BOUND('',#15639,.T.);
#9849=FACE_OUTER_BOUND('',#15640,.T.);
#9850=FACE_OUTER_BOUND('',#15641,.T.);
#9851=FACE_OUTER_BOUND('',#15642,.T.);
#9852=FACE_OUTER_BOUND('',#15643,.T.);
#9853=FACE_OUTER_BOUND('',#15644,.T.);
#9854=FACE_OUTER_BOUND('',#15645,.T.);
#9855=FACE_OUTER_BOUND('',#15646,.T.);
#9856=FACE_OUTER_BOUND('',#15647,.T.);
#9857=FACE_OUTER_BOUND('',#15648,.T.);
#9858=FACE_OUTER_BOUND('',#15649,.T.);
#9859=FACE_OUTER_BOUND('',#15650,.T.);
#9860=FACE_OUTER_BOUND('',#15651,.T.);
#9861=FACE_OUTER_BOUND('',#15652,.T.);
#9862=FACE_OUTER_BOUND('',#15653,.T.);
#9863=FACE_OUTER_BOUND('',#15654,.T.);
#9864=FACE_OUTER_BOUND('',#15655,.T.);
#9865=FACE_OUTER_BOUND('',#15656,.T.);
#9866=FACE_OUTER_BOUND('',#15657,.T.);
#9867=FACE_OUTER_BOUND('',#15658,.T.);
#9868=FACE_OUTER_BOUND('',#15659,.T.);
#9869=FACE_OUTER_BOUND('',#15660,.T.);
#9870=FACE_OUTER_BOUND('',#15661,.T.);
#9871=FACE_OUTER_BOUND('',#15662,.T.);
#9872=FACE_OUTER_BOUND('',#15663,.T.);
#9873=FACE_OUTER_BOUND('',#15664,.T.);
#9874=FACE_OUTER_BOUND('',#15665,.T.);
#9875=FACE_OUTER_BOUND('',#15666,.T.);
#9876=FACE_OUTER_BOUND('',#15667,.T.);
#9877=FACE_OUTER_BOUND('',#15668,.T.);
#9878=FACE_OUTER_BOUND('',#15669,.T.);
#9879=FACE_OUTER_BOUND('',#15670,.T.);
#9880=FACE_OUTER_BOUND('',#15671,.T.);
#9881=FACE_OUTER_BOUND('',#15672,.T.);
#9882=FACE_OUTER_BOUND('',#15673,.T.);
#9883=FACE_OUTER_BOUND('',#15674,.T.);
#9884=FACE_OUTER_BOUND('',#15675,.T.);
#9885=FACE_OUTER_BOUND('',#15676,.T.);
#9886=FACE_OUTER_BOUND('',#15677,.T.);
#9887=FACE_OUTER_BOUND('',#15678,.T.);
#9888=FACE_OUTER_BOUND('',#15679,.T.);
#9889=FACE_OUTER_BOUND('',#15680,.T.);
#9890=FACE_OUTER_BOUND('',#15681,.T.);
#9891=FACE_OUTER_BOUND('',#15682,.T.);
#9892=FACE_OUTER_BOUND('',#15683,.T.);
#9893=FACE_OUTER_BOUND('',#15684,.T.);
#9894=FACE_OUTER_BOUND('',#15685,.T.);
#9895=FACE_OUTER_BOUND('',#15686,.T.);
#9896=FACE_OUTER_BOUND('',#15687,.T.);
#9897=FACE_OUTER_BOUND('',#15688,.T.);
#9898=FACE_OUTER_BOUND('',#15689,.T.);
#9899=FACE_OUTER_BOUND('',#15690,.T.);
#9900=FACE_OUTER_BOUND('',#15691,.T.);
#9901=FACE_OUTER_BOUND('',#15692,.T.);
#9902=FACE_OUTER_BOUND('',#15693,.T.);
#9903=FACE_OUTER_BOUND('',#15694,.T.);
#9904=FACE_OUTER_BOUND('',#15695,.T.);
#9905=FACE_OUTER_BOUND('',#15696,.T.);
#9906=FACE_OUTER_BOUND('',#15697,.T.);
#9907=FACE_OUTER_BOUND('',#15698,.T.);
#9908=FACE_OUTER_BOUND('',#15699,.T.);
#9909=FACE_OUTER_BOUND('',#15700,.T.);
#9910=FACE_OUTER_BOUND('',#15701,.T.);
#9911=FACE_OUTER_BOUND('',#15702,.T.);
#9912=FACE_OUTER_BOUND('',#15703,.T.);
#9913=FACE_OUTER_BOUND('',#15704,.T.);
#9914=FACE_OUTER_BOUND('',#15705,.T.);
#9915=FACE_OUTER_BOUND('',#15706,.T.);
#9916=FACE_OUTER_BOUND('',#15707,.T.);
#9917=FACE_OUTER_BOUND('',#15708,.T.);
#9918=FACE_OUTER_BOUND('',#15709,.T.);
#9919=FACE_OUTER_BOUND('',#15710,.T.);
#9920=FACE_OUTER_BOUND('',#15711,.T.);
#9921=FACE_OUTER_BOUND('',#15712,.T.);
#9922=FACE_OUTER_BOUND('',#15713,.T.);
#9923=FACE_OUTER_BOUND('',#15714,.T.);
#9924=FACE_OUTER_BOUND('',#15715,.T.);
#9925=FACE_OUTER_BOUND('',#15716,.T.);
#9926=FACE_OUTER_BOUND('',#15717,.T.);
#9927=FACE_OUTER_BOUND('',#15718,.T.);
#9928=FACE_OUTER_BOUND('',#15719,.T.);
#9929=FACE_OUTER_BOUND('',#15720,.T.);
#9930=FACE_OUTER_BOUND('',#15721,.T.);
#9931=FACE_OUTER_BOUND('',#15722,.T.);
#9932=FACE_OUTER_BOUND('',#15723,.T.);
#9933=FACE_OUTER_BOUND('',#15724,.T.);
#9934=FACE_OUTER_BOUND('',#15725,.T.);
#9935=FACE_OUTER_BOUND('',#15726,.T.);
#9936=FACE_OUTER_BOUND('',#15727,.T.);
#9937=FACE_OUTER_BOUND('',#15728,.T.);
#9938=FACE_OUTER_BOUND('',#15729,.T.);
#9939=FACE_OUTER_BOUND('',#15730,.T.);
#9940=FACE_OUTER_BOUND('',#15731,.T.);
#9941=FACE_OUTER_BOUND('',#15732,.T.);
#9942=FACE_OUTER_BOUND('',#15733,.T.);
#9943=FACE_OUTER_BOUND('',#15734,.T.);
#9944=FACE_OUTER_BOUND('',#15735,.T.);
#9945=FACE_OUTER_BOUND('',#15736,.T.);
#9946=FACE_OUTER_BOUND('',#15737,.T.);
#9947=FACE_OUTER_BOUND('',#15738,.T.);
#9948=FACE_OUTER_BOUND('',#15739,.T.);
#9949=FACE_OUTER_BOUND('',#15740,.T.);
#9950=FACE_OUTER_BOUND('',#15741,.T.);
#9951=FACE_OUTER_BOUND('',#15742,.T.);
#9952=FACE_OUTER_BOUND('',#15743,.T.);
#9953=FACE_OUTER_BOUND('',#15744,.T.);
#9954=FACE_OUTER_BOUND('',#15745,.T.);
#9955=FACE_OUTER_BOUND('',#15746,.T.);
#9956=FACE_OUTER_BOUND('',#15747,.T.);
#9957=FACE_OUTER_BOUND('',#15748,.T.);
#9958=FACE_OUTER_BOUND('',#15749,.T.);
#9959=FACE_OUTER_BOUND('',#15750,.T.);
#9960=FACE_OUTER_BOUND('',#15751,.T.);
#9961=FACE_OUTER_BOUND('',#15752,.T.);
#9962=FACE_OUTER_BOUND('',#15753,.T.);
#9963=FACE_OUTER_BOUND('',#15754,.T.);
#9964=FACE_OUTER_BOUND('',#15755,.T.);
#9965=FACE_OUTER_BOUND('',#15756,.T.);
#9966=FACE_OUTER_BOUND('',#15757,.T.);
#9967=FACE_OUTER_BOUND('',#15758,.T.);
#9968=FACE_OUTER_BOUND('',#15759,.T.);
#9969=FACE_OUTER_BOUND('',#15760,.T.);
#9970=FACE_OUTER_BOUND('',#15761,.T.);
#9971=FACE_OUTER_BOUND('',#15762,.T.);
#9972=FACE_OUTER_BOUND('',#15763,.T.);
#9973=FACE_OUTER_BOUND('',#15764,.T.);
#9974=FACE_OUTER_BOUND('',#15765,.T.);
#9975=FACE_OUTER_BOUND('',#15766,.T.);
#9976=FACE_OUTER_BOUND('',#15767,.T.);
#9977=FACE_OUTER_BOUND('',#15768,.T.);
#9978=FACE_OUTER_BOUND('',#15769,.T.);
#9979=FACE_OUTER_BOUND('',#15770,.T.);
#9980=FACE_OUTER_BOUND('',#15771,.T.);
#9981=FACE_OUTER_BOUND('',#15772,.T.);
#9982=FACE_OUTER_BOUND('',#15773,.T.);
#9983=FACE_OUTER_BOUND('',#15774,.T.);
#9984=FACE_OUTER_BOUND('',#15775,.T.);
#9985=FACE_OUTER_BOUND('',#15776,.T.);
#9986=FACE_OUTER_BOUND('',#15777,.T.);
#9987=FACE_OUTER_BOUND('',#15778,.T.);
#9988=FACE_OUTER_BOUND('',#15779,.T.);
#9989=FACE_OUTER_BOUND('',#15780,.T.);
#9990=FACE_OUTER_BOUND('',#15781,.T.);
#9991=FACE_OUTER_BOUND('',#15782,.T.);
#9992=FACE_OUTER_BOUND('',#15783,.T.);
#9993=FACE_OUTER_BOUND('',#15784,.T.);
#9994=FACE_OUTER_BOUND('',#15785,.T.);
#9995=FACE_OUTER_BOUND('',#15786,.T.);
#9996=FACE_OUTER_BOUND('',#15787,.T.);
#9997=FACE_OUTER_BOUND('',#15788,.T.);
#9998=FACE_OUTER_BOUND('',#15789,.T.);
#9999=FACE_OUTER_BOUND('',#15790,.T.);
#10000=FACE_OUTER_BOUND('',#15791,.T.);
#10001=FACE_OUTER_BOUND('',#15792,.T.);
#10002=FACE_OUTER_BOUND('',#15793,.T.);
#10003=FACE_OUTER_BOUND('',#15794,.T.);
#10004=FACE_OUTER_BOUND('',#15795,.T.);
#10005=FACE_OUTER_BOUND('',#15796,.T.);
#10006=FACE_OUTER_BOUND('',#15797,.T.);
#10007=FACE_OUTER_BOUND('',#15798,.T.);
#10008=FACE_OUTER_BOUND('',#15799,.T.);
#10009=FACE_OUTER_BOUND('',#15800,.T.);
#10010=FACE_OUTER_BOUND('',#15801,.T.);
#10011=FACE_OUTER_BOUND('',#15802,.T.);
#10012=FACE_OUTER_BOUND('',#15803,.T.);
#10013=FACE_OUTER_BOUND('',#15804,.T.);
#10014=FACE_OUTER_BOUND('',#15805,.T.);
#10015=FACE_OUTER_BOUND('',#15806,.T.);
#10016=FACE_OUTER_BOUND('',#15807,.T.);
#10017=FACE_OUTER_BOUND('',#15808,.T.);
#10018=FACE_OUTER_BOUND('',#15809,.T.);
#10019=FACE_OUTER_BOUND('',#15810,.T.);
#10020=FACE_OUTER_BOUND('',#15811,.T.);
#10021=FACE_OUTER_BOUND('',#15812,.T.);
#10022=FACE_OUTER_BOUND('',#15813,.T.);
#10023=FACE_OUTER_BOUND('',#15814,.T.);
#10024=FACE_OUTER_BOUND('',#15815,.T.);
#10025=FACE_OUTER_BOUND('',#15816,.T.);
#10026=FACE_OUTER_BOUND('',#15817,.T.);
#10027=FACE_OUTER_BOUND('',#15818,.T.);
#10028=FACE_OUTER_BOUND('',#15819,.T.);
#10029=FACE_OUTER_BOUND('',#15820,.T.);
#10030=FACE_OUTER_BOUND('',#15821,.T.);
#10031=FACE_OUTER_BOUND('',#15822,.T.);
#10032=FACE_OUTER_BOUND('',#15823,.T.);
#10033=FACE_OUTER_BOUND('',#15824,.T.);
#10034=FACE_OUTER_BOUND('',#15825,.T.);
#10035=FACE_OUTER_BOUND('',#15826,.T.);
#10036=FACE_OUTER_BOUND('',#15827,.T.);
#10037=FACE_OUTER_BOUND('',#15828,.T.);
#10038=FACE_OUTER_BOUND('',#15829,.T.);
#10039=FACE_OUTER_BOUND('',#15830,.T.);
#10040=FACE_OUTER_BOUND('',#15831,.T.);
#10041=FACE_OUTER_BOUND('',#15832,.T.);
#10042=FACE_OUTER_BOUND('',#15833,.T.);
#10043=FACE_OUTER_BOUND('',#15834,.T.);
#10044=FACE_OUTER_BOUND('',#15835,.T.);
#10045=FACE_OUTER_BOUND('',#15836,.T.);
#10046=FACE_OUTER_BOUND('',#15837,.T.);
#10047=FACE_OUTER_BOUND('',#15838,.T.);
#10048=FACE_OUTER_BOUND('',#15839,.T.);
#10049=FACE_OUTER_BOUND('',#15840,.T.);
#10050=FACE_OUTER_BOUND('',#15841,.T.);
#10051=FACE_OUTER_BOUND('',#15842,.T.);
#10052=FACE_OUTER_BOUND('',#15843,.T.);
#10053=FACE_OUTER_BOUND('',#15844,.T.);
#10054=FACE_OUTER_BOUND('',#15845,.T.);
#10055=FACE_OUTER_BOUND('',#15846,.T.);
#10056=FACE_OUTER_BOUND('',#15847,.T.);
#10057=FACE_OUTER_BOUND('',#15848,.T.);
#10058=FACE_OUTER_BOUND('',#15849,.T.);
#10059=FACE_OUTER_BOUND('',#15850,.T.);
#10060=FACE_OUTER_BOUND('',#15851,.T.);
#10061=FACE_OUTER_BOUND('',#15852,.T.);
#10062=FACE_OUTER_BOUND('',#15853,.T.);
#10063=FACE_OUTER_BOUND('',#15854,.T.);
#10064=FACE_OUTER_BOUND('',#15855,.T.);
#10065=FACE_OUTER_BOUND('',#15856,.T.);
#10066=FACE_OUTER_BOUND('',#15857,.T.);
#10067=FACE_OUTER_BOUND('',#15858,.T.);
#10068=FACE_OUTER_BOUND('',#15859,.T.);
#10069=FACE_OUTER_BOUND('',#15860,.T.);
#10070=FACE_OUTER_BOUND('',#15861,.T.);
#10071=FACE_OUTER_BOUND('',#15862,.T.);
#10072=FACE_OUTER_BOUND('',#15863,.T.);
#10073=FACE_OUTER_BOUND('',#15864,.T.);
#10074=FACE_OUTER_BOUND('',#15865,.T.);
#10075=FACE_OUTER_BOUND('',#15866,.T.);
#10076=FACE_OUTER_BOUND('',#15867,.T.);
#10077=FACE_OUTER_BOUND('',#15868,.T.);
#10078=FACE_OUTER_BOUND('',#15869,.T.);
#10079=FACE_OUTER_BOUND('',#15870,.T.);
#10080=FACE_OUTER_BOUND('',#15871,.T.);
#10081=FACE_OUTER_BOUND('',#15872,.T.);
#10082=FACE_OUTER_BOUND('',#15873,.T.);
#10083=FACE_OUTER_BOUND('',#15874,.T.);
#10084=FACE_OUTER_BOUND('',#15875,.T.);
#10085=FACE_OUTER_BOUND('',#15876,.T.);
#10086=FACE_OUTER_BOUND('',#15877,.T.);
#10087=FACE_OUTER_BOUND('',#15878,.T.);
#10088=FACE_OUTER_BOUND('',#15879,.T.);
#10089=FACE_OUTER_BOUND('',#15880,.T.);
#10090=FACE_OUTER_BOUND('',#15881,.T.);
#10091=FACE_OUTER_BOUND('',#15882,.T.);
#10092=FACE_OUTER_BOUND('',#15883,.T.);
#10093=FACE_OUTER_BOUND('',#15884,.T.);
#10094=FACE_OUTER_BOUND('',#15885,.T.);
#10095=FACE_OUTER_BOUND('',#15886,.T.);
#10096=FACE_OUTER_BOUND('',#15887,.T.);
#10097=FACE_OUTER_BOUND('',#15888,.T.);
#10098=FACE_OUTER_BOUND('',#15889,.T.);
#10099=FACE_OUTER_BOUND('',#15890,.T.);
#10100=FACE_OUTER_BOUND('',#15891,.T.);
#10101=FACE_OUTER_BOUND('',#15892,.T.);
#10102=FACE_OUTER_BOUND('',#15893,.T.);
#10103=FACE_OUTER_BOUND('',#15894,.T.);
#10104=FACE_OUTER_BOUND('',#15895,.T.);
#10105=FACE_OUTER_BOUND('',#15896,.T.);
#10106=FACE_OUTER_BOUND('',#15897,.T.);
#10107=FACE_OUTER_BOUND('',#15898,.T.);
#10108=FACE_OUTER_BOUND('',#15899,.T.);
#10109=FACE_OUTER_BOUND('',#15900,.T.);
#10110=FACE_OUTER_BOUND('',#15901,.T.);
#10111=FACE_OUTER_BOUND('',#15902,.T.);
#10112=FACE_OUTER_BOUND('',#15903,.T.);
#10113=FACE_OUTER_BOUND('',#15904,.T.);
#10114=FACE_OUTER_BOUND('',#15905,.T.);
#10115=FACE_OUTER_BOUND('',#15906,.T.);
#10116=FACE_OUTER_BOUND('',#15907,.T.);
#10117=FACE_OUTER_BOUND('',#15908,.T.);
#10118=FACE_OUTER_BOUND('',#15909,.T.);
#10119=FACE_OUTER_BOUND('',#15910,.T.);
#10120=FACE_OUTER_BOUND('',#15911,.T.);
#10121=FACE_OUTER_BOUND('',#15912,.T.);
#10122=FACE_OUTER_BOUND('',#15913,.T.);
#10123=FACE_OUTER_BOUND('',#15914,.T.);
#10124=FACE_OUTER_BOUND('',#15915,.T.);
#10125=FACE_OUTER_BOUND('',#15916,.T.);
#10126=FACE_OUTER_BOUND('',#15917,.T.);
#10127=FACE_OUTER_BOUND('',#15918,.T.);
#10128=FACE_OUTER_BOUND('',#15919,.T.);
#10129=FACE_OUTER_BOUND('',#15920,.T.);
#10130=FACE_OUTER_BOUND('',#15921,.T.);
#10131=FACE_OUTER_BOUND('',#15922,.T.);
#10132=FACE_OUTER_BOUND('',#15923,.T.);
#10133=FACE_OUTER_BOUND('',#15924,.T.);
#10134=FACE_OUTER_BOUND('',#15925,.T.);
#10135=FACE_OUTER_BOUND('',#15926,.T.);
#10136=FACE_OUTER_BOUND('',#15927,.T.);
#10137=FACE_OUTER_BOUND('',#15928,.T.);
#10138=FACE_OUTER_BOUND('',#15929,.T.);
#10139=FACE_OUTER_BOUND('',#15930,.T.);
#10140=FACE_OUTER_BOUND('',#15931,.T.);
#10141=FACE_OUTER_BOUND('',#15932,.T.);
#10142=FACE_OUTER_BOUND('',#15933,.T.);
#10143=FACE_OUTER_BOUND('',#15934,.T.);
#10144=FACE_OUTER_BOUND('',#15935,.T.);
#10145=FACE_OUTER_BOUND('',#15936,.T.);
#10146=FACE_OUTER_BOUND('',#15937,.T.);
#10147=FACE_OUTER_BOUND('',#15938,.T.);
#10148=FACE_OUTER_BOUND('',#15939,.T.);
#10149=FACE_OUTER_BOUND('',#15940,.T.);
#10150=FACE_OUTER_BOUND('',#15941,.T.);
#10151=FACE_OUTER_BOUND('',#15942,.T.);
#10152=FACE_OUTER_BOUND('',#15943,.T.);
#10153=FACE_OUTER_BOUND('',#15944,.T.);
#10154=FACE_OUTER_BOUND('',#15945,.T.);
#10155=FACE_OUTER_BOUND('',#15946,.T.);
#10156=FACE_OUTER_BOUND('',#15947,.T.);
#10157=FACE_OUTER_BOUND('',#15948,.T.);
#10158=FACE_OUTER_BOUND('',#15949,.T.);
#10159=FACE_OUTER_BOUND('',#15950,.T.);
#10160=FACE_OUTER_BOUND('',#15951,.T.);
#10161=FACE_OUTER_BOUND('',#15952,.T.);
#10162=FACE_OUTER_BOUND('',#15953,.T.);
#10163=FACE_OUTER_BOUND('',#15954,.T.);
#10164=FACE_OUTER_BOUND('',#15955,.T.);
#10165=FACE_OUTER_BOUND('',#15956,.T.);
#10166=FACE_OUTER_BOUND('',#15957,.T.);
#10167=FACE_OUTER_BOUND('',#15958,.T.);
#10168=FACE_OUTER_BOUND('',#15959,.T.);
#10169=FACE_OUTER_BOUND('',#15960,.T.);
#10170=FACE_OUTER_BOUND('',#15961,.T.);
#10171=FACE_OUTER_BOUND('',#15962,.T.);
#10172=FACE_OUTER_BOUND('',#15963,.T.);
#10173=FACE_OUTER_BOUND('',#15964,.T.);
#10174=FACE_OUTER_BOUND('',#15965,.T.);
#10175=FACE_OUTER_BOUND('',#15966,.T.);
#10176=FACE_OUTER_BOUND('',#15967,.T.);
#10177=FACE_OUTER_BOUND('',#15968,.T.);
#10178=FACE_OUTER_BOUND('',#15969,.T.);
#10179=FACE_OUTER_BOUND('',#15970,.T.);
#10180=FACE_OUTER_BOUND('',#15971,.T.);
#10181=FACE_OUTER_BOUND('',#15972,.T.);
#10182=FACE_OUTER_BOUND('',#15973,.T.);
#10183=FACE_OUTER_BOUND('',#15974,.T.);
#10184=FACE_OUTER_BOUND('',#15975,.T.);
#10185=FACE_OUTER_BOUND('',#15976,.T.);
#10186=FACE_OUTER_BOUND('',#15977,.T.);
#10187=FACE_OUTER_BOUND('',#15978,.T.);
#10188=FACE_OUTER_BOUND('',#15979,.T.);
#10189=FACE_OUTER_BOUND('',#15980,.T.);
#10190=FACE_OUTER_BOUND('',#15981,.T.);
#10191=FACE_OUTER_BOUND('',#15982,.T.);
#10192=FACE_OUTER_BOUND('',#15983,.T.);
#10193=FACE_OUTER_BOUND('',#15984,.T.);
#10194=FACE_OUTER_BOUND('',#15985,.T.);
#10195=FACE_OUTER_BOUND('',#15986,.T.);
#10196=FACE_OUTER_BOUND('',#15987,.T.);
#10197=FACE_OUTER_BOUND('',#15988,.T.);
#10198=FACE_OUTER_BOUND('',#15989,.T.);
#10199=FACE_OUTER_BOUND('',#15990,.T.);
#10200=FACE_OUTER_BOUND('',#15991,.T.);
#10201=FACE_OUTER_BOUND('',#15992,.T.);
#10202=FACE_OUTER_BOUND('',#15993,.T.);
#10203=FACE_OUTER_BOUND('',#15994,.T.);
#10204=FACE_OUTER_BOUND('',#15995,.T.);
#10205=FACE_OUTER_BOUND('',#15996,.T.);
#10206=FACE_OUTER_BOUND('',#15997,.T.);
#10207=FACE_OUTER_BOUND('',#15998,.T.);
#10208=FACE_OUTER_BOUND('',#15999,.T.);
#10209=FACE_OUTER_BOUND('',#16000,.T.);
#10210=FACE_OUTER_BOUND('',#16001,.T.);
#10211=FACE_OUTER_BOUND('',#16002,.T.);
#10212=FACE_OUTER_BOUND('',#16003,.T.);
#10213=FACE_OUTER_BOUND('',#16004,.T.);
#10214=FACE_OUTER_BOUND('',#16005,.T.);
#10215=FACE_OUTER_BOUND('',#16006,.T.);
#10216=FACE_OUTER_BOUND('',#16007,.T.);
#10217=FACE_OUTER_BOUND('',#16008,.T.);
#10218=FACE_OUTER_BOUND('',#16009,.T.);
#10219=FACE_OUTER_BOUND('',#16010,.T.);
#10220=FACE_OUTER_BOUND('',#16011,.T.);
#10221=FACE_OUTER_BOUND('',#16012,.T.);
#10222=FACE_OUTER_BOUND('',#16013,.T.);
#10223=FACE_OUTER_BOUND('',#16014,.T.);
#10224=FACE_OUTER_BOUND('',#16015,.T.);
#10225=FACE_OUTER_BOUND('',#16016,.T.);
#10226=FACE_OUTER_BOUND('',#16017,.T.);
#10227=FACE_OUTER_BOUND('',#16018,.T.);
#10228=FACE_OUTER_BOUND('',#16019,.T.);
#10229=FACE_OUTER_BOUND('',#16020,.T.);
#10230=FACE_OUTER_BOUND('',#16021,.T.);
#10231=FACE_OUTER_BOUND('',#16022,.T.);
#10232=FACE_OUTER_BOUND('',#16023,.T.);
#10233=FACE_OUTER_BOUND('',#16024,.T.);
#10234=FACE_OUTER_BOUND('',#16025,.T.);
#10235=FACE_OUTER_BOUND('',#16026,.T.);
#10236=FACE_OUTER_BOUND('',#16027,.T.);
#10237=FACE_OUTER_BOUND('',#16028,.T.);
#10238=FACE_OUTER_BOUND('',#16029,.T.);
#10239=FACE_OUTER_BOUND('',#16030,.T.);
#10240=FACE_OUTER_BOUND('',#16031,.T.);
#10241=FACE_OUTER_BOUND('',#16032,.T.);
#10242=FACE_OUTER_BOUND('',#16033,.T.);
#10243=FACE_OUTER_BOUND('',#16034,.T.);
#10244=FACE_OUTER_BOUND('',#16035,.T.);
#10245=FACE_OUTER_BOUND('',#16036,.T.);
#10246=FACE_OUTER_BOUND('',#16037,.T.);
#10247=FACE_OUTER_BOUND('',#16038,.T.);
#10248=FACE_OUTER_BOUND('',#16039,.T.);
#10249=FACE_OUTER_BOUND('',#16040,.T.);
#10250=FACE_OUTER_BOUND('',#16041,.T.);
#10251=FACE_OUTER_BOUND('',#16042,.T.);
#10252=FACE_OUTER_BOUND('',#16043,.T.);
#10253=FACE_OUTER_BOUND('',#16044,.T.);
#10254=FACE_OUTER_BOUND('',#16045,.T.);
#10255=FACE_OUTER_BOUND('',#16046,.T.);
#10256=FACE_OUTER_BOUND('',#16047,.T.);
#10257=FACE_OUTER_BOUND('',#16048,.T.);
#10258=FACE_OUTER_BOUND('',#16049,.T.);
#10259=FACE_OUTER_BOUND('',#16050,.T.);
#10260=FACE_OUTER_BOUND('',#16051,.T.);
#10261=FACE_OUTER_BOUND('',#16052,.T.);
#10262=FACE_OUTER_BOUND('',#16053,.T.);
#10263=FACE_OUTER_BOUND('',#16054,.T.);
#10264=FACE_OUTER_BOUND('',#16055,.T.);
#10265=FACE_OUTER_BOUND('',#16056,.T.);
#10266=FACE_OUTER_BOUND('',#16057,.T.);
#10267=FACE_OUTER_BOUND('',#16058,.T.);
#10268=FACE_OUTER_BOUND('',#16059,.T.);
#10269=FACE_OUTER_BOUND('',#16060,.T.);
#10270=FACE_OUTER_BOUND('',#16061,.T.);
#10271=FACE_OUTER_BOUND('',#16062,.T.);
#10272=FACE_OUTER_BOUND('',#16063,.T.);
#10273=FACE_OUTER_BOUND('',#16064,.T.);
#10274=FACE_OUTER_BOUND('',#16065,.T.);
#10275=FACE_OUTER_BOUND('',#16066,.T.);
#10276=FACE_OUTER_BOUND('',#16067,.T.);
#10277=FACE_OUTER_BOUND('',#16068,.T.);
#10278=FACE_OUTER_BOUND('',#16069,.T.);
#10279=FACE_OUTER_BOUND('',#16070,.T.);
#10280=FACE_OUTER_BOUND('',#16071,.T.);
#10281=FACE_OUTER_BOUND('',#16072,.T.);
#10282=FACE_OUTER_BOUND('',#16073,.T.);
#10283=FACE_OUTER_BOUND('',#16074,.T.);
#10284=FACE_OUTER_BOUND('',#16075,.T.);
#10285=FACE_OUTER_BOUND('',#16076,.T.);
#10286=FACE_OUTER_BOUND('',#16077,.T.);
#10287=FACE_OUTER_BOUND('',#16078,.T.);
#10288=FACE_OUTER_BOUND('',#16079,.T.);
#10289=FACE_OUTER_BOUND('',#16080,.T.);
#10290=FACE_OUTER_BOUND('',#16081,.T.);
#10291=FACE_OUTER_BOUND('',#16082,.T.);
#10292=FACE_OUTER_BOUND('',#16083,.T.);
#10293=FACE_OUTER_BOUND('',#16084,.T.);
#10294=FACE_OUTER_BOUND('',#16085,.T.);
#10295=FACE_OUTER_BOUND('',#16086,.T.);
#10296=FACE_OUTER_BOUND('',#16087,.T.);
#10297=FACE_OUTER_BOUND('',#16088,.T.);
#10298=FACE_OUTER_BOUND('',#16089,.T.);
#10299=FACE_OUTER_BOUND('',#16090,.T.);
#10300=FACE_OUTER_BOUND('',#16091,.T.);
#10301=FACE_OUTER_BOUND('',#16092,.T.);
#10302=FACE_OUTER_BOUND('',#16093,.T.);
#10303=FACE_OUTER_BOUND('',#16094,.T.);
#10304=FACE_OUTER_BOUND('',#16095,.T.);
#10305=FACE_OUTER_BOUND('',#16096,.T.);
#10306=FACE_OUTER_BOUND('',#16097,.T.);
#10307=FACE_OUTER_BOUND('',#16098,.T.);
#10308=FACE_OUTER_BOUND('',#16099,.T.);
#10309=FACE_OUTER_BOUND('',#16100,.T.);
#10310=FACE_OUTER_BOUND('',#16101,.T.);
#10311=FACE_OUTER_BOUND('',#16102,.T.);
#10312=FACE_OUTER_BOUND('',#16103,.T.);
#10313=FACE_OUTER_BOUND('',#16104,.T.);
#10314=FACE_OUTER_BOUND('',#16105,.T.);
#10315=FACE_OUTER_BOUND('',#16106,.T.);
#10316=FACE_OUTER_BOUND('',#16107,.T.);
#10317=FACE_OUTER_BOUND('',#16108,.T.);
#10318=FACE_OUTER_BOUND('',#16109,.T.);
#10319=FACE_OUTER_BOUND('',#16110,.T.);
#10320=FACE_OUTER_BOUND('',#16111,.T.);
#10321=FACE_OUTER_BOUND('',#16112,.T.);
#10322=FACE_OUTER_BOUND('',#16113,.T.);
#10323=FACE_OUTER_BOUND('',#16114,.T.);
#10324=FACE_OUTER_BOUND('',#16115,.T.);
#10325=FACE_OUTER_BOUND('',#16116,.T.);
#10326=FACE_OUTER_BOUND('',#16117,.T.);
#10327=FACE_OUTER_BOUND('',#16118,.T.);
#10328=FACE_OUTER_BOUND('',#16119,.T.);
#10329=FACE_OUTER_BOUND('',#16120,.T.);
#10330=FACE_OUTER_BOUND('',#16121,.T.);
#10331=FACE_OUTER_BOUND('',#16122,.T.);
#10332=FACE_OUTER_BOUND('',#16123,.T.);
#10333=FACE_OUTER_BOUND('',#16124,.T.);
#10334=FACE_OUTER_BOUND('',#16125,.T.);
#10335=FACE_OUTER_BOUND('',#16126,.T.);
#10336=FACE_OUTER_BOUND('',#16127,.T.);
#10337=FACE_OUTER_BOUND('',#16128,.T.);
#10338=FACE_OUTER_BOUND('',#16129,.T.);
#10339=FACE_OUTER_BOUND('',#16130,.T.);
#10340=FACE_OUTER_BOUND('',#16131,.T.);
#10341=FACE_OUTER_BOUND('',#16132,.T.);
#10342=FACE_OUTER_BOUND('',#16133,.T.);
#10343=FACE_OUTER_BOUND('',#16134,.T.);
#10344=FACE_OUTER_BOUND('',#16135,.T.);
#10345=FACE_OUTER_BOUND('',#16136,.T.);
#10346=FACE_OUTER_BOUND('',#16137,.T.);
#10347=FACE_OUTER_BOUND('',#16138,.T.);
#10348=FACE_OUTER_BOUND('',#16139,.T.);
#10349=FACE_OUTER_BOUND('',#16140,.T.);
#10350=FACE_OUTER_BOUND('',#16141,.T.);
#10351=FACE_OUTER_BOUND('',#16142,.T.);
#10352=FACE_OUTER_BOUND('',#16143,.T.);
#10353=FACE_OUTER_BOUND('',#16144,.T.);
#10354=FACE_OUTER_BOUND('',#16145,.T.);
#10355=FACE_OUTER_BOUND('',#16146,.T.);
#10356=FACE_OUTER_BOUND('',#16147,.T.);
#10357=FACE_OUTER_BOUND('',#16148,.T.);
#10358=FACE_OUTER_BOUND('',#16149,.T.);
#10359=FACE_OUTER_BOUND('',#16150,.T.);
#10360=FACE_OUTER_BOUND('',#16151,.T.);
#10361=FACE_OUTER_BOUND('',#16152,.T.);
#10362=FACE_OUTER_BOUND('',#16153,.T.);
#10363=FACE_OUTER_BOUND('',#16154,.T.);
#10364=FACE_OUTER_BOUND('',#16155,.T.);
#10365=FACE_OUTER_BOUND('',#16156,.T.);
#10366=FACE_OUTER_BOUND('',#16157,.T.);
#10367=FACE_OUTER_BOUND('',#16158,.T.);
#10368=FACE_OUTER_BOUND('',#16159,.T.);
#10369=FACE_OUTER_BOUND('',#16160,.T.);
#10370=FACE_OUTER_BOUND('',#16161,.T.);
#10371=FACE_OUTER_BOUND('',#16162,.T.);
#10372=FACE_OUTER_BOUND('',#16163,.T.);
#10373=FACE_OUTER_BOUND('',#16164,.T.);
#10374=FACE_OUTER_BOUND('',#16165,.T.);
#10375=FACE_OUTER_BOUND('',#16166,.T.);
#10376=FACE_OUTER_BOUND('',#16167,.T.);
#10377=FACE_OUTER_BOUND('',#16168,.T.);
#10378=FACE_OUTER_BOUND('',#16169,.T.);
#10379=FACE_OUTER_BOUND('',#16170,.T.);
#10380=FACE_OUTER_BOUND('',#16171,.T.);
#10381=FACE_OUTER_BOUND('',#16172,.T.);
#10382=FACE_OUTER_BOUND('',#16173,.T.);
#10383=FACE_OUTER_BOUND('',#16174,.T.);
#10384=FACE_OUTER_BOUND('',#16175,.T.);
#10385=FACE_OUTER_BOUND('',#16176,.T.);
#10386=FACE_OUTER_BOUND('',#16177,.T.);
#10387=FACE_OUTER_BOUND('',#16178,.T.);
#10388=FACE_OUTER_BOUND('',#16179,.T.);
#10389=FACE_OUTER_BOUND('',#16180,.T.);
#10390=FACE_OUTER_BOUND('',#16181,.T.);
#10391=FACE_OUTER_BOUND('',#16182,.T.);
#10392=FACE_OUTER_BOUND('',#16183,.T.);
#10393=FACE_OUTER_BOUND('',#16184,.T.);
#10394=FACE_OUTER_BOUND('',#16185,.T.);
#10395=FACE_OUTER_BOUND('',#16186,.T.);
#10396=FACE_OUTER_BOUND('',#16187,.T.);
#10397=FACE_OUTER_BOUND('',#16188,.T.);
#10398=FACE_OUTER_BOUND('',#16189,.T.);
#10399=FACE_OUTER_BOUND('',#16190,.T.);
#10400=FACE_OUTER_BOUND('',#16191,.T.);
#10401=FACE_OUTER_BOUND('',#16192,.T.);
#10402=FACE_OUTER_BOUND('',#16193,.T.);
#10403=FACE_OUTER_BOUND('',#16194,.T.);
#10404=FACE_OUTER_BOUND('',#16195,.T.);
#10405=FACE_OUTER_BOUND('',#16196,.T.);
#10406=FACE_OUTER_BOUND('',#16197,.T.);
#10407=FACE_OUTER_BOUND('',#16198,.T.);
#10408=FACE_OUTER_BOUND('',#16199,.T.);
#10409=FACE_OUTER_BOUND('',#16200,.T.);
#10410=FACE_OUTER_BOUND('',#16201,.T.);
#10411=FACE_OUTER_BOUND('',#16202,.T.);
#10412=FACE_OUTER_BOUND('',#16203,.T.);
#10413=FACE_OUTER_BOUND('',#16204,.T.);
#10414=FACE_OUTER_BOUND('',#16205,.T.);
#10415=FACE_OUTER_BOUND('',#16206,.T.);
#10416=FACE_OUTER_BOUND('',#16207,.T.);
#10417=FACE_OUTER_BOUND('',#16208,.T.);
#10418=FACE_OUTER_BOUND('',#16209,.T.);
#10419=FACE_OUTER_BOUND('',#16210,.T.);
#10420=FACE_OUTER_BOUND('',#16211,.T.);
#10421=FACE_OUTER_BOUND('',#16212,.T.);
#10422=FACE_OUTER_BOUND('',#16213,.T.);
#10423=FACE_OUTER_BOUND('',#16214,.T.);
#10424=FACE_OUTER_BOUND('',#16215,.T.);
#10425=FACE_OUTER_BOUND('',#16216,.T.);
#10426=FACE_OUTER_BOUND('',#16217,.T.);
#10427=FACE_OUTER_BOUND('',#16218,.T.);
#10428=FACE_OUTER_BOUND('',#16219,.T.);
#10429=FACE_OUTER_BOUND('',#16220,.T.);
#10430=FACE_OUTER_BOUND('',#16221,.T.);
#10431=FACE_OUTER_BOUND('',#16222,.T.);
#10432=FACE_OUTER_BOUND('',#16223,.T.);
#10433=FACE_OUTER_BOUND('',#16224,.T.);
#10434=FACE_OUTER_BOUND('',#16225,.T.);
#10435=FACE_OUTER_BOUND('',#16226,.T.);
#10436=FACE_OUTER_BOUND('',#16227,.T.);
#10437=FACE_OUTER_BOUND('',#16228,.T.);
#10438=FACE_OUTER_BOUND('',#16229,.T.);
#10439=FACE_OUTER_BOUND('',#16230,.T.);
#10440=FACE_OUTER_BOUND('',#16231,.T.);
#10441=FACE_OUTER_BOUND('',#16232,.T.);
#10442=FACE_OUTER_BOUND('',#16233,.T.);
#10443=FACE_OUTER_BOUND('',#16234,.T.);
#10444=FACE_OUTER_BOUND('',#16235,.T.);
#10445=FACE_OUTER_BOUND('',#16236,.T.);
#10446=FACE_OUTER_BOUND('',#16237,.T.);
#10447=FACE_OUTER_BOUND('',#16238,.T.);
#10448=FACE_OUTER_BOUND('',#16239,.T.);
#10449=FACE_OUTER_BOUND('',#16240,.T.);
#10450=FACE_OUTER_BOUND('',#16241,.T.);
#10451=FACE_OUTER_BOUND('',#16242,.T.);
#10452=FACE_OUTER_BOUND('',#16243,.T.);
#10453=FACE_OUTER_BOUND('',#16244,.T.);
#10454=FACE_OUTER_BOUND('',#16245,.T.);
#10455=FACE_OUTER_BOUND('',#16246,.T.);
#10456=FACE_OUTER_BOUND('',#16247,.T.);
#10457=FACE_OUTER_BOUND('',#16248,.T.);
#10458=FACE_OUTER_BOUND('',#16249,.T.);
#10459=FACE_OUTER_BOUND('',#16250,.T.);
#10460=FACE_OUTER_BOUND('',#16251,.T.);
#10461=FACE_OUTER_BOUND('',#16252,.T.);
#10462=FACE_OUTER_BOUND('',#16253,.T.);
#10463=FACE_OUTER_BOUND('',#16254,.T.);
#10464=FACE_OUTER_BOUND('',#16255,.T.);
#10465=FACE_OUTER_BOUND('',#16256,.T.);
#10466=FACE_OUTER_BOUND('',#16257,.T.);
#10467=FACE_OUTER_BOUND('',#16258,.T.);
#10468=FACE_OUTER_BOUND('',#16259,.T.);
#10469=FACE_OUTER_BOUND('',#16260,.T.);
#10470=FACE_OUTER_BOUND('',#16261,.T.);
#10471=FACE_OUTER_BOUND('',#16262,.T.);
#10472=FACE_OUTER_BOUND('',#16263,.T.);
#10473=FACE_OUTER_BOUND('',#16264,.T.);
#10474=FACE_OUTER_BOUND('',#16265,.T.);
#10475=FACE_OUTER_BOUND('',#16266,.T.);
#10476=FACE_OUTER_BOUND('',#16267,.T.);
#10477=FACE_OUTER_BOUND('',#16268,.T.);
#10478=FACE_OUTER_BOUND('',#16269,.T.);
#10479=FACE_OUTER_BOUND('',#16270,.T.);
#10480=FACE_OUTER_BOUND('',#16271,.T.);
#10481=FACE_OUTER_BOUND('',#16272,.T.);
#10482=FACE_OUTER_BOUND('',#16273,.T.);
#10483=FACE_OUTER_BOUND('',#16274,.T.);
#10484=FACE_OUTER_BOUND('',#16275,.T.);
#10485=FACE_OUTER_BOUND('',#16276,.T.);
#10486=FACE_OUTER_BOUND('',#16277,.T.);
#10487=FACE_OUTER_BOUND('',#16278,.T.);
#10488=FACE_OUTER_BOUND('',#16279,.T.);
#10489=FACE_OUTER_BOUND('',#16280,.T.);
#10490=FACE_OUTER_BOUND('',#16281,.T.);
#10491=FACE_OUTER_BOUND('',#16282,.T.);
#10492=FACE_OUTER_BOUND('',#16283,.T.);
#10493=FACE_OUTER_BOUND('',#16284,.T.);
#10494=FACE_OUTER_BOUND('',#16285,.T.);
#10495=FACE_OUTER_BOUND('',#16286,.T.);
#10496=FACE_OUTER_BOUND('',#16287,.T.);
#10497=FACE_OUTER_BOUND('',#16288,.T.);
#10498=FACE_OUTER_BOUND('',#16289,.T.);
#10499=FACE_OUTER_BOUND('',#16290,.T.);
#10500=FACE_OUTER_BOUND('',#16291,.T.);
#10501=FACE_OUTER_BOUND('',#16292,.T.);
#10502=FACE_OUTER_BOUND('',#16293,.T.);
#10503=FACE_OUTER_BOUND('',#16294,.T.);
#10504=FACE_OUTER_BOUND('',#16295,.T.);
#10505=FACE_OUTER_BOUND('',#16296,.T.);
#10506=FACE_OUTER_BOUND('',#16297,.T.);
#10507=FACE_OUTER_BOUND('',#16298,.T.);
#10508=FACE_OUTER_BOUND('',#16299,.T.);
#10509=FACE_OUTER_BOUND('',#16300,.T.);
#10510=FACE_OUTER_BOUND('',#16301,.T.);
#10511=FACE_OUTER_BOUND('',#16302,.T.);
#10512=FACE_OUTER_BOUND('',#16303,.T.);
#10513=FACE_OUTER_BOUND('',#16304,.T.);
#10514=FACE_OUTER_BOUND('',#16305,.T.);
#10515=FACE_OUTER_BOUND('',#16306,.T.);
#10516=FACE_OUTER_BOUND('',#16307,.T.);
#10517=FACE_OUTER_BOUND('',#16308,.T.);
#10518=FACE_OUTER_BOUND('',#16309,.T.);
#10519=FACE_OUTER_BOUND('',#16310,.T.);
#10520=FACE_OUTER_BOUND('',#16311,.T.);
#10521=FACE_OUTER_BOUND('',#16312,.T.);
#10522=FACE_OUTER_BOUND('',#16313,.T.);
#10523=FACE_OUTER_BOUND('',#16314,.T.);
#10524=FACE_OUTER_BOUND('',#16315,.T.);
#10525=FACE_OUTER_BOUND('',#16316,.T.);
#10526=FACE_OUTER_BOUND('',#16317,.T.);
#10527=FACE_OUTER_BOUND('',#16318,.T.);
#10528=FACE_OUTER_BOUND('',#16319,.T.);
#10529=FACE_OUTER_BOUND('',#16320,.T.);
#10530=FACE_OUTER_BOUND('',#16321,.T.);
#10531=FACE_OUTER_BOUND('',#16322,.T.);
#10532=FACE_OUTER_BOUND('',#16323,.T.);
#10533=FACE_OUTER_BOUND('',#16324,.T.);
#10534=FACE_OUTER_BOUND('',#16325,.T.);
#10535=FACE_OUTER_BOUND('',#16326,.T.);
#10536=FACE_OUTER_BOUND('',#16327,.T.);
#10537=FACE_OUTER_BOUND('',#16328,.T.);
#10538=FACE_OUTER_BOUND('',#16329,.T.);
#10539=FACE_OUTER_BOUND('',#16330,.T.);
#10540=FACE_OUTER_BOUND('',#16331,.T.);
#10541=FACE_OUTER_BOUND('',#16332,.T.);
#10542=FACE_OUTER_BOUND('',#16333,.T.);
#10543=FACE_OUTER_BOUND('',#16334,.T.);
#10544=FACE_OUTER_BOUND('',#16335,.T.);
#10545=FACE_OUTER_BOUND('',#16336,.T.);
#10546=FACE_OUTER_BOUND('',#16337,.T.);
#10547=FACE_OUTER_BOUND('',#16338,.T.);
#10548=FACE_OUTER_BOUND('',#16339,.T.);
#10549=FACE_OUTER_BOUND('',#16340,.T.);
#10550=FACE_OUTER_BOUND('',#16341,.T.);
#10551=FACE_OUTER_BOUND('',#16342,.T.);
#10552=FACE_OUTER_BOUND('',#16343,.T.);
#10553=FACE_OUTER_BOUND('',#16344,.T.);
#10554=FACE_OUTER_BOUND('',#16345,.T.);
#10555=FACE_OUTER_BOUND('',#16346,.T.);
#10556=FACE_OUTER_BOUND('',#16347,.T.);
#10557=FACE_OUTER_BOUND('',#16348,.T.);
#10558=FACE_OUTER_BOUND('',#16349,.T.);
#10559=FACE_OUTER_BOUND('',#16350,.T.);
#10560=FACE_OUTER_BOUND('',#16351,.T.);
#10561=FACE_OUTER_BOUND('',#16352,.T.);
#10562=FACE_OUTER_BOUND('',#16353,.T.);
#10563=FACE_OUTER_BOUND('',#16354,.T.);
#10564=FACE_OUTER_BOUND('',#16355,.T.);
#10565=FACE_OUTER_BOUND('',#16356,.T.);
#10566=FACE_OUTER_BOUND('',#16357,.T.);
#10567=FACE_OUTER_BOUND('',#16358,.T.);
#10568=FACE_OUTER_BOUND('',#16359,.T.);
#10569=FACE_OUTER_BOUND('',#16360,.T.);
#10570=FACE_OUTER_BOUND('',#16362,.T.);
#10571=FACE_OUTER_BOUND('',#16363,.T.);
#10572=FACE_OUTER_BOUND('',#16364,.T.);
#10573=FACE_OUTER_BOUND('',#16365,.T.);
#10574=FACE_OUTER_BOUND('',#16366,.T.);
#10575=FACE_OUTER_BOUND('',#16367,.T.);
#10576=FACE_OUTER_BOUND('',#16368,.T.);
#10577=FACE_OUTER_BOUND('',#16369,.T.);
#10578=FACE_OUTER_BOUND('',#16370,.T.);
#10579=FACE_OUTER_BOUND('',#16372,.T.);
#10580=FACE_OUTER_BOUND('',#16373,.T.);
#10581=FACE_OUTER_BOUND('',#16374,.T.);
#10582=FACE_OUTER_BOUND('',#16375,.T.);
#10583=FACE_OUTER_BOUND('',#16376,.T.);
#10584=FACE_OUTER_BOUND('',#16377,.T.);
#10585=FACE_OUTER_BOUND('',#16378,.T.);
#10586=FACE_OUTER_BOUND('',#16379,.T.);
#10587=FACE_OUTER_BOUND('',#16380,.T.);
#10588=FACE_OUTER_BOUND('',#16381,.T.);
#10589=FACE_OUTER_BOUND('',#16382,.T.);
#10590=FACE_OUTER_BOUND('',#16383,.T.);
#10591=FACE_OUTER_BOUND('',#16384,.T.);
#10592=FACE_OUTER_BOUND('',#16385,.T.);
#10593=FACE_OUTER_BOUND('',#16386,.T.);
#10594=FACE_OUTER_BOUND('',#16387,.T.);
#10595=FACE_OUTER_BOUND('',#16388,.T.);
#10596=FACE_OUTER_BOUND('',#16389,.T.);
#10597=FACE_OUTER_BOUND('',#16390,.T.);
#10598=FACE_OUTER_BOUND('',#16391,.T.);
#10599=FACE_OUTER_BOUND('',#16392,.T.);
#10600=FACE_OUTER_BOUND('',#16393,.T.);
#10601=FACE_OUTER_BOUND('',#16394,.T.);
#10602=FACE_OUTER_BOUND('',#16395,.T.);
#10603=FACE_OUTER_BOUND('',#16396,.T.);
#10604=FACE_OUTER_BOUND('',#16397,.T.);
#10605=FACE_OUTER_BOUND('',#16398,.T.);
#10606=FACE_OUTER_BOUND('',#16399,.T.);
#10607=FACE_OUTER_BOUND('',#16400,.T.);
#10608=FACE_OUTER_BOUND('',#16401,.T.);
#10609=FACE_OUTER_BOUND('',#16402,.T.);
#10610=FACE_OUTER_BOUND('',#16403,.T.);
#10611=FACE_OUTER_BOUND('',#16404,.T.);
#10612=FACE_OUTER_BOUND('',#16405,.T.);
#10613=FACE_OUTER_BOUND('',#16406,.T.);
#10614=FACE_OUTER_BOUND('',#16407,.T.);
#10615=FACE_OUTER_BOUND('',#16408,.T.);
#10616=FACE_OUTER_BOUND('',#16409,.T.);
#10617=FACE_OUTER_BOUND('',#16410,.T.);
#10618=FACE_OUTER_BOUND('',#16411,.T.);
#10619=FACE_OUTER_BOUND('',#16412,.T.);
#10620=FACE_OUTER_BOUND('',#16413,.T.);
#10621=FACE_OUTER_BOUND('',#16414,.T.);
#10622=FACE_OUTER_BOUND('',#16415,.T.);
#10623=FACE_OUTER_BOUND('',#16416,.T.);
#10624=FACE_OUTER_BOUND('',#16417,.T.);
#10625=FACE_OUTER_BOUND('',#16418,.T.);
#10626=FACE_OUTER_BOUND('',#16419,.T.);
#10627=FACE_OUTER_BOUND('',#16420,.T.);
#10628=FACE_OUTER_BOUND('',#16421,.T.);
#10629=FACE_OUTER_BOUND('',#16422,.T.);
#10630=FACE_OUTER_BOUND('',#16423,.T.);
#10631=FACE_OUTER_BOUND('',#16424,.T.);
#10632=FACE_OUTER_BOUND('',#16425,.T.);
#10633=FACE_OUTER_BOUND('',#16426,.T.);
#10634=FACE_OUTER_BOUND('',#16427,.T.);
#10635=FACE_OUTER_BOUND('',#16428,.T.);
#10636=FACE_OUTER_BOUND('',#16429,.T.);
#10637=FACE_OUTER_BOUND('',#16430,.T.);
#10638=FACE_OUTER_BOUND('',#16431,.T.);
#10639=FACE_OUTER_BOUND('',#16432,.T.);
#10640=FACE_OUTER_BOUND('',#16433,.T.);
#10641=FACE_OUTER_BOUND('',#16434,.T.);
#10642=FACE_OUTER_BOUND('',#16435,.T.);
#10643=FACE_OUTER_BOUND('',#16436,.T.);
#10644=FACE_OUTER_BOUND('',#16437,.T.);
#10645=FACE_OUTER_BOUND('',#16438,.T.);
#10646=FACE_OUTER_BOUND('',#16439,.T.);
#10647=FACE_OUTER_BOUND('',#16440,.T.);
#10648=FACE_OUTER_BOUND('',#16441,.T.);
#10649=FACE_OUTER_BOUND('',#16442,.T.);
#10650=FACE_OUTER_BOUND('',#16443,.T.);
#10651=FACE_OUTER_BOUND('',#16444,.T.);
#10652=FACE_OUTER_BOUND('',#16445,.T.);
#10653=FACE_OUTER_BOUND('',#16446,.T.);
#10654=FACE_OUTER_BOUND('',#16447,.T.);
#10655=FACE_OUTER_BOUND('',#16448,.T.);
#10656=FACE_OUTER_BOUND('',#16449,.T.);
#10657=FACE_OUTER_BOUND('',#16450,.T.);
#10658=FACE_OUTER_BOUND('',#16451,.T.);
#10659=FACE_OUTER_BOUND('',#16452,.T.);
#10660=FACE_OUTER_BOUND('',#16453,.T.);
#10661=FACE_OUTER_BOUND('',#16454,.T.);
#10662=FACE_OUTER_BOUND('',#16455,.T.);
#10663=FACE_OUTER_BOUND('',#16456,.T.);
#10664=FACE_OUTER_BOUND('',#16457,.T.);
#10665=FACE_OUTER_BOUND('',#16458,.T.);
#10666=FACE_OUTER_BOUND('',#16459,.T.);
#10667=FACE_OUTER_BOUND('',#16460,.T.);
#10668=FACE_OUTER_BOUND('',#16461,.T.);
#10669=FACE_OUTER_BOUND('',#16462,.T.);
#10670=FACE_OUTER_BOUND('',#16463,.T.);
#10671=FACE_OUTER_BOUND('',#16464,.T.);
#10672=FACE_OUTER_BOUND('',#16465,.T.);
#10673=FACE_OUTER_BOUND('',#16466,.T.);
#10674=FACE_OUTER_BOUND('',#16467,.T.);
#10675=FACE_OUTER_BOUND('',#16468,.T.);
#10676=FACE_OUTER_BOUND('',#16469,.T.);
#10677=FACE_OUTER_BOUND('',#16470,.T.);
#10678=FACE_OUTER_BOUND('',#16471,.T.);
#10679=FACE_OUTER_BOUND('',#16472,.T.);
#10680=FACE_OUTER_BOUND('',#16473,.T.);
#10681=FACE_OUTER_BOUND('',#16474,.T.);
#10682=FACE_OUTER_BOUND('',#16475,.T.);
#10683=FACE_OUTER_BOUND('',#16476,.T.);
#10684=FACE_OUTER_BOUND('',#16477,.T.);
#10685=FACE_OUTER_BOUND('',#16478,.T.);
#10686=FACE_OUTER_BOUND('',#16479,.T.);
#10687=FACE_OUTER_BOUND('',#16480,.T.);
#10688=FACE_OUTER_BOUND('',#16481,.T.);
#10689=FACE_OUTER_BOUND('',#16482,.T.);
#10690=FACE_OUTER_BOUND('',#16483,.T.);
#10691=FACE_OUTER_BOUND('',#16484,.T.);
#10692=FACE_OUTER_BOUND('',#16485,.T.);
#10693=FACE_OUTER_BOUND('',#16486,.T.);
#10694=FACE_OUTER_BOUND('',#16487,.T.);
#10695=FACE_OUTER_BOUND('',#16488,.T.);
#10696=FACE_OUTER_BOUND('',#16489,.T.);
#10697=FACE_OUTER_BOUND('',#16490,.T.);
#10698=FACE_OUTER_BOUND('',#16491,.T.);
#10699=FACE_OUTER_BOUND('',#16492,.T.);
#10700=FACE_OUTER_BOUND('',#16493,.T.);
#10701=FACE_OUTER_BOUND('',#16494,.T.);
#10702=FACE_OUTER_BOUND('',#16495,.T.);
#10703=FACE_OUTER_BOUND('',#16496,.T.);
#10704=FACE_OUTER_BOUND('',#16497,.T.);
#10705=FACE_OUTER_BOUND('',#16498,.T.);
#10706=FACE_OUTER_BOUND('',#16499,.T.);
#10707=FACE_OUTER_BOUND('',#16500,.T.);
#10708=FACE_OUTER_BOUND('',#16501,.T.);
#10709=FACE_OUTER_BOUND('',#16502,.T.);
#10710=FACE_OUTER_BOUND('',#16503,.T.);
#10711=FACE_OUTER_BOUND('',#16504,.T.);
#10712=FACE_OUTER_BOUND('',#16505,.T.);
#10713=FACE_OUTER_BOUND('',#16506,.T.);
#10714=FACE_OUTER_BOUND('',#16507,.T.);
#10715=FACE_OUTER_BOUND('',#16508,.T.);
#10716=FACE_OUTER_BOUND('',#16509,.T.);
#10717=FACE_OUTER_BOUND('',#16510,.T.);
#10718=FACE_OUTER_BOUND('',#16511,.T.);
#10719=FACE_OUTER_BOUND('',#16512,.T.);
#10720=FACE_OUTER_BOUND('',#16513,.T.);
#10721=FACE_OUTER_BOUND('',#16514,.T.);
#10722=FACE_OUTER_BOUND('',#16515,.T.);
#10723=FACE_OUTER_BOUND('',#16516,.T.);
#10724=FACE_OUTER_BOUND('',#16517,.T.);
#10725=FACE_OUTER_BOUND('',#16518,.T.);
#10726=FACE_OUTER_BOUND('',#16519,.T.);
#10727=FACE_OUTER_BOUND('',#16520,.T.);
#10728=FACE_OUTER_BOUND('',#16521,.T.);
#10729=FACE_OUTER_BOUND('',#16522,.T.);
#10730=FACE_OUTER_BOUND('',#16523,.T.);
#10731=FACE_OUTER_BOUND('',#16524,.T.);
#10732=FACE_OUTER_BOUND('',#16525,.T.);
#10733=FACE_OUTER_BOUND('',#16526,.T.);
#10734=FACE_OUTER_BOUND('',#16527,.T.);
#10735=FACE_OUTER_BOUND('',#16528,.T.);
#10736=FACE_OUTER_BOUND('',#16529,.T.);
#10737=FACE_OUTER_BOUND('',#16530,.T.);
#10738=FACE_OUTER_BOUND('',#16531,.T.);
#10739=FACE_OUTER_BOUND('',#16532,.T.);
#10740=FACE_OUTER_BOUND('',#16533,.T.);
#10741=FACE_OUTER_BOUND('',#16534,.T.);
#10742=FACE_OUTER_BOUND('',#16535,.T.);
#10743=FACE_OUTER_BOUND('',#16536,.T.);
#10744=FACE_OUTER_BOUND('',#16537,.T.);
#10745=FACE_OUTER_BOUND('',#16538,.T.);
#10746=FACE_OUTER_BOUND('',#16539,.T.);
#10747=FACE_OUTER_BOUND('',#16540,.T.);
#10748=FACE_OUTER_BOUND('',#16541,.T.);
#10749=FACE_OUTER_BOUND('',#16542,.T.);
#10750=FACE_OUTER_BOUND('',#16543,.T.);
#10751=FACE_OUTER_BOUND('',#16544,.T.);
#10752=FACE_OUTER_BOUND('',#16545,.T.);
#10753=FACE_OUTER_BOUND('',#16546,.T.);
#10754=FACE_OUTER_BOUND('',#16547,.T.);
#10755=FACE_OUTER_BOUND('',#16548,.T.);
#10756=FACE_OUTER_BOUND('',#16549,.T.);
#10757=FACE_OUTER_BOUND('',#16550,.T.);
#10758=FACE_OUTER_BOUND('',#16551,.T.);
#10759=FACE_OUTER_BOUND('',#16552,.T.);
#10760=FACE_OUTER_BOUND('',#16553,.T.);
#10761=FACE_OUTER_BOUND('',#16554,.T.);
#10762=FACE_OUTER_BOUND('',#16555,.T.);
#10763=FACE_OUTER_BOUND('',#16556,.T.);
#10764=FACE_OUTER_BOUND('',#16557,.T.);
#10765=FACE_OUTER_BOUND('',#16558,.T.);
#10766=FACE_OUTER_BOUND('',#16559,.T.);
#10767=FACE_OUTER_BOUND('',#16560,.T.);
#10768=FACE_OUTER_BOUND('',#16561,.T.);
#10769=FACE_OUTER_BOUND('',#16562,.T.);
#10770=FACE_OUTER_BOUND('',#16563,.T.);
#10771=FACE_OUTER_BOUND('',#16564,.T.);
#10772=FACE_OUTER_BOUND('',#16565,.T.);
#10773=FACE_OUTER_BOUND('',#16566,.T.);
#10774=FACE_OUTER_BOUND('',#16567,.T.);
#10775=FACE_OUTER_BOUND('',#16568,.T.);
#10776=FACE_OUTER_BOUND('',#16569,.T.);
#10777=FACE_OUTER_BOUND('',#16570,.T.);
#10778=FACE_OUTER_BOUND('',#16571,.T.);
#10779=FACE_OUTER_BOUND('',#16572,.T.);
#10780=FACE_OUTER_BOUND('',#16573,.T.);
#10781=FACE_OUTER_BOUND('',#16574,.T.);
#10782=FACE_OUTER_BOUND('',#16575,.T.);
#10783=FACE_OUTER_BOUND('',#16576,.T.);
#10784=FACE_OUTER_BOUND('',#16577,.T.);
#10785=FACE_OUTER_BOUND('',#16578,.T.);
#10786=FACE_OUTER_BOUND('',#16579,.T.);
#10787=FACE_OUTER_BOUND('',#16580,.T.);
#10788=FACE_OUTER_BOUND('',#16581,.T.);
#10789=FACE_OUTER_BOUND('',#16582,.T.);
#10790=FACE_OUTER_BOUND('',#16583,.T.);
#10791=FACE_OUTER_BOUND('',#16584,.T.);
#10792=FACE_OUTER_BOUND('',#16585,.T.);
#10793=FACE_OUTER_BOUND('',#16586,.T.);
#10794=FACE_OUTER_BOUND('',#16587,.T.);
#10795=FACE_OUTER_BOUND('',#16588,.T.);
#10796=FACE_OUTER_BOUND('',#16589,.T.);
#10797=FACE_OUTER_BOUND('',#16590,.T.);
#10798=FACE_OUTER_BOUND('',#16591,.T.);
#10799=FACE_OUTER_BOUND('',#16592,.T.);
#10800=FACE_OUTER_BOUND('',#16593,.T.);
#10801=FACE_OUTER_BOUND('',#16594,.T.);
#10802=FACE_OUTER_BOUND('',#16595,.T.);
#10803=FACE_OUTER_BOUND('',#16596,.T.);
#10804=FACE_OUTER_BOUND('',#16597,.T.);
#10805=FACE_OUTER_BOUND('',#16598,.T.);
#10806=FACE_OUTER_BOUND('',#16599,.T.);
#10807=FACE_OUTER_BOUND('',#16600,.T.);
#10808=FACE_OUTER_BOUND('',#16601,.T.);
#10809=FACE_OUTER_BOUND('',#16602,.T.);
#10810=FACE_OUTER_BOUND('',#16603,.T.);
#10811=FACE_OUTER_BOUND('',#16604,.T.);
#10812=FACE_OUTER_BOUND('',#16605,.T.);
#10813=FACE_OUTER_BOUND('',#16606,.T.);
#10814=FACE_OUTER_BOUND('',#16607,.T.);
#10815=FACE_OUTER_BOUND('',#16608,.T.);
#10816=FACE_OUTER_BOUND('',#16609,.T.);
#10817=FACE_OUTER_BOUND('',#16610,.T.);
#10818=FACE_OUTER_BOUND('',#16611,.T.);
#10819=FACE_OUTER_BOUND('',#16612,.T.);
#10820=FACE_OUTER_BOUND('',#16613,.T.);
#10821=FACE_OUTER_BOUND('',#16614,.T.);
#10822=FACE_OUTER_BOUND('',#16615,.T.);
#10823=FACE_OUTER_BOUND('',#16616,.T.);
#10824=FACE_OUTER_BOUND('',#16617,.T.);
#10825=FACE_OUTER_BOUND('',#16618,.T.);
#10826=FACE_OUTER_BOUND('',#16619,.T.);
#10827=FACE_OUTER_BOUND('',#16620,.T.);
#10828=FACE_OUTER_BOUND('',#16621,.T.);
#10829=FACE_OUTER_BOUND('',#16622,.T.);
#10830=FACE_OUTER_BOUND('',#16623,.T.);
#10831=FACE_OUTER_BOUND('',#16624,.T.);
#10832=FACE_OUTER_BOUND('',#16625,.T.);
#10833=FACE_OUTER_BOUND('',#16626,.T.);
#10834=FACE_OUTER_BOUND('',#16627,.T.);
#10835=FACE_OUTER_BOUND('',#16628,.T.);
#10836=FACE_OUTER_BOUND('',#16629,.T.);
#10837=FACE_OUTER_BOUND('',#16630,.T.);
#10838=FACE_OUTER_BOUND('',#16631,.T.);
#10839=FACE_OUTER_BOUND('',#16632,.T.);
#10840=FACE_OUTER_BOUND('',#16633,.T.);
#10841=FACE_OUTER_BOUND('',#16634,.T.);
#10842=FACE_OUTER_BOUND('',#16635,.T.);
#10843=FACE_OUTER_BOUND('',#16636,.T.);
#10844=FACE_OUTER_BOUND('',#16637,.T.);
#10845=FACE_OUTER_BOUND('',#16638,.T.);
#10846=FACE_OUTER_BOUND('',#16639,.T.);
#10847=FACE_OUTER_BOUND('',#16640,.T.);
#10848=FACE_OUTER_BOUND('',#16641,.T.);
#10849=FACE_OUTER_BOUND('',#16642,.T.);
#10850=FACE_OUTER_BOUND('',#16643,.T.);
#10851=FACE_OUTER_BOUND('',#16644,.T.);
#10852=FACE_OUTER_BOUND('',#16645,.T.);
#10853=FACE_OUTER_BOUND('',#16646,.T.);
#10854=FACE_OUTER_BOUND('',#16647,.T.);
#10855=FACE_OUTER_BOUND('',#16648,.T.);
#10856=FACE_OUTER_BOUND('',#16649,.T.);
#10857=FACE_OUTER_BOUND('',#16650,.T.);
#10858=FACE_OUTER_BOUND('',#16651,.T.);
#10859=FACE_OUTER_BOUND('',#16652,.T.);
#10860=FACE_OUTER_BOUND('',#16653,.T.);
#10861=FACE_OUTER_BOUND('',#16654,.T.);
#10862=FACE_OUTER_BOUND('',#16655,.T.);
#10863=FACE_OUTER_BOUND('',#16656,.T.);
#10864=FACE_OUTER_BOUND('',#16657,.T.);
#10865=FACE_OUTER_BOUND('',#16658,.T.);
#10866=FACE_OUTER_BOUND('',#16659,.T.);
#10867=FACE_OUTER_BOUND('',#16660,.T.);
#10868=FACE_OUTER_BOUND('',#16661,.T.);
#10869=FACE_OUTER_BOUND('',#16662,.T.);
#10870=FACE_OUTER_BOUND('',#16663,.T.);
#10871=FACE_OUTER_BOUND('',#16664,.T.);
#10872=FACE_OUTER_BOUND('',#16665,.T.);
#10873=FACE_OUTER_BOUND('',#16666,.T.);
#10874=FACE_OUTER_BOUND('',#16667,.T.);
#10875=FACE_OUTER_BOUND('',#16668,.T.);
#10876=FACE_OUTER_BOUND('',#16669,.T.);
#10877=FACE_OUTER_BOUND('',#16670,.T.);
#10878=FACE_OUTER_BOUND('',#16671,.T.);
#10879=FACE_OUTER_BOUND('',#16672,.T.);
#10880=FACE_OUTER_BOUND('',#16673,.T.);
#10881=FACE_OUTER_BOUND('',#16674,.T.);
#10882=FACE_OUTER_BOUND('',#16675,.T.);
#10883=FACE_OUTER_BOUND('',#16676,.T.);
#10884=FACE_OUTER_BOUND('',#16677,.T.);
#10885=FACE_OUTER_BOUND('',#16678,.T.);
#10886=FACE_OUTER_BOUND('',#16679,.T.);
#10887=FACE_OUTER_BOUND('',#16680,.T.);
#10888=FACE_OUTER_BOUND('',#16681,.T.);
#10889=FACE_OUTER_BOUND('',#16682,.T.);
#10890=FACE_OUTER_BOUND('',#16683,.T.);
#10891=FACE_OUTER_BOUND('',#16684,.T.);
#10892=FACE_OUTER_BOUND('',#16685,.T.);
#10893=FACE_OUTER_BOUND('',#16686,.T.);
#10894=FACE_OUTER_BOUND('',#16687,.T.);
#10895=FACE_OUTER_BOUND('',#16688,.T.);
#10896=FACE_OUTER_BOUND('',#16689,.T.);
#10897=FACE_OUTER_BOUND('',#16690,.T.);
#10898=FACE_OUTER_BOUND('',#16691,.T.);
#10899=FACE_OUTER_BOUND('',#16692,.T.);
#10900=FACE_OUTER_BOUND('',#16693,.T.);
#10901=FACE_OUTER_BOUND('',#16694,.T.);
#10902=FACE_OUTER_BOUND('',#16695,.T.);
#10903=FACE_OUTER_BOUND('',#16696,.T.);
#10904=FACE_OUTER_BOUND('',#16697,.T.);
#10905=FACE_OUTER_BOUND('',#16698,.T.);
#10906=FACE_OUTER_BOUND('',#16699,.T.);
#10907=FACE_OUTER_BOUND('',#16700,.T.);
#10908=FACE_OUTER_BOUND('',#16701,.T.);
#10909=FACE_OUTER_BOUND('',#16702,.T.);
#10910=FACE_OUTER_BOUND('',#16703,.T.);
#10911=FACE_OUTER_BOUND('',#16704,.T.);
#10912=FACE_OUTER_BOUND('',#16705,.T.);
#10913=FACE_OUTER_BOUND('',#16706,.T.);
#10914=FACE_OUTER_BOUND('',#16707,.T.);
#10915=FACE_OUTER_BOUND('',#16708,.T.);
#10916=FACE_OUTER_BOUND('',#16709,.T.);
#10917=FACE_OUTER_BOUND('',#16710,.T.);
#10918=FACE_OUTER_BOUND('',#16711,.T.);
#10919=FACE_OUTER_BOUND('',#16712,.T.);
#10920=FACE_OUTER_BOUND('',#16713,.T.);
#10921=FACE_OUTER_BOUND('',#16714,.T.);
#10922=FACE_OUTER_BOUND('',#16715,.T.);
#10923=FACE_OUTER_BOUND('',#16716,.T.);
#10924=FACE_OUTER_BOUND('',#16717,.T.);
#10925=FACE_OUTER_BOUND('',#16718,.T.);
#10926=FACE_OUTER_BOUND('',#16719,.T.);
#10927=FACE_OUTER_BOUND('',#16720,.T.);
#10928=FACE_OUTER_BOUND('',#16721,.T.);
#10929=FACE_OUTER_BOUND('',#16722,.T.);
#10930=FACE_OUTER_BOUND('',#16723,.T.);
#10931=FACE_OUTER_BOUND('',#16724,.T.);
#10932=FACE_OUTER_BOUND('',#16725,.T.);
#10933=FACE_OUTER_BOUND('',#16726,.T.);
#10934=FACE_OUTER_BOUND('',#16727,.T.);
#10935=FACE_OUTER_BOUND('',#16728,.T.);
#10936=FACE_OUTER_BOUND('',#16729,.T.);
#10937=FACE_OUTER_BOUND('',#16730,.T.);
#10938=FACE_OUTER_BOUND('',#16731,.T.);
#10939=FACE_OUTER_BOUND('',#16732,.T.);
#10940=FACE_OUTER_BOUND('',#16733,.T.);
#10941=FACE_OUTER_BOUND('',#16734,.T.);
#10942=FACE_OUTER_BOUND('',#16735,.T.);
#10943=FACE_OUTER_BOUND('',#16736,.T.);
#10944=FACE_OUTER_BOUND('',#16737,.T.);
#10945=FACE_OUTER_BOUND('',#16738,.T.);
#10946=FACE_OUTER_BOUND('',#16739,.T.);
#10947=FACE_OUTER_BOUND('',#16740,.T.);
#10948=FACE_OUTER_BOUND('',#16741,.T.);
#10949=FACE_OUTER_BOUND('',#16742,.T.);
#10950=FACE_OUTER_BOUND('',#16743,.T.);
#10951=FACE_OUTER_BOUND('',#16744,.T.);
#10952=FACE_OUTER_BOUND('',#16745,.T.);
#10953=FACE_OUTER_BOUND('',#16746,.T.);
#10954=FACE_OUTER_BOUND('',#16747,.T.);
#10955=FACE_OUTER_BOUND('',#16748,.T.);
#10956=FACE_OUTER_BOUND('',#16749,.T.);
#10957=FACE_OUTER_BOUND('',#16750,.T.);
#10958=FACE_OUTER_BOUND('',#16751,.T.);
#10959=FACE_OUTER_BOUND('',#16752,.T.);
#10960=FACE_OUTER_BOUND('',#16753,.T.);
#10961=FACE_OUTER_BOUND('',#16754,.T.);
#10962=FACE_OUTER_BOUND('',#16755,.T.);
#10963=FACE_OUTER_BOUND('',#16756,.T.);
#10964=FACE_OUTER_BOUND('',#16757,.T.);
#10965=FACE_OUTER_BOUND('',#16758,.T.);
#10966=FACE_OUTER_BOUND('',#16759,.T.);
#10967=FACE_OUTER_BOUND('',#16760,.T.);
#10968=FACE_OUTER_BOUND('',#16761,.T.);
#10969=FACE_OUTER_BOUND('',#16762,.T.);
#10970=FACE_OUTER_BOUND('',#16763,.T.);
#10971=FACE_OUTER_BOUND('',#16764,.T.);
#10972=FACE_OUTER_BOUND('',#16765,.T.);
#10973=FACE_OUTER_BOUND('',#16766,.T.);
#10974=FACE_OUTER_BOUND('',#16767,.T.);
#10975=FACE_OUTER_BOUND('',#16768,.T.);
#10976=FACE_OUTER_BOUND('',#16769,.T.);
#10977=FACE_OUTER_BOUND('',#16770,.T.);
#10978=FACE_OUTER_BOUND('',#16771,.T.);
#10979=FACE_OUTER_BOUND('',#16772,.T.);
#10980=FACE_OUTER_BOUND('',#16773,.T.);
#10981=FACE_OUTER_BOUND('',#16774,.T.);
#10982=FACE_OUTER_BOUND('',#16775,.T.);
#10983=FACE_OUTER_BOUND('',#16776,.T.);
#10984=FACE_OUTER_BOUND('',#16777,.T.);
#10985=FACE_OUTER_BOUND('',#16778,.T.);
#10986=FACE_OUTER_BOUND('',#16779,.T.);
#10987=FACE_OUTER_BOUND('',#16780,.T.);
#10988=FACE_OUTER_BOUND('',#16781,.T.);
#10989=FACE_OUTER_BOUND('',#16782,.T.);
#10990=FACE_OUTER_BOUND('',#16783,.T.);
#10991=FACE_OUTER_BOUND('',#16784,.T.);
#10992=FACE_OUTER_BOUND('',#16785,.T.);
#10993=FACE_OUTER_BOUND('',#16786,.T.);
#10994=FACE_OUTER_BOUND('',#16787,.T.);
#10995=FACE_OUTER_BOUND('',#16788,.T.);
#10996=FACE_OUTER_BOUND('',#16789,.T.);
#10997=FACE_OUTER_BOUND('',#16790,.T.);
#10998=FACE_OUTER_BOUND('',#16791,.T.);
#10999=FACE_OUTER_BOUND('',#16792,.T.);
#11000=FACE_OUTER_BOUND('',#16793,.T.);
#11001=FACE_OUTER_BOUND('',#16794,.T.);
#11002=FACE_OUTER_BOUND('',#16799,.T.);
#11003=FACE_OUTER_BOUND('',#16800,.T.);
#11004=FACE_OUTER_BOUND('',#16801,.T.);
#11005=FACE_OUTER_BOUND('',#16802,.T.);
#11006=FACE_OUTER_BOUND('',#16803,.T.);
#11007=FACE_OUTER_BOUND('',#16804,.T.);
#11008=FACE_OUTER_BOUND('',#16805,.T.);
#11009=FACE_OUTER_BOUND('',#16806,.T.);
#11010=FACE_OUTER_BOUND('',#16807,.T.);
#11011=FACE_OUTER_BOUND('',#16808,.T.);
#11012=FACE_OUTER_BOUND('',#16809,.T.);
#11013=FACE_OUTER_BOUND('',#16810,.T.);
#11014=FACE_OUTER_BOUND('',#16815,.T.);
#11015=FACE_OUTER_BOUND('',#16816,.T.);
#11016=FACE_OUTER_BOUND('',#16817,.T.);
#11017=FACE_OUTER_BOUND('',#16818,.T.);
#11018=FACE_OUTER_BOUND('',#16819,.T.);
#11019=FACE_OUTER_BOUND('',#16820,.T.);
#11020=FACE_OUTER_BOUND('',#16821,.T.);
#11021=FACE_OUTER_BOUND('',#16822,.T.);
#11022=FACE_OUTER_BOUND('',#16823,.T.);
#11023=FACE_OUTER_BOUND('',#16824,.T.);
#11024=FACE_OUTER_BOUND('',#16825,.T.);
#11025=FACE_OUTER_BOUND('',#16826,.T.);
#11026=FACE_OUTER_BOUND('',#16827,.T.);
#11027=FACE_OUTER_BOUND('',#16828,.T.);
#11028=FACE_OUTER_BOUND('',#16829,.T.);
#11029=FACE_OUTER_BOUND('',#16830,.T.);
#11030=FACE_OUTER_BOUND('',#16832,.T.);
#11031=FACE_OUTER_BOUND('',#16833,.T.);
#11032=FACE_OUTER_BOUND('',#16834,.T.);
#11033=FACE_OUTER_BOUND('',#16835,.T.);
#11034=FACE_OUTER_BOUND('',#16836,.T.);
#11035=FACE_OUTER_BOUND('',#16838,.T.);
#11036=FACE_OUTER_BOUND('',#16839,.T.);
#11037=FACE_OUTER_BOUND('',#16840,.T.);
#11038=FACE_OUTER_BOUND('',#16841,.T.);
#11039=FACE_OUTER_BOUND('',#16842,.T.);
#11040=FACE_OUTER_BOUND('',#16843,.T.);
#11041=FACE_OUTER_BOUND('',#16844,.T.);
#11042=FACE_OUTER_BOUND('',#16845,.T.);
#11043=FACE_OUTER_BOUND('',#16846,.T.);
#11044=FACE_OUTER_BOUND('',#16847,.T.);
#11045=FACE_OUTER_BOUND('',#16848,.T.);
#11046=FACE_OUTER_BOUND('',#16849,.T.);
#11047=FACE_OUTER_BOUND('',#16850,.T.);
#11048=FACE_OUTER_BOUND('',#16851,.T.);
#11049=FACE_OUTER_BOUND('',#16852,.T.);
#11050=FACE_OUTER_BOUND('',#16853,.T.);
#11051=FACE_OUTER_BOUND('',#16854,.T.);
#11052=FACE_OUTER_BOUND('',#16855,.T.);
#11053=FACE_OUTER_BOUND('',#16856,.T.);
#11054=FACE_OUTER_BOUND('',#16857,.T.);
#11055=FACE_OUTER_BOUND('',#16858,.T.);
#11056=FACE_OUTER_BOUND('',#16859,.T.);
#11057=FACE_OUTER_BOUND('',#16860,.T.);
#11058=FACE_OUTER_BOUND('',#16861,.T.);
#11059=FACE_OUTER_BOUND('',#16862,.T.);
#11060=FACE_OUTER_BOUND('',#16863,.T.);
#11061=FACE_OUTER_BOUND('',#16864,.T.);
#11062=FACE_OUTER_BOUND('',#16865,.T.);
#11063=FACE_OUTER_BOUND('',#16866,.T.);
#11064=FACE_OUTER_BOUND('',#16867,.T.);
#11065=FACE_OUTER_BOUND('',#16868,.T.);
#11066=FACE_OUTER_BOUND('',#16869,.T.);
#11067=FACE_OUTER_BOUND('',#16870,.T.);
#11068=FACE_OUTER_BOUND('',#16871,.T.);
#11069=FACE_OUTER_BOUND('',#16872,.T.);
#11070=FACE_OUTER_BOUND('',#16873,.T.);
#11071=FACE_OUTER_BOUND('',#16874,.T.);
#11072=FACE_OUTER_BOUND('',#16875,.T.);
#11073=FACE_OUTER_BOUND('',#16876,.T.);
#11074=FACE_OUTER_BOUND('',#16877,.T.);
#11075=FACE_OUTER_BOUND('',#16878,.T.);
#11076=FACE_OUTER_BOUND('',#16879,.T.);
#11077=FACE_OUTER_BOUND('',#16880,.T.);
#11078=FACE_OUTER_BOUND('',#16881,.T.);
#11079=FACE_OUTER_BOUND('',#16882,.T.);
#11080=FACE_OUTER_BOUND('',#16883,.T.);
#11081=FACE_OUTER_BOUND('',#16884,.T.);
#11082=FACE_OUTER_BOUND('',#16885,.T.);
#11083=FACE_OUTER_BOUND('',#16886,.T.);
#11084=FACE_OUTER_BOUND('',#16887,.T.);
#11085=FACE_OUTER_BOUND('',#16888,.T.);
#11086=FACE_OUTER_BOUND('',#16889,.T.);
#11087=FACE_OUTER_BOUND('',#16890,.T.);
#11088=FACE_OUTER_BOUND('',#16891,.T.);
#11089=FACE_OUTER_BOUND('',#16892,.T.);
#11090=FACE_OUTER_BOUND('',#16893,.T.);
#11091=FACE_OUTER_BOUND('',#16894,.T.);
#11092=FACE_OUTER_BOUND('',#16895,.T.);
#11093=FACE_OUTER_BOUND('',#16896,.T.);
#11094=FACE_OUTER_BOUND('',#16897,.T.);
#11095=FACE_OUTER_BOUND('',#16898,.T.);
#11096=FACE_OUTER_BOUND('',#16899,.T.);
#11097=FACE_OUTER_BOUND('',#16900,.T.);
#11098=FACE_OUTER_BOUND('',#16901,.T.);
#11099=FACE_OUTER_BOUND('',#16902,.T.);
#11100=FACE_OUTER_BOUND('',#16903,.T.);
#11101=FACE_OUTER_BOUND('',#16904,.T.);
#11102=FACE_OUTER_BOUND('',#16905,.T.);
#11103=FACE_OUTER_BOUND('',#16906,.T.);
#11104=FACE_OUTER_BOUND('',#16907,.T.);
#11105=FACE_OUTER_BOUND('',#16908,.T.);
#11106=FACE_OUTER_BOUND('',#16909,.T.);
#11107=FACE_OUTER_BOUND('',#16910,.T.);
#11108=FACE_OUTER_BOUND('',#16911,.T.);
#11109=FACE_OUTER_BOUND('',#16912,.T.);
#11110=FACE_OUTER_BOUND('',#16913,.T.);
#11111=FACE_OUTER_BOUND('',#16914,.T.);
#11112=FACE_OUTER_BOUND('',#16915,.T.);
#11113=FACE_OUTER_BOUND('',#16916,.T.);
#11114=FACE_OUTER_BOUND('',#16917,.T.);
#11115=FACE_OUTER_BOUND('',#16918,.T.);
#11116=FACE_OUTER_BOUND('',#16919,.T.);
#11117=FACE_OUTER_BOUND('',#16920,.T.);
#11118=FACE_OUTER_BOUND('',#16921,.T.);
#11119=FACE_OUTER_BOUND('',#16922,.T.);
#11120=FACE_OUTER_BOUND('',#16923,.T.);
#11121=FACE_OUTER_BOUND('',#16924,.T.);
#11122=FACE_OUTER_BOUND('',#16925,.T.);
#11123=FACE_OUTER_BOUND('',#16926,.T.);
#11124=FACE_OUTER_BOUND('',#16927,.T.);
#11125=FACE_OUTER_BOUND('',#16928,.T.);
#11126=FACE_OUTER_BOUND('',#16929,.T.);
#11127=FACE_OUTER_BOUND('',#16930,.T.);
#11128=FACE_OUTER_BOUND('',#16931,.T.);
#11129=FACE_OUTER_BOUND('',#16932,.T.);
#11130=FACE_OUTER_BOUND('',#16933,.T.);
#11131=FACE_OUTER_BOUND('',#16934,.T.);
#11132=FACE_OUTER_BOUND('',#16935,.T.);
#11133=FACE_OUTER_BOUND('',#16936,.T.);
#11134=FACE_OUTER_BOUND('',#16937,.T.);
#11135=FACE_OUTER_BOUND('',#16938,.T.);
#11136=FACE_OUTER_BOUND('',#16939,.T.);
#11137=FACE_OUTER_BOUND('',#16940,.T.);
#11138=FACE_OUTER_BOUND('',#16941,.T.);
#11139=FACE_OUTER_BOUND('',#16942,.T.);
#11140=FACE_OUTER_BOUND('',#16943,.T.);
#11141=FACE_OUTER_BOUND('',#16944,.T.);
#11142=FACE_OUTER_BOUND('',#16945,.T.);
#11143=FACE_OUTER_BOUND('',#16946,.T.);
#11144=FACE_OUTER_BOUND('',#16947,.T.);
#11145=FACE_OUTER_BOUND('',#16948,.T.);
#11146=FACE_OUTER_BOUND('',#16949,.T.);
#11147=FACE_OUTER_BOUND('',#16950,.T.);
#11148=FACE_OUTER_BOUND('',#16951,.T.);
#11149=FACE_OUTER_BOUND('',#16952,.T.);
#11150=FACE_OUTER_BOUND('',#16953,.T.);
#11151=FACE_OUTER_BOUND('',#16954,.T.);
#11152=FACE_OUTER_BOUND('',#16955,.T.);
#11153=FACE_OUTER_BOUND('',#16956,.T.);
#11154=FACE_OUTER_BOUND('',#16957,.T.);
#11155=FACE_OUTER_BOUND('',#16958,.T.);
#11156=FACE_OUTER_BOUND('',#16959,.T.);
#11157=FACE_OUTER_BOUND('',#16960,.T.);
#11158=FACE_OUTER_BOUND('',#16961,.T.);
#11159=FACE_OUTER_BOUND('',#16962,.T.);
#11160=FACE_OUTER_BOUND('',#16963,.T.);
#11161=FACE_OUTER_BOUND('',#16964,.T.);
#11162=FACE_OUTER_BOUND('',#16965,.T.);
#11163=FACE_OUTER_BOUND('',#16966,.T.);
#11164=FACE_OUTER_BOUND('',#16967,.T.);
#11165=FACE_OUTER_BOUND('',#16968,.T.);
#11166=FACE_OUTER_BOUND('',#16969,.T.);
#11167=FACE_OUTER_BOUND('',#16970,.T.);
#11168=FACE_OUTER_BOUND('',#16971,.T.);
#11169=FACE_OUTER_BOUND('',#16972,.T.);
#11170=FACE_OUTER_BOUND('',#16973,.T.);
#11171=FACE_OUTER_BOUND('',#16974,.T.);
#11172=FACE_OUTER_BOUND('',#16975,.T.);
#11173=FACE_OUTER_BOUND('',#16976,.T.);
#11174=FACE_OUTER_BOUND('',#16977,.T.);
#11175=FACE_OUTER_BOUND('',#16978,.T.);
#11176=FACE_OUTER_BOUND('',#16979,.T.);
#11177=FACE_OUTER_BOUND('',#16980,.T.);
#11178=FACE_OUTER_BOUND('',#16981,.T.);
#11179=FACE_OUTER_BOUND('',#16982,.T.);
#11180=FACE_OUTER_BOUND('',#16983,.T.);
#11181=FACE_OUTER_BOUND('',#16984,.T.);
#11182=FACE_OUTER_BOUND('',#16985,.T.);
#11183=FACE_OUTER_BOUND('',#16986,.T.);
#11184=FACE_OUTER_BOUND('',#16987,.T.);
#11185=FACE_OUTER_BOUND('',#16988,.T.);
#11186=FACE_OUTER_BOUND('',#16989,.T.);
#11187=FACE_OUTER_BOUND('',#16990,.T.);
#11188=FACE_OUTER_BOUND('',#16991,.T.);
#11189=FACE_OUTER_BOUND('',#16992,.T.);
#11190=FACE_OUTER_BOUND('',#16993,.T.);
#11191=FACE_OUTER_BOUND('',#16994,.T.);
#11192=FACE_OUTER_BOUND('',#16995,.T.);
#11193=FACE_OUTER_BOUND('',#16996,.T.);
#11194=FACE_OUTER_BOUND('',#16997,.T.);
#11195=FACE_OUTER_BOUND('',#16998,.T.);
#11196=FACE_OUTER_BOUND('',#16999,.T.);
#11197=FACE_OUTER_BOUND('',#17000,.T.);
#11198=FACE_OUTER_BOUND('',#17001,.T.);
#11199=FACE_OUTER_BOUND('',#17002,.T.);
#11200=FACE_OUTER_BOUND('',#17003,.T.);
#11201=FACE_OUTER_BOUND('',#17004,.T.);
#11202=FACE_OUTER_BOUND('',#17005,.T.);
#11203=FACE_OUTER_BOUND('',#17006,.T.);
#11204=FACE_OUTER_BOUND('',#17007,.T.);
#11205=FACE_OUTER_BOUND('',#17008,.T.);
#11206=FACE_OUTER_BOUND('',#17009,.T.);
#11207=FACE_OUTER_BOUND('',#17010,.T.);
#11208=FACE_OUTER_BOUND('',#17011,.T.);
#11209=FACE_OUTER_BOUND('',#17012,.T.);
#11210=FACE_OUTER_BOUND('',#17013,.T.);
#11211=FACE_OUTER_BOUND('',#17014,.T.);
#11212=FACE_OUTER_BOUND('',#17015,.T.);
#11213=FACE_OUTER_BOUND('',#17016,.T.);
#11214=FACE_OUTER_BOUND('',#17017,.T.);
#11215=FACE_OUTER_BOUND('',#17018,.T.);
#11216=FACE_OUTER_BOUND('',#17019,.T.);
#11217=FACE_OUTER_BOUND('',#17020,.T.);
#11218=FACE_OUTER_BOUND('',#17021,.T.);
#11219=FACE_OUTER_BOUND('',#17022,.T.);
#11220=FACE_OUTER_BOUND('',#17023,.T.);
#11221=FACE_OUTER_BOUND('',#17024,.T.);
#11222=FACE_OUTER_BOUND('',#17025,.T.);
#11223=FACE_OUTER_BOUND('',#17026,.T.);
#11224=FACE_OUTER_BOUND('',#17027,.T.);
#11225=FACE_OUTER_BOUND('',#17028,.T.);
#11226=FACE_OUTER_BOUND('',#17029,.T.);
#11227=FACE_OUTER_BOUND('',#17030,.T.);
#11228=FACE_OUTER_BOUND('',#17031,.T.);
#11229=FACE_OUTER_BOUND('',#17032,.T.);
#11230=FACE_OUTER_BOUND('',#17033,.T.);
#11231=FACE_OUTER_BOUND('',#17034,.T.);
#11232=FACE_OUTER_BOUND('',#17035,.T.);
#11233=FACE_OUTER_BOUND('',#17036,.T.);
#11234=FACE_OUTER_BOUND('',#17037,.T.);
#11235=FACE_OUTER_BOUND('',#17038,.T.);
#11236=FACE_OUTER_BOUND('',#17039,.T.);
#11237=FACE_OUTER_BOUND('',#17040,.T.);
#11238=FACE_OUTER_BOUND('',#17041,.T.);
#11239=FACE_OUTER_BOUND('',#17042,.T.);
#11240=FACE_OUTER_BOUND('',#17043,.T.);
#11241=FACE_OUTER_BOUND('',#17044,.T.);
#11242=FACE_OUTER_BOUND('',#17045,.T.);
#11243=FACE_OUTER_BOUND('',#17046,.T.);
#11244=FACE_OUTER_BOUND('',#17047,.T.);
#11245=FACE_OUTER_BOUND('',#17048,.T.);
#11246=FACE_OUTER_BOUND('',#17049,.T.);
#11247=FACE_OUTER_BOUND('',#17050,.T.);
#11248=FACE_OUTER_BOUND('',#17051,.T.);
#11249=FACE_OUTER_BOUND('',#17052,.T.);
#11250=FACE_OUTER_BOUND('',#17053,.T.);
#11251=FACE_OUTER_BOUND('',#17054,.T.);
#11252=FACE_OUTER_BOUND('',#17055,.T.);
#11253=FACE_OUTER_BOUND('',#17056,.T.);
#11254=FACE_OUTER_BOUND('',#17057,.T.);
#11255=FACE_OUTER_BOUND('',#17058,.T.);
#11256=FACE_OUTER_BOUND('',#17059,.T.);
#11257=FACE_OUTER_BOUND('',#17060,.T.);
#11258=FACE_OUTER_BOUND('',#17061,.T.);
#11259=FACE_OUTER_BOUND('',#17062,.T.);
#11260=FACE_OUTER_BOUND('',#17063,.T.);
#11261=FACE_OUTER_BOUND('',#17064,.T.);
#11262=FACE_OUTER_BOUND('',#17065,.T.);
#11263=FACE_OUTER_BOUND('',#17066,.T.);
#11264=FACE_OUTER_BOUND('',#17067,.T.);
#11265=FACE_OUTER_BOUND('',#17068,.T.);
#11266=FACE_OUTER_BOUND('',#17069,.T.);
#11267=FACE_OUTER_BOUND('',#17070,.T.);
#11268=FACE_OUTER_BOUND('',#17071,.T.);
#11269=FACE_OUTER_BOUND('',#17072,.T.);
#11270=FACE_OUTER_BOUND('',#17073,.T.);
#11271=FACE_OUTER_BOUND('',#17074,.T.);
#11272=FACE_OUTER_BOUND('',#17075,.T.);
#11273=FACE_OUTER_BOUND('',#17076,.T.);
#11274=FACE_OUTER_BOUND('',#17077,.T.);
#11275=FACE_OUTER_BOUND('',#17078,.T.);
#11276=FACE_OUTER_BOUND('',#17079,.T.);
#11277=FACE_OUTER_BOUND('',#17080,.T.);
#11278=FACE_OUTER_BOUND('',#17081,.T.);
#11279=FACE_OUTER_BOUND('',#17082,.T.);
#11280=FACE_OUTER_BOUND('',#17083,.T.);
#11281=FACE_OUTER_BOUND('',#17084,.T.);
#11282=FACE_OUTER_BOUND('',#17085,.T.);
#11283=FACE_OUTER_BOUND('',#17086,.T.);
#11284=FACE_OUTER_BOUND('',#17087,.T.);
#11285=FACE_OUTER_BOUND('',#17088,.T.);
#11286=FACE_OUTER_BOUND('',#17089,.T.);
#11287=FACE_OUTER_BOUND('',#17090,.T.);
#11288=FACE_OUTER_BOUND('',#17091,.T.);
#11289=FACE_OUTER_BOUND('',#17092,.T.);
#11290=FACE_OUTER_BOUND('',#17093,.T.);
#11291=FACE_OUTER_BOUND('',#17094,.T.);
#11292=FACE_OUTER_BOUND('',#17095,.T.);
#11293=FACE_OUTER_BOUND('',#17096,.T.);
#11294=FACE_OUTER_BOUND('',#17097,.T.);
#11295=FACE_OUTER_BOUND('',#17098,.T.);
#11296=FACE_OUTER_BOUND('',#17099,.T.);
#11297=FACE_OUTER_BOUND('',#17100,.T.);
#11298=FACE_OUTER_BOUND('',#17101,.T.);
#11299=FACE_OUTER_BOUND('',#17102,.T.);
#11300=FACE_OUTER_BOUND('',#17103,.T.);
#11301=FACE_OUTER_BOUND('',#17104,.T.);
#11302=FACE_OUTER_BOUND('',#17105,.T.);
#11303=FACE_OUTER_BOUND('',#17106,.T.);
#11304=FACE_OUTER_BOUND('',#17107,.T.);
#11305=FACE_OUTER_BOUND('',#17108,.T.);
#11306=FACE_OUTER_BOUND('',#17109,.T.);
#11307=FACE_OUTER_BOUND('',#17110,.T.);
#11308=FACE_OUTER_BOUND('',#17111,.T.);
#11309=FACE_OUTER_BOUND('',#17112,.T.);
#11310=FACE_OUTER_BOUND('',#17113,.T.);
#11311=FACE_OUTER_BOUND('',#17114,.T.);
#11312=FACE_OUTER_BOUND('',#17115,.T.);
#11313=FACE_OUTER_BOUND('',#17116,.T.);
#11314=FACE_OUTER_BOUND('',#17117,.T.);
#11315=FACE_OUTER_BOUND('',#17118,.T.);
#11316=FACE_OUTER_BOUND('',#17119,.T.);
#11317=FACE_OUTER_BOUND('',#17120,.T.);
#11318=FACE_OUTER_BOUND('',#17121,.T.);
#11319=FACE_OUTER_BOUND('',#17122,.T.);
#11320=FACE_OUTER_BOUND('',#17123,.T.);
#11321=FACE_OUTER_BOUND('',#17124,.T.);
#11322=FACE_OUTER_BOUND('',#17125,.T.);
#11323=FACE_OUTER_BOUND('',#17126,.T.);
#11324=FACE_OUTER_BOUND('',#17127,.T.);
#11325=FACE_OUTER_BOUND('',#17128,.T.);
#11326=FACE_OUTER_BOUND('',#17129,.T.);
#11327=FACE_OUTER_BOUND('',#17130,.T.);
#11328=FACE_OUTER_BOUND('',#17131,.T.);
#11329=FACE_OUTER_BOUND('',#17132,.T.);
#11330=FACE_OUTER_BOUND('',#17133,.T.);
#11331=FACE_OUTER_BOUND('',#17134,.T.);
#11332=FACE_OUTER_BOUND('',#17135,.T.);
#11333=FACE_OUTER_BOUND('',#17136,.T.);
#11334=FACE_OUTER_BOUND('',#17137,.T.);
#11335=FACE_OUTER_BOUND('',#17138,.T.);
#11336=FACE_OUTER_BOUND('',#17139,.T.);
#11337=FACE_OUTER_BOUND('',#17140,.T.);
#11338=FACE_OUTER_BOUND('',#17141,.T.);
#11339=FACE_OUTER_BOUND('',#17142,.T.);
#11340=FACE_OUTER_BOUND('',#17143,.T.);
#11341=FACE_OUTER_BOUND('',#17144,.T.);
#11342=FACE_OUTER_BOUND('',#17145,.T.);
#11343=FACE_OUTER_BOUND('',#17146,.T.);
#11344=FACE_OUTER_BOUND('',#17147,.T.);
#11345=FACE_OUTER_BOUND('',#17148,.T.);
#11346=FACE_OUTER_BOUND('',#17149,.T.);
#11347=FACE_OUTER_BOUND('',#17150,.T.);
#11348=FACE_OUTER_BOUND('',#17151,.T.);
#11349=FACE_OUTER_BOUND('',#17152,.T.);
#11350=FACE_OUTER_BOUND('',#17153,.T.);
#11351=FACE_OUTER_BOUND('',#17154,.T.);
#11352=FACE_OUTER_BOUND('',#17155,.T.);
#11353=FACE_OUTER_BOUND('',#17156,.T.);
#11354=FACE_OUTER_BOUND('',#17157,.T.);
#11355=FACE_OUTER_BOUND('',#17158,.T.);
#11356=FACE_OUTER_BOUND('',#17159,.T.);
#11357=FACE_OUTER_BOUND('',#17160,.T.);
#11358=FACE_OUTER_BOUND('',#17161,.T.);
#11359=FACE_OUTER_BOUND('',#17162,.T.);
#11360=FACE_OUTER_BOUND('',#17163,.T.);
#11361=FACE_OUTER_BOUND('',#17164,.T.);
#11362=FACE_OUTER_BOUND('',#17165,.T.);
#11363=FACE_OUTER_BOUND('',#17166,.T.);
#11364=FACE_OUTER_BOUND('',#17167,.T.);
#11365=FACE_OUTER_BOUND('',#17168,.T.);
#11366=FACE_OUTER_BOUND('',#17169,.T.);
#11367=FACE_OUTER_BOUND('',#17170,.T.);
#11368=FACE_OUTER_BOUND('',#17171,.T.);
#11369=FACE_OUTER_BOUND('',#17172,.T.);
#11370=FACE_OUTER_BOUND('',#17173,.T.);
#11371=FACE_OUTER_BOUND('',#17174,.T.);
#11372=FACE_OUTER_BOUND('',#17175,.T.);
#11373=FACE_OUTER_BOUND('',#17176,.T.);
#11374=FACE_OUTER_BOUND('',#17177,.T.);
#11375=FACE_OUTER_BOUND('',#17178,.T.);
#11376=FACE_OUTER_BOUND('',#17179,.T.);
#11377=FACE_OUTER_BOUND('',#17180,.T.);
#11378=FACE_OUTER_BOUND('',#17181,.T.);
#11379=FACE_OUTER_BOUND('',#17182,.T.);
#11380=FACE_OUTER_BOUND('',#17183,.T.);
#11381=FACE_OUTER_BOUND('',#17184,.T.);
#11382=FACE_OUTER_BOUND('',#17185,.T.);
#11383=FACE_OUTER_BOUND('',#17186,.T.);
#11384=FACE_OUTER_BOUND('',#17187,.T.);
#11385=FACE_OUTER_BOUND('',#17188,.T.);
#11386=FACE_OUTER_BOUND('',#17189,.T.);
#11387=FACE_OUTER_BOUND('',#17190,.T.);
#11388=FACE_OUTER_BOUND('',#17191,.T.);
#11389=FACE_OUTER_BOUND('',#17192,.T.);
#11390=FACE_OUTER_BOUND('',#17193,.T.);
#11391=FACE_OUTER_BOUND('',#17194,.T.);
#11392=FACE_OUTER_BOUND('',#17195,.T.);
#11393=FACE_OUTER_BOUND('',#17196,.T.);
#11394=FACE_OUTER_BOUND('',#17197,.T.);
#11395=FACE_OUTER_BOUND('',#17198,.T.);
#11396=FACE_OUTER_BOUND('',#17199,.T.);
#11397=FACE_OUTER_BOUND('',#17200,.T.);
#11398=FACE_OUTER_BOUND('',#17201,.T.);
#11399=FACE_OUTER_BOUND('',#17202,.T.);
#11400=FACE_OUTER_BOUND('',#17203,.T.);
#11401=FACE_OUTER_BOUND('',#17204,.T.);
#11402=FACE_OUTER_BOUND('',#17205,.T.);
#11403=FACE_OUTER_BOUND('',#17206,.T.);
#11404=FACE_OUTER_BOUND('',#17207,.T.);
#11405=FACE_OUTER_BOUND('',#17208,.T.);
#11406=FACE_OUTER_BOUND('',#17209,.T.);
#11407=FACE_OUTER_BOUND('',#17210,.T.);
#11408=FACE_OUTER_BOUND('',#17211,.T.);
#11409=FACE_OUTER_BOUND('',#17212,.T.);
#11410=FACE_OUTER_BOUND('',#17213,.T.);
#11411=FACE_OUTER_BOUND('',#17214,.T.);
#11412=FACE_OUTER_BOUND('',#17215,.T.);
#11413=FACE_OUTER_BOUND('',#17216,.T.);
#11414=FACE_OUTER_BOUND('',#17217,.T.);
#11415=FACE_OUTER_BOUND('',#17218,.T.);
#11416=FACE_OUTER_BOUND('',#17219,.T.);
#11417=FACE_OUTER_BOUND('',#17220,.T.);
#11418=FACE_OUTER_BOUND('',#17221,.T.);
#11419=FACE_OUTER_BOUND('',#17222,.T.);
#11420=FACE_OUTER_BOUND('',#17223,.T.);
#11421=FACE_OUTER_BOUND('',#17224,.T.);
#11422=FACE_OUTER_BOUND('',#17225,.T.);
#11423=FACE_OUTER_BOUND('',#17226,.T.);
#11424=FACE_OUTER_BOUND('',#17227,.T.);
#11425=FACE_OUTER_BOUND('',#17228,.T.);
#11426=FACE_OUTER_BOUND('',#17229,.T.);
#11427=FACE_OUTER_BOUND('',#17230,.T.);
#11428=FACE_OUTER_BOUND('',#17231,.T.);
#11429=FACE_OUTER_BOUND('',#17232,.T.);
#11430=FACE_OUTER_BOUND('',#17233,.T.);
#11431=FACE_OUTER_BOUND('',#17234,.T.);
#11432=FACE_OUTER_BOUND('',#17235,.T.);
#11433=FACE_OUTER_BOUND('',#17236,.T.);
#11434=FACE_OUTER_BOUND('',#17237,.T.);
#11435=FACE_OUTER_BOUND('',#17238,.T.);
#11436=FACE_OUTER_BOUND('',#17239,.T.);
#11437=FACE_OUTER_BOUND('',#17240,.T.);
#11438=FACE_OUTER_BOUND('',#17241,.T.);
#11439=FACE_OUTER_BOUND('',#17242,.T.);
#11440=FACE_OUTER_BOUND('',#17243,.T.);
#11441=FACE_OUTER_BOUND('',#17244,.T.);
#11442=FACE_OUTER_BOUND('',#17245,.T.);
#11443=FACE_OUTER_BOUND('',#17246,.T.);
#11444=FACE_OUTER_BOUND('',#17247,.T.);
#11445=FACE_OUTER_BOUND('',#17248,.T.);
#11446=FACE_OUTER_BOUND('',#17249,.T.);
#11447=FACE_OUTER_BOUND('',#17250,.T.);
#11448=FACE_OUTER_BOUND('',#17251,.T.);
#11449=FACE_OUTER_BOUND('',#17252,.T.);
#11450=FACE_OUTER_BOUND('',#17253,.T.);
#11451=FACE_OUTER_BOUND('',#17254,.T.);
#11452=FACE_OUTER_BOUND('',#17255,.T.);
#11453=FACE_OUTER_BOUND('',#17256,.T.);
#11454=FACE_OUTER_BOUND('',#17257,.T.);
#11455=FACE_OUTER_BOUND('',#17258,.T.);
#11456=FACE_OUTER_BOUND('',#17259,.T.);
#11457=FACE_OUTER_BOUND('',#17260,.T.);
#11458=FACE_OUTER_BOUND('',#17261,.T.);
#11459=FACE_OUTER_BOUND('',#17262,.T.);
#11460=FACE_OUTER_BOUND('',#17263,.T.);
#11461=FACE_OUTER_BOUND('',#17264,.T.);
#11462=FACE_OUTER_BOUND('',#17265,.T.);
#11463=FACE_OUTER_BOUND('',#17266,.T.);
#11464=FACE_OUTER_BOUND('',#17267,.T.);
#11465=FACE_OUTER_BOUND('',#17268,.T.);
#11466=FACE_OUTER_BOUND('',#17269,.T.);
#11467=FACE_OUTER_BOUND('',#17270,.T.);
#11468=FACE_OUTER_BOUND('',#17271,.T.);
#11469=FACE_OUTER_BOUND('',#17272,.T.);
#11470=FACE_OUTER_BOUND('',#17273,.T.);
#11471=FACE_OUTER_BOUND('',#17274,.T.);
#11472=FACE_OUTER_BOUND('',#17275,.T.);
#11473=FACE_OUTER_BOUND('',#17276,.T.);
#11474=FACE_OUTER_BOUND('',#17277,.T.);
#11475=FACE_OUTER_BOUND('',#17278,.T.);
#11476=FACE_OUTER_BOUND('',#17279,.T.);
#11477=FACE_OUTER_BOUND('',#17280,.T.);
#11478=FACE_OUTER_BOUND('',#17281,.T.);
#11479=FACE_OUTER_BOUND('',#17282,.T.);
#11480=FACE_OUTER_BOUND('',#17283,.T.);
#11481=FACE_OUTER_BOUND('',#17284,.T.);
#11482=FACE_OUTER_BOUND('',#17285,.T.);
#11483=FACE_OUTER_BOUND('',#17286,.T.);
#11484=FACE_OUTER_BOUND('',#17287,.T.);
#11485=FACE_OUTER_BOUND('',#17288,.T.);
#11486=FACE_OUTER_BOUND('',#17289,.T.);
#11487=FACE_OUTER_BOUND('',#17290,.T.);
#11488=FACE_OUTER_BOUND('',#17291,.T.);
#11489=FACE_OUTER_BOUND('',#17292,.T.);
#11490=FACE_OUTER_BOUND('',#17293,.T.);
#11491=FACE_OUTER_BOUND('',#17294,.T.);
#11492=FACE_OUTER_BOUND('',#17295,.T.);
#11493=FACE_OUTER_BOUND('',#17296,.T.);
#11494=FACE_OUTER_BOUND('',#17297,.T.);
#11495=FACE_OUTER_BOUND('',#17298,.T.);
#11496=FACE_OUTER_BOUND('',#17299,.T.);
#11497=FACE_OUTER_BOUND('',#17300,.T.);
#11498=FACE_OUTER_BOUND('',#17301,.T.);
#11499=FACE_OUTER_BOUND('',#17302,.T.);
#11500=FACE_OUTER_BOUND('',#17303,.T.);
#11501=FACE_OUTER_BOUND('',#17304,.T.);
#11502=FACE_OUTER_BOUND('',#17305,.T.);
#11503=FACE_OUTER_BOUND('',#17306,.T.);
#11504=FACE_OUTER_BOUND('',#17307,.T.);
#11505=FACE_OUTER_BOUND('',#17308,.T.);
#11506=FACE_OUTER_BOUND('',#17309,.T.);
#11507=FACE_OUTER_BOUND('',#17310,.T.);
#11508=FACE_OUTER_BOUND('',#17311,.T.);
#11509=FACE_OUTER_BOUND('',#17312,.T.);
#11510=FACE_OUTER_BOUND('',#17313,.T.);
#11511=FACE_OUTER_BOUND('',#17314,.T.);
#11512=FACE_OUTER_BOUND('',#17315,.T.);
#11513=FACE_OUTER_BOUND('',#17316,.T.);
#11514=FACE_OUTER_BOUND('',#17317,.T.);
#11515=FACE_OUTER_BOUND('',#17318,.T.);
#11516=FACE_OUTER_BOUND('',#17319,.T.);
#11517=FACE_OUTER_BOUND('',#17320,.T.);
#11518=FACE_OUTER_BOUND('',#17321,.T.);
#11519=FACE_OUTER_BOUND('',#17322,.T.);
#11520=FACE_OUTER_BOUND('',#17323,.T.);
#11521=FACE_OUTER_BOUND('',#17324,.T.);
#11522=FACE_OUTER_BOUND('',#17325,.T.);
#11523=FACE_OUTER_BOUND('',#17326,.T.);
#11524=FACE_OUTER_BOUND('',#17327,.T.);
#11525=FACE_OUTER_BOUND('',#17328,.T.);
#11526=FACE_OUTER_BOUND('',#17329,.T.);
#11527=FACE_OUTER_BOUND('',#17330,.T.);
#11528=FACE_OUTER_BOUND('',#17331,.T.);
#11529=FACE_OUTER_BOUND('',#17332,.T.);
#11530=FACE_OUTER_BOUND('',#17333,.T.);
#11531=FACE_OUTER_BOUND('',#17334,.T.);
#11532=FACE_OUTER_BOUND('',#17335,.T.);
#11533=FACE_OUTER_BOUND('',#17336,.T.);
#11534=FACE_OUTER_BOUND('',#17337,.T.);
#11535=FACE_OUTER_BOUND('',#17338,.T.);
#11536=FACE_OUTER_BOUND('',#17339,.T.);
#11537=FACE_OUTER_BOUND('',#17340,.T.);
#11538=FACE_OUTER_BOUND('',#17341,.T.);
#11539=FACE_OUTER_BOUND('',#17342,.T.);
#11540=FACE_OUTER_BOUND('',#17343,.T.);
#11541=FACE_OUTER_BOUND('',#17344,.T.);
#11542=FACE_OUTER_BOUND('',#17345,.T.);
#11543=FACE_OUTER_BOUND('',#17346,.T.);
#11544=FACE_OUTER_BOUND('',#17347,.T.);
#11545=FACE_OUTER_BOUND('',#17348,.T.);
#11546=FACE_OUTER_BOUND('',#17349,.T.);
#11547=FACE_OUTER_BOUND('',#17350,.T.);
#11548=FACE_OUTER_BOUND('',#17351,.T.);
#11549=FACE_OUTER_BOUND('',#17352,.T.);
#11550=FACE_OUTER_BOUND('',#17353,.T.);
#11551=FACE_OUTER_BOUND('',#17354,.T.);
#11552=FACE_OUTER_BOUND('',#17355,.T.);
#11553=FACE_OUTER_BOUND('',#17356,.T.);
#11554=FACE_OUTER_BOUND('',#17357,.T.);
#11555=FACE_OUTER_BOUND('',#17358,.T.);
#11556=FACE_OUTER_BOUND('',#17359,.T.);
#11557=FACE_OUTER_BOUND('',#17360,.T.);
#11558=FACE_OUTER_BOUND('',#17361,.T.);
#11559=FACE_OUTER_BOUND('',#17362,.T.);
#11560=FACE_OUTER_BOUND('',#17363,.T.);
#11561=FACE_OUTER_BOUND('',#17364,.T.);
#11562=FACE_OUTER_BOUND('',#17365,.T.);
#11563=FACE_OUTER_BOUND('',#17366,.T.);
#11564=FACE_OUTER_BOUND('',#17367,.T.);
#11565=FACE_OUTER_BOUND('',#17368,.T.);
#11566=FACE_OUTER_BOUND('',#17369,.T.);
#11567=FACE_OUTER_BOUND('',#17370,.T.);
#11568=FACE_OUTER_BOUND('',#17371,.T.);
#11569=FACE_OUTER_BOUND('',#17372,.T.);
#11570=FACE_OUTER_BOUND('',#17373,.T.);
#11571=FACE_OUTER_BOUND('',#17374,.T.);
#11572=FACE_OUTER_BOUND('',#17375,.T.);
#11573=FACE_OUTER_BOUND('',#17376,.T.);
#11574=FACE_OUTER_BOUND('',#17377,.T.);
#11575=FACE_OUTER_BOUND('',#17378,.T.);
#11576=FACE_OUTER_BOUND('',#17379,.T.);
#11577=FACE_OUTER_BOUND('',#17380,.T.);
#11578=FACE_OUTER_BOUND('',#17381,.T.);
#11579=FACE_OUTER_BOUND('',#17382,.T.);
#11580=FACE_OUTER_BOUND('',#17383,.T.);
#11581=FACE_OUTER_BOUND('',#17384,.T.);
#11582=FACE_OUTER_BOUND('',#17385,.T.);
#11583=FACE_OUTER_BOUND('',#17386,.T.);
#11584=FACE_OUTER_BOUND('',#17387,.T.);
#11585=FACE_OUTER_BOUND('',#17388,.T.);
#11586=FACE_OUTER_BOUND('',#17389,.T.);
#11587=FACE_OUTER_BOUND('',#17390,.T.);
#11588=FACE_OUTER_BOUND('',#17391,.T.);
#11589=FACE_OUTER_BOUND('',#17392,.T.);
#11590=FACE_OUTER_BOUND('',#17393,.T.);
#11591=FACE_OUTER_BOUND('',#17394,.T.);
#11592=FACE_OUTER_BOUND('',#17395,.T.);
#11593=FACE_OUTER_BOUND('',#17396,.T.);
#11594=FACE_OUTER_BOUND('',#17397,.T.);
#11595=FACE_OUTER_BOUND('',#17398,.T.);
#11596=FACE_OUTER_BOUND('',#17399,.T.);
#11597=FACE_OUTER_BOUND('',#17400,.T.);
#11598=FACE_OUTER_BOUND('',#17401,.T.);
#11599=FACE_OUTER_BOUND('',#17402,.T.);
#11600=FACE_OUTER_BOUND('',#17403,.T.);
#11601=FACE_OUTER_BOUND('',#17404,.T.);
#11602=FACE_OUTER_BOUND('',#17405,.T.);
#11603=FACE_OUTER_BOUND('',#17406,.T.);
#11604=FACE_OUTER_BOUND('',#17407,.T.);
#11605=FACE_OUTER_BOUND('',#17408,.T.);
#11606=FACE_OUTER_BOUND('',#17409,.T.);
#11607=FACE_OUTER_BOUND('',#17410,.T.);
#11608=FACE_OUTER_BOUND('',#17411,.T.);
#11609=FACE_OUTER_BOUND('',#17412,.T.);
#11610=FACE_OUTER_BOUND('',#17413,.T.);
#11611=FACE_OUTER_BOUND('',#17414,.T.);
#11612=FACE_OUTER_BOUND('',#17415,.T.);
#11613=FACE_OUTER_BOUND('',#17416,.T.);
#11614=FACE_OUTER_BOUND('',#17417,.T.);
#11615=FACE_OUTER_BOUND('',#17418,.T.);
#11616=FACE_OUTER_BOUND('',#17419,.T.);
#11617=FACE_OUTER_BOUND('',#17420,.T.);
#11618=FACE_OUTER_BOUND('',#17421,.T.);
#11619=FACE_OUTER_BOUND('',#17422,.T.);
#11620=FACE_OUTER_BOUND('',#17423,.T.);
#11621=FACE_OUTER_BOUND('',#17424,.T.);
#11622=FACE_OUTER_BOUND('',#17425,.T.);
#11623=FACE_OUTER_BOUND('',#17426,.T.);
#11624=FACE_OUTER_BOUND('',#17427,.T.);
#11625=FACE_OUTER_BOUND('',#17428,.T.);
#11626=FACE_OUTER_BOUND('',#17429,.T.);
#11627=FACE_OUTER_BOUND('',#17430,.T.);
#11628=FACE_OUTER_BOUND('',#17431,.T.);
#11629=FACE_OUTER_BOUND('',#17432,.T.);
#11630=FACE_OUTER_BOUND('',#17433,.T.);
#11631=FACE_OUTER_BOUND('',#17434,.T.);
#11632=FACE_OUTER_BOUND('',#17435,.T.);
#11633=FACE_OUTER_BOUND('',#17436,.T.);
#11634=FACE_OUTER_BOUND('',#17437,.T.);
#11635=FACE_OUTER_BOUND('',#17438,.T.);
#11636=FACE_OUTER_BOUND('',#17439,.T.);
#11637=FACE_OUTER_BOUND('',#17440,.T.);
#11638=FACE_OUTER_BOUND('',#17441,.T.);
#11639=FACE_OUTER_BOUND('',#17442,.T.);
#11640=FACE_OUTER_BOUND('',#17443,.T.);
#11641=FACE_OUTER_BOUND('',#17444,.T.);
#11642=FACE_OUTER_BOUND('',#17445,.T.);
#11643=FACE_OUTER_BOUND('',#17446,.T.);
#11644=FACE_OUTER_BOUND('',#17447,.T.);
#11645=FACE_OUTER_BOUND('',#17448,.T.);
#11646=FACE_OUTER_BOUND('',#17449,.T.);
#11647=FACE_OUTER_BOUND('',#17450,.T.);
#11648=FACE_OUTER_BOUND('',#17451,.T.);
#11649=FACE_OUTER_BOUND('',#17452,.T.);
#11650=FACE_OUTER_BOUND('',#17453,.T.);
#11651=FACE_OUTER_BOUND('',#17454,.T.);
#11652=FACE_OUTER_BOUND('',#17455,.T.);
#11653=FACE_OUTER_BOUND('',#17456,.T.);
#11654=FACE_OUTER_BOUND('',#17457,.T.);
#11655=FACE_OUTER_BOUND('',#17458,.T.);
#11656=FACE_OUTER_BOUND('',#17459,.T.);
#11657=FACE_OUTER_BOUND('',#17460,.T.);
#11658=FACE_OUTER_BOUND('',#17461,.T.);
#11659=FACE_OUTER_BOUND('',#17462,.T.);
#11660=FACE_OUTER_BOUND('',#17463,.T.);
#11661=FACE_OUTER_BOUND('',#17464,.T.);
#11662=FACE_OUTER_BOUND('',#17465,.T.);
#11663=FACE_OUTER_BOUND('',#17466,.T.);
#11664=FACE_OUTER_BOUND('',#17467,.T.);
#11665=FACE_OUTER_BOUND('',#17468,.T.);
#11666=FACE_OUTER_BOUND('',#17469,.T.);
#11667=FACE_OUTER_BOUND('',#17470,.T.);
#11668=FACE_OUTER_BOUND('',#17471,.T.);
#11669=FACE_OUTER_BOUND('',#17472,.T.);
#11670=FACE_OUTER_BOUND('',#17473,.T.);
#11671=FACE_OUTER_BOUND('',#17474,.T.);
#11672=FACE_OUTER_BOUND('',#17475,.T.);
#11673=FACE_OUTER_BOUND('',#17476,.T.);
#11674=FACE_OUTER_BOUND('',#17477,.T.);
#11675=FACE_OUTER_BOUND('',#17478,.T.);
#11676=FACE_OUTER_BOUND('',#17479,.T.);
#11677=FACE_OUTER_BOUND('',#17480,.T.);
#11678=FACE_OUTER_BOUND('',#17481,.T.);
#11679=FACE_OUTER_BOUND('',#17482,.T.);
#11680=FACE_OUTER_BOUND('',#17483,.T.);
#11681=FACE_OUTER_BOUND('',#17484,.T.);
#11682=FACE_OUTER_BOUND('',#17485,.T.);
#11683=FACE_OUTER_BOUND('',#17486,.T.);
#11684=FACE_OUTER_BOUND('',#17487,.T.);
#11685=FACE_OUTER_BOUND('',#17488,.T.);
#11686=FACE_OUTER_BOUND('',#17489,.T.);
#11687=FACE_OUTER_BOUND('',#17490,.T.);
#11688=FACE_OUTER_BOUND('',#17491,.T.);
#11689=FACE_OUTER_BOUND('',#17492,.T.);
#11690=FACE_OUTER_BOUND('',#17493,.T.);
#11691=FACE_OUTER_BOUND('',#17494,.T.);
#11692=FACE_OUTER_BOUND('',#17495,.T.);
#11693=FACE_OUTER_BOUND('',#17496,.T.);
#11694=FACE_OUTER_BOUND('',#17497,.T.);
#11695=FACE_OUTER_BOUND('',#17498,.T.);
#11696=FACE_OUTER_BOUND('',#17499,.T.);
#11697=FACE_OUTER_BOUND('',#17500,.T.);
#11698=FACE_OUTER_BOUND('',#17501,.T.);
#11699=FACE_OUTER_BOUND('',#17502,.T.);
#11700=FACE_OUTER_BOUND('',#17503,.T.);
#11701=FACE_OUTER_BOUND('',#17504,.T.);
#11702=FACE_OUTER_BOUND('',#17505,.T.);
#11703=FACE_OUTER_BOUND('',#17506,.T.);
#11704=FACE_OUTER_BOUND('',#17507,.T.);
#11705=FACE_OUTER_BOUND('',#17508,.T.);
#11706=FACE_OUTER_BOUND('',#17509,.T.);
#11707=FACE_OUTER_BOUND('',#17510,.T.);
#11708=FACE_OUTER_BOUND('',#17511,.T.);
#11709=FACE_OUTER_BOUND('',#17512,.T.);
#11710=FACE_OUTER_BOUND('',#17513,.T.);
#11711=FACE_OUTER_BOUND('',#17514,.T.);
#11712=FACE_OUTER_BOUND('',#17515,.T.);
#11713=FACE_OUTER_BOUND('',#17516,.T.);
#11714=FACE_OUTER_BOUND('',#17517,.T.);
#11715=FACE_OUTER_BOUND('',#17518,.T.);
#11716=FACE_OUTER_BOUND('',#17519,.T.);
#11717=FACE_OUTER_BOUND('',#17520,.T.);
#11718=FACE_OUTER_BOUND('',#17521,.T.);
#11719=FACE_OUTER_BOUND('',#17522,.T.);
#11720=FACE_OUTER_BOUND('',#17523,.T.);
#11721=FACE_OUTER_BOUND('',#17524,.T.);
#11722=FACE_OUTER_BOUND('',#17525,.T.);
#11723=FACE_OUTER_BOUND('',#17526,.T.);
#11724=FACE_OUTER_BOUND('',#17527,.T.);
#11725=FACE_OUTER_BOUND('',#17528,.T.);
#11726=FACE_OUTER_BOUND('',#17529,.T.);
#11727=FACE_OUTER_BOUND('',#17530,.T.);
#11728=FACE_OUTER_BOUND('',#17531,.T.);
#11729=FACE_OUTER_BOUND('',#17532,.T.);
#11730=FACE_OUTER_BOUND('',#17533,.T.);
#11731=FACE_OUTER_BOUND('',#17534,.T.);
#11732=FACE_OUTER_BOUND('',#17535,.T.);
#11733=FACE_OUTER_BOUND('',#17536,.T.);
#11734=FACE_OUTER_BOUND('',#17537,.T.);
#11735=FACE_OUTER_BOUND('',#17538,.T.);
#11736=FACE_OUTER_BOUND('',#17539,.T.);
#11737=FACE_OUTER_BOUND('',#17540,.T.);
#11738=FACE_OUTER_BOUND('',#17541,.T.);
#11739=FACE_OUTER_BOUND('',#17542,.T.);
#11740=FACE_OUTER_BOUND('',#17543,.T.);
#11741=FACE_OUTER_BOUND('',#17544,.T.);
#11742=FACE_OUTER_BOUND('',#17545,.T.);
#11743=FACE_OUTER_BOUND('',#17546,.T.);
#11744=FACE_OUTER_BOUND('',#17547,.T.);
#11745=FACE_OUTER_BOUND('',#17548,.T.);
#11746=FACE_OUTER_BOUND('',#17549,.T.);
#11747=FACE_OUTER_BOUND('',#17550,.T.);
#11748=FACE_OUTER_BOUND('',#17551,.T.);
#11749=FACE_OUTER_BOUND('',#17552,.T.);
#11750=FACE_OUTER_BOUND('',#17553,.T.);
#11751=FACE_OUTER_BOUND('',#17554,.T.);
#11752=FACE_OUTER_BOUND('',#17555,.T.);
#11753=FACE_OUTER_BOUND('',#17556,.T.);
#11754=FACE_OUTER_BOUND('',#17557,.T.);
#11755=FACE_OUTER_BOUND('',#17558,.T.);
#11756=FACE_OUTER_BOUND('',#17559,.T.);
#11757=FACE_OUTER_BOUND('',#17560,.T.);
#11758=FACE_OUTER_BOUND('',#17561,.T.);
#11759=FACE_OUTER_BOUND('',#17562,.T.);
#11760=FACE_OUTER_BOUND('',#17563,.T.);
#11761=FACE_OUTER_BOUND('',#17564,.T.);
#11762=FACE_OUTER_BOUND('',#17566,.T.);
#11763=FACE_OUTER_BOUND('',#17567,.T.);
#11764=FACE_OUTER_BOUND('',#17568,.T.);
#11765=FACE_OUTER_BOUND('',#17569,.T.);
#11766=FACE_OUTER_BOUND('',#17570,.T.);
#11767=FACE_OUTER_BOUND('',#17571,.T.);
#11768=FACE_OUTER_BOUND('',#17572,.T.);
#11769=FACE_OUTER_BOUND('',#17573,.T.);
#11770=FACE_OUTER_BOUND('',#17574,.T.);
#11771=FACE_OUTER_BOUND('',#17575,.T.);
#11772=FACE_OUTER_BOUND('',#17576,.T.);
#11773=FACE_OUTER_BOUND('',#17577,.T.);
#11774=FACE_OUTER_BOUND('',#17578,.T.);
#11775=FACE_OUTER_BOUND('',#17579,.T.);
#11776=FACE_OUTER_BOUND('',#17580,.T.);
#11777=FACE_OUTER_BOUND('',#17581,.T.);
#11778=FACE_OUTER_BOUND('',#17582,.T.);
#11779=FACE_OUTER_BOUND('',#17583,.T.);
#11780=FACE_OUTER_BOUND('',#17584,.T.);
#11781=FACE_OUTER_BOUND('',#17585,.T.);
#11782=FACE_OUTER_BOUND('',#17586,.T.);
#11783=FACE_OUTER_BOUND('',#17587,.T.);
#11784=FACE_OUTER_BOUND('',#17588,.T.);
#11785=FACE_OUTER_BOUND('',#17589,.T.);
#11786=FACE_OUTER_BOUND('',#17590,.T.);
#11787=FACE_OUTER_BOUND('',#17591,.T.);
#11788=FACE_OUTER_BOUND('',#17592,.T.);
#11789=FACE_OUTER_BOUND('',#17593,.T.);
#11790=FACE_OUTER_BOUND('',#17594,.T.);
#11791=FACE_OUTER_BOUND('',#17595,.T.);
#11792=FACE_OUTER_BOUND('',#17596,.T.);
#11793=FACE_OUTER_BOUND('',#17597,.T.);
#11794=FACE_OUTER_BOUND('',#17598,.T.);
#11795=FACE_OUTER_BOUND('',#17599,.T.);
#11796=FACE_OUTER_BOUND('',#17600,.T.);
#11797=FACE_OUTER_BOUND('',#17601,.T.);
#11798=FACE_OUTER_BOUND('',#17602,.T.);
#11799=FACE_OUTER_BOUND('',#17603,.T.);
#11800=FACE_OUTER_BOUND('',#17604,.T.);
#11801=FACE_OUTER_BOUND('',#17605,.T.);
#11802=FACE_OUTER_BOUND('',#17606,.T.);
#11803=FACE_OUTER_BOUND('',#17607,.T.);
#11804=FACE_OUTER_BOUND('',#17608,.T.);
#11805=FACE_OUTER_BOUND('',#17609,.T.);
#11806=FACE_OUTER_BOUND('',#17610,.T.);
#11807=FACE_OUTER_BOUND('',#17611,.T.);
#11808=FACE_OUTER_BOUND('',#17612,.T.);
#11809=FACE_OUTER_BOUND('',#17613,.T.);
#11810=FACE_OUTER_BOUND('',#17614,.T.);
#11811=FACE_OUTER_BOUND('',#17615,.T.);
#11812=FACE_OUTER_BOUND('',#17616,.T.);
#11813=FACE_OUTER_BOUND('',#17617,.T.);
#11814=FACE_OUTER_BOUND('',#17618,.T.);
#11815=FACE_OUTER_BOUND('',#17619,.T.);
#11816=FACE_OUTER_BOUND('',#17620,.T.);
#11817=FACE_OUTER_BOUND('',#17621,.T.);
#11818=FACE_OUTER_BOUND('',#17622,.T.);
#11819=FACE_OUTER_BOUND('',#17623,.T.);
#11820=FACE_OUTER_BOUND('',#17624,.T.);
#11821=FACE_OUTER_BOUND('',#17625,.T.);
#11822=FACE_OUTER_BOUND('',#17626,.T.);
#11823=FACE_OUTER_BOUND('',#17627,.T.);
#11824=FACE_OUTER_BOUND('',#17628,.T.);
#11825=FACE_OUTER_BOUND('',#17629,.T.);
#11826=FACE_OUTER_BOUND('',#17630,.T.);
#11827=FACE_OUTER_BOUND('',#17631,.T.);
#11828=FACE_OUTER_BOUND('',#17632,.T.);
#11829=FACE_OUTER_BOUND('',#17633,.T.);
#11830=FACE_OUTER_BOUND('',#17634,.T.);
#11831=FACE_OUTER_BOUND('',#17635,.T.);
#11832=FACE_OUTER_BOUND('',#17636,.T.);
#11833=FACE_OUTER_BOUND('',#17637,.T.);
#11834=FACE_OUTER_BOUND('',#17638,.T.);
#11835=FACE_OUTER_BOUND('',#17639,.T.);
#11836=FACE_OUTER_BOUND('',#17640,.T.);
#11837=FACE_OUTER_BOUND('',#17641,.T.);
#11838=FACE_OUTER_BOUND('',#17642,.T.);
#11839=FACE_OUTER_BOUND('',#17643,.T.);
#11840=FACE_OUTER_BOUND('',#17644,.T.);
#11841=FACE_OUTER_BOUND('',#17645,.T.);
#11842=FACE_OUTER_BOUND('',#17646,.T.);
#11843=FACE_OUTER_BOUND('',#17647,.T.);
#11844=FACE_OUTER_BOUND('',#17648,.T.);
#11845=FACE_OUTER_BOUND('',#17649,.T.);
#11846=FACE_OUTER_BOUND('',#17650,.T.);
#11847=FACE_OUTER_BOUND('',#17651,.T.);
#11848=FACE_OUTER_BOUND('',#17652,.T.);
#11849=FACE_OUTER_BOUND('',#17653,.T.);
#11850=FACE_OUTER_BOUND('',#17654,.T.);
#11851=FACE_OUTER_BOUND('',#17655,.T.);
#11852=FACE_OUTER_BOUND('',#17656,.T.);
#11853=FACE_OUTER_BOUND('',#17657,.T.);
#11854=FACE_OUTER_BOUND('',#17658,.T.);
#11855=FACE_OUTER_BOUND('',#17659,.T.);
#11856=FACE_OUTER_BOUND('',#17660,.T.);
#11857=FACE_OUTER_BOUND('',#17661,.T.);
#11858=FACE_OUTER_BOUND('',#17662,.T.);
#11859=FACE_OUTER_BOUND('',#17663,.T.);
#11860=FACE_OUTER_BOUND('',#17664,.T.);
#11861=FACE_OUTER_BOUND('',#17665,.T.);
#11862=FACE_OUTER_BOUND('',#17666,.T.);
#11863=FACE_OUTER_BOUND('',#17667,.T.);
#11864=FACE_OUTER_BOUND('',#17668,.T.);
#11865=FACE_OUTER_BOUND('',#17669,.T.);
#11866=FACE_OUTER_BOUND('',#17670,.T.);
#11867=FACE_OUTER_BOUND('',#17671,.T.);
#11868=FACE_OUTER_BOUND('',#17672,.T.);
#11869=FACE_OUTER_BOUND('',#17673,.T.);
#11870=FACE_OUTER_BOUND('',#17674,.T.);
#11871=FACE_OUTER_BOUND('',#17675,.T.);
#11872=FACE_OUTER_BOUND('',#17676,.T.);
#11873=FACE_OUTER_BOUND('',#17677,.T.);
#11874=FACE_OUTER_BOUND('',#17678,.T.);
#11875=FACE_OUTER_BOUND('',#17679,.T.);
#11876=FACE_OUTER_BOUND('',#17680,.T.);
#11877=FACE_OUTER_BOUND('',#17681,.T.);
#11878=FACE_OUTER_BOUND('',#17682,.T.);
#11879=FACE_OUTER_BOUND('',#17683,.T.);
#11880=FACE_OUTER_BOUND('',#17684,.T.);
#11881=FACE_OUTER_BOUND('',#17685,.T.);
#11882=FACE_OUTER_BOUND('',#17686,.T.);
#11883=FACE_OUTER_BOUND('',#17687,.T.);
#11884=FACE_OUTER_BOUND('',#17688,.T.);
#11885=FACE_OUTER_BOUND('',#17689,.T.);
#11886=FACE_OUTER_BOUND('',#17690,.T.);
#11887=FACE_OUTER_BOUND('',#17691,.T.);
#11888=FACE_OUTER_BOUND('',#17692,.T.);
#11889=FACE_OUTER_BOUND('',#17693,.T.);
#11890=FACE_OUTER_BOUND('',#17694,.T.);
#11891=FACE_OUTER_BOUND('',#17695,.T.);
#11892=FACE_OUTER_BOUND('',#17696,.T.);
#11893=FACE_OUTER_BOUND('',#17697,.T.);
#11894=FACE_OUTER_BOUND('',#17698,.T.);
#11895=FACE_OUTER_BOUND('',#17699,.T.);
#11896=FACE_OUTER_BOUND('',#17700,.T.);
#11897=FACE_OUTER_BOUND('',#17701,.T.);
#11898=FACE_OUTER_BOUND('',#17702,.T.);
#11899=FACE_OUTER_BOUND('',#17703,.T.);
#11900=FACE_OUTER_BOUND('',#17704,.T.);
#11901=FACE_OUTER_BOUND('',#17705,.T.);
#11902=FACE_OUTER_BOUND('',#17706,.T.);
#11903=FACE_OUTER_BOUND('',#17707,.T.);
#11904=FACE_OUTER_BOUND('',#17708,.T.);
#11905=FACE_OUTER_BOUND('',#17709,.T.);
#11906=FACE_OUTER_BOUND('',#17710,.T.);
#11907=FACE_OUTER_BOUND('',#17711,.T.);
#11908=FACE_OUTER_BOUND('',#17712,.T.);
#11909=FACE_OUTER_BOUND('',#17713,.T.);
#11910=FACE_OUTER_BOUND('',#17714,.T.);
#11911=FACE_OUTER_BOUND('',#17715,.T.);
#11912=FACE_OUTER_BOUND('',#17716,.T.);
#11913=FACE_OUTER_BOUND('',#17717,.T.);
#11914=FACE_OUTER_BOUND('',#17718,.T.);
#11915=FACE_OUTER_BOUND('',#17719,.T.);
#11916=FACE_OUTER_BOUND('',#17720,.T.);
#11917=FACE_OUTER_BOUND('',#17721,.T.);
#11918=FACE_OUTER_BOUND('',#17722,.T.);
#11919=FACE_OUTER_BOUND('',#17723,.T.);
#11920=FACE_OUTER_BOUND('',#17724,.T.);
#11921=FACE_OUTER_BOUND('',#17725,.T.);
#11922=FACE_OUTER_BOUND('',#17726,.T.);
#11923=FACE_OUTER_BOUND('',#17727,.T.);
#11924=FACE_OUTER_BOUND('',#17728,.T.);
#11925=FACE_OUTER_BOUND('',#17729,.T.);
#11926=FACE_OUTER_BOUND('',#17730,.T.);
#11927=FACE_OUTER_BOUND('',#17731,.T.);
#11928=FACE_OUTER_BOUND('',#17732,.T.);
#11929=FACE_OUTER_BOUND('',#17733,.T.);
#11930=FACE_OUTER_BOUND('',#17734,.T.);
#11931=FACE_OUTER_BOUND('',#17735,.T.);
#11932=FACE_OUTER_BOUND('',#17736,.T.);
#11933=FACE_OUTER_BOUND('',#17737,.T.);
#11934=FACE_OUTER_BOUND('',#17738,.T.);
#11935=FACE_OUTER_BOUND('',#17739,.T.);
#11936=FACE_OUTER_BOUND('',#17740,.T.);
#11937=FACE_OUTER_BOUND('',#17741,.T.);
#11938=FACE_OUTER_BOUND('',#17742,.T.);
#11939=FACE_OUTER_BOUND('',#17743,.T.);
#11940=FACE_OUTER_BOUND('',#17744,.T.);
#11941=FACE_OUTER_BOUND('',#17745,.T.);
#11942=FACE_OUTER_BOUND('',#17746,.T.);
#11943=FACE_OUTER_BOUND('',#17747,.T.);
#11944=FACE_OUTER_BOUND('',#17748,.T.);
#11945=FACE_OUTER_BOUND('',#17749,.T.);
#11946=FACE_OUTER_BOUND('',#17750,.T.);
#11947=FACE_OUTER_BOUND('',#17751,.T.);
#11948=FACE_OUTER_BOUND('',#17752,.T.);
#11949=FACE_OUTER_BOUND('',#17753,.T.);
#11950=FACE_OUTER_BOUND('',#17754,.T.);
#11951=FACE_OUTER_BOUND('',#17755,.T.);
#11952=FACE_OUTER_BOUND('',#17756,.T.);
#11953=FACE_OUTER_BOUND('',#17757,.T.);
#11954=FACE_OUTER_BOUND('',#17758,.T.);
#11955=FACE_OUTER_BOUND('',#17759,.T.);
#11956=FACE_OUTER_BOUND('',#17760,.T.);
#11957=FACE_OUTER_BOUND('',#17761,.T.);
#11958=FACE_OUTER_BOUND('',#17762,.T.);
#11959=FACE_OUTER_BOUND('',#17763,.T.);
#11960=FACE_OUTER_BOUND('',#17764,.T.);
#11961=FACE_OUTER_BOUND('',#17765,.T.);
#11962=FACE_OUTER_BOUND('',#17766,.T.);
#11963=FACE_OUTER_BOUND('',#17767,.T.);
#11964=FACE_OUTER_BOUND('',#17768,.T.);
#11965=FACE_OUTER_BOUND('',#17769,.T.);
#11966=FACE_OUTER_BOUND('',#17770,.T.);
#11967=FACE_OUTER_BOUND('',#17771,.T.);
#11968=FACE_OUTER_BOUND('',#17772,.T.);
#11969=FACE_OUTER_BOUND('',#17773,.T.);
#11970=FACE_OUTER_BOUND('',#17774,.T.);
#11971=FACE_OUTER_BOUND('',#17775,.T.);
#11972=FACE_OUTER_BOUND('',#17776,.T.);
#11973=FACE_OUTER_BOUND('',#17777,.T.);
#11974=FACE_OUTER_BOUND('',#17778,.T.);
#11975=FACE_OUTER_BOUND('',#17779,.T.);
#11976=FACE_OUTER_BOUND('',#17780,.T.);
#11977=FACE_OUTER_BOUND('',#17781,.T.);
#11978=FACE_OUTER_BOUND('',#17782,.T.);
#11979=FACE_OUTER_BOUND('',#17783,.T.);
#11980=FACE_OUTER_BOUND('',#17784,.T.);
#11981=FACE_OUTER_BOUND('',#17785,.T.);
#11982=FACE_OUTER_BOUND('',#17786,.T.);
#11983=FACE_OUTER_BOUND('',#17787,.T.);
#11984=FACE_OUTER_BOUND('',#17788,.T.);
#11985=FACE_OUTER_BOUND('',#17789,.T.);
#11986=FACE_OUTER_BOUND('',#17790,.T.);
#11987=FACE_OUTER_BOUND('',#17791,.T.);
#11988=FACE_OUTER_BOUND('',#17792,.T.);
#11989=FACE_OUTER_BOUND('',#17793,.T.);
#11990=FACE_OUTER_BOUND('',#17794,.T.);
#11991=FACE_OUTER_BOUND('',#17795,.T.);
#11992=FACE_OUTER_BOUND('',#17796,.T.);
#11993=FACE_OUTER_BOUND('',#17797,.T.);
#11994=FACE_OUTER_BOUND('',#17798,.T.);
#11995=FACE_OUTER_BOUND('',#17799,.T.);
#11996=FACE_OUTER_BOUND('',#17800,.T.);
#11997=FACE_OUTER_BOUND('',#17801,.T.);
#11998=FACE_OUTER_BOUND('',#17802,.T.);
#11999=FACE_OUTER_BOUND('',#17803,.T.);
#12000=FACE_OUTER_BOUND('',#17804,.T.);
#12001=FACE_OUTER_BOUND('',#17805,.T.);
#12002=FACE_OUTER_BOUND('',#17806,.T.);
#12003=FACE_OUTER_BOUND('',#17807,.T.);
#12004=FACE_OUTER_BOUND('',#17808,.T.);
#12005=FACE_OUTER_BOUND('',#17809,.T.);
#12006=FACE_OUTER_BOUND('',#17810,.T.);
#12007=FACE_OUTER_BOUND('',#17811,.T.);
#12008=FACE_OUTER_BOUND('',#17812,.T.);
#12009=FACE_OUTER_BOUND('',#17813,.T.);
#12010=FACE_OUTER_BOUND('',#17814,.T.);
#12011=FACE_OUTER_BOUND('',#17815,.T.);
#12012=FACE_OUTER_BOUND('',#17816,.T.);
#12013=FACE_OUTER_BOUND('',#17817,.T.);
#12014=FACE_OUTER_BOUND('',#17818,.T.);
#12015=FACE_OUTER_BOUND('',#17819,.T.);
#12016=FACE_OUTER_BOUND('',#17820,.T.);
#12017=FACE_OUTER_BOUND('',#17821,.T.);
#12018=FACE_OUTER_BOUND('',#17822,.T.);
#12019=FACE_OUTER_BOUND('',#17823,.T.);
#12020=FACE_OUTER_BOUND('',#17824,.T.);
#12021=FACE_OUTER_BOUND('',#17825,.T.);
#12022=FACE_OUTER_BOUND('',#17826,.T.);
#12023=FACE_OUTER_BOUND('',#17827,.T.);
#12024=FACE_OUTER_BOUND('',#17828,.T.);
#12025=FACE_OUTER_BOUND('',#17829,.T.);
#12026=FACE_OUTER_BOUND('',#17830,.T.);
#12027=FACE_OUTER_BOUND('',#17831,.T.);
#12028=FACE_OUTER_BOUND('',#17832,.T.);
#12029=FACE_OUTER_BOUND('',#17833,.T.);
#12030=FACE_OUTER_BOUND('',#17834,.T.);
#12031=FACE_OUTER_BOUND('',#17835,.T.);
#12032=FACE_OUTER_BOUND('',#17836,.T.);
#12033=FACE_OUTER_BOUND('',#17837,.T.);
#12034=FACE_OUTER_BOUND('',#17838,.T.);
#12035=FACE_OUTER_BOUND('',#17839,.T.);
#12036=FACE_OUTER_BOUND('',#17840,.T.);
#12037=FACE_OUTER_BOUND('',#17841,.T.);
#12038=FACE_OUTER_BOUND('',#17842,.T.);
#12039=FACE_OUTER_BOUND('',#17843,.T.);
#12040=FACE_OUTER_BOUND('',#17844,.T.);
#12041=FACE_OUTER_BOUND('',#17845,.T.);
#12042=FACE_OUTER_BOUND('',#17846,.T.);
#12043=FACE_OUTER_BOUND('',#17847,.T.);
#12044=FACE_OUTER_BOUND('',#17848,.T.);
#12045=FACE_OUTER_BOUND('',#17849,.T.);
#12046=FACE_OUTER_BOUND('',#17850,.T.);
#12047=FACE_OUTER_BOUND('',#17851,.T.);
#12048=FACE_OUTER_BOUND('',#17852,.T.);
#12049=FACE_OUTER_BOUND('',#17853,.T.);
#12050=FACE_OUTER_BOUND('',#17854,.T.);
#12051=FACE_OUTER_BOUND('',#17855,.T.);
#12052=FACE_OUTER_BOUND('',#17856,.T.);
#12053=FACE_OUTER_BOUND('',#17857,.T.);
#12054=FACE_OUTER_BOUND('',#17858,.T.);
#12055=FACE_OUTER_BOUND('',#17859,.T.);
#12056=FACE_OUTER_BOUND('',#17860,.T.);
#12057=FACE_OUTER_BOUND('',#17861,.T.);
#12058=FACE_OUTER_BOUND('',#17862,.T.);
#12059=FACE_OUTER_BOUND('',#17863,.T.);
#12060=FACE_OUTER_BOUND('',#17864,.T.);
#12061=FACE_OUTER_BOUND('',#17865,.T.);
#12062=FACE_OUTER_BOUND('',#17866,.T.);
#12063=FACE_OUTER_BOUND('',#17867,.T.);
#12064=FACE_OUTER_BOUND('',#17868,.T.);
#12065=FACE_OUTER_BOUND('',#17869,.T.);
#12066=FACE_OUTER_BOUND('',#17870,.T.);
#12067=FACE_OUTER_BOUND('',#17871,.T.);
#12068=FACE_OUTER_BOUND('',#17872,.T.);
#12069=FACE_OUTER_BOUND('',#17873,.T.);
#12070=FACE_OUTER_BOUND('',#17874,.T.);
#12071=FACE_OUTER_BOUND('',#17875,.T.);
#12072=FACE_OUTER_BOUND('',#17876,.T.);
#12073=FACE_OUTER_BOUND('',#17877,.T.);
#12074=FACE_OUTER_BOUND('',#17878,.T.);
#12075=FACE_OUTER_BOUND('',#17879,.T.);
#12076=FACE_OUTER_BOUND('',#17880,.T.);
#12077=FACE_OUTER_BOUND('',#17881,.T.);
#12078=FACE_OUTER_BOUND('',#17882,.T.);
#12079=FACE_OUTER_BOUND('',#17883,.T.);
#12080=FACE_OUTER_BOUND('',#17884,.T.);
#12081=FACE_OUTER_BOUND('',#17885,.T.);
#12082=FACE_OUTER_BOUND('',#17886,.T.);
#12083=FACE_OUTER_BOUND('',#17887,.T.);
#12084=FACE_OUTER_BOUND('',#17888,.T.);
#12085=FACE_OUTER_BOUND('',#17889,.T.);
#12086=FACE_OUTER_BOUND('',#17890,.T.);
#12087=FACE_OUTER_BOUND('',#17891,.T.);
#12088=FACE_OUTER_BOUND('',#17892,.T.);
#12089=FACE_OUTER_BOUND('',#17893,.T.);
#12090=FACE_OUTER_BOUND('',#17894,.T.);
#12091=FACE_OUTER_BOUND('',#17895,.T.);
#12092=FACE_OUTER_BOUND('',#17896,.T.);
#12093=FACE_OUTER_BOUND('',#17897,.T.);
#12094=FACE_OUTER_BOUND('',#17898,.T.);
#12095=FACE_OUTER_BOUND('',#17899,.T.);
#12096=FACE_OUTER_BOUND('',#17900,.T.);
#12097=FACE_OUTER_BOUND('',#17901,.T.);
#12098=FACE_OUTER_BOUND('',#17902,.T.);
#12099=FACE_OUTER_BOUND('',#17903,.T.);
#12100=FACE_OUTER_BOUND('',#17904,.T.);
#12101=FACE_OUTER_BOUND('',#17905,.T.);
#12102=FACE_OUTER_BOUND('',#17906,.T.);
#12103=FACE_OUTER_BOUND('',#17907,.T.);
#12104=FACE_OUTER_BOUND('',#17908,.T.);
#12105=FACE_OUTER_BOUND('',#17909,.T.);
#12106=FACE_OUTER_BOUND('',#17910,.T.);
#12107=FACE_OUTER_BOUND('',#17911,.T.);
#12108=FACE_OUTER_BOUND('',#17912,.T.);
#12109=FACE_OUTER_BOUND('',#17913,.T.);
#12110=FACE_OUTER_BOUND('',#17914,.T.);
#12111=FACE_OUTER_BOUND('',#17915,.T.);
#12112=FACE_OUTER_BOUND('',#17916,.T.);
#12113=FACE_OUTER_BOUND('',#17917,.T.);
#12114=FACE_OUTER_BOUND('',#17918,.T.);
#12115=FACE_OUTER_BOUND('',#17919,.T.);
#12116=FACE_OUTER_BOUND('',#17920,.T.);
#12117=FACE_OUTER_BOUND('',#17921,.T.);
#12118=FACE_OUTER_BOUND('',#17922,.T.);
#12119=FACE_OUTER_BOUND('',#17923,.T.);
#12120=FACE_OUTER_BOUND('',#17924,.T.);
#12121=FACE_OUTER_BOUND('',#17925,.T.);
#12122=FACE_OUTER_BOUND('',#17926,.T.);
#12123=FACE_OUTER_BOUND('',#17927,.T.);
#12124=FACE_OUTER_BOUND('',#17928,.T.);
#12125=FACE_OUTER_BOUND('',#17929,.T.);
#12126=FACE_OUTER_BOUND('',#17930,.T.);
#12127=FACE_OUTER_BOUND('',#17931,.T.);
#12128=FACE_OUTER_BOUND('',#17932,.T.);
#12129=FACE_OUTER_BOUND('',#17933,.T.);
#12130=FACE_OUTER_BOUND('',#17934,.T.);
#12131=FACE_OUTER_BOUND('',#17935,.T.);
#12132=FACE_OUTER_BOUND('',#17936,.T.);
#12133=FACE_OUTER_BOUND('',#17937,.T.);
#12134=FACE_OUTER_BOUND('',#17938,.T.);
#12135=FACE_OUTER_BOUND('',#17939,.T.);
#12136=FACE_OUTER_BOUND('',#17940,.T.);
#12137=FACE_OUTER_BOUND('',#17941,.T.);
#12138=FACE_OUTER_BOUND('',#17942,.T.);
#12139=FACE_OUTER_BOUND('',#17943,.T.);
#12140=FACE_OUTER_BOUND('',#17944,.T.);
#12141=FACE_OUTER_BOUND('',#17945,.T.);
#12142=FACE_OUTER_BOUND('',#17946,.T.);
#12143=FACE_OUTER_BOUND('',#17947,.T.);
#12144=FACE_OUTER_BOUND('',#17948,.T.);
#12145=FACE_OUTER_BOUND('',#17949,.T.);
#12146=FACE_OUTER_BOUND('',#17950,.T.);
#12147=FACE_OUTER_BOUND('',#17951,.T.);
#12148=FACE_OUTER_BOUND('',#17952,.T.);
#12149=FACE_OUTER_BOUND('',#17953,.T.);
#12150=FACE_OUTER_BOUND('',#17954,.T.);
#12151=FACE_OUTER_BOUND('',#17955,.T.);
#12152=FACE_OUTER_BOUND('',#17956,.T.);
#12153=FACE_OUTER_BOUND('',#17957,.T.);
#12154=FACE_OUTER_BOUND('',#17958,.T.);
#12155=FACE_OUTER_BOUND('',#17959,.T.);
#12156=FACE_OUTER_BOUND('',#17960,.T.);
#12157=FACE_OUTER_BOUND('',#17961,.T.);
#12158=FACE_OUTER_BOUND('',#17962,.T.);
#12159=FACE_OUTER_BOUND('',#17963,.T.);
#12160=FACE_OUTER_BOUND('',#17964,.T.);
#12161=FACE_OUTER_BOUND('',#17965,.T.);
#12162=FACE_OUTER_BOUND('',#17966,.T.);
#12163=FACE_OUTER_BOUND('',#17967,.T.);
#12164=FACE_OUTER_BOUND('',#17968,.T.);
#12165=FACE_OUTER_BOUND('',#17969,.T.);
#12166=FACE_OUTER_BOUND('',#17970,.T.);
#12167=FACE_OUTER_BOUND('',#17971,.T.);
#12168=FACE_OUTER_BOUND('',#17972,.T.);
#12169=FACE_OUTER_BOUND('',#17973,.T.);
#12170=FACE_OUTER_BOUND('',#17974,.T.);
#12171=FACE_OUTER_BOUND('',#17975,.T.);
#12172=FACE_OUTER_BOUND('',#17976,.T.);
#12173=FACE_OUTER_BOUND('',#17977,.T.);
#12174=FACE_OUTER_BOUND('',#17978,.T.);
#12175=FACE_OUTER_BOUND('',#17979,.T.);
#12176=FACE_OUTER_BOUND('',#17980,.T.);
#12177=FACE_OUTER_BOUND('',#17981,.T.);
#12178=FACE_OUTER_BOUND('',#17982,.T.);
#12179=FACE_OUTER_BOUND('',#17983,.T.);
#12180=FACE_OUTER_BOUND('',#17984,.T.);
#12181=FACE_OUTER_BOUND('',#17985,.T.);
#12182=FACE_OUTER_BOUND('',#17986,.T.);
#12183=FACE_OUTER_BOUND('',#17987,.T.);
#12184=FACE_OUTER_BOUND('',#17988,.T.);
#12185=FACE_OUTER_BOUND('',#17989,.T.);
#12186=FACE_OUTER_BOUND('',#17990,.T.);
#12187=FACE_OUTER_BOUND('',#17991,.T.);
#12188=FACE_OUTER_BOUND('',#17992,.T.);
#12189=FACE_OUTER_BOUND('',#17993,.T.);
#12190=FACE_OUTER_BOUND('',#17994,.T.);
#12191=FACE_OUTER_BOUND('',#17995,.T.);
#12192=FACE_OUTER_BOUND('',#17996,.T.);
#12193=FACE_OUTER_BOUND('',#17997,.T.);
#12194=FACE_OUTER_BOUND('',#17998,.T.);
#12195=FACE_OUTER_BOUND('',#17999,.T.);
#12196=FACE_OUTER_BOUND('',#18000,.T.);
#12197=FACE_OUTER_BOUND('',#18001,.T.);
#12198=FACE_OUTER_BOUND('',#18002,.T.);
#12199=FACE_OUTER_BOUND('',#18003,.T.);
#12200=FACE_OUTER_BOUND('',#18004,.T.);
#12201=FACE_OUTER_BOUND('',#18005,.T.);
#12202=FACE_OUTER_BOUND('',#18006,.T.);
#12203=FACE_OUTER_BOUND('',#18007,.T.);
#12204=FACE_OUTER_BOUND('',#18008,.T.);
#12205=FACE_OUTER_BOUND('',#18009,.T.);
#12206=FACE_OUTER_BOUND('',#18010,.T.);
#12207=FACE_OUTER_BOUND('',#18011,.T.);
#12208=FACE_OUTER_BOUND('',#18012,.T.);
#12209=FACE_OUTER_BOUND('',#18013,.T.);
#12210=FACE_OUTER_BOUND('',#18014,.T.);
#12211=FACE_OUTER_BOUND('',#18015,.T.);
#12212=FACE_OUTER_BOUND('',#18016,.T.);
#12213=FACE_OUTER_BOUND('',#18017,.T.);
#12214=FACE_OUTER_BOUND('',#18018,.T.);
#12215=FACE_OUTER_BOUND('',#18019,.T.);
#12216=FACE_OUTER_BOUND('',#18020,.T.);
#12217=FACE_OUTER_BOUND('',#18021,.T.);
#12218=FACE_OUTER_BOUND('',#18022,.T.);
#12219=FACE_OUTER_BOUND('',#18023,.T.);
#12220=FACE_OUTER_BOUND('',#18024,.T.);
#12221=FACE_OUTER_BOUND('',#18025,.T.);
#12222=FACE_OUTER_BOUND('',#18026,.T.);
#12223=FACE_OUTER_BOUND('',#18027,.T.);
#12224=FACE_OUTER_BOUND('',#18028,.T.);
#12225=FACE_OUTER_BOUND('',#18029,.T.);
#12226=FACE_OUTER_BOUND('',#18030,.T.);
#12227=FACE_OUTER_BOUND('',#18031,.T.);
#12228=FACE_OUTER_BOUND('',#18032,.T.);
#12229=FACE_OUTER_BOUND('',#18033,.T.);
#12230=FACE_OUTER_BOUND('',#18034,.T.);
#12231=FACE_OUTER_BOUND('',#18035,.T.);
#12232=FACE_OUTER_BOUND('',#18036,.T.);
#12233=FACE_OUTER_BOUND('',#18037,.T.);
#12234=FACE_OUTER_BOUND('',#18038,.T.);
#12235=FACE_OUTER_BOUND('',#18039,.T.);
#12236=FACE_OUTER_BOUND('',#18040,.T.);
#12237=FACE_OUTER_BOUND('',#18041,.T.);
#12238=FACE_OUTER_BOUND('',#18042,.T.);
#12239=FACE_OUTER_BOUND('',#18043,.T.);
#12240=FACE_OUTER_BOUND('',#18044,.T.);
#12241=FACE_OUTER_BOUND('',#18045,.T.);
#12242=FACE_OUTER_BOUND('',#18046,.T.);
#12243=FACE_OUTER_BOUND('',#18047,.T.);
#12244=FACE_OUTER_BOUND('',#18048,.T.);
#12245=FACE_OUTER_BOUND('',#18049,.T.);
#12246=FACE_OUTER_BOUND('',#18050,.T.);
#12247=FACE_OUTER_BOUND('',#18051,.T.);
#12248=FACE_OUTER_BOUND('',#18052,.T.);
#12249=FACE_OUTER_BOUND('',#18053,.T.);
#12250=FACE_OUTER_BOUND('',#18054,.T.);
#12251=FACE_OUTER_BOUND('',#18055,.T.);
#12252=FACE_OUTER_BOUND('',#18056,.T.);
#12253=FACE_OUTER_BOUND('',#18057,.T.);
#12254=FACE_OUTER_BOUND('',#18058,.T.);
#12255=FACE_OUTER_BOUND('',#18059,.T.);
#12256=FACE_OUTER_BOUND('',#18060,.T.);
#12257=FACE_OUTER_BOUND('',#18061,.T.);
#12258=FACE_OUTER_BOUND('',#18062,.T.);
#12259=FACE_OUTER_BOUND('',#18063,.T.);
#12260=FACE_OUTER_BOUND('',#18064,.T.);
#12261=FACE_OUTER_BOUND('',#18065,.T.);
#12262=FACE_OUTER_BOUND('',#18066,.T.);
#12263=FACE_OUTER_BOUND('',#18067,.T.);
#12264=FACE_OUTER_BOUND('',#18068,.T.);
#12265=FACE_OUTER_BOUND('',#18069,.T.);
#12266=FACE_OUTER_BOUND('',#18070,.T.);
#12267=FACE_OUTER_BOUND('',#18071,.T.);
#12268=FACE_OUTER_BOUND('',#18072,.T.);
#12269=FACE_OUTER_BOUND('',#18073,.T.);
#12270=FACE_OUTER_BOUND('',#18074,.T.);
#12271=FACE_OUTER_BOUND('',#18075,.T.);
#12272=FACE_OUTER_BOUND('',#18076,.T.);
#12273=FACE_OUTER_BOUND('',#18077,.T.);
#12274=FACE_OUTER_BOUND('',#18078,.T.);
#12275=FACE_OUTER_BOUND('',#18079,.T.);
#12276=FACE_OUTER_BOUND('',#18080,.T.);
#12277=FACE_OUTER_BOUND('',#18081,.T.);
#12278=FACE_OUTER_BOUND('',#18082,.T.);
#12279=FACE_OUTER_BOUND('',#18083,.T.);
#12280=FACE_OUTER_BOUND('',#18084,.T.);
#12281=FACE_OUTER_BOUND('',#18085,.T.);
#12282=FACE_OUTER_BOUND('',#18086,.T.);
#12283=FACE_OUTER_BOUND('',#18087,.T.);
#12284=FACE_OUTER_BOUND('',#18088,.T.);
#12285=FACE_OUTER_BOUND('',#18089,.T.);
#12286=FACE_OUTER_BOUND('',#18090,.T.);
#12287=FACE_OUTER_BOUND('',#18091,.T.);
#12288=FACE_OUTER_BOUND('',#18092,.T.);
#12289=FACE_OUTER_BOUND('',#18093,.T.);
#12290=FACE_OUTER_BOUND('',#18094,.T.);
#12291=FACE_OUTER_BOUND('',#18095,.T.);
#12292=FACE_OUTER_BOUND('',#18096,.T.);
#12293=FACE_OUTER_BOUND('',#18097,.T.);
#12294=FACE_OUTER_BOUND('',#18098,.T.);
#12295=FACE_OUTER_BOUND('',#18099,.T.);
#12296=FACE_OUTER_BOUND('',#18100,.T.);
#12297=FACE_OUTER_BOUND('',#18101,.T.);
#12298=FACE_OUTER_BOUND('',#18102,.T.);
#12299=FACE_OUTER_BOUND('',#18103,.T.);
#12300=FACE_OUTER_BOUND('',#18104,.T.);
#12301=FACE_OUTER_BOUND('',#18105,.T.);
#12302=FACE_OUTER_BOUND('',#18106,.T.);
#12303=FACE_OUTER_BOUND('',#18107,.T.);
#12304=FACE_OUTER_BOUND('',#18108,.T.);
#12305=FACE_OUTER_BOUND('',#18109,.T.);
#12306=FACE_OUTER_BOUND('',#18110,.T.);
#12307=FACE_OUTER_BOUND('',#18111,.T.);
#12308=FACE_OUTER_BOUND('',#18112,.T.);
#12309=FACE_OUTER_BOUND('',#18113,.T.);
#12310=FACE_OUTER_BOUND('',#18114,.T.);
#12311=FACE_OUTER_BOUND('',#18115,.T.);
#12312=FACE_OUTER_BOUND('',#18116,.T.);
#12313=FACE_OUTER_BOUND('',#18117,.T.);
#12314=FACE_OUTER_BOUND('',#18118,.T.);
#12315=FACE_OUTER_BOUND('',#18119,.T.);
#12316=FACE_OUTER_BOUND('',#18120,.T.);
#12317=FACE_OUTER_BOUND('',#18121,.T.);
#12318=FACE_OUTER_BOUND('',#18122,.T.);
#12319=FACE_OUTER_BOUND('',#18123,.T.);
#12320=FACE_OUTER_BOUND('',#18124,.T.);
#12321=FACE_OUTER_BOUND('',#18125,.T.);
#12322=FACE_OUTER_BOUND('',#18126,.T.);
#12323=FACE_OUTER_BOUND('',#18127,.T.);
#12324=FACE_OUTER_BOUND('',#18128,.T.);
#12325=FACE_OUTER_BOUND('',#18129,.T.);
#12326=FACE_OUTER_BOUND('',#18130,.T.);
#12327=FACE_OUTER_BOUND('',#18131,.T.);
#12328=FACE_OUTER_BOUND('',#18132,.T.);
#12329=FACE_OUTER_BOUND('',#18133,.T.);
#12330=FACE_OUTER_BOUND('',#18134,.T.);
#12331=FACE_OUTER_BOUND('',#18135,.T.);
#12332=FACE_OUTER_BOUND('',#18136,.T.);
#12333=FACE_OUTER_BOUND('',#18137,.T.);
#12334=FACE_OUTER_BOUND('',#18138,.T.);
#12335=FACE_OUTER_BOUND('',#18139,.T.);
#12336=FACE_OUTER_BOUND('',#18140,.T.);
#12337=FACE_OUTER_BOUND('',#18141,.T.);
#12338=FACE_OUTER_BOUND('',#18142,.T.);
#12339=FACE_OUTER_BOUND('',#18143,.T.);
#12340=FACE_OUTER_BOUND('',#18144,.T.);
#12341=FACE_OUTER_BOUND('',#18145,.T.);
#12342=FACE_OUTER_BOUND('',#18146,.T.);
#12343=FACE_OUTER_BOUND('',#18147,.T.);
#12344=FACE_OUTER_BOUND('',#18148,.T.);
#12345=FACE_OUTER_BOUND('',#18149,.T.);
#12346=FACE_OUTER_BOUND('',#18150,.T.);
#12347=FACE_OUTER_BOUND('',#18151,.T.);
#12348=FACE_OUTER_BOUND('',#18152,.T.);
#12349=FACE_OUTER_BOUND('',#18153,.T.);
#12350=FACE_OUTER_BOUND('',#18154,.T.);
#12351=FACE_OUTER_BOUND('',#18155,.T.);
#12352=FACE_OUTER_BOUND('',#18156,.T.);
#12353=FACE_OUTER_BOUND('',#18157,.T.);
#12354=FACE_OUTER_BOUND('',#18158,.T.);
#12355=FACE_OUTER_BOUND('',#18159,.T.);
#12356=FACE_OUTER_BOUND('',#18160,.T.);
#12357=FACE_OUTER_BOUND('',#18161,.T.);
#12358=FACE_OUTER_BOUND('',#18162,.T.);
#12359=FACE_OUTER_BOUND('',#18163,.T.);
#12360=FACE_OUTER_BOUND('',#18164,.T.);
#12361=FACE_OUTER_BOUND('',#18165,.T.);
#12362=FACE_OUTER_BOUND('',#18166,.T.);
#12363=FACE_OUTER_BOUND('',#18167,.T.);
#12364=FACE_OUTER_BOUND('',#18168,.T.);
#12365=FACE_OUTER_BOUND('',#18169,.T.);
#12366=FACE_OUTER_BOUND('',#18170,.T.);
#12367=FACE_OUTER_BOUND('',#18171,.T.);
#12368=FACE_OUTER_BOUND('',#18172,.T.);
#12369=FACE_OUTER_BOUND('',#18173,.T.);
#12370=FACE_OUTER_BOUND('',#18174,.T.);
#12371=FACE_OUTER_BOUND('',#18175,.T.);
#12372=FACE_OUTER_BOUND('',#18176,.T.);
#12373=FACE_OUTER_BOUND('',#18177,.T.);
#12374=FACE_OUTER_BOUND('',#18178,.T.);
#12375=FACE_OUTER_BOUND('',#18179,.T.);
#12376=FACE_OUTER_BOUND('',#18180,.T.);
#12377=FACE_OUTER_BOUND('',#18181,.T.);
#12378=FACE_OUTER_BOUND('',#18182,.T.);
#12379=FACE_OUTER_BOUND('',#18183,.T.);
#12380=FACE_OUTER_BOUND('',#18184,.T.);
#12381=FACE_OUTER_BOUND('',#18185,.T.);
#12382=FACE_OUTER_BOUND('',#18186,.T.);
#12383=FACE_OUTER_BOUND('',#18187,.T.);
#12384=FACE_OUTER_BOUND('',#18188,.T.);
#12385=FACE_OUTER_BOUND('',#18189,.T.);
#12386=FACE_OUTER_BOUND('',#18190,.T.);
#12387=FACE_OUTER_BOUND('',#18191,.T.);
#12388=FACE_OUTER_BOUND('',#18192,.T.);
#12389=FACE_OUTER_BOUND('',#18193,.T.);
#12390=FACE_OUTER_BOUND('',#18194,.T.);
#12391=FACE_OUTER_BOUND('',#18195,.T.);
#12392=FACE_OUTER_BOUND('',#18196,.T.);
#12393=FACE_OUTER_BOUND('',#18197,.T.);
#12394=FACE_OUTER_BOUND('',#18198,.T.);
#12395=FACE_OUTER_BOUND('',#18199,.T.);
#12396=FACE_OUTER_BOUND('',#18200,.T.);
#12397=FACE_OUTER_BOUND('',#18201,.T.);
#12398=FACE_OUTER_BOUND('',#18202,.T.);
#12399=FACE_OUTER_BOUND('',#18203,.T.);
#12400=FACE_OUTER_BOUND('',#18204,.T.);
#12401=FACE_OUTER_BOUND('',#18205,.T.);
#12402=FACE_OUTER_BOUND('',#18206,.T.);
#12403=FACE_OUTER_BOUND('',#18207,.T.);
#12404=FACE_OUTER_BOUND('',#18208,.T.);
#12405=FACE_OUTER_BOUND('',#18209,.T.);
#12406=FACE_OUTER_BOUND('',#18210,.T.);
#12407=FACE_OUTER_BOUND('',#18211,.T.);
#12408=FACE_OUTER_BOUND('',#18212,.T.);
#12409=FACE_OUTER_BOUND('',#18213,.T.);
#12410=FACE_OUTER_BOUND('',#18214,.T.);
#12411=FACE_OUTER_BOUND('',#18215,.T.);
#12412=FACE_OUTER_BOUND('',#18216,.T.);
#12413=FACE_OUTER_BOUND('',#18217,.T.);
#12414=FACE_OUTER_BOUND('',#18218,.T.);
#12415=FACE_OUTER_BOUND('',#18219,.T.);
#12416=FACE_OUTER_BOUND('',#18220,.T.);
#12417=FACE_OUTER_BOUND('',#18221,.T.);
#12418=FACE_OUTER_BOUND('',#18222,.T.);
#12419=FACE_OUTER_BOUND('',#18223,.T.);
#12420=FACE_OUTER_BOUND('',#18224,.T.);
#12421=FACE_OUTER_BOUND('',#18225,.T.);
#12422=FACE_OUTER_BOUND('',#18226,.T.);
#12423=FACE_OUTER_BOUND('',#18227,.T.);
#12424=FACE_OUTER_BOUND('',#18228,.T.);
#12425=FACE_OUTER_BOUND('',#18229,.T.);
#12426=FACE_OUTER_BOUND('',#18230,.T.);
#12427=FACE_OUTER_BOUND('',#18231,.T.);
#12428=FACE_OUTER_BOUND('',#18232,.T.);
#12429=FACE_OUTER_BOUND('',#18233,.T.);
#12430=FACE_OUTER_BOUND('',#18234,.T.);
#12431=FACE_OUTER_BOUND('',#18235,.T.);
#12432=FACE_OUTER_BOUND('',#18236,.T.);
#12433=FACE_OUTER_BOUND('',#18237,.T.);
#12434=FACE_OUTER_BOUND('',#18238,.T.);
#12435=FACE_OUTER_BOUND('',#18239,.T.);
#12436=FACE_OUTER_BOUND('',#18240,.T.);
#12437=FACE_OUTER_BOUND('',#18241,.T.);
#12438=FACE_OUTER_BOUND('',#18242,.T.);
#12439=FACE_OUTER_BOUND('',#18243,.T.);
#12440=FACE_OUTER_BOUND('',#18244,.T.);
#12441=FACE_OUTER_BOUND('',#18245,.T.);
#12442=FACE_OUTER_BOUND('',#18246,.T.);
#12443=FACE_OUTER_BOUND('',#18247,.T.);
#12444=FACE_OUTER_BOUND('',#18248,.T.);
#12445=FACE_OUTER_BOUND('',#18249,.T.);
#12446=FACE_OUTER_BOUND('',#18250,.T.);
#12447=FACE_OUTER_BOUND('',#18251,.T.);
#12448=FACE_OUTER_BOUND('',#18252,.T.);
#12449=FACE_OUTER_BOUND('',#18253,.T.);
#12450=FACE_OUTER_BOUND('',#18254,.T.);
#12451=FACE_OUTER_BOUND('',#18255,.T.);
#12452=FACE_OUTER_BOUND('',#18256,.T.);
#12453=FACE_OUTER_BOUND('',#18257,.T.);
#12454=FACE_OUTER_BOUND('',#18258,.T.);
#12455=FACE_OUTER_BOUND('',#18259,.T.);
#12456=FACE_OUTER_BOUND('',#18260,.T.);
#12457=FACE_OUTER_BOUND('',#18261,.T.);
#12458=FACE_OUTER_BOUND('',#18262,.T.);
#12459=FACE_OUTER_BOUND('',#18263,.T.);
#12460=FACE_OUTER_BOUND('',#18264,.T.);
#12461=FACE_OUTER_BOUND('',#18265,.T.);
#12462=FACE_OUTER_BOUND('',#18266,.T.);
#12463=FACE_OUTER_BOUND('',#18267,.T.);
#12464=FACE_OUTER_BOUND('',#18268,.T.);
#12465=FACE_OUTER_BOUND('',#18269,.T.);
#12466=FACE_OUTER_BOUND('',#18270,.T.);
#12467=FACE_OUTER_BOUND('',#18271,.T.);
#12468=FACE_OUTER_BOUND('',#18272,.T.);
#12469=FACE_OUTER_BOUND('',#18273,.T.);
#12470=FACE_OUTER_BOUND('',#18274,.T.);
#12471=FACE_OUTER_BOUND('',#18275,.T.);
#12472=FACE_OUTER_BOUND('',#18276,.T.);
#12473=FACE_OUTER_BOUND('',#18277,.T.);
#12474=FACE_OUTER_BOUND('',#18278,.T.);
#12475=FACE_OUTER_BOUND('',#18279,.T.);
#12476=FACE_OUTER_BOUND('',#18281,.T.);
#12477=FACE_OUTER_BOUND('',#18282,.T.);
#12478=FACE_OUTER_BOUND('',#18283,.T.);
#12479=FACE_OUTER_BOUND('',#18284,.T.);
#12480=FACE_OUTER_BOUND('',#18285,.T.);
#12481=FACE_OUTER_BOUND('',#18286,.T.);
#12482=FACE_OUTER_BOUND('',#18287,.T.);
#12483=FACE_OUTER_BOUND('',#18288,.T.);
#12484=FACE_OUTER_BOUND('',#18289,.T.);
#12485=FACE_OUTER_BOUND('',#18290,.T.);
#12486=FACE_OUTER_BOUND('',#18291,.T.);
#12487=FACE_OUTER_BOUND('',#18292,.T.);
#12488=FACE_OUTER_BOUND('',#18293,.T.);
#12489=FACE_OUTER_BOUND('',#18294,.T.);
#12490=FACE_OUTER_BOUND('',#18295,.T.);
#12491=FACE_OUTER_BOUND('',#18296,.T.);
#12492=FACE_OUTER_BOUND('',#18297,.T.);
#12493=FACE_OUTER_BOUND('',#18298,.T.);
#12494=FACE_OUTER_BOUND('',#18299,.T.);
#12495=FACE_OUTER_BOUND('',#18300,.T.);
#12496=FACE_OUTER_BOUND('',#18301,.T.);
#12497=FACE_OUTER_BOUND('',#18302,.T.);
#12498=FACE_OUTER_BOUND('',#18303,.T.);
#12499=FACE_OUTER_BOUND('',#18304,.T.);
#12500=FACE_OUTER_BOUND('',#18305,.T.);
#12501=FACE_OUTER_BOUND('',#18306,.T.);
#12502=FACE_OUTER_BOUND('',#18307,.T.);
#12503=FACE_OUTER_BOUND('',#18308,.T.);
#12504=FACE_OUTER_BOUND('',#18309,.T.);
#12505=FACE_OUTER_BOUND('',#18310,.T.);
#12506=FACE_OUTER_BOUND('',#18311,.T.);
#12507=FACE_OUTER_BOUND('',#18312,.T.);
#12508=FACE_OUTER_BOUND('',#18313,.T.);
#12509=FACE_OUTER_BOUND('',#18314,.T.);
#12510=FACE_OUTER_BOUND('',#18315,.T.);
#12511=FACE_OUTER_BOUND('',#18316,.T.);
#12512=FACE_OUTER_BOUND('',#18317,.T.);
#12513=FACE_OUTER_BOUND('',#18318,.T.);
#12514=FACE_OUTER_BOUND('',#18319,.T.);
#12515=FACE_OUTER_BOUND('',#18320,.T.);
#12516=FACE_OUTER_BOUND('',#18321,.T.);
#12517=FACE_OUTER_BOUND('',#18322,.T.);
#12518=FACE_OUTER_BOUND('',#18323,.T.);
#12519=FACE_OUTER_BOUND('',#18324,.T.);
#12520=FACE_OUTER_BOUND('',#18325,.T.);
#12521=FACE_OUTER_BOUND('',#18326,.T.);
#12522=FACE_OUTER_BOUND('',#18327,.T.);
#12523=FACE_OUTER_BOUND('',#18328,.T.);
#12524=FACE_OUTER_BOUND('',#18329,.T.);
#12525=FACE_OUTER_BOUND('',#18330,.T.);
#12526=FACE_OUTER_BOUND('',#18331,.T.);
#12527=FACE_OUTER_BOUND('',#18332,.T.);
#12528=FACE_OUTER_BOUND('',#18333,.T.);
#12529=FACE_OUTER_BOUND('',#18334,.T.);
#12530=FACE_OUTER_BOUND('',#18335,.T.);
#12531=FACE_OUTER_BOUND('',#18336,.T.);
#12532=FACE_OUTER_BOUND('',#18337,.T.);
#12533=FACE_OUTER_BOUND('',#18338,.T.);
#12534=FACE_OUTER_BOUND('',#18339,.T.);
#12535=FACE_OUTER_BOUND('',#18340,.T.);
#12536=FACE_OUTER_BOUND('',#18341,.T.);
#12537=FACE_OUTER_BOUND('',#18342,.T.);
#12538=FACE_OUTER_BOUND('',#18343,.T.);
#12539=FACE_OUTER_BOUND('',#18344,.T.);
#12540=FACE_OUTER_BOUND('',#18345,.T.);
#12541=FACE_OUTER_BOUND('',#18346,.T.);
#12542=FACE_OUTER_BOUND('',#18347,.T.);
#12543=FACE_OUTER_BOUND('',#18348,.T.);
#12544=FACE_OUTER_BOUND('',#18349,.T.);
#12545=FACE_OUTER_BOUND('',#18350,.T.);
#12546=FACE_OUTER_BOUND('',#18351,.T.);
#12547=FACE_OUTER_BOUND('',#18420,.T.);
#12548=FACE_OUTER_BOUND('',#18421,.T.);
#12549=FACE_OUTER_BOUND('',#18422,.T.);
#12550=FACE_OUTER_BOUND('',#18423,.T.);
#12551=FACE_OUTER_BOUND('',#18424,.T.);
#12552=FACE_OUTER_BOUND('',#18425,.T.);
#12553=FACE_OUTER_BOUND('',#18426,.T.);
#12554=FACE_OUTER_BOUND('',#18427,.T.);
#12555=FACE_OUTER_BOUND('',#18428,.T.);
#12556=FACE_OUTER_BOUND('',#18429,.T.);
#12557=FACE_OUTER_BOUND('',#18430,.T.);
#12558=FACE_OUTER_BOUND('',#18431,.T.);
#12559=FACE_OUTER_BOUND('',#18432,.T.);
#12560=FACE_OUTER_BOUND('',#18433,.T.);
#12561=FACE_OUTER_BOUND('',#18434,.T.);
#12562=FACE_OUTER_BOUND('',#18435,.T.);
#12563=FACE_OUTER_BOUND('',#18436,.T.);
#12564=FACE_OUTER_BOUND('',#18437,.T.);
#12565=FACE_OUTER_BOUND('',#18438,.T.);
#12566=FACE_OUTER_BOUND('',#18439,.T.);
#12567=FACE_OUTER_BOUND('',#18440,.T.);
#12568=FACE_OUTER_BOUND('',#18441,.T.);
#12569=FACE_OUTER_BOUND('',#18442,.T.);
#12570=FACE_OUTER_BOUND('',#18443,.T.);
#12571=FACE_OUTER_BOUND('',#18444,.T.);
#12572=FACE_OUTER_BOUND('',#18445,.T.);
#12573=FACE_OUTER_BOUND('',#18446,.T.);
#12574=FACE_OUTER_BOUND('',#18447,.T.);
#12575=FACE_OUTER_BOUND('',#18448,.T.);
#12576=FACE_OUTER_BOUND('',#18449,.T.);
#12577=FACE_OUTER_BOUND('',#18450,.T.);
#12578=FACE_OUTER_BOUND('',#18451,.T.);
#12579=FACE_OUTER_BOUND('',#18452,.T.);
#12580=FACE_OUTER_BOUND('',#18453,.T.);
#12581=FACE_OUTER_BOUND('',#18454,.T.);
#12582=FACE_OUTER_BOUND('',#18455,.T.);
#12583=FACE_OUTER_BOUND('',#18456,.T.);
#12584=FACE_OUTER_BOUND('',#18457,.T.);
#12585=FACE_OUTER_BOUND('',#18458,.T.);
#12586=FACE_OUTER_BOUND('',#18459,.T.);
#12587=FACE_OUTER_BOUND('',#18460,.T.);
#12588=FACE_OUTER_BOUND('',#18462,.T.);
#12589=FACE_OUTER_BOUND('',#18463,.T.);
#12590=FACE_OUTER_BOUND('',#18464,.T.);
#12591=FACE_OUTER_BOUND('',#18465,.T.);
#12592=FACE_OUTER_BOUND('',#18466,.T.);
#12593=FACE_OUTER_BOUND('',#18467,.T.);
#12594=FACE_OUTER_BOUND('',#18468,.T.);
#12595=FACE_OUTER_BOUND('',#18469,.T.);
#12596=FACE_OUTER_BOUND('',#18470,.T.);
#12597=FACE_OUTER_BOUND('',#18471,.T.);
#12598=FACE_OUTER_BOUND('',#18472,.T.);
#12599=FACE_OUTER_BOUND('',#18473,.T.);
#12600=FACE_OUTER_BOUND('',#18474,.T.);
#12601=FACE_OUTER_BOUND('',#18475,.T.);
#12602=FACE_OUTER_BOUND('',#18476,.T.);
#12603=FACE_OUTER_BOUND('',#18477,.T.);
#12604=FACE_OUTER_BOUND('',#18478,.T.);
#12605=FACE_OUTER_BOUND('',#18479,.T.);
#12606=FACE_OUTER_BOUND('',#18480,.T.);
#12607=FACE_OUTER_BOUND('',#18481,.T.);
#12608=FACE_OUTER_BOUND('',#18482,.T.);
#12609=FACE_OUTER_BOUND('',#18483,.T.);
#12610=FACE_OUTER_BOUND('',#18484,.T.);
#12611=FACE_OUTER_BOUND('',#18485,.T.);
#12612=FACE_OUTER_BOUND('',#18486,.T.);
#12613=FACE_OUTER_BOUND('',#18487,.T.);
#12614=FACE_OUTER_BOUND('',#18488,.T.);
#12615=FACE_OUTER_BOUND('',#18489,.T.);
#12616=FACE_OUTER_BOUND('',#18490,.T.);
#12617=FACE_OUTER_BOUND('',#18491,.T.);
#12618=FACE_OUTER_BOUND('',#18492,.T.);
#12619=FACE_OUTER_BOUND('',#18493,.T.);
#12620=FACE_OUTER_BOUND('',#18494,.T.);
#12621=FACE_OUTER_BOUND('',#18495,.T.);
#12622=FACE_OUTER_BOUND('',#18496,.T.);
#12623=FACE_OUTER_BOUND('',#18497,.T.);
#12624=FACE_OUTER_BOUND('',#18498,.T.);
#12625=FACE_OUTER_BOUND('',#18499,.T.);
#12626=FACE_OUTER_BOUND('',#18500,.T.);
#12627=FACE_OUTER_BOUND('',#18501,.T.);
#12628=FACE_OUTER_BOUND('',#18502,.T.);
#12629=FACE_OUTER_BOUND('',#18503,.T.);
#12630=FACE_OUTER_BOUND('',#18504,.T.);
#12631=FACE_OUTER_BOUND('',#18505,.T.);
#12632=FACE_OUTER_BOUND('',#18506,.T.);
#12633=FACE_OUTER_BOUND('',#18507,.T.);
#12634=FACE_OUTER_BOUND('',#18508,.T.);
#12635=FACE_OUTER_BOUND('',#18509,.T.);
#12636=FACE_OUTER_BOUND('',#18510,.T.);
#12637=FACE_OUTER_BOUND('',#18511,.T.);
#12638=FACE_OUTER_BOUND('',#18512,.T.);
#12639=FACE_OUTER_BOUND('',#18514,.T.);
#12640=FACE_OUTER_BOUND('',#18515,.T.);
#12641=FACE_OUTER_BOUND('',#18516,.T.);
#12642=FACE_OUTER_BOUND('',#18517,.T.);
#12643=FACE_OUTER_BOUND('',#18518,.T.);
#12644=FACE_OUTER_BOUND('',#18519,.T.);
#12645=FACE_OUTER_BOUND('',#18520,.T.);
#12646=FACE_OUTER_BOUND('',#18521,.T.);
#12647=FACE_OUTER_BOUND('',#18522,.T.);
#12648=FACE_OUTER_BOUND('',#18523,.T.);
#12649=FACE_OUTER_BOUND('',#18524,.T.);
#12650=FACE_OUTER_BOUND('',#18525,.T.);
#12651=FACE_OUTER_BOUND('',#18526,.T.);
#12652=FACE_OUTER_BOUND('',#18527,.T.);
#12653=FACE_OUTER_BOUND('',#18528,.T.);
#12654=FACE_OUTER_BOUND('',#18529,.T.);
#12655=FACE_OUTER_BOUND('',#18530,.T.);
#12656=FACE_OUTER_BOUND('',#18592,.T.);
#12657=FACE_OUTER_BOUND('',#18593,.T.);
#12658=FACE_OUTER_BOUND('',#18594,.T.);
#12659=FACE_OUTER_BOUND('',#18595,.T.);
#12660=FACE_OUTER_BOUND('',#18596,.T.);
#12661=FACE_OUTER_BOUND('',#18597,.T.);
#12662=FACE_OUTER_BOUND('',#18598,.T.);
#12663=FACE_OUTER_BOUND('',#18599,.T.);
#12664=FACE_OUTER_BOUND('',#18600,.T.);
#12665=FACE_OUTER_BOUND('',#18601,.T.);
#12666=FACE_OUTER_BOUND('',#18603,.T.);
#12667=FACE_OUTER_BOUND('',#18604,.T.);
#12668=FACE_OUTER_BOUND('',#18605,.T.);
#12669=FACE_OUTER_BOUND('',#18606,.T.);
#12670=FACE_OUTER_BOUND('',#18607,.T.);
#12671=FACE_OUTER_BOUND('',#18608,.T.);
#12672=FACE_OUTER_BOUND('',#18609,.T.);
#12673=FACE_OUTER_BOUND('',#18610,.T.);
#12674=FACE_OUTER_BOUND('',#18611,.T.);
#12675=FACE_OUTER_BOUND('',#18612,.T.);
#12676=FACE_OUTER_BOUND('',#18613,.T.);
#12677=FACE_OUTER_BOUND('',#18614,.T.);
#12678=FACE_OUTER_BOUND('',#18615,.T.);
#12679=FACE_OUTER_BOUND('',#18616,.T.);
#12680=FACE_OUTER_BOUND('',#18617,.T.);
#12681=FACE_OUTER_BOUND('',#18618,.T.);
#12682=FACE_OUTER_BOUND('',#18619,.T.);
#12683=FACE_OUTER_BOUND('',#18620,.T.);
#12684=FACE_OUTER_BOUND('',#18621,.T.);
#12685=FACE_OUTER_BOUND('',#18622,.T.);
#12686=FACE_OUTER_BOUND('',#18623,.T.);
#12687=FACE_OUTER_BOUND('',#18625,.T.);
#12688=FACE_OUTER_BOUND('',#18627,.T.);
#12689=FACE_OUTER_BOUND('',#18628,.T.);
#12690=FACE_OUTER_BOUND('',#18629,.T.);
#12691=FACE_OUTER_BOUND('',#18630,.T.);
#12692=FACE_OUTER_BOUND('',#18631,.T.);
#12693=FACE_OUTER_BOUND('',#18632,.T.);
#12694=FACE_OUTER_BOUND('',#18633,.T.);
#12695=FACE_OUTER_BOUND('',#18634,.T.);
#12696=FACE_OUTER_BOUND('',#18635,.T.);
#12697=FACE_OUTER_BOUND('',#18636,.T.);
#12698=FACE_OUTER_BOUND('',#18637,.T.);
#12699=FACE_OUTER_BOUND('',#18638,.T.);
#12700=FACE_OUTER_BOUND('',#18639,.T.);
#12701=FACE_OUTER_BOUND('',#18640,.T.);
#12702=FACE_OUTER_BOUND('',#18641,.T.);
#12703=FACE_OUTER_BOUND('',#18643,.T.);
#12704=FACE_OUTER_BOUND('',#18644,.T.);
#12705=FACE_OUTER_BOUND('',#18645,.T.);
#12706=FACE_OUTER_BOUND('',#18646,.T.);
#12707=FACE_OUTER_BOUND('',#18647,.T.);
#12708=FACE_OUTER_BOUND('',#18648,.T.);
#12709=FACE_OUTER_BOUND('',#18649,.T.);
#12710=FACE_OUTER_BOUND('',#18650,.T.);
#12711=FACE_OUTER_BOUND('',#18651,.T.);
#12712=FACE_OUTER_BOUND('',#18652,.T.);
#12713=FACE_OUTER_BOUND('',#18653,.T.);
#12714=FACE_OUTER_BOUND('',#18654,.T.);
#12715=FACE_OUTER_BOUND('',#18655,.T.);
#12716=FACE_OUTER_BOUND('',#18656,.T.);
#12717=FACE_OUTER_BOUND('',#18657,.T.);
#12718=FACE_OUTER_BOUND('',#18658,.T.);
#12719=FACE_OUTER_BOUND('',#18659,.T.);
#12720=FACE_OUTER_BOUND('',#18660,.T.);
#12721=FACE_OUTER_BOUND('',#18661,.T.);
#12722=FACE_OUTER_BOUND('',#18662,.T.);
#12723=FACE_OUTER_BOUND('',#18663,.T.);
#12724=FACE_OUTER_BOUND('',#18664,.T.);
#12725=FACE_OUTER_BOUND('',#18665,.T.);
#12726=FACE_OUTER_BOUND('',#18666,.T.);
#12727=FACE_OUTER_BOUND('',#18667,.T.);
#12728=FACE_OUTER_BOUND('',#18669,.T.);
#12729=FACE_OUTER_BOUND('',#18670,.T.);
#12730=FACE_OUTER_BOUND('',#18671,.T.);
#12731=FACE_OUTER_BOUND('',#18672,.T.);
#12732=FACE_OUTER_BOUND('',#18673,.T.);
#12733=FACE_OUTER_BOUND('',#18674,.T.);
#12734=FACE_OUTER_BOUND('',#18675,.T.);
#12735=FACE_OUTER_BOUND('',#18676,.T.);
#12736=FACE_OUTER_BOUND('',#18677,.T.);
#12737=FACE_OUTER_BOUND('',#18678,.T.);
#12738=FACE_OUTER_BOUND('',#18679,.T.);
#12739=FACE_OUTER_BOUND('',#18680,.T.);
#12740=FACE_OUTER_BOUND('',#18681,.T.);
#12741=FACE_OUTER_BOUND('',#18682,.T.);
#12742=FACE_OUTER_BOUND('',#18683,.T.);
#12743=FACE_OUTER_BOUND('',#18684,.T.);
#12744=FACE_OUTER_BOUND('',#18685,.T.);
#12745=FACE_OUTER_BOUND('',#18686,.T.);
#12746=FACE_OUTER_BOUND('',#18687,.T.);
#12747=FACE_OUTER_BOUND('',#18688,.T.);
#12748=FACE_OUTER_BOUND('',#18689,.T.);
#12749=FACE_OUTER_BOUND('',#18690,.T.);
#12750=FACE_OUTER_BOUND('',#18691,.T.);
#12751=FACE_OUTER_BOUND('',#18692,.T.);
#12752=FACE_OUTER_BOUND('',#18693,.T.);
#12753=FACE_OUTER_BOUND('',#18694,.T.);
#12754=FACE_OUTER_BOUND('',#18695,.T.);
#12755=FACE_OUTER_BOUND('',#18696,.T.);
#12756=FACE_OUTER_BOUND('',#18697,.T.);
#12757=FACE_OUTER_BOUND('',#18698,.T.);
#12758=FACE_OUTER_BOUND('',#18699,.T.);
#12759=FACE_OUTER_BOUND('',#18700,.T.);
#12760=FACE_OUTER_BOUND('',#18701,.T.);
#12761=FACE_OUTER_BOUND('',#18702,.T.);
#12762=FACE_OUTER_BOUND('',#18703,.T.);
#12763=FACE_OUTER_BOUND('',#18704,.T.);
#12764=FACE_OUTER_BOUND('',#18705,.T.);
#12765=FACE_OUTER_BOUND('',#18706,.T.);
#12766=FACE_OUTER_BOUND('',#18707,.T.);
#12767=FACE_OUTER_BOUND('',#18708,.T.);
#12768=FACE_OUTER_BOUND('',#18709,.T.);
#12769=FACE_OUTER_BOUND('',#18710,.T.);
#12770=FACE_OUTER_BOUND('',#18711,.T.);
#12771=FACE_OUTER_BOUND('',#18712,.T.);
#12772=FACE_OUTER_BOUND('',#18713,.T.);
#12773=FACE_OUTER_BOUND('',#18714,.T.);
#12774=FACE_OUTER_BOUND('',#18715,.T.);
#12775=FACE_OUTER_BOUND('',#18716,.T.);
#12776=FACE_OUTER_BOUND('',#18717,.T.);
#12777=FACE_OUTER_BOUND('',#18718,.T.);
#12778=FACE_OUTER_BOUND('',#18719,.T.);
#12779=FACE_OUTER_BOUND('',#18720,.T.);
#12780=FACE_OUTER_BOUND('',#18721,.T.);
#12781=FACE_OUTER_BOUND('',#18722,.T.);
#12782=FACE_OUTER_BOUND('',#18723,.T.);
#12783=FACE_OUTER_BOUND('',#18724,.T.);
#12784=FACE_OUTER_BOUND('',#18725,.T.);
#12785=FACE_OUTER_BOUND('',#18726,.T.);
#12786=FACE_OUTER_BOUND('',#18727,.T.);
#12787=FACE_OUTER_BOUND('',#18728,.T.);
#12788=FACE_OUTER_BOUND('',#18729,.T.);
#12789=FACE_OUTER_BOUND('',#18730,.T.);
#12790=FACE_OUTER_BOUND('',#18731,.T.);
#12791=FACE_OUTER_BOUND('',#18732,.T.);
#12792=FACE_OUTER_BOUND('',#18733,.T.);
#12793=FACE_OUTER_BOUND('',#18734,.T.);
#12794=FACE_OUTER_BOUND('',#18735,.T.);
#12795=FACE_OUTER_BOUND('',#18737,.T.);
#12796=FACE_OUTER_BOUND('',#18738,.T.);
#12797=FACE_OUTER_BOUND('',#18739,.T.);
#12798=FACE_OUTER_BOUND('',#18740,.T.);
#12799=FACE_OUTER_BOUND('',#18741,.T.);
#12800=FACE_OUTER_BOUND('',#18742,.T.);
#12801=FACE_OUTER_BOUND('',#18743,.T.);
#12802=FACE_OUTER_BOUND('',#18744,.T.);
#12803=FACE_OUTER_BOUND('',#18745,.T.);
#12804=FACE_OUTER_BOUND('',#18746,.T.);
#12805=FACE_OUTER_BOUND('',#18747,.T.);
#12806=FACE_OUTER_BOUND('',#18748,.T.);
#12807=FACE_OUTER_BOUND('',#18749,.T.);
#12808=FACE_OUTER_BOUND('',#18750,.T.);
#12809=FACE_OUTER_BOUND('',#18751,.T.);
#12810=FACE_OUTER_BOUND('',#18752,.T.);
#12811=FACE_OUTER_BOUND('',#18753,.T.);
#12812=FACE_OUTER_BOUND('',#18754,.T.);
#12813=FACE_OUTER_BOUND('',#18755,.T.);
#12814=FACE_OUTER_BOUND('',#18756,.T.);
#12815=FACE_OUTER_BOUND('',#18757,.T.);
#12816=FACE_OUTER_BOUND('',#18758,.T.);
#12817=FACE_OUTER_BOUND('',#18759,.T.);
#12818=FACE_OUTER_BOUND('',#18760,.T.);
#12819=FACE_OUTER_BOUND('',#18761,.T.);
#12820=FACE_OUTER_BOUND('',#18762,.T.);
#12821=FACE_OUTER_BOUND('',#18763,.T.);
#12822=FACE_OUTER_BOUND('',#18764,.T.);
#12823=FACE_OUTER_BOUND('',#18765,.T.);
#12824=FACE_OUTER_BOUND('',#18766,.T.);
#12825=FACE_OUTER_BOUND('',#18767,.T.);
#12826=FACE_OUTER_BOUND('',#18768,.T.);
#12827=FACE_OUTER_BOUND('',#18769,.T.);
#12828=FACE_OUTER_BOUND('',#18770,.T.);
#12829=FACE_OUTER_BOUND('',#18771,.T.);
#12830=FACE_OUTER_BOUND('',#18772,.T.);
#12831=FACE_OUTER_BOUND('',#18773,.T.);
#12832=FACE_OUTER_BOUND('',#18774,.T.);
#12833=FACE_OUTER_BOUND('',#18775,.T.);
#12834=FACE_OUTER_BOUND('',#18776,.T.);
#12835=FACE_OUTER_BOUND('',#18777,.T.);
#12836=FACE_OUTER_BOUND('',#18778,.T.);
#12837=FACE_OUTER_BOUND('',#18779,.T.);
#12838=FACE_OUTER_BOUND('',#18780,.T.);
#12839=FACE_OUTER_BOUND('',#18781,.T.);
#12840=FACE_OUTER_BOUND('',#18782,.T.);
#12841=FACE_OUTER_BOUND('',#18783,.T.);
#12842=FACE_OUTER_BOUND('',#18784,.T.);
#12843=FACE_OUTER_BOUND('',#18785,.T.);
#12844=FACE_OUTER_BOUND('',#18786,.T.);
#12845=FACE_OUTER_BOUND('',#18787,.T.);
#12846=FACE_OUTER_BOUND('',#18788,.T.);
#12847=FACE_OUTER_BOUND('',#18789,.T.);
#12848=FACE_OUTER_BOUND('',#18790,.T.);
#12849=FACE_OUTER_BOUND('',#18791,.T.);
#12850=FACE_OUTER_BOUND('',#18792,.T.);
#12851=FACE_OUTER_BOUND('',#18793,.T.);
#12852=FACE_OUTER_BOUND('',#18795,.T.);
#12853=FACE_OUTER_BOUND('',#18796,.T.);
#12854=FACE_OUTER_BOUND('',#18798,.T.);
#12855=FACE_OUTER_BOUND('',#18799,.T.);
#12856=FACE_OUTER_BOUND('',#18800,.T.);
#12857=FACE_OUTER_BOUND('',#18801,.T.);
#12858=FACE_OUTER_BOUND('',#18802,.T.);
#12859=FACE_OUTER_BOUND('',#18803,.T.);
#12860=FACE_OUTER_BOUND('',#18804,.T.);
#12861=FACE_OUTER_BOUND('',#18805,.T.);
#12862=FACE_OUTER_BOUND('',#18806,.T.);
#12863=FACE_OUTER_BOUND('',#18807,.T.);
#12864=FACE_OUTER_BOUND('',#18808,.T.);
#12865=FACE_OUTER_BOUND('',#18810,.T.);
#12866=FACE_OUTER_BOUND('',#18811,.T.);
#12867=FACE_OUTER_BOUND('',#18812,.T.);
#12868=FACE_OUTER_BOUND('',#18813,.T.);
#12869=FACE_OUTER_BOUND('',#18815,.T.);
#12870=FACE_OUTER_BOUND('',#18816,.T.);
#12871=FACE_OUTER_BOUND('',#18817,.T.);
#12872=FACE_OUTER_BOUND('',#18818,.T.);
#12873=FACE_OUTER_BOUND('',#18819,.T.);
#12874=FACE_OUTER_BOUND('',#18820,.T.);
#12875=FACE_OUTER_BOUND('',#18821,.T.);
#12876=FACE_OUTER_BOUND('',#18822,.T.);
#12877=FACE_OUTER_BOUND('',#18823,.T.);
#12878=FACE_OUTER_BOUND('',#18824,.T.);
#12879=FACE_OUTER_BOUND('',#18825,.T.);
#12880=FACE_OUTER_BOUND('',#18826,.T.);
#12881=FACE_OUTER_BOUND('',#18827,.T.);
#12882=FACE_OUTER_BOUND('',#18828,.T.);
#12883=FACE_OUTER_BOUND('',#18831,.T.);
#12884=FACE_OUTER_BOUND('',#18832,.T.);
#12885=FACE_OUTER_BOUND('',#18833,.T.);
#12886=FACE_OUTER_BOUND('',#18834,.T.);
#12887=FACE_OUTER_BOUND('',#18835,.T.);
#12888=FACE_OUTER_BOUND('',#18836,.T.);
#12889=FACE_OUTER_BOUND('',#18837,.T.);
#12890=FACE_OUTER_BOUND('',#18838,.T.);
#12891=FACE_OUTER_BOUND('',#18839,.T.);
#12892=FACE_OUTER_BOUND('',#18840,.T.);
#12893=FACE_OUTER_BOUND('',#18841,.T.);
#12894=FACE_OUTER_BOUND('',#18842,.T.);
#12895=FACE_OUTER_BOUND('',#18843,.T.);
#12896=FACE_OUTER_BOUND('',#18844,.T.);
#12897=FACE_OUTER_BOUND('',#18845,.T.);
#12898=FACE_OUTER_BOUND('',#18846,.T.);
#12899=FACE_OUTER_BOUND('',#18847,.T.);
#12900=FACE_OUTER_BOUND('',#18850,.T.);
#12901=FACE_OUTER_BOUND('',#18851,.T.);
#12902=FACE_OUTER_BOUND('',#18852,.T.);
#12903=FACE_OUTER_BOUND('',#18853,.T.);
#12904=FACE_OUTER_BOUND('',#18854,.T.);
#12905=FACE_OUTER_BOUND('',#18855,.T.);
#12906=FACE_OUTER_BOUND('',#18856,.T.);
#12907=FACE_OUTER_BOUND('',#18857,.T.);
#12908=FACE_OUTER_BOUND('',#18858,.T.);
#12909=FACE_OUTER_BOUND('',#18859,.T.);
#12910=FACE_OUTER_BOUND('',#18861,.T.);
#12911=FACE_OUTER_BOUND('',#18862,.T.);
#12912=FACE_OUTER_BOUND('',#18863,.T.);
#12913=FACE_OUTER_BOUND('',#18864,.T.);
#12914=FACE_OUTER_BOUND('',#18865,.T.);
#12915=FACE_OUTER_BOUND('',#18866,.T.);
#12916=FACE_OUTER_BOUND('',#18867,.T.);
#12917=FACE_OUTER_BOUND('',#18869,.T.);
#12918=FACE_OUTER_BOUND('',#18870,.T.);
#12919=FACE_OUTER_BOUND('',#18871,.T.);
#12920=FACE_OUTER_BOUND('',#18872,.T.);
#12921=FACE_OUTER_BOUND('',#18873,.T.);
#12922=FACE_OUTER_BOUND('',#18874,.T.);
#12923=FACE_OUTER_BOUND('',#18875,.T.);
#12924=FACE_OUTER_BOUND('',#18876,.T.);
#12925=FACE_OUTER_BOUND('',#18877,.T.);
#12926=FACE_OUTER_BOUND('',#18878,.T.);
#12927=FACE_OUTER_BOUND('',#18879,.T.);
#12928=FACE_OUTER_BOUND('',#18881,.T.);
#12929=FACE_OUTER_BOUND('',#18882,.T.);
#12930=FACE_OUTER_BOUND('',#18883,.T.);
#12931=FACE_OUTER_BOUND('',#18884,.T.);
#12932=FACE_OUTER_BOUND('',#18885,.T.);
#12933=FACE_OUTER_BOUND('',#18886,.T.);
#12934=FACE_OUTER_BOUND('',#18887,.T.);
#12935=FACE_OUTER_BOUND('',#18888,.T.);
#12936=FACE_OUTER_BOUND('',#18889,.T.);
#12937=FACE_OUTER_BOUND('',#18890,.T.);
#12938=FACE_OUTER_BOUND('',#18891,.T.);
#12939=FACE_OUTER_BOUND('',#18892,.T.);
#12940=FACE_OUTER_BOUND('',#18893,.T.);
#12941=FACE_OUTER_BOUND('',#18894,.T.);
#12942=FACE_OUTER_BOUND('',#18895,.T.);
#12943=FACE_OUTER_BOUND('',#18896,.T.);
#12944=FACE_OUTER_BOUND('',#18897,.T.);
#12945=FACE_OUTER_BOUND('',#18898,.T.);
#12946=FACE_OUTER_BOUND('',#18899,.T.);
#12947=FACE_OUTER_BOUND('',#18900,.T.);
#12948=FACE_OUTER_BOUND('',#18901,.T.);
#12949=FACE_OUTER_BOUND('',#18902,.T.);
#12950=FACE_OUTER_BOUND('',#18903,.T.);
#12951=FACE_OUTER_BOUND('',#18904,.T.);
#12952=FACE_OUTER_BOUND('',#18905,.T.);
#12953=FACE_OUTER_BOUND('',#18906,.T.);
#12954=FACE_OUTER_BOUND('',#18907,.T.);
#12955=FACE_OUTER_BOUND('',#18908,.T.);
#12956=FACE_OUTER_BOUND('',#18909,.T.);
#12957=FACE_OUTER_BOUND('',#18910,.T.);
#12958=FACE_OUTER_BOUND('',#18911,.T.);
#12959=FACE_OUTER_BOUND('',#18912,.T.);
#12960=FACE_OUTER_BOUND('',#18913,.T.);
#12961=FACE_OUTER_BOUND('',#18914,.T.);
#12962=FACE_OUTER_BOUND('',#18915,.T.);
#12963=FACE_OUTER_BOUND('',#18916,.T.);
#12964=FACE_OUTER_BOUND('',#18917,.T.);
#12965=FACE_OUTER_BOUND('',#18918,.T.);
#12966=FACE_OUTER_BOUND('',#18919,.T.);
#12967=FACE_OUTER_BOUND('',#18920,.T.);
#12968=FACE_OUTER_BOUND('',#18921,.T.);
#12969=FACE_OUTER_BOUND('',#18922,.T.);
#12970=FACE_OUTER_BOUND('',#18923,.T.);
#12971=FACE_OUTER_BOUND('',#18924,.T.);
#12972=FACE_OUTER_BOUND('',#18925,.T.);
#12973=FACE_OUTER_BOUND('',#18926,.T.);
#12974=FACE_OUTER_BOUND('',#18927,.T.);
#12975=FACE_OUTER_BOUND('',#18928,.T.);
#12976=FACE_OUTER_BOUND('',#18929,.T.);
#12977=FACE_OUTER_BOUND('',#18930,.T.);
#12978=FACE_OUTER_BOUND('',#18931,.T.);
#12979=FACE_OUTER_BOUND('',#18932,.T.);
#12980=FACE_OUTER_BOUND('',#18933,.T.);
#12981=FACE_OUTER_BOUND('',#18934,.T.);
#12982=FACE_OUTER_BOUND('',#18935,.T.);
#12983=FACE_OUTER_BOUND('',#18936,.T.);
#12984=FACE_OUTER_BOUND('',#18937,.T.);
#12985=FACE_OUTER_BOUND('',#18938,.T.);
#12986=FACE_OUTER_BOUND('',#18939,.T.);
#12987=FACE_OUTER_BOUND('',#18940,.T.);
#12988=FACE_OUTER_BOUND('',#18941,.T.);
#12989=FACE_OUTER_BOUND('',#18942,.T.);
#12990=FACE_OUTER_BOUND('',#18943,.T.);
#12991=FACE_OUTER_BOUND('',#18944,.T.);
#12992=FACE_OUTER_BOUND('',#18945,.T.);
#12993=FACE_OUTER_BOUND('',#18946,.T.);
#12994=FACE_OUTER_BOUND('',#18947,.T.);
#12995=FACE_OUTER_BOUND('',#18948,.T.);
#12996=FACE_OUTER_BOUND('',#18949,.T.);
#12997=FACE_OUTER_BOUND('',#18950,.T.);
#12998=FACE_OUTER_BOUND('',#18951,.T.);
#12999=FACE_OUTER_BOUND('',#18952,.T.);
#13000=FACE_OUTER_BOUND('',#18953,.T.);
#13001=FACE_OUTER_BOUND('',#18954,.T.);
#13002=FACE_OUTER_BOUND('',#18955,.T.);
#13003=FACE_OUTER_BOUND('',#18956,.T.);
#13004=FACE_OUTER_BOUND('',#18957,.T.);
#13005=FACE_OUTER_BOUND('',#18958,.T.);
#13006=FACE_OUTER_BOUND('',#18959,.T.);
#13007=FACE_OUTER_BOUND('',#18960,.T.);
#13008=FACE_OUTER_BOUND('',#18961,.T.);
#13009=FACE_OUTER_BOUND('',#18962,.T.);
#13010=FACE_OUTER_BOUND('',#18963,.T.);
#13011=FACE_OUTER_BOUND('',#18964,.T.);
#13012=FACE_OUTER_BOUND('',#18965,.T.);
#13013=FACE_OUTER_BOUND('',#18966,.T.);
#13014=FACE_OUTER_BOUND('',#18967,.T.);
#13015=FACE_OUTER_BOUND('',#18968,.T.);
#13016=FACE_OUTER_BOUND('',#18969,.T.);
#13017=FACE_OUTER_BOUND('',#18970,.T.);
#13018=FACE_OUTER_BOUND('',#18971,.T.);
#13019=FACE_OUTER_BOUND('',#18972,.T.);
#13020=FACE_OUTER_BOUND('',#18973,.T.);
#13021=FACE_OUTER_BOUND('',#18974,.T.);
#13022=FACE_OUTER_BOUND('',#18975,.T.);
#13023=FACE_OUTER_BOUND('',#18976,.T.);
#13024=FACE_OUTER_BOUND('',#18977,.T.);
#13025=FACE_OUTER_BOUND('',#18978,.T.);
#13026=FACE_OUTER_BOUND('',#18979,.T.);
#13027=FACE_OUTER_BOUND('',#18980,.T.);
#13028=FACE_OUTER_BOUND('',#18981,.T.);
#13029=FACE_OUTER_BOUND('',#18982,.T.);
#13030=FACE_OUTER_BOUND('',#18983,.T.);
#13031=FACE_OUTER_BOUND('',#18984,.T.);
#13032=FACE_OUTER_BOUND('',#18985,.T.);
#13033=FACE_OUTER_BOUND('',#18986,.T.);
#13034=FACE_OUTER_BOUND('',#18987,.T.);
#13035=FACE_OUTER_BOUND('',#18988,.T.);
#13036=FACE_OUTER_BOUND('',#18989,.T.);
#13037=FACE_OUTER_BOUND('',#18990,.T.);
#13038=FACE_OUTER_BOUND('',#18991,.T.);
#13039=FACE_OUTER_BOUND('',#18992,.T.);
#13040=FACE_OUTER_BOUND('',#18993,.T.);
#13041=FACE_OUTER_BOUND('',#18994,.T.);
#13042=FACE_OUTER_BOUND('',#18995,.T.);
#13043=FACE_OUTER_BOUND('',#18996,.T.);
#13044=FACE_OUTER_BOUND('',#18997,.T.);
#13045=FACE_OUTER_BOUND('',#18998,.T.);
#13046=FACE_OUTER_BOUND('',#18999,.T.);
#13047=FACE_OUTER_BOUND('',#19000,.T.);
#13048=FACE_OUTER_BOUND('',#19001,.T.);
#13049=FACE_OUTER_BOUND('',#19002,.T.);
#13050=FACE_OUTER_BOUND('',#19003,.T.);
#13051=FACE_OUTER_BOUND('',#19004,.T.);
#13052=FACE_OUTER_BOUND('',#19005,.T.);
#13053=FACE_OUTER_BOUND('',#19006,.T.);
#13054=FACE_OUTER_BOUND('',#19007,.T.);
#13055=FACE_OUTER_BOUND('',#19008,.T.);
#13056=FACE_OUTER_BOUND('',#19009,.T.);
#13057=FACE_OUTER_BOUND('',#19010,.T.);
#13058=FACE_OUTER_BOUND('',#19011,.T.);
#13059=FACE_OUTER_BOUND('',#19012,.T.);
#13060=FACE_OUTER_BOUND('',#19013,.T.);
#13061=FACE_OUTER_BOUND('',#19014,.T.);
#13062=FACE_OUTER_BOUND('',#19015,.T.);
#13063=FACE_OUTER_BOUND('',#19016,.T.);
#13064=FACE_OUTER_BOUND('',#19017,.T.);
#13065=FACE_OUTER_BOUND('',#19018,.T.);
#13066=FACE_OUTER_BOUND('',#19019,.T.);
#13067=FACE_OUTER_BOUND('',#19020,.T.);
#13068=FACE_OUTER_BOUND('',#19021,.T.);
#13069=FACE_OUTER_BOUND('',#19022,.T.);
#13070=FACE_OUTER_BOUND('',#19023,.T.);
#13071=FACE_OUTER_BOUND('',#19024,.T.);
#13072=FACE_OUTER_BOUND('',#19025,.T.);
#13073=FACE_OUTER_BOUND('',#19026,.T.);
#13074=FACE_OUTER_BOUND('',#19027,.T.);
#13075=FACE_OUTER_BOUND('',#19028,.T.);
#13076=FACE_OUTER_BOUND('',#19029,.T.);
#13077=FACE_OUTER_BOUND('',#19030,.T.);
#13078=FACE_OUTER_BOUND('',#19031,.T.);
#13079=FACE_OUTER_BOUND('',#19032,.T.);
#13080=FACE_OUTER_BOUND('',#19033,.T.);
#13081=FACE_OUTER_BOUND('',#19034,.T.);
#13082=FACE_OUTER_BOUND('',#19035,.T.);
#13083=FACE_OUTER_BOUND('',#19036,.T.);
#13084=FACE_OUTER_BOUND('',#19037,.T.);
#13085=FACE_OUTER_BOUND('',#19038,.T.);
#13086=FACE_OUTER_BOUND('',#19039,.T.);
#13087=FACE_OUTER_BOUND('',#19040,.T.);
#13088=FACE_OUTER_BOUND('',#19041,.T.);
#13089=FACE_OUTER_BOUND('',#19042,.T.);
#13090=FACE_OUTER_BOUND('',#19043,.T.);
#13091=FACE_OUTER_BOUND('',#19044,.T.);
#13092=FACE_OUTER_BOUND('',#19045,.T.);
#13093=FACE_OUTER_BOUND('',#19046,.T.);
#13094=FACE_OUTER_BOUND('',#19047,.T.);
#13095=FACE_OUTER_BOUND('',#19048,.T.);
#13096=FACE_OUTER_BOUND('',#19049,.T.);
#13097=FACE_OUTER_BOUND('',#19050,.T.);
#13098=FACE_OUTER_BOUND('',#19051,.T.);
#13099=FACE_OUTER_BOUND('',#19052,.T.);
#13100=FACE_OUTER_BOUND('',#19053,.T.);
#13101=FACE_OUTER_BOUND('',#19054,.T.);
#13102=FACE_OUTER_BOUND('',#19055,.T.);
#13103=FACE_OUTER_BOUND('',#19056,.T.);
#13104=FACE_OUTER_BOUND('',#19057,.T.);
#13105=FACE_OUTER_BOUND('',#19058,.T.);
#13106=FACE_OUTER_BOUND('',#19059,.T.);
#13107=FACE_OUTER_BOUND('',#19060,.T.);
#13108=FACE_OUTER_BOUND('',#19061,.T.);
#13109=FACE_OUTER_BOUND('',#19062,.T.);
#13110=FACE_OUTER_BOUND('',#19063,.T.);
#13111=FACE_OUTER_BOUND('',#19064,.T.);
#13112=FACE_OUTER_BOUND('',#19065,.T.);
#13113=FACE_OUTER_BOUND('',#19066,.T.);
#13114=FACE_OUTER_BOUND('',#19067,.T.);
#13115=FACE_OUTER_BOUND('',#19068,.T.);
#13116=FACE_OUTER_BOUND('',#19069,.T.);
#13117=FACE_OUTER_BOUND('',#19070,.T.);
#13118=FACE_OUTER_BOUND('',#19071,.T.);
#13119=FACE_OUTER_BOUND('',#19072,.T.);
#13120=FACE_OUTER_BOUND('',#19073,.T.);
#13121=FACE_OUTER_BOUND('',#19074,.T.);
#13122=FACE_OUTER_BOUND('',#19075,.T.);
#13123=FACE_OUTER_BOUND('',#19076,.T.);
#13124=FACE_OUTER_BOUND('',#19077,.T.);
#13125=FACE_OUTER_BOUND('',#19078,.T.);
#13126=FACE_OUTER_BOUND('',#19079,.T.);
#13127=FACE_OUTER_BOUND('',#19080,.T.);
#13128=FACE_OUTER_BOUND('',#19081,.T.);
#13129=FACE_OUTER_BOUND('',#19082,.T.);
#13130=FACE_OUTER_BOUND('',#19083,.T.);
#13131=FACE_OUTER_BOUND('',#19084,.T.);
#13132=FACE_OUTER_BOUND('',#19085,.T.);
#13133=FACE_OUTER_BOUND('',#19086,.T.);
#13134=FACE_OUTER_BOUND('',#19087,.T.);
#13135=FACE_OUTER_BOUND('',#19088,.T.);
#13136=FACE_OUTER_BOUND('',#19089,.T.);
#13137=FACE_OUTER_BOUND('',#19090,.T.);
#13138=FACE_OUTER_BOUND('',#19091,.T.);
#13139=FACE_OUTER_BOUND('',#19092,.T.);
#13140=FACE_OUTER_BOUND('',#19093,.T.);
#13141=FACE_OUTER_BOUND('',#19094,.T.);
#13142=FACE_OUTER_BOUND('',#19095,.T.);
#13143=FACE_OUTER_BOUND('',#19096,.T.);
#13144=FACE_OUTER_BOUND('',#19097,.T.);
#13145=FACE_OUTER_BOUND('',#19098,.T.);
#13146=FACE_OUTER_BOUND('',#19099,.T.);
#13147=FACE_OUTER_BOUND('',#19100,.T.);
#13148=FACE_OUTER_BOUND('',#19101,.T.);
#13149=FACE_OUTER_BOUND('',#19102,.T.);
#13150=FACE_OUTER_BOUND('',#19103,.T.);
#13151=FACE_OUTER_BOUND('',#19104,.T.);
#13152=FACE_OUTER_BOUND('',#19105,.T.);
#13153=FACE_OUTER_BOUND('',#19106,.T.);
#13154=FACE_OUTER_BOUND('',#19107,.T.);
#13155=FACE_OUTER_BOUND('',#19108,.T.);
#13156=FACE_OUTER_BOUND('',#19109,.T.);
#13157=FACE_OUTER_BOUND('',#19110,.T.);
#13158=FACE_OUTER_BOUND('',#19111,.T.);
#13159=FACE_OUTER_BOUND('',#19112,.T.);
#13160=FACE_OUTER_BOUND('',#19113,.T.);
#13161=FACE_OUTER_BOUND('',#19114,.T.);
#13162=FACE_OUTER_BOUND('',#19115,.T.);
#13163=FACE_OUTER_BOUND('',#19116,.T.);
#13164=FACE_OUTER_BOUND('',#19117,.T.);
#13165=FACE_OUTER_BOUND('',#19118,.T.);
#13166=FACE_OUTER_BOUND('',#19119,.T.);
#13167=FACE_OUTER_BOUND('',#19120,.T.);
#13168=FACE_OUTER_BOUND('',#19121,.T.);
#13169=FACE_OUTER_BOUND('',#19122,.T.);
#13170=FACE_OUTER_BOUND('',#19123,.T.);
#13171=FACE_OUTER_BOUND('',#19124,.T.);
#13172=FACE_OUTER_BOUND('',#19125,.T.);
#13173=FACE_OUTER_BOUND('',#19126,.T.);
#13174=FACE_OUTER_BOUND('',#19127,.T.);
#13175=FACE_OUTER_BOUND('',#19128,.T.);
#13176=FACE_OUTER_BOUND('',#19129,.T.);
#13177=FACE_OUTER_BOUND('',#19130,.T.);
#13178=FACE_OUTER_BOUND('',#19131,.T.);
#13179=FACE_OUTER_BOUND('',#19132,.T.);
#13180=FACE_OUTER_BOUND('',#19133,.T.);
#13181=FACE_OUTER_BOUND('',#19134,.T.);
#13182=FACE_OUTER_BOUND('',#19135,.T.);
#13183=FACE_OUTER_BOUND('',#19136,.T.);
#13184=FACE_OUTER_BOUND('',#19137,.T.);
#13185=FACE_OUTER_BOUND('',#19138,.T.);
#13186=FACE_OUTER_BOUND('',#19139,.T.);
#13187=FACE_OUTER_BOUND('',#19140,.T.);
#13188=FACE_OUTER_BOUND('',#19141,.T.);
#13189=FACE_OUTER_BOUND('',#19142,.T.);
#13190=FACE_OUTER_BOUND('',#19143,.T.);
#13191=FACE_OUTER_BOUND('',#19144,.T.);
#13192=FACE_OUTER_BOUND('',#19145,.T.);
#13193=FACE_OUTER_BOUND('',#19147,.T.);
#13194=FACE_OUTER_BOUND('',#19148,.T.);
#13195=FACE_OUTER_BOUND('',#19149,.T.);
#13196=FACE_OUTER_BOUND('',#19150,.T.);
#13197=FACE_OUTER_BOUND('',#19151,.T.);
#13198=FACE_OUTER_BOUND('',#19152,.T.);
#13199=FACE_OUTER_BOUND('',#19153,.T.);
#13200=FACE_OUTER_BOUND('',#19154,.T.);
#13201=FACE_OUTER_BOUND('',#19155,.T.);
#13202=FACE_OUTER_BOUND('',#19156,.T.);
#13203=FACE_OUTER_BOUND('',#19157,.T.);
#13204=FACE_OUTER_BOUND('',#19158,.T.);
#13205=FACE_OUTER_BOUND('',#19159,.T.);
#13206=FACE_OUTER_BOUND('',#19160,.T.);
#13207=FACE_OUTER_BOUND('',#19161,.T.);
#13208=FACE_OUTER_BOUND('',#19162,.T.);
#13209=FACE_OUTER_BOUND('',#19163,.T.);
#13210=FACE_OUTER_BOUND('',#19164,.T.);
#13211=FACE_OUTER_BOUND('',#19165,.T.);
#13212=FACE_OUTER_BOUND('',#19166,.T.);
#13213=FACE_OUTER_BOUND('',#19167,.T.);
#13214=FACE_OUTER_BOUND('',#19168,.T.);
#13215=FACE_OUTER_BOUND('',#19169,.T.);
#13216=FACE_OUTER_BOUND('',#19170,.T.);
#13217=FACE_OUTER_BOUND('',#19171,.T.);
#13218=FACE_OUTER_BOUND('',#19172,.T.);
#13219=FACE_OUTER_BOUND('',#19173,.T.);
#13220=FACE_OUTER_BOUND('',#19174,.T.);
#13221=FACE_OUTER_BOUND('',#19175,.T.);
#13222=FACE_OUTER_BOUND('',#19176,.T.);
#13223=FACE_OUTER_BOUND('',#19177,.T.);
#13224=FACE_OUTER_BOUND('',#19178,.T.);
#13225=FACE_OUTER_BOUND('',#19179,.T.);
#13226=FACE_OUTER_BOUND('',#19180,.T.);
#13227=FACE_OUTER_BOUND('',#19181,.T.);
#13228=FACE_OUTER_BOUND('',#19182,.T.);
#13229=FACE_OUTER_BOUND('',#19183,.T.);
#13230=FACE_OUTER_BOUND('',#19184,.T.);
#13231=FACE_OUTER_BOUND('',#19185,.T.);
#13232=FACE_OUTER_BOUND('',#19186,.T.);
#13233=FACE_OUTER_BOUND('',#19187,.T.);
#13234=FACE_OUTER_BOUND('',#19188,.T.);
#13235=FACE_OUTER_BOUND('',#19189,.T.);
#13236=FACE_OUTER_BOUND('',#19190,.T.);
#13237=FACE_OUTER_BOUND('',#19191,.T.);
#13238=FACE_OUTER_BOUND('',#19192,.T.);
#13239=FACE_OUTER_BOUND('',#19193,.T.);
#13240=FACE_OUTER_BOUND('',#19194,.T.);
#13241=FACE_OUTER_BOUND('',#19195,.T.);
#13242=FACE_OUTER_BOUND('',#19196,.T.);
#13243=FACE_OUTER_BOUND('',#19197,.T.);
#13244=FACE_OUTER_BOUND('',#19198,.T.);
#13245=FACE_OUTER_BOUND('',#19199,.T.);
#13246=FACE_OUTER_BOUND('',#19200,.T.);
#13247=FACE_OUTER_BOUND('',#19201,.T.);
#13248=FACE_OUTER_BOUND('',#19202,.T.);
#13249=FACE_OUTER_BOUND('',#19203,.T.);
#13250=FACE_OUTER_BOUND('',#19204,.T.);
#13251=FACE_OUTER_BOUND('',#19205,.T.);
#13252=FACE_OUTER_BOUND('',#19206,.T.);
#13253=FACE_OUTER_BOUND('',#19207,.T.);
#13254=FACE_OUTER_BOUND('',#19208,.T.);
#13255=FACE_OUTER_BOUND('',#19209,.T.);
#13256=FACE_OUTER_BOUND('',#19210,.T.);
#13257=FACE_OUTER_BOUND('',#19211,.T.);
#13258=FACE_OUTER_BOUND('',#19212,.T.);
#13259=FACE_OUTER_BOUND('',#19213,.T.);
#13260=FACE_OUTER_BOUND('',#19214,.T.);
#13261=FACE_OUTER_BOUND('',#19215,.T.);
#13262=FACE_OUTER_BOUND('',#19216,.T.);
#13263=FACE_OUTER_BOUND('',#19217,.T.);
#13264=FACE_OUTER_BOUND('',#19218,.T.);
#13265=FACE_OUTER_BOUND('',#19219,.T.);
#13266=FACE_OUTER_BOUND('',#19220,.T.);
#13267=FACE_OUTER_BOUND('',#19221,.T.);
#13268=FACE_OUTER_BOUND('',#19222,.T.);
#13269=FACE_OUTER_BOUND('',#19223,.T.);
#13270=FACE_OUTER_BOUND('',#19224,.T.);
#13271=FACE_OUTER_BOUND('',#19225,.T.);
#13272=FACE_OUTER_BOUND('',#19226,.T.);
#13273=FACE_OUTER_BOUND('',#19227,.T.);
#13274=FACE_OUTER_BOUND('',#19228,.T.);
#13275=FACE_OUTER_BOUND('',#19229,.T.);
#13276=FACE_OUTER_BOUND('',#19230,.T.);
#13277=FACE_OUTER_BOUND('',#19231,.T.);
#13278=FACE_OUTER_BOUND('',#19232,.T.);
#13279=FACE_OUTER_BOUND('',#19233,.T.);
#13280=FACE_OUTER_BOUND('',#19234,.T.);
#13281=FACE_OUTER_BOUND('',#19235,.T.);
#13282=FACE_OUTER_BOUND('',#19236,.T.);
#13283=FACE_OUTER_BOUND('',#19237,.T.);
#13284=FACE_OUTER_BOUND('',#19238,.T.);
#13285=FACE_OUTER_BOUND('',#19239,.T.);
#13286=FACE_OUTER_BOUND('',#19240,.T.);
#13287=FACE_OUTER_BOUND('',#19241,.T.);
#13288=FACE_OUTER_BOUND('',#19242,.T.);
#13289=FACE_OUTER_BOUND('',#19243,.T.);
#13290=FACE_OUTER_BOUND('',#19244,.T.);
#13291=FACE_OUTER_BOUND('',#19245,.T.);
#13292=FACE_OUTER_BOUND('',#19246,.T.);
#13293=FACE_OUTER_BOUND('',#19247,.T.);
#13294=FACE_OUTER_BOUND('',#19248,.T.);
#13295=FACE_OUTER_BOUND('',#19249,.T.);
#13296=FACE_OUTER_BOUND('',#19250,.T.);
#13297=FACE_OUTER_BOUND('',#19251,.T.);
#13298=FACE_OUTER_BOUND('',#19252,.T.);
#13299=FACE_OUTER_BOUND('',#19253,.T.);
#13300=FACE_OUTER_BOUND('',#19254,.T.);
#13301=FACE_OUTER_BOUND('',#19255,.T.);
#13302=FACE_OUTER_BOUND('',#19256,.T.);
#13303=FACE_OUTER_BOUND('',#19257,.T.);
#13304=FACE_OUTER_BOUND('',#19258,.T.);
#13305=FACE_OUTER_BOUND('',#19259,.T.);
#13306=FACE_OUTER_BOUND('',#19260,.T.);
#13307=FACE_OUTER_BOUND('',#19261,.T.);
#13308=FACE_OUTER_BOUND('',#19262,.T.);
#13309=FACE_OUTER_BOUND('',#19263,.T.);
#13310=FACE_OUTER_BOUND('',#19264,.T.);
#13311=FACE_OUTER_BOUND('',#19265,.T.);
#13312=FACE_OUTER_BOUND('',#19266,.T.);
#13313=FACE_OUTER_BOUND('',#19267,.T.);
#13314=FACE_OUTER_BOUND('',#19268,.T.);
#13315=FACE_OUTER_BOUND('',#19269,.T.);
#13316=FACE_OUTER_BOUND('',#19270,.T.);
#13317=FACE_OUTER_BOUND('',#19271,.T.);
#13318=FACE_OUTER_BOUND('',#19272,.T.);
#13319=FACE_OUTER_BOUND('',#19273,.T.);
#13320=FACE_OUTER_BOUND('',#19274,.T.);
#13321=FACE_OUTER_BOUND('',#19275,.T.);
#13322=FACE_OUTER_BOUND('',#19276,.T.);
#13323=FACE_OUTER_BOUND('',#19277,.T.);
#13324=FACE_OUTER_BOUND('',#19278,.T.);
#13325=FACE_OUTER_BOUND('',#19279,.T.);
#13326=FACE_OUTER_BOUND('',#19280,.T.);
#13327=FACE_OUTER_BOUND('',#19281,.T.);
#13328=FACE_OUTER_BOUND('',#19282,.T.);
#13329=FACE_OUTER_BOUND('',#19283,.T.);
#13330=FACE_OUTER_BOUND('',#19284,.T.);
#13331=FACE_OUTER_BOUND('',#19285,.T.);
#13332=FACE_OUTER_BOUND('',#19286,.T.);
#13333=FACE_OUTER_BOUND('',#19287,.T.);
#13334=FACE_OUTER_BOUND('',#19288,.T.);
#13335=FACE_OUTER_BOUND('',#19289,.T.);
#13336=FACE_OUTER_BOUND('',#19290,.T.);
#13337=FACE_OUTER_BOUND('',#19291,.T.);
#13338=FACE_OUTER_BOUND('',#19292,.T.);
#13339=FACE_OUTER_BOUND('',#19293,.T.);
#13340=FACE_OUTER_BOUND('',#19294,.T.);
#13341=FACE_OUTER_BOUND('',#19295,.T.);
#13342=FACE_OUTER_BOUND('',#19296,.T.);
#13343=FACE_OUTER_BOUND('',#19297,.T.);
#13344=FACE_OUTER_BOUND('',#19298,.T.);
#13345=FACE_OUTER_BOUND('',#19299,.T.);
#13346=FACE_OUTER_BOUND('',#19300,.T.);
#13347=FACE_OUTER_BOUND('',#19301,.T.);
#13348=FACE_OUTER_BOUND('',#19302,.T.);
#13349=FACE_OUTER_BOUND('',#19303,.T.);
#13350=FACE_OUTER_BOUND('',#19304,.T.);
#13351=FACE_OUTER_BOUND('',#19305,.T.);
#13352=FACE_OUTER_BOUND('',#19306,.T.);
#13353=FACE_OUTER_BOUND('',#19307,.T.);
#13354=FACE_OUTER_BOUND('',#19308,.T.);
#13355=FACE_OUTER_BOUND('',#19309,.T.);
#13356=FACE_OUTER_BOUND('',#19310,.T.);
#13357=FACE_OUTER_BOUND('',#19311,.T.);
#13358=FACE_OUTER_BOUND('',#19312,.T.);
#13359=FACE_OUTER_BOUND('',#19313,.T.);
#13360=FACE_OUTER_BOUND('',#19314,.T.);
#13361=FACE_OUTER_BOUND('',#19315,.T.);
#13362=FACE_OUTER_BOUND('',#19316,.T.);
#13363=FACE_OUTER_BOUND('',#19317,.T.);
#13364=FACE_OUTER_BOUND('',#19318,.T.);
#13365=FACE_OUTER_BOUND('',#19319,.T.);
#13366=FACE_OUTER_BOUND('',#19320,.T.);
#13367=FACE_OUTER_BOUND('',#19321,.T.);
#13368=FACE_OUTER_BOUND('',#19322,.T.);
#13369=FACE_OUTER_BOUND('',#19323,.T.);
#13370=FACE_OUTER_BOUND('',#19324,.T.);
#13371=FACE_OUTER_BOUND('',#19325,.T.);
#13372=FACE_OUTER_BOUND('',#19326,.T.);
#13373=FACE_OUTER_BOUND('',#19327,.T.);
#13374=FACE_OUTER_BOUND('',#19328,.T.);
#13375=FACE_OUTER_BOUND('',#19329,.T.);
#13376=FACE_OUTER_BOUND('',#19330,.T.);
#13377=FACE_OUTER_BOUND('',#19331,.T.);
#13378=FACE_OUTER_BOUND('',#19332,.T.);
#13379=FACE_OUTER_BOUND('',#19333,.T.);
#13380=FACE_OUTER_BOUND('',#19334,.T.);
#13381=FACE_OUTER_BOUND('',#19335,.T.);
#13382=FACE_OUTER_BOUND('',#19336,.T.);
#13383=FACE_OUTER_BOUND('',#19337,.T.);
#13384=FACE_OUTER_BOUND('',#19338,.T.);
#13385=FACE_OUTER_BOUND('',#19339,.T.);
#13386=FACE_OUTER_BOUND('',#19340,.T.);
#13387=FACE_OUTER_BOUND('',#19341,.T.);
#13388=FACE_OUTER_BOUND('',#19342,.T.);
#13389=FACE_OUTER_BOUND('',#19343,.T.);
#13390=FACE_OUTER_BOUND('',#19344,.T.);
#13391=FACE_OUTER_BOUND('',#19345,.T.);
#13392=FACE_OUTER_BOUND('',#19346,.T.);
#13393=FACE_OUTER_BOUND('',#19347,.T.);
#13394=FACE_OUTER_BOUND('',#19348,.T.);
#13395=FACE_OUTER_BOUND('',#19349,.T.);
#13396=FACE_OUTER_BOUND('',#19350,.T.);
#13397=FACE_OUTER_BOUND('',#19351,.T.);
#13398=FACE_OUTER_BOUND('',#19352,.T.);
#13399=FACE_OUTER_BOUND('',#19353,.T.);
#13400=FACE_OUTER_BOUND('',#19354,.T.);
#13401=FACE_OUTER_BOUND('',#19355,.T.);
#13402=FACE_OUTER_BOUND('',#19356,.T.);
#13403=FACE_OUTER_BOUND('',#19357,.T.);
#13404=FACE_OUTER_BOUND('',#19358,.T.);
#13405=FACE_OUTER_BOUND('',#19359,.T.);
#13406=FACE_OUTER_BOUND('',#19360,.T.);
#13407=FACE_OUTER_BOUND('',#19361,.T.);
#13408=FACE_OUTER_BOUND('',#19362,.T.);
#13409=FACE_OUTER_BOUND('',#19363,.T.);
#13410=FACE_OUTER_BOUND('',#19364,.T.);
#13411=FACE_OUTER_BOUND('',#19365,.T.);
#13412=FACE_OUTER_BOUND('',#19366,.T.);
#13413=FACE_OUTER_BOUND('',#19367,.T.);
#13414=FACE_OUTER_BOUND('',#19368,.T.);
#13415=FACE_OUTER_BOUND('',#19369,.T.);
#13416=FACE_OUTER_BOUND('',#19373,.T.);
#13417=FACE_OUTER_BOUND('',#19375,.T.);
#13418=FACE_OUTER_BOUND('',#19376,.T.);
#13419=FACE_OUTER_BOUND('',#19377,.T.);
#13420=FACE_OUTER_BOUND('',#19378,.T.);
#13421=FACE_OUTER_BOUND('',#19380,.T.);
#13422=FACE_OUTER_BOUND('',#19381,.T.);
#13423=FACE_OUTER_BOUND('',#19382,.T.);
#13424=FACE_OUTER_BOUND('',#19383,.T.);
#13425=FACE_OUTER_BOUND('',#19385,.T.);
#13426=FACE_OUTER_BOUND('',#19386,.T.);
#13427=FACE_OUTER_BOUND('',#19387,.T.);
#13428=FACE_OUTER_BOUND('',#19388,.T.);
#13429=FACE_OUTER_BOUND('',#19390,.T.);
#13430=FACE_OUTER_BOUND('',#19391,.T.);
#13431=FACE_OUTER_BOUND('',#19392,.T.);
#13432=FACE_OUTER_BOUND('',#19393,.T.);
#13433=FACE_OUTER_BOUND('',#19394,.T.);
#13434=FACE_OUTER_BOUND('',#19395,.T.);
#13435=FACE_OUTER_BOUND('',#19396,.T.);
#13436=FACE_OUTER_BOUND('',#19397,.T.);
#13437=FACE_OUTER_BOUND('',#19398,.T.);
#13438=FACE_OUTER_BOUND('',#19399,.T.);
#13439=FACE_OUTER_BOUND('',#19400,.T.);
#13440=FACE_OUTER_BOUND('',#19401,.T.);
#13441=FACE_OUTER_BOUND('',#19402,.T.);
#13442=FACE_OUTER_BOUND('',#19403,.T.);
#13443=FACE_OUTER_BOUND('',#19404,.T.);
#13444=FACE_OUTER_BOUND('',#19405,.T.);
#13445=FACE_OUTER_BOUND('',#19406,.T.);
#13446=FACE_OUTER_BOUND('',#19407,.T.);
#13447=FACE_OUTER_BOUND('',#19408,.T.);
#13448=FACE_OUTER_BOUND('',#19409,.T.);
#13449=FACE_OUTER_BOUND('',#19410,.T.);
#13450=FACE_OUTER_BOUND('',#19412,.T.);
#13451=FACE_OUTER_BOUND('',#19413,.T.);
#13452=FACE_OUTER_BOUND('',#19414,.T.);
#13453=FACE_OUTER_BOUND('',#19415,.T.);
#13454=FACE_OUTER_BOUND('',#19416,.T.);
#13455=FACE_OUTER_BOUND('',#19417,.T.);
#13456=FACE_OUTER_BOUND('',#19418,.T.);
#13457=FACE_OUTER_BOUND('',#19419,.T.);
#13458=FACE_OUTER_BOUND('',#19420,.T.);
#13459=FACE_OUTER_BOUND('',#19421,.T.);
#13460=FACE_OUTER_BOUND('',#19422,.T.);
#13461=FACE_OUTER_BOUND('',#19423,.T.);
#13462=FACE_OUTER_BOUND('',#19424,.T.);
#13463=FACE_OUTER_BOUND('',#19425,.T.);
#13464=FACE_OUTER_BOUND('',#19426,.T.);
#13465=FACE_OUTER_BOUND('',#19427,.T.);
#13466=FACE_OUTER_BOUND('',#19428,.T.);
#13467=FACE_OUTER_BOUND('',#19429,.T.);
#13468=FACE_OUTER_BOUND('',#19430,.T.);
#13469=FACE_OUTER_BOUND('',#19431,.T.);
#13470=FACE_OUTER_BOUND('',#19432,.T.);
#13471=FACE_OUTER_BOUND('',#19433,.T.);
#13472=FACE_OUTER_BOUND('',#19434,.T.);
#13473=FACE_OUTER_BOUND('',#19435,.T.);
#13474=FACE_OUTER_BOUND('',#19436,.T.);
#13475=FACE_OUTER_BOUND('',#19437,.T.);
#13476=FACE_OUTER_BOUND('',#19438,.T.);
#13477=FACE_OUTER_BOUND('',#19439,.T.);
#13478=FACE_OUTER_BOUND('',#19440,.T.);
#13479=FACE_OUTER_BOUND('',#19441,.T.);
#13480=FACE_OUTER_BOUND('',#19442,.T.);
#13481=FACE_OUTER_BOUND('',#19443,.T.);
#13482=FACE_OUTER_BOUND('',#19444,.T.);
#13483=FACE_OUTER_BOUND('',#19445,.T.);
#13484=FACE_OUTER_BOUND('',#19446,.T.);
#13485=FACE_OUTER_BOUND('',#19447,.T.);
#13486=FACE_OUTER_BOUND('',#19448,.T.);
#13487=FACE_OUTER_BOUND('',#19449,.T.);
#13488=FACE_OUTER_BOUND('',#19450,.T.);
#13489=FACE_OUTER_BOUND('',#19451,.T.);
#13490=FACE_OUTER_BOUND('',#19452,.T.);
#13491=FACE_OUTER_BOUND('',#19453,.T.);
#13492=FACE_OUTER_BOUND('',#19454,.T.);
#13493=FACE_OUTER_BOUND('',#19455,.T.);
#13494=FACE_OUTER_BOUND('',#19456,.T.);
#13495=FACE_OUTER_BOUND('',#19457,.T.);
#13496=FACE_OUTER_BOUND('',#19458,.T.);
#13497=FACE_OUTER_BOUND('',#19459,.T.);
#13498=FACE_OUTER_BOUND('',#19460,.T.);
#13499=FACE_OUTER_BOUND('',#19461,.T.);
#13500=FACE_OUTER_BOUND('',#19462,.T.);
#13501=FACE_OUTER_BOUND('',#19463,.T.);
#13502=FACE_OUTER_BOUND('',#19464,.T.);
#13503=FACE_OUTER_BOUND('',#19465,.T.);
#13504=FACE_OUTER_BOUND('',#19466,.T.);
#13505=FACE_OUTER_BOUND('',#19467,.T.);
#13506=FACE_OUTER_BOUND('',#19468,.T.);
#13507=FACE_OUTER_BOUND('',#19469,.T.);
#13508=FACE_OUTER_BOUND('',#19470,.T.);
#13509=FACE_OUTER_BOUND('',#19471,.T.);
#13510=FACE_OUTER_BOUND('',#19472,.T.);
#13511=FACE_OUTER_BOUND('',#19473,.T.);
#13512=FACE_OUTER_BOUND('',#19474,.T.);
#13513=FACE_OUTER_BOUND('',#19475,.T.);
#13514=FACE_OUTER_BOUND('',#19476,.T.);
#13515=FACE_OUTER_BOUND('',#19477,.T.);
#13516=FACE_OUTER_BOUND('',#19478,.T.);
#13517=FACE_OUTER_BOUND('',#19479,.T.);
#13518=FACE_OUTER_BOUND('',#19480,.T.);
#13519=FACE_OUTER_BOUND('',#19481,.T.);
#13520=FACE_OUTER_BOUND('',#19482,.T.);
#13521=FACE_OUTER_BOUND('',#19483,.T.);
#13522=FACE_OUTER_BOUND('',#19484,.T.);
#13523=FACE_OUTER_BOUND('',#19485,.T.);
#13524=FACE_OUTER_BOUND('',#19486,.T.);
#13525=FACE_OUTER_BOUND('',#19487,.T.);
#13526=FACE_OUTER_BOUND('',#19488,.T.);
#13527=FACE_OUTER_BOUND('',#19489,.T.);
#13528=FACE_OUTER_BOUND('',#19490,.T.);
#13529=FACE_OUTER_BOUND('',#19491,.T.);
#13530=FACE_OUTER_BOUND('',#19492,.T.);
#13531=FACE_OUTER_BOUND('',#19493,.T.);
#13532=FACE_OUTER_BOUND('',#19494,.T.);
#13533=FACE_OUTER_BOUND('',#19495,.T.);
#13534=FACE_OUTER_BOUND('',#19496,.T.);
#13535=FACE_OUTER_BOUND('',#19497,.T.);
#13536=FACE_OUTER_BOUND('',#19498,.T.);
#13537=FACE_OUTER_BOUND('',#19499,.T.);
#13538=FACE_OUTER_BOUND('',#19500,.T.);
#13539=FACE_OUTER_BOUND('',#19501,.T.);
#13540=FACE_OUTER_BOUND('',#19502,.T.);
#13541=FACE_OUTER_BOUND('',#19503,.T.);
#13542=FACE_OUTER_BOUND('',#19504,.T.);
#13543=FACE_OUTER_BOUND('',#19505,.T.);
#13544=FACE_OUTER_BOUND('',#19506,.T.);
#13545=FACE_OUTER_BOUND('',#19507,.T.);
#13546=FACE_OUTER_BOUND('',#19508,.T.);
#13547=FACE_OUTER_BOUND('',#19509,.T.);
#13548=FACE_OUTER_BOUND('',#19510,.T.);
#13549=FACE_OUTER_BOUND('',#19511,.T.);
#13550=FACE_OUTER_BOUND('',#19512,.T.);
#13551=FACE_OUTER_BOUND('',#19513,.T.);
#13552=FACE_OUTER_BOUND('',#19514,.T.);
#13553=FACE_OUTER_BOUND('',#19515,.T.);
#13554=FACE_OUTER_BOUND('',#19516,.T.);
#13555=FACE_OUTER_BOUND('',#19517,.T.);
#13556=FACE_OUTER_BOUND('',#19518,.T.);
#13557=FACE_OUTER_BOUND('',#19519,.T.);
#13558=FACE_OUTER_BOUND('',#19520,.T.);
#13559=FACE_OUTER_BOUND('',#19521,.T.);
#13560=FACE_OUTER_BOUND('',#19522,.T.);
#13561=FACE_OUTER_BOUND('',#19523,.T.);
#13562=FACE_OUTER_BOUND('',#19524,.T.);
#13563=FACE_OUTER_BOUND('',#19525,.T.);
#13564=FACE_OUTER_BOUND('',#19526,.T.);
#13565=FACE_OUTER_BOUND('',#19527,.T.);
#13566=FACE_OUTER_BOUND('',#19528,.T.);
#13567=FACE_OUTER_BOUND('',#19529,.T.);
#13568=FACE_OUTER_BOUND('',#19530,.T.);
#13569=FACE_OUTER_BOUND('',#19531,.T.);
#13570=FACE_OUTER_BOUND('',#19532,.T.);
#13571=FACE_OUTER_BOUND('',#19533,.T.);
#13572=FACE_OUTER_BOUND('',#19534,.T.);
#13573=FACE_OUTER_BOUND('',#19535,.T.);
#13574=FACE_OUTER_BOUND('',#19536,.T.);
#13575=FACE_OUTER_BOUND('',#19537,.T.);
#13576=FACE_OUTER_BOUND('',#19538,.T.);
#13577=FACE_OUTER_BOUND('',#19539,.T.);
#13578=FACE_OUTER_BOUND('',#19540,.T.);
#13579=FACE_OUTER_BOUND('',#19541,.T.);
#13580=FACE_OUTER_BOUND('',#19542,.T.);
#13581=FACE_OUTER_BOUND('',#19543,.T.);
#13582=FACE_OUTER_BOUND('',#19544,.T.);
#13583=FACE_OUTER_BOUND('',#19545,.T.);
#13584=FACE_OUTER_BOUND('',#19546,.T.);
#13585=FACE_OUTER_BOUND('',#19547,.T.);
#13586=FACE_OUTER_BOUND('',#19548,.T.);
#13587=FACE_OUTER_BOUND('',#19549,.T.);
#13588=FACE_OUTER_BOUND('',#19550,.T.);
#13589=FACE_OUTER_BOUND('',#19551,.T.);
#13590=FACE_OUTER_BOUND('',#19552,.T.);
#13591=FACE_OUTER_BOUND('',#19553,.T.);
#13592=FACE_OUTER_BOUND('',#19554,.T.);
#13593=FACE_OUTER_BOUND('',#19555,.T.);
#13594=FACE_OUTER_BOUND('',#19556,.T.);
#13595=FACE_OUTER_BOUND('',#19561,.T.);
#13596=FACE_OUTER_BOUND('',#19562,.T.);
#13597=FACE_OUTER_BOUND('',#19563,.T.);
#13598=FACE_OUTER_BOUND('',#19564,.T.);
#13599=FACE_OUTER_BOUND('',#19565,.T.);
#13600=FACE_OUTER_BOUND('',#19566,.T.);
#13601=FACE_OUTER_BOUND('',#19567,.T.);
#13602=FACE_OUTER_BOUND('',#19568,.T.);
#13603=FACE_OUTER_BOUND('',#19573,.T.);
#13604=FACE_OUTER_BOUND('',#19574,.T.);
#13605=FACE_OUTER_BOUND('',#19575,.T.);
#13606=FACE_OUTER_BOUND('',#19576,.T.);
#13607=FACE_OUTER_BOUND('',#19577,.T.);
#13608=FACE_OUTER_BOUND('',#19578,.T.);
#13609=FACE_OUTER_BOUND('',#19579,.T.);
#13610=FACE_OUTER_BOUND('',#19580,.T.);
#13611=FACE_OUTER_BOUND('',#19581,.T.);
#13612=FACE_OUTER_BOUND('',#19582,.T.);
#13613=FACE_OUTER_BOUND('',#19583,.T.);
#13614=FACE_OUTER_BOUND('',#19584,.T.);
#13615=FACE_OUTER_BOUND('',#19585,.T.);
#13616=FACE_OUTER_BOUND('',#19586,.T.);
#13617=FACE_OUTER_BOUND('',#19587,.T.);
#13618=FACE_OUTER_BOUND('',#19588,.T.);
#13619=FACE_OUTER_BOUND('',#19589,.T.);
#13620=FACE_OUTER_BOUND('',#19590,.T.);
#13621=FACE_OUTER_BOUND('',#19591,.T.);
#13622=FACE_OUTER_BOUND('',#19592,.T.);
#13623=FACE_OUTER_BOUND('',#19593,.T.);
#13624=FACE_OUTER_BOUND('',#19594,.T.);
#13625=FACE_OUTER_BOUND('',#19595,.T.);
#13626=FACE_OUTER_BOUND('',#19596,.T.);
#13627=FACE_OUTER_BOUND('',#19597,.T.);
#13628=FACE_OUTER_BOUND('',#19598,.T.);
#14527=EDGE_LOOP('',(#57945,#57946,#57947,#57948));
#14528=EDGE_LOOP('',(#57949));
#14529=EDGE_LOOP('',(#57950,#57951,#57952,#57953));
#14530=EDGE_LOOP('',(#57954));
#14531=EDGE_LOOP('',(#57955));
#14532=EDGE_LOOP('',(#57956,#57957,#57958,#57959));
#14533=EDGE_LOOP('',(#57960));
#14534=EDGE_LOOP('',(#57961,#57962,#57963,#57964));
#14535=EDGE_LOOP('',(#57965));
#14536=EDGE_LOOP('',(#57966,#57967,#57968,#57969));
#14537=EDGE_LOOP('',(#57970));
#14538=EDGE_LOOP('',(#57971));
#14539=EDGE_LOOP('',(#57972,#57973,#57974,#57975));
#14540=EDGE_LOOP('',(#57976));
#14541=EDGE_LOOP('',(#57977,#57978,#57979,#57980,#57981,#57982));
#14542=EDGE_LOOP('',(#57983,#57984,#57985,#57986,#57987));
#14543=EDGE_LOOP('',(#57988,#57989,#57990,#57991));
#14544=EDGE_LOOP('',(#57992,#57993,#57994,#57995));
#14545=EDGE_LOOP('',(#57996,#57997,#57998,#57999));
#14546=EDGE_LOOP('',(#58000,#58001,#58002,#58003,#58004,#58005,#58006,#58007,
#58008,#58009,#58010,#58011,#58012,#58013,#58014,#58015,#58016,#58017,#58018));
#14547=EDGE_LOOP('',(#58019,#58020,#58021,#58022));
#14548=EDGE_LOOP('',(#58023,#58024,#58025,#58026));
#14549=EDGE_LOOP('',(#58027,#58028,#58029,#58030));
#14550=EDGE_LOOP('',(#58031,#58032,#58033,#58034));
#14551=EDGE_LOOP('',(#58035,#58036,#58037,#58038,#58039,#58040,#58041,#58042,
#58043,#58044,#58045,#58046,#58047,#58048,#58049,#58050,#58051,#58052,#58053));
#14552=EDGE_LOOP('',(#58054,#58055,#58056,#58057));
#14553=EDGE_LOOP('',(#58058,#58059,#58060,#58061));
#14554=EDGE_LOOP('',(#58062,#58063,#58064,#58065));
#14555=EDGE_LOOP('',(#58066,#58067,#58068,#58069,#58070,#58071));
#14556=EDGE_LOOP('',(#58072,#58073,#58074,#58075,#58076));
#14557=EDGE_LOOP('',(#58077,#58078,#58079,#58080));
#14558=EDGE_LOOP('',(#58081,#58082,#58083,#58084));
#14559=EDGE_LOOP('',(#58085,#58086,#58087,#58088));
#14560=EDGE_LOOP('',(#58089,#58090,#58091,#58092));
#14561=EDGE_LOOP('',(#58093,#58094,#58095,#58096,#58097));
#14562=EDGE_LOOP('',(#58098,#58099,#58100,#58101));
#14563=EDGE_LOOP('',(#58102,#58103,#58104,#58105));
#14564=EDGE_LOOP('',(#58106,#58107,#58108,#58109));
#14565=EDGE_LOOP('',(#58110,#58111,#58112,#58113));
#14566=EDGE_LOOP('',(#58114,#58115,#58116,#58117));
#14567=EDGE_LOOP('',(#58118,#58119,#58120,#58121));
#14568=EDGE_LOOP('',(#58122,#58123,#58124,#58125));
#14569=EDGE_LOOP('',(#58126,#58127,#58128,#58129));
#14570=EDGE_LOOP('',(#58130,#58131,#58132,#58133));
#14571=EDGE_LOOP('',(#58134,#58135,#58136,#58137));
#14572=EDGE_LOOP('',(#58138,#58139,#58140,#58141));
#14573=EDGE_LOOP('',(#58142,#58143,#58144,#58145));
#14574=EDGE_LOOP('',(#58146,#58147,#58148,#58149));
#14575=EDGE_LOOP('',(#58150,#58151,#58152,#58153));
#14576=EDGE_LOOP('',(#58154,#58155,#58156,#58157));
#14577=EDGE_LOOP('',(#58158,#58159,#58160,#58161));
#14578=EDGE_LOOP('',(#58162,#58163,#58164,#58165));
#14579=EDGE_LOOP('',(#58166,#58167,#58168,#58169));
#14580=EDGE_LOOP('',(#58170,#58171,#58172,#58173));
#14581=EDGE_LOOP('',(#58174,#58175,#58176,#58177));
#14582=EDGE_LOOP('',(#58178,#58179,#58180,#58181));
#14583=EDGE_LOOP('',(#58182,#58183,#58184,#58185));
#14584=EDGE_LOOP('',(#58186,#58187,#58188,#58189));
#14585=EDGE_LOOP('',(#58190,#58191,#58192,#58193));
#14586=EDGE_LOOP('',(#58194,#58195,#58196,#58197));
#14587=EDGE_LOOP('',(#58198,#58199,#58200,#58201));
#14588=EDGE_LOOP('',(#58202,#58203,#58204,#58205));
#14589=EDGE_LOOP('',(#58206,#58207,#58208,#58209));
#14590=EDGE_LOOP('',(#58210,#58211,#58212,#58213));
#14591=EDGE_LOOP('',(#58214,#58215,#58216,#58217));
#14592=EDGE_LOOP('',(#58218,#58219,#58220,#58221,#58222,#58223));
#14593=EDGE_LOOP('',(#58224,#58225,#58226,#58227,#58228,#58229,#58230,#58231,
#58232,#58233,#58234,#58235,#58236,#58237,#58238,#58239,#58240,#58241,#58242,
#58243,#58244,#58245,#58246,#58247,#58248,#58249,#58250,#58251,#58252,#58253,
#58254,#58255,#58256,#58257,#58258,#58259,#58260,#58261));
#14594=EDGE_LOOP('',(#58262,#58263,#58264,#58265));
#14595=EDGE_LOOP('',(#58266,#58267,#58268,#58269));
#14596=EDGE_LOOP('',(#58270,#58271,#58272,#58273));
#14597=EDGE_LOOP('',(#58274,#58275,#58276,#58277));
#14598=EDGE_LOOP('',(#58278,#58279,#58280,#58281,#58282,#58283,#58284,#58285,
#58286,#58287,#58288,#58289,#58290,#58291,#58292,#58293,#58294,#58295,#58296));
#14599=EDGE_LOOP('',(#58297,#58298,#58299,#58300));
#14600=EDGE_LOOP('',(#58301,#58302,#58303,#58304));
#14601=EDGE_LOOP('',(#58305,#58306,#58307,#58308));
#14602=EDGE_LOOP('',(#58309,#58310,#58311,#58312));
#14603=EDGE_LOOP('',(#58313,#58314,#58315,#58316,#58317,#58318,#58319,#58320,
#58321,#58322,#58323,#58324,#58325,#58326,#58327,#58328));
#14604=EDGE_LOOP('',(#58329,#58330,#58331,#58332));
#14605=EDGE_LOOP('',(#58333,#58334,#58335,#58336));
#14606=EDGE_LOOP('',(#58337,#58338,#58339,#58340));
#14607=EDGE_LOOP('',(#58341,#58342,#58343,#58344));
#14608=EDGE_LOOP('',(#58345,#58346,#58347,#58348));
#14609=EDGE_LOOP('',(#58349,#58350,#58351,#58352));
#14610=EDGE_LOOP('',(#58353,#58354,#58355,#58356));
#14611=EDGE_LOOP('',(#58357,#58358,#58359,#58360));
#14612=EDGE_LOOP('',(#58361,#58362,#58363,#58364));
#14613=EDGE_LOOP('',(#58365,#58366,#58367,#58368));
#14614=EDGE_LOOP('',(#58369,#58370,#58371,#58372));
#14615=EDGE_LOOP('',(#58373,#58374,#58375,#58376));
#14616=EDGE_LOOP('',(#58377,#58378,#58379,#58380));
#14617=EDGE_LOOP('',(#58381,#58382,#58383,#58384));
#14618=EDGE_LOOP('',(#58385,#58386,#58387,#58388));
#14619=EDGE_LOOP('',(#58389,#58390,#58391,#58392));
#14620=EDGE_LOOP('',(#58393,#58394,#58395,#58396));
#14621=EDGE_LOOP('',(#58397,#58398,#58399,#58400));
#14622=EDGE_LOOP('',(#58401,#58402,#58403,#58404));
#14623=EDGE_LOOP('',(#58405,#58406,#58407,#58408));
#14624=EDGE_LOOP('',(#58409,#58410,#58411,#58412));
#14625=EDGE_LOOP('',(#58413,#58414,#58415,#58416));
#14626=EDGE_LOOP('',(#58417,#58418,#58419,#58420));
#14627=EDGE_LOOP('',(#58421,#58422,#58423,#58424));
#14628=EDGE_LOOP('',(#58425,#58426,#58427,#58428));
#14629=EDGE_LOOP('',(#58429,#58430,#58431,#58432));
#14630=EDGE_LOOP('',(#58433,#58434,#58435,#58436));
#14631=EDGE_LOOP('',(#58437,#58438,#58439,#58440));
#14632=EDGE_LOOP('',(#58441,#58442,#58443,#58444));
#14633=EDGE_LOOP('',(#58445,#58446,#58447,#58448));
#14634=EDGE_LOOP('',(#58449,#58450,#58451,#58452));
#14635=EDGE_LOOP('',(#58453,#58454,#58455,#58456));
#14636=EDGE_LOOP('',(#58457,#58458,#58459,#58460));
#14637=EDGE_LOOP('',(#58461,#58462,#58463,#58464));
#14638=EDGE_LOOP('',(#58465,#58466,#58467,#58468));
#14639=EDGE_LOOP('',(#58469,#58470,#58471,#58472));
#14640=EDGE_LOOP('',(#58473,#58474,#58475,#58476));
#14641=EDGE_LOOP('',(#58477,#58478,#58479,#58480));
#14642=EDGE_LOOP('',(#58481,#58482,#58483,#58484));
#14643=EDGE_LOOP('',(#58485,#58486,#58487,#58488));
#14644=EDGE_LOOP('',(#58489,#58490,#58491,#58492));
#14645=EDGE_LOOP('',(#58493,#58494,#58495,#58496));
#14646=EDGE_LOOP('',(#58497,#58498,#58499,#58500));
#14647=EDGE_LOOP('',(#58501,#58502,#58503,#58504));
#14648=EDGE_LOOP('',(#58505,#58506,#58507,#58508));
#14649=EDGE_LOOP('',(#58509,#58510,#58511,#58512));
#14650=EDGE_LOOP('',(#58513,#58514,#58515,#58516));
#14651=EDGE_LOOP('',(#58517,#58518,#58519,#58520));
#14652=EDGE_LOOP('',(#58521,#58522,#58523,#58524));
#14653=EDGE_LOOP('',(#58525,#58526,#58527,#58528));
#14654=EDGE_LOOP('',(#58529,#58530,#58531,#58532));
#14655=EDGE_LOOP('',(#58533,#58534,#58535,#58536));
#14656=EDGE_LOOP('',(#58537,#58538,#58539,#58540));
#14657=EDGE_LOOP('',(#58541,#58542,#58543,#58544));
#14658=EDGE_LOOP('',(#58545,#58546,#58547,#58548));
#14659=EDGE_LOOP('',(#58549,#58550,#58551,#58552));
#14660=EDGE_LOOP('',(#58553,#58554,#58555,#58556));
#14661=EDGE_LOOP('',(#58557,#58558,#58559,#58560));
#14662=EDGE_LOOP('',(#58561,#58562,#58563,#58564));
#14663=EDGE_LOOP('',(#58565,#58566,#58567,#58568));
#14664=EDGE_LOOP('',(#58569,#58570,#58571,#58572));
#14665=EDGE_LOOP('',(#58573,#58574,#58575,#58576));
#14666=EDGE_LOOP('',(#58577,#58578,#58579,#58580));
#14667=EDGE_LOOP('',(#58581,#58582,#58583,#58584));
#14668=EDGE_LOOP('',(#58585,#58586,#58587,#58588));
#14669=EDGE_LOOP('',(#58589,#58590,#58591,#58592));
#14670=EDGE_LOOP('',(#58593,#58594,#58595,#58596));
#14671=EDGE_LOOP('',(#58597,#58598,#58599,#58600));
#14672=EDGE_LOOP('',(#58601,#58602,#58603,#58604));
#14673=EDGE_LOOP('',(#58605,#58606,#58607,#58608));
#14674=EDGE_LOOP('',(#58609,#58610,#58611,#58612));
#14675=EDGE_LOOP('',(#58613,#58614,#58615,#58616));
#14676=EDGE_LOOP('',(#58617,#58618,#58619,#58620));
#14677=EDGE_LOOP('',(#58621,#58622,#58623,#58624));
#14678=EDGE_LOOP('',(#58625,#58626,#58627,#58628));
#14679=EDGE_LOOP('',(#58629,#58630,#58631,#58632));
#14680=EDGE_LOOP('',(#58633,#58634,#58635,#58636,#58637));
#14681=EDGE_LOOP('',(#58638,#58639,#58640,#58641));
#14682=EDGE_LOOP('',(#58642,#58643,#58644,#58645));
#14683=EDGE_LOOP('',(#58646,#58647,#58648,#58649));
#14684=EDGE_LOOP('',(#58650,#58651,#58652,#58653));
#14685=EDGE_LOOP('',(#58654,#58655,#58656,#58657));
#14686=EDGE_LOOP('',(#58658,#58659,#58660,#58661));
#14687=EDGE_LOOP('',(#58662,#58663,#58664,#58665));
#14688=EDGE_LOOP('',(#58666,#58667,#58668,#58669));
#14689=EDGE_LOOP('',(#58670,#58671,#58672,#58673));
#14690=EDGE_LOOP('',(#58674,#58675,#58676,#58677));
#14691=EDGE_LOOP('',(#58678,#58679,#58680,#58681));
#14692=EDGE_LOOP('',(#58682,#58683,#58684,#58685));
#14693=EDGE_LOOP('',(#58686,#58687,#58688,#58689));
#14694=EDGE_LOOP('',(#58690,#58691,#58692,#58693));
#14695=EDGE_LOOP('',(#58694,#58695,#58696,#58697));
#14696=EDGE_LOOP('',(#58698,#58699,#58700,#58701));
#14697=EDGE_LOOP('',(#58702,#58703,#58704,#58705));
#14698=EDGE_LOOP('',(#58706,#58707,#58708,#58709));
#14699=EDGE_LOOP('',(#58710,#58711,#58712,#58713));
#14700=EDGE_LOOP('',(#58714,#58715,#58716,#58717,#58718));
#14701=EDGE_LOOP('',(#58719,#58720,#58721,#58722,#58723,#58724));
#14702=EDGE_LOOP('',(#58725,#58726,#58727,#58728));
#14703=EDGE_LOOP('',(#58729,#58730,#58731,#58732,#58733,#58734,#58735,#58736,
#58737,#58738,#58739,#58740));
#14704=EDGE_LOOP('',(#58741,#58742,#58743,#58744,#58745,#58746,#58747,#58748,
#58749));
#14705=EDGE_LOOP('',(#58750,#58751,#58752,#58753,#58754));
#14706=EDGE_LOOP('',(#58755,#58756,#58757,#58758,#58759));
#14707=EDGE_LOOP('',(#58760,#58761,#58762,#58763));
#14708=EDGE_LOOP('',(#58764,#58765,#58766,#58767));
#14709=EDGE_LOOP('',(#58768,#58769,#58770,#58771,#58772));
#14710=EDGE_LOOP('',(#58773,#58774,#58775,#58776));
#14711=EDGE_LOOP('',(#58777,#58778,#58779,#58780));
#14712=EDGE_LOOP('',(#58781,#58782,#58783,#58784,#58785,#58786,#58787,#58788,
#58789));
#14713=EDGE_LOOP('',(#58790,#58791,#58792,#58793));
#14714=EDGE_LOOP('',(#58794,#58795,#58796,#58797));
#14715=EDGE_LOOP('',(#58798,#58799,#58800,#58801));
#14716=EDGE_LOOP('',(#58802,#58803,#58804,#58805));
#14717=EDGE_LOOP('',(#58806,#58807,#58808,#58809));
#14718=EDGE_LOOP('',(#58810,#58811,#58812,#58813,#58814,#58815));
#14719=EDGE_LOOP('',(#58816,#58817,#58818,#58819));
#14720=EDGE_LOOP('',(#58820,#58821,#58822,#58823));
#14721=EDGE_LOOP('',(#58824,#58825,#58826,#58827));
#14722=EDGE_LOOP('',(#58828,#58829,#58830,#58831));
#14723=EDGE_LOOP('',(#58832,#58833,#58834,#58835));
#14724=EDGE_LOOP('',(#58836,#58837,#58838));
#14725=EDGE_LOOP('',(#58839,#58840,#58841,#58842,#58843));
#14726=EDGE_LOOP('',(#58844,#58845,#58846,#58847));
#14727=EDGE_LOOP('',(#58848,#58849,#58850,#58851));
#14728=EDGE_LOOP('',(#58852,#58853,#58854,#58855));
#14729=EDGE_LOOP('',(#58856,#58857,#58858,#58859));
#14730=EDGE_LOOP('',(#58860,#58861,#58862,#58863));
#14731=EDGE_LOOP('',(#58864,#58865,#58866,#58867));
#14732=EDGE_LOOP('',(#58868,#58869,#58870,#58871));
#14733=EDGE_LOOP('',(#58872,#58873,#58874,#58875));
#14734=EDGE_LOOP('',(#58876,#58877,#58878,#58879));
#14735=EDGE_LOOP('',(#58880,#58881,#58882,#58883));
#14736=EDGE_LOOP('',(#58884,#58885,#58886,#58887));
#14737=EDGE_LOOP('',(#58888,#58889,#58890,#58891));
#14738=EDGE_LOOP('',(#58892,#58893,#58894,#58895));
#14739=EDGE_LOOP('',(#58896,#58897,#58898,#58899));
#14740=EDGE_LOOP('',(#58900,#58901,#58902,#58903,#58904,#58905,#58906,#58907,
#58908));
#14741=EDGE_LOOP('',(#58909,#58910,#58911,#58912));
#14742=EDGE_LOOP('',(#58913,#58914,#58915,#58916));
#14743=EDGE_LOOP('',(#58917,#58918,#58919,#58920));
#14744=EDGE_LOOP('',(#58921,#58922,#58923,#58924));
#14745=EDGE_LOOP('',(#58925,#58926,#58927,#58928));
#14746=EDGE_LOOP('',(#58929,#58930,#58931,#58932));
#14747=EDGE_LOOP('',(#58933,#58934,#58935,#58936));
#14748=EDGE_LOOP('',(#58937,#58938,#58939,#58940));
#14749=EDGE_LOOP('',(#58941,#58942,#58943,#58944));
#14750=EDGE_LOOP('',(#58945,#58946,#58947,#58948));
#14751=EDGE_LOOP('',(#58949,#58950,#58951,#58952));
#14752=EDGE_LOOP('',(#58953,#58954,#58955,#58956));
#14753=EDGE_LOOP('',(#58957,#58958,#58959,#58960));
#14754=EDGE_LOOP('',(#58961,#58962,#58963,#58964));
#14755=EDGE_LOOP('',(#58965,#58966,#58967,#58968));
#14756=EDGE_LOOP('',(#58969,#58970,#58971,#58972));
#14757=EDGE_LOOP('',(#58973,#58974,#58975,#58976));
#14758=EDGE_LOOP('',(#58977,#58978,#58979,#58980));
#14759=EDGE_LOOP('',(#58981,#58982,#58983,#58984));
#14760=EDGE_LOOP('',(#58985,#58986,#58987,#58988,#58989,#58990,#58991,#58992));
#14761=EDGE_LOOP('',(#58993,#58994,#58995,#58996,#58997,#58998,#58999,#59000));
#14762=EDGE_LOOP('',(#59001,#59002,#59003,#59004));
#14763=EDGE_LOOP('',(#59005,#59006,#59007,#59008));
#14764=EDGE_LOOP('',(#59009,#59010,#59011,#59012));
#14765=EDGE_LOOP('',(#59013,#59014,#59015,#59016));
#14766=EDGE_LOOP('',(#59017,#59018,#59019,#59020));
#14767=EDGE_LOOP('',(#59021,#59022,#59023,#59024));
#14768=EDGE_LOOP('',(#59025,#59026,#59027,#59028));
#14769=EDGE_LOOP('',(#59029,#59030,#59031,#59032));
#14770=EDGE_LOOP('',(#59033,#59034,#59035,#59036));
#14771=EDGE_LOOP('',(#59037,#59038,#59039,#59040));
#14772=EDGE_LOOP('',(#59041,#59042,#59043,#59044));
#14773=EDGE_LOOP('',(#59045,#59046,#59047,#59048));
#14774=EDGE_LOOP('',(#59049,#59050,#59051,#59052));
#14775=EDGE_LOOP('',(#59053,#59054,#59055,#59056));
#14776=EDGE_LOOP('',(#59057,#59058,#59059,#59060));
#14777=EDGE_LOOP('',(#59061,#59062,#59063,#59064));
#14778=EDGE_LOOP('',(#59065,#59066,#59067,#59068));
#14779=EDGE_LOOP('',(#59069,#59070,#59071,#59072,#59073,#59074));
#14780=EDGE_LOOP('',(#59075,#59076,#59077,#59078));
#14781=EDGE_LOOP('',(#59079,#59080,#59081,#59082));
#14782=EDGE_LOOP('',(#59083,#59084,#59085,#59086));
#14783=EDGE_LOOP('',(#59087,#59088,#59089,#59090));
#14784=EDGE_LOOP('',(#59091,#59092,#59093,#59094));
#14785=EDGE_LOOP('',(#59095,#59096,#59097,#59098));
#14786=EDGE_LOOP('',(#59099,#59100,#59101,#59102,#59103,#59104,#59105,#59106,
#59107,#59108,#59109,#59110));
#14787=EDGE_LOOP('',(#59111,#59112,#59113,#59114));
#14788=EDGE_LOOP('',(#59115,#59116,#59117,#59118,#59119));
#14789=EDGE_LOOP('',(#59120,#59121,#59122,#59123,#59124,#59125,#59126,#59127,
#59128,#59129,#59130,#59131));
#14790=EDGE_LOOP('',(#59132,#59133,#59134,#59135));
#14791=EDGE_LOOP('',(#59136,#59137,#59138,#59139));
#14792=EDGE_LOOP('',(#59140,#59141,#59142,#59143));
#14793=EDGE_LOOP('',(#59144,#59145,#59146,#59147));
#14794=EDGE_LOOP('',(#59148,#59149,#59150,#59151,#59152,#59153,#59154,#59155,
#59156,#59157,#59158,#59159));
#14795=EDGE_LOOP('',(#59160,#59161,#59162,#59163));
#14796=EDGE_LOOP('',(#59164,#59165,#59166,#59167,#59168));
#14797=EDGE_LOOP('',(#59169,#59170,#59171,#59172,#59173,#59174,#59175,#59176,
#59177,#59178,#59179,#59180,#59181,#59182));
#14798=EDGE_LOOP('',(#59183,#59184,#59185,#59186));
#14799=EDGE_LOOP('',(#59187,#59188,#59189,#59190));
#14800=EDGE_LOOP('',(#59191,#59192,#59193,#59194));
#14801=EDGE_LOOP('',(#59195,#59196,#59197,#59198));
#14802=EDGE_LOOP('',(#59199,#59200,#59201,#59202,#59203,#59204,#59205,#59206,
#59207,#59208,#59209,#59210,#59211,#59212));
#14803=EDGE_LOOP('',(#59213,#59214,#59215,#59216));
#14804=EDGE_LOOP('',(#59217,#59218,#59219,#59220));
#14805=EDGE_LOOP('',(#59221,#59222,#59223,#59224,#59225,#59226,#59227,#59228,
#59229,#59230,#59231,#59232,#59233,#59234));
#14806=EDGE_LOOP('',(#59235,#59236,#59237,#59238));
#14807=EDGE_LOOP('',(#59239,#59240,#59241,#59242,#59243,#59244));
#14808=EDGE_LOOP('',(#59245,#59246,#59247,#59248));
#14809=EDGE_LOOP('',(#59249,#59250,#59251,#59252,#59253,#59254,#59255,#59256,
#59257,#59258,#59259));
#14810=EDGE_LOOP('',(#59260,#59261,#59262,#59263));
#14811=EDGE_LOOP('',(#59264,#59265,#59266,#59267));
#14812=EDGE_LOOP('',(#59268,#59269,#59270,#59271));
#14813=EDGE_LOOP('',(#59272,#59273,#59274,#59275,#59276,#59277,#59278,#59279,
#59280,#59281));
#14814=EDGE_LOOP('',(#59282,#59283,#59284,#59285));
#14815=EDGE_LOOP('',(#59286,#59287,#59288,#59289));
#14816=EDGE_LOOP('',(#59290,#59291,#59292,#59293));
#14817=EDGE_LOOP('',(#59294,#59295,#59296,#59297,#59298,#59299,#59300,#59301,
#59302));
#14818=EDGE_LOOP('',(#59303,#59304,#59305,#59306));
#14819=EDGE_LOOP('',(#59307,#59308,#59309,#59310));
#14820=EDGE_LOOP('',(#59311,#59312,#59313,#59314));
#14821=EDGE_LOOP('',(#59315,#59316,#59317,#59318));
#14822=EDGE_LOOP('',(#59319,#59320,#59321,#59322,#59323,#59324,#59325));
#14823=EDGE_LOOP('',(#59326,#59327,#59328,#59329));
#14824=EDGE_LOOP('',(#59330,#59331,#59332,#59333));
#14825=EDGE_LOOP('',(#59334,#59335,#59336,#59337,#59338,#59339,#59340));
#14826=EDGE_LOOP('',(#59341,#59342,#59343,#59344));
#14827=EDGE_LOOP('',(#59345,#59346,#59347,#59348));
#14828=EDGE_LOOP('',(#59349,#59350,#59351,#59352));
#14829=EDGE_LOOP('',(#59353,#59354,#59355,#59356,#59357,#59358,#59359));
#14830=EDGE_LOOP('',(#59360,#59361,#59362,#59363,#59364));
#14831=EDGE_LOOP('',(#59365,#59366,#59367,#59368));
#14832=EDGE_LOOP('',(#59369,#59370,#59371,#59372,#59373));
#14833=EDGE_LOOP('',(#59374,#59375,#59376,#59377,#59378));
#14834=EDGE_LOOP('',(#59379,#59380,#59381,#59382));
#14835=EDGE_LOOP('',(#59383,#59384,#59385,#59386,#59387));
#14836=EDGE_LOOP('',(#59388,#59389,#59390,#59391,#59392,#59393,#59394,#59395,
#59396,#59397,#59398,#59399,#59400,#59401));
#14837=EDGE_LOOP('',(#59402,#59403,#59404,#59405));
#14838=EDGE_LOOP('',(#59406,#59407,#59408,#59409));
#14839=EDGE_LOOP('',(#59410,#59411,#59412,#59413));
#14840=EDGE_LOOP('',(#59414,#59415,#59416,#59417,#59418,#59419,#59420,#59421,
#59422,#59423,#59424,#59425,#59426,#59427));
#14841=EDGE_LOOP('',(#59428,#59429,#59430,#59431));
#14842=EDGE_LOOP('',(#59432,#59433,#59434,#59435));
#14843=EDGE_LOOP('',(#59436,#59437,#59438,#59439));
#14844=EDGE_LOOP('',(#59440,#59441,#59442,#59443));
#14845=EDGE_LOOP('',(#59444,#59445,#59446,#59447,#59448,#59449,#59450,#59451,
#59452,#59453,#59454,#59455,#59456));
#14846=EDGE_LOOP('',(#59457,#59458,#59459,#59460));
#14847=EDGE_LOOP('',(#59461,#59462,#59463,#59464));
#14848=EDGE_LOOP('',(#59465,#59466,#59467,#59468,#59469,#59470,#59471,#59472,
#59473,#59474,#59475,#59476));
#14849=EDGE_LOOP('',(#59477,#59478,#59479,#59480));
#14850=EDGE_LOOP('',(#59481,#59482,#59483,#59484));
#14851=EDGE_LOOP('',(#59485,#59486,#59487,#59488));
#14852=EDGE_LOOP('',(#59489,#59490,#59491,#59492));
#14853=EDGE_LOOP('',(#59493,#59494,#59495,#59496,#59497,#59498,#59499,#59500,
#59501,#59502,#59503,#59504));
#14854=EDGE_LOOP('',(#59505,#59506,#59507,#59508));
#14855=EDGE_LOOP('',(#59509,#59510,#59511,#59512));
#14856=EDGE_LOOP('',(#59513,#59514,#59515,#59516,#59517,#59518,#59519,#59520,
#59521,#59522,#59523,#59524));
#14857=EDGE_LOOP('',(#59525,#59526,#59527,#59528));
#14858=EDGE_LOOP('',(#59529,#59530,#59531,#59532));
#14859=EDGE_LOOP('',(#59533,#59534,#59535,#59536));
#14860=EDGE_LOOP('',(#59537,#59538,#59539,#59540));
#14861=EDGE_LOOP('',(#59541,#59542,#59543,#59544,#59545,#59546,#59547,#59548,
#59549,#59550,#59551,#59552));
#14862=EDGE_LOOP('',(#59553,#59554,#59555,#59556));
#14863=EDGE_LOOP('',(#59557,#59558,#59559,#59560));
#14864=EDGE_LOOP('',(#59561,#59562,#59563,#59564,#59565,#59566,#59567,#59568,
#59569,#59570,#59571,#59572));
#14865=EDGE_LOOP('',(#59573,#59574,#59575,#59576));
#14866=EDGE_LOOP('',(#59577,#59578,#59579,#59580));
#14867=EDGE_LOOP('',(#59581,#59582,#59583,#59584));
#14868=EDGE_LOOP('',(#59585,#59586,#59587,#59588));
#14869=EDGE_LOOP('',(#59589,#59590,#59591,#59592,#59593,#59594,#59595,#59596,
#59597,#59598,#59599,#59600));
#14870=EDGE_LOOP('',(#59601,#59602,#59603,#59604));
#14871=EDGE_LOOP('',(#59605,#59606,#59607,#59608));
#14872=EDGE_LOOP('',(#59609,#59610,#59611,#59612,#59613,#59614,#59615,#59616,
#59617,#59618,#59619,#59620,#59621));
#14873=EDGE_LOOP('',(#59622,#59623,#59624,#59625));
#14874=EDGE_LOOP('',(#59626,#59627,#59628,#59629));
#14875=EDGE_LOOP('',(#59630,#59631,#59632,#59633));
#14876=EDGE_LOOP('',(#59634,#59635,#59636,#59637));
#14877=EDGE_LOOP('',(#59638,#59639,#59640,#59641,#59642,#59643,#59644,#59645,
#59646,#59647,#59648,#59649,#59650,#59651));
#14878=EDGE_LOOP('',(#59652,#59653,#59654,#59655));
#14879=EDGE_LOOP('',(#59656,#59657,#59658,#59659));
#14880=EDGE_LOOP('',(#59660,#59661,#59662,#59663,#59664,#59665,#59666,#59667,
#59668,#59669,#59670,#59671,#59672,#59673));
#14881=EDGE_LOOP('',(#59674,#59675,#59676,#59677,#59678));
#14882=EDGE_LOOP('',(#59679,#59680,#59681,#59682));
#14883=EDGE_LOOP('',(#59683,#59684,#59685,#59686));
#14884=EDGE_LOOP('',(#59687,#59688,#59689,#59690,#59691,#59692,#59693,#59694,
#59695,#59696,#59697,#59698,#59699,#59700,#59701,#59702,#59703));
#14885=EDGE_LOOP('',(#59704,#59705,#59706,#59707));
#14886=EDGE_LOOP('',(#59708,#59709,#59710,#59711));
#14887=EDGE_LOOP('',(#59712,#59713,#59714,#59715));
#14888=EDGE_LOOP('',(#59716,#59717,#59718,#59719,#59720,#59721,#59722,#59723,
#59724,#59725,#59726,#59727,#59728,#59729,#59730,#59731));
#14889=EDGE_LOOP('',(#59732,#59733,#59734,#59735));
#14890=EDGE_LOOP('',(#59736,#59737,#59738,#59739));
#14891=EDGE_LOOP('',(#59740,#59741,#59742,#59743,#59744,#59745,#59746,#59747,
#59748,#59749,#59750,#59751,#59752,#59753,#59754,#59755));
#14892=EDGE_LOOP('',(#59756,#59757,#59758,#59759,#59760));
#14893=EDGE_LOOP('',(#59761,#59762,#59763));
#14894=EDGE_LOOP('',(#59764,#59765,#59766,#59767));
#14895=EDGE_LOOP('',(#59768,#59769,#59770,#59771,#59772,#59773,#59774,#59775,
#59776,#59777,#59778,#59779,#59780,#59781,#59782,#59783,#59784,#59785));
#14896=EDGE_LOOP('',(#59786,#59787,#59788,#59789));
#14897=EDGE_LOOP('',(#59790,#59791,#59792,#59793));
#14898=EDGE_LOOP('',(#59794,#59795,#59796,#59797));
#14899=EDGE_LOOP('',(#59798,#59799,#59800,#59801,#59802,#59803,#59804,#59805,
#59806,#59807,#59808,#59809,#59810,#59811,#59812,#59813,#59814,#59815));
#14900=EDGE_LOOP('',(#59816,#59817,#59818,#59819));
#14901=EDGE_LOOP('',(#59820,#59821,#59822,#59823));
#14902=EDGE_LOOP('',(#59824,#59825,#59826,#59827));
#14903=EDGE_LOOP('',(#59828,#59829,#59830,#59831,#59832,#59833,#59834,#59835,
#59836,#59837,#59838,#59839));
#14904=EDGE_LOOP('',(#59840,#59841,#59842,#59843));
#14905=EDGE_LOOP('',(#59844,#59845,#59846,#59847));
#14906=EDGE_LOOP('',(#59848,#59849,#59850,#59851));
#14907=EDGE_LOOP('',(#59852,#59853,#59854,#59855,#59856,#59857,#59858,#59859,
#59860,#59861,#59862));
#14908=EDGE_LOOP('',(#59863,#59864,#59865,#59866));
#14909=EDGE_LOOP('',(#59867,#59868,#59869,#59870));
#14910=EDGE_LOOP('',(#59871,#59872,#59873,#59874,#59875,#59876,#59877,#59878));
#14911=EDGE_LOOP('',(#59879,#59880,#59881,#59882));
#14912=EDGE_LOOP('',(#59883,#59884,#59885,#59886));
#14913=EDGE_LOOP('',(#59887,#59888,#59889,#59890));
#14914=EDGE_LOOP('',(#59891,#59892,#59893,#59894,#59895,#59896,#59897,#59898,
#59899,#59900,#59901,#59902));
#14915=EDGE_LOOP('',(#59903,#59904,#59905,#59906));
#14916=EDGE_LOOP('',(#59907,#59908,#59909,#59910));
#14917=EDGE_LOOP('',(#59911,#59912,#59913,#59914));
#14918=EDGE_LOOP('',(#59915,#59916,#59917,#59918,#59919,#59920,#59921,#59922,
#59923,#59924,#59925,#59926,#59927,#59928,#59929,#59930,#59931,#59932));
#14919=EDGE_LOOP('',(#59933,#59934,#59935,#59936));
#14920=EDGE_LOOP('',(#59937,#59938,#59939,#59940));
#14921=EDGE_LOOP('',(#59941,#59942,#59943,#59944));
#14922=EDGE_LOOP('',(#59945,#59946,#59947,#59948));
#14923=EDGE_LOOP('',(#59949,#59950,#59951,#59952,#59953,#59954,#59955,#59956,
#59957,#59958,#59959,#59960,#59961,#59962,#59963,#59964,#59965,#59966));
#14924=EDGE_LOOP('',(#59967,#59968,#59969,#59970,#59971,#59972,#59973,#59974,
#59975,#59976,#59977,#59978,#59979,#59980,#59981,#59982,#59983));
#14925=EDGE_LOOP('',(#59984,#59985,#59986,#59987));
#14926=EDGE_LOOP('',(#59988,#59989,#59990));
#14927=EDGE_LOOP('',(#59991,#59992,#59993,#59994,#59995,#59996));
#14928=EDGE_LOOP('',(#59997,#59998,#59999));
#14929=EDGE_LOOP('',(#60000,#60001,#60002,#60003));
#14930=EDGE_LOOP('',(#60004,#60005,#60006,#60007,#60008,#60009,#60010,#60011,
#60012,#60013,#60014,#60015,#60016,#60017,#60018,#60019,#60020,#60021));
#14931=EDGE_LOOP('',(#60022,#60023,#60024,#60025));
#14932=EDGE_LOOP('',(#60026,#60027,#60028,#60029));
#14933=EDGE_LOOP('',(#60030,#60031,#60032,#60033));
#14934=EDGE_LOOP('',(#60034,#60035,#60036,#60037,#60038,#60039,#60040,#60041,
#60042,#60043,#60044,#60045,#60046,#60047,#60048,#60049,#60050,#60051));
#14935=EDGE_LOOP('',(#60052,#60053,#60054,#60055,#60056));
#14936=EDGE_LOOP('',(#60057,#60058,#60059,#60060));
#14937=EDGE_LOOP('',(#60061,#60062,#60063,#60064,#60065,#60066,#60067,#60068,
#60069,#60070,#60071,#60072,#60073,#60074,#60075,#60076));
#14938=EDGE_LOOP('',(#60077,#60078,#60079,#60080));
#14939=EDGE_LOOP('',(#60081,#60082,#60083,#60084,#60085,#60086,#60087,#60088,
#60089,#60090,#60091,#60092,#60093,#60094,#60095,#60096));
#14940=EDGE_LOOP('',(#60097,#60098,#60099,#60100));
#14941=EDGE_LOOP('',(#60101,#60102,#60103,#60104));
#14942=EDGE_LOOP('',(#60105,#60106,#60107,#60108));
#14943=EDGE_LOOP('',(#60109,#60110,#60111,#60112,#60113,#60114,#60115,#60116,
#60117,#60118,#60119,#60120,#60121,#60122,#60123,#60124,#60125,#60126));
#14944=EDGE_LOOP('',(#60127,#60128,#60129,#60130));
#14945=EDGE_LOOP('',(#60131,#60132,#60133,#60134));
#14946=EDGE_LOOP('',(#60135,#60136,#60137,#60138));
#14947=EDGE_LOOP('',(#60139,#60140,#60141,#60142,#60143,#60144,#60145,#60146,
#60147,#60148,#60149,#60150,#60151,#60152,#60153,#60154,#60155,#60156));
#14948=EDGE_LOOP('',(#60157,#60158,#60159,#60160));
#14949=EDGE_LOOP('',(#60161,#60162,#60163,#60164));
#14950=EDGE_LOOP('',(#60165,#60166,#60167,#60168));
#14951=EDGE_LOOP('',(#60169,#60170,#60171,#60172,#60173));
#14952=EDGE_LOOP('',(#60174,#60175,#60176,#60177,#60178,#60179,#60180,#60181,
#60182,#60183,#60184,#60185,#60186,#60187,#60188,#60189,#60190,#60191));
#14953=EDGE_LOOP('',(#60192,#60193,#60194));
#14954=EDGE_LOOP('',(#60195,#60196,#60197,#60198));
#14955=EDGE_LOOP('',(#60199,#60200,#60201,#60202));
#14956=EDGE_LOOP('',(#60203));
#14957=EDGE_LOOP('',(#60204));
#14958=EDGE_LOOP('',(#60205,#60206,#60207,#60208,#60209,#60210));
#14959=EDGE_LOOP('',(#60211,#60212,#60213,#60214));
#14960=EDGE_LOOP('',(#60215,#60216,#60217,#60218));
#14961=EDGE_LOOP('',(#60219,#60220,#60221,#60222));
#14962=EDGE_LOOP('',(#60223,#60224,#60225,#60226));
#14963=EDGE_LOOP('',(#60227,#60228,#60229,#60230));
#14964=EDGE_LOOP('',(#60231,#60232,#60233,#60234));
#14965=EDGE_LOOP('',(#60235,#60236,#60237,#60238));
#14966=EDGE_LOOP('',(#60239));
#14967=EDGE_LOOP('',(#60240));
#14968=EDGE_LOOP('',(#60241,#60242,#60243,#60244,#60245,#60246,#60247,#60248));
#14969=EDGE_LOOP('',(#60249,#60250,#60251,#60252));
#14970=EDGE_LOOP('',(#60253,#60254,#60255,#60256));
#14971=EDGE_LOOP('',(#60257,#60258,#60259,#60260));
#14972=EDGE_LOOP('',(#60261,#60262,#60263,#60264));
#14973=EDGE_LOOP('',(#60265,#60266,#60267,#60268));
#14974=EDGE_LOOP('',(#60269,#60270,#60271,#60272));
#14975=EDGE_LOOP('',(#60273,#60274,#60275,#60276));
#14976=EDGE_LOOP('',(#60277,#60278,#60279,#60280));
#14977=EDGE_LOOP('',(#60281,#60282,#60283,#60284));
#14978=EDGE_LOOP('',(#60285,#60286,#60287,#60288));
#14979=EDGE_LOOP('',(#60289,#60290,#60291,#60292));
#14980=EDGE_LOOP('',(#60293,#60294,#60295,#60296));
#14981=EDGE_LOOP('',(#60297,#60298,#60299,#60300));
#14982=EDGE_LOOP('',(#60301,#60302,#60303,#60304));
#14983=EDGE_LOOP('',(#60305,#60306,#60307,#60308,#60309));
#14984=EDGE_LOOP('',(#60310,#60311,#60312,#60313,#60314));
#14985=EDGE_LOOP('',(#60315,#60316,#60317,#60318));
#14986=EDGE_LOOP('',(#60319,#60320,#60321,#60322));
#14987=EDGE_LOOP('',(#60323,#60324,#60325,#60326));
#14988=EDGE_LOOP('',(#60327,#60328,#60329,#60330));
#14989=EDGE_LOOP('',(#60331,#60332,#60333,#60334));
#14990=EDGE_LOOP('',(#60335,#60336,#60337,#60338,#60339));
#14991=EDGE_LOOP('',(#60340,#60341,#60342));
#14992=EDGE_LOOP('',(#60343,#60344,#60345,#60346));
#14993=EDGE_LOOP('',(#60347,#60348,#60349,#60350));
#14994=EDGE_LOOP('',(#60351,#60352,#60353,#60354));
#14995=EDGE_LOOP('',(#60355,#60356,#60357,#60358));
#14996=EDGE_LOOP('',(#60359,#60360,#60361,#60362));
#14997=EDGE_LOOP('',(#60363,#60364,#60365,#60366));
#14998=EDGE_LOOP('',(#60367,#60368,#60369,#60370));
#14999=EDGE_LOOP('',(#60371,#60372,#60373,#60374));
#15000=EDGE_LOOP('',(#60375,#60376,#60377,#60378));
#15001=EDGE_LOOP('',(#60379,#60380,#60381,#60382));
#15002=EDGE_LOOP('',(#60383,#60384,#60385,#60386));
#15003=EDGE_LOOP('',(#60387,#60388,#60389,#60390));
#15004=EDGE_LOOP('',(#60391,#60392,#60393,#60394));
#15005=EDGE_LOOP('',(#60395,#60396,#60397,#60398));
#15006=EDGE_LOOP('',(#60399,#60400,#60401,#60402));
#15007=EDGE_LOOP('',(#60403,#60404,#60405,#60406));
#15008=EDGE_LOOP('',(#60407,#60408,#60409,#60410));
#15009=EDGE_LOOP('',(#60411,#60412,#60413,#60414));
#15010=EDGE_LOOP('',(#60415,#60416,#60417,#60418));
#15011=EDGE_LOOP('',(#60419,#60420,#60421,#60422));
#15012=EDGE_LOOP('',(#60423,#60424,#60425,#60426,#60427,#60428,#60429));
#15013=EDGE_LOOP('',(#60430,#60431,#60432,#60433));
#15014=EDGE_LOOP('',(#60434,#60435,#60436,#60437));
#15015=EDGE_LOOP('',(#60438,#60439,#60440,#60441));
#15016=EDGE_LOOP('',(#60442,#60443,#60444,#60445,#60446,#60447,#60448,#60449,
#60450,#60451,#60452,#60453,#60454,#60455,#60456,#60457,#60458));
#15017=EDGE_LOOP('',(#60459,#60460,#60461,#60462,#60463,#60464));
#15018=EDGE_LOOP('',(#60465,#60466,#60467,#60468,#60469,#60470,#60471,#60472,
#60473,#60474,#60475,#60476,#60477,#60478,#60479,#60480,#60481,#60482,#60483,
#60484,#60485,#60486,#60487,#60488,#60489,#60490,#60491,#60492,#60493,#60494,
#60495,#60496,#60497,#60498,#60499,#60500,#60501,#60502,#60503,#60504,#60505,
#60506,#60507,#60508));
#15019=EDGE_LOOP('',(#60509,#60510,#60511,#60512,#60513,#60514));
#15020=EDGE_LOOP('',(#60515,#60516,#60517,#60518,#60519,#60520,#60521,#60522,
#60523,#60524,#60525,#60526,#60527,#60528,#60529,#60530,#60531));
#15021=EDGE_LOOP('',(#60532,#60533,#60534,#60535));
#15022=EDGE_LOOP('',(#60536,#60537,#60538,#60539));
#15023=EDGE_LOOP('',(#60540,#60541,#60542,#60543));
#15024=EDGE_LOOP('',(#60544,#60545,#60546,#60547,#60548,#60549,#60550,#60551,
#60552,#60553,#60554,#60555,#60556,#60557,#60558,#60559,#60560));
#15025=EDGE_LOOP('',(#60561,#60562,#60563,#60564));
#15026=EDGE_LOOP('',(#60565,#60566,#60567,#60568,#60569,#60570,#60571,#60572,
#60573));
#15027=EDGE_LOOP('',(#60574,#60575,#60576,#60577));
#15028=EDGE_LOOP('',(#60578,#60579,#60580,#60581));
#15029=EDGE_LOOP('',(#60582,#60583,#60584,#60585,#60586));
#15030=EDGE_LOOP('',(#60587,#60588,#60589,#60590,#60591,#60592,#60593,#60594));
#15031=EDGE_LOOP('',(#60595,#60596,#60597));
#15032=EDGE_LOOP('',(#60598,#60599,#60600,#60601));
#15033=EDGE_LOOP('',(#60602,#60603,#60604,#60605));
#15034=EDGE_LOOP('',(#60606,#60607,#60608,#60609));
#15035=EDGE_LOOP('',(#60610,#60611,#60612,#60613));
#15036=EDGE_LOOP('',(#60614,#60615,#60616,#60617));
#15037=EDGE_LOOP('',(#60618,#60619,#60620,#60621));
#15038=EDGE_LOOP('',(#60622,#60623,#60624,#60625));
#15039=EDGE_LOOP('',(#60626,#60627,#60628,#60629));
#15040=EDGE_LOOP('',(#60630,#60631,#60632,#60633));
#15041=EDGE_LOOP('',(#60634,#60635,#60636,#60637));
#15042=EDGE_LOOP('',(#60638,#60639,#60640,#60641));
#15043=EDGE_LOOP('',(#60642,#60643,#60644,#60645));
#15044=EDGE_LOOP('',(#60646,#60647,#60648,#60649));
#15045=EDGE_LOOP('',(#60650,#60651,#60652,#60653));
#15046=EDGE_LOOP('',(#60654,#60655,#60656,#60657));
#15047=EDGE_LOOP('',(#60658,#60659,#60660,#60661));
#15048=EDGE_LOOP('',(#60662,#60663,#60664,#60665));
#15049=EDGE_LOOP('',(#60666,#60667,#60668,#60669));
#15050=EDGE_LOOP('',(#60670,#60671,#60672,#60673));
#15051=EDGE_LOOP('',(#60674,#60675,#60676,#60677,#60678));
#15052=EDGE_LOOP('',(#60679,#60680,#60681,#60682));
#15053=EDGE_LOOP('',(#60683,#60684,#60685,#60686));
#15054=EDGE_LOOP('',(#60687,#60688,#60689,#60690));
#15055=EDGE_LOOP('',(#60691,#60692,#60693,#60694));
#15056=EDGE_LOOP('',(#60695,#60696,#60697,#60698));
#15057=EDGE_LOOP('',(#60699,#60700,#60701,#60702));
#15058=EDGE_LOOP('',(#60703,#60704,#60705,#60706));
#15059=EDGE_LOOP('',(#60707,#60708,#60709,#60710));
#15060=EDGE_LOOP('',(#60711,#60712,#60713,#60714));
#15061=EDGE_LOOP('',(#60715,#60716,#60717,#60718));
#15062=EDGE_LOOP('',(#60719,#60720,#60721,#60722));
#15063=EDGE_LOOP('',(#60723,#60724,#60725,#60726));
#15064=EDGE_LOOP('',(#60727,#60728,#60729,#60730));
#15065=EDGE_LOOP('',(#60731,#60732,#60733,#60734));
#15066=EDGE_LOOP('',(#60735,#60736,#60737,#60738));
#15067=EDGE_LOOP('',(#60739,#60740,#60741,#60742));
#15068=EDGE_LOOP('',(#60743,#60744,#60745,#60746));
#15069=EDGE_LOOP('',(#60747,#60748,#60749,#60750));
#15070=EDGE_LOOP('',(#60751,#60752,#60753,#60754));
#15071=EDGE_LOOP('',(#60755,#60756,#60757,#60758));
#15072=EDGE_LOOP('',(#60759,#60760,#60761,#60762));
#15073=EDGE_LOOP('',(#60763,#60764,#60765,#60766));
#15074=EDGE_LOOP('',(#60767,#60768,#60769,#60770));
#15075=EDGE_LOOP('',(#60771,#60772,#60773,#60774));
#15076=EDGE_LOOP('',(#60775,#60776,#60777,#60778));
#15077=EDGE_LOOP('',(#60779,#60780,#60781,#60782));
#15078=EDGE_LOOP('',(#60783,#60784,#60785,#60786));
#15079=EDGE_LOOP('',(#60787,#60788,#60789,#60790));
#15080=EDGE_LOOP('',(#60791,#60792,#60793,#60794));
#15081=EDGE_LOOP('',(#60795,#60796,#60797,#60798));
#15082=EDGE_LOOP('',(#60799,#60800,#60801,#60802));
#15083=EDGE_LOOP('',(#60803,#60804,#60805,#60806));
#15084=EDGE_LOOP('',(#60807,#60808,#60809,#60810));
#15085=EDGE_LOOP('',(#60811,#60812,#60813,#60814));
#15086=EDGE_LOOP('',(#60815,#60816,#60817,#60818));
#15087=EDGE_LOOP('',(#60819,#60820,#60821,#60822));
#15088=EDGE_LOOP('',(#60823,#60824,#60825,#60826));
#15089=EDGE_LOOP('',(#60827,#60828,#60829,#60830));
#15090=EDGE_LOOP('',(#60831,#60832,#60833,#60834));
#15091=EDGE_LOOP('',(#60835,#60836,#60837,#60838));
#15092=EDGE_LOOP('',(#60839,#60840,#60841,#60842));
#15093=EDGE_LOOP('',(#60843,#60844,#60845,#60846));
#15094=EDGE_LOOP('',(#60847,#60848,#60849,#60850));
#15095=EDGE_LOOP('',(#60851,#60852,#60853,#60854));
#15096=EDGE_LOOP('',(#60855,#60856,#60857,#60858));
#15097=EDGE_LOOP('',(#60859,#60860,#60861,#60862));
#15098=EDGE_LOOP('',(#60863,#60864,#60865,#60866));
#15099=EDGE_LOOP('',(#60867,#60868,#60869,#60870));
#15100=EDGE_LOOP('',(#60871,#60872,#60873,#60874));
#15101=EDGE_LOOP('',(#60875,#60876,#60877,#60878));
#15102=EDGE_LOOP('',(#60879,#60880,#60881,#60882));
#15103=EDGE_LOOP('',(#60883,#60884,#60885,#60886));
#15104=EDGE_LOOP('',(#60887,#60888,#60889,#60890));
#15105=EDGE_LOOP('',(#60891,#60892,#60893,#60894));
#15106=EDGE_LOOP('',(#60895,#60896,#60897,#60898));
#15107=EDGE_LOOP('',(#60899,#60900,#60901,#60902));
#15108=EDGE_LOOP('',(#60903,#60904,#60905,#60906));
#15109=EDGE_LOOP('',(#60907,#60908,#60909,#60910));
#15110=EDGE_LOOP('',(#60911,#60912,#60913,#60914));
#15111=EDGE_LOOP('',(#60915,#60916,#60917,#60918));
#15112=EDGE_LOOP('',(#60919,#60920,#60921,#60922));
#15113=EDGE_LOOP('',(#60923,#60924,#60925,#60926));
#15114=EDGE_LOOP('',(#60927,#60928,#60929,#60930));
#15115=EDGE_LOOP('',(#60931,#60932,#60933,#60934));
#15116=EDGE_LOOP('',(#60935,#60936,#60937,#60938));
#15117=EDGE_LOOP('',(#60939,#60940,#60941,#60942));
#15118=EDGE_LOOP('',(#60943,#60944,#60945,#60946));
#15119=EDGE_LOOP('',(#60947,#60948,#60949,#60950));
#15120=EDGE_LOOP('',(#60951,#60952,#60953,#60954));
#15121=EDGE_LOOP('',(#60955,#60956,#60957,#60958));
#15122=EDGE_LOOP('',(#60959,#60960,#60961,#60962));
#15123=EDGE_LOOP('',(#60963,#60964,#60965,#60966));
#15124=EDGE_LOOP('',(#60967,#60968,#60969,#60970));
#15125=EDGE_LOOP('',(#60971,#60972,#60973,#60974));
#15126=EDGE_LOOP('',(#60975,#60976,#60977,#60978));
#15127=EDGE_LOOP('',(#60979,#60980,#60981,#60982));
#15128=EDGE_LOOP('',(#60983,#60984,#60985,#60986));
#15129=EDGE_LOOP('',(#60987,#60988,#60989,#60990));
#15130=EDGE_LOOP('',(#60991,#60992,#60993,#60994));
#15131=EDGE_LOOP('',(#60995,#60996,#60997,#60998));
#15132=EDGE_LOOP('',(#60999,#61000,#61001,#61002));
#15133=EDGE_LOOP('',(#61003,#61004,#61005,#61006));
#15134=EDGE_LOOP('',(#61007,#61008,#61009,#61010));
#15135=EDGE_LOOP('',(#61011,#61012,#61013,#61014));
#15136=EDGE_LOOP('',(#61015,#61016,#61017,#61018));
#15137=EDGE_LOOP('',(#61019,#61020,#61021,#61022));
#15138=EDGE_LOOP('',(#61023,#61024,#61025,#61026));
#15139=EDGE_LOOP('',(#61027,#61028,#61029,#61030));
#15140=EDGE_LOOP('',(#61031,#61032,#61033,#61034));
#15141=EDGE_LOOP('',(#61035,#61036,#61037,#61038));
#15142=EDGE_LOOP('',(#61039,#61040,#61041,#61042));
#15143=EDGE_LOOP('',(#61043,#61044,#61045,#61046));
#15144=EDGE_LOOP('',(#61047,#61048,#61049,#61050));
#15145=EDGE_LOOP('',(#61051,#61052,#61053,#61054));
#15146=EDGE_LOOP('',(#61055,#61056,#61057,#61058));
#15147=EDGE_LOOP('',(#61059,#61060,#61061,#61062,#61063));
#15148=EDGE_LOOP('',(#61064,#61065,#61066,#61067));
#15149=EDGE_LOOP('',(#61068,#61069,#61070,#61071));
#15150=EDGE_LOOP('',(#61072,#61073,#61074,#61075));
#15151=EDGE_LOOP('',(#61076,#61077,#61078,#61079));
#15152=EDGE_LOOP('',(#61080,#61081,#61082,#61083));
#15153=EDGE_LOOP('',(#61084,#61085,#61086,#61087));
#15154=EDGE_LOOP('',(#61088,#61089,#61090,#61091));
#15155=EDGE_LOOP('',(#61092,#61093,#61094,#61095));
#15156=EDGE_LOOP('',(#61096,#61097,#61098,#61099));
#15157=EDGE_LOOP('',(#61100,#61101,#61102,#61103));
#15158=EDGE_LOOP('',(#61104,#61105,#61106,#61107));
#15159=EDGE_LOOP('',(#61108,#61109,#61110,#61111));
#15160=EDGE_LOOP('',(#61112,#61113,#61114,#61115));
#15161=EDGE_LOOP('',(#61116,#61117,#61118,#61119));
#15162=EDGE_LOOP('',(#61120,#61121,#61122,#61123));
#15163=EDGE_LOOP('',(#61124,#61125,#61126,#61127));
#15164=EDGE_LOOP('',(#61128,#61129,#61130,#61131));
#15165=EDGE_LOOP('',(#61132,#61133,#61134,#61135));
#15166=EDGE_LOOP('',(#61136,#61137,#61138,#61139));
#15167=EDGE_LOOP('',(#61140,#61141,#61142,#61143));
#15168=EDGE_LOOP('',(#61144,#61145,#61146,#61147));
#15169=EDGE_LOOP('',(#61148,#61149,#61150,#61151));
#15170=EDGE_LOOP('',(#61152,#61153,#61154,#61155));
#15171=EDGE_LOOP('',(#61156,#61157,#61158,#61159));
#15172=EDGE_LOOP('',(#61160,#61161,#61162,#61163));
#15173=EDGE_LOOP('',(#61164,#61165,#61166,#61167));
#15174=EDGE_LOOP('',(#61168,#61169,#61170,#61171));
#15175=EDGE_LOOP('',(#61172,#61173,#61174,#61175));
#15176=EDGE_LOOP('',(#61176,#61177,#61178,#61179));
#15177=EDGE_LOOP('',(#61180,#61181,#61182,#61183));
#15178=EDGE_LOOP('',(#61184,#61185,#61186,#61187));
#15179=EDGE_LOOP('',(#61188,#61189,#61190,#61191));
#15180=EDGE_LOOP('',(#61192,#61193,#61194,#61195));
#15181=EDGE_LOOP('',(#61196,#61197,#61198,#61199));
#15182=EDGE_LOOP('',(#61200,#61201,#61202,#61203));
#15183=EDGE_LOOP('',(#61204,#61205,#61206,#61207));
#15184=EDGE_LOOP('',(#61208,#61209,#61210,#61211));
#15185=EDGE_LOOP('',(#61212,#61213,#61214,#61215));
#15186=EDGE_LOOP('',(#61216,#61217,#61218,#61219));
#15187=EDGE_LOOP('',(#61220,#61221,#61222,#61223));
#15188=EDGE_LOOP('',(#61224,#61225,#61226,#61227));
#15189=EDGE_LOOP('',(#61228,#61229,#61230,#61231));
#15190=EDGE_LOOP('',(#61232,#61233,#61234,#61235));
#15191=EDGE_LOOP('',(#61236,#61237,#61238,#61239));
#15192=EDGE_LOOP('',(#61240,#61241,#61242,#61243));
#15193=EDGE_LOOP('',(#61244,#61245,#61246,#61247));
#15194=EDGE_LOOP('',(#61248,#61249,#61250,#61251));
#15195=EDGE_LOOP('',(#61252,#61253,#61254,#61255));
#15196=EDGE_LOOP('',(#61256,#61257,#61258,#61259));
#15197=EDGE_LOOP('',(#61260,#61261,#61262,#61263));
#15198=EDGE_LOOP('',(#61264,#61265,#61266,#61267));
#15199=EDGE_LOOP('',(#61268,#61269,#61270,#61271));
#15200=EDGE_LOOP('',(#61272,#61273,#61274,#61275));
#15201=EDGE_LOOP('',(#61276,#61277,#61278,#61279));
#15202=EDGE_LOOP('',(#61280,#61281,#61282,#61283));
#15203=EDGE_LOOP('',(#61284,#61285,#61286,#61287));
#15204=EDGE_LOOP('',(#61288,#61289,#61290,#61291));
#15205=EDGE_LOOP('',(#61292,#61293,#61294,#61295));
#15206=EDGE_LOOP('',(#61296,#61297,#61298,#61299));
#15207=EDGE_LOOP('',(#61300,#61301,#61302,#61303));
#15208=EDGE_LOOP('',(#61304,#61305,#61306,#61307));
#15209=EDGE_LOOP('',(#61308,#61309,#61310,#61311));
#15210=EDGE_LOOP('',(#61312,#61313,#61314,#61315));
#15211=EDGE_LOOP('',(#61316,#61317,#61318,#61319));
#15212=EDGE_LOOP('',(#61320,#61321,#61322,#61323));
#15213=EDGE_LOOP('',(#61324,#61325,#61326,#61327));
#15214=EDGE_LOOP('',(#61328,#61329,#61330,#61331));
#15215=EDGE_LOOP('',(#61332,#61333,#61334,#61335));
#15216=EDGE_LOOP('',(#61336,#61337,#61338,#61339));
#15217=EDGE_LOOP('',(#61340,#61341,#61342,#61343));
#15218=EDGE_LOOP('',(#61344,#61345,#61346,#61347));
#15219=EDGE_LOOP('',(#61348,#61349,#61350,#61351));
#15220=EDGE_LOOP('',(#61352,#61353,#61354,#61355));
#15221=EDGE_LOOP('',(#61356,#61357,#61358,#61359));
#15222=EDGE_LOOP('',(#61360,#61361,#61362,#61363,#61364));
#15223=EDGE_LOOP('',(#61365,#61366,#61367,#61368));
#15224=EDGE_LOOP('',(#61369,#61370,#61371,#61372));
#15225=EDGE_LOOP('',(#61373,#61374,#61375,#61376));
#15226=EDGE_LOOP('',(#61377,#61378,#61379,#61380));
#15227=EDGE_LOOP('',(#61381,#61382,#61383,#61384));
#15228=EDGE_LOOP('',(#61385,#61386,#61387,#61388));
#15229=EDGE_LOOP('',(#61389,#61390,#61391,#61392));
#15230=EDGE_LOOP('',(#61393,#61394,#61395,#61396));
#15231=EDGE_LOOP('',(#61397,#61398,#61399,#61400));
#15232=EDGE_LOOP('',(#61401,#61402,#61403,#61404));
#15233=EDGE_LOOP('',(#61405,#61406,#61407,#61408));
#15234=EDGE_LOOP('',(#61409,#61410,#61411,#61412));
#15235=EDGE_LOOP('',(#61413,#61414,#61415,#61416));
#15236=EDGE_LOOP('',(#61417,#61418,#61419,#61420));
#15237=EDGE_LOOP('',(#61421,#61422,#61423,#61424));
#15238=EDGE_LOOP('',(#61425,#61426,#61427,#61428));
#15239=EDGE_LOOP('',(#61429,#61430,#61431,#61432));
#15240=EDGE_LOOP('',(#61433,#61434,#61435,#61436));
#15241=EDGE_LOOP('',(#61437,#61438,#61439,#61440));
#15242=EDGE_LOOP('',(#61441,#61442,#61443,#61444));
#15243=EDGE_LOOP('',(#61445,#61446,#61447,#61448));
#15244=EDGE_LOOP('',(#61449,#61450,#61451,#61452));
#15245=EDGE_LOOP('',(#61453,#61454,#61455,#61456));
#15246=EDGE_LOOP('',(#61457,#61458,#61459,#61460));
#15247=EDGE_LOOP('',(#61461,#61462,#61463,#61464));
#15248=EDGE_LOOP('',(#61465,#61466,#61467,#61468));
#15249=EDGE_LOOP('',(#61469,#61470,#61471,#61472));
#15250=EDGE_LOOP('',(#61473,#61474,#61475,#61476));
#15251=EDGE_LOOP('',(#61477,#61478,#61479,#61480));
#15252=EDGE_LOOP('',(#61481,#61482,#61483,#61484,#61485));
#15253=EDGE_LOOP('',(#61486,#61487,#61488,#61489,#61490));
#15254=EDGE_LOOP('',(#61491,#61492,#61493,#61494));
#15255=EDGE_LOOP('',(#61495,#61496,#61497,#61498));
#15256=EDGE_LOOP('',(#61499,#61500,#61501,#61502));
#15257=EDGE_LOOP('',(#61503,#61504,#61505,#61506));
#15258=EDGE_LOOP('',(#61507,#61508,#61509,#61510));
#15259=EDGE_LOOP('',(#61511,#61512,#61513,#61514));
#15260=EDGE_LOOP('',(#61515,#61516,#61517,#61518));
#15261=EDGE_LOOP('',(#61519,#61520,#61521,#61522));
#15262=EDGE_LOOP('',(#61523,#61524,#61525,#61526));
#15263=EDGE_LOOP('',(#61527,#61528,#61529,#61530));
#15264=EDGE_LOOP('',(#61531,#61532,#61533,#61534));
#15265=EDGE_LOOP('',(#61535,#61536,#61537,#61538));
#15266=EDGE_LOOP('',(#61539,#61540,#61541,#61542));
#15267=EDGE_LOOP('',(#61543,#61544,#61545,#61546));
#15268=EDGE_LOOP('',(#61547,#61548,#61549,#61550));
#15269=EDGE_LOOP('',(#61551,#61552,#61553,#61554));
#15270=EDGE_LOOP('',(#61555,#61556,#61557,#61558));
#15271=EDGE_LOOP('',(#61559,#61560,#61561,#61562));
#15272=EDGE_LOOP('',(#61563,#61564,#61565,#61566));
#15273=EDGE_LOOP('',(#61567,#61568,#61569,#61570));
#15274=EDGE_LOOP('',(#61571,#61572,#61573,#61574));
#15275=EDGE_LOOP('',(#61575,#61576,#61577,#61578));
#15276=EDGE_LOOP('',(#61579,#61580,#61581,#61582));
#15277=EDGE_LOOP('',(#61583,#61584,#61585,#61586));
#15278=EDGE_LOOP('',(#61587,#61588,#61589,#61590));
#15279=EDGE_LOOP('',(#61591,#61592,#61593,#61594));
#15280=EDGE_LOOP('',(#61595,#61596,#61597,#61598));
#15281=EDGE_LOOP('',(#61599,#61600,#61601,#61602));
#15282=EDGE_LOOP('',(#61603,#61604,#61605,#61606));
#15283=EDGE_LOOP('',(#61607,#61608,#61609,#61610));
#15284=EDGE_LOOP('',(#61611,#61612,#61613,#61614));
#15285=EDGE_LOOP('',(#61615,#61616,#61617,#61618));
#15286=EDGE_LOOP('',(#61619,#61620,#61621,#61622));
#15287=EDGE_LOOP('',(#61623,#61624,#61625,#61626));
#15288=EDGE_LOOP('',(#61627,#61628,#61629,#61630));
#15289=EDGE_LOOP('',(#61631,#61632,#61633,#61634));
#15290=EDGE_LOOP('',(#61635,#61636,#61637,#61638));
#15291=EDGE_LOOP('',(#61639,#61640,#61641,#61642));
#15292=EDGE_LOOP('',(#61643,#61644,#61645,#61646));
#15293=EDGE_LOOP('',(#61647,#61648,#61649,#61650));
#15294=EDGE_LOOP('',(#61651,#61652,#61653,#61654));
#15295=EDGE_LOOP('',(#61655,#61656,#61657,#61658));
#15296=EDGE_LOOP('',(#61659,#61660,#61661,#61662));
#15297=EDGE_LOOP('',(#61663,#61664,#61665,#61666));
#15298=EDGE_LOOP('',(#61667,#61668,#61669,#61670));
#15299=EDGE_LOOP('',(#61671,#61672,#61673,#61674));
#15300=EDGE_LOOP('',(#61675,#61676,#61677,#61678));
#15301=EDGE_LOOP('',(#61679,#61680,#61681,#61682));
#15302=EDGE_LOOP('',(#61683,#61684,#61685,#61686));
#15303=EDGE_LOOP('',(#61687,#61688,#61689,#61690));
#15304=EDGE_LOOP('',(#61691,#61692,#61693,#61694));
#15305=EDGE_LOOP('',(#61695,#61696,#61697,#61698));
#15306=EDGE_LOOP('',(#61699,#61700,#61701,#61702));
#15307=EDGE_LOOP('',(#61703,#61704,#61705,#61706));
#15308=EDGE_LOOP('',(#61707,#61708,#61709,#61710));
#15309=EDGE_LOOP('',(#61711,#61712,#61713,#61714));
#15310=EDGE_LOOP('',(#61715,#61716,#61717,#61718));
#15311=EDGE_LOOP('',(#61719,#61720,#61721,#61722));
#15312=EDGE_LOOP('',(#61723,#61724,#61725,#61726));
#15313=EDGE_LOOP('',(#61727,#61728,#61729,#61730));
#15314=EDGE_LOOP('',(#61731,#61732,#61733,#61734));
#15315=EDGE_LOOP('',(#61735,#61736,#61737,#61738));
#15316=EDGE_LOOP('',(#61739,#61740,#61741,#61742));
#15317=EDGE_LOOP('',(#61743,#61744,#61745,#61746));
#15318=EDGE_LOOP('',(#61747,#61748,#61749,#61750));
#15319=EDGE_LOOP('',(#61751,#61752,#61753,#61754));
#15320=EDGE_LOOP('',(#61755,#61756,#61757,#61758));
#15321=EDGE_LOOP('',(#61759,#61760,#61761,#61762));
#15322=EDGE_LOOP('',(#61763,#61764,#61765,#61766));
#15323=EDGE_LOOP('',(#61767,#61768,#61769,#61770));
#15324=EDGE_LOOP('',(#61771,#61772,#61773,#61774));
#15325=EDGE_LOOP('',(#61775,#61776,#61777,#61778));
#15326=EDGE_LOOP('',(#61779,#61780,#61781,#61782));
#15327=EDGE_LOOP('',(#61783,#61784,#61785,#61786));
#15328=EDGE_LOOP('',(#61787,#61788,#61789,#61790));
#15329=EDGE_LOOP('',(#61791,#61792,#61793,#61794));
#15330=EDGE_LOOP('',(#61795,#61796,#61797,#61798));
#15331=EDGE_LOOP('',(#61799,#61800,#61801,#61802));
#15332=EDGE_LOOP('',(#61803,#61804,#61805,#61806));
#15333=EDGE_LOOP('',(#61807,#61808,#61809,#61810));
#15334=EDGE_LOOP('',(#61811,#61812,#61813,#61814));
#15335=EDGE_LOOP('',(#61815,#61816,#61817,#61818));
#15336=EDGE_LOOP('',(#61819,#61820,#61821,#61822));
#15337=EDGE_LOOP('',(#61823,#61824,#61825,#61826));
#15338=EDGE_LOOP('',(#61827,#61828,#61829,#61830));
#15339=EDGE_LOOP('',(#61831,#61832,#61833,#61834));
#15340=EDGE_LOOP('',(#61835,#61836,#61837,#61838));
#15341=EDGE_LOOP('',(#61839,#61840,#61841,#61842));
#15342=EDGE_LOOP('',(#61843,#61844,#61845,#61846));
#15343=EDGE_LOOP('',(#61847,#61848,#61849,#61850,#61851));
#15344=EDGE_LOOP('',(#61852,#61853,#61854,#61855,#61856));
#15345=EDGE_LOOP('',(#61857,#61858,#61859,#61860));
#15346=EDGE_LOOP('',(#61861,#61862,#61863,#61864));
#15347=EDGE_LOOP('',(#61865,#61866,#61867,#61868));
#15348=EDGE_LOOP('',(#61869,#61870,#61871,#61872));
#15349=EDGE_LOOP('',(#61873,#61874,#61875,#61876));
#15350=EDGE_LOOP('',(#61877,#61878,#61879,#61880));
#15351=EDGE_LOOP('',(#61881,#61882,#61883,#61884));
#15352=EDGE_LOOP('',(#61885,#61886,#61887,#61888));
#15353=EDGE_LOOP('',(#61889,#61890,#61891,#61892));
#15354=EDGE_LOOP('',(#61893,#61894,#61895,#61896));
#15355=EDGE_LOOP('',(#61897,#61898,#61899,#61900));
#15356=EDGE_LOOP('',(#61901,#61902,#61903,#61904));
#15357=EDGE_LOOP('',(#61905,#61906,#61907,#61908));
#15358=EDGE_LOOP('',(#61909,#61910,#61911,#61912));
#15359=EDGE_LOOP('',(#61913,#61914,#61915,#61916));
#15360=EDGE_LOOP('',(#61917,#61918,#61919,#61920,#61921));
#15361=EDGE_LOOP('',(#61922,#61923,#61924,#61925));
#15362=EDGE_LOOP('',(#61926,#61927,#61928,#61929));
#15363=EDGE_LOOP('',(#61930,#61931,#61932,#61933));
#15364=EDGE_LOOP('',(#61934,#61935,#61936,#61937));
#15365=EDGE_LOOP('',(#61938,#61939,#61940,#61941));
#15366=EDGE_LOOP('',(#61942,#61943,#61944,#61945));
#15367=EDGE_LOOP('',(#61946,#61947,#61948,#61949));
#15368=EDGE_LOOP('',(#61950,#61951,#61952,#61953,#61954));
#15369=EDGE_LOOP('',(#61955,#61956,#61957,#61958));
#15370=EDGE_LOOP('',(#61959,#61960,#61961,#61962));
#15371=EDGE_LOOP('',(#61963,#61964,#61965,#61966));
#15372=EDGE_LOOP('',(#61967,#61968,#61969,#61970));
#15373=EDGE_LOOP('',(#61971,#61972,#61973,#61974));
#15374=EDGE_LOOP('',(#61975,#61976,#61977,#61978));
#15375=EDGE_LOOP('',(#61979,#61980,#61981,#61982));
#15376=EDGE_LOOP('',(#61983,#61984,#61985,#61986));
#15377=EDGE_LOOP('',(#61987,#61988,#61989,#61990));
#15378=EDGE_LOOP('',(#61991,#61992,#61993,#61994));
#15379=EDGE_LOOP('',(#61995,#61996,#61997,#61998));
#15380=EDGE_LOOP('',(#61999,#62000,#62001,#62002));
#15381=EDGE_LOOP('',(#62003,#62004,#62005,#62006));
#15382=EDGE_LOOP('',(#62007,#62008,#62009,#62010));
#15383=EDGE_LOOP('',(#62011,#62012,#62013,#62014));
#15384=EDGE_LOOP('',(#62015,#62016,#62017,#62018));
#15385=EDGE_LOOP('',(#62019,#62020,#62021,#62022));
#15386=EDGE_LOOP('',(#62023,#62024,#62025,#62026));
#15387=EDGE_LOOP('',(#62027,#62028,#62029,#62030));
#15388=EDGE_LOOP('',(#62031,#62032,#62033,#62034));
#15389=EDGE_LOOP('',(#62035,#62036,#62037,#62038));
#15390=EDGE_LOOP('',(#62039,#62040,#62041,#62042));
#15391=EDGE_LOOP('',(#62043,#62044,#62045,#62046));
#15392=EDGE_LOOP('',(#62047,#62048,#62049,#62050));
#15393=EDGE_LOOP('',(#62051,#62052,#62053,#62054));
#15394=EDGE_LOOP('',(#62055,#62056,#62057,#62058));
#15395=EDGE_LOOP('',(#62059,#62060,#62061,#62062));
#15396=EDGE_LOOP('',(#62063,#62064,#62065,#62066));
#15397=EDGE_LOOP('',(#62067,#62068,#62069,#62070));
#15398=EDGE_LOOP('',(#62071,#62072,#62073,#62074));
#15399=EDGE_LOOP('',(#62075,#62076,#62077,#62078));
#15400=EDGE_LOOP('',(#62079,#62080,#62081,#62082));
#15401=EDGE_LOOP('',(#62083,#62084,#62085,#62086));
#15402=EDGE_LOOP('',(#62087,#62088,#62089,#62090));
#15403=EDGE_LOOP('',(#62091,#62092,#62093,#62094));
#15404=EDGE_LOOP('',(#62095,#62096,#62097,#62098));
#15405=EDGE_LOOP('',(#62099,#62100,#62101,#62102));
#15406=EDGE_LOOP('',(#62103,#62104,#62105,#62106));
#15407=EDGE_LOOP('',(#62107,#62108,#62109,#62110));
#15408=EDGE_LOOP('',(#62111,#62112,#62113,#62114));
#15409=EDGE_LOOP('',(#62115,#62116,#62117,#62118));
#15410=EDGE_LOOP('',(#62119,#62120,#62121,#62122));
#15411=EDGE_LOOP('',(#62123,#62124,#62125,#62126));
#15412=EDGE_LOOP('',(#62127,#62128,#62129,#62130));
#15413=EDGE_LOOP('',(#62131,#62132,#62133,#62134));
#15414=EDGE_LOOP('',(#62135,#62136,#62137,#62138));
#15415=EDGE_LOOP('',(#62139,#62140,#62141,#62142));
#15416=EDGE_LOOP('',(#62143,#62144,#62145,#62146));
#15417=EDGE_LOOP('',(#62147,#62148,#62149,#62150,#62151));
#15418=EDGE_LOOP('',(#62152,#62153,#62154,#62155));
#15419=EDGE_LOOP('',(#62156,#62157,#62158,#62159));
#15420=EDGE_LOOP('',(#62160,#62161,#62162,#62163));
#15421=EDGE_LOOP('',(#62164,#62165,#62166,#62167));
#15422=EDGE_LOOP('',(#62168,#62169,#62170,#62171));
#15423=EDGE_LOOP('',(#62172,#62173,#62174,#62175));
#15424=EDGE_LOOP('',(#62176,#62177,#62178,#62179));
#15425=EDGE_LOOP('',(#62180,#62181,#62182,#62183));
#15426=EDGE_LOOP('',(#62184,#62185,#62186,#62187));
#15427=EDGE_LOOP('',(#62188,#62189,#62190,#62191));
#15428=EDGE_LOOP('',(#62192,#62193,#62194,#62195));
#15429=EDGE_LOOP('',(#62196,#62197,#62198,#62199));
#15430=EDGE_LOOP('',(#62200,#62201,#62202,#62203));
#15431=EDGE_LOOP('',(#62204,#62205,#62206,#62207));
#15432=EDGE_LOOP('',(#62208,#62209,#62210,#62211));
#15433=EDGE_LOOP('',(#62212,#62213,#62214,#62215));
#15434=EDGE_LOOP('',(#62216,#62217,#62218,#62219));
#15435=EDGE_LOOP('',(#62220,#62221,#62222,#62223));
#15436=EDGE_LOOP('',(#62224,#62225,#62226,#62227));
#15437=EDGE_LOOP('',(#62228,#62229,#62230,#62231));
#15438=EDGE_LOOP('',(#62232,#62233,#62234,#62235));
#15439=EDGE_LOOP('',(#62236,#62237,#62238,#62239,#62240));
#15440=EDGE_LOOP('',(#62241,#62242,#62243,#62244,#62245));
#15441=EDGE_LOOP('',(#62246,#62247,#62248,#62249));
#15442=EDGE_LOOP('',(#62250,#62251,#62252,#62253));
#15443=EDGE_LOOP('',(#62254,#62255,#62256,#62257));
#15444=EDGE_LOOP('',(#62258,#62259,#62260,#62261));
#15445=EDGE_LOOP('',(#62262,#62263,#62264,#62265));
#15446=EDGE_LOOP('',(#62266,#62267,#62268,#62269));
#15447=EDGE_LOOP('',(#62270,#62271,#62272,#62273));
#15448=EDGE_LOOP('',(#62274,#62275,#62276,#62277));
#15449=EDGE_LOOP('',(#62278,#62279,#62280,#62281));
#15450=EDGE_LOOP('',(#62282,#62283,#62284,#62285));
#15451=EDGE_LOOP('',(#62286,#62287,#62288,#62289));
#15452=EDGE_LOOP('',(#62290,#62291,#62292,#62293));
#15453=EDGE_LOOP('',(#62294,#62295,#62296,#62297));
#15454=EDGE_LOOP('',(#62298,#62299,#62300,#62301));
#15455=EDGE_LOOP('',(#62302,#62303,#62304,#62305));
#15456=EDGE_LOOP('',(#62306,#62307,#62308,#62309));
#15457=EDGE_LOOP('',(#62310,#62311,#62312,#62313));
#15458=EDGE_LOOP('',(#62314,#62315,#62316,#62317));
#15459=EDGE_LOOP('',(#62318,#62319,#62320,#62321));
#15460=EDGE_LOOP('',(#62322,#62323,#62324,#62325));
#15461=EDGE_LOOP('',(#62326,#62327,#62328,#62329));
#15462=EDGE_LOOP('',(#62330,#62331,#62332,#62333));
#15463=EDGE_LOOP('',(#62334,#62335,#62336,#62337));
#15464=EDGE_LOOP('',(#62338,#62339,#62340,#62341));
#15465=EDGE_LOOP('',(#62342,#62343,#62344,#62345));
#15466=EDGE_LOOP('',(#62346,#62347,#62348,#62349));
#15467=EDGE_LOOP('',(#62350,#62351,#62352,#62353));
#15468=EDGE_LOOP('',(#62354,#62355,#62356,#62357));
#15469=EDGE_LOOP('',(#62358,#62359,#62360,#62361));
#15470=EDGE_LOOP('',(#62362,#62363,#62364,#62365));
#15471=EDGE_LOOP('',(#62366,#62367,#62368,#62369));
#15472=EDGE_LOOP('',(#62370,#62371,#62372,#62373,#62374));
#15473=EDGE_LOOP('',(#62375,#62376,#62377,#62378,#62379));
#15474=EDGE_LOOP('',(#62380,#62381,#62382,#62383));
#15475=EDGE_LOOP('',(#62384,#62385,#62386,#62387));
#15476=EDGE_LOOP('',(#62388,#62389,#62390,#62391));
#15477=EDGE_LOOP('',(#62392,#62393,#62394,#62395));
#15478=EDGE_LOOP('',(#62396,#62397,#62398,#62399));
#15479=EDGE_LOOP('',(#62400,#62401,#62402,#62403));
#15480=EDGE_LOOP('',(#62404,#62405,#62406,#62407));
#15481=EDGE_LOOP('',(#62408,#62409,#62410,#62411));
#15482=EDGE_LOOP('',(#62412,#62413,#62414,#62415));
#15483=EDGE_LOOP('',(#62416,#62417,#62418,#62419));
#15484=EDGE_LOOP('',(#62420,#62421,#62422,#62423));
#15485=EDGE_LOOP('',(#62424,#62425,#62426,#62427));
#15486=EDGE_LOOP('',(#62428,#62429,#62430,#62431));
#15487=EDGE_LOOP('',(#62432,#62433,#62434,#62435));
#15488=EDGE_LOOP('',(#62436,#62437,#62438));
#15489=EDGE_LOOP('',(#62439,#62440,#62441,#62442));
#15490=EDGE_LOOP('',(#62443,#62444,#62445,#62446));
#15491=EDGE_LOOP('',(#62447,#62448,#62449,#62450));
#15492=EDGE_LOOP('',(#62451,#62452,#62453,#62454));
#15493=EDGE_LOOP('',(#62455,#62456,#62457,#62458));
#15494=EDGE_LOOP('',(#62459,#62460,#62461,#62462));
#15495=EDGE_LOOP('',(#62463,#62464,#62465,#62466));
#15496=EDGE_LOOP('',(#62467,#62468,#62469,#62470));
#15497=EDGE_LOOP('',(#62471,#62472,#62473,#62474));
#15498=EDGE_LOOP('',(#62475,#62476,#62477,#62478));
#15499=EDGE_LOOP('',(#62479,#62480,#62481,#62482));
#15500=EDGE_LOOP('',(#62483,#62484,#62485,#62486));
#15501=EDGE_LOOP('',(#62487,#62488,#62489,#62490));
#15502=EDGE_LOOP('',(#62491,#62492,#62493,#62494));
#15503=EDGE_LOOP('',(#62495,#62496,#62497,#62498));
#15504=EDGE_LOOP('',(#62499,#62500,#62501,#62502));
#15505=EDGE_LOOP('',(#62503,#62504,#62505,#62506));
#15506=EDGE_LOOP('',(#62507,#62508,#62509,#62510));
#15507=EDGE_LOOP('',(#62511,#62512,#62513,#62514));
#15508=EDGE_LOOP('',(#62515,#62516,#62517,#62518));
#15509=EDGE_LOOP('',(#62519,#62520,#62521,#62522));
#15510=EDGE_LOOP('',(#62523,#62524,#62525,#62526));
#15511=EDGE_LOOP('',(#62527,#62528,#62529,#62530));
#15512=EDGE_LOOP('',(#62531,#62532,#62533,#62534));
#15513=EDGE_LOOP('',(#62535,#62536,#62537,#62538));
#15514=EDGE_LOOP('',(#62539,#62540,#62541,#62542));
#15515=EDGE_LOOP('',(#62543,#62544,#62545,#62546));
#15516=EDGE_LOOP('',(#62547,#62548,#62549,#62550));
#15517=EDGE_LOOP('',(#62551,#62552,#62553,#62554));
#15518=EDGE_LOOP('',(#62555,#62556,#62557,#62558));
#15519=EDGE_LOOP('',(#62559,#62560,#62561,#62562));
#15520=EDGE_LOOP('',(#62563,#62564,#62565,#62566));
#15521=EDGE_LOOP('',(#62567,#62568,#62569,#62570));
#15522=EDGE_LOOP('',(#62571,#62572,#62573,#62574));
#15523=EDGE_LOOP('',(#62575,#62576,#62577,#62578));
#15524=EDGE_LOOP('',(#62579,#62580,#62581,#62582));
#15525=EDGE_LOOP('',(#62583,#62584,#62585,#62586));
#15526=EDGE_LOOP('',(#62587,#62588,#62589,#62590));
#15527=EDGE_LOOP('',(#62591,#62592,#62593,#62594));
#15528=EDGE_LOOP('',(#62595,#62596,#62597,#62598));
#15529=EDGE_LOOP('',(#62599,#62600,#62601,#62602));
#15530=EDGE_LOOP('',(#62603,#62604,#62605,#62606));
#15531=EDGE_LOOP('',(#62607,#62608,#62609,#62610));
#15532=EDGE_LOOP('',(#62611,#62612,#62613,#62614));
#15533=EDGE_LOOP('',(#62615,#62616,#62617,#62618));
#15534=EDGE_LOOP('',(#62619,#62620,#62621,#62622));
#15535=EDGE_LOOP('',(#62623,#62624,#62625,#62626));
#15536=EDGE_LOOP('',(#62627,#62628,#62629,#62630));
#15537=EDGE_LOOP('',(#62631,#62632,#62633,#62634));
#15538=EDGE_LOOP('',(#62635,#62636,#62637,#62638));
#15539=EDGE_LOOP('',(#62639,#62640,#62641,#62642));
#15540=EDGE_LOOP('',(#62643,#62644,#62645,#62646));
#15541=EDGE_LOOP('',(#62647,#62648,#62649,#62650));
#15542=EDGE_LOOP('',(#62651,#62652,#62653,#62654));
#15543=EDGE_LOOP('',(#62655,#62656,#62657,#62658));
#15544=EDGE_LOOP('',(#62659,#62660,#62661,#62662));
#15545=EDGE_LOOP('',(#62663,#62664,#62665,#62666));
#15546=EDGE_LOOP('',(#62667,#62668,#62669,#62670));
#15547=EDGE_LOOP('',(#62671,#62672,#62673,#62674));
#15548=EDGE_LOOP('',(#62675,#62676,#62677,#62678));
#15549=EDGE_LOOP('',(#62679,#62680,#62681,#62682));
#15550=EDGE_LOOP('',(#62683,#62684,#62685,#62686));
#15551=EDGE_LOOP('',(#62687,#62688,#62689,#62690));
#15552=EDGE_LOOP('',(#62691,#62692,#62693,#62694));
#15553=EDGE_LOOP('',(#62695,#62696,#62697,#62698));
#15554=EDGE_LOOP('',(#62699,#62700,#62701,#62702));
#15555=EDGE_LOOP('',(#62703,#62704,#62705,#62706));
#15556=EDGE_LOOP('',(#62707,#62708,#62709,#62710));
#15557=EDGE_LOOP('',(#62711,#62712,#62713,#62714));
#15558=EDGE_LOOP('',(#62715,#62716,#62717,#62718));
#15559=EDGE_LOOP('',(#62719,#62720,#62721,#62722));
#15560=EDGE_LOOP('',(#62723,#62724,#62725,#62726));
#15561=EDGE_LOOP('',(#62727,#62728,#62729,#62730));
#15562=EDGE_LOOP('',(#62731,#62732,#62733,#62734));
#15563=EDGE_LOOP('',(#62735,#62736,#62737,#62738));
#15564=EDGE_LOOP('',(#62739,#62740,#62741,#62742,#62743,#62744));
#15565=EDGE_LOOP('',(#62745,#62746,#62747,#62748));
#15566=EDGE_LOOP('',(#62749,#62750,#62751,#62752));
#15567=EDGE_LOOP('',(#62753,#62754,#62755,#62756));
#15568=EDGE_LOOP('',(#62757,#62758,#62759,#62760));
#15569=EDGE_LOOP('',(#62761,#62762,#62763,#62764));
#15570=EDGE_LOOP('',(#62765,#62766,#62767,#62768));
#15571=EDGE_LOOP('',(#62769,#62770,#62771,#62772));
#15572=EDGE_LOOP('',(#62773,#62774,#62775,#62776));
#15573=EDGE_LOOP('',(#62777,#62778,#62779,#62780));
#15574=EDGE_LOOP('',(#62781,#62782,#62783,#62784));
#15575=EDGE_LOOP('',(#62785,#62786,#62787,#62788));
#15576=EDGE_LOOP('',(#62789,#62790,#62791,#62792));
#15577=EDGE_LOOP('',(#62793,#62794,#62795,#62796));
#15578=EDGE_LOOP('',(#62797,#62798,#62799,#62800));
#15579=EDGE_LOOP('',(#62801,#62802,#62803,#62804));
#15580=EDGE_LOOP('',(#62805,#62806,#62807));
#15581=EDGE_LOOP('',(#62808,#62809,#62810,#62811));
#15582=EDGE_LOOP('',(#62812,#62813,#62814,#62815));
#15583=EDGE_LOOP('',(#62816,#62817,#62818,#62819));
#15584=EDGE_LOOP('',(#62820,#62821,#62822,#62823));
#15585=EDGE_LOOP('',(#62824,#62825,#62826,#62827));
#15586=EDGE_LOOP('',(#62828,#62829,#62830,#62831));
#15587=EDGE_LOOP('',(#62832,#62833,#62834,#62835));
#15588=EDGE_LOOP('',(#62836,#62837,#62838,#62839));
#15589=EDGE_LOOP('',(#62840,#62841,#62842,#62843));
#15590=EDGE_LOOP('',(#62844,#62845,#62846,#62847));
#15591=EDGE_LOOP('',(#62848,#62849,#62850,#62851));
#15592=EDGE_LOOP('',(#62852,#62853,#62854,#62855));
#15593=EDGE_LOOP('',(#62856,#62857,#62858,#62859));
#15594=EDGE_LOOP('',(#62860,#62861,#62862,#62863));
#15595=EDGE_LOOP('',(#62864,#62865,#62866,#62867));
#15596=EDGE_LOOP('',(#62868,#62869,#62870));
#15597=EDGE_LOOP('',(#62871,#62872,#62873,#62874));
#15598=EDGE_LOOP('',(#62875,#62876,#62877,#62878));
#15599=EDGE_LOOP('',(#62879,#62880,#62881,#62882));
#15600=EDGE_LOOP('',(#62883,#62884,#62885,#62886));
#15601=EDGE_LOOP('',(#62887,#62888,#62889,#62890));
#15602=EDGE_LOOP('',(#62891,#62892,#62893,#62894));
#15603=EDGE_LOOP('',(#62895,#62896,#62897,#62898));
#15604=EDGE_LOOP('',(#62899,#62900,#62901,#62902));
#15605=EDGE_LOOP('',(#62903,#62904,#62905,#62906,#62907));
#15606=EDGE_LOOP('',(#62908,#62909,#62910));
#15607=EDGE_LOOP('',(#62911,#62912,#62913,#62914));
#15608=EDGE_LOOP('',(#62915,#62916,#62917,#62918));
#15609=EDGE_LOOP('',(#62919,#62920,#62921,#62922));
#15610=EDGE_LOOP('',(#62923,#62924,#62925,#62926));
#15611=EDGE_LOOP('',(#62927,#62928,#62929,#62930,#62931));
#15612=EDGE_LOOP('',(#62932,#62933,#62934));
#15613=EDGE_LOOP('',(#62935,#62936,#62937,#62938,#62939));
#15614=EDGE_LOOP('',(#62940,#62941,#62942,#62943));
#15615=EDGE_LOOP('',(#62944,#62945,#62946,#62947));
#15616=EDGE_LOOP('',(#62948,#62949,#62950,#62951));
#15617=EDGE_LOOP('',(#62952,#62953,#62954,#62955));
#15618=EDGE_LOOP('',(#62956,#62957,#62958,#62959));
#15619=EDGE_LOOP('',(#62960,#62961,#62962,#62963));
#15620=EDGE_LOOP('',(#62964,#62965,#62966));
#15621=EDGE_LOOP('',(#62967,#62968,#62969,#62970));
#15622=EDGE_LOOP('',(#62971,#62972,#62973,#62974));
#15623=EDGE_LOOP('',(#62975,#62976,#62977,#62978));
#15624=EDGE_LOOP('',(#62979,#62980,#62981));
#15625=EDGE_LOOP('',(#62982,#62983,#62984,#62985));
#15626=EDGE_LOOP('',(#62986,#62987,#62988,#62989));
#15627=EDGE_LOOP('',(#62990,#62991,#62992,#62993));
#15628=EDGE_LOOP('',(#62994,#62995,#62996,#62997));
#15629=EDGE_LOOP('',(#62998,#62999,#63000,#63001));
#15630=EDGE_LOOP('',(#63002,#63003,#63004,#63005));
#15631=EDGE_LOOP('',(#63006,#63007,#63008,#63009));
#15632=EDGE_LOOP('',(#63010,#63011,#63012,#63013));
#15633=EDGE_LOOP('',(#63014,#63015,#63016,#63017));
#15634=EDGE_LOOP('',(#63018,#63019,#63020,#63021));
#15635=EDGE_LOOP('',(#63022,#63023,#63024,#63025));
#15636=EDGE_LOOP('',(#63026,#63027,#63028,#63029,#63030,#63031));
#15637=EDGE_LOOP('',(#63032,#63033,#63034,#63035));
#15638=EDGE_LOOP('',(#63036,#63037,#63038,#63039));
#15639=EDGE_LOOP('',(#63040,#63041,#63042,#63043));
#15640=EDGE_LOOP('',(#63044,#63045,#63046,#63047));
#15641=EDGE_LOOP('',(#63048,#63049,#63050));
#15642=EDGE_LOOP('',(#63051,#63052,#63053,#63054));
#15643=EDGE_LOOP('',(#63055,#63056,#63057,#63058));
#15644=EDGE_LOOP('',(#63059,#63060,#63061,#63062));
#15645=EDGE_LOOP('',(#63063,#63064,#63065,#63066));
#15646=EDGE_LOOP('',(#63067,#63068,#63069,#63070));
#15647=EDGE_LOOP('',(#63071,#63072,#63073,#63074));
#15648=EDGE_LOOP('',(#63075,#63076,#63077,#63078));
#15649=EDGE_LOOP('',(#63079,#63080,#63081,#63082,#63083,#63084));
#15650=EDGE_LOOP('',(#63085,#63086,#63087,#63088));
#15651=EDGE_LOOP('',(#63089,#63090,#63091,#63092));
#15652=EDGE_LOOP('',(#63093,#63094,#63095,#63096));
#15653=EDGE_LOOP('',(#63097,#63098,#63099,#63100));
#15654=EDGE_LOOP('',(#63101,#63102,#63103,#63104));
#15655=EDGE_LOOP('',(#63105,#63106,#63107,#63108));
#15656=EDGE_LOOP('',(#63109,#63110,#63111,#63112));
#15657=EDGE_LOOP('',(#63113,#63114,#63115,#63116));
#15658=EDGE_LOOP('',(#63117,#63118,#63119,#63120));
#15659=EDGE_LOOP('',(#63121,#63122,#63123,#63124));
#15660=EDGE_LOOP('',(#63125,#63126,#63127,#63128));
#15661=EDGE_LOOP('',(#63129,#63130,#63131,#63132));
#15662=EDGE_LOOP('',(#63133,#63134,#63135,#63136));
#15663=EDGE_LOOP('',(#63137,#63138,#63139));
#15664=EDGE_LOOP('',(#63140,#63141,#63142));
#15665=EDGE_LOOP('',(#63143,#63144,#63145,#63146));
#15666=EDGE_LOOP('',(#63147,#63148,#63149,#63150));
#15667=EDGE_LOOP('',(#63151,#63152,#63153,#63154));
#15668=EDGE_LOOP('',(#63155,#63156,#63157,#63158));
#15669=EDGE_LOOP('',(#63159,#63160,#63161,#63162));
#15670=EDGE_LOOP('',(#63163,#63164,#63165,#63166));
#15671=EDGE_LOOP('',(#63167,#63168,#63169,#63170));
#15672=EDGE_LOOP('',(#63171,#63172,#63173,#63174));
#15673=EDGE_LOOP('',(#63175,#63176,#63177,#63178));
#15674=EDGE_LOOP('',(#63179,#63180,#63181,#63182));
#15675=EDGE_LOOP('',(#63183,#63184,#63185,#63186));
#15676=EDGE_LOOP('',(#63187,#63188,#63189,#63190));
#15677=EDGE_LOOP('',(#63191,#63192,#63193,#63194));
#15678=EDGE_LOOP('',(#63195,#63196,#63197,#63198,#63199,#63200));
#15679=EDGE_LOOP('',(#63201,#63202,#63203,#63204));
#15680=EDGE_LOOP('',(#63205,#63206,#63207,#63208));
#15681=EDGE_LOOP('',(#63209,#63210,#63211,#63212));
#15682=EDGE_LOOP('',(#63213,#63214,#63215,#63216));
#15683=EDGE_LOOP('',(#63217,#63218,#63219,#63220));
#15684=EDGE_LOOP('',(#63221,#63222,#63223,#63224));
#15685=EDGE_LOOP('',(#63225,#63226,#63227,#63228));
#15686=EDGE_LOOP('',(#63229,#63230,#63231));
#15687=EDGE_LOOP('',(#63232,#63233,#63234,#63235));
#15688=EDGE_LOOP('',(#63236,#63237,#63238,#63239));
#15689=EDGE_LOOP('',(#63240,#63241,#63242,#63243));
#15690=EDGE_LOOP('',(#63244,#63245,#63246,#63247));
#15691=EDGE_LOOP('',(#63248,#63249,#63250,#63251,#63252,#63253));
#15692=EDGE_LOOP('',(#63254,#63255,#63256,#63257));
#15693=EDGE_LOOP('',(#63258,#63259,#63260,#63261));
#15694=EDGE_LOOP('',(#63262,#63263,#63264,#63265));
#15695=EDGE_LOOP('',(#63266,#63267,#63268,#63269));
#15696=EDGE_LOOP('',(#63270,#63271,#63272,#63273));
#15697=EDGE_LOOP('',(#63274,#63275,#63276,#63277));
#15698=EDGE_LOOP('',(#63278,#63279,#63280,#63281));
#15699=EDGE_LOOP('',(#63282,#63283,#63284,#63285));
#15700=EDGE_LOOP('',(#63286,#63287,#63288,#63289));
#15701=EDGE_LOOP('',(#63290,#63291,#63292,#63293));
#15702=EDGE_LOOP('',(#63294,#63295,#63296,#63297));
#15703=EDGE_LOOP('',(#63298,#63299,#63300));
#15704=EDGE_LOOP('',(#63301,#63302,#63303,#63304));
#15705=EDGE_LOOP('',(#63305,#63306,#63307,#63308));
#15706=EDGE_LOOP('',(#63309,#63310,#63311,#63312));
#15707=EDGE_LOOP('',(#63313,#63314,#63315));
#15708=EDGE_LOOP('',(#63316,#63317,#63318,#63319));
#15709=EDGE_LOOP('',(#63320,#63321,#63322,#63323));
#15710=EDGE_LOOP('',(#63324,#63325,#63326,#63327));
#15711=EDGE_LOOP('',(#63328,#63329,#63330,#63331));
#15712=EDGE_LOOP('',(#63332,#63333,#63334,#63335));
#15713=EDGE_LOOP('',(#63336,#63337,#63338,#63339));
#15714=EDGE_LOOP('',(#63340,#63341,#63342,#63343,#63344));
#15715=EDGE_LOOP('',(#63345,#63346,#63347));
#15716=EDGE_LOOP('',(#63348,#63349,#63350,#63351,#63352));
#15717=EDGE_LOOP('',(#63353,#63354,#63355,#63356));
#15718=EDGE_LOOP('',(#63357,#63358,#63359,#63360));
#15719=EDGE_LOOP('',(#63361,#63362,#63363,#63364));
#15720=EDGE_LOOP('',(#63365,#63366,#63367,#63368));
#15721=EDGE_LOOP('',(#63369,#63370,#63371));
#15722=EDGE_LOOP('',(#63372,#63373,#63374,#63375,#63376));
#15723=EDGE_LOOP('',(#63377,#63378,#63379,#63380));
#15724=EDGE_LOOP('',(#63381,#63382,#63383,#63384));
#15725=EDGE_LOOP('',(#63385,#63386,#63387,#63388));
#15726=EDGE_LOOP('',(#63389,#63390,#63391,#63392));
#15727=EDGE_LOOP('',(#63393,#63394,#63395,#63396));
#15728=EDGE_LOOP('',(#63397,#63398,#63399,#63400));
#15729=EDGE_LOOP('',(#63401,#63402,#63403,#63404));
#15730=EDGE_LOOP('',(#63405,#63406,#63407,#63408));
#15731=EDGE_LOOP('',(#63409,#63410,#63411));
#15732=EDGE_LOOP('',(#63412,#63413,#63414,#63415));
#15733=EDGE_LOOP('',(#63416,#63417,#63418,#63419));
#15734=EDGE_LOOP('',(#63420,#63421,#63422,#63423));
#15735=EDGE_LOOP('',(#63424,#63425,#63426,#63427));
#15736=EDGE_LOOP('',(#63428,#63429,#63430,#63431));
#15737=EDGE_LOOP('',(#63432,#63433,#63434,#63435));
#15738=EDGE_LOOP('',(#63436,#63437,#63438,#63439));
#15739=EDGE_LOOP('',(#63440,#63441,#63442,#63443));
#15740=EDGE_LOOP('',(#63444,#63445,#63446,#63447));
#15741=EDGE_LOOP('',(#63448,#63449,#63450,#63451));
#15742=EDGE_LOOP('',(#63452,#63453,#63454,#63455));
#15743=EDGE_LOOP('',(#63456,#63457,#63458,#63459));
#15744=EDGE_LOOP('',(#63460,#63461,#63462,#63463));
#15745=EDGE_LOOP('',(#63464,#63465,#63466,#63467));
#15746=EDGE_LOOP('',(#63468,#63469,#63470,#63471));
#15747=EDGE_LOOP('',(#63472,#63473,#63474));
#15748=EDGE_LOOP('',(#63475,#63476,#63477,#63478));
#15749=EDGE_LOOP('',(#63479,#63480,#63481,#63482));
#15750=EDGE_LOOP('',(#63483,#63484,#63485,#63486));
#15751=EDGE_LOOP('',(#63487,#63488,#63489,#63490));
#15752=EDGE_LOOP('',(#63491,#63492,#63493,#63494));
#15753=EDGE_LOOP('',(#63495,#63496,#63497,#63498));
#15754=EDGE_LOOP('',(#63499,#63500,#63501,#63502));
#15755=EDGE_LOOP('',(#63503,#63504,#63505,#63506));
#15756=EDGE_LOOP('',(#63507,#63508,#63509,#63510));
#15757=EDGE_LOOP('',(#63511,#63512,#63513,#63514));
#15758=EDGE_LOOP('',(#63515,#63516,#63517,#63518));
#15759=EDGE_LOOP('',(#63519,#63520,#63521,#63522));
#15760=EDGE_LOOP('',(#63523,#63524,#63525,#63526));
#15761=EDGE_LOOP('',(#63527,#63528,#63529,#63530));
#15762=EDGE_LOOP('',(#63531,#63532,#63533,#63534));
#15763=EDGE_LOOP('',(#63535,#63536,#63537,#63538,#63539,#63540));
#15764=EDGE_LOOP('',(#63541,#63542,#63543,#63544));
#15765=EDGE_LOOP('',(#63545,#63546,#63547,#63548));
#15766=EDGE_LOOP('',(#63549,#63550,#63551,#63552));
#15767=EDGE_LOOP('',(#63553,#63554,#63555,#63556));
#15768=EDGE_LOOP('',(#63557,#63558,#63559,#63560));
#15769=EDGE_LOOP('',(#63561,#63562,#63563,#63564));
#15770=EDGE_LOOP('',(#63565,#63566,#63567,#63568));
#15771=EDGE_LOOP('',(#63569,#63570,#63571,#63572));
#15772=EDGE_LOOP('',(#63573,#63574,#63575,#63576));
#15773=EDGE_LOOP('',(#63577,#63578,#63579,#63580));
#15774=EDGE_LOOP('',(#63581,#63582,#63583,#63584));
#15775=EDGE_LOOP('',(#63585,#63586,#63587,#63588));
#15776=EDGE_LOOP('',(#63589,#63590,#63591,#63592));
#15777=EDGE_LOOP('',(#63593,#63594,#63595,#63596));
#15778=EDGE_LOOP('',(#63597,#63598,#63599,#63600));
#15779=EDGE_LOOP('',(#63601,#63602,#63603,#63604));
#15780=EDGE_LOOP('',(#63605,#63606,#63607,#63608));
#15781=EDGE_LOOP('',(#63609,#63610,#63611,#63612));
#15782=EDGE_LOOP('',(#63613,#63614,#63615,#63616));
#15783=EDGE_LOOP('',(#63617,#63618,#63619,#63620));
#15784=EDGE_LOOP('',(#63621,#63622,#63623,#63624));
#15785=EDGE_LOOP('',(#63625,#63626,#63627,#63628));
#15786=EDGE_LOOP('',(#63629,#63630,#63631,#63632));
#15787=EDGE_LOOP('',(#63633,#63634,#63635,#63636));
#15788=EDGE_LOOP('',(#63637,#63638,#63639,#63640));
#15789=EDGE_LOOP('',(#63641,#63642,#63643,#63644));
#15790=EDGE_LOOP('',(#63645,#63646,#63647,#63648));
#15791=EDGE_LOOP('',(#63649,#63650,#63651,#63652));
#15792=EDGE_LOOP('',(#63653,#63654,#63655,#63656));
#15793=EDGE_LOOP('',(#63657,#63658,#63659,#63660));
#15794=EDGE_LOOP('',(#63661,#63662,#63663,#63664));
#15795=EDGE_LOOP('',(#63665,#63666,#63667,#63668));
#15796=EDGE_LOOP('',(#63669,#63670,#63671,#63672));
#15797=EDGE_LOOP('',(#63673,#63674,#63675,#63676));
#15798=EDGE_LOOP('',(#63677,#63678,#63679,#63680));
#15799=EDGE_LOOP('',(#63681,#63682,#63683,#63684));
#15800=EDGE_LOOP('',(#63685,#63686,#63687,#63688));
#15801=EDGE_LOOP('',(#63689,#63690,#63691,#63692));
#15802=EDGE_LOOP('',(#63693,#63694,#63695,#63696));
#15803=EDGE_LOOP('',(#63697,#63698,#63699,#63700));
#15804=EDGE_LOOP('',(#63701,#63702,#63703,#63704));
#15805=EDGE_LOOP('',(#63705,#63706,#63707,#63708));
#15806=EDGE_LOOP('',(#63709,#63710,#63711,#63712));
#15807=EDGE_LOOP('',(#63713,#63714,#63715,#63716));
#15808=EDGE_LOOP('',(#63717,#63718,#63719,#63720));
#15809=EDGE_LOOP('',(#63721,#63722,#63723,#63724));
#15810=EDGE_LOOP('',(#63725,#63726,#63727,#63728));
#15811=EDGE_LOOP('',(#63729,#63730,#63731,#63732));
#15812=EDGE_LOOP('',(#63733,#63734,#63735,#63736));
#15813=EDGE_LOOP('',(#63737,#63738,#63739,#63740));
#15814=EDGE_LOOP('',(#63741,#63742,#63743,#63744));
#15815=EDGE_LOOP('',(#63745,#63746,#63747,#63748));
#15816=EDGE_LOOP('',(#63749,#63750,#63751,#63752));
#15817=EDGE_LOOP('',(#63753,#63754,#63755,#63756));
#15818=EDGE_LOOP('',(#63757,#63758,#63759,#63760));
#15819=EDGE_LOOP('',(#63761,#63762,#63763,#63764));
#15820=EDGE_LOOP('',(#63765,#63766,#63767,#63768));
#15821=EDGE_LOOP('',(#63769,#63770,#63771,#63772));
#15822=EDGE_LOOP('',(#63773,#63774,#63775,#63776));
#15823=EDGE_LOOP('',(#63777,#63778,#63779,#63780));
#15824=EDGE_LOOP('',(#63781,#63782,#63783,#63784));
#15825=EDGE_LOOP('',(#63785,#63786,#63787,#63788));
#15826=EDGE_LOOP('',(#63789,#63790,#63791,#63792));
#15827=EDGE_LOOP('',(#63793,#63794,#63795,#63796));
#15828=EDGE_LOOP('',(#63797,#63798,#63799,#63800));
#15829=EDGE_LOOP('',(#63801,#63802,#63803,#63804));
#15830=EDGE_LOOP('',(#63805,#63806,#63807,#63808));
#15831=EDGE_LOOP('',(#63809,#63810,#63811,#63812));
#15832=EDGE_LOOP('',(#63813,#63814,#63815,#63816));
#15833=EDGE_LOOP('',(#63817,#63818,#63819,#63820));
#15834=EDGE_LOOP('',(#63821,#63822,#63823,#63824));
#15835=EDGE_LOOP('',(#63825,#63826,#63827,#63828));
#15836=EDGE_LOOP('',(#63829,#63830,#63831,#63832));
#15837=EDGE_LOOP('',(#63833,#63834,#63835,#63836));
#15838=EDGE_LOOP('',(#63837,#63838,#63839,#63840));
#15839=EDGE_LOOP('',(#63841,#63842,#63843));
#15840=EDGE_LOOP('',(#63844,#63845,#63846,#63847));
#15841=EDGE_LOOP('',(#63848,#63849,#63850,#63851));
#15842=EDGE_LOOP('',(#63852,#63853,#63854,#63855));
#15843=EDGE_LOOP('',(#63856,#63857,#63858,#63859));
#15844=EDGE_LOOP('',(#63860,#63861,#63862,#63863));
#15845=EDGE_LOOP('',(#63864,#63865,#63866,#63867));
#15846=EDGE_LOOP('',(#63868,#63869,#63870,#63871));
#15847=EDGE_LOOP('',(#63872,#63873,#63874,#63875));
#15848=EDGE_LOOP('',(#63876,#63877,#63878,#63879));
#15849=EDGE_LOOP('',(#63880,#63881,#63882,#63883));
#15850=EDGE_LOOP('',(#63884,#63885,#63886,#63887));
#15851=EDGE_LOOP('',(#63888,#63889,#63890,#63891));
#15852=EDGE_LOOP('',(#63892,#63893,#63894,#63895));
#15853=EDGE_LOOP('',(#63896,#63897,#63898,#63899));
#15854=EDGE_LOOP('',(#63900,#63901,#63902,#63903,#63904));
#15855=EDGE_LOOP('',(#63905,#63906,#63907,#63908,#63909));
#15856=EDGE_LOOP('',(#63910,#63911,#63912,#63913));
#15857=EDGE_LOOP('',(#63914,#63915,#63916,#63917));
#15858=EDGE_LOOP('',(#63918,#63919,#63920,#63921));
#15859=EDGE_LOOP('',(#63922,#63923,#63924,#63925));
#15860=EDGE_LOOP('',(#63926,#63927,#63928,#63929));
#15861=EDGE_LOOP('',(#63930,#63931,#63932,#63933));
#15862=EDGE_LOOP('',(#63934,#63935,#63936,#63937));
#15863=EDGE_LOOP('',(#63938,#63939,#63940,#63941));
#15864=EDGE_LOOP('',(#63942,#63943,#63944,#63945));
#15865=EDGE_LOOP('',(#63946,#63947,#63948,#63949));
#15866=EDGE_LOOP('',(#63950,#63951,#63952,#63953));
#15867=EDGE_LOOP('',(#63954,#63955,#63956,#63957));
#15868=EDGE_LOOP('',(#63958,#63959,#63960,#63961));
#15869=EDGE_LOOP('',(#63962,#63963,#63964,#63965));
#15870=EDGE_LOOP('',(#63966,#63967,#63968,#63969));
#15871=EDGE_LOOP('',(#63970,#63971,#63972,#63973));
#15872=EDGE_LOOP('',(#63974,#63975,#63976,#63977));
#15873=EDGE_LOOP('',(#63978,#63979,#63980,#63981));
#15874=EDGE_LOOP('',(#63982,#63983,#63984,#63985));
#15875=EDGE_LOOP('',(#63986,#63987,#63988,#63989));
#15876=EDGE_LOOP('',(#63990,#63991,#63992,#63993));
#15877=EDGE_LOOP('',(#63994,#63995,#63996,#63997));
#15878=EDGE_LOOP('',(#63998,#63999,#64000,#64001));
#15879=EDGE_LOOP('',(#64002,#64003,#64004,#64005));
#15880=EDGE_LOOP('',(#64006,#64007,#64008,#64009));
#15881=EDGE_LOOP('',(#64010,#64011,#64012,#64013));
#15882=EDGE_LOOP('',(#64014,#64015,#64016,#64017));
#15883=EDGE_LOOP('',(#64018,#64019,#64020,#64021));
#15884=EDGE_LOOP('',(#64022,#64023,#64024,#64025));
#15885=EDGE_LOOP('',(#64026,#64027,#64028,#64029));
#15886=EDGE_LOOP('',(#64030,#64031,#64032,#64033));
#15887=EDGE_LOOP('',(#64034,#64035,#64036,#64037,#64038));
#15888=EDGE_LOOP('',(#64039,#64040,#64041,#64042,#64043));
#15889=EDGE_LOOP('',(#64044,#64045,#64046,#64047));
#15890=EDGE_LOOP('',(#64048,#64049,#64050,#64051));
#15891=EDGE_LOOP('',(#64052,#64053,#64054,#64055));
#15892=EDGE_LOOP('',(#64056,#64057,#64058,#64059));
#15893=EDGE_LOOP('',(#64060,#64061,#64062,#64063));
#15894=EDGE_LOOP('',(#64064,#64065,#64066,#64067));
#15895=EDGE_LOOP('',(#64068,#64069,#64070,#64071));
#15896=EDGE_LOOP('',(#64072,#64073,#64074,#64075));
#15897=EDGE_LOOP('',(#64076,#64077,#64078,#64079));
#15898=EDGE_LOOP('',(#64080,#64081,#64082,#64083));
#15899=EDGE_LOOP('',(#64084,#64085,#64086,#64087));
#15900=EDGE_LOOP('',(#64088,#64089,#64090,#64091));
#15901=EDGE_LOOP('',(#64092,#64093,#64094,#64095));
#15902=EDGE_LOOP('',(#64096,#64097,#64098,#64099));
#15903=EDGE_LOOP('',(#64100,#64101,#64102,#64103));
#15904=EDGE_LOOP('',(#64104,#64105,#64106,#64107));
#15905=EDGE_LOOP('',(#64108,#64109,#64110,#64111));
#15906=EDGE_LOOP('',(#64112,#64113,#64114,#64115));
#15907=EDGE_LOOP('',(#64116,#64117,#64118,#64119));
#15908=EDGE_LOOP('',(#64120,#64121,#64122,#64123));
#15909=EDGE_LOOP('',(#64124,#64125,#64126,#64127));
#15910=EDGE_LOOP('',(#64128,#64129,#64130,#64131,#64132));
#15911=EDGE_LOOP('',(#64133,#64134,#64135,#64136));
#15912=EDGE_LOOP('',(#64137,#64138,#64139,#64140));
#15913=EDGE_LOOP('',(#64141,#64142,#64143,#64144));
#15914=EDGE_LOOP('',(#64145,#64146,#64147,#64148));
#15915=EDGE_LOOP('',(#64149,#64150,#64151,#64152));
#15916=EDGE_LOOP('',(#64153,#64154,#64155,#64156));
#15917=EDGE_LOOP('',(#64157,#64158,#64159,#64160));
#15918=EDGE_LOOP('',(#64161,#64162,#64163,#64164));
#15919=EDGE_LOOP('',(#64165,#64166,#64167,#64168));
#15920=EDGE_LOOP('',(#64169,#64170,#64171,#64172));
#15921=EDGE_LOOP('',(#64173,#64174,#64175,#64176));
#15922=EDGE_LOOP('',(#64177,#64178,#64179,#64180));
#15923=EDGE_LOOP('',(#64181,#64182,#64183,#64184));
#15924=EDGE_LOOP('',(#64185,#64186,#64187,#64188));
#15925=EDGE_LOOP('',(#64189,#64190,#64191,#64192));
#15926=EDGE_LOOP('',(#64193,#64194,#64195,#64196));
#15927=EDGE_LOOP('',(#64197,#64198,#64199,#64200));
#15928=EDGE_LOOP('',(#64201,#64202,#64203,#64204));
#15929=EDGE_LOOP('',(#64205,#64206,#64207,#64208));
#15930=EDGE_LOOP('',(#64209,#64210,#64211,#64212));
#15931=EDGE_LOOP('',(#64213,#64214,#64215,#64216));
#15932=EDGE_LOOP('',(#64217,#64218,#64219,#64220));
#15933=EDGE_LOOP('',(#64221,#64222,#64223,#64224));
#15934=EDGE_LOOP('',(#64225,#64226,#64227,#64228));
#15935=EDGE_LOOP('',(#64229,#64230,#64231,#64232));
#15936=EDGE_LOOP('',(#64233,#64234,#64235,#64236));
#15937=EDGE_LOOP('',(#64237,#64238,#64239,#64240));
#15938=EDGE_LOOP('',(#64241,#64242,#64243,#64244));
#15939=EDGE_LOOP('',(#64245,#64246,#64247,#64248));
#15940=EDGE_LOOP('',(#64249,#64250,#64251,#64252));
#15941=EDGE_LOOP('',(#64253,#64254,#64255,#64256));
#15942=EDGE_LOOP('',(#64257,#64258,#64259,#64260));
#15943=EDGE_LOOP('',(#64261,#64262,#64263,#64264));
#15944=EDGE_LOOP('',(#64265,#64266,#64267,#64268));
#15945=EDGE_LOOP('',(#64269,#64270,#64271,#64272));
#15946=EDGE_LOOP('',(#64273,#64274,#64275,#64276));
#15947=EDGE_LOOP('',(#64277,#64278,#64279,#64280));
#15948=EDGE_LOOP('',(#64281,#64282,#64283,#64284));
#15949=EDGE_LOOP('',(#64285,#64286,#64287,#64288));
#15950=EDGE_LOOP('',(#64289,#64290,#64291,#64292));
#15951=EDGE_LOOP('',(#64293,#64294,#64295,#64296));
#15952=EDGE_LOOP('',(#64297,#64298,#64299,#64300));
#15953=EDGE_LOOP('',(#64301,#64302,#64303,#64304));
#15954=EDGE_LOOP('',(#64305,#64306,#64307,#64308));
#15955=EDGE_LOOP('',(#64309,#64310,#64311,#64312));
#15956=EDGE_LOOP('',(#64313,#64314,#64315,#64316));
#15957=EDGE_LOOP('',(#64317,#64318,#64319,#64320));
#15958=EDGE_LOOP('',(#64321,#64322,#64323,#64324));
#15959=EDGE_LOOP('',(#64325,#64326,#64327,#64328,#64329));
#15960=EDGE_LOOP('',(#64330,#64331,#64332,#64333));
#15961=EDGE_LOOP('',(#64334,#64335,#64336,#64337));
#15962=EDGE_LOOP('',(#64338,#64339,#64340,#64341));
#15963=EDGE_LOOP('',(#64342,#64343,#64344,#64345));
#15964=EDGE_LOOP('',(#64346,#64347,#64348,#64349));
#15965=EDGE_LOOP('',(#64350,#64351,#64352,#64353));
#15966=EDGE_LOOP('',(#64354,#64355,#64356,#64357));
#15967=EDGE_LOOP('',(#64358,#64359,#64360,#64361,#64362));
#15968=EDGE_LOOP('',(#64363,#64364,#64365,#64366));
#15969=EDGE_LOOP('',(#64367,#64368,#64369,#64370));
#15970=EDGE_LOOP('',(#64371,#64372,#64373,#64374));
#15971=EDGE_LOOP('',(#64375,#64376,#64377,#64378));
#15972=EDGE_LOOP('',(#64379,#64380,#64381,#64382));
#15973=EDGE_LOOP('',(#64383,#64384,#64385,#64386));
#15974=EDGE_LOOP('',(#64387,#64388,#64389,#64390));
#15975=EDGE_LOOP('',(#64391,#64392,#64393,#64394));
#15976=EDGE_LOOP('',(#64395,#64396,#64397,#64398));
#15977=EDGE_LOOP('',(#64399,#64400,#64401,#64402));
#15978=EDGE_LOOP('',(#64403,#64404,#64405,#64406));
#15979=EDGE_LOOP('',(#64407,#64408,#64409,#64410));
#15980=EDGE_LOOP('',(#64411,#64412,#64413,#64414));
#15981=EDGE_LOOP('',(#64415,#64416,#64417,#64418));
#15982=EDGE_LOOP('',(#64419,#64420,#64421,#64422));
#15983=EDGE_LOOP('',(#64423,#64424,#64425,#64426,#64427));
#15984=EDGE_LOOP('',(#64428,#64429,#64430,#64431,#64432));
#15985=EDGE_LOOP('',(#64433,#64434,#64435,#64436));
#15986=EDGE_LOOP('',(#64437,#64438,#64439,#64440));
#15987=EDGE_LOOP('',(#64441,#64442,#64443,#64444));
#15988=EDGE_LOOP('',(#64445,#64446,#64447,#64448));
#15989=EDGE_LOOP('',(#64449,#64450,#64451,#64452));
#15990=EDGE_LOOP('',(#64453,#64454,#64455,#64456));
#15991=EDGE_LOOP('',(#64457,#64458,#64459,#64460));
#15992=EDGE_LOOP('',(#64461,#64462,#64463,#64464));
#15993=EDGE_LOOP('',(#64465,#64466,#64467,#64468));
#15994=EDGE_LOOP('',(#64469,#64470,#64471,#64472));
#15995=EDGE_LOOP('',(#64473,#64474,#64475,#64476));
#15996=EDGE_LOOP('',(#64477,#64478,#64479,#64480));
#15997=EDGE_LOOP('',(#64481,#64482,#64483,#64484));
#15998=EDGE_LOOP('',(#64485,#64486,#64487,#64488));
#15999=EDGE_LOOP('',(#64489,#64490,#64491,#64492));
#16000=EDGE_LOOP('',(#64493,#64494,#64495,#64496));
#16001=EDGE_LOOP('',(#64497,#64498,#64499,#64500));
#16002=EDGE_LOOP('',(#64501,#64502,#64503,#64504));
#16003=EDGE_LOOP('',(#64505,#64506,#64507,#64508));
#16004=EDGE_LOOP('',(#64509,#64510,#64511,#64512));
#16005=EDGE_LOOP('',(#64513,#64514,#64515,#64516));
#16006=EDGE_LOOP('',(#64517,#64518,#64519,#64520));
#16007=EDGE_LOOP('',(#64521,#64522,#64523,#64524));
#16008=EDGE_LOOP('',(#64525,#64526,#64527,#64528));
#16009=EDGE_LOOP('',(#64529,#64530,#64531,#64532));
#16010=EDGE_LOOP('',(#64533,#64534,#64535,#64536));
#16011=EDGE_LOOP('',(#64537,#64538,#64539,#64540));
#16012=EDGE_LOOP('',(#64541,#64542,#64543,#64544));
#16013=EDGE_LOOP('',(#64545,#64546,#64547,#64548));
#16014=EDGE_LOOP('',(#64549,#64550,#64551,#64552));
#16015=EDGE_LOOP('',(#64553,#64554,#64555,#64556));
#16016=EDGE_LOOP('',(#64557,#64558,#64559,#64560));
#16017=EDGE_LOOP('',(#64561,#64562,#64563,#64564));
#16018=EDGE_LOOP('',(#64565,#64566,#64567,#64568));
#16019=EDGE_LOOP('',(#64569,#64570,#64571,#64572));
#16020=EDGE_LOOP('',(#64573,#64574,#64575,#64576));
#16021=EDGE_LOOP('',(#64577,#64578,#64579,#64580));
#16022=EDGE_LOOP('',(#64581,#64582,#64583,#64584));
#16023=EDGE_LOOP('',(#64585,#64586,#64587,#64588));
#16024=EDGE_LOOP('',(#64589,#64590,#64591,#64592));
#16025=EDGE_LOOP('',(#64593,#64594,#64595,#64596));
#16026=EDGE_LOOP('',(#64597,#64598,#64599,#64600));
#16027=EDGE_LOOP('',(#64601,#64602,#64603,#64604));
#16028=EDGE_LOOP('',(#64605,#64606,#64607,#64608));
#16029=EDGE_LOOP('',(#64609,#64610,#64611,#64612));
#16030=EDGE_LOOP('',(#64613,#64614,#64615,#64616));
#16031=EDGE_LOOP('',(#64617,#64618,#64619,#64620));
#16032=EDGE_LOOP('',(#64621,#64622,#64623,#64624));
#16033=EDGE_LOOP('',(#64625,#64626,#64627,#64628));
#16034=EDGE_LOOP('',(#64629,#64630,#64631,#64632));
#16035=EDGE_LOOP('',(#64633,#64634,#64635,#64636));
#16036=EDGE_LOOP('',(#64637,#64638,#64639,#64640));
#16037=EDGE_LOOP('',(#64641,#64642,#64643,#64644));
#16038=EDGE_LOOP('',(#64645,#64646,#64647,#64648));
#16039=EDGE_LOOP('',(#64649,#64650,#64651,#64652));
#16040=EDGE_LOOP('',(#64653,#64654,#64655,#64656));
#16041=EDGE_LOOP('',(#64657,#64658,#64659,#64660));
#16042=EDGE_LOOP('',(#64661,#64662,#64663,#64664));
#16043=EDGE_LOOP('',(#64665,#64666,#64667,#64668));
#16044=EDGE_LOOP('',(#64669,#64670,#64671,#64672));
#16045=EDGE_LOOP('',(#64673,#64674,#64675,#64676));
#16046=EDGE_LOOP('',(#64677,#64678,#64679,#64680));
#16047=EDGE_LOOP('',(#64681,#64682,#64683,#64684));
#16048=EDGE_LOOP('',(#64685,#64686,#64687,#64688));
#16049=EDGE_LOOP('',(#64689,#64690,#64691,#64692));
#16050=EDGE_LOOP('',(#64693,#64694,#64695,#64696));
#16051=EDGE_LOOP('',(#64697,#64698,#64699,#64700));
#16052=EDGE_LOOP('',(#64701,#64702,#64703,#64704));
#16053=EDGE_LOOP('',(#64705,#64706,#64707,#64708));
#16054=EDGE_LOOP('',(#64709,#64710,#64711,#64712));
#16055=EDGE_LOOP('',(#64713,#64714,#64715,#64716));
#16056=EDGE_LOOP('',(#64717,#64718,#64719,#64720));
#16057=EDGE_LOOP('',(#64721,#64722,#64723,#64724));
#16058=EDGE_LOOP('',(#64725,#64726,#64727,#64728));
#16059=EDGE_LOOP('',(#64729,#64730,#64731,#64732));
#16060=EDGE_LOOP('',(#64733,#64734,#64735,#64736));
#16061=EDGE_LOOP('',(#64737,#64738,#64739,#64740));
#16062=EDGE_LOOP('',(#64741,#64742,#64743,#64744));
#16063=EDGE_LOOP('',(#64745,#64746,#64747,#64748));
#16064=EDGE_LOOP('',(#64749,#64750,#64751,#64752));
#16065=EDGE_LOOP('',(#64753,#64754,#64755,#64756));
#16066=EDGE_LOOP('',(#64757,#64758,#64759,#64760));
#16067=EDGE_LOOP('',(#64761,#64762,#64763,#64764));
#16068=EDGE_LOOP('',(#64765,#64766,#64767,#64768));
#16069=EDGE_LOOP('',(#64769,#64770,#64771,#64772));
#16070=EDGE_LOOP('',(#64773,#64774,#64775,#64776));
#16071=EDGE_LOOP('',(#64777,#64778,#64779,#64780));
#16072=EDGE_LOOP('',(#64781,#64782,#64783,#64784));
#16073=EDGE_LOOP('',(#64785,#64786,#64787,#64788));
#16074=EDGE_LOOP('',(#64789,#64790,#64791,#64792,#64793));
#16075=EDGE_LOOP('',(#64794,#64795,#64796,#64797,#64798));
#16076=EDGE_LOOP('',(#64799,#64800,#64801,#64802));
#16077=EDGE_LOOP('',(#64803,#64804,#64805,#64806));
#16078=EDGE_LOOP('',(#64807,#64808,#64809,#64810));
#16079=EDGE_LOOP('',(#64811,#64812,#64813,#64814));
#16080=EDGE_LOOP('',(#64815,#64816,#64817,#64818));
#16081=EDGE_LOOP('',(#64819,#64820,#64821,#64822));
#16082=EDGE_LOOP('',(#64823,#64824,#64825,#64826));
#16083=EDGE_LOOP('',(#64827,#64828,#64829,#64830));
#16084=EDGE_LOOP('',(#64831,#64832,#64833,#64834));
#16085=EDGE_LOOP('',(#64835,#64836,#64837,#64838));
#16086=EDGE_LOOP('',(#64839,#64840,#64841,#64842));
#16087=EDGE_LOOP('',(#64843,#64844,#64845,#64846));
#16088=EDGE_LOOP('',(#64847,#64848,#64849,#64850));
#16089=EDGE_LOOP('',(#64851,#64852,#64853,#64854));
#16090=EDGE_LOOP('',(#64855,#64856,#64857,#64858));
#16091=EDGE_LOOP('',(#64859,#64860,#64861,#64862));
#16092=EDGE_LOOP('',(#64863,#64864,#64865,#64866));
#16093=EDGE_LOOP('',(#64867,#64868,#64869,#64870));
#16094=EDGE_LOOP('',(#64871,#64872,#64873,#64874));
#16095=EDGE_LOOP('',(#64875,#64876,#64877,#64878));
#16096=EDGE_LOOP('',(#64879,#64880,#64881,#64882));
#16097=EDGE_LOOP('',(#64883,#64884,#64885,#64886));
#16098=EDGE_LOOP('',(#64887,#64888,#64889,#64890));
#16099=EDGE_LOOP('',(#64891,#64892,#64893,#64894));
#16100=EDGE_LOOP('',(#64895,#64896,#64897,#64898));
#16101=EDGE_LOOP('',(#64899,#64900,#64901,#64902));
#16102=EDGE_LOOP('',(#64903,#64904,#64905,#64906));
#16103=EDGE_LOOP('',(#64907,#64908,#64909,#64910));
#16104=EDGE_LOOP('',(#64911,#64912,#64913,#64914));
#16105=EDGE_LOOP('',(#64915,#64916,#64917,#64918,#64919));
#16106=EDGE_LOOP('',(#64920,#64921,#64922,#64923));
#16107=EDGE_LOOP('',(#64924,#64925,#64926,#64927));
#16108=EDGE_LOOP('',(#64928,#64929,#64930,#64931));
#16109=EDGE_LOOP('',(#64932,#64933,#64934,#64935));
#16110=EDGE_LOOP('',(#64936,#64937,#64938,#64939));
#16111=EDGE_LOOP('',(#64940,#64941,#64942,#64943));
#16112=EDGE_LOOP('',(#64944,#64945,#64946,#64947));
#16113=EDGE_LOOP('',(#64948,#64949,#64950,#64951));
#16114=EDGE_LOOP('',(#64952,#64953,#64954,#64955));
#16115=EDGE_LOOP('',(#64956,#64957,#64958,#64959));
#16116=EDGE_LOOP('',(#64960,#64961,#64962,#64963));
#16117=EDGE_LOOP('',(#64964,#64965,#64966,#64967));
#16118=EDGE_LOOP('',(#64968,#64969,#64970,#64971));
#16119=EDGE_LOOP('',(#64972,#64973,#64974,#64975));
#16120=EDGE_LOOP('',(#64976,#64977,#64978,#64979));
#16121=EDGE_LOOP('',(#64980,#64981,#64982,#64983));
#16122=EDGE_LOOP('',(#64984,#64985,#64986,#64987));
#16123=EDGE_LOOP('',(#64988,#64989,#64990,#64991));
#16124=EDGE_LOOP('',(#64992,#64993,#64994,#64995));
#16125=EDGE_LOOP('',(#64996,#64997,#64998,#64999));
#16126=EDGE_LOOP('',(#65000,#65001,#65002,#65003));
#16127=EDGE_LOOP('',(#65004,#65005,#65006,#65007));
#16128=EDGE_LOOP('',(#65008,#65009,#65010,#65011));
#16129=EDGE_LOOP('',(#65012,#65013,#65014,#65015));
#16130=EDGE_LOOP('',(#65016,#65017,#65018,#65019));
#16131=EDGE_LOOP('',(#65020,#65021,#65022,#65023));
#16132=EDGE_LOOP('',(#65024,#65025,#65026,#65027));
#16133=EDGE_LOOP('',(#65028,#65029,#65030,#65031));
#16134=EDGE_LOOP('',(#65032,#65033,#65034,#65035));
#16135=EDGE_LOOP('',(#65036,#65037,#65038,#65039));
#16136=EDGE_LOOP('',(#65040,#65041,#65042,#65043));
#16137=EDGE_LOOP('',(#65044,#65045,#65046,#65047));
#16138=EDGE_LOOP('',(#65048,#65049,#65050,#65051));
#16139=EDGE_LOOP('',(#65052,#65053,#65054,#65055));
#16140=EDGE_LOOP('',(#65056,#65057,#65058,#65059));
#16141=EDGE_LOOP('',(#65060,#65061,#65062,#65063));
#16142=EDGE_LOOP('',(#65064,#65065,#65066,#65067));
#16143=EDGE_LOOP('',(#65068,#65069,#65070,#65071));
#16144=EDGE_LOOP('',(#65072,#65073,#65074,#65075));
#16145=EDGE_LOOP('',(#65076,#65077,#65078,#65079));
#16146=EDGE_LOOP('',(#65080,#65081,#65082,#65083));
#16147=EDGE_LOOP('',(#65084,#65085,#65086,#65087));
#16148=EDGE_LOOP('',(#65088,#65089,#65090,#65091));
#16149=EDGE_LOOP('',(#65092,#65093,#65094,#65095));
#16150=EDGE_LOOP('',(#65096,#65097,#65098,#65099));
#16151=EDGE_LOOP('',(#65100,#65101,#65102,#65103));
#16152=EDGE_LOOP('',(#65104,#65105,#65106,#65107));
#16153=EDGE_LOOP('',(#65108,#65109,#65110,#65111));
#16154=EDGE_LOOP('',(#65112,#65113,#65114,#65115));
#16155=EDGE_LOOP('',(#65116,#65117,#65118,#65119));
#16156=EDGE_LOOP('',(#65120,#65121,#65122,#65123));
#16157=EDGE_LOOP('',(#65124,#65125,#65126,#65127));
#16158=EDGE_LOOP('',(#65128,#65129,#65130,#65131));
#16159=EDGE_LOOP('',(#65132,#65133,#65134,#65135));
#16160=EDGE_LOOP('',(#65136,#65137,#65138,#65139));
#16161=EDGE_LOOP('',(#65140,#65141,#65142,#65143));
#16162=EDGE_LOOP('',(#65144,#65145,#65146,#65147));
#16163=EDGE_LOOP('',(#65148,#65149,#65150,#65151));
#16164=EDGE_LOOP('',(#65152,#65153,#65154,#65155));
#16165=EDGE_LOOP('',(#65156,#65157,#65158,#65159));
#16166=EDGE_LOOP('',(#65160,#65161,#65162,#65163));
#16167=EDGE_LOOP('',(#65164,#65165,#65166,#65167));
#16168=EDGE_LOOP('',(#65168,#65169,#65170,#65171));
#16169=EDGE_LOOP('',(#65172,#65173,#65174,#65175));
#16170=EDGE_LOOP('',(#65176,#65177,#65178,#65179));
#16171=EDGE_LOOP('',(#65180,#65181,#65182,#65183));
#16172=EDGE_LOOP('',(#65184,#65185,#65186,#65187));
#16173=EDGE_LOOP('',(#65188,#65189,#65190,#65191));
#16174=EDGE_LOOP('',(#65192,#65193,#65194,#65195));
#16175=EDGE_LOOP('',(#65196,#65197,#65198,#65199));
#16176=EDGE_LOOP('',(#65200,#65201,#65202,#65203));
#16177=EDGE_LOOP('',(#65204,#65205,#65206,#65207));
#16178=EDGE_LOOP('',(#65208,#65209,#65210,#65211));
#16179=EDGE_LOOP('',(#65212,#65213,#65214,#65215));
#16180=EDGE_LOOP('',(#65216,#65217,#65218,#65219,#65220));
#16181=EDGE_LOOP('',(#65221,#65222,#65223,#65224));
#16182=EDGE_LOOP('',(#65225,#65226,#65227,#65228));
#16183=EDGE_LOOP('',(#65229,#65230,#65231,#65232));
#16184=EDGE_LOOP('',(#65233,#65234,#65235,#65236));
#16185=EDGE_LOOP('',(#65237,#65238,#65239,#65240));
#16186=EDGE_LOOP('',(#65241,#65242,#65243,#65244));
#16187=EDGE_LOOP('',(#65245,#65246,#65247,#65248));
#16188=EDGE_LOOP('',(#65249,#65250,#65251,#65252));
#16189=EDGE_LOOP('',(#65253,#65254,#65255,#65256));
#16190=EDGE_LOOP('',(#65257,#65258,#65259,#65260));
#16191=EDGE_LOOP('',(#65261,#65262,#65263,#65264));
#16192=EDGE_LOOP('',(#65265,#65266,#65267,#65268));
#16193=EDGE_LOOP('',(#65269,#65270,#65271,#65272));
#16194=EDGE_LOOP('',(#65273,#65274,#65275,#65276));
#16195=EDGE_LOOP('',(#65277,#65278,#65279,#65280));
#16196=EDGE_LOOP('',(#65281,#65282,#65283,#65284));
#16197=EDGE_LOOP('',(#65285,#65286,#65287,#65288));
#16198=EDGE_LOOP('',(#65289,#65290,#65291,#65292));
#16199=EDGE_LOOP('',(#65293,#65294,#65295,#65296));
#16200=EDGE_LOOP('',(#65297,#65298,#65299,#65300));
#16201=EDGE_LOOP('',(#65301,#65302,#65303,#65304));
#16202=EDGE_LOOP('',(#65305,#65306,#65307,#65308));
#16203=EDGE_LOOP('',(#65309,#65310,#65311,#65312));
#16204=EDGE_LOOP('',(#65313,#65314,#65315,#65316));
#16205=EDGE_LOOP('',(#65317,#65318,#65319,#65320));
#16206=EDGE_LOOP('',(#65321,#65322,#65323,#65324));
#16207=EDGE_LOOP('',(#65325,#65326,#65327,#65328));
#16208=EDGE_LOOP('',(#65329,#65330,#65331,#65332));
#16209=EDGE_LOOP('',(#65333,#65334,#65335,#65336));
#16210=EDGE_LOOP('',(#65337,#65338,#65339,#65340));
#16211=EDGE_LOOP('',(#65341,#65342,#65343,#65344));
#16212=EDGE_LOOP('',(#65345,#65346,#65347,#65348));
#16213=EDGE_LOOP('',(#65349,#65350,#65351,#65352));
#16214=EDGE_LOOP('',(#65353,#65354,#65355,#65356));
#16215=EDGE_LOOP('',(#65357,#65358,#65359,#65360));
#16216=EDGE_LOOP('',(#65361,#65362,#65363,#65364));
#16217=EDGE_LOOP('',(#65365,#65366,#65367,#65368));
#16218=EDGE_LOOP('',(#65369,#65370,#65371,#65372));
#16219=EDGE_LOOP('',(#65373,#65374,#65375,#65376));
#16220=EDGE_LOOP('',(#65377,#65378,#65379,#65380));
#16221=EDGE_LOOP('',(#65381,#65382,#65383,#65384));
#16222=EDGE_LOOP('',(#65385,#65386,#65387,#65388));
#16223=EDGE_LOOP('',(#65389,#65390,#65391,#65392));
#16224=EDGE_LOOP('',(#65393,#65394,#65395,#65396));
#16225=EDGE_LOOP('',(#65397,#65398,#65399,#65400));
#16226=EDGE_LOOP('',(#65401,#65402,#65403,#65404));
#16227=EDGE_LOOP('',(#65405,#65406,#65407,#65408));
#16228=EDGE_LOOP('',(#65409,#65410,#65411,#65412));
#16229=EDGE_LOOP('',(#65413,#65414,#65415,#65416));
#16230=EDGE_LOOP('',(#65417,#65418,#65419,#65420));
#16231=EDGE_LOOP('',(#65421,#65422,#65423,#65424));
#16232=EDGE_LOOP('',(#65425,#65426,#65427,#65428));
#16233=EDGE_LOOP('',(#65429,#65430,#65431,#65432));
#16234=EDGE_LOOP('',(#65433,#65434,#65435,#65436));
#16235=EDGE_LOOP('',(#65437,#65438,#65439,#65440));
#16236=EDGE_LOOP('',(#65441,#65442,#65443,#65444));
#16237=EDGE_LOOP('',(#65445,#65446,#65447,#65448));
#16238=EDGE_LOOP('',(#65449,#65450,#65451,#65452));
#16239=EDGE_LOOP('',(#65453,#65454,#65455,#65456));
#16240=EDGE_LOOP('',(#65457,#65458,#65459,#65460));
#16241=EDGE_LOOP('',(#65461,#65462,#65463,#65464));
#16242=EDGE_LOOP('',(#65465,#65466,#65467,#65468));
#16243=EDGE_LOOP('',(#65469,#65470,#65471,#65472));
#16244=EDGE_LOOP('',(#65473,#65474,#65475,#65476));
#16245=EDGE_LOOP('',(#65477,#65478,#65479,#65480));
#16246=EDGE_LOOP('',(#65481,#65482,#65483,#65484));
#16247=EDGE_LOOP('',(#65485,#65486,#65487,#65488));
#16248=EDGE_LOOP('',(#65489,#65490,#65491,#65492));
#16249=EDGE_LOOP('',(#65493,#65494,#65495,#65496));
#16250=EDGE_LOOP('',(#65497,#65498,#65499,#65500));
#16251=EDGE_LOOP('',(#65501,#65502,#65503,#65504));
#16252=EDGE_LOOP('',(#65505,#65506,#65507,#65508));
#16253=EDGE_LOOP('',(#65509,#65510,#65511,#65512));
#16254=EDGE_LOOP('',(#65513,#65514,#65515,#65516));
#16255=EDGE_LOOP('',(#65517,#65518,#65519,#65520));
#16256=EDGE_LOOP('',(#65521,#65522,#65523,#65524));
#16257=EDGE_LOOP('',(#65525,#65526,#65527,#65528));
#16258=EDGE_LOOP('',(#65529,#65530,#65531,#65532));
#16259=EDGE_LOOP('',(#65533,#65534,#65535,#65536));
#16260=EDGE_LOOP('',(#65537,#65538,#65539,#65540));
#16261=EDGE_LOOP('',(#65541,#65542,#65543,#65544));
#16262=EDGE_LOOP('',(#65545,#65546,#65547,#65548));
#16263=EDGE_LOOP('',(#65549,#65550,#65551,#65552));
#16264=EDGE_LOOP('',(#65553,#65554,#65555,#65556));
#16265=EDGE_LOOP('',(#65557,#65558,#65559,#65560));
#16266=EDGE_LOOP('',(#65561,#65562,#65563,#65564));
#16267=EDGE_LOOP('',(#65565,#65566,#65567,#65568));
#16268=EDGE_LOOP('',(#65569,#65570,#65571,#65572));
#16269=EDGE_LOOP('',(#65573,#65574,#65575,#65576));
#16270=EDGE_LOOP('',(#65577,#65578,#65579,#65580));
#16271=EDGE_LOOP('',(#65581,#65582,#65583,#65584));
#16272=EDGE_LOOP('',(#65585,#65586,#65587,#65588));
#16273=EDGE_LOOP('',(#65589,#65590,#65591,#65592));
#16274=EDGE_LOOP('',(#65593,#65594,#65595,#65596));
#16275=EDGE_LOOP('',(#65597,#65598,#65599,#65600));
#16276=EDGE_LOOP('',(#65601,#65602,#65603,#65604,#65605));
#16277=EDGE_LOOP('',(#65606,#65607,#65608,#65609));
#16278=EDGE_LOOP('',(#65610,#65611,#65612,#65613));
#16279=EDGE_LOOP('',(#65614,#65615,#65616,#65617));
#16280=EDGE_LOOP('',(#65618,#65619,#65620,#65621));
#16281=EDGE_LOOP('',(#65622,#65623,#65624,#65625));
#16282=EDGE_LOOP('',(#65626,#65627,#65628,#65629));
#16283=EDGE_LOOP('',(#65630,#65631,#65632,#65633));
#16284=EDGE_LOOP('',(#65634,#65635,#65636,#65637));
#16285=EDGE_LOOP('',(#65638,#65639,#65640,#65641));
#16286=EDGE_LOOP('',(#65642,#65643,#65644,#65645));
#16287=EDGE_LOOP('',(#65646,#65647,#65648,#65649));
#16288=EDGE_LOOP('',(#65650,#65651,#65652,#65653));
#16289=EDGE_LOOP('',(#65654,#65655,#65656,#65657));
#16290=EDGE_LOOP('',(#65658,#65659,#65660,#65661));
#16291=EDGE_LOOP('',(#65662,#65663,#65664,#65665));
#16292=EDGE_LOOP('',(#65666,#65667,#65668,#65669));
#16293=EDGE_LOOP('',(#65670,#65671,#65672,#65673));
#16294=EDGE_LOOP('',(#65674,#65675,#65676,#65677));
#16295=EDGE_LOOP('',(#65678,#65679,#65680,#65681));
#16296=EDGE_LOOP('',(#65682,#65683,#65684));
#16297=EDGE_LOOP('',(#65685,#65686,#65687,#65688,#65689,#65690,#65691,#65692));
#16298=EDGE_LOOP('',(#65693,#65694,#65695,#65696,#65697));
#16299=EDGE_LOOP('',(#65698,#65699,#65700,#65701));
#16300=EDGE_LOOP('',(#65702,#65703,#65704,#65705));
#16301=EDGE_LOOP('',(#65706,#65707,#65708,#65709,#65710,#65711,#65712,#65713,
#65714));
#16302=EDGE_LOOP('',(#65715,#65716,#65717,#65718));
#16303=EDGE_LOOP('',(#65719,#65720,#65721,#65722,#65723,#65724,#65725,#65726,
#65727,#65728,#65729,#65730,#65731,#65732,#65733,#65734,#65735));
#16304=EDGE_LOOP('',(#65736,#65737,#65738,#65739));
#16305=EDGE_LOOP('',(#65740,#65741,#65742,#65743));
#16306=EDGE_LOOP('',(#65744,#65745,#65746,#65747));
#16307=EDGE_LOOP('',(#65748,#65749,#65750,#65751,#65752,#65753,#65754,#65755,
#65756,#65757,#65758,#65759,#65760,#65761,#65762,#65763,#65764));
#16308=EDGE_LOOP('',(#65765,#65766,#65767,#65768,#65769,#65770));
#16309=EDGE_LOOP('',(#65771,#65772,#65773,#65774,#65775,#65776,#65777,#65778,
#65779,#65780,#65781,#65782,#65783,#65784,#65785,#65786,#65787,#65788,#65789,
#65790,#65791,#65792,#65793,#65794,#65795,#65796,#65797,#65798,#65799,#65800,
#65801,#65802,#65803,#65804,#65805,#65806,#65807,#65808,#65809,#65810,#65811,
#65812,#65813,#65814));
#16310=EDGE_LOOP('',(#65815,#65816,#65817,#65818,#65819,#65820));
#16311=EDGE_LOOP('',(#65821,#65822,#65823,#65824,#65825,#65826,#65827,#65828,
#65829,#65830,#65831,#65832,#65833,#65834,#65835,#65836,#65837));
#16312=EDGE_LOOP('',(#65838,#65839,#65840,#65841));
#16313=EDGE_LOOP('',(#65842,#65843,#65844,#65845));
#16314=EDGE_LOOP('',(#65846,#65847,#65848,#65849));
#16315=EDGE_LOOP('',(#65850,#65851,#65852,#65853,#65854,#65855,#65856));
#16316=EDGE_LOOP('',(#65857,#65858,#65859,#65860));
#16317=EDGE_LOOP('',(#65861,#65862,#65863,#65864));
#16318=EDGE_LOOP('',(#65865,#65866,#65867,#65868));
#16319=EDGE_LOOP('',(#65869,#65870,#65871,#65872));
#16320=EDGE_LOOP('',(#65873,#65874,#65875,#65876));
#16321=EDGE_LOOP('',(#65877,#65878,#65879,#65880));
#16322=EDGE_LOOP('',(#65881,#65882,#65883,#65884));
#16323=EDGE_LOOP('',(#65885,#65886,#65887,#65888));
#16324=EDGE_LOOP('',(#65889,#65890,#65891,#65892));
#16325=EDGE_LOOP('',(#65893,#65894,#65895,#65896));
#16326=EDGE_LOOP('',(#65897,#65898,#65899,#65900));
#16327=EDGE_LOOP('',(#65901,#65902,#65903,#65904));
#16328=EDGE_LOOP('',(#65905,#65906,#65907,#65908));
#16329=EDGE_LOOP('',(#65909,#65910,#65911,#65912));
#16330=EDGE_LOOP('',(#65913,#65914,#65915,#65916));
#16331=EDGE_LOOP('',(#65917,#65918,#65919,#65920));
#16332=EDGE_LOOP('',(#65921,#65922,#65923,#65924));
#16333=EDGE_LOOP('',(#65925,#65926,#65927,#65928));
#16334=EDGE_LOOP('',(#65929,#65930,#65931,#65932));
#16335=EDGE_LOOP('',(#65933,#65934,#65935,#65936));
#16336=EDGE_LOOP('',(#65937,#65938,#65939));
#16337=EDGE_LOOP('',(#65940,#65941,#65942,#65943,#65944));
#16338=EDGE_LOOP('',(#65945,#65946,#65947,#65948));
#16339=EDGE_LOOP('',(#65949,#65950,#65951,#65952));
#16340=EDGE_LOOP('',(#65953,#65954,#65955,#65956));
#16341=EDGE_LOOP('',(#65957,#65958,#65959,#65960));
#16342=EDGE_LOOP('',(#65961,#65962,#65963,#65964));
#16343=EDGE_LOOP('',(#65965,#65966,#65967,#65968,#65969));
#16344=EDGE_LOOP('',(#65970,#65971,#65972,#65973,#65974));
#16345=EDGE_LOOP('',(#65975,#65976,#65977,#65978));
#16346=EDGE_LOOP('',(#65979,#65980,#65981,#65982));
#16347=EDGE_LOOP('',(#65983,#65984,#65985,#65986));
#16348=EDGE_LOOP('',(#65987,#65988,#65989,#65990));
#16349=EDGE_LOOP('',(#65991,#65992,#65993,#65994));
#16350=EDGE_LOOP('',(#65995,#65996,#65997,#65998));
#16351=EDGE_LOOP('',(#65999,#66000,#66001,#66002));
#16352=EDGE_LOOP('',(#66003,#66004,#66005,#66006));
#16353=EDGE_LOOP('',(#66007,#66008,#66009,#66010));
#16354=EDGE_LOOP('',(#66011,#66012,#66013,#66014));
#16355=EDGE_LOOP('',(#66015,#66016,#66017,#66018));
#16356=EDGE_LOOP('',(#66019,#66020,#66021,#66022));
#16357=EDGE_LOOP('',(#66023,#66024,#66025,#66026));
#16358=EDGE_LOOP('',(#66027,#66028,#66029,#66030));
#16359=EDGE_LOOP('',(#66031,#66032,#66033,#66034,#66035,#66036,#66037,#66038));
#16360=EDGE_LOOP('',(#66039));
#16361=EDGE_LOOP('',(#66040));
#16362=EDGE_LOOP('',(#66041,#66042,#66043,#66044));
#16363=EDGE_LOOP('',(#66045,#66046,#66047,#66048));
#16364=EDGE_LOOP('',(#66049,#66050,#66051,#66052));
#16365=EDGE_LOOP('',(#66053,#66054,#66055,#66056));
#16366=EDGE_LOOP('',(#66057,#66058,#66059,#66060));
#16367=EDGE_LOOP('',(#66061,#66062,#66063,#66064));
#16368=EDGE_LOOP('',(#66065,#66066,#66067,#66068));
#16369=EDGE_LOOP('',(#66069,#66070,#66071,#66072,#66073,#66074));
#16370=EDGE_LOOP('',(#66075));
#16371=EDGE_LOOP('',(#66076));
#16372=EDGE_LOOP('',(#66077,#66078,#66079,#66080));
#16373=EDGE_LOOP('',(#66081,#66082,#66083,#66084));
#16374=EDGE_LOOP('',(#66085,#66086,#66087));
#16375=EDGE_LOOP('',(#66088,#66089,#66090,#66091,#66092,#66093,#66094,#66095,
#66096,#66097,#66098,#66099,#66100,#66101,#66102,#66103,#66104,#66105));
#16376=EDGE_LOOP('',(#66106,#66107,#66108,#66109,#66110));
#16377=EDGE_LOOP('',(#66111,#66112,#66113,#66114));
#16378=EDGE_LOOP('',(#66115,#66116,#66117,#66118));
#16379=EDGE_LOOP('',(#66119,#66120,#66121,#66122));
#16380=EDGE_LOOP('',(#66123,#66124,#66125,#66126,#66127,#66128,#66129,#66130,
#66131,#66132,#66133,#66134,#66135,#66136,#66137,#66138,#66139,#66140));
#16381=EDGE_LOOP('',(#66141,#66142,#66143,#66144));
#16382=EDGE_LOOP('',(#66145,#66146,#66147,#66148));
#16383=EDGE_LOOP('',(#66149,#66150,#66151,#66152));
#16384=EDGE_LOOP('',(#66153,#66154,#66155,#66156,#66157,#66158,#66159,#66160,
#66161,#66162,#66163,#66164,#66165,#66166,#66167,#66168,#66169,#66170));
#16385=EDGE_LOOP('',(#66171,#66172,#66173,#66174));
#16386=EDGE_LOOP('',(#66175,#66176,#66177,#66178));
#16387=EDGE_LOOP('',(#66179,#66180,#66181,#66182));
#16388=EDGE_LOOP('',(#66183,#66184,#66185,#66186,#66187,#66188,#66189,#66190,
#66191,#66192,#66193,#66194,#66195,#66196,#66197,#66198));
#16389=EDGE_LOOP('',(#66199,#66200,#66201,#66202));
#16390=EDGE_LOOP('',(#66203,#66204,#66205,#66206,#66207,#66208,#66209,#66210,
#66211,#66212,#66213,#66214,#66215,#66216,#66217,#66218));
#16391=EDGE_LOOP('',(#66219,#66220,#66221,#66222));
#16392=EDGE_LOOP('',(#66223,#66224,#66225,#66226,#66227));
#16393=EDGE_LOOP('',(#66228,#66229,#66230,#66231,#66232,#66233,#66234,#66235,
#66236,#66237,#66238,#66239,#66240,#66241,#66242,#66243,#66244,#66245));
#16394=EDGE_LOOP('',(#66246,#66247,#66248,#66249));
#16395=EDGE_LOOP('',(#66250,#66251,#66252,#66253));
#16396=EDGE_LOOP('',(#66254,#66255,#66256,#66257));
#16397=EDGE_LOOP('',(#66258,#66259,#66260,#66261,#66262,#66263,#66264,#66265,
#66266,#66267,#66268,#66269,#66270,#66271,#66272,#66273,#66274,#66275));
#16398=EDGE_LOOP('',(#66276,#66277,#66278,#66279));
#16399=EDGE_LOOP('',(#66280,#66281,#66282));
#16400=EDGE_LOOP('',(#66283,#66284,#66285,#66286,#66287,#66288));
#16401=EDGE_LOOP('',(#66289,#66290,#66291));
#16402=EDGE_LOOP('',(#66292,#66293,#66294,#66295));
#16403=EDGE_LOOP('',(#66296,#66297,#66298,#66299,#66300,#66301,#66302,#66303,
#66304,#66305,#66306,#66307,#66308,#66309,#66310,#66311,#66312));
#16404=EDGE_LOOP('',(#66313,#66314,#66315,#66316,#66317,#66318,#66319,#66320,
#66321,#66322,#66323,#66324,#66325,#66326,#66327,#66328,#66329,#66330));
#16405=EDGE_LOOP('',(#66331,#66332,#66333,#66334));
#16406=EDGE_LOOP('',(#66335,#66336,#66337,#66338));
#16407=EDGE_LOOP('',(#66339,#66340,#66341,#66342));
#16408=EDGE_LOOP('',(#66343,#66344,#66345,#66346));
#16409=EDGE_LOOP('',(#66347,#66348,#66349,#66350,#66351,#66352,#66353,#66354,
#66355,#66356,#66357,#66358,#66359,#66360,#66361,#66362,#66363,#66364));
#16410=EDGE_LOOP('',(#66365,#66366,#66367,#66368));
#16411=EDGE_LOOP('',(#66369,#66370,#66371,#66372));
#16412=EDGE_LOOP('',(#66373,#66374,#66375,#66376));
#16413=EDGE_LOOP('',(#66377,#66378,#66379,#66380,#66381,#66382,#66383,#66384,
#66385,#66386,#66387,#66388));
#16414=EDGE_LOOP('',(#66389,#66390,#66391,#66392));
#16415=EDGE_LOOP('',(#66393,#66394,#66395,#66396));
#16416=EDGE_LOOP('',(#66397,#66398,#66399,#66400));
#16417=EDGE_LOOP('',(#66401,#66402,#66403,#66404,#66405,#66406,#66407,#66408));
#16418=EDGE_LOOP('',(#66409,#66410,#66411,#66412));
#16419=EDGE_LOOP('',(#66413,#66414,#66415,#66416));
#16420=EDGE_LOOP('',(#66417,#66418,#66419,#66420,#66421,#66422,#66423,#66424,
#66425,#66426,#66427));
#16421=EDGE_LOOP('',(#66428,#66429,#66430,#66431));
#16422=EDGE_LOOP('',(#66432,#66433,#66434,#66435));
#16423=EDGE_LOOP('',(#66436,#66437,#66438,#66439));
#16424=EDGE_LOOP('',(#66440,#66441,#66442,#66443,#66444,#66445,#66446,#66447,
#66448,#66449,#66450,#66451));
#16425=EDGE_LOOP('',(#66452,#66453,#66454,#66455));
#16426=EDGE_LOOP('',(#66456,#66457,#66458,#66459));
#16427=EDGE_LOOP('',(#66460,#66461,#66462,#66463));
#16428=EDGE_LOOP('',(#66464,#66465,#66466,#66467,#66468,#66469,#66470,#66471,
#66472,#66473,#66474,#66475,#66476,#66477,#66478,#66479,#66480,#66481));
#16429=EDGE_LOOP('',(#66482,#66483,#66484,#66485));
#16430=EDGE_LOOP('',(#66486,#66487,#66488,#66489));
#16431=EDGE_LOOP('',(#66490,#66491,#66492,#66493));
#16432=EDGE_LOOP('',(#66494,#66495,#66496,#66497,#66498,#66499,#66500,#66501,
#66502,#66503,#66504,#66505,#66506,#66507,#66508,#66509,#66510,#66511));
#16433=EDGE_LOOP('',(#66512,#66513,#66514,#66515));
#16434=EDGE_LOOP('',(#66516,#66517,#66518));
#16435=EDGE_LOOP('',(#66519,#66520,#66521,#66522,#66523));
#16436=EDGE_LOOP('',(#66524,#66525,#66526,#66527,#66528,#66529,#66530,#66531,
#66532,#66533,#66534,#66535,#66536,#66537,#66538,#66539));
#16437=EDGE_LOOP('',(#66540,#66541,#66542,#66543));
#16438=EDGE_LOOP('',(#66544,#66545,#66546,#66547));
#16439=EDGE_LOOP('',(#66548,#66549,#66550,#66551,#66552,#66553,#66554,#66555,
#66556,#66557,#66558,#66559,#66560,#66561,#66562,#66563));
#16440=EDGE_LOOP('',(#66564,#66565,#66566,#66567));
#16441=EDGE_LOOP('',(#66568,#66569,#66570,#66571));
#16442=EDGE_LOOP('',(#66572,#66573,#66574,#66575));
#16443=EDGE_LOOP('',(#66576,#66577,#66578,#66579,#66580,#66581,#66582,#66583,
#66584,#66585,#66586,#66587,#66588,#66589,#66590,#66591,#66592));
#16444=EDGE_LOOP('',(#66593,#66594,#66595,#66596));
#16445=EDGE_LOOP('',(#66597,#66598,#66599,#66600));
#16446=EDGE_LOOP('',(#66601,#66602,#66603,#66604,#66605));
#16447=EDGE_LOOP('',(#66606,#66607,#66608,#66609,#66610,#66611,#66612,#66613,
#66614,#66615,#66616,#66617,#66618,#66619));
#16448=EDGE_LOOP('',(#66620,#66621,#66622,#66623));
#16449=EDGE_LOOP('',(#66624,#66625,#66626,#66627));
#16450=EDGE_LOOP('',(#66628,#66629,#66630,#66631,#66632,#66633,#66634,#66635,
#66636,#66637,#66638,#66639,#66640,#66641));
#16451=EDGE_LOOP('',(#66642,#66643,#66644,#66645));
#16452=EDGE_LOOP('',(#66646,#66647,#66648,#66649));
#16453=EDGE_LOOP('',(#66650,#66651,#66652,#66653));
#16454=EDGE_LOOP('',(#66654,#66655,#66656,#66657));
#16455=EDGE_LOOP('',(#66658,#66659,#66660,#66661,#66662,#66663,#66664,#66665,
#66666,#66667,#66668,#66669,#66670));
#16456=EDGE_LOOP('',(#66671,#66672,#66673,#66674));
#16457=EDGE_LOOP('',(#66675,#66676,#66677,#66678));
#16458=EDGE_LOOP('',(#66679,#66680,#66681,#66682,#66683,#66684,#66685,#66686,
#66687,#66688,#66689,#66690));
#16459=EDGE_LOOP('',(#66691,#66692,#66693,#66694));
#16460=EDGE_LOOP('',(#66695,#66696,#66697,#66698));
#16461=EDGE_LOOP('',(#66699,#66700,#66701,#66702));
#16462=EDGE_LOOP('',(#66703,#66704,#66705,#66706));
#16463=EDGE_LOOP('',(#66707,#66708,#66709,#66710,#66711,#66712,#66713,#66714,
#66715,#66716,#66717,#66718));
#16464=EDGE_LOOP('',(#66719,#66720,#66721,#66722));
#16465=EDGE_LOOP('',(#66723,#66724,#66725,#66726));
#16466=EDGE_LOOP('',(#66727,#66728,#66729,#66730,#66731,#66732,#66733,#66734,
#66735,#66736,#66737,#66738));
#16467=EDGE_LOOP('',(#66739,#66740,#66741,#66742));
#16468=EDGE_LOOP('',(#66743,#66744,#66745,#66746));
#16469=EDGE_LOOP('',(#66747,#66748,#66749,#66750));
#16470=EDGE_LOOP('',(#66751,#66752,#66753,#66754));
#16471=EDGE_LOOP('',(#66755,#66756,#66757,#66758,#66759,#66760,#66761,#66762,
#66763,#66764,#66765,#66766));
#16472=EDGE_LOOP('',(#66767,#66768,#66769,#66770));
#16473=EDGE_LOOP('',(#66771,#66772,#66773,#66774));
#16474=EDGE_LOOP('',(#66775,#66776,#66777,#66778,#66779,#66780,#66781,#66782,
#66783,#66784,#66785,#66786));
#16475=EDGE_LOOP('',(#66787,#66788,#66789,#66790));
#16476=EDGE_LOOP('',(#66791,#66792,#66793,#66794));
#16477=EDGE_LOOP('',(#66795,#66796,#66797,#66798));
#16478=EDGE_LOOP('',(#66799,#66800,#66801,#66802));
#16479=EDGE_LOOP('',(#66803,#66804,#66805,#66806,#66807,#66808,#66809,#66810,
#66811,#66812,#66813,#66814));
#16480=EDGE_LOOP('',(#66815,#66816,#66817,#66818));
#16481=EDGE_LOOP('',(#66819,#66820,#66821,#66822));
#16482=EDGE_LOOP('',(#66823,#66824,#66825,#66826,#66827,#66828,#66829,#66830,
#66831,#66832,#66833,#66834,#66835));
#16483=EDGE_LOOP('',(#66836,#66837,#66838,#66839));
#16484=EDGE_LOOP('',(#66840,#66841,#66842,#66843));
#16485=EDGE_LOOP('',(#66844,#66845,#66846,#66847));
#16486=EDGE_LOOP('',(#66848,#66849,#66850,#66851));
#16487=EDGE_LOOP('',(#66852,#66853,#66854,#66855,#66856,#66857,#66858,#66859,
#66860,#66861,#66862,#66863,#66864,#66865));
#16488=EDGE_LOOP('',(#66866,#66867,#66868,#66869));
#16489=EDGE_LOOP('',(#66870,#66871,#66872,#66873));
#16490=EDGE_LOOP('',(#66874,#66875,#66876,#66877));
#16491=EDGE_LOOP('',(#66878,#66879,#66880,#66881,#66882,#66883,#66884,#66885,
#66886,#66887,#66888,#66889,#66890,#66891));
#16492=EDGE_LOOP('',(#66892,#66893,#66894,#66895,#66896));
#16493=EDGE_LOOP('',(#66897,#66898,#66899,#66900));
#16494=EDGE_LOOP('',(#66901,#66902,#66903,#66904,#66905));
#16495=EDGE_LOOP('',(#66906,#66907,#66908,#66909,#66910));
#16496=EDGE_LOOP('',(#66911,#66912,#66913,#66914));
#16497=EDGE_LOOP('',(#66915,#66916,#66917,#66918,#66919));
#16498=EDGE_LOOP('',(#66920,#66921,#66922,#66923,#66924,#66925,#66926));
#16499=EDGE_LOOP('',(#66927,#66928,#66929,#66930));
#16500=EDGE_LOOP('',(#66931,#66932,#66933,#66934));
#16501=EDGE_LOOP('',(#66935,#66936,#66937,#66938));
#16502=EDGE_LOOP('',(#66939,#66940,#66941,#66942,#66943,#66944,#66945));
#16503=EDGE_LOOP('',(#66946,#66947,#66948,#66949));
#16504=EDGE_LOOP('',(#66950,#66951,#66952,#66953));
#16505=EDGE_LOOP('',(#66954,#66955,#66956,#66957,#66958,#66959,#66960));
#16506=EDGE_LOOP('',(#66961,#66962,#66963,#66964));
#16507=EDGE_LOOP('',(#66965,#66966,#66967,#66968));
#16508=EDGE_LOOP('',(#66969,#66970,#66971,#66972));
#16509=EDGE_LOOP('',(#66973,#66974,#66975,#66976));
#16510=EDGE_LOOP('',(#66977,#66978,#66979,#66980,#66981,#66982,#66983,#66984,
#66985));
#16511=EDGE_LOOP('',(#66986,#66987,#66988,#66989));
#16512=EDGE_LOOP('',(#66990,#66991,#66992,#66993));
#16513=EDGE_LOOP('',(#66994,#66995,#66996,#66997));
#16514=EDGE_LOOP('',(#66998,#66999,#67000,#67001,#67002,#67003,#67004,#67005,
#67006,#67007));
#16515=EDGE_LOOP('',(#67008,#67009,#67010,#67011));
#16516=EDGE_LOOP('',(#67012,#67013,#67014,#67015));
#16517=EDGE_LOOP('',(#67016,#67017,#67018,#67019));
#16518=EDGE_LOOP('',(#67020,#67021,#67022,#67023,#67024,#67025,#67026,#67027,
#67028,#67029,#67030));
#16519=EDGE_LOOP('',(#67031,#67032,#67033,#67034));
#16520=EDGE_LOOP('',(#67035,#67036,#67037,#67038,#67039,#67040));
#16521=EDGE_LOOP('',(#67041,#67042,#67043,#67044));
#16522=EDGE_LOOP('',(#67045,#67046,#67047,#67048,#67049,#67050,#67051,#67052,
#67053,#67054,#67055,#67056,#67057,#67058));
#16523=EDGE_LOOP('',(#67059,#67060,#67061,#67062));
#16524=EDGE_LOOP('',(#67063,#67064,#67065,#67066));
#16525=EDGE_LOOP('',(#67067,#67068,#67069,#67070,#67071,#67072,#67073,#67074,
#67075,#67076,#67077,#67078,#67079,#67080));
#16526=EDGE_LOOP('',(#67081,#67082,#67083,#67084));
#16527=EDGE_LOOP('',(#67085,#67086,#67087,#67088));
#16528=EDGE_LOOP('',(#67089,#67090,#67091,#67092));
#16529=EDGE_LOOP('',(#67093,#67094,#67095,#67096));
#16530=EDGE_LOOP('',(#67097,#67098,#67099,#67100,#67101,#67102,#67103,#67104,
#67105,#67106,#67107,#67108,#67109,#67110));
#16531=EDGE_LOOP('',(#67111,#67112,#67113,#67114,#67115));
#16532=EDGE_LOOP('',(#67116,#67117,#67118,#67119));
#16533=EDGE_LOOP('',(#67120,#67121,#67122,#67123,#67124,#67125,#67126,#67127,
#67128,#67129,#67130,#67131));
#16534=EDGE_LOOP('',(#67132,#67133,#67134,#67135));
#16535=EDGE_LOOP('',(#67136,#67137,#67138,#67139));
#16536=EDGE_LOOP('',(#67140,#67141,#67142,#67143));
#16537=EDGE_LOOP('',(#67144,#67145,#67146,#67147));
#16538=EDGE_LOOP('',(#67148,#67149,#67150,#67151,#67152,#67153,#67154,#67155,
#67156,#67157,#67158,#67159));
#16539=EDGE_LOOP('',(#67160,#67161,#67162,#67163,#67164));
#16540=EDGE_LOOP('',(#67165,#67166,#67167,#67168));
#16541=EDGE_LOOP('',(#67169,#67170,#67171,#67172,#67173,#67174,#67175,#67176,
#67177,#67178,#67179,#67180));
#16542=EDGE_LOOP('',(#67181,#67182,#67183,#67184));
#16543=EDGE_LOOP('',(#67185,#67186,#67187,#67188));
#16544=EDGE_LOOP('',(#67189,#67190,#67191,#67192));
#16545=EDGE_LOOP('',(#67193,#67194,#67195,#67196));
#16546=EDGE_LOOP('',(#67197,#67198,#67199,#67200));
#16547=EDGE_LOOP('',(#67201,#67202,#67203,#67204));
#16548=EDGE_LOOP('',(#67205,#67206,#67207,#67208,#67209,#67210));
#16549=EDGE_LOOP('',(#67211,#67212,#67213,#67214));
#16550=EDGE_LOOP('',(#67215,#67216,#67217,#67218));
#16551=EDGE_LOOP('',(#67219,#67220,#67221,#67222));
#16552=EDGE_LOOP('',(#67223,#67224,#67225,#67226));
#16553=EDGE_LOOP('',(#67227,#67228,#67229,#67230));
#16554=EDGE_LOOP('',(#67231,#67232,#67233,#67234));
#16555=EDGE_LOOP('',(#67235,#67236,#67237,#67238));
#16556=EDGE_LOOP('',(#67239,#67240,#67241,#67242));
#16557=EDGE_LOOP('',(#67243,#67244,#67245,#67246));
#16558=EDGE_LOOP('',(#67247,#67248,#67249,#67250));
#16559=EDGE_LOOP('',(#67251,#67252,#67253,#67254));
#16560=EDGE_LOOP('',(#67255,#67256,#67257,#67258));
#16561=EDGE_LOOP('',(#67259,#67260,#67261,#67262));
#16562=EDGE_LOOP('',(#67263,#67264,#67265,#67266));
#16563=EDGE_LOOP('',(#67267,#67268,#67269,#67270));
#16564=EDGE_LOOP('',(#67271,#67272,#67273,#67274));
#16565=EDGE_LOOP('',(#67275,#67276,#67277,#67278));
#16566=EDGE_LOOP('',(#67279,#67280,#67281,#67282,#67283,#67284,#67285,#67286));
#16567=EDGE_LOOP('',(#67287,#67288,#67289,#67290,#67291,#67292,#67293,#67294));
#16568=EDGE_LOOP('',(#67295,#67296,#67297,#67298));
#16569=EDGE_LOOP('',(#67299,#67300,#67301,#67302));
#16570=EDGE_LOOP('',(#67303,#67304,#67305,#67306));
#16571=EDGE_LOOP('',(#67307,#67308,#67309,#67310));
#16572=EDGE_LOOP('',(#67311,#67312,#67313,#67314));
#16573=EDGE_LOOP('',(#67315,#67316,#67317,#67318));
#16574=EDGE_LOOP('',(#67319,#67320,#67321,#67322));
#16575=EDGE_LOOP('',(#67323,#67324,#67325,#67326));
#16576=EDGE_LOOP('',(#67327,#67328,#67329,#67330));
#16577=EDGE_LOOP('',(#67331,#67332,#67333,#67334));
#16578=EDGE_LOOP('',(#67335,#67336,#67337,#67338));
#16579=EDGE_LOOP('',(#67339,#67340,#67341,#67342));
#16580=EDGE_LOOP('',(#67343,#67344,#67345,#67346));
#16581=EDGE_LOOP('',(#67347,#67348,#67349,#67350));
#16582=EDGE_LOOP('',(#67351,#67352,#67353,#67354));
#16583=EDGE_LOOP('',(#67355,#67356,#67357,#67358));
#16584=EDGE_LOOP('',(#67359,#67360,#67361,#67362));
#16585=EDGE_LOOP('',(#67363,#67364,#67365,#67366));
#16586=EDGE_LOOP('',(#67367,#67368,#67369,#67370));
#16587=EDGE_LOOP('',(#67371,#67372,#67373,#67374,#67375,#67376,#67377,#67378,
#67379));
#16588=EDGE_LOOP('',(#67380,#67381,#67382,#67383));
#16589=EDGE_LOOP('',(#67384,#67385,#67386,#67387));
#16590=EDGE_LOOP('',(#67388,#67389,#67390,#67391));
#16591=EDGE_LOOP('',(#67392,#67393,#67394,#67395));
#16592=EDGE_LOOP('',(#67396,#67397,#67398,#67399));
#16593=EDGE_LOOP('',(#67400,#67401,#67402,#67403));
#16594=EDGE_LOOP('',(#67404,#67405,#67406,#67407));
#16595=EDGE_LOOP('',(#67408,#67409,#67410,#67411));
#16596=EDGE_LOOP('',(#67412,#67413,#67414,#67415));
#16597=EDGE_LOOP('',(#67416,#67417,#67418,#67419));
#16598=EDGE_LOOP('',(#67420,#67421,#67422,#67423));
#16599=EDGE_LOOP('',(#67424,#67425,#67426,#67427));
#16600=EDGE_LOOP('',(#67428,#67429,#67430,#67431));
#16601=EDGE_LOOP('',(#67432,#67433,#67434,#67435));
#16602=EDGE_LOOP('',(#67436,#67437,#67438,#67439,#67440));
#16603=EDGE_LOOP('',(#67441,#67442,#67443));
#16604=EDGE_LOOP('',(#67444,#67445,#67446,#67447));
#16605=EDGE_LOOP('',(#67448,#67449,#67450,#67451));
#16606=EDGE_LOOP('',(#67452,#67453,#67454,#67455));
#16607=EDGE_LOOP('',(#67456,#67457,#67458,#67459));
#16608=EDGE_LOOP('',(#67460,#67461,#67462,#67463));
#16609=EDGE_LOOP('',(#67464,#67465,#67466,#67467,#67468,#67469));
#16610=EDGE_LOOP('',(#67470,#67471,#67472,#67473));
#16611=EDGE_LOOP('',(#67474,#67475,#67476,#67477));
#16612=EDGE_LOOP('',(#67478,#67479,#67480,#67481));
#16613=EDGE_LOOP('',(#67482,#67483,#67484,#67485));
#16614=EDGE_LOOP('',(#67486,#67487,#67488,#67489));
#16615=EDGE_LOOP('',(#67490,#67491,#67492,#67493,#67494,#67495,#67496,#67497,
#67498));
#16616=EDGE_LOOP('',(#67499,#67500,#67501,#67502));
#16617=EDGE_LOOP('',(#67503,#67504,#67505,#67506));
#16618=EDGE_LOOP('',(#67507,#67508,#67509,#67510,#67511));
#16619=EDGE_LOOP('',(#67512,#67513,#67514,#67515));
#16620=EDGE_LOOP('',(#67516,#67517,#67518,#67519));
#16621=EDGE_LOOP('',(#67520,#67521,#67522,#67523,#67524));
#16622=EDGE_LOOP('',(#67525,#67526,#67527,#67528,#67529));
#16623=EDGE_LOOP('',(#67530,#67531,#67532,#67533,#67534,#67535,#67536,#67537,
#67538));
#16624=EDGE_LOOP('',(#67539,#67540,#67541,#67542,#67543,#67544,#67545,#67546,
#67547,#67548,#67549,#67550));
#16625=EDGE_LOOP('',(#67551,#67552,#67553,#67554));
#16626=EDGE_LOOP('',(#67555,#67556,#67557,#67558,#67559,#67560));
#16627=EDGE_LOOP('',(#67561,#67562,#67563,#67564,#67565));
#16628=EDGE_LOOP('',(#67566,#67567,#67568,#67569));
#16629=EDGE_LOOP('',(#67570,#67571,#67572,#67573));
#16630=EDGE_LOOP('',(#67574,#67575,#67576,#67577));
#16631=EDGE_LOOP('',(#67578,#67579,#67580,#67581));
#16632=EDGE_LOOP('',(#67582,#67583,#67584,#67585));
#16633=EDGE_LOOP('',(#67586,#67587,#67588,#67589));
#16634=EDGE_LOOP('',(#67590,#67591,#67592,#67593));
#16635=EDGE_LOOP('',(#67594,#67595,#67596,#67597));
#16636=EDGE_LOOP('',(#67598,#67599,#67600,#67601));
#16637=EDGE_LOOP('',(#67602,#67603,#67604,#67605));
#16638=EDGE_LOOP('',(#67606,#67607,#67608,#67609));
#16639=EDGE_LOOP('',(#67610,#67611,#67612,#67613));
#16640=EDGE_LOOP('',(#67614,#67615,#67616,#67617));
#16641=EDGE_LOOP('',(#67618,#67619,#67620,#67621));
#16642=EDGE_LOOP('',(#67622,#67623,#67624,#67625));
#16643=EDGE_LOOP('',(#67626,#67627,#67628,#67629));
#16644=EDGE_LOOP('',(#67630,#67631,#67632,#67633));
#16645=EDGE_LOOP('',(#67634,#67635,#67636,#67637));
#16646=EDGE_LOOP('',(#67638,#67639,#67640,#67641));
#16647=EDGE_LOOP('',(#67642,#67643,#67644,#67645,#67646));
#16648=EDGE_LOOP('',(#67647,#67648,#67649,#67650));
#16649=EDGE_LOOP('',(#67651,#67652,#67653,#67654));
#16650=EDGE_LOOP('',(#67655,#67656,#67657,#67658));
#16651=EDGE_LOOP('',(#67659,#67660,#67661,#67662));
#16652=EDGE_LOOP('',(#67663,#67664,#67665,#67666));
#16653=EDGE_LOOP('',(#67667,#67668,#67669,#67670));
#16654=EDGE_LOOP('',(#67671,#67672,#67673,#67674));
#16655=EDGE_LOOP('',(#67675,#67676,#67677,#67678));
#16656=EDGE_LOOP('',(#67679,#67680,#67681,#67682));
#16657=EDGE_LOOP('',(#67683,#67684,#67685,#67686));
#16658=EDGE_LOOP('',(#67687,#67688,#67689,#67690));
#16659=EDGE_LOOP('',(#67691,#67692,#67693,#67694));
#16660=EDGE_LOOP('',(#67695,#67696,#67697,#67698));
#16661=EDGE_LOOP('',(#67699,#67700,#67701,#67702));
#16662=EDGE_LOOP('',(#67703,#67704,#67705,#67706));
#16663=EDGE_LOOP('',(#67707,#67708,#67709,#67710));
#16664=EDGE_LOOP('',(#67711,#67712,#67713,#67714));
#16665=EDGE_LOOP('',(#67715,#67716,#67717,#67718));
#16666=EDGE_LOOP('',(#67719,#67720,#67721,#67722));
#16667=EDGE_LOOP('',(#67723,#67724,#67725,#67726));
#16668=EDGE_LOOP('',(#67727,#67728,#67729,#67730));
#16669=EDGE_LOOP('',(#67731,#67732,#67733,#67734));
#16670=EDGE_LOOP('',(#67735,#67736,#67737,#67738));
#16671=EDGE_LOOP('',(#67739,#67740,#67741,#67742));
#16672=EDGE_LOOP('',(#67743,#67744,#67745,#67746));
#16673=EDGE_LOOP('',(#67747,#67748,#67749,#67750));
#16674=EDGE_LOOP('',(#67751,#67752,#67753,#67754));
#16675=EDGE_LOOP('',(#67755,#67756,#67757,#67758));
#16676=EDGE_LOOP('',(#67759,#67760,#67761,#67762));
#16677=EDGE_LOOP('',(#67763,#67764,#67765,#67766));
#16678=EDGE_LOOP('',(#67767,#67768,#67769,#67770));
#16679=EDGE_LOOP('',(#67771,#67772,#67773,#67774));
#16680=EDGE_LOOP('',(#67775,#67776,#67777,#67778));
#16681=EDGE_LOOP('',(#67779,#67780,#67781,#67782));
#16682=EDGE_LOOP('',(#67783,#67784,#67785,#67786));
#16683=EDGE_LOOP('',(#67787,#67788,#67789,#67790));
#16684=EDGE_LOOP('',(#67791,#67792,#67793,#67794));
#16685=EDGE_LOOP('',(#67795,#67796,#67797,#67798));
#16686=EDGE_LOOP('',(#67799,#67800,#67801,#67802));
#16687=EDGE_LOOP('',(#67803,#67804,#67805,#67806));
#16688=EDGE_LOOP('',(#67807,#67808,#67809,#67810));
#16689=EDGE_LOOP('',(#67811,#67812,#67813,#67814));
#16690=EDGE_LOOP('',(#67815,#67816,#67817,#67818));
#16691=EDGE_LOOP('',(#67819,#67820,#67821,#67822));
#16692=EDGE_LOOP('',(#67823,#67824,#67825,#67826));
#16693=EDGE_LOOP('',(#67827,#67828,#67829,#67830));
#16694=EDGE_LOOP('',(#67831,#67832,#67833,#67834));
#16695=EDGE_LOOP('',(#67835,#67836,#67837,#67838));
#16696=EDGE_LOOP('',(#67839,#67840,#67841,#67842));
#16697=EDGE_LOOP('',(#67843,#67844,#67845,#67846));
#16698=EDGE_LOOP('',(#67847,#67848,#67849,#67850));
#16699=EDGE_LOOP('',(#67851,#67852,#67853,#67854));
#16700=EDGE_LOOP('',(#67855,#67856,#67857,#67858));
#16701=EDGE_LOOP('',(#67859,#67860,#67861,#67862));
#16702=EDGE_LOOP('',(#67863,#67864,#67865,#67866));
#16703=EDGE_LOOP('',(#67867,#67868,#67869,#67870));
#16704=EDGE_LOOP('',(#67871,#67872,#67873,#67874));
#16705=EDGE_LOOP('',(#67875,#67876,#67877,#67878));
#16706=EDGE_LOOP('',(#67879,#67880,#67881,#67882));
#16707=EDGE_LOOP('',(#67883,#67884,#67885,#67886));
#16708=EDGE_LOOP('',(#67887,#67888,#67889,#67890));
#16709=EDGE_LOOP('',(#67891,#67892,#67893,#67894));
#16710=EDGE_LOOP('',(#67895,#67896,#67897,#67898));
#16711=EDGE_LOOP('',(#67899,#67900,#67901,#67902));
#16712=EDGE_LOOP('',(#67903,#67904,#67905,#67906));
#16713=EDGE_LOOP('',(#67907,#67908,#67909,#67910));
#16714=EDGE_LOOP('',(#67911,#67912,#67913,#67914));
#16715=EDGE_LOOP('',(#67915,#67916,#67917,#67918));
#16716=EDGE_LOOP('',(#67919,#67920,#67921,#67922));
#16717=EDGE_LOOP('',(#67923,#67924,#67925,#67926));
#16718=EDGE_LOOP('',(#67927,#67928,#67929,#67930));
#16719=EDGE_LOOP('',(#67931,#67932,#67933,#67934));
#16720=EDGE_LOOP('',(#67935,#67936,#67937,#67938));
#16721=EDGE_LOOP('',(#67939,#67940,#67941,#67942));
#16722=EDGE_LOOP('',(#67943,#67944,#67945,#67946));
#16723=EDGE_LOOP('',(#67947,#67948,#67949,#67950));
#16724=EDGE_LOOP('',(#67951,#67952,#67953,#67954,#67955,#67956,#67957,#67958,
#67959,#67960,#67961,#67962,#67963,#67964,#67965,#67966));
#16725=EDGE_LOOP('',(#67967,#67968,#67969,#67970));
#16726=EDGE_LOOP('',(#67971,#67972,#67973,#67974));
#16727=EDGE_LOOP('',(#67975,#67976,#67977,#67978));
#16728=EDGE_LOOP('',(#67979,#67980,#67981,#67982));
#16729=EDGE_LOOP('',(#67983,#67984,#67985,#67986,#67987,#67988,#67989,#67990,
#67991,#67992,#67993,#67994,#67995,#67996,#67997,#67998,#67999,#68000,#68001));
#16730=EDGE_LOOP('',(#68002,#68003,#68004,#68005));
#16731=EDGE_LOOP('',(#68006,#68007,#68008,#68009));
#16732=EDGE_LOOP('',(#68010,#68011,#68012,#68013));
#16733=EDGE_LOOP('',(#68014,#68015,#68016,#68017));
#16734=EDGE_LOOP('',(#68018,#68019,#68020,#68021,#68022,#68023,#68024,#68025,
#68026,#68027,#68028,#68029,#68030,#68031,#68032,#68033,#68034,#68035,#68036,
#68037,#68038,#68039,#68040,#68041,#68042,#68043,#68044,#68045,#68046,#68047,
#68048,#68049,#68050,#68051,#68052,#68053,#68054,#68055));
#16735=EDGE_LOOP('',(#68056,#68057,#68058,#68059,#68060,#68061));
#16736=EDGE_LOOP('',(#68062,#68063,#68064,#68065));
#16737=EDGE_LOOP('',(#68066,#68067,#68068,#68069));
#16738=EDGE_LOOP('',(#68070,#68071,#68072,#68073));
#16739=EDGE_LOOP('',(#68074,#68075,#68076,#68077));
#16740=EDGE_LOOP('',(#68078,#68079,#68080,#68081));
#16741=EDGE_LOOP('',(#68082,#68083,#68084,#68085));
#16742=EDGE_LOOP('',(#68086,#68087,#68088,#68089));
#16743=EDGE_LOOP('',(#68090,#68091,#68092,#68093));
#16744=EDGE_LOOP('',(#68094,#68095,#68096,#68097));
#16745=EDGE_LOOP('',(#68098,#68099,#68100,#68101));
#16746=EDGE_LOOP('',(#68102,#68103,#68104,#68105));
#16747=EDGE_LOOP('',(#68106,#68107,#68108,#68109));
#16748=EDGE_LOOP('',(#68110,#68111,#68112,#68113));
#16749=EDGE_LOOP('',(#68114,#68115,#68116,#68117));
#16750=EDGE_LOOP('',(#68118,#68119,#68120,#68121));
#16751=EDGE_LOOP('',(#68122,#68123,#68124,#68125));
#16752=EDGE_LOOP('',(#68126,#68127,#68128,#68129));
#16753=EDGE_LOOP('',(#68130,#68131,#68132,#68133));
#16754=EDGE_LOOP('',(#68134,#68135,#68136,#68137));
#16755=EDGE_LOOP('',(#68138,#68139,#68140,#68141));
#16756=EDGE_LOOP('',(#68142,#68143,#68144,#68145));
#16757=EDGE_LOOP('',(#68146,#68147,#68148,#68149));
#16758=EDGE_LOOP('',(#68150,#68151,#68152,#68153));
#16759=EDGE_LOOP('',(#68154,#68155,#68156,#68157));
#16760=EDGE_LOOP('',(#68158,#68159,#68160,#68161));
#16761=EDGE_LOOP('',(#68162,#68163,#68164,#68165));
#16762=EDGE_LOOP('',(#68166,#68167,#68168,#68169));
#16763=EDGE_LOOP('',(#68170,#68171,#68172,#68173));
#16764=EDGE_LOOP('',(#68174,#68175,#68176,#68177));
#16765=EDGE_LOOP('',(#68178,#68179,#68180,#68181));
#16766=EDGE_LOOP('',(#68182,#68183,#68184,#68185,#68186));
#16767=EDGE_LOOP('',(#68187,#68188,#68189,#68190));
#16768=EDGE_LOOP('',(#68191,#68192,#68193,#68194));
#16769=EDGE_LOOP('',(#68195,#68196,#68197,#68198));
#16770=EDGE_LOOP('',(#68199,#68200,#68201,#68202));
#16771=EDGE_LOOP('',(#68203,#68204,#68205,#68206,#68207));
#16772=EDGE_LOOP('',(#68208,#68209,#68210,#68211,#68212,#68213));
#16773=EDGE_LOOP('',(#68214,#68215,#68216,#68217));
#16774=EDGE_LOOP('',(#68218,#68219,#68220,#68221));
#16775=EDGE_LOOP('',(#68222,#68223,#68224,#68225));
#16776=EDGE_LOOP('',(#68226,#68227,#68228,#68229,#68230,#68231,#68232,#68233,
#68234,#68235,#68236,#68237,#68238,#68239,#68240,#68241,#68242,#68243,#68244,
#68245,#68246,#68247,#68248,#68249,#68250,#68251,#68252,#68253,#68254,#68255,
#68256,#68257,#68258,#68259,#68260,#68261,#68262,#68263,#68264,#68265));
#16777=EDGE_LOOP('',(#68266,#68267,#68268,#68269,#68270,#68271,#68272,#68273,
#68274,#68275,#68276,#68277,#68278,#68279,#68280,#68281,#68282,#68283,#68284));
#16778=EDGE_LOOP('',(#68285,#68286,#68287,#68288));
#16779=EDGE_LOOP('',(#68289,#68290,#68291,#68292));
#16780=EDGE_LOOP('',(#68293,#68294,#68295,#68296));
#16781=EDGE_LOOP('',(#68297,#68298,#68299,#68300));
#16782=EDGE_LOOP('',(#68301,#68302,#68303,#68304,#68305,#68306,#68307,#68308,
#68309,#68310,#68311,#68312,#68313,#68314,#68315,#68316,#68317,#68318,#68319));
#16783=EDGE_LOOP('',(#68320,#68321,#68322,#68323));
#16784=EDGE_LOOP('',(#68324,#68325,#68326,#68327));
#16785=EDGE_LOOP('',(#68328,#68329,#68330,#68331));
#16786=EDGE_LOOP('',(#68332,#68333,#68334,#68335,#68336));
#16787=EDGE_LOOP('',(#68337,#68338,#68339,#68340));
#16788=EDGE_LOOP('',(#68341,#68342,#68343,#68344));
#16789=EDGE_LOOP('',(#68345,#68346,#68347,#68348));
#16790=EDGE_LOOP('',(#68349,#68350,#68351,#68352));
#16791=EDGE_LOOP('',(#68353,#68354,#68355,#68356));
#16792=EDGE_LOOP('',(#68357,#68358,#68359,#68360,#68361,#68362,#68363,#68364,
#68365,#68366,#68367,#68368,#68369,#68370,#68371,#68372,#68373,#68374,#68375,
#68376,#68377,#68378,#68379,#68380,#68381,#68382,#68383,#68384,#68385,#68386,
#68387,#68388,#68389,#68390,#68391,#68392,#68393,#68394,#68395,#68396,#68397,
#68398));
#16793=EDGE_LOOP('',(#68399,#68400,#68401,#68402));
#16794=EDGE_LOOP('',(#68403,#68404,#68405,#68406,#68407,#68408,#68409,#68410,
#68411,#68412,#68413,#68414,#68415,#68416,#68417,#68418,#68419,#68420,#68421,
#68422,#68423,#68424,#68425,#68426,#68427,#68428,#68429,#68430,#68431,#68432,
#68433,#68434));
#16795=EDGE_LOOP('',(#68435));
#16796=EDGE_LOOP('',(#68436));
#16797=EDGE_LOOP('',(#68437));
#16798=EDGE_LOOP('',(#68438));
#16799=EDGE_LOOP('',(#68439,#68440,#68441,#68442));
#16800=EDGE_LOOP('',(#68443,#68444,#68445,#68446));
#16801=EDGE_LOOP('',(#68447,#68448,#68449,#68450));
#16802=EDGE_LOOP('',(#68451,#68452,#68453,#68454,#68455,#68456,#68457,#68458));
#16803=EDGE_LOOP('',(#68459,#68460,#68461,#68462,#68463,#68464,#68465,#68466));
#16804=EDGE_LOOP('',(#68467,#68468,#68469,#68470,#68471,#68472,#68473,#68474,
#68475,#68476,#68477,#68478,#68479,#68480,#68481,#68482,#68483,#68484,#68485,
#68486,#68487,#68488,#68489,#68490,#68491,#68492,#68493,#68494,#68495,#68496,
#68497,#68498,#68499,#68500,#68501,#68502,#68503,#68504,#68505,#68506,#68507,
#68508,#68509,#68510,#68511,#68512,#68513,#68514,#68515,#68516,#68517,#68518,
#68519,#68520,#68521,#68522,#68523,#68524,#68525,#68526,#68527,#68528));
#16805=EDGE_LOOP('',(#68529,#68530,#68531,#68532,#68533,#68534));
#16806=EDGE_LOOP('',(#68535,#68536,#68537,#68538));
#16807=EDGE_LOOP('',(#68539,#68540,#68541,#68542));
#16808=EDGE_LOOP('',(#68543,#68544,#68545,#68546,#68547,#68548,#68549,#68550,
#68551,#68552,#68553,#68554,#68555,#68556,#68557,#68558,#68559,#68560,#68561,
#68562,#68563,#68564,#68565,#68566,#68567,#68568,#68569,#68570,#68571,#68572,
#68573,#68574,#68575,#68576,#68577,#68578,#68579,#68580,#68581,#68582));
#16809=EDGE_LOOP('',(#68583,#68584,#68585,#68586,#68587,#68588));
#16810=EDGE_LOOP('',(#68589,#68590,#68591,#68592,#68593,#68594,#68595,#68596,
#68597,#68598,#68599,#68600,#68601,#68602,#68603,#68604,#68605,#68606,#68607,
#68608,#68609,#68610,#68611,#68612,#68613,#68614,#68615,#68616,#68617,#68618,
#68619,#68620));
#16811=EDGE_LOOP('',(#68621));
#16812=EDGE_LOOP('',(#68622));
#16813=EDGE_LOOP('',(#68623));
#16814=EDGE_LOOP('',(#68624));
#16815=EDGE_LOOP('',(#68625,#68626,#68627,#68628));
#16816=EDGE_LOOP('',(#68629,#68630,#68631,#68632));
#16817=EDGE_LOOP('',(#68633,#68634,#68635,#68636));
#16818=EDGE_LOOP('',(#68637,#68638,#68639,#68640));
#16819=EDGE_LOOP('',(#68641,#68642,#68643,#68644));
#16820=EDGE_LOOP('',(#68645,#68646,#68647,#68648));
#16821=EDGE_LOOP('',(#68649,#68650,#68651,#68652,#68653,#68654,#68655,#68656));
#16822=EDGE_LOOP('',(#68657,#68658));
#16823=EDGE_LOOP('',(#68659,#68660));
#16824=EDGE_LOOP('',(#68661,#68662));
#16825=EDGE_LOOP('',(#68663,#68664));
#16826=EDGE_LOOP('',(#68665,#68666));
#16827=EDGE_LOOP('',(#68667,#68668));
#16828=EDGE_LOOP('',(#68669,#68670,#68671,#68672,#68673));
#16829=EDGE_LOOP('',(#68674));
#16830=EDGE_LOOP('',(#68675));
#16831=EDGE_LOOP('',(#68676,#68677,#68678,#68679,#68680,#68681));
#16832=EDGE_LOOP('',(#68682,#68683,#68684,#68685,#68686));
#16833=EDGE_LOOP('',(#68687,#68688,#68689,#68690));
#16834=EDGE_LOOP('',(#68691));
#16835=EDGE_LOOP('',(#68692,#68693,#68694,#68695));
#16836=EDGE_LOOP('',(#68696));
#16837=EDGE_LOOP('',(#68697));
#16838=EDGE_LOOP('',(#68698,#68699,#68700,#68701));
#16839=EDGE_LOOP('',(#68702));
#16840=EDGE_LOOP('',(#68703,#68704,#68705,#68706));
#16841=EDGE_LOOP('',(#68707,#68708,#68709,#68710,#68711));
#16842=EDGE_LOOP('',(#68712,#68713,#68714,#68715));
#16843=EDGE_LOOP('',(#68716,#68717,#68718,#68719));
#16844=EDGE_LOOP('',(#68720,#68721,#68722));
#16845=EDGE_LOOP('',(#68723,#68724,#68725,#68726));
#16846=EDGE_LOOP('',(#68727,#68728,#68729,#68730));
#16847=EDGE_LOOP('',(#68731,#68732,#68733,#68734));
#16848=EDGE_LOOP('',(#68735,#68736,#68737,#68738));
#16849=EDGE_LOOP('',(#68739,#68740,#68741,#68742));
#16850=EDGE_LOOP('',(#68743,#68744,#68745,#68746));
#16851=EDGE_LOOP('',(#68747,#68748,#68749,#68750));
#16852=EDGE_LOOP('',(#68751,#68752,#68753,#68754));
#16853=EDGE_LOOP('',(#68755,#68756,#68757,#68758,#68759));
#16854=EDGE_LOOP('',(#68760,#68761,#68762));
#16855=EDGE_LOOP('',(#68763,#68764,#68765,#68766));
#16856=EDGE_LOOP('',(#68767,#68768,#68769,#68770));
#16857=EDGE_LOOP('',(#68771,#68772,#68773,#68774));
#16858=EDGE_LOOP('',(#68775,#68776,#68777,#68778));
#16859=EDGE_LOOP('',(#68779,#68780,#68781,#68782));
#16860=EDGE_LOOP('',(#68783,#68784,#68785));
#16861=EDGE_LOOP('',(#68786,#68787,#68788,#68789));
#16862=EDGE_LOOP('',(#68790,#68791,#68792,#68793));
#16863=EDGE_LOOP('',(#68794,#68795,#68796,#68797));
#16864=EDGE_LOOP('',(#68798,#68799,#68800,#68801));
#16865=EDGE_LOOP('',(#68802,#68803,#68804));
#16866=EDGE_LOOP('',(#68805,#68806,#68807,#68808));
#16867=EDGE_LOOP('',(#68809,#68810,#68811,#68812));
#16868=EDGE_LOOP('',(#68813,#68814,#68815,#68816));
#16869=EDGE_LOOP('',(#68817,#68818,#68819,#68820));
#16870=EDGE_LOOP('',(#68821,#68822,#68823,#68824));
#16871=EDGE_LOOP('',(#68825,#68826,#68827,#68828));
#16872=EDGE_LOOP('',(#68829,#68830,#68831,#68832));
#16873=EDGE_LOOP('',(#68833,#68834,#68835,#68836));
#16874=EDGE_LOOP('',(#68837,#68838,#68839,#68840));
#16875=EDGE_LOOP('',(#68841,#68842,#68843,#68844));
#16876=EDGE_LOOP('',(#68845,#68846,#68847,#68848));
#16877=EDGE_LOOP('',(#68849,#68850,#68851,#68852));
#16878=EDGE_LOOP('',(#68853,#68854,#68855,#68856));
#16879=EDGE_LOOP('',(#68857,#68858,#68859,#68860));
#16880=EDGE_LOOP('',(#68861,#68862,#68863,#68864));
#16881=EDGE_LOOP('',(#68865,#68866,#68867,#68868));
#16882=EDGE_LOOP('',(#68869,#68870,#68871,#68872));
#16883=EDGE_LOOP('',(#68873,#68874,#68875,#68876));
#16884=EDGE_LOOP('',(#68877,#68878,#68879,#68880));
#16885=EDGE_LOOP('',(#68881,#68882,#68883,#68884));
#16886=EDGE_LOOP('',(#68885,#68886,#68887,#68888));
#16887=EDGE_LOOP('',(#68889,#68890,#68891,#68892));
#16888=EDGE_LOOP('',(#68893,#68894,#68895,#68896));
#16889=EDGE_LOOP('',(#68897,#68898,#68899,#68900));
#16890=EDGE_LOOP('',(#68901,#68902,#68903,#68904));
#16891=EDGE_LOOP('',(#68905,#68906,#68907,#68908));
#16892=EDGE_LOOP('',(#68909,#68910,#68911,#68912));
#16893=EDGE_LOOP('',(#68913,#68914,#68915,#68916));
#16894=EDGE_LOOP('',(#68917,#68918,#68919,#68920,#68921));
#16895=EDGE_LOOP('',(#68922,#68923,#68924,#68925));
#16896=EDGE_LOOP('',(#68926,#68927,#68928,#68929));
#16897=EDGE_LOOP('',(#68930,#68931,#68932,#68933));
#16898=EDGE_LOOP('',(#68934,#68935,#68936,#68937));
#16899=EDGE_LOOP('',(#68938,#68939,#68940,#68941));
#16900=EDGE_LOOP('',(#68942,#68943,#68944,#68945));
#16901=EDGE_LOOP('',(#68946,#68947,#68948,#68949));
#16902=EDGE_LOOP('',(#68950,#68951,#68952,#68953,#68954,#68955));
#16903=EDGE_LOOP('',(#68956,#68957,#68958,#68959));
#16904=EDGE_LOOP('',(#68960,#68961,#68962,#68963));
#16905=EDGE_LOOP('',(#68964,#68965,#68966,#68967,#68968));
#16906=EDGE_LOOP('',(#68969,#68970,#68971,#68972));
#16907=EDGE_LOOP('',(#68973,#68974,#68975,#68976));
#16908=EDGE_LOOP('',(#68977,#68978,#68979,#68980));
#16909=EDGE_LOOP('',(#68981,#68982,#68983,#68984,#68985));
#16910=EDGE_LOOP('',(#68986,#68987,#68988,#68989));
#16911=EDGE_LOOP('',(#68990,#68991,#68992,#68993));
#16912=EDGE_LOOP('',(#68994,#68995,#68996,#68997));
#16913=EDGE_LOOP('',(#68998,#68999,#69000,#69001));
#16914=EDGE_LOOP('',(#69002,#69003,#69004,#69005,#69006));
#16915=EDGE_LOOP('',(#69007,#69008,#69009,#69010));
#16916=EDGE_LOOP('',(#69011,#69012,#69013,#69014));
#16917=EDGE_LOOP('',(#69015,#69016,#69017,#69018));
#16918=EDGE_LOOP('',(#69019,#69020,#69021,#69022));
#16919=EDGE_LOOP('',(#69023,#69024,#69025,#69026));
#16920=EDGE_LOOP('',(#69027,#69028,#69029,#69030,#69031));
#16921=EDGE_LOOP('',(#69032,#69033,#69034,#69035,#69036,#69037));
#16922=EDGE_LOOP('',(#69038,#69039,#69040,#69041,#69042,#69043));
#16923=EDGE_LOOP('',(#69044,#69045,#69046,#69047,#69048,#69049));
#16924=EDGE_LOOP('',(#69050,#69051,#69052,#69053,#69054));
#16925=EDGE_LOOP('',(#69055,#69056,#69057,#69058,#69059,#69060,#69061));
#16926=EDGE_LOOP('',(#69062,#69063,#69064,#69065,#69066));
#16927=EDGE_LOOP('',(#69067,#69068,#69069,#69070,#69071));
#16928=EDGE_LOOP('',(#69072,#69073,#69074,#69075));
#16929=EDGE_LOOP('',(#69076,#69077,#69078,#69079));
#16930=EDGE_LOOP('',(#69080,#69081,#69082,#69083));
#16931=EDGE_LOOP('',(#69084,#69085,#69086,#69087));
#16932=EDGE_LOOP('',(#69088,#69089,#69090,#69091));
#16933=EDGE_LOOP('',(#69092,#69093,#69094,#69095));
#16934=EDGE_LOOP('',(#69096,#69097,#69098,#69099));
#16935=EDGE_LOOP('',(#69100,#69101,#69102,#69103));
#16936=EDGE_LOOP('',(#69104,#69105,#69106,#69107));
#16937=EDGE_LOOP('',(#69108,#69109,#69110,#69111));
#16938=EDGE_LOOP('',(#69112,#69113,#69114,#69115));
#16939=EDGE_LOOP('',(#69116,#69117,#69118,#69119));
#16940=EDGE_LOOP('',(#69120,#69121,#69122,#69123));
#16941=EDGE_LOOP('',(#69124,#69125,#69126,#69127));
#16942=EDGE_LOOP('',(#69128,#69129,#69130,#69131));
#16943=EDGE_LOOP('',(#69132,#69133,#69134,#69135));
#16944=EDGE_LOOP('',(#69136,#69137,#69138,#69139));
#16945=EDGE_LOOP('',(#69140,#69141,#69142,#69143));
#16946=EDGE_LOOP('',(#69144,#69145,#69146,#69147));
#16947=EDGE_LOOP('',(#69148,#69149,#69150,#69151));
#16948=EDGE_LOOP('',(#69152,#69153,#69154,#69155));
#16949=EDGE_LOOP('',(#69156,#69157,#69158,#69159));
#16950=EDGE_LOOP('',(#69160,#69161,#69162,#69163));
#16951=EDGE_LOOP('',(#69164,#69165,#69166,#69167));
#16952=EDGE_LOOP('',(#69168,#69169,#69170,#69171));
#16953=EDGE_LOOP('',(#69172,#69173,#69174,#69175));
#16954=EDGE_LOOP('',(#69176,#69177,#69178,#69179));
#16955=EDGE_LOOP('',(#69180,#69181,#69182,#69183));
#16956=EDGE_LOOP('',(#69184,#69185,#69186,#69187));
#16957=EDGE_LOOP('',(#69188,#69189,#69190,#69191));
#16958=EDGE_LOOP('',(#69192,#69193,#69194,#69195));
#16959=EDGE_LOOP('',(#69196,#69197,#69198,#69199));
#16960=EDGE_LOOP('',(#69200,#69201,#69202,#69203));
#16961=EDGE_LOOP('',(#69204,#69205,#69206,#69207));
#16962=EDGE_LOOP('',(#69208,#69209,#69210,#69211));
#16963=EDGE_LOOP('',(#69212,#69213,#69214,#69215));
#16964=EDGE_LOOP('',(#69216,#69217,#69218,#69219));
#16965=EDGE_LOOP('',(#69220,#69221,#69222,#69223));
#16966=EDGE_LOOP('',(#69224,#69225,#69226,#69227));
#16967=EDGE_LOOP('',(#69228,#69229,#69230,#69231));
#16968=EDGE_LOOP('',(#69232,#69233,#69234,#69235));
#16969=EDGE_LOOP('',(#69236,#69237,#69238,#69239));
#16970=EDGE_LOOP('',(#69240,#69241,#69242,#69243));
#16971=EDGE_LOOP('',(#69244,#69245,#69246,#69247));
#16972=EDGE_LOOP('',(#69248,#69249,#69250,#69251));
#16973=EDGE_LOOP('',(#69252,#69253,#69254,#69255));
#16974=EDGE_LOOP('',(#69256,#69257,#69258,#69259));
#16975=EDGE_LOOP('',(#69260,#69261,#69262,#69263));
#16976=EDGE_LOOP('',(#69264,#69265,#69266,#69267));
#16977=EDGE_LOOP('',(#69268,#69269,#69270,#69271));
#16978=EDGE_LOOP('',(#69272,#69273,#69274,#69275));
#16979=EDGE_LOOP('',(#69276,#69277,#69278,#69279));
#16980=EDGE_LOOP('',(#69280,#69281,#69282,#69283));
#16981=EDGE_LOOP('',(#69284,#69285,#69286,#69287));
#16982=EDGE_LOOP('',(#69288,#69289,#69290,#69291));
#16983=EDGE_LOOP('',(#69292,#69293,#69294,#69295));
#16984=EDGE_LOOP('',(#69296,#69297,#69298,#69299));
#16985=EDGE_LOOP('',(#69300,#69301,#69302,#69303));
#16986=EDGE_LOOP('',(#69304,#69305,#69306,#69307));
#16987=EDGE_LOOP('',(#69308,#69309,#69310,#69311));
#16988=EDGE_LOOP('',(#69312,#69313,#69314,#69315));
#16989=EDGE_LOOP('',(#69316,#69317,#69318,#69319));
#16990=EDGE_LOOP('',(#69320,#69321,#69322,#69323));
#16991=EDGE_LOOP('',(#69324,#69325,#69326,#69327));
#16992=EDGE_LOOP('',(#69328,#69329,#69330,#69331));
#16993=EDGE_LOOP('',(#69332,#69333,#69334,#69335));
#16994=EDGE_LOOP('',(#69336,#69337,#69338,#69339));
#16995=EDGE_LOOP('',(#69340,#69341,#69342,#69343));
#16996=EDGE_LOOP('',(#69344,#69345,#69346,#69347));
#16997=EDGE_LOOP('',(#69348,#69349,#69350,#69351));
#16998=EDGE_LOOP('',(#69352,#69353,#69354,#69355));
#16999=EDGE_LOOP('',(#69356,#69357,#69358,#69359));
#17000=EDGE_LOOP('',(#69360,#69361,#69362,#69363));
#17001=EDGE_LOOP('',(#69364,#69365,#69366,#69367));
#17002=EDGE_LOOP('',(#69368,#69369,#69370,#69371));
#17003=EDGE_LOOP('',(#69372,#69373,#69374,#69375));
#17004=EDGE_LOOP('',(#69376,#69377,#69378,#69379));
#17005=EDGE_LOOP('',(#69380,#69381,#69382,#69383));
#17006=EDGE_LOOP('',(#69384,#69385,#69386,#69387));
#17007=EDGE_LOOP('',(#69388,#69389,#69390,#69391));
#17008=EDGE_LOOP('',(#69392,#69393,#69394,#69395));
#17009=EDGE_LOOP('',(#69396,#69397,#69398,#69399));
#17010=EDGE_LOOP('',(#69400,#69401,#69402,#69403));
#17011=EDGE_LOOP('',(#69404,#69405,#69406,#69407));
#17012=EDGE_LOOP('',(#69408,#69409,#69410,#69411));
#17013=EDGE_LOOP('',(#69412,#69413,#69414,#69415));
#17014=EDGE_LOOP('',(#69416,#69417,#69418,#69419));
#17015=EDGE_LOOP('',(#69420,#69421,#69422,#69423));
#17016=EDGE_LOOP('',(#69424,#69425,#69426,#69427));
#17017=EDGE_LOOP('',(#69428,#69429,#69430,#69431));
#17018=EDGE_LOOP('',(#69432,#69433,#69434,#69435));
#17019=EDGE_LOOP('',(#69436,#69437,#69438,#69439));
#17020=EDGE_LOOP('',(#69440,#69441,#69442,#69443));
#17021=EDGE_LOOP('',(#69444,#69445,#69446,#69447));
#17022=EDGE_LOOP('',(#69448,#69449,#69450,#69451));
#17023=EDGE_LOOP('',(#69452,#69453,#69454,#69455));
#17024=EDGE_LOOP('',(#69456,#69457,#69458,#69459));
#17025=EDGE_LOOP('',(#69460,#69461,#69462,#69463));
#17026=EDGE_LOOP('',(#69464,#69465,#69466,#69467));
#17027=EDGE_LOOP('',(#69468,#69469,#69470,#69471));
#17028=EDGE_LOOP('',(#69472,#69473,#69474,#69475));
#17029=EDGE_LOOP('',(#69476,#69477,#69478,#69479));
#17030=EDGE_LOOP('',(#69480,#69481,#69482,#69483));
#17031=EDGE_LOOP('',(#69484,#69485,#69486,#69487));
#17032=EDGE_LOOP('',(#69488,#69489,#69490,#69491));
#17033=EDGE_LOOP('',(#69492,#69493,#69494,#69495));
#17034=EDGE_LOOP('',(#69496,#69497,#69498,#69499));
#17035=EDGE_LOOP('',(#69500,#69501,#69502,#69503));
#17036=EDGE_LOOP('',(#69504,#69505,#69506,#69507));
#17037=EDGE_LOOP('',(#69508,#69509,#69510,#69511));
#17038=EDGE_LOOP('',(#69512,#69513,#69514,#69515));
#17039=EDGE_LOOP('',(#69516,#69517,#69518,#69519));
#17040=EDGE_LOOP('',(#69520,#69521,#69522,#69523));
#17041=EDGE_LOOP('',(#69524,#69525,#69526,#69527));
#17042=EDGE_LOOP('',(#69528,#69529,#69530,#69531));
#17043=EDGE_LOOP('',(#69532,#69533,#69534,#69535));
#17044=EDGE_LOOP('',(#69536,#69537,#69538,#69539));
#17045=EDGE_LOOP('',(#69540,#69541,#69542,#69543));
#17046=EDGE_LOOP('',(#69544,#69545,#69546,#69547));
#17047=EDGE_LOOP('',(#69548,#69549,#69550,#69551));
#17048=EDGE_LOOP('',(#69552,#69553,#69554,#69555));
#17049=EDGE_LOOP('',(#69556,#69557,#69558,#69559));
#17050=EDGE_LOOP('',(#69560,#69561,#69562,#69563));
#17051=EDGE_LOOP('',(#69564,#69565,#69566,#69567));
#17052=EDGE_LOOP('',(#69568,#69569,#69570,#69571));
#17053=EDGE_LOOP('',(#69572,#69573,#69574,#69575));
#17054=EDGE_LOOP('',(#69576,#69577,#69578,#69579));
#17055=EDGE_LOOP('',(#69580,#69581,#69582,#69583));
#17056=EDGE_LOOP('',(#69584,#69585,#69586,#69587));
#17057=EDGE_LOOP('',(#69588,#69589,#69590,#69591));
#17058=EDGE_LOOP('',(#69592,#69593,#69594,#69595));
#17059=EDGE_LOOP('',(#69596,#69597,#69598,#69599));
#17060=EDGE_LOOP('',(#69600,#69601,#69602,#69603));
#17061=EDGE_LOOP('',(#69604,#69605,#69606,#69607));
#17062=EDGE_LOOP('',(#69608,#69609,#69610,#69611));
#17063=EDGE_LOOP('',(#69612,#69613,#69614,#69615));
#17064=EDGE_LOOP('',(#69616,#69617,#69618,#69619));
#17065=EDGE_LOOP('',(#69620,#69621,#69622,#69623));
#17066=EDGE_LOOP('',(#69624,#69625,#69626,#69627));
#17067=EDGE_LOOP('',(#69628,#69629,#69630,#69631));
#17068=EDGE_LOOP('',(#69632,#69633,#69634,#69635));
#17069=EDGE_LOOP('',(#69636,#69637,#69638,#69639));
#17070=EDGE_LOOP('',(#69640,#69641,#69642,#69643));
#17071=EDGE_LOOP('',(#69644,#69645,#69646,#69647));
#17072=EDGE_LOOP('',(#69648,#69649,#69650,#69651));
#17073=EDGE_LOOP('',(#69652,#69653,#69654,#69655));
#17074=EDGE_LOOP('',(#69656,#69657,#69658,#69659));
#17075=EDGE_LOOP('',(#69660,#69661,#69662,#69663));
#17076=EDGE_LOOP('',(#69664,#69665,#69666,#69667));
#17077=EDGE_LOOP('',(#69668,#69669,#69670,#69671));
#17078=EDGE_LOOP('',(#69672,#69673,#69674,#69675));
#17079=EDGE_LOOP('',(#69676,#69677,#69678,#69679));
#17080=EDGE_LOOP('',(#69680,#69681,#69682,#69683));
#17081=EDGE_LOOP('',(#69684,#69685,#69686,#69687));
#17082=EDGE_LOOP('',(#69688,#69689,#69690,#69691));
#17083=EDGE_LOOP('',(#69692,#69693,#69694,#69695));
#17084=EDGE_LOOP('',(#69696,#69697,#69698,#69699));
#17085=EDGE_LOOP('',(#69700,#69701,#69702,#69703));
#17086=EDGE_LOOP('',(#69704,#69705,#69706,#69707));
#17087=EDGE_LOOP('',(#69708,#69709,#69710,#69711));
#17088=EDGE_LOOP('',(#69712,#69713,#69714,#69715));
#17089=EDGE_LOOP('',(#69716,#69717,#69718,#69719));
#17090=EDGE_LOOP('',(#69720,#69721,#69722,#69723));
#17091=EDGE_LOOP('',(#69724,#69725,#69726,#69727));
#17092=EDGE_LOOP('',(#69728,#69729,#69730,#69731));
#17093=EDGE_LOOP('',(#69732,#69733,#69734,#69735));
#17094=EDGE_LOOP('',(#69736,#69737,#69738,#69739));
#17095=EDGE_LOOP('',(#69740,#69741,#69742,#69743));
#17096=EDGE_LOOP('',(#69744,#69745,#69746,#69747));
#17097=EDGE_LOOP('',(#69748,#69749,#69750,#69751));
#17098=EDGE_LOOP('',(#69752,#69753,#69754,#69755));
#17099=EDGE_LOOP('',(#69756,#69757,#69758,#69759));
#17100=EDGE_LOOP('',(#69760,#69761,#69762,#69763));
#17101=EDGE_LOOP('',(#69764,#69765,#69766,#69767));
#17102=EDGE_LOOP('',(#69768,#69769,#69770,#69771));
#17103=EDGE_LOOP('',(#69772,#69773,#69774,#69775));
#17104=EDGE_LOOP('',(#69776,#69777,#69778,#69779));
#17105=EDGE_LOOP('',(#69780,#69781,#69782,#69783));
#17106=EDGE_LOOP('',(#69784,#69785,#69786,#69787));
#17107=EDGE_LOOP('',(#69788,#69789,#69790,#69791));
#17108=EDGE_LOOP('',(#69792,#69793,#69794,#69795));
#17109=EDGE_LOOP('',(#69796,#69797,#69798,#69799));
#17110=EDGE_LOOP('',(#69800,#69801,#69802,#69803));
#17111=EDGE_LOOP('',(#69804,#69805,#69806,#69807));
#17112=EDGE_LOOP('',(#69808,#69809,#69810,#69811));
#17113=EDGE_LOOP('',(#69812,#69813,#69814,#69815));
#17114=EDGE_LOOP('',(#69816,#69817,#69818,#69819));
#17115=EDGE_LOOP('',(#69820,#69821,#69822,#69823));
#17116=EDGE_LOOP('',(#69824,#69825,#69826,#69827));
#17117=EDGE_LOOP('',(#69828,#69829,#69830,#69831));
#17118=EDGE_LOOP('',(#69832,#69833,#69834,#69835));
#17119=EDGE_LOOP('',(#69836,#69837,#69838,#69839));
#17120=EDGE_LOOP('',(#69840,#69841,#69842,#69843));
#17121=EDGE_LOOP('',(#69844,#69845,#69846,#69847));
#17122=EDGE_LOOP('',(#69848,#69849,#69850,#69851));
#17123=EDGE_LOOP('',(#69852,#69853,#69854,#69855));
#17124=EDGE_LOOP('',(#69856,#69857,#69858,#69859));
#17125=EDGE_LOOP('',(#69860,#69861,#69862,#69863));
#17126=EDGE_LOOP('',(#69864,#69865,#69866,#69867));
#17127=EDGE_LOOP('',(#69868,#69869,#69870,#69871));
#17128=EDGE_LOOP('',(#69872,#69873,#69874,#69875));
#17129=EDGE_LOOP('',(#69876,#69877,#69878,#69879));
#17130=EDGE_LOOP('',(#69880,#69881,#69882,#69883));
#17131=EDGE_LOOP('',(#69884,#69885,#69886,#69887));
#17132=EDGE_LOOP('',(#69888,#69889,#69890,#69891));
#17133=EDGE_LOOP('',(#69892,#69893,#69894,#69895));
#17134=EDGE_LOOP('',(#69896,#69897,#69898,#69899));
#17135=EDGE_LOOP('',(#69900,#69901,#69902,#69903));
#17136=EDGE_LOOP('',(#69904,#69905,#69906,#69907));
#17137=EDGE_LOOP('',(#69908,#69909,#69910,#69911));
#17138=EDGE_LOOP('',(#69912,#69913,#69914,#69915));
#17139=EDGE_LOOP('',(#69916,#69917,#69918,#69919));
#17140=EDGE_LOOP('',(#69920,#69921,#69922,#69923));
#17141=EDGE_LOOP('',(#69924,#69925,#69926,#69927));
#17142=EDGE_LOOP('',(#69928,#69929,#69930,#69931));
#17143=EDGE_LOOP('',(#69932,#69933,#69934,#69935));
#17144=EDGE_LOOP('',(#69936,#69937,#69938,#69939));
#17145=EDGE_LOOP('',(#69940,#69941,#69942,#69943));
#17146=EDGE_LOOP('',(#69944,#69945,#69946,#69947));
#17147=EDGE_LOOP('',(#69948,#69949,#69950,#69951));
#17148=EDGE_LOOP('',(#69952,#69953,#69954,#69955));
#17149=EDGE_LOOP('',(#69956,#69957,#69958,#69959));
#17150=EDGE_LOOP('',(#69960,#69961,#69962,#69963));
#17151=EDGE_LOOP('',(#69964,#69965,#69966,#69967));
#17152=EDGE_LOOP('',(#69968,#69969,#69970,#69971));
#17153=EDGE_LOOP('',(#69972,#69973,#69974,#69975));
#17154=EDGE_LOOP('',(#69976,#69977,#69978,#69979));
#17155=EDGE_LOOP('',(#69980,#69981,#69982,#69983));
#17156=EDGE_LOOP('',(#69984,#69985,#69986,#69987));
#17157=EDGE_LOOP('',(#69988,#69989,#69990,#69991));
#17158=EDGE_LOOP('',(#69992,#69993,#69994,#69995));
#17159=EDGE_LOOP('',(#69996,#69997,#69998,#69999));
#17160=EDGE_LOOP('',(#70000,#70001,#70002,#70003));
#17161=EDGE_LOOP('',(#70004,#70005,#70006,#70007));
#17162=EDGE_LOOP('',(#70008,#70009,#70010,#70011));
#17163=EDGE_LOOP('',(#70012,#70013,#70014,#70015));
#17164=EDGE_LOOP('',(#70016,#70017,#70018,#70019));
#17165=EDGE_LOOP('',(#70020,#70021,#70022,#70023));
#17166=EDGE_LOOP('',(#70024,#70025,#70026,#70027));
#17167=EDGE_LOOP('',(#70028,#70029,#70030,#70031));
#17168=EDGE_LOOP('',(#70032,#70033,#70034,#70035));
#17169=EDGE_LOOP('',(#70036,#70037,#70038,#70039));
#17170=EDGE_LOOP('',(#70040,#70041,#70042,#70043));
#17171=EDGE_LOOP('',(#70044,#70045,#70046,#70047));
#17172=EDGE_LOOP('',(#70048,#70049,#70050,#70051));
#17173=EDGE_LOOP('',(#70052,#70053,#70054,#70055));
#17174=EDGE_LOOP('',(#70056,#70057,#70058,#70059));
#17175=EDGE_LOOP('',(#70060,#70061,#70062,#70063));
#17176=EDGE_LOOP('',(#70064,#70065,#70066,#70067));
#17177=EDGE_LOOP('',(#70068,#70069,#70070,#70071));
#17178=EDGE_LOOP('',(#70072,#70073,#70074,#70075));
#17179=EDGE_LOOP('',(#70076,#70077,#70078,#70079));
#17180=EDGE_LOOP('',(#70080,#70081,#70082,#70083));
#17181=EDGE_LOOP('',(#70084,#70085,#70086,#70087));
#17182=EDGE_LOOP('',(#70088,#70089,#70090,#70091));
#17183=EDGE_LOOP('',(#70092,#70093,#70094,#70095));
#17184=EDGE_LOOP('',(#70096,#70097,#70098,#70099));
#17185=EDGE_LOOP('',(#70100,#70101,#70102,#70103));
#17186=EDGE_LOOP('',(#70104,#70105,#70106,#70107));
#17187=EDGE_LOOP('',(#70108,#70109,#70110,#70111));
#17188=EDGE_LOOP('',(#70112,#70113,#70114,#70115));
#17189=EDGE_LOOP('',(#70116,#70117,#70118,#70119));
#17190=EDGE_LOOP('',(#70120,#70121,#70122,#70123));
#17191=EDGE_LOOP('',(#70124,#70125,#70126,#70127));
#17192=EDGE_LOOP('',(#70128,#70129,#70130,#70131));
#17193=EDGE_LOOP('',(#70132,#70133,#70134,#70135));
#17194=EDGE_LOOP('',(#70136,#70137,#70138,#70139));
#17195=EDGE_LOOP('',(#70140,#70141,#70142,#70143));
#17196=EDGE_LOOP('',(#70144,#70145,#70146,#70147));
#17197=EDGE_LOOP('',(#70148,#70149,#70150,#70151));
#17198=EDGE_LOOP('',(#70152,#70153,#70154,#70155));
#17199=EDGE_LOOP('',(#70156,#70157,#70158,#70159));
#17200=EDGE_LOOP('',(#70160,#70161,#70162,#70163));
#17201=EDGE_LOOP('',(#70164,#70165,#70166,#70167));
#17202=EDGE_LOOP('',(#70168,#70169,#70170,#70171));
#17203=EDGE_LOOP('',(#70172,#70173,#70174,#70175));
#17204=EDGE_LOOP('',(#70176,#70177,#70178,#70179));
#17205=EDGE_LOOP('',(#70180,#70181,#70182,#70183));
#17206=EDGE_LOOP('',(#70184,#70185,#70186,#70187));
#17207=EDGE_LOOP('',(#70188,#70189,#70190,#70191));
#17208=EDGE_LOOP('',(#70192,#70193,#70194,#70195));
#17209=EDGE_LOOP('',(#70196,#70197,#70198,#70199));
#17210=EDGE_LOOP('',(#70200,#70201,#70202,#70203));
#17211=EDGE_LOOP('',(#70204,#70205,#70206,#70207));
#17212=EDGE_LOOP('',(#70208,#70209,#70210,#70211));
#17213=EDGE_LOOP('',(#70212,#70213,#70214,#70215));
#17214=EDGE_LOOP('',(#70216,#70217,#70218,#70219));
#17215=EDGE_LOOP('',(#70220,#70221,#70222,#70223));
#17216=EDGE_LOOP('',(#70224,#70225,#70226,#70227));
#17217=EDGE_LOOP('',(#70228,#70229,#70230,#70231));
#17218=EDGE_LOOP('',(#70232,#70233,#70234,#70235));
#17219=EDGE_LOOP('',(#70236,#70237,#70238,#70239));
#17220=EDGE_LOOP('',(#70240,#70241,#70242,#70243));
#17221=EDGE_LOOP('',(#70244,#70245,#70246,#70247));
#17222=EDGE_LOOP('',(#70248,#70249,#70250,#70251));
#17223=EDGE_LOOP('',(#70252,#70253,#70254,#70255));
#17224=EDGE_LOOP('',(#70256,#70257,#70258,#70259));
#17225=EDGE_LOOP('',(#70260,#70261,#70262,#70263));
#17226=EDGE_LOOP('',(#70264,#70265,#70266,#70267));
#17227=EDGE_LOOP('',(#70268,#70269,#70270,#70271,#70272,#70273));
#17228=EDGE_LOOP('',(#70274,#70275,#70276,#70277));
#17229=EDGE_LOOP('',(#70278,#70279,#70280,#70281));
#17230=EDGE_LOOP('',(#70282,#70283,#70284,#70285));
#17231=EDGE_LOOP('',(#70286,#70287,#70288,#70289));
#17232=EDGE_LOOP('',(#70290,#70291,#70292,#70293));
#17233=EDGE_LOOP('',(#70294,#70295,#70296,#70297));
#17234=EDGE_LOOP('',(#70298,#70299,#70300,#70301));
#17235=EDGE_LOOP('',(#70302,#70303,#70304,#70305,#70306,#70307,#70308,#70309,
#70310));
#17236=EDGE_LOOP('',(#70311,#70312,#70313,#70314));
#17237=EDGE_LOOP('',(#70315,#70316,#70317,#70318));
#17238=EDGE_LOOP('',(#70319,#70320,#70321,#70322));
#17239=EDGE_LOOP('',(#70323,#70324,#70325,#70326));
#17240=EDGE_LOOP('',(#70327,#70328,#70329,#70330));
#17241=EDGE_LOOP('',(#70331,#70332,#70333,#70334));
#17242=EDGE_LOOP('',(#70335,#70336,#70337,#70338));
#17243=EDGE_LOOP('',(#70339,#70340,#70341,#70342,#70343));
#17244=EDGE_LOOP('',(#70344,#70345,#70346,#70347));
#17245=EDGE_LOOP('',(#70348,#70349,#70350,#70351));
#17246=EDGE_LOOP('',(#70352,#70353,#70354,#70355));
#17247=EDGE_LOOP('',(#70356,#70357,#70358,#70359,#70360));
#17248=EDGE_LOOP('',(#70361,#70362,#70363,#70364));
#17249=EDGE_LOOP('',(#70365,#70366,#70367));
#17250=EDGE_LOOP('',(#70368,#70369,#70370,#70371,#70372,#70373,#70374,#70375,
#70376,#70377));
#17251=EDGE_LOOP('',(#70378,#70379,#70380));
#17252=EDGE_LOOP('',(#70381,#70382,#70383,#70384));
#17253=EDGE_LOOP('',(#70385,#70386,#70387,#70388,#70389));
#17254=EDGE_LOOP('',(#70390,#70391,#70392,#70393));
#17255=EDGE_LOOP('',(#70394,#70395,#70396,#70397));
#17256=EDGE_LOOP('',(#70398,#70399,#70400,#70401));
#17257=EDGE_LOOP('',(#70402,#70403,#70404,#70405,#70406));
#17258=EDGE_LOOP('',(#70407,#70408,#70409));
#17259=EDGE_LOOP('',(#70410,#70411,#70412,#70413));
#17260=EDGE_LOOP('',(#70414,#70415,#70416,#70417,#70418));
#17261=EDGE_LOOP('',(#70419,#70420,#70421,#70422));
#17262=EDGE_LOOP('',(#70423,#70424,#70425,#70426));
#17263=EDGE_LOOP('',(#70427,#70428,#70429,#70430));
#17264=EDGE_LOOP('',(#70431,#70432,#70433,#70434,#70435));
#17265=EDGE_LOOP('',(#70436,#70437,#70438,#70439));
#17266=EDGE_LOOP('',(#70440,#70441,#70442,#70443,#70444,#70445,#70446));
#17267=EDGE_LOOP('',(#70447,#70448,#70449));
#17268=EDGE_LOOP('',(#70450,#70451,#70452,#70453,#70454));
#17269=EDGE_LOOP('',(#70455,#70456,#70457,#70458));
#17270=EDGE_LOOP('',(#70459,#70460,#70461,#70462));
#17271=EDGE_LOOP('',(#70463,#70464,#70465,#70466));
#17272=EDGE_LOOP('',(#70467,#70468,#70469,#70470));
#17273=EDGE_LOOP('',(#70471,#70472,#70473,#70474,#70475));
#17274=EDGE_LOOP('',(#70476,#70477,#70478,#70479));
#17275=EDGE_LOOP('',(#70480,#70481,#70482,#70483));
#17276=EDGE_LOOP('',(#70484,#70485,#70486,#70487));
#17277=EDGE_LOOP('',(#70488,#70489,#70490,#70491));
#17278=EDGE_LOOP('',(#70492,#70493,#70494,#70495));
#17279=EDGE_LOOP('',(#70496,#70497,#70498,#70499));
#17280=EDGE_LOOP('',(#70500,#70501,#70502,#70503));
#17281=EDGE_LOOP('',(#70504,#70505,#70506,#70507));
#17282=EDGE_LOOP('',(#70508,#70509,#70510,#70511));
#17283=EDGE_LOOP('',(#70512,#70513,#70514,#70515));
#17284=EDGE_LOOP('',(#70516,#70517,#70518,#70519));
#17285=EDGE_LOOP('',(#70520,#70521,#70522,#70523));
#17286=EDGE_LOOP('',(#70524,#70525,#70526,#70527));
#17287=EDGE_LOOP('',(#70528,#70529,#70530,#70531));
#17288=EDGE_LOOP('',(#70532,#70533,#70534,#70535));
#17289=EDGE_LOOP('',(#70536,#70537,#70538,#70539));
#17290=EDGE_LOOP('',(#70540,#70541,#70542,#70543));
#17291=EDGE_LOOP('',(#70544,#70545,#70546,#70547));
#17292=EDGE_LOOP('',(#70548,#70549,#70550,#70551));
#17293=EDGE_LOOP('',(#70552,#70553,#70554,#70555));
#17294=EDGE_LOOP('',(#70556,#70557,#70558,#70559));
#17295=EDGE_LOOP('',(#70560,#70561,#70562,#70563));
#17296=EDGE_LOOP('',(#70564,#70565,#70566,#70567));
#17297=EDGE_LOOP('',(#70568,#70569,#70570,#70571));
#17298=EDGE_LOOP('',(#70572,#70573,#70574,#70575));
#17299=EDGE_LOOP('',(#70576,#70577,#70578,#70579));
#17300=EDGE_LOOP('',(#70580,#70581,#70582,#70583));
#17301=EDGE_LOOP('',(#70584,#70585,#70586,#70587));
#17302=EDGE_LOOP('',(#70588,#70589,#70590,#70591));
#17303=EDGE_LOOP('',(#70592,#70593,#70594,#70595));
#17304=EDGE_LOOP('',(#70596,#70597,#70598,#70599));
#17305=EDGE_LOOP('',(#70600,#70601,#70602,#70603));
#17306=EDGE_LOOP('',(#70604,#70605,#70606,#70607));
#17307=EDGE_LOOP('',(#70608,#70609,#70610,#70611));
#17308=EDGE_LOOP('',(#70612,#70613,#70614,#70615));
#17309=EDGE_LOOP('',(#70616,#70617,#70618,#70619));
#17310=EDGE_LOOP('',(#70620,#70621,#70622,#70623));
#17311=EDGE_LOOP('',(#70624,#70625,#70626,#70627));
#17312=EDGE_LOOP('',(#70628,#70629,#70630,#70631));
#17313=EDGE_LOOP('',(#70632,#70633,#70634,#70635));
#17314=EDGE_LOOP('',(#70636,#70637,#70638,#70639));
#17315=EDGE_LOOP('',(#70640,#70641,#70642,#70643));
#17316=EDGE_LOOP('',(#70644,#70645,#70646,#70647));
#17317=EDGE_LOOP('',(#70648,#70649,#70650,#70651));
#17318=EDGE_LOOP('',(#70652,#70653,#70654,#70655));
#17319=EDGE_LOOP('',(#70656,#70657,#70658,#70659));
#17320=EDGE_LOOP('',(#70660,#70661,#70662,#70663));
#17321=EDGE_LOOP('',(#70664,#70665,#70666,#70667));
#17322=EDGE_LOOP('',(#70668,#70669,#70670,#70671));
#17323=EDGE_LOOP('',(#70672,#70673,#70674,#70675));
#17324=EDGE_LOOP('',(#70676,#70677,#70678,#70679));
#17325=EDGE_LOOP('',(#70680,#70681,#70682,#70683));
#17326=EDGE_LOOP('',(#70684,#70685,#70686,#70687));
#17327=EDGE_LOOP('',(#70688,#70689,#70690,#70691));
#17328=EDGE_LOOP('',(#70692,#70693,#70694,#70695));
#17329=EDGE_LOOP('',(#70696,#70697,#70698,#70699));
#17330=EDGE_LOOP('',(#70700,#70701,#70702,#70703));
#17331=EDGE_LOOP('',(#70704,#70705,#70706,#70707));
#17332=EDGE_LOOP('',(#70708,#70709,#70710,#70711));
#17333=EDGE_LOOP('',(#70712,#70713,#70714,#70715));
#17334=EDGE_LOOP('',(#70716,#70717,#70718,#70719));
#17335=EDGE_LOOP('',(#70720,#70721,#70722,#70723));
#17336=EDGE_LOOP('',(#70724,#70725,#70726,#70727));
#17337=EDGE_LOOP('',(#70728,#70729,#70730,#70731));
#17338=EDGE_LOOP('',(#70732,#70733,#70734,#70735));
#17339=EDGE_LOOP('',(#70736,#70737,#70738,#70739));
#17340=EDGE_LOOP('',(#70740,#70741,#70742,#70743));
#17341=EDGE_LOOP('',(#70744,#70745,#70746,#70747));
#17342=EDGE_LOOP('',(#70748,#70749,#70750,#70751));
#17343=EDGE_LOOP('',(#70752,#70753,#70754,#70755));
#17344=EDGE_LOOP('',(#70756,#70757,#70758,#70759));
#17345=EDGE_LOOP('',(#70760,#70761,#70762,#70763));
#17346=EDGE_LOOP('',(#70764,#70765,#70766,#70767));
#17347=EDGE_LOOP('',(#70768,#70769,#70770,#70771));
#17348=EDGE_LOOP('',(#70772,#70773,#70774,#70775));
#17349=EDGE_LOOP('',(#70776,#70777,#70778,#70779));
#17350=EDGE_LOOP('',(#70780,#70781,#70782,#70783));
#17351=EDGE_LOOP('',(#70784,#70785,#70786,#70787));
#17352=EDGE_LOOP('',(#70788,#70789,#70790,#70791));
#17353=EDGE_LOOP('',(#70792,#70793,#70794,#70795));
#17354=EDGE_LOOP('',(#70796,#70797,#70798,#70799));
#17355=EDGE_LOOP('',(#70800,#70801,#70802,#70803));
#17356=EDGE_LOOP('',(#70804,#70805,#70806,#70807));
#17357=EDGE_LOOP('',(#70808,#70809,#70810,#70811));
#17358=EDGE_LOOP('',(#70812,#70813,#70814,#70815));
#17359=EDGE_LOOP('',(#70816,#70817,#70818,#70819));
#17360=EDGE_LOOP('',(#70820,#70821,#70822,#70823));
#17361=EDGE_LOOP('',(#70824,#70825,#70826,#70827));
#17362=EDGE_LOOP('',(#70828,#70829,#70830,#70831));
#17363=EDGE_LOOP('',(#70832,#70833,#70834,#70835));
#17364=EDGE_LOOP('',(#70836,#70837,#70838,#70839));
#17365=EDGE_LOOP('',(#70840,#70841,#70842,#70843));
#17366=EDGE_LOOP('',(#70844,#70845,#70846,#70847));
#17367=EDGE_LOOP('',(#70848,#70849,#70850,#70851));
#17368=EDGE_LOOP('',(#70852,#70853,#70854,#70855));
#17369=EDGE_LOOP('',(#70856,#70857,#70858,#70859));
#17370=EDGE_LOOP('',(#70860,#70861,#70862,#70863));
#17371=EDGE_LOOP('',(#70864,#70865,#70866,#70867));
#17372=EDGE_LOOP('',(#70868,#70869,#70870,#70871));
#17373=EDGE_LOOP('',(#70872,#70873,#70874,#70875));
#17374=EDGE_LOOP('',(#70876,#70877,#70878,#70879));
#17375=EDGE_LOOP('',(#70880,#70881,#70882,#70883));
#17376=EDGE_LOOP('',(#70884,#70885,#70886,#70887));
#17377=EDGE_LOOP('',(#70888,#70889,#70890,#70891));
#17378=EDGE_LOOP('',(#70892,#70893,#70894,#70895));
#17379=EDGE_LOOP('',(#70896,#70897,#70898,#70899));
#17380=EDGE_LOOP('',(#70900,#70901,#70902,#70903));
#17381=EDGE_LOOP('',(#70904,#70905,#70906,#70907));
#17382=EDGE_LOOP('',(#70908,#70909,#70910,#70911));
#17383=EDGE_LOOP('',(#70912,#70913,#70914,#70915));
#17384=EDGE_LOOP('',(#70916,#70917,#70918,#70919));
#17385=EDGE_LOOP('',(#70920,#70921,#70922,#70923));
#17386=EDGE_LOOP('',(#70924,#70925,#70926,#70927));
#17387=EDGE_LOOP('',(#70928,#70929,#70930,#70931));
#17388=EDGE_LOOP('',(#70932,#70933,#70934,#70935));
#17389=EDGE_LOOP('',(#70936,#70937,#70938,#70939));
#17390=EDGE_LOOP('',(#70940,#70941,#70942,#70943));
#17391=EDGE_LOOP('',(#70944,#70945,#70946,#70947));
#17392=EDGE_LOOP('',(#70948,#70949,#70950,#70951));
#17393=EDGE_LOOP('',(#70952,#70953,#70954,#70955));
#17394=EDGE_LOOP('',(#70956,#70957,#70958,#70959));
#17395=EDGE_LOOP('',(#70960,#70961,#70962,#70963));
#17396=EDGE_LOOP('',(#70964,#70965,#70966,#70967));
#17397=EDGE_LOOP('',(#70968,#70969,#70970,#70971));
#17398=EDGE_LOOP('',(#70972,#70973,#70974,#70975));
#17399=EDGE_LOOP('',(#70976,#70977,#70978,#70979));
#17400=EDGE_LOOP('',(#70980,#70981,#70982,#70983));
#17401=EDGE_LOOP('',(#70984,#70985,#70986,#70987));
#17402=EDGE_LOOP('',(#70988,#70989,#70990,#70991));
#17403=EDGE_LOOP('',(#70992,#70993,#70994,#70995));
#17404=EDGE_LOOP('',(#70996,#70997,#70998,#70999));
#17405=EDGE_LOOP('',(#71000,#71001,#71002,#71003));
#17406=EDGE_LOOP('',(#71004,#71005,#71006,#71007));
#17407=EDGE_LOOP('',(#71008,#71009,#71010,#71011));
#17408=EDGE_LOOP('',(#71012,#71013,#71014,#71015));
#17409=EDGE_LOOP('',(#71016,#71017,#71018,#71019));
#17410=EDGE_LOOP('',(#71020,#71021,#71022,#71023));
#17411=EDGE_LOOP('',(#71024,#71025,#71026,#71027));
#17412=EDGE_LOOP('',(#71028,#71029,#71030,#71031));
#17413=EDGE_LOOP('',(#71032,#71033,#71034,#71035));
#17414=EDGE_LOOP('',(#71036,#71037,#71038,#71039));
#17415=EDGE_LOOP('',(#71040,#71041,#71042,#71043));
#17416=EDGE_LOOP('',(#71044,#71045,#71046,#71047));
#17417=EDGE_LOOP('',(#71048,#71049,#71050,#71051));
#17418=EDGE_LOOP('',(#71052,#71053,#71054,#71055));
#17419=EDGE_LOOP('',(#71056,#71057,#71058,#71059));
#17420=EDGE_LOOP('',(#71060,#71061,#71062,#71063));
#17421=EDGE_LOOP('',(#71064,#71065,#71066,#71067));
#17422=EDGE_LOOP('',(#71068,#71069,#71070,#71071));
#17423=EDGE_LOOP('',(#71072,#71073,#71074,#71075));
#17424=EDGE_LOOP('',(#71076,#71077,#71078,#71079));
#17425=EDGE_LOOP('',(#71080,#71081,#71082,#71083));
#17426=EDGE_LOOP('',(#71084,#71085,#71086,#71087));
#17427=EDGE_LOOP('',(#71088,#71089,#71090,#71091));
#17428=EDGE_LOOP('',(#71092,#71093,#71094,#71095));
#17429=EDGE_LOOP('',(#71096,#71097,#71098,#71099));
#17430=EDGE_LOOP('',(#71100,#71101,#71102,#71103));
#17431=EDGE_LOOP('',(#71104,#71105,#71106,#71107));
#17432=EDGE_LOOP('',(#71108,#71109,#71110,#71111));
#17433=EDGE_LOOP('',(#71112,#71113,#71114,#71115));
#17434=EDGE_LOOP('',(#71116,#71117,#71118,#71119));
#17435=EDGE_LOOP('',(#71120,#71121,#71122,#71123));
#17436=EDGE_LOOP('',(#71124,#71125,#71126,#71127));
#17437=EDGE_LOOP('',(#71128,#71129,#71130,#71131));
#17438=EDGE_LOOP('',(#71132,#71133,#71134,#71135));
#17439=EDGE_LOOP('',(#71136,#71137,#71138,#71139));
#17440=EDGE_LOOP('',(#71140,#71141,#71142,#71143));
#17441=EDGE_LOOP('',(#71144,#71145,#71146,#71147));
#17442=EDGE_LOOP('',(#71148,#71149,#71150,#71151));
#17443=EDGE_LOOP('',(#71152,#71153,#71154,#71155));
#17444=EDGE_LOOP('',(#71156,#71157,#71158,#71159));
#17445=EDGE_LOOP('',(#71160,#71161,#71162,#71163));
#17446=EDGE_LOOP('',(#71164,#71165,#71166,#71167));
#17447=EDGE_LOOP('',(#71168,#71169,#71170,#71171));
#17448=EDGE_LOOP('',(#71172,#71173,#71174,#71175));
#17449=EDGE_LOOP('',(#71176,#71177,#71178,#71179));
#17450=EDGE_LOOP('',(#71180,#71181,#71182,#71183));
#17451=EDGE_LOOP('',(#71184,#71185,#71186,#71187));
#17452=EDGE_LOOP('',(#71188,#71189,#71190,#71191));
#17453=EDGE_LOOP('',(#71192,#71193,#71194,#71195));
#17454=EDGE_LOOP('',(#71196,#71197,#71198,#71199));
#17455=EDGE_LOOP('',(#71200,#71201,#71202,#71203));
#17456=EDGE_LOOP('',(#71204,#71205,#71206,#71207));
#17457=EDGE_LOOP('',(#71208,#71209,#71210,#71211));
#17458=EDGE_LOOP('',(#71212,#71213,#71214,#71215));
#17459=EDGE_LOOP('',(#71216,#71217,#71218,#71219));
#17460=EDGE_LOOP('',(#71220,#71221,#71222,#71223));
#17461=EDGE_LOOP('',(#71224,#71225,#71226,#71227));
#17462=EDGE_LOOP('',(#71228,#71229,#71230,#71231));
#17463=EDGE_LOOP('',(#71232,#71233,#71234,#71235));
#17464=EDGE_LOOP('',(#71236,#71237,#71238,#71239));
#17465=EDGE_LOOP('',(#71240,#71241,#71242,#71243));
#17466=EDGE_LOOP('',(#71244,#71245,#71246,#71247));
#17467=EDGE_LOOP('',(#71248,#71249,#71250,#71251));
#17468=EDGE_LOOP('',(#71252,#71253,#71254,#71255));
#17469=EDGE_LOOP('',(#71256,#71257,#71258,#71259));
#17470=EDGE_LOOP('',(#71260,#71261,#71262,#71263));
#17471=EDGE_LOOP('',(#71264,#71265,#71266,#71267));
#17472=EDGE_LOOP('',(#71268,#71269,#71270,#71271));
#17473=EDGE_LOOP('',(#71272,#71273,#71274,#71275));
#17474=EDGE_LOOP('',(#71276,#71277,#71278,#71279));
#17475=EDGE_LOOP('',(#71280,#71281,#71282,#71283));
#17476=EDGE_LOOP('',(#71284,#71285,#71286,#71287));
#17477=EDGE_LOOP('',(#71288,#71289,#71290,#71291));
#17478=EDGE_LOOP('',(#71292,#71293,#71294,#71295));
#17479=EDGE_LOOP('',(#71296,#71297,#71298,#71299));
#17480=EDGE_LOOP('',(#71300,#71301,#71302,#71303));
#17481=EDGE_LOOP('',(#71304,#71305,#71306,#71307));
#17482=EDGE_LOOP('',(#71308,#71309,#71310,#71311));
#17483=EDGE_LOOP('',(#71312,#71313,#71314,#71315));
#17484=EDGE_LOOP('',(#71316,#71317,#71318,#71319));
#17485=EDGE_LOOP('',(#71320,#71321,#71322,#71323));
#17486=EDGE_LOOP('',(#71324,#71325,#71326,#71327));
#17487=EDGE_LOOP('',(#71328,#71329,#71330,#71331));
#17488=EDGE_LOOP('',(#71332,#71333,#71334,#71335));
#17489=EDGE_LOOP('',(#71336,#71337,#71338,#71339));
#17490=EDGE_LOOP('',(#71340,#71341,#71342,#71343));
#17491=EDGE_LOOP('',(#71344,#71345,#71346,#71347));
#17492=EDGE_LOOP('',(#71348,#71349,#71350,#71351));
#17493=EDGE_LOOP('',(#71352,#71353,#71354));
#17494=EDGE_LOOP('',(#71355,#71356,#71357));
#17495=EDGE_LOOP('',(#71358,#71359,#71360));
#17496=EDGE_LOOP('',(#71361,#71362,#71363,#71364));
#17497=EDGE_LOOP('',(#71365,#71366,#71367,#71368));
#17498=EDGE_LOOP('',(#71369,#71370,#71371,#71372));
#17499=EDGE_LOOP('',(#71373,#71374,#71375,#71376));
#17500=EDGE_LOOP('',(#71377,#71378,#71379,#71380));
#17501=EDGE_LOOP('',(#71381,#71382,#71383,#71384));
#17502=EDGE_LOOP('',(#71385,#71386,#71387,#71388));
#17503=EDGE_LOOP('',(#71389,#71390,#71391,#71392));
#17504=EDGE_LOOP('',(#71393,#71394,#71395,#71396));
#17505=EDGE_LOOP('',(#71397,#71398,#71399,#71400));
#17506=EDGE_LOOP('',(#71401,#71402,#71403,#71404));
#17507=EDGE_LOOP('',(#71405,#71406,#71407,#71408));
#17508=EDGE_LOOP('',(#71409,#71410,#71411,#71412));
#17509=EDGE_LOOP('',(#71413,#71414,#71415,#71416,#71417));
#17510=EDGE_LOOP('',(#71418,#71419,#71420,#71421,#71422));
#17511=EDGE_LOOP('',(#71423,#71424,#71425,#71426,#71427));
#17512=EDGE_LOOP('',(#71428,#71429,#71430,#71431,#71432));
#17513=EDGE_LOOP('',(#71433,#71434,#71435,#71436,#71437));
#17514=EDGE_LOOP('',(#71438,#71439,#71440,#71441,#71442,#71443,#71444,#71445));
#17515=EDGE_LOOP('',(#71446,#71447,#71448,#71449,#71450));
#17516=EDGE_LOOP('',(#71451,#71452,#71453,#71454,#71455));
#17517=EDGE_LOOP('',(#71456,#71457,#71458,#71459,#71460,#71461,#71462,#71463));
#17518=EDGE_LOOP('',(#71464,#71465,#71466,#71467,#71468));
#17519=EDGE_LOOP('',(#71469,#71470,#71471,#71472));
#17520=EDGE_LOOP('',(#71473,#71474,#71475,#71476));
#17521=EDGE_LOOP('',(#71477,#71478,#71479,#71480));
#17522=EDGE_LOOP('',(#71481,#71482,#71483,#71484));
#17523=EDGE_LOOP('',(#71485,#71486,#71487,#71488));
#17524=EDGE_LOOP('',(#71489,#71490,#71491,#71492));
#17525=EDGE_LOOP('',(#71493,#71494,#71495,#71496));
#17526=EDGE_LOOP('',(#71497,#71498,#71499,#71500));
#17527=EDGE_LOOP('',(#71501,#71502,#71503,#71504));
#17528=EDGE_LOOP('',(#71505,#71506,#71507,#71508,#71509,#71510,#71511,#71512));
#17529=EDGE_LOOP('',(#71513,#71514,#71515,#71516));
#17530=EDGE_LOOP('',(#71517,#71518,#71519,#71520,#71521,#71522,#71523,#71524,
#71525,#71526,#71527,#71528));
#17531=EDGE_LOOP('',(#71529,#71530,#71531,#71532));
#17532=EDGE_LOOP('',(#71533,#71534,#71535,#71536,#71537,#71538));
#17533=EDGE_LOOP('',(#71539,#71540,#71541,#71542,#71543,#71544,#71545,#71546,
#71547,#71548,#71549,#71550,#71551,#71552,#71553,#71554,#71555,#71556));
#17534=EDGE_LOOP('',(#71557,#71558,#71559,#71560,#71561,#71562));
#17535=EDGE_LOOP('',(#71563,#71564,#71565,#71566,#71567,#71568,#71569,#71570,
#71571,#71572,#71573,#71574,#71575,#71576,#71577,#71578));
#17536=EDGE_LOOP('',(#71579,#71580));
#17537=EDGE_LOOP('',(#71581,#71582,#71583,#71584,#71585,#71586,#71587,#71588,
#71589,#71590,#71591,#71592));
#17538=EDGE_LOOP('',(#71593,#71594));
#17539=EDGE_LOOP('',(#71595,#71596));
#17540=EDGE_LOOP('',(#71597,#71598));
#17541=EDGE_LOOP('',(#71599,#71600));
#17542=EDGE_LOOP('',(#71601,#71602,#71603));
#17543=EDGE_LOOP('',(#71604,#71605,#71606,#71607));
#17544=EDGE_LOOP('',(#71608,#71609,#71610,#71611));
#17545=EDGE_LOOP('',(#71612,#71613,#71614,#71615));
#17546=EDGE_LOOP('',(#71616,#71617,#71618,#71619));
#17547=EDGE_LOOP('',(#71620,#71621,#71622,#71623,#71624,#71625));
#17548=EDGE_LOOP('',(#71626,#71627,#71628));
#17549=EDGE_LOOP('',(#71629,#71630,#71631,#71632,#71633,#71634,#71635,#71636));
#17550=EDGE_LOOP('',(#71637,#71638,#71639));
#17551=EDGE_LOOP('',(#71640,#71641,#71642,#71643,#71644,#71645,#71646,#71647,
#71648,#71649,#71650,#71651,#71652,#71653,#71654,#71655,#71656,#71657,#71658,
#71659,#71660,#71661));
#17552=EDGE_LOOP('',(#71662,#71663,#71664,#71665,#71666,#71667));
#17553=EDGE_LOOP('',(#71668,#71669,#71670,#71671));
#17554=EDGE_LOOP('',(#71672,#71673,#71674,#71675));
#17555=EDGE_LOOP('',(#71676,#71677,#71678,#71679));
#17556=EDGE_LOOP('',(#71680,#71681,#71682,#71683));
#17557=EDGE_LOOP('',(#71684,#71685,#71686,#71687));
#17558=EDGE_LOOP('',(#71688,#71689,#71690,#71691));
#17559=EDGE_LOOP('',(#71692,#71693,#71694,#71695));
#17560=EDGE_LOOP('',(#71696));
#17561=EDGE_LOOP('',(#71697,#71698,#71699,#71700,#71701,#71702));
#17562=EDGE_LOOP('',(#71703));
#17563=EDGE_LOOP('',(#71704,#71705,#71706,#71707,#71708));
#17564=EDGE_LOOP('',(#71709,#71710,#71711,#71712,#71713,#71714));
#17565=EDGE_LOOP('',(#71715));
#17566=EDGE_LOOP('',(#71716,#71717,#71718));
#17567=EDGE_LOOP('',(#71719,#71720,#71721));
#17568=EDGE_LOOP('',(#71722,#71723,#71724,#71725));
#17569=EDGE_LOOP('',(#71726,#71727,#71728,#71729,#71730,#71731,#71732,#71733));
#17570=EDGE_LOOP('',(#71734,#71735,#71736));
#17571=EDGE_LOOP('',(#71737,#71738,#71739));
#17572=EDGE_LOOP('',(#71740,#71741,#71742,#71743));
#17573=EDGE_LOOP('',(#71744,#71745,#71746,#71747));
#17574=EDGE_LOOP('',(#71748,#71749,#71750,#71751));
#17575=EDGE_LOOP('',(#71752,#71753,#71754,#71755));
#17576=EDGE_LOOP('',(#71756,#71757,#71758,#71759));
#17577=EDGE_LOOP('',(#71760,#71761,#71762,#71763));
#17578=EDGE_LOOP('',(#71764,#71765,#71766,#71767));
#17579=EDGE_LOOP('',(#71768,#71769,#71770,#71771,#71772,#71773,#71774,#71775,
#71776,#71777,#71778,#71779,#71780,#71781,#71782,#71783,#71784));
#17580=EDGE_LOOP('',(#71785,#71786,#71787,#71788));
#17581=EDGE_LOOP('',(#71789,#71790,#71791,#71792));
#17582=EDGE_LOOP('',(#71793,#71794,#71795,#71796));
#17583=EDGE_LOOP('',(#71797,#71798,#71799,#71800));
#17584=EDGE_LOOP('',(#71801,#71802,#71803,#71804));
#17585=EDGE_LOOP('',(#71805,#71806,#71807,#71808));
#17586=EDGE_LOOP('',(#71809,#71810,#71811,#71812));
#17587=EDGE_LOOP('',(#71813,#71814,#71815,#71816));
#17588=EDGE_LOOP('',(#71817,#71818,#71819,#71820));
#17589=EDGE_LOOP('',(#71821,#71822,#71823,#71824));
#17590=EDGE_LOOP('',(#71825,#71826,#71827,#71828));
#17591=EDGE_LOOP('',(#71829,#71830,#71831,#71832));
#17592=EDGE_LOOP('',(#71833,#71834,#71835,#71836));
#17593=EDGE_LOOP('',(#71837,#71838,#71839,#71840));
#17594=EDGE_LOOP('',(#71841,#71842,#71843,#71844,#71845));
#17595=EDGE_LOOP('',(#71846,#71847,#71848,#71849,#71850));
#17596=EDGE_LOOP('',(#71851,#71852,#71853,#71854,#71855));
#17597=EDGE_LOOP('',(#71856,#71857,#71858,#71859,#71860));
#17598=EDGE_LOOP('',(#71861,#71862,#71863,#71864,#71865));
#17599=EDGE_LOOP('',(#71866,#71867,#71868,#71869,#71870,#71871,#71872,#71873));
#17600=EDGE_LOOP('',(#71874,#71875,#71876,#71877,#71878));
#17601=EDGE_LOOP('',(#71879,#71880,#71881,#71882,#71883));
#17602=EDGE_LOOP('',(#71884,#71885,#71886,#71887,#71888,#71889,#71890,#71891));
#17603=EDGE_LOOP('',(#71892,#71893,#71894,#71895,#71896));
#17604=EDGE_LOOP('',(#71897,#71898,#71899,#71900));
#17605=EDGE_LOOP('',(#71901,#71902,#71903,#71904));
#17606=EDGE_LOOP('',(#71905,#71906,#71907,#71908));
#17607=EDGE_LOOP('',(#71909,#71910,#71911,#71912));
#17608=EDGE_LOOP('',(#71913,#71914,#71915,#71916));
#17609=EDGE_LOOP('',(#71917,#71918,#71919,#71920));
#17610=EDGE_LOOP('',(#71921,#71922,#71923,#71924));
#17611=EDGE_LOOP('',(#71925,#71926,#71927,#71928));
#17612=EDGE_LOOP('',(#71929,#71930,#71931,#71932));
#17613=EDGE_LOOP('',(#71933,#71934,#71935,#71936,#71937,#71938,#71939,#71940));
#17614=EDGE_LOOP('',(#71941,#71942,#71943,#71944));
#17615=EDGE_LOOP('',(#71945,#71946,#71947,#71948));
#17616=EDGE_LOOP('',(#71949,#71950,#71951,#71952,#71953,#71954,#71955,#71956));
#17617=EDGE_LOOP('',(#71957,#71958,#71959,#71960,#71961,#71962,#71963,#71964,
#71965,#71966,#71967,#71968,#71969,#71970,#71971,#71972,#71973,#71974));
#17618=EDGE_LOOP('',(#71975,#71976,#71977,#71978,#71979,#71980,#71981,#71982,
#71983,#71984));
#17619=EDGE_LOOP('',(#71985,#71986,#71987,#71988,#71989,#71990,#71991,#71992,
#71993,#71994,#71995,#71996,#71997,#71998,#71999,#72000,#72001,#72002,#72003,
#72004));
#17620=EDGE_LOOP('',(#72005,#72006,#72007,#72008));
#17621=EDGE_LOOP('',(#72009,#72010,#72011,#72012));
#17622=EDGE_LOOP('',(#72013,#72014,#72015,#72016));
#17623=EDGE_LOOP('',(#72017,#72018,#72019,#72020));
#17624=EDGE_LOOP('',(#72021,#72022,#72023,#72024));
#17625=EDGE_LOOP('',(#72025,#72026,#72027,#72028));
#17626=EDGE_LOOP('',(#72029,#72030,#72031,#72032));
#17627=EDGE_LOOP('',(#72033,#72034,#72035,#72036));
#17628=EDGE_LOOP('',(#72037,#72038,#72039,#72040));
#17629=EDGE_LOOP('',(#72041,#72042,#72043,#72044));
#17630=EDGE_LOOP('',(#72045,#72046,#72047,#72048));
#17631=EDGE_LOOP('',(#72049,#72050,#72051,#72052));
#17632=EDGE_LOOP('',(#72053,#72054,#72055,#72056));
#17633=EDGE_LOOP('',(#72057,#72058,#72059,#72060));
#17634=EDGE_LOOP('',(#72061,#72062,#72063,#72064));
#17635=EDGE_LOOP('',(#72065,#72066,#72067,#72068));
#17636=EDGE_LOOP('',(#72069,#72070,#72071,#72072));
#17637=EDGE_LOOP('',(#72073,#72074,#72075,#72076));
#17638=EDGE_LOOP('',(#72077,#72078,#72079,#72080));
#17639=EDGE_LOOP('',(#72081,#72082,#72083,#72084));
#17640=EDGE_LOOP('',(#72085,#72086,#72087,#72088));
#17641=EDGE_LOOP('',(#72089,#72090,#72091,#72092));
#17642=EDGE_LOOP('',(#72093,#72094,#72095,#72096));
#17643=EDGE_LOOP('',(#72097,#72098,#72099,#72100));
#17644=EDGE_LOOP('',(#72101,#72102,#72103,#72104));
#17645=EDGE_LOOP('',(#72105,#72106,#72107,#72108));
#17646=EDGE_LOOP('',(#72109,#72110,#72111,#72112));
#17647=EDGE_LOOP('',(#72113,#72114,#72115,#72116));
#17648=EDGE_LOOP('',(#72117,#72118,#72119,#72120));
#17649=EDGE_LOOP('',(#72121,#72122,#72123,#72124));
#17650=EDGE_LOOP('',(#72125,#72126,#72127,#72128));
#17651=EDGE_LOOP('',(#72129,#72130,#72131,#72132));
#17652=EDGE_LOOP('',(#72133,#72134,#72135,#72136));
#17653=EDGE_LOOP('',(#72137,#72138,#72139,#72140));
#17654=EDGE_LOOP('',(#72141,#72142,#72143,#72144));
#17655=EDGE_LOOP('',(#72145,#72146,#72147,#72148));
#17656=EDGE_LOOP('',(#72149,#72150,#72151,#72152));
#17657=EDGE_LOOP('',(#72153,#72154,#72155,#72156));
#17658=EDGE_LOOP('',(#72157,#72158,#72159,#72160));
#17659=EDGE_LOOP('',(#72161,#72162,#72163,#72164));
#17660=EDGE_LOOP('',(#72165,#72166,#72167,#72168));
#17661=EDGE_LOOP('',(#72169,#72170,#72171,#72172));
#17662=EDGE_LOOP('',(#72173,#72174,#72175,#72176));
#17663=EDGE_LOOP('',(#72177,#72178,#72179,#72180));
#17664=EDGE_LOOP('',(#72181,#72182,#72183,#72184));
#17665=EDGE_LOOP('',(#72185,#72186,#72187,#72188));
#17666=EDGE_LOOP('',(#72189,#72190,#72191,#72192));
#17667=EDGE_LOOP('',(#72193,#72194,#72195,#72196));
#17668=EDGE_LOOP('',(#72197,#72198,#72199,#72200));
#17669=EDGE_LOOP('',(#72201,#72202,#72203,#72204));
#17670=EDGE_LOOP('',(#72205,#72206,#72207,#72208));
#17671=EDGE_LOOP('',(#72209,#72210,#72211,#72212));
#17672=EDGE_LOOP('',(#72213,#72214,#72215,#72216));
#17673=EDGE_LOOP('',(#72217,#72218,#72219,#72220));
#17674=EDGE_LOOP('',(#72221,#72222,#72223,#72224));
#17675=EDGE_LOOP('',(#72225,#72226,#72227,#72228));
#17676=EDGE_LOOP('',(#72229,#72230,#72231,#72232));
#17677=EDGE_LOOP('',(#72233,#72234,#72235,#72236));
#17678=EDGE_LOOP('',(#72237,#72238,#72239,#72240));
#17679=EDGE_LOOP('',(#72241,#72242,#72243,#72244));
#17680=EDGE_LOOP('',(#72245,#72246,#72247,#72248));
#17681=EDGE_LOOP('',(#72249,#72250,#72251,#72252));
#17682=EDGE_LOOP('',(#72253,#72254,#72255,#72256));
#17683=EDGE_LOOP('',(#72257,#72258,#72259,#72260));
#17684=EDGE_LOOP('',(#72261,#72262,#72263,#72264));
#17685=EDGE_LOOP('',(#72265,#72266,#72267,#72268));
#17686=EDGE_LOOP('',(#72269,#72270,#72271,#72272));
#17687=EDGE_LOOP('',(#72273,#72274,#72275,#72276));
#17688=EDGE_LOOP('',(#72277,#72278,#72279,#72280));
#17689=EDGE_LOOP('',(#72281,#72282,#72283,#72284,#72285));
#17690=EDGE_LOOP('',(#72286,#72287,#72288,#72289,#72290));
#17691=EDGE_LOOP('',(#72291,#72292,#72293,#72294));
#17692=EDGE_LOOP('',(#72295,#72296,#72297,#72298));
#17693=EDGE_LOOP('',(#72299,#72300,#72301));
#17694=EDGE_LOOP('',(#72302,#72303,#72304,#72305));
#17695=EDGE_LOOP('',(#72306,#72307,#72308,#72309));
#17696=EDGE_LOOP('',(#72310,#72311,#72312,#72313));
#17697=EDGE_LOOP('',(#72314,#72315,#72316,#72317));
#17698=EDGE_LOOP('',(#72318,#72319,#72320,#72321));
#17699=EDGE_LOOP('',(#72322,#72323,#72324,#72325));
#17700=EDGE_LOOP('',(#72326,#72327,#72328,#72329));
#17701=EDGE_LOOP('',(#72330,#72331,#72332,#72333));
#17702=EDGE_LOOP('',(#72334,#72335,#72336,#72337,#72338));
#17703=EDGE_LOOP('',(#72339,#72340,#72341));
#17704=EDGE_LOOP('',(#72342,#72343,#72344,#72345));
#17705=EDGE_LOOP('',(#72346,#72347,#72348,#72349));
#17706=EDGE_LOOP('',(#72350,#72351,#72352,#72353));
#17707=EDGE_LOOP('',(#72354,#72355,#72356,#72357));
#17708=EDGE_LOOP('',(#72358,#72359,#72360,#72361));
#17709=EDGE_LOOP('',(#72362,#72363,#72364));
#17710=EDGE_LOOP('',(#72365,#72366,#72367,#72368));
#17711=EDGE_LOOP('',(#72369,#72370,#72371,#72372));
#17712=EDGE_LOOP('',(#72373,#72374,#72375,#72376));
#17713=EDGE_LOOP('',(#72377,#72378,#72379,#72380));
#17714=EDGE_LOOP('',(#72381,#72382,#72383));
#17715=EDGE_LOOP('',(#72384,#72385,#72386,#72387));
#17716=EDGE_LOOP('',(#72388,#72389,#72390,#72391));
#17717=EDGE_LOOP('',(#72392,#72393,#72394,#72395));
#17718=EDGE_LOOP('',(#72396,#72397,#72398,#72399));
#17719=EDGE_LOOP('',(#72400,#72401,#72402,#72403));
#17720=EDGE_LOOP('',(#72404,#72405,#72406,#72407));
#17721=EDGE_LOOP('',(#72408,#72409,#72410,#72411));
#17722=EDGE_LOOP('',(#72412,#72413,#72414,#72415));
#17723=EDGE_LOOP('',(#72416,#72417,#72418,#72419));
#17724=EDGE_LOOP('',(#72420,#72421,#72422,#72423));
#17725=EDGE_LOOP('',(#72424,#72425,#72426,#72427));
#17726=EDGE_LOOP('',(#72428,#72429,#72430,#72431));
#17727=EDGE_LOOP('',(#72432,#72433,#72434,#72435));
#17728=EDGE_LOOP('',(#72436,#72437,#72438,#72439));
#17729=EDGE_LOOP('',(#72440,#72441,#72442,#72443));
#17730=EDGE_LOOP('',(#72444,#72445,#72446,#72447));
#17731=EDGE_LOOP('',(#72448,#72449,#72450,#72451));
#17732=EDGE_LOOP('',(#72452,#72453,#72454,#72455));
#17733=EDGE_LOOP('',(#72456,#72457,#72458,#72459));
#17734=EDGE_LOOP('',(#72460,#72461,#72462,#72463));
#17735=EDGE_LOOP('',(#72464,#72465,#72466,#72467));
#17736=EDGE_LOOP('',(#72468,#72469,#72470,#72471));
#17737=EDGE_LOOP('',(#72472,#72473,#72474,#72475));
#17738=EDGE_LOOP('',(#72476,#72477,#72478,#72479));
#17739=EDGE_LOOP('',(#72480,#72481,#72482,#72483));
#17740=EDGE_LOOP('',(#72484,#72485,#72486,#72487));
#17741=EDGE_LOOP('',(#72488,#72489,#72490,#72491));
#17742=EDGE_LOOP('',(#72492,#72493,#72494,#72495));
#17743=EDGE_LOOP('',(#72496,#72497,#72498,#72499));
#17744=EDGE_LOOP('',(#72500,#72501,#72502,#72503));
#17745=EDGE_LOOP('',(#72504,#72505,#72506,#72507,#72508));
#17746=EDGE_LOOP('',(#72509,#72510,#72511,#72512));
#17747=EDGE_LOOP('',(#72513,#72514,#72515,#72516));
#17748=EDGE_LOOP('',(#72517,#72518,#72519,#72520));
#17749=EDGE_LOOP('',(#72521,#72522,#72523,#72524));
#17750=EDGE_LOOP('',(#72525,#72526,#72527,#72528));
#17751=EDGE_LOOP('',(#72529,#72530,#72531,#72532));
#17752=EDGE_LOOP('',(#72533,#72534,#72535,#72536));
#17753=EDGE_LOOP('',(#72537,#72538,#72539,#72540,#72541,#72542));
#17754=EDGE_LOOP('',(#72543,#72544,#72545,#72546));
#17755=EDGE_LOOP('',(#72547,#72548,#72549,#72550));
#17756=EDGE_LOOP('',(#72551,#72552,#72553,#72554,#72555));
#17757=EDGE_LOOP('',(#72556,#72557,#72558,#72559));
#17758=EDGE_LOOP('',(#72560,#72561,#72562,#72563));
#17759=EDGE_LOOP('',(#72564,#72565,#72566,#72567));
#17760=EDGE_LOOP('',(#72568,#72569,#72570,#72571,#72572));
#17761=EDGE_LOOP('',(#72573,#72574,#72575,#72576));
#17762=EDGE_LOOP('',(#72577,#72578,#72579,#72580));
#17763=EDGE_LOOP('',(#72581,#72582,#72583,#72584));
#17764=EDGE_LOOP('',(#72585,#72586,#72587,#72588));
#17765=EDGE_LOOP('',(#72589,#72590,#72591,#72592,#72593));
#17766=EDGE_LOOP('',(#72594,#72595,#72596,#72597));
#17767=EDGE_LOOP('',(#72598,#72599,#72600,#72601));
#17768=EDGE_LOOP('',(#72602,#72603,#72604,#72605));
#17769=EDGE_LOOP('',(#72606,#72607,#72608,#72609));
#17770=EDGE_LOOP('',(#72610,#72611,#72612,#72613));
#17771=EDGE_LOOP('',(#72614,#72615,#72616,#72617,#72618));
#17772=EDGE_LOOP('',(#72619,#72620,#72621,#72622,#72623,#72624));
#17773=EDGE_LOOP('',(#72625,#72626,#72627,#72628,#72629,#72630));
#17774=EDGE_LOOP('',(#72631,#72632,#72633,#72634,#72635,#72636));
#17775=EDGE_LOOP('',(#72637,#72638,#72639,#72640,#72641));
#17776=EDGE_LOOP('',(#72642,#72643,#72644,#72645,#72646,#72647,#72648));
#17777=EDGE_LOOP('',(#72649,#72650,#72651,#72652,#72653));
#17778=EDGE_LOOP('',(#72654,#72655,#72656,#72657,#72658));
#17779=EDGE_LOOP('',(#72659,#72660,#72661,#72662));
#17780=EDGE_LOOP('',(#72663,#72664,#72665,#72666));
#17781=EDGE_LOOP('',(#72667,#72668,#72669,#72670));
#17782=EDGE_LOOP('',(#72671,#72672,#72673,#72674));
#17783=EDGE_LOOP('',(#72675,#72676,#72677,#72678));
#17784=EDGE_LOOP('',(#72679,#72680,#72681,#72682));
#17785=EDGE_LOOP('',(#72683,#72684,#72685,#72686));
#17786=EDGE_LOOP('',(#72687,#72688,#72689,#72690));
#17787=EDGE_LOOP('',(#72691,#72692,#72693,#72694));
#17788=EDGE_LOOP('',(#72695,#72696,#72697,#72698));
#17789=EDGE_LOOP('',(#72699,#72700,#72701,#72702));
#17790=EDGE_LOOP('',(#72703,#72704,#72705,#72706));
#17791=EDGE_LOOP('',(#72707,#72708,#72709,#72710));
#17792=EDGE_LOOP('',(#72711,#72712,#72713,#72714));
#17793=EDGE_LOOP('',(#72715,#72716,#72717,#72718));
#17794=EDGE_LOOP('',(#72719,#72720,#72721,#72722));
#17795=EDGE_LOOP('',(#72723,#72724,#72725,#72726));
#17796=EDGE_LOOP('',(#72727,#72728,#72729,#72730));
#17797=EDGE_LOOP('',(#72731,#72732,#72733,#72734));
#17798=EDGE_LOOP('',(#72735,#72736,#72737,#72738));
#17799=EDGE_LOOP('',(#72739,#72740,#72741,#72742));
#17800=EDGE_LOOP('',(#72743,#72744,#72745,#72746));
#17801=EDGE_LOOP('',(#72747,#72748,#72749,#72750));
#17802=EDGE_LOOP('',(#72751,#72752,#72753,#72754));
#17803=EDGE_LOOP('',(#72755,#72756,#72757,#72758));
#17804=EDGE_LOOP('',(#72759,#72760,#72761,#72762));
#17805=EDGE_LOOP('',(#72763,#72764,#72765,#72766));
#17806=EDGE_LOOP('',(#72767,#72768,#72769,#72770));
#17807=EDGE_LOOP('',(#72771,#72772,#72773,#72774));
#17808=EDGE_LOOP('',(#72775,#72776,#72777,#72778));
#17809=EDGE_LOOP('',(#72779,#72780,#72781,#72782));
#17810=EDGE_LOOP('',(#72783,#72784,#72785,#72786));
#17811=EDGE_LOOP('',(#72787,#72788,#72789,#72790));
#17812=EDGE_LOOP('',(#72791,#72792,#72793,#72794));
#17813=EDGE_LOOP('',(#72795,#72796,#72797,#72798));
#17814=EDGE_LOOP('',(#72799,#72800,#72801,#72802));
#17815=EDGE_LOOP('',(#72803,#72804,#72805,#72806));
#17816=EDGE_LOOP('',(#72807,#72808,#72809,#72810));
#17817=EDGE_LOOP('',(#72811,#72812,#72813,#72814));
#17818=EDGE_LOOP('',(#72815,#72816,#72817,#72818));
#17819=EDGE_LOOP('',(#72819,#72820,#72821,#72822));
#17820=EDGE_LOOP('',(#72823,#72824,#72825,#72826));
#17821=EDGE_LOOP('',(#72827,#72828,#72829,#72830));
#17822=EDGE_LOOP('',(#72831,#72832,#72833,#72834));
#17823=EDGE_LOOP('',(#72835,#72836,#72837,#72838));
#17824=EDGE_LOOP('',(#72839,#72840,#72841,#72842));
#17825=EDGE_LOOP('',(#72843,#72844,#72845,#72846));
#17826=EDGE_LOOP('',(#72847,#72848,#72849,#72850));
#17827=EDGE_LOOP('',(#72851,#72852,#72853,#72854));
#17828=EDGE_LOOP('',(#72855,#72856,#72857,#72858));
#17829=EDGE_LOOP('',(#72859,#72860,#72861,#72862));
#17830=EDGE_LOOP('',(#72863,#72864,#72865,#72866));
#17831=EDGE_LOOP('',(#72867,#72868,#72869,#72870));
#17832=EDGE_LOOP('',(#72871,#72872,#72873,#72874));
#17833=EDGE_LOOP('',(#72875,#72876,#72877,#72878));
#17834=EDGE_LOOP('',(#72879,#72880,#72881,#72882));
#17835=EDGE_LOOP('',(#72883,#72884,#72885,#72886));
#17836=EDGE_LOOP('',(#72887,#72888,#72889,#72890));
#17837=EDGE_LOOP('',(#72891,#72892,#72893,#72894));
#17838=EDGE_LOOP('',(#72895,#72896,#72897,#72898));
#17839=EDGE_LOOP('',(#72899,#72900,#72901,#72902));
#17840=EDGE_LOOP('',(#72903,#72904,#72905,#72906));
#17841=EDGE_LOOP('',(#72907,#72908,#72909,#72910));
#17842=EDGE_LOOP('',(#72911,#72912,#72913,#72914));
#17843=EDGE_LOOP('',(#72915,#72916,#72917,#72918));
#17844=EDGE_LOOP('',(#72919,#72920,#72921,#72922));
#17845=EDGE_LOOP('',(#72923,#72924,#72925,#72926));
#17846=EDGE_LOOP('',(#72927,#72928,#72929,#72930));
#17847=EDGE_LOOP('',(#72931,#72932,#72933,#72934));
#17848=EDGE_LOOP('',(#72935,#72936,#72937,#72938));
#17849=EDGE_LOOP('',(#72939,#72940,#72941,#72942));
#17850=EDGE_LOOP('',(#72943,#72944,#72945,#72946));
#17851=EDGE_LOOP('',(#72947,#72948,#72949,#72950));
#17852=EDGE_LOOP('',(#72951,#72952,#72953,#72954));
#17853=EDGE_LOOP('',(#72955,#72956,#72957,#72958));
#17854=EDGE_LOOP('',(#72959,#72960,#72961,#72962));
#17855=EDGE_LOOP('',(#72963,#72964,#72965,#72966));
#17856=EDGE_LOOP('',(#72967,#72968,#72969,#72970));
#17857=EDGE_LOOP('',(#72971,#72972,#72973,#72974));
#17858=EDGE_LOOP('',(#72975,#72976,#72977,#72978));
#17859=EDGE_LOOP('',(#72979,#72980,#72981,#72982));
#17860=EDGE_LOOP('',(#72983,#72984,#72985,#72986));
#17861=EDGE_LOOP('',(#72987,#72988,#72989,#72990));
#17862=EDGE_LOOP('',(#72991,#72992,#72993,#72994));
#17863=EDGE_LOOP('',(#72995,#72996,#72997,#72998));
#17864=EDGE_LOOP('',(#72999,#73000,#73001,#73002));
#17865=EDGE_LOOP('',(#73003,#73004,#73005,#73006));
#17866=EDGE_LOOP('',(#73007,#73008,#73009,#73010));
#17867=EDGE_LOOP('',(#73011,#73012,#73013,#73014));
#17868=EDGE_LOOP('',(#73015,#73016,#73017,#73018));
#17869=EDGE_LOOP('',(#73019,#73020,#73021,#73022));
#17870=EDGE_LOOP('',(#73023,#73024,#73025,#73026));
#17871=EDGE_LOOP('',(#73027,#73028,#73029,#73030));
#17872=EDGE_LOOP('',(#73031,#73032,#73033,#73034));
#17873=EDGE_LOOP('',(#73035,#73036,#73037,#73038));
#17874=EDGE_LOOP('',(#73039,#73040,#73041,#73042));
#17875=EDGE_LOOP('',(#73043,#73044,#73045,#73046));
#17876=EDGE_LOOP('',(#73047,#73048,#73049,#73050));
#17877=EDGE_LOOP('',(#73051,#73052,#73053,#73054));
#17878=EDGE_LOOP('',(#73055,#73056,#73057,#73058));
#17879=EDGE_LOOP('',(#73059,#73060,#73061,#73062));
#17880=EDGE_LOOP('',(#73063,#73064,#73065,#73066));
#17881=EDGE_LOOP('',(#73067,#73068,#73069,#73070));
#17882=EDGE_LOOP('',(#73071,#73072,#73073,#73074));
#17883=EDGE_LOOP('',(#73075,#73076,#73077,#73078));
#17884=EDGE_LOOP('',(#73079,#73080,#73081,#73082));
#17885=EDGE_LOOP('',(#73083,#73084,#73085,#73086));
#17886=EDGE_LOOP('',(#73087,#73088,#73089,#73090));
#17887=EDGE_LOOP('',(#73091,#73092,#73093,#73094));
#17888=EDGE_LOOP('',(#73095,#73096,#73097,#73098));
#17889=EDGE_LOOP('',(#73099,#73100,#73101,#73102));
#17890=EDGE_LOOP('',(#73103,#73104,#73105,#73106));
#17891=EDGE_LOOP('',(#73107,#73108,#73109,#73110));
#17892=EDGE_LOOP('',(#73111,#73112,#73113,#73114));
#17893=EDGE_LOOP('',(#73115,#73116,#73117,#73118));
#17894=EDGE_LOOP('',(#73119,#73120,#73121,#73122));
#17895=EDGE_LOOP('',(#73123,#73124,#73125,#73126));
#17896=EDGE_LOOP('',(#73127,#73128,#73129,#73130));
#17897=EDGE_LOOP('',(#73131,#73132,#73133,#73134));
#17898=EDGE_LOOP('',(#73135,#73136,#73137,#73138));
#17899=EDGE_LOOP('',(#73139,#73140,#73141,#73142));
#17900=EDGE_LOOP('',(#73143,#73144,#73145,#73146));
#17901=EDGE_LOOP('',(#73147,#73148,#73149,#73150));
#17902=EDGE_LOOP('',(#73151,#73152,#73153,#73154));
#17903=EDGE_LOOP('',(#73155,#73156,#73157,#73158));
#17904=EDGE_LOOP('',(#73159,#73160,#73161,#73162));
#17905=EDGE_LOOP('',(#73163,#73164,#73165,#73166));
#17906=EDGE_LOOP('',(#73167,#73168,#73169,#73170));
#17907=EDGE_LOOP('',(#73171,#73172,#73173,#73174));
#17908=EDGE_LOOP('',(#73175,#73176,#73177,#73178));
#17909=EDGE_LOOP('',(#73179,#73180,#73181,#73182));
#17910=EDGE_LOOP('',(#73183,#73184,#73185,#73186));
#17911=EDGE_LOOP('',(#73187,#73188,#73189,#73190));
#17912=EDGE_LOOP('',(#73191,#73192,#73193,#73194));
#17913=EDGE_LOOP('',(#73195,#73196,#73197,#73198));
#17914=EDGE_LOOP('',(#73199,#73200,#73201,#73202));
#17915=EDGE_LOOP('',(#73203,#73204,#73205,#73206));
#17916=EDGE_LOOP('',(#73207,#73208,#73209,#73210));
#17917=EDGE_LOOP('',(#73211,#73212,#73213,#73214));
#17918=EDGE_LOOP('',(#73215,#73216,#73217,#73218));
#17919=EDGE_LOOP('',(#73219,#73220,#73221,#73222));
#17920=EDGE_LOOP('',(#73223,#73224,#73225,#73226));
#17921=EDGE_LOOP('',(#73227,#73228,#73229,#73230));
#17922=EDGE_LOOP('',(#73231,#73232,#73233,#73234));
#17923=EDGE_LOOP('',(#73235,#73236,#73237,#73238));
#17924=EDGE_LOOP('',(#73239,#73240,#73241,#73242));
#17925=EDGE_LOOP('',(#73243,#73244,#73245,#73246));
#17926=EDGE_LOOP('',(#73247,#73248,#73249,#73250));
#17927=EDGE_LOOP('',(#73251,#73252,#73253,#73254));
#17928=EDGE_LOOP('',(#73255,#73256,#73257,#73258));
#17929=EDGE_LOOP('',(#73259,#73260,#73261,#73262));
#17930=EDGE_LOOP('',(#73263,#73264,#73265,#73266));
#17931=EDGE_LOOP('',(#73267,#73268,#73269,#73270));
#17932=EDGE_LOOP('',(#73271,#73272,#73273,#73274));
#17933=EDGE_LOOP('',(#73275,#73276,#73277,#73278));
#17934=EDGE_LOOP('',(#73279,#73280,#73281,#73282));
#17935=EDGE_LOOP('',(#73283,#73284,#73285,#73286));
#17936=EDGE_LOOP('',(#73287,#73288,#73289,#73290));
#17937=EDGE_LOOP('',(#73291,#73292,#73293,#73294));
#17938=EDGE_LOOP('',(#73295,#73296,#73297,#73298));
#17939=EDGE_LOOP('',(#73299,#73300,#73301,#73302));
#17940=EDGE_LOOP('',(#73303,#73304,#73305,#73306));
#17941=EDGE_LOOP('',(#73307,#73308,#73309,#73310));
#17942=EDGE_LOOP('',(#73311,#73312,#73313,#73314));
#17943=EDGE_LOOP('',(#73315,#73316,#73317,#73318));
#17944=EDGE_LOOP('',(#73319,#73320,#73321,#73322));
#17945=EDGE_LOOP('',(#73323,#73324,#73325,#73326));
#17946=EDGE_LOOP('',(#73327,#73328,#73329,#73330));
#17947=EDGE_LOOP('',(#73331,#73332,#73333,#73334));
#17948=EDGE_LOOP('',(#73335,#73336,#73337,#73338));
#17949=EDGE_LOOP('',(#73339,#73340,#73341,#73342));
#17950=EDGE_LOOP('',(#73343,#73344,#73345,#73346));
#17951=EDGE_LOOP('',(#73347,#73348,#73349,#73350));
#17952=EDGE_LOOP('',(#73351,#73352,#73353,#73354));
#17953=EDGE_LOOP('',(#73355,#73356,#73357,#73358));
#17954=EDGE_LOOP('',(#73359,#73360,#73361,#73362));
#17955=EDGE_LOOP('',(#73363,#73364,#73365,#73366));
#17956=EDGE_LOOP('',(#73367,#73368,#73369,#73370));
#17957=EDGE_LOOP('',(#73371,#73372,#73373,#73374));
#17958=EDGE_LOOP('',(#73375,#73376,#73377,#73378));
#17959=EDGE_LOOP('',(#73379,#73380,#73381,#73382));
#17960=EDGE_LOOP('',(#73383,#73384,#73385,#73386));
#17961=EDGE_LOOP('',(#73387,#73388,#73389,#73390));
#17962=EDGE_LOOP('',(#73391,#73392,#73393,#73394));
#17963=EDGE_LOOP('',(#73395,#73396,#73397,#73398));
#17964=EDGE_LOOP('',(#73399,#73400,#73401,#73402));
#17965=EDGE_LOOP('',(#73403,#73404,#73405,#73406));
#17966=EDGE_LOOP('',(#73407,#73408,#73409,#73410));
#17967=EDGE_LOOP('',(#73411,#73412,#73413,#73414));
#17968=EDGE_LOOP('',(#73415,#73416,#73417,#73418));
#17969=EDGE_LOOP('',(#73419,#73420,#73421,#73422));
#17970=EDGE_LOOP('',(#73423,#73424,#73425,#73426));
#17971=EDGE_LOOP('',(#73427,#73428,#73429,#73430));
#17972=EDGE_LOOP('',(#73431,#73432,#73433,#73434));
#17973=EDGE_LOOP('',(#73435,#73436,#73437,#73438));
#17974=EDGE_LOOP('',(#73439,#73440,#73441,#73442));
#17975=EDGE_LOOP('',(#73443,#73444,#73445,#73446));
#17976=EDGE_LOOP('',(#73447,#73448,#73449,#73450));
#17977=EDGE_LOOP('',(#73451,#73452,#73453,#73454));
#17978=EDGE_LOOP('',(#73455,#73456,#73457,#73458));
#17979=EDGE_LOOP('',(#73459,#73460,#73461,#73462));
#17980=EDGE_LOOP('',(#73463,#73464,#73465,#73466));
#17981=EDGE_LOOP('',(#73467,#73468,#73469,#73470));
#17982=EDGE_LOOP('',(#73471,#73472,#73473,#73474));
#17983=EDGE_LOOP('',(#73475,#73476,#73477,#73478));
#17984=EDGE_LOOP('',(#73479,#73480,#73481,#73482));
#17985=EDGE_LOOP('',(#73483,#73484,#73485,#73486));
#17986=EDGE_LOOP('',(#73487,#73488,#73489,#73490));
#17987=EDGE_LOOP('',(#73491,#73492,#73493,#73494));
#17988=EDGE_LOOP('',(#73495,#73496,#73497,#73498));
#17989=EDGE_LOOP('',(#73499,#73500,#73501,#73502));
#17990=EDGE_LOOP('',(#73503,#73504,#73505,#73506));
#17991=EDGE_LOOP('',(#73507,#73508,#73509,#73510));
#17992=EDGE_LOOP('',(#73511,#73512,#73513,#73514));
#17993=EDGE_LOOP('',(#73515,#73516,#73517,#73518));
#17994=EDGE_LOOP('',(#73519,#73520,#73521,#73522));
#17995=EDGE_LOOP('',(#73523,#73524,#73525,#73526));
#17996=EDGE_LOOP('',(#73527,#73528,#73529,#73530));
#17997=EDGE_LOOP('',(#73531,#73532,#73533,#73534));
#17998=EDGE_LOOP('',(#73535,#73536,#73537,#73538));
#17999=EDGE_LOOP('',(#73539,#73540,#73541,#73542));
#18000=EDGE_LOOP('',(#73543,#73544,#73545,#73546));
#18001=EDGE_LOOP('',(#73547,#73548,#73549,#73550));
#18002=EDGE_LOOP('',(#73551,#73552,#73553,#73554));
#18003=EDGE_LOOP('',(#73555,#73556,#73557,#73558));
#18004=EDGE_LOOP('',(#73559,#73560,#73561,#73562));
#18005=EDGE_LOOP('',(#73563,#73564,#73565,#73566));
#18006=EDGE_LOOP('',(#73567,#73568,#73569,#73570));
#18007=EDGE_LOOP('',(#73571,#73572,#73573,#73574));
#18008=EDGE_LOOP('',(#73575,#73576,#73577,#73578));
#18009=EDGE_LOOP('',(#73579,#73580,#73581,#73582));
#18010=EDGE_LOOP('',(#73583,#73584,#73585,#73586));
#18011=EDGE_LOOP('',(#73587,#73588,#73589,#73590));
#18012=EDGE_LOOP('',(#73591,#73592,#73593,#73594));
#18013=EDGE_LOOP('',(#73595,#73596,#73597,#73598));
#18014=EDGE_LOOP('',(#73599,#73600,#73601,#73602));
#18015=EDGE_LOOP('',(#73603,#73604,#73605,#73606));
#18016=EDGE_LOOP('',(#73607,#73608,#73609,#73610));
#18017=EDGE_LOOP('',(#73611,#73612,#73613,#73614));
#18018=EDGE_LOOP('',(#73615,#73616,#73617,#73618));
#18019=EDGE_LOOP('',(#73619,#73620,#73621,#73622));
#18020=EDGE_LOOP('',(#73623,#73624,#73625,#73626));
#18021=EDGE_LOOP('',(#73627,#73628,#73629,#73630));
#18022=EDGE_LOOP('',(#73631,#73632,#73633,#73634));
#18023=EDGE_LOOP('',(#73635,#73636,#73637,#73638));
#18024=EDGE_LOOP('',(#73639,#73640,#73641,#73642));
#18025=EDGE_LOOP('',(#73643,#73644,#73645,#73646));
#18026=EDGE_LOOP('',(#73647,#73648,#73649,#73650));
#18027=EDGE_LOOP('',(#73651,#73652,#73653,#73654));
#18028=EDGE_LOOP('',(#73655,#73656,#73657,#73658));
#18029=EDGE_LOOP('',(#73659,#73660,#73661,#73662));
#18030=EDGE_LOOP('',(#73663,#73664,#73665,#73666));
#18031=EDGE_LOOP('',(#73667,#73668,#73669,#73670));
#18032=EDGE_LOOP('',(#73671,#73672,#73673,#73674));
#18033=EDGE_LOOP('',(#73675,#73676,#73677,#73678));
#18034=EDGE_LOOP('',(#73679,#73680,#73681,#73682));
#18035=EDGE_LOOP('',(#73683,#73684,#73685,#73686));
#18036=EDGE_LOOP('',(#73687,#73688,#73689,#73690));
#18037=EDGE_LOOP('',(#73691,#73692,#73693,#73694));
#18038=EDGE_LOOP('',(#73695,#73696,#73697,#73698));
#18039=EDGE_LOOP('',(#73699,#73700,#73701,#73702));
#18040=EDGE_LOOP('',(#73703,#73704,#73705,#73706));
#18041=EDGE_LOOP('',(#73707,#73708,#73709,#73710));
#18042=EDGE_LOOP('',(#73711,#73712,#73713,#73714));
#18043=EDGE_LOOP('',(#73715,#73716,#73717,#73718));
#18044=EDGE_LOOP('',(#73719,#73720,#73721,#73722));
#18045=EDGE_LOOP('',(#73723,#73724,#73725,#73726));
#18046=EDGE_LOOP('',(#73727,#73728,#73729,#73730));
#18047=EDGE_LOOP('',(#73731,#73732,#73733,#73734));
#18048=EDGE_LOOP('',(#73735,#73736,#73737,#73738));
#18049=EDGE_LOOP('',(#73739,#73740,#73741,#73742));
#18050=EDGE_LOOP('',(#73743,#73744,#73745,#73746));
#18051=EDGE_LOOP('',(#73747,#73748,#73749,#73750));
#18052=EDGE_LOOP('',(#73751,#73752,#73753,#73754));
#18053=EDGE_LOOP('',(#73755,#73756,#73757,#73758));
#18054=EDGE_LOOP('',(#73759,#73760,#73761,#73762));
#18055=EDGE_LOOP('',(#73763,#73764,#73765,#73766));
#18056=EDGE_LOOP('',(#73767,#73768,#73769,#73770));
#18057=EDGE_LOOP('',(#73771,#73772,#73773,#73774));
#18058=EDGE_LOOP('',(#73775,#73776,#73777,#73778));
#18059=EDGE_LOOP('',(#73779,#73780,#73781,#73782));
#18060=EDGE_LOOP('',(#73783,#73784,#73785,#73786));
#18061=EDGE_LOOP('',(#73787,#73788,#73789,#73790));
#18062=EDGE_LOOP('',(#73791,#73792,#73793,#73794));
#18063=EDGE_LOOP('',(#73795,#73796,#73797,#73798));
#18064=EDGE_LOOP('',(#73799,#73800,#73801,#73802));
#18065=EDGE_LOOP('',(#73803,#73804,#73805,#73806));
#18066=EDGE_LOOP('',(#73807,#73808,#73809,#73810));
#18067=EDGE_LOOP('',(#73811,#73812,#73813,#73814));
#18068=EDGE_LOOP('',(#73815,#73816,#73817,#73818));
#18069=EDGE_LOOP('',(#73819,#73820,#73821,#73822));
#18070=EDGE_LOOP('',(#73823,#73824,#73825,#73826));
#18071=EDGE_LOOP('',(#73827,#73828,#73829,#73830));
#18072=EDGE_LOOP('',(#73831,#73832,#73833,#73834));
#18073=EDGE_LOOP('',(#73835,#73836,#73837,#73838));
#18074=EDGE_LOOP('',(#73839,#73840,#73841,#73842));
#18075=EDGE_LOOP('',(#73843,#73844,#73845,#73846));
#18076=EDGE_LOOP('',(#73847,#73848,#73849,#73850));
#18077=EDGE_LOOP('',(#73851,#73852,#73853,#73854));
#18078=EDGE_LOOP('',(#73855,#73856,#73857,#73858));
#18079=EDGE_LOOP('',(#73859,#73860,#73861,#73862));
#18080=EDGE_LOOP('',(#73863,#73864,#73865,#73866));
#18081=EDGE_LOOP('',(#73867,#73868,#73869,#73870));
#18082=EDGE_LOOP('',(#73871,#73872,#73873,#73874));
#18083=EDGE_LOOP('',(#73875,#73876,#73877,#73878));
#18084=EDGE_LOOP('',(#73879,#73880,#73881,#73882));
#18085=EDGE_LOOP('',(#73883,#73884,#73885,#73886));
#18086=EDGE_LOOP('',(#73887,#73888,#73889,#73890,#73891,#73892));
#18087=EDGE_LOOP('',(#73893,#73894,#73895,#73896));
#18088=EDGE_LOOP('',(#73897,#73898,#73899,#73900));
#18089=EDGE_LOOP('',(#73901,#73902,#73903,#73904));
#18090=EDGE_LOOP('',(#73905,#73906,#73907,#73908));
#18091=EDGE_LOOP('',(#73909,#73910,#73911,#73912));
#18092=EDGE_LOOP('',(#73913,#73914,#73915,#73916));
#18093=EDGE_LOOP('',(#73917,#73918,#73919,#73920));
#18094=EDGE_LOOP('',(#73921,#73922,#73923,#73924,#73925,#73926,#73927,#73928,
#73929));
#18095=EDGE_LOOP('',(#73930,#73931,#73932,#73933));
#18096=EDGE_LOOP('',(#73934,#73935,#73936,#73937));
#18097=EDGE_LOOP('',(#73938,#73939,#73940,#73941));
#18098=EDGE_LOOP('',(#73942,#73943,#73944,#73945));
#18099=EDGE_LOOP('',(#73946,#73947,#73948,#73949));
#18100=EDGE_LOOP('',(#73950,#73951,#73952,#73953));
#18101=EDGE_LOOP('',(#73954,#73955,#73956,#73957));
#18102=EDGE_LOOP('',(#73958,#73959,#73960,#73961,#73962,#73963,#73964,#73965,
#73966));
#18103=EDGE_LOOP('',(#73967,#73968,#73969,#73970,#73971));
#18104=EDGE_LOOP('',(#73972,#73973,#73974,#73975));
#18105=EDGE_LOOP('',(#73976,#73977,#73978,#73979));
#18106=EDGE_LOOP('',(#73980,#73981,#73982,#73983));
#18107=EDGE_LOOP('',(#73984,#73985,#73986,#73987,#73988));
#18108=EDGE_LOOP('',(#73989,#73990,#73991,#73992));
#18109=EDGE_LOOP('',(#73993,#73994,#73995));
#18110=EDGE_LOOP('',(#73996,#73997,#73998,#73999,#74000,#74001,#74002,#74003,
#74004,#74005));
#18111=EDGE_LOOP('',(#74006,#74007,#74008));
#18112=EDGE_LOOP('',(#74009,#74010,#74011,#74012));
#18113=EDGE_LOOP('',(#74013,#74014,#74015,#74016,#74017));
#18114=EDGE_LOOP('',(#74018,#74019,#74020,#74021));
#18115=EDGE_LOOP('',(#74022,#74023,#74024,#74025));
#18116=EDGE_LOOP('',(#74026,#74027,#74028,#74029));
#18117=EDGE_LOOP('',(#74030,#74031,#74032,#74033,#74034));
#18118=EDGE_LOOP('',(#74035,#74036,#74037,#74038,#74039,#74040,#74041,#74042,
#74043,#74044,#74045));
#18119=EDGE_LOOP('',(#74046,#74047,#74048));
#18120=EDGE_LOOP('',(#74049,#74050,#74051,#74052));
#18121=EDGE_LOOP('',(#74053,#74054,#74055,#74056,#74057));
#18122=EDGE_LOOP('',(#74058,#74059,#74060,#74061));
#18123=EDGE_LOOP('',(#74062,#74063,#74064,#74065));
#18124=EDGE_LOOP('',(#74066,#74067,#74068,#74069));
#18125=EDGE_LOOP('',(#74070,#74071,#74072,#74073,#74074));
#18126=EDGE_LOOP('',(#74075,#74076,#74077,#74078));
#18127=EDGE_LOOP('',(#74079,#74080,#74081,#74082,#74083,#74084,#74085));
#18128=EDGE_LOOP('',(#74086,#74087,#74088));
#18129=EDGE_LOOP('',(#74089,#74090,#74091,#74092,#74093));
#18130=EDGE_LOOP('',(#74094,#74095,#74096,#74097));
#18131=EDGE_LOOP('',(#74098,#74099,#74100,#74101));
#18132=EDGE_LOOP('',(#74102,#74103,#74104,#74105));
#18133=EDGE_LOOP('',(#74106,#74107,#74108,#74109));
#18134=EDGE_LOOP('',(#74110,#74111,#74112,#74113,#74114));
#18135=EDGE_LOOP('',(#74115,#74116,#74117,#74118));
#18136=EDGE_LOOP('',(#74119,#74120,#74121,#74122));
#18137=EDGE_LOOP('',(#74123,#74124,#74125,#74126));
#18138=EDGE_LOOP('',(#74127,#74128,#74129,#74130));
#18139=EDGE_LOOP('',(#74131,#74132,#74133,#74134));
#18140=EDGE_LOOP('',(#74135,#74136,#74137,#74138));
#18141=EDGE_LOOP('',(#74139,#74140,#74141,#74142));
#18142=EDGE_LOOP('',(#74143,#74144,#74145,#74146));
#18143=EDGE_LOOP('',(#74147,#74148,#74149,#74150));
#18144=EDGE_LOOP('',(#74151,#74152,#74153,#74154));
#18145=EDGE_LOOP('',(#74155,#74156,#74157,#74158));
#18146=EDGE_LOOP('',(#74159,#74160,#74161,#74162));
#18147=EDGE_LOOP('',(#74163,#74164,#74165,#74166));
#18148=EDGE_LOOP('',(#74167,#74168,#74169,#74170));
#18149=EDGE_LOOP('',(#74171,#74172,#74173,#74174));
#18150=EDGE_LOOP('',(#74175,#74176,#74177,#74178));
#18151=EDGE_LOOP('',(#74179,#74180,#74181,#74182));
#18152=EDGE_LOOP('',(#74183,#74184,#74185,#74186));
#18153=EDGE_LOOP('',(#74187,#74188,#74189,#74190));
#18154=EDGE_LOOP('',(#74191,#74192,#74193,#74194));
#18155=EDGE_LOOP('',(#74195,#74196,#74197,#74198));
#18156=EDGE_LOOP('',(#74199,#74200,#74201,#74202));
#18157=EDGE_LOOP('',(#74203,#74204,#74205,#74206));
#18158=EDGE_LOOP('',(#74207,#74208,#74209,#74210));
#18159=EDGE_LOOP('',(#74211,#74212,#74213,#74214));
#18160=EDGE_LOOP('',(#74215,#74216,#74217,#74218));
#18161=EDGE_LOOP('',(#74219,#74220,#74221,#74222));
#18162=EDGE_LOOP('',(#74223,#74224,#74225,#74226));
#18163=EDGE_LOOP('',(#74227,#74228,#74229,#74230));
#18164=EDGE_LOOP('',(#74231,#74232,#74233,#74234));
#18165=EDGE_LOOP('',(#74235,#74236,#74237,#74238));
#18166=EDGE_LOOP('',(#74239,#74240,#74241,#74242));
#18167=EDGE_LOOP('',(#74243,#74244,#74245,#74246));
#18168=EDGE_LOOP('',(#74247,#74248,#74249,#74250));
#18169=EDGE_LOOP('',(#74251,#74252,#74253,#74254));
#18170=EDGE_LOOP('',(#74255,#74256,#74257,#74258));
#18171=EDGE_LOOP('',(#74259,#74260,#74261,#74262));
#18172=EDGE_LOOP('',(#74263,#74264,#74265,#74266));
#18173=EDGE_LOOP('',(#74267,#74268,#74269,#74270));
#18174=EDGE_LOOP('',(#74271,#74272,#74273,#74274));
#18175=EDGE_LOOP('',(#74275,#74276,#74277,#74278));
#18176=EDGE_LOOP('',(#74279,#74280,#74281,#74282));
#18177=EDGE_LOOP('',(#74283,#74284,#74285,#74286));
#18178=EDGE_LOOP('',(#74287,#74288,#74289,#74290));
#18179=EDGE_LOOP('',(#74291,#74292,#74293,#74294));
#18180=EDGE_LOOP('',(#74295,#74296,#74297,#74298));
#18181=EDGE_LOOP('',(#74299,#74300,#74301,#74302));
#18182=EDGE_LOOP('',(#74303,#74304,#74305,#74306));
#18183=EDGE_LOOP('',(#74307,#74308,#74309,#74310));
#18184=EDGE_LOOP('',(#74311,#74312,#74313,#74314));
#18185=EDGE_LOOP('',(#74315,#74316,#74317,#74318));
#18186=EDGE_LOOP('',(#74319,#74320,#74321,#74322));
#18187=EDGE_LOOP('',(#74323,#74324,#74325,#74326));
#18188=EDGE_LOOP('',(#74327,#74328,#74329,#74330));
#18189=EDGE_LOOP('',(#74331,#74332,#74333,#74334));
#18190=EDGE_LOOP('',(#74335,#74336,#74337,#74338));
#18191=EDGE_LOOP('',(#74339,#74340,#74341,#74342));
#18192=EDGE_LOOP('',(#74343,#74344,#74345,#74346));
#18193=EDGE_LOOP('',(#74347,#74348,#74349,#74350));
#18194=EDGE_LOOP('',(#74351,#74352,#74353,#74354));
#18195=EDGE_LOOP('',(#74355,#74356,#74357,#74358));
#18196=EDGE_LOOP('',(#74359,#74360,#74361,#74362));
#18197=EDGE_LOOP('',(#74363,#74364,#74365,#74366));
#18198=EDGE_LOOP('',(#74367,#74368,#74369,#74370));
#18199=EDGE_LOOP('',(#74371,#74372,#74373,#74374));
#18200=EDGE_LOOP('',(#74375,#74376,#74377,#74378));
#18201=EDGE_LOOP('',(#74379,#74380,#74381,#74382));
#18202=EDGE_LOOP('',(#74383,#74384,#74385,#74386));
#18203=EDGE_LOOP('',(#74387,#74388,#74389,#74390));
#18204=EDGE_LOOP('',(#74391,#74392,#74393,#74394));
#18205=EDGE_LOOP('',(#74395,#74396,#74397,#74398));
#18206=EDGE_LOOP('',(#74399,#74400,#74401,#74402));
#18207=EDGE_LOOP('',(#74403,#74404,#74405,#74406));
#18208=EDGE_LOOP('',(#74407,#74408,#74409,#74410));
#18209=EDGE_LOOP('',(#74411,#74412,#74413,#74414));
#18210=EDGE_LOOP('',(#74415,#74416,#74417,#74418));
#18211=EDGE_LOOP('',(#74419,#74420,#74421,#74422));
#18212=EDGE_LOOP('',(#74423,#74424,#74425,#74426));
#18213=EDGE_LOOP('',(#74427,#74428,#74429,#74430));
#18214=EDGE_LOOP('',(#74431,#74432,#74433,#74434));
#18215=EDGE_LOOP('',(#74435,#74436,#74437,#74438));
#18216=EDGE_LOOP('',(#74439,#74440,#74441,#74442));
#18217=EDGE_LOOP('',(#74443,#74444,#74445,#74446));
#18218=EDGE_LOOP('',(#74447,#74448,#74449,#74450));
#18219=EDGE_LOOP('',(#74451,#74452,#74453,#74454));
#18220=EDGE_LOOP('',(#74455,#74456,#74457,#74458));
#18221=EDGE_LOOP('',(#74459,#74460,#74461,#74462));
#18222=EDGE_LOOP('',(#74463,#74464,#74465,#74466));
#18223=EDGE_LOOP('',(#74467,#74468,#74469,#74470));
#18224=EDGE_LOOP('',(#74471,#74472,#74473,#74474));
#18225=EDGE_LOOP('',(#74475,#74476,#74477,#74478));
#18226=EDGE_LOOP('',(#74479,#74480,#74481,#74482));
#18227=EDGE_LOOP('',(#74483,#74484,#74485,#74486));
#18228=EDGE_LOOP('',(#74487,#74488,#74489,#74490));
#18229=EDGE_LOOP('',(#74491,#74492,#74493,#74494));
#18230=EDGE_LOOP('',(#74495,#74496,#74497,#74498));
#18231=EDGE_LOOP('',(#74499,#74500,#74501,#74502));
#18232=EDGE_LOOP('',(#74503,#74504,#74505,#74506));
#18233=EDGE_LOOP('',(#74507,#74508,#74509,#74510));
#18234=EDGE_LOOP('',(#74511,#74512,#74513,#74514));
#18235=EDGE_LOOP('',(#74515,#74516,#74517,#74518));
#18236=EDGE_LOOP('',(#74519,#74520,#74521,#74522));
#18237=EDGE_LOOP('',(#74523,#74524,#74525,#74526));
#18238=EDGE_LOOP('',(#74527,#74528,#74529,#74530));
#18239=EDGE_LOOP('',(#74531,#74532,#74533,#74534));
#18240=EDGE_LOOP('',(#74535,#74536,#74537,#74538));
#18241=EDGE_LOOP('',(#74539,#74540,#74541,#74542));
#18242=EDGE_LOOP('',(#74543,#74544,#74545,#74546));
#18243=EDGE_LOOP('',(#74547,#74548,#74549,#74550));
#18244=EDGE_LOOP('',(#74551,#74552,#74553,#74554));
#18245=EDGE_LOOP('',(#74555,#74556,#74557,#74558));
#18246=EDGE_LOOP('',(#74559,#74560,#74561,#74562));
#18247=EDGE_LOOP('',(#74563,#74564,#74565,#74566));
#18248=EDGE_LOOP('',(#74567,#74568,#74569,#74570));
#18249=EDGE_LOOP('',(#74571,#74572,#74573,#74574));
#18250=EDGE_LOOP('',(#74575,#74576,#74577,#74578));
#18251=EDGE_LOOP('',(#74579,#74580,#74581,#74582));
#18252=EDGE_LOOP('',(#74583,#74584,#74585,#74586));
#18253=EDGE_LOOP('',(#74587,#74588,#74589,#74590));
#18254=EDGE_LOOP('',(#74591,#74592,#74593,#74594));
#18255=EDGE_LOOP('',(#74595,#74596,#74597,#74598));
#18256=EDGE_LOOP('',(#74599,#74600,#74601,#74602));
#18257=EDGE_LOOP('',(#74603,#74604,#74605,#74606));
#18258=EDGE_LOOP('',(#74607,#74608,#74609,#74610));
#18259=EDGE_LOOP('',(#74611,#74612,#74613,#74614));
#18260=EDGE_LOOP('',(#74615,#74616,#74617,#74618));
#18261=EDGE_LOOP('',(#74619,#74620,#74621,#74622));
#18262=EDGE_LOOP('',(#74623,#74624,#74625,#74626));
#18263=EDGE_LOOP('',(#74627,#74628,#74629,#74630));
#18264=EDGE_LOOP('',(#74631,#74632,#74633,#74634));
#18265=EDGE_LOOP('',(#74635,#74636,#74637,#74638));
#18266=EDGE_LOOP('',(#74639,#74640,#74641,#74642));
#18267=EDGE_LOOP('',(#74643,#74644,#74645,#74646));
#18268=EDGE_LOOP('',(#74647,#74648,#74649,#74650));
#18269=EDGE_LOOP('',(#74651,#74652,#74653,#74654));
#18270=EDGE_LOOP('',(#74655,#74656,#74657,#74658));
#18271=EDGE_LOOP('',(#74659,#74660,#74661,#74662));
#18272=EDGE_LOOP('',(#74663,#74664,#74665,#74666));
#18273=EDGE_LOOP('',(#74667,#74668,#74669,#74670));
#18274=EDGE_LOOP('',(#74671,#74672,#74673,#74674));
#18275=EDGE_LOOP('',(#74675,#74676,#74677,#74678));
#18276=EDGE_LOOP('',(#74679,#74680,#74681,#74682));
#18277=EDGE_LOOP('',(#74683));
#18278=EDGE_LOOP('',(#74684,#74685,#74686,#74687));
#18279=EDGE_LOOP('',(#74688));
#18280=EDGE_LOOP('',(#74689));
#18281=EDGE_LOOP('',(#74690,#74691,#74692,#74693));
#18282=EDGE_LOOP('',(#74694,#74695,#74696,#74697));
#18283=EDGE_LOOP('',(#74698,#74699,#74700,#74701,#74702,#74703,#74704,#74705,
#74706,#74707,#74708,#74709,#74710,#74711,#74712,#74713,#74714,#74715,#74716,
#74717,#74718,#74719,#74720,#74721,#74722,#74723,#74724,#74725,#74726,#74727,
#74728,#74729,#74730,#74731,#74732,#74733,#74734,#74735,#74736,#74737,#74738,
#74739,#74740,#74741,#74742,#74743,#74744,#74745,#74746,#74747,#74748,#74749));
#18284=EDGE_LOOP('',(#74750,#74751,#74752,#74753));
#18285=EDGE_LOOP('',(#74754,#74755,#74756,#74757));
#18286=EDGE_LOOP('',(#74758,#74759,#74760,#74761));
#18287=EDGE_LOOP('',(#74762,#74763,#74764,#74765));
#18288=EDGE_LOOP('',(#74766,#74767,#74768,#74769));
#18289=EDGE_LOOP('',(#74770,#74771,#74772,#74773));
#18290=EDGE_LOOP('',(#74774,#74775,#74776,#74777));
#18291=EDGE_LOOP('',(#74778,#74779,#74780,#74781));
#18292=EDGE_LOOP('',(#74782,#74783,#74784,#74785));
#18293=EDGE_LOOP('',(#74786,#74787,#74788,#74789));
#18294=EDGE_LOOP('',(#74790,#74791,#74792,#74793));
#18295=EDGE_LOOP('',(#74794,#74795,#74796,#74797));
#18296=EDGE_LOOP('',(#74798,#74799,#74800,#74801));
#18297=EDGE_LOOP('',(#74802,#74803,#74804,#74805));
#18298=EDGE_LOOP('',(#74806,#74807,#74808,#74809));
#18299=EDGE_LOOP('',(#74810,#74811,#74812,#74813));
#18300=EDGE_LOOP('',(#74814,#74815,#74816,#74817));
#18301=EDGE_LOOP('',(#74818,#74819,#74820,#74821));
#18302=EDGE_LOOP('',(#74822,#74823,#74824,#74825));
#18303=EDGE_LOOP('',(#74826,#74827,#74828,#74829));
#18304=EDGE_LOOP('',(#74830,#74831,#74832,#74833));
#18305=EDGE_LOOP('',(#74834,#74835,#74836,#74837));
#18306=EDGE_LOOP('',(#74838,#74839,#74840,#74841));
#18307=EDGE_LOOP('',(#74842,#74843,#74844,#74845));
#18308=EDGE_LOOP('',(#74846,#74847,#74848,#74849));
#18309=EDGE_LOOP('',(#74850,#74851,#74852,#74853));
#18310=EDGE_LOOP('',(#74854,#74855,#74856,#74857));
#18311=EDGE_LOOP('',(#74858,#74859,#74860,#74861));
#18312=EDGE_LOOP('',(#74862,#74863,#74864,#74865));
#18313=EDGE_LOOP('',(#74866,#74867,#74868,#74869));
#18314=EDGE_LOOP('',(#74870,#74871,#74872,#74873));
#18315=EDGE_LOOP('',(#74874,#74875,#74876,#74877));
#18316=EDGE_LOOP('',(#74878,#74879,#74880,#74881));
#18317=EDGE_LOOP('',(#74882,#74883,#74884,#74885));
#18318=EDGE_LOOP('',(#74886,#74887,#74888,#74889));
#18319=EDGE_LOOP('',(#74890,#74891,#74892,#74893));
#18320=EDGE_LOOP('',(#74894,#74895,#74896,#74897));
#18321=EDGE_LOOP('',(#74898,#74899,#74900,#74901));
#18322=EDGE_LOOP('',(#74902,#74903,#74904,#74905));
#18323=EDGE_LOOP('',(#74906,#74907,#74908,#74909));
#18324=EDGE_LOOP('',(#74910,#74911,#74912,#74913));
#18325=EDGE_LOOP('',(#74914,#74915,#74916,#74917));
#18326=EDGE_LOOP('',(#74918,#74919,#74920,#74921));
#18327=EDGE_LOOP('',(#74922,#74923,#74924,#74925));
#18328=EDGE_LOOP('',(#74926,#74927,#74928,#74929));
#18329=EDGE_LOOP('',(#74930,#74931,#74932,#74933));
#18330=EDGE_LOOP('',(#74934,#74935,#74936,#74937));
#18331=EDGE_LOOP('',(#74938,#74939,#74940,#74941));
#18332=EDGE_LOOP('',(#74942,#74943,#74944,#74945));
#18333=EDGE_LOOP('',(#74946,#74947,#74948,#74949));
#18334=EDGE_LOOP('',(#74950,#74951,#74952,#74953));
#18335=EDGE_LOOP('',(#74954,#74955,#74956,#74957));
#18336=EDGE_LOOP('',(#74958,#74959,#74960,#74961));
#18337=EDGE_LOOP('',(#74962,#74963,#74964,#74965));
#18338=EDGE_LOOP('',(#74966,#74967,#74968,#74969));
#18339=EDGE_LOOP('',(#74970,#74971,#74972,#74973));
#18340=EDGE_LOOP('',(#74974,#74975,#74976,#74977));
#18341=EDGE_LOOP('',(#74978,#74979,#74980,#74981));
#18342=EDGE_LOOP('',(#74982,#74983,#74984,#74985));
#18343=EDGE_LOOP('',(#74986,#74987,#74988,#74989));
#18344=EDGE_LOOP('',(#74990,#74991,#74992,#74993));
#18345=EDGE_LOOP('',(#74994,#74995,#74996,#74997));
#18346=EDGE_LOOP('',(#74998,#74999,#75000,#75001));
#18347=EDGE_LOOP('',(#75002,#75003,#75004,#75005));
#18348=EDGE_LOOP('',(#75006,#75007,#75008,#75009));
#18349=EDGE_LOOP('',(#75010,#75011,#75012,#75013));
#18350=EDGE_LOOP('',(#75014,#75015,#75016,#75017));
#18351=EDGE_LOOP('',(#75018,#75019,#75020,#75021,#75022,#75023,#75024,#75025,
#75026,#75027,#75028,#75029,#75030,#75031,#75032,#75033,#75034,#75035,#75036,
#75037,#75038,#75039,#75040,#75041));
#18352=EDGE_LOOP('',(#75042,#75043,#75044,#75045,#75046,#75047,#75048,#75049));
#18353=EDGE_LOOP('',(#75050,#75051,#75052,#75053,#75054,#75055,#75056,#75057));
#18354=EDGE_LOOP('',(#75058,#75059,#75060,#75061,#75062,#75063,#75064,#75065));
#18355=EDGE_LOOP('',(#75066,#75067,#75068,#75069,#75070,#75071,#75072,#75073));
#18356=EDGE_LOOP('',(#75074,#75075,#75076,#75077,#75078,#75079,#75080,#75081));
#18357=EDGE_LOOP('',(#75082,#75083,#75084,#75085,#75086,#75087,#75088,#75089));
#18358=EDGE_LOOP('',(#75090,#75091,#75092,#75093,#75094,#75095,#75096,#75097));
#18359=EDGE_LOOP('',(#75098,#75099,#75100,#75101,#75102,#75103,#75104,#75105));
#18360=EDGE_LOOP('',(#75106,#75107,#75108,#75109,#75110,#75111,#75112,#75113));
#18361=EDGE_LOOP('',(#75114,#75115,#75116,#75117,#75118,#75119,#75120,#75121));
#18362=EDGE_LOOP('',(#75122,#75123,#75124,#75125,#75126,#75127,#75128,#75129,
#75130,#75131));
#18363=EDGE_LOOP('',(#75132,#75133,#75134,#75135,#75136,#75137,#75138,#75139,
#75140,#75141));
#18364=EDGE_LOOP('',(#75142,#75143,#75144,#75145,#75146,#75147,#75148,#75149));
#18365=EDGE_LOOP('',(#75150,#75151,#75152,#75153,#75154,#75155,#75156,#75157));
#18366=EDGE_LOOP('',(#75158,#75159,#75160,#75161,#75162,#75163,#75164,#75165));
#18367=EDGE_LOOP('',(#75166,#75167,#75168,#75169,#75170,#75171,#75172,#75173));
#18368=EDGE_LOOP('',(#75174,#75175,#75176,#75177,#75178,#75179,#75180,#75181));
#18369=EDGE_LOOP('',(#75182,#75183,#75184,#75185,#75186,#75187));
#18370=EDGE_LOOP('',(#75188,#75189,#75190,#75191,#75192,#75193,#75194,#75195));
#18371=EDGE_LOOP('',(#75196,#75197,#75198,#75199,#75200,#75201,#75202,#75203));
#18372=EDGE_LOOP('',(#75204,#75205,#75206,#75207,#75208,#75209,#75210,#75211));
#18373=EDGE_LOOP('',(#75212,#75213,#75214,#75215,#75216,#75217,#75218,#75219,
#75220,#75221));
#18374=EDGE_LOOP('',(#75222,#75223,#75224,#75225,#75226,#75227,#75228,#75229,
#75230,#75231));
#18375=EDGE_LOOP('',(#75232,#75233,#75234,#75235,#75236,#75237,#75238,#75239));
#18376=EDGE_LOOP('',(#75240,#75241,#75242,#75243,#75244,#75245,#75246,#75247));
#18377=EDGE_LOOP('',(#75248,#75249,#75250,#75251,#75252,#75253));
#18378=EDGE_LOOP('',(#75254,#75255,#75256,#75257,#75258,#75259,#75260,#75261,
#75262,#75263));
#18379=EDGE_LOOP('',(#75264,#75265,#75266,#75267,#75268,#75269,#75270,#75271));
#18380=EDGE_LOOP('',(#75272,#75273,#75274,#75275,#75276,#75277,#75278,#75279));
#18381=EDGE_LOOP('',(#75280,#75281,#75282,#75283,#75284,#75285,#75286,#75287,
#75288));
#18382=EDGE_LOOP('',(#75289,#75290,#75291,#75292,#75293,#75294,#75295,#75296));
#18383=EDGE_LOOP('',(#75297,#75298,#75299,#75300,#75301,#75302,#75303,#75304,
#75305));
#18384=EDGE_LOOP('',(#75306,#75307,#75308,#75309,#75310,#75311,#75312,#75313));
#18385=EDGE_LOOP('',(#75314,#75315,#75316,#75317,#75318,#75319,#75320,#75321,
#75322,#75323));
#18386=EDGE_LOOP('',(#75324,#75325,#75326,#75327,#75328,#75329,#75330,#75331));
#18387=EDGE_LOOP('',(#75332,#75333,#75334,#75335,#75336,#75337,#75338,#75339));
#18388=EDGE_LOOP('',(#75340,#75341,#75342,#75343,#75344,#75345,#75346,#75347));
#18389=EDGE_LOOP('',(#75348,#75349,#75350,#75351,#75352,#75353,#75354,#75355));
#18390=EDGE_LOOP('',(#75356,#75357,#75358,#75359,#75360,#75361,#75362,#75363));
#18391=EDGE_LOOP('',(#75364,#75365,#75366,#75367,#75368,#75369,#75370,#75371));
#18392=EDGE_LOOP('',(#75372,#75373,#75374,#75375,#75376,#75377,#75378,#75379));
#18393=EDGE_LOOP('',(#75380,#75381,#75382,#75383,#75384,#75385,#75386,#75387));
#18394=EDGE_LOOP('',(#75388,#75389,#75390,#75391,#75392,#75393,#75394,#75395));
#18395=EDGE_LOOP('',(#75396,#75397,#75398,#75399,#75400,#75401,#75402,#75403));
#18396=EDGE_LOOP('',(#75404,#75405,#75406,#75407,#75408,#75409,#75410,#75411,
#75412,#75413));
#18397=EDGE_LOOP('',(#75414,#75415,#75416,#75417,#75418,#75419,#75420,#75421,
#75422,#75423));
#18398=EDGE_LOOP('',(#75424,#75425,#75426,#75427,#75428,#75429,#75430,#75431));
#18399=EDGE_LOOP('',(#75432,#75433,#75434,#75435,#75436,#75437,#75438,#75439));
#18400=EDGE_LOOP('',(#75440,#75441,#75442,#75443,#75444,#75445,#75446,#75447));
#18401=EDGE_LOOP('',(#75448,#75449,#75450,#75451,#75452,#75453,#75454,#75455));
#18402=EDGE_LOOP('',(#75456,#75457,#75458,#75459,#75460,#75461,#75462,#75463));
#18403=EDGE_LOOP('',(#75464,#75465,#75466,#75467,#75468,#75469));
#18404=EDGE_LOOP('',(#75470,#75471,#75472,#75473,#75474,#75475,#75476,#75477));
#18405=EDGE_LOOP('',(#75478,#75479,#75480,#75481,#75482,#75483,#75484,#75485));
#18406=EDGE_LOOP('',(#75486,#75487,#75488,#75489,#75490,#75491,#75492,#75493));
#18407=EDGE_LOOP('',(#75494,#75495,#75496,#75497,#75498,#75499,#75500,#75501,
#75502,#75503));
#18408=EDGE_LOOP('',(#75504,#75505,#75506,#75507,#75508,#75509,#75510,#75511,
#75512,#75513));
#18409=EDGE_LOOP('',(#75514,#75515,#75516,#75517,#75518,#75519,#75520,#75521));
#18410=EDGE_LOOP('',(#75522,#75523,#75524,#75525,#75526,#75527,#75528,#75529));
#18411=EDGE_LOOP('',(#75530,#75531,#75532,#75533,#75534,#75535));
#18412=EDGE_LOOP('',(#75536,#75537,#75538,#75539,#75540,#75541,#75542,#75543,
#75544,#75545));
#18413=EDGE_LOOP('',(#75546,#75547,#75548,#75549,#75550,#75551,#75552,#75553));
#18414=EDGE_LOOP('',(#75554,#75555,#75556,#75557,#75558,#75559,#75560,#75561));
#18415=EDGE_LOOP('',(#75562,#75563,#75564,#75565,#75566,#75567,#75568,#75569,
#75570));
#18416=EDGE_LOOP('',(#75571,#75572,#75573,#75574,#75575,#75576,#75577,#75578));
#18417=EDGE_LOOP('',(#75579,#75580,#75581,#75582,#75583,#75584,#75585,#75586,
#75587));
#18418=EDGE_LOOP('',(#75588,#75589,#75590,#75591,#75592,#75593,#75594,#75595));
#18419=EDGE_LOOP('',(#75596,#75597,#75598,#75599,#75600,#75601,#75602,#75603,
#75604,#75605));
#18420=EDGE_LOOP('',(#75606,#75607,#75608,#75609));
#18421=EDGE_LOOP('',(#75610,#75611,#75612,#75613));
#18422=EDGE_LOOP('',(#75614,#75615,#75616,#75617));
#18423=EDGE_LOOP('',(#75618,#75619,#75620,#75621));
#18424=EDGE_LOOP('',(#75622,#75623,#75624,#75625));
#18425=EDGE_LOOP('',(#75626,#75627,#75628,#75629));
#18426=EDGE_LOOP('',(#75630,#75631,#75632,#75633));
#18427=EDGE_LOOP('',(#75634,#75635,#75636,#75637));
#18428=EDGE_LOOP('',(#75638,#75639,#75640,#75641));
#18429=EDGE_LOOP('',(#75642,#75643,#75644));
#18430=EDGE_LOOP('',(#75645,#75646,#75647));
#18431=EDGE_LOOP('',(#75648,#75649,#75650));
#18432=EDGE_LOOP('',(#75651,#75652,#75653,#75654));
#18433=EDGE_LOOP('',(#75655,#75656,#75657,#75658));
#18434=EDGE_LOOP('',(#75659,#75660,#75661,#75662));
#18435=EDGE_LOOP('',(#75663,#75664,#75665,#75666));
#18436=EDGE_LOOP('',(#75667,#75668,#75669,#75670));
#18437=EDGE_LOOP('',(#75671,#75672,#75673,#75674));
#18438=EDGE_LOOP('',(#75675,#75676,#75677,#75678,#75679,#75680,#75681,#75682,
#75683,#75684,#75685,#75686,#75687,#75688,#75689,#75690));
#18439=EDGE_LOOP('',(#75691,#75692,#75693,#75694,#75695,#75696,#75697,#75698,
#75699,#75700,#75701,#75702));
#18440=EDGE_LOOP('',(#75703,#75704,#75705,#75706));
#18441=EDGE_LOOP('',(#75707,#75708,#75709,#75710));
#18442=EDGE_LOOP('',(#75711,#75712,#75713,#75714,#75715,#75716,#75717,#75718,
#75719,#75720,#75721,#75722));
#18443=EDGE_LOOP('',(#75723,#75724,#75725,#75726));
#18444=EDGE_LOOP('',(#75727,#75728,#75729,#75730));
#18445=EDGE_LOOP('',(#75731,#75732,#75733,#75734));
#18446=EDGE_LOOP('',(#75735,#75736,#75737,#75738));
#18447=EDGE_LOOP('',(#75739,#75740,#75741,#75742));
#18448=EDGE_LOOP('',(#75743,#75744,#75745,#75746));
#18449=EDGE_LOOP('',(#75747,#75748,#75749,#75750,#75751));
#18450=EDGE_LOOP('',(#75752,#75753,#75754,#75755,#75756));
#18451=EDGE_LOOP('',(#75757,#75758,#75759,#75760,#75761));
#18452=EDGE_LOOP('',(#75762,#75763,#75764,#75765,#75766));
#18453=EDGE_LOOP('',(#75767,#75768,#75769,#75770,#75771));
#18454=EDGE_LOOP('',(#75772,#75773,#75774,#75775,#75776,#75777,#75778,#75779));
#18455=EDGE_LOOP('',(#75780,#75781,#75782,#75783,#75784));
#18456=EDGE_LOOP('',(#75785,#75786,#75787,#75788,#75789));
#18457=EDGE_LOOP('',(#75790,#75791,#75792,#75793,#75794,#75795,#75796,#75797));
#18458=EDGE_LOOP('',(#75798,#75799,#75800,#75801,#75802));
#18459=EDGE_LOOP('',(#75803,#75804,#75805,#75806,#75807,#75808,#75809,#75810));
#18460=EDGE_LOOP('',(#75811,#75812,#75813,#75814,#75815,#75816,#75817,#75818,
#75819,#75820,#75821,#75822,#75823,#75824,#75825,#75826));
#18461=EDGE_LOOP('',(#75827,#75828,#75829,#75830,#75831,#75832,#75833,#75834,
#75835,#75836,#75837,#75838,#75839,#75840,#75841,#75842));
#18462=EDGE_LOOP('',(#75843,#75844,#75845,#75846));
#18463=EDGE_LOOP('',(#75847,#75848,#75849,#75850));
#18464=EDGE_LOOP('',(#75851,#75852,#75853,#75854));
#18465=EDGE_LOOP('',(#75855,#75856,#75857,#75858));
#18466=EDGE_LOOP('',(#75859,#75860,#75861,#75862));
#18467=EDGE_LOOP('',(#75863,#75864,#75865,#75866));
#18468=EDGE_LOOP('',(#75867,#75868,#75869,#75870));
#18469=EDGE_LOOP('',(#75871,#75872,#75873,#75874));
#18470=EDGE_LOOP('',(#75875,#75876,#75877,#75878));
#18471=EDGE_LOOP('',(#75879,#75880,#75881,#75882));
#18472=EDGE_LOOP('',(#75883,#75884,#75885,#75886));
#18473=EDGE_LOOP('',(#75887,#75888,#75889,#75890,#75891,#75892,#75893,#75894));
#18474=EDGE_LOOP('',(#75895,#75896,#75897,#75898));
#18475=EDGE_LOOP('',(#75899,#75900,#75901,#75902,#75903,#75904,#75905,#75906));
#18476=EDGE_LOOP('',(#75907,#75908,#75909,#75910,#75911,#75912,#75913,#75914,
#75915,#75916,#75917,#75918));
#18477=EDGE_LOOP('',(#75919,#75920,#75921,#75922));
#18478=EDGE_LOOP('',(#75923,#75924,#75925,#75926,#75927,#75928));
#18479=EDGE_LOOP('',(#75929,#75930,#75931,#75932,#75933,#75934,#75935,#75936,
#75937,#75938,#75939,#75940,#75941,#75942,#75943,#75944,#75945,#75946));
#18480=EDGE_LOOP('',(#75947,#75948,#75949,#75950,#75951,#75952));
#18481=EDGE_LOOP('',(#75953,#75954,#75955,#75956,#75957,#75958,#75959,#75960,
#75961,#75962,#75963,#75964,#75965,#75966,#75967,#75968));
#18482=EDGE_LOOP('',(#75969,#75970));
#18483=EDGE_LOOP('',(#75971,#75972));
#18484=EDGE_LOOP('',(#75973,#75974,#75975,#75976,#75977,#75978,#75979,#75980,
#75981,#75982,#75983,#75984));
#18485=EDGE_LOOP('',(#75985,#75986));
#18486=EDGE_LOOP('',(#75987,#75988));
#18487=EDGE_LOOP('',(#75989,#75990));
#18488=EDGE_LOOP('',(#75991,#75992));
#18489=EDGE_LOOP('',(#75993,#75994));
#18490=EDGE_LOOP('',(#75995,#75996,#75997));
#18491=EDGE_LOOP('',(#75998,#75999,#76000,#76001));
#18492=EDGE_LOOP('',(#76002,#76003,#76004,#76005));
#18493=EDGE_LOOP('',(#76006,#76007,#76008,#76009));
#18494=EDGE_LOOP('',(#76010,#76011,#76012,#76013));
#18495=EDGE_LOOP('',(#76014,#76015,#76016,#76017,#76018,#76019));
#18496=EDGE_LOOP('',(#76020,#76021,#76022));
#18497=EDGE_LOOP('',(#76023,#76024,#76025,#76026,#76027,#76028,#76029,#76030));
#18498=EDGE_LOOP('',(#76031,#76032,#76033));
#18499=EDGE_LOOP('',(#76034,#76035,#76036,#76037,#76038,#76039,#76040,#76041,
#76042,#76043,#76044,#76045,#76046,#76047,#76048,#76049,#76050,#76051,#76052,
#76053,#76054,#76055));
#18500=EDGE_LOOP('',(#76056,#76057,#76058,#76059,#76060,#76061));
#18501=EDGE_LOOP('',(#76062,#76063,#76064,#76065));
#18502=EDGE_LOOP('',(#76066,#76067,#76068,#76069));
#18503=EDGE_LOOP('',(#76070,#76071,#76072,#76073));
#18504=EDGE_LOOP('',(#76074,#76075,#76076,#76077));
#18505=EDGE_LOOP('',(#76078,#76079,#76080,#76081));
#18506=EDGE_LOOP('',(#76082,#76083,#76084,#76085));
#18507=EDGE_LOOP('',(#76086,#76087,#76088,#76089));
#18508=EDGE_LOOP('',(#76090));
#18509=EDGE_LOOP('',(#76091,#76092,#76093,#76094,#76095,#76096));
#18510=EDGE_LOOP('',(#76097));
#18511=EDGE_LOOP('',(#76098,#76099,#76100,#76101,#76102));
#18512=EDGE_LOOP('',(#76103,#76104,#76105,#76106,#76107,#76108));
#18513=EDGE_LOOP('',(#76109));
#18514=EDGE_LOOP('',(#76110,#76111,#76112));
#18515=EDGE_LOOP('',(#76113,#76114,#76115));
#18516=EDGE_LOOP('',(#76116,#76117,#76118,#76119));
#18517=EDGE_LOOP('',(#76120,#76121,#76122,#76123,#76124,#76125,#76126,#76127));
#18518=EDGE_LOOP('',(#76128,#76129,#76130));
#18519=EDGE_LOOP('',(#76131,#76132,#76133));
#18520=EDGE_LOOP('',(#76134,#76135,#76136,#76137));
#18521=EDGE_LOOP('',(#76138,#76139,#76140,#76141));
#18522=EDGE_LOOP('',(#76142,#76143,#76144,#76145));
#18523=EDGE_LOOP('',(#76146,#76147,#76148,#76149));
#18524=EDGE_LOOP('',(#76150,#76151,#76152,#76153));
#18525=EDGE_LOOP('',(#76154,#76155,#76156,#76157));
#18526=EDGE_LOOP('',(#76158,#76159,#76160,#76161));
#18527=EDGE_LOOP('',(#76162,#76163,#76164,#76165,#76166,#76167,#76168,#76169,
#76170,#76171,#76172,#76173,#76174,#76175,#76176,#76177,#76178,#76179));
#18528=EDGE_LOOP('',(#76180,#76181,#76182,#76183,#76184,#76185,#76186,#76187,
#76188,#76189,#76190,#76191,#76192,#76193,#76194,#76195,#76196,#76197,#76198,
#76199));
#18529=EDGE_LOOP('',(#76200,#76201,#76202,#76203,#76204,#76205,#76206,#76207,
#76208,#76209,#76210,#76211,#76212,#76213,#76214,#76215,#76216));
#18530=EDGE_LOOP('',(#76217,#76218,#76219,#76220,#76221,#76222,#76223,#76224,
#76225,#76226,#76227,#76228,#76229,#76230,#76231,#76232));
#18531=EDGE_LOOP('',(#76233,#76234,#76235,#76236,#76237,#76238,#76239,#76240,
#76241,#76242));
#18532=EDGE_LOOP('',(#76243,#76244,#76245,#76246,#76247,#76248,#76249,#76250));
#18533=EDGE_LOOP('',(#76251,#76252,#76253,#76254,#76255,#76256,#76257,#76258));
#18534=EDGE_LOOP('',(#76259,#76260,#76261,#76262,#76263,#76264,#76265,#76266));
#18535=EDGE_LOOP('',(#76267,#76268,#76269,#76270,#76271,#76272,#76273,#76274,
#76275));
#18536=EDGE_LOOP('',(#76276,#76277,#76278,#76279,#76280,#76281,#76282,#76283));
#18537=EDGE_LOOP('',(#76284,#76285,#76286,#76287,#76288,#76289,#76290,#76291));
#18538=EDGE_LOOP('',(#76292,#76293,#76294,#76295,#76296,#76297,#76298,#76299));
#18539=EDGE_LOOP('',(#76300,#76301,#76302,#76303,#76304,#76305,#76306,#76307));
#18540=EDGE_LOOP('',(#76308,#76309,#76310,#76311,#76312,#76313,#76314,#76315));
#18541=EDGE_LOOP('',(#76316,#76317,#76318,#76319,#76320,#76321,#76322,#76323,
#76324,#76325));
#18542=EDGE_LOOP('',(#76326,#76327,#76328,#76329,#76330,#76331,#76332,#76333));
#18543=EDGE_LOOP('',(#76334,#76335,#76336,#76337,#76338,#76339,#76340,#76341));
#18544=EDGE_LOOP('',(#76342,#76343,#76344,#76345,#76346,#76347,#76348,#76349,
#76350,#76351));
#18545=EDGE_LOOP('',(#76352,#76353,#76354,#76355,#76356,#76357,#76358,#76359,
#76360,#76361));
#18546=EDGE_LOOP('',(#76362,#76363,#76364,#76365,#76366,#76367,#76368,#76369));
#18547=EDGE_LOOP('',(#76370,#76371,#76372,#76373,#76374,#76375,#76376,#76377));
#18548=EDGE_LOOP('',(#76378,#76379,#76380,#76381,#76382,#76383,#76384,#76385));
#18549=EDGE_LOOP('',(#76386,#76387,#76388,#76389,#76390,#76391,#76392,#76393));
#18550=EDGE_LOOP('',(#76394,#76395,#76396,#76397,#76398,#76399,#76400,#76401,
#76402));
#18551=EDGE_LOOP('',(#76403,#76404,#76405,#76406,#76407,#76408,#76409,#76410));
#18552=EDGE_LOOP('',(#76411,#76412,#76413,#76414,#76415,#76416,#76417,#76418,
#76419,#76420));
#18553=EDGE_LOOP('',(#76421,#76422,#76423,#76424,#76425,#76426,#76427,#76428));
#18554=EDGE_LOOP('',(#76429,#76430,#76431,#76432,#76433,#76434,#76435,#76436,
#76437,#76438));
#18555=EDGE_LOOP('',(#76439,#76440,#76441,#76442,#76443,#76444,#76445,#76446));
#18556=EDGE_LOOP('',(#76447,#76448,#76449,#76450,#76451,#76452,#76453,#76454));
#18557=EDGE_LOOP('',(#76455,#76456,#76457,#76458,#76459,#76460,#76461,#76462));
#18558=EDGE_LOOP('',(#76463,#76464,#76465,#76466,#76467,#76468,#76469,#76470));
#18559=EDGE_LOOP('',(#76471,#76472,#76473,#76474,#76475,#76476));
#18560=EDGE_LOOP('',(#76477,#76478,#76479,#76480,#76481,#76482));
#18561=EDGE_LOOP('',(#76483,#76484,#76485,#76486,#76487,#76488,#76489,#76490,
#76491,#76492,#76493,#76494,#76495,#76496,#76497,#76498,#76499,#76500,#76501,
#76502,#76503,#76504,#76505,#76506,#76507,#76508,#76509,#76510,#76511,#76512,
#76513,#76514,#76515,#76516,#76517,#76518,#76519,#76520,#76521,#76522,#76523,
#76524,#76525,#76526,#76527,#76528,#76529,#76530,#76531,#76532,#76533,#76534,
#76535,#76536,#76537,#76538,#76539,#76540,#76541,#76542,#76543,#76544,#76545,
#76546,#76547));
#18562=EDGE_LOOP('',(#76548,#76549,#76550,#76551,#76552,#76553,#76554,#76555,
#76556,#76557));
#18563=EDGE_LOOP('',(#76558,#76559,#76560,#76561,#76562,#76563,#76564,#76565));
#18564=EDGE_LOOP('',(#76566,#76567,#76568,#76569,#76570,#76571,#76572,#76573));
#18565=EDGE_LOOP('',(#76574,#76575,#76576,#76577,#76578,#76579,#76580,#76581));
#18566=EDGE_LOOP('',(#76582,#76583,#76584,#76585,#76586,#76587,#76588,#76589,
#76590));
#18567=EDGE_LOOP('',(#76591,#76592,#76593,#76594,#76595,#76596,#76597,#76598));
#18568=EDGE_LOOP('',(#76599,#76600,#76601,#76602,#76603,#76604,#76605,#76606));
#18569=EDGE_LOOP('',(#76607,#76608,#76609,#76610,#76611,#76612,#76613,#76614));
#18570=EDGE_LOOP('',(#76615,#76616,#76617,#76618,#76619,#76620,#76621,#76622));
#18571=EDGE_LOOP('',(#76623,#76624,#76625,#76626,#76627,#76628,#76629,#76630));
#18572=EDGE_LOOP('',(#76631,#76632,#76633,#76634,#76635,#76636,#76637,#76638,
#76639,#76640));
#18573=EDGE_LOOP('',(#76641,#76642,#76643,#76644,#76645,#76646,#76647,#76648));
#18574=EDGE_LOOP('',(#76649,#76650,#76651,#76652,#76653,#76654,#76655,#76656));
#18575=EDGE_LOOP('',(#76657,#76658,#76659,#76660,#76661,#76662,#76663,#76664,
#76665,#76666));
#18576=EDGE_LOOP('',(#76667,#76668,#76669,#76670,#76671,#76672,#76673,#76674,
#76675,#76676));
#18577=EDGE_LOOP('',(#76677,#76678,#76679,#76680,#76681,#76682,#76683,#76684));
#18578=EDGE_LOOP('',(#76685,#76686,#76687,#76688,#76689,#76690,#76691,#76692));
#18579=EDGE_LOOP('',(#76693,#76694,#76695,#76696,#76697,#76698,#76699,#76700));
#18580=EDGE_LOOP('',(#76701,#76702,#76703,#76704,#76705,#76706,#76707,#76708));
#18581=EDGE_LOOP('',(#76709,#76710,#76711,#76712,#76713,#76714,#76715,#76716,
#76717));
#18582=EDGE_LOOP('',(#76718,#76719,#76720,#76721,#76722,#76723,#76724,#76725));
#18583=EDGE_LOOP('',(#76726,#76727,#76728,#76729,#76730,#76731,#76732,#76733,
#76734,#76735));
#18584=EDGE_LOOP('',(#76736,#76737,#76738,#76739,#76740,#76741,#76742,#76743));
#18585=EDGE_LOOP('',(#76744,#76745,#76746,#76747,#76748,#76749,#76750,#76751,
#76752,#76753));
#18586=EDGE_LOOP('',(#76754,#76755,#76756,#76757,#76758,#76759,#76760,#76761));
#18587=EDGE_LOOP('',(#76762,#76763,#76764,#76765,#76766,#76767,#76768,#76769));
#18588=EDGE_LOOP('',(#76770,#76771,#76772,#76773,#76774,#76775,#76776,#76777));
#18589=EDGE_LOOP('',(#76778,#76779,#76780,#76781,#76782,#76783,#76784,#76785));
#18590=EDGE_LOOP('',(#76786,#76787,#76788,#76789,#76790,#76791));
#18591=EDGE_LOOP('',(#76792,#76793,#76794,#76795,#76796,#76797));
#18592=EDGE_LOOP('',(#76798,#76799,#76800,#76801));
#18593=EDGE_LOOP('',(#76802,#76803,#76804,#76805));
#18594=EDGE_LOOP('',(#76806,#76807,#76808,#76809));
#18595=EDGE_LOOP('',(#76810,#76811,#76812,#76813));
#18596=EDGE_LOOP('',(#76814,#76815,#76816,#76817));
#18597=EDGE_LOOP('',(#76818,#76819,#76820,#76821));
#18598=EDGE_LOOP('',(#76822,#76823,#76824,#76825));
#18599=EDGE_LOOP('',(#76826,#76827,#76828,#76829));
#18600=EDGE_LOOP('',(#76830,#76831,#76832,#76833));
#18601=EDGE_LOOP('',(#76834,#76835,#76836,#76837,#76838,#76839,#76840,#76841,
#76842,#76843,#76844,#76845,#76846,#76847,#76848,#76849));
#18602=EDGE_LOOP('',(#76850,#76851,#76852,#76853,#76854,#76855,#76856,#76857,
#76858,#76859,#76860,#76861,#76862,#76863,#76864,#76865));
#18603=EDGE_LOOP('',(#76866,#76867,#76868,#76869));
#18604=EDGE_LOOP('',(#76870,#76871,#76872,#76873));
#18605=EDGE_LOOP('',(#76874,#76875,#76876,#76877));
#18606=EDGE_LOOP('',(#76878,#76879,#76880,#76881));
#18607=EDGE_LOOP('',(#76882,#76883,#76884,#76885));
#18608=EDGE_LOOP('',(#76886,#76887,#76888,#76889));
#18609=EDGE_LOOP('',(#76890,#76891,#76892,#76893));
#18610=EDGE_LOOP('',(#76894,#76895,#76896,#76897));
#18611=EDGE_LOOP('',(#76898,#76899,#76900,#76901));
#18612=EDGE_LOOP('',(#76902,#76903,#76904,#76905,#76906));
#18613=EDGE_LOOP('',(#76907,#76908,#76909,#76910,#76911));
#18614=EDGE_LOOP('',(#76912,#76913,#76914,#76915,#76916));
#18615=EDGE_LOOP('',(#76917,#76918,#76919,#76920,#76921));
#18616=EDGE_LOOP('',(#76922,#76923,#76924,#76925,#76926));
#18617=EDGE_LOOP('',(#76927,#76928,#76929,#76930,#76931,#76932,#76933,#76934));
#18618=EDGE_LOOP('',(#76935,#76936,#76937,#76938,#76939));
#18619=EDGE_LOOP('',(#76940,#76941,#76942,#76943,#76944));
#18620=EDGE_LOOP('',(#76945,#76946,#76947,#76948,#76949,#76950,#76951,#76952));
#18621=EDGE_LOOP('',(#76953,#76954,#76955,#76956,#76957));
#18622=EDGE_LOOP('',(#76958,#76959,#76960,#76961,#76962,#76963,#76964,#76965));
#18623=EDGE_LOOP('',(#76966,#76967,#76968,#76969,#76970,#76971,#76972,#76973,
#76974,#76975,#76976,#76977,#76978,#76979,#76980,#76981));
#18624=EDGE_LOOP('',(#76982,#76983,#76984,#76985,#76986,#76987,#76988,#76989,
#76990,#76991,#76992,#76993,#76994,#76995,#76996,#76997));
#18625=EDGE_LOOP('',(#76998,#76999,#77000,#77001,#77002,#77003,#77004,#77005,
#77006,#77007,#77008,#77009,#77010,#77011,#77012,#77013));
#18626=EDGE_LOOP('',(#77014,#77015,#77016,#77017,#77018,#77019,#77020,#77021,
#77022,#77023,#77024,#77025,#77026,#77027,#77028,#77029));
#18627=EDGE_LOOP('',(#77030,#77031,#77032,#77033));
#18628=EDGE_LOOP('',(#77034,#77035,#77036,#77037));
#18629=EDGE_LOOP('',(#77038,#77039,#77040,#77041));
#18630=EDGE_LOOP('',(#77042,#77043,#77044,#77045));
#18631=EDGE_LOOP('',(#77046,#77047,#77048,#77049));
#18632=EDGE_LOOP('',(#77050,#77051,#77052,#77053));
#18633=EDGE_LOOP('',(#77054,#77055,#77056,#77057));
#18634=EDGE_LOOP('',(#77058,#77059,#77060,#77061));
#18635=EDGE_LOOP('',(#77062,#77063,#77064,#77065));
#18636=EDGE_LOOP('',(#77066,#77067,#77068,#77069));
#18637=EDGE_LOOP('',(#77070,#77071,#77072,#77073));
#18638=EDGE_LOOP('',(#77074,#77075,#77076,#77077,#77078,#77079,#77080,#77081));
#18639=EDGE_LOOP('',(#77082,#77083,#77084,#77085));
#18640=EDGE_LOOP('',(#77086,#77087,#77088,#77089,#77090,#77091,#77092,#77093,
#77094,#77095,#77096));
#18641=EDGE_LOOP('',(#77097,#77098,#77099,#77100,#77101,#77102,#77103,#77104,
#77105,#77106,#77107,#77108,#77109,#77110,#77111,#77112,#77113,#77114,#77115,
#77116,#77117,#77118,#77119,#77120,#77121,#77122,#77123,#77124,#77125,#77126,
#77127,#77128,#77129));
#18642=EDGE_LOOP('',(#77130,#77131,#77132,#77133,#77134,#77135,#77136,#77137,
#77138,#77139,#77140,#77141,#77142,#77143,#77144,#77145));
#18643=EDGE_LOOP('',(#77146,#77147,#77148,#77149));
#18644=EDGE_LOOP('',(#77150,#77151,#77152,#77153,#77154,#77155,#77156,#77157));
#18645=EDGE_LOOP('',(#77158,#77159,#77160,#77161,#77162,#77163,#77164,#77165,
#77166,#77167,#77168,#77169,#77170,#77171,#77172,#77173,#77174,#77175));
#18646=EDGE_LOOP('',(#77176,#77177,#77178,#77179,#77180,#77181,#77182,#77183,
#77184,#77185));
#18647=EDGE_LOOP('',(#77186,#77187,#77188,#77189,#77190,#77191,#77192,#77193,
#77194,#77195,#77196,#77197,#77198,#77199,#77200,#77201,#77202,#77203,#77204,
#77205));
#18648=EDGE_LOOP('',(#77206,#77207,#77208,#77209));
#18649=EDGE_LOOP('',(#77210,#77211,#77212,#77213));
#18650=EDGE_LOOP('',(#77214,#77215,#77216,#77217));
#18651=EDGE_LOOP('',(#77218,#77219,#77220,#77221));
#18652=EDGE_LOOP('',(#77222,#77223,#77224,#77225));
#18653=EDGE_LOOP('',(#77226,#77227,#77228,#77229));
#18654=EDGE_LOOP('',(#77230,#77231,#77232,#77233));
#18655=EDGE_LOOP('',(#77234,#77235,#77236,#77237));
#18656=EDGE_LOOP('',(#77238,#77239,#77240,#77241));
#18657=EDGE_LOOP('',(#77242,#77243,#77244,#77245));
#18658=EDGE_LOOP('',(#77246,#77247,#77248,#77249));
#18659=EDGE_LOOP('',(#77250,#77251,#77252,#77253));
#18660=EDGE_LOOP('',(#77254,#77255,#77256,#77257));
#18661=EDGE_LOOP('',(#77258,#77259,#77260,#77261));
#18662=EDGE_LOOP('',(#77262,#77263,#77264,#77265));
#18663=EDGE_LOOP('',(#77266,#77267,#77268,#77269));
#18664=EDGE_LOOP('',(#77270,#77271,#77272,#77273));
#18665=EDGE_LOOP('',(#77274,#77275,#77276,#77277));
#18666=EDGE_LOOP('',(#77278,#77279,#77280,#77281));
#18667=EDGE_LOOP('',(#77282,#77283,#77284,#77285,#77286,#77287,#77288,#77289,
#77290,#77291,#77292,#77293,#77294,#77295,#77296,#77297,#77298,#77299,#77300,
#77301,#77302,#77303,#77304,#77305,#77306,#77307,#77308,#77309,#77310,#77311,
#77312,#77313,#77314,#77315,#77316,#77317,#77318,#77319,#77320,#77321));
#18668=EDGE_LOOP('',(#77322,#77323,#77324,#77325,#77326,#77327,#77328,#77329,
#77330,#77331,#77332,#77333,#77334,#77335,#77336,#77337,#77338,#77339,#77340,
#77341,#77342,#77343,#77344,#77345));
#18669=EDGE_LOOP('',(#77346,#77347,#77348,#77349));
#18670=EDGE_LOOP('',(#77350,#77351,#77352,#77353));
#18671=EDGE_LOOP('',(#77354,#77355,#77356,#77357));
#18672=EDGE_LOOP('',(#77358,#77359,#77360,#77361));
#18673=EDGE_LOOP('',(#77362,#77363,#77364,#77365));
#18674=EDGE_LOOP('',(#77366,#77367,#77368,#77369));
#18675=EDGE_LOOP('',(#77370,#77371,#77372,#77373));
#18676=EDGE_LOOP('',(#77374,#77375,#77376,#77377));
#18677=EDGE_LOOP('',(#77378,#77379,#77380,#77381));
#18678=EDGE_LOOP('',(#77382,#77383,#77384,#77385));
#18679=EDGE_LOOP('',(#77386,#77387,#77388,#77389));
#18680=EDGE_LOOP('',(#77390,#77391,#77392,#77393));
#18681=EDGE_LOOP('',(#77394,#77395,#77396,#77397));
#18682=EDGE_LOOP('',(#77398,#77399,#77400,#77401));
#18683=EDGE_LOOP('',(#77402,#77403,#77404,#77405));
#18684=EDGE_LOOP('',(#77406,#77407,#77408,#77409));
#18685=EDGE_LOOP('',(#77410,#77411,#77412,#77413));
#18686=EDGE_LOOP('',(#77414,#77415,#77416,#77417));
#18687=EDGE_LOOP('',(#77418,#77419,#77420,#77421));
#18688=EDGE_LOOP('',(#77422,#77423,#77424,#77425));
#18689=EDGE_LOOP('',(#77426,#77427,#77428,#77429));
#18690=EDGE_LOOP('',(#77430,#77431,#77432,#77433));
#18691=EDGE_LOOP('',(#77434,#77435,#77436,#77437));
#18692=EDGE_LOOP('',(#77438,#77439,#77440,#77441));
#18693=EDGE_LOOP('',(#77442,#77443,#77444,#77445));
#18694=EDGE_LOOP('',(#77446,#77447,#77448,#77449));
#18695=EDGE_LOOP('',(#77450,#77451,#77452,#77453));
#18696=EDGE_LOOP('',(#77454,#77455,#77456,#77457));
#18697=EDGE_LOOP('',(#77458,#77459,#77460,#77461));
#18698=EDGE_LOOP('',(#77462,#77463,#77464,#77465));
#18699=EDGE_LOOP('',(#77466,#77467,#77468,#77469));
#18700=EDGE_LOOP('',(#77470,#77471,#77472,#77473));
#18701=EDGE_LOOP('',(#77474,#77475,#77476,#77477));
#18702=EDGE_LOOP('',(#77478,#77479,#77480,#77481));
#18703=EDGE_LOOP('',(#77482,#77483,#77484,#77485));
#18704=EDGE_LOOP('',(#77486,#77487,#77488,#77489));
#18705=EDGE_LOOP('',(#77490,#77491,#77492,#77493));
#18706=EDGE_LOOP('',(#77494,#77495,#77496,#77497));
#18707=EDGE_LOOP('',(#77498,#77499,#77500,#77501));
#18708=EDGE_LOOP('',(#77502,#77503,#77504,#77505));
#18709=EDGE_LOOP('',(#77506,#77507,#77508,#77509));
#18710=EDGE_LOOP('',(#77510,#77511,#77512,#77513));
#18711=EDGE_LOOP('',(#77514,#77515,#77516,#77517));
#18712=EDGE_LOOP('',(#77518,#77519,#77520,#77521));
#18713=EDGE_LOOP('',(#77522,#77523,#77524,#77525));
#18714=EDGE_LOOP('',(#77526,#77527,#77528,#77529));
#18715=EDGE_LOOP('',(#77530,#77531,#77532,#77533));
#18716=EDGE_LOOP('',(#77534,#77535,#77536,#77537));
#18717=EDGE_LOOP('',(#77538,#77539,#77540,#77541));
#18718=EDGE_LOOP('',(#77542,#77543,#77544,#77545));
#18719=EDGE_LOOP('',(#77546,#77547,#77548,#77549,#77550));
#18720=EDGE_LOOP('',(#77551,#77552,#77553,#77554));
#18721=EDGE_LOOP('',(#77555,#77556,#77557,#77558));
#18722=EDGE_LOOP('',(#77559,#77560,#77561,#77562));
#18723=EDGE_LOOP('',(#77563,#77564,#77565,#77566));
#18724=EDGE_LOOP('',(#77567,#77568,#77569,#77570));
#18725=EDGE_LOOP('',(#77571,#77572,#77573,#77574));
#18726=EDGE_LOOP('',(#77575,#77576,#77577,#77578,#77579,#77580,#77581,#77582));
#18727=EDGE_LOOP('',(#77583,#77584));
#18728=EDGE_LOOP('',(#77585,#77586));
#18729=EDGE_LOOP('',(#77587,#77588));
#18730=EDGE_LOOP('',(#77589,#77590));
#18731=EDGE_LOOP('',(#77591,#77592));
#18732=EDGE_LOOP('',(#77593,#77594));
#18733=EDGE_LOOP('',(#77595,#77596,#77597,#77598,#77599));
#18734=EDGE_LOOP('',(#77600));
#18735=EDGE_LOOP('',(#77601));
#18736=EDGE_LOOP('',(#77602,#77603,#77604,#77605,#77606,#77607));
#18737=EDGE_LOOP('',(#77608,#77609,#77610,#77611,#77612));
#18738=EDGE_LOOP('',(#77613,#77614,#77615,#77616,#77617,#77618));
#18739=EDGE_LOOP('',(#77619,#77620,#77621));
#18740=EDGE_LOOP('',(#77622,#77623,#77624));
#18741=EDGE_LOOP('',(#77625,#77626,#77627));
#18742=EDGE_LOOP('',(#77628,#77629,#77630));
#18743=EDGE_LOOP('',(#77631,#77632,#77633));
#18744=EDGE_LOOP('',(#77634,#77635,#77636));
#18745=EDGE_LOOP('',(#77637,#77638,#77639,#77640,#77641,#77642));
#18746=EDGE_LOOP('',(#77643,#77644,#77645));
#18747=EDGE_LOOP('',(#77646,#77647,#77648));
#18748=EDGE_LOOP('',(#77649,#77650,#77651));
#18749=EDGE_LOOP('',(#77652,#77653,#77654));
#18750=EDGE_LOOP('',(#77655,#77656,#77657));
#18751=EDGE_LOOP('',(#77658,#77659,#77660));
#18752=EDGE_LOOP('',(#77661,#77662,#77663,#77664,#77665,#77666));
#18753=EDGE_LOOP('',(#77667,#77668,#77669,#77670,#77671,#77672));
#18754=EDGE_LOOP('',(#77673,#77674,#77675,#77676,#77677,#77678));
#18755=EDGE_LOOP('',(#77679,#77680,#77681,#77682,#77683,#77684));
#18756=EDGE_LOOP('',(#77685,#77686,#77687,#77688,#77689,#77690));
#18757=EDGE_LOOP('',(#77691,#77692,#77693,#77694,#77695,#77696));
#18758=EDGE_LOOP('',(#77697,#77698,#77699,#77700,#77701,#77702));
#18759=EDGE_LOOP('',(#77703,#77704,#77705));
#18760=EDGE_LOOP('',(#77706,#77707,#77708));
#18761=EDGE_LOOP('',(#77709,#77710,#77711));
#18762=EDGE_LOOP('',(#77712,#77713,#77714));
#18763=EDGE_LOOP('',(#77715,#77716,#77717));
#18764=EDGE_LOOP('',(#77718,#77719,#77720));
#18765=EDGE_LOOP('',(#77721,#77722,#77723,#77724,#77725,#77726));
#18766=EDGE_LOOP('',(#77727,#77728,#77729));
#18767=EDGE_LOOP('',(#77730,#77731,#77732));
#18768=EDGE_LOOP('',(#77733,#77734,#77735));
#18769=EDGE_LOOP('',(#77736,#77737,#77738));
#18770=EDGE_LOOP('',(#77739,#77740,#77741));
#18771=EDGE_LOOP('',(#77742,#77743,#77744));
#18772=EDGE_LOOP('',(#77745,#77746,#77747,#77748,#77749,#77750));
#18773=EDGE_LOOP('',(#77751,#77752,#77753,#77754,#77755,#77756));
#18774=EDGE_LOOP('',(#77757,#77758,#77759,#77760,#77761,#77762));
#18775=EDGE_LOOP('',(#77763,#77764,#77765,#77766,#77767,#77768));
#18776=EDGE_LOOP('',(#77769,#77770,#77771,#77772,#77773,#77774));
#18777=EDGE_LOOP('',(#77775,#77776,#77777,#77778,#77779,#77780));
#18778=EDGE_LOOP('',(#77781,#77782,#77783,#77784));
#18779=EDGE_LOOP('',(#77785,#77786,#77787,#77788));
#18780=EDGE_LOOP('',(#77789,#77790,#77791,#77792));
#18781=EDGE_LOOP('',(#77793,#77794,#77795,#77796));
#18782=EDGE_LOOP('',(#77797,#77798,#77799,#77800));
#18783=EDGE_LOOP('',(#77801,#77802,#77803,#77804));
#18784=EDGE_LOOP('',(#77805,#77806,#77807,#77808,#77809,#77810,#77811,#77812));
#18785=EDGE_LOOP('',(#77813,#77814));
#18786=EDGE_LOOP('',(#77815,#77816));
#18787=EDGE_LOOP('',(#77817,#77818));
#18788=EDGE_LOOP('',(#77819,#77820));
#18789=EDGE_LOOP('',(#77821,#77822));
#18790=EDGE_LOOP('',(#77823,#77824));
#18791=EDGE_LOOP('',(#77825,#77826,#77827,#77828,#77829));
#18792=EDGE_LOOP('',(#77830));
#18793=EDGE_LOOP('',(#77831));
#18794=EDGE_LOOP('',(#77832,#77833,#77834,#77835,#77836,#77837));
#18795=EDGE_LOOP('',(#77838,#77839,#77840,#77841,#77842));
#18796=EDGE_LOOP('',(#77843));
#18797=EDGE_LOOP('',(#77844,#77845,#77846,#77847));
#18798=EDGE_LOOP('',(#77848,#77849,#77850,#77851,#77852));
#18799=EDGE_LOOP('',(#77853,#77854,#77855,#77856,#77857));
#18800=EDGE_LOOP('',(#77858,#77859,#77860,#77861));
#18801=EDGE_LOOP('',(#77862,#77863,#77864,#77865));
#18802=EDGE_LOOP('',(#77866,#77867,#77868,#77869));
#18803=EDGE_LOOP('',(#77870,#77871,#77872,#77873));
#18804=EDGE_LOOP('',(#77874,#77875,#77876,#77877));
#18805=EDGE_LOOP('',(#77878));
#18806=EDGE_LOOP('',(#77879,#77880,#77881,#77882));
#18807=EDGE_LOOP('',(#77883,#77884,#77885,#77886,#77887,#77888));
#18808=EDGE_LOOP('',(#77889));
#18809=EDGE_LOOP('',(#77890));
#18810=EDGE_LOOP('',(#77891,#77892,#77893,#77894));
#18811=EDGE_LOOP('',(#77895));
#18812=EDGE_LOOP('',(#77896,#77897,#77898,#77899));
#18813=EDGE_LOOP('',(#77900));
#18814=EDGE_LOOP('',(#77901));
#18815=EDGE_LOOP('',(#77902,#77903,#77904,#77905));
#18816=EDGE_LOOP('',(#77906));
#18817=EDGE_LOOP('',(#77907,#77908,#77909,#77910));
#18818=EDGE_LOOP('',(#77911,#77912,#77913,#77914));
#18819=EDGE_LOOP('',(#77915,#77916,#77917,#77918));
#18820=EDGE_LOOP('',(#77919,#77920,#77921,#77922));
#18821=EDGE_LOOP('',(#77923,#77924,#77925,#77926));
#18822=EDGE_LOOP('',(#77927,#77928,#77929,#77930));
#18823=EDGE_LOOP('',(#77931,#77932,#77933,#77934));
#18824=EDGE_LOOP('',(#77935,#77936,#77937,#77938));
#18825=EDGE_LOOP('',(#77939,#77940,#77941,#77942));
#18826=EDGE_LOOP('',(#77943,#77944,#77945,#77946));
#18827=EDGE_LOOP('',(#77947,#77948,#77949,#77950));
#18828=EDGE_LOOP('',(#77951,#77952,#77953,#77954));
#18829=EDGE_LOOP('',(#77955));
#18830=EDGE_LOOP('',(#77956));
#18831=EDGE_LOOP('',(#77957,#77958,#77959,#77960));
#18832=EDGE_LOOP('',(#77961,#77962,#77963,#77964));
#18833=EDGE_LOOP('',(#77965,#77966,#77967,#77968));
#18834=EDGE_LOOP('',(#77969,#77970,#77971,#77972));
#18835=EDGE_LOOP('',(#77973,#77974,#77975,#77976));
#18836=EDGE_LOOP('',(#77977,#77978,#77979,#77980));
#18837=EDGE_LOOP('',(#77981,#77982,#77983,#77984));
#18838=EDGE_LOOP('',(#77985,#77986,#77987,#77988));
#18839=EDGE_LOOP('',(#77989,#77990,#77991,#77992));
#18840=EDGE_LOOP('',(#77993,#77994,#77995,#77996));
#18841=EDGE_LOOP('',(#77997,#77998,#77999,#78000));
#18842=EDGE_LOOP('',(#78001,#78002,#78003,#78004));
#18843=EDGE_LOOP('',(#78005,#78006,#78007,#78008));
#18844=EDGE_LOOP('',(#78009,#78010,#78011,#78012));
#18845=EDGE_LOOP('',(#78013,#78014,#78015,#78016));
#18846=EDGE_LOOP('',(#78017,#78018,#78019,#78020));
#18847=EDGE_LOOP('',(#78021,#78022,#78023,#78024));
#18848=EDGE_LOOP('',(#78025));
#18849=EDGE_LOOP('',(#78026));
#18850=EDGE_LOOP('',(#78027,#78028,#78029,#78030));
#18851=EDGE_LOOP('',(#78031,#78032,#78033,#78034));
#18852=EDGE_LOOP('',(#78035,#78036,#78037,#78038));
#18853=EDGE_LOOP('',(#78039,#78040,#78041,#78042));
#18854=EDGE_LOOP('',(#78043,#78044,#78045,#78046));
#18855=EDGE_LOOP('',(#78047,#78048,#78049,#78050,#78051,#78052,#78053,#78054));
#18856=EDGE_LOOP('',(#78055,#78056,#78057,#78058));
#18857=EDGE_LOOP('',(#78059,#78060,#78061,#78062));
#18858=EDGE_LOOP('',(#78063,#78064,#78065,#78066));
#18859=EDGE_LOOP('',(#78067,#78068,#78069,#78070,#78071,#78072,#78073,#78074));
#18860=EDGE_LOOP('',(#78075,#78076,#78077,#78078,#78079,#78080,#78081,#78082));
#18861=EDGE_LOOP('',(#78083,#78084,#78085,#78086));
#18862=EDGE_LOOP('',(#78087,#78088,#78089,#78090));
#18863=EDGE_LOOP('',(#78091,#78092,#78093,#78094));
#18864=EDGE_LOOP('',(#78095,#78096,#78097,#78098));
#18865=EDGE_LOOP('',(#78099,#78100,#78101,#78102));
#18866=EDGE_LOOP('',(#78103,#78104,#78105,#78106,#78107,#78108,#78109,#78110));
#18867=EDGE_LOOP('',(#78111));
#18868=EDGE_LOOP('',(#78112,#78113,#78114,#78115));
#18869=EDGE_LOOP('',(#78116,#78117,#78118,#78119,#78120));
#18870=EDGE_LOOP('',(#78121,#78122,#78123,#78124,#78125));
#18871=EDGE_LOOP('',(#78126,#78127,#78128,#78129));
#18872=EDGE_LOOP('',(#78130,#78131,#78132,#78133));
#18873=EDGE_LOOP('',(#78134,#78135,#78136,#78137));
#18874=EDGE_LOOP('',(#78138,#78139,#78140,#78141));
#18875=EDGE_LOOP('',(#78142,#78143,#78144,#78145));
#18876=EDGE_LOOP('',(#78146));
#18877=EDGE_LOOP('',(#78147,#78148,#78149,#78150));
#18878=EDGE_LOOP('',(#78151,#78152,#78153,#78154,#78155,#78156));
#18879=EDGE_LOOP('',(#78157));
#18880=EDGE_LOOP('',(#78158));
#18881=EDGE_LOOP('',(#78159,#78160,#78161,#78162));
#18882=EDGE_LOOP('',(#78163,#78164,#78165,#78166));
#18883=EDGE_LOOP('',(#78167,#78168,#78169,#78170));
#18884=EDGE_LOOP('',(#78171,#78172,#78173,#78174));
#18885=EDGE_LOOP('',(#78175,#78176,#78177,#78178));
#18886=EDGE_LOOP('',(#78179,#78180,#78181,#78182));
#18887=EDGE_LOOP('',(#78183,#78184,#78185,#78186));
#18888=EDGE_LOOP('',(#78187,#78188,#78189,#78190));
#18889=EDGE_LOOP('',(#78191,#78192,#78193,#78194));
#18890=EDGE_LOOP('',(#78195,#78196,#78197,#78198));
#18891=EDGE_LOOP('',(#78199,#78200,#78201,#78202));
#18892=EDGE_LOOP('',(#78203,#78204,#78205,#78206));
#18893=EDGE_LOOP('',(#78207,#78208,#78209,#78210));
#18894=EDGE_LOOP('',(#78211,#78212,#78213,#78214));
#18895=EDGE_LOOP('',(#78215,#78216,#78217,#78218));
#18896=EDGE_LOOP('',(#78219,#78220,#78221,#78222));
#18897=EDGE_LOOP('',(#78223,#78224,#78225,#78226));
#18898=EDGE_LOOP('',(#78227,#78228,#78229,#78230));
#18899=EDGE_LOOP('',(#78231,#78232,#78233,#78234));
#18900=EDGE_LOOP('',(#78235,#78236,#78237,#78238));
#18901=EDGE_LOOP('',(#78239,#78240,#78241,#78242));
#18902=EDGE_LOOP('',(#78243,#78244,#78245,#78246));
#18903=EDGE_LOOP('',(#78247,#78248,#78249,#78250));
#18904=EDGE_LOOP('',(#78251,#78252,#78253,#78254));
#18905=EDGE_LOOP('',(#78255,#78256,#78257,#78258));
#18906=EDGE_LOOP('',(#78259,#78260,#78261,#78262));
#18907=EDGE_LOOP('',(#78263,#78264,#78265,#78266));
#18908=EDGE_LOOP('',(#78267,#78268,#78269,#78270));
#18909=EDGE_LOOP('',(#78271,#78272,#78273,#78274));
#18910=EDGE_LOOP('',(#78275,#78276,#78277,#78278));
#18911=EDGE_LOOP('',(#78279,#78280,#78281,#78282));
#18912=EDGE_LOOP('',(#78283,#78284,#78285,#78286));
#18913=EDGE_LOOP('',(#78287,#78288,#78289,#78290));
#18914=EDGE_LOOP('',(#78291,#78292,#78293,#78294));
#18915=EDGE_LOOP('',(#78295,#78296,#78297,#78298));
#18916=EDGE_LOOP('',(#78299,#78300,#78301,#78302));
#18917=EDGE_LOOP('',(#78303,#78304,#78305,#78306));
#18918=EDGE_LOOP('',(#78307,#78308,#78309,#78310));
#18919=EDGE_LOOP('',(#78311,#78312,#78313,#78314));
#18920=EDGE_LOOP('',(#78315,#78316,#78317,#78318));
#18921=EDGE_LOOP('',(#78319,#78320,#78321,#78322));
#18922=EDGE_LOOP('',(#78323,#78324,#78325,#78326));
#18923=EDGE_LOOP('',(#78327,#78328,#78329,#78330));
#18924=EDGE_LOOP('',(#78331,#78332,#78333,#78334));
#18925=EDGE_LOOP('',(#78335,#78336,#78337,#78338));
#18926=EDGE_LOOP('',(#78339,#78340,#78341,#78342));
#18927=EDGE_LOOP('',(#78343,#78344,#78345,#78346));
#18928=EDGE_LOOP('',(#78347,#78348,#78349,#78350));
#18929=EDGE_LOOP('',(#78351,#78352,#78353,#78354));
#18930=EDGE_LOOP('',(#78355,#78356,#78357,#78358));
#18931=EDGE_LOOP('',(#78359,#78360,#78361,#78362));
#18932=EDGE_LOOP('',(#78363,#78364,#78365,#78366));
#18933=EDGE_LOOP('',(#78367,#78368,#78369,#78370));
#18934=EDGE_LOOP('',(#78371,#78372,#78373,#78374));
#18935=EDGE_LOOP('',(#78375,#78376,#78377,#78378));
#18936=EDGE_LOOP('',(#78379,#78380,#78381,#78382));
#18937=EDGE_LOOP('',(#78383,#78384,#78385,#78386));
#18938=EDGE_LOOP('',(#78387,#78388,#78389,#78390));
#18939=EDGE_LOOP('',(#78391,#78392,#78393,#78394));
#18940=EDGE_LOOP('',(#78395,#78396,#78397,#78398));
#18941=EDGE_LOOP('',(#78399,#78400,#78401,#78402));
#18942=EDGE_LOOP('',(#78403,#78404,#78405,#78406));
#18943=EDGE_LOOP('',(#78407,#78408,#78409,#78410));
#18944=EDGE_LOOP('',(#78411,#78412,#78413,#78414));
#18945=EDGE_LOOP('',(#78415,#78416,#78417,#78418));
#18946=EDGE_LOOP('',(#78419,#78420,#78421,#78422));
#18947=EDGE_LOOP('',(#78423,#78424,#78425,#78426));
#18948=EDGE_LOOP('',(#78427,#78428,#78429,#78430));
#18949=EDGE_LOOP('',(#78431,#78432,#78433,#78434));
#18950=EDGE_LOOP('',(#78435,#78436,#78437,#78438));
#18951=EDGE_LOOP('',(#78439,#78440,#78441,#78442));
#18952=EDGE_LOOP('',(#78443,#78444,#78445,#78446));
#18953=EDGE_LOOP('',(#78447,#78448,#78449,#78450));
#18954=EDGE_LOOP('',(#78451,#78452,#78453,#78454));
#18955=EDGE_LOOP('',(#78455,#78456,#78457,#78458));
#18956=EDGE_LOOP('',(#78459,#78460,#78461,#78462));
#18957=EDGE_LOOP('',(#78463,#78464,#78465,#78466));
#18958=EDGE_LOOP('',(#78467,#78468,#78469,#78470));
#18959=EDGE_LOOP('',(#78471,#78472,#78473,#78474));
#18960=EDGE_LOOP('',(#78475,#78476,#78477,#78478));
#18961=EDGE_LOOP('',(#78479,#78480,#78481,#78482));
#18962=EDGE_LOOP('',(#78483,#78484,#78485,#78486));
#18963=EDGE_LOOP('',(#78487,#78488,#78489,#78490));
#18964=EDGE_LOOP('',(#78491,#78492,#78493,#78494));
#18965=EDGE_LOOP('',(#78495,#78496,#78497,#78498));
#18966=EDGE_LOOP('',(#78499,#78500,#78501,#78502));
#18967=EDGE_LOOP('',(#78503,#78504,#78505,#78506));
#18968=EDGE_LOOP('',(#78507,#78508,#78509,#78510));
#18969=EDGE_LOOP('',(#78511,#78512,#78513,#78514));
#18970=EDGE_LOOP('',(#78515,#78516,#78517,#78518));
#18971=EDGE_LOOP('',(#78519,#78520,#78521,#78522));
#18972=EDGE_LOOP('',(#78523,#78524,#78525,#78526));
#18973=EDGE_LOOP('',(#78527,#78528,#78529,#78530));
#18974=EDGE_LOOP('',(#78531,#78532,#78533,#78534));
#18975=EDGE_LOOP('',(#78535,#78536,#78537,#78538));
#18976=EDGE_LOOP('',(#78539,#78540,#78541,#78542));
#18977=EDGE_LOOP('',(#78543,#78544,#78545,#78546));
#18978=EDGE_LOOP('',(#78547,#78548,#78549,#78550));
#18979=EDGE_LOOP('',(#78551,#78552,#78553,#78554));
#18980=EDGE_LOOP('',(#78555,#78556,#78557,#78558));
#18981=EDGE_LOOP('',(#78559,#78560,#78561,#78562));
#18982=EDGE_LOOP('',(#78563,#78564,#78565,#78566));
#18983=EDGE_LOOP('',(#78567,#78568,#78569,#78570));
#18984=EDGE_LOOP('',(#78571,#78572,#78573,#78574));
#18985=EDGE_LOOP('',(#78575,#78576,#78577,#78578));
#18986=EDGE_LOOP('',(#78579,#78580,#78581,#78582));
#18987=EDGE_LOOP('',(#78583,#78584,#78585,#78586));
#18988=EDGE_LOOP('',(#78587,#78588,#78589,#78590));
#18989=EDGE_LOOP('',(#78591,#78592,#78593,#78594));
#18990=EDGE_LOOP('',(#78595,#78596,#78597,#78598));
#18991=EDGE_LOOP('',(#78599,#78600,#78601,#78602));
#18992=EDGE_LOOP('',(#78603,#78604,#78605,#78606));
#18993=EDGE_LOOP('',(#78607,#78608,#78609,#78610));
#18994=EDGE_LOOP('',(#78611,#78612,#78613,#78614));
#18995=EDGE_LOOP('',(#78615,#78616,#78617,#78618));
#18996=EDGE_LOOP('',(#78619,#78620,#78621,#78622));
#18997=EDGE_LOOP('',(#78623,#78624,#78625,#78626));
#18998=EDGE_LOOP('',(#78627,#78628,#78629,#78630));
#18999=EDGE_LOOP('',(#78631,#78632,#78633,#78634));
#19000=EDGE_LOOP('',(#78635,#78636,#78637,#78638));
#19001=EDGE_LOOP('',(#78639,#78640,#78641,#78642));
#19002=EDGE_LOOP('',(#78643,#78644,#78645,#78646));
#19003=EDGE_LOOP('',(#78647,#78648,#78649,#78650));
#19004=EDGE_LOOP('',(#78651,#78652,#78653,#78654));
#19005=EDGE_LOOP('',(#78655,#78656,#78657,#78658));
#19006=EDGE_LOOP('',(#78659,#78660,#78661,#78662));
#19007=EDGE_LOOP('',(#78663,#78664,#78665,#78666));
#19008=EDGE_LOOP('',(#78667,#78668,#78669,#78670));
#19009=EDGE_LOOP('',(#78671,#78672,#78673,#78674));
#19010=EDGE_LOOP('',(#78675,#78676,#78677,#78678));
#19011=EDGE_LOOP('',(#78679,#78680,#78681,#78682));
#19012=EDGE_LOOP('',(#78683,#78684,#78685,#78686));
#19013=EDGE_LOOP('',(#78687,#78688,#78689,#78690));
#19014=EDGE_LOOP('',(#78691,#78692,#78693,#78694));
#19015=EDGE_LOOP('',(#78695,#78696,#78697,#78698));
#19016=EDGE_LOOP('',(#78699,#78700,#78701,#78702));
#19017=EDGE_LOOP('',(#78703,#78704,#78705,#78706));
#19018=EDGE_LOOP('',(#78707,#78708,#78709,#78710));
#19019=EDGE_LOOP('',(#78711,#78712,#78713,#78714,#78715,#78716,#78717,#78718,
#78719,#78720,#78721,#78722,#78723,#78724,#78725,#78726,#78727,#78728,#78729,
#78730,#78731,#78732,#78733,#78734,#78735,#78736,#78737,#78738,#78739,#78740,
#78741,#78742,#78743,#78744,#78745,#78746,#78747,#78748,#78749,#78750,#78751,
#78752,#78753,#78754,#78755,#78756,#78757,#78758,#78759,#78760,#78761,#78762,
#78763,#78764,#78765,#78766,#78767,#78768,#78769,#78770,#78771,#78772,#78773,
#78774,#78775,#78776,#78777,#78778,#78779,#78780,#78781,#78782,#78783,#78784,
#78785,#78786,#78787,#78788,#78789,#78790,#78791,#78792,#78793,#78794));
#19020=EDGE_LOOP('',(#78795,#78796,#78797,#78798,#78799));
#19021=EDGE_LOOP('',(#78800,#78801,#78802,#78803,#78804));
#19022=EDGE_LOOP('',(#78805,#78806,#78807,#78808));
#19023=EDGE_LOOP('',(#78809,#78810,#78811,#78812));
#19024=EDGE_LOOP('',(#78813,#78814,#78815,#78816));
#19025=EDGE_LOOP('',(#78817,#78818,#78819,#78820,#78821));
#19026=EDGE_LOOP('',(#78822,#78823,#78824,#78825,#78826));
#19027=EDGE_LOOP('',(#78827,#78828,#78829,#78830,#78831));
#19028=EDGE_LOOP('',(#78832,#78833,#78834,#78835,#78836));
#19029=EDGE_LOOP('',(#78837,#78838,#78839,#78840,#78841));
#19030=EDGE_LOOP('',(#78842,#78843,#78844,#78845,#78846));
#19031=EDGE_LOOP('',(#78847,#78848,#78849,#78850,#78851));
#19032=EDGE_LOOP('',(#78852,#78853,#78854,#78855,#78856));
#19033=EDGE_LOOP('',(#78857,#78858,#78859,#78860,#78861));
#19034=EDGE_LOOP('',(#78862,#78863,#78864,#78865,#78866));
#19035=EDGE_LOOP('',(#78867,#78868,#78869,#78870));
#19036=EDGE_LOOP('',(#78871,#78872,#78873,#78874));
#19037=EDGE_LOOP('',(#78875,#78876,#78877,#78878));
#19038=EDGE_LOOP('',(#78879,#78880,#78881,#78882,#78883));
#19039=EDGE_LOOP('',(#78884,#78885,#78886,#78887,#78888));
#19040=EDGE_LOOP('',(#78889,#78890,#78891,#78892));
#19041=EDGE_LOOP('',(#78893,#78894,#78895,#78896));
#19042=EDGE_LOOP('',(#78897,#78898,#78899,#78900));
#19043=EDGE_LOOP('',(#78901,#78902,#78903,#78904,#78905));
#19044=EDGE_LOOP('',(#78906,#78907,#78908,#78909,#78910));
#19045=EDGE_LOOP('',(#78911,#78912,#78913,#78914));
#19046=EDGE_LOOP('',(#78915,#78916,#78917,#78918));
#19047=EDGE_LOOP('',(#78919,#78920,#78921,#78922));
#19048=EDGE_LOOP('',(#78923,#78924,#78925,#78926,#78927));
#19049=EDGE_LOOP('',(#78928,#78929,#78930,#78931,#78932));
#19050=EDGE_LOOP('',(#78933,#78934,#78935,#78936));
#19051=EDGE_LOOP('',(#78937,#78938,#78939,#78940));
#19052=EDGE_LOOP('',(#78941,#78942,#78943,#78944));
#19053=EDGE_LOOP('',(#78945,#78946,#78947,#78948,#78949));
#19054=EDGE_LOOP('',(#78950,#78951,#78952,#78953,#78954));
#19055=EDGE_LOOP('',(#78955,#78956,#78957,#78958));
#19056=EDGE_LOOP('',(#78959,#78960,#78961,#78962));
#19057=EDGE_LOOP('',(#78963,#78964,#78965,#78966));
#19058=EDGE_LOOP('',(#78967,#78968,#78969,#78970));
#19059=EDGE_LOOP('',(#78971,#78972,#78973,#78974));
#19060=EDGE_LOOP('',(#78975,#78976,#78977,#78978));
#19061=EDGE_LOOP('',(#78979,#78980,#78981,#78982,#78983));
#19062=EDGE_LOOP('',(#78984,#78985,#78986,#78987,#78988,#78989,#78990,#78991,
#78992,#78993,#78994,#78995,#78996,#78997,#78998,#78999,#79000,#79001,#79002,
#79003,#79004,#79005,#79006,#79007,#79008,#79009,#79010,#79011,#79012,#79013,
#79014,#79015,#79016,#79017,#79018,#79019,#79020,#79021,#79022,#79023,#79024,
#79025,#79026,#79027,#79028,#79029,#79030,#79031,#79032,#79033,#79034,#79035,
#79036,#79037,#79038,#79039,#79040,#79041,#79042,#79043,#79044,#79045,#79046,
#79047,#79048,#79049,#79050,#79051,#79052,#79053,#79054,#79055,#79056,#79057,
#79058,#79059,#79060,#79061,#79062,#79063,#79064,#79065,#79066,#79067,#79068,
#79069,#79070,#79071,#79072,#79073,#79074,#79075,#79076,#79077,#79078,#79079,
#79080,#79081,#79082,#79083,#79084,#79085,#79086,#79087,#79088,#79089));
#19063=EDGE_LOOP('',(#79090,#79091,#79092,#79093));
#19064=EDGE_LOOP('',(#79094,#79095,#79096,#79097,#79098));
#19065=EDGE_LOOP('',(#79099,#79100,#79101,#79102));
#19066=EDGE_LOOP('',(#79103,#79104,#79105,#79106));
#19067=EDGE_LOOP('',(#79107,#79108,#79109,#79110));
#19068=EDGE_LOOP('',(#79111,#79112,#79113,#79114));
#19069=EDGE_LOOP('',(#79115,#79116,#79117,#79118));
#19070=EDGE_LOOP('',(#79119,#79120,#79121,#79122));
#19071=EDGE_LOOP('',(#79123,#79124,#79125,#79126));
#19072=EDGE_LOOP('',(#79127,#79128,#79129,#79130));
#19073=EDGE_LOOP('',(#79131,#79132,#79133,#79134));
#19074=EDGE_LOOP('',(#79135,#79136,#79137,#79138));
#19075=EDGE_LOOP('',(#79139,#79140,#79141,#79142));
#19076=EDGE_LOOP('',(#79143,#79144,#79145,#79146));
#19077=EDGE_LOOP('',(#79147,#79148,#79149,#79150));
#19078=EDGE_LOOP('',(#79151,#79152,#79153,#79154));
#19079=EDGE_LOOP('',(#79155,#79156,#79157,#79158));
#19080=EDGE_LOOP('',(#79159,#79160,#79161,#79162));
#19081=EDGE_LOOP('',(#79163,#79164,#79165,#79166,#79167));
#19082=EDGE_LOOP('',(#79168,#79169,#79170,#79171));
#19083=EDGE_LOOP('',(#79172,#79173,#79174,#79175));
#19084=EDGE_LOOP('',(#79176,#79177,#79178,#79179));
#19085=EDGE_LOOP('',(#79180,#79181,#79182,#79183,#79184,#79185));
#19086=EDGE_LOOP('',(#79186,#79187,#79188,#79189));
#19087=EDGE_LOOP('',(#79190,#79191,#79192,#79193,#79194));
#19088=EDGE_LOOP('',(#79195,#79196,#79197,#79198));
#19089=EDGE_LOOP('',(#79199,#79200,#79201,#79202,#79203,#79204));
#19090=EDGE_LOOP('',(#79205,#79206,#79207,#79208,#79209,#79210));
#19091=EDGE_LOOP('',(#79211,#79212,#79213));
#19092=EDGE_LOOP('',(#79214,#79215,#79216));
#19093=EDGE_LOOP('',(#79217,#79218,#79219));
#19094=EDGE_LOOP('',(#79220,#79221,#79222));
#19095=EDGE_LOOP('',(#79223,#79224,#79225));
#19096=EDGE_LOOP('',(#79226,#79227,#79228));
#19097=EDGE_LOOP('',(#79229,#79230,#79231,#79232,#79233,#79234));
#19098=EDGE_LOOP('',(#79235,#79236,#79237));
#19099=EDGE_LOOP('',(#79238,#79239,#79240));
#19100=EDGE_LOOP('',(#79241,#79242,#79243));
#19101=EDGE_LOOP('',(#79244,#79245,#79246));
#19102=EDGE_LOOP('',(#79247,#79248,#79249));
#19103=EDGE_LOOP('',(#79250,#79251,#79252));
#19104=EDGE_LOOP('',(#79253,#79254,#79255,#79256,#79257,#79258));
#19105=EDGE_LOOP('',(#79259,#79260,#79261,#79262,#79263,#79264));
#19106=EDGE_LOOP('',(#79265,#79266,#79267,#79268,#79269,#79270));
#19107=EDGE_LOOP('',(#79271,#79272,#79273,#79274,#79275,#79276));
#19108=EDGE_LOOP('',(#79277,#79278,#79279,#79280,#79281,#79282));
#19109=EDGE_LOOP('',(#79283,#79284,#79285,#79286,#79287,#79288));
#19110=EDGE_LOOP('',(#79289,#79290,#79291,#79292,#79293,#79294));
#19111=EDGE_LOOP('',(#79295,#79296,#79297));
#19112=EDGE_LOOP('',(#79298,#79299,#79300));
#19113=EDGE_LOOP('',(#79301,#79302,#79303));
#19114=EDGE_LOOP('',(#79304,#79305,#79306));
#19115=EDGE_LOOP('',(#79307,#79308,#79309));
#19116=EDGE_LOOP('',(#79310,#79311,#79312));
#19117=EDGE_LOOP('',(#79313,#79314,#79315,#79316,#79317,#79318));
#19118=EDGE_LOOP('',(#79319,#79320,#79321));
#19119=EDGE_LOOP('',(#79322,#79323,#79324));
#19120=EDGE_LOOP('',(#79325,#79326,#79327));
#19121=EDGE_LOOP('',(#79328,#79329,#79330));
#19122=EDGE_LOOP('',(#79331,#79332,#79333));
#19123=EDGE_LOOP('',(#79334,#79335,#79336));
#19124=EDGE_LOOP('',(#79337,#79338,#79339,#79340,#79341,#79342));
#19125=EDGE_LOOP('',(#79343,#79344,#79345,#79346,#79347,#79348));
#19126=EDGE_LOOP('',(#79349,#79350,#79351,#79352,#79353,#79354));
#19127=EDGE_LOOP('',(#79355,#79356,#79357,#79358,#79359,#79360));
#19128=EDGE_LOOP('',(#79361,#79362,#79363,#79364,#79365,#79366));
#19129=EDGE_LOOP('',(#79367,#79368,#79369,#79370,#79371,#79372));
#19130=EDGE_LOOP('',(#79373,#79374,#79375,#79376));
#19131=EDGE_LOOP('',(#79377,#79378,#79379,#79380));
#19132=EDGE_LOOP('',(#79381,#79382,#79383,#79384));
#19133=EDGE_LOOP('',(#79385,#79386,#79387,#79388));
#19134=EDGE_LOOP('',(#79389,#79390,#79391,#79392));
#19135=EDGE_LOOP('',(#79393,#79394,#79395,#79396));
#19136=EDGE_LOOP('',(#79397,#79398,#79399,#79400,#79401,#79402,#79403,#79404));
#19137=EDGE_LOOP('',(#79405,#79406));
#19138=EDGE_LOOP('',(#79407,#79408));
#19139=EDGE_LOOP('',(#79409,#79410));
#19140=EDGE_LOOP('',(#79411,#79412));
#19141=EDGE_LOOP('',(#79413,#79414));
#19142=EDGE_LOOP('',(#79415,#79416));
#19143=EDGE_LOOP('',(#79417,#79418,#79419,#79420,#79421));
#19144=EDGE_LOOP('',(#79422));
#19145=EDGE_LOOP('',(#79423));
#19146=EDGE_LOOP('',(#79424,#79425,#79426,#79427,#79428,#79429));
#19147=EDGE_LOOP('',(#79430,#79431,#79432,#79433,#79434));
#19148=EDGE_LOOP('',(#79435,#79436,#79437));
#19149=EDGE_LOOP('',(#79438,#79439,#79440));
#19150=EDGE_LOOP('',(#79441,#79442,#79443,#79444));
#19151=EDGE_LOOP('',(#79445,#79446,#79447,#79448));
#19152=EDGE_LOOP('',(#79449,#79450,#79451));
#19153=EDGE_LOOP('',(#79452,#79453,#79454,#79455));
#19154=EDGE_LOOP('',(#79456,#79457,#79458));
#19155=EDGE_LOOP('',(#79459,#79460,#79461));
#19156=EDGE_LOOP('',(#79462,#79463,#79464));
#19157=EDGE_LOOP('',(#79465,#79466,#79467));
#19158=EDGE_LOOP('',(#79468,#79469,#79470,#79471));
#19159=EDGE_LOOP('',(#79472,#79473,#79474));
#19160=EDGE_LOOP('',(#79475,#79476,#79477,#79478));
#19161=EDGE_LOOP('',(#79479,#79480,#79481,#79482));
#19162=EDGE_LOOP('',(#79483,#79484,#79485,#79486));
#19163=EDGE_LOOP('',(#79487,#79488,#79489,#79490));
#19164=EDGE_LOOP('',(#79491,#79492,#79493,#79494));
#19165=EDGE_LOOP('',(#79495,#79496,#79497,#79498,#79499,#79500,#79501,#79502,
#79503,#79504));
#19166=EDGE_LOOP('',(#79505,#79506,#79507));
#19167=EDGE_LOOP('',(#79508,#79509,#79510));
#19168=EDGE_LOOP('',(#79511,#79512,#79513,#79514));
#19169=EDGE_LOOP('',(#79515,#79516,#79517,#79518));
#19170=EDGE_LOOP('',(#79519,#79520,#79521));
#19171=EDGE_LOOP('',(#79522,#79523,#79524,#79525));
#19172=EDGE_LOOP('',(#79526,#79527,#79528));
#19173=EDGE_LOOP('',(#79529,#79530,#79531));
#19174=EDGE_LOOP('',(#79532,#79533,#79534));
#19175=EDGE_LOOP('',(#79535,#79536,#79537));
#19176=EDGE_LOOP('',(#79538,#79539,#79540,#79541));
#19177=EDGE_LOOP('',(#79542,#79543,#79544));
#19178=EDGE_LOOP('',(#79545,#79546,#79547,#79548));
#19179=EDGE_LOOP('',(#79549,#79550,#79551,#79552));
#19180=EDGE_LOOP('',(#79553,#79554,#79555,#79556));
#19181=EDGE_LOOP('',(#79557,#79558,#79559,#79560));
#19182=EDGE_LOOP('',(#79561,#79562,#79563,#79564));
#19183=EDGE_LOOP('',(#79565,#79566,#79567,#79568));
#19184=EDGE_LOOP('',(#79569,#79570,#79571,#79572));
#19185=EDGE_LOOP('',(#79573,#79574,#79575,#79576,#79577,#79578,#79579,#79580,
#79581,#79582));
#19186=EDGE_LOOP('',(#79583,#79584,#79585,#79586));
#19187=EDGE_LOOP('',(#79587,#79588,#79589,#79590));
#19188=EDGE_LOOP('',(#79591,#79592,#79593,#79594));
#19189=EDGE_LOOP('',(#79595,#79596,#79597,#79598));
#19190=EDGE_LOOP('',(#79599,#79600,#79601,#79602));
#19191=EDGE_LOOP('',(#79603,#79604,#79605,#79606));
#19192=EDGE_LOOP('',(#79607,#79608,#79609,#79610));
#19193=EDGE_LOOP('',(#79611,#79612,#79613,#79614));
#19194=EDGE_LOOP('',(#79615,#79616,#79617,#79618));
#19195=EDGE_LOOP('',(#79619,#79620,#79621,#79622));
#19196=EDGE_LOOP('',(#79623,#79624,#79625,#79626,#79627,#79628,#79629,#79630));
#19197=EDGE_LOOP('',(#79631,#79632,#79633,#79634));
#19198=EDGE_LOOP('',(#79635,#79636,#79637,#79638));
#19199=EDGE_LOOP('',(#79639,#79640,#79641,#79642));
#19200=EDGE_LOOP('',(#79643,#79644,#79645,#79646));
#19201=EDGE_LOOP('',(#79647,#79648,#79649,#79650));
#19202=EDGE_LOOP('',(#79651,#79652,#79653,#79654));
#19203=EDGE_LOOP('',(#79655,#79656,#79657,#79658));
#19204=EDGE_LOOP('',(#79659,#79660,#79661,#79662));
#19205=EDGE_LOOP('',(#79663,#79664,#79665,#79666));
#19206=EDGE_LOOP('',(#79667,#79668,#79669,#79670,#79671,#79672,#79673,#79674,
#79675,#79676,#79677,#79678,#79679,#79680,#79681,#79682,#79683,#79684,#79685,
#79686,#79687,#79688,#79689,#79690,#79691,#79692,#79693,#79694,#79695,#79696,
#79697,#79698,#79699,#79700,#79701,#79702,#79703,#79704,#79705,#79706,#79707,
#79708,#79709,#79710,#79711,#79712,#79713,#79714,#79715,#79716,#79717,#79718));
#19207=EDGE_LOOP('',(#79719,#79720,#79721,#79722,#79723,#79724,#79725,#79726,
#79727,#79728,#79729,#79730,#79731,#79732,#79733,#79734));
#19208=EDGE_LOOP('',(#79735,#79736,#79737,#79738,#79739,#79740,#79741,#79742,
#79743,#79744,#79745,#79746,#79747,#79748));
#19209=EDGE_LOOP('',(#79749,#79750,#79751,#79752));
#19210=EDGE_LOOP('',(#79753,#79754,#79755,#79756));
#19211=EDGE_LOOP('',(#79757,#79758,#79759,#79760));
#19212=EDGE_LOOP('',(#79761,#79762,#79763,#79764));
#19213=EDGE_LOOP('',(#79765,#79766,#79767,#79768));
#19214=EDGE_LOOP('',(#79769,#79770,#79771,#79772));
#19215=EDGE_LOOP('',(#79773,#79774,#79775,#79776));
#19216=EDGE_LOOP('',(#79777,#79778,#79779,#79780));
#19217=EDGE_LOOP('',(#79781,#79782,#79783,#79784));
#19218=EDGE_LOOP('',(#79785,#79786,#79787,#79788));
#19219=EDGE_LOOP('',(#79789,#79790,#79791,#79792));
#19220=EDGE_LOOP('',(#79793,#79794,#79795,#79796));
#19221=EDGE_LOOP('',(#79797,#79798,#79799,#79800));
#19222=EDGE_LOOP('',(#79801,#79802,#79803,#79804));
#19223=EDGE_LOOP('',(#79805,#79806,#79807,#79808));
#19224=EDGE_LOOP('',(#79809,#79810,#79811,#79812));
#19225=EDGE_LOOP('',(#79813,#79814,#79815,#79816));
#19226=EDGE_LOOP('',(#79817,#79818,#79819,#79820));
#19227=EDGE_LOOP('',(#79821,#79822,#79823,#79824));
#19228=EDGE_LOOP('',(#79825,#79826,#79827,#79828));
#19229=EDGE_LOOP('',(#79829,#79830,#79831,#79832));
#19230=EDGE_LOOP('',(#79833,#79834,#79835,#79836));
#19231=EDGE_LOOP('',(#79837,#79838,#79839,#79840));
#19232=EDGE_LOOP('',(#79841,#79842,#79843,#79844));
#19233=EDGE_LOOP('',(#79845,#79846,#79847,#79848));
#19234=EDGE_LOOP('',(#79849,#79850,#79851,#79852));
#19235=EDGE_LOOP('',(#79853,#79854,#79855,#79856));
#19236=EDGE_LOOP('',(#79857,#79858,#79859,#79860));
#19237=EDGE_LOOP('',(#79861,#79862,#79863,#79864));
#19238=EDGE_LOOP('',(#79865,#79866,#79867,#79868));
#19239=EDGE_LOOP('',(#79869,#79870,#79871,#79872));
#19240=EDGE_LOOP('',(#79873,#79874,#79875,#79876));
#19241=EDGE_LOOP('',(#79877,#79878,#79879,#79880));
#19242=EDGE_LOOP('',(#79881,#79882,#79883,#79884));
#19243=EDGE_LOOP('',(#79885,#79886,#79887,#79888));
#19244=EDGE_LOOP('',(#79889,#79890,#79891,#79892));
#19245=EDGE_LOOP('',(#79893,#79894,#79895,#79896));
#19246=EDGE_LOOP('',(#79897,#79898,#79899,#79900));
#19247=EDGE_LOOP('',(#79901,#79902,#79903,#79904));
#19248=EDGE_LOOP('',(#79905,#79906,#79907,#79908));
#19249=EDGE_LOOP('',(#79909,#79910,#79911,#79912));
#19250=EDGE_LOOP('',(#79913,#79914,#79915,#79916,#79917,#79918));
#19251=EDGE_LOOP('',(#79919,#79920,#79921,#79922));
#19252=EDGE_LOOP('',(#79923,#79924,#79925,#79926));
#19253=EDGE_LOOP('',(#79927,#79928,#79929,#79930));
#19254=EDGE_LOOP('',(#79931,#79932,#79933,#79934));
#19255=EDGE_LOOP('',(#79935,#79936,#79937,#79938));
#19256=EDGE_LOOP('',(#79939,#79940,#79941,#79942));
#19257=EDGE_LOOP('',(#79943,#79944,#79945,#79946));
#19258=EDGE_LOOP('',(#79947,#79948,#79949,#79950));
#19259=EDGE_LOOP('',(#79951,#79952,#79953,#79954));
#19260=EDGE_LOOP('',(#79955,#79956,#79957,#79958));
#19261=EDGE_LOOP('',(#79959,#79960,#79961,#79962));
#19262=EDGE_LOOP('',(#79963,#79964,#79965,#79966));
#19263=EDGE_LOOP('',(#79967,#79968,#79969,#79970));
#19264=EDGE_LOOP('',(#79971,#79972,#79973,#79974));
#19265=EDGE_LOOP('',(#79975,#79976,#79977,#79978));
#19266=EDGE_LOOP('',(#79979,#79980,#79981,#79982));
#19267=EDGE_LOOP('',(#79983,#79984,#79985));
#19268=EDGE_LOOP('',(#79986,#79987,#79988,#79989));
#19269=EDGE_LOOP('',(#79990,#79991,#79992,#79993));
#19270=EDGE_LOOP('',(#79994,#79995,#79996,#79997));
#19271=EDGE_LOOP('',(#79998,#79999,#80000,#80001));
#19272=EDGE_LOOP('',(#80002,#80003,#80004,#80005));
#19273=EDGE_LOOP('',(#80006,#80007,#80008,#80009));
#19274=EDGE_LOOP('',(#80010,#80011,#80012,#80013));
#19275=EDGE_LOOP('',(#80014,#80015,#80016,#80017));
#19276=EDGE_LOOP('',(#80018,#80019,#80020,#80021));
#19277=EDGE_LOOP('',(#80022,#80023,#80024,#80025));
#19278=EDGE_LOOP('',(#80026,#80027,#80028,#80029));
#19279=EDGE_LOOP('',(#80030,#80031,#80032,#80033));
#19280=EDGE_LOOP('',(#80034,#80035,#80036,#80037));
#19281=EDGE_LOOP('',(#80038,#80039,#80040,#80041));
#19282=EDGE_LOOP('',(#80042,#80043,#80044,#80045));
#19283=EDGE_LOOP('',(#80046,#80047,#80048,#80049));
#19284=EDGE_LOOP('',(#80050,#80051,#80052,#80053));
#19285=EDGE_LOOP('',(#80054,#80055,#80056,#80057,#80058,#80059));
#19286=EDGE_LOOP('',(#80060,#80061,#80062,#80063));
#19287=EDGE_LOOP('',(#80064,#80065,#80066,#80067,#80068,#80069));
#19288=EDGE_LOOP('',(#80070,#80071,#80072,#80073));
#19289=EDGE_LOOP('',(#80074,#80075,#80076,#80077));
#19290=EDGE_LOOP('',(#80078,#80079,#80080,#80081));
#19291=EDGE_LOOP('',(#80082,#80083,#80084,#80085));
#19292=EDGE_LOOP('',(#80086,#80087,#80088,#80089));
#19293=EDGE_LOOP('',(#80090,#80091,#80092,#80093));
#19294=EDGE_LOOP('',(#80094,#80095,#80096,#80097));
#19295=EDGE_LOOP('',(#80098,#80099,#80100,#80101));
#19296=EDGE_LOOP('',(#80102,#80103,#80104,#80105));
#19297=EDGE_LOOP('',(#80106,#80107,#80108,#80109));
#19298=EDGE_LOOP('',(#80110,#80111,#80112,#80113));
#19299=EDGE_LOOP('',(#80114,#80115,#80116,#80117));
#19300=EDGE_LOOP('',(#80118,#80119,#80120,#80121));
#19301=EDGE_LOOP('',(#80122,#80123,#80124,#80125));
#19302=EDGE_LOOP('',(#80126,#80127,#80128,#80129));
#19303=EDGE_LOOP('',(#80130,#80131,#80132,#80133));
#19304=EDGE_LOOP('',(#80134,#80135,#80136));
#19305=EDGE_LOOP('',(#80137,#80138,#80139));
#19306=EDGE_LOOP('',(#80140,#80141,#80142,#80143));
#19307=EDGE_LOOP('',(#80144,#80145,#80146,#80147));
#19308=EDGE_LOOP('',(#80148,#80149,#80150,#80151));
#19309=EDGE_LOOP('',(#80152,#80153,#80154,#80155));
#19310=EDGE_LOOP('',(#80156,#80157,#80158,#80159));
#19311=EDGE_LOOP('',(#80160,#80161,#80162,#80163));
#19312=EDGE_LOOP('',(#80164,#80165,#80166,#80167));
#19313=EDGE_LOOP('',(#80168,#80169,#80170,#80171));
#19314=EDGE_LOOP('',(#80172,#80173,#80174,#80175));
#19315=EDGE_LOOP('',(#80176,#80177,#80178,#80179));
#19316=EDGE_LOOP('',(#80180,#80181,#80182,#80183));
#19317=EDGE_LOOP('',(#80184,#80185,#80186,#80187));
#19318=EDGE_LOOP('',(#80188,#80189,#80190,#80191));
#19319=EDGE_LOOP('',(#80192,#80193,#80194,#80195));
#19320=EDGE_LOOP('',(#80196,#80197,#80198,#80199));
#19321=EDGE_LOOP('',(#80200,#80201,#80202,#80203));
#19322=EDGE_LOOP('',(#80204,#80205,#80206,#80207));
#19323=EDGE_LOOP('',(#80208,#80209,#80210,#80211));
#19324=EDGE_LOOP('',(#80212,#80213,#80214,#80215));
#19325=EDGE_LOOP('',(#80216,#80217,#80218,#80219,#80220,#80221));
#19326=EDGE_LOOP('',(#80222,#80223,#80224,#80225));
#19327=EDGE_LOOP('',(#80226,#80227,#80228,#80229));
#19328=EDGE_LOOP('',(#80230,#80231,#80232,#80233));
#19329=EDGE_LOOP('',(#80234,#80235,#80236,#80237));
#19330=EDGE_LOOP('',(#80238,#80239,#80240,#80241));
#19331=EDGE_LOOP('',(#80242,#80243,#80244,#80245));
#19332=EDGE_LOOP('',(#80246,#80247,#80248,#80249));
#19333=EDGE_LOOP('',(#80250,#80251,#80252,#80253));
#19334=EDGE_LOOP('',(#80254,#80255,#80256,#80257));
#19335=EDGE_LOOP('',(#80258,#80259,#80260,#80261));
#19336=EDGE_LOOP('',(#80262,#80263,#80264,#80265));
#19337=EDGE_LOOP('',(#80266,#80267,#80268,#80269));
#19338=EDGE_LOOP('',(#80270,#80271,#80272,#80273));
#19339=EDGE_LOOP('',(#80274,#80275,#80276,#80277));
#19340=EDGE_LOOP('',(#80278,#80279,#80280,#80281));
#19341=EDGE_LOOP('',(#80282,#80283,#80284,#80285));
#19342=EDGE_LOOP('',(#80286,#80287,#80288));
#19343=EDGE_LOOP('',(#80289,#80290,#80291,#80292));
#19344=EDGE_LOOP('',(#80293,#80294,#80295,#80296,#80297,#80298));
#19345=EDGE_LOOP('',(#80299,#80300,#80301,#80302));
#19346=EDGE_LOOP('',(#80303,#80304,#80305,#80306));
#19347=EDGE_LOOP('',(#80307,#80308,#80309,#80310));
#19348=EDGE_LOOP('',(#80311,#80312,#80313,#80314));
#19349=EDGE_LOOP('',(#80315,#80316,#80317,#80318));
#19350=EDGE_LOOP('',(#80319,#80320,#80321,#80322));
#19351=EDGE_LOOP('',(#80323,#80324,#80325,#80326));
#19352=EDGE_LOOP('',(#80327,#80328,#80329,#80330));
#19353=EDGE_LOOP('',(#80331,#80332,#80333,#80334));
#19354=EDGE_LOOP('',(#80335,#80336,#80337,#80338));
#19355=EDGE_LOOP('',(#80339,#80340,#80341,#80342));
#19356=EDGE_LOOP('',(#80343,#80344,#80345,#80346));
#19357=EDGE_LOOP('',(#80347,#80348,#80349,#80350));
#19358=EDGE_LOOP('',(#80351,#80352,#80353,#80354));
#19359=EDGE_LOOP('',(#80355,#80356,#80357,#80358));
#19360=EDGE_LOOP('',(#80359,#80360,#80361,#80362));
#19361=EDGE_LOOP('',(#80363,#80364,#80365));
#19362=EDGE_LOOP('',(#80366,#80367,#80368,#80369,#80370,#80371,#80372,#80373));
#19363=EDGE_LOOP('',(#80374,#80375,#80376,#80377,#80378,#80379));
#19364=EDGE_LOOP('',(#80380,#80381,#80382,#80383,#80384,#80385,#80386));
#19365=EDGE_LOOP('',(#80387,#80388,#80389,#80390));
#19366=EDGE_LOOP('',(#80391,#80392,#80393,#80394));
#19367=EDGE_LOOP('',(#80395,#80396,#80397,#80398));
#19368=EDGE_LOOP('',(#80399,#80400,#80401,#80402));
#19369=EDGE_LOOP('',(#80403,#80404,#80405,#80406,#80407,#80408,#80409,#80410));
#19370=EDGE_LOOP('',(#80411));
#19371=EDGE_LOOP('',(#80412));
#19372=EDGE_LOOP('',(#80413,#80414,#80415,#80416,#80417,#80418,#80419,#80420,
#80421,#80422,#80423,#80424,#80425,#80426));
#19373=EDGE_LOOP('',(#80427));
#19374=EDGE_LOOP('',(#80428));
#19375=EDGE_LOOP('',(#80429,#80430,#80431,#80432));
#19376=EDGE_LOOP('',(#80433,#80434,#80435,#80436));
#19377=EDGE_LOOP('',(#80437));
#19378=EDGE_LOOP('',(#80438));
#19379=EDGE_LOOP('',(#80439));
#19380=EDGE_LOOP('',(#80440,#80441,#80442,#80443));
#19381=EDGE_LOOP('',(#80444,#80445,#80446,#80447));
#19382=EDGE_LOOP('',(#80448));
#19383=EDGE_LOOP('',(#80449));
#19384=EDGE_LOOP('',(#80450));
#19385=EDGE_LOOP('',(#80451,#80452,#80453,#80454));
#19386=EDGE_LOOP('',(#80455,#80456,#80457,#80458,#80459,#80460));
#19387=EDGE_LOOP('',(#80461));
#19388=EDGE_LOOP('',(#80462));
#19389=EDGE_LOOP('',(#80463));
#19390=EDGE_LOOP('',(#80464,#80465,#80466,#80467));
#19391=EDGE_LOOP('',(#80468,#80469,#80470,#80471,#80472,#80473));
#19392=EDGE_LOOP('',(#80474));
#19393=EDGE_LOOP('',(#80475,#80476,#80477,#80478,#80479));
#19394=EDGE_LOOP('',(#80480,#80481,#80482,#80483,#80484));
#19395=EDGE_LOOP('',(#80485,#80486,#80487,#80488,#80489,#80490));
#19396=EDGE_LOOP('',(#80491,#80492,#80493,#80494));
#19397=EDGE_LOOP('',(#80495,#80496,#80497,#80498));
#19398=EDGE_LOOP('',(#80499,#80500,#80501,#80502));
#19399=EDGE_LOOP('',(#80503,#80504,#80505,#80506));
#19400=EDGE_LOOP('',(#80507,#80508,#80509,#80510));
#19401=EDGE_LOOP('',(#80511,#80512,#80513,#80514));
#19402=EDGE_LOOP('',(#80515,#80516,#80517,#80518,#80519,#80520,#80521,#80522));
#19403=EDGE_LOOP('',(#80523,#80524));
#19404=EDGE_LOOP('',(#80525,#80526));
#19405=EDGE_LOOP('',(#80527,#80528));
#19406=EDGE_LOOP('',(#80529,#80530));
#19407=EDGE_LOOP('',(#80531,#80532));
#19408=EDGE_LOOP('',(#80533,#80534));
#19409=EDGE_LOOP('',(#80535,#80536,#80537,#80538,#80539,#80540));
#19410=EDGE_LOOP('',(#80541));
#19411=EDGE_LOOP('',(#80542,#80543,#80544,#80545,#80546,#80547));
#19412=EDGE_LOOP('',(#80548,#80549,#80550,#80551,#80552,#80553,#80554));
#19413=EDGE_LOOP('',(#80555,#80556));
#19414=EDGE_LOOP('',(#80557,#80558));
#19415=EDGE_LOOP('',(#80559,#80560));
#19416=EDGE_LOOP('',(#80561,#80562));
#19417=EDGE_LOOP('',(#80563,#80564,#80565));
#19418=EDGE_LOOP('',(#80566,#80567,#80568,#80569,#80570,#80571));
#19419=EDGE_LOOP('',(#80572,#80573,#80574,#80575));
#19420=EDGE_LOOP('',(#80576,#80577,#80578,#80579));
#19421=EDGE_LOOP('',(#80580,#80581,#80582,#80583));
#19422=EDGE_LOOP('',(#80584,#80585,#80586,#80587,#80588));
#19423=EDGE_LOOP('',(#80589,#80590,#80591));
#19424=EDGE_LOOP('',(#80592,#80593,#80594,#80595));
#19425=EDGE_LOOP('',(#80596,#80597,#80598));
#19426=EDGE_LOOP('',(#80599,#80600,#80601));
#19427=EDGE_LOOP('',(#80602,#80603,#80604,#80605));
#19428=EDGE_LOOP('',(#80606,#80607,#80608));
#19429=EDGE_LOOP('',(#80609,#80610,#80611,#80612,#80613));
#19430=EDGE_LOOP('',(#80614,#80615,#80616,#80617,#80618));
#19431=EDGE_LOOP('',(#80619,#80620,#80621,#80622,#80623));
#19432=EDGE_LOOP('',(#80624,#80625,#80626,#80627,#80628,#80629));
#19433=EDGE_LOOP('',(#80630,#80631,#80632,#80633,#80634,#80635));
#19434=EDGE_LOOP('',(#80636,#80637,#80638,#80639));
#19435=EDGE_LOOP('',(#80640,#80641,#80642,#80643,#80644));
#19436=EDGE_LOOP('',(#80645,#80646,#80647,#80648));
#19437=EDGE_LOOP('',(#80649,#80650,#80651,#80652));
#19438=EDGE_LOOP('',(#80653,#80654,#80655));
#19439=EDGE_LOOP('',(#80656,#80657,#80658,#80659));
#19440=EDGE_LOOP('',(#80660,#80661,#80662,#80663));
#19441=EDGE_LOOP('',(#80664,#80665,#80666,#80667));
#19442=EDGE_LOOP('',(#80668,#80669,#80670,#80671));
#19443=EDGE_LOOP('',(#80672,#80673,#80674));
#19444=EDGE_LOOP('',(#80675,#80676,#80677,#80678));
#19445=EDGE_LOOP('',(#80679,#80680,#80681,#80682));
#19446=EDGE_LOOP('',(#80683,#80684,#80685,#80686));
#19447=EDGE_LOOP('',(#80687,#80688,#80689,#80690));
#19448=EDGE_LOOP('',(#80691,#80692,#80693,#80694,#80695,#80696,#80697,#80698));
#19449=EDGE_LOOP('',(#80699,#80700,#80701,#80702,#80703));
#19450=EDGE_LOOP('',(#80704,#80705,#80706,#80707,#80708,#80709));
#19451=EDGE_LOOP('',(#80710,#80711,#80712,#80713,#80714,#80715,#80716,#80717,
#80718,#80719,#80720,#80721,#80722));
#19452=EDGE_LOOP('',(#80723,#80724,#80725,#80726));
#19453=EDGE_LOOP('',(#80727,#80728,#80729,#80730));
#19454=EDGE_LOOP('',(#80731,#80732,#80733,#80734));
#19455=EDGE_LOOP('',(#80735,#80736,#80737,#80738));
#19456=EDGE_LOOP('',(#80739,#80740,#80741,#80742));
#19457=EDGE_LOOP('',(#80743,#80744,#80745,#80746));
#19458=EDGE_LOOP('',(#80747,#80748,#80749,#80750));
#19459=EDGE_LOOP('',(#80751,#80752,#80753,#80754));
#19460=EDGE_LOOP('',(#80755,#80756,#80757,#80758));
#19461=EDGE_LOOP('',(#80759,#80760,#80761,#80762));
#19462=EDGE_LOOP('',(#80763,#80764,#80765,#80766));
#19463=EDGE_LOOP('',(#80767,#80768,#80769,#80770));
#19464=EDGE_LOOP('',(#80771,#80772,#80773,#80774));
#19465=EDGE_LOOP('',(#80775,#80776,#80777,#80778));
#19466=EDGE_LOOP('',(#80779,#80780,#80781,#80782,#80783));
#19467=EDGE_LOOP('',(#80784,#80785,#80786,#80787));
#19468=EDGE_LOOP('',(#80788,#80789,#80790,#80791));
#19469=EDGE_LOOP('',(#80792,#80793,#80794,#80795));
#19470=EDGE_LOOP('',(#80796,#80797,#80798,#80799));
#19471=EDGE_LOOP('',(#80800,#80801,#80802,#80803));
#19472=EDGE_LOOP('',(#80804,#80805,#80806,#80807));
#19473=EDGE_LOOP('',(#80808,#80809,#80810,#80811));
#19474=EDGE_LOOP('',(#80812,#80813,#80814,#80815));
#19475=EDGE_LOOP('',(#80816,#80817,#80818,#80819));
#19476=EDGE_LOOP('',(#80820,#80821,#80822,#80823));
#19477=EDGE_LOOP('',(#80824,#80825,#80826,#80827));
#19478=EDGE_LOOP('',(#80828,#80829,#80830,#80831));
#19479=EDGE_LOOP('',(#80832,#80833,#80834,#80835));
#19480=EDGE_LOOP('',(#80836,#80837,#80838,#80839));
#19481=EDGE_LOOP('',(#80840,#80841,#80842,#80843));
#19482=EDGE_LOOP('',(#80844,#80845,#80846,#80847));
#19483=EDGE_LOOP('',(#80848,#80849,#80850,#80851));
#19484=EDGE_LOOP('',(#80852,#80853,#80854,#80855));
#19485=EDGE_LOOP('',(#80856,#80857,#80858,#80859));
#19486=EDGE_LOOP('',(#80860,#80861,#80862,#80863));
#19487=EDGE_LOOP('',(#80864,#80865,#80866,#80867));
#19488=EDGE_LOOP('',(#80868,#80869,#80870,#80871));
#19489=EDGE_LOOP('',(#80872,#80873,#80874,#80875));
#19490=EDGE_LOOP('',(#80876,#80877,#80878,#80879));
#19491=EDGE_LOOP('',(#80880,#80881,#80882,#80883));
#19492=EDGE_LOOP('',(#80884,#80885,#80886,#80887));
#19493=EDGE_LOOP('',(#80888,#80889,#80890,#80891));
#19494=EDGE_LOOP('',(#80892,#80893,#80894,#80895));
#19495=EDGE_LOOP('',(#80896,#80897,#80898,#80899));
#19496=EDGE_LOOP('',(#80900,#80901,#80902,#80903));
#19497=EDGE_LOOP('',(#80904,#80905,#80906,#80907));
#19498=EDGE_LOOP('',(#80908,#80909,#80910,#80911));
#19499=EDGE_LOOP('',(#80912,#80913,#80914,#80915));
#19500=EDGE_LOOP('',(#80916,#80917,#80918,#80919));
#19501=EDGE_LOOP('',(#80920,#80921,#80922,#80923));
#19502=EDGE_LOOP('',(#80924,#80925,#80926,#80927));
#19503=EDGE_LOOP('',(#80928,#80929,#80930,#80931));
#19504=EDGE_LOOP('',(#80932,#80933,#80934,#80935));
#19505=EDGE_LOOP('',(#80936,#80937,#80938,#80939));
#19506=EDGE_LOOP('',(#80940,#80941,#80942,#80943));
#19507=EDGE_LOOP('',(#80944,#80945,#80946,#80947));
#19508=EDGE_LOOP('',(#80948,#80949,#80950,#80951));
#19509=EDGE_LOOP('',(#80952,#80953,#80954,#80955));
#19510=EDGE_LOOP('',(#80956,#80957,#80958,#80959));
#19511=EDGE_LOOP('',(#80960,#80961,#80962,#80963));
#19512=EDGE_LOOP('',(#80964,#80965,#80966,#80967));
#19513=EDGE_LOOP('',(#80968,#80969,#80970,#80971));
#19514=EDGE_LOOP('',(#80972,#80973,#80974,#80975,#80976));
#19515=EDGE_LOOP('',(#80977,#80978,#80979,#80980,#80981,#80982));
#19516=EDGE_LOOP('',(#80983,#80984,#80985,#80986));
#19517=EDGE_LOOP('',(#80987,#80988));
#19518=EDGE_LOOP('',(#80989,#80990));
#19519=EDGE_LOOP('',(#80991,#80992,#80993,#80994));
#19520=EDGE_LOOP('',(#80995,#80996));
#19521=EDGE_LOOP('',(#80997,#80998,#80999));
#19522=EDGE_LOOP('',(#81000,#81001,#81002,#81003,#81004));
#19523=EDGE_LOOP('',(#81005,#81006,#81007,#81008,#81009,#81010,#81011,#81012,
#81013,#81014));
#19524=EDGE_LOOP('',(#81015,#81016,#81017,#81018));
#19525=EDGE_LOOP('',(#81019,#81020));
#19526=EDGE_LOOP('',(#81021,#81022,#81023,#81024,#81025,#81026,#81027,#81028,
#81029,#81030,#81031,#81032,#81033,#81034,#81035,#81036,#81037,#81038,#81039,
#81040,#81041,#81042,#81043,#81044,#81045,#81046,#81047,#81048,#81049,#81050,
#81051,#81052,#81053,#81054,#81055,#81056,#81057,#81058,#81059,#81060,#81061,
#81062,#81063,#81064));
#19527=EDGE_LOOP('',(#81065,#81066,#81067,#81068));
#19528=EDGE_LOOP('',(#81069,#81070,#81071,#81072,#81073,#81074,#81075,#81076,
#81077,#81078,#81079,#81080,#81081,#81082,#81083,#81084,#81085,#81086,#81087,
#81088,#81089,#81090,#81091,#81092,#81093,#81094,#81095,#81096,#81097,#81098,
#81099,#81100,#81101,#81102,#81103,#81104,#81105,#81106,#81107,#81108,#81109));
#19529=EDGE_LOOP('',(#81110,#81111));
#19530=EDGE_LOOP('',(#81112,#81113));
#19531=EDGE_LOOP('',(#81114,#81115,#81116,#81117));
#19532=EDGE_LOOP('',(#81118,#81119,#81120));
#19533=EDGE_LOOP('',(#81121,#81122,#81123,#81124,#81125,#81126,#81127,#81128));
#19534=EDGE_LOOP('',(#81129,#81130,#81131,#81132));
#19535=EDGE_LOOP('',(#81133,#81134));
#19536=EDGE_LOOP('',(#81135,#81136,#81137,#81138,#81139,#81140,#81141,#81142,
#81143,#81144,#81145,#81146,#81147,#81148,#81149,#81150,#81151,#81152,#81153,
#81154,#81155,#81156,#81157,#81158,#81159,#81160,#81161,#81162,#81163,#81164,
#81165,#81166,#81167,#81168,#81169,#81170,#81171,#81172,#81173,#81174,#81175,
#81176,#81177,#81178));
#19537=EDGE_LOOP('',(#81179,#81180,#81181,#81182,#81183));
#19538=EDGE_LOOP('',(#81184,#81185,#81186,#81187,#81188,#81189,#81190,#81191,
#81192,#81193,#81194,#81195,#81196,#81197,#81198,#81199,#81200,#81201,#81202,
#81203,#81204,#81205,#81206,#81207,#81208,#81209,#81210,#81211,#81212,#81213,
#81214,#81215,#81216,#81217,#81218,#81219,#81220,#81221,#81222,#81223));
#19539=EDGE_LOOP('',(#81224,#81225,#81226,#81227));
#19540=EDGE_LOOP('',(#81228,#81229,#81230,#81231,#81232,#81233));
#19541=EDGE_LOOP('',(#81234,#81235));
#19542=EDGE_LOOP('',(#81236,#81237,#81238,#81239));
#19543=EDGE_LOOP('',(#81240,#81241,#81242));
#19544=EDGE_LOOP('',(#81243,#81244,#81245,#81246,#81247,#81248,#81249,#81250));
#19545=EDGE_LOOP('',(#81251,#81252,#81253,#81254));
#19546=EDGE_LOOP('',(#81255,#81256));
#19547=EDGE_LOOP('',(#81257,#81258,#81259,#81260,#81261,#81262,#81263,#81264,
#81265,#81266,#81267,#81268,#81269,#81270,#81271,#81272,#81273,#81274,#81275,
#81276,#81277,#81278,#81279,#81280,#81281,#81282,#81283,#81284,#81285,#81286,
#81287,#81288,#81289,#81290,#81291,#81292,#81293,#81294,#81295,#81296,#81297,
#81298,#81299));
#19548=EDGE_LOOP('',(#81300,#81301,#81302,#81303,#81304));
#19549=EDGE_LOOP('',(#81305,#81306,#81307,#81308,#81309,#81310,#81311,#81312,
#81313,#81314,#81315,#81316,#81317,#81318,#81319,#81320,#81321,#81322,#81323,
#81324,#81325,#81326,#81327,#81328,#81329,#81330,#81331,#81332,#81333,#81334,
#81335,#81336,#81337,#81338,#81339,#81340,#81341,#81342,#81343,#81344));
#19550=EDGE_LOOP('',(#81345,#81346,#81347,#81348));
#19551=EDGE_LOOP('',(#81349,#81350,#81351,#81352));
#19552=EDGE_LOOP('',(#81353,#81354));
#19553=EDGE_LOOP('',(#81355,#81356,#81357));
#19554=EDGE_LOOP('',(#81358,#81359,#81360,#81361,#81362));
#19555=EDGE_LOOP('',(#81363,#81364,#81365,#81366,#81367,#81368,#81369,#81370,
#81371,#81372));
#19556=EDGE_LOOP('',(#81373,#81374,#81375,#81376,#81377,#81378,#81379,#81380,
#81381,#81382,#81383,#81384,#81385,#81386,#81387,#81388,#81389,#81390,#81391,
#81392,#81393,#81394,#81395,#81396,#81397,#81398,#81399,#81400,#81401,#81402,
#81403,#81404));
#19557=EDGE_LOOP('',(#81405,#81406,#81407,#81408));
#19558=EDGE_LOOP('',(#81409,#81410,#81411,#81412));
#19559=EDGE_LOOP('',(#81413,#81414,#81415,#81416));
#19560=EDGE_LOOP('',(#81417,#81418,#81419,#81420));
#19561=EDGE_LOOP('',(#81421,#81422,#81423,#81424));
#19562=EDGE_LOOP('',(#81425,#81426));
#19563=EDGE_LOOP('',(#81427,#81428,#81429,#81430,#81431,#81432,#81433,#81434,
#81435,#81436,#81437,#81438,#81439,#81440,#81441,#81442,#81443,#81444,#81445,
#81446,#81447,#81448,#81449,#81450,#81451,#81452,#81453,#81454,#81455,#81456,
#81457,#81458,#81459,#81460,#81461,#81462,#81463,#81464,#81465,#81466,#81467,
#81468,#81469));
#19564=EDGE_LOOP('',(#81470,#81471,#81472));
#19565=EDGE_LOOP('',(#81473,#81474,#81475,#81476,#81477,#81478,#81479,#81480,
#81481,#81482,#81483,#81484,#81485,#81486,#81487,#81488,#81489,#81490,#81491,
#81492,#81493,#81494,#81495,#81496,#81497,#81498,#81499,#81500,#81501,#81502,
#81503,#81504,#81505,#81506,#81507,#81508,#81509,#81510,#81511,#81512,#81513));
#19566=EDGE_LOOP('',(#81514,#81515,#81516,#81517,#81518,#81519));
#19567=EDGE_LOOP('',(#81520,#81521,#81522,#81523,#81524,#81525));
#19568=EDGE_LOOP('',(#81526,#81527,#81528,#81529,#81530,#81531,#81532,#81533,
#81534,#81535,#81536,#81537,#81538,#81539,#81540,#81541,#81542,#81543,#81544,
#81545,#81546,#81547,#81548,#81549,#81550,#81551,#81552,#81553,#81554,#81555,
#81556,#81557,#81558,#81559,#81560,#81561,#81562,#81563));
#19569=EDGE_LOOP('',(#81564,#81565));
#19570=EDGE_LOOP('',(#81566,#81567));
#19571=EDGE_LOOP('',(#81568,#81569));
#19572=EDGE_LOOP('',(#81570,#81571));
#19573=EDGE_LOOP('',(#81572,#81573,#81574,#81575));
#19574=EDGE_LOOP('',(#81576,#81577,#81578,#81579,#81580,#81581));
#19575=EDGE_LOOP('',(#81582,#81583,#81584));
#19576=EDGE_LOOP('',(#81585,#81586,#81587,#81588,#81589));
#19577=EDGE_LOOP('',(#81590,#81591,#81592,#81593,#81594,#81595,#81596,#81597));
#19578=EDGE_LOOP('',(#81598,#81599,#81600));
#19579=EDGE_LOOP('',(#81601,#81602,#81603,#81604,#81605,#81606));
#19580=EDGE_LOOP('',(#81607,#81608,#81609,#81610,#81611,#81612));
#19581=EDGE_LOOP('',(#81613,#81614,#81615));
#19582=EDGE_LOOP('',(#81616,#81617,#81618,#81619,#81620,#81621));
#19583=EDGE_LOOP('',(#81622,#81623,#81624,#81625,#81626,#81627));
#19584=EDGE_LOOP('',(#81628,#81629,#81630));
#19585=EDGE_LOOP('',(#81631,#81632,#81633,#81634,#81635));
#19586=EDGE_LOOP('',(#81636,#81637,#81638,#81639));
#19587=EDGE_LOOP('',(#81640,#81641,#81642,#81643,#81644,#81645,#81646,#81647));
#19588=EDGE_LOOP('',(#81648,#81649,#81650,#81651));
#19589=EDGE_LOOP('',(#81652,#81653,#81654,#81655));
#19590=EDGE_LOOP('',(#81656,#81657,#81658,#81659));
#19591=EDGE_LOOP('',(#81660,#81661,#81662,#81663));
#19592=EDGE_LOOP('',(#81664,#81665,#81666,#81667));
#19593=EDGE_LOOP('',(#81668,#81669,#81670,#81671));
#19594=EDGE_LOOP('',(#81672,#81673,#81674));
#19595=EDGE_LOOP('',(#81675,#81676,#81677));
#19596=EDGE_LOOP('',(#81678,#81679,#81680,#81681));
#19597=EDGE_LOOP('',(#81682,#81683,#81684,#81685,#81686,#81687,#81688));
#19598=EDGE_LOOP('',(#81689,#81690,#81691,#81692));
#20561=LINE('',#131313,#24908);
#20562=LINE('',#131319,#24909);
#20563=LINE('',#131326,#24910);
#20564=LINE('',#131332,#24911);
#20565=LINE('',#131338,#24912);
#20566=LINE('',#131345,#24913);
#20567=LINE('',#131350,#24914);
#20568=LINE('',#131354,#24915);
#20569=LINE('',#131374,#24916);
#20570=LINE('',#131378,#24917);
#20571=LINE('',#131416,#24918);
#20572=LINE('',#131420,#24919);
#20573=LINE('',#131425,#24920);
#20574=LINE('',#131427,#24921);
#20575=LINE('',#131437,#24922);
#20576=LINE('',#131447,#24923);
#20577=LINE('',#131449,#24924);
#20578=LINE('',#131471,#24925);
#20579=LINE('',#131509,#24926);
#20580=LINE('',#131511,#24927);
#20581=LINE('',#131513,#24928);
#20582=LINE('',#131523,#24929);
#20583=LINE('',#131532,#24930);
#20584=LINE('',#131542,#24931);
#20585=LINE('',#131546,#24932);
#20586=LINE('',#131549,#24933);
#20587=LINE('',#131550,#24934);
#20588=LINE('',#131580,#24935);
#20589=LINE('',#131582,#24936);
#20590=LINE('',#131592,#24937);
#20591=LINE('',#131602,#24938);
#20592=LINE('',#131604,#24939);
#20593=LINE('',#131606,#24940);
#20594=LINE('',#131616,#24941);
#20595=LINE('',#131626,#24942);
#20596=LINE('',#131627,#24943);
#20597=LINE('',#131628,#24944);
#20598=LINE('',#131631,#24945);
#20599=LINE('',#131682,#24946);
#20600=LINE('',#131683,#24947);
#20601=LINE('',#131697,#24948);
#20602=LINE('',#131702,#24949);
#20603=LINE('',#131894,#24950);
#20604=LINE('',#131895,#24951);
#20605=LINE('',#131909,#24952);
#20606=LINE('',#131913,#24953);
#20607=LINE('',#132070,#24954);
#20608=LINE('',#132071,#24955);
#20609=LINE('',#132085,#24956);
#20610=LINE('',#132087,#24957);
#20611=LINE('',#132180,#24958);
#20612=LINE('',#132184,#24959);
#20613=LINE('',#132220,#24960);
#20614=LINE('',#132222,#24961);
#20615=LINE('',#132353,#24962);
#20616=LINE('',#132356,#24963);
#20617=LINE('',#132370,#24964);
#20618=LINE('',#132372,#24965);
#20619=LINE('',#132513,#24966);
#20620=LINE('',#132514,#24967);
#20621=LINE('',#132528,#24968);
#20622=LINE('',#132530,#24969);
#20623=LINE('',#132701,#24970);
#20624=LINE('',#132702,#24971);
#20625=LINE('',#132754,#24972);
#20626=LINE('',#132758,#24973);
#20627=LINE('',#132781,#24974);
#20628=LINE('',#132785,#24975);
#20629=LINE('',#132840,#24976);
#20630=LINE('',#132844,#24977);
#20631=LINE('',#132910,#24978);
#20632=LINE('',#132914,#24979);
#20633=LINE('',#132952,#24980);
#20634=LINE('',#132956,#24981);
#20635=LINE('',#133051,#24982);
#20636=LINE('',#133055,#24983);
#20637=LINE('',#133112,#24984);
#20638=LINE('',#133116,#24985);
#20639=LINE('',#133176,#24986);
#20640=LINE('',#133180,#24987);
#20641=LINE('',#133185,#24988);
#20642=LINE('',#133187,#24989);
#20643=LINE('',#133197,#24990);
#20644=LINE('',#133207,#24991);
#20645=LINE('',#133209,#24992);
#20646=LINE('',#133231,#24993);
#20647=LINE('',#133233,#24994);
#20648=LINE('',#133235,#24995);
#20649=LINE('',#133237,#24996);
#20650=LINE('',#133247,#24997);
#20651=LINE('',#133256,#24998);
#20652=LINE('',#133266,#24999);
#20653=LINE('',#133270,#25000);
#20654=LINE('',#133273,#25001);
#20655=LINE('',#133274,#25002);
#20656=LINE('',#133284,#25003);
#20657=LINE('',#133286,#25004);
#20658=LINE('',#133296,#25005);
#20659=LINE('',#133306,#25006);
#20660=LINE('',#133307,#25007);
#20661=LINE('',#133308,#25008);
#20662=LINE('',#133327,#25009);
#20663=LINE('',#133337,#25010);
#20664=LINE('',#133346,#25011);
#20665=LINE('',#133376,#25012);
#20666=LINE('',#133387,#25013);
#20667=LINE('',#133472,#25014);
#20668=LINE('',#133484,#25015);
#20669=LINE('',#133632,#25016);
#20670=LINE('',#133644,#25017);
#20671=LINE('',#133825,#25018);
#20672=LINE('',#133837,#25019);
#20673=LINE('',#133932,#25020);
#20674=LINE('',#133943,#25021);
#20675=LINE('',#134047,#25022);
#20676=LINE('',#134058,#25023);
#20677=LINE('',#134095,#25024);
#20678=LINE('',#134121,#25025);
#20679=LINE('',#134151,#25026);
#20680=LINE('',#134181,#25027);
#20681=LINE('',#134184,#25028);
#20682=LINE('',#134224,#25029);
#20683=LINE('',#134260,#25030);
#20684=LINE('',#134276,#25031);
#20685=LINE('',#134306,#25032);
#20686=LINE('',#134336,#25033);
#20687=LINE('',#134338,#25034);
#20688=LINE('',#134368,#25035);
#20689=LINE('',#134393,#25036);
#20690=LINE('',#134424,#25037);
#20691=LINE('',#134454,#25038);
#20692=LINE('',#134494,#25039);
#20693=LINE('',#134510,#25040);
#20694=LINE('',#134540,#25041);
#20695=LINE('',#134570,#25042);
#20696=LINE('',#134572,#25043);
#20697=LINE('',#134576,#25044);
#20698=LINE('',#134601,#25045);
#20699=LINE('',#134632,#25046);
#20700=LINE('',#134662,#25047);
#20701=LINE('',#134665,#25048);
#20702=LINE('',#134694,#25049);
#20703=LINE('',#134739,#25050);
#20704=LINE('',#134755,#25051);
#20705=LINE('',#134785,#25052);
#20706=LINE('',#134815,#25053);
#20707=LINE('',#134853,#25054);
#20708=LINE('',#134870,#25055);
#20709=LINE('',#134886,#25056);
#20710=LINE('',#134916,#25057);
#20711=LINE('',#134946,#25058);
#20712=LINE('',#134950,#25059);
#20713=LINE('',#134976,#25060);
#20714=LINE('',#135006,#25061);
#20715=LINE('',#135040,#25062);
#20716=LINE('',#135043,#25063);
#20717=LINE('',#135056,#25064);
#20718=LINE('',#135064,#25065);
#20719=LINE('',#135067,#25066);
#20720=LINE('',#135070,#25067);
#20721=LINE('',#135075,#25068);
#20722=LINE('',#135078,#25069);
#20723=LINE('',#135080,#25070);
#20724=LINE('',#135081,#25071);
#20725=LINE('',#135084,#25072);
#20726=LINE('',#135243,#25073);
#20727=LINE('',#135246,#25074);
#20728=LINE('',#135269,#25075);
#20729=LINE('',#135281,#25076);
#20730=LINE('',#135285,#25077);
#20731=LINE('',#135289,#25078);
#20732=LINE('',#135292,#25079);
#20733=LINE('',#135301,#25080);
#20734=LINE('',#135304,#25081);
#20735=LINE('',#135313,#25082);
#20736=LINE('',#135316,#25083);
#20737=LINE('',#135386,#25084);
#20738=LINE('',#135389,#25085);
#20739=LINE('',#135398,#25086);
#20740=LINE('',#135401,#25087);
#20741=LINE('',#135410,#25088);
#20742=LINE('',#135413,#25089);
#20743=LINE('',#135466,#25090);
#20744=LINE('',#135468,#25091);
#20745=LINE('',#135474,#25092);
#20746=LINE('',#135477,#25093);
#20747=LINE('',#135486,#25094);
#20748=LINE('',#135489,#25095);
#20749=LINE('',#135498,#25096);
#20750=LINE('',#135501,#25097);
#20751=LINE('',#135504,#25098);
#20752=LINE('',#135508,#25099);
#20753=LINE('',#135514,#25100);
#20754=LINE('',#135517,#25101);
#20755=LINE('',#135526,#25102);
#20756=LINE('',#135529,#25103);
#20757=LINE('',#135538,#25104);
#20758=LINE('',#135541,#25105);
#20759=LINE('',#135544,#25106);
#20760=LINE('',#135548,#25107);
#20761=LINE('',#135553,#25108);
#20762=LINE('',#135554,#25109);
#20763=LINE('',#135557,#25110);
#20764=LINE('',#135559,#25111);
#20765=LINE('',#135561,#25112);
#20766=LINE('',#135563,#25113);
#20767=LINE('',#135576,#25114);
#20768=LINE('',#135609,#25115);
#20769=LINE('',#135614,#25116);
#20770=LINE('',#135637,#25117);
#20771=LINE('',#135638,#25118);
#20772=LINE('',#135641,#25119);
#20773=LINE('',#135644,#25120);
#20774=LINE('',#135655,#25121);
#20775=LINE('',#135656,#25122);
#20776=LINE('',#135679,#25123);
#20777=LINE('',#135680,#25124);
#20778=LINE('',#135703,#25125);
#20779=LINE('',#135704,#25126);
#20780=LINE('',#135727,#25127);
#20781=LINE('',#135728,#25128);
#20782=LINE('',#135767,#25129);
#20783=LINE('',#135805,#25130);
#20784=LINE('',#135927,#25131);
#20785=LINE('',#135930,#25132);
#20786=LINE('',#135944,#25133);
#20787=LINE('',#135946,#25134);
#20788=LINE('',#136104,#25135);
#20789=LINE('',#136107,#25136);
#20790=LINE('',#136121,#25137);
#20791=LINE('',#136123,#25138);
#20792=LINE('',#136281,#25139);
#20793=LINE('',#136284,#25140);
#20794=LINE('',#136298,#25141);
#20795=LINE('',#136300,#25142);
#20796=LINE('',#136396,#25143);
#20797=LINE('',#136402,#25144);
#20798=LINE('',#136404,#25145);
#20799=LINE('',#136512,#25146);
#20800=LINE('',#136515,#25147);
#20801=LINE('',#136625,#25148);
#20802=LINE('',#136715,#25149);
#20803=LINE('',#136775,#25150);
#20804=LINE('',#137031,#25151);
#20805=LINE('',#137052,#25152);
#20806=LINE('',#137107,#25153);
#20807=LINE('',#137111,#25154);
#20808=LINE('',#137114,#25155);
#20809=LINE('',#137140,#25156);
#20810=LINE('',#137161,#25157);
#20811=LINE('',#137165,#25158);
#20812=LINE('',#137166,#25159);
#20813=LINE('',#137169,#25160);
#20814=LINE('',#137188,#25161);
#20815=LINE('',#137192,#25162);
#20816=LINE('',#137217,#25163);
#20817=LINE('',#137273,#25164);
#20818=LINE('',#137277,#25165);
#20819=LINE('',#137280,#25166);
#20820=LINE('',#137315,#25167);
#20821=LINE('',#137372,#25168);
#20822=LINE('',#137375,#25169);
#20823=LINE('',#137379,#25170);
#20824=LINE('',#137405,#25171);
#20825=LINE('',#137409,#25172);
#20826=LINE('',#137410,#25173);
#20827=LINE('',#137413,#25174);
#20828=LINE('',#137433,#25175);
#20829=LINE('',#137436,#25176);
#20830=LINE('',#137549,#25177);
#20831=LINE('',#137834,#25178);
#20832=LINE('',#137892,#25179);
#20833=LINE('',#138042,#25180);
#20834=LINE('',#138045,#25181);
#20835=LINE('',#138048,#25182);
#20836=LINE('',#138051,#25183);
#20837=LINE('',#138052,#25184);
#20838=LINE('',#138055,#25185);
#20839=LINE('',#138059,#25186);
#20840=LINE('',#138062,#25187);
#20841=LINE('',#138065,#25188);
#20842=LINE('',#138066,#25189);
#20843=LINE('',#138069,#25190);
#20844=LINE('',#138074,#25191);
#20845=LINE('',#138078,#25192);
#20846=LINE('',#138117,#25193);
#20847=LINE('',#138151,#25194);
#20848=LINE('',#138204,#25195);
#20849=LINE('',#138208,#25196);
#20850=LINE('',#138212,#25197);
#20851=LINE('',#138214,#25198);
#20852=LINE('',#138235,#25199);
#20853=LINE('',#138262,#25200);
#20854=LINE('',#138266,#25201);
#20855=LINE('',#138267,#25202);
#20856=LINE('',#138270,#25203);
#20857=LINE('',#138314,#25204);
#20858=LINE('',#138340,#25205);
#20859=LINE('',#138344,#25206);
#20860=LINE('',#138439,#25207);
#20861=LINE('',#138479,#25208);
#20862=LINE('',#138502,#25209);
#20863=LINE('',#138743,#25210);
#20864=LINE('',#138764,#25211);
#20865=LINE('',#138786,#25212);
#20866=LINE('',#138850,#25213);
#20867=LINE('',#138878,#25214);
#20868=LINE('',#138889,#25215);
#20869=LINE('',#139046,#25216);
#20870=LINE('',#139057,#25217);
#20871=LINE('',#139084,#25218);
#20872=LINE('',#139159,#25219);
#20873=LINE('',#139199,#25220);
#20874=LINE('',#139222,#25221);
#20875=LINE('',#139447,#25222);
#20876=LINE('',#139470,#25223);
#20877=LINE('',#139512,#25224);
#20878=LINE('',#139551,#25225);
#20879=LINE('',#139555,#25226);
#20880=LINE('',#139559,#25227);
#20881=LINE('',#139588,#25228);
#20882=LINE('',#139612,#25229);
#20883=LINE('',#139616,#25230);
#20884=LINE('',#139617,#25231);
#20885=LINE('',#139620,#25232);
#20886=LINE('',#139656,#25233);
#20887=LINE('',#139685,#25234);
#20888=LINE('',#139687,#25235);
#20889=LINE('',#139691,#25236);
#20890=LINE('',#139769,#25237);
#20891=LINE('',#139803,#25238);
#20892=LINE('',#139807,#25239);
#20893=LINE('',#139808,#25240);
#20894=LINE('',#139818,#25241);
#20895=LINE('',#139819,#25242);
#20896=LINE('',#139918,#25243);
#20897=LINE('',#139968,#25244);
#20898=LINE('',#140003,#25245);
#20899=LINE('',#140005,#25246);
#20900=LINE('',#140009,#25247);
#20901=LINE('',#140013,#25248);
#20902=LINE('',#140014,#25249);
#20903=LINE('',#140017,#25250);
#20904=LINE('',#140021,#25251);
#20905=LINE('',#140022,#25252);
#20906=LINE('',#140025,#25253);
#20907=LINE('',#140062,#25254);
#20908=LINE('',#140075,#25255);
#20909=LINE('',#140077,#25256);
#20910=LINE('',#140081,#25257);
#20911=LINE('',#140095,#25258);
#20912=LINE('',#140135,#25259);
#20913=LINE('',#140137,#25260);
#20914=LINE('',#140138,#25261);
#20915=LINE('',#140224,#25262);
#20916=LINE('',#140228,#25263);
#20917=LINE('',#140252,#25264);
#20918=LINE('',#140300,#25265);
#20919=LINE('',#140317,#25266);
#20920=LINE('',#140362,#25267);
#20921=LINE('',#140366,#25268);
#20922=LINE('',#140370,#25269);
#20923=LINE('',#140372,#25270);
#20924=LINE('',#140385,#25271);
#20925=LINE('',#140429,#25272);
#20926=LINE('',#140463,#25273);
#20927=LINE('',#140466,#25274);
#20928=LINE('',#140470,#25275);
#20929=LINE('',#140471,#25276);
#20930=LINE('',#140474,#25277);
#20931=LINE('',#140479,#25278);
#20932=LINE('',#140483,#25279);
#20933=LINE('',#140486,#25280);
#20934=LINE('',#140542,#25281);
#20935=LINE('',#140583,#25282);
#20936=LINE('',#140595,#25283);
#20937=LINE('',#140600,#25284);
#20938=LINE('',#140601,#25285);
#20939=LINE('',#140688,#25286);
#20940=LINE('',#140691,#25287);
#20941=LINE('',#140695,#25288);
#20942=LINE('',#140735,#25289);
#20943=LINE('',#140738,#25290);
#20944=LINE('',#140742,#25291);
#20945=LINE('',#140743,#25292);
#20946=LINE('',#140746,#25293);
#20947=LINE('',#140830,#25294);
#20948=LINE('',#140833,#25295);
#20949=LINE('',#140920,#25296);
#20950=LINE('',#140921,#25297);
#20951=LINE('',#140923,#25298);
#20952=LINE('',#140927,#25299);
#20953=LINE('',#140928,#25300);
#20954=LINE('',#140931,#25301);
#20955=LINE('',#140935,#25302);
#20956=LINE('',#140936,#25303);
#20957=LINE('',#140939,#25304);
#20958=LINE('',#140943,#25305);
#20959=LINE('',#140946,#25306);
#20960=LINE('',#140990,#25307);
#20961=LINE('',#140996,#25308);
#20962=LINE('',#140997,#25309);
#20963=LINE('',#141096,#25310);
#20964=LINE('',#141143,#25311);
#20965=LINE('',#141180,#25312);
#20966=LINE('',#141182,#25313);
#20967=LINE('',#141186,#25314);
#20968=LINE('',#141190,#25315);
#20969=LINE('',#141191,#25316);
#20970=LINE('',#141194,#25317);
#20971=LINE('',#141198,#25318);
#20972=LINE('',#141199,#25319);
#20973=LINE('',#141202,#25320);
#20974=LINE('',#141249,#25321);
#20975=LINE('',#141251,#25322);
#20976=LINE('',#141273,#25323);
#20977=LINE('',#141286,#25324);
#20978=LINE('',#141288,#25325);
#20979=LINE('',#141292,#25326);
#20980=LINE('',#141295,#25327);
#20981=LINE('',#141317,#25328);
#20982=LINE('',#141319,#25329);
#20983=LINE('',#141324,#25330);
#20984=LINE('',#141328,#25331);
#20985=LINE('',#141362,#25332);
#20986=LINE('',#141416,#25333);
#20987=LINE('',#141467,#25334);
#20988=LINE('',#141512,#25335);
#20989=LINE('',#141516,#25336);
#20990=LINE('',#141520,#25337);
#20991=LINE('',#141522,#25338);
#20992=LINE('',#141535,#25339);
#20993=LINE('',#141579,#25340);
#20994=LINE('',#141616,#25341);
#20995=LINE('',#141619,#25342);
#20996=LINE('',#141623,#25343);
#20997=LINE('',#141624,#25344);
#20998=LINE('',#141627,#25345);
#20999=LINE('',#141632,#25346);
#21000=LINE('',#141636,#25347);
#21001=LINE('',#141639,#25348);
#21002=LINE('',#141689,#25349);
#21003=LINE('',#141730,#25350);
#21004=LINE('',#141742,#25351);
#21005=LINE('',#141858,#25352);
#21006=LINE('',#141897,#25353);
#21007=LINE('',#141901,#25354);
#21008=LINE('',#141902,#25355);
#21009=LINE('',#141959,#25356);
#21010=LINE('',#141993,#25357);
#21011=LINE('',#141995,#25358);
#21012=LINE('',#141997,#25359);
#21013=LINE('',#142027,#25360);
#21014=LINE('',#142029,#25361);
#21015=LINE('',#142033,#25362);
#21016=LINE('',#142037,#25363);
#21017=LINE('',#142038,#25364);
#21018=LINE('',#142041,#25365);
#21019=LINE('',#142045,#25366);
#21020=LINE('',#142046,#25367);
#21021=LINE('',#142049,#25368);
#21022=LINE('',#142054,#25369);
#21023=LINE('',#142058,#25370);
#21024=LINE('',#142072,#25371);
#21025=LINE('',#142119,#25372);
#21026=LINE('',#142157,#25373);
#21027=LINE('',#142169,#25374);
#21028=LINE('',#142205,#25375);
#21029=LINE('',#142206,#25376);
#21030=LINE('',#142254,#25377);
#21031=LINE('',#142258,#25378);
#21032=LINE('',#142262,#25379);
#21033=LINE('',#142264,#25380);
#21034=LINE('',#142277,#25381);
#21035=LINE('',#142327,#25382);
#21036=LINE('',#142367,#25383);
#21037=LINE('',#142370,#25384);
#21038=LINE('',#142374,#25385);
#21039=LINE('',#142375,#25386);
#21040=LINE('',#142378,#25387);
#21041=LINE('',#142425,#25388);
#21042=LINE('',#142429,#25389);
#21043=LINE('',#142432,#25390);
#21044=LINE('',#142488,#25391);
#21045=LINE('',#142526,#25392);
#21046=LINE('',#142538,#25393);
#21047=LINE('',#142540,#25394);
#21048=LINE('',#142547,#25395);
#21049=LINE('',#142554,#25396);
#21050=LINE('',#142608,#25397);
#21051=LINE('',#142614,#25398);
#21052=LINE('',#142668,#25399);
#21053=LINE('',#142674,#25400);
#21054=LINE('',#142678,#25401);
#21055=LINE('',#142679,#25402);
#21056=LINE('',#142795,#25403);
#21057=LINE('',#142797,#25404);
#21058=LINE('',#142874,#25405);
#21059=LINE('',#142876,#25406);
#21060=LINE('',#142972,#25407);
#21061=LINE('',#142985,#25408);
#21062=LINE('',#142989,#25409);
#21063=LINE('',#142990,#25410);
#21064=LINE('',#143005,#25411);
#21065=LINE('',#143023,#25412);
#21066=LINE('',#143036,#25413);
#21067=LINE('',#143040,#25414);
#21068=LINE('',#143041,#25415);
#21069=LINE('',#143056,#25416);
#21070=LINE('',#143071,#25417);
#21071=LINE('',#143088,#25418);
#21072=LINE('',#143123,#25419);
#21073=LINE('',#143169,#25420);
#21074=LINE('',#143215,#25421);
#21075=LINE('',#143216,#25422);
#21076=LINE('',#143219,#25423);
#21077=LINE('',#143223,#25424);
#21078=LINE('',#143227,#25425);
#21079=LINE('',#143231,#25426);
#21080=LINE('',#143233,#25427);
#21081=LINE('',#143249,#25428);
#21082=LINE('',#143251,#25429);
#21083=LINE('',#143261,#25430);
#21084=LINE('',#143271,#25431);
#21085=LINE('',#143273,#25432);
#21086=LINE('',#143275,#25433);
#21087=LINE('',#143285,#25434);
#21088=LINE('',#143294,#25435);
#21089=LINE('',#143298,#25436);
#21090=LINE('',#143304,#25437);
#21091=LINE('',#143313,#25438);
#21092=LINE('',#143366,#25439);
#21093=LINE('',#143370,#25440);
#21094=LINE('',#143392,#25441);
#21095=LINE('',#143396,#25442);
#21096=LINE('',#143453,#25443);
#21097=LINE('',#143457,#25444);
#21098=LINE('',#143511,#25445);
#21099=LINE('',#143515,#25446);
#21100=LINE('',#143576,#25447);
#21101=LINE('',#143580,#25448);
#21102=LINE('',#143641,#25449);
#21103=LINE('',#143645,#25450);
#21104=LINE('',#143698,#25451);
#21105=LINE('',#143705,#25452);
#21106=LINE('',#143715,#25453);
#21107=LINE('',#143717,#25454);
#21108=LINE('',#143727,#25455);
#21109=LINE('',#143737,#25456);
#21110=LINE('',#143739,#25457);
#21111=LINE('',#143754,#25458);
#21112=LINE('',#143756,#25459);
#21113=LINE('',#143758,#25460);
#21114=LINE('',#143768,#25461);
#21115=LINE('',#143777,#25462);
#21116=LINE('',#143780,#25463);
#21117=LINE('',#143784,#25464);
#21118=LINE('',#143788,#25465);
#21119=LINE('',#143792,#25466);
#21120=LINE('',#143808,#25467);
#21121=LINE('',#143810,#25468);
#21122=LINE('',#143820,#25469);
#21123=LINE('',#143830,#25470);
#21124=LINE('',#143832,#25471);
#21125=LINE('',#143834,#25472);
#21126=LINE('',#143844,#25473);
#21127=LINE('',#143853,#25474);
#21128=LINE('',#143889,#25475);
#21129=LINE('',#143897,#25476);
#21130=LINE('',#143898,#25477);
#21131=LINE('',#143899,#25478);
#21132=LINE('',#143934,#25479);
#21133=LINE('',#143937,#25480);
#21134=LINE('',#143972,#25481);
#21135=LINE('',#143980,#25482);
#21136=LINE('',#143981,#25483);
#21137=LINE('',#143983,#25484);
#21138=LINE('',#143987,#25485);
#21139=LINE('',#144034,#25486);
#21140=LINE('',#144038,#25487);
#21141=LINE('',#144039,#25488);
#21142=LINE('',#144324,#25489);
#21143=LINE('',#144327,#25490);
#21144=LINE('',#144372,#25491);
#21145=LINE('',#144472,#25492);
#21146=LINE('',#144530,#25493);
#21147=LINE('',#144532,#25494);
#21148=LINE('',#144608,#25495);
#21149=LINE('',#144709,#25496);
#21150=LINE('',#144776,#25497);
#21151=LINE('',#144782,#25498);
#21152=LINE('',#144862,#25499);
#21153=LINE('',#144890,#25500);
#21154=LINE('',#144969,#25501);
#21155=LINE('',#145038,#25502);
#21156=LINE('',#145254,#25503);
#21157=LINE('',#145264,#25504);
#21158=LINE('',#145270,#25505);
#21159=LINE('',#145355,#25506);
#21160=LINE('',#145427,#25507);
#21161=LINE('',#145540,#25508);
#21162=LINE('',#145613,#25509);
#21163=LINE('',#145629,#25510);
#21164=LINE('',#145635,#25511);
#21165=LINE('',#145660,#25512);
#21166=LINE('',#145743,#25513);
#21167=LINE('',#145894,#25514);
#21168=LINE('',#146025,#25515);
#21169=LINE('',#146028,#25516);
#21170=LINE('',#146214,#25517);
#21171=LINE('',#146329,#25518);
#21172=LINE('',#146469,#25519);
#21173=LINE('',#146472,#25520);
#21174=LINE('',#146596,#25521);
#21175=LINE('',#146702,#25522);
#21176=LINE('',#146885,#25523);
#21177=LINE('',#146888,#25524);
#21178=LINE('',#147055,#25525);
#21179=LINE('',#147171,#25526);
#21180=LINE('',#147276,#25527);
#21181=LINE('',#147282,#25528);
#21182=LINE('',#147307,#25529);
#21183=LINE('',#147314,#25530);
#21184=LINE('',#147447,#25531);
#21185=LINE('',#147558,#25532);
#21186=LINE('',#147574,#25533);
#21187=LINE('',#147597,#25534);
#21188=LINE('',#147766,#25535);
#21189=LINE('',#147780,#25536);
#21190=LINE('',#147853,#25537);
#21191=LINE('',#147971,#25538);
#21192=LINE('',#147974,#25539);
#21193=LINE('',#147986,#25540);
#21194=LINE('',#148021,#25541);
#21195=LINE('',#148028,#25542);
#21196=LINE('',#148199,#25543);
#21197=LINE('',#148253,#25544);
#21198=LINE('',#148345,#25545);
#21199=LINE('',#148481,#25546);
#21200=LINE('',#148529,#25547);
#21201=LINE('',#148543,#25548);
#21202=LINE('',#148549,#25549);
#21203=LINE('',#148555,#25550);
#21204=LINE('',#148611,#25551);
#21205=LINE('',#148725,#25552);
#21206=LINE('',#148798,#25553);
#21207=LINE('',#149017,#25554);
#21208=LINE('',#149177,#25555);
#21209=LINE('',#149191,#25556);
#21210=LINE('',#149327,#25557);
#21211=LINE('',#149468,#25558);
#21212=LINE('',#149471,#25559);
#21213=LINE('',#149476,#25560);
#21214=LINE('',#149510,#25561);
#21215=LINE('',#149517,#25562);
#21216=LINE('',#149585,#25563);
#21217=LINE('',#149742,#25564);
#21218=LINE('',#149832,#25565);
#21219=LINE('',#149927,#25566);
#21220=LINE('',#150033,#25567);
#21221=LINE('',#150081,#25568);
#21222=LINE('',#150095,#25569);
#21223=LINE('',#150101,#25570);
#21224=LINE('',#150107,#25571);
#21225=LINE('',#150163,#25572);
#21226=LINE('',#150277,#25573);
#21227=LINE('',#150388,#25574);
#21228=LINE('',#150496,#25575);
#21229=LINE('',#150503,#25576);
#21230=LINE('',#150583,#25577);
#21231=LINE('',#150707,#25578);
#21232=LINE('',#150721,#25579);
#21233=LINE('',#150758,#25580);
#21234=LINE('',#150765,#25581);
#21235=LINE('',#150771,#25582);
#21236=LINE('',#150829,#25583);
#21237=LINE('',#150974,#25584);
#21238=LINE('',#151117,#25585);
#21239=LINE('',#151240,#25586);
#21240=LINE('',#151360,#25587);
#21241=LINE('',#151408,#25588);
#21242=LINE('',#151422,#25589);
#21243=LINE('',#151428,#25590);
#21244=LINE('',#151435,#25591);
#21245=LINE('',#151493,#25592);
#21246=LINE('',#151585,#25593);
#21247=LINE('',#151669,#25594);
#21248=LINE('',#151676,#25595);
#21249=LINE('',#151751,#25596);
#21250=LINE('',#151771,#25597);
#21251=LINE('',#151793,#25598);
#21252=LINE('',#151815,#25599);
#21253=LINE('',#152356,#25600);
#21254=LINE('',#152378,#25601);
#21255=LINE('',#152426,#25602);
#21256=LINE('',#152448,#25603);
#21257=LINE('',#152495,#25604);
#21258=LINE('',#152515,#25605);
#21259=LINE('',#152537,#25606);
#21260=LINE('',#152559,#25607);
#21261=LINE('',#152639,#25608);
#21262=LINE('',#152732,#25609);
#21263=LINE('',#152734,#25610);
#21264=LINE('',#152736,#25611);
#21265=LINE('',#152785,#25612);
#21266=LINE('',#152786,#25613);
#21267=LINE('',#152788,#25614);
#21268=LINE('',#153027,#25615);
#21269=LINE('',#153029,#25616);
#21270=LINE('',#153030,#25617);
#21271=LINE('',#153080,#25618);
#21272=LINE('',#153104,#25619);
#21273=LINE('',#153106,#25620);
#21274=LINE('',#153197,#25621);
#21275=LINE('',#153199,#25622);
#21276=LINE('',#153209,#25623);
#21277=LINE('',#153211,#25624);
#21278=LINE('',#153331,#25625);
#21279=LINE('',#153333,#25626);
#21280=LINE('',#153410,#25627);
#21281=LINE('',#153412,#25628);
#21282=LINE('',#153462,#25629);
#21283=LINE('',#153464,#25630);
#21284=LINE('',#153472,#25631);
#21285=LINE('',#153473,#25632);
#21286=LINE('',#153477,#25633);
#21287=LINE('',#153479,#25634);
#21288=LINE('',#153481,#25635);
#21289=LINE('',#153482,#25636);
#21290=LINE('',#153487,#25637);
#21291=LINE('',#153491,#25638);
#21292=LINE('',#153493,#25639);
#21293=LINE('',#153494,#25640);
#21294=LINE('',#153798,#25641);
#21295=LINE('',#153799,#25642);
#21296=LINE('',#154231,#25643);
#21297=LINE('',#154232,#25644);
#21298=LINE('',#154233,#25645);
#21299=LINE('',#154237,#25646);
#21300=LINE('',#154239,#25647);
#21301=LINE('',#154241,#25648);
#21302=LINE('',#154242,#25649);
#21303=LINE('',#154247,#25650);
#21304=LINE('',#154251,#25651);
#21305=LINE('',#154253,#25652);
#21306=LINE('',#154254,#25653);
#21307=LINE('',#154603,#25654);
#21308=LINE('',#154618,#25655);
#21309=LINE('',#154810,#25656);
#21310=LINE('',#154812,#25657);
#21311=LINE('',#154814,#25658);
#21312=LINE('',#154815,#25659);
#21313=LINE('',#154820,#25660);
#21314=LINE('',#154824,#25661);
#21315=LINE('',#154826,#25662);
#21316=LINE('',#154827,#25663);
#21317=LINE('',#154831,#25664);
#21318=LINE('',#154833,#25665);
#21319=LINE('',#154997,#25666);
#21320=LINE('',#154998,#25667);
#21321=LINE('',#155371,#25668);
#21322=LINE('',#155373,#25669);
#21323=LINE('',#155376,#25670);
#21324=LINE('',#155810,#25671);
#21325=LINE('',#155816,#25672);
#21326=LINE('',#156128,#25673);
#21327=LINE('',#156130,#25674);
#21328=LINE('',#156132,#25675);
#21329=LINE('',#156133,#25676);
#21330=LINE('',#156137,#25677);
#21331=LINE('',#156142,#25678);
#21332=LINE('',#156144,#25679);
#21333=LINE('',#156145,#25680);
#21334=LINE('',#156240,#25681);
#21335=LINE('',#156242,#25682);
#21336=LINE('',#156244,#25683);
#21337=LINE('',#156245,#25684);
#21338=LINE('',#156250,#25685);
#21339=LINE('',#156254,#25686);
#21340=LINE('',#156256,#25687);
#21341=LINE('',#156257,#25688);
#21342=LINE('',#156261,#25689);
#21343=LINE('',#156263,#25690);
#21344=LINE('',#156427,#25691);
#21345=LINE('',#156428,#25692);
#21346=LINE('',#156709,#25693);
#21347=LINE('',#156711,#25694);
#21348=LINE('',#156714,#25695);
#21349=LINE('',#157090,#25696);
#21350=LINE('',#157096,#25697);
#21351=LINE('',#157100,#25698);
#21352=LINE('',#157102,#25699);
#21353=LINE('',#157104,#25700);
#21354=LINE('',#157105,#25701);
#21355=LINE('',#157109,#25702);
#21356=LINE('',#157114,#25703);
#21357=LINE('',#157116,#25704);
#21358=LINE('',#157117,#25705);
#21359=LINE('',#157344,#25706);
#21360=LINE('',#157348,#25707);
#21361=LINE('',#157352,#25708);
#21362=LINE('',#157355,#25709);
#21363=LINE('',#157379,#25710);
#21364=LINE('',#157400,#25711);
#21365=LINE('',#157647,#25712);
#21366=LINE('',#157651,#25713);
#21367=LINE('',#157652,#25714);
#21368=LINE('',#157656,#25715);
#21369=LINE('',#157658,#25716);
#21370=LINE('',#157660,#25717);
#21371=LINE('',#157661,#25718);
#21372=LINE('',#157722,#25719);
#21373=LINE('',#157743,#25720);
#21374=LINE('',#158254,#25721);
#21375=LINE('',#158281,#25722);
#21376=LINE('',#158569,#25723);
#21377=LINE('',#158593,#25724);
#21378=LINE('',#158974,#25725);
#21379=LINE('',#158995,#25726);
#21380=LINE('',#159250,#25727);
#21381=LINE('',#159270,#25728);
#21382=LINE('',#159272,#25729);
#21383=LINE('',#159274,#25730);
#21384=LINE('',#159275,#25731);
#21385=LINE('',#159279,#25732);
#21386=LINE('',#159283,#25733);
#21387=LINE('',#159288,#25734);
#21388=LINE('',#159292,#25735);
#21389=LINE('',#159317,#25736);
#21390=LINE('',#159338,#25737);
#21391=LINE('',#159553,#25738);
#21392=LINE('',#159556,#25739);
#21393=LINE('',#159560,#25740);
#21394=LINE('',#159561,#25741);
#21395=LINE('',#159562,#25742);
#21396=LINE('',#159566,#25743);
#21397=LINE('',#159567,#25744);
#21398=LINE('',#159568,#25745);
#21399=LINE('',#159592,#25746);
#21400=LINE('',#159610,#25747);
#21401=LINE('',#159614,#25748);
#21402=LINE('',#159616,#25749);
#21403=LINE('',#159618,#25750);
#21404=LINE('',#159619,#25751);
#21405=LINE('',#159640,#25752);
#21406=LINE('',#159658,#25753);
#21407=LINE('',#159688,#25754);
#21408=LINE('',#159715,#25755);
#21409=LINE('',#159719,#25756);
#21410=LINE('',#159723,#25757);
#21411=LINE('',#160105,#25758);
#21412=LINE('',#160415,#25759);
#21413=LINE('',#160576,#25760);
#21414=LINE('',#160655,#25761);
#21415=LINE('',#160886,#25762);
#21416=LINE('',#160965,#25763);
#21417=LINE('',#161038,#25764);
#21418=LINE('',#161139,#25765);
#21419=LINE('',#161300,#25766);
#21420=LINE('',#161337,#25767);
#21421=LINE('',#161409,#25768);
#21422=LINE('',#161491,#25769);
#21423=LINE('',#161576,#25770);
#21424=LINE('',#163686,#25771);
#21425=LINE('',#163847,#25772);
#21426=LINE('',#163926,#25773);
#21427=LINE('',#164157,#25774);
#21428=LINE('',#164236,#25775);
#21429=LINE('',#164309,#25776);
#21430=LINE('',#164331,#25777);
#21431=LINE('',#164403,#25778);
#21432=LINE('',#164892,#25779);
#21433=LINE('',#164893,#25780);
#21434=LINE('',#164894,#25781);
#21435=LINE('',#164898,#25782);
#21436=LINE('',#164941,#25783);
#21437=LINE('',#164947,#25784);
#21438=LINE('',#164948,#25785);
#21439=LINE('',#164957,#25786);
#21440=LINE('',#165053,#25787);
#21441=LINE('',#165156,#25788);
#21442=LINE('',#165202,#25789);
#21443=LINE('',#165203,#25790);
#21444=LINE('',#165205,#25791);
#21445=LINE('',#165211,#25792);
#21446=LINE('',#165214,#25793);
#21447=LINE('',#165223,#25794);
#21448=LINE('',#165233,#25795);
#21449=LINE('',#165240,#25796);
#21450=LINE('',#165243,#25797);
#21451=LINE('',#165245,#25798);
#21452=LINE('',#165290,#25799);
#21453=LINE('',#165399,#25800);
#21454=LINE('',#165576,#25801);
#21455=LINE('',#165579,#25802);
#21456=LINE('',#165661,#25803);
#21457=LINE('',#165668,#25804);
#21458=LINE('',#165670,#25805);
#21459=LINE('',#165793,#25806);
#21460=LINE('',#165909,#25807);
#21461=LINE('',#165955,#25808);
#21462=LINE('',#165956,#25809);
#21463=LINE('',#165958,#25810);
#21464=LINE('',#165967,#25811);
#21465=LINE('',#165973,#25812);
#21466=LINE('',#165976,#25813);
#21467=LINE('',#165979,#25814);
#21468=LINE('',#165982,#25815);
#21469=LINE('',#165985,#25816);
#21470=LINE('',#166083,#25817);
#21471=LINE('',#166089,#25818);
#21472=LINE('',#166093,#25819);
#21473=LINE('',#166094,#25820);
#21474=LINE('',#166227,#25821);
#21475=LINE('',#166333,#25822);
#21476=LINE('',#166340,#25823);
#21477=LINE('',#166344,#25824);
#21478=LINE('',#166345,#25825);
#21479=LINE('',#166469,#25826);
#21480=LINE('',#166637,#25827);
#21481=LINE('',#166737,#25828);
#21482=LINE('',#166781,#25829);
#21483=LINE('',#166782,#25830);
#21484=LINE('',#166784,#25831);
#21485=LINE('',#166793,#25832);
#21486=LINE('',#166803,#25833);
#21487=LINE('',#166810,#25834);
#21488=LINE('',#166813,#25835);
#21489=LINE('',#166815,#25836);
#21490=LINE('',#166860,#25837);
#21491=LINE('',#166981,#25838);
#21492=LINE('',#167068,#25839);
#21493=LINE('',#167071,#25840);
#21494=LINE('',#167224,#25841);
#21495=LINE('',#167345,#25842);
#21496=LINE('',#167471,#25843);
#21497=LINE('',#167472,#25844);
#21498=LINE('',#167474,#25845);
#21499=LINE('',#167477,#25846);
#21500=LINE('',#167479,#25847);
#21501=LINE('',#167485,#25848);
#21502=LINE('',#167488,#25849);
#21503=LINE('',#167532,#25850);
#21504=LINE('',#167533,#25851);
#21505=LINE('',#167536,#25852);
#21506=LINE('',#167544,#25853);
#21507=LINE('',#167621,#25854);
#21508=LINE('',#167668,#25855);
#21509=LINE('',#167675,#25856);
#21510=LINE('',#167799,#25857);
#21511=LINE('',#167999,#25858);
#21512=LINE('',#168006,#25859);
#21513=LINE('',#168010,#25860);
#21514=LINE('',#168012,#25861);
#21515=LINE('',#168056,#25862);
#21516=LINE('',#168059,#25863);
#21517=LINE('',#168064,#25864);
#21518=LINE('',#168065,#25865);
#21519=LINE('',#168251,#25866);
#21520=LINE('',#168254,#25867);
#21521=LINE('',#168266,#25868);
#21522=LINE('',#168269,#25869);
#21523=LINE('',#168278,#25870);
#21524=LINE('',#168374,#25871);
#21525=LINE('',#168397,#25872);
#21526=LINE('',#168483,#25873);
#21527=LINE('',#168486,#25874);
#21528=LINE('',#168498,#25875);
#21529=LINE('',#168500,#25876);
#21530=LINE('',#168512,#25877);
#21531=LINE('',#168515,#25878);
#21532=LINE('',#168693,#25879);
#21533=LINE('',#168694,#25880);
#21534=LINE('',#168699,#25881);
#21535=LINE('',#168700,#25882);
#21536=LINE('',#168711,#25883);
#21537=LINE('',#168885,#25884);
#21538=LINE('',#168985,#25885);
#21539=LINE('',#169029,#25886);
#21540=LINE('',#169030,#25887);
#21541=LINE('',#169032,#25888);
#21542=LINE('',#169041,#25889);
#21543=LINE('',#169051,#25890);
#21544=LINE('',#169058,#25891);
#21545=LINE('',#169061,#25892);
#21546=LINE('',#169063,#25893);
#21547=LINE('',#169108,#25894);
#21548=LINE('',#169229,#25895);
#21549=LINE('',#169307,#25896);
#21550=LINE('',#169310,#25897);
#21551=LINE('',#169451,#25898);
#21552=LINE('',#169515,#25899);
#21553=LINE('',#169695,#25900);
#21554=LINE('',#169698,#25901);
#21555=LINE('',#169742,#25902);
#21556=LINE('',#169743,#25903);
#21557=LINE('',#169746,#25904);
#21558=LINE('',#169755,#25905);
#21559=LINE('',#169847,#25906);
#21560=LINE('',#169849,#25907);
#21561=LINE('',#169850,#25908);
#21562=LINE('',#169855,#25909);
#21563=LINE('',#169856,#25910);
#21564=LINE('',#169865,#25911);
#21565=LINE('',#169872,#25912);
#21566=LINE('',#169986,#25913);
#21567=LINE('',#170112,#25914);
#21568=LINE('',#170119,#25915);
#21569=LINE('',#170123,#25916);
#21570=LINE('',#170125,#25917);
#21571=LINE('',#170173,#25918);
#21572=LINE('',#170176,#25919);
#21573=LINE('',#170179,#25920);
#21574=LINE('',#170182,#25921);
#21575=LINE('',#170276,#25922);
#21576=LINE('',#170363,#25923);
#21577=LINE('',#170370,#25924);
#21578=LINE('',#170374,#25925);
#21579=LINE('',#170375,#25926);
#21580=LINE('',#170583,#25927);
#21581=LINE('',#170663,#25928);
#21582=LINE('',#170664,#25929);
#21583=LINE('',#170667,#25930);
#21584=LINE('',#170675,#25931);
#21585=LINE('',#170744,#25932);
#21586=LINE('',#170754,#25933);
#21587=LINE('',#170760,#25934);
#21588=LINE('',#170762,#25935);
#21589=LINE('',#170843,#25936);
#21590=LINE('',#171193,#25937);
#21591=LINE('',#171261,#25938);
#21592=LINE('',#171262,#25939);
#21593=LINE('',#171386,#25940);
#21594=LINE('',#171387,#25941);
#21595=LINE('',#171394,#25942);
#21596=LINE('',#171399,#25943);
#21597=LINE('',#171482,#25944);
#21598=LINE('',#171484,#25945);
#21599=LINE('',#171553,#25946);
#21600=LINE('',#171774,#25947);
#21601=LINE('',#171824,#25948);
#21602=LINE('',#171825,#25949);
#21603=LINE('',#171916,#25950);
#21604=LINE('',#171917,#25951);
#21605=LINE('',#171921,#25952);
#21606=LINE('',#171926,#25953);
#21607=LINE('',#171985,#25954);
#21608=LINE('',#171987,#25955);
#21609=LINE('',#172038,#25956);
#21610=LINE('',#172247,#25957);
#21611=LINE('',#172315,#25958);
#21612=LINE('',#172316,#25959);
#21613=LINE('',#172431,#25960);
#21614=LINE('',#172434,#25961);
#21615=LINE('',#172441,#25962);
#21616=LINE('',#172446,#25963);
#21617=LINE('',#172529,#25964);
#21618=LINE('',#172531,#25965);
#21619=LINE('',#172600,#25966);
#21620=LINE('',#172905,#25967);
#21621=LINE('',#172982,#25968);
#21622=LINE('',#172983,#25969);
#21623=LINE('',#172990,#25970);
#21624=LINE('',#173071,#25971);
#21625=LINE('',#173081,#25972);
#21626=LINE('',#173088,#25973);
#21627=LINE('',#173091,#25974);
#21628=LINE('',#173093,#25975);
#21629=LINE('',#173166,#25976);
#21630=LINE('',#173510,#25977);
#21631=LINE('',#173629,#25978);
#21632=LINE('',#173716,#25979);
#21633=LINE('',#173717,#25980);
#21634=LINE('',#173719,#25981);
#21635=LINE('',#173728,#25982);
#21636=LINE('',#173742,#25983);
#21637=LINE('',#174056,#25984);
#21638=LINE('',#174059,#25985);
#21639=LINE('',#174071,#25986);
#21640=LINE('',#174073,#25987);
#21641=LINE('',#174085,#25988);
#21642=LINE('',#174088,#25989);
#21643=LINE('',#174293,#25990);
#21644=LINE('',#174386,#25991);
#21645=LINE('',#174587,#25992);
#21646=LINE('',#174630,#25993);
#21647=LINE('',#174748,#25994);
#21648=LINE('',#174758,#25995);
#21649=LINE('',#174842,#25996);
#21650=LINE('',#175171,#25997);
#21651=LINE('',#175279,#25998);
#21652=LINE('',#175282,#25999);
#21653=LINE('',#175290,#26000);
#21654=LINE('',#175299,#26001);
#21655=LINE('',#175371,#26002);
#21656=LINE('',#175607,#26003);
#21657=LINE('',#175687,#26004);
#21658=LINE('',#175690,#26005);
#21659=LINE('',#175746,#26006);
#21660=LINE('',#175805,#26007);
#21661=LINE('',#175806,#26008);
#21662=LINE('',#176249,#26009);
#21663=LINE('',#176267,#26010);
#21664=LINE('',#176271,#26011);
#21665=LINE('',#176290,#26012);
#21666=LINE('',#176329,#26013);
#21667=LINE('',#176403,#26014);
#21668=LINE('',#176406,#26015);
#21669=LINE('',#176648,#26016);
#21670=LINE('',#176650,#26017);
#21671=LINE('',#176651,#26018);
#21672=LINE('',#176655,#26019);
#21673=LINE('',#176659,#26020);
#21674=LINE('',#176663,#26021);
#21675=LINE('',#176666,#26022);
#21676=LINE('',#176667,#26023);
#21677=LINE('',#176670,#26024);
#21678=LINE('',#176674,#26025);
#21679=LINE('',#176679,#26026);
#21680=LINE('',#176682,#26027);
#21681=LINE('',#176683,#26028);
#21682=LINE('',#176687,#26029);
#21683=LINE('',#176691,#26030);
#21684=LINE('',#176695,#26031);
#21685=LINE('',#176699,#26032);
#21686=LINE('',#176701,#26033);
#21687=LINE('',#176716,#26034);
#21688=LINE('',#176717,#26035);
#21689=LINE('',#176849,#26036);
#21690=LINE('',#176895,#26037);
#21691=LINE('',#176978,#26038);
#21692=LINE('',#176981,#26039);
#21693=LINE('',#176983,#26040);
#21694=LINE('',#177000,#26041);
#21695=LINE('',#177017,#26042);
#21696=LINE('',#177020,#26043);
#21697=LINE('',#177023,#26044);
#21698=LINE('',#177024,#26045);
#21699=LINE('',#177028,#26046);
#21700=LINE('',#177044,#26047);
#21701=LINE('',#177061,#26048);
#21702=LINE('',#177064,#26049);
#21703=LINE('',#177067,#26050);
#21704=LINE('',#177068,#26051);
#21705=LINE('',#177072,#26052);
#21706=LINE('',#177090,#26053);
#21707=LINE('',#177367,#26054);
#21708=LINE('',#177371,#26055);
#21709=LINE('',#177375,#26056);
#21710=LINE('',#177377,#26057);
#21711=LINE('',#177383,#26058);
#21712=LINE('',#177589,#26059);
#21713=LINE('',#177593,#26060);
#21714=LINE('',#177597,#26061);
#21715=LINE('',#177599,#26062);
#21716=LINE('',#177608,#26063);
#21717=LINE('',#177729,#26064);
#21718=LINE('',#177730,#26065);
#21719=LINE('',#177838,#26066);
#21720=LINE('',#177839,#26067);
#21721=LINE('',#177843,#26068);
#21722=LINE('',#177851,#26069);
#21723=LINE('',#177854,#26070);
#21724=LINE('',#177857,#26071);
#21725=LINE('',#177862,#26072);
#21726=LINE('',#177871,#26073);
#21727=LINE('',#177876,#26074);
#21728=LINE('',#177877,#26075);
#21729=LINE('',#177882,#26076);
#21730=LINE('',#177885,#26077);
#21731=LINE('',#177915,#26078);
#21732=LINE('',#177916,#26079);
#21733=LINE('',#177920,#26080);
#21734=LINE('',#177928,#26081);
#21735=LINE('',#177931,#26082);
#21736=LINE('',#177934,#26083);
#21737=LINE('',#177937,#26084);
#21738=LINE('',#177952,#26085);
#21739=LINE('',#177953,#26086);
#21740=LINE('',#178118,#26087);
#21741=LINE('',#178121,#26088);
#21742=LINE('',#178122,#26089);
#21743=LINE('',#178171,#26090);
#21744=LINE('',#178174,#26091);
#21745=LINE('',#178291,#26092);
#21746=LINE('',#178410,#26093);
#21747=LINE('',#178411,#26094);
#21748=LINE('',#178469,#26095);
#21749=LINE('',#178472,#26096);
#21750=LINE('',#178473,#26097);
#21751=LINE('',#178522,#26098);
#21752=LINE('',#178525,#26099);
#21753=LINE('',#178640,#26100);
#21754=LINE('',#178642,#26101);
#21755=LINE('',#178833,#26102);
#21756=LINE('',#178834,#26103);
#21757=LINE('',#178886,#26104);
#21758=LINE('',#178889,#26105);
#21759=LINE('',#178890,#26106);
#21760=LINE('',#178945,#26107);
#21761=LINE('',#178948,#26108);
#21762=LINE('',#179070,#26109);
#21763=LINE('',#179172,#26110);
#21764=LINE('',#179173,#26111);
#21765=LINE('',#179187,#26112);
#21766=LINE('',#179188,#26113);
#21767=LINE('',#179342,#26114);
#21768=LINE('',#179345,#26115);
#21769=LINE('',#179346,#26116);
#21770=LINE('',#179401,#26117);
#21771=LINE('',#179404,#26118);
#21772=LINE('',#179626,#26119);
#21773=LINE('',#179628,#26120);
#21774=LINE('',#179641,#26121);
#21775=LINE('',#179642,#26122);
#21776=LINE('',#179700,#26123);
#21777=LINE('',#179703,#26124);
#21778=LINE('',#179704,#26125);
#21779=LINE('',#179753,#26126);
#21780=LINE('',#179756,#26127);
#21781=LINE('',#180023,#26128);
#21782=LINE('',#180024,#26129);
#21783=LINE('',#180025,#26130);
#21784=LINE('',#180083,#26131);
#21785=LINE('',#180086,#26132);
#21786=LINE('',#180087,#26133);
#21787=LINE('',#180136,#26134);
#21788=LINE('',#180139,#26135);
#21789=LINE('',#180150,#26136);
#21790=LINE('',#180359,#26137);
#21791=LINE('',#180373,#26138);
#21792=LINE('',#180374,#26139);
#21793=LINE('',#180426,#26140);
#21794=LINE('',#180429,#26141);
#21795=LINE('',#180430,#26142);
#21796=LINE('',#180485,#26143);
#21797=LINE('',#180488,#26144);
#21798=LINE('',#180610,#26145);
#21799=LINE('',#180667,#26146);
#21800=LINE('',#180668,#26147);
#21801=LINE('',#180820,#26148);
#21802=LINE('',#180821,#26149);
#21803=LINE('',#180873,#26150);
#21804=LINE('',#180876,#26151);
#21805=LINE('',#180877,#26152);
#21806=LINE('',#180932,#26153);
#21807=LINE('',#180935,#26154);
#21808=LINE('',#181157,#26155);
#21809=LINE('',#181160,#26156);
#21810=LINE('',#181162,#26157);
#21811=LINE('',#181185,#26158);
#21812=LINE('',#181186,#26159);
#21813=LINE('',#181222,#26160);
#21814=LINE('',#181226,#26161);
#21815=LINE('',#181281,#26162);
#21816=LINE('',#181284,#26163);
#21817=LINE('',#181307,#26164);
#21818=LINE('',#181731,#26165);
#21819=LINE('',#181754,#26166);
#21820=LINE('',#182148,#26167);
#21821=LINE('',#182171,#26168);
#21822=LINE('',#182580,#26169);
#21823=LINE('',#182603,#26170);
#21824=LINE('',#182604,#26171);
#21825=LINE('',#182671,#26172);
#21826=LINE('',#182675,#26173);
#21827=LINE('',#182754,#26174);
#21828=LINE('',#182757,#26175);
#21829=LINE('',#182807,#26176);
#21830=LINE('',#182808,#26177);
#21831=LINE('',#182859,#26178);
#21832=LINE('',#182863,#26179);
#21833=LINE('',#182918,#26180);
#21834=LINE('',#182922,#26181);
#21835=LINE('',#182983,#26182);
#21836=LINE('',#183013,#26183);
#21837=LINE('',#183459,#26184);
#21838=LINE('',#183461,#26185);
#21839=LINE('',#183484,#26186);
#21840=LINE('',#183546,#26187);
#21841=LINE('',#184038,#26188);
#21842=LINE('',#184040,#26189);
#21843=LINE('',#184077,#26190);
#21844=LINE('',#184078,#26191);
#21845=LINE('',#184079,#26192);
#21846=LINE('',#184164,#26193);
#21847=LINE('',#184168,#26194);
#21848=LINE('',#184187,#26195);
#21849=LINE('',#184190,#26196);
#21850=LINE('',#184192,#26197);
#21851=LINE('',#184294,#26198);
#21852=LINE('',#184366,#26199);
#21853=LINE('',#184369,#26200);
#21854=LINE('',#184371,#26201);
#21855=LINE('',#184390,#26202);
#21856=LINE('',#184394,#26203);
#21857=LINE('',#184395,#26204);
#21858=LINE('',#184431,#26205);
#21859=LINE('',#184435,#26206);
#21860=LINE('',#184490,#26207);
#21861=LINE('',#184493,#26208);
#21862=LINE('',#184495,#26209);
#21863=LINE('',#184516,#26210);
#21864=LINE('',#184520,#26211);
#21865=LINE('',#185013,#26212);
#21866=LINE('',#185015,#26213);
#21867=LINE('',#185066,#26214);
#21868=LINE('',#185070,#26215);
#21869=LINE('',#185109,#26216);
#21870=LINE('',#185274,#26217);
#21871=LINE('',#185470,#26218);
#21872=LINE('',#185525,#26219);
#21873=LINE('',#185531,#26220);
#21874=LINE('',#185683,#26221);
#21875=LINE('',#185689,#26222);
#21876=LINE('',#185815,#26223);
#21877=LINE('',#185821,#26224);
#21878=LINE('',#185897,#26225);
#21879=LINE('',#185901,#26226);
#21880=LINE('',#185911,#26227);
#21881=LINE('',#185927,#26228);
#21882=LINE('',#185943,#26229);
#21883=LINE('',#185959,#26230);
#21884=LINE('',#185969,#26231);
#21885=LINE('',#185974,#26232);
#21886=LINE('',#185981,#26233);
#21887=LINE('',#185983,#26234);
#21888=LINE('',#185987,#26235);
#21889=LINE('',#185988,#26236);
#21890=LINE('',#185992,#26237);
#21891=LINE('',#185994,#26238);
#21892=LINE('',#185998,#26239);
#21893=LINE('',#186006,#26240);
#21894=LINE('',#186012,#26241);
#21895=LINE('',#186014,#26242);
#21896=LINE('',#186018,#26243);
#21897=LINE('',#186026,#26244);
#21898=LINE('',#186032,#26245);
#21899=LINE('',#186035,#26246);
#21900=LINE('',#186068,#26247);
#21901=LINE('',#186076,#26248);
#21902=LINE('',#186082,#26249);
#21903=LINE('',#186088,#26250);
#21904=LINE('',#186096,#26251);
#21905=LINE('',#186104,#26252);
#21906=LINE('',#186108,#26253);
#21907=LINE('',#186112,#26254);
#21908=LINE('',#186326,#26255);
#21909=LINE('',#186333,#26256);
#21910=LINE('',#186335,#26257);
#21911=LINE('',#186339,#26258);
#21912=LINE('',#186343,#26259);
#21913=LINE('',#186345,#26260);
#21914=LINE('',#186349,#26261);
#21915=LINE('',#186353,#26262);
#21916=LINE('',#186359,#26263);
#21917=LINE('',#186391,#26264);
#21918=LINE('',#186420,#26265);
#21919=LINE('',#186422,#26266);
#21920=LINE('',#186426,#26267);
#21921=LINE('',#186457,#26268);
#21922=LINE('',#186486,#26269);
#21923=LINE('',#186489,#26270);
#21924=LINE('',#186509,#26271);
#21925=LINE('',#186549,#26272);
#21926=LINE('',#186581,#26273);
#21927=LINE('',#186610,#26274);
#21928=LINE('',#186613,#26275);
#21929=LINE('',#186655,#26276);
#21930=LINE('',#186673,#26277);
#21931=LINE('',#186677,#26278);
#21932=LINE('',#186708,#26279);
#21933=LINE('',#186738,#26280);
#21934=LINE('',#186740,#26281);
#21935=LINE('',#186746,#26282);
#21936=LINE('',#186750,#26283);
#21937=LINE('',#186781,#26284);
#21938=LINE('',#186810,#26285);
#21939=LINE('',#186813,#26286);
#21940=LINE('',#186854,#26287);
#21941=LINE('',#186884,#26288);
#21942=LINE('',#186914,#26289);
#21943=LINE('',#186916,#26290);
#21944=LINE('',#187000,#26291);
#21945=LINE('',#187003,#26292);
#21946=LINE('',#187035,#26293);
#21947=LINE('',#187064,#26294);
#21948=LINE('',#187067,#26295);
#21949=LINE('',#187108,#26296);
#21950=LINE('',#187169,#26297);
#21951=LINE('',#187174,#26298);
#21952=LINE('',#187205,#26299);
#21953=LINE('',#187234,#26300);
#21954=LINE('',#187236,#26301);
#21955=LINE('',#187333,#26302);
#21956=LINE('',#187338,#26303);
#21957=LINE('',#187459,#26304);
#21958=LINE('',#187464,#26305);
#21959=LINE('',#187620,#26306);
#21960=LINE('',#187625,#26307);
#21961=LINE('',#187746,#26308);
#21962=LINE('',#187751,#26309);
#21963=LINE('',#187928,#26310);
#21964=LINE('',#187933,#26311);
#21965=LINE('',#188102,#26312);
#21966=LINE('',#188108,#26313);
#21967=LINE('',#188183,#26314);
#21968=LINE('',#188185,#26315);
#21969=LINE('',#188186,#26316);
#21970=LINE('',#188191,#26317);
#21971=LINE('',#188193,#26318);
#21972=LINE('',#188194,#26319);
#21973=LINE('',#188201,#26320);
#21974=LINE('',#188203,#26321);
#21975=LINE('',#188204,#26322);
#21976=LINE('',#188259,#26323);
#21977=LINE('',#188260,#26324);
#21978=LINE('',#188333,#26325);
#21979=LINE('',#188476,#26326);
#21980=LINE('',#188481,#26327);
#21981=LINE('',#188606,#26328);
#21982=LINE('',#188612,#26329);
#21983=LINE('',#188730,#26330);
#21984=LINE('',#188735,#26331);
#21985=LINE('',#188819,#26332);
#21986=LINE('',#188824,#26333);
#21987=LINE('',#188945,#26334);
#21988=LINE('',#188950,#26335);
#21989=LINE('',#189117,#26336);
#21990=LINE('',#189122,#26337);
#21991=LINE('',#189169,#26338);
#21992=LINE('',#189172,#26339);
#21993=LINE('',#189174,#26340);
#21994=LINE('',#189175,#26341);
#21995=LINE('',#189180,#26342);
#21996=LINE('',#189182,#26343);
#21997=LINE('',#189183,#26344);
#21998=LINE('',#189190,#26345);
#21999=LINE('',#189192,#26346);
#22000=LINE('',#189193,#26347);
#22001=LINE('',#189294,#26348);
#22002=LINE('',#189296,#26349);
#22003=LINE('',#189313,#26350);
#22004=LINE('',#189319,#26351);
#22005=LINE('',#189326,#26352);
#22006=LINE('',#189336,#26353);
#22007=LINE('',#189346,#26354);
#22008=LINE('',#189356,#26355);
#22009=LINE('',#189372,#26356);
#22010=LINE('',#189398,#26357);
#22011=LINE('',#189403,#26358);
#22012=LINE('',#189409,#26359);
#22013=LINE('',#189416,#26360);
#22014=LINE('',#191638,#26361);
#22015=LINE('',#191641,#26362);
#22016=LINE('',#191678,#26363);
#22017=LINE('',#191679,#26364);
#22018=LINE('',#191682,#26365);
#22019=LINE('',#191685,#26366);
#22020=LINE('',#191721,#26367);
#22021=LINE('',#191722,#26368);
#22022=LINE('',#191725,#26369);
#22023=LINE('',#191728,#26370);
#22024=LINE('',#191764,#26371);
#22025=LINE('',#191765,#26372);
#22026=LINE('',#191768,#26373);
#22027=LINE('',#191771,#26374);
#22028=LINE('',#191807,#26375);
#22029=LINE('',#191808,#26376);
#22030=LINE('',#191810,#26377);
#22031=LINE('',#191811,#26378);
#22032=LINE('',#191813,#26379);
#22033=LINE('',#191814,#26380);
#22034=LINE('',#191816,#26381);
#22035=LINE('',#191817,#26382);
#22036=LINE('',#191819,#26383);
#22037=LINE('',#191820,#26384);
#22038=LINE('',#191822,#26385);
#22039=LINE('',#191823,#26386);
#22040=LINE('',#191825,#26387);
#22041=LINE('',#191826,#26388);
#22042=LINE('',#191828,#26389);
#22043=LINE('',#191829,#26390);
#22044=LINE('',#191831,#26391);
#22045=LINE('',#191832,#26392);
#22046=LINE('',#191846,#26393);
#22047=LINE('',#191847,#26394);
#22048=LINE('',#191870,#26395);
#22049=LINE('',#191871,#26396);
#22050=LINE('',#191891,#26397);
#22051=LINE('',#191892,#26398);
#22052=LINE('',#191906,#26399);
#22053=LINE('',#191907,#26400);
#22054=LINE('',#191930,#26401);
#22055=LINE('',#191931,#26402);
#22056=LINE('',#191936,#26403);
#22057=LINE('',#191937,#26404);
#22058=LINE('',#191954,#26405);
#22059=LINE('',#191955,#26406);
#22060=LINE('',#191978,#26407);
#22061=LINE('',#191979,#26408);
#22062=LINE('',#191984,#26409);
#22063=LINE('',#191985,#26410);
#22064=LINE('',#192002,#26411);
#22065=LINE('',#192003,#26412);
#22066=LINE('',#192008,#26413);
#22067=LINE('',#192009,#26414);
#22068=LINE('',#192026,#26415);
#22069=LINE('',#192027,#26416);
#22070=LINE('',#192032,#26417);
#22071=LINE('',#192033,#26418);
#22072=LINE('',#192050,#26419);
#22073=LINE('',#192051,#26420);
#22074=LINE('',#192056,#26421);
#22075=LINE('',#192057,#26422);
#22076=LINE('',#192080,#26423);
#22077=LINE('',#192081,#26424);
#22078=LINE('',#192104,#26425);
#22079=LINE('',#192105,#26426);
#22080=LINE('',#192110,#26427);
#22081=LINE('',#192111,#26428);
#22082=LINE('',#192128,#26429);
#22083=LINE('',#192129,#26430);
#22084=LINE('',#192134,#26431);
#22085=LINE('',#192135,#26432);
#22086=LINE('',#192152,#26433);
#22087=LINE('',#192153,#26434);
#22088=LINE('',#192158,#26435);
#22089=LINE('',#192159,#26436);
#22090=LINE('',#192176,#26437);
#22091=LINE('',#192177,#26438);
#22092=LINE('',#192182,#26439);
#22093=LINE('',#192183,#26440);
#22094=LINE('',#192200,#26441);
#22095=LINE('',#192201,#26442);
#22096=LINE('',#192206,#26443);
#22097=LINE('',#192207,#26444);
#22098=LINE('',#192224,#26445);
#22099=LINE('',#192225,#26446);
#22100=LINE('',#192230,#26447);
#22101=LINE('',#192231,#26448);
#22102=LINE('',#192248,#26449);
#22103=LINE('',#192249,#26450);
#22104=LINE('',#192254,#26451);
#22105=LINE('',#192255,#26452);
#22106=LINE('',#192272,#26453);
#22107=LINE('',#192273,#26454);
#22108=LINE('',#192278,#26455);
#22109=LINE('',#192279,#26456);
#22110=LINE('',#192296,#26457);
#22111=LINE('',#192297,#26458);
#22112=LINE('',#192302,#26459);
#22113=LINE('',#192303,#26460);
#22114=LINE('',#192320,#26461);
#22115=LINE('',#192321,#26462);
#22116=LINE('',#192344,#26463);
#22117=LINE('',#192345,#26464);
#22118=LINE('',#192350,#26465);
#22119=LINE('',#192351,#26466);
#22120=LINE('',#192368,#26467);
#22121=LINE('',#192369,#26468);
#22122=LINE('',#192404,#26469);
#22123=LINE('',#192405,#26470);
#22124=LINE('',#192410,#26471);
#22125=LINE('',#192411,#26472);
#22126=LINE('',#192428,#26473);
#22127=LINE('',#192429,#26474);
#22128=LINE('',#192452,#26475);
#22129=LINE('',#192453,#26476);
#22130=LINE('',#192458,#26477);
#22131=LINE('',#192459,#26478);
#22132=LINE('',#192476,#26479);
#22133=LINE('',#192477,#26480);
#22134=LINE('',#192482,#26481);
#22135=LINE('',#192483,#26482);
#22136=LINE('',#192500,#26483);
#22137=LINE('',#192501,#26484);
#22138=LINE('',#192524,#26485);
#22139=LINE('',#192525,#26486);
#22140=LINE('',#192530,#26487);
#22141=LINE('',#192531,#26488);
#22142=LINE('',#192545,#26489);
#22143=LINE('',#192546,#26490);
#22144=LINE('',#192560,#26491);
#22145=LINE('',#192561,#26492);
#22146=LINE('',#192566,#26493);
#22147=LINE('',#192567,#26494);
#22148=LINE('',#192584,#26495);
#22149=LINE('',#192585,#26496);
#22150=LINE('',#192605,#26497);
#22151=LINE('',#192606,#26498);
#22152=LINE('',#192620,#26499);
#22153=LINE('',#192621,#26500);
#22154=LINE('',#192626,#26501);
#22155=LINE('',#192627,#26502);
#22156=LINE('',#192644,#26503);
#22157=LINE('',#192645,#26504);
#22158=LINE('',#192650,#26505);
#22159=LINE('',#192651,#26506);
#22160=LINE('',#192668,#26507);
#22161=LINE('',#192669,#26508);
#22162=LINE('',#192674,#26509);
#22163=LINE('',#192675,#26510);
#22164=LINE('',#192698,#26511);
#22165=LINE('',#192699,#26512);
#22166=LINE('',#192716,#26513);
#22167=LINE('',#192717,#26514);
#22168=LINE('',#192722,#26515);
#22169=LINE('',#192723,#26516);
#22170=LINE('',#192740,#26517);
#22171=LINE('',#192741,#26518);
#22172=LINE('',#192746,#26519);
#22173=LINE('',#192747,#26520);
#22174=LINE('',#192764,#26521);
#22175=LINE('',#192765,#26522);
#22176=LINE('',#192770,#26523);
#22177=LINE('',#192771,#26524);
#22178=LINE('',#192788,#26525);
#22179=LINE('',#192789,#26526);
#22180=LINE('',#192794,#26527);
#22181=LINE('',#192795,#26528);
#22182=LINE('',#192812,#26529);
#22183=LINE('',#192813,#26530);
#22184=LINE('',#192818,#26531);
#22185=LINE('',#192819,#26532);
#22186=LINE('',#192836,#26533);
#22187=LINE('',#192837,#26534);
#22188=LINE('',#192866,#26535);
#22189=LINE('',#192867,#26536);
#22190=LINE('',#192872,#26537);
#22191=LINE('',#192873,#26538);
#22192=LINE('',#192896,#26539);
#22193=LINE('',#192897,#26540);
#22194=LINE('',#192914,#26541);
#22195=LINE('',#192915,#26542);
#22196=LINE('',#192920,#26543);
#22197=LINE('',#192921,#26544);
#22198=LINE('',#192944,#26545);
#22199=LINE('',#192945,#26546);
#22200=LINE('',#192974,#26547);
#22201=LINE('',#192975,#26548);
#22202=LINE('',#192980,#26549);
#22203=LINE('',#192981,#26550);
#22204=LINE('',#192998,#26551);
#22205=LINE('',#192999,#26552);
#22206=LINE('',#193004,#26553);
#22207=LINE('',#193005,#26554);
#22208=LINE('',#193022,#26555);
#22209=LINE('',#193023,#26556);
#22210=LINE('',#193028,#26557);
#22211=LINE('',#193029,#26558);
#22212=LINE('',#193046,#26559);
#22213=LINE('',#193047,#26560);
#22214=LINE('',#193082,#26561);
#22215=LINE('',#193083,#26562);
#22216=LINE('',#193088,#26563);
#22217=LINE('',#193089,#26564);
#22218=LINE('',#193106,#26565);
#22219=LINE('',#193107,#26566);
#22220=LINE('',#193130,#26567);
#22221=LINE('',#193131,#26568);
#22222=LINE('',#193136,#26569);
#22223=LINE('',#193137,#26570);
#22224=LINE('',#193154,#26571);
#22225=LINE('',#193155,#26572);
#22226=LINE('',#193160,#26573);
#22227=LINE('',#193161,#26574);
#22228=LINE('',#193178,#26575);
#22229=LINE('',#193179,#26576);
#22230=LINE('',#193184,#26577);
#22231=LINE('',#193185,#26578);
#22232=LINE('',#193202,#26579);
#22233=LINE('',#193203,#26580);
#22234=LINE('',#193226,#26581);
#22235=LINE('',#193227,#26582);
#22236=LINE('',#193232,#26583);
#22237=LINE('',#193233,#26584);
#22238=LINE('',#193250,#26585);
#22239=LINE('',#193251,#26586);
#22240=LINE('',#193256,#26587);
#22241=LINE('',#193257,#26588);
#22242=LINE('',#193274,#26589);
#22243=LINE('',#193275,#26590);
#22244=LINE('',#193295,#26591);
#22245=LINE('',#193296,#26592);
#22246=LINE('',#193310,#26593);
#22247=LINE('',#193311,#26594);
#22248=LINE('',#193331,#26595);
#22249=LINE('',#193332,#26596);
#22250=LINE('',#193445,#26597);
#22251=LINE('',#193446,#26598);
#22252=LINE('',#193469,#26599);
#22253=LINE('',#193470,#26600);
#22254=LINE('',#193508,#26601);
#22255=LINE('',#193509,#26602);
#22256=LINE('',#193532,#26603);
#22257=LINE('',#193533,#26604);
#22258=LINE('',#193571,#26605);
#22259=LINE('',#193572,#26606);
#22260=LINE('',#193595,#26607);
#22261=LINE('',#193596,#26608);
#22262=LINE('',#193634,#26609);
#22263=LINE('',#193635,#26610);
#22264=LINE('',#193658,#26611);
#22265=LINE('',#193659,#26612);
#22266=LINE('',#199112,#26613);
#22267=LINE('',#199113,#26614);
#22268=LINE('',#199116,#26615);
#22269=LINE('',#199119,#26616);
#22270=LINE('',#199122,#26617);
#22271=LINE('',#199125,#26618);
#22272=LINE('',#199128,#26619);
#22273=LINE('',#199131,#26620);
#22274=LINE('',#199134,#26621);
#22275=LINE('',#199137,#26622);
#22276=LINE('',#199140,#26623);
#22277=LINE('',#199143,#26624);
#22278=LINE('',#199146,#26625);
#22279=LINE('',#199149,#26626);
#22280=LINE('',#199152,#26627);
#22281=LINE('',#199155,#26628);
#22282=LINE('',#199158,#26629);
#22283=LINE('',#199161,#26630);
#22284=LINE('',#199166,#26631);
#22285=LINE('',#199167,#26632);
#22286=LINE('',#199170,#26633);
#22287=LINE('',#199173,#26634);
#22288=LINE('',#199176,#26635);
#22289=LINE('',#199179,#26636);
#22290=LINE('',#199182,#26637);
#22291=LINE('',#199185,#26638);
#22292=LINE('',#199188,#26639);
#22293=LINE('',#199191,#26640);
#22294=LINE('',#199194,#26641);
#22295=LINE('',#199197,#26642);
#22296=LINE('',#199200,#26643);
#22297=LINE('',#199203,#26644);
#22298=LINE('',#199206,#26645);
#22299=LINE('',#199209,#26646);
#22300=LINE('',#199212,#26647);
#22301=LINE('',#199215,#26648);
#22302=LINE('',#199218,#26649);
#22303=LINE('',#199221,#26650);
#22304=LINE('',#199224,#26651);
#22305=LINE('',#199227,#26652);
#22306=LINE('',#199230,#26653);
#22307=LINE('',#199233,#26654);
#22308=LINE('',#199236,#26655);
#22309=LINE('',#199239,#26656);
#22310=LINE('',#199242,#26657);
#22311=LINE('',#199245,#26658);
#22312=LINE('',#199248,#26659);
#22313=LINE('',#199251,#26660);
#22314=LINE('',#199254,#26661);
#22315=LINE('',#199257,#26662);
#22316=LINE('',#199260,#26663);
#22317=LINE('',#199263,#26664);
#22318=LINE('',#199266,#26665);
#22319=LINE('',#199269,#26666);
#22320=LINE('',#199274,#26667);
#22321=LINE('',#199275,#26668);
#22322=LINE('',#199278,#26669);
#22323=LINE('',#199281,#26670);
#22324=LINE('',#199284,#26671);
#22325=LINE('',#199287,#26672);
#22326=LINE('',#199290,#26673);
#22327=LINE('',#199293,#26674);
#22328=LINE('',#199296,#26675);
#22329=LINE('',#199299,#26676);
#22330=LINE('',#199302,#26677);
#22331=LINE('',#199305,#26678);
#22332=LINE('',#199308,#26679);
#22333=LINE('',#199311,#26680);
#22334=LINE('',#199314,#26681);
#22335=LINE('',#199317,#26682);
#22336=LINE('',#199320,#26683);
#22337=LINE('',#199323,#26684);
#22338=LINE('',#199326,#26685);
#22339=LINE('',#199329,#26686);
#22340=LINE('',#199332,#26687);
#22341=LINE('',#199335,#26688);
#22342=LINE('',#199338,#26689);
#22343=LINE('',#199341,#26690);
#22344=LINE('',#199344,#26691);
#22345=LINE('',#199347,#26692);
#22346=LINE('',#199350,#26693);
#22347=LINE('',#199353,#26694);
#22348=LINE('',#199356,#26695);
#22349=LINE('',#199359,#26696);
#22350=LINE('',#199362,#26697);
#22351=LINE('',#199365,#26698);
#22352=LINE('',#199368,#26699);
#22353=LINE('',#199371,#26700);
#22354=LINE('',#199374,#26701);
#22355=LINE('',#199377,#26702);
#22356=LINE('',#199380,#26703);
#22357=LINE('',#199383,#26704);
#22358=LINE('',#199386,#26705);
#22359=LINE('',#199389,#26706);
#22360=LINE('',#199392,#26707);
#22361=LINE('',#199395,#26708);
#22362=LINE('',#199398,#26709);
#22363=LINE('',#199401,#26710);
#22364=LINE('',#199404,#26711);
#22365=LINE('',#199407,#26712);
#22366=LINE('',#199410,#26713);
#22367=LINE('',#199413,#26714);
#22368=LINE('',#199416,#26715);
#22369=LINE('',#199419,#26716);
#22370=LINE('',#199422,#26717);
#22371=LINE('',#199425,#26718);
#22372=LINE('',#199428,#26719);
#22373=LINE('',#199431,#26720);
#22374=LINE('',#199434,#26721);
#22375=LINE('',#199437,#26722);
#22376=LINE('',#199440,#26723);
#22377=LINE('',#199443,#26724);
#22378=LINE('',#199446,#26725);
#22379=LINE('',#199449,#26726);
#22380=LINE('',#199452,#26727);
#22381=LINE('',#199455,#26728);
#22382=LINE('',#199458,#26729);
#22383=LINE('',#199461,#26730);
#22384=LINE('',#199464,#26731);
#22385=LINE('',#199467,#26732);
#22386=LINE('',#199470,#26733);
#22387=LINE('',#199473,#26734);
#22388=LINE('',#199476,#26735);
#22389=LINE('',#199479,#26736);
#22390=LINE('',#199482,#26737);
#22391=LINE('',#199485,#26738);
#22392=LINE('',#199488,#26739);
#22393=LINE('',#199491,#26740);
#22394=LINE('',#199494,#26741);
#22395=LINE('',#199497,#26742);
#22396=LINE('',#199500,#26743);
#22397=LINE('',#199503,#26744);
#22398=LINE('',#199506,#26745);
#22399=LINE('',#199509,#26746);
#22400=LINE('',#199512,#26747);
#22401=LINE('',#199515,#26748);
#22402=LINE('',#199518,#26749);
#22403=LINE('',#199521,#26750);
#22404=LINE('',#199524,#26751);
#22405=LINE('',#199527,#26752);
#22406=LINE('',#199530,#26753);
#22407=LINE('',#199533,#26754);
#22408=LINE('',#199536,#26755);
#22409=LINE('',#199539,#26756);
#22410=LINE('',#199542,#26757);
#22411=LINE('',#199545,#26758);
#22412=LINE('',#199548,#26759);
#22413=LINE('',#199551,#26760);
#22414=LINE('',#199554,#26761);
#22415=LINE('',#199557,#26762);
#22416=LINE('',#199560,#26763);
#22417=LINE('',#199563,#26764);
#22418=LINE('',#199566,#26765);
#22419=LINE('',#199569,#26766);
#22420=LINE('',#199572,#26767);
#22421=LINE('',#199575,#26768);
#22422=LINE('',#199578,#26769);
#22423=LINE('',#199581,#26770);
#22424=LINE('',#199584,#26771);
#22425=LINE('',#199587,#26772);
#22426=LINE('',#199590,#26773);
#22427=LINE('',#199593,#26774);
#22428=LINE('',#199596,#26775);
#22429=LINE('',#199599,#26776);
#22430=LINE('',#199602,#26777);
#22431=LINE('',#199605,#26778);
#22432=LINE('',#199608,#26779);
#22433=LINE('',#199611,#26780);
#22434=LINE('',#199614,#26781);
#22435=LINE('',#199617,#26782);
#22436=LINE('',#199622,#26783);
#22437=LINE('',#199623,#26784);
#22438=LINE('',#199626,#26785);
#22439=LINE('',#199629,#26786);
#22440=LINE('',#199632,#26787);
#22441=LINE('',#199635,#26788);
#22442=LINE('',#199638,#26789);
#22443=LINE('',#199641,#26790);
#22444=LINE('',#199644,#26791);
#22445=LINE('',#199647,#26792);
#22446=LINE('',#199650,#26793);
#22447=LINE('',#199653,#26794);
#22448=LINE('',#199656,#26795);
#22449=LINE('',#199659,#26796);
#22450=LINE('',#199662,#26797);
#22451=LINE('',#199665,#26798);
#22452=LINE('',#199668,#26799);
#22453=LINE('',#199671,#26800);
#22454=LINE('',#199674,#26801);
#22455=LINE('',#199677,#26802);
#22456=LINE('',#199680,#26803);
#22457=LINE('',#199683,#26804);
#22458=LINE('',#199686,#26805);
#22459=LINE('',#199689,#26806);
#22460=LINE('',#199692,#26807);
#22461=LINE('',#199695,#26808);
#22462=LINE('',#199698,#26809);
#22463=LINE('',#199701,#26810);
#22464=LINE('',#199704,#26811);
#22465=LINE('',#199707,#26812);
#22466=LINE('',#199710,#26813);
#22467=LINE('',#199713,#26814);
#22468=LINE('',#199716,#26815);
#22469=LINE('',#199719,#26816);
#22470=LINE('',#199722,#26817);
#22471=LINE('',#199725,#26818);
#22472=LINE('',#199728,#26819);
#22473=LINE('',#199731,#26820);
#22474=LINE('',#199734,#26821);
#22475=LINE('',#199737,#26822);
#22476=LINE('',#199740,#26823);
#22477=LINE('',#199743,#26824);
#22478=LINE('',#199746,#26825);
#22479=LINE('',#199749,#26826);
#22480=LINE('',#199752,#26827);
#22481=LINE('',#199755,#26828);
#22482=LINE('',#199758,#26829);
#22483=LINE('',#199761,#26830);
#22484=LINE('',#199766,#26831);
#22485=LINE('',#199767,#26832);
#22486=LINE('',#199770,#26833);
#22487=LINE('',#199773,#26834);
#22488=LINE('',#199776,#26835);
#22489=LINE('',#199779,#26836);
#22490=LINE('',#199782,#26837);
#22491=LINE('',#199785,#26838);
#22492=LINE('',#199788,#26839);
#22493=LINE('',#199791,#26840);
#22494=LINE('',#199794,#26841);
#22495=LINE('',#199797,#26842);
#22496=LINE('',#199800,#26843);
#22497=LINE('',#199803,#26844);
#22498=LINE('',#199806,#26845);
#22499=LINE('',#199809,#26846);
#22500=LINE('',#199812,#26847);
#22501=LINE('',#199815,#26848);
#22502=LINE('',#199818,#26849);
#22503=LINE('',#199821,#26850);
#22504=LINE('',#199824,#26851);
#22505=LINE('',#199827,#26852);
#22506=LINE('',#199830,#26853);
#22507=LINE('',#199833,#26854);
#22508=LINE('',#199836,#26855);
#22509=LINE('',#199839,#26856);
#22510=LINE('',#199842,#26857);
#22511=LINE('',#199845,#26858);
#22512=LINE('',#199848,#26859);
#22513=LINE('',#199851,#26860);
#22514=LINE('',#199854,#26861);
#22515=LINE('',#199857,#26862);
#22516=LINE('',#199862,#26863);
#22517=LINE('',#199863,#26864);
#22518=LINE('',#199866,#26865);
#22519=LINE('',#199869,#26866);
#22520=LINE('',#199872,#26867);
#22521=LINE('',#199875,#26868);
#22522=LINE('',#199878,#26869);
#22523=LINE('',#199881,#26870);
#22524=LINE('',#199884,#26871);
#22525=LINE('',#199887,#26872);
#22526=LINE('',#199892,#26873);
#22527=LINE('',#199893,#26874);
#22528=LINE('',#199896,#26875);
#22529=LINE('',#199899,#26876);
#22530=LINE('',#199904,#26877);
#22531=LINE('',#199905,#26878);
#22532=LINE('',#199908,#26879);
#22533=LINE('',#199911,#26880);
#22534=LINE('',#199914,#26881);
#22535=LINE('',#199917,#26882);
#22536=LINE('',#199920,#26883);
#22537=LINE('',#199923,#26884);
#22538=LINE('',#199926,#26885);
#22539=LINE('',#199931,#26886);
#22540=LINE('',#199939,#26887);
#22541=LINE('',#199941,#26888);
#22542=LINE('',#199949,#26889);
#22543=LINE('',#199951,#26890);
#22544=LINE('',#199957,#26891);
#22545=LINE('',#199959,#26892);
#22546=LINE('',#199961,#26893);
#22547=LINE('',#199963,#26894);
#22548=LINE('',#199965,#26895);
#22549=LINE('',#199967,#26896);
#22550=LINE('',#199969,#26897);
#22551=LINE('',#199971,#26898);
#22552=LINE('',#199973,#26899);
#22553=LINE('',#199975,#26900);
#22554=LINE('',#199977,#26901);
#22555=LINE('',#199979,#26902);
#22556=LINE('',#199981,#26903);
#22557=LINE('',#199983,#26904);
#22558=LINE('',#199985,#26905);
#22559=LINE('',#199987,#26906);
#22560=LINE('',#199989,#26907);
#22561=LINE('',#199991,#26908);
#22562=LINE('',#199993,#26909);
#22563=LINE('',#199995,#26910);
#22564=LINE('',#199997,#26911);
#22565=LINE('',#199999,#26912);
#22566=LINE('',#200001,#26913);
#22567=LINE('',#200003,#26914);
#22568=LINE('',#200005,#26915);
#22569=LINE('',#200007,#26916);
#22570=LINE('',#200009,#26917);
#22571=LINE('',#200011,#26918);
#22572=LINE('',#200013,#26919);
#22573=LINE('',#200015,#26920);
#22574=LINE('',#200017,#26921);
#22575=LINE('',#200019,#26922);
#22576=LINE('',#200023,#26923);
#22577=LINE('',#200025,#26924);
#22578=LINE('',#200027,#26925);
#22579=LINE('',#200028,#26926);
#22580=LINE('',#200032,#26927);
#22581=LINE('',#200033,#26928);
#22582=LINE('',#200034,#26929);
#22583=LINE('',#200037,#26930);
#22584=LINE('',#200039,#26931);
#22585=LINE('',#200040,#26932);
#22586=LINE('',#200042,#26933);
#22587=LINE('',#200044,#26934);
#22588=LINE('',#200046,#26935);
#22589=LINE('',#200048,#26936);
#22590=LINE('',#200050,#26937);
#22591=LINE('',#200052,#26938);
#22592=LINE('',#200054,#26939);
#22593=LINE('',#200056,#26940);
#22594=LINE('',#200058,#26941);
#22595=LINE('',#200060,#26942);
#22596=LINE('',#200062,#26943);
#22597=LINE('',#200064,#26944);
#22598=LINE('',#200066,#26945);
#22599=LINE('',#200068,#26946);
#22600=LINE('',#200070,#26947);
#22601=LINE('',#200072,#26948);
#22602=LINE('',#200074,#26949);
#22603=LINE('',#200076,#26950);
#22604=LINE('',#200078,#26951);
#22605=LINE('',#200080,#26952);
#22606=LINE('',#200082,#26953);
#22607=LINE('',#200084,#26954);
#22608=LINE('',#200088,#26955);
#22609=LINE('',#200092,#26956);
#22610=LINE('',#200098,#26957);
#22611=LINE('',#200104,#26958);
#22612=LINE('',#200110,#26959);
#22613=LINE('',#200116,#26960);
#22614=LINE('',#200122,#26961);
#22615=LINE('',#200128,#26962);
#22616=LINE('',#200133,#26963);
#22617=LINE('',#200137,#26964);
#22618=LINE('',#200152,#26965);
#22619=LINE('',#200164,#26966);
#22620=LINE('',#200173,#26967);
#22621=LINE('',#200181,#26968);
#22622=LINE('',#200183,#26969);
#22623=LINE('',#200204,#26970);
#22624=LINE('',#200205,#26971);
#22625=LINE('',#200223,#26972);
#22626=LINE('',#200224,#26973);
#22627=LINE('',#200232,#26974);
#22628=LINE('',#200234,#26975);
#22629=LINE('',#200249,#26976);
#22630=LINE('',#200252,#26977);
#22631=LINE('',#200258,#26978);
#22632=LINE('',#200261,#26979);
#22633=LINE('',#200266,#26980);
#22634=LINE('',#200272,#26981);
#22635=LINE('',#200290,#26982);
#22636=LINE('',#200293,#26983);
#22637=LINE('',#202386,#26984);
#22638=LINE('',#202394,#26985);
#22639=LINE('',#202412,#26986);
#22640=LINE('',#202418,#26987);
#22641=LINE('',#202423,#26988);
#22642=LINE('',#202426,#26989);
#22643=LINE('',#202438,#26990);
#22644=LINE('',#202452,#26991);
#22645=LINE('',#202458,#26992);
#22646=LINE('',#202461,#26993);
#22647=LINE('',#202467,#26994);
#22648=LINE('',#202473,#26995);
#22649=LINE('',#202479,#26996);
#22650=LINE('',#202485,#26997);
#22651=LINE('',#202488,#26998);
#22652=LINE('',#202494,#26999);
#22653=LINE('',#203630,#27000);
#22654=LINE('',#203728,#27001);
#22655=LINE('',#203730,#27002);
#22656=LINE('',#204868,#27003);
#22657=LINE('',#204871,#27004);
#22658=LINE('',#204875,#27005);
#22659=LINE('',#204879,#27006);
#22660=LINE('',#204884,#27007);
#22661=LINE('',#204887,#27008);
#22662=LINE('',#204892,#27009);
#22663=LINE('',#204895,#27010);
#22664=LINE('',#204901,#27011);
#22665=LINE('',#204908,#27012);
#22666=LINE('',#205010,#27013);
#22667=LINE('',#205013,#27014);
#22668=LINE('',#205016,#27015);
#22669=LINE('',#205020,#27016);
#22670=LINE('',#205024,#27017);
#22671=LINE('',#205028,#27018);
#22672=LINE('',#205032,#27019);
#22673=LINE('',#205037,#27020);
#22674=LINE('',#205040,#27021);
#22675=LINE('',#205043,#27022);
#22676=LINE('',#205046,#27023);
#22677=LINE('',#205049,#27024);
#22678=LINE('',#205053,#27025);
#22679=LINE('',#205057,#27026);
#22680=LINE('',#205061,#27027);
#22681=LINE('',#205065,#27028);
#22682=LINE('',#205149,#27029);
#22683=LINE('',#205248,#27030);
#22684=LINE('',#205334,#27031);
#22685=LINE('',#205454,#27032);
#22686=LINE('',#205460,#27033);
#22687=LINE('',#205461,#27034);
#22688=LINE('',#205463,#27035);
#22689=LINE('',#205465,#27036);
#22690=LINE('',#205467,#27037);
#22691=LINE('',#205468,#27038);
#22692=LINE('',#205470,#27039);
#22693=LINE('',#205472,#27040);
#22694=LINE('',#205475,#27041);
#22695=LINE('',#205478,#27042);
#22696=LINE('',#205482,#27043);
#22697=LINE('',#205486,#27044);
#22698=LINE('',#205490,#27045);
#22699=LINE('',#205493,#27046);
#22700=LINE('',#205496,#27047);
#22701=LINE('',#205500,#27048);
#22702=LINE('',#206972,#27049);
#22703=LINE('',#206974,#27050);
#22704=LINE('',#206976,#27051);
#22705=LINE('',#206978,#27052);
#22706=LINE('',#206980,#27053);
#22707=LINE('',#206982,#27054);
#22708=LINE('',#206984,#27055);
#22709=LINE('',#206986,#27056);
#22710=LINE('',#206988,#27057);
#22711=LINE('',#206990,#27058);
#22712=LINE('',#206999,#27059);
#22713=LINE('',#207001,#27060);
#22714=LINE('',#207003,#27061);
#22715=LINE('',#207005,#27062);
#22716=LINE('',#207007,#27063);
#22717=LINE('',#207009,#27064);
#22718=LINE('',#207011,#27065);
#22719=LINE('',#207013,#27066);
#22720=LINE('',#207015,#27067);
#22721=LINE('',#207017,#27068);
#22722=LINE('',#207019,#27069);
#22723=LINE('',#207021,#27070);
#22724=LINE('',#207023,#27071);
#22725=LINE('',#207025,#27072);
#22726=LINE('',#207043,#27073);
#22727=LINE('',#207045,#27074);
#22728=LINE('',#207047,#27075);
#22729=LINE('',#207049,#27076);
#22730=LINE('',#207051,#27077);
#22731=LINE('',#207053,#27078);
#22732=LINE('',#207055,#27079);
#22733=LINE('',#207057,#27080);
#22734=LINE('',#207059,#27081);
#22735=LINE('',#207061,#27082);
#22736=LINE('',#207063,#27083);
#22737=LINE('',#207065,#27084);
#22738=LINE('',#207067,#27085);
#22739=LINE('',#207069,#27086);
#22740=LINE('',#207071,#27087);
#22741=LINE('',#207073,#27088);
#22742=LINE('',#207075,#27089);
#22743=LINE('',#207077,#27090);
#22744=LINE('',#207079,#27091);
#22745=LINE('',#207081,#27092);
#22746=LINE('',#207083,#27093);
#22747=LINE('',#207085,#27094);
#22748=LINE('',#207087,#27095);
#22749=LINE('',#207089,#27096);
#22750=LINE('',#207091,#27097);
#22751=LINE('',#207093,#27098);
#22752=LINE('',#207095,#27099);
#22753=LINE('',#207097,#27100);
#22754=LINE('',#210831,#27101);
#22755=LINE('',#210833,#27102);
#22756=LINE('',#210871,#27103);
#22757=LINE('',#210872,#27104);
#22758=LINE('',#210875,#27105);
#22759=LINE('',#210877,#27106);
#22760=LINE('',#210914,#27107);
#22761=LINE('',#210915,#27108);
#22762=LINE('',#210918,#27109);
#22763=LINE('',#210920,#27110);
#22764=LINE('',#210957,#27111);
#22765=LINE('',#210958,#27112);
#22766=LINE('',#210961,#27113);
#22767=LINE('',#210963,#27114);
#22768=LINE('',#211000,#27115);
#22769=LINE('',#211001,#27116);
#22770=LINE('',#211003,#27117);
#22771=LINE('',#211004,#27118);
#22772=LINE('',#211006,#27119);
#22773=LINE('',#211007,#27120);
#22774=LINE('',#211009,#27121);
#22775=LINE('',#211010,#27122);
#22776=LINE('',#211012,#27123);
#22777=LINE('',#211013,#27124);
#22778=LINE('',#211015,#27125);
#22779=LINE('',#211016,#27126);
#22780=LINE('',#211018,#27127);
#22781=LINE('',#211019,#27128);
#22782=LINE('',#211021,#27129);
#22783=LINE('',#211022,#27130);
#22784=LINE('',#211024,#27131);
#22785=LINE('',#211025,#27132);
#22786=LINE('',#211039,#27133);
#22787=LINE('',#211040,#27134);
#22788=LINE('',#211063,#27135);
#22789=LINE('',#211064,#27136);
#22790=LINE('',#211084,#27137);
#22791=LINE('',#211085,#27138);
#22792=LINE('',#211099,#27139);
#22793=LINE('',#211100,#27140);
#22794=LINE('',#211123,#27141);
#22795=LINE('',#211124,#27142);
#22796=LINE('',#211129,#27143);
#22797=LINE('',#211130,#27144);
#22798=LINE('',#211147,#27145);
#22799=LINE('',#211148,#27146);
#22800=LINE('',#211171,#27147);
#22801=LINE('',#211172,#27148);
#22802=LINE('',#211177,#27149);
#22803=LINE('',#211178,#27150);
#22804=LINE('',#211195,#27151);
#22805=LINE('',#211196,#27152);
#22806=LINE('',#211201,#27153);
#22807=LINE('',#211202,#27154);
#22808=LINE('',#211219,#27155);
#22809=LINE('',#211220,#27156);
#22810=LINE('',#211225,#27157);
#22811=LINE('',#211226,#27158);
#22812=LINE('',#211243,#27159);
#22813=LINE('',#211244,#27160);
#22814=LINE('',#211249,#27161);
#22815=LINE('',#211250,#27162);
#22816=LINE('',#211273,#27163);
#22817=LINE('',#211274,#27164);
#22818=LINE('',#211297,#27165);
#22819=LINE('',#211298,#27166);
#22820=LINE('',#211303,#27167);
#22821=LINE('',#211304,#27168);
#22822=LINE('',#211321,#27169);
#22823=LINE('',#211322,#27170);
#22824=LINE('',#211327,#27171);
#22825=LINE('',#211328,#27172);
#22826=LINE('',#211345,#27173);
#22827=LINE('',#211346,#27174);
#22828=LINE('',#211351,#27175);
#22829=LINE('',#211352,#27176);
#22830=LINE('',#211369,#27177);
#22831=LINE('',#211370,#27178);
#22832=LINE('',#211375,#27179);
#22833=LINE('',#211376,#27180);
#22834=LINE('',#211393,#27181);
#22835=LINE('',#211394,#27182);
#22836=LINE('',#211399,#27183);
#22837=LINE('',#211400,#27184);
#22838=LINE('',#211417,#27185);
#22839=LINE('',#211418,#27186);
#22840=LINE('',#211423,#27187);
#22841=LINE('',#211424,#27188);
#22842=LINE('',#211441,#27189);
#22843=LINE('',#211442,#27190);
#22844=LINE('',#211447,#27191);
#22845=LINE('',#211448,#27192);
#22846=LINE('',#211465,#27193);
#22847=LINE('',#211466,#27194);
#22848=LINE('',#211471,#27195);
#22849=LINE('',#211472,#27196);
#22850=LINE('',#211489,#27197);
#22851=LINE('',#211490,#27198);
#22852=LINE('',#211495,#27199);
#22853=LINE('',#211496,#27200);
#22854=LINE('',#211513,#27201);
#22855=LINE('',#211514,#27202);
#22856=LINE('',#211537,#27203);
#22857=LINE('',#211538,#27204);
#22858=LINE('',#211543,#27205);
#22859=LINE('',#211544,#27206);
#22860=LINE('',#211561,#27207);
#22861=LINE('',#211562,#27208);
#22862=LINE('',#211597,#27209);
#22863=LINE('',#211598,#27210);
#22864=LINE('',#211603,#27211);
#22865=LINE('',#211604,#27212);
#22866=LINE('',#211621,#27213);
#22867=LINE('',#211622,#27214);
#22868=LINE('',#211645,#27215);
#22869=LINE('',#211646,#27216);
#22870=LINE('',#211651,#27217);
#22871=LINE('',#211652,#27218);
#22872=LINE('',#211669,#27219);
#22873=LINE('',#211670,#27220);
#22874=LINE('',#211675,#27221);
#22875=LINE('',#211676,#27222);
#22876=LINE('',#211693,#27223);
#22877=LINE('',#211694,#27224);
#22878=LINE('',#211717,#27225);
#22879=LINE('',#211718,#27226);
#22880=LINE('',#211723,#27227);
#22881=LINE('',#211724,#27228);
#22882=LINE('',#211738,#27229);
#22883=LINE('',#211739,#27230);
#22884=LINE('',#211753,#27231);
#22885=LINE('',#211754,#27232);
#22886=LINE('',#211759,#27233);
#22887=LINE('',#211760,#27234);
#22888=LINE('',#211777,#27235);
#22889=LINE('',#211778,#27236);
#22890=LINE('',#211798,#27237);
#22891=LINE('',#211799,#27238);
#22892=LINE('',#211813,#27239);
#22893=LINE('',#211814,#27240);
#22894=LINE('',#211819,#27241);
#22895=LINE('',#211820,#27242);
#22896=LINE('',#211837,#27243);
#22897=LINE('',#211838,#27244);
#22898=LINE('',#211843,#27245);
#22899=LINE('',#211844,#27246);
#22900=LINE('',#211861,#27247);
#22901=LINE('',#211862,#27248);
#22902=LINE('',#211867,#27249);
#22903=LINE('',#211868,#27250);
#22904=LINE('',#211891,#27251);
#22905=LINE('',#211892,#27252);
#22906=LINE('',#211909,#27253);
#22907=LINE('',#211910,#27254);
#22908=LINE('',#211915,#27255);
#22909=LINE('',#211916,#27256);
#22910=LINE('',#211933,#27257);
#22911=LINE('',#211934,#27258);
#22912=LINE('',#211939,#27259);
#22913=LINE('',#211940,#27260);
#22914=LINE('',#211957,#27261);
#22915=LINE('',#211958,#27262);
#22916=LINE('',#211963,#27263);
#22917=LINE('',#211964,#27264);
#22918=LINE('',#211981,#27265);
#22919=LINE('',#211982,#27266);
#22920=LINE('',#211987,#27267);
#22921=LINE('',#211988,#27268);
#22922=LINE('',#212005,#27269);
#22923=LINE('',#212006,#27270);
#22924=LINE('',#212011,#27271);
#22925=LINE('',#212012,#27272);
#22926=LINE('',#212029,#27273);
#22927=LINE('',#212030,#27274);
#22928=LINE('',#212059,#27275);
#22929=LINE('',#212060,#27276);
#22930=LINE('',#212065,#27277);
#22931=LINE('',#212066,#27278);
#22932=LINE('',#212089,#27279);
#22933=LINE('',#212090,#27280);
#22934=LINE('',#212107,#27281);
#22935=LINE('',#212108,#27282);
#22936=LINE('',#212113,#27283);
#22937=LINE('',#212114,#27284);
#22938=LINE('',#212137,#27285);
#22939=LINE('',#212138,#27286);
#22940=LINE('',#212167,#27287);
#22941=LINE('',#212168,#27288);
#22942=LINE('',#212173,#27289);
#22943=LINE('',#212174,#27290);
#22944=LINE('',#212191,#27291);
#22945=LINE('',#212192,#27292);
#22946=LINE('',#212197,#27293);
#22947=LINE('',#212198,#27294);
#22948=LINE('',#212215,#27295);
#22949=LINE('',#212216,#27296);
#22950=LINE('',#212221,#27297);
#22951=LINE('',#212222,#27298);
#22952=LINE('',#212239,#27299);
#22953=LINE('',#212240,#27300);
#22954=LINE('',#212275,#27301);
#22955=LINE('',#212276,#27302);
#22956=LINE('',#212281,#27303);
#22957=LINE('',#212282,#27304);
#22958=LINE('',#212299,#27305);
#22959=LINE('',#212300,#27306);
#22960=LINE('',#212323,#27307);
#22961=LINE('',#212324,#27308);
#22962=LINE('',#212329,#27309);
#22963=LINE('',#212330,#27310);
#22964=LINE('',#212347,#27311);
#22965=LINE('',#212348,#27312);
#22966=LINE('',#212353,#27313);
#22967=LINE('',#212354,#27314);
#22968=LINE('',#212371,#27315);
#22969=LINE('',#212372,#27316);
#22970=LINE('',#212377,#27317);
#22971=LINE('',#212378,#27318);
#22972=LINE('',#212395,#27319);
#22973=LINE('',#212396,#27320);
#22974=LINE('',#212419,#27321);
#22975=LINE('',#212420,#27322);
#22976=LINE('',#212425,#27323);
#22977=LINE('',#212426,#27324);
#22978=LINE('',#212443,#27325);
#22979=LINE('',#212444,#27326);
#22980=LINE('',#212449,#27327);
#22981=LINE('',#212450,#27328);
#22982=LINE('',#212467,#27329);
#22983=LINE('',#212468,#27330);
#22984=LINE('',#212488,#27331);
#22985=LINE('',#212489,#27332);
#22986=LINE('',#212503,#27333);
#22987=LINE('',#212504,#27334);
#22988=LINE('',#212524,#27335);
#22989=LINE('',#212525,#27336);
#22990=LINE('',#212662,#27337);
#22991=LINE('',#212663,#27338);
#22992=LINE('',#212686,#27339);
#22993=LINE('',#212687,#27340);
#22994=LINE('',#212725,#27341);
#22995=LINE('',#212726,#27342);
#22996=LINE('',#212749,#27343);
#22997=LINE('',#212750,#27344);
#22998=LINE('',#212788,#27345);
#22999=LINE('',#212789,#27346);
#23000=LINE('',#212812,#27347);
#23001=LINE('',#212813,#27348);
#23002=LINE('',#212851,#27349);
#23003=LINE('',#212852,#27350);
#23004=LINE('',#212875,#27351);
#23005=LINE('',#212876,#27352);
#23006=LINE('',#222192,#27353);
#23007=LINE('',#222193,#27354);
#23008=LINE('',#222196,#27355);
#23009=LINE('',#222198,#27356);
#23010=LINE('',#222202,#27357);
#23011=LINE('',#222204,#27358);
#23012=LINE('',#222208,#27359);
#23013=LINE('',#222210,#27360);
#23014=LINE('',#222214,#27361);
#23015=LINE('',#222216,#27362);
#23016=LINE('',#222220,#27363);
#23017=LINE('',#222222,#27364);
#23018=LINE('',#222226,#27365);
#23019=LINE('',#222228,#27366);
#23020=LINE('',#222232,#27367);
#23021=LINE('',#222234,#27368);
#23022=LINE('',#222238,#27369);
#23023=LINE('',#222240,#27370);
#23024=LINE('',#222246,#27371);
#23025=LINE('',#222247,#27372);
#23026=LINE('',#222250,#27373);
#23027=LINE('',#222252,#27374);
#23028=LINE('',#222256,#27375);
#23029=LINE('',#222258,#27376);
#23030=LINE('',#222262,#27377);
#23031=LINE('',#222264,#27378);
#23032=LINE('',#222268,#27379);
#23033=LINE('',#222270,#27380);
#23034=LINE('',#222274,#27381);
#23035=LINE('',#222276,#27382);
#23036=LINE('',#222280,#27383);
#23037=LINE('',#222282,#27384);
#23038=LINE('',#222286,#27385);
#23039=LINE('',#222288,#27386);
#23040=LINE('',#222292,#27387);
#23041=LINE('',#222294,#27388);
#23042=LINE('',#222298,#27389);
#23043=LINE('',#222300,#27390);
#23044=LINE('',#222304,#27391);
#23045=LINE('',#222306,#27392);
#23046=LINE('',#222310,#27393);
#23047=LINE('',#222312,#27394);
#23048=LINE('',#222316,#27395);
#23049=LINE('',#222318,#27396);
#23050=LINE('',#222322,#27397);
#23051=LINE('',#222324,#27398);
#23052=LINE('',#222328,#27399);
#23053=LINE('',#222330,#27400);
#23054=LINE('',#222334,#27401);
#23055=LINE('',#222336,#27402);
#23056=LINE('',#222340,#27403);
#23057=LINE('',#222342,#27404);
#23058=LINE('',#222346,#27405);
#23059=LINE('',#222348,#27406);
#23060=LINE('',#222354,#27407);
#23061=LINE('',#222355,#27408);
#23062=LINE('',#222358,#27409);
#23063=LINE('',#222360,#27410);
#23064=LINE('',#222364,#27411);
#23065=LINE('',#222366,#27412);
#23066=LINE('',#222370,#27413);
#23067=LINE('',#222372,#27414);
#23068=LINE('',#222376,#27415);
#23069=LINE('',#222378,#27416);
#23070=LINE('',#222382,#27417);
#23071=LINE('',#222384,#27418);
#23072=LINE('',#222388,#27419);
#23073=LINE('',#222390,#27420);
#23074=LINE('',#222394,#27421);
#23075=LINE('',#222396,#27422);
#23076=LINE('',#222400,#27423);
#23077=LINE('',#222402,#27424);
#23078=LINE('',#222406,#27425);
#23079=LINE('',#222408,#27426);
#23080=LINE('',#222412,#27427);
#23081=LINE('',#222414,#27428);
#23082=LINE('',#222418,#27429);
#23083=LINE('',#222420,#27430);
#23084=LINE('',#222424,#27431);
#23085=LINE('',#222426,#27432);
#23086=LINE('',#222430,#27433);
#23087=LINE('',#222432,#27434);
#23088=LINE('',#222436,#27435);
#23089=LINE('',#222438,#27436);
#23090=LINE('',#222442,#27437);
#23091=LINE('',#222444,#27438);
#23092=LINE('',#222448,#27439);
#23093=LINE('',#222450,#27440);
#23094=LINE('',#222454,#27441);
#23095=LINE('',#222456,#27442);
#23096=LINE('',#222460,#27443);
#23097=LINE('',#222462,#27444);
#23098=LINE('',#222466,#27445);
#23099=LINE('',#222468,#27446);
#23100=LINE('',#222472,#27447);
#23101=LINE('',#222474,#27448);
#23102=LINE('',#222478,#27449);
#23103=LINE('',#222480,#27450);
#23104=LINE('',#222484,#27451);
#23105=LINE('',#222486,#27452);
#23106=LINE('',#222490,#27453);
#23107=LINE('',#222492,#27454);
#23108=LINE('',#222496,#27455);
#23109=LINE('',#222498,#27456);
#23110=LINE('',#222502,#27457);
#23111=LINE('',#222504,#27458);
#23112=LINE('',#222508,#27459);
#23113=LINE('',#222510,#27460);
#23114=LINE('',#222514,#27461);
#23115=LINE('',#222516,#27462);
#23116=LINE('',#222520,#27463);
#23117=LINE('',#222522,#27464);
#23118=LINE('',#222526,#27465);
#23119=LINE('',#222528,#27466);
#23120=LINE('',#222532,#27467);
#23121=LINE('',#222534,#27468);
#23122=LINE('',#222538,#27469);
#23123=LINE('',#222540,#27470);
#23124=LINE('',#222544,#27471);
#23125=LINE('',#222546,#27472);
#23126=LINE('',#222550,#27473);
#23127=LINE('',#222552,#27474);
#23128=LINE('',#222556,#27475);
#23129=LINE('',#222558,#27476);
#23130=LINE('',#222562,#27477);
#23131=LINE('',#222564,#27478);
#23132=LINE('',#222568,#27479);
#23133=LINE('',#222570,#27480);
#23134=LINE('',#222574,#27481);
#23135=LINE('',#222576,#27482);
#23136=LINE('',#222580,#27483);
#23137=LINE('',#222582,#27484);
#23138=LINE('',#222586,#27485);
#23139=LINE('',#222588,#27486);
#23140=LINE('',#222592,#27487);
#23141=LINE('',#222594,#27488);
#23142=LINE('',#222598,#27489);
#23143=LINE('',#222600,#27490);
#23144=LINE('',#222604,#27491);
#23145=LINE('',#222606,#27492);
#23146=LINE('',#222610,#27493);
#23147=LINE('',#222612,#27494);
#23148=LINE('',#222616,#27495);
#23149=LINE('',#222618,#27496);
#23150=LINE('',#222622,#27497);
#23151=LINE('',#222624,#27498);
#23152=LINE('',#222628,#27499);
#23153=LINE('',#222630,#27500);
#23154=LINE('',#222634,#27501);
#23155=LINE('',#222636,#27502);
#23156=LINE('',#222640,#27503);
#23157=LINE('',#222642,#27504);
#23158=LINE('',#222646,#27505);
#23159=LINE('',#222648,#27506);
#23160=LINE('',#222652,#27507);
#23161=LINE('',#222654,#27508);
#23162=LINE('',#222658,#27509);
#23163=LINE('',#222660,#27510);
#23164=LINE('',#222664,#27511);
#23165=LINE('',#222666,#27512);
#23166=LINE('',#222670,#27513);
#23167=LINE('',#222672,#27514);
#23168=LINE('',#222676,#27515);
#23169=LINE('',#222678,#27516);
#23170=LINE('',#222682,#27517);
#23171=LINE('',#222684,#27518);
#23172=LINE('',#222688,#27519);
#23173=LINE('',#222690,#27520);
#23174=LINE('',#222694,#27521);
#23175=LINE('',#222696,#27522);
#23176=LINE('',#222702,#27523);
#23177=LINE('',#222703,#27524);
#23178=LINE('',#222706,#27525);
#23179=LINE('',#222708,#27526);
#23180=LINE('',#222712,#27527);
#23181=LINE('',#222714,#27528);
#23182=LINE('',#222718,#27529);
#23183=LINE('',#222720,#27530);
#23184=LINE('',#222724,#27531);
#23185=LINE('',#222726,#27532);
#23186=LINE('',#222730,#27533);
#23187=LINE('',#222732,#27534);
#23188=LINE('',#222736,#27535);
#23189=LINE('',#222738,#27536);
#23190=LINE('',#222742,#27537);
#23191=LINE('',#222744,#27538);
#23192=LINE('',#222748,#27539);
#23193=LINE('',#222750,#27540);
#23194=LINE('',#222754,#27541);
#23195=LINE('',#222756,#27542);
#23196=LINE('',#222760,#27543);
#23197=LINE('',#222762,#27544);
#23198=LINE('',#222766,#27545);
#23199=LINE('',#222768,#27546);
#23200=LINE('',#222772,#27547);
#23201=LINE('',#222774,#27548);
#23202=LINE('',#222778,#27549);
#23203=LINE('',#222780,#27550);
#23204=LINE('',#222784,#27551);
#23205=LINE('',#222786,#27552);
#23206=LINE('',#222790,#27553);
#23207=LINE('',#222792,#27554);
#23208=LINE('',#222796,#27555);
#23209=LINE('',#222798,#27556);
#23210=LINE('',#222802,#27557);
#23211=LINE('',#222804,#27558);
#23212=LINE('',#222808,#27559);
#23213=LINE('',#222810,#27560);
#23214=LINE('',#222814,#27561);
#23215=LINE('',#222816,#27562);
#23216=LINE('',#222820,#27563);
#23217=LINE('',#222822,#27564);
#23218=LINE('',#222826,#27565);
#23219=LINE('',#222828,#27566);
#23220=LINE('',#222832,#27567);
#23221=LINE('',#222834,#27568);
#23222=LINE('',#222838,#27569);
#23223=LINE('',#222840,#27570);
#23224=LINE('',#222846,#27571);
#23225=LINE('',#222847,#27572);
#23226=LINE('',#222850,#27573);
#23227=LINE('',#222852,#27574);
#23228=LINE('',#222856,#27575);
#23229=LINE('',#222858,#27576);
#23230=LINE('',#222862,#27577);
#23231=LINE('',#222864,#27578);
#23232=LINE('',#222868,#27579);
#23233=LINE('',#222870,#27580);
#23234=LINE('',#222874,#27581);
#23235=LINE('',#222876,#27582);
#23236=LINE('',#222880,#27583);
#23237=LINE('',#222882,#27584);
#23238=LINE('',#222886,#27585);
#23239=LINE('',#222888,#27586);
#23240=LINE('',#222892,#27587);
#23241=LINE('',#222894,#27588);
#23242=LINE('',#222898,#27589);
#23243=LINE('',#222900,#27590);
#23244=LINE('',#222904,#27591);
#23245=LINE('',#222906,#27592);
#23246=LINE('',#222910,#27593);
#23247=LINE('',#222912,#27594);
#23248=LINE('',#222916,#27595);
#23249=LINE('',#222918,#27596);
#23250=LINE('',#222922,#27597);
#23251=LINE('',#222924,#27598);
#23252=LINE('',#222928,#27599);
#23253=LINE('',#222930,#27600);
#23254=LINE('',#222934,#27601);
#23255=LINE('',#222936,#27602);
#23256=LINE('',#222942,#27603);
#23257=LINE('',#222943,#27604);
#23258=LINE('',#222946,#27605);
#23259=LINE('',#222948,#27606);
#23260=LINE('',#222952,#27607);
#23261=LINE('',#222954,#27608);
#23262=LINE('',#222958,#27609);
#23263=LINE('',#222960,#27610);
#23264=LINE('',#222964,#27611);
#23265=LINE('',#222966,#27612);
#23266=LINE('',#222972,#27613);
#23267=LINE('',#222973,#27614);
#23268=LINE('',#222976,#27615);
#23269=LINE('',#222978,#27616);
#23270=LINE('',#222984,#27617);
#23271=LINE('',#222985,#27618);
#23272=LINE('',#222988,#27619);
#23273=LINE('',#222990,#27620);
#23274=LINE('',#222994,#27621);
#23275=LINE('',#222996,#27622);
#23276=LINE('',#223000,#27623);
#23277=LINE('',#223002,#27624);
#23278=LINE('',#223006,#27625);
#23279=LINE('',#223010,#27626);
#23280=LINE('',#223016,#27627);
#23281=LINE('',#223024,#27628);
#23282=LINE('',#223045,#27629);
#23283=LINE('',#223047,#27630);
#23284=LINE('',#223055,#27631);
#23285=LINE('',#223057,#27632);
#23286=LINE('',#223063,#27633);
#23287=LINE('',#223065,#27634);
#23288=LINE('',#223067,#27635);
#23289=LINE('',#223069,#27636);
#23290=LINE('',#223071,#27637);
#23291=LINE('',#223073,#27638);
#23292=LINE('',#223075,#27639);
#23293=LINE('',#223077,#27640);
#23294=LINE('',#223079,#27641);
#23295=LINE('',#223081,#27642);
#23296=LINE('',#223083,#27643);
#23297=LINE('',#223085,#27644);
#23298=LINE('',#223087,#27645);
#23299=LINE('',#223089,#27646);
#23300=LINE('',#223091,#27647);
#23301=LINE('',#223093,#27648);
#23302=LINE('',#223095,#27649);
#23303=LINE('',#223097,#27650);
#23304=LINE('',#223099,#27651);
#23305=LINE('',#223101,#27652);
#23306=LINE('',#223103,#27653);
#23307=LINE('',#223105,#27654);
#23308=LINE('',#223107,#27655);
#23309=LINE('',#223109,#27656);
#23310=LINE('',#223111,#27657);
#23311=LINE('',#223113,#27658);
#23312=LINE('',#223115,#27659);
#23313=LINE('',#223117,#27660);
#23314=LINE('',#223119,#27661);
#23315=LINE('',#223121,#27662);
#23316=LINE('',#223123,#27663);
#23317=LINE('',#223125,#27664);
#23318=LINE('',#223129,#27665);
#23319=LINE('',#223131,#27666);
#23320=LINE('',#223133,#27667);
#23321=LINE('',#223134,#27668);
#23322=LINE('',#223138,#27669);
#23323=LINE('',#223139,#27670);
#23324=LINE('',#223140,#27671);
#23325=LINE('',#223143,#27672);
#23326=LINE('',#223145,#27673);
#23327=LINE('',#223146,#27674);
#23328=LINE('',#223148,#27675);
#23329=LINE('',#223150,#27676);
#23330=LINE('',#223152,#27677);
#23331=LINE('',#223154,#27678);
#23332=LINE('',#223156,#27679);
#23333=LINE('',#223158,#27680);
#23334=LINE('',#223160,#27681);
#23335=LINE('',#223162,#27682);
#23336=LINE('',#223164,#27683);
#23337=LINE('',#223166,#27684);
#23338=LINE('',#223168,#27685);
#23339=LINE('',#223170,#27686);
#23340=LINE('',#223172,#27687);
#23341=LINE('',#223174,#27688);
#23342=LINE('',#223176,#27689);
#23343=LINE('',#223178,#27690);
#23344=LINE('',#223180,#27691);
#23345=LINE('',#223182,#27692);
#23346=LINE('',#223184,#27693);
#23347=LINE('',#223186,#27694);
#23348=LINE('',#223188,#27695);
#23349=LINE('',#223190,#27696);
#23350=LINE('',#223211,#27697);
#23351=LINE('',#223212,#27698);
#23352=LINE('',#223213,#27699);
#23353=LINE('',#223214,#27700);
#23354=LINE('',#223215,#27701);
#23355=LINE('',#223216,#27702);
#23356=LINE('',#223217,#27703);
#23357=LINE('',#223218,#27704);
#23358=LINE('',#223219,#27705);
#23359=LINE('',#223221,#27706);
#23360=LINE('',#223223,#27707);
#23361=LINE('',#223224,#27708);
#23362=LINE('',#223225,#27709);
#23363=LINE('',#223226,#27710);
#23364=LINE('',#223227,#27711);
#23365=LINE('',#223229,#27712);
#23366=LINE('',#223230,#27713);
#23367=LINE('',#223236,#27714);
#23368=LINE('',#223237,#27715);
#23369=LINE('',#223243,#27716);
#23370=LINE('',#223244,#27717);
#23371=LINE('',#223246,#27718);
#23372=LINE('',#223247,#27719);
#23373=LINE('',#223249,#27720);
#23374=LINE('',#223250,#27721);
#23375=LINE('',#223252,#27722);
#23376=LINE('',#223253,#27723);
#23377=LINE('',#223255,#27724);
#23378=LINE('',#223256,#27725);
#23379=LINE('',#223257,#27726);
#23380=LINE('',#223259,#27727);
#23381=LINE('',#223260,#27728);
#23382=LINE('',#223261,#27729);
#23383=LINE('',#223262,#27730);
#23384=LINE('',#223263,#27731);
#23385=LINE('',#223264,#27732);
#23386=LINE('',#223265,#27733);
#23387=LINE('',#223266,#27734);
#23388=LINE('',#223272,#27735);
#23389=LINE('',#223278,#27736);
#23390=LINE('',#223279,#27737);
#23391=LINE('',#223280,#27738);
#23392=LINE('',#223281,#27739);
#23393=LINE('',#223282,#27740);
#23394=LINE('',#223284,#27741);
#23395=LINE('',#223285,#27742);
#23396=LINE('',#223286,#27743);
#23397=LINE('',#223287,#27744);
#23398=LINE('',#223288,#27745);
#23399=LINE('',#223289,#27746);
#23400=LINE('',#223290,#27747);
#23401=LINE('',#223291,#27748);
#23402=LINE('',#223294,#27749);
#23403=LINE('',#223296,#27750);
#23404=LINE('',#223301,#27751);
#23405=LINE('',#223304,#27752);
#23406=LINE('',#223308,#27753);
#23407=LINE('',#223312,#27754);
#23408=LINE('',#223317,#27755);
#23409=LINE('',#223320,#27756);
#23410=LINE('',#223327,#27757);
#23411=LINE('',#223336,#27758);
#23412=LINE('',#223340,#27759);
#23413=LINE('',#223341,#27760);
#23414=LINE('',#223347,#27761);
#23415=LINE('',#223362,#27762);
#23416=LINE('',#223377,#27763);
#23417=LINE('',#223378,#27764);
#23418=LINE('',#223386,#27765);
#23419=LINE('',#223388,#27766);
#23420=LINE('',#223405,#27767);
#23421=LINE('',#223407,#27768);
#23422=LINE('',#223428,#27769);
#23423=LINE('',#223429,#27770);
#23424=LINE('',#225928,#27771);
#23425=LINE('',#225931,#27772);
#23426=LINE('',#225939,#27773);
#23427=LINE('',#225948,#27774);
#23428=LINE('',#225954,#27775);
#23429=LINE('',#225960,#27776);
#23430=LINE('',#225977,#27777);
#23431=LINE('',#225980,#27778);
#23432=LINE('',#228081,#27779);
#23433=LINE('',#228088,#27780);
#23434=LINE('',#228101,#27781);
#23435=LINE('',#228111,#27782);
#23436=LINE('',#228118,#27783);
#23437=LINE('',#228120,#27784);
#23438=LINE('',#228131,#27785);
#23439=LINE('',#228143,#27786);
#23440=LINE('',#228177,#27787);
#23441=LINE('',#228178,#27788);
#23442=LINE('',#228182,#27789);
#23443=LINE('',#228186,#27790);
#23444=LINE('',#228190,#27791);
#23445=LINE('',#228196,#27792);
#23446=LINE('',#228200,#27793);
#23447=LINE('',#228204,#27794);
#23448=LINE('',#229182,#27795);
#23449=LINE('',#229254,#27796);
#23450=LINE('',#229256,#27797);
#23451=LINE('',#230393,#27798);
#23452=LINE('',#230394,#27799);
#23453=LINE('',#230396,#27800);
#23454=LINE('',#230398,#27801);
#23455=LINE('',#230401,#27802);
#23456=LINE('',#230402,#27803);
#23457=LINE('',#230405,#27804);
#23458=LINE('',#230406,#27805);
#23459=LINE('',#230411,#27806);
#23460=LINE('',#230416,#27807);
#23461=LINE('',#230770,#27808);
#23462=LINE('',#230772,#27809);
#23463=LINE('',#230776,#27810);
#23464=LINE('',#230780,#27811);
#23465=LINE('',#230784,#27812);
#23466=LINE('',#230788,#27813);
#23467=LINE('',#230792,#27814);
#23468=LINE('',#230799,#27815);
#23469=LINE('',#230821,#27816);
#23470=LINE('',#230822,#27817);
#23471=LINE('',#230825,#27818);
#23472=LINE('',#230827,#27819);
#23473=LINE('',#230829,#27820);
#23474=LINE('',#230831,#27821);
#23475=LINE('',#230833,#27822);
#23476=LINE('',#230835,#27823);
#23477=LINE('',#230918,#27824);
#23478=LINE('',#231017,#27825);
#23479=LINE('',#231103,#27826);
#23480=LINE('',#231223,#27827);
#23481=LINE('',#231229,#27828);
#23482=LINE('',#231230,#27829);
#23483=LINE('',#231232,#27830);
#23484=LINE('',#231234,#27831);
#23485=LINE('',#231236,#27832);
#23486=LINE('',#231237,#27833);
#23487=LINE('',#231239,#27834);
#23488=LINE('',#231241,#27835);
#23489=LINE('',#231263,#27836);
#23490=LINE('',#231264,#27837);
#23491=LINE('',#231266,#27838);
#23492=LINE('',#231268,#27839);
#23493=LINE('',#231270,#27840);
#23494=LINE('',#231273,#27841);
#23495=LINE('',#231275,#27842);
#23496=LINE('',#231277,#27843);
#23497=LINE('',#232815,#27844);
#23498=LINE('',#232821,#27845);
#23499=LINE('',#232828,#27846);
#23500=LINE('',#232838,#27847);
#23501=LINE('',#232848,#27848);
#23502=LINE('',#232858,#27849);
#23503=LINE('',#232874,#27850);
#23504=LINE('',#232900,#27851);
#23505=LINE('',#233024,#27852);
#23506=LINE('',#233025,#27853);
#23507=LINE('',#233027,#27854);
#23508=LINE('',#233029,#27855);
#23509=LINE('',#233031,#27856);
#23510=LINE('',#233033,#27857);
#23511=LINE('',#233158,#27858);
#23512=LINE('',#233159,#27859);
#23513=LINE('',#233161,#27860);
#23514=LINE('',#233163,#27861);
#23515=LINE('',#233165,#27862);
#23516=LINE('',#233167,#27863);
#23517=LINE('',#233172,#27864);
#23518=LINE('',#233178,#27865);
#23519=LINE('',#233185,#27866);
#23520=LINE('',#233195,#27867);
#23521=LINE('',#233205,#27868);
#23522=LINE('',#233215,#27869);
#23523=LINE('',#233231,#27870);
#23524=LINE('',#233257,#27871);
#23525=LINE('',#233322,#27872);
#23526=LINE('',#233325,#27873);
#23527=LINE('',#233327,#27874);
#23528=LINE('',#233328,#27875);
#23529=LINE('',#233330,#27876);
#23530=LINE('',#233332,#27877);
#23531=LINE('',#233340,#27878);
#23532=LINE('',#233342,#27879);
#23533=LINE('',#233348,#27880);
#23534=LINE('',#233354,#27881);
#23535=LINE('',#233361,#27882);
#23536=LINE('',#233376,#27883);
#23537=LINE('',#233377,#27884);
#23538=LINE('',#233382,#27885);
#23539=LINE('',#233383,#27886);
#23540=LINE('',#233400,#27887);
#23541=LINE('',#233401,#27888);
#23542=LINE('',#233406,#27889);
#23543=LINE('',#233407,#27890);
#23544=LINE('',#233413,#27891);
#23545=LINE('',#233415,#27892);
#23546=LINE('',#233416,#27893);
#23547=LINE('',#233419,#27894);
#23548=LINE('',#233423,#27895);
#23549=LINE('',#233428,#27896);
#23550=LINE('',#233430,#27897);
#23551=LINE('',#233432,#27898);
#23552=LINE('',#233433,#27899);
#23553=LINE('',#233449,#27900);
#23554=LINE('',#233458,#27901);
#23555=LINE('',#233475,#27902);
#23556=LINE('',#233477,#27903);
#23557=LINE('',#233481,#27904);
#23558=LINE('',#233485,#27905);
#23559=LINE('',#233491,#27906);
#23560=LINE('',#233494,#27907);
#23561=LINE('',#233507,#27908);
#23562=LINE('',#233509,#27909);
#23563=LINE('',#233519,#27910);
#23564=LINE('',#233521,#27911);
#23565=LINE('',#233533,#27912);
#23566=LINE('',#233535,#27913);
#23567=LINE('',#233539,#27914);
#23568=LINE('',#233541,#27915);
#23569=LINE('',#233544,#27916);
#23570=LINE('',#233545,#27917);
#23571=LINE('',#233547,#27918);
#23572=LINE('',#233549,#27919);
#23573=LINE('',#233551,#27920);
#23574=LINE('',#233553,#27921);
#23575=LINE('',#233555,#27922);
#23576=LINE('',#233557,#27923);
#23577=LINE('',#233560,#27924);
#23578=LINE('',#233562,#27925);
#23579=LINE('',#233564,#27926);
#23580=LINE('',#233566,#27927);
#23581=LINE('',#233568,#27928);
#23582=LINE('',#233634,#27929);
#23583=LINE('',#233637,#27930);
#23584=LINE('',#233639,#27931);
#23585=LINE('',#233640,#27932);
#23586=LINE('',#233642,#27933);
#23587=LINE('',#233644,#27934);
#23588=LINE('',#233652,#27935);
#23589=LINE('',#233654,#27936);
#23590=LINE('',#233661,#27937);
#23591=LINE('',#233673,#27938);
#23592=LINE('',#233684,#27939);
#23593=LINE('',#233685,#27940);
#23594=LINE('',#233705,#27941);
#23595=LINE('',#233706,#27942);
#23596=LINE('',#233712,#27943);
#23597=LINE('',#233715,#27944);
#23598=LINE('',#233726,#27945);
#23599=LINE('',#233727,#27946);
#23600=LINE('',#233747,#27947);
#23601=LINE('',#233748,#27948);
#23602=LINE('',#233754,#27949);
#23603=LINE('',#233757,#27950);
#23604=LINE('',#233768,#27951);
#23605=LINE('',#233769,#27952);
#23606=LINE('',#233780,#27953);
#23607=LINE('',#233781,#27954);
#23608=LINE('',#233792,#27955);
#23609=LINE('',#233793,#27956);
#23610=LINE('',#233804,#27957);
#23611=LINE('',#233805,#27958);
#23612=LINE('',#233811,#27959);
#23613=LINE('',#233814,#27960);
#23614=LINE('',#233825,#27961);
#23615=LINE('',#233826,#27962);
#23616=LINE('',#233846,#27963);
#23617=LINE('',#233847,#27964);
#23618=LINE('',#233853,#27965);
#23619=LINE('',#233856,#27966);
#23620=LINE('',#233867,#27967);
#23621=LINE('',#233868,#27968);
#23622=LINE('',#233885,#27969);
#23623=LINE('',#233886,#27970);
#23624=LINE('',#233897,#27971);
#23625=LINE('',#233898,#27972);
#23626=LINE('',#233909,#27973);
#23627=LINE('',#233910,#27974);
#23628=LINE('',#233916,#27975);
#23629=LINE('',#233919,#27976);
#23630=LINE('',#233930,#27977);
#23631=LINE('',#233931,#27978);
#23632=LINE('',#233954,#27979);
#23633=LINE('',#233955,#27980);
#23634=LINE('',#233966,#27981);
#23635=LINE('',#233967,#27982);
#23636=LINE('',#233973,#27983);
#23637=LINE('',#233976,#27984);
#23638=LINE('',#233987,#27985);
#23639=LINE('',#233988,#27986);
#23640=LINE('',#234011,#27987);
#23641=LINE('',#234012,#27988);
#23642=LINE('',#234023,#27989);
#23643=LINE('',#234024,#27990);
#23644=LINE('',#234030,#27991);
#23645=LINE('',#234033,#27992);
#23646=LINE('',#234044,#27993);
#23647=LINE('',#234045,#27994);
#23648=LINE('',#234068,#27995);
#23649=LINE('',#234069,#27996);
#23650=LINE('',#234080,#27997);
#23651=LINE('',#234081,#27998);
#23652=LINE('',#234087,#27999);
#23653=LINE('',#234090,#28000);
#23654=LINE('',#234101,#28001);
#23655=LINE('',#234102,#28002);
#23656=LINE('',#234125,#28003);
#23657=LINE('',#234126,#28004);
#23658=LINE('',#234137,#28005);
#23659=LINE('',#234138,#28006);
#23660=LINE('',#234144,#28007);
#23661=LINE('',#234147,#28008);
#23662=LINE('',#234158,#28009);
#23663=LINE('',#234159,#28010);
#23664=LINE('',#234182,#28011);
#23665=LINE('',#234183,#28012);
#23666=LINE('',#234194,#28013);
#23667=LINE('',#234195,#28014);
#23668=LINE('',#234201,#28015);
#23669=LINE('',#234204,#28016);
#23670=LINE('',#234215,#28017);
#23671=LINE('',#234216,#28018);
#23672=LINE('',#234239,#28019);
#23673=LINE('',#234240,#28020);
#23674=LINE('',#234251,#28021);
#23675=LINE('',#234252,#28022);
#23676=LINE('',#234258,#28023);
#23677=LINE('',#234261,#28024);
#23678=LINE('',#234272,#28025);
#23679=LINE('',#234273,#28026);
#23680=LINE('',#234284,#28027);
#23681=LINE('',#234285,#28028);
#23682=LINE('',#234302,#28029);
#23683=LINE('',#234303,#28030);
#23684=LINE('',#234314,#28031);
#23685=LINE('',#234315,#28032);
#23686=LINE('',#234321,#28033);
#23687=LINE('',#234324,#28034);
#23688=LINE('',#234335,#28035);
#23689=LINE('',#234336,#28036);
#23690=LINE('',#234347,#28037);
#23691=LINE('',#234348,#28038);
#23692=LINE('',#234359,#28039);
#23693=LINE('',#234360,#28040);
#23694=LINE('',#234371,#28041);
#23695=LINE('',#234372,#28042);
#23696=LINE('',#234387,#28043);
#23697=LINE('',#234390,#28044);
#23698=LINE('',#234401,#28045);
#23699=LINE('',#234402,#28046);
#23700=LINE('',#234413,#28047);
#23701=LINE('',#234414,#28048);
#23702=LINE('',#234417,#28049);
#23703=LINE('',#234419,#28050);
#23704=LINE('',#234423,#28051);
#23705=LINE('',#234425,#28052);
#23706=LINE('',#234429,#28053);
#23707=LINE('',#234431,#28054);
#23708=LINE('',#234435,#28055);
#23709=LINE('',#234437,#28056);
#23710=LINE('',#234441,#28057);
#23711=LINE('',#234443,#28058);
#23712=LINE('',#234447,#28059);
#23713=LINE('',#234449,#28060);
#23714=LINE('',#234453,#28061);
#23715=LINE('',#234455,#28062);
#23716=LINE('',#234459,#28063);
#23717=LINE('',#234461,#28064);
#23718=LINE('',#234465,#28065);
#23719=LINE('',#234467,#28066);
#23720=LINE('',#234471,#28067);
#23721=LINE('',#234473,#28068);
#23722=LINE('',#234477,#28069);
#23723=LINE('',#234479,#28070);
#23724=LINE('',#234483,#28071);
#23725=LINE('',#234485,#28072);
#23726=LINE('',#234489,#28073);
#23727=LINE('',#234491,#28074);
#23728=LINE('',#234495,#28075);
#23729=LINE('',#234497,#28076);
#23730=LINE('',#234501,#28077);
#23731=LINE('',#234503,#28078);
#23732=LINE('',#234507,#28079);
#23733=LINE('',#234509,#28080);
#23734=LINE('',#234513,#28081);
#23735=LINE('',#234515,#28082);
#23736=LINE('',#234519,#28083);
#23737=LINE('',#234521,#28084);
#23738=LINE('',#234525,#28085);
#23739=LINE('',#234527,#28086);
#23740=LINE('',#234531,#28087);
#23741=LINE('',#234533,#28088);
#23742=LINE('',#234537,#28089);
#23743=LINE('',#234539,#28090);
#23744=LINE('',#234543,#28091);
#23745=LINE('',#234545,#28092);
#23746=LINE('',#234549,#28093);
#23747=LINE('',#234551,#28094);
#23748=LINE('',#234555,#28095);
#23749=LINE('',#234557,#28096);
#23750=LINE('',#234561,#28097);
#23751=LINE('',#234563,#28098);
#23752=LINE('',#234567,#28099);
#23753=LINE('',#234569,#28100);
#23754=LINE('',#234576,#28101);
#23755=LINE('',#234577,#28102);
#23756=LINE('',#234579,#28103);
#23757=LINE('',#234580,#28104);
#23758=LINE('',#234581,#28105);
#23759=LINE('',#234582,#28106);
#23760=LINE('',#234583,#28107);
#23761=LINE('',#234584,#28108);
#23762=LINE('',#234585,#28109);
#23763=LINE('',#234586,#28110);
#23764=LINE('',#234587,#28111);
#23765=LINE('',#234588,#28112);
#23766=LINE('',#234589,#28113);
#23767=LINE('',#234591,#28114);
#23768=LINE('',#234594,#28115);
#23769=LINE('',#234597,#28116);
#23770=LINE('',#234599,#28117);
#23771=LINE('',#234601,#28118);
#23772=LINE('',#234604,#28119);
#23773=LINE('',#234605,#28120);
#23774=LINE('',#234607,#28121);
#23775=LINE('',#234609,#28122);
#23776=LINE('',#234611,#28123);
#23777=LINE('',#234613,#28124);
#23778=LINE('',#234615,#28125);
#23779=LINE('',#234617,#28126);
#23780=LINE('',#234619,#28127);
#23781=LINE('',#234621,#28128);
#23782=LINE('',#234623,#28129);
#23783=LINE('',#234625,#28130);
#23784=LINE('',#234627,#28131);
#23785=LINE('',#234628,#28132);
#23786=LINE('',#234633,#28133);
#23787=LINE('',#234635,#28134);
#23788=LINE('',#234637,#28135);
#23789=LINE('',#234638,#28136);
#23790=LINE('',#234643,#28137);
#23791=LINE('',#234645,#28138);
#23792=LINE('',#234647,#28139);
#23793=LINE('',#234648,#28140);
#23794=LINE('',#234653,#28141);
#23795=LINE('',#234655,#28142);
#23796=LINE('',#234657,#28143);
#23797=LINE('',#234658,#28144);
#23798=LINE('',#234663,#28145);
#23799=LINE('',#234665,#28146);
#23800=LINE('',#234667,#28147);
#23801=LINE('',#234668,#28148);
#23802=LINE('',#234671,#28149);
#23803=LINE('',#234674,#28150);
#23804=LINE('',#234677,#28151);
#23805=LINE('',#234680,#28152);
#23806=LINE('',#234683,#28153);
#23807=LINE('',#234685,#28154);
#23808=LINE('',#234686,#28155);
#23809=LINE('',#234687,#28156);
#23810=LINE('',#234688,#28157);
#23811=LINE('',#234690,#28158);
#23812=LINE('',#234692,#28159);
#23813=LINE('',#234693,#28160);
#23814=LINE('',#234694,#28161);
#23815=LINE('',#234695,#28162);
#23816=LINE('',#234696,#28163);
#23817=LINE('',#234698,#28164);
#23818=LINE('',#234701,#28165);
#23819=LINE('',#234703,#28166);
#23820=LINE('',#234704,#28167);
#23821=LINE('',#234705,#28168);
#23822=LINE('',#234707,#28169);
#23823=LINE('',#234710,#28170);
#23824=LINE('',#234714,#28171);
#23825=LINE('',#234717,#28172);
#23826=LINE('',#234720,#28173);
#23827=LINE('',#234723,#28174);
#23828=LINE('',#234727,#28175);
#23829=LINE('',#234732,#28176);
#23830=LINE('',#234735,#28177);
#23831=LINE('',#234737,#28178);
#23832=LINE('',#234741,#28179);
#23833=LINE('',#234743,#28180);
#23834=LINE('',#234747,#28181);
#23835=LINE('',#234872,#28182);
#23836=LINE('',#234873,#28183);
#23837=LINE('',#234875,#28184);
#23838=LINE('',#234877,#28185);
#23839=LINE('',#234879,#28186);
#23840=LINE('',#234881,#28187);
#23841=LINE('',#235006,#28188);
#23842=LINE('',#235007,#28189);
#23843=LINE('',#235009,#28190);
#23844=LINE('',#235011,#28191);
#23845=LINE('',#235013,#28192);
#23846=LINE('',#235015,#28193);
#23847=LINE('',#235020,#28194);
#23848=LINE('',#235026,#28195);
#23849=LINE('',#235033,#28196);
#23850=LINE('',#235043,#28197);
#23851=LINE('',#235053,#28198);
#23852=LINE('',#235063,#28199);
#23853=LINE('',#235079,#28200);
#23854=LINE('',#235105,#28201);
#23855=LINE('',#235112,#28202);
#23856=LINE('',#235116,#28203);
#23857=LINE('',#235128,#28204);
#23858=LINE('',#235131,#28205);
#23859=LINE('',#235212,#28206);
#23860=LINE('',#235215,#28207);
#23861=LINE('',#235221,#28208);
#23862=LINE('',#235233,#28209);
#23863=LINE('',#235235,#28210);
#23864=LINE('',#235236,#28211);
#23865=LINE('',#235238,#28212);
#23866=LINE('',#235239,#28213);
#23867=LINE('',#235241,#28214);
#23868=LINE('',#235243,#28215);
#23869=LINE('',#235245,#28216);
#23870=LINE('',#235247,#28217);
#23871=LINE('',#235249,#28218);
#23872=LINE('',#235250,#28219);
#23873=LINE('',#235254,#28220);
#23874=LINE('',#235264,#28221);
#23875=LINE('',#235275,#28222);
#23876=LINE('',#235276,#28223);
#23877=LINE('',#235357,#28224);
#23878=LINE('',#235360,#28225);
#23879=LINE('',#235366,#28226);
#23880=LINE('',#235444,#28227);
#23881=LINE('',#235446,#28228);
#23882=LINE('',#235447,#28229);
#23883=LINE('',#235449,#28230);
#23884=LINE('',#235450,#28231);
#23885=LINE('',#235452,#28232);
#23886=LINE('',#235453,#28233);
#23887=LINE('',#235455,#28234);
#23888=LINE('',#235456,#28235);
#23889=LINE('',#235458,#28236);
#23890=LINE('',#235460,#28237);
#23891=LINE('',#235462,#28238);
#23892=LINE('',#235464,#28239);
#23893=LINE('',#235466,#28240);
#23894=LINE('',#235467,#28241);
#23895=LINE('',#235471,#28242);
#23896=LINE('',#235517,#28243);
#23897=LINE('',#235525,#28244);
#23898=LINE('',#235526,#28245);
#23899=LINE('',#235530,#28246);
#23900=LINE('',#235538,#28247);
#23901=LINE('',#235539,#28248);
#23902=LINE('',#235543,#28249);
#23903=LINE('',#235547,#28250);
#23904=LINE('',#235550,#28251);
#23905=LINE('',#235554,#28252);
#23906=LINE('',#235558,#28253);
#23907=LINE('',#235602,#28254);
#23908=LINE('',#235606,#28255);
#23909=LINE('',#235614,#28256);
#23910=LINE('',#235615,#28257);
#23911=LINE('',#235619,#28258);
#23912=LINE('',#235627,#28259);
#23913=LINE('',#235628,#28260);
#23914=LINE('',#235630,#28261);
#23915=LINE('',#235631,#28262);
#23916=LINE('',#235633,#28263);
#23917=LINE('',#235635,#28264);
#23918=LINE('',#235641,#28265);
#23919=LINE('',#235696,#28266);
#23920=LINE('',#235772,#28267);
#23921=LINE('',#235850,#28268);
#23922=LINE('',#235928,#28269);
#23923=LINE('',#236004,#28270);
#23924=LINE('',#236080,#28271);
#23925=LINE('',#236156,#28272);
#23926=LINE('',#236232,#28273);
#23927=LINE('',#236310,#28274);
#23928=LINE('',#236388,#28275);
#23929=LINE('',#236464,#28276);
#23930=LINE('',#236540,#28277);
#23931=LINE('',#236616,#28278);
#23932=LINE('',#236692,#28279);
#23933=LINE('',#236768,#28280);
#23934=LINE('',#236846,#28281);
#23935=LINE('',#236924,#28282);
#23936=LINE('',#237000,#28283);
#23937=LINE('',#237028,#28284);
#23938=LINE('',#237065,#28285);
#23939=LINE('',#237141,#28286);
#23940=LINE('',#237219,#28287);
#23941=LINE('',#237295,#28288);
#23942=LINE('',#237371,#28289);
#23943=LINE('',#237447,#28290);
#23944=LINE('',#237523,#28291);
#23945=LINE('',#237601,#28292);
#23946=LINE('',#237677,#28293);
#23947=LINE('',#237755,#28294);
#23948=LINE('',#237831,#28295);
#23949=LINE('',#237907,#28296);
#23950=LINE('',#237983,#28297);
#23951=LINE('',#238059,#28298);
#23952=LINE('',#238137,#28299);
#23953=LINE('',#238213,#28300);
#23954=LINE('',#238291,#28301);
#23955=LINE('',#238367,#28302);
#23956=LINE('',#238413,#28303);
#23957=LINE('',#238431,#28304);
#23958=LINE('',#238476,#28305);
#23959=LINE('',#238506,#28306);
#23960=LINE('',#238536,#28307);
#23961=LINE('',#238566,#28308);
#23962=LINE('',#238596,#28309);
#23963=LINE('',#238626,#28310);
#23964=LINE('',#238656,#28311);
#23965=LINE('',#238686,#28312);
#23966=LINE('',#238716,#28313);
#23967=LINE('',#238746,#28314);
#23968=LINE('',#238776,#28315);
#23969=LINE('',#238806,#28316);
#23970=LINE('',#238836,#28317);
#23971=LINE('',#238866,#28318);
#23972=LINE('',#238896,#28319);
#23973=LINE('',#238926,#28320);
#23974=LINE('',#238956,#28321);
#23975=LINE('',#238967,#28322);
#23976=LINE('',#239038,#28323);
#23977=LINE('',#239114,#28324);
#23978=LINE('',#239190,#28325);
#23979=LINE('',#239268,#28326);
#23980=LINE('',#239344,#28327);
#23981=LINE('',#239420,#28328);
#23982=LINE('',#239498,#28329);
#23983=LINE('',#239574,#28330);
#23984=LINE('',#239650,#28331);
#23985=LINE('',#239726,#28332);
#23986=LINE('',#239804,#28333);
#23987=LINE('',#239880,#28334);
#23988=LINE('',#239956,#28335);
#23989=LINE('',#240034,#28336);
#23990=LINE('',#240110,#28337);
#23991=LINE('',#240186,#28338);
#23992=LINE('',#240262,#28339);
#23993=LINE('',#240347,#28340);
#23994=LINE('',#240375,#28341);
#23995=LINE('',#240420,#28342);
#23996=LINE('',#240450,#28343);
#23997=LINE('',#240480,#28344);
#23998=LINE('',#240510,#28345);
#23999=LINE('',#240540,#28346);
#24000=LINE('',#240570,#28347);
#24001=LINE('',#240600,#28348);
#24002=LINE('',#240630,#28349);
#24003=LINE('',#240660,#28350);
#24004=LINE('',#240690,#28351);
#24005=LINE('',#240720,#28352);
#24006=LINE('',#240750,#28353);
#24007=LINE('',#240780,#28354);
#24008=LINE('',#240810,#28355);
#24009=LINE('',#240840,#28356);
#24010=LINE('',#240870,#28357);
#24011=LINE('',#240900,#28358);
#24012=LINE('',#240911,#28359);
#24013=LINE('',#240927,#28360);
#24014=LINE('',#241005,#28361);
#24015=LINE('',#241081,#28362);
#24016=LINE('',#241157,#28363);
#24017=LINE('',#241233,#28364);
#24018=LINE('',#241309,#28365);
#24019=LINE('',#241385,#28366);
#24020=LINE('',#241463,#28367);
#24021=LINE('',#241541,#28368);
#24022=LINE('',#241617,#28369);
#24023=LINE('',#241693,#28370);
#24024=LINE('',#241769,#28371);
#24025=LINE('',#241845,#28372);
#24026=LINE('',#241921,#28373);
#24027=LINE('',#242001,#28374);
#24028=LINE('',#242077,#28375);
#24029=LINE('',#242153,#28376);
#24030=LINE('',#242229,#28377);
#24031=LINE('',#242293,#28378);
#24032=LINE('',#242311,#28379);
#24033=LINE('',#242356,#28380);
#24034=LINE('',#242386,#28381);
#24035=LINE('',#242416,#28382);
#24036=LINE('',#242446,#28383);
#24037=LINE('',#242476,#28384);
#24038=LINE('',#242506,#28385);
#24039=LINE('',#242536,#28386);
#24040=LINE('',#242566,#28387);
#24041=LINE('',#242596,#28388);
#24042=LINE('',#242626,#28389);
#24043=LINE('',#242656,#28390);
#24044=LINE('',#242686,#28391);
#24045=LINE('',#242716,#28392);
#24046=LINE('',#242746,#28393);
#24047=LINE('',#242776,#28394);
#24048=LINE('',#242806,#28395);
#24049=LINE('',#242836,#28396);
#24050=LINE('',#242847,#28397);
#24051=LINE('',#242865,#28398);
#24052=LINE('',#242910,#28399);
#24053=LINE('',#242940,#28400);
#24054=LINE('',#242970,#28401);
#24055=LINE('',#243000,#28402);
#24056=LINE('',#243030,#28403);
#24057=LINE('',#243060,#28404);
#24058=LINE('',#243090,#28405);
#24059=LINE('',#243120,#28406);
#24060=LINE('',#243150,#28407);
#24061=LINE('',#243180,#28408);
#24062=LINE('',#243210,#28409);
#24063=LINE('',#243240,#28410);
#24064=LINE('',#243270,#28411);
#24065=LINE('',#243300,#28412);
#24066=LINE('',#243330,#28413);
#24067=LINE('',#243360,#28414);
#24068=LINE('',#243390,#28415);
#24069=LINE('',#243401,#28416);
#24070=LINE('',#243403,#28417);
#24071=LINE('',#243405,#28418);
#24072=LINE('',#243407,#28419);
#24073=LINE('',#243409,#28420);
#24074=LINE('',#243411,#28421);
#24075=LINE('',#243413,#28422);
#24076=LINE('',#243414,#28423);
#24077=LINE('',#243418,#28424);
#24078=LINE('',#243421,#28425);
#24079=LINE('',#243423,#28426);
#24080=LINE('',#243468,#28427);
#24081=LINE('',#243470,#28428);
#24082=LINE('',#243472,#28429);
#24083=LINE('',#243474,#28430);
#24084=LINE('',#243521,#28431);
#24085=LINE('',#243523,#28432);
#24086=LINE('',#243525,#28433);
#24087=LINE('',#243526,#28434);
#24088=LINE('',#243529,#28435);
#24089=LINE('',#243531,#28436);
#24090=LINE('',#243532,#28437);
#24091=LINE('',#243535,#28438);
#24092=LINE('',#243537,#28439);
#24093=LINE('',#243538,#28440);
#24094=LINE('',#243540,#28441);
#24095=LINE('',#243541,#28442);
#24096=LINE('',#243544,#28443);
#24097=LINE('',#243548,#28444);
#24098=LINE('',#243550,#28445);
#24099=LINE('',#243553,#28446);
#24100=LINE('',#243575,#28447);
#24101=LINE('',#243725,#28448);
#24102=LINE('',#243729,#28449);
#24103=LINE('',#243816,#28450);
#24104=LINE('',#243840,#28451);
#24105=LINE('',#243843,#28452);
#24106=LINE('',#243852,#28453);
#24107=LINE('',#243855,#28454);
#24108=LINE('',#243864,#28455);
#24109=LINE('',#243886,#28456);
#24110=LINE('',#243913,#28457);
#24111=LINE('',#243918,#28458);
#24112=LINE('',#243947,#28459);
#24113=LINE('',#243953,#28460);
#24114=LINE('',#243960,#28461);
#24115=LINE('',#243970,#28462);
#24116=LINE('',#243980,#28463);
#24117=LINE('',#243990,#28464);
#24118=LINE('',#244006,#28465);
#24119=LINE('',#244020,#28466);
#24120=LINE('',#244023,#28467);
#24121=LINE('',#246688,#28468);
#24122=LINE('',#246702,#28469);
#24123=LINE('',#246877,#28470);
#24124=LINE('',#247114,#28471);
#24125=LINE('',#247116,#28472);
#24126=LINE('',#247489,#28473);
#24127=LINE('',#247490,#28474);
#24128=LINE('',#247673,#28475);
#24129=LINE('',#247674,#28476);
#24130=LINE('',#247839,#28477);
#24131=LINE('',#247865,#28478);
#24132=LINE('',#247866,#28479);
#24133=LINE('',#247962,#28480);
#24134=LINE('',#247975,#28481);
#24135=LINE('',#247979,#28482);
#24136=LINE('',#247999,#28483);
#24137=LINE('',#248003,#28484);
#24138=LINE('',#248023,#28485);
#24139=LINE('',#248027,#28486);
#24140=LINE('',#248076,#28487);
#24141=LINE('',#248080,#28488);
#24142=LINE('',#248090,#28489);
#24143=LINE('',#248094,#28490);
#24144=LINE('',#248102,#28491);
#24145=LINE('',#248187,#28492);
#24146=LINE('',#248224,#28493);
#24147=LINE('',#248228,#28494);
#24148=LINE('',#248238,#28495);
#24149=LINE('',#248242,#28496);
#24150=LINE('',#248255,#28497);
#24151=LINE('',#248256,#28498);
#24152=LINE('',#248337,#28499);
#24153=LINE('',#248498,#28500);
#24154=LINE('',#248520,#28501);
#24155=LINE('',#248525,#28502);
#24156=LINE('',#248547,#28503);
#24157=LINE('',#248552,#28504);
#24158=LINE('',#248574,#28505);
#24159=LINE('',#248579,#28506);
#24160=LINE('',#248601,#28507);
#24161=LINE('',#248638,#28508);
#24162=LINE('',#248663,#28509);
#24163=LINE('',#248668,#28510);
#24164=LINE('',#248693,#28511);
#24165=LINE('',#248700,#28512);
#24166=LINE('',#248785,#28513);
#24167=LINE('',#248850,#28514);
#24168=LINE('',#248875,#28515);
#24169=LINE('',#248880,#28516);
#24170=LINE('',#248905,#28517);
#24171=LINE('',#248912,#28518);
#24172=LINE('',#248997,#28519);
#24173=LINE('',#249165,#28520);
#24174=LINE('',#251064,#28521);
#24175=LINE('',#251466,#28522);
#24176=LINE('',#252014,#28523);
#24177=LINE('',#252036,#28524);
#24178=LINE('',#255718,#28525);
#24179=LINE('',#255959,#28526);
#24180=LINE('',#256078,#28527);
#24181=LINE('',#259888,#28528);
#24182=LINE('',#260125,#28529);
#24183=LINE('',#260242,#28530);
#24184=LINE('',#263459,#28531);
#24185=LINE('',#263853,#28532);
#24186=LINE('',#264375,#28533);
#24187=LINE('',#264397,#28534);
#24188=LINE('',#268790,#28535);
#24189=LINE('',#269480,#28536);
#24190=LINE('',#271077,#28537);
#24191=LINE('',#271078,#28538);
#24908=VECTOR('',#105188,1.47499999999998);
#24909=VECTOR('',#105197,2.);
#24910=VECTOR('',#105206,2.5);
#24911=VECTOR('',#105213,1.47499999999998);
#24912=VECTOR('',#105222,2.);
#24913=VECTOR('',#105231,2.5);
#24914=VECTOR('',#105236,1000.);
#24915=VECTOR('',#105239,1000.);
#24916=VECTOR('',#105246,1000.);
#24917=VECTOR('',#105249,1000.);
#24918=VECTOR('',#105262,1000.);
#24919=VECTOR('',#105265,1000.);
#24920=VECTOR('',#105270,1000.);
#24921=VECTOR('',#105271,1000.);
#24922=VECTOR('',#105272,1000.);
#24923=VECTOR('',#105273,1000.);
#24924=VECTOR('',#105274,1000.);
#24925=VECTOR('',#105275,1000.);
#24926=VECTOR('',#105276,1000.);
#24927=VECTOR('',#105277,1000.);
#24928=VECTOR('',#105278,1000.);
#24929=VECTOR('',#105279,1000.);
#24930=VECTOR('',#105280,1000.);
#24931=VECTOR('',#105291,1000.);
#24932=VECTOR('',#105294,1000.);
#24933=VECTOR('',#105299,1000.);
#24934=VECTOR('',#105300,1000.);
#24935=VECTOR('',#105311,1000.);
#24936=VECTOR('',#105312,1000.);
#24937=VECTOR('',#105313,1000.);
#24938=VECTOR('',#105314,1000.);
#24939=VECTOR('',#105315,1000.);
#24940=VECTOR('',#105316,1000.);
#24941=VECTOR('',#105317,1000.);
#24942=VECTOR('',#105318,1000.);
#24943=VECTOR('',#105319,1000.);
#24944=VECTOR('',#105320,1000.);
#24945=VECTOR('',#105323,1000.);
#24946=VECTOR('',#105332,1000.);
#24947=VECTOR('',#105333,1000.);
#24948=VECTOR('',#105348,1000.);
#24949=VECTOR('',#105353,1000.);
#24950=VECTOR('',#105370,1000.);
#24951=VECTOR('',#105371,1000.);
#24952=VECTOR('',#105386,1000.);
#24953=VECTOR('',#105391,1000.);
#24954=VECTOR('',#105408,1000.);
#24955=VECTOR('',#105409,1000.);
#24956=VECTOR('',#105424,1000.);
#24957=VECTOR('',#105427,1000.);
#24958=VECTOR('',#105438,1000.);
#24959=VECTOR('',#105441,1000.);
#24960=VECTOR('',#105454,1000.);
#24961=VECTOR('',#105457,1000.);
#24962=VECTOR('',#105472,1000.);
#24963=VECTOR('',#105475,1000.);
#24964=VECTOR('',#105490,1000.);
#24965=VECTOR('',#105493,1000.);
#24966=VECTOR('',#105508,1000.);
#24967=VECTOR('',#105509,1000.);
#24968=VECTOR('',#105524,1000.);
#24969=VECTOR('',#105527,1000.);
#24970=VECTOR('',#105542,1000.);
#24971=VECTOR('',#105543,1000.);
#24972=VECTOR('',#105558,1000.);
#24973=VECTOR('',#105561,1000.);
#24974=VECTOR('',#105570,1000.);
#24975=VECTOR('',#105573,1000.);
#24976=VECTOR('',#105576,1000.);
#24977=VECTOR('',#105579,1000.);
#24978=VECTOR('',#105582,1000.);
#24979=VECTOR('',#105585,1000.);
#24980=VECTOR('',#105588,1000.);
#24981=VECTOR('',#105591,1000.);
#24982=VECTOR('',#105594,1000.);
#24983=VECTOR('',#105597,1000.);
#24984=VECTOR('',#105600,1000.);
#24985=VECTOR('',#105603,1000.);
#24986=VECTOR('',#105618,1000.);
#24987=VECTOR('',#105621,1000.);
#24988=VECTOR('',#105626,1000.);
#24989=VECTOR('',#105627,1000.);
#24990=VECTOR('',#105628,1000.);
#24991=VECTOR('',#105629,1000.);
#24992=VECTOR('',#105630,1000.);
#24993=VECTOR('',#105631,1000.);
#24994=VECTOR('',#105634,1000.);
#24995=VECTOR('',#105635,1000.);
#24996=VECTOR('',#105636,1000.);
#24997=VECTOR('',#105637,1000.);
#24998=VECTOR('',#105638,1000.);
#24999=VECTOR('',#105649,1000.);
#25000=VECTOR('',#105652,1000.);
#25001=VECTOR('',#105657,1000.);
#25002=VECTOR('',#105658,1000.);
#25003=VECTOR('',#105669,1000.);
#25004=VECTOR('',#105670,1000.);
#25005=VECTOR('',#105671,1000.);
#25006=VECTOR('',#105672,1000.);
#25007=VECTOR('',#105673,1000.);
#25008=VECTOR('',#105674,1000.);
#25009=VECTOR('',#105675,1000.);
#25010=VECTOR('',#105676,1000.);
#25011=VECTOR('',#105677,1000.);
#25012=VECTOR('',#105684,1000.);
#25013=VECTOR('',#105697,1000.);
#25014=VECTOR('',#105714,1000.);
#25015=VECTOR('',#105729,1000.);
#25016=VECTOR('',#105742,1000.);
#25017=VECTOR('',#105757,1000.);
#25018=VECTOR('',#105770,1000.);
#25019=VECTOR('',#105785,1000.);
#25020=VECTOR('',#105798,1000.);
#25021=VECTOR('',#105811,1000.);
#25022=VECTOR('',#105828,1000.);
#25023=VECTOR('',#105841,1000.);
#25024=VECTOR('',#105846,1000.);
#25025=VECTOR('',#105853,1000.);
#25026=VECTOR('',#105860,1000.);
#25027=VECTOR('',#105867,1000.);
#25028=VECTOR('',#105870,1000.);
#25029=VECTOR('',#105877,1000.);
#25030=VECTOR('',#105882,1000.);
#25031=VECTOR('',#105889,1000.);
#25032=VECTOR('',#105896,1000.);
#25033=VECTOR('',#105903,1000.);
#25034=VECTOR('',#105906,1000.);
#25035=VECTOR('',#105911,1000.);
#25036=VECTOR('',#105916,1000.);
#25037=VECTOR('',#105925,1000.);
#25038=VECTOR('',#105932,1000.);
#25039=VECTOR('',#105935,1000.);
#25040=VECTOR('',#105942,1000.);
#25041=VECTOR('',#105949,1000.);
#25042=VECTOR('',#105956,1000.);
#25043=VECTOR('',#105959,1000.);
#25044=VECTOR('',#105962,1000.);
#25045=VECTOR('',#105967,1000.);
#25046=VECTOR('',#105976,1000.);
#25047=VECTOR('',#105983,1000.);
#25048=VECTOR('',#105986,1000.);
#25049=VECTOR('',#105995,1000.);
#25050=VECTOR('',#106002,1000.);
#25051=VECTOR('',#106009,1000.);
#25052=VECTOR('',#106016,1000.);
#25053=VECTOR('',#106023,1000.);
#25054=VECTOR('',#106030,1000.);
#25055=VECTOR('',#106037,1000.);
#25056=VECTOR('',#106044,1000.);
#25057=VECTOR('',#106051,1000.);
#25058=VECTOR('',#106058,1000.);
#25059=VECTOR('',#106061,1000.);
#25060=VECTOR('',#106068,1000.);
#25061=VECTOR('',#106075,1000.);
#25062=VECTOR('',#106086,1000.);
#25063=VECTOR('',#106089,1000.);
#25064=VECTOR('',#106092,1000.);
#25065=VECTOR('',#106099,1000.);
#25066=VECTOR('',#106102,1000.);
#25067=VECTOR('',#106105,1000.);
#25068=VECTOR('',#106110,1000.);
#25069=VECTOR('',#106113,1000.);
#25070=VECTOR('',#106114,1000.);
#25071=VECTOR('',#106115,1000.);
#25072=VECTOR('',#106118,1000.);
#25073=VECTOR('',#106143,1000.);
#25074=VECTOR('',#106146,1000.);
#25075=VECTOR('',#106149,1000.);
#25076=VECTOR('',#106150,1000.);
#25077=VECTOR('',#106153,1000.);
#25078=VECTOR('',#106158,1000.);
#25079=VECTOR('',#106161,1000.);
#25080=VECTOR('',#106172,1000.);
#25081=VECTOR('',#106175,1000.);
#25082=VECTOR('',#106186,1000.);
#25083=VECTOR('',#106189,1000.);
#25084=VECTOR('',#106204,1000.);
#25085=VECTOR('',#106207,1000.);
#25086=VECTOR('',#106218,1000.);
#25087=VECTOR('',#106221,1000.);
#25088=VECTOR('',#106232,1000.);
#25089=VECTOR('',#106235,1000.);
#25090=VECTOR('',#106248,1000.);
#25091=VECTOR('',#106249,1000.);
#25092=VECTOR('',#106256,1000.);
#25093=VECTOR('',#106259,1000.);
#25094=VECTOR('',#106270,1000.);
#25095=VECTOR('',#106273,1000.);
#25096=VECTOR('',#106284,1000.);
#25097=VECTOR('',#106287,1000.);
#25098=VECTOR('',#106290,1000.);
#25099=VECTOR('',#106293,1000.);
#25100=VECTOR('',#106300,1000.);
#25101=VECTOR('',#106303,1000.);
#25102=VECTOR('',#106314,1000.);
#25103=VECTOR('',#106317,1000.);
#25104=VECTOR('',#106328,1000.);
#25105=VECTOR('',#106331,1000.);
#25106=VECTOR('',#106334,1000.);
#25107=VECTOR('',#106337,1000.);
#25108=VECTOR('',#106344,1000.);
#25109=VECTOR('',#106345,1000.);
#25110=VECTOR('',#106348,1000.);
#25111=VECTOR('',#106349,1000.);
#25112=VECTOR('',#106350,1000.);
#25113=VECTOR('',#106351,1000.);
#25114=VECTOR('',#106352,1000.);
#25115=VECTOR('',#106353,1000.);
#25116=VECTOR('',#106358,1000.);
#25117=VECTOR('',#106373,1000.);
#25118=VECTOR('',#106374,1000.);
#25119=VECTOR('',#106377,1000.);
#25120=VECTOR('',#106380,1000.);
#25121=VECTOR('',#106393,1000.);
#25122=VECTOR('',#106394,1000.);
#25123=VECTOR('',#106423,1000.);
#25124=VECTOR('',#106424,1000.);
#25125=VECTOR('',#106453,1000.);
#25126=VECTOR('',#106454,1000.);
#25127=VECTOR('',#106483,1000.);
#25128=VECTOR('',#106484,1000.);
#25129=VECTOR('',#106497,2.75);
#25130=VECTOR('',#106508,2.75);
#25131=VECTOR('',#106519,1000.);
#25132=VECTOR('',#106522,1000.);
#25133=VECTOR('',#106537,1000.);
#25134=VECTOR('',#106540,1000.);
#25135=VECTOR('',#106555,1000.);
#25136=VECTOR('',#106558,1000.);
#25137=VECTOR('',#106573,1000.);
#25138=VECTOR('',#106576,1000.);
#25139=VECTOR('',#106589,1000.);
#25140=VECTOR('',#106592,1000.);
#25141=VECTOR('',#106607,1000.);
#25142=VECTOR('',#106610,1000.);
#25143=VECTOR('',#106615,1000.);
#25144=VECTOR('',#106616,1000.);
#25145=VECTOR('',#106617,1000.);
#25146=VECTOR('',#106632,1000.);
#25147=VECTOR('',#106635,1000.);
#25148=VECTOR('',#106644,1000.);
#25149=VECTOR('',#106657,1000.);
#25150=VECTOR('',#106660,1000.);
#25151=VECTOR('',#106671,1000.);
#25152=VECTOR('',#106672,1000.);
#25153=VECTOR('',#106683,1000.);
#25154=VECTOR('',#106686,1000.);
#25155=VECTOR('',#106689,1000.);
#25156=VECTOR('',#106692,1000.);
#25157=VECTOR('',#106695,1000.);
#25158=VECTOR('',#106700,1000.);
#25159=VECTOR('',#106701,1000.);
#25160=VECTOR('',#106704,1000.);
#25161=VECTOR('',#106713,1000.);
#25162=VECTOR('',#106716,1000.);
#25163=VECTOR('',#106719,1000.);
#25164=VECTOR('',#106730,1000.);
#25165=VECTOR('',#106733,1000.);
#25166=VECTOR('',#106736,1000.);
#25167=VECTOR('',#106739,1000.);
#25168=VECTOR('',#106756,1000.);
#25169=VECTOR('',#106759,1000.);
#25170=VECTOR('',#106762,1000.);
#25171=VECTOR('',#106767,1000.);
#25172=VECTOR('',#106772,1000.);
#25173=VECTOR('',#106773,1000.);
#25174=VECTOR('',#106776,1000.);
#25175=VECTOR('',#106783,1000.);
#25176=VECTOR('',#106786,1000.);
#25177=VECTOR('',#106799,1000.);
#25178=VECTOR('',#106814,1000.);
#25179=VECTOR('',#106823,1000.);
#25180=VECTOR('',#106830,1000.);
#25181=VECTOR('',#106833,1000.);
#25182=VECTOR('',#106836,1000.);
#25183=VECTOR('',#106839,1000.);
#25184=VECTOR('',#106840,1000.);
#25185=VECTOR('',#106843,1000.);
#25186=VECTOR('',#106848,1000.);
#25187=VECTOR('',#106851,1000.);
#25188=VECTOR('',#106854,1000.);
#25189=VECTOR('',#106855,1000.);
#25190=VECTOR('',#106858,1000.);
#25191=VECTOR('',#106863,1000.);
#25192=VECTOR('',#106866,1000.);
#25193=VECTOR('',#106871,1000.);
#25194=VECTOR('',#106874,1000.);
#25195=VECTOR('',#106885,1000.);
#25196=VECTOR('',#106888,1000.);
#25197=VECTOR('',#106891,1000.);
#25198=VECTOR('',#106892,1000.);
#25199=VECTOR('',#106895,1000.);
#25200=VECTOR('',#106898,1000.);
#25201=VECTOR('',#106903,1000.);
#25202=VECTOR('',#106904,1000.);
#25203=VECTOR('',#106907,1000.);
#25204=VECTOR('',#106916,1000.);
#25205=VECTOR('',#106919,1000.);
#25206=VECTOR('',#106922,1000.);
#25207=VECTOR('',#106933,1000.);
#25208=VECTOR('',#106934,1000.);
#25209=VECTOR('',#106937,1000.);
#25210=VECTOR('',#106948,1000.);
#25211=VECTOR('',#106949,1000.);
#25212=VECTOR('',#106952,1000.);
#25213=VECTOR('',#106961,1000.);
#25214=VECTOR('',#106962,1000.);
#25215=VECTOR('',#106967,1000.);
#25216=VECTOR('',#106984,1000.);
#25217=VECTOR('',#106989,1000.);
#25218=VECTOR('',#106990,1000.);
#25219=VECTOR('',#106999,1000.);
#25220=VECTOR('',#107000,1000.);
#25221=VECTOR('',#107003,1000.);
#25222=VECTOR('',#107014,1000.);
#25223=VECTOR('',#107017,1000.);
#25224=VECTOR('',#107018,1000.);
#25225=VECTOR('',#107027,1000.);
#25226=VECTOR('',#107030,1000.);
#25227=VECTOR('',#107033,1000.);
#25228=VECTOR('',#107036,1000.);
#25229=VECTOR('',#107039,1000.);
#25230=VECTOR('',#107044,1000.);
#25231=VECTOR('',#107045,1000.);
#25232=VECTOR('',#107048,1000.);
#25233=VECTOR('',#107057,1000.);
#25234=VECTOR('',#107060,1000.);
#25235=VECTOR('',#107061,1000.);
#25236=VECTOR('',#107064,1000.);
#25237=VECTOR('',#107077,1000.);
#25238=VECTOR('',#107080,1000.);
#25239=VECTOR('',#107083,1000.);
#25240=VECTOR('',#107084,1000.);
#25241=VECTOR('',#107089,1000.);
#25242=VECTOR('',#107090,1000.);
#25243=VECTOR('',#107097,1000.);
#25244=VECTOR('',#107098,1000.);
#25245=VECTOR('',#107099,1000.);
#25246=VECTOR('',#107100,1000.);
#25247=VECTOR('',#107103,1000.);
#25248=VECTOR('',#107106,1000.);
#25249=VECTOR('',#107107,1000.);
#25250=VECTOR('',#107110,1000.);
#25251=VECTOR('',#107115,1000.);
#25252=VECTOR('',#107116,1000.);
#25253=VECTOR('',#107119,1000.);
#25254=VECTOR('',#107124,1000.);
#25255=VECTOR('',#107125,1000.);
#25256=VECTOR('',#107126,1000.);
#25257=VECTOR('',#107129,1000.);
#25258=VECTOR('',#107132,1000.);
#25259=VECTOR('',#107133,1000.);
#25260=VECTOR('',#107134,1000.);
#25261=VECTOR('',#107135,1000.);
#25262=VECTOR('',#107142,1000.);
#25263=VECTOR('',#107145,1000.);
#25264=VECTOR('',#107150,1000.);
#25265=VECTOR('',#107151,1000.);
#25266=VECTOR('',#107162,1000.);
#25267=VECTOR('',#107167,1000.);
#25268=VECTOR('',#107170,1000.);
#25269=VECTOR('',#107173,1000.);
#25270=VECTOR('',#107174,1000.);
#25271=VECTOR('',#107175,1000.);
#25272=VECTOR('',#107176,1000.);
#25273=VECTOR('',#107177,1000.);
#25274=VECTOR('',#107180,1000.);
#25275=VECTOR('',#107185,1000.);
#25276=VECTOR('',#107186,1000.);
#25277=VECTOR('',#107189,1000.);
#25278=VECTOR('',#107194,1000.);
#25279=VECTOR('',#107197,1000.);
#25280=VECTOR('',#107200,1000.);
#25281=VECTOR('',#107201,1000.);
#25282=VECTOR('',#107202,1000.);
#25283=VECTOR('',#107203,1000.);
#25284=VECTOR('',#107208,1000.);
#25285=VECTOR('',#107209,1000.);
#25286=VECTOR('',#107216,1000.);
#25287=VECTOR('',#107219,1000.);
#25288=VECTOR('',#107222,1000.);
#25289=VECTOR('',#107223,1000.);
#25290=VECTOR('',#107226,1000.);
#25291=VECTOR('',#107231,1000.);
#25292=VECTOR('',#107232,1000.);
#25293=VECTOR('',#107235,1000.);
#25294=VECTOR('',#107240,1000.);
#25295=VECTOR('',#107243,1000.);
#25296=VECTOR('',#107252,1000.);
#25297=VECTOR('',#107253,1000.);
#25298=VECTOR('',#107254,1000.);
#25299=VECTOR('',#107257,1000.);
#25300=VECTOR('',#107258,1000.);
#25301=VECTOR('',#107261,1000.);
#25302=VECTOR('',#107266,1000.);
#25303=VECTOR('',#107267,1000.);
#25304=VECTOR('',#107270,1000.);
#25305=VECTOR('',#107275,1000.);
#25306=VECTOR('',#107278,1000.);
#25307=VECTOR('',#107279,1000.);
#25308=VECTOR('',#107286,1000.);
#25309=VECTOR('',#107287,1000.);
#25310=VECTOR('',#107294,1000.);
#25311=VECTOR('',#107295,1000.);
#25312=VECTOR('',#107296,1000.);
#25313=VECTOR('',#107297,1000.);
#25314=VECTOR('',#107300,1000.);
#25315=VECTOR('',#107303,1000.);
#25316=VECTOR('',#107304,1000.);
#25317=VECTOR('',#107307,1000.);
#25318=VECTOR('',#107312,1000.);
#25319=VECTOR('',#107313,1000.);
#25320=VECTOR('',#107316,1000.);
#25321=VECTOR('',#107323,1000.);
#25322=VECTOR('',#107324,1000.);
#25323=VECTOR('',#107325,1000.);
#25324=VECTOR('',#107326,1000.);
#25325=VECTOR('',#107327,1000.);
#25326=VECTOR('',#107330,1000.);
#25327=VECTOR('',#107333,1000.);
#25328=VECTOR('',#107334,1000.);
#25329=VECTOR('',#107335,1000.);
#25330=VECTOR('',#107340,1000.);
#25331=VECTOR('',#107343,1000.);
#25332=VECTOR('',#107352,1000.);
#25333=VECTOR('',#107353,1000.);
#25334=VECTOR('',#107366,1000.);
#25335=VECTOR('',#107371,1000.);
#25336=VECTOR('',#107374,1000.);
#25337=VECTOR('',#107377,1000.);
#25338=VECTOR('',#107378,1000.);
#25339=VECTOR('',#107379,1000.);
#25340=VECTOR('',#107380,1000.);
#25341=VECTOR('',#107381,1000.);
#25342=VECTOR('',#107384,1000.);
#25343=VECTOR('',#107389,1000.);
#25344=VECTOR('',#107390,1000.);
#25345=VECTOR('',#107393,1000.);
#25346=VECTOR('',#107398,1000.);
#25347=VECTOR('',#107401,1000.);
#25348=VECTOR('',#107404,1000.);
#25349=VECTOR('',#107405,1000.);
#25350=VECTOR('',#107406,1000.);
#25351=VECTOR('',#107407,1000.);
#25352=VECTOR('',#107420,1000.);
#25353=VECTOR('',#107425,1000.);
#25354=VECTOR('',#107428,1000.);
#25355=VECTOR('',#107429,1000.);
#25356=VECTOR('',#107434,1000.);
#25357=VECTOR('',#107435,1000.);
#25358=VECTOR('',#107436,1000.);
#25359=VECTOR('',#107437,1000.);
#25360=VECTOR('',#107438,1000.);
#25361=VECTOR('',#107439,1000.);
#25362=VECTOR('',#107442,1000.);
#25363=VECTOR('',#107445,1000.);
#25364=VECTOR('',#107446,1000.);
#25365=VECTOR('',#107449,1000.);
#25366=VECTOR('',#107454,1000.);
#25367=VECTOR('',#107455,1000.);
#25368=VECTOR('',#107458,1000.);
#25369=VECTOR('',#107463,1000.);
#25370=VECTOR('',#107466,1000.);
#25371=VECTOR('',#107469,1000.);
#25372=VECTOR('',#107470,1000.);
#25373=VECTOR('',#107471,1000.);
#25374=VECTOR('',#107472,1000.);
#25375=VECTOR('',#107479,1000.);
#25376=VECTOR('',#107480,1000.);
#25377=VECTOR('',#107485,1000.);
#25378=VECTOR('',#107488,1000.);
#25379=VECTOR('',#107491,1000.);
#25380=VECTOR('',#107492,1000.);
#25381=VECTOR('',#107493,1000.);
#25382=VECTOR('',#107494,1000.);
#25383=VECTOR('',#107495,1000.);
#25384=VECTOR('',#107498,1000.);
#25385=VECTOR('',#107503,1000.);
#25386=VECTOR('',#107504,1000.);
#25387=VECTOR('',#107507,1000.);
#25388=VECTOR('',#107514,1000.);
#25389=VECTOR('',#107517,1000.);
#25390=VECTOR('',#107520,1000.);
#25391=VECTOR('',#107521,1000.);
#25392=VECTOR('',#107522,1000.);
#25393=VECTOR('',#107523,1000.);
#25394=VECTOR('',#107526,1000.);
#25395=VECTOR('',#107535,2.);
#25396=VECTOR('',#107544,2.75);
#25397=VECTOR('',#107575,2.);
#25398=VECTOR('',#107584,2.75);
#25399=VECTOR('',#107595,1000.);
#25400=VECTOR('',#107604,1000.);
#25401=VECTOR('',#107609,1000.);
#25402=VECTOR('',#107610,1000.);
#25403=VECTOR('',#107629,1000.);
#25404=VECTOR('',#107632,1000.);
#25405=VECTOR('',#107641,1000.);
#25406=VECTOR('',#107644,1000.);
#25407=VECTOR('',#107657,1000.);
#25408=VECTOR('',#107662,1000.);
#25409=VECTOR('',#107667,1000.);
#25410=VECTOR('',#107668,1000.);
#25411=VECTOR('',#107677,1000.);
#25412=VECTOR('',#107678,1000.);
#25413=VECTOR('',#107683,1000.);
#25414=VECTOR('',#107688,1000.);
#25415=VECTOR('',#107689,1000.);
#25416=VECTOR('',#107698,1000.);
#25417=VECTOR('',#107699,1000.);
#25418=VECTOR('',#107712,1000.);
#25419=VECTOR('',#107719,1000.);
#25420=VECTOR('',#107726,1000.);
#25421=VECTOR('',#107729,1000.);
#25422=VECTOR('',#107730,1000.);
#25423=VECTOR('',#107733,1000.);
#25424=VECTOR('',#107738,1000.);
#25425=VECTOR('',#107743,1000.);
#25426=VECTOR('',#107748,1000.);
#25427=VECTOR('',#107749,1000.);
#25428=VECTOR('',#107750,1000.);
#25429=VECTOR('',#107751,1000.);
#25430=VECTOR('',#107752,1000.);
#25431=VECTOR('',#107753,1000.);
#25432=VECTOR('',#107754,1000.);
#25433=VECTOR('',#107755,1000.);
#25434=VECTOR('',#107756,1000.);
#25435=VECTOR('',#107757,1000.);
#25436=VECTOR('',#107760,1000.);
#25437=VECTOR('',#107761,1000.);
#25438=VECTOR('',#107764,1000.);
#25439=VECTOR('',#107769,1000.);
#25440=VECTOR('',#107772,1000.);
#25441=VECTOR('',#107777,1000.);
#25442=VECTOR('',#107780,1000.);
#25443=VECTOR('',#107783,1000.);
#25444=VECTOR('',#107786,1000.);
#25445=VECTOR('',#107789,1000.);
#25446=VECTOR('',#107792,1000.);
#25447=VECTOR('',#107795,1000.);
#25448=VECTOR('',#107798,1000.);
#25449=VECTOR('',#107801,1000.);
#25450=VECTOR('',#107804,1000.);
#25451=VECTOR('',#107809,1000.);
#25452=VECTOR('',#107810,1000.);
#25453=VECTOR('',#107813,1000.);
#25454=VECTOR('',#107814,1000.);
#25455=VECTOR('',#107815,1000.);
#25456=VECTOR('',#107816,1000.);
#25457=VECTOR('',#107817,1000.);
#25458=VECTOR('',#107818,1000.);
#25459=VECTOR('',#107819,1000.);
#25460=VECTOR('',#107820,1000.);
#25461=VECTOR('',#107821,1000.);
#25462=VECTOR('',#107822,1000.);
#25463=VECTOR('',#107825,1000.);
#25464=VECTOR('',#107830,1000.);
#25465=VECTOR('',#107835,1000.);
#25466=VECTOR('',#107840,1000.);
#25467=VECTOR('',#107841,1000.);
#25468=VECTOR('',#107842,1000.);
#25469=VECTOR('',#107843,1000.);
#25470=VECTOR('',#107844,1000.);
#25471=VECTOR('',#107845,1000.);
#25472=VECTOR('',#107846,1000.);
#25473=VECTOR('',#107847,1000.);
#25474=VECTOR('',#107848,1000.);
#25475=VECTOR('',#107855,1000.);
#25476=VECTOR('',#107862,1000.);
#25477=VECTOR('',#107863,1000.);
#25478=VECTOR('',#107864,1000.);
#25479=VECTOR('',#107871,1000.);
#25480=VECTOR('',#107874,1000.);
#25481=VECTOR('',#107881,1000.);
#25482=VECTOR('',#107888,1000.);
#25483=VECTOR('',#107889,1000.);
#25484=VECTOR('',#107892,1000.);
#25485=VECTOR('',#107897,1000.);
#25486=VECTOR('',#107906,1000.);
#25487=VECTOR('',#107911,1000.);
#25488=VECTOR('',#107912,1000.);
#25489=VECTOR('',#107943,1000.);
#25490=VECTOR('',#107948,1000.);
#25491=VECTOR('',#107961,1000.);
#25492=VECTOR('',#107972,1000.);
#25493=VECTOR('',#107977,1000.);
#25494=VECTOR('',#107980,1000.);
#25495=VECTOR('',#107993,1000.);
#25496=VECTOR('',#108002,1000.);
#25497=VECTOR('',#108015,1000.);
#25498=VECTOR('',#108024,1000.);
#25499=VECTOR('',#108039,1000.);
#25500=VECTOR('',#108044,1000.);
#25501=VECTOR('',#108057,1000.);
#25502=VECTOR('',#108070,1000.);
#25503=VECTOR('',#108113,1000.);
#25504=VECTOR('',#108128,1000.);
#25505=VECTOR('',#108135,1000.);
#25506=VECTOR('',#108156,1000.);
#25507=VECTOR('',#108163,1000.);
#25508=VECTOR('',#108176,1000.);
#25509=VECTOR('',#108193,1000.);
#25510=VECTOR('',#108204,1000.);
#25511=VECTOR('',#108213,1000.);
#25512=VECTOR('',#108224,1000.);
#25513=VECTOR('',#108249,1000.);
#25514=VECTOR('',#108258,1000.);
#25515=VECTOR('',#108275,1000.);
#25516=VECTOR('',#108278,1000.);
#25517=VECTOR('',#108303,1000.);
#25518=VECTOR('',#108314,1000.);
#25519=VECTOR('',#108333,1000.);
#25520=VECTOR('',#108336,1000.);
#25521=VECTOR('',#108365,1000.);
#25522=VECTOR('',#108376,1000.);
#25523=VECTOR('',#108393,1000.);
#25524=VECTOR('',#108396,1000.);
#25525=VECTOR('',#108421,1000.);
#25526=VECTOR('',#108430,1000.);
#25527=VECTOR('',#108455,1000.);
#25528=VECTOR('',#108464,1000.);
#25529=VECTOR('',#108475,1000.);
#25530=VECTOR('',#108484,1000.);
#25531=VECTOR('',#108503,1000.);
#25532=VECTOR('',#108520,1000.);
#25533=VECTOR('',#108529,1000.);
#25534=VECTOR('',#108536,1000.);
#25535=VECTOR('',#108567,1000.);
#25536=VECTOR('',#108578,1000.);
#25537=VECTOR('',#108591,1000.);
#25538=VECTOR('',#108602,1000.);
#25539=VECTOR('',#108605,1000.);
#25540=VECTOR('',#108626,1000.);
#25541=VECTOR('',#108633,1000.);
#25542=VECTOR('',#108642,1000.);
#25543=VECTOR('',#108669,1000.);
#25544=VECTOR('',#108676,1000.);
#25545=VECTOR('',#108697,1000.);
#25546=VECTOR('',#108708,1000.);
#25547=VECTOR('',#108719,1000.);
#25548=VECTOR('',#108730,1000.);
#25549=VECTOR('',#108739,1000.);
#25550=VECTOR('',#108746,1000.);
#25551=VECTOR('',#108761,1000.);
#25552=VECTOR('',#108772,1000.);
#25553=VECTOR('',#108781,1000.);
#25554=VECTOR('',#108824,1000.);
#25555=VECTOR('',#108873,1000.);
#25556=VECTOR('',#108884,1000.);
#25557=VECTOR('',#108899,1000.);
#25558=VECTOR('',#108908,1000.);
#25559=VECTOR('',#108911,1000.);
#25560=VECTOR('',#108920,1000.);
#25561=VECTOR('',#108925,1000.);
#25562=VECTOR('',#108934,1000.);
#25563=VECTOR('',#108951,1000.);
#25564=VECTOR('',#108974,1000.);
#25565=VECTOR('',#108985,1000.);
#25566=VECTOR('',#109006,1000.);
#25567=VECTOR('',#109017,1000.);
#25568=VECTOR('',#109028,1000.);
#25569=VECTOR('',#109039,1000.);
#25570=VECTOR('',#109048,1000.);
#25571=VECTOR('',#109055,1000.);
#25572=VECTOR('',#109070,1000.);
#25573=VECTOR('',#109081,1000.);
#25574=VECTOR('',#109090,1000.);
#25575=VECTOR('',#109115,1000.);
#25576=VECTOR('',#109126,1000.);
#25577=VECTOR('',#109135,1000.);
#25578=VECTOR('',#109154,1000.);
#25579=VECTOR('',#109165,1000.);
#25580=VECTOR('',#109176,1000.);
#25581=VECTOR('',#109187,1000.);
#25582=VECTOR('',#109194,1000.);
#25583=VECTOR('',#109211,1000.);
#25584=VECTOR('',#109222,1000.);
#25585=VECTOR('',#109235,1000.);
#25586=VECTOR('',#109258,1000.);
#25587=VECTOR('',#109269,1000.);
#25588=VECTOR('',#109280,1000.);
#25589=VECTOR('',#109291,1000.);
#25590=VECTOR('',#109300,1000.);
#25591=VECTOR('',#109309,1000.);
#25592=VECTOR('',#109326,1000.);
#25593=VECTOR('',#109337,1000.);
#25594=VECTOR('',#109344,1000.);
#25595=VECTOR('',#109357,1000.);
#25596=VECTOR('',#109384,1000.);
#25597=VECTOR('',#109387,1000.);
#25598=VECTOR('',#109394,1000.);
#25599=VECTOR('',#109399,1000.);
#25600=VECTOR('',#109488,1000.);
#25601=VECTOR('',#109495,1000.);
#25602=VECTOR('',#109504,1000.);
#25603=VECTOR('',#109511,1000.);
#25604=VECTOR('',#109532,1000.);
#25605=VECTOR('',#109535,1000.);
#25606=VECTOR('',#109542,1000.);
#25607=VECTOR('',#109547,1000.);
#25608=VECTOR('',#109550,1000.);
#25609=VECTOR('',#109569,1000.);
#25610=VECTOR('',#109572,1000.);
#25611=VECTOR('',#109575,1000.);
#25612=VECTOR('',#109584,1000.);
#25613=VECTOR('',#109585,1000.);
#25614=VECTOR('',#109588,1000.);
#25615=VECTOR('',#109611,1000.);
#25616=VECTOR('',#109614,1000.);
#25617=VECTOR('',#109615,1000.);
#25618=VECTOR('',#109626,1000.);
#25619=VECTOR('',#109633,1000.);
#25620=VECTOR('',#109636,1000.);
#25621=VECTOR('',#109661,1000.);
#25622=VECTOR('',#109664,1000.);
#25623=VECTOR('',#109675,1000.);
#25624=VECTOR('',#109678,1000.);
#25625=VECTOR('',#109707,1000.);
#25626=VECTOR('',#109710,1000.);
#25627=VECTOR('',#109725,1000.);
#25628=VECTOR('',#109728,1000.);
#25629=VECTOR('',#109747,1000.);
#25630=VECTOR('',#109750,1000.);
#25631=VECTOR('',#109759,1000.);
#25632=VECTOR('',#109760,1000.);
#25633=VECTOR('',#109763,1000.);
#25634=VECTOR('',#109764,1000.);
#25635=VECTOR('',#109765,1000.);
#25636=VECTOR('',#109766,1000.);
#25637=VECTOR('',#109771,1000.);
#25638=VECTOR('',#109776,1000.);
#25639=VECTOR('',#109777,1000.);
#25640=VECTOR('',#109778,1000.);
#25641=VECTOR('',#109785,1000.);
#25642=VECTOR('',#109786,1000.);
#25643=VECTOR('',#109797,1000.);
#25644=VECTOR('',#109798,1000.);
#25645=VECTOR('',#109799,1000.);
#25646=VECTOR('',#109802,1000.);
#25647=VECTOR('',#109803,1000.);
#25648=VECTOR('',#109804,1000.);
#25649=VECTOR('',#109805,1000.);
#25650=VECTOR('',#109810,1000.);
#25651=VECTOR('',#109815,1000.);
#25652=VECTOR('',#109816,1000.);
#25653=VECTOR('',#109817,1000.);
#25654=VECTOR('',#109828,1000.);
#25655=VECTOR('',#109829,1000.);
#25656=VECTOR('',#109832,1000.);
#25657=VECTOR('',#109833,1000.);
#25658=VECTOR('',#109834,1000.);
#25659=VECTOR('',#109835,1000.);
#25660=VECTOR('',#109840,1000.);
#25661=VECTOR('',#109845,1000.);
#25662=VECTOR('',#109846,1000.);
#25663=VECTOR('',#109847,1000.);
#25664=VECTOR('',#109850,1000.);
#25665=VECTOR('',#109851,1000.);
#25666=VECTOR('',#109856,1000.);
#25667=VECTOR('',#109857,1000.);
#25668=VECTOR('',#109868,1000.);
#25669=VECTOR('',#109869,1000.);
#25670=VECTOR('',#109872,1000.);
#25671=VECTOR('',#109881,1000.);
#25672=VECTOR('',#109882,1000.);
#25673=VECTOR('',#109885,1000.);
#25674=VECTOR('',#109886,1000.);
#25675=VECTOR('',#109887,1000.);
#25676=VECTOR('',#109888,1000.);
#25677=VECTOR('',#109891,1000.);
#25678=VECTOR('',#109898,1000.);
#25679=VECTOR('',#109899,1000.);
#25680=VECTOR('',#109900,1000.);
#25681=VECTOR('',#109915,1000.);
#25682=VECTOR('',#109916,1000.);
#25683=VECTOR('',#109917,1000.);
#25684=VECTOR('',#109918,1000.);
#25685=VECTOR('',#109923,1000.);
#25686=VECTOR('',#109928,1000.);
#25687=VECTOR('',#109929,1000.);
#25688=VECTOR('',#109930,1000.);
#25689=VECTOR('',#109933,1000.);
#25690=VECTOR('',#109934,1000.);
#25691=VECTOR('',#109939,1000.);
#25692=VECTOR('',#109940,1000.);
#25693=VECTOR('',#109955,1000.);
#25694=VECTOR('',#109956,1000.);
#25695=VECTOR('',#109959,1000.);
#25696=VECTOR('',#109970,1000.);
#25697=VECTOR('',#109971,1000.);
#25698=VECTOR('',#109974,1000.);
#25699=VECTOR('',#109975,1000.);
#25700=VECTOR('',#109976,1000.);
#25701=VECTOR('',#109977,1000.);
#25702=VECTOR('',#109980,1000.);
#25703=VECTOR('',#109987,1000.);
#25704=VECTOR('',#109988,1000.);
#25705=VECTOR('',#109989,1000.);
#25706=VECTOR('',#109996,1000.);
#25707=VECTOR('',#109999,1000.);
#25708=VECTOR('',#110004,1000.);
#25709=VECTOR('',#110007,1000.);
#25710=VECTOR('',#110010,1000.);
#25711=VECTOR('',#110011,1000.);
#25712=VECTOR('',#110018,1000.);
#25713=VECTOR('',#110021,1000.);
#25714=VECTOR('',#110022,1000.);
#25715=VECTOR('',#110025,1000.);
#25716=VECTOR('',#110026,1000.);
#25717=VECTOR('',#110027,1000.);
#25718=VECTOR('',#110028,1000.);
#25719=VECTOR('',#110041,1000.);
#25720=VECTOR('',#110042,1000.);
#25721=VECTOR('',#110051,1000.);
#25722=VECTOR('',#110052,1000.);
#25723=VECTOR('',#110065,1000.);
#25724=VECTOR('',#110066,1000.);
#25725=VECTOR('',#110077,1000.);
#25726=VECTOR('',#110078,1000.);
#25727=VECTOR('',#110085,1000.);
#25728=VECTOR('',#110090,1000.);
#25729=VECTOR('',#110091,1000.);
#25730=VECTOR('',#110092,1000.);
#25731=VECTOR('',#110093,1000.);
#25732=VECTOR('',#110098,1000.);
#25733=VECTOR('',#110103,1000.);
#25734=VECTOR('',#110108,1000.);
#25735=VECTOR('',#110111,1000.);
#25736=VECTOR('',#110116,1000.);
#25737=VECTOR('',#110117,1000.);
#25738=VECTOR('',#110124,1000.);
#25739=VECTOR('',#110127,1000.);
#25740=VECTOR('',#110130,1000.);
#25741=VECTOR('',#110131,1000.);
#25742=VECTOR('',#110132,1000.);
#25743=VECTOR('',#110135,1000.);
#25744=VECTOR('',#110136,1000.);
#25745=VECTOR('',#110137,1000.);
#25746=VECTOR('',#110140,1000.);
#25747=VECTOR('',#110141,1000.);
#25748=VECTOR('',#110144,1000.);
#25749=VECTOR('',#110145,1000.);
#25750=VECTOR('',#110146,1000.);
#25751=VECTOR('',#110147,1000.);
#25752=VECTOR('',#110150,1000.);
#25753=VECTOR('',#110151,1000.);
#25754=VECTOR('',#110154,1000.);
#25755=VECTOR('',#110155,1000.);
#25756=VECTOR('',#110158,1000.);
#25757=VECTOR('',#110161,1000.);
#25758=VECTOR('',#110174,1000.);
#25759=VECTOR('',#110191,1000.);
#25760=VECTOR('',#110198,1000.);
#25761=VECTOR('',#110205,1000.);
#25762=VECTOR('',#110212,1000.);
#25763=VECTOR('',#110219,1000.);
#25764=VECTOR('',#110220,1000.);
#25765=VECTOR('',#110253,1000.);
#25766=VECTOR('',#110260,1000.);
#25767=VECTOR('',#110267,1000.);
#25768=VECTOR('',#110268,1000.);
#25769=VECTOR('',#110275,1000.);
#25770=VECTOR('',#110282,1000.);
#25771=VECTOR('',#110429,1000.);
#25772=VECTOR('',#110436,1000.);
#25773=VECTOR('',#110443,1000.);
#25774=VECTOR('',#110450,1000.);
#25775=VECTOR('',#110457,1000.);
#25776=VECTOR('',#110458,1000.);
#25777=VECTOR('',#110487,1000.);
#25778=VECTOR('',#110488,1000.);
#25779=VECTOR('',#110499,1000.);
#25780=VECTOR('',#110500,1000.);
#25781=VECTOR('',#110501,1000.);
#25782=VECTOR('',#110504,1000.);
#25783=VECTOR('',#110505,1000.);
#25784=VECTOR('',#110512,1000.);
#25785=VECTOR('',#110513,1000.);
#25786=VECTOR('',#110524,1000.);
#25787=VECTOR('',#110537,1000.);
#25788=VECTOR('',#110548,1000.);
#25789=VECTOR('',#110555,1000.);
#25790=VECTOR('',#110556,1000.);
#25791=VECTOR('',#110559,1000.);
#25792=VECTOR('',#110564,1000.);
#25793=VECTOR('',#110567,1000.);
#25794=VECTOR('',#110578,1000.);
#25795=VECTOR('',#110591,1000.);
#25796=VECTOR('',#110602,1000.);
#25797=VECTOR('',#110605,1000.);
#25798=VECTOR('',#110608,1000.);
#25799=VECTOR('',#110613,1000.);
#25800=VECTOR('',#110624,1000.);
#25801=VECTOR('',#110635,1000.);
#25802=VECTOR('',#110638,1000.);
#25803=VECTOR('',#110653,1000.);
#25804=VECTOR('',#110660,1000.);
#25805=VECTOR('',#110663,1000.);
#25806=VECTOR('',#110672,1000.);
#25807=VECTOR('',#110685,1000.);
#25808=VECTOR('',#110692,1000.);
#25809=VECTOR('',#110693,1000.);
#25810=VECTOR('',#110696,1000.);
#25811=VECTOR('',#110707,1000.);
#25812=VECTOR('',#110714,1000.);
#25813=VECTOR('',#110717,1000.);
#25814=VECTOR('',#110720,1000.);
#25815=VECTOR('',#110723,1000.);
#25816=VECTOR('',#110726,1000.);
#25817=VECTOR('',#110743,1000.);
#25818=VECTOR('',#110752,1000.);
#25819=VECTOR('',#110757,1000.);
#25820=VECTOR('',#110758,1000.);
#25821=VECTOR('',#110771,1000.);
#25822=VECTOR('',#110780,1000.);
#25823=VECTOR('',#110791,1000.);
#25824=VECTOR('',#110796,1000.);
#25825=VECTOR('',#110797,1000.);
#25826=VECTOR('',#110818,1000.);
#25827=VECTOR('',#110833,1000.);
#25828=VECTOR('',#110844,1000.);
#25829=VECTOR('',#110849,1000.);
#25830=VECTOR('',#110850,1000.);
#25831=VECTOR('',#110853,1000.);
#25832=VECTOR('',#110864,1000.);
#25833=VECTOR('',#110877,1000.);
#25834=VECTOR('',#110888,1000.);
#25835=VECTOR('',#110891,1000.);
#25836=VECTOR('',#110894,1000.);
#25837=VECTOR('',#110899,1000.);
#25838=VECTOR('',#110910,1000.);
#25839=VECTOR('',#110921,1000.);
#25840=VECTOR('',#110924,1000.);
#25841=VECTOR('',#110939,1000.);
#25842=VECTOR('',#110960,1000.);
#25843=VECTOR('',#110973,1000.);
#25844=VECTOR('',#110974,1000.);
#25845=VECTOR('',#110977,1000.);
#25846=VECTOR('',#110980,1000.);
#25847=VECTOR('',#110981,1000.);
#25848=VECTOR('',#110988,1000.);
#25849=VECTOR('',#110991,1000.);
#25850=VECTOR('',#110996,1000.);
#25851=VECTOR('',#110997,1000.);
#25852=VECTOR('',#111000,1000.);
#25853=VECTOR('',#111011,1000.);
#25854=VECTOR('',#111020,1000.);
#25855=VECTOR('',#111033,1000.);
#25856=VECTOR('',#111042,1000.);
#25857=VECTOR('',#111053,1000.);
#25858=VECTOR('',#111070,1000.);
#25859=VECTOR('',#111081,1000.);
#25860=VECTOR('',#111086,1000.);
#25861=VECTOR('',#111087,1000.);
#25862=VECTOR('',#111092,1000.);
#25863=VECTOR('',#111095,1000.);
#25864=VECTOR('',#111100,1000.);
#25865=VECTOR('',#111101,1000.);
#25866=VECTOR('',#111116,1000.);
#25867=VECTOR('',#111119,1000.);
#25868=VECTOR('',#111132,1000.);
#25869=VECTOR('',#111135,1000.);
#25870=VECTOR('',#111146,1000.);
#25871=VECTOR('',#111147,1000.);
#25872=VECTOR('',#111150,1000.);
#25873=VECTOR('',#111161,1000.);
#25874=VECTOR('',#111164,1000.);
#25875=VECTOR('',#111177,1000.);
#25876=VECTOR('',#111178,1000.);
#25877=VECTOR('',#111193,1000.);
#25878=VECTOR('',#111196,1000.);
#25879=VECTOR('',#111207,1000.);
#25880=VECTOR('',#111208,1000.);
#25881=VECTOR('',#111213,1000.);
#25882=VECTOR('',#111214,1000.);
#25883=VECTOR('',#111229,1000.);
#25884=VECTOR('',#111244,1000.);
#25885=VECTOR('',#111255,1000.);
#25886=VECTOR('',#111260,1000.);
#25887=VECTOR('',#111261,1000.);
#25888=VECTOR('',#111264,1000.);
#25889=VECTOR('',#111275,1000.);
#25890=VECTOR('',#111288,1000.);
#25891=VECTOR('',#111299,1000.);
#25892=VECTOR('',#111302,1000.);
#25893=VECTOR('',#111305,1000.);
#25894=VECTOR('',#111310,1000.);
#25895=VECTOR('',#111321,1000.);
#25896=VECTOR('',#111332,1000.);
#25897=VECTOR('',#111335,1000.);
#25898=VECTOR('',#111350,1000.);
#25899=VECTOR('',#111363,1000.);
#25900=VECTOR('',#111380,1000.);
#25901=VECTOR('',#111383,1000.);
#25902=VECTOR('',#111388,1000.);
#25903=VECTOR('',#111389,1000.);
#25904=VECTOR('',#111392,1000.);
#25905=VECTOR('',#111405,1000.);
#25906=VECTOR('',#111412,1000.);
#25907=VECTOR('',#111415,1000.);
#25908=VECTOR('',#111416,1000.);
#25909=VECTOR('',#111421,1000.);
#25910=VECTOR('',#111422,1000.);
#25911=VECTOR('',#111433,1000.);
#25912=VECTOR('',#111442,1000.);
#25913=VECTOR('',#111451,1000.);
#25914=VECTOR('',#111468,1000.);
#25915=VECTOR('',#111479,1000.);
#25916=VECTOR('',#111484,1000.);
#25917=VECTOR('',#111485,1000.);
#25918=VECTOR('',#111496,1000.);
#25919=VECTOR('',#111499,1000.);
#25920=VECTOR('',#111502,1000.);
#25921=VECTOR('',#111505,1000.);
#25922=VECTOR('',#111516,1000.);
#25923=VECTOR('',#111523,1000.);
#25924=VECTOR('',#111534,1000.);
#25925=VECTOR('',#111539,1000.);
#25926=VECTOR('',#111540,1000.);
#25927=VECTOR('',#111553,1000.);
#25928=VECTOR('',#111564,1000.);
#25929=VECTOR('',#111565,1000.);
#25930=VECTOR('',#111568,1000.);
#25931=VECTOR('',#111579,1000.);
#25932=VECTOR('',#111594,1000.);
#25933=VECTOR('',#111607,1000.);
#25934=VECTOR('',#111616,1000.);
#25935=VECTOR('',#111619,1000.);
#25936=VECTOR('',#111630,1000.);
#25937=VECTOR('',#111645,1000.);
#25938=VECTOR('',#111656,1000.);
#25939=VECTOR('',#111657,1000.);
#25940=VECTOR('',#111666,1000.);
#25941=VECTOR('',#111667,1000.);
#25942=VECTOR('',#111670,1000.);
#25943=VECTOR('',#111675,1000.);
#25944=VECTOR('',#111680,1000.);
#25945=VECTOR('',#111683,1000.);
#25946=VECTOR('',#111694,1000.);
#25947=VECTOR('',#111713,1000.);
#25948=VECTOR('',#111726,1000.);
#25949=VECTOR('',#111727,1000.);
#25950=VECTOR('',#111736,1000.);
#25951=VECTOR('',#111737,1000.);
#25952=VECTOR('',#111742,1000.);
#25953=VECTOR('',#111747,1000.);
#25954=VECTOR('',#111752,1000.);
#25955=VECTOR('',#111755,1000.);
#25956=VECTOR('',#111768,1000.);
#25957=VECTOR('',#111787,1000.);
#25958=VECTOR('',#111798,1000.);
#25959=VECTOR('',#111799,1000.);
#25960=VECTOR('',#111806,1000.);
#25961=VECTOR('',#111809,1000.);
#25962=VECTOR('',#111812,1000.);
#25963=VECTOR('',#111817,1000.);
#25964=VECTOR('',#111822,1000.);
#25965=VECTOR('',#111825,1000.);
#25966=VECTOR('',#111836,1000.);
#25967=VECTOR('',#111851,1000.);
#25968=VECTOR('',#111862,1000.);
#25969=VECTOR('',#111863,1000.);
#25970=VECTOR('',#111872,1000.);
#25971=VECTOR('',#111887,1000.);
#25972=VECTOR('',#111900,1000.);
#25973=VECTOR('',#111911,1000.);
#25974=VECTOR('',#111914,1000.);
#25975=VECTOR('',#111917,1000.);
#25976=VECTOR('',#111928,1000.);
#25977=VECTOR('',#111945,1000.);
#25978=VECTOR('',#111956,1000.);
#25979=VECTOR('',#111969,1000.);
#25980=VECTOR('',#111970,1000.);
#25981=VECTOR('',#111973,1000.);
#25982=VECTOR('',#111984,1000.);
#25983=VECTOR('',#112003,1000.);
#25984=VECTOR('',#112036,1000.);
#25985=VECTOR('',#112039,1000.);
#25986=VECTOR('',#112052,1000.);
#25987=VECTOR('',#112053,1000.);
#25988=VECTOR('',#112068,1000.);
#25989=VECTOR('',#112071,1000.);
#25990=VECTOR('',#112100,1000.);
#25991=VECTOR('',#112117,1000.);
#25992=VECTOR('',#112134,1000.);
#25993=VECTOR('',#112145,1000.);
#25994=VECTOR('',#112162,1000.);
#25995=VECTOR('',#112175,1000.);
#25996=VECTOR('',#112192,1000.);
#25997=VECTOR('',#112207,1000.);
#25998=VECTOR('',#112218,1000.);
#25999=VECTOR('',#112221,1000.);
#26000=VECTOR('',#112224,1000.);
#26001=VECTOR('',#112229,1000.);
#26002=VECTOR('',#112240,1000.);
#26003=VECTOR('',#112259,1000.);
#26004=VECTOR('',#112270,1000.);
#26005=VECTOR('',#112273,1000.);
#26006=VECTOR('',#112276,1000.);
#26007=VECTOR('',#112283,1000.);
#26008=VECTOR('',#112284,1000.);
#26009=VECTOR('',#112321,1000.);
#26010=VECTOR('',#112322,1000.);
#26011=VECTOR('',#112327,1000.);
#26012=VECTOR('',#112330,1000.);
#26013=VECTOR('',#112349,1000.);
#26014=VECTOR('',#112354,1000.);
#26015=VECTOR('',#112357,1000.);
#26016=VECTOR('',#112372,1000.);
#26017=VECTOR('',#112373,1000.);
#26018=VECTOR('',#112374,1000.);
#26019=VECTOR('',#112379,1000.);
#26020=VECTOR('',#112384,1000.);
#26021=VECTOR('',#112389,1000.);
#26022=VECTOR('',#112392,1000.);
#26023=VECTOR('',#112393,1000.);
#26024=VECTOR('',#112396,1000.);
#26025=VECTOR('',#112401,1000.);
#26026=VECTOR('',#112408,1000.);
#26027=VECTOR('',#112411,1000.);
#26028=VECTOR('',#112412,1000.);
#26029=VECTOR('',#112417,1000.);
#26030=VECTOR('',#112422,1000.);
#26031=VECTOR('',#112427,1000.);
#26032=VECTOR('',#112430,1000.);
#26033=VECTOR('',#112431,1000.);
#26034=VECTOR('',#112432,1000.);
#26035=VECTOR('',#112433,1000.);
#26036=VECTOR('',#112442,1000.);
#26037=VECTOR('',#112449,1000.);
#26038=VECTOR('',#112454,1000.);
#26039=VECTOR('',#112457,1000.);
#26040=VECTOR('',#112458,1000.);
#26041=VECTOR('',#112469,1000.);
#26042=VECTOR('',#112478,1000.);
#26043=VECTOR('',#112481,1000.);
#26044=VECTOR('',#112484,1000.);
#26045=VECTOR('',#112485,1000.);
#26046=VECTOR('',#112490,1000.);
#26047=VECTOR('',#112499,1000.);
#26048=VECTOR('',#112508,1000.);
#26049=VECTOR('',#112511,1000.);
#26050=VECTOR('',#112514,1000.);
#26051=VECTOR('',#112515,1000.);
#26052=VECTOR('',#112520,1000.);
#26053=VECTOR('',#112531,1000.);
#26054=VECTOR('',#112542,1000.);
#26055=VECTOR('',#112545,1000.);
#26056=VECTOR('',#112550,1000.);
#26057=VECTOR('',#112551,1000.);
#26058=VECTOR('',#112558,1000.);
#26059=VECTOR('',#112571,1000.);
#26060=VECTOR('',#112574,1000.);
#26061=VECTOR('',#112579,1000.);
#26062=VECTOR('',#112580,1000.);
#26063=VECTOR('',#112585,1000.);
#26064=VECTOR('',#112598,1000.);
#26065=VECTOR('',#112599,1000.);
#26066=VECTOR('',#112612,1000.);
#26067=VECTOR('',#112613,1000.);
#26068=VECTOR('',#112618,1000.);
#26069=VECTOR('',#112629,1000.);
#26070=VECTOR('',#112632,1000.);
#26071=VECTOR('',#112635,1000.);
#26072=VECTOR('',#112640,2.75);
#26073=VECTOR('',#112653,2.);
#26074=VECTOR('',#112658,1000.);
#26075=VECTOR('',#112659,1000.);
#26076=VECTOR('',#112664,1000.);
#26077=VECTOR('',#112667,1000.);
#26078=VECTOR('',#112684,1000.);
#26079=VECTOR('',#112685,1000.);
#26080=VECTOR('',#112690,2.75);
#26081=VECTOR('',#112701,2.);
#26082=VECTOR('',#112704,1000.);
#26083=VECTOR('',#112707,1000.);
#26084=VECTOR('',#112710,1000.);
#26085=VECTOR('',#112715,1000.);
#26086=VECTOR('',#112716,1000.);
#26087=VECTOR('',#112723,1000.);
#26088=VECTOR('',#112726,1000.);
#26089=VECTOR('',#112727,1000.);
#26090=VECTOR('',#112730,1000.);
#26091=VECTOR('',#112733,1000.);
#26092=VECTOR('',#112738,1000.);
#26093=VECTOR('',#112743,1000.);
#26094=VECTOR('',#112744,1000.);
#26095=VECTOR('',#112747,1000.);
#26096=VECTOR('',#112750,1000.);
#26097=VECTOR('',#112751,1000.);
#26098=VECTOR('',#112754,1000.);
#26099=VECTOR('',#112757,1000.);
#26100=VECTOR('',#112762,1000.);
#26101=VECTOR('',#112763,1000.);
#26102=VECTOR('',#112770,1000.);
#26103=VECTOR('',#112771,1000.);
#26104=VECTOR('',#112774,1000.);
#26105=VECTOR('',#112777,1000.);
#26106=VECTOR('',#112778,1000.);
#26107=VECTOR('',#112781,1000.);
#26108=VECTOR('',#112784,1000.);
#26109=VECTOR('',#112791,1000.);
#26110=VECTOR('',#112802,1000.);
#26111=VECTOR('',#112803,1000.);
#26112=VECTOR('',#112806,1000.);
#26113=VECTOR('',#112807,1000.);
#26114=VECTOR('',#112812,1000.);
#26115=VECTOR('',#112815,1000.);
#26116=VECTOR('',#112816,1000.);
#26117=VECTOR('',#112819,1000.);
#26118=VECTOR('',#112822,1000.);
#26119=VECTOR('',#112829,1000.);
#26120=VECTOR('',#112832,1000.);
#26121=VECTOR('',#112833,1000.);
#26122=VECTOR('',#112834,1000.);
#26123=VECTOR('',#112837,1000.);
#26124=VECTOR('',#112840,1000.);
#26125=VECTOR('',#112841,1000.);
#26126=VECTOR('',#112844,1000.);
#26127=VECTOR('',#112847,1000.);
#26128=VECTOR('',#112854,1000.);
#26129=VECTOR('',#112855,1000.);
#26130=VECTOR('',#112856,1000.);
#26131=VECTOR('',#112859,1000.);
#26132=VECTOR('',#112862,1000.);
#26133=VECTOR('',#112863,1000.);
#26134=VECTOR('',#112866,1000.);
#26135=VECTOR('',#112869,1000.);
#26136=VECTOR('',#112870,1000.);
#26137=VECTOR('',#112877,1000.);
#26138=VECTOR('',#112880,1000.);
#26139=VECTOR('',#112881,1000.);
#26140=VECTOR('',#112884,1000.);
#26141=VECTOR('',#112887,1000.);
#26142=VECTOR('',#112888,1000.);
#26143=VECTOR('',#112891,1000.);
#26144=VECTOR('',#112894,1000.);
#26145=VECTOR('',#112901,1000.);
#26146=VECTOR('',#112906,1000.);
#26147=VECTOR('',#112907,1000.);
#26148=VECTOR('',#112914,1000.);
#26149=VECTOR('',#112915,1000.);
#26150=VECTOR('',#112918,1000.);
#26151=VECTOR('',#112921,1000.);
#26152=VECTOR('',#112922,1000.);
#26153=VECTOR('',#112925,1000.);
#26154=VECTOR('',#112928,1000.);
#26155=VECTOR('',#112935,1000.);
#26156=VECTOR('',#112938,1000.);
#26157=VECTOR('',#112939,1000.);
#26158=VECTOR('',#112954,1000.);
#26159=VECTOR('',#112955,1000.);
#26160=VECTOR('',#112962,1000.);
#26161=VECTOR('',#112967,1000.);
#26162=VECTOR('',#112970,1000.);
#26163=VECTOR('',#112973,1000.);
#26164=VECTOR('',#112988,1000.);
#26165=VECTOR('',#112997,1000.);
#26166=VECTOR('',#113012,1000.);
#26167=VECTOR('',#113021,1000.);
#26168=VECTOR('',#113036,1000.);
#26169=VECTOR('',#113045,1000.);
#26170=VECTOR('',#113060,1000.);
#26171=VECTOR('',#113061,1000.);
#26172=VECTOR('',#113068,1000.);
#26173=VECTOR('',#113073,1000.);
#26174=VECTOR('',#113076,1000.);
#26175=VECTOR('',#113079,1000.);
#26176=VECTOR('',#113096,1000.);
#26177=VECTOR('',#113097,1000.);
#26178=VECTOR('',#113100,1000.);
#26179=VECTOR('',#113105,1000.);
#26180=VECTOR('',#113114,1000.);
#26181=VECTOR('',#113119,1000.);
#26182=VECTOR('',#113126,1000.);
#26183=VECTOR('',#113127,1000.);
#26184=VECTOR('',#113132,1000.);
#26185=VECTOR('',#113135,1000.);
#26186=VECTOR('',#113150,1000.);
#26187=VECTOR('',#113151,1000.);
#26188=VECTOR('',#113160,1000.);
#26189=VECTOR('',#113163,1000.);
#26190=VECTOR('',#113180,1000.);
#26191=VECTOR('',#113181,1000.);
#26192=VECTOR('',#113182,1000.);
#26193=VECTOR('',#113185,1000.);
#26194=VECTOR('',#113190,1000.);
#26195=VECTOR('',#113193,1000.);
#26196=VECTOR('',#113196,1000.);
#26197=VECTOR('',#113199,1000.);
#26198=VECTOR('',#113208,1000.);
#26199=VECTOR('',#113209,1000.);
#26200=VECTOR('',#113212,1000.);
#26201=VECTOR('',#113215,1000.);
#26202=VECTOR('',#113226,1000.);
#26203=VECTOR('',#113229,1000.);
#26204=VECTOR('',#113230,1000.);
#26205=VECTOR('',#113237,1000.);
#26206=VECTOR('',#113242,1000.);
#26207=VECTOR('',#113245,1000.);
#26208=VECTOR('',#113248,1000.);
#26209=VECTOR('',#113251,1000.);
#26210=VECTOR('',#113264,1000.);
#26211=VECTOR('',#113267,1000.);
#26212=VECTOR('',#113276,1000.);
#26213=VECTOR('',#113279,1000.);
#26214=VECTOR('',#113292,1000.);
#26215=VECTOR('',#113295,1000.);
#26216=VECTOR('',#113296,1000.);
#26217=VECTOR('',#113307,1000.);
#26218=VECTOR('',#113318,1000.);
#26219=VECTOR('',#113327,1000.);
#26220=VECTOR('',#113336,1000.);
#26221=VECTOR('',#113347,1000.);
#26222=VECTOR('',#113356,1000.);
#26223=VECTOR('',#113369,1000.);
#26224=VECTOR('',#113378,1000.);
#26225=VECTOR('',#113381,2.75);
#26226=VECTOR('',#113386,2.75);
#26227=VECTOR('',#113399,1000.);
#26228=VECTOR('',#113422,1000.);
#26229=VECTOR('',#113445,1000.);
#26230=VECTOR('',#113468,1000.);
#26231=VECTOR('',#113481,1000.);
#26232=VECTOR('',#113488,1000.);
#26233=VECTOR('',#113497,1000.);
#26234=VECTOR('',#113498,1000.);
#26235=VECTOR('',#113503,1000.);
#26236=VECTOR('',#113504,1000.);
#26237=VECTOR('',#113509,1000.);
#26238=VECTOR('',#113512,1000.);
#26239=VECTOR('',#113517,1000.);
#26240=VECTOR('',#113528,1000.);
#26241=VECTOR('',#113537,1000.);
#26242=VECTOR('',#113540,1000.);
#26243=VECTOR('',#113545,1000.);
#26244=VECTOR('',#113556,1000.);
#26245=VECTOR('',#113565,1000.);
#26246=VECTOR('',#113568,1000.);
#26247=VECTOR('',#113581,1000.);
#26248=VECTOR('',#113592,1000.);
#26249=VECTOR('',#113601,1000.);
#26250=VECTOR('',#113610,1000.);
#26251=VECTOR('',#113621,1000.);
#26252=VECTOR('',#113632,1000.);
#26253=VECTOR('',#113637,1000.);
#26254=VECTOR('',#113642,1000.);
#26255=VECTOR('',#113659,1000.);
#26256=VECTOR('',#113668,1000.);
#26257=VECTOR('',#113669,1000.);
#26258=VECTOR('',#113672,1000.);
#26259=VECTOR('',#113677,1000.);
#26260=VECTOR('',#113678,1000.);
#26261=VECTOR('',#113681,1000.);
#26262=VECTOR('',#113686,1000.);
#26263=VECTOR('',#113693,1000.);
#26264=VECTOR('',#113702,1000.);
#26265=VECTOR('',#113707,1000.);
#26266=VECTOR('',#113710,1000.);
#26267=VECTOR('',#113715,1000.);
#26268=VECTOR('',#113722,1000.);
#26269=VECTOR('',#113727,1000.);
#26270=VECTOR('',#113730,1000.);
#26271=VECTOR('',#113741,1000.);
#26272=VECTOR('',#113744,1000.);
#26273=VECTOR('',#113753,1000.);
#26274=VECTOR('',#113758,1000.);
#26275=VECTOR('',#113761,1000.);
#26276=VECTOR('',#113768,1000.);
#26277=VECTOR('',#113775,1000.);
#26278=VECTOR('',#113780,1000.);
#26279=VECTOR('',#113787,1000.);
#26280=VECTOR('',#113794,1000.);
#26281=VECTOR('',#113797,1000.);
#26282=VECTOR('',#113804,1000.);
#26283=VECTOR('',#113809,1000.);
#26284=VECTOR('',#113816,1000.);
#26285=VECTOR('',#113821,1000.);
#26286=VECTOR('',#113824,1000.);
#26287=VECTOR('',#113833,1000.);
#26288=VECTOR('',#113838,1000.);
#26289=VECTOR('',#113845,1000.);
#26290=VECTOR('',#113848,1000.);
#26291=VECTOR('',#113857,1000.);
#26292=VECTOR('',#113860,1000.);
#26293=VECTOR('',#113869,1000.);
#26294=VECTOR('',#113874,1000.);
#26295=VECTOR('',#113877,1000.);
#26296=VECTOR('',#113882,1000.);
#26297=VECTOR('',#113889,1000.);
#26298=VECTOR('',#113896,1000.);
#26299=VECTOR('',#113903,1000.);
#26300=VECTOR('',#113908,1000.);
#26301=VECTOR('',#113911,1000.);
#26302=VECTOR('',#113918,1000.);
#26303=VECTOR('',#113925,1000.);
#26304=VECTOR('',#113940,1000.);
#26305=VECTOR('',#113947,1000.);
#26306=VECTOR('',#113960,1000.);
#26307=VECTOR('',#113967,1000.);
#26308=VECTOR('',#113980,1000.);
#26309=VECTOR('',#113987,1000.);
#26310=VECTOR('',#114000,1000.);
#26311=VECTOR('',#114007,1000.);
#26312=VECTOR('',#114022,1000.);
#26313=VECTOR('',#114031,1000.);
#26314=VECTOR('',#114036,1000.);
#26315=VECTOR('',#114037,1000.);
#26316=VECTOR('',#114038,1000.);
#26317=VECTOR('',#114045,1000.);
#26318=VECTOR('',#114046,1000.);
#26319=VECTOR('',#114047,1000.);
#26320=VECTOR('',#114058,1000.);
#26321=VECTOR('',#114059,1000.);
#26322=VECTOR('',#114060,1000.);
#26323=VECTOR('',#114079,1000.);
#26324=VECTOR('',#114080,1000.);
#26325=VECTOR('',#114095,1000.);
#26326=VECTOR('',#114108,1000.);
#26327=VECTOR('',#114115,1000.);
#26328=VECTOR('',#114128,1000.);
#26329=VECTOR('',#114137,1000.);
#26330=VECTOR('',#114150,1000.);
#26331=VECTOR('',#114157,1000.);
#26332=VECTOR('',#114172,1000.);
#26333=VECTOR('',#114179,1000.);
#26334=VECTOR('',#114194,1000.);
#26335=VECTOR('',#114201,1000.);
#26336=VECTOR('',#114216,1000.);
#26337=VECTOR('',#114223,1000.);
#26338=VECTOR('',#114234,1000.);
#26339=VECTOR('',#114237,1000.);
#26340=VECTOR('',#114238,1000.);
#26341=VECTOR('',#114239,1000.);
#26342=VECTOR('',#114246,1000.);
#26343=VECTOR('',#114247,1000.);
#26344=VECTOR('',#114248,1000.);
#26345=VECTOR('',#114259,1000.);
#26346=VECTOR('',#114260,1000.);
#26347=VECTOR('',#114261,1000.);
#26348=VECTOR('',#114314,1000.);
#26349=VECTOR('',#114317,1000.);
#26350=VECTOR('',#114346,1000.);
#26351=VECTOR('',#114347,1000.);
#26352=VECTOR('',#114350,1000.);
#26353=VECTOR('',#114353,1000.);
#26354=VECTOR('',#114356,1000.);
#26355=VECTOR('',#114359,1000.);
#26356=VECTOR('',#114364,2.);
#26357=VECTOR('',#114407,3.25);
#26358=VECTOR('',#114412,1.47499999999998);
#26359=VECTOR('',#114421,2.);
#26360=VECTOR('',#114430,2.5);
#26361=VECTOR('',#114693,1000.);
#26362=VECTOR('',#114696,1000.);
#26363=VECTOR('',#114721,1000.);
#26364=VECTOR('',#114722,1000.);
#26365=VECTOR('',#114725,1000.);
#26366=VECTOR('',#114728,1000.);
#26367=VECTOR('',#114751,1000.);
#26368=VECTOR('',#114752,1000.);
#26369=VECTOR('',#114755,1000.);
#26370=VECTOR('',#114758,1000.);
#26371=VECTOR('',#114781,1000.);
#26372=VECTOR('',#114782,1000.);
#26373=VECTOR('',#114785,1000.);
#26374=VECTOR('',#114788,1000.);
#26375=VECTOR('',#114811,1000.);
#26376=VECTOR('',#114812,1000.);
#26377=VECTOR('',#114815,1000.);
#26378=VECTOR('',#114816,1000.);
#26379=VECTOR('',#114819,1000.);
#26380=VECTOR('',#114820,1000.);
#26381=VECTOR('',#114823,1000.);
#26382=VECTOR('',#114824,1000.);
#26383=VECTOR('',#114827,1000.);
#26384=VECTOR('',#114828,1000.);
#26385=VECTOR('',#114831,1000.);
#26386=VECTOR('',#114832,1000.);
#26387=VECTOR('',#114835,1000.);
#26388=VECTOR('',#114836,1000.);
#26389=VECTOR('',#114839,1000.);
#26390=VECTOR('',#114840,1000.);
#26391=VECTOR('',#114843,1000.);
#26392=VECTOR('',#114844,1000.);
#26393=VECTOR('',#114859,1000.);
#26394=VECTOR('',#114860,1000.);
#26395=VECTOR('',#114889,1000.);
#26396=VECTOR('',#114890,1000.);
#26397=VECTOR('',#114917,1000.);
#26398=VECTOR('',#114918,1000.);
#26399=VECTOR('',#114933,1000.);
#26400=VECTOR('',#114934,1000.);
#26401=VECTOR('',#114963,1000.);
#26402=VECTOR('',#114964,1000.);
#26403=VECTOR('',#114969,1000.);
#26404=VECTOR('',#114970,1000.);
#26405=VECTOR('',#114991,1000.);
#26406=VECTOR('',#114992,1000.);
#26407=VECTOR('',#115021,1000.);
#26408=VECTOR('',#115022,1000.);
#26409=VECTOR('',#115027,1000.);
#26410=VECTOR('',#115028,1000.);
#26411=VECTOR('',#115049,1000.);
#26412=VECTOR('',#115050,1000.);
#26413=VECTOR('',#115055,1000.);
#26414=VECTOR('',#115056,1000.);
#26415=VECTOR('',#115077,1000.);
#26416=VECTOR('',#115078,1000.);
#26417=VECTOR('',#115083,1000.);
#26418=VECTOR('',#115084,1000.);
#26419=VECTOR('',#115105,1000.);
#26420=VECTOR('',#115106,1000.);
#26421=VECTOR('',#115111,1000.);
#26422=VECTOR('',#115112,1000.);
#26423=VECTOR('',#115141,1000.);
#26424=VECTOR('',#115142,1000.);
#26425=VECTOR('',#115171,1000.);
#26426=VECTOR('',#115172,1000.);
#26427=VECTOR('',#115177,1000.);
#26428=VECTOR('',#115178,1000.);
#26429=VECTOR('',#115199,1000.);
#26430=VECTOR('',#115200,1000.);
#26431=VECTOR('',#115205,1000.);
#26432=VECTOR('',#115206,1000.);
#26433=VECTOR('',#115227,1000.);
#26434=VECTOR('',#115228,1000.);
#26435=VECTOR('',#115233,1000.);
#26436=VECTOR('',#115234,1000.);
#26437=VECTOR('',#115255,1000.);
#26438=VECTOR('',#115256,1000.);
#26439=VECTOR('',#115261,1000.);
#26440=VECTOR('',#115262,1000.);
#26441=VECTOR('',#115283,1000.);
#26442=VECTOR('',#115284,1000.);
#26443=VECTOR('',#115289,1000.);
#26444=VECTOR('',#115290,1000.);
#26445=VECTOR('',#115311,1000.);
#26446=VECTOR('',#115312,1000.);
#26447=VECTOR('',#115317,1000.);
#26448=VECTOR('',#115318,1000.);
#26449=VECTOR('',#115339,1000.);
#26450=VECTOR('',#115340,1000.);
#26451=VECTOR('',#115345,1000.);
#26452=VECTOR('',#115346,1000.);
#26453=VECTOR('',#115367,1000.);
#26454=VECTOR('',#115368,1000.);
#26455=VECTOR('',#115373,1000.);
#26456=VECTOR('',#115374,1000.);
#26457=VECTOR('',#115395,1000.);
#26458=VECTOR('',#115396,1000.);
#26459=VECTOR('',#115401,1000.);
#26460=VECTOR('',#115402,1000.);
#26461=VECTOR('',#115423,1000.);
#26462=VECTOR('',#115424,1000.);
#26463=VECTOR('',#115453,1000.);
#26464=VECTOR('',#115454,1000.);
#26465=VECTOR('',#115459,1000.);
#26466=VECTOR('',#115460,1000.);
#26467=VECTOR('',#115481,1000.);
#26468=VECTOR('',#115482,1000.);
#26469=VECTOR('',#115527,1000.);
#26470=VECTOR('',#115528,1000.);
#26471=VECTOR('',#115533,1000.);
#26472=VECTOR('',#115534,1000.);
#26473=VECTOR('',#115555,1000.);
#26474=VECTOR('',#115556,1000.);
#26475=VECTOR('',#115585,1000.);
#26476=VECTOR('',#115586,1000.);
#26477=VECTOR('',#115591,1000.);
#26478=VECTOR('',#115592,1000.);
#26479=VECTOR('',#115613,1000.);
#26480=VECTOR('',#115614,1000.);
#26481=VECTOR('',#115619,1000.);
#26482=VECTOR('',#115620,1000.);
#26483=VECTOR('',#115641,1000.);
#26484=VECTOR('',#115642,1000.);
#26485=VECTOR('',#115671,1000.);
#26486=VECTOR('',#115672,1000.);
#26487=VECTOR('',#115677,1000.);
#26488=VECTOR('',#115678,1000.);
#26489=VECTOR('',#115697,1000.);
#26490=VECTOR('',#115698,1000.);
#26491=VECTOR('',#115713,1000.);
#26492=VECTOR('',#115714,1000.);
#26493=VECTOR('',#115719,1000.);
#26494=VECTOR('',#115720,1000.);
#26495=VECTOR('',#115741,1000.);
#26496=VECTOR('',#115742,1000.);
#26497=VECTOR('',#115769,1000.);
#26498=VECTOR('',#115770,1000.);
#26499=VECTOR('',#115785,1000.);
#26500=VECTOR('',#115786,1000.);
#26501=VECTOR('',#115791,1000.);
#26502=VECTOR('',#115792,1000.);
#26503=VECTOR('',#115813,1000.);
#26504=VECTOR('',#115814,1000.);
#26505=VECTOR('',#115819,1000.);
#26506=VECTOR('',#115820,1000.);
#26507=VECTOR('',#115841,1000.);
#26508=VECTOR('',#115842,1000.);
#26509=VECTOR('',#115847,1000.);
#26510=VECTOR('',#115848,1000.);
#26511=VECTOR('',#115877,1000.);
#26512=VECTOR('',#115878,1000.);
#26513=VECTOR('',#115899,1000.);
#26514=VECTOR('',#115900,1000.);
#26515=VECTOR('',#115905,1000.);
#26516=VECTOR('',#115906,1000.);
#26517=VECTOR('',#115927,1000.);
#26518=VECTOR('',#115928,1000.);
#26519=VECTOR('',#115933,1000.);
#26520=VECTOR('',#115934,1000.);
#26521=VECTOR('',#115955,1000.);
#26522=VECTOR('',#115956,1000.);
#26523=VECTOR('',#115961,1000.);
#26524=VECTOR('',#115962,1000.);
#26525=VECTOR('',#115983,1000.);
#26526=VECTOR('',#115984,1000.);
#26527=VECTOR('',#115989,1000.);
#26528=VECTOR('',#115990,1000.);
#26529=VECTOR('',#116011,1000.);
#26530=VECTOR('',#116012,1000.);
#26531=VECTOR('',#116017,1000.);
#26532=VECTOR('',#116018,1000.);
#26533=VECTOR('',#116039,1000.);
#26534=VECTOR('',#116040,1000.);
#26535=VECTOR('',#116077,1000.);
#26536=VECTOR('',#116078,1000.);
#26537=VECTOR('',#116083,1000.);
#26538=VECTOR('',#116084,1000.);
#26539=VECTOR('',#116113,1000.);
#26540=VECTOR('',#116114,1000.);
#26541=VECTOR('',#116135,1000.);
#26542=VECTOR('',#116136,1000.);
#26543=VECTOR('',#116141,1000.);
#26544=VECTOR('',#116142,1000.);
#26545=VECTOR('',#116171,1000.);
#26546=VECTOR('',#116172,1000.);
#26547=VECTOR('',#116209,1000.);
#26548=VECTOR('',#116210,1000.);
#26549=VECTOR('',#116215,1000.);
#26550=VECTOR('',#116216,1000.);
#26551=VECTOR('',#116237,1000.);
#26552=VECTOR('',#116238,1000.);
#26553=VECTOR('',#116243,1000.);
#26554=VECTOR('',#116244,1000.);
#26555=VECTOR('',#116265,1000.);
#26556=VECTOR('',#116266,1000.);
#26557=VECTOR('',#116271,1000.);
#26558=VECTOR('',#116272,1000.);
#26559=VECTOR('',#116293,1000.);
#26560=VECTOR('',#116294,1000.);
#26561=VECTOR('',#116339,1000.);
#26562=VECTOR('',#116340,1000.);
#26563=VECTOR('',#116345,1000.);
#26564=VECTOR('',#116346,1000.);
#26565=VECTOR('',#116367,1000.);
#26566=VECTOR('',#116368,1000.);
#26567=VECTOR('',#116397,1000.);
#26568=VECTOR('',#116398,1000.);
#26569=VECTOR('',#116403,1000.);
#26570=VECTOR('',#116404,1000.);
#26571=VECTOR('',#116425,1000.);
#26572=VECTOR('',#116426,1000.);
#26573=VECTOR('',#116431,1000.);
#26574=VECTOR('',#116432,1000.);
#26575=VECTOR('',#116453,1000.);
#26576=VECTOR('',#116454,1000.);
#26577=VECTOR('',#116459,1000.);
#26578=VECTOR('',#116460,1000.);
#26579=VECTOR('',#116481,1000.);
#26580=VECTOR('',#116482,1000.);
#26581=VECTOR('',#116511,1000.);
#26582=VECTOR('',#116512,1000.);
#26583=VECTOR('',#116517,1000.);
#26584=VECTOR('',#116518,1000.);
#26585=VECTOR('',#116539,1000.);
#26586=VECTOR('',#116540,1000.);
#26587=VECTOR('',#116545,1000.);
#26588=VECTOR('',#116546,1000.);
#26589=VECTOR('',#116567,1000.);
#26590=VECTOR('',#116568,1000.);
#26591=VECTOR('',#116595,1000.);
#26592=VECTOR('',#116596,1000.);
#26593=VECTOR('',#116611,1000.);
#26594=VECTOR('',#116612,1000.);
#26595=VECTOR('',#116639,1000.);
#26596=VECTOR('',#116640,1000.);
#26597=VECTOR('',#116769,1000.);
#26598=VECTOR('',#116770,1000.);
#26599=VECTOR('',#116799,1000.);
#26600=VECTOR('',#116800,1000.);
#26601=VECTOR('',#116819,1000.);
#26602=VECTOR('',#116820,1000.);
#26603=VECTOR('',#116849,1000.);
#26604=VECTOR('',#116850,1000.);
#26605=VECTOR('',#116869,1000.);
#26606=VECTOR('',#116870,1000.);
#26607=VECTOR('',#116899,1000.);
#26608=VECTOR('',#116900,1000.);
#26609=VECTOR('',#116919,1000.);
#26610=VECTOR('',#116920,1000.);
#26611=VECTOR('',#116949,1000.);
#26612=VECTOR('',#116950,1000.);
#26613=VECTOR('',#117167,1000.);
#26614=VECTOR('',#117168,1000.);
#26615=VECTOR('',#117171,1000.);
#26616=VECTOR('',#117174,1000.);
#26617=VECTOR('',#117177,1000.);
#26618=VECTOR('',#117180,1000.);
#26619=VECTOR('',#117183,1000.);
#26620=VECTOR('',#117186,1000.);
#26621=VECTOR('',#117189,1000.);
#26622=VECTOR('',#117192,1000.);
#26623=VECTOR('',#117195,1000.);
#26624=VECTOR('',#117198,1000.);
#26625=VECTOR('',#117201,1000.);
#26626=VECTOR('',#117204,1000.);
#26627=VECTOR('',#117207,1000.);
#26628=VECTOR('',#117210,1000.);
#26629=VECTOR('',#117213,1000.);
#26630=VECTOR('',#117216,1000.);
#26631=VECTOR('',#117221,1000.);
#26632=VECTOR('',#117222,1000.);
#26633=VECTOR('',#117225,1000.);
#26634=VECTOR('',#117228,1000.);
#26635=VECTOR('',#117231,1000.);
#26636=VECTOR('',#117234,1000.);
#26637=VECTOR('',#117237,1000.);
#26638=VECTOR('',#117240,1000.);
#26639=VECTOR('',#117243,1000.);
#26640=VECTOR('',#117246,1000.);
#26641=VECTOR('',#117249,1000.);
#26642=VECTOR('',#117252,1000.);
#26643=VECTOR('',#117255,1000.);
#26644=VECTOR('',#117258,1000.);
#26645=VECTOR('',#117261,1000.);
#26646=VECTOR('',#117264,1000.);
#26647=VECTOR('',#117267,1000.);
#26648=VECTOR('',#117270,1000.);
#26649=VECTOR('',#117273,1000.);
#26650=VECTOR('',#117276,1000.);
#26651=VECTOR('',#117279,1000.);
#26652=VECTOR('',#117282,1000.);
#26653=VECTOR('',#117285,1000.);
#26654=VECTOR('',#117288,1000.);
#26655=VECTOR('',#117291,1000.);
#26656=VECTOR('',#117294,1000.);
#26657=VECTOR('',#117297,1000.);
#26658=VECTOR('',#117300,1000.);
#26659=VECTOR('',#117303,1000.);
#26660=VECTOR('',#117306,1000.);
#26661=VECTOR('',#117309,1000.);
#26662=VECTOR('',#117312,1000.);
#26663=VECTOR('',#117315,1000.);
#26664=VECTOR('',#117318,1000.);
#26665=VECTOR('',#117321,1000.);
#26666=VECTOR('',#117324,1000.);
#26667=VECTOR('',#117329,1000.);
#26668=VECTOR('',#117330,1000.);
#26669=VECTOR('',#117333,1000.);
#26670=VECTOR('',#117336,1000.);
#26671=VECTOR('',#117339,1000.);
#26672=VECTOR('',#117342,1000.);
#26673=VECTOR('',#117345,1000.);
#26674=VECTOR('',#117348,1000.);
#26675=VECTOR('',#117351,1000.);
#26676=VECTOR('',#117354,1000.);
#26677=VECTOR('',#117357,1000.);
#26678=VECTOR('',#117360,1000.);
#26679=VECTOR('',#117363,1000.);
#26680=VECTOR('',#117366,1000.);
#26681=VECTOR('',#117369,1000.);
#26682=VECTOR('',#117372,1000.);
#26683=VECTOR('',#117375,1000.);
#26684=VECTOR('',#117378,1000.);
#26685=VECTOR('',#117381,1000.);
#26686=VECTOR('',#117384,1000.);
#26687=VECTOR('',#117387,1000.);
#26688=VECTOR('',#117390,1000.);
#26689=VECTOR('',#117393,1000.);
#26690=VECTOR('',#117396,1000.);
#26691=VECTOR('',#117399,1000.);
#26692=VECTOR('',#117402,1000.);
#26693=VECTOR('',#117405,1000.);
#26694=VECTOR('',#117408,1000.);
#26695=VECTOR('',#117411,1000.);
#26696=VECTOR('',#117414,1000.);
#26697=VECTOR('',#117417,1000.);
#26698=VECTOR('',#117420,1000.);
#26699=VECTOR('',#117423,1000.);
#26700=VECTOR('',#117426,1000.);
#26701=VECTOR('',#117429,1000.);
#26702=VECTOR('',#117432,1000.);
#26703=VECTOR('',#117435,1000.);
#26704=VECTOR('',#117438,1000.);
#26705=VECTOR('',#117441,1000.);
#26706=VECTOR('',#117444,1000.);
#26707=VECTOR('',#117447,1000.);
#26708=VECTOR('',#117450,1000.);
#26709=VECTOR('',#117453,1000.);
#26710=VECTOR('',#117456,1000.);
#26711=VECTOR('',#117459,1000.);
#26712=VECTOR('',#117462,1000.);
#26713=VECTOR('',#117465,1000.);
#26714=VECTOR('',#117468,1000.);
#26715=VECTOR('',#117471,1000.);
#26716=VECTOR('',#117474,1000.);
#26717=VECTOR('',#117477,1000.);
#26718=VECTOR('',#117480,1000.);
#26719=VECTOR('',#117483,1000.);
#26720=VECTOR('',#117486,1000.);
#26721=VECTOR('',#117489,1000.);
#26722=VECTOR('',#117492,1000.);
#26723=VECTOR('',#117495,1000.);
#26724=VECTOR('',#117498,1000.);
#26725=VECTOR('',#117501,1000.);
#26726=VECTOR('',#117504,1000.);
#26727=VECTOR('',#117507,1000.);
#26728=VECTOR('',#117510,1000.);
#26729=VECTOR('',#117513,1000.);
#26730=VECTOR('',#117516,1000.);
#26731=VECTOR('',#117519,1000.);
#26732=VECTOR('',#117522,1000.);
#26733=VECTOR('',#117525,1000.);
#26734=VECTOR('',#117528,1000.);
#26735=VECTOR('',#117531,1000.);
#26736=VECTOR('',#117534,1000.);
#26737=VECTOR('',#117537,1000.);
#26738=VECTOR('',#117540,1000.);
#26739=VECTOR('',#117543,1000.);
#26740=VECTOR('',#117546,1000.);
#26741=VECTOR('',#117549,1000.);
#26742=VECTOR('',#117552,1000.);
#26743=VECTOR('',#117555,1000.);
#26744=VECTOR('',#117558,1000.);
#26745=VECTOR('',#117561,1000.);
#26746=VECTOR('',#117564,1000.);
#26747=VECTOR('',#117567,1000.);
#26748=VECTOR('',#117570,1000.);
#26749=VECTOR('',#117573,1000.);
#26750=VECTOR('',#117576,1000.);
#26751=VECTOR('',#117579,1000.);
#26752=VECTOR('',#117582,1000.);
#26753=VECTOR('',#117585,1000.);
#26754=VECTOR('',#117588,1000.);
#26755=VECTOR('',#117591,1000.);
#26756=VECTOR('',#117594,1000.);
#26757=VECTOR('',#117597,1000.);
#26758=VECTOR('',#117600,1000.);
#26759=VECTOR('',#117603,1000.);
#26760=VECTOR('',#117606,1000.);
#26761=VECTOR('',#117609,1000.);
#26762=VECTOR('',#117612,1000.);
#26763=VECTOR('',#117615,1000.);
#26764=VECTOR('',#117618,1000.);
#26765=VECTOR('',#117621,1000.);
#26766=VECTOR('',#117624,1000.);
#26767=VECTOR('',#117627,1000.);
#26768=VECTOR('',#117630,1000.);
#26769=VECTOR('',#117633,1000.);
#26770=VECTOR('',#117636,1000.);
#26771=VECTOR('',#117639,1000.);
#26772=VECTOR('',#117642,1000.);
#26773=VECTOR('',#117645,1000.);
#26774=VECTOR('',#117648,1000.);
#26775=VECTOR('',#117651,1000.);
#26776=VECTOR('',#117654,1000.);
#26777=VECTOR('',#117657,1000.);
#26778=VECTOR('',#117660,1000.);
#26779=VECTOR('',#117663,1000.);
#26780=VECTOR('',#117666,1000.);
#26781=VECTOR('',#117669,1000.);
#26782=VECTOR('',#117672,1000.);
#26783=VECTOR('',#117677,1000.);
#26784=VECTOR('',#117678,1000.);
#26785=VECTOR('',#117681,1000.);
#26786=VECTOR('',#117684,1000.);
#26787=VECTOR('',#117687,1000.);
#26788=VECTOR('',#117690,1000.);
#26789=VECTOR('',#117693,1000.);
#26790=VECTOR('',#117696,1000.);
#26791=VECTOR('',#117699,1000.);
#26792=VECTOR('',#117702,1000.);
#26793=VECTOR('',#117705,1000.);
#26794=VECTOR('',#117708,1000.);
#26795=VECTOR('',#117711,1000.);
#26796=VECTOR('',#117714,1000.);
#26797=VECTOR('',#117717,1000.);
#26798=VECTOR('',#117720,1000.);
#26799=VECTOR('',#117723,1000.);
#26800=VECTOR('',#117726,1000.);
#26801=VECTOR('',#117729,1000.);
#26802=VECTOR('',#117732,1000.);
#26803=VECTOR('',#117735,1000.);
#26804=VECTOR('',#117738,1000.);
#26805=VECTOR('',#117741,1000.);
#26806=VECTOR('',#117744,1000.);
#26807=VECTOR('',#117747,1000.);
#26808=VECTOR('',#117750,1000.);
#26809=VECTOR('',#117753,1000.);
#26810=VECTOR('',#117756,1000.);
#26811=VECTOR('',#117759,1000.);
#26812=VECTOR('',#117762,1000.);
#26813=VECTOR('',#117765,1000.);
#26814=VECTOR('',#117768,1000.);
#26815=VECTOR('',#117771,1000.);
#26816=VECTOR('',#117774,1000.);
#26817=VECTOR('',#117777,1000.);
#26818=VECTOR('',#117780,1000.);
#26819=VECTOR('',#117783,1000.);
#26820=VECTOR('',#117786,1000.);
#26821=VECTOR('',#117789,1000.);
#26822=VECTOR('',#117792,1000.);
#26823=VECTOR('',#117795,1000.);
#26824=VECTOR('',#117798,1000.);
#26825=VECTOR('',#117801,1000.);
#26826=VECTOR('',#117804,1000.);
#26827=VECTOR('',#117807,1000.);
#26828=VECTOR('',#117810,1000.);
#26829=VECTOR('',#117813,1000.);
#26830=VECTOR('',#117816,1000.);
#26831=VECTOR('',#117821,1000.);
#26832=VECTOR('',#117822,1000.);
#26833=VECTOR('',#117825,1000.);
#26834=VECTOR('',#117828,1000.);
#26835=VECTOR('',#117831,1000.);
#26836=VECTOR('',#117834,1000.);
#26837=VECTOR('',#117837,1000.);
#26838=VECTOR('',#117840,1000.);
#26839=VECTOR('',#117843,1000.);
#26840=VECTOR('',#117846,1000.);
#26841=VECTOR('',#117849,1000.);
#26842=VECTOR('',#117852,1000.);
#26843=VECTOR('',#117855,1000.);
#26844=VECTOR('',#117858,1000.);
#26845=VECTOR('',#117861,1000.);
#26846=VECTOR('',#117864,1000.);
#26847=VECTOR('',#117867,1000.);
#26848=VECTOR('',#117870,1000.);
#26849=VECTOR('',#117873,1000.);
#26850=VECTOR('',#117876,1000.);
#26851=VECTOR('',#117879,1000.);
#26852=VECTOR('',#117882,1000.);
#26853=VECTOR('',#117885,1000.);
#26854=VECTOR('',#117888,1000.);
#26855=VECTOR('',#117891,1000.);
#26856=VECTOR('',#117894,1000.);
#26857=VECTOR('',#117897,1000.);
#26858=VECTOR('',#117900,1000.);
#26859=VECTOR('',#117903,1000.);
#26860=VECTOR('',#117906,1000.);
#26861=VECTOR('',#117909,1000.);
#26862=VECTOR('',#117912,1000.);
#26863=VECTOR('',#117917,1000.);
#26864=VECTOR('',#117918,1000.);
#26865=VECTOR('',#117921,1000.);
#26866=VECTOR('',#117924,1000.);
#26867=VECTOR('',#117927,1000.);
#26868=VECTOR('',#117930,1000.);
#26869=VECTOR('',#117933,1000.);
#26870=VECTOR('',#117936,1000.);
#26871=VECTOR('',#117939,1000.);
#26872=VECTOR('',#117942,1000.);
#26873=VECTOR('',#117947,1000.);
#26874=VECTOR('',#117948,1000.);
#26875=VECTOR('',#117951,1000.);
#26876=VECTOR('',#117954,1000.);
#26877=VECTOR('',#117959,1000.);
#26878=VECTOR('',#117960,1000.);
#26879=VECTOR('',#117963,1000.);
#26880=VECTOR('',#117966,1000.);
#26881=VECTOR('',#117969,1000.);
#26882=VECTOR('',#117972,1000.);
#26883=VECTOR('',#117975,1000.);
#26884=VECTOR('',#117978,1000.);
#26885=VECTOR('',#117981,1000.);
#26886=VECTOR('',#117988,1000.);
#26887=VECTOR('',#118003,1000.);
#26888=VECTOR('',#118006,1000.);
#26889=VECTOR('',#118021,1000.);
#26890=VECTOR('',#118024,1000.);
#26891=VECTOR('',#118035,1000.);
#26892=VECTOR('',#118038,1000.);
#26893=VECTOR('',#118041,1000.);
#26894=VECTOR('',#118044,1000.);
#26895=VECTOR('',#118047,1000.);
#26896=VECTOR('',#118050,1000.);
#26897=VECTOR('',#118053,1000.);
#26898=VECTOR('',#118056,1000.);
#26899=VECTOR('',#118059,1000.);
#26900=VECTOR('',#118062,1000.);
#26901=VECTOR('',#118065,1000.);
#26902=VECTOR('',#118068,1000.);
#26903=VECTOR('',#118071,1000.);
#26904=VECTOR('',#118074,1000.);
#26905=VECTOR('',#118077,1000.);
#26906=VECTOR('',#118080,1000.);
#26907=VECTOR('',#118083,1000.);
#26908=VECTOR('',#118086,1000.);
#26909=VECTOR('',#118089,1000.);
#26910=VECTOR('',#118092,1000.);
#26911=VECTOR('',#118095,1000.);
#26912=VECTOR('',#118098,1000.);
#26913=VECTOR('',#118101,1000.);
#26914=VECTOR('',#118104,1000.);
#26915=VECTOR('',#118107,1000.);
#26916=VECTOR('',#118110,1000.);
#26917=VECTOR('',#118113,1000.);
#26918=VECTOR('',#118116,1000.);
#26919=VECTOR('',#118119,1000.);
#26920=VECTOR('',#118122,1000.);
#26921=VECTOR('',#118125,1000.);
#26922=VECTOR('',#118128,1000.);
#26923=VECTOR('',#118131,1000.);
#26924=VECTOR('',#118132,1000.);
#26925=VECTOR('',#118133,1000.);
#26926=VECTOR('',#118134,1000.);
#26927=VECTOR('',#118137,1000.);
#26928=VECTOR('',#118138,1000.);
#26929=VECTOR('',#118139,1000.);
#26930=VECTOR('',#118142,1000.);
#26931=VECTOR('',#118143,1000.);
#26932=VECTOR('',#118144,1000.);
#26933=VECTOR('',#118147,1000.);
#26934=VECTOR('',#118150,1000.);
#26935=VECTOR('',#118153,1000.);
#26936=VECTOR('',#118156,1000.);
#26937=VECTOR('',#118159,1000.);
#26938=VECTOR('',#118162,1000.);
#26939=VECTOR('',#118165,1000.);
#26940=VECTOR('',#118168,1000.);
#26941=VECTOR('',#118171,1000.);
#26942=VECTOR('',#118174,1000.);
#26943=VECTOR('',#118177,1000.);
#26944=VECTOR('',#118180,1000.);
#26945=VECTOR('',#118183,1000.);
#26946=VECTOR('',#118186,1000.);
#26947=VECTOR('',#118189,1000.);
#26948=VECTOR('',#118192,1000.);
#26949=VECTOR('',#118195,1000.);
#26950=VECTOR('',#118198,1000.);
#26951=VECTOR('',#118201,1000.);
#26952=VECTOR('',#118204,1000.);
#26953=VECTOR('',#118207,1000.);
#26954=VECTOR('',#118210,1000.);
#26955=VECTOR('',#118213,1000.);
#26956=VECTOR('',#118216,1000.);
#26957=VECTOR('',#118223,1000.);
#26958=VECTOR('',#118230,1000.);
#26959=VECTOR('',#118237,1000.);
#26960=VECTOR('',#118244,1000.);
#26961=VECTOR('',#118251,1000.);
#26962=VECTOR('',#118258,1000.);
#26963=VECTOR('',#118263,1000.);
#26964=VECTOR('',#118266,1000.);
#26965=VECTOR('',#118269,10.);
#26966=VECTOR('',#118274,1000.);
#26967=VECTOR('',#118277,10.);
#26968=VECTOR('',#118280,1000.);
#26969=VECTOR('',#118281,1000.);
#26970=VECTOR('',#118284,1000.);
#26971=VECTOR('',#118285,1000.);
#26972=VECTOR('',#118294,1000.);
#26973=VECTOR('',#118295,1000.);
#26974=VECTOR('',#118298,1000.);
#26975=VECTOR('',#118299,1000.);
#26976=VECTOR('',#118310,1000.);
#26977=VECTOR('',#118313,1000.);
#26978=VECTOR('',#118318,1000.);
#26979=VECTOR('',#118321,1000.);
#26980=VECTOR('',#118326,1000.);
#26981=VECTOR('',#118333,1000.);
#26982=VECTOR('',#118346,1000.);
#26983=VECTOR('',#118349,1000.);
#26984=VECTOR('',#118360,1000.);
#26985=VECTOR('',#118361,1000.);
#26986=VECTOR('',#118364,1000.);
#26987=VECTOR('',#118373,1000.);
#26988=VECTOR('',#118378,1000.);
#26989=VECTOR('',#118381,1000.);
#26990=VECTOR('',#118384,1000.);
#26991=VECTOR('',#118393,1000.);
#26992=VECTOR('',#118398,1000.);
#26993=VECTOR('',#118401,1000.);
#26994=VECTOR('',#118408,1000.);
#26995=VECTOR('',#118415,1000.);
#26996=VECTOR('',#118422,1000.);
#26997=VECTOR('',#118427,1000.);
#26998=VECTOR('',#118430,1000.);
#26999=VECTOR('',#118437,1000.);
#27000=VECTOR('',#118494,1000.);
#27001=VECTOR('',#118517,10.);
#27002=VECTOR('',#118520,10.);
#27003=VECTOR('',#118527,1000.);
#27004=VECTOR('',#118530,1000.);
#27005=VECTOR('',#118535,1000.);
#27006=VECTOR('',#118540,1000.);
#27007=VECTOR('',#118547,1000.);
#27008=VECTOR('',#118550,1000.);
#27009=VECTOR('',#118557,1000.);
#27010=VECTOR('',#118560,1000.);
#27011=VECTOR('',#118567,3.35);
#27012=VECTOR('',#118578,3.35000000000079);
#27013=VECTOR('',#118611,1000.);
#27014=VECTOR('',#118614,1000.);
#27015=VECTOR('',#118617,1000.);
#27016=VECTOR('',#118622,1000.);
#27017=VECTOR('',#118627,1000.);
#27018=VECTOR('',#118632,1000.);
#27019=VECTOR('',#118637,1000.);
#27020=VECTOR('',#118644,1000.);
#27021=VECTOR('',#118647,1000.);
#27022=VECTOR('',#118650,1000.);
#27023=VECTOR('',#118653,1000.);
#27024=VECTOR('',#118656,1000.);
#27025=VECTOR('',#118661,1000.);
#27026=VECTOR('',#118666,1000.);
#27027=VECTOR('',#118671,1000.);
#27028=VECTOR('',#118676,1000.);
#27029=VECTOR('',#118681,1000.);
#27030=VECTOR('',#118682,1000.);
#27031=VECTOR('',#118683,1000.);
#27032=VECTOR('',#118684,1000.);
#27033=VECTOR('',#118687,1000.);
#27034=VECTOR('',#118688,1000.);
#27035=VECTOR('',#118691,1000.);
#27036=VECTOR('',#118694,1000.);
#27037=VECTOR('',#118697,1000.);
#27038=VECTOR('',#118698,1000.);
#27039=VECTOR('',#118701,1000.);
#27040=VECTOR('',#118704,1000.);
#27041=VECTOR('',#118707,1000.);
#27042=VECTOR('',#118710,1000.);
#27043=VECTOR('',#118715,1000.);
#27044=VECTOR('',#118720,1000.);
#27045=VECTOR('',#118725,1000.);
#27046=VECTOR('',#118728,1000.);
#27047=VECTOR('',#118731,1000.);
#27048=VECTOR('',#118736,1000.);
#27049=VECTOR('',#118769,1000.);
#27050=VECTOR('',#118772,1000.);
#27051=VECTOR('',#118775,1000.);
#27052=VECTOR('',#118778,1000.);
#27053=VECTOR('',#118781,1000.);
#27054=VECTOR('',#118784,1000.);
#27055=VECTOR('',#118787,1000.);
#27056=VECTOR('',#118790,1000.);
#27057=VECTOR('',#118793,1000.);
#27058=VECTOR('',#118796,1000.);
#27059=VECTOR('',#118813,1000.);
#27060=VECTOR('',#118816,1000.);
#27061=VECTOR('',#118819,1000.);
#27062=VECTOR('',#118822,1000.);
#27063=VECTOR('',#118825,1000.);
#27064=VECTOR('',#118828,1000.);
#27065=VECTOR('',#118831,1000.);
#27066=VECTOR('',#118834,1000.);
#27067=VECTOR('',#118837,1000.);
#27068=VECTOR('',#118840,1000.);
#27069=VECTOR('',#118843,1000.);
#27070=VECTOR('',#118846,1000.);
#27071=VECTOR('',#118849,1000.);
#27072=VECTOR('',#118852,1000.);
#27073=VECTOR('',#118887,1000.);
#27074=VECTOR('',#118890,1000.);
#27075=VECTOR('',#118893,1000.);
#27076=VECTOR('',#118896,1000.);
#27077=VECTOR('',#118899,1000.);
#27078=VECTOR('',#118902,1000.);
#27079=VECTOR('',#118905,1000.);
#27080=VECTOR('',#118908,1000.);
#27081=VECTOR('',#118911,1000.);
#27082=VECTOR('',#118914,1000.);
#27083=VECTOR('',#118917,1000.);
#27084=VECTOR('',#118920,1000.);
#27085=VECTOR('',#118923,1000.);
#27086=VECTOR('',#118926,1000.);
#27087=VECTOR('',#118929,1000.);
#27088=VECTOR('',#118932,1000.);
#27089=VECTOR('',#118935,1000.);
#27090=VECTOR('',#118938,1000.);
#27091=VECTOR('',#118941,1000.);
#27092=VECTOR('',#118944,1000.);
#27093=VECTOR('',#118947,1000.);
#27094=VECTOR('',#118950,1000.);
#27095=VECTOR('',#118953,1000.);
#27096=VECTOR('',#118956,1000.);
#27097=VECTOR('',#118959,1000.);
#27098=VECTOR('',#118962,1000.);
#27099=VECTOR('',#118965,1000.);
#27100=VECTOR('',#118968,1000.);
#27101=VECTOR('',#119249,1000.);
#27102=VECTOR('',#119250,1000.);
#27103=VECTOR('',#119277,1000.);
#27104=VECTOR('',#119278,1000.);
#27105=VECTOR('',#119281,1000.);
#27106=VECTOR('',#119282,1000.);
#27107=VECTOR('',#119307,1000.);
#27108=VECTOR('',#119308,1000.);
#27109=VECTOR('',#119311,1000.);
#27110=VECTOR('',#119312,1000.);
#27111=VECTOR('',#119337,1000.);
#27112=VECTOR('',#119338,1000.);
#27113=VECTOR('',#119341,1000.);
#27114=VECTOR('',#119342,1000.);
#27115=VECTOR('',#119367,1000.);
#27116=VECTOR('',#119368,1000.);
#27117=VECTOR('',#119371,1000.);
#27118=VECTOR('',#119372,1000.);
#27119=VECTOR('',#119375,1000.);
#27120=VECTOR('',#119376,1000.);
#27121=VECTOR('',#119379,1000.);
#27122=VECTOR('',#119380,1000.);
#27123=VECTOR('',#119383,1000.);
#27124=VECTOR('',#119384,1000.);
#27125=VECTOR('',#119387,1000.);
#27126=VECTOR('',#119388,1000.);
#27127=VECTOR('',#119391,1000.);
#27128=VECTOR('',#119392,1000.);
#27129=VECTOR('',#119395,1000.);
#27130=VECTOR('',#119396,1000.);
#27131=VECTOR('',#119399,1000.);
#27132=VECTOR('',#119400,1000.);
#27133=VECTOR('',#119415,1000.);
#27134=VECTOR('',#119416,1000.);
#27135=VECTOR('',#119445,1000.);
#27136=VECTOR('',#119446,1000.);
#27137=VECTOR('',#119473,1000.);
#27138=VECTOR('',#119474,1000.);
#27139=VECTOR('',#119489,1000.);
#27140=VECTOR('',#119490,1000.);
#27141=VECTOR('',#119519,1000.);
#27142=VECTOR('',#119520,1000.);
#27143=VECTOR('',#119525,1000.);
#27144=VECTOR('',#119526,1000.);
#27145=VECTOR('',#119547,1000.);
#27146=VECTOR('',#119548,1000.);
#27147=VECTOR('',#119577,1000.);
#27148=VECTOR('',#119578,1000.);
#27149=VECTOR('',#119583,1000.);
#27150=VECTOR('',#119584,1000.);
#27151=VECTOR('',#119605,1000.);
#27152=VECTOR('',#119606,1000.);
#27153=VECTOR('',#119611,1000.);
#27154=VECTOR('',#119612,1000.);
#27155=VECTOR('',#119633,1000.);
#27156=VECTOR('',#119634,1000.);
#27157=VECTOR('',#119639,1000.);
#27158=VECTOR('',#119640,1000.);
#27159=VECTOR('',#119661,1000.);
#27160=VECTOR('',#119662,1000.);
#27161=VECTOR('',#119667,1000.);
#27162=VECTOR('',#119668,1000.);
#27163=VECTOR('',#119697,1000.);
#27164=VECTOR('',#119698,1000.);
#27165=VECTOR('',#119727,1000.);
#27166=VECTOR('',#119728,1000.);
#27167=VECTOR('',#119733,1000.);
#27168=VECTOR('',#119734,1000.);
#27169=VECTOR('',#119755,1000.);
#27170=VECTOR('',#119756,1000.);
#27171=VECTOR('',#119761,1000.);
#27172=VECTOR('',#119762,1000.);
#27173=VECTOR('',#119783,1000.);
#27174=VECTOR('',#119784,1000.);
#27175=VECTOR('',#119789,1000.);
#27176=VECTOR('',#119790,1000.);
#27177=VECTOR('',#119811,1000.);
#27178=VECTOR('',#119812,1000.);
#27179=VECTOR('',#119817,1000.);
#27180=VECTOR('',#119818,1000.);
#27181=VECTOR('',#119839,1000.);
#27182=VECTOR('',#119840,1000.);
#27183=VECTOR('',#119845,1000.);
#27184=VECTOR('',#119846,1000.);
#27185=VECTOR('',#119867,1000.);
#27186=VECTOR('',#119868,1000.);
#27187=VECTOR('',#119873,1000.);
#27188=VECTOR('',#119874,1000.);
#27189=VECTOR('',#119895,1000.);
#27190=VECTOR('',#119896,1000.);
#27191=VECTOR('',#119901,1000.);
#27192=VECTOR('',#119902,1000.);
#27193=VECTOR('',#119923,1000.);
#27194=VECTOR('',#119924,1000.);
#27195=VECTOR('',#119929,1000.);
#27196=VECTOR('',#119930,1000.);
#27197=VECTOR('',#119951,1000.);
#27198=VECTOR('',#119952,1000.);
#27199=VECTOR('',#119957,1000.);
#27200=VECTOR('',#119958,1000.);
#27201=VECTOR('',#119979,1000.);
#27202=VECTOR('',#119980,1000.);
#27203=VECTOR('',#120009,1000.);
#27204=VECTOR('',#120010,1000.);
#27205=VECTOR('',#120015,1000.);
#27206=VECTOR('',#120016,1000.);
#27207=VECTOR('',#120037,1000.);
#27208=VECTOR('',#120038,1000.);
#27209=VECTOR('',#120083,1000.);
#27210=VECTOR('',#120084,1000.);
#27211=VECTOR('',#120089,1000.);
#27212=VECTOR('',#120090,1000.);
#27213=VECTOR('',#120111,1000.);
#27214=VECTOR('',#120112,1000.);
#27215=VECTOR('',#120141,1000.);
#27216=VECTOR('',#120142,1000.);
#27217=VECTOR('',#120147,1000.);
#27218=VECTOR('',#120148,1000.);
#27219=VECTOR('',#120169,1000.);
#27220=VECTOR('',#120170,1000.);
#27221=VECTOR('',#120175,1000.);
#27222=VECTOR('',#120176,1000.);
#27223=VECTOR('',#120197,1000.);
#27224=VECTOR('',#120198,1000.);
#27225=VECTOR('',#120227,1000.);
#27226=VECTOR('',#120228,1000.);
#27227=VECTOR('',#120233,1000.);
#27228=VECTOR('',#120234,1000.);
#27229=VECTOR('',#120253,1000.);
#27230=VECTOR('',#120254,1000.);
#27231=VECTOR('',#120269,1000.);
#27232=VECTOR('',#120270,1000.);
#27233=VECTOR('',#120275,1000.);
#27234=VECTOR('',#120276,1000.);
#27235=VECTOR('',#120297,1000.);
#27236=VECTOR('',#120298,1000.);
#27237=VECTOR('',#120325,1000.);
#27238=VECTOR('',#120326,1000.);
#27239=VECTOR('',#120341,1000.);
#27240=VECTOR('',#120342,1000.);
#27241=VECTOR('',#120347,1000.);
#27242=VECTOR('',#120348,1000.);
#27243=VECTOR('',#120369,1000.);
#27244=VECTOR('',#120370,1000.);
#27245=VECTOR('',#120375,1000.);
#27246=VECTOR('',#120376,1000.);
#27247=VECTOR('',#120397,1000.);
#27248=VECTOR('',#120398,1000.);
#27249=VECTOR('',#120403,1000.);
#27250=VECTOR('',#120404,1000.);
#27251=VECTOR('',#120433,1000.);
#27252=VECTOR('',#120434,1000.);
#27253=VECTOR('',#120455,1000.);
#27254=VECTOR('',#120456,1000.);
#27255=VECTOR('',#120461,1000.);
#27256=VECTOR('',#120462,1000.);
#27257=VECTOR('',#120483,1000.);
#27258=VECTOR('',#120484,1000.);
#27259=VECTOR('',#120489,1000.);
#27260=VECTOR('',#120490,1000.);
#27261=VECTOR('',#120511,1000.);
#27262=VECTOR('',#120512,1000.);
#27263=VECTOR('',#120517,1000.);
#27264=VECTOR('',#120518,1000.);
#27265=VECTOR('',#120539,1000.);
#27266=VECTOR('',#120540,1000.);
#27267=VECTOR('',#120545,1000.);
#27268=VECTOR('',#120546,1000.);
#27269=VECTOR('',#120567,1000.);
#27270=VECTOR('',#120568,1000.);
#27271=VECTOR('',#120573,1000.);
#27272=VECTOR('',#120574,1000.);
#27273=VECTOR('',#120595,1000.);
#27274=VECTOR('',#120596,1000.);
#27275=VECTOR('',#120633,1000.);
#27276=VECTOR('',#120634,1000.);
#27277=VECTOR('',#120639,1000.);
#27278=VECTOR('',#120640,1000.);
#27279=VECTOR('',#120669,1000.);
#27280=VECTOR('',#120670,1000.);
#27281=VECTOR('',#120691,1000.);
#27282=VECTOR('',#120692,1000.);
#27283=VECTOR('',#120697,1000.);
#27284=VECTOR('',#120698,1000.);
#27285=VECTOR('',#120727,1000.);
#27286=VECTOR('',#120728,1000.);
#27287=VECTOR('',#120765,1000.);
#27288=VECTOR('',#120766,1000.);
#27289=VECTOR('',#120771,1000.);
#27290=VECTOR('',#120772,1000.);
#27291=VECTOR('',#120793,1000.);
#27292=VECTOR('',#120794,1000.);
#27293=VECTOR('',#120799,1000.);
#27294=VECTOR('',#120800,1000.);
#27295=VECTOR('',#120821,1000.);
#27296=VECTOR('',#120822,1000.);
#27297=VECTOR('',#120827,1000.);
#27298=VECTOR('',#120828,1000.);
#27299=VECTOR('',#120849,1000.);
#27300=VECTOR('',#120850,1000.);
#27301=VECTOR('',#120895,1000.);
#27302=VECTOR('',#120896,1000.);
#27303=VECTOR('',#120901,1000.);
#27304=VECTOR('',#120902,1000.);
#27305=VECTOR('',#120923,1000.);
#27306=VECTOR('',#120924,1000.);
#27307=VECTOR('',#120953,1000.);
#27308=VECTOR('',#120954,1000.);
#27309=VECTOR('',#120959,1000.);
#27310=VECTOR('',#120960,1000.);
#27311=VECTOR('',#120981,1000.);
#27312=VECTOR('',#120982,1000.);
#27313=VECTOR('',#120987,1000.);
#27314=VECTOR('',#120988,1000.);
#27315=VECTOR('',#121009,1000.);
#27316=VECTOR('',#121010,1000.);
#27317=VECTOR('',#121015,1000.);
#27318=VECTOR('',#121016,1000.);
#27319=VECTOR('',#121037,1000.);
#27320=VECTOR('',#121038,1000.);
#27321=VECTOR('',#121067,1000.);
#27322=VECTOR('',#121068,1000.);
#27323=VECTOR('',#121073,1000.);
#27324=VECTOR('',#121074,1000.);
#27325=VECTOR('',#121095,1000.);
#27326=VECTOR('',#121096,1000.);
#27327=VECTOR('',#121101,1000.);
#27328=VECTOR('',#121102,1000.);
#27329=VECTOR('',#121123,1000.);
#27330=VECTOR('',#121124,1000.);
#27331=VECTOR('',#121151,1000.);
#27332=VECTOR('',#121152,1000.);
#27333=VECTOR('',#121167,1000.);
#27334=VECTOR('',#121168,1000.);
#27335=VECTOR('',#121195,1000.);
#27336=VECTOR('',#121196,1000.);
#27337=VECTOR('',#121365,1000.);
#27338=VECTOR('',#121366,1000.);
#27339=VECTOR('',#121395,1000.);
#27340=VECTOR('',#121396,1000.);
#27341=VECTOR('',#121415,1000.);
#27342=VECTOR('',#121416,1000.);
#27343=VECTOR('',#121445,1000.);
#27344=VECTOR('',#121446,1000.);
#27345=VECTOR('',#121465,1000.);
#27346=VECTOR('',#121466,1000.);
#27347=VECTOR('',#121495,1000.);
#27348=VECTOR('',#121496,1000.);
#27349=VECTOR('',#121515,1000.);
#27350=VECTOR('',#121516,1000.);
#27351=VECTOR('',#121545,1000.);
#27352=VECTOR('',#121546,1000.);
#27353=VECTOR('',#121775,1000.);
#27354=VECTOR('',#121776,1000.);
#27355=VECTOR('',#121779,1000.);
#27356=VECTOR('',#121780,1000.);
#27357=VECTOR('',#121785,1000.);
#27358=VECTOR('',#121786,1000.);
#27359=VECTOR('',#121791,1000.);
#27360=VECTOR('',#121792,1000.);
#27361=VECTOR('',#121797,1000.);
#27362=VECTOR('',#121798,1000.);
#27363=VECTOR('',#121803,1000.);
#27364=VECTOR('',#121804,1000.);
#27365=VECTOR('',#121809,1000.);
#27366=VECTOR('',#121810,1000.);
#27367=VECTOR('',#121815,1000.);
#27368=VECTOR('',#121816,1000.);
#27369=VECTOR('',#121821,1000.);
#27370=VECTOR('',#121822,1000.);
#27371=VECTOR('',#121829,1000.);
#27372=VECTOR('',#121830,1000.);
#27373=VECTOR('',#121833,1000.);
#27374=VECTOR('',#121834,1000.);
#27375=VECTOR('',#121839,1000.);
#27376=VECTOR('',#121840,1000.);
#27377=VECTOR('',#121845,1000.);
#27378=VECTOR('',#121846,1000.);
#27379=VECTOR('',#121851,1000.);
#27380=VECTOR('',#121852,1000.);
#27381=VECTOR('',#121857,1000.);
#27382=VECTOR('',#121858,1000.);
#27383=VECTOR('',#121863,1000.);
#27384=VECTOR('',#121864,1000.);
#27385=VECTOR('',#121869,1000.);
#27386=VECTOR('',#121870,1000.);
#27387=VECTOR('',#121875,1000.);
#27388=VECTOR('',#121876,1000.);
#27389=VECTOR('',#121881,1000.);
#27390=VECTOR('',#121882,1000.);
#27391=VECTOR('',#121887,1000.);
#27392=VECTOR('',#121888,1000.);
#27393=VECTOR('',#121893,1000.);
#27394=VECTOR('',#121894,1000.);
#27395=VECTOR('',#121899,1000.);
#27396=VECTOR('',#121900,1000.);
#27397=VECTOR('',#121905,1000.);
#27398=VECTOR('',#121906,1000.);
#27399=VECTOR('',#121911,1000.);
#27400=VECTOR('',#121912,1000.);
#27401=VECTOR('',#121917,1000.);
#27402=VECTOR('',#121918,1000.);
#27403=VECTOR('',#121923,1000.);
#27404=VECTOR('',#121924,1000.);
#27405=VECTOR('',#121929,1000.);
#27406=VECTOR('',#121930,1000.);
#27407=VECTOR('',#121937,1000.);
#27408=VECTOR('',#121938,1000.);
#27409=VECTOR('',#121941,1000.);
#27410=VECTOR('',#121942,1000.);
#27411=VECTOR('',#121947,1000.);
#27412=VECTOR('',#121948,1000.);
#27413=VECTOR('',#121953,1000.);
#27414=VECTOR('',#121954,1000.);
#27415=VECTOR('',#121959,1000.);
#27416=VECTOR('',#121960,1000.);
#27417=VECTOR('',#121965,1000.);
#27418=VECTOR('',#121966,1000.);
#27419=VECTOR('',#121971,1000.);
#27420=VECTOR('',#121972,1000.);
#27421=VECTOR('',#121977,1000.);
#27422=VECTOR('',#121978,1000.);
#27423=VECTOR('',#121983,1000.);
#27424=VECTOR('',#121984,1000.);
#27425=VECTOR('',#121989,1000.);
#27426=VECTOR('',#121990,1000.);
#27427=VECTOR('',#121995,1000.);
#27428=VECTOR('',#121996,1000.);
#27429=VECTOR('',#122001,1000.);
#27430=VECTOR('',#122002,1000.);
#27431=VECTOR('',#122007,1000.);
#27432=VECTOR('',#122008,1000.);
#27433=VECTOR('',#122013,1000.);
#27434=VECTOR('',#122014,1000.);
#27435=VECTOR('',#122019,1000.);
#27436=VECTOR('',#122020,1000.);
#27437=VECTOR('',#122025,1000.);
#27438=VECTOR('',#122026,1000.);
#27439=VECTOR('',#122031,1000.);
#27440=VECTOR('',#122032,1000.);
#27441=VECTOR('',#122037,1000.);
#27442=VECTOR('',#122038,1000.);
#27443=VECTOR('',#122043,1000.);
#27444=VECTOR('',#122044,1000.);
#27445=VECTOR('',#122049,1000.);
#27446=VECTOR('',#122050,1000.);
#27447=VECTOR('',#122055,1000.);
#27448=VECTOR('',#122056,1000.);
#27449=VECTOR('',#122061,1000.);
#27450=VECTOR('',#122062,1000.);
#27451=VECTOR('',#122067,1000.);
#27452=VECTOR('',#122068,1000.);
#27453=VECTOR('',#122073,1000.);
#27454=VECTOR('',#122074,1000.);
#27455=VECTOR('',#122079,1000.);
#27456=VECTOR('',#122080,1000.);
#27457=VECTOR('',#122085,1000.);
#27458=VECTOR('',#122086,1000.);
#27459=VECTOR('',#122091,1000.);
#27460=VECTOR('',#122092,1000.);
#27461=VECTOR('',#122097,1000.);
#27462=VECTOR('',#122098,1000.);
#27463=VECTOR('',#122103,1000.);
#27464=VECTOR('',#122104,1000.);
#27465=VECTOR('',#122109,1000.);
#27466=VECTOR('',#122110,1000.);
#27467=VECTOR('',#122115,1000.);
#27468=VECTOR('',#122116,1000.);
#27469=VECTOR('',#122121,1000.);
#27470=VECTOR('',#122122,1000.);
#27471=VECTOR('',#122127,1000.);
#27472=VECTOR('',#122128,1000.);
#27473=VECTOR('',#122133,1000.);
#27474=VECTOR('',#122134,1000.);
#27475=VECTOR('',#122139,1000.);
#27476=VECTOR('',#122140,1000.);
#27477=VECTOR('',#122145,1000.);
#27478=VECTOR('',#122146,1000.);
#27479=VECTOR('',#122151,1000.);
#27480=VECTOR('',#122152,1000.);
#27481=VECTOR('',#122157,1000.);
#27482=VECTOR('',#122158,1000.);
#27483=VECTOR('',#122163,1000.);
#27484=VECTOR('',#122164,1000.);
#27485=VECTOR('',#122169,1000.);
#27486=VECTOR('',#122170,1000.);
#27487=VECTOR('',#122175,1000.);
#27488=VECTOR('',#122176,1000.);
#27489=VECTOR('',#122181,1000.);
#27490=VECTOR('',#122182,1000.);
#27491=VECTOR('',#122187,1000.);
#27492=VECTOR('',#122188,1000.);
#27493=VECTOR('',#122193,1000.);
#27494=VECTOR('',#122194,1000.);
#27495=VECTOR('',#122199,1000.);
#27496=VECTOR('',#122200,1000.);
#27497=VECTOR('',#122205,1000.);
#27498=VECTOR('',#122206,1000.);
#27499=VECTOR('',#122211,1000.);
#27500=VECTOR('',#122212,1000.);
#27501=VECTOR('',#122217,1000.);
#27502=VECTOR('',#122218,1000.);
#27503=VECTOR('',#122223,1000.);
#27504=VECTOR('',#122224,1000.);
#27505=VECTOR('',#122229,1000.);
#27506=VECTOR('',#122230,1000.);
#27507=VECTOR('',#122235,1000.);
#27508=VECTOR('',#122236,1000.);
#27509=VECTOR('',#122241,1000.);
#27510=VECTOR('',#122242,1000.);
#27511=VECTOR('',#122247,1000.);
#27512=VECTOR('',#122248,1000.);
#27513=VECTOR('',#122253,1000.);
#27514=VECTOR('',#122254,1000.);
#27515=VECTOR('',#122259,1000.);
#27516=VECTOR('',#122260,1000.);
#27517=VECTOR('',#122265,1000.);
#27518=VECTOR('',#122266,1000.);
#27519=VECTOR('',#122271,1000.);
#27520=VECTOR('',#122272,1000.);
#27521=VECTOR('',#122277,1000.);
#27522=VECTOR('',#122278,1000.);
#27523=VECTOR('',#122285,1000.);
#27524=VECTOR('',#122286,1000.);
#27525=VECTOR('',#122289,1000.);
#27526=VECTOR('',#122290,1000.);
#27527=VECTOR('',#122295,1000.);
#27528=VECTOR('',#122296,1000.);
#27529=VECTOR('',#122301,1000.);
#27530=VECTOR('',#122302,1000.);
#27531=VECTOR('',#122307,1000.);
#27532=VECTOR('',#122308,1000.);
#27533=VECTOR('',#122313,1000.);
#27534=VECTOR('',#122314,1000.);
#27535=VECTOR('',#122319,1000.);
#27536=VECTOR('',#122320,1000.);
#27537=VECTOR('',#122325,1000.);
#27538=VECTOR('',#122326,1000.);
#27539=VECTOR('',#122331,1000.);
#27540=VECTOR('',#122332,1000.);
#27541=VECTOR('',#122337,1000.);
#27542=VECTOR('',#122338,1000.);
#27543=VECTOR('',#122343,1000.);
#27544=VECTOR('',#122344,1000.);
#27545=VECTOR('',#122349,1000.);
#27546=VECTOR('',#122350,1000.);
#27547=VECTOR('',#122355,1000.);
#27548=VECTOR('',#122356,1000.);
#27549=VECTOR('',#122361,1000.);
#27550=VECTOR('',#122362,1000.);
#27551=VECTOR('',#122367,1000.);
#27552=VECTOR('',#122368,1000.);
#27553=VECTOR('',#122373,1000.);
#27554=VECTOR('',#122374,1000.);
#27555=VECTOR('',#122379,1000.);
#27556=VECTOR('',#122380,1000.);
#27557=VECTOR('',#122385,1000.);
#27558=VECTOR('',#122386,1000.);
#27559=VECTOR('',#122391,1000.);
#27560=VECTOR('',#122392,1000.);
#27561=VECTOR('',#122397,1000.);
#27562=VECTOR('',#122398,1000.);
#27563=VECTOR('',#122403,1000.);
#27564=VECTOR('',#122404,1000.);
#27565=VECTOR('',#122409,1000.);
#27566=VECTOR('',#122410,1000.);
#27567=VECTOR('',#122415,1000.);
#27568=VECTOR('',#122416,1000.);
#27569=VECTOR('',#122421,1000.);
#27570=VECTOR('',#122422,1000.);
#27571=VECTOR('',#122429,1000.);
#27572=VECTOR('',#122430,1000.);
#27573=VECTOR('',#122433,1000.);
#27574=VECTOR('',#122434,1000.);
#27575=VECTOR('',#122439,1000.);
#27576=VECTOR('',#122440,1000.);
#27577=VECTOR('',#122445,1000.);
#27578=VECTOR('',#122446,1000.);
#27579=VECTOR('',#122451,1000.);
#27580=VECTOR('',#122452,1000.);
#27581=VECTOR('',#122457,1000.);
#27582=VECTOR('',#122458,1000.);
#27583=VECTOR('',#122463,1000.);
#27584=VECTOR('',#122464,1000.);
#27585=VECTOR('',#122469,1000.);
#27586=VECTOR('',#122470,1000.);
#27587=VECTOR('',#122475,1000.);
#27588=VECTOR('',#122476,1000.);
#27589=VECTOR('',#122481,1000.);
#27590=VECTOR('',#122482,1000.);
#27591=VECTOR('',#122487,1000.);
#27592=VECTOR('',#122488,1000.);
#27593=VECTOR('',#122493,1000.);
#27594=VECTOR('',#122494,1000.);
#27595=VECTOR('',#122499,1000.);
#27596=VECTOR('',#122500,1000.);
#27597=VECTOR('',#122505,1000.);
#27598=VECTOR('',#122506,1000.);
#27599=VECTOR('',#122511,1000.);
#27600=VECTOR('',#122512,1000.);
#27601=VECTOR('',#122517,1000.);
#27602=VECTOR('',#122518,1000.);
#27603=VECTOR('',#122525,1000.);
#27604=VECTOR('',#122526,1000.);
#27605=VECTOR('',#122529,1000.);
#27606=VECTOR('',#122530,1000.);
#27607=VECTOR('',#122535,1000.);
#27608=VECTOR('',#122536,1000.);
#27609=VECTOR('',#122541,1000.);
#27610=VECTOR('',#122542,1000.);
#27611=VECTOR('',#122547,1000.);
#27612=VECTOR('',#122548,1000.);
#27613=VECTOR('',#122555,1000.);
#27614=VECTOR('',#122556,1000.);
#27615=VECTOR('',#122559,1000.);
#27616=VECTOR('',#122560,1000.);
#27617=VECTOR('',#122567,1000.);
#27618=VECTOR('',#122568,1000.);
#27619=VECTOR('',#122571,1000.);
#27620=VECTOR('',#122572,1000.);
#27621=VECTOR('',#122577,1000.);
#27622=VECTOR('',#122578,1000.);
#27623=VECTOR('',#122583,1000.);
#27624=VECTOR('',#122584,1000.);
#27625=VECTOR('',#122589,1000.);
#27626=VECTOR('',#122594,1000.);
#27627=VECTOR('',#122603,4.62535);
#27628=VECTOR('',#122616,8.10553955266686);
#27629=VECTOR('',#122657,1000.);
#27630=VECTOR('',#122660,1000.);
#27631=VECTOR('',#122675,1000.);
#27632=VECTOR('',#122678,1000.);
#27633=VECTOR('',#122689,1000.);
#27634=VECTOR('',#122692,1000.);
#27635=VECTOR('',#122695,1000.);
#27636=VECTOR('',#122698,1000.);
#27637=VECTOR('',#122701,1000.);
#27638=VECTOR('',#122704,1000.);
#27639=VECTOR('',#122707,1000.);
#27640=VECTOR('',#122710,1000.);
#27641=VECTOR('',#122713,1000.);
#27642=VECTOR('',#122716,1000.);
#27643=VECTOR('',#122719,1000.);
#27644=VECTOR('',#122722,1000.);
#27645=VECTOR('',#122725,1000.);
#27646=VECTOR('',#122728,1000.);
#27647=VECTOR('',#122731,1000.);
#27648=VECTOR('',#122734,1000.);
#27649=VECTOR('',#122737,1000.);
#27650=VECTOR('',#122740,1000.);
#27651=VECTOR('',#122743,1000.);
#27652=VECTOR('',#122746,1000.);
#27653=VECTOR('',#122749,1000.);
#27654=VECTOR('',#122752,1000.);
#27655=VECTOR('',#122755,1000.);
#27656=VECTOR('',#122758,1000.);
#27657=VECTOR('',#122761,1000.);
#27658=VECTOR('',#122764,1000.);
#27659=VECTOR('',#122767,1000.);
#27660=VECTOR('',#122770,1000.);
#27661=VECTOR('',#122773,1000.);
#27662=VECTOR('',#122776,1000.);
#27663=VECTOR('',#122779,1000.);
#27664=VECTOR('',#122782,1000.);
#27665=VECTOR('',#122785,1000.);
#27666=VECTOR('',#122786,1000.);
#27667=VECTOR('',#122787,1000.);
#27668=VECTOR('',#122788,1000.);
#27669=VECTOR('',#122791,1000.);
#27670=VECTOR('',#122792,1000.);
#27671=VECTOR('',#122793,1000.);
#27672=VECTOR('',#122796,1000.);
#27673=VECTOR('',#122797,1000.);
#27674=VECTOR('',#122798,1000.);
#27675=VECTOR('',#122801,1000.);
#27676=VECTOR('',#122804,1000.);
#27677=VECTOR('',#122807,1000.);
#27678=VECTOR('',#122810,1000.);
#27679=VECTOR('',#122813,1000.);
#27680=VECTOR('',#122816,1000.);
#27681=VECTOR('',#122819,1000.);
#27682=VECTOR('',#122822,1000.);
#27683=VECTOR('',#122825,1000.);
#27684=VECTOR('',#122828,1000.);
#27685=VECTOR('',#122831,1000.);
#27686=VECTOR('',#122834,1000.);
#27687=VECTOR('',#122837,1000.);
#27688=VECTOR('',#122840,1000.);
#27689=VECTOR('',#122843,1000.);
#27690=VECTOR('',#122846,1000.);
#27691=VECTOR('',#122849,1000.);
#27692=VECTOR('',#122852,1000.);
#27693=VECTOR('',#122855,1000.);
#27694=VECTOR('',#122858,1000.);
#27695=VECTOR('',#122861,1000.);
#27696=VECTOR('',#122864,1000.);
#27697=VECTOR('',#122889,1000.);
#27698=VECTOR('',#122890,1000.);
#27699=VECTOR('',#122891,1000.);
#27700=VECTOR('',#122892,1000.);
#27701=VECTOR('',#122893,1000.);
#27702=VECTOR('',#122894,1000.);
#27703=VECTOR('',#122895,1000.);
#27704=VECTOR('',#122896,1000.);
#27705=VECTOR('',#122897,1000.);
#27706=VECTOR('',#122900,1000.);
#27707=VECTOR('',#122903,1000.);
#27708=VECTOR('',#122904,1000.);
#27709=VECTOR('',#122905,1000.);
#27710=VECTOR('',#122906,1000.);
#27711=VECTOR('',#122907,1000.);
#27712=VECTOR('',#122910,1000.);
#27713=VECTOR('',#122911,1000.);
#27714=VECTOR('',#122918,1000.);
#27715=VECTOR('',#122919,1000.);
#27716=VECTOR('',#122926,1000.);
#27717=VECTOR('',#122927,1000.);
#27718=VECTOR('',#122930,1000.);
#27719=VECTOR('',#122931,1000.);
#27720=VECTOR('',#122934,1000.);
#27721=VECTOR('',#122935,1000.);
#27722=VECTOR('',#122938,1000.);
#27723=VECTOR('',#122939,1000.);
#27724=VECTOR('',#122942,1000.);
#27725=VECTOR('',#122943,1000.);
#27726=VECTOR('',#122944,1000.);
#27727=VECTOR('',#122947,1000.);
#27728=VECTOR('',#122948,1000.);
#27729=VECTOR('',#122949,1000.);
#27730=VECTOR('',#122950,1000.);
#27731=VECTOR('',#122951,1000.);
#27732=VECTOR('',#122952,1000.);
#27733=VECTOR('',#122953,1000.);
#27734=VECTOR('',#122954,1000.);
#27735=VECTOR('',#122961,1000.);
#27736=VECTOR('',#122968,1000.);
#27737=VECTOR('',#122969,1000.);
#27738=VECTOR('',#122970,1000.);
#27739=VECTOR('',#122971,1000.);
#27740=VECTOR('',#122972,1000.);
#27741=VECTOR('',#122975,1000.);
#27742=VECTOR('',#122976,1000.);
#27743=VECTOR('',#122977,1000.);
#27744=VECTOR('',#122978,1000.);
#27745=VECTOR('',#122979,1000.);
#27746=VECTOR('',#122980,1000.);
#27747=VECTOR('',#122981,1000.);
#27748=VECTOR('',#122982,1000.);
#27749=VECTOR('',#122985,1000.);
#27750=VECTOR('',#122986,1000.);
#27751=VECTOR('',#122993,1000.);
#27752=VECTOR('',#122996,1000.);
#27753=VECTOR('',#123001,1000.);
#27754=VECTOR('',#123006,1000.);
#27755=VECTOR('',#123013,1000.);
#27756=VECTOR('',#123016,1000.);
#27757=VECTOR('',#123025,1000.);
#27758=VECTOR('',#123026,1000.);
#27759=VECTOR('',#123031,10.);
#27760=VECTOR('',#123032,10.);
#27761=VECTOR('',#123037,1000.);
#27762=VECTOR('',#123040,10.);
#27763=VECTOR('',#123043,1000.);
#27764=VECTOR('',#123044,1000.);
#27765=VECTOR('',#123047,1000.);
#27766=VECTOR('',#123048,1000.);
#27767=VECTOR('',#123057,1000.);
#27768=VECTOR('',#123058,1000.);
#27769=VECTOR('',#123061,1000.);
#27770=VECTOR('',#123062,1000.);
#27771=VECTOR('',#123073,1000.);
#27772=VECTOR('',#123076,1000.);
#27773=VECTOR('',#123087,1000.);
#27774=VECTOR('',#123100,1000.);
#27775=VECTOR('',#123107,1000.);
#27776=VECTOR('',#123114,1000.);
#27777=VECTOR('',#123125,1000.);
#27778=VECTOR('',#123128,1000.);
#27779=VECTOR('',#123139,1000.);
#27780=VECTOR('',#123140,1000.);
#27781=VECTOR('',#123145,1000.);
#27782=VECTOR('',#123150,1000.);
#27783=VECTOR('',#123157,1000.);
#27784=VECTOR('',#123160,1000.);
#27785=VECTOR('',#123165,1000.);
#27786=VECTOR('',#123170,1000.);
#27787=VECTOR('',#123205,1000.);
#27788=VECTOR('',#123206,1000.);
#27789=VECTOR('',#123211,1000.);
#27790=VECTOR('',#123216,1000.);
#27791=VECTOR('',#123221,1000.);
#27792=VECTOR('',#123230,1000.);
#27793=VECTOR('',#123235,1000.);
#27794=VECTOR('',#123240,1000.);
#27795=VECTOR('',#123293,1000.);
#27796=VECTOR('',#123318,10.);
#27797=VECTOR('',#123321,10.);
#27798=VECTOR('',#123328,1000.);
#27799=VECTOR('',#123329,1000.);
#27800=VECTOR('',#123332,1000.);
#27801=VECTOR('',#123335,1000.);
#27802=VECTOR('',#123340,1000.);
#27803=VECTOR('',#123341,1000.);
#27804=VECTOR('',#123346,1000.);
#27805=VECTOR('',#123347,1000.);
#27806=VECTOR('',#123354,3.35);
#27807=VECTOR('',#123361,3.35000000000079);
#27808=VECTOR('',#123394,1000.);
#27809=VECTOR('',#123395,1000.);
#27810=VECTOR('',#123400,1000.);
#27811=VECTOR('',#123405,1000.);
#27812=VECTOR('',#123410,1000.);
#27813=VECTOR('',#123415,1000.);
#27814=VECTOR('',#123420,1000.);
#27815=VECTOR('',#123431,1000.);
#27816=VECTOR('',#123458,1000.);
#27817=VECTOR('',#123459,1000.);
#27818=VECTOR('',#123464,1000.);
#27819=VECTOR('',#123467,1000.);
#27820=VECTOR('',#123470,1000.);
#27821=VECTOR('',#123473,1000.);
#27822=VECTOR('',#123476,1000.);
#27823=VECTOR('',#123479,1000.);
#27824=VECTOR('',#123482,1000.);
#27825=VECTOR('',#123483,1000.);
#27826=VECTOR('',#123484,1000.);
#27827=VECTOR('',#123485,1000.);
#27828=VECTOR('',#123488,1000.);
#27829=VECTOR('',#123489,1000.);
#27830=VECTOR('',#123492,1000.);
#27831=VECTOR('',#123495,1000.);
#27832=VECTOR('',#123498,1000.);
#27833=VECTOR('',#123499,1000.);
#27834=VECTOR('',#123502,1000.);
#27835=VECTOR('',#123505,1000.);
#27836=VECTOR('',#123532,1000.);
#27837=VECTOR('',#123533,1000.);
#27838=VECTOR('',#123536,1000.);
#27839=VECTOR('',#123539,1000.);
#27840=VECTOR('',#123542,1000.);
#27841=VECTOR('',#123547,1000.);
#27842=VECTOR('',#123550,1000.);
#27843=VECTOR('',#123553,1000.);
#27844=VECTOR('',#123714,1000.);
#27845=VECTOR('',#123715,1000.);
#27846=VECTOR('',#123718,1000.);
#27847=VECTOR('',#123721,1000.);
#27848=VECTOR('',#123724,1000.);
#27849=VECTOR('',#123727,1000.);
#27850=VECTOR('',#123732,2.);
#27851=VECTOR('',#123775,3.25);
#27852=VECTOR('',#123830,1000.);
#27853=VECTOR('',#123831,1000.);
#27854=VECTOR('',#123834,1000.);
#27855=VECTOR('',#123837,1000.);
#27856=VECTOR('',#123840,1000.);
#27857=VECTOR('',#123843,1000.);
#27858=VECTOR('',#123900,1000.);
#27859=VECTOR('',#123901,1000.);
#27860=VECTOR('',#123904,1000.);
#27861=VECTOR('',#123907,1000.);
#27862=VECTOR('',#123910,1000.);
#27863=VECTOR('',#123913,1000.);
#27864=VECTOR('',#123918,1000.);
#27865=VECTOR('',#123919,1000.);
#27866=VECTOR('',#123922,1000.);
#27867=VECTOR('',#123925,1000.);
#27868=VECTOR('',#123928,1000.);
#27869=VECTOR('',#123931,1000.);
#27870=VECTOR('',#123936,2.);
#27871=VECTOR('',#123979,3.25);
#27872=VECTOR('',#124010,1000.);
#27873=VECTOR('',#124013,1000.);
#27874=VECTOR('',#124016,1000.);
#27875=VECTOR('',#124017,1000.);
#27876=VECTOR('',#124020,1000.);
#27877=VECTOR('',#124023,1000.);
#27878=VECTOR('',#124034,7.8);
#27879=VECTOR('',#124037,8.8);
#27880=VECTOR('',#124044,1.47499999999998);
#27881=VECTOR('',#124053,2.);
#27882=VECTOR('',#124062,2.5);
#27883=VECTOR('',#124079,1000.);
#27884=VECTOR('',#124080,1000.);
#27885=VECTOR('',#124085,1000.);
#27886=VECTOR('',#124086,1000.);
#27887=VECTOR('',#124107,1000.);
#27888=VECTOR('',#124108,1000.);
#27889=VECTOR('',#124113,1000.);
#27890=VECTOR('',#124114,1000.);
#27891=VECTOR('',#124123,1000.);
#27892=VECTOR('',#124124,1000.);
#27893=VECTOR('',#124125,1000.);
#27894=VECTOR('',#124128,1000.);
#27895=VECTOR('',#124133,1000.);
#27896=VECTOR('',#124138,1000.);
#27897=VECTOR('',#124139,1000.);
#27898=VECTOR('',#124140,1000.);
#27899=VECTOR('',#124141,1000.);
#27900=VECTOR('',#124160,1000.);
#27901=VECTOR('',#124171,1000.);
#27902=VECTOR('',#124194,1000.);
#27903=VECTOR('',#124197,1000.);
#27904=VECTOR('',#124200,1000.);
#27905=VECTOR('',#124203,1000.);
#27906=VECTOR('',#124210,1000.);
#27907=VECTOR('',#124213,1000.);
#27908=VECTOR('',#124230,1000.);
#27909=VECTOR('',#124231,1000.);
#27910=VECTOR('',#124244,1000.);
#27911=VECTOR('',#124247,1000.);
#27912=VECTOR('',#124262,1000.);
#27913=VECTOR('',#124263,1000.);
#27914=VECTOR('',#124268,1000.);
#27915=VECTOR('',#124269,1000.);
#27916=VECTOR('',#124274,1000.);
#27917=VECTOR('',#124275,1000.);
#27918=VECTOR('',#124278,1000.);
#27919=VECTOR('',#124281,1000.);
#27920=VECTOR('',#124284,1000.);
#27921=VECTOR('',#124287,1000.);
#27922=VECTOR('',#124290,1000.);
#27923=VECTOR('',#124293,1000.);
#27924=VECTOR('',#124298,1000.);
#27925=VECTOR('',#124301,1000.);
#27926=VECTOR('',#124304,7.8);
#27927=VECTOR('',#124307,7.8);
#27928=VECTOR('',#124310,1000.);
#27929=VECTOR('',#124343,1000.);
#27930=VECTOR('',#124346,1000.);
#27931=VECTOR('',#124349,1000.);
#27932=VECTOR('',#124350,1000.);
#27933=VECTOR('',#124353,1000.);
#27934=VECTOR('',#124356,1000.);
#27935=VECTOR('',#124367,7.8);
#27936=VECTOR('',#124370,8.8);
#27937=VECTOR('',#124377,1000.);
#27938=VECTOR('',#124378,1000.);
#27939=VECTOR('',#124391,1000.);
#27940=VECTOR('',#124392,1000.);
#27941=VECTOR('',#124403,1000.);
#27942=VECTOR('',#124404,1000.);
#27943=VECTOR('',#124409,1000.);
#27944=VECTOR('',#124412,1000.);
#27945=VECTOR('',#124425,1000.);
#27946=VECTOR('',#124426,1000.);
#27947=VECTOR('',#124437,1000.);
#27948=VECTOR('',#124438,1000.);
#27949=VECTOR('',#124443,1000.);
#27950=VECTOR('',#124446,1000.);
#27951=VECTOR('',#124459,1000.);
#27952=VECTOR('',#124460,1000.);
#27953=VECTOR('',#124473,1000.);
#27954=VECTOR('',#124474,1000.);
#27955=VECTOR('',#124487,1000.);
#27956=VECTOR('',#124488,1000.);
#27957=VECTOR('',#124501,1000.);
#27958=VECTOR('',#124502,1000.);
#27959=VECTOR('',#124507,1000.);
#27960=VECTOR('',#124510,1000.);
#27961=VECTOR('',#124523,1000.);
#27962=VECTOR('',#124524,1000.);
#27963=VECTOR('',#124535,1000.);
#27964=VECTOR('',#124536,1000.);
#27965=VECTOR('',#124541,1000.);
#27966=VECTOR('',#124544,1000.);
#27967=VECTOR('',#124557,1000.);
#27968=VECTOR('',#124558,1000.);
#27969=VECTOR('',#124579,1000.);
#27970=VECTOR('',#124580,1000.);
#27971=VECTOR('',#124593,1000.);
#27972=VECTOR('',#124594,1000.);
#27973=VECTOR('',#124607,1000.);
#27974=VECTOR('',#124608,1000.);
#27975=VECTOR('',#124613,1000.);
#27976=VECTOR('',#124616,1000.);
#27977=VECTOR('',#124629,1000.);
#27978=VECTOR('',#124630,1000.);
#27979=VECTOR('',#124659,1000.);
#27980=VECTOR('',#124660,1000.);
#27981=VECTOR('',#124673,1000.);
#27982=VECTOR('',#124674,1000.);
#27983=VECTOR('',#124679,1000.);
#27984=VECTOR('',#124682,1000.);
#27985=VECTOR('',#124695,1000.);
#27986=VECTOR('',#124696,1000.);
#27987=VECTOR('',#124725,1000.);
#27988=VECTOR('',#124726,1000.);
#27989=VECTOR('',#124739,1000.);
#27990=VECTOR('',#124740,1000.);
#27991=VECTOR('',#124745,1000.);
#27992=VECTOR('',#124748,1000.);
#27993=VECTOR('',#124761,1000.);
#27994=VECTOR('',#124762,1000.);
#27995=VECTOR('',#124791,1000.);
#27996=VECTOR('',#124792,1000.);
#27997=VECTOR('',#124805,1000.);
#27998=VECTOR('',#124806,1000.);
#27999=VECTOR('',#124811,1000.);
#28000=VECTOR('',#124814,1000.);
#28001=VECTOR('',#124827,1000.);
#28002=VECTOR('',#124828,1000.);
#28003=VECTOR('',#124857,1000.);
#28004=VECTOR('',#124858,1000.);
#28005=VECTOR('',#124871,1000.);
#28006=VECTOR('',#124872,1000.);
#28007=VECTOR('',#124877,1000.);
#28008=VECTOR('',#124880,1000.);
#28009=VECTOR('',#124893,1000.);
#28010=VECTOR('',#124894,1000.);
#28011=VECTOR('',#124923,1000.);
#28012=VECTOR('',#124924,1000.);
#28013=VECTOR('',#124937,1000.);
#28014=VECTOR('',#124938,1000.);
#28015=VECTOR('',#124943,1000.);
#28016=VECTOR('',#124946,1000.);
#28017=VECTOR('',#124959,1000.);
#28018=VECTOR('',#124960,1000.);
#28019=VECTOR('',#124989,1000.);
#28020=VECTOR('',#124990,1000.);
#28021=VECTOR('',#125003,1000.);
#28022=VECTOR('',#125004,1000.);
#28023=VECTOR('',#125009,1000.);
#28024=VECTOR('',#125012,1000.);
#28025=VECTOR('',#125025,1000.);
#28026=VECTOR('',#125026,1000.);
#28027=VECTOR('',#125039,1000.);
#28028=VECTOR('',#125040,1000.);
#28029=VECTOR('',#125061,1000.);
#28030=VECTOR('',#125062,1000.);
#28031=VECTOR('',#125075,1000.);
#28032=VECTOR('',#125076,1000.);
#28033=VECTOR('',#125081,1000.);
#28034=VECTOR('',#125084,1000.);
#28035=VECTOR('',#125097,1000.);
#28036=VECTOR('',#125098,1000.);
#28037=VECTOR('',#125111,1000.);
#28038=VECTOR('',#125112,1000.);
#28039=VECTOR('',#125125,1000.);
#28040=VECTOR('',#125126,1000.);
#28041=VECTOR('',#125139,1000.);
#28042=VECTOR('',#125140,1000.);
#28043=VECTOR('',#125143,1000.);
#28044=VECTOR('',#125146,1000.);
#28045=VECTOR('',#125159,1000.);
#28046=VECTOR('',#125160,1000.);
#28047=VECTOR('',#125173,1000.);
#28048=VECTOR('',#125174,1000.);
#28049=VECTOR('',#125177,1000.);
#28050=VECTOR('',#125178,1000.);
#28051=VECTOR('',#125183,1000.);
#28052=VECTOR('',#125184,1000.);
#28053=VECTOR('',#125189,1000.);
#28054=VECTOR('',#125190,1000.);
#28055=VECTOR('',#125195,1000.);
#28056=VECTOR('',#125196,1000.);
#28057=VECTOR('',#125201,1000.);
#28058=VECTOR('',#125202,1000.);
#28059=VECTOR('',#125207,1000.);
#28060=VECTOR('',#125208,1000.);
#28061=VECTOR('',#125213,1000.);
#28062=VECTOR('',#125214,1000.);
#28063=VECTOR('',#125219,1000.);
#28064=VECTOR('',#125220,1000.);
#28065=VECTOR('',#125225,1000.);
#28066=VECTOR('',#125226,1000.);
#28067=VECTOR('',#125231,1000.);
#28068=VECTOR('',#125232,1000.);
#28069=VECTOR('',#125237,1000.);
#28070=VECTOR('',#125238,1000.);
#28071=VECTOR('',#125243,1000.);
#28072=VECTOR('',#125244,1000.);
#28073=VECTOR('',#125249,1000.);
#28074=VECTOR('',#125250,1000.);
#28075=VECTOR('',#125255,1000.);
#28076=VECTOR('',#125256,1000.);
#28077=VECTOR('',#125261,1000.);
#28078=VECTOR('',#125262,1000.);
#28079=VECTOR('',#125267,1000.);
#28080=VECTOR('',#125268,1000.);
#28081=VECTOR('',#125273,1000.);
#28082=VECTOR('',#125274,1000.);
#28083=VECTOR('',#125279,1000.);
#28084=VECTOR('',#125280,1000.);
#28085=VECTOR('',#125285,1000.);
#28086=VECTOR('',#125286,1000.);
#28087=VECTOR('',#125291,1000.);
#28088=VECTOR('',#125292,1000.);
#28089=VECTOR('',#125297,1000.);
#28090=VECTOR('',#125298,1000.);
#28091=VECTOR('',#125303,1000.);
#28092=VECTOR('',#125304,1000.);
#28093=VECTOR('',#125309,1000.);
#28094=VECTOR('',#125310,1000.);
#28095=VECTOR('',#125315,1000.);
#28096=VECTOR('',#125316,1000.);
#28097=VECTOR('',#125321,1000.);
#28098=VECTOR('',#125322,1000.);
#28099=VECTOR('',#125327,1000.);
#28100=VECTOR('',#125328,1000.);
#28101=VECTOR('',#125337,1000.);
#28102=VECTOR('',#125338,1000.);
#28103=VECTOR('',#125341,1000.);
#28104=VECTOR('',#125342,1000.);
#28105=VECTOR('',#125343,1000.);
#28106=VECTOR('',#125344,1000.);
#28107=VECTOR('',#125345,1000.);
#28108=VECTOR('',#125346,1000.);
#28109=VECTOR('',#125347,1000.);
#28110=VECTOR('',#125348,1000.);
#28111=VECTOR('',#125349,1000.);
#28112=VECTOR('',#125350,1000.);
#28113=VECTOR('',#125351,1000.);
#28114=VECTOR('',#125354,1000.);
#28115=VECTOR('',#125357,1000.);
#28116=VECTOR('',#125360,1000.);
#28117=VECTOR('',#125363,1000.);
#28118=VECTOR('',#125366,1000.);
#28119=VECTOR('',#125369,1000.);
#28120=VECTOR('',#125370,1000.);
#28121=VECTOR('',#125373,1000.);
#28122=VECTOR('',#125376,1000.);
#28123=VECTOR('',#125379,1000.);
#28124=VECTOR('',#125382,1000.);
#28125=VECTOR('',#125385,1000.);
#28126=VECTOR('',#125388,1000.);
#28127=VECTOR('',#125391,1000.);
#28128=VECTOR('',#125394,1000.);
#28129=VECTOR('',#125397,1000.);
#28130=VECTOR('',#125400,1000.);
#28131=VECTOR('',#125403,1000.);
#28132=VECTOR('',#125404,1000.);
#28133=VECTOR('',#125413,1000.);
#28134=VECTOR('',#125416,1000.);
#28135=VECTOR('',#125419,1000.);
#28136=VECTOR('',#125420,1000.);
#28137=VECTOR('',#125429,1000.);
#28138=VECTOR('',#125432,1000.);
#28139=VECTOR('',#125435,1000.);
#28140=VECTOR('',#125436,1000.);
#28141=VECTOR('',#125445,1000.);
#28142=VECTOR('',#125448,1000.);
#28143=VECTOR('',#125451,1000.);
#28144=VECTOR('',#125452,1000.);
#28145=VECTOR('',#125461,1000.);
#28146=VECTOR('',#125464,1000.);
#28147=VECTOR('',#125467,1000.);
#28148=VECTOR('',#125468,1000.);
#28149=VECTOR('',#125473,1000.);
#28150=VECTOR('',#125476,1000.);
#28151=VECTOR('',#125481,1000.);
#28152=VECTOR('',#125484,1000.);
#28153=VECTOR('',#125489,1000.);
#28154=VECTOR('',#125492,1000.);
#28155=VECTOR('',#125493,1000.);
#28156=VECTOR('',#125494,1000.);
#28157=VECTOR('',#125495,1000.);
#28158=VECTOR('',#125498,1000.);
#28159=VECTOR('',#125501,1000.);
#28160=VECTOR('',#125502,1000.);
#28161=VECTOR('',#125503,1000.);
#28162=VECTOR('',#125504,1000.);
#28163=VECTOR('',#125505,1000.);
#28164=VECTOR('',#125506,1000.);
#28165=VECTOR('',#125509,1000.);
#28166=VECTOR('',#125510,1000.);
#28167=VECTOR('',#125511,1000.);
#28168=VECTOR('',#125512,1000.);
#28169=VECTOR('',#125513,1000.);
#28170=VECTOR('',#125516,1000.);
#28171=VECTOR('',#125523,1000.);
#28172=VECTOR('',#125528,1000.);
#28173=VECTOR('',#125533,1000.);
#28174=VECTOR('',#125538,1000.);
#28175=VECTOR('',#125545,1000.);
#28176=VECTOR('',#125554,1000.);
#28177=VECTOR('',#125559,1000.);
#28178=VECTOR('',#125562,1000.);
#28179=VECTOR('',#125569,1000.);
#28180=VECTOR('',#125572,1000.);
#28181=VECTOR('',#125579,1000.);
#28182=VECTOR('',#125636,1000.);
#28183=VECTOR('',#125637,1000.);
#28184=VECTOR('',#125640,1000.);
#28185=VECTOR('',#125643,1000.);
#28186=VECTOR('',#125646,1000.);
#28187=VECTOR('',#125649,1000.);
#28188=VECTOR('',#125706,1000.);
#28189=VECTOR('',#125707,1000.);
#28190=VECTOR('',#125710,1000.);
#28191=VECTOR('',#125713,1000.);
#28192=VECTOR('',#125716,1000.);
#28193=VECTOR('',#125719,1000.);
#28194=VECTOR('',#125724,1000.);
#28195=VECTOR('',#125725,1000.);
#28196=VECTOR('',#125728,1000.);
#28197=VECTOR('',#125731,1000.);
#28198=VECTOR('',#125734,1000.);
#28199=VECTOR('',#125737,1000.);
#28200=VECTOR('',#125742,2.);
#28201=VECTOR('',#125785,3.25);
#28202=VECTOR('',#125792,1000.);
#28203=VECTOR('',#125795,1000.);
#28204=VECTOR('',#125810,1000.);
#28205=VECTOR('',#125813,1000.);
#28206=VECTOR('',#125872,1000.);
#28207=VECTOR('',#125875,1000.);
#28208=VECTOR('',#125880,1000.);
#28209=VECTOR('',#125881,1000.);
#28210=VECTOR('',#125884,1000.);
#28211=VECTOR('',#125885,1000.);
#28212=VECTOR('',#125888,1000.);
#28213=VECTOR('',#125889,1000.);
#28214=VECTOR('',#125892,1000.);
#28215=VECTOR('',#125893,1000.);
#28216=VECTOR('',#125894,1000.);
#28217=VECTOR('',#125895,1000.);
#28218=VECTOR('',#125896,1000.);
#28219=VECTOR('',#125897,1000.);
#28220=VECTOR('',#125900,1000.);
#28221=VECTOR('',#125911,1000.);
#28222=VECTOR('',#125924,1000.);
#28223=VECTOR('',#125925,1000.);
#28224=VECTOR('',#125984,1000.);
#28225=VECTOR('',#125987,1000.);
#28226=VECTOR('',#125992,1000.);
#28227=VECTOR('',#125993,1000.);
#28228=VECTOR('',#125996,1000.);
#28229=VECTOR('',#125997,1000.);
#28230=VECTOR('',#126000,1000.);
#28231=VECTOR('',#126001,1000.);
#28232=VECTOR('',#126004,1000.);
#28233=VECTOR('',#126005,1000.);
#28234=VECTOR('',#126008,1000.);
#28235=VECTOR('',#126009,1000.);
#28236=VECTOR('',#126012,1000.);
#28237=VECTOR('',#126013,1000.);
#28238=VECTOR('',#126014,1000.);
#28239=VECTOR('',#126015,1000.);
#28240=VECTOR('',#126016,1000.);
#28241=VECTOR('',#126017,1000.);
#28242=VECTOR('',#126022,1000.);
#28243=VECTOR('',#126029,1000.);
#28244=VECTOR('',#126040,1000.);
#28245=VECTOR('',#126041,1000.);
#28246=VECTOR('',#126046,1000.);
#28247=VECTOR('',#126057,1000.);
#28248=VECTOR('',#126058,1000.);
#28249=VECTOR('',#126063,1000.);
#28250=VECTOR('',#126068,1000.);
#28251=VECTOR('',#126071,1000.);
#28252=VECTOR('',#126076,1000.);
#28253=VECTOR('',#126081,1000.);
#28254=VECTOR('',#126086,1000.);
#28255=VECTOR('',#126091,1000.);
#28256=VECTOR('',#126102,1000.);
#28257=VECTOR('',#126103,1000.);
#28258=VECTOR('',#126108,1000.);
#28259=VECTOR('',#126119,1000.);
#28260=VECTOR('',#126120,1000.);
#28261=VECTOR('',#126123,1000.);
#28262=VECTOR('',#126124,1000.);
#28263=VECTOR('',#126127,1000.);
#28264=VECTOR('',#126130,1000.);
#28265=VECTOR('',#126137,2.);
#28266=VECTOR('',#126142,2.);
#28267=VECTOR('',#126145,2.);
#28268=VECTOR('',#126148,2.);
#28269=VECTOR('',#126151,2.);
#28270=VECTOR('',#126154,2.);
#28271=VECTOR('',#126157,2.);
#28272=VECTOR('',#126160,2.);
#28273=VECTOR('',#126163,2.);
#28274=VECTOR('',#126166,2.);
#28275=VECTOR('',#126169,2.);
#28276=VECTOR('',#126172,2.);
#28277=VECTOR('',#126175,2.);
#28278=VECTOR('',#126178,2.);
#28279=VECTOR('',#126181,2.);
#28280=VECTOR('',#126184,2.);
#28281=VECTOR('',#126187,2.);
#28282=VECTOR('',#126190,2.);
#28283=VECTOR('',#126193,2.);
#28284=VECTOR('',#126196,2.);
#28285=VECTOR('',#126201,2.);
#28286=VECTOR('',#126204,2.);
#28287=VECTOR('',#126207,2.);
#28288=VECTOR('',#126210,2.);
#28289=VECTOR('',#126213,2.);
#28290=VECTOR('',#126216,2.);
#28291=VECTOR('',#126219,2.);
#28292=VECTOR('',#126222,2.);
#28293=VECTOR('',#126225,2.);
#28294=VECTOR('',#126228,2.);
#28295=VECTOR('',#126231,2.);
#28296=VECTOR('',#126234,2.);
#28297=VECTOR('',#126237,2.);
#28298=VECTOR('',#126240,2.);
#28299=VECTOR('',#126243,2.);
#28300=VECTOR('',#126246,2.);
#28301=VECTOR('',#126249,2.);
#28302=VECTOR('',#126252,2.);
#28303=VECTOR('',#126255,1.66874528305244);
#28304=VECTOR('',#126258,1.66874528305244);
#28305=VECTOR('',#126261,1.66874528305244);
#28306=VECTOR('',#126264,1.66874528305244);
#28307=VECTOR('',#126267,1.66874528305244);
#28308=VECTOR('',#126270,1.66874528305244);
#28309=VECTOR('',#126273,1.66874528305244);
#28310=VECTOR('',#126276,1.66874528305244);
#28311=VECTOR('',#126279,1.66874528305244);
#28312=VECTOR('',#126282,1.66874528305244);
#28313=VECTOR('',#126285,1.66874528305244);
#28314=VECTOR('',#126288,1.66874528305244);
#28315=VECTOR('',#126291,1.66874528305244);
#28316=VECTOR('',#126294,1.66874528305244);
#28317=VECTOR('',#126297,1.66874528305244);
#28318=VECTOR('',#126300,1.66874528305244);
#28319=VECTOR('',#126303,1.66874528305244);
#28320=VECTOR('',#126306,1.66874528305244);
#28321=VECTOR('',#126309,1.66874528305244);
#28322=VECTOR('',#126314,2.);
#28323=VECTOR('',#126319,2.);
#28324=VECTOR('',#126322,2.);
#28325=VECTOR('',#126325,2.);
#28326=VECTOR('',#126328,2.);
#28327=VECTOR('',#126331,2.);
#28328=VECTOR('',#126334,2.);
#28329=VECTOR('',#126337,2.);
#28330=VECTOR('',#126340,2.);
#28331=VECTOR('',#126343,2.);
#28332=VECTOR('',#126346,2.);
#28333=VECTOR('',#126349,2.);
#28334=VECTOR('',#126352,2.);
#28335=VECTOR('',#126355,2.);
#28336=VECTOR('',#126358,2.);
#28337=VECTOR('',#126361,2.);
#28338=VECTOR('',#126364,2.);
#28339=VECTOR('',#126367,2.);
#28340=VECTOR('',#126372,1.66874528305248);
#28341=VECTOR('',#126375,1.66874528305248);
#28342=VECTOR('',#126378,1.66874528305248);
#28343=VECTOR('',#126381,1.66874528305248);
#28344=VECTOR('',#126384,1.66874528305248);
#28345=VECTOR('',#126387,1.66874528305248);
#28346=VECTOR('',#126390,1.66874528305248);
#28347=VECTOR('',#126393,1.66874528305248);
#28348=VECTOR('',#126396,1.66874528305248);
#28349=VECTOR('',#126399,1.66874528305248);
#28350=VECTOR('',#126402,1.66874528305248);
#28351=VECTOR('',#126405,1.66874528305248);
#28352=VECTOR('',#126408,1.66874528305248);
#28353=VECTOR('',#126411,1.66874528305248);
#28354=VECTOR('',#126414,1.66874528305248);
#28355=VECTOR('',#126417,1.66874528305248);
#28356=VECTOR('',#126420,1.66874528305248);
#28357=VECTOR('',#126423,1.66874528305248);
#28358=VECTOR('',#126426,1.66874528305248);
#28359=VECTOR('',#126431,2.);
#28360=VECTOR('',#126436,2.);
#28361=VECTOR('',#126439,2.);
#28362=VECTOR('',#126442,2.);
#28363=VECTOR('',#126445,2.);
#28364=VECTOR('',#126448,2.);
#28365=VECTOR('',#126451,2.);
#28366=VECTOR('',#126454,2.);
#28367=VECTOR('',#126457,2.);
#28368=VECTOR('',#126460,2.);
#28369=VECTOR('',#126463,2.);
#28370=VECTOR('',#126466,2.);
#28371=VECTOR('',#126469,2.);
#28372=VECTOR('',#126472,2.);
#28373=VECTOR('',#126475,2.);
#28374=VECTOR('',#126478,2.);
#28375=VECTOR('',#126481,2.);
#28376=VECTOR('',#126484,2.);
#28377=VECTOR('',#126487,2.);
#28378=VECTOR('',#126490,1.66874528305242);
#28379=VECTOR('',#126493,1.66874528305242);
#28380=VECTOR('',#126496,1.66874528305242);
#28381=VECTOR('',#126499,1.66874528305242);
#28382=VECTOR('',#126502,1.66874528305242);
#28383=VECTOR('',#126505,1.66874528305242);
#28384=VECTOR('',#126508,1.66874528305242);
#28385=VECTOR('',#126511,1.66874528305242);
#28386=VECTOR('',#126514,1.66874528305242);
#28387=VECTOR('',#126517,1.66874528305242);
#28388=VECTOR('',#126520,1.66874528305242);
#28389=VECTOR('',#126523,1.66874528305242);
#28390=VECTOR('',#126526,1.66874528305242);
#28391=VECTOR('',#126529,1.66874528305242);
#28392=VECTOR('',#126532,1.66874528305242);
#28393=VECTOR('',#126535,1.66874528305242);
#28394=VECTOR('',#126538,1.66874528305242);
#28395=VECTOR('',#126541,1.66874528305242);
#28396=VECTOR('',#126544,1.66874528305242);
#28397=VECTOR('',#126549,1.66874528305242);
#28398=VECTOR('',#126552,1.66874528305242);
#28399=VECTOR('',#126555,1.66874528305242);
#28400=VECTOR('',#126558,1.66874528305242);
#28401=VECTOR('',#126561,1.66874528305242);
#28402=VECTOR('',#126564,1.66874528305242);
#28403=VECTOR('',#126567,1.66874528305242);
#28404=VECTOR('',#126570,1.66874528305242);
#28405=VECTOR('',#126573,1.66874528305242);
#28406=VECTOR('',#126576,1.66874528305242);
#28407=VECTOR('',#126579,1.66874528305242);
#28408=VECTOR('',#126582,1.66874528305242);
#28409=VECTOR('',#126585,1.66874528305242);
#28410=VECTOR('',#126588,1.66874528305242);
#28411=VECTOR('',#126591,1.66874528305242);
#28412=VECTOR('',#126594,1.66874528305242);
#28413=VECTOR('',#126597,1.66874528305242);
#28414=VECTOR('',#126600,1.66874528305242);
#28415=VECTOR('',#126603,1.66874528305242);
#28416=VECTOR('',#126608,1000.);
#28417=VECTOR('',#126609,1000.);
#28418=VECTOR('',#126610,1000.);
#28419=VECTOR('',#126611,1000.);
#28420=VECTOR('',#126612,1000.);
#28421=VECTOR('',#126613,1000.);
#28422=VECTOR('',#126614,1000.);
#28423=VECTOR('',#126615,1000.);
#28424=VECTOR('',#126618,1000.);
#28425=VECTOR('',#126621,1000.);
#28426=VECTOR('',#126622,1000.);
#28427=VECTOR('',#126627,1000.);
#28428=VECTOR('',#126628,1000.);
#28429=VECTOR('',#126629,1000.);
#28430=VECTOR('',#126630,1000.);
#28431=VECTOR('',#126633,1000.);
#28432=VECTOR('',#126634,1000.);
#28433=VECTOR('',#126635,1000.);
#28434=VECTOR('',#126636,1000.);
#28435=VECTOR('',#126639,1000.);
#28436=VECTOR('',#126640,1000.);
#28437=VECTOR('',#126641,1000.);
#28438=VECTOR('',#126644,1000.);
#28439=VECTOR('',#126645,1000.);
#28440=VECTOR('',#126646,1000.);
#28441=VECTOR('',#126649,1000.);
#28442=VECTOR('',#126650,1000.);
#28443=VECTOR('',#126653,1000.);
#28444=VECTOR('',#126656,1000.);
#28445=VECTOR('',#126657,1000.);
#28446=VECTOR('',#126660,1000.);
#28447=VECTOR('',#126665,1000.);
#28448=VECTOR('',#126666,1000.);
#28449=VECTOR('',#126669,1000.);
#28450=VECTOR('',#126670,1000.);
#28451=VECTOR('',#126681,3.);
#28452=VECTOR('',#126686,6.);
#28453=VECTOR('',#126697,3.);
#28454=VECTOR('',#126702,6.);
#28455=VECTOR('',#126713,3.);
#28456=VECTOR('',#126718,6.);
#28457=VECTOR('',#126729,3.);
#28458=VECTOR('',#126736,6.00000000000001);
#28459=VECTOR('',#126773,1000.);
#28460=VECTOR('',#126774,1000.);
#28461=VECTOR('',#126777,1000.);
#28462=VECTOR('',#126780,1000.);
#28463=VECTOR('',#126783,1000.);
#28464=VECTOR('',#126786,1000.);
#28465=VECTOR('',#126791,3.);
#28466=VECTOR('',#126818,6.);
#28467=VECTOR('',#126823,7.);
#28468=VECTOR('',#126846,10.);
#28469=VECTOR('',#126847,10.);
#28470=VECTOR('',#126852,10.);
#28471=VECTOR('',#126861,1000.);
#28472=VECTOR('',#126862,1000.);
#28473=VECTOR('',#126873,1000.);
#28474=VECTOR('',#126874,1000.);
#28475=VECTOR('',#126897,1000.);
#28476=VECTOR('',#126898,1000.);
#28477=VECTOR('',#126903,1000.);
#28478=VECTOR('',#126920,1000.);
#28479=VECTOR('',#126921,1000.);
#28480=VECTOR('',#126926,1000.);
#28481=VECTOR('',#126941,1000.);
#28482=VECTOR('',#126944,1000.);
#28483=VECTOR('',#126947,1000.);
#28484=VECTOR('',#126950,1000.);
#28485=VECTOR('',#126953,1000.);
#28486=VECTOR('',#126956,1000.);
#28487=VECTOR('',#126963,1000.);
#28488=VECTOR('',#126966,1000.);
#28489=VECTOR('',#126969,1000.);
#28490=VECTOR('',#126972,1000.);
#28491=VECTOR('',#126975,1000.);
#28492=VECTOR('',#126992,1000.);
#28493=VECTOR('',#126999,1000.);
#28494=VECTOR('',#127002,1000.);
#28495=VECTOR('',#127005,1000.);
#28496=VECTOR('',#127008,1000.);
#28497=VECTOR('',#127011,1000.);
#28498=VECTOR('',#127012,1000.);
#28499=VECTOR('',#127029,1000.);
#28500=VECTOR('',#127044,1000.);
#28501=VECTOR('',#127045,1000.);
#28502=VECTOR('',#127050,1000.);
#28503=VECTOR('',#127051,1000.);
#28504=VECTOR('',#127056,1000.);
#28505=VECTOR('',#127057,1000.);
#28506=VECTOR('',#127062,1000.);
#28507=VECTOR('',#127063,1000.);
#28508=VECTOR('',#127078,1000.);
#28509=VECTOR('',#127079,1000.);
#28510=VECTOR('',#127084,1000.);
#28511=VECTOR('',#127085,1000.);
#28512=VECTOR('',#127090,1000.);
#28513=VECTOR('',#127107,1000.);
#28514=VECTOR('',#127124,1000.);
#28515=VECTOR('',#127125,1000.);
#28516=VECTOR('',#127130,1000.);
#28517=VECTOR('',#127131,1000.);
#28518=VECTOR('',#127136,1000.);
#28519=VECTOR('',#127153,1000.);
#28520=VECTOR('',#127196,1000.);
#28521=VECTOR('',#127211,10.);
#28522=VECTOR('',#127212,10.);
#28523=VECTOR('',#127215,10.);
#28524=VECTOR('',#127216,10.);
#28525=VECTOR('',#127223,10.);
#28526=VECTOR('',#127226,10.);
#28527=VECTOR('',#127227,10.);
#28528=VECTOR('',#127234,10.);
#28529=VECTOR('',#127237,10.);
#28530=VECTOR('',#127238,10.);
#28531=VECTOR('',#127245,10.);
#28532=VECTOR('',#127246,10.);
#28533=VECTOR('',#127249,10.);
#28534=VECTOR('',#127250,10.);
#28535=VECTOR('',#127265,10.);
#28536=VECTOR('',#127266,10.);
#28537=VECTOR('',#127271,1000.);
#28538=VECTOR('',#127272,1000.);
#29239=CIRCLE('',#94084,2.);
#29240=CIRCLE('',#94085,1.47499999999998);
#29241=CIRCLE('',#94088,2.);
#29242=CIRCLE('',#94090,2.5);
#29243=CIRCLE('',#94092,2.5);
#29244=CIRCLE('',#94095,2.);
#29245=CIRCLE('',#94096,1.47499999999998);
#29246=CIRCLE('',#94099,2.);
#29247=CIRCLE('',#94101,2.5);
#29248=CIRCLE('',#94103,2.5);
#29249=CIRCLE('',#94106,5.);
#29250=CIRCLE('',#94107,5.);
#29251=CIRCLE('',#94109,3.);
#29252=CIRCLE('',#94110,3.);
#29253=CIRCLE('',#94112,0.499999999999997);
#29254=CIRCLE('',#94113,0.499999999999997);
#29255=CIRCLE('',#94114,2.5);
#29256=CIRCLE('',#94115,0.499999999999999);
#29257=CIRCLE('',#94117,3.);
#29258=CIRCLE('',#94118,3.);
#29259=CIRCLE('',#94121,1.);
#29260=CIRCLE('',#94122,1.);
#29261=CIRCLE('',#94123,2.);
#29262=CIRCLE('',#94125,3.);
#29263=CIRCLE('',#94126,3.);
#29264=CIRCLE('',#94129,0.999999999999996);
#29265=CIRCLE('',#94130,1.);
#29266=CIRCLE('',#94131,2.);
#29267=CIRCLE('',#94134,0.5);
#29268=CIRCLE('',#94135,0.500000000000004);
#29269=CIRCLE('',#94137,0.5);
#29270=CIRCLE('',#94139,58.2938077870648);
#29271=CIRCLE('',#94140,0.999575812491136);
#29272=CIRCLE('',#94141,58.3875000000282);
#29273=CIRCLE('',#94144,0.5);
#29274=CIRCLE('',#94145,0.5);
#29275=CIRCLE('',#94146,0.5);
#29276=CIRCLE('',#94147,0.5);
#29277=CIRCLE('',#94148,0.499999999999999);
#29278=CIRCLE('',#94149,57.7596339908719);
#29279=CIRCLE('',#94150,0.499999999999994);
#29280=CIRCLE('',#94151,67.9400604629212);
#29281=CIRCLE('',#94152,0.5);
#29282=CIRCLE('',#94154,0.5);
#29283=CIRCLE('',#94156,58.2938077870648);
#29284=CIRCLE('',#94158,58.3875000000282);
#29285=CIRCLE('',#94161,0.5);
#29286=CIRCLE('',#94162,0.5);
#29287=CIRCLE('',#94163,0.5);
#29288=CIRCLE('',#94164,0.499999999999998);
#29289=CIRCLE('',#94166,58.3875000000282);
#29290=CIRCLE('',#94167,0.499999999999999);
#29291=CIRCLE('',#94168,58.8875000000282);
#29292=CIRCLE('',#94169,0.5);
#29293=CIRCLE('',#94171,0.5);
#29294=CIRCLE('',#94173,58.2938077870648);
#29295=CIRCLE('',#94175,58.3875000000282);
#29296=CIRCLE('',#94178,0.5);
#29297=CIRCLE('',#94179,0.5);
#29298=CIRCLE('',#94180,0.499999999999997);
#29299=CIRCLE('',#94182,58.3875000000282);
#29300=CIRCLE('',#94183,58.8875000000282);
#29301=CIRCLE('',#94185,5.);
#29302=CIRCLE('',#94187,58.2060351304332);
#29303=CIRCLE('',#94188,0.999999999999997);
#29304=CIRCLE('',#94189,58.3875000000282);
#29305=CIRCLE('',#94191,0.5);
#29306=CIRCLE('',#94192,0.5);
#29307=CIRCLE('',#94193,0.499999999999999);
#29308=CIRCLE('',#94195,0.5);
#29309=CIRCLE('',#94196,58.8875000000282);
#29310=CIRCLE('',#94197,58.3875000000282);
#29311=CIRCLE('',#94198,0.5);
#29312=CIRCLE('',#94200,0.5);
#29313=CIRCLE('',#94202,58.2938077870648);
#29314=CIRCLE('',#94204,58.3875000000282);
#29315=CIRCLE('',#94207,0.5);
#29316=CIRCLE('',#94208,0.5);
#29317=CIRCLE('',#94209,0.499999999999999);
#29318=CIRCLE('',#94210,0.500000000000003);
#29319=CIRCLE('',#94211,64.7291249062775);
#29320=CIRCLE('',#94212,56.5371804123853);
#29321=CIRCLE('',#94213,0.5);
#29322=CIRCLE('',#94215,0.5);
#29323=CIRCLE('',#94217,58.2938077870648);
#29324=CIRCLE('',#94219,58.3875000000282);
#29325=CIRCLE('',#94220,0.991843022345032);
#29326=CIRCLE('',#94222,0.5);
#29327=CIRCLE('',#94223,0.5);
#29328=CIRCLE('',#94224,0.5);
#29329=CIRCLE('',#94225,0.500000000000002);
#29330=CIRCLE('',#94226,68.2241973717388);
#29331=CIRCLE('',#94227,57.986356128794);
#29332=CIRCLE('',#94228,0.5);
#29333=CIRCLE('',#94230,0.5);
#29334=CIRCLE('',#94231,0.500000000000004);
#29335=CIRCLE('',#94232,0.499999999999998);
#29336=CIRCLE('',#94234,0.500000000000002);
#29337=CIRCLE('',#94235,4.5);
#29338=CIRCLE('',#94236,0.5);
#29339=CIRCLE('',#94238,5.);
#29340=CIRCLE('',#94239,5.);
#29341=CIRCLE('',#94240,1.41062672174051);
#29342=CIRCLE('',#94242,58.3875000000282);
#29343=CIRCLE('',#94243,58.3875000000282);
#29344=CIRCLE('',#94244,58.3875000000282);
#29345=CIRCLE('',#94245,58.3875000000282);
#29346=CIRCLE('',#94246,57.8151740222928);
#29347=CIRCLE('',#94247,58.3875000000282);
#29348=CIRCLE('',#94248,57.9944820942039);
#29349=CIRCLE('',#94249,58.3875000000282);
#29350=CIRCLE('',#94250,57.7939200862669);
#29351=CIRCLE('',#94251,58.3875000000282);
#29352=CIRCLE('',#94252,58.3875000000282);
#29353=CIRCLE('',#94253,58.3875000000282);
#29354=CIRCLE('',#94254,0.500000000000002);
#29355=CIRCLE('',#94255,0.499999999999999);
#29356=CIRCLE('',#94257,0.500000000000002);
#29357=CIRCLE('',#94258,4.5);
#29358=CIRCLE('',#94259,0.5);
#29359=CIRCLE('',#94261,3.);
#29360=CIRCLE('',#94262,3.);
#29361=CIRCLE('',#94266,0.999999999999997);
#29362=CIRCLE('',#94267,1.);
#29363=CIRCLE('',#94268,2.);
#29364=CIRCLE('',#94270,3.);
#29365=CIRCLE('',#94271,3.);
#29366=CIRCLE('',#94274,0.999999999999996);
#29367=CIRCLE('',#94275,0.999999999999997);
#29368=CIRCLE('',#94276,2.);
#29369=CIRCLE('',#94278,0.5);
#29370=CIRCLE('',#94280,0.5);
#29371=CIRCLE('',#94282,58.2938077870648);
#29372=CIRCLE('',#94286,0.5);
#29373=CIRCLE('',#94287,0.5);
#29374=CIRCLE('',#94288,0.499999999999999);
#29375=CIRCLE('',#94290,0.500000000000001);
#29376=CIRCLE('',#94291,58.8875000000282);
#29377=CIRCLE('',#94292,0.5);
#29378=CIRCLE('',#94294,0.5);
#29379=CIRCLE('',#94296,58.2938077870648);
#29380=CIRCLE('',#94300,0.5);
#29381=CIRCLE('',#94301,0.5);
#29382=CIRCLE('',#94302,0.500000000000001);
#29383=CIRCLE('',#94303,0.499999999999998);
#29384=CIRCLE('',#94304,67.9880753527063);
#29385=CIRCLE('',#94305,0.5);
#29386=CIRCLE('',#94307,0.5);
#29387=CIRCLE('',#94309,58.2938077870648);
#29388=CIRCLE('',#94311,0.999496026332483);
#29389=CIRCLE('',#94313,0.5);
#29390=CIRCLE('',#94314,0.5);
#29391=CIRCLE('',#94315,0.499999999999998);
#29392=CIRCLE('',#94316,0.499999999999999);
#29393=CIRCLE('',#94317,68.156308837608);
#29394=CIRCLE('',#94318,0.5);
#29395=CIRCLE('',#94320,0.5);
#29396=CIRCLE('',#94322,58.2938077870648);
#29397=CIRCLE('',#94323,0.999648707757584);
#29398=CIRCLE('',#94326,0.5);
#29399=CIRCLE('',#94327,0.5);
#29400=CIRCLE('',#94328,0.499999999999997);
#29401=CIRCLE('',#94329,0.500000000000001);
#29402=CIRCLE('',#94330,68.0319603210185);
#29403=CIRCLE('',#94331,0.5);
#29404=CIRCLE('',#94333,0.5);
#29405=CIRCLE('',#94335,58.2938077870648);
#29406=CIRCLE('',#94339,0.5);
#29407=CIRCLE('',#94340,0.5);
#29408=CIRCLE('',#94341,0.500000000000001);
#29409=CIRCLE('',#94343,0.499999999999998);
#29410=CIRCLE('',#94344,58.8875000000282);
#29411=CIRCLE('',#94345,0.5);
#29412=CIRCLE('',#94347,0.5);
#29413=CIRCLE('',#94349,58.2938077870648);
#29414=CIRCLE('',#94353,0.5);
#29415=CIRCLE('',#94354,0.5);
#29416=CIRCLE('',#94357,0.5);
#29417=CIRCLE('',#94358,0.5);
#29418=CIRCLE('',#94359,0.500000000000005);
#29419=CIRCLE('',#94361,0.500000000000005);
#29420=CIRCLE('',#94362,0.5);
#29421=CIRCLE('',#94364,0.5);
#29422=CIRCLE('',#94366,0.5);
#29423=CIRCLE('',#94368,0.5);
#29424=CIRCLE('',#94369,0.999999999999996);
#29425=CIRCLE('',#94372,0.5);
#29426=CIRCLE('',#94373,0.5);
#29427=CIRCLE('',#94374,0.500000000000005);
#29428=CIRCLE('',#94376,0.500000000000005);
#29429=CIRCLE('',#94377,0.5);
#29430=CIRCLE('',#94379,0.5);
#29431=CIRCLE('',#94381,1.);
#29432=CIRCLE('',#94384,0.5);
#29433=CIRCLE('',#94385,0.5);
#29434=CIRCLE('',#94386,0.499999999999999);
#29435=CIRCLE('',#94388,0.499999999999999);
#29436=CIRCLE('',#94389,0.5);
#29437=CIRCLE('',#94391,0.5);
#29438=CIRCLE('',#94394,0.5);
#29439=CIRCLE('',#94395,0.5);
#29440=CIRCLE('',#94396,0.499999999999999);
#29441=CIRCLE('',#94398,0.499999999999999);
#29442=CIRCLE('',#94399,0.5);
#29443=CIRCLE('',#94401,0.5);
#29444=CIRCLE('',#94405,0.5);
#29445=CIRCLE('',#94406,0.5);
#29446=CIRCLE('',#94407,0.499999999999999);
#29447=CIRCLE('',#94409,0.499999999999999);
#29448=CIRCLE('',#94410,0.5);
#29449=CIRCLE('',#94412,0.5);
#29450=CIRCLE('',#94414,0.5);
#29451=CIRCLE('',#94417,0.5);
#29452=CIRCLE('',#94418,0.999999999999998);
#29453=CIRCLE('',#94419,1.);
#29454=CIRCLE('',#94422,0.5);
#29455=CIRCLE('',#94423,0.5);
#29456=CIRCLE('',#94424,0.499999999999999);
#29457=CIRCLE('',#94426,0.499999999999999);
#29458=CIRCLE('',#94427,0.5);
#29459=CIRCLE('',#94429,0.5);
#29460=CIRCLE('',#94430,1.);
#29461=CIRCLE('',#94432,0.5);
#29462=CIRCLE('',#94433,0.5);
#29463=CIRCLE('',#94437,0.5);
#29464=CIRCLE('',#94438,0.5);
#29465=CIRCLE('',#94439,0.499999999999998);
#29466=CIRCLE('',#94441,0.499999999999998);
#29467=CIRCLE('',#94442,0.5);
#29468=CIRCLE('',#94444,0.5);
#29469=CIRCLE('',#94447,0.5);
#29470=CIRCLE('',#94448,0.5);
#29471=CIRCLE('',#94449,0.499999999999998);
#29472=CIRCLE('',#94451,0.499999999999998);
#29473=CIRCLE('',#94452,0.5);
#29474=CIRCLE('',#94453,0.5);
#29475=CIRCLE('',#94455,0.5);
#29476=CIRCLE('',#94456,0.5);
#29477=CIRCLE('',#94459,0.5);
#29478=CIRCLE('',#94460,59.);
#29479=CIRCLE('',#94461,0.5);
#29480=CIRCLE('',#94462,2.75);
#29481=CIRCLE('',#94464,2.75);
#29482=CIRCLE('',#94465,2.75);
#29483=CIRCLE('',#94468,0.5);
#29484=CIRCLE('',#94469,0.499999999999999);
#29485=CIRCLE('',#94472,0.500000000000001);
#29486=CIRCLE('',#94473,0.5);
#29487=CIRCLE('',#94475,0.5);
#29488=CIRCLE('',#94476,1.);
#29489=CIRCLE('',#94477,0.5);
#29490=CIRCLE('',#94478,0.5);
#29491=CIRCLE('',#94480,0.5);
#29492=CIRCLE('',#94482,3.);
#29493=CIRCLE('',#94483,3.);
#29494=CIRCLE('',#94485,0.5);
#29495=CIRCLE('',#94487,1.);
#29496=CIRCLE('',#94488,0.5);
#29497=CIRCLE('',#94489,0.5);
#29498=CIRCLE('',#94491,0.5);
#29499=CIRCLE('',#94493,1.);
#29500=CIRCLE('',#94494,0.5);
#29501=CIRCLE('',#94495,0.5);
#29502=CIRCLE('',#94497,0.5);
#29503=CIRCLE('',#94500,44.2689250265968);
#29504=CIRCLE('',#94502,45.1752328136335);
#29505=CIRCLE('',#94504,0.5);
#29506=CIRCLE('',#94505,0.5);
#29507=CIRCLE('',#94507,1.);
#29508=CIRCLE('',#94508,0.5);
#29509=CIRCLE('',#94509,0.5);
#29510=CIRCLE('',#94511,0.5);
#29511=CIRCLE('',#94513,0.999999999999999);
#29512=CIRCLE('',#94514,0.5);
#29513=CIRCLE('',#94515,0.5);
#29514=CIRCLE('',#94517,0.5);
#29515=CIRCLE('',#94519,45.1752328136335);
#29516=CIRCLE('',#94520,1.);
#29517=CIRCLE('',#94521,1.02387173403494);
#29518=CIRCLE('',#94522,1.);
#29519=CIRCLE('',#94524,1.);
#29520=CIRCLE('',#94526,0.5);
#29521=CIRCLE('',#94527,0.5);
#29522=CIRCLE('',#94529,1.);
#29523=CIRCLE('',#94530,0.5);
#29524=CIRCLE('',#94531,0.5);
#29525=CIRCLE('',#94533,0.5);
#29526=CIRCLE('',#94535,1.);
#29527=CIRCLE('',#94536,0.5);
#29528=CIRCLE('',#94537,0.5);
#29529=CIRCLE('',#94539,0.5);
#29530=CIRCLE('',#94541,1.);
#29531=CIRCLE('',#94542,1.);
#29532=CIRCLE('',#94544,0.5);
#29533=CIRCLE('',#94545,0.5);
#29534=CIRCLE('',#94547,1.);
#29535=CIRCLE('',#94548,0.5);
#29536=CIRCLE('',#94549,0.5);
#29537=CIRCLE('',#94551,0.5);
#29538=CIRCLE('',#94553,1.);
#29539=CIRCLE('',#94554,0.5);
#29540=CIRCLE('',#94555,0.5);
#29541=CIRCLE('',#94557,0.5);
#29542=CIRCLE('',#94559,1.);
#29543=CIRCLE('',#94560,1.);
#29544=CIRCLE('',#94562,0.5);
#29545=CIRCLE('',#94565,3.);
#29546=CIRCLE('',#94567,0.5);
#29547=CIRCLE('',#94568,4.5);
#29548=CIRCLE('',#94569,0.500000000000003);
#29549=CIRCLE('',#94570,5.);
#29550=CIRCLE('',#94572,0.499999999999999);
#29551=CIRCLE('',#94574,5.);
#29552=CIRCLE('',#94576,0.250000000000003);
#29553=CIRCLE('',#94577,0.249999999999998);
#29554=CIRCLE('',#94578,5.25);
#29555=CIRCLE('',#94580,0.250000000000003);
#29556=CIRCLE('',#94582,0.250000000000003);
#29557=CIRCLE('',#94583,3.);
#29558=CIRCLE('',#94584,2.75);
#29559=CIRCLE('',#94586,0.250000000000003);
#29560=CIRCLE('',#94587,67.5);
#29561=CIRCLE('',#94588,67.25);
#29562=CIRCLE('',#94590,0.249999999999997);
#29563=CIRCLE('',#94591,3.);
#29564=CIRCLE('',#94592,2.75);
#29565=CIRCLE('',#94594,0.249999999999997);
#29566=CIRCLE('',#94596,0.249999999999997);
#29567=CIRCLE('',#94597,5.);
#29568=CIRCLE('',#94598,5.25);
#29569=CIRCLE('',#94600,0.249999999999997);
#29570=CIRCLE('',#94601,58.5);
#29571=CIRCLE('',#94602,58.25);
#29572=CIRCLE('',#94604,0.249999999999997);
#29573=CIRCLE('',#94605,5.);
#29574=CIRCLE('',#94606,5.25);
#29575=CIRCLE('',#94608,0.250000000000003);
#29576=CIRCLE('',#94610,0.250000000000003);
#29577=CIRCLE('',#94611,3.);
#29578=CIRCLE('',#94612,2.75);
#29579=CIRCLE('',#94614,0.250000000000003);
#29580=CIRCLE('',#94615,67.5);
#29581=CIRCLE('',#94616,67.25);
#29582=CIRCLE('',#94618,0.250000000000003);
#29583=CIRCLE('',#94619,3.);
#29584=CIRCLE('',#94620,2.75);
#29585=CIRCLE('',#94622,0.250000000000003);
#29586=CIRCLE('',#94624,0.250000000000002);
#29587=CIRCLE('',#94625,3.);
#29588=CIRCLE('',#94626,3.25);
#29589=CIRCLE('',#94628,2.75);
#29590=CIRCLE('',#94629,2.75);
#29591=CIRCLE('',#94630,2.75);
#29592=CIRCLE('',#94631,2.75);
#29593=CIRCLE('',#94633,2.75);
#29594=CIRCLE('',#94634,2.75);
#29595=CIRCLE('',#94635,2.75);
#29596=CIRCLE('',#94636,0.5);
#29597=CIRCLE('',#94637,0.500000000000001);
#29598=CIRCLE('',#94639,0.5);
#29599=CIRCLE('',#94641,58.5);
#29600=CIRCLE('',#94643,58.4063077870367);
#29601=CIRCLE('',#94646,0.5);
#29602=CIRCLE('',#94647,0.5);
#29603=CIRCLE('',#94648,0.500000000000002);
#29604=CIRCLE('',#94650,0.500000000000005);
#29605=CIRCLE('',#94651,59.);
#29606=CIRCLE('',#94652,58.5);
#29607=CIRCLE('',#94653,0.5);
#29608=CIRCLE('',#94655,0.5);
#29609=CIRCLE('',#94657,58.5);
#29610=CIRCLE('',#94659,58.4063077870367);
#29611=CIRCLE('',#94662,0.5);
#29612=CIRCLE('',#94663,0.5);
#29613=CIRCLE('',#94664,0.499999999999999);
#29614=CIRCLE('',#94665,0.500000000000005);
#29615=CIRCLE('',#94666,68.1417998565621);
#29616=CIRCLE('',#94667,57.9169670944157);
#29617=CIRCLE('',#94668,0.5);
#29618=CIRCLE('',#94670,0.5);
#29619=CIRCLE('',#94672,58.5);
#29620=CIRCLE('',#94673,0.999577393236284);
#29621=CIRCLE('',#94674,58.4063077870366);
#29622=CIRCLE('',#94677,0.5);
#29623=CIRCLE('',#94678,0.5);
#29624=CIRCLE('',#94679,0.500000000000002);
#29625=CIRCLE('',#94681,0.499999999999999);
#29626=CIRCLE('',#94682,0.499999999999998);
#29627=CIRCLE('',#94684,59.);
#29628=CIRCLE('',#94685,58.5);
#29629=CIRCLE('',#94686,0.5);
#29630=CIRCLE('',#94688,0.5);
#29631=CIRCLE('',#94689,0.499999999999994);
#29632=CIRCLE('',#94696,0.499999999999998);
#29633=CIRCLE('',#94700,0.5);
#29634=CIRCLE('',#94701,0.5);
#29635=CIRCLE('',#94702,0.500000000000005);
#29636=CIRCLE('',#94707,0.500000000000001);
#29637=CIRCLE('',#94710,2.5);
#29638=CIRCLE('',#94711,2.5);
#29639=CIRCLE('',#94714,0.5);
#29640=CIRCLE('',#94717,0.5);
#29641=CIRCLE('',#94718,0.499999999999997);
#29642=CIRCLE('',#94721,2.5);
#29643=CIRCLE('',#94722,2.5);
#29644=CIRCLE('',#94725,0.499999999999998);
#29645=CIRCLE('',#94728,2.5);
#29646=CIRCLE('',#94729,2.5);
#29647=CIRCLE('',#94732,0.5);
#29648=CIRCLE('',#94734,58.1182624738004);
#29649=CIRCLE('',#94735,0.99506488582092);
#29650=CIRCLE('',#94737,0.500000000000003);
#29651=CIRCLE('',#94739,2.5);
#29652=CIRCLE('',#94740,0.5);
#29653=CIRCLE('',#94741,0.491297296893067);
#29654=CIRCLE('',#94743,0.5);
#29655=CIRCLE('',#94746,0.5);
#29656=CIRCLE('',#94749,0.5);
#29657=CIRCLE('',#94750,2.5);
#29658=CIRCLE('',#94751,0.500000000000001);
#29659=CIRCLE('',#94754,0.499999999999999);
#29660=CIRCLE('',#94756,0.551233577645565);
#29661=CIRCLE('',#94757,0.5);
#29662=CIRCLE('',#94758,64.5806717409052);
#29663=CIRCLE('',#94759,0.5);
#29664=CIRCLE('',#94760,0.500000000000002);
#29665=CIRCLE('',#94765,0.500000000000001);
#29666=CIRCLE('',#94767,0.5);
#29667=CIRCLE('',#94768,0.5);
#29668=CIRCLE('',#94771,0.5);
#29669=CIRCLE('',#94774,0.5);
#29670=CIRCLE('',#94776,0.5);
#29671=CIRCLE('',#94779,0.5);
#29672=CIRCLE('',#94781,2.5);
#29673=CIRCLE('',#94782,2.5);
#29674=CIRCLE('',#94785,0.499999999999998);
#29675=CIRCLE('',#94788,0.499999999999997);
#29676=CIRCLE('',#94790,2.5);
#29677=CIRCLE('',#94791,2.5);
#29678=CIRCLE('',#94794,0.5);
#29679=CIRCLE('',#94797,0.5);
#29680=CIRCLE('',#94798,0.5);
#29681=CIRCLE('',#94802,2.5);
#29682=CIRCLE('',#94803,2.5);
#29683=CIRCLE('',#94805,0.499999999999998);
#29684=CIRCLE('',#94809,0.5);
#29685=CIRCLE('',#94810,0.5);
#29686=CIRCLE('',#94811,0.499999999999998);
#29687=CIRCLE('',#94816,0.500000000000002);
#29688=CIRCLE('',#94822,0.5);
#29689=CIRCLE('',#94823,109.36143880173);
#29690=CIRCLE('',#94824,0.5);
#29691=CIRCLE('',#94825,0.5);
#29692=CIRCLE('',#94832,0.5);
#29693=CIRCLE('',#94836,0.5);
#29694=CIRCLE('',#94837,0.5);
#29695=CIRCLE('',#94838,0.500000000000001);
#29696=CIRCLE('',#94844,0.500000000000003);
#29697=CIRCLE('',#94846,2.5);
#29698=CIRCLE('',#94847,2.5);
#29699=CIRCLE('',#94850,0.5);
#29700=CIRCLE('',#94853,0.5);
#29701=CIRCLE('',#94854,0.499999999999999);
#29702=CIRCLE('',#94858,2.5);
#29703=CIRCLE('',#94859,2.5);
#29704=CIRCLE('',#94862,0.499999999999999);
#29705=CIRCLE('',#94865,2.5);
#29706=CIRCLE('',#94866,2.5);
#29707=CIRCLE('',#94868,59.024570260837);
#29708=CIRCLE('',#94869,0.5);
#29709=CIRCLE('',#94870,0.5);
#29710=CIRCLE('',#94872,2.5);
#29711=CIRCLE('',#94873,2.5);
#29712=CIRCLE('',#94875,0.5);
#29713=CIRCLE('',#94878,0.5);
#29714=CIRCLE('',#94880,2.5);
#29715=CIRCLE('',#94881,2.5);
#29716=CIRCLE('',#94882,0.5);
#29717=CIRCLE('',#94883,0.5);
#29718=CIRCLE('',#94885,2.5);
#29719=CIRCLE('',#94886,2.5);
#29720=CIRCLE('',#94889,58.1182624738004);
#29721=CIRCLE('',#94891,59.024570260837);
#29722=CIRCLE('',#94893,0.5);
#29723=CIRCLE('',#94895,2.5);
#29724=CIRCLE('',#94896,2.5);
#29725=CIRCLE('',#94898,0.5);
#29726=CIRCLE('',#94901,0.5);
#29727=CIRCLE('',#94903,2.5);
#29728=CIRCLE('',#94904,2.5);
#29729=CIRCLE('',#94906,59.024570260837);
#29730=CIRCLE('',#94907,0.5);
#29731=CIRCLE('',#94908,0.5);
#29732=CIRCLE('',#94910,2.5);
#29733=CIRCLE('',#94911,0.5);
#29734=CIRCLE('',#94913,0.5);
#29735=CIRCLE('',#94916,0.5);
#29736=CIRCLE('',#94918,0.5);
#29737=CIRCLE('',#94919,2.5);
#29738=CIRCLE('',#94920,0.499999999999997);
#29739=CIRCLE('',#94921,0.5);
#29740=CIRCLE('',#94923,2.5);
#29741=CIRCLE('',#94925,0.5);
#29742=CIRCLE('',#94928,0.5);
#29743=CIRCLE('',#94930,2.5);
#29744=CIRCLE('',#94931,0.5);
#29745=CIRCLE('',#94933,59.024570260837);
#29746=CIRCLE('',#94934,0.5);
#29747=CIRCLE('',#94935,0.5);
#29748=CIRCLE('',#94937,2.5);
#29749=CIRCLE('',#94938,2.5);
#29750=CIRCLE('',#94940,0.5);
#29751=CIRCLE('',#94943,0.5);
#29752=CIRCLE('',#94944,0.5);
#29753=CIRCLE('',#94946,2.5);
#29754=CIRCLE('',#94947,2.5);
#29755=CIRCLE('',#94948,3.5);
#29756=CIRCLE('',#94950,2.5);
#29757=CIRCLE('',#94951,2.5);
#29758=CIRCLE('',#94955,0.5);
#29759=CIRCLE('',#94957,58.1182624738004);
#29760=CIRCLE('',#94959,59.024570260837);
#29761=CIRCLE('',#94961,0.5);
#29762=CIRCLE('',#94963,2.5);
#29763=CIRCLE('',#94964,2.5);
#29764=CIRCLE('',#94966,0.5);
#29765=CIRCLE('',#94969,0.5);
#29766=CIRCLE('',#94971,2.5);
#29767=CIRCLE('',#94972,2.5);
#29768=CIRCLE('',#94974,58.1182624738004);
#29769=CIRCLE('',#94975,59.024570260837);
#29770=CIRCLE('',#94977,0.499999999999998);
#29771=CIRCLE('',#94980,2.5);
#29772=CIRCLE('',#94981,2.5);
#29773=CIRCLE('',#94982,0.5);
#29774=CIRCLE('',#94984,2.5);
#29775=CIRCLE('',#94985,2.5);
#29776=CIRCLE('',#94987,0.5);
#29777=CIRCLE('',#94990,0.5);
#29778=CIRCLE('',#94992,2.5);
#29779=CIRCLE('',#94993,2.5);
#29780=CIRCLE('',#94994,0.5);
#29781=CIRCLE('',#94996,59.024570260837);
#29782=CIRCLE('',#94997,0.5);
#29783=CIRCLE('',#94999,2.5);
#29784=CIRCLE('',#95000,2.5);
#29785=CIRCLE('',#95002,0.5);
#29786=CIRCLE('',#95005,0.5);
#29787=CIRCLE('',#95006,0.5);
#29788=CIRCLE('',#95008,2.5);
#29789=CIRCLE('',#95009,2.5);
#29790=CIRCLE('',#95012,0.5);
#29791=CIRCLE('',#95014,2.);
#29792=CIRCLE('',#95015,2.);
#29793=CIRCLE('',#95017,2.75);
#29794=CIRCLE('',#95020,0.5);
#29795=CIRCLE('',#95021,0.5);
#29796=CIRCLE('',#95022,0.5);
#29797=CIRCLE('',#95023,1.);
#29798=CIRCLE('',#95025,0.500000000000002);
#29799=CIRCLE('',#95026,58.5);
#29800=CIRCLE('',#95027,0.5);
#29801=CIRCLE('',#95028,1.);
#29802=CIRCLE('',#95031,0.5);
#29803=CIRCLE('',#95033,2.);
#29804=CIRCLE('',#95034,2.);
#29805=CIRCLE('',#95036,2.75);
#29806=CIRCLE('',#95038,2.75);
#29807=CIRCLE('',#95040,0.5);
#29808=CIRCLE('',#95042,3.);
#29809=CIRCLE('',#95043,3.);
#29810=CIRCLE('',#95045,0.5);
#29811=CIRCLE('',#95047,0.5);
#29812=CIRCLE('',#95049,0.5);
#29813=CIRCLE('',#95050,0.500000000000001);
#29814=CIRCLE('',#95051,0.500000000000002);
#29815=CIRCLE('',#95053,0.5);
#29816=CIRCLE('',#95055,0.5);
#29817=CIRCLE('',#95056,0.5);
#29818=CIRCLE('',#95060,0.500000000000001);
#29819=CIRCLE('',#95061,0.5);
#29820=CIRCLE('',#95065,0.499999999999998);
#29821=CIRCLE('',#95066,0.499999999999999);
#29822=CIRCLE('',#95070,0.5);
#29823=CIRCLE('',#95072,0.5);
#29824=CIRCLE('',#95075,0.5);
#29825=CIRCLE('',#95076,0.5);
#29826=CIRCLE('',#95078,0.5);
#29827=CIRCLE('',#95080,0.5);
#29828=CIRCLE('',#95083,0.5);
#29829=CIRCLE('',#95084,0.5);
#29830=CIRCLE('',#95086,0.5);
#29831=CIRCLE('',#95088,0.5);
#29832=CIRCLE('',#95090,0.5);
#29833=CIRCLE('',#95091,0.5);
#29834=CIRCLE('',#95092,0.5);
#29835=CIRCLE('',#95094,0.5);
#29836=CIRCLE('',#95095,0.5);
#29837=CIRCLE('',#95097,0.5);
#29838=CIRCLE('',#95100,3.);
#29839=CIRCLE('',#95102,67.5);
#29840=CIRCLE('',#95104,3.);
#29841=CIRCLE('',#95109,58.5);
#29842=CIRCLE('',#95110,58.5);
#29843=CIRCLE('',#95111,58.5);
#29844=CIRCLE('',#95113,58.5);
#29845=CIRCLE('',#95114,57.9482170030838);
#29846=CIRCLE('',#95115,58.5);
#29847=CIRCLE('',#95116,58.1064453881508);
#29848=CIRCLE('',#95117,58.5);
#29849=CIRCLE('',#95118,57.9666974474879);
#29850=CIRCLE('',#95119,58.5);
#29851=CIRCLE('',#95120,58.5);
#29852=CIRCLE('',#95121,58.5);
#29853=CIRCLE('',#95122,58.5);
#29854=CIRCLE('',#95126,3.);
#29855=CIRCLE('',#95128,67.5);
#29856=CIRCLE('',#95130,3.);
#29857=CIRCLE('',#95132,0.5);
#29858=CIRCLE('',#95133,0.5);
#29859=CIRCLE('',#95135,2.);
#29860=CIRCLE('',#95136,66.5);
#29861=CIRCLE('',#95137,2.);
#29862=CIRCLE('',#95138,0.5);
#29863=CIRCLE('',#95139,0.5);
#29864=CIRCLE('',#95141,0.5);
#29865=CIRCLE('',#95142,0.5);
#29866=CIRCLE('',#95143,0.5);
#29867=CIRCLE('',#95145,2.);
#29868=CIRCLE('',#95146,66.5);
#29869=CIRCLE('',#95147,2.);
#29870=CIRCLE('',#95150,0.5);
#29871=CIRCLE('',#95151,0.499999999999997);
#29872=CIRCLE('',#95153,0.499999999999998);
#29873=CIRCLE('',#95155,0.5);
#29874=CIRCLE('',#95158,0.5);
#29875=CIRCLE('',#95159,0.499999999999994);
#29876=CIRCLE('',#95161,0.500000000000001);
#29877=CIRCLE('',#95162,0.5);
#29878=CIRCLE('',#95163,0.5);
#29879=CIRCLE('',#95164,0.500000000000002);
#29880=CIRCLE('',#95166,0.500000000000003);
#29881=CIRCLE('',#95168,0.5);
#29882=CIRCLE('',#95169,0.5);
#29883=CIRCLE('',#95170,0.999999999999994);
#29884=CIRCLE('',#95172,0.5);
#29885=CIRCLE('',#95174,0.499999999999999);
#29886=CIRCLE('',#95175,0.499999999999998);
#29887=CIRCLE('',#95176,0.5);
#29888=CIRCLE('',#95179,0.5);
#29889=CIRCLE('',#95181,0.499999999999998);
#29890=CIRCLE('',#95182,0.5);
#29891=CIRCLE('',#95184,0.5);
#29892=CIRCLE('',#95185,0.499999999999998);
#29893=CIRCLE('',#95189,0.500000000000003);
#29894=CIRCLE('',#95190,0.499999999999994);
#29895=CIRCLE('',#95191,0.5);
#29896=CIRCLE('',#95193,0.5);
#29897=CIRCLE('',#95194,0.499999999999999);
#29898=CIRCLE('',#95195,0.5);
#29899=CIRCLE('',#95197,0.5);
#29900=CIRCLE('',#95198,0.499999999999999);
#29901=CIRCLE('',#95200,0.5);
#29902=CIRCLE('',#95201,3.);
#29903=CIRCLE('',#95203,0.5);
#29904=CIRCLE('',#95205,3.);
#29905=CIRCLE('',#95207,3.);
#29906=CIRCLE('',#95209,0.5);
#29907=CIRCLE('',#95210,0.499999999999999);
#29908=CIRCLE('',#95211,0.500000000000003);
#29909=CIRCLE('',#95212,0.5);
#29910=CIRCLE('',#95214,0.5);
#29911=CIRCLE('',#95216,0.5);
#29912=CIRCLE('',#95218,3.);
#29913=CIRCLE('',#95219,0.499999999999997);
#29914=CIRCLE('',#95220,0.5);
#29915=CIRCLE('',#95222,0.5);
#29916=CIRCLE('',#95223,0.500000000000003);
#29917=CIRCLE('',#95225,0.5);
#29918=CIRCLE('',#95226,3.);
#29919=CIRCLE('',#95228,0.5);
#29920=CIRCLE('',#95231,0.500000000000002);
#29921=CIRCLE('',#95232,0.499999999999999);
#29922=CIRCLE('',#95233,0.5);
#29923=CIRCLE('',#95234,0.5);
#29924=CIRCLE('',#95237,3.);
#29925=CIRCLE('',#95239,3.);
#29926=CIRCLE('',#95242,0.5);
#29927=CIRCLE('',#95243,0.500000000000001);
#29928=CIRCLE('',#95244,0.500000000000001);
#29929=CIRCLE('',#95246,3.);
#29930=CIRCLE('',#95247,0.5);
#29931=CIRCLE('',#95249,3.);
#29932=CIRCLE('',#95251,0.5);
#29933=CIRCLE('',#95253,3.);
#29934=CIRCLE('',#95254,0.5);
#29935=CIRCLE('',#95256,3.);
#29936=CIRCLE('',#95258,0.5);
#29937=CIRCLE('',#95260,0.5);
#29938=CIRCLE('',#95262,0.5);
#29939=CIRCLE('',#95263,0.5);
#29940=CIRCLE('',#95264,0.499999999999994);
#29941=CIRCLE('',#95266,0.500000000000001);
#29942=CIRCLE('',#95267,0.5);
#29943=CIRCLE('',#95269,0.5);
#29944=CIRCLE('',#95270,0.500000000000001);
#29945=CIRCLE('',#95272,0.5);
#29946=CIRCLE('',#95274,3.);
#29947=CIRCLE('',#95275,0.500000000000002);
#29948=CIRCLE('',#95276,0.5);
#29949=CIRCLE('',#95278,0.5);
#29950=CIRCLE('',#95279,0.500000000000003);
#29951=CIRCLE('',#95280,0.500000000000001);
#29952=CIRCLE('',#95281,0.5);
#29953=CIRCLE('',#95284,0.5);
#29954=CIRCLE('',#95286,0.5);
#29955=CIRCLE('',#95288,0.5);
#29956=CIRCLE('',#95289,3.);
#29957=CIRCLE('',#95291,0.5);
#29958=CIRCLE('',#95293,3.);
#29959=CIRCLE('',#95295,3.);
#29960=CIRCLE('',#95297,0.5);
#29961=CIRCLE('',#95298,0.500000000000001);
#29962=CIRCLE('',#95300,0.5);
#29963=CIRCLE('',#95302,0.5);
#29964=CIRCLE('',#95303,3.);
#29965=CIRCLE('',#95305,0.5);
#29966=CIRCLE('',#95306,0.5);
#29967=CIRCLE('',#95307,0.500000000000002);
#29968=CIRCLE('',#95309,0.499999999999994);
#29969=CIRCLE('',#95310,0.5);
#29970=CIRCLE('',#95312,0.5);
#29971=CIRCLE('',#95313,0.500000000000001);
#29972=CIRCLE('',#95314,0.5);
#29973=CIRCLE('',#95316,0.5);
#29974=CIRCLE('',#95317,0.500000000000001);
#29975=CIRCLE('',#95318,0.499999999999999);
#29976=CIRCLE('',#95319,0.5);
#29977=CIRCLE('',#95322,0.5);
#29978=CIRCLE('',#95323,0.5);
#29979=CIRCLE('',#95327,0.5);
#29980=CIRCLE('',#95328,0.5);
#29981=CIRCLE('',#95330,0.5);
#29982=CIRCLE('',#95331,0.5);
#29983=CIRCLE('',#95332,0.500000000000003);
#29984=CIRCLE('',#95334,0.500000000000006);
#29985=CIRCLE('',#95335,0.5);
#29986=CIRCLE('',#95337,0.5);
#29987=CIRCLE('',#95339,0.499999999999999);
#29988=CIRCLE('',#95340,0.5);
#29989=CIRCLE('',#95342,0.5);
#29990=CIRCLE('',#95343,0.499999999999999);
#29991=CIRCLE('',#95345,0.500000000000001);
#29992=CIRCLE('',#95346,0.5);
#29993=CIRCLE('',#95347,0.999497967753729);
#29994=CIRCLE('',#95349,0.5);
#29995=CIRCLE('',#95350,0.5);
#29996=CIRCLE('',#95353,98.8061397010869);
#29997=CIRCLE('',#95355,0.5);
#29998=CIRCLE('',#95356,0.5);
#29999=CIRCLE('',#95358,0.5);
#30000=CIRCLE('',#95359,0.5);
#30001=CIRCLE('',#95360,0.499999999999996);
#30002=CIRCLE('',#95361,0.999650016963681);
#30003=CIRCLE('',#95362,0.499999999999999);
#30004=CIRCLE('',#95363,0.5);
#30005=CIRCLE('',#95366,0.5);
#30006=CIRCLE('',#95368,0.500000000000002);
#30007=CIRCLE('',#95369,0.5);
#30008=CIRCLE('',#95371,0.5);
#30009=CIRCLE('',#95372,0.500000000000002);
#30010=CIRCLE('',#95373,0.499999999999998);
#30011=CIRCLE('',#95374,0.5);
#30012=CIRCLE('',#95377,0.5);
#30013=CIRCLE('',#95378,0.5);
#30014=CIRCLE('',#95382,0.5);
#30015=CIRCLE('',#95383,0.499999999999999);
#30016=CIRCLE('',#95385,0.5);
#30017=CIRCLE('',#95386,0.5);
#30018=CIRCLE('',#95387,0.499999999999999);
#30019=CIRCLE('',#95389,0.500000000000002);
#30020=CIRCLE('',#95390,0.5);
#30021=CIRCLE('',#95392,0.5);
#30022=CIRCLE('',#95393,0.499999999999999);
#30023=CIRCLE('',#95394,0.5);
#30024=CIRCLE('',#95396,0.5);
#30025=CIRCLE('',#95397,0.499999999999999);
#30026=CIRCLE('',#95398,0.499999999999998);
#30027=CIRCLE('',#95399,0.5);
#30028=CIRCLE('',#95402,0.5);
#30029=CIRCLE('',#95404,0.5);
#30030=CIRCLE('',#95405,3.);
#30031=CIRCLE('',#95406,0.5);
#30032=CIRCLE('',#95408,0.5);
#30033=CIRCLE('',#95410,3.);
#30034=CIRCLE('',#95412,3.);
#30035=CIRCLE('',#95414,0.5);
#30036=CIRCLE('',#95415,0.500000000000003);
#30037=CIRCLE('',#95417,0.5);
#30038=CIRCLE('',#95419,0.5);
#30039=CIRCLE('',#95420,3.);
#30040=CIRCLE('',#95423,0.5);
#30041=CIRCLE('',#95424,0.5);
#30042=CIRCLE('',#95425,0.499999999999996);
#30043=CIRCLE('',#95427,0.499999999999997);
#30044=CIRCLE('',#95428,0.5);
#30045=CIRCLE('',#95430,0.5);
#30046=CIRCLE('',#95431,0.500000000000002);
#30047=CIRCLE('',#95432,0.499999999999999);
#30048=CIRCLE('',#95433,0.5);
#30049=CIRCLE('',#95436,0.5);
#30050=CIRCLE('',#95438,0.5);
#30051=CIRCLE('',#95440,0.5);
#30052=CIRCLE('',#95441,3.);
#30053=CIRCLE('',#95443,0.5);
#30054=CIRCLE('',#95445,0.5);
#30055=CIRCLE('',#95446,0.499999999999997);
#30056=CIRCLE('',#95447,0.999999999999999);
#30057=CIRCLE('',#95449,0.5);
#30058=CIRCLE('',#95451,0.5);
#30059=CIRCLE('',#95453,58.1182624738004);
#30060=CIRCLE('',#95454,0.5);
#30061=CIRCLE('',#95455,0.5);
#30062=CIRCLE('',#95456,0.5);
#30063=CIRCLE('',#95458,0.5);
#30064=CIRCLE('',#95460,0.5);
#30065=CIRCLE('',#95462,0.5);
#30066=CIRCLE('',#95463,3.);
#30067=CIRCLE('',#95465,0.5);
#30068=CIRCLE('',#95467,3.);
#30069=CIRCLE('',#95468,0.500000000000002);
#30070=CIRCLE('',#95469,0.5);
#30071=CIRCLE('',#95471,0.5);
#30072=CIRCLE('',#95472,0.499999999999999);
#30073=CIRCLE('',#95473,0.499999999999993);
#30074=CIRCLE('',#95474,0.5);
#30075=CIRCLE('',#95478,3.);
#30076=CIRCLE('',#95480,0.5);
#30077=CIRCLE('',#95482,0.5);
#30078=CIRCLE('',#95484,1.);
#30079=CIRCLE('',#95485,1.);
#30080=CIRCLE('',#95487,0.5);
#30081=CIRCLE('',#95488,0.5);
#30082=CIRCLE('',#95490,0.5);
#30083=CIRCLE('',#95492,0.5);
#30084=CIRCLE('',#95493,3.);
#30085=CIRCLE('',#95496,0.5);
#30086=CIRCLE('',#95497,0.5);
#30087=CIRCLE('',#95498,0.5);
#30088=CIRCLE('',#95500,0.499999999999998);
#30089=CIRCLE('',#95501,0.5);
#30090=CIRCLE('',#95502,0.5);
#30091=CIRCLE('',#95503,0.992001837837135);
#30092=CIRCLE('',#95504,0.499999999999998);
#30093=CIRCLE('',#95505,0.5);
#30094=CIRCLE('',#95507,0.5);
#30095=CIRCLE('',#95508,0.499999999999998);
#30096=CIRCLE('',#95510,0.5);
#30097=CIRCLE('',#95512,3.);
#30098=CIRCLE('',#95514,0.500000000000004);
#30099=CIRCLE('',#95515,0.5);
#30100=CIRCLE('',#95517,0.5);
#30101=CIRCLE('',#95518,0.5);
#30102=CIRCLE('',#95520,0.5);
#30103=CIRCLE('',#95521,0.500000000000001);
#30104=CIRCLE('',#95522,0.500000000000001);
#30105=CIRCLE('',#95523,0.5);
#30106=CIRCLE('',#95525,0.5);
#30107=CIRCLE('',#95526,0.5);
#30108=CIRCLE('',#95528,0.5);
#30109=CIRCLE('',#95530,0.5);
#30110=CIRCLE('',#95532,0.5);
#30111=CIRCLE('',#95533,3.);
#30112=CIRCLE('',#95535,0.5);
#30113=CIRCLE('',#95537,3.);
#30114=CIRCLE('',#95539,3.);
#30115=CIRCLE('',#95541,0.5);
#30116=CIRCLE('',#95543,0.5);
#30117=CIRCLE('',#95545,0.5);
#30118=CIRCLE('',#95546,0.5);
#30119=CIRCLE('',#95547,0.5);
#30120=CIRCLE('',#95549,0.5);
#30121=CIRCLE('',#95550,0.500000000000001);
#30122=CIRCLE('',#95551,0.500000000000002);
#30123=CIRCLE('',#95552,0.5);
#30124=CIRCLE('',#95554,0.5);
#30125=CIRCLE('',#95555,0.500000000000001);
#30126=CIRCLE('',#95556,0.500000000000002);
#30127=CIRCLE('',#95558,0.5);
#30128=CIRCLE('',#95560,3.);
#30129=CIRCLE('',#95562,58.1182624738004);
#30130=CIRCLE('',#95564,0.5);
#30131=CIRCLE('',#95566,0.5);
#30132=CIRCLE('',#95567,0.500000000000003);
#30133=CIRCLE('',#95568,0.500000000000001);
#30134=CIRCLE('',#95569,0.5);
#30135=CIRCLE('',#95572,3.);
#30136=CIRCLE('',#95574,3.);
#30137=CIRCLE('',#95577,0.5);
#30138=CIRCLE('',#95578,0.5);
#30139=CIRCLE('',#95581,0.5);
#30140=CIRCLE('',#95583,3.);
#30141=CIRCLE('',#95585,3.);
#30142=CIRCLE('',#95588,0.5);
#30143=CIRCLE('',#95589,0.500000000000002);
#30144=CIRCLE('',#95590,0.500000000000001);
#30145=CIRCLE('',#95592,58.1182624738004);
#30146=CIRCLE('',#95594,0.5);
#30147=CIRCLE('',#95596,0.5);
#30148=CIRCLE('',#95597,0.5);
#30149=CIRCLE('',#95598,0.5);
#30150=CIRCLE('',#95599,0.5);
#30151=CIRCLE('',#95601,0.5);
#30152=CIRCLE('',#95603,0.5);
#30153=CIRCLE('',#95605,0.5);
#30154=CIRCLE('',#95606,3.);
#30155=CIRCLE('',#95608,0.5);
#30156=CIRCLE('',#95610,3.);
#30157=CIRCLE('',#95611,0.499999999999998);
#30158=CIRCLE('',#95612,0.499999999999999);
#30159=CIRCLE('',#95613,0.5);
#30160=CIRCLE('',#95615,0.5);
#30161=CIRCLE('',#95616,0.500000000000001);
#30162=CIRCLE('',#95617,0.5);
#30163=CIRCLE('',#95618,0.5);
#30164=CIRCLE('',#95621,3.);
#30165=CIRCLE('',#95623,0.5);
#30166=CIRCLE('',#95626,0.5);
#30167=CIRCLE('',#95628,0.5);
#30168=CIRCLE('',#95629,3.);
#30169=CIRCLE('',#95632,0.5);
#30170=CIRCLE('',#95633,0.5);
#30171=CIRCLE('',#95634,0.5);
#30172=CIRCLE('',#95637,0.5);
#30173=CIRCLE('',#95639,0.5);
#30174=CIRCLE('',#95641,0.5);
#30175=CIRCLE('',#95642,0.5);
#30176=CIRCLE('',#95643,0.500000000000003);
#30177=CIRCLE('',#95644,0.500000000000004);
#30178=CIRCLE('',#95645,0.992138051716334);
#30179=CIRCLE('',#95646,0.499999999999999);
#30180=CIRCLE('',#95647,0.5);
#30181=CIRCLE('',#95649,0.5);
#30182=CIRCLE('',#95650,0.500000000000001);
#30183=CIRCLE('',#95651,0.499999999999998);
#30184=CIRCLE('',#95652,0.500000000000002);
#30185=CIRCLE('',#95654,0.5);
#30186=CIRCLE('',#95656,3.);
#30187=CIRCLE('',#95658,0.499999999999997);
#30188=CIRCLE('',#95659,0.5);
#30189=CIRCLE('',#95661,0.499999999999998);
#30190=CIRCLE('',#95662,0.5);
#30191=CIRCLE('',#95664,0.5);
#30192=CIRCLE('',#95665,0.499999999999999);
#30193=CIRCLE('',#95666,0.499999999999994);
#30194=CIRCLE('',#95667,0.5);
#30195=CIRCLE('',#95669,0.5);
#30196=CIRCLE('',#95670,0.5);
#30197=CIRCLE('',#95672,0.5);
#30198=CIRCLE('',#95674,0.5);
#30199=CIRCLE('',#95676,0.5);
#30200=CIRCLE('',#95677,3.);
#30201=CIRCLE('',#95679,0.5);
#30202=CIRCLE('',#95681,3.);
#30203=CIRCLE('',#95683,3.);
#30204=CIRCLE('',#95685,0.5);
#30205=CIRCLE('',#95687,0.5);
#30206=CIRCLE('',#95689,0.5);
#30207=CIRCLE('',#95690,0.5);
#30208=CIRCLE('',#95691,0.5);
#30209=CIRCLE('',#95693,0.5);
#30210=CIRCLE('',#95694,0.499999999999994);
#30211=CIRCLE('',#95695,0.500000000000001);
#30212=CIRCLE('',#95696,0.5);
#30213=CIRCLE('',#95698,0.5);
#30214=CIRCLE('',#95699,0.499999999999999);
#30215=CIRCLE('',#95700,0.500000000000003);
#30216=CIRCLE('',#95702,0.5);
#30217=CIRCLE('',#95704,3.);
#30218=CIRCLE('',#95706,0.500000000000002);
#30219=CIRCLE('',#95707,0.499999999999999);
#30220=CIRCLE('',#95708,0.5);
#30221=CIRCLE('',#95709,0.5);
#30222=CIRCLE('',#95710,0.5);
#30223=CIRCLE('',#95712,0.5);
#30224=CIRCLE('',#95714,0.5);
#30225=CIRCLE('',#95717,0.5);
#30226=CIRCLE('',#95718,3.);
#30227=CIRCLE('',#95720,0.500000000000002);
#30228=CIRCLE('',#95721,0.5);
#30229=CIRCLE('',#95723,0.5);
#30230=CIRCLE('',#95724,0.500000000000002);
#30231=CIRCLE('',#95725,0.499999999999998);
#30232=CIRCLE('',#95727,0.5);
#30233=CIRCLE('',#95728,0.5);
#30234=CIRCLE('',#95730,0.5);
#30235=CIRCLE('',#95732,0.5);
#30236=CIRCLE('',#95734,0.5);
#30237=CIRCLE('',#95735,3.);
#30238=CIRCLE('',#95737,0.5);
#30239=CIRCLE('',#95739,3.);
#30240=CIRCLE('',#95740,0.5);
#30241=CIRCLE('',#95742,0.5);
#30242=CIRCLE('',#95744,0.5);
#30243=CIRCLE('',#95747,3.);
#30244=CIRCLE('',#95749,0.5);
#30245=CIRCLE('',#95751,0.5);
#30246=CIRCLE('',#95753,0.5);
#30247=CIRCLE('',#95754,0.5);
#30248=CIRCLE('',#95755,0.5);
#30249=CIRCLE('',#95756,0.5);
#30250=CIRCLE('',#95758,0.5);
#30251=CIRCLE('',#95759,0.499999999999996);
#30252=CIRCLE('',#95760,0.499999999999999);
#30253=CIRCLE('',#95761,0.5);
#30254=CIRCLE('',#95763,0.5);
#30255=CIRCLE('',#95764,0.499999999999999);
#30256=CIRCLE('',#95765,0.500000000000001);
#30257=CIRCLE('',#95766,0.5);
#30258=CIRCLE('',#95769,0.5);
#30259=CIRCLE('',#95771,3.);
#30260=CIRCLE('',#95773,58.1182624738004);
#30261=CIRCLE('',#95775,0.5);
#30262=CIRCLE('',#95776,0.499999999999998);
#30263=CIRCLE('',#95777,0.500000000000003);
#30264=CIRCLE('',#95778,0.5);
#30265=CIRCLE('',#95780,0.5);
#30266=CIRCLE('',#95781,0.499999999999997);
#30267=CIRCLE('',#95782,0.5);
#30268=CIRCLE('',#95783,0.5);
#30269=CIRCLE('',#95785,0.5);
#30270=CIRCLE('',#95786,0.5);
#30271=CIRCLE('',#95788,0.5);
#30272=CIRCLE('',#95790,0.5);
#30273=CIRCLE('',#95792,0.5);
#30274=CIRCLE('',#95793,3.);
#30275=CIRCLE('',#95795,0.5);
#30276=CIRCLE('',#95797,3.);
#30277=CIRCLE('',#95799,3.);
#30278=CIRCLE('',#95801,0.5);
#30279=CIRCLE('',#95804,0.5);
#30280=CIRCLE('',#95806,0.5);
#30281=CIRCLE('',#95807,0.5);
#30282=CIRCLE('',#95808,0.5);
#30283=CIRCLE('',#95809,0.5);
#30284=CIRCLE('',#95811,0.5);
#30285=CIRCLE('',#95812,0.500000000000007);
#30286=CIRCLE('',#95813,0.499999999999999);
#30287=CIRCLE('',#95814,0.5);
#30288=CIRCLE('',#95816,0.5);
#30289=CIRCLE('',#95817,0.499999999999999);
#30290=CIRCLE('',#95819,0.5);
#30291=CIRCLE('',#95821,3.);
#30292=CIRCLE('',#95823,0.5);
#30293=CIRCLE('',#95828,0.999999999999999);
#30294=CIRCLE('',#95830,1.);
#30295=CIRCLE('',#95832,0.999999999999998);
#30296=CIRCLE('',#95834,1.);
#30297=CIRCLE('',#95836,0.5);
#30298=CIRCLE('',#95838,0.5);
#30299=CIRCLE('',#95840,0.5);
#30300=CIRCLE('',#95842,0.5);
#30301=CIRCLE('',#95844,1.);
#30302=CIRCLE('',#95845,0.999999999999997);
#30303=CIRCLE('',#95846,0.499999999999997);
#30304=CIRCLE('',#95847,0.499999999999998);
#30305=CIRCLE('',#95849,0.499999999999999);
#30306=CIRCLE('',#95850,59.);
#30307=CIRCLE('',#95852,58.4063077870367);
#30308=CIRCLE('',#95853,0.499999999999999);
#30309=CIRCLE('',#95855,0.500000000000003);
#30310=CIRCLE('',#95856,59.);
#30311=CIRCLE('',#95857,0.5);
#30312=CIRCLE('',#95859,58.4063077870367);
#30313=CIRCLE('',#95860,0.5);
#30314=CIRCLE('',#95861,0.500000000000004);
#30315=CIRCLE('',#95862,68.2176100637577);
#30316=CIRCLE('',#95864,58.4063077870366);
#30317=CIRCLE('',#95865,0.499999999999997);
#30318=CIRCLE('',#95866,0.500000000000001);
#30319=CIRCLE('',#95867,68.2630953041282);
#30320=CIRCLE('',#95869,58.4063077870367);
#30321=CIRCLE('',#95870,0.500000000000003);
#30322=CIRCLE('',#95871,0.500000000000002);
#30323=CIRCLE('',#95872,68.1807062067102);
#30324=CIRCLE('',#95874,58.4063077870367);
#30325=CIRCLE('',#95875,0.500000000000001);
#30326=CIRCLE('',#95876,0.500000000000002);
#30327=CIRCLE('',#95878,0.500000000000001);
#30328=CIRCLE('',#95879,59.);
#30329=CIRCLE('',#95881,58.4063077870367);
#30330=CIRCLE('',#95882,0.499999999999997);
#30331=CIRCLE('',#95884,0.500000000000002);
#30332=CIRCLE('',#95885,59.);
#30333=CIRCLE('',#95886,0.499999999999997);
#30334=CIRCLE('',#95887,0.999999999999996);
#30335=CIRCLE('',#95889,0.5);
#30336=CIRCLE('',#95891,0.499999999999998);
#30337=CIRCLE('',#95893,1.);
#30338=CIRCLE('',#95894,1.);
#30339=CIRCLE('',#95896,0.5);
#30340=CIRCLE('',#95898,0.5);
#30341=CIRCLE('',#95900,0.999999999999998);
#30342=CIRCLE('',#95902,1.);
#30343=CIRCLE('',#95904,0.999999999999999);
#30344=CIRCLE('',#95906,0.500000000000007);
#30345=CIRCLE('',#95908,0.500000000000006);
#30346=CIRCLE('',#95910,0.500000000000006);
#30347=CIRCLE('',#95912,0.500000000000006);
#30348=CIRCLE('',#95914,0.999999999999999);
#30349=CIRCLE('',#95917,59.1370702608075);
#30350=CIRCLE('',#95918,58.2307624737709);
#30351=CIRCLE('',#95955,5.38573144442823);
#30352=CIRCLE('',#95956,0.999999999999997);
#30353=CIRCLE('',#95958,59.1370702608075);
#30354=CIRCLE('',#95959,58.2307624737709);
#30355=CIRCLE('',#95975,58.2307624737709);
#30356=CIRCLE('',#95977,59.1370702608075);
#30357=CIRCLE('',#95980,59.1370702608075);
#30358=CIRCLE('',#95981,58.2307624737709);
#30359=CIRCLE('',#95990,58.2307624737708);
#30360=CIRCLE('',#95992,59.1370702608075);
#30361=CIRCLE('',#95997,59.1370702608075);
#30362=CIRCLE('',#95999,58.2307624737708);
#30363=CIRCLE('',#96008,59.1370702608075);
#30364=CIRCLE('',#96011,3.);
#30365=CIRCLE('',#96012,3.);
#30366=CIRCLE('',#96015,58.1182624738004);
#30367=CIRCLE('',#96018,58.2307624737708);
#30368=CIRCLE('',#96020,59.1370702608075);
#30369=CIRCLE('',#96024,3.);
#30370=CIRCLE('',#96025,3.);
#30371=CIRCLE('',#96028,0.995738858064582);
#30372=CIRCLE('',#96029,58.2307624737708);
#30373=CIRCLE('',#96034,3.);
#30374=CIRCLE('',#96035,3.);
#30375=CIRCLE('',#96038,59.1370702608075);
#30376=CIRCLE('',#96041,58.2307624737709);
#30377=CIRCLE('',#96043,0.994758623428062);
#30378=CIRCLE('',#96045,59.1370702608075);
#30379=CIRCLE('',#96047,58.2307624737709);
#30380=CIRCLE('',#96052,3.);
#30381=CIRCLE('',#96053,3.);
#30382=CIRCLE('',#96056,58.1182624738004);
#30383=CIRCLE('',#96058,58.1182624738004);
#30384=CIRCLE('',#96060,58.2307624737709);
#30385=CIRCLE('',#96063,3.);
#30386=CIRCLE('',#96064,3.);
#30387=CIRCLE('',#96067,59.1370702608075);
#30388=CIRCLE('',#96070,58.2307624737709);
#30389=CIRCLE('',#96071,0.5);
#30390=CIRCLE('',#96072,1.);
#30391=CIRCLE('',#96073,0.5);
#30392=CIRCLE('',#96074,0.5);
#30393=CIRCLE('',#96076,59.1370702608075);
#30394=CIRCLE('',#96079,0.999999999999997);
#30395=CIRCLE('',#96080,5.38573144425447);
#30396=CIRCLE('',#96084,3.);
#30397=CIRCLE('',#96085,3.);
#30398=CIRCLE('',#96088,58.1182624738004);
#30399=CIRCLE('',#96090,3.);
#30400=CIRCLE('',#96091,3.);
#30401=CIRCLE('',#96093,59.);
#30402=CIRCLE('',#96096,58.4063077870367);
#30403=CIRCLE('',#96098,59.);
#30404=CIRCLE('',#96101,3.);
#30405=CIRCLE('',#96102,3.);
#30406=CIRCLE('',#96104,0.5);
#30407=CIRCLE('',#96107,58.4063077870367);
#30408=CIRCLE('',#96108,68.2195020909334);
#30409=CIRCLE('',#96112,58.4063077870366);
#30410=CIRCLE('',#96113,68.2630953041282);
#30411=CIRCLE('',#96114,98.8061397010869);
#30412=CIRCLE('',#96118,58.4063077870367);
#30413=CIRCLE('',#96119,68.1826171111001);
#30414=CIRCLE('',#96122,58.4063077870367);
#30415=CIRCLE('',#96124,0.5);
#30416=CIRCLE('',#96127,3.);
#30417=CIRCLE('',#96128,3.);
#30418=CIRCLE('',#96130,59.);
#30419=CIRCLE('',#96132,3.);
#30420=CIRCLE('',#96133,3.);
#30421=CIRCLE('',#96136,58.4063077870367);
#30422=CIRCLE('',#96138,59.);
#30423=CIRCLE('',#96146,3.);
#30424=CIRCLE('',#96147,3.);
#30425=CIRCLE('',#96149,0.994491935959051);
#30426=CIRCLE('',#96152,3.);
#30427=CIRCLE('',#96153,3.);
#30428=CIRCLE('',#96154,0.5);
#30429=CIRCLE('',#96155,0.5);
#30430=CIRCLE('',#96156,0.5);
#30431=CIRCLE('',#96157,1.);
#30432=CIRCLE('',#96158,0.999999999999999);
#30433=CIRCLE('',#96159,0.999999999999994);
#30434=CIRCLE('',#96161,0.500000000000006);
#30435=CIRCLE('',#96162,0.5);
#30436=CIRCLE('',#96164,0.500000000000006);
#30437=CIRCLE('',#96165,0.5);
#30438=CIRCLE('',#96167,0.5);
#30439=CIRCLE('',#96168,0.500000000000006);
#30440=CIRCLE('',#96170,0.500000000000007);
#30441=CIRCLE('',#96171,0.5);
#30442=CIRCLE('',#96173,0.999999999999999);
#30443=CIRCLE('',#96175,3.);
#30444=CIRCLE('',#96176,1.);
#30445=CIRCLE('',#96177,2.);
#30446=CIRCLE('',#96179,67.5);
#30447=CIRCLE('',#96180,0.999999999999998);
#30448=CIRCLE('',#96181,66.5);
#30449=CIRCLE('',#96183,3.);
#30450=CIRCLE('',#96184,1.);
#30451=CIRCLE('',#96185,2.);
#30452=CIRCLE('',#96186,0.5);
#30453=CIRCLE('',#96187,0.5);
#30454=CIRCLE('',#96189,0.5);
#30455=CIRCLE('',#96190,0.5);
#30456=CIRCLE('',#96192,1.);
#30457=CIRCLE('',#96193,0.999999999999996);
#30458=CIRCLE('',#96195,0.5);
#30459=CIRCLE('',#96196,0.499999999999998);
#30460=CIRCLE('',#96198,0.5);
#30461=CIRCLE('',#96199,0.5);
#30462=CIRCLE('',#96201,0.5);
#30463=CIRCLE('',#96202,0.499999999999997);
#30464=CIRCLE('',#96204,0.500000000000002);
#30465=CIRCLE('',#96207,58.5);
#30466=CIRCLE('',#96208,0.499999999999997);
#30467=CIRCLE('',#96209,0.5);
#30468=CIRCLE('',#96211,58.5);
#30469=CIRCLE('',#96214,0.500000000000001);
#30470=CIRCLE('',#96215,0.5);
#30471=CIRCLE('',#96217,0.500000000000002);
#30472=CIRCLE('',#96218,58.5);
#30473=CIRCLE('',#96219,0.500000000000001);
#30474=CIRCLE('',#96220,0.5);
#30475=CIRCLE('',#96223,58.5);
#30476=CIRCLE('',#96226,0.500000000000002);
#30477=CIRCLE('',#96227,0.5);
#30478=CIRCLE('',#96228,57.9482170028185);
#30479=CIRCLE('',#96229,0.500000000000003);
#30480=CIRCLE('',#96230,0.5);
#30481=CIRCLE('',#96232,58.5);
#30482=CIRCLE('',#96235,0.500000000000001);
#30483=CIRCLE('',#96236,0.5);
#30484=CIRCLE('',#96237,58.1061766845785);
#30485=CIRCLE('',#96238,0.499999999999997);
#30486=CIRCLE('',#96239,0.5);
#30487=CIRCLE('',#96241,58.5);
#30488=CIRCLE('',#96244,0.500000000000004);
#30489=CIRCLE('',#96245,0.5);
#30490=CIRCLE('',#96246,57.9664310113591);
#30491=CIRCLE('',#96247,0.5);
#30492=CIRCLE('',#96248,0.5);
#30493=CIRCLE('',#96250,58.5);
#30494=CIRCLE('',#96253,0.5);
#30495=CIRCLE('',#96254,0.5);
#30496=CIRCLE('',#96255,0.500000000000003);
#30497=CIRCLE('',#96257,0.499999999999999);
#30498=CIRCLE('',#96258,58.5);
#30499=CIRCLE('',#96259,0.5);
#30500=CIRCLE('',#96261,58.5);
#30501=CIRCLE('',#96264,0.5);
#30502=CIRCLE('',#96265,0.499999999999999);
#30503=CIRCLE('',#96267,58.5);
#30504=CIRCLE('',#96268,0.499999999999998);
#30505=CIRCLE('',#96269,0.499999999999997);
#30506=CIRCLE('',#96270,0.999999999999997);
#30507=CIRCLE('',#96271,0.5);
#30508=CIRCLE('',#96272,1.);
#30509=CIRCLE('',#96274,0.5);
#30510=CIRCLE('',#96275,0.5);
#30511=CIRCLE('',#96277,0.5);
#30512=CIRCLE('',#96278,0.5);
#30513=CIRCLE('',#96280,0.5);
#30514=CIRCLE('',#96281,0.5);
#30515=CIRCLE('',#96283,0.5);
#30516=CIRCLE('',#96284,0.5);
#30517=CIRCLE('',#96286,1.);
#30518=CIRCLE('',#96288,3.);
#30519=CIRCLE('',#96289,0.999999999999998);
#30520=CIRCLE('',#96290,2.);
#30521=CIRCLE('',#96292,67.5);
#30522=CIRCLE('',#96293,1.);
#30523=CIRCLE('',#96294,66.5);
#30524=CIRCLE('',#96296,3.);
#30525=CIRCLE('',#96297,0.999999999999999);
#30526=CIRCLE('',#96298,2.);
#30527=CIRCLE('',#96301,0.5);
#30528=CIRCLE('',#96302,0.5);
#30529=CIRCLE('',#96303,0.5);
#30530=CIRCLE('',#96306,58.5);
#30531=CIRCLE('',#96308,2.75);
#30532=CIRCLE('',#96310,0.5);
#30533=CIRCLE('',#96311,2.5);
#30534=CIRCLE('',#96312,0.5);
#30535=CIRCLE('',#96314,0.5);
#30536=CIRCLE('',#96315,0.499999999999999);
#30537=CIRCLE('',#96316,0.499999999999999);
#30538=CIRCLE('',#96317,0.5);
#30539=CIRCLE('',#96319,0.5);
#30540=CIRCLE('',#96320,0.499999999999999);
#30541=CIRCLE('',#96321,0.500000000000007);
#30542=CIRCLE('',#96322,0.5);
#30543=CIRCLE('',#96324,0.5);
#30544=CIRCLE('',#96325,0.5);
#30545=CIRCLE('',#96326,0.5);
#30546=CIRCLE('',#96330,0.5);
#30547=CIRCLE('',#96331,0.5);
#30548=CIRCLE('',#96333,2.5);
#30549=CIRCLE('',#96334,0.5);
#30550=CIRCLE('',#96335,3.);
#30551=CIRCLE('',#96337,3.);
#30552=CIRCLE('',#96339,0.5);
#30553=CIRCLE('',#96340,2.5);
#30554=CIRCLE('',#96341,0.5);
#30555=CIRCLE('',#96343,0.5);
#30556=CIRCLE('',#96345,2.5);
#30557=CIRCLE('',#96346,0.5);
#30558=CIRCLE('',#96349,0.5);
#30559=CIRCLE('',#96350,0.5);
#30560=CIRCLE('',#96352,0.5);
#30561=CIRCLE('',#96353,0.5);
#30562=CIRCLE('',#96354,0.499999999999997);
#30563=CIRCLE('',#96355,0.5);
#30564=CIRCLE('',#96357,0.5);
#30565=CIRCLE('',#96358,0.500000000000003);
#30566=CIRCLE('',#96359,0.499999999999998);
#30567=CIRCLE('',#96360,0.5);
#30568=CIRCLE('',#96362,0.5);
#30569=CIRCLE('',#96364,59.024570260837);
#30570=CIRCLE('',#96366,0.5);
#30571=CIRCLE('',#96367,2.5);
#30572=CIRCLE('',#96368,0.5);
#30573=CIRCLE('',#96370,0.5);
#30574=CIRCLE('',#96372,0.5);
#30575=CIRCLE('',#96373,0.5);
#30576=CIRCLE('',#96374,0.500000000000001);
#30577=CIRCLE('',#96375,0.499999999999999);
#30578=CIRCLE('',#96376,0.5);
#30579=CIRCLE('',#96378,0.5);
#30580=CIRCLE('',#96379,0.499999999999999);
#30581=CIRCLE('',#96380,0.499999999999996);
#30582=CIRCLE('',#96381,0.5);
#30583=CIRCLE('',#96383,0.5);
#30584=CIRCLE('',#96384,0.5);
#30585=CIRCLE('',#96385,0.5);
#30586=CIRCLE('',#96389,2.5);
#30587=CIRCLE('',#96390,0.5);
#30588=CIRCLE('',#96391,3.);
#30589=CIRCLE('',#96393,3.);
#30590=CIRCLE('',#96395,0.5);
#30591=CIRCLE('',#96396,0.5);
#30592=CIRCLE('',#96398,0.5);
#30593=CIRCLE('',#96400,0.5);
#30594=CIRCLE('',#96401,0.5);
#30595=CIRCLE('',#96403,0.5);
#30596=CIRCLE('',#96404,0.5);
#30597=CIRCLE('',#96405,2.5);
#30598=CIRCLE('',#96407,0.5);
#30599=CIRCLE('',#96409,0.5);
#30600=CIRCLE('',#96410,2.5);
#30601=CIRCLE('',#96413,0.5);
#30602=CIRCLE('',#96414,0.499999999999998);
#30603=CIRCLE('',#96415,0.5);
#30604=CIRCLE('',#96416,0.500000000000002);
#30605=CIRCLE('',#96417,0.5);
#30606=CIRCLE('',#96419,0.5);
#30607=CIRCLE('',#96420,0.500000000000002);
#30608=CIRCLE('',#96421,0.500000000000002);
#30609=CIRCLE('',#96423,0.5);
#30610=CIRCLE('',#96424,0.5);
#30611=CIRCLE('',#96426,2.5);
#30612=CIRCLE('',#96427,0.5);
#30613=CIRCLE('',#96430,0.5);
#30614=CIRCLE('',#96431,0.499999999999998);
#30615=CIRCLE('',#96435,58.1182624738004);
#30616=CIRCLE('',#96437,0.5);
#30617=CIRCLE('',#96438,2.5);
#30618=CIRCLE('',#96439,0.5);
#30619=CIRCLE('',#96441,0.5);
#30620=CIRCLE('',#96442,0.500000000000003);
#30621=CIRCLE('',#96443,0.5);
#30622=CIRCLE('',#96444,0.499999999999999);
#30623=CIRCLE('',#96445,0.5);
#30624=CIRCLE('',#96447,0.5);
#30625=CIRCLE('',#96448,0.500000000000001);
#30626=CIRCLE('',#96449,0.499999999999994);
#30627=CIRCLE('',#96450,0.5);
#30628=CIRCLE('',#96452,0.5);
#30629=CIRCLE('',#96453,0.5);
#30630=CIRCLE('',#96457,2.5);
#30631=CIRCLE('',#96458,0.5);
#30632=CIRCLE('',#96459,3.);
#30633=CIRCLE('',#96461,3.);
#30634=CIRCLE('',#96463,0.5);
#30635=CIRCLE('',#96464,2.5);
#30636=CIRCLE('',#96465,0.5);
#30637=CIRCLE('',#96467,0.5);
#30638=CIRCLE('',#96469,2.5);
#30639=CIRCLE('',#96470,0.5);
#30640=CIRCLE('',#96473,0.5);
#30641=CIRCLE('',#96474,0.5);
#30642=CIRCLE('',#96476,0.5);
#30643=CIRCLE('',#96477,0.499999999999994);
#30644=CIRCLE('',#96478,0.499999999999999);
#30645=CIRCLE('',#96479,0.5);
#30646=CIRCLE('',#96481,0.5);
#30647=CIRCLE('',#96482,0.499999999999998);
#30648=CIRCLE('',#96483,0.499999999999997);
#30649=CIRCLE('',#96485,0.5);
#30650=CIRCLE('',#96486,0.5);
#30651=CIRCLE('',#96488,58.1182624738004);
#30652=CIRCLE('',#96490,0.5);
#30653=CIRCLE('',#96491,2.5);
#30654=CIRCLE('',#96492,0.5);
#30655=CIRCLE('',#96494,0.5);
#30656=CIRCLE('',#96495,0.5);
#30657=CIRCLE('',#96497,0.500000000000002);
#30658=CIRCLE('',#96499,0.499999999999998);
#30659=CIRCLE('',#96501,0.500000000000001);
#30660=CIRCLE('',#96502,0.5);
#30661=CIRCLE('',#96504,0.5);
#30662=CIRCLE('',#96505,0.499999999999999);
#30663=CIRCLE('',#96506,0.500000000000004);
#30664=CIRCLE('',#96507,0.500000000000003);
#30665=CIRCLE('',#96508,0.5);
#30666=CIRCLE('',#96512,0.5);
#30667=CIRCLE('',#96514,0.5);
#30668=CIRCLE('',#96515,0.5);
#30669=CIRCLE('',#96516,0.5);
#30670=CIRCLE('',#96519,0.5);
#30671=CIRCLE('',#96521,2.5);
#30672=CIRCLE('',#96522,0.5);
#30673=CIRCLE('',#96524,0.5);
#30674=CIRCLE('',#96525,0.5);
#30675=CIRCLE('',#96526,0.5);
#30676=CIRCLE('',#96528,1.);
#30677=CIRCLE('',#96530,2.5);
#30678=CIRCLE('',#96531,0.5);
#30679=CIRCLE('',#96532,3.);
#30680=CIRCLE('',#96534,3.);
#30681=CIRCLE('',#96536,0.5);
#30682=CIRCLE('',#96537,0.5);
#30683=CIRCLE('',#96538,0.5);
#30684=CIRCLE('',#96539,0.500000000000001);
#30685=CIRCLE('',#96540,0.5);
#30686=CIRCLE('',#96542,0.5);
#30687=CIRCLE('',#96543,0.499999999999999);
#30688=CIRCLE('',#96544,0.499999999999998);
#30689=CIRCLE('',#96545,0.5);
#30690=CIRCLE('',#96547,0.5);
#30691=CIRCLE('',#96548,2.5);
#30692=CIRCLE('',#96549,0.5);
#30693=CIRCLE('',#96551,0.5);
#30694=CIRCLE('',#96553,2.5);
#30695=CIRCLE('',#96554,0.5);
#30696=CIRCLE('',#96557,0.5);
#30697=CIRCLE('',#96558,0.5);
#30698=CIRCLE('',#96560,0.5);
#30699=CIRCLE('',#96562,0.5);
#30700=CIRCLE('',#96564,59.024570260837);
#30701=CIRCLE('',#96565,0.5);
#30702=CIRCLE('',#96566,0.500000000000001);
#30703=CIRCLE('',#96567,0.500000000000002);
#30704=CIRCLE('',#96568,0.5);
#30705=CIRCLE('',#96570,0.5);
#30706=CIRCLE('',#96572,0.5);
#30707=CIRCLE('',#96573,2.5);
#30708=CIRCLE('',#96574,0.5);
#30709=CIRCLE('',#96575,3.);
#30710=CIRCLE('',#96577,3.);
#30711=CIRCLE('',#96579,0.5);
#30712=CIRCLE('',#96580,2.5);
#30713=CIRCLE('',#96581,0.5);
#30714=CIRCLE('',#96584,1.);
#30715=CIRCLE('',#96585,0.499999999999999);
#30716=CIRCLE('',#96586,0.5);
#30717=CIRCLE('',#96587,0.5);
#30718=CIRCLE('',#96589,0.5);
#30719=CIRCLE('',#96591,0.5);
#30720=CIRCLE('',#96592,2.5);
#30721=CIRCLE('',#96593,0.5);
#30722=CIRCLE('',#96594,3.);
#30723=CIRCLE('',#96596,3.);
#30724=CIRCLE('',#96598,0.5);
#30725=CIRCLE('',#96599,2.5);
#30726=CIRCLE('',#96600,0.5);
#30727=CIRCLE('',#96602,0.5);
#30728=CIRCLE('',#96603,0.5);
#30729=CIRCLE('',#96604,0.500000000000001);
#30730=CIRCLE('',#96605,0.500000000000003);
#30731=CIRCLE('',#96606,0.5);
#30732=CIRCLE('',#96608,0.5);
#30733=CIRCLE('',#96610,0.5);
#30734=CIRCLE('',#96612,59.024570260837);
#30735=CIRCLE('',#96614,0.5);
#30736=CIRCLE('',#96615,2.5);
#30737=CIRCLE('',#96616,0.5);
#30738=CIRCLE('',#96618,0.5);
#30739=CIRCLE('',#96619,0.500000000000002);
#30740=CIRCLE('',#96620,0.5);
#30741=CIRCLE('',#96621,0.500000000000001);
#30742=CIRCLE('',#96622,0.5);
#30743=CIRCLE('',#96624,0.5);
#30744=CIRCLE('',#96625,0.500000000000002);
#30745=CIRCLE('',#96626,0.500000000000001);
#30746=CIRCLE('',#96627,0.5);
#30747=CIRCLE('',#96629,0.5);
#30748=CIRCLE('',#96630,0.5);
#30749=CIRCLE('',#96634,2.5);
#30750=CIRCLE('',#96635,0.5);
#30751=CIRCLE('',#96636,3.);
#30752=CIRCLE('',#96638,3.);
#30753=CIRCLE('',#96640,0.5);
#30754=CIRCLE('',#96641,2.5);
#30755=CIRCLE('',#96642,0.5);
#30756=CIRCLE('',#96644,0.5);
#30757=CIRCLE('',#96646,2.5);
#30758=CIRCLE('',#96647,0.5);
#30759=CIRCLE('',#96650,0.5);
#30760=CIRCLE('',#96651,0.5);
#30761=CIRCLE('',#96653,0.5);
#30762=CIRCLE('',#96654,0.500000000000001);
#30763=CIRCLE('',#96655,0.500000000000001);
#30764=CIRCLE('',#96656,0.5);
#30765=CIRCLE('',#96658,0.5);
#30766=CIRCLE('',#96659,0.5);
#30767=CIRCLE('',#96660,0.500000000000004);
#30768=CIRCLE('',#96662,0.5);
#30769=CIRCLE('',#96663,0.5);
#30770=CIRCLE('',#96665,58.1182624738004);
#30771=CIRCLE('',#96667,0.5);
#30772=CIRCLE('',#96668,2.5);
#30773=CIRCLE('',#96669,0.5);
#30774=CIRCLE('',#96671,0.5);
#30775=CIRCLE('',#96672,0.499999999999998);
#30776=CIRCLE('',#96673,0.499999999999998);
#30777=CIRCLE('',#96674,0.5);
#30778=CIRCLE('',#96676,0.5);
#30779=CIRCLE('',#96677,0.499999999999998);
#30780=CIRCLE('',#96678,0.5);
#30781=CIRCLE('',#96679,0.5);
#30782=CIRCLE('',#96680,0.5);
#30783=CIRCLE('',#96681,0.5);
#30784=CIRCLE('',#96684,0.5);
#30785=CIRCLE('',#96685,0.5);
#30786=CIRCLE('',#96686,0.5);
#30787=CIRCLE('',#96689,0.5);
#30788=CIRCLE('',#96691,0.5);
#30789=CIRCLE('',#96692,2.5);
#30790=CIRCLE('',#96694,0.5);
#30791=CIRCLE('',#96695,0.5);
#30792=CIRCLE('',#96696,0.5);
#30793=CIRCLE('',#96700,0.5);
#30794=CIRCLE('',#96702,0.5);
#30795=CIRCLE('',#96703,3.);
#30796=CIRCLE('',#96704,2.5);
#30797=CIRCLE('',#96706,3.);
#30798=CIRCLE('',#96708,0.5);
#30799=CIRCLE('',#96709,0.5);
#30800=CIRCLE('',#96710,0.499999999999993);
#30801=CIRCLE('',#96711,0.499999999999999);
#30802=CIRCLE('',#96712,0.5);
#30803=CIRCLE('',#96714,0.5);
#30804=CIRCLE('',#96715,0.500000000000002);
#30805=CIRCLE('',#96716,0.5);
#30806=CIRCLE('',#96718,0.5);
#30807=CIRCLE('',#96719,2.5);
#30808=CIRCLE('',#96720,0.5);
#30809=CIRCLE('',#96722,0.5);
#30810=CIRCLE('',#96724,2.5);
#30811=CIRCLE('',#96725,0.5);
#30812=CIRCLE('',#96728,0.5);
#30813=CIRCLE('',#96729,0.5);
#30814=CIRCLE('',#96731,59.024570260837);
#30815=CIRCLE('',#96732,0.999999999999999);
#30816=CIRCLE('',#96734,0.5);
#30817=CIRCLE('',#96736,0.5);
#30818=CIRCLE('',#96737,0.499999999999997);
#30819=CIRCLE('',#96738,0.499999999999999);
#30820=CIRCLE('',#96739,0.5);
#30821=CIRCLE('',#96741,0.5);
#30822=CIRCLE('',#96742,0.500000000000002);
#30823=CIRCLE('',#96744,0.5);
#30824=CIRCLE('',#96745,0.5);
#30825=CIRCLE('',#96747,2.5);
#30826=CIRCLE('',#96748,0.5);
#30827=CIRCLE('',#96751,0.5);
#30828=CIRCLE('',#96753,0.499999999999999);
#30829=CIRCLE('',#96754,0.5);
#30830=CIRCLE('',#96755,0.500000000000003);
#30831=CIRCLE('',#96757,0.5);
#30832=CIRCLE('',#96758,0.499999999999997);
#30833=CIRCLE('',#96759,0.499999999999996);
#30834=CIRCLE('',#96761,0.5);
#30835=CIRCLE('',#96764,0.5);
#30836=CIRCLE('',#96766,2.5);
#30837=CIRCLE('',#96767,0.5);
#30838=CIRCLE('',#96769,0.5);
#30839=CIRCLE('',#96770,0.499999999999999);
#30840=CIRCLE('',#96772,2.5);
#30841=CIRCLE('',#96773,0.5);
#30842=CIRCLE('',#96774,3.);
#30843=CIRCLE('',#96776,3.);
#30844=CIRCLE('',#96778,0.5);
#30845=CIRCLE('',#96779,2.5);
#30846=CIRCLE('',#96780,0.5);
#30847=CIRCLE('',#96782,0.5);
#30848=CIRCLE('',#96784,2.5);
#30849=CIRCLE('',#96786,0.5);
#30850=CIRCLE('',#96788,0.499999999999998);
#30851=CIRCLE('',#96789,0.499999999999999);
#30852=CIRCLE('',#96790,0.5);
#30853=CIRCLE('',#96792,0.5);
#30854=CIRCLE('',#96793,0.499999999999999);
#30855=CIRCLE('',#96794,0.500000000000003);
#30856=CIRCLE('',#96795,0.5);
#30857=CIRCLE('',#96796,0.499999999999999);
#30858=CIRCLE('',#96798,0.5);
#30859=CIRCLE('',#96799,0.500000000000002);
#30860=CIRCLE('',#96800,0.499999999999999);
#30861=CIRCLE('',#96801,0.5);
#30862=CIRCLE('',#96804,0.5);
#30863=CIRCLE('',#96805,0.500000000000001);
#30864=CIRCLE('',#96807,0.5);
#30865=CIRCLE('',#96810,0.5);
#30866=CIRCLE('',#96811,0.5);
#30867=CIRCLE('',#96813,0.5);
#30868=CIRCLE('',#96815,0.499999999999998);
#30869=CIRCLE('',#96816,0.500000000000002);
#30870=CIRCLE('',#96817,0.5);
#30871=CIRCLE('',#96819,0.5);
#30872=CIRCLE('',#96820,0.500000000000002);
#30873=CIRCLE('',#96821,0.5);
#30874=CIRCLE('',#96823,0.5);
#30875=CIRCLE('',#96824,0.5);
#30876=CIRCLE('',#96827,0.5);
#30877=CIRCLE('',#96828,0.499999999999999);
#30878=CIRCLE('',#96830,0.499999999999996);
#30879=CIRCLE('',#96831,0.5);
#30880=CIRCLE('',#96834,0.5);
#30881=CIRCLE('',#96835,0.5);
#30882=CIRCLE('',#96837,0.5);
#30883=CIRCLE('',#96839,109.361438801731);
#30884=CIRCLE('',#96841,0.5);
#30885=CIRCLE('',#96842,0.5);
#30886=CIRCLE('',#96844,0.5);
#30887=CIRCLE('',#96846,0.500000000000001);
#30888=CIRCLE('',#96847,0.499999999999999);
#30889=CIRCLE('',#96849,0.5);
#30890=CIRCLE('',#96851,0.5);
#30891=CIRCLE('',#96853,0.499999999999999);
#30892=CIRCLE('',#96855,0.500000000000002);
#30893=CIRCLE('',#96856,0.5);
#30894=CIRCLE('',#96857,0.5);
#30895=CIRCLE('',#96859,0.5);
#30896=CIRCLE('',#96860,0.500000000000006);
#30897=CIRCLE('',#96861,0.500000000000003);
#30898=CIRCLE('',#96862,0.5);
#30899=CIRCLE('',#96865,0.5);
#30900=CIRCLE('',#96866,0.499999999999998);
#30901=CIRCLE('',#96868,0.5);
#30902=CIRCLE('',#96871,0.5);
#30903=CIRCLE('',#96872,0.5);
#30904=CIRCLE('',#96874,0.5);
#30905=CIRCLE('',#96876,0.499999999999999);
#30906=CIRCLE('',#96877,0.500000000000001);
#30907=CIRCLE('',#96878,0.5);
#30908=CIRCLE('',#96880,0.5);
#30909=CIRCLE('',#96881,0.500000000000001);
#30910=CIRCLE('',#96882,0.499999999999998);
#30911=CIRCLE('',#96883,0.5);
#30912=CIRCLE('',#96884,0.500000000000001);
#30913=CIRCLE('',#96886,0.5);
#30914=CIRCLE('',#96887,0.499999999999994);
#30915=CIRCLE('',#96888,0.500000000000002);
#30916=CIRCLE('',#96890,0.5);
#30917=CIRCLE('',#96893,2.5);
#30918=CIRCLE('',#96894,0.5);
#30919=CIRCLE('',#96896,0.5);
#30920=CIRCLE('',#96897,0.5);
#30921=CIRCLE('',#96899,2.5);
#30922=CIRCLE('',#96900,0.5);
#30923=CIRCLE('',#96901,3.);
#30924=CIRCLE('',#96903,3.);
#30925=CIRCLE('',#96905,0.5);
#30926=CIRCLE('',#96906,2.5);
#30927=CIRCLE('',#96907,0.5);
#30928=CIRCLE('',#96909,0.5);
#30929=CIRCLE('',#96911,2.5);
#30930=CIRCLE('',#96912,0.5);
#30931=CIRCLE('',#96915,0.5);
#30932=CIRCLE('',#96917,0.500000000000001);
#30933=CIRCLE('',#96918,0.500000000000003);
#30934=CIRCLE('',#96919,0.5);
#30935=CIRCLE('',#96921,0.5);
#30936=CIRCLE('',#96922,0.500000000000002);
#30937=CIRCLE('',#96923,0.499999999999997);
#30938=CIRCLE('',#96925,0.5);
#30939=CIRCLE('',#96926,2.5);
#30940=CIRCLE('',#96927,0.5);
#30941=CIRCLE('',#96929,0.5);
#30942=CIRCLE('',#96930,0.499999999999998);
#30943=CIRCLE('',#96931,0.500000000000001);
#30944=CIRCLE('',#96932,0.5);
#30945=CIRCLE('',#96934,0.5);
#30946=CIRCLE('',#96935,0.500000000000001);
#30947=CIRCLE('',#96936,0.499999999999994);
#30948=CIRCLE('',#96938,0.5);
#30949=CIRCLE('',#96942,2.5);
#30950=CIRCLE('',#96943,0.5);
#30951=CIRCLE('',#96944,3.);
#30952=CIRCLE('',#96946,3.);
#30953=CIRCLE('',#96948,0.5);
#30954=CIRCLE('',#96949,2.5);
#30955=CIRCLE('',#96951,2.5);
#30956=CIRCLE('',#96952,0.5);
#30957=CIRCLE('',#96953,3.);
#30958=CIRCLE('',#96955,3.);
#30959=CIRCLE('',#96957,0.5);
#30960=CIRCLE('',#96958,2.5);
#30961=CIRCLE('',#96959,0.500000000000001);
#30962=CIRCLE('',#96960,0.500000000000001);
#30963=CIRCLE('',#96961,0.500000000000002);
#30964=CIRCLE('',#96962,0.5);
#30965=CIRCLE('',#96963,0.500000000000001);
#30966=CIRCLE('',#96965,0.499999999999999);
#30967=CIRCLE('',#96966,0.499999999999999);
#30968=CIRCLE('',#96967,0.500000000000001);
#30969=CIRCLE('',#96968,0.500000000000001);
#30970=CIRCLE('',#96969,0.5);
#30971=CIRCLE('',#96971,0.5);
#30972=CIRCLE('',#96973,0.5);
#30973=CIRCLE('',#96974,2.5);
#30974=CIRCLE('',#96975,0.5);
#30975=CIRCLE('',#96976,3.);
#30976=CIRCLE('',#96978,3.);
#30977=CIRCLE('',#96980,0.5);
#30978=CIRCLE('',#96981,2.5);
#30979=CIRCLE('',#96982,0.5);
#30980=CIRCLE('',#96984,0.5);
#30981=CIRCLE('',#96985,0.5);
#30982=CIRCLE('',#96986,0.5);
#30983=CIRCLE('',#96987,0.500000000000002);
#30984=CIRCLE('',#96988,0.499999999999997);
#30985=CIRCLE('',#96989,0.500000000000003);
#30986=CIRCLE('',#96990,0.993248606213802);
#30987=CIRCLE('',#96991,0.491297296891938);
#30988=CIRCLE('',#96993,58.1182624738004);
#30989=CIRCLE('',#96995,0.5);
#30990=CIRCLE('',#96996,2.5);
#30991=CIRCLE('',#96997,0.5);
#30992=CIRCLE('',#96998,3.);
#30993=CIRCLE('',#97000,0.5);
#30994=CIRCLE('',#97002,2.5);
#30995=CIRCLE('',#97003,0.5);
#30996=CIRCLE('',#97004,0.499999999999997);
#30997=CIRCLE('',#97005,0.500000000000003);
#30998=CIRCLE('',#97006,0.5);
#30999=CIRCLE('',#97008,0.5);
#31000=CIRCLE('',#97009,0.499999999999997);
#31001=CIRCLE('',#97010,0.499999999999998);
#31002=CIRCLE('',#97012,0.5);
#31003=CIRCLE('',#97013,2.5);
#31004=CIRCLE('',#97014,0.5);
#31005=CIRCLE('',#97016,0.5);
#31006=CIRCLE('',#97017,0.5);
#31007=CIRCLE('',#97018,0.499999999999999);
#31008=CIRCLE('',#97020,0.5);
#31009=CIRCLE('',#97021,0.500000000000003);
#31010=CIRCLE('',#97022,0.499999999999998);
#31011=CIRCLE('',#97023,0.499999999999997);
#31012=CIRCLE('',#97025,2.5);
#31013=CIRCLE('',#97026,0.5);
#31014=CIRCLE('',#97027,3.);
#31015=CIRCLE('',#97029,3.);
#31016=CIRCLE('',#97031,0.5);
#31017=CIRCLE('',#97032,2.5);
#31018=CIRCLE('',#97033,0.5);
#31019=CIRCLE('',#97035,0.5);
#31020=CIRCLE('',#97037,2.5);
#31021=CIRCLE('',#97038,0.5);
#31022=CIRCLE('',#97039,0.499999999999994);
#31023=CIRCLE('',#97040,0.499999999999999);
#31024=CIRCLE('',#97041,0.5);
#31025=CIRCLE('',#97043,0.5);
#31026=CIRCLE('',#97044,0.499999999999999);
#31027=CIRCLE('',#97045,0.500000000000001);
#31028=CIRCLE('',#97046,0.5);
#31029=CIRCLE('',#97047,0.500000000000003);
#31030=CIRCLE('',#97049,0.5);
#31031=CIRCLE('',#97050,0.499999999999994);
#31032=CIRCLE('',#97051,0.500000000000001);
#31033=CIRCLE('',#97052,0.500000000000005);
#31034=CIRCLE('',#97054,0.5);
#31035=CIRCLE('',#97055,0.5);
#31036=CIRCLE('',#97058,0.5);
#31037=CIRCLE('',#97059,0.5);
#31038=CIRCLE('',#97060,0.500000000000002);
#31039=CIRCLE('',#97061,0.499999999999998);
#31040=CIRCLE('',#97062,0.5);
#31041=CIRCLE('',#97064,0.5);
#31042=CIRCLE('',#97065,0.499999999999998);
#31043=CIRCLE('',#97066,0.499999999999998);
#31044=CIRCLE('',#97068,0.5);
#31045=CIRCLE('',#97069,0.499999999999999);
#31046=CIRCLE('',#97072,0.5);
#31047=CIRCLE('',#97073,0.499999999999998);
#31048=CIRCLE('',#97075,0.500000000000003);
#31049=CIRCLE('',#97076,0.499999999999994);
#31050=CIRCLE('',#97078,59.);
#31051=CIRCLE('',#97080,0.499999999999998);
#31052=CIRCLE('',#97081,0.5);
#31053=CIRCLE('',#97083,0.5);
#31054=CIRCLE('',#97087,58.4063077870366);
#31055=CIRCLE('',#97088,0.5);
#31056=CIRCLE('',#97091,68.1438279981623);
#31057=CIRCLE('',#97092,0.5);
#31058=CIRCLE('',#97096,58.4063077870367);
#31059=CIRCLE('',#97097,0.5);
#31060=CIRCLE('',#97102,59.);
#31061=CIRCLE('',#97104,0.5);
#31062=CIRCLE('',#97108,58.4063077870367);
#31063=CIRCLE('',#97109,0.5);
#31064=CIRCLE('',#97114,2.75);
#31065=CIRCLE('',#97116,2.75);
#31066=CIRCLE('',#97118,2.75);
#31067=CIRCLE('',#97120,2.75);
#31068=CIRCLE('',#97121,2.75);
#31069=CIRCLE('',#97124,3.);
#31070=CIRCLE('',#97126,67.5);
#31071=CIRCLE('',#97128,3.);
#31072=CIRCLE('',#97131,5.);
#31073=CIRCLE('',#97133,58.5);
#31074=CIRCLE('',#97135,5.);
#31075=CIRCLE('',#97138,3.);
#31076=CIRCLE('',#97140,67.5);
#31077=CIRCLE('',#97142,3.);
#31078=CIRCLE('',#97144,0.5);
#31079=CIRCLE('',#97145,0.499999999999999);
#31080=CIRCLE('',#97147,0.5);
#31081=CIRCLE('',#97148,0.5);
#31082=CIRCLE('',#97150,0.5);
#31083=CIRCLE('',#97151,0.5);
#31084=CIRCLE('',#97154,0.5);
#31085=CIRCLE('',#97155,0.5);
#31086=CIRCLE('',#97156,0.5);
#31087=CIRCLE('',#97157,1.);
#31088=CIRCLE('',#97159,1.);
#31089=CIRCLE('',#97160,0.5);
#31090=CIRCLE('',#97161,0.5);
#31091=CIRCLE('',#97163,0.5);
#31092=CIRCLE('',#97166,0.5);
#31093=CIRCLE('',#97167,0.5);
#31094=CIRCLE('',#97168,0.5);
#31095=CIRCLE('',#97169,1.);
#31096=CIRCLE('',#97171,1.);
#31097=CIRCLE('',#97172,0.5);
#31098=CIRCLE('',#97173,0.5);
#31099=CIRCLE('',#97175,0.5);
#31100=CIRCLE('',#97178,0.5);
#31101=CIRCLE('',#97179,0.5);
#31102=CIRCLE('',#97180,0.5);
#31103=CIRCLE('',#97181,1.);
#31104=CIRCLE('',#97184,0.499999999999998);
#31105=CIRCLE('',#97185,0.5);
#31106=CIRCLE('',#97186,0.551233577645565);
#31107=CIRCLE('',#97187,1.02402724953616);
#31108=CIRCLE('',#97189,0.5);
#31109=CIRCLE('',#97190,0.5);
#31110=CIRCLE('',#97192,64.5806717409052);
#31111=CIRCLE('',#97194,0.5);
#31112=CIRCLE('',#97195,0.5);
#31113=CIRCLE('',#97196,0.5);
#31114=CIRCLE('',#97199,0.5);
#31115=CIRCLE('',#97201,0.5);
#31116=CIRCLE('',#97202,0.5);
#31117=CIRCLE('',#97205,0.5);
#31118=CIRCLE('',#97206,0.5);
#31119=CIRCLE('',#97207,0.5);
#31120=CIRCLE('',#97208,0.500000000000001);
#31121=CIRCLE('',#97209,0.5);
#31122=CIRCLE('',#97211,0.5);
#31123=CIRCLE('',#97213,0.500000000000002);
#31124=CIRCLE('',#97214,3.5);
#31125=CIRCLE('',#97215,3.);
#31126=CIRCLE('',#97216,0.5);
#31127=CIRCLE('',#97219,0.5);
#31128=CIRCLE('',#97221,2.5);
#31129=CIRCLE('',#97222,0.5);
#31130=CIRCLE('',#97223,3.);
#31131=CIRCLE('',#97226,0.5);
#31132=CIRCLE('',#97228,2.75);
#31133=CIRCLE('',#97229,2.75);
#31134=CIRCLE('',#97230,2.75);
#31135=CIRCLE('',#97232,2.);
#31136=CIRCLE('',#97234,2.);
#31137=CIRCLE('',#97236,0.5);
#31138=CIRCLE('',#97238,0.5);
#31139=CIRCLE('',#97239,0.5);
#31140=CIRCLE('',#97240,0.500000000000002);
#31141=CIRCLE('',#97241,0.5);
#31142=CIRCLE('',#97243,0.5);
#31143=CIRCLE('',#97244,59.);
#31144=CIRCLE('',#97245,0.5);
#31145=CIRCLE('',#97246,0.5);
#31146=CIRCLE('',#97249,2.75);
#31147=CIRCLE('',#97250,2.75);
#31148=CIRCLE('',#97252,2.);
#31149=CIRCLE('',#97254,2.);
#31150=CIRCLE('',#97256,0.5);
#31151=CIRCLE('',#97258,59.024570260837);
#31152=CIRCLE('',#97260,0.5);
#31153=CIRCLE('',#97261,0.5);
#31154=CIRCLE('',#97266,0.5);
#31155=CIRCLE('',#97268,0.5);
#31156=CIRCLE('',#97274,0.5);
#31157=CIRCLE('',#97276,0.5);
#31158=CIRCLE('',#97283,0.5);
#31159=CIRCLE('',#97285,59.024570260837);
#31160=CIRCLE('',#97287,1.);
#31161=CIRCLE('',#97288,0.5);
#31162=CIRCLE('',#97292,0.5);
#31163=CIRCLE('',#97297,0.5);
#31164=CIRCLE('',#97298,0.5);
#31165=CIRCLE('',#97305,0.5);
#31166=CIRCLE('',#97306,0.5);
#31167=CIRCLE('',#97312,0.5);
#31168=CIRCLE('',#97313,0.5);
#31169=CIRCLE('',#97320,0.5);
#31170=CIRCLE('',#97322,59.024570260837);
#31171=CIRCLE('',#97325,0.5);
#31172=CIRCLE('',#97326,0.5);
#31173=CIRCLE('',#97332,0.5);
#31174=CIRCLE('',#97333,0.5);
#31175=CIRCLE('',#97337,0.5);
#31176=CIRCLE('',#97340,58.2938077870648);
#31177=CIRCLE('',#97344,0.5);
#31178=CIRCLE('',#97347,58.8875000000282);
#31179=CIRCLE('',#97351,0.5);
#31180=CIRCLE('',#97354,58.2938077870648);
#31181=CIRCLE('',#97358,0.5);
#31182=CIRCLE('',#97359,68.0339423779013);
#31183=CIRCLE('',#97362,0.5);
#31184=CIRCLE('',#97365,58.2938077870648);
#31185=CIRCLE('',#97369,0.5);
#31186=CIRCLE('',#97370,68.156308837608);
#31187=CIRCLE('',#97373,0.5);
#31188=CIRCLE('',#97376,58.2938077870648);
#31189=CIRCLE('',#97380,0.5);
#31190=CIRCLE('',#97381,67.990141838142);
#31191=CIRCLE('',#97384,0.5);
#31192=CIRCLE('',#97387,58.2938077870648);
#31193=CIRCLE('',#97391,0.5);
#31194=CIRCLE('',#97394,58.8875000000282);
#31195=CIRCLE('',#97398,0.5);
#31196=CIRCLE('',#97401,58.2938077870648);
#31197=CIRCLE('',#97402,0.5);
#31198=CIRCLE('',#97407,4.5);
#31199=CIRCLE('',#97413,4.5);
#31200=CIRCLE('',#97417,68.2241973717388);
#31201=CIRCLE('',#97420,0.5);
#31202=CIRCLE('',#97423,44.2689250265968);
#31203=CIRCLE('',#97424,58.2938077870648);
#31204=CIRCLE('',#97428,0.5);
#31205=CIRCLE('',#97429,64.7291249062775);
#31206=CIRCLE('',#97432,0.5);
#31207=CIRCLE('',#97435,58.2938077870648);
#31208=CIRCLE('',#97436,0.5);
#31209=CIRCLE('',#97442,58.8875000000282);
#31210=CIRCLE('',#97446,0.5);
#31211=CIRCLE('',#97448,58.2060351304332);
#31212=CIRCLE('',#97452,0.5);
#31213=CIRCLE('',#97455,58.2938077870648);
#31214=CIRCLE('',#97459,0.5);
#31215=CIRCLE('',#97462,58.8875000000282);
#31216=CIRCLE('',#97466,0.5);
#31217=CIRCLE('',#97467,0.5);
#31218=CIRCLE('',#97470,58.2938077870648);
#31219=CIRCLE('',#97474,0.5);
#31220=CIRCLE('',#97475,67.9422846909627);
#31221=CIRCLE('',#97478,0.5);
#31222=CIRCLE('',#97479,0.5);
#31223=CIRCLE('',#97482,58.2938077870648);
#31224=CIRCLE('',#97486,0.5);
#31225=CIRCLE('',#97487,0.5);
#31226=CIRCLE('',#97489,0.5);
#31227=CIRCLE('',#97491,0.500000000000001);
#31228=CIRCLE('',#97492,58.5);
#31229=CIRCLE('',#97493,0.499999999999999);
#31230=CIRCLE('',#97495,3.);
#31231=CIRCLE('',#97496,0.500000000000002);
#31232=CIRCLE('',#97497,0.5);
#31233=CIRCLE('',#97500,58.5);
#31234=CIRCLE('',#97502,0.5);
#31235=CIRCLE('',#97503,0.500000000000005);
#31236=CIRCLE('',#97504,57.916967095156);
#31237=CIRCLE('',#97505,0.499999999999999);
#31238=CIRCLE('',#97506,0.5);
#31239=CIRCLE('',#97509,58.5);
#31240=CIRCLE('',#97511,0.5);
#31241=CIRCLE('',#97512,0.500000000000005);
#31242=CIRCLE('',#97514,58.5);
#31243=CIRCLE('',#97515,0.500000000000002);
#31244=CIRCLE('',#97516,0.5);
#31245=CIRCLE('',#97519,58.5);
#31246=CIRCLE('',#97521,0.5);
#31247=CIRCLE('',#97523,2.75);
#31248=CIRCLE('',#97525,2.75);
#31249=CIRCLE('',#97527,0.250000000000002);
#31250=CIRCLE('',#97528,3.25);
#31251=CIRCLE('',#97529,0.250000000000003);
#31252=CIRCLE('',#97531,0.250000000000003);
#31253=CIRCLE('',#97533,2.75);
#31254=CIRCLE('',#97534,0.250000000000003);
#31255=CIRCLE('',#97536,67.25);
#31256=CIRCLE('',#97537,0.250000000000003);
#31257=CIRCLE('',#97539,2.75);
#31258=CIRCLE('',#97540,0.250000000000003);
#31259=CIRCLE('',#97542,0.249999999999997);
#31260=CIRCLE('',#97544,5.25);
#31261=CIRCLE('',#97545,0.249999999999997);
#31262=CIRCLE('',#97547,58.25);
#31263=CIRCLE('',#97548,0.249999999999997);
#31264=CIRCLE('',#97550,5.25);
#31265=CIRCLE('',#97551,0.249999999999997);
#31266=CIRCLE('',#97553,0.249999999999997);
#31267=CIRCLE('',#97555,2.75);
#31268=CIRCLE('',#97556,0.250000000000003);
#31269=CIRCLE('',#97558,67.25);
#31270=CIRCLE('',#97559,0.250000000000003);
#31271=CIRCLE('',#97561,2.75);
#31272=CIRCLE('',#97562,0.250000000000003);
#31273=CIRCLE('',#97564,0.250000000000003);
#31274=CIRCLE('',#97566,5.25);
#31275=CIRCLE('',#97567,0.249999999999998);
#31276=CIRCLE('',#97568,5.);
#31277=CIRCLE('',#97570,5.);
#31278=CIRCLE('',#97572,0.5);
#31279=CIRCLE('',#97574,0.500000000000003);
#31280=CIRCLE('',#97575,4.5);
#31281=CIRCLE('',#97577,3.);
#31282=CIRCLE('',#97580,0.5);
#31283=CIRCLE('',#97583,0.5);
#31284=CIRCLE('',#97585,0.5);
#31285=CIRCLE('',#97586,1.);
#31286=CIRCLE('',#97588,0.5);
#31287=CIRCLE('',#97590,0.5);
#31288=CIRCLE('',#97591,1.);
#31289=CIRCLE('',#97595,0.5);
#31290=CIRCLE('',#97597,0.5);
#31291=CIRCLE('',#97598,1.);
#31292=CIRCLE('',#97600,0.5);
#31293=CIRCLE('',#97602,0.5);
#31294=CIRCLE('',#97603,1.);
#31295=CIRCLE('',#97606,1.);
#31296=CIRCLE('',#97607,1.);
#31297=CIRCLE('',#97609,45.1752328136335);
#31298=CIRCLE('',#97611,0.5);
#31299=CIRCLE('',#97613,0.5);
#31300=CIRCLE('',#97614,0.999999999999999);
#31301=CIRCLE('',#97616,0.5);
#31302=CIRCLE('',#97618,0.5);
#31303=CIRCLE('',#97619,1.);
#31304=CIRCLE('',#97622,45.1752328136335);
#31305=CIRCLE('',#97624,0.5);
#31306=CIRCLE('',#97626,0.5);
#31307=CIRCLE('',#97627,1.);
#31308=CIRCLE('',#97629,0.5);
#31309=CIRCLE('',#97631,0.5);
#31310=CIRCLE('',#97632,1.);
#31311=CIRCLE('',#97634,0.5);
#31312=CIRCLE('',#97636,3.);
#31313=CIRCLE('',#97638,0.5);
#31314=CIRCLE('',#97640,1.);
#31315=CIRCLE('',#97641,0.500000000000001);
#31316=CIRCLE('',#97643,0.499999999999999);
#31317=CIRCLE('',#97645,0.5);
#31318=CIRCLE('',#97648,2.5);
#31319=CIRCLE('',#97649,58.8875000000282);
#31320=CIRCLE('',#97651,2.);
#31321=CIRCLE('',#97652,2.);
#31322=CIRCLE('',#97654,2.);
#31323=CIRCLE('',#97655,2.);
#31324=CIRCLE('',#97657,1.);
#31325=CIRCLE('',#97659,0.5);
#31326=CIRCLE('',#97660,0.5);
#31327=CIRCLE('',#97661,0.499999999999998);
#31328=CIRCLE('',#97663,0.499999999999998);
#31329=CIRCLE('',#97664,0.5);
#31330=CIRCLE('',#97668,0.5);
#31331=CIRCLE('',#97669,0.499999999999998);
#31332=CIRCLE('',#97671,0.499999999999998);
#31333=CIRCLE('',#97672,0.5);
#31334=CIRCLE('',#97675,1.);
#31335=CIRCLE('',#97676,0.500000000000004);
#31336=CIRCLE('',#97678,0.5);
#31337=CIRCLE('',#97681,0.5);
#31338=CIRCLE('',#97682,0.499999999999999);
#31339=CIRCLE('',#97684,0.499999999999999);
#31340=CIRCLE('',#97685,0.5);
#31341=CIRCLE('',#97688,0.999999999999998);
#31342=CIRCLE('',#97690,0.5);
#31343=CIRCLE('',#97691,0.5);
#31344=CIRCLE('',#97694,0.999999999999997);
#31345=CIRCLE('',#97696,0.5);
#31346=CIRCLE('',#97697,0.499999999999999);
#31347=CIRCLE('',#97699,0.499999999999999);
#31348=CIRCLE('',#97700,0.5);
#31349=CIRCLE('',#97704,1.);
#31350=CIRCLE('',#97705,0.999999999999996);
#31351=CIRCLE('',#97707,0.5);
#31352=CIRCLE('',#97708,0.499999999999999);
#31353=CIRCLE('',#97710,0.499999999999999);
#31354=CIRCLE('',#97711,0.5);
#31355=CIRCLE('',#97714,0.999999999999997);
#31356=CIRCLE('',#97715,1.);
#31357=CIRCLE('',#97717,0.5);
#31358=CIRCLE('',#97718,0.499999999999999);
#31359=CIRCLE('',#97720,0.499999999999999);
#31360=CIRCLE('',#97721,0.5);
#31361=CIRCLE('',#97724,0.999999999999997);
#31362=CIRCLE('',#97726,1.);
#31363=CIRCLE('',#97727,0.999999999999996);
#31364=CIRCLE('',#97729,0.5);
#31365=CIRCLE('',#97730,0.500000000000005);
#31366=CIRCLE('',#97732,0.500000000000005);
#31367=CIRCLE('',#97733,0.5);
#31368=CIRCLE('',#97736,0.999999999999996);
#31369=CIRCLE('',#97738,0.5);
#31370=CIRCLE('',#97739,0.499999999999999);
#31371=CIRCLE('',#97741,1.);
#31372=CIRCLE('',#97743,0.5);
#31373=CIRCLE('',#97744,0.500000000000005);
#31374=CIRCLE('',#97746,0.500000000000005);
#31375=CIRCLE('',#97747,0.5);
#31376=CIRCLE('',#97750,0.499999999999999);
#31377=CIRCLE('',#97751,0.5);
#31378=CIRCLE('',#97754,58.3875000000282);
#31379=CIRCLE('',#97756,0.5);
#31380=CIRCLE('',#97757,0.499999999999998);
#31381=CIRCLE('',#97759,58.3875000000282);
#31382=CIRCLE('',#97760,0.500000000000001);
#31383=CIRCLE('',#97761,0.5);
#31384=CIRCLE('',#97764,58.3875000000282);
#31385=CIRCLE('',#97766,0.5);
#31386=CIRCLE('',#97767,0.500000000000001);
#31387=CIRCLE('',#97768,0.499999999999997);
#31388=CIRCLE('',#97769,57.8151740222928);
#31389=CIRCLE('',#97770,0.5);
#31390=CIRCLE('',#97773,58.3875000000282);
#31391=CIRCLE('',#97775,0.5);
#31392=CIRCLE('',#97776,0.499999999999999);
#31393=CIRCLE('',#97777,0.499999999999998);
#31394=CIRCLE('',#97778,57.9942131824662);
#31395=CIRCLE('',#97779,0.5);
#31396=CIRCLE('',#97782,58.3875000000282);
#31397=CIRCLE('',#97784,0.5);
#31398=CIRCLE('',#97785,0.499999999999998);
#31399=CIRCLE('',#97786,0.500000000000001);
#31400=CIRCLE('',#97787,57.7939200874014);
#31401=CIRCLE('',#97788,0.5);
#31402=CIRCLE('',#97791,58.3875000000282);
#31403=CIRCLE('',#97793,0.5);
#31404=CIRCLE('',#97794,0.500000000000001);
#31405=CIRCLE('',#97796,58.3875000000282);
#31406=CIRCLE('',#97797,0.499999999999999);
#31407=CIRCLE('',#97798,0.5);
#31408=CIRCLE('',#97801,58.3875000000282);
#31409=CIRCLE('',#97803,0.5);
#31410=CIRCLE('',#97804,0.5);
#31411=CIRCLE('',#97807,3.);
#31412=CIRCLE('',#97810,3.);
#31413=CIRCLE('',#97812,3.);
#31414=CIRCLE('',#97815,3.);
#31415=CIRCLE('',#97816,0.500000000000002);
#31416=CIRCLE('',#97818,0.500000000000002);
#31417=CIRCLE('',#97819,5.);
#31418=CIRCLE('',#97820,1.40932613287356);
#31419=CIRCLE('',#97822,58.3875000000282);
#31420=CIRCLE('',#97824,5.);
#31421=CIRCLE('',#97825,0.500000000000002);
#31422=CIRCLE('',#97827,0.499999999999998);
#31423=CIRCLE('',#97828,5.);
#31424=CIRCLE('',#97830,0.5);
#31425=CIRCLE('',#97831,0.500000000000002);
#31426=CIRCLE('',#97832,57.9863561268404);
#31427=CIRCLE('',#97833,0.5);
#31428=CIRCLE('',#97834,0.5);
#31429=CIRCLE('',#97837,58.3875000000282);
#31430=CIRCLE('',#97839,0.5);
#31431=CIRCLE('',#97840,0.500000000000003);
#31432=CIRCLE('',#97841,56.5371804123359);
#31433=CIRCLE('',#97842,0.499999999999999);
#31434=CIRCLE('',#97843,0.5);
#31435=CIRCLE('',#97846,58.3875000000282);
#31436=CIRCLE('',#97848,0.5);
#31437=CIRCLE('',#97849,0.5);
#31438=CIRCLE('',#97851,58.3875000000282);
#31439=CIRCLE('',#97852,0.499999999999999);
#31440=CIRCLE('',#97853,0.5);
#31441=CIRCLE('',#97856,58.3875000000282);
#31442=CIRCLE('',#97858,5.);
#31443=CIRCLE('',#97860,0.499999999999997);
#31444=CIRCLE('',#97861,0.499999999999997);
#31445=CIRCLE('',#97862,58.3875000000282);
#31446=CIRCLE('',#97863,0.5);
#31447=CIRCLE('',#97866,58.3875000000282);
#31448=CIRCLE('',#97868,0.5);
#31449=CIRCLE('',#97869,0.499999999999999);
#31450=CIRCLE('',#97871,0.499999999999998);
#31451=CIRCLE('',#97872,58.3875000000282);
#31452=CIRCLE('',#97873,0.5);
#31453=CIRCLE('',#97876,58.3875000000282);
#31454=CIRCLE('',#97878,0.5);
#31455=CIRCLE('',#97879,0.499999999999994);
#31456=CIRCLE('',#97880,0.499999999999999);
#31457=CIRCLE('',#97881,57.7596339908634);
#31458=CIRCLE('',#97882,0.5);
#31459=CIRCLE('',#97883,0.5);
#31460=CIRCLE('',#97886,58.3875000000282);
#31461=CIRCLE('',#97888,0.5);
#31462=CIRCLE('',#97889,0.500000000000004);
#31463=CIRCLE('',#97891,58.3875000000282);
#31464=CIRCLE('',#97892,57.9914298998865);
#31465=CIRCLE('',#97895,3.);
#31466=CIRCLE('',#97898,3.);
#31467=CIRCLE('',#97900,3.);
#31468=CIRCLE('',#97903,3.);
#31469=CIRCLE('',#97904,0.499999999999997);
#31470=CIRCLE('',#97906,3.);
#31471=CIRCLE('',#97908,3.);
#31472=CIRCLE('',#97909,68.1760805737352);
#31473=CIRCLE('',#97910,121.707040772094);
#31474=CIRCLE('',#97912,109.54163477943);
#31475=CIRCLE('',#97913,68.2880455456965);
#31476=CIRCLE('',#97914,58.1059293197714);
#31477=CIRCLE('',#97916,58.5);
#31478=CIRCLE('',#97918,58.25);
#31479=CIRCLE('',#97920,58.25);
#31480=CIRCLE('',#97922,58.5);
#31481=CIRCLE('',#97924,58.5);
#31482=CIRCLE('',#97926,59.);
#31483=CIRCLE('',#97930,45.1752328136335);
#31484=CIRCLE('',#97932,44.2689250265968);
#31485=CIRCLE('',#97934,58.2938077870648);
#31486=CIRCLE('',#97936,58.3875000000282);
#31487=CIRCLE('',#97938,58.3875000000282);
#31488=CIRCLE('',#97940,5.);
#31489=CIRCLE('',#97950,1.73205080756888);
#31490=CIRCLE('',#97952,1.73205080756888);
#31491=CIRCLE('',#97954,1.73205080756888);
#31492=CIRCLE('',#97956,1.73205080756888);
#31493=CIRCLE('',#97958,1.73205080756888);
#31494=CIRCLE('',#97960,1.73205080756888);
#31495=CIRCLE('',#97962,3.);
#31496=CIRCLE('',#97963,0.25);
#31497=CIRCLE('',#97964,3.25);
#31498=CIRCLE('',#97965,3.25);
#31499=CIRCLE('',#97967,3.25);
#31500=CIRCLE('',#97971,2.);
#31501=CIRCLE('',#97972,1.47499999999998);
#31502=CIRCLE('',#97975,2.);
#31503=CIRCLE('',#97977,2.5);
#31504=CIRCLE('',#97979,2.5);
#31505=CIRCLE('',#97981,0.500000000000001);
#31506=CIRCLE('',#97982,0.499999999999997);
#31507=CIRCLE('',#97984,4.01589928084082);
#31508=CIRCLE('',#97985,0.5);
#31509=CIRCLE('',#97986,3.51597543326262);
#31510=CIRCLE('',#97987,3.51597543326262);
#31511=CIRCLE('',#97988,0.499999999999999);
#31512=CIRCLE('',#97989,0.500000000000002);
#31513=CIRCLE('',#97990,0.50000000000001);
#31514=CIRCLE('',#97992,0.500000000000004);
#31515=CIRCLE('',#97993,0.500000000000002);
#31516=CIRCLE('',#97994,0.499999999999999);
#31517=CIRCLE('',#97996,0.499999999999997);
#31518=CIRCLE('',#97997,2.);
#31519=CIRCLE('',#97998,1.49999999999999);
#31520=CIRCLE('',#97999,0.500000000000002);
#31521=CIRCLE('',#98001,0.5);
#31522=CIRCLE('',#98002,74.3);
#31523=CIRCLE('',#98003,73.8);
#31524=CIRCLE('',#98004,0.500000000000002);
#31525=CIRCLE('',#98006,0.499999999999999);
#31526=CIRCLE('',#98007,2.);
#31527=CIRCLE('',#98008,1.5);
#31528=CIRCLE('',#98009,0.499999999999993);
#31529=CIRCLE('',#98010,0.500000000000006);
#31530=CIRCLE('',#98011,0.500000000000012);
#31531=CIRCLE('',#98014,0.499999999999999);
#31532=CIRCLE('',#98015,0.500000000000001);
#31533=CIRCLE('',#98016,0.499999999999998);
#31534=CIRCLE('',#98017,0.5);
#31535=CIRCLE('',#98018,0.5);
#31536=CIRCLE('',#98019,0.500000000000006);
#31537=CIRCLE('',#98020,0.500000000000001);
#31538=CIRCLE('',#98022,0.500000000000003);
#31539=CIRCLE('',#98023,0.499999999999998);
#31540=CIRCLE('',#98024,0.50000000000001);
#31541=CIRCLE('',#98025,0.499999999999999);
#31542=CIRCLE('',#98026,0.499999999999999);
#31543=CIRCLE('',#98028,0.499999999999998);
#31544=CIRCLE('',#98029,1.5);
#31545=CIRCLE('',#98030,2.);
#31546=CIRCLE('',#98032,0.499999999999997);
#31547=CIRCLE('',#98033,0.499999999999998);
#31548=CIRCLE('',#98035,0.5);
#31549=CIRCLE('',#98036,73.8);
#31550=CIRCLE('',#98037,74.3);
#31551=CIRCLE('',#98038,0.499999999999997);
#31552=CIRCLE('',#98040,2.);
#31553=CIRCLE('',#98041,1.5);
#31554=CIRCLE('',#98043,0.500000000000001);
#31555=CIRCLE('',#98044,12.0057534629026);
#31556=CIRCLE('',#98045,0.500000000000002);
#31557=CIRCLE('',#98046,11.5058296153244);
#31558=CIRCLE('',#98048,0.500000000000001);
#31559=CIRCLE('',#98049,77.6552534828746);
#31560=CIRCLE('',#98050,77.1553296352964);
#31561=CIRCLE('',#98052,0.499999999999998);
#31562=CIRCLE('',#98053,12.0057534629026);
#31563=CIRCLE('',#98054,11.5058296153244);
#31564=CIRCLE('',#98056,0.499999999999998);
#31565=CIRCLE('',#98057,1067.5427534629);
#31566=CIRCLE('',#98058,1067.04282961532);
#31567=CIRCLE('',#98060,0.499999999999999);
#31568=CIRCLE('',#98061,12.0057534629025);
#31569=CIRCLE('',#98062,11.5058296153244);
#31570=CIRCLE('',#98064,0.500000000000001);
#31571=CIRCLE('',#98065,77.6552534828746);
#31572=CIRCLE('',#98066,77.1553296352964);
#31573=CIRCLE('',#98068,0.500000000000002);
#31574=CIRCLE('',#98069,12.0057534629026);
#31575=CIRCLE('',#98070,11.5058296153244);
#31576=CIRCLE('',#98071,64.9438263390348);
#31577=CIRCLE('',#98072,0.500000000000001);
#31578=CIRCLE('',#98073,64.8942562468481);
#31579=CIRCLE('',#98074,0.499999999999998);
#31580=CIRCLE('',#98076,0.499999999999996);
#31581=CIRCLE('',#98077,0.500000000000001);
#31582=CIRCLE('',#98078,0.50000000000001);
#31583=CIRCLE('',#98079,368.00584558015);
#31584=CIRCLE('',#98080,365.618325533514);
#31585=CIRCLE('',#98081,0.499999999999998);
#31586=CIRCLE('',#98082,431.08166328569);
#31587=CIRCLE('',#98083,429.776000990187);
#31588=CIRCLE('',#98084,0.5);
#31589=CIRCLE('',#98085,0.499999999999998);
#31590=CIRCLE('',#98086,0.5);
#31591=CIRCLE('',#98087,0.499999999999998);
#31592=CIRCLE('',#98088,0.499999999999998);
#31593=CIRCLE('',#98089,0.499999999999997);
#31594=CIRCLE('',#98091,77.1139810037387);
#31595=CIRCLE('',#98092,77.1139048513169);
#31596=CIRCLE('',#98093,0.500000000000002);
#31597=CIRCLE('',#98094,0.500000000000003);
#31598=CIRCLE('',#98096,0.499999999999998);
#31599=CIRCLE('',#98097,77.1139048513167);
#31600=CIRCLE('',#98098,77.1139810037385);
#31601=CIRCLE('',#98099,0.500000000000003);
#31602=CIRCLE('',#98100,0.5);
#31603=CIRCLE('',#98101,0.499999999999995);
#31604=CIRCLE('',#98102,0.500000000000002);
#31605=CIRCLE('',#98103,0.500000000000004);
#31606=CIRCLE('',#98104,329.616230392321);
#31607=CIRCLE('',#98105,329.186676134887);
#31608=CIRCLE('',#98106,0.499999999999997);
#31609=CIRCLE('',#98107,0.499999999999999);
#31610=CIRCLE('',#98108,462.991628528349);
#31611=CIRCLE('',#98109,463.797803513665);
#31612=CIRCLE('',#98111,0.750000000000001);
#31613=CIRCLE('',#98112,1.5);
#31614=CIRCLE('',#98113,0.750000000000001);
#31615=CIRCLE('',#98114,0.75);
#31616=CIRCLE('',#98116,73.05);
#31617=CIRCLE('',#98117,0.750000000000002);
#31618=CIRCLE('',#98118,73.8);
#31619=CIRCLE('',#98119,73.05);
#31620=CIRCLE('',#98120,0.749999999999996);
#31621=CIRCLE('',#98121,1.5);
#31622=CIRCLE('',#98122,0.750000000000001);
#31623=CIRCLE('',#98125,0.750000000000003);
#31624=CIRCLE('',#98126,1.5);
#31625=CIRCLE('',#98127,0.750000000000001);
#31626=CIRCLE('',#98128,0.750000000000004);
#31627=CIRCLE('',#98130,0.749999999999998);
#31628=CIRCLE('',#98131,77.1139048513167);
#31629=CIRCLE('',#98132,76.3639048513167);
#31630=CIRCLE('',#98133,0.75);
#31631=CIRCLE('',#98134,1.5);
#31632=CIRCLE('',#98135,0.750000000000001);
#31633=CIRCLE('',#98138,0.749999999999999);
#31634=CIRCLE('',#98139,0.749999999999999);
#31635=CIRCLE('',#98140,1.5);
#31636=CIRCLE('',#98141,0.750000000000001);
#31637=CIRCLE('',#98143,0.75);
#31638=CIRCLE('',#98144,77.1139048513169);
#31639=CIRCLE('',#98145,76.3639048513169);
#31640=CIRCLE('',#98146,0.750000000000001);
#31641=CIRCLE('',#98147,0.750000000000005);
#31642=CIRCLE('',#98148,1.5);
#31643=CIRCLE('',#98151,0.75);
#31644=CIRCLE('',#98152,0.750000000000003);
#31645=CIRCLE('',#98153,1.49999999999999);
#31646=CIRCLE('',#98154,0.749999999999994);
#31647=CIRCLE('',#98156,0.750000000000004);
#31648=CIRCLE('',#98157,73.8);
#31649=CIRCLE('',#98158,73.05);
#31650=CIRCLE('',#98159,0.750000000000001);
#31651=CIRCLE('',#98160,0.75);
#31652=CIRCLE('',#98161,1.5);
#31653=CIRCLE('',#98172,1.2);
#31654=CIRCLE('',#98173,0.450000000000006);
#31655=CIRCLE('',#98174,0.750000000000001);
#31656=CIRCLE('',#98175,0.450000000000001);
#31657=CIRCLE('',#98177,0.450000000000006);
#31658=CIRCLE('',#98179,0.45);
#31659=CIRCLE('',#98180,204.945690815561);
#31660=CIRCLE('',#98181,204.49569081556);
#31661=CIRCLE('',#98183,0.450000000000006);
#31662=CIRCLE('',#98184,0.750000000000001);
#31663=CIRCLE('',#98185,1.2);
#31664=CIRCLE('',#98187,0.450000000000001);
#31665=CIRCLE('',#98188,1.45);
#31666=CIRCLE('',#98189,1.);
#31667=CIRCLE('',#98191,0.450000000000006);
#31668=CIRCLE('',#98193,0.450000000000001);
#31669=CIRCLE('',#98194,48.45);
#31670=CIRCLE('',#98195,48.);
#31671=CIRCLE('',#98197,0.450000000000006);
#31672=CIRCLE('',#98198,0.750000000000001);
#31673=CIRCLE('',#98199,1.2);
#31674=CIRCLE('',#98201,0.450000000000006);
#31675=CIRCLE('',#98202,1.2);
#31676=CIRCLE('',#98203,0.750000000000001);
#31677=CIRCLE('',#98206,1.2);
#31678=CIRCLE('',#98207,0.450000000000006);
#31679=CIRCLE('',#98208,0.750000000000001);
#31680=CIRCLE('',#98209,0.450000000000001);
#31681=CIRCLE('',#98211,0.450000000000006);
#31682=CIRCLE('',#98213,0.449999999999999);
#31683=CIRCLE('',#98214,204.945690815561);
#31684=CIRCLE('',#98215,204.49569081556);
#31685=CIRCLE('',#98217,0.450000000000006);
#31686=CIRCLE('',#98218,0.750000000000001);
#31687=CIRCLE('',#98219,1.2);
#31688=CIRCLE('',#98221,0.450000000000006);
#31689=CIRCLE('',#98222,1.2);
#31690=CIRCLE('',#98223,0.750000000000001);
#31691=CIRCLE('',#98225,0.450000000000006);
#31692=CIRCLE('',#98227,0.450000000000006);
#31693=CIRCLE('',#98229,1.2);
#31694=CIRCLE('',#98230,0.750000000000001);
#31695=CIRCLE('',#98232,1.2);
#31696=CIRCLE('',#98233,0.450000000000006);
#31697=CIRCLE('',#98234,0.750000000000001);
#31698=CIRCLE('',#98235,0.449999999999999);
#31699=CIRCLE('',#98237,0.450000000000006);
#31700=CIRCLE('',#98239,0.450000000000001);
#31701=CIRCLE('',#98240,204.945690815561);
#31702=CIRCLE('',#98241,204.49569081556);
#31703=CIRCLE('',#98243,0.450000000000006);
#31704=CIRCLE('',#98244,0.750000000000001);
#31705=CIRCLE('',#98245,1.2);
#31706=CIRCLE('',#98247,0.450000000000006);
#31707=CIRCLE('',#98248,1.2);
#31708=CIRCLE('',#98249,0.750000000000001);
#31709=CIRCLE('',#98251,0.450000000000006);
#31710=CIRCLE('',#98253,0.450000000000006);
#31711=CIRCLE('',#98255,1.2);
#31712=CIRCLE('',#98256,0.750000000000001);
#31713=CIRCLE('',#98258,0.449999999999999);
#31714=CIRCLE('',#98259,1.2);
#31715=CIRCLE('',#98260,0.450000000000006);
#31716=CIRCLE('',#98261,0.750000000000001);
#31717=CIRCLE('',#98263,0.450000000000006);
#31718=CIRCLE('',#98265,0.450000000000006);
#31719=CIRCLE('',#98267,0.450000000000006);
#31720=CIRCLE('',#98268,0.750000000000001);
#31721=CIRCLE('',#98269,1.2);
#31722=CIRCLE('',#98271,0.450000000000006);
#31723=CIRCLE('',#98272,1.2);
#31724=CIRCLE('',#98273,0.750000000000001);
#31725=CIRCLE('',#98275,0.450000000000006);
#31726=CIRCLE('',#98277,0.450000000000006);
#31727=CIRCLE('',#98279,1.2);
#31728=CIRCLE('',#98280,0.750000000000001);
#31729=CIRCLE('',#98282,0.450000000000006);
#31730=CIRCLE('',#98283,1.2);
#31731=CIRCLE('',#98284,0.450000000000006);
#31732=CIRCLE('',#98285,0.750000000000001);
#31733=CIRCLE('',#98287,0.450000000000006);
#31734=CIRCLE('',#98289,0.450000000000006);
#31735=CIRCLE('',#98291,0.45);
#31736=CIRCLE('',#98292,0.75);
#31737=CIRCLE('',#98293,1.2);
#31738=CIRCLE('',#98295,0.450000000000006);
#31739=CIRCLE('',#98296,1.2);
#31740=CIRCLE('',#98297,0.750000000000001);
#31741=CIRCLE('',#98299,0.45);
#31742=CIRCLE('',#98300,13.1055395526668);
#31743=CIRCLE('',#98301,12.6555395526668);
#31744=CIRCLE('',#98303,0.450000000000001);
#31745=CIRCLE('',#98305,0.45);
#31746=CIRCLE('',#98306,10.);
#31747=CIRCLE('',#98307,10.45);
#31748=CIRCLE('',#98309,0.75);
#31749=CIRCLE('',#98310,1.2);
#31750=CIRCLE('',#98312,0.450000000000006);
#31751=CIRCLE('',#98313,1.2);
#31752=CIRCLE('',#98314,0.450000000000006);
#31753=CIRCLE('',#98315,0.750000000000001);
#31754=CIRCLE('',#98317,0.450000000000001);
#31755=CIRCLE('',#98319,0.450000000000006);
#31756=CIRCLE('',#98321,0.450000000000006);
#31757=CIRCLE('',#98322,0.75);
#31758=CIRCLE('',#98323,1.2);
#31759=CIRCLE('',#98325,0.450000000000006);
#31760=CIRCLE('',#98326,1.2);
#31761=CIRCLE('',#98327,0.750000000000001);
#31762=CIRCLE('',#98329,0.450000000000006);
#31763=CIRCLE('',#98331,0.449999999999999);
#31764=CIRCLE('',#98333,1.2);
#31765=CIRCLE('',#98334,0.75);
#31766=CIRCLE('',#98336,0.450000000000006);
#31767=CIRCLE('',#98337,1.2);
#31768=CIRCLE('',#98338,0.450000000000006);
#31769=CIRCLE('',#98339,0.750000000000001);
#31770=CIRCLE('',#98341,0.450000000000006);
#31771=CIRCLE('',#98343,0.450000000000006);
#31772=CIRCLE('',#98345,0.450000000000006);
#31773=CIRCLE('',#98346,0.750000000000001);
#31774=CIRCLE('',#98347,1.2);
#31775=CIRCLE('',#98349,0.450000000000006);
#31776=CIRCLE('',#98350,1.2);
#31777=CIRCLE('',#98351,0.750000000000001);
#31778=CIRCLE('',#98353,0.450000000000006);
#31779=CIRCLE('',#98355,0.450000000000006);
#31780=CIRCLE('',#98357,1.2);
#31781=CIRCLE('',#98358,0.750000000000001);
#31782=CIRCLE('',#98360,0.450000000000006);
#31783=CIRCLE('',#98361,1.2);
#31784=CIRCLE('',#98362,0.450000000000006);
#31785=CIRCLE('',#98363,0.750000000000001);
#31786=CIRCLE('',#98365,0.450000000000006);
#31787=CIRCLE('',#98367,0.450000000000006);
#31788=CIRCLE('',#98369,0.450000000000006);
#31789=CIRCLE('',#98370,0.750000000000001);
#31790=CIRCLE('',#98371,1.2);
#31791=CIRCLE('',#98373,0.450000000000006);
#31792=CIRCLE('',#98374,1.2);
#31793=CIRCLE('',#98375,0.750000000000001);
#31794=CIRCLE('',#98377,0.450000000000006);
#31795=CIRCLE('',#98379,0.450000000000006);
#31796=CIRCLE('',#98381,1.2);
#31797=CIRCLE('',#98382,0.750000000000001);
#31798=CIRCLE('',#98384,0.450000000000006);
#31799=CIRCLE('',#98385,1.2);
#31800=CIRCLE('',#98386,0.450000000000006);
#31801=CIRCLE('',#98387,0.750000000000001);
#31802=CIRCLE('',#98389,0.449999999999999);
#31803=CIRCLE('',#98391,0.450000000000006);
#31804=CIRCLE('',#98393,0.450000000000006);
#31805=CIRCLE('',#98394,0.75);
#31806=CIRCLE('',#98395,1.2);
#31807=CIRCLE('',#98397,0.450000000000006);
#31808=CIRCLE('',#98398,1.2);
#31809=CIRCLE('',#98399,0.750000000000001);
#31810=CIRCLE('',#98401,0.450000000000006);
#31811=CIRCLE('',#98403,0.450000000000006);
#31812=CIRCLE('',#98405,1.2);
#31813=CIRCLE('',#98406,0.75);
#31814=CIRCLE('',#98408,0.450000000000006);
#31815=CIRCLE('',#98409,1.2);
#31816=CIRCLE('',#98410,0.450000000000006);
#31817=CIRCLE('',#98411,0.750000000000001);
#31818=CIRCLE('',#98413,0.449999999999999);
#31819=CIRCLE('',#98415,0.450000000000006);
#31820=CIRCLE('',#98417,0.450000000000006);
#31821=CIRCLE('',#98418,0.75);
#31822=CIRCLE('',#98419,1.2);
#31823=CIRCLE('',#98421,0.449999999999997);
#31824=CIRCLE('',#98422,1.2);
#31825=CIRCLE('',#98423,0.750000000000001);
#31826=CIRCLE('',#98425,0.450000000000006);
#31827=CIRCLE('',#98427,0.449999999999998);
#31828=CIRCLE('',#98428,677.884816028482);
#31829=CIRCLE('',#98429,677.434816028482);
#31830=CIRCLE('',#98431,1.2);
#31831=CIRCLE('',#98432,0.75);
#31832=CIRCLE('',#98434,0.450000000000006);
#31833=CIRCLE('',#98435,1.2);
#31834=CIRCLE('',#98436,0.450000000000006);
#31835=CIRCLE('',#98437,0.750000000000001);
#31836=CIRCLE('',#98439,0.450000000000006);
#31837=CIRCLE('',#98441,0.450000000000006);
#31838=CIRCLE('',#98443,0.450000000000006);
#31839=CIRCLE('',#98444,0.750000000000001);
#31840=CIRCLE('',#98445,1.2);
#31841=CIRCLE('',#98447,0.449999999999998);
#31842=CIRCLE('',#98448,1.2);
#31843=CIRCLE('',#98449,0.750000000000001);
#31844=CIRCLE('',#98451,0.450000000000006);
#31845=CIRCLE('',#98453,0.45);
#31846=CIRCLE('',#98454,48.45);
#31847=CIRCLE('',#98455,48.);
#31848=CIRCLE('',#98457,0.449999999999997);
#31849=CIRCLE('',#98458,0.750000000000001);
#31850=CIRCLE('',#98459,1.2);
#31851=CIRCLE('',#98461,0.449999999999997);
#31852=CIRCLE('',#98462,1.45);
#31853=CIRCLE('',#98463,0.999999999999999);
#31854=CIRCLE('',#98465,677.884816028482);
#31855=CIRCLE('',#98466,677.434816028482);
#31856=CIRCLE('',#98468,0.450000000000006);
#31857=CIRCLE('',#98469,1.2);
#31858=CIRCLE('',#98470,0.450000000000006);
#31859=CIRCLE('',#98471,0.75);
#31860=CIRCLE('',#98473,0.449999999999999);
#31861=CIRCLE('',#98475,0.450000000000006);
#31862=CIRCLE('',#98477,0.450000000000006);
#31863=CIRCLE('',#98478,0.750000000000001);
#31864=CIRCLE('',#98479,1.2);
#31865=CIRCLE('',#98481,0.45);
#31866=CIRCLE('',#98482,1.2);
#31867=CIRCLE('',#98483,0.75);
#31868=CIRCLE('',#98485,0.450000000000006);
#31869=CIRCLE('',#98487,0.449999999999999);
#31870=CIRCLE('',#98488,677.884816028482);
#31871=CIRCLE('',#98489,677.434816028482);
#31872=CIRCLE('',#98491,1.2);
#31873=CIRCLE('',#98492,0.750000000000001);
#31874=CIRCLE('',#98494,0.450000000000006);
#31875=CIRCLE('',#98495,1.2);
#31876=CIRCLE('',#98496,0.450000000000006);
#31877=CIRCLE('',#98497,0.75);
#31878=CIRCLE('',#98499,0.449999999999999);
#31879=CIRCLE('',#98501,0.450000000000006);
#31880=CIRCLE('',#98503,0.450000000000006);
#31881=CIRCLE('',#98504,0.750000000000001);
#31882=CIRCLE('',#98505,1.2);
#31883=CIRCLE('',#98507,0.450000000000006);
#31884=CIRCLE('',#98508,1.2);
#31885=CIRCLE('',#98509,0.75);
#31886=CIRCLE('',#98511,0.450000000000006);
#31887=CIRCLE('',#98513,0.450000000000006);
#31888=CIRCLE('',#98515,1.2);
#31889=CIRCLE('',#98516,0.750000000000001);
#31890=CIRCLE('',#98518,0.45);
#31891=CIRCLE('',#98519,1.2);
#31892=CIRCLE('',#98520,0.450000000000006);
#31893=CIRCLE('',#98521,0.750000000000001);
#31894=CIRCLE('',#98523,0.450000000000006);
#31895=CIRCLE('',#98525,0.45);
#31896=CIRCLE('',#98526,11.6555395526668);
#31897=CIRCLE('',#98527,12.1055395526668);
#31898=CIRCLE('',#98529,0.450000000000006);
#31899=CIRCLE('',#98530,0.750000000000001);
#31900=CIRCLE('',#98531,1.2);
#31901=CIRCLE('',#98533,0.450000000000006);
#31902=CIRCLE('',#98534,10.45);
#31903=CIRCLE('',#98535,10.);
#31904=CIRCLE('',#98537,0.450000000000006);
#31905=CIRCLE('',#98539,0.450000000000006);
#31906=CIRCLE('',#98541,0.450000000000006);
#31907=CIRCLE('',#98542,0.75);
#31908=CIRCLE('',#98543,1.2);
#31909=CIRCLE('',#98545,0.450000000000006);
#31910=CIRCLE('',#98546,1.2);
#31911=CIRCLE('',#98547,0.75);
#31912=CIRCLE('',#98550,0.450000000000001);
#31913=CIRCLE('',#98551,1.2);
#31914=CIRCLE('',#98552,0.450000000000006);
#31915=CIRCLE('',#98553,0.750000000000001);
#31916=CIRCLE('',#98555,0.450000000000006);
#31917=CIRCLE('',#98557,0.450000000000006);
#31918=CIRCLE('',#98559,0.450000000000006);
#31919=CIRCLE('',#98560,0.750000000000001);
#31920=CIRCLE('',#98561,1.2);
#31921=CIRCLE('',#98563,0.450000000000001);
#31922=CIRCLE('',#98564,10.45);
#31923=CIRCLE('',#98565,10.);
#31924=CIRCLE('',#98567,0.449999999999999);
#31925=CIRCLE('',#98569,0.45);
#31926=CIRCLE('',#98570,11.6555395526668);
#31927=CIRCLE('',#98571,12.1055395526668);
#31928=CIRCLE('',#98573,0.450000000000006);
#31929=CIRCLE('',#98574,0.750000000000001);
#31930=CIRCLE('',#98575,1.2);
#31931=CIRCLE('',#98577,0.450000000000006);
#31932=CIRCLE('',#98578,1.2);
#31933=CIRCLE('',#98579,0.750000000000001);
#31934=CIRCLE('',#98582,0.450000000000006);
#31935=CIRCLE('',#98583,1.2);
#31936=CIRCLE('',#98584,0.450000000000006);
#31937=CIRCLE('',#98585,0.750000000000001);
#31938=CIRCLE('',#98587,0.450000000000006);
#31939=CIRCLE('',#98589,0.450000000000006);
#31940=CIRCLE('',#98591,0.450000000000006);
#31941=CIRCLE('',#98592,0.750000000000001);
#31942=CIRCLE('',#98593,1.2);
#31943=CIRCLE('',#98595,0.450000000000006);
#31944=CIRCLE('',#98596,1.2);
#31945=CIRCLE('',#98597,0.750000000000001);
#31946=CIRCLE('',#98599,0.449999999999999);
#31947=CIRCLE('',#98601,0.450000000000006);
#31948=CIRCLE('',#98603,1.2);
#31949=CIRCLE('',#98604,0.750000000000001);
#31950=CIRCLE('',#98606,0.450000000000006);
#31951=CIRCLE('',#98607,1.2);
#31952=CIRCLE('',#98608,0.450000000000006);
#31953=CIRCLE('',#98609,0.750000000000001);
#31954=CIRCLE('',#98611,0.450000000000006);
#31955=CIRCLE('',#98613,0.450000000000006);
#31956=CIRCLE('',#98615,0.45);
#31957=CIRCLE('',#98616,0.750000000000001);
#31958=CIRCLE('',#98617,1.2);
#31959=CIRCLE('',#98619,0.450000000000006);
#31960=CIRCLE('',#98620,1.2);
#31961=CIRCLE('',#98621,0.750000000000001);
#31962=CIRCLE('',#98623,0.449999999999999);
#31963=CIRCLE('',#98624,677.434816028482);
#31964=CIRCLE('',#98625,677.884816028482);
#31965=CIRCLE('',#98627,0.450000000000006);
#31966=CIRCLE('',#98629,1.2);
#31967=CIRCLE('',#98630,0.750000000000001);
#31968=CIRCLE('',#98632,0.450000000000006);
#31969=CIRCLE('',#98633,1.2);
#31970=CIRCLE('',#98634,0.450000000000006);
#31971=CIRCLE('',#98635,0.750000000000001);
#31972=CIRCLE('',#98637,0.450000000000006);
#31973=CIRCLE('',#98639,0.450000000000006);
#31974=CIRCLE('',#98641,0.450000000000006);
#31975=CIRCLE('',#98642,0.750000000000001);
#31976=CIRCLE('',#98643,1.2);
#31977=CIRCLE('',#98645,0.450000000000006);
#31978=CIRCLE('',#98646,1.2);
#31979=CIRCLE('',#98647,0.750000000000001);
#31980=CIRCLE('',#98649,0.449999999999999);
#31981=CIRCLE('',#98651,0.450000000000006);
#31982=CIRCLE('',#98653,1.2);
#31983=CIRCLE('',#98654,0.750000000000001);
#31984=CIRCLE('',#98656,0.450000000000006);
#31985=CIRCLE('',#98657,1.2);
#31986=CIRCLE('',#98658,0.450000000000006);
#31987=CIRCLE('',#98659,0.750000000000001);
#31988=CIRCLE('',#98661,0.450000000000006);
#31989=CIRCLE('',#98663,0.450000000000006);
#31990=CIRCLE('',#98665,0.450000000000006);
#31991=CIRCLE('',#98666,0.750000000000001);
#31992=CIRCLE('',#98667,1.2);
#31993=CIRCLE('',#98669,0.450000000000006);
#31994=CIRCLE('',#98670,1.2);
#31995=CIRCLE('',#98671,0.750000000000001);
#31996=CIRCLE('',#98673,0.450000000000001);
#31997=CIRCLE('',#98675,0.450000000000006);
#31998=CIRCLE('',#98677,1.2);
#31999=CIRCLE('',#98678,0.750000000000001);
#32000=CIRCLE('',#98680,0.450000000000006);
#32001=CIRCLE('',#98681,1.2);
#32002=CIRCLE('',#98682,0.449999999999999);
#32003=CIRCLE('',#98683,0.750000000000001);
#32004=CIRCLE('',#98685,0.450000000000006);
#32005=CIRCLE('',#98687,0.450000000000006);
#32006=CIRCLE('',#98689,0.450000000000006);
#32007=CIRCLE('',#98690,0.750000000000001);
#32008=CIRCLE('',#98691,1.2);
#32009=CIRCLE('',#98693,0.45);
#32010=CIRCLE('',#98694,1.2);
#32011=CIRCLE('',#98695,0.750000000000001);
#32012=CIRCLE('',#98697,0.450000000000006);
#32013=CIRCLE('',#98699,0.45);
#32014=CIRCLE('',#98700,12.6555395526668);
#32015=CIRCLE('',#98701,13.1055395526668);
#32016=CIRCLE('',#98703,1.2);
#32017=CIRCLE('',#98704,0.450000000000001);
#32018=CIRCLE('',#98705,0.750000000000001);
#32019=CIRCLE('',#98707,10.);
#32020=CIRCLE('',#98708,10.45);
#32021=CIRCLE('',#98710,0.450000000000006);
#32022=CIRCLE('',#98711,1.2);
#32023=CIRCLE('',#98712,0.450000000000006);
#32024=CIRCLE('',#98713,0.750000000000001);
#32025=CIRCLE('',#98715,0.450000000000006);
#32026=CIRCLE('',#98717,0.450000000000006);
#32027=CIRCLE('',#98719,0.449999999999997);
#32028=CIRCLE('',#98720,0.750000000000001);
#32029=CIRCLE('',#98721,1.2);
#32030=CIRCLE('',#98723,0.450000000000006);
#32031=CIRCLE('',#98724,1.2);
#32032=CIRCLE('',#98725,0.750000000000001);
#32033=CIRCLE('',#98727,0.449999999999998);
#32034=CIRCLE('',#98728,677.434816028482);
#32035=CIRCLE('',#98729,677.884816028482);
#32036=CIRCLE('',#98731,0.450000000000006);
#32037=CIRCLE('',#98733,1.2);
#32038=CIRCLE('',#98734,0.750000000000001);
#32039=CIRCLE('',#98736,0.449999999999999);
#32040=CIRCLE('',#98737,1.2);
#32041=CIRCLE('',#98738,0.450000000000006);
#32042=CIRCLE('',#98739,0.750000000000001);
#32043=CIRCLE('',#98741,0.450000000000006);
#32044=CIRCLE('',#98743,0.450000000000006);
#32045=CIRCLE('',#98745,0.45);
#32046=CIRCLE('',#98746,0.750000000000001);
#32047=CIRCLE('',#98747,1.2);
#32048=CIRCLE('',#98749,0.450000000000006);
#32049=CIRCLE('',#98750,1.2);
#32050=CIRCLE('',#98751,0.750000000000001);
#32051=CIRCLE('',#98753,0.45);
#32052=CIRCLE('',#98754,48.);
#32053=CIRCLE('',#98755,48.45);
#32054=CIRCLE('',#98757,0.450000000000006);
#32055=CIRCLE('',#98759,0.449999999999997);
#32056=CIRCLE('',#98760,1.);
#32057=CIRCLE('',#98761,1.45);
#32058=CIRCLE('',#98763,0.449999999999997);
#32059=CIRCLE('',#98764,1.2);
#32060=CIRCLE('',#98765,0.750000000000001);
#32061=CIRCLE('',#98767,677.884816028482);
#32062=CIRCLE('',#98768,677.434816028482);
#32063=CIRCLE('',#98770,0.450000000000006);
#32064=CIRCLE('',#98771,1.2);
#32065=CIRCLE('',#98772,0.450000000000006);
#32066=CIRCLE('',#98773,0.750000000000001);
#32067=CIRCLE('',#98775,0.450000000000006);
#32068=CIRCLE('',#98777,0.450000000000006);
#32069=CIRCLE('',#98779,0.450000000000006);
#32070=CIRCLE('',#98780,0.750000000000001);
#32071=CIRCLE('',#98781,1.2);
#32072=CIRCLE('',#98783,0.450000000000006);
#32073=CIRCLE('',#98784,1.2);
#32074=CIRCLE('',#98785,0.750000000000001);
#32075=CIRCLE('',#98787,0.449999999999999);
#32076=CIRCLE('',#98789,0.450000000000006);
#32077=CIRCLE('',#98791,1.2);
#32078=CIRCLE('',#98792,0.750000000000001);
#32079=CIRCLE('',#98794,0.449999999999999);
#32080=CIRCLE('',#98795,1.2);
#32081=CIRCLE('',#98796,0.450000000000006);
#32082=CIRCLE('',#98797,0.750000000000001);
#32083=CIRCLE('',#98799,0.450000000000006);
#32084=CIRCLE('',#98801,0.450000000000006);
#32085=CIRCLE('',#98803,0.450000000000006);
#32086=CIRCLE('',#98804,0.750000000000001);
#32087=CIRCLE('',#98805,1.2);
#32088=CIRCLE('',#98807,0.45);
#32089=CIRCLE('',#98808,1.2);
#32090=CIRCLE('',#98809,0.750000000000001);
#32091=CIRCLE('',#98811,0.450000000000006);
#32092=CIRCLE('',#98813,0.45);
#32093=CIRCLE('',#98814,48.45);
#32094=CIRCLE('',#98815,48.);
#32095=CIRCLE('',#98817,0.450000000000003);
#32096=CIRCLE('',#98818,0.750000000000001);
#32097=CIRCLE('',#98819,1.2);
#32098=CIRCLE('',#98821,0.450000000000001);
#32099=CIRCLE('',#98822,1.44999999999997);
#32100=CIRCLE('',#98823,0.999999999999959);
#32101=CIRCLE('',#98825,677.884816028482);
#32102=CIRCLE('',#98826,677.434816028482);
#32103=CIRCLE('',#98828,0.449999999999999);
#32104=CIRCLE('',#98829,1.2);
#32105=CIRCLE('',#98830,0.450000000000006);
#32106=CIRCLE('',#98831,0.750000000000001);
#32107=CIRCLE('',#98833,0.450000000000006);
#32108=CIRCLE('',#98835,0.450000000000006);
#32109=CIRCLE('',#98837,0.450000000000006);
#32110=CIRCLE('',#98838,0.750000000000001);
#32111=CIRCLE('',#98839,1.2);
#32112=CIRCLE('',#98841,0.450000000000003);
#32113=CIRCLE('',#98842,1.2);
#32114=CIRCLE('',#98843,0.750000000000001);
#32115=CIRCLE('',#98845,0.450000000000006);
#32116=CIRCLE('',#98847,0.449999999999998);
#32117=CIRCLE('',#98848,677.884816028482);
#32118=CIRCLE('',#98849,677.434816028482);
#32119=CIRCLE('',#98851,1.2);
#32120=CIRCLE('',#98852,0.750000000000001);
#32121=CIRCLE('',#98854,0.450000000000001);
#32122=CIRCLE('',#98855,1.2);
#32123=CIRCLE('',#98856,0.450000000000006);
#32124=CIRCLE('',#98857,0.750000000000001);
#32125=CIRCLE('',#98859,0.450000000000006);
#32126=CIRCLE('',#98861,0.450000000000006);
#32127=CIRCLE('',#98863,0.450000000000006);
#32128=CIRCLE('',#98864,0.750000000000001);
#32129=CIRCLE('',#98865,1.2);
#32130=CIRCLE('',#98867,0.450000000000006);
#32131=CIRCLE('',#98868,1.2);
#32132=CIRCLE('',#98869,0.750000000000001);
#32133=CIRCLE('',#98871,0.449999999999999);
#32134=CIRCLE('',#98873,0.450000000000006);
#32135=CIRCLE('',#98875,1.2);
#32136=CIRCLE('',#98876,0.750000000000001);
#32137=CIRCLE('',#98878,0.450000000000006);
#32138=CIRCLE('',#98879,1.2);
#32139=CIRCLE('',#98880,0.450000000000006);
#32140=CIRCLE('',#98881,0.750000000000001);
#32141=CIRCLE('',#98883,0.449999999999999);
#32142=CIRCLE('',#98885,0.450000000000006);
#32143=CIRCLE('',#98887,0.450000000000006);
#32144=CIRCLE('',#98888,0.750000000000001);
#32145=CIRCLE('',#98889,1.2);
#32146=CIRCLE('',#98891,0.449999999999999);
#32147=CIRCLE('',#98892,1.2);
#32148=CIRCLE('',#98893,0.750000000000001);
#32149=CIRCLE('',#98895,0.450000000000006);
#32150=CIRCLE('',#98897,0.449999999999999);
#32151=CIRCLE('',#98898,677.884816028482);
#32152=CIRCLE('',#98899,677.434816028482);
#32153=CIRCLE('',#98901,1.2);
#32154=CIRCLE('',#98902,0.750000000000001);
#32155=CIRCLE('',#98904,0.450000000000006);
#32156=CIRCLE('',#98905,1.2);
#32157=CIRCLE('',#98906,0.449999999999999);
#32158=CIRCLE('',#98907,0.750000000000001);
#32159=CIRCLE('',#98909,0.450000000000006);
#32160=CIRCLE('',#98911,0.450000000000006);
#32161=CIRCLE('',#98913,0.450000000000006);
#32162=CIRCLE('',#98914,0.750000000000001);
#32163=CIRCLE('',#98915,1.2);
#32164=CIRCLE('',#98917,0.449999999999999);
#32165=CIRCLE('',#98918,1.2);
#32166=CIRCLE('',#98919,0.750000000000001);
#32167=CIRCLE('',#98921,0.450000000000006);
#32168=CIRCLE('',#98923,0.450000000000006);
#32169=CIRCLE('',#98925,1.2);
#32170=CIRCLE('',#98926,0.750000000000001);
#32171=CIRCLE('',#98928,0.449999999999999);
#32172=CIRCLE('',#98929,1.2);
#32173=CIRCLE('',#98930,0.450000000000006);
#32174=CIRCLE('',#98931,0.750000000000001);
#32175=CIRCLE('',#98933,0.450000000000006);
#32176=CIRCLE('',#98935,0.45);
#32177=CIRCLE('',#98936,48.45);
#32178=CIRCLE('',#98937,48.);
#32179=CIRCLE('',#98939,0.450000000000006);
#32180=CIRCLE('',#98940,0.750000000000001);
#32181=CIRCLE('',#98941,1.2);
#32182=CIRCLE('',#98943,0.450000000000006);
#32183=CIRCLE('',#98944,1.2);
#32184=CIRCLE('',#98945,0.750000000000001);
#32185=CIRCLE('',#98948,1.2);
#32186=CIRCLE('',#98949,0.450000000000006);
#32187=CIRCLE('',#98950,0.750000000000001);
#32188=CIRCLE('',#98951,0.450000000000002);
#32189=CIRCLE('',#98953,0.450000000000006);
#32190=CIRCLE('',#98955,0.449999999999999);
#32191=CIRCLE('',#98956,48.45);
#32192=CIRCLE('',#98957,48.);
#32193=CIRCLE('',#98959,0.450000000000006);
#32194=CIRCLE('',#98960,0.750000000000001);
#32195=CIRCLE('',#98961,1.2);
#32196=CIRCLE('',#98963,0.450000000000006);
#32197=CIRCLE('',#98964,1.2);
#32198=CIRCLE('',#98965,0.750000000000001);
#32199=CIRCLE('',#98968,0.450000000000002);
#32200=CIRCLE('',#98969,5.99999999999992);
#32201=CIRCLE('',#98970,0.45);
#32202=CIRCLE('',#98971,6.44999999999991);
#32203=CIRCLE('',#98973,0.45);
#32204=CIRCLE('',#98974,53.);
#32205=CIRCLE('',#98975,53.45);
#32206=CIRCLE('',#98977,0.449999999999997);
#32207=CIRCLE('',#98978,6.);
#32208=CIRCLE('',#98979,6.45);
#32209=CIRCLE('',#98981,0.449999999999997);
#32210=CIRCLE('',#98982,682.434816028482);
#32211=CIRCLE('',#98983,682.884816028482);
#32212=CIRCLE('',#98985,0.45);
#32213=CIRCLE('',#98986,6.);
#32214=CIRCLE('',#98987,6.45);
#32215=CIRCLE('',#98989,0.449999999999998);
#32216=CIRCLE('',#98990,53.);
#32217=CIRCLE('',#98991,53.45);
#32218=CIRCLE('',#98993,0.45);
#32219=CIRCLE('',#98994,6.);
#32220=CIRCLE('',#98995,6.45);
#32221=CIRCLE('',#98997,0.450000000000002);
#32222=CIRCLE('',#98998,4.34999999999995);
#32223=CIRCLE('',#98999,0.45);
#32224=CIRCLE('',#99000,4.8);
#32225=CIRCLE('',#99002,0.45);
#32226=CIRCLE('',#99003,51.35);
#32227=CIRCLE('',#99004,51.8);
#32228=CIRCLE('',#99006,0.449999999999997);
#32229=CIRCLE('',#99007,4.35);
#32230=CIRCLE('',#99008,4.8);
#32231=CIRCLE('',#99010,0.449999999999997);
#32232=CIRCLE('',#99011,680.784816028482);
#32233=CIRCLE('',#99012,681.234816028482);
#32234=CIRCLE('',#99014,0.45);
#32235=CIRCLE('',#99015,4.35);
#32236=CIRCLE('',#99016,4.8);
#32237=CIRCLE('',#99018,0.450000000000002);
#32238=CIRCLE('',#99019,51.35);
#32239=CIRCLE('',#99020,51.8);
#32240=CIRCLE('',#99022,0.45);
#32241=CIRCLE('',#99023,4.35);
#32242=CIRCLE('',#99024,4.8);
#32243=CIRCLE('',#99026,0.45);
#32244=CIRCLE('',#99027,1.2);
#32245=CIRCLE('',#99028,0.75);
#32246=CIRCLE('',#99030,0.45);
#32247=CIRCLE('',#99032,1.2);
#32248=CIRCLE('',#99033,0.75);
#32249=CIRCLE('',#99034,0.45);
#32250=CIRCLE('',#99036,0.450000000000001);
#32251=CIRCLE('',#99037,11.5555395526669);
#32252=CIRCLE('',#99038,11.1055395526669);
#32253=CIRCLE('',#99040,0.450000000000006);
#32254=CIRCLE('',#99041,1.2);
#32255=CIRCLE('',#99042,0.750000000000001);
#32256=CIRCLE('',#99044,0.450000000000006);
#32257=CIRCLE('',#99046,1.2);
#32258=CIRCLE('',#99047,0.750000000000001);
#32259=CIRCLE('',#99049,0.450000000000006);
#32260=CIRCLE('',#99050,1.2);
#32261=CIRCLE('',#99051,0.750000000000001);
#32262=CIRCLE('',#99053,0.450000000000006);
#32263=CIRCLE('',#99055,0.450000000000001);
#32264=CIRCLE('',#99056,1.2);
#32265=CIRCLE('',#99057,0.750000000000001);
#32266=CIRCLE('',#99059,0.449999999999999);
#32267=CIRCLE('',#99060,11.5555395526669);
#32268=CIRCLE('',#99061,11.1055395526669);
#32269=CIRCLE('',#99063,0.45);
#32270=CIRCLE('',#99064,1.2);
#32271=CIRCLE('',#99065,0.750000000000001);
#32272=CIRCLE('',#99067,0.45);
#32273=CIRCLE('',#99069,1.2);
#32274=CIRCLE('',#99070,0.750000000000001);
#32275=CIRCLE('',#99072,0.45);
#32276=CIRCLE('',#99073,1.2);
#32277=CIRCLE('',#99074,0.75);
#32278=CIRCLE('',#99076,0.450000000000006);
#32279=CIRCLE('',#99078,1.2);
#32280=CIRCLE('',#99079,0.75);
#32281=CIRCLE('',#99080,0.45);
#32282=CIRCLE('',#99082,0.45);
#32283=CIRCLE('',#99083,11.5555395526669);
#32284=CIRCLE('',#99084,11.1055395526669);
#32285=CIRCLE('',#99086,0.45);
#32286=CIRCLE('',#99087,1.2);
#32287=CIRCLE('',#99088,0.75);
#32288=CIRCLE('',#99090,0.45);
#32289=CIRCLE('',#99092,1.2);
#32290=CIRCLE('',#99093,0.75);
#32291=CIRCLE('',#99095,0.750000000000001);
#32292=CIRCLE('',#99096,0.45);
#32293=CIRCLE('',#99097,1.2);
#32294=CIRCLE('',#99099,0.45);
#32295=CIRCLE('',#99101,0.450000000000001);
#32296=CIRCLE('',#99102,1.2);
#32297=CIRCLE('',#99103,0.750000000000001);
#32298=CIRCLE('',#99105,0.450000000000001);
#32299=CIRCLE('',#99106,11.5555395526669);
#32300=CIRCLE('',#99107,11.1055395526669);
#32301=CIRCLE('',#99109,0.450000000000006);
#32302=CIRCLE('',#99110,1.2);
#32303=CIRCLE('',#99111,0.750000000000001);
#32304=CIRCLE('',#99113,0.450000000000006);
#32305=CIRCLE('',#99115,1.2);
#32306=CIRCLE('',#99116,0.750000000000001);
#32307=CIRCLE('',#99118,1.5);
#32308=CIRCLE('',#99119,14.0401304794059);
#32309=CIRCLE('',#99120,1.5);
#32310=CIRCLE('',#99121,12.5403589366713);
#32311=CIRCLE('',#99123,1.5);
#32312=CIRCLE('',#99124,79.6896304993778);
#32313=CIRCLE('',#99125,78.1898589566432);
#32314=CIRCLE('',#99127,1.5);
#32315=CIRCLE('',#99128,14.0401304794058);
#32316=CIRCLE('',#99129,12.5403589366712);
#32317=CIRCLE('',#99131,1.5);
#32318=CIRCLE('',#99132,1069.5771304794);
#32319=CIRCLE('',#99133,1068.07735893667);
#32320=CIRCLE('',#99135,1.5);
#32321=CIRCLE('',#99136,14.0401304794058);
#32322=CIRCLE('',#99137,12.5403589366712);
#32323=CIRCLE('',#99139,1.5);
#32324=CIRCLE('',#99140,79.6896304993778);
#32325=CIRCLE('',#99141,78.1898589566432);
#32326=CIRCLE('',#99143,1.50000000000001);
#32327=CIRCLE('',#99144,14.0401304794059);
#32328=CIRCLE('',#99145,12.5403589366713);
#32329=CIRCLE('',#99146,1.5);
#32330=CIRCLE('',#99147,1.5);
#32331=CIRCLE('',#99148,1.5);
#32332=CIRCLE('',#99149,1.5);
#32333=CIRCLE('',#99150,213.52922045504);
#32334=CIRCLE('',#99151,211.963156195019);
#32335=CIRCLE('',#99152,1.5);
#32336=CIRCLE('',#99153,1.5);
#32337=CIRCLE('',#99154,1.5);
#32338=CIRCLE('',#99155,1.5);
#32339=CIRCLE('',#99156,687.655553461799);
#32340=CIRCLE('',#99157,696.813945754993);
#32341=CIRCLE('',#99158,1.5);
#32342=CIRCLE('',#99159,1.5);
#32343=CIRCLE('',#99160,1.5);
#32344=CIRCLE('',#99161,1.5);
#32345=CIRCLE('',#99162,687.392615253502);
#32346=CIRCLE('',#99163,696.57627117557);
#32347=CIRCLE('',#99164,1.5);
#32348=CIRCLE('',#99165,1.5);
#32349=CIRCLE('',#99166,1.5);
#32350=CIRCLE('',#99167,1.5);
#32351=CIRCLE('',#99168,687.588787872307);
#32352=CIRCLE('',#99169,697.569175020784);
#32353=CIRCLE('',#99170,1.5);
#32354=CIRCLE('',#99171,5.);
#32355=CIRCLE('',#99172,72.6244975536409);
#32356=CIRCLE('',#99173,5.);
#32357=CIRCLE('',#99174,5.16933481208913);
#32358=CIRCLE('',#99175,10.1322440903793);
#32359=CIRCLE('',#99176,4.99999999999999);
#32360=CIRCLE('',#99177,5.);
#32361=CIRCLE('',#99178,1029.30060997527);
#32362=CIRCLE('',#99179,1066.87927691535);
#32363=CIRCLE('',#99180,3.);
#32364=CIRCLE('',#99181,3.);
#32365=CIRCLE('',#99182,3.);
#32366=CIRCLE('',#99183,3.);
#32367=CIRCLE('',#99184,1066.87014162396);
#32368=CIRCLE('',#99185,5.);
#32369=CIRCLE('',#99186,1029.24694971421);
#32370=CIRCLE('',#99187,4.99999999999999);
#32371=CIRCLE('',#99188,5.00000000000001);
#32372=CIRCLE('',#99189,5.);
#32373=CIRCLE('',#99190,4.98383829446029);
#32374=CIRCLE('',#99191,9.93127307062933);
#32375=CIRCLE('',#99193,3.);
#32376=CIRCLE('',#99194,3.);
#32377=CIRCLE('',#99197,1067.00041769809);
#32378=CIRCLE('',#99198,5.);
#32379=CIRCLE('',#99199,1032.95041731725);
#32380=CIRCLE('',#99200,5.00000000000001);
#32381=CIRCLE('',#99201,5.);
#32382=CIRCLE('',#99202,5.);
#32383=CIRCLE('',#99203,10.1961875685922);
#32384=CIRCLE('',#99206,5.);
#32385=CIRCLE('',#99208,5.00000000000001);
#32386=CIRCLE('',#99210,3.);
#32387=CIRCLE('',#99211,5.);
#32388=CIRCLE('',#99213,2.28316188307923);
#32389=CIRCLE('',#99214,3.);
#32390=CIRCLE('',#99215,5.);
#32391=CIRCLE('',#99216,5.);
#32392=CIRCLE('',#99217,5.);
#32393=CIRCLE('',#99218,9.92561537912225);
#32394=CIRCLE('',#99219,5.01368139939068);
#32395=CIRCLE('',#99221,0.75);
#32396=CIRCLE('',#99223,0.750000000000001);
#32397=CIRCLE('',#99225,0.750000000000001);
#32398=CIRCLE('',#99227,0.750000000000001);
#32399=CIRCLE('',#99229,0.750000000000001);
#32400=CIRCLE('',#99231,0.750000000000001);
#32401=CIRCLE('',#99233,0.75);
#32402=CIRCLE('',#99235,0.75);
#32403=CIRCLE('',#99237,0.75);
#32404=CIRCLE('',#99239,0.750000000000001);
#32405=CIRCLE('',#99241,0.750000000000001);
#32406=CIRCLE('',#99243,0.750000000000001);
#32407=CIRCLE('',#99245,0.750000000000001);
#32408=CIRCLE('',#99247,0.750000000000001);
#32409=CIRCLE('',#99249,0.750000000000001);
#32410=CIRCLE('',#99251,0.750000000000001);
#32411=CIRCLE('',#99253,0.75);
#32412=CIRCLE('',#99255,0.75);
#32413=CIRCLE('',#99257,0.75);
#32414=CIRCLE('',#99259,0.750000000000001);
#32415=CIRCLE('',#99261,0.750000000000001);
#32416=CIRCLE('',#99263,0.75);
#32417=CIRCLE('',#99265,0.750000000000001);
#32418=CIRCLE('',#99267,0.750000000000001);
#32419=CIRCLE('',#99269,0.750000000000001);
#32420=CIRCLE('',#99271,0.750000000000001);
#32421=CIRCLE('',#99273,0.750000000000001);
#32422=CIRCLE('',#99275,0.750000000000001);
#32423=CIRCLE('',#99277,0.750000000000001);
#32424=CIRCLE('',#99279,0.750000000000001);
#32425=CIRCLE('',#99281,0.750000000000001);
#32426=CIRCLE('',#99283,0.750000000000001);
#32427=CIRCLE('',#99285,0.750000000000001);
#32428=CIRCLE('',#99287,0.750000000000001);
#32429=CIRCLE('',#99289,0.75);
#32430=CIRCLE('',#99291,0.75);
#32431=CIRCLE('',#99293,0.750000000000001);
#32432=CIRCLE('',#99295,0.750000000000001);
#32433=CIRCLE('',#99297,0.750000000000001);
#32434=CIRCLE('',#99299,0.750000000000001);
#32435=CIRCLE('',#99301,0.750000000000001);
#32436=CIRCLE('',#99303,0.750000000000001);
#32437=CIRCLE('',#99305,0.750000000000001);
#32438=CIRCLE('',#99307,0.750000000000001);
#32439=CIRCLE('',#99309,0.75);
#32440=CIRCLE('',#99311,0.75);
#32441=CIRCLE('',#99313,0.750000000000001);
#32442=CIRCLE('',#99315,0.750000000000001);
#32443=CIRCLE('',#99317,0.750000000000001);
#32444=CIRCLE('',#99319,0.750000000000001);
#32445=CIRCLE('',#99321,0.750000000000001);
#32446=CIRCLE('',#99323,0.750000000000001);
#32447=CIRCLE('',#99325,0.750000000000001);
#32448=CIRCLE('',#99327,0.750000000000001);
#32449=CIRCLE('',#99329,0.750000000000001);
#32450=CIRCLE('',#99331,0.750000000000001);
#32451=CIRCLE('',#99333,0.750000000000001);
#32452=CIRCLE('',#99335,0.750000000000001);
#32453=CIRCLE('',#99337,0.750000000000001);
#32454=CIRCLE('',#99339,0.750000000000001);
#32455=CIRCLE('',#99341,0.750000000000001);
#32456=CIRCLE('',#99343,0.750000000000001);
#32457=CIRCLE('',#99345,0.750000000000001);
#32458=CIRCLE('',#99347,0.750000000000001);
#32459=CIRCLE('',#99349,0.750000000000001);
#32460=CIRCLE('',#99351,0.750000000000001);
#32461=CIRCLE('',#99353,0.750000000000001);
#32462=CIRCLE('',#99355,0.750000000000001);
#32463=CIRCLE('',#99357,0.750000000000001);
#32464=CIRCLE('',#99359,0.750000000000001);
#32465=CIRCLE('',#99361,0.750000000000001);
#32466=CIRCLE('',#99363,0.75);
#32467=CIRCLE('',#99365,0.750000000000001);
#32468=CIRCLE('',#99367,0.750000000000001);
#32469=CIRCLE('',#99369,0.75);
#32470=CIRCLE('',#99371,0.750000000000001);
#32471=CIRCLE('',#99373,0.75);
#32472=CIRCLE('',#99375,0.75);
#32473=CIRCLE('',#99377,0.750000000000001);
#32474=CIRCLE('',#99379,0.750000000000001);
#32475=CIRCLE('',#99381,0.750000000000001);
#32476=CIRCLE('',#99383,0.750000000000001);
#32477=CIRCLE('',#99385,0.750000000000001);
#32478=CIRCLE('',#99387,0.750000000000001);
#32479=CIRCLE('',#99389,0.750000000000001);
#32480=CIRCLE('',#99391,0.750000000000001);
#32481=CIRCLE('',#99393,0.750000000000001);
#32482=CIRCLE('',#99395,0.750000000000001);
#32483=CIRCLE('',#99397,0.750000000000001);
#32484=CIRCLE('',#99399,0.750000000000001);
#32485=CIRCLE('',#99401,0.750000000000001);
#32486=CIRCLE('',#99403,0.750000000000001);
#32487=CIRCLE('',#99405,0.750000000000001);
#32488=CIRCLE('',#99407,0.750000000000001);
#32489=CIRCLE('',#99409,0.750000000000001);
#32490=CIRCLE('',#99411,0.750000000000001);
#32491=CIRCLE('',#99413,0.750000000000001);
#32492=CIRCLE('',#99415,0.75);
#32493=CIRCLE('',#99417,0.75);
#32494=CIRCLE('',#99419,0.750000000000001);
#32495=CIRCLE('',#99421,0.750000000000001);
#32496=CIRCLE('',#99423,0.750000000000001);
#32497=CIRCLE('',#99425,0.750000000000001);
#32498=CIRCLE('',#99427,0.750000000000001);
#32499=CIRCLE('',#99429,0.750000000000001);
#32500=CIRCLE('',#99431,0.750000000000001);
#32501=CIRCLE('',#99433,0.750000000000001);
#32502=CIRCLE('',#99435,0.750000000000001);
#32503=CIRCLE('',#99437,0.750000000000001);
#32504=CIRCLE('',#99439,0.750000000000001);
#32505=CIRCLE('',#99441,0.750000000000001);
#32506=CIRCLE('',#99443,0.750000000000001);
#32507=CIRCLE('',#99445,0.750000000000001);
#32508=CIRCLE('',#99447,0.750000000000001);
#32509=CIRCLE('',#99449,0.750000000000001);
#32510=CIRCLE('',#99451,0.750000000000001);
#32511=CIRCLE('',#99453,0.750000000000001);
#32512=CIRCLE('',#99455,0.750000000000001);
#32513=CIRCLE('',#99457,0.750000000000001);
#32514=CIRCLE('',#99459,0.750000000000001);
#32515=CIRCLE('',#99461,0.750000000000001);
#32516=CIRCLE('',#99463,0.750000000000001);
#32517=CIRCLE('',#99465,0.750000000000001);
#32518=CIRCLE('',#99467,0.750000000000001);
#32519=CIRCLE('',#99469,0.750000000000001);
#32520=CIRCLE('',#99471,0.750000000000001);
#32521=CIRCLE('',#99473,0.750000000000001);
#32522=CIRCLE('',#99475,0.750000000000001);
#32523=CIRCLE('',#99477,0.750000000000001);
#32524=CIRCLE('',#99479,0.75);
#32525=CIRCLE('',#99481,0.75);
#32526=CIRCLE('',#99483,0.750000000000001);
#32527=CIRCLE('',#99485,0.750000000000001);
#32528=CIRCLE('',#99487,0.750000000000001);
#32529=CIRCLE('',#99489,10.);
#32530=CIRCLE('',#99491,10.);
#32531=CIRCLE('',#99493,10.);
#32532=CIRCLE('',#99495,10.);
#32533=CIRCLE('',#99497,13.1055395526668);
#32534=CIRCLE('',#99499,13.1055395526668);
#32535=CIRCLE('',#99501,11.1055395526669);
#32536=CIRCLE('',#99505,11.1055395526669);
#32537=CIRCLE('',#99507,12.1055395526668);
#32538=CIRCLE('',#99509,11.1055395526669);
#32539=CIRCLE('',#99513,11.1055395526669);
#32540=CIRCLE('',#99515,12.1055395526668);
#32541=CIRCLE('',#99574,3.5);
#32542=CIRCLE('',#99575,3.5);
#32543=CIRCLE('',#99577,50.5);
#32544=CIRCLE('',#99578,50.5);
#32545=CIRCLE('',#99580,3.5);
#32546=CIRCLE('',#99581,3.5);
#32547=CIRCLE('',#99583,679.934816028482);
#32548=CIRCLE('',#99584,679.934816028482);
#32549=CIRCLE('',#99586,3.5);
#32550=CIRCLE('',#99587,3.5);
#32551=CIRCLE('',#99589,50.5);
#32552=CIRCLE('',#99590,50.5);
#32553=CIRCLE('',#99592,3.49999999999996);
#32554=CIRCLE('',#99593,3.49999999999996);
#32555=CIRCLE('',#99595,5.98129380707219);
#32556=CIRCLE('',#99598,5.9812938070714);
#32557=CIRCLE('',#99603,74.6139048513169);
#32558=CIRCLE('',#99604,74.6139048513169);
#32559=CIRCLE('',#99608,74.6139048513167);
#32560=CIRCLE('',#99609,74.6139048513167);
#32561=CIRCLE('',#99611,8.5);
#32562=CIRCLE('',#99612,8.5);
#32563=CIRCLE('',#99614,8.5);
#32564=CIRCLE('',#99615,8.5);
#32565=CIRCLE('',#99617,55.5);
#32566=CIRCLE('',#99618,55.5);
#32567=CIRCLE('',#99620,8.5);
#32568=CIRCLE('',#99621,8.5);
#32569=CIRCLE('',#99623,684.934816028482);
#32570=CIRCLE('',#99624,684.934816028482);
#32571=CIRCLE('',#99626,8.5);
#32572=CIRCLE('',#99627,8.5);
#32573=CIRCLE('',#99629,55.5);
#32574=CIRCLE('',#99630,55.5);
#32575=CIRCLE('',#99632,9.05766167355557);
#32576=CIRCLE('',#99634,74.7071616935275);
#32577=CIRCLE('',#99636,9.05766167355546);
#32578=CIRCLE('',#99637,6.68387219307026);
#32579=CIRCLE('',#99639,9.05766167355555);
#32580=CIRCLE('',#99640,6.41600556626386);
#32581=CIRCLE('',#99642,74.7071616935275);
#32582=CIRCLE('',#99644,9.05766167355558);
#32583=CIRCLE('',#99645,6.41130036340322);
#32584=CIRCLE('',#99647,1067.49961917989);
#32585=CIRCLE('',#99648,1067.09466167355);
#32586=CIRCLE('',#99650,11.9626191798902);
#32587=CIRCLE('',#99651,11.5576616735555);
#32588=CIRCLE('',#99653,77.6121191998622);
#32589=CIRCLE('',#99654,77.2071616935275);
#32590=CIRCLE('',#99656,11.9626191798902);
#32591=CIRCLE('',#99657,11.5576616735556);
#32592=CIRCLE('',#99659,11.9626191798902);
#32593=CIRCLE('',#99660,11.5576616735556);
#32594=CIRCLE('',#99662,77.6121191998622);
#32595=CIRCLE('',#99663,77.2071616935275);
#32596=CIRCLE('',#99665,11.9626191798902);
#32597=CIRCLE('',#99666,11.5576616735555);
#32598=CIRCLE('',#99668,1064.59466167355);
#32599=CIRCLE('',#99669,211.167112167648);
#32600=CIRCLE('',#99671,684.934816028482);
#32601=CIRCLE('',#99672,705.368683747858);
#32602=CIRCLE('',#99673,684.934816028482);
#32603=CIRCLE('',#99675,5.80674315778922);
#32604=CIRCLE('',#99677,5.80674315779001);
#32605=CIRCLE('',#99679,211.99569081556);
#32606=CIRCLE('',#99681,211.99569081556);
#32607=CIRCLE('',#99683,684.934816028482);
#32608=CIRCLE('',#99685,684.934816028482);
#32609=CIRCLE('',#99687,684.934816028482);
#32610=CIRCLE('',#99689,684.934816028482);
#32611=CIRCLE('',#99691,5.9812938070714);
#32612=CIRCLE('',#99693,684.934816028482);
#32613=CIRCLE('',#99695,684.934816028482);
#32614=CIRCLE('',#99697,684.934816028482);
#32615=CIRCLE('',#99699,684.934816028482);
#32616=CIRCLE('',#99701,684.934816028482);
#32617=CIRCLE('',#99707,1.);
#32618=CIRCLE('',#99709,48.);
#32619=CIRCLE('',#99711,0.999999999999999);
#32620=CIRCLE('',#99713,677.434816028482);
#32621=CIRCLE('',#99715,1.);
#32622=CIRCLE('',#99717,48.);
#32623=CIRCLE('',#99719,0.999999999999959);
#32624=CIRCLE('',#99721,3.35);
#32625=CIRCLE('',#99723,3.51597543326183);
#32626=CIRCLE('',#99724,3.51597543326183);
#32627=CIRCLE('',#99726,3.35000000000079);
#32628=CIRCLE('',#99733,4.01589928084002);
#32629=CIRCLE('',#99744,51.8);
#32630=CIRCLE('',#99746,4.8);
#32631=CIRCLE('',#99748,681.234816028482);
#32632=CIRCLE('',#99750,4.8);
#32633=CIRCLE('',#99752,51.8);
#32634=CIRCLE('',#99754,4.8);
#32635=CIRCLE('',#99756,4.8);
#32636=CIRCLE('',#99758,5.99999999999992);
#32637=CIRCLE('',#99760,6.);
#32638=CIRCLE('',#99762,53.);
#32639=CIRCLE('',#99764,6.);
#32640=CIRCLE('',#99766,682.434816028482);
#32641=CIRCLE('',#99768,6.);
#32642=CIRCLE('',#99770,53.);
#32643=CIRCLE('',#99778,1070.);
#32644=CIRCLE('',#99780,14.463);
#32645=CIRCLE('',#99782,80.1125000199719);
#32646=CIRCLE('',#99784,14.463);
#32647=CIRCLE('',#99786,14.463);
#32648=CIRCLE('',#99788,80.1125000199719);
#32649=CIRCLE('',#99790,14.463);
#32650=CIRCLE('',#99795,677.434816028482);
#32651=CIRCLE('',#99797,677.434816028482);
#32652=CIRCLE('',#99799,677.434816028482);
#32653=CIRCLE('',#99801,677.434816028482);
#32654=CIRCLE('',#99803,677.434816028482);
#32655=CIRCLE('',#99815,204.49569081556);
#32656=CIRCLE('',#99817,677.434816028482);
#32657=CIRCLE('',#99819,206.99569081556);
#32658=CIRCLE('',#99820,206.99569081556);
#32659=CIRCLE('',#99836,204.49569081556);
#32660=CIRCLE('',#99838,204.49569081556);
#32661=CIRCLE('',#99840,677.434816028482);
#32662=CIRCLE('',#99842,677.434816028482);
#32663=CIRCLE('',#99844,48.);
#32664=CIRCLE('',#99846,48.);
#32665=CIRCLE('',#99848,48.);
#32666=CIRCLE('',#99850,48.);
#32667=CIRCLE('',#99879,0.500000000000001);
#32668=CIRCLE('',#99880,0.499999999999997);
#32669=CIRCLE('',#99882,4.01589928084002);
#32670=CIRCLE('',#99883,3.51597543326183);
#32671=CIRCLE('',#99884,3.51597543326183);
#32672=CIRCLE('',#99886,4.01589928084082);
#32673=CIRCLE('',#99887,0.5);
#32674=CIRCLE('',#99888,3.51597543326262);
#32675=CIRCLE('',#99889,3.51597543326262);
#32676=CIRCLE('',#99890,0.499999999999999);
#32677=CIRCLE('',#99891,0.500000000000002);
#32678=CIRCLE('',#99892,0.50000000000001);
#32679=CIRCLE('',#99894,0.500000000000004);
#32680=CIRCLE('',#99895,0.500000000000002);
#32681=CIRCLE('',#99896,0.499999999999999);
#32682=CIRCLE('',#99898,0.499999999999997);
#32683=CIRCLE('',#99899,1.49999999999999);
#32684=CIRCLE('',#99900,2.);
#32685=CIRCLE('',#99901,0.500000000000002);
#32686=CIRCLE('',#99903,0.5);
#32687=CIRCLE('',#99904,73.8);
#32688=CIRCLE('',#99905,74.3);
#32689=CIRCLE('',#99906,0.500000000000002);
#32690=CIRCLE('',#99908,0.499999999999999);
#32691=CIRCLE('',#99909,1.5);
#32692=CIRCLE('',#99910,2.);
#32693=CIRCLE('',#99911,0.499999999999993);
#32694=CIRCLE('',#99912,0.500000000000006);
#32695=CIRCLE('',#99913,0.500000000000012);
#32696=CIRCLE('',#99916,0.499999999999999);
#32697=CIRCLE('',#99917,0.500000000000001);
#32698=CIRCLE('',#99918,0.499999999999998);
#32699=CIRCLE('',#99919,0.5);
#32700=CIRCLE('',#99920,0.5);
#32701=CIRCLE('',#99921,0.500000000000006);
#32702=CIRCLE('',#99922,0.500000000000001);
#32703=CIRCLE('',#99924,0.500000000000003);
#32704=CIRCLE('',#99925,0.499999999999998);
#32705=CIRCLE('',#99926,0.50000000000001);
#32706=CIRCLE('',#99927,0.499999999999999);
#32707=CIRCLE('',#99928,0.499999999999999);
#32708=CIRCLE('',#99930,0.499999999999998);
#32709=CIRCLE('',#99931,2.);
#32710=CIRCLE('',#99932,1.5);
#32711=CIRCLE('',#99934,0.499999999999997);
#32712=CIRCLE('',#99935,0.499999999999998);
#32713=CIRCLE('',#99937,0.5);
#32714=CIRCLE('',#99938,74.3);
#32715=CIRCLE('',#99939,73.8);
#32716=CIRCLE('',#99940,0.499999999999997);
#32717=CIRCLE('',#99942,1.5);
#32718=CIRCLE('',#99943,2.);
#32719=CIRCLE('',#99945,232.042829615324);
#32720=CIRCLE('',#99946,232.542753462903);
#32721=CIRCLE('',#99947,0.500000000000002);
#32722=CIRCLE('',#99949,0.500000000000001);
#32723=CIRCLE('',#99950,11.5058296153244);
#32724=CIRCLE('',#99951,12.0057534629026);
#32725=CIRCLE('',#99953,0.500000000000001);
#32726=CIRCLE('',#99954,77.1553296352964);
#32727=CIRCLE('',#99955,77.6552534828746);
#32728=CIRCLE('',#99957,0.499999999999998);
#32729=CIRCLE('',#99958,11.5058296153244);
#32730=CIRCLE('',#99959,12.0057534629026);
#32731=CIRCLE('',#99961,0.499999999999998);
#32732=CIRCLE('',#99962,1067.04282961532);
#32733=CIRCLE('',#99963,1067.5427534629);
#32734=CIRCLE('',#99965,0.499999999999999);
#32735=CIRCLE('',#99966,11.5058296153244);
#32736=CIRCLE('',#99967,12.0057534629025);
#32737=CIRCLE('',#99969,0.500000000000001);
#32738=CIRCLE('',#99970,77.1553296352964);
#32739=CIRCLE('',#99971,77.6552534828746);
#32740=CIRCLE('',#99973,0.500000000000002);
#32741=CIRCLE('',#99974,11.5058296153244);
#32742=CIRCLE('',#99975,12.0057534629026);
#32743=CIRCLE('',#99977,1067.5427534629);
#32744=CIRCLE('',#99978,1067.04282961532);
#32745=CIRCLE('',#99979,64.9438262487296);
#32746=CIRCLE('',#99980,64.8942573619905);
#32747=CIRCLE('',#99981,0.500000000000001);
#32748=CIRCLE('',#99982,0.499999999999998);
#32749=CIRCLE('',#99984,0.499999999999996);
#32750=CIRCLE('',#99985,0.500000000000001);
#32751=CIRCLE('',#99986,0.50000000000001);
#32752=CIRCLE('',#99987,365.618325533514);
#32753=CIRCLE('',#99988,368.00584558015);
#32754=CIRCLE('',#99989,0.499999999999998);
#32755=CIRCLE('',#99990,429.776000990187);
#32756=CIRCLE('',#99991,431.08166328569);
#32757=CIRCLE('',#99992,0.5);
#32758=CIRCLE('',#99993,0.499999999999998);
#32759=CIRCLE('',#99994,0.5);
#32760=CIRCLE('',#99995,0.499999999999998);
#32761=CIRCLE('',#99996,0.499999999999998);
#32762=CIRCLE('',#99997,0.499999999999997);
#32763=CIRCLE('',#99999,77.1139048513169);
#32764=CIRCLE('',#100000,77.1139810037387);
#32765=CIRCLE('',#100001,0.500000000000002);
#32766=CIRCLE('',#100002,0.500000000000003);
#32767=CIRCLE('',#100004,0.499999999999998);
#32768=CIRCLE('',#100005,77.1139810037385);
#32769=CIRCLE('',#100006,77.1139048513167);
#32770=CIRCLE('',#100007,0.500000000000003);
#32771=CIRCLE('',#100008,0.5);
#32772=CIRCLE('',#100009,0.499999999999995);
#32773=CIRCLE('',#100010,0.500000000000002);
#32774=CIRCLE('',#100011,0.500000000000004);
#32775=CIRCLE('',#100012,329.186676141438);
#32776=CIRCLE('',#100013,329.616230392321);
#32777=CIRCLE('',#100014,0.499999999999997);
#32778=CIRCLE('',#100015,0.499999999999999);
#32779=CIRCLE('',#100016,463.797803513665);
#32780=CIRCLE('',#100017,462.991628528349);
#32781=CIRCLE('',#100019,0.750000000000001);
#32782=CIRCLE('',#100020,1.5);
#32783=CIRCLE('',#100021,0.75);
#32784=CIRCLE('',#100022,0.750000000000001);
#32785=CIRCLE('',#100024,73.05);
#32786=CIRCLE('',#100025,73.05);
#32787=CIRCLE('',#100026,73.8);
#32788=CIRCLE('',#100027,0.750000000000002);
#32789=CIRCLE('',#100028,0.749999999999996);
#32790=CIRCLE('',#100029,0.750000000000001);
#32791=CIRCLE('',#100030,1.5);
#32792=CIRCLE('',#100033,0.750000000000003);
#32793=CIRCLE('',#100034,1.5);
#32794=CIRCLE('',#100035,0.750000000000004);
#32795=CIRCLE('',#100036,0.750000000000001);
#32796=CIRCLE('',#100038,0.749999999999998);
#32797=CIRCLE('',#100039,76.3639048513167);
#32798=CIRCLE('',#100040,77.1139048513167);
#32799=CIRCLE('',#100041,0.75);
#32800=CIRCLE('',#100042,0.750000000000001);
#32801=CIRCLE('',#100043,1.5);
#32802=CIRCLE('',#100046,0.749999999999999);
#32803=CIRCLE('',#100047,0.749999999999999);
#32804=CIRCLE('',#100048,0.750000000000001);
#32805=CIRCLE('',#100049,1.5);
#32806=CIRCLE('',#100051,0.75);
#32807=CIRCLE('',#100052,76.3639048513169);
#32808=CIRCLE('',#100053,77.1139048513169);
#32809=CIRCLE('',#100054,0.750000000000001);
#32810=CIRCLE('',#100055,1.5);
#32811=CIRCLE('',#100056,0.750000000000005);
#32812=CIRCLE('',#100059,0.75);
#32813=CIRCLE('',#100060,0.750000000000003);
#32814=CIRCLE('',#100061,0.749999999999994);
#32815=CIRCLE('',#100062,1.49999999999999);
#32816=CIRCLE('',#100064,0.750000000000004);
#32817=CIRCLE('',#100065,73.05);
#32818=CIRCLE('',#100066,73.8);
#32819=CIRCLE('',#100067,0.750000000000001);
#32820=CIRCLE('',#100068,1.5);
#32821=CIRCLE('',#100069,0.75);
#32822=CIRCLE('',#100080,1.2);
#32823=CIRCLE('',#100081,0.450000000000001);
#32824=CIRCLE('',#100082,0.750000000000001);
#32825=CIRCLE('',#100083,0.450000000000006);
#32826=CIRCLE('',#100085,0.450000000000006);
#32827=CIRCLE('',#100087,0.45);
#32828=CIRCLE('',#100088,204.49569081556);
#32829=CIRCLE('',#100089,204.945690815561);
#32830=CIRCLE('',#100091,0.450000000000006);
#32831=CIRCLE('',#100092,1.2);
#32832=CIRCLE('',#100093,0.750000000000001);
#32833=CIRCLE('',#100095,0.450000000000001);
#32834=CIRCLE('',#100096,1.);
#32835=CIRCLE('',#100097,1.45);
#32836=CIRCLE('',#100099,0.450000000000006);
#32837=CIRCLE('',#100101,0.450000000000001);
#32838=CIRCLE('',#100102,48.);
#32839=CIRCLE('',#100103,48.45);
#32840=CIRCLE('',#100105,0.450000000000006);
#32841=CIRCLE('',#100106,1.2);
#32842=CIRCLE('',#100107,0.750000000000001);
#32843=CIRCLE('',#100109,0.450000000000006);
#32844=CIRCLE('',#100110,0.750000000000001);
#32845=CIRCLE('',#100111,1.2);
#32846=CIRCLE('',#100114,1.2);
#32847=CIRCLE('',#100115,0.450000000000001);
#32848=CIRCLE('',#100116,0.750000000000001);
#32849=CIRCLE('',#100117,0.450000000000006);
#32850=CIRCLE('',#100119,0.450000000000006);
#32851=CIRCLE('',#100121,0.449999999999999);
#32852=CIRCLE('',#100122,204.49569081556);
#32853=CIRCLE('',#100123,204.945690815561);
#32854=CIRCLE('',#100125,0.450000000000006);
#32855=CIRCLE('',#100126,1.2);
#32856=CIRCLE('',#100127,0.750000000000001);
#32857=CIRCLE('',#100129,0.450000000000006);
#32858=CIRCLE('',#100130,0.750000000000001);
#32859=CIRCLE('',#100131,1.2);
#32860=CIRCLE('',#100133,0.450000000000006);
#32861=CIRCLE('',#100135,0.450000000000006);
#32862=CIRCLE('',#100137,0.750000000000001);
#32863=CIRCLE('',#100138,1.2);
#32864=CIRCLE('',#100140,1.2);
#32865=CIRCLE('',#100141,0.449999999999999);
#32866=CIRCLE('',#100142,0.750000000000001);
#32867=CIRCLE('',#100143,0.450000000000006);
#32868=CIRCLE('',#100145,0.450000000000006);
#32869=CIRCLE('',#100147,0.450000000000001);
#32870=CIRCLE('',#100148,204.49569081556);
#32871=CIRCLE('',#100149,204.945690815561);
#32872=CIRCLE('',#100151,0.450000000000006);
#32873=CIRCLE('',#100152,1.2);
#32874=CIRCLE('',#100153,0.750000000000001);
#32875=CIRCLE('',#100155,0.450000000000006);
#32876=CIRCLE('',#100156,0.750000000000001);
#32877=CIRCLE('',#100157,1.2);
#32878=CIRCLE('',#100159,0.450000000000006);
#32879=CIRCLE('',#100161,0.450000000000006);
#32880=CIRCLE('',#100163,0.750000000000001);
#32881=CIRCLE('',#100164,1.2);
#32882=CIRCLE('',#100166,0.449999999999999);
#32883=CIRCLE('',#100167,0.750000000000001);
#32884=CIRCLE('',#100168,0.450000000000006);
#32885=CIRCLE('',#100169,1.2);
#32886=CIRCLE('',#100171,0.450000000000006);
#32887=CIRCLE('',#100173,0.450000000000006);
#32888=CIRCLE('',#100175,0.450000000000006);
#32889=CIRCLE('',#100176,1.2);
#32890=CIRCLE('',#100177,0.750000000000001);
#32891=CIRCLE('',#100179,0.450000000000006);
#32892=CIRCLE('',#100180,0.750000000000001);
#32893=CIRCLE('',#100181,1.2);
#32894=CIRCLE('',#100183,0.450000000000006);
#32895=CIRCLE('',#100185,0.450000000000006);
#32896=CIRCLE('',#100187,0.750000000000001);
#32897=CIRCLE('',#100188,1.2);
#32898=CIRCLE('',#100190,0.450000000000006);
#32899=CIRCLE('',#100191,0.750000000000001);
#32900=CIRCLE('',#100192,0.450000000000006);
#32901=CIRCLE('',#100193,1.2);
#32902=CIRCLE('',#100195,0.450000000000006);
#32903=CIRCLE('',#100197,0.450000000000006);
#32904=CIRCLE('',#100199,0.45);
#32905=CIRCLE('',#100200,1.2);
#32906=CIRCLE('',#100201,0.75);
#32907=CIRCLE('',#100203,0.450000000000006);
#32908=CIRCLE('',#100204,0.750000000000001);
#32909=CIRCLE('',#100205,1.2);
#32910=CIRCLE('',#100207,0.45);
#32911=CIRCLE('',#100208,12.6555395526668);
#32912=CIRCLE('',#100209,13.1055395526668);
#32913=CIRCLE('',#100211,0.450000000000001);
#32914=CIRCLE('',#100213,0.45);
#32915=CIRCLE('',#100214,10.45);
#32916=CIRCLE('',#100215,10.);
#32917=CIRCLE('',#100217,1.2);
#32918=CIRCLE('',#100218,0.75);
#32919=CIRCLE('',#100220,0.450000000000006);
#32920=CIRCLE('',#100221,0.750000000000001);
#32921=CIRCLE('',#100222,0.450000000000006);
#32922=CIRCLE('',#100223,1.2);
#32923=CIRCLE('',#100225,0.450000000000001);
#32924=CIRCLE('',#100227,0.450000000000006);
#32925=CIRCLE('',#100229,0.450000000000006);
#32926=CIRCLE('',#100230,1.2);
#32927=CIRCLE('',#100231,0.75);
#32928=CIRCLE('',#100233,0.450000000000006);
#32929=CIRCLE('',#100234,0.750000000000001);
#32930=CIRCLE('',#100235,1.2);
#32931=CIRCLE('',#100237,0.450000000000006);
#32932=CIRCLE('',#100239,0.449999999999999);
#32933=CIRCLE('',#100241,0.75);
#32934=CIRCLE('',#100242,1.2);
#32935=CIRCLE('',#100244,0.450000000000006);
#32936=CIRCLE('',#100245,0.750000000000001);
#32937=CIRCLE('',#100246,0.450000000000006);
#32938=CIRCLE('',#100247,1.2);
#32939=CIRCLE('',#100249,0.450000000000006);
#32940=CIRCLE('',#100251,0.450000000000006);
#32941=CIRCLE('',#100253,0.450000000000006);
#32942=CIRCLE('',#100254,1.2);
#32943=CIRCLE('',#100255,0.750000000000001);
#32944=CIRCLE('',#100257,0.450000000000006);
#32945=CIRCLE('',#100258,0.750000000000001);
#32946=CIRCLE('',#100259,1.2);
#32947=CIRCLE('',#100261,0.450000000000006);
#32948=CIRCLE('',#100263,0.450000000000006);
#32949=CIRCLE('',#100265,0.750000000000001);
#32950=CIRCLE('',#100266,1.2);
#32951=CIRCLE('',#100268,0.450000000000006);
#32952=CIRCLE('',#100269,0.750000000000001);
#32953=CIRCLE('',#100270,0.450000000000006);
#32954=CIRCLE('',#100271,1.2);
#32955=CIRCLE('',#100273,0.450000000000006);
#32956=CIRCLE('',#100275,0.450000000000006);
#32957=CIRCLE('',#100277,0.450000000000006);
#32958=CIRCLE('',#100278,1.2);
#32959=CIRCLE('',#100279,0.750000000000001);
#32960=CIRCLE('',#100281,0.450000000000006);
#32961=CIRCLE('',#100282,0.750000000000001);
#32962=CIRCLE('',#100283,1.2);
#32963=CIRCLE('',#100285,0.450000000000006);
#32964=CIRCLE('',#100287,0.450000000000006);
#32965=CIRCLE('',#100289,0.750000000000001);
#32966=CIRCLE('',#100290,1.2);
#32967=CIRCLE('',#100292,0.450000000000006);
#32968=CIRCLE('',#100293,0.750000000000001);
#32969=CIRCLE('',#100294,0.450000000000006);
#32970=CIRCLE('',#100295,1.2);
#32971=CIRCLE('',#100297,0.449999999999999);
#32972=CIRCLE('',#100299,0.450000000000006);
#32973=CIRCLE('',#100301,0.450000000000006);
#32974=CIRCLE('',#100302,1.2);
#32975=CIRCLE('',#100303,0.75);
#32976=CIRCLE('',#100305,0.450000000000006);
#32977=CIRCLE('',#100306,0.750000000000001);
#32978=CIRCLE('',#100307,1.2);
#32979=CIRCLE('',#100309,0.450000000000006);
#32980=CIRCLE('',#100311,0.450000000000006);
#32981=CIRCLE('',#100313,0.75);
#32982=CIRCLE('',#100314,1.2);
#32983=CIRCLE('',#100316,0.450000000000006);
#32984=CIRCLE('',#100317,0.750000000000001);
#32985=CIRCLE('',#100318,0.450000000000006);
#32986=CIRCLE('',#100319,1.2);
#32987=CIRCLE('',#100321,0.449999999999999);
#32988=CIRCLE('',#100323,0.450000000000006);
#32989=CIRCLE('',#100325,0.450000000000006);
#32990=CIRCLE('',#100326,1.2);
#32991=CIRCLE('',#100327,0.75);
#32992=CIRCLE('',#100329,0.449999999999997);
#32993=CIRCLE('',#100330,0.750000000000001);
#32994=CIRCLE('',#100331,1.2);
#32995=CIRCLE('',#100333,0.450000000000006);
#32996=CIRCLE('',#100335,0.449999999999998);
#32997=CIRCLE('',#100336,677.434816028482);
#32998=CIRCLE('',#100337,677.884816028482);
#32999=CIRCLE('',#100339,0.75);
#33000=CIRCLE('',#100340,1.2);
#33001=CIRCLE('',#100342,0.450000000000006);
#33002=CIRCLE('',#100343,0.750000000000001);
#33003=CIRCLE('',#100344,0.450000000000006);
#33004=CIRCLE('',#100345,1.2);
#33005=CIRCLE('',#100347,0.450000000000006);
#33006=CIRCLE('',#100349,0.450000000000006);
#33007=CIRCLE('',#100351,0.450000000000006);
#33008=CIRCLE('',#100352,1.2);
#33009=CIRCLE('',#100353,0.750000000000001);
#33010=CIRCLE('',#100355,0.449999999999998);
#33011=CIRCLE('',#100356,0.750000000000001);
#33012=CIRCLE('',#100357,1.2);
#33013=CIRCLE('',#100359,0.450000000000006);
#33014=CIRCLE('',#100361,0.45);
#33015=CIRCLE('',#100362,48.);
#33016=CIRCLE('',#100363,48.45);
#33017=CIRCLE('',#100365,0.449999999999997);
#33018=CIRCLE('',#100366,1.2);
#33019=CIRCLE('',#100367,0.750000000000001);
#33020=CIRCLE('',#100369,0.449999999999997);
#33021=CIRCLE('',#100370,0.999999999999999);
#33022=CIRCLE('',#100371,1.45);
#33023=CIRCLE('',#100373,677.434816028482);
#33024=CIRCLE('',#100374,677.884816028482);
#33025=CIRCLE('',#100376,0.450000000000006);
#33026=CIRCLE('',#100377,0.75);
#33027=CIRCLE('',#100378,0.450000000000006);
#33028=CIRCLE('',#100379,1.2);
#33029=CIRCLE('',#100381,0.449999999999999);
#33030=CIRCLE('',#100383,0.450000000000006);
#33031=CIRCLE('',#100385,0.450000000000006);
#33032=CIRCLE('',#100386,1.2);
#33033=CIRCLE('',#100387,0.750000000000001);
#33034=CIRCLE('',#100389,0.45);
#33035=CIRCLE('',#100390,0.75);
#33036=CIRCLE('',#100391,1.2);
#33037=CIRCLE('',#100393,0.450000000000006);
#33038=CIRCLE('',#100395,0.449999999999999);
#33039=CIRCLE('',#100396,677.434816028482);
#33040=CIRCLE('',#100397,677.884816028482);
#33041=CIRCLE('',#100399,0.750000000000001);
#33042=CIRCLE('',#100400,1.2);
#33043=CIRCLE('',#100402,0.450000000000006);
#33044=CIRCLE('',#100403,0.75);
#33045=CIRCLE('',#100404,0.450000000000006);
#33046=CIRCLE('',#100405,1.2);
#33047=CIRCLE('',#100407,0.449999999999999);
#33048=CIRCLE('',#100409,0.450000000000006);
#33049=CIRCLE('',#100411,0.450000000000006);
#33050=CIRCLE('',#100412,1.2);
#33051=CIRCLE('',#100413,0.750000000000001);
#33052=CIRCLE('',#100415,0.450000000000006);
#33053=CIRCLE('',#100416,0.75);
#33054=CIRCLE('',#100417,1.2);
#33055=CIRCLE('',#100419,0.450000000000006);
#33056=CIRCLE('',#100421,0.450000000000006);
#33057=CIRCLE('',#100423,0.750000000000001);
#33058=CIRCLE('',#100424,1.2);
#33059=CIRCLE('',#100426,0.45);
#33060=CIRCLE('',#100427,0.750000000000001);
#33061=CIRCLE('',#100428,0.450000000000006);
#33062=CIRCLE('',#100429,1.2);
#33063=CIRCLE('',#100431,0.450000000000006);
#33064=CIRCLE('',#100433,0.45);
#33065=CIRCLE('',#100434,12.1055395526668);
#33066=CIRCLE('',#100435,11.6555395526668);
#33067=CIRCLE('',#100437,0.450000000000006);
#33068=CIRCLE('',#100438,1.2);
#33069=CIRCLE('',#100439,0.750000000000001);
#33070=CIRCLE('',#100441,0.450000000000006);
#33071=CIRCLE('',#100442,10.);
#33072=CIRCLE('',#100443,10.45);
#33073=CIRCLE('',#100445,0.450000000000006);
#33074=CIRCLE('',#100447,0.450000000000006);
#33075=CIRCLE('',#100449,0.450000000000006);
#33076=CIRCLE('',#100450,1.2);
#33077=CIRCLE('',#100451,0.75);
#33078=CIRCLE('',#100453,0.450000000000006);
#33079=CIRCLE('',#100454,0.75);
#33080=CIRCLE('',#100455,1.2);
#33081=CIRCLE('',#100458,0.450000000000001);
#33082=CIRCLE('',#100459,0.750000000000001);
#33083=CIRCLE('',#100460,0.450000000000006);
#33084=CIRCLE('',#100461,1.2);
#33085=CIRCLE('',#100463,0.450000000000006);
#33086=CIRCLE('',#100465,0.450000000000006);
#33087=CIRCLE('',#100467,0.450000000000006);
#33088=CIRCLE('',#100468,1.2);
#33089=CIRCLE('',#100469,0.750000000000001);
#33090=CIRCLE('',#100471,0.450000000000001);
#33091=CIRCLE('',#100472,10.);
#33092=CIRCLE('',#100473,10.45);
#33093=CIRCLE('',#100475,0.449999999999999);
#33094=CIRCLE('',#100477,0.45);
#33095=CIRCLE('',#100478,12.1055395526668);
#33096=CIRCLE('',#100479,11.6555395526668);
#33097=CIRCLE('',#100481,0.450000000000006);
#33098=CIRCLE('',#100482,1.2);
#33099=CIRCLE('',#100483,0.750000000000001);
#33100=CIRCLE('',#100485,0.450000000000006);
#33101=CIRCLE('',#100486,0.750000000000001);
#33102=CIRCLE('',#100487,1.2);
#33103=CIRCLE('',#100490,0.450000000000006);
#33104=CIRCLE('',#100491,0.750000000000001);
#33105=CIRCLE('',#100492,0.450000000000006);
#33106=CIRCLE('',#100493,1.2);
#33107=CIRCLE('',#100495,0.450000000000006);
#33108=CIRCLE('',#100497,0.450000000000006);
#33109=CIRCLE('',#100499,0.450000000000006);
#33110=CIRCLE('',#100500,1.2);
#33111=CIRCLE('',#100501,0.750000000000001);
#33112=CIRCLE('',#100503,0.450000000000006);
#33113=CIRCLE('',#100504,0.750000000000001);
#33114=CIRCLE('',#100505,1.2);
#33115=CIRCLE('',#100507,0.449999999999999);
#33116=CIRCLE('',#100509,0.450000000000006);
#33117=CIRCLE('',#100511,0.750000000000001);
#33118=CIRCLE('',#100512,1.2);
#33119=CIRCLE('',#100514,0.450000000000006);
#33120=CIRCLE('',#100515,0.750000000000001);
#33121=CIRCLE('',#100516,0.450000000000006);
#33122=CIRCLE('',#100517,1.2);
#33123=CIRCLE('',#100519,0.450000000000006);
#33124=CIRCLE('',#100521,0.450000000000006);
#33125=CIRCLE('',#100523,0.45);
#33126=CIRCLE('',#100524,1.2);
#33127=CIRCLE('',#100525,0.750000000000001);
#33128=CIRCLE('',#100527,0.450000000000006);
#33129=CIRCLE('',#100528,0.750000000000001);
#33130=CIRCLE('',#100529,1.2);
#33131=CIRCLE('',#100531,0.449999999999999);
#33132=CIRCLE('',#100532,677.884816028482);
#33133=CIRCLE('',#100533,677.434816028482);
#33134=CIRCLE('',#100535,0.450000000000006);
#33135=CIRCLE('',#100537,0.750000000000001);
#33136=CIRCLE('',#100538,1.2);
#33137=CIRCLE('',#100540,0.450000000000006);
#33138=CIRCLE('',#100541,0.750000000000001);
#33139=CIRCLE('',#100542,0.450000000000006);
#33140=CIRCLE('',#100543,1.2);
#33141=CIRCLE('',#100545,0.450000000000006);
#33142=CIRCLE('',#100547,0.450000000000006);
#33143=CIRCLE('',#100549,0.450000000000006);
#33144=CIRCLE('',#100550,1.2);
#33145=CIRCLE('',#100551,0.750000000000001);
#33146=CIRCLE('',#100553,0.450000000000006);
#33147=CIRCLE('',#100554,0.750000000000001);
#33148=CIRCLE('',#100555,1.2);
#33149=CIRCLE('',#100557,0.449999999999999);
#33150=CIRCLE('',#100559,0.450000000000006);
#33151=CIRCLE('',#100561,0.750000000000001);
#33152=CIRCLE('',#100562,1.2);
#33153=CIRCLE('',#100564,0.450000000000006);
#33154=CIRCLE('',#100565,0.750000000000001);
#33155=CIRCLE('',#100566,0.450000000000006);
#33156=CIRCLE('',#100567,1.2);
#33157=CIRCLE('',#100569,0.450000000000006);
#33158=CIRCLE('',#100571,0.450000000000006);
#33159=CIRCLE('',#100573,0.450000000000006);
#33160=CIRCLE('',#100574,1.2);
#33161=CIRCLE('',#100575,0.750000000000001);
#33162=CIRCLE('',#100577,0.450000000000006);
#33163=CIRCLE('',#100578,0.750000000000001);
#33164=CIRCLE('',#100579,1.2);
#33165=CIRCLE('',#100581,0.450000000000001);
#33166=CIRCLE('',#100583,0.450000000000006);
#33167=CIRCLE('',#100585,0.750000000000001);
#33168=CIRCLE('',#100586,1.2);
#33169=CIRCLE('',#100588,0.450000000000006);
#33170=CIRCLE('',#100589,0.750000000000001);
#33171=CIRCLE('',#100590,0.449999999999999);
#33172=CIRCLE('',#100591,1.2);
#33173=CIRCLE('',#100593,0.450000000000006);
#33174=CIRCLE('',#100595,0.450000000000006);
#33175=CIRCLE('',#100597,0.450000000000006);
#33176=CIRCLE('',#100598,1.2);
#33177=CIRCLE('',#100599,0.750000000000001);
#33178=CIRCLE('',#100601,0.45);
#33179=CIRCLE('',#100602,0.750000000000001);
#33180=CIRCLE('',#100603,1.2);
#33181=CIRCLE('',#100605,0.450000000000006);
#33182=CIRCLE('',#100607,0.45);
#33183=CIRCLE('',#100608,13.1055395526668);
#33184=CIRCLE('',#100609,12.6555395526668);
#33185=CIRCLE('',#100611,1.2);
#33186=CIRCLE('',#100612,0.750000000000001);
#33187=CIRCLE('',#100613,0.450000000000001);
#33188=CIRCLE('',#100615,10.45);
#33189=CIRCLE('',#100616,10.);
#33190=CIRCLE('',#100618,0.450000000000006);
#33191=CIRCLE('',#100619,0.750000000000001);
#33192=CIRCLE('',#100620,0.450000000000006);
#33193=CIRCLE('',#100621,1.2);
#33194=CIRCLE('',#100623,0.450000000000006);
#33195=CIRCLE('',#100625,0.450000000000006);
#33196=CIRCLE('',#100627,0.449999999999997);
#33197=CIRCLE('',#100628,1.2);
#33198=CIRCLE('',#100629,0.750000000000001);
#33199=CIRCLE('',#100631,0.450000000000006);
#33200=CIRCLE('',#100632,0.750000000000001);
#33201=CIRCLE('',#100633,1.2);
#33202=CIRCLE('',#100635,0.449999999999998);
#33203=CIRCLE('',#100636,677.884816028482);
#33204=CIRCLE('',#100637,677.434816028482);
#33205=CIRCLE('',#100639,0.450000000000006);
#33206=CIRCLE('',#100641,0.750000000000001);
#33207=CIRCLE('',#100642,1.2);
#33208=CIRCLE('',#100644,0.449999999999999);
#33209=CIRCLE('',#100645,0.750000000000001);
#33210=CIRCLE('',#100646,0.450000000000006);
#33211=CIRCLE('',#100647,1.2);
#33212=CIRCLE('',#100649,0.450000000000006);
#33213=CIRCLE('',#100651,0.450000000000006);
#33214=CIRCLE('',#100653,0.45);
#33215=CIRCLE('',#100654,1.2);
#33216=CIRCLE('',#100655,0.750000000000001);
#33217=CIRCLE('',#100657,0.450000000000006);
#33218=CIRCLE('',#100658,0.750000000000001);
#33219=CIRCLE('',#100659,1.2);
#33220=CIRCLE('',#100661,0.45);
#33221=CIRCLE('',#100662,48.45);
#33222=CIRCLE('',#100663,48.);
#33223=CIRCLE('',#100665,0.450000000000006);
#33224=CIRCLE('',#100667,0.449999999999997);
#33225=CIRCLE('',#100668,1.45);
#33226=CIRCLE('',#100669,1.);
#33227=CIRCLE('',#100671,0.449999999999997);
#33228=CIRCLE('',#100672,0.750000000000001);
#33229=CIRCLE('',#100673,1.2);
#33230=CIRCLE('',#100675,677.434816028482);
#33231=CIRCLE('',#100676,677.884816028482);
#33232=CIRCLE('',#100678,0.450000000000006);
#33233=CIRCLE('',#100679,0.750000000000001);
#33234=CIRCLE('',#100680,0.450000000000006);
#33235=CIRCLE('',#100681,1.2);
#33236=CIRCLE('',#100683,0.450000000000006);
#33237=CIRCLE('',#100685,0.450000000000006);
#33238=CIRCLE('',#100687,0.450000000000006);
#33239=CIRCLE('',#100688,1.2);
#33240=CIRCLE('',#100689,0.750000000000001);
#33241=CIRCLE('',#100691,0.450000000000006);
#33242=CIRCLE('',#100692,0.750000000000001);
#33243=CIRCLE('',#100693,1.2);
#33244=CIRCLE('',#100695,0.449999999999999);
#33245=CIRCLE('',#100697,0.450000000000006);
#33246=CIRCLE('',#100699,0.750000000000001);
#33247=CIRCLE('',#100700,1.2);
#33248=CIRCLE('',#100702,0.449999999999999);
#33249=CIRCLE('',#100703,0.750000000000001);
#33250=CIRCLE('',#100704,0.450000000000006);
#33251=CIRCLE('',#100705,1.2);
#33252=CIRCLE('',#100707,0.450000000000006);
#33253=CIRCLE('',#100709,0.450000000000006);
#33254=CIRCLE('',#100711,0.450000000000006);
#33255=CIRCLE('',#100712,1.2);
#33256=CIRCLE('',#100713,0.750000000000001);
#33257=CIRCLE('',#100715,0.45);
#33258=CIRCLE('',#100716,0.750000000000001);
#33259=CIRCLE('',#100717,1.2);
#33260=CIRCLE('',#100719,0.450000000000006);
#33261=CIRCLE('',#100721,0.45);
#33262=CIRCLE('',#100722,48.);
#33263=CIRCLE('',#100723,48.45);
#33264=CIRCLE('',#100725,0.450000000000003);
#33265=CIRCLE('',#100726,1.2);
#33266=CIRCLE('',#100727,0.750000000000001);
#33267=CIRCLE('',#100729,0.450000000000001);
#33268=CIRCLE('',#100730,0.999999999999959);
#33269=CIRCLE('',#100731,1.44999999999997);
#33270=CIRCLE('',#100733,677.434816028482);
#33271=CIRCLE('',#100734,677.884816028482);
#33272=CIRCLE('',#100736,0.449999999999999);
#33273=CIRCLE('',#100737,0.750000000000001);
#33274=CIRCLE('',#100738,0.450000000000006);
#33275=CIRCLE('',#100739,1.2);
#33276=CIRCLE('',#100741,0.450000000000006);
#33277=CIRCLE('',#100743,0.450000000000006);
#33278=CIRCLE('',#100745,0.450000000000006);
#33279=CIRCLE('',#100746,1.2);
#33280=CIRCLE('',#100747,0.750000000000001);
#33281=CIRCLE('',#100749,0.450000000000003);
#33282=CIRCLE('',#100750,0.750000000000001);
#33283=CIRCLE('',#100751,1.2);
#33284=CIRCLE('',#100753,0.450000000000006);
#33285=CIRCLE('',#100755,0.449999999999998);
#33286=CIRCLE('',#100756,677.434816028482);
#33287=CIRCLE('',#100757,677.884816028482);
#33288=CIRCLE('',#100759,0.750000000000001);
#33289=CIRCLE('',#100760,1.2);
#33290=CIRCLE('',#100762,0.450000000000001);
#33291=CIRCLE('',#100763,0.750000000000001);
#33292=CIRCLE('',#100764,0.450000000000006);
#33293=CIRCLE('',#100765,1.2);
#33294=CIRCLE('',#100767,0.450000000000006);
#33295=CIRCLE('',#100769,0.450000000000006);
#33296=CIRCLE('',#100771,0.450000000000006);
#33297=CIRCLE('',#100772,1.2);
#33298=CIRCLE('',#100773,0.750000000000001);
#33299=CIRCLE('',#100775,0.450000000000006);
#33300=CIRCLE('',#100776,0.750000000000001);
#33301=CIRCLE('',#100777,1.2);
#33302=CIRCLE('',#100779,0.449999999999999);
#33303=CIRCLE('',#100781,0.450000000000006);
#33304=CIRCLE('',#100783,0.750000000000001);
#33305=CIRCLE('',#100784,1.2);
#33306=CIRCLE('',#100786,0.450000000000006);
#33307=CIRCLE('',#100787,0.750000000000001);
#33308=CIRCLE('',#100788,0.450000000000006);
#33309=CIRCLE('',#100789,1.2);
#33310=CIRCLE('',#100791,0.449999999999999);
#33311=CIRCLE('',#100793,0.450000000000006);
#33312=CIRCLE('',#100795,0.450000000000006);
#33313=CIRCLE('',#100796,1.2);
#33314=CIRCLE('',#100797,0.750000000000001);
#33315=CIRCLE('',#100799,0.449999999999999);
#33316=CIRCLE('',#100800,0.750000000000001);
#33317=CIRCLE('',#100801,1.2);
#33318=CIRCLE('',#100803,0.450000000000006);
#33319=CIRCLE('',#100805,0.449999999999999);
#33320=CIRCLE('',#100806,677.434816028482);
#33321=CIRCLE('',#100807,677.884816028482);
#33322=CIRCLE('',#100809,0.750000000000001);
#33323=CIRCLE('',#100810,1.2);
#33324=CIRCLE('',#100812,0.450000000000006);
#33325=CIRCLE('',#100813,0.750000000000001);
#33326=CIRCLE('',#100814,0.449999999999999);
#33327=CIRCLE('',#100815,1.2);
#33328=CIRCLE('',#100817,0.450000000000006);
#33329=CIRCLE('',#100819,0.450000000000006);
#33330=CIRCLE('',#100821,0.450000000000006);
#33331=CIRCLE('',#100822,1.2);
#33332=CIRCLE('',#100823,0.750000000000001);
#33333=CIRCLE('',#100825,0.449999999999999);
#33334=CIRCLE('',#100826,0.750000000000001);
#33335=CIRCLE('',#100827,1.2);
#33336=CIRCLE('',#100829,0.450000000000006);
#33337=CIRCLE('',#100831,0.450000000000006);
#33338=CIRCLE('',#100833,0.750000000000001);
#33339=CIRCLE('',#100834,1.2);
#33340=CIRCLE('',#100836,0.449999999999999);
#33341=CIRCLE('',#100837,0.750000000000001);
#33342=CIRCLE('',#100838,0.450000000000006);
#33343=CIRCLE('',#100839,1.2);
#33344=CIRCLE('',#100841,0.450000000000006);
#33345=CIRCLE('',#100843,0.45);
#33346=CIRCLE('',#100844,48.);
#33347=CIRCLE('',#100845,48.45);
#33348=CIRCLE('',#100847,0.450000000000006);
#33349=CIRCLE('',#100848,1.2);
#33350=CIRCLE('',#100849,0.750000000000001);
#33351=CIRCLE('',#100851,0.450000000000006);
#33352=CIRCLE('',#100852,0.750000000000001);
#33353=CIRCLE('',#100853,1.2);
#33354=CIRCLE('',#100856,1.2);
#33355=CIRCLE('',#100857,0.450000000000002);
#33356=CIRCLE('',#100858,0.750000000000001);
#33357=CIRCLE('',#100859,0.450000000000006);
#33358=CIRCLE('',#100861,0.450000000000006);
#33359=CIRCLE('',#100863,0.449999999999999);
#33360=CIRCLE('',#100864,48.);
#33361=CIRCLE('',#100865,48.45);
#33362=CIRCLE('',#100867,0.450000000000006);
#33363=CIRCLE('',#100868,1.2);
#33364=CIRCLE('',#100869,0.750000000000001);
#33365=CIRCLE('',#100871,0.450000000000006);
#33366=CIRCLE('',#100872,0.750000000000001);
#33367=CIRCLE('',#100873,1.2);
#33368=CIRCLE('',#100876,7.65553955266686);
#33369=CIRCLE('',#100877,0.45);
#33370=CIRCLE('',#100878,8.10553955266686);
#33371=CIRCLE('',#100880,4.62535);
#33372=CIRCLE('',#100881,0.45);
#33373=CIRCLE('',#100882,5.07535);
#33374=CIRCLE('',#100884,0.45);
#33375=CIRCLE('',#100885,682.884816028482);
#33376=CIRCLE('',#100886,682.434816028482);
#33377=CIRCLE('',#100888,0.450000000000002);
#33378=CIRCLE('',#100889,6.44999999999991);
#33379=CIRCLE('',#100890,5.99999999999992);
#33380=CIRCLE('',#100892,0.45);
#33381=CIRCLE('',#100893,53.45);
#33382=CIRCLE('',#100894,53.);
#33383=CIRCLE('',#100896,0.449999999999997);
#33384=CIRCLE('',#100897,6.45);
#33385=CIRCLE('',#100898,6.);
#33386=CIRCLE('',#100900,0.449999999999997);
#33387=CIRCLE('',#100901,682.884816028482);
#33388=CIRCLE('',#100902,682.434816028482);
#33389=CIRCLE('',#100904,0.45);
#33390=CIRCLE('',#100905,6.45);
#33391=CIRCLE('',#100906,6.);
#33392=CIRCLE('',#100908,0.449999999999998);
#33393=CIRCLE('',#100909,53.45);
#33394=CIRCLE('',#100910,53.);
#33395=CIRCLE('',#100912,0.45);
#33396=CIRCLE('',#100913,6.45);
#33397=CIRCLE('',#100914,6.);
#33398=CIRCLE('',#100916,209.945690815561);
#33399=CIRCLE('',#100917,209.495690815561);
#33400=CIRCLE('',#100919,0.45);
#33401=CIRCLE('',#100920,681.234816028482);
#33402=CIRCLE('',#100921,680.784816028482);
#33403=CIRCLE('',#100923,0.450000000000002);
#33404=CIRCLE('',#100924,4.8);
#33405=CIRCLE('',#100925,4.34999999999995);
#33406=CIRCLE('',#100927,0.45);
#33407=CIRCLE('',#100928,51.8);
#33408=CIRCLE('',#100929,51.35);
#33409=CIRCLE('',#100931,0.449999999999997);
#33410=CIRCLE('',#100932,4.8);
#33411=CIRCLE('',#100933,4.35);
#33412=CIRCLE('',#100935,0.449999999999997);
#33413=CIRCLE('',#100936,681.234816028482);
#33414=CIRCLE('',#100937,680.784816028482);
#33415=CIRCLE('',#100939,0.45);
#33416=CIRCLE('',#100940,4.8);
#33417=CIRCLE('',#100941,4.35);
#33418=CIRCLE('',#100943,0.450000000000002);
#33419=CIRCLE('',#100944,51.8);
#33420=CIRCLE('',#100945,51.35);
#33421=CIRCLE('',#100947,0.45);
#33422=CIRCLE('',#100948,4.8);
#33423=CIRCLE('',#100949,4.35);
#33424=CIRCLE('',#100951,208.29569081556);
#33425=CIRCLE('',#100952,207.845690815561);
#33426=CIRCLE('',#100954,0.45);
#33427=CIRCLE('',#100955,0.75);
#33428=CIRCLE('',#100956,1.2);
#33429=CIRCLE('',#100958,0.45);
#33430=CIRCLE('',#100960,1.2);
#33431=CIRCLE('',#100961,0.45);
#33432=CIRCLE('',#100962,0.75);
#33433=CIRCLE('',#100964,0.450000000000001);
#33434=CIRCLE('',#100965,11.1055395526669);
#33435=CIRCLE('',#100966,11.5555395526669);
#33436=CIRCLE('',#100968,0.450000000000006);
#33437=CIRCLE('',#100969,0.750000000000001);
#33438=CIRCLE('',#100970,1.2);
#33439=CIRCLE('',#100972,0.450000000000006);
#33440=CIRCLE('',#100974,0.750000000000001);
#33441=CIRCLE('',#100975,1.2);
#33442=CIRCLE('',#100977,0.450000000000006);
#33443=CIRCLE('',#100978,0.750000000000001);
#33444=CIRCLE('',#100979,1.2);
#33445=CIRCLE('',#100981,0.450000000000006);
#33446=CIRCLE('',#100983,0.450000000000001);
#33447=CIRCLE('',#100984,0.750000000000001);
#33448=CIRCLE('',#100985,1.2);
#33449=CIRCLE('',#100987,0.449999999999999);
#33450=CIRCLE('',#100988,11.1055395526669);
#33451=CIRCLE('',#100989,11.5555395526669);
#33452=CIRCLE('',#100991,0.45);
#33453=CIRCLE('',#100992,0.750000000000001);
#33454=CIRCLE('',#100993,1.2);
#33455=CIRCLE('',#100995,0.45);
#33456=CIRCLE('',#100997,0.750000000000001);
#33457=CIRCLE('',#100998,1.2);
#33458=CIRCLE('',#101000,0.45);
#33459=CIRCLE('',#101001,0.75);
#33460=CIRCLE('',#101002,1.2);
#33461=CIRCLE('',#101004,0.450000000000006);
#33462=CIRCLE('',#101006,1.2);
#33463=CIRCLE('',#101007,0.45);
#33464=CIRCLE('',#101008,0.75);
#33465=CIRCLE('',#101010,0.45);
#33466=CIRCLE('',#101011,11.1055395526669);
#33467=CIRCLE('',#101012,11.5555395526669);
#33468=CIRCLE('',#101014,0.45);
#33469=CIRCLE('',#101015,0.75);
#33470=CIRCLE('',#101016,1.2);
#33471=CIRCLE('',#101018,0.45);
#33472=CIRCLE('',#101020,0.75);
#33473=CIRCLE('',#101021,1.2);
#33474=CIRCLE('',#101023,1.2);
#33475=CIRCLE('',#101024,0.45);
#33476=CIRCLE('',#101025,0.750000000000001);
#33477=CIRCLE('',#101027,0.45);
#33478=CIRCLE('',#101029,0.450000000000001);
#33479=CIRCLE('',#101030,0.750000000000001);
#33480=CIRCLE('',#101031,1.2);
#33481=CIRCLE('',#101033,0.450000000000001);
#33482=CIRCLE('',#101034,11.1055395526669);
#33483=CIRCLE('',#101035,11.5555395526669);
#33484=CIRCLE('',#101037,0.450000000000006);
#33485=CIRCLE('',#101038,0.750000000000001);
#33486=CIRCLE('',#101039,1.2);
#33487=CIRCLE('',#101041,0.450000000000006);
#33488=CIRCLE('',#101043,0.750000000000001);
#33489=CIRCLE('',#101044,1.2);
#33490=CIRCLE('',#101046,233.077358936672);
#33491=CIRCLE('',#101047,234.577130479406);
#33492=CIRCLE('',#101048,1.5);
#33493=CIRCLE('',#101050,1.5);
#33494=CIRCLE('',#101051,12.5403589366713);
#33495=CIRCLE('',#101052,14.0401304794059);
#33496=CIRCLE('',#101054,1.5);
#33497=CIRCLE('',#101055,78.1898589566432);
#33498=CIRCLE('',#101056,79.6896304993778);
#33499=CIRCLE('',#101058,1.5);
#33500=CIRCLE('',#101059,12.5403589366712);
#33501=CIRCLE('',#101060,14.0401304794058);
#33502=CIRCLE('',#101062,1.5);
#33503=CIRCLE('',#101063,1068.07735893667);
#33504=CIRCLE('',#101064,1069.5771304794);
#33505=CIRCLE('',#101066,1.5);
#33506=CIRCLE('',#101067,12.5403589366712);
#33507=CIRCLE('',#101068,14.0401304794058);
#33508=CIRCLE('',#101070,1.5);
#33509=CIRCLE('',#101071,78.1898589566432);
#33510=CIRCLE('',#101072,79.6896304993778);
#33511=CIRCLE('',#101074,1.50000000000001);
#33512=CIRCLE('',#101075,12.5403589366713);
#33513=CIRCLE('',#101076,14.0401304794059);
#33514=CIRCLE('',#101078,1068.07735893667);
#33515=CIRCLE('',#101079,1069.5771304794);
#33516=CIRCLE('',#101080,1.5);
#33517=CIRCLE('',#101081,1.5);
#33518=CIRCLE('',#101083,1.5);
#33519=CIRCLE('',#101084,211.96315619496);
#33520=CIRCLE('',#101085,213.52922045504);
#33521=CIRCLE('',#101086,1.5);
#33522=CIRCLE('',#101087,1.5);
#33523=CIRCLE('',#101088,1.5);
#33524=CIRCLE('',#101089,1.5);
#33525=CIRCLE('',#101090,696.813945754987);
#33526=CIRCLE('',#101091,687.655553461799);
#33527=CIRCLE('',#101092,1.5);
#33528=CIRCLE('',#101093,1.5);
#33529=CIRCLE('',#101094,1.5);
#33530=CIRCLE('',#101095,1.5);
#33531=CIRCLE('',#101096,696.576271176166);
#33532=CIRCLE('',#101097,687.392615253502);
#33533=CIRCLE('',#101098,1.5);
#33534=CIRCLE('',#101099,1.5);
#33535=CIRCLE('',#101100,1.5);
#33536=CIRCLE('',#101101,1.5);
#33537=CIRCLE('',#101102,697.569175023773);
#33538=CIRCLE('',#101103,687.588787872307);
#33539=CIRCLE('',#101104,1.5);
#33540=CIRCLE('',#101105,72.6268730892939);
#33541=CIRCLE('',#101106,5.);
#33542=CIRCLE('',#101107,5.);
#33543=CIRCLE('',#101108,10.1322440903793);
#33544=CIRCLE('',#101110,4.99999999999999);
#33545=CIRCLE('',#101111,5.);
#33546=CIRCLE('',#101112,1066.87927691535);
#33547=CIRCLE('',#101113,1029.30060997527);
#33548=CIRCLE('',#101115,3.);
#33549=CIRCLE('',#101116,3.);
#33550=CIRCLE('',#101117,3.);
#33551=CIRCLE('',#101118,3.);
#33552=CIRCLE('',#101119,1029.24694971421);
#33553=CIRCLE('',#101120,5.);
#33554=CIRCLE('',#101121,1066.87014162396);
#33555=CIRCLE('',#101122,4.99999999999999);
#33556=CIRCLE('',#101123,5.00000000000001);
#33557=CIRCLE('',#101124,5.);
#33558=CIRCLE('',#101125,9.93127307062933);
#33559=CIRCLE('',#101126,4.98383829944567);
#33560=CIRCLE('',#101128,3.);
#33561=CIRCLE('',#101130,3.);
#33562=CIRCLE('',#101133,1032.95041731725);
#33563=CIRCLE('',#101134,5.);
#33564=CIRCLE('',#101135,1067.00041835739);
#33565=CIRCLE('',#101136,5.00000000000001);
#33566=CIRCLE('',#101137,5.);
#33567=CIRCLE('',#101138,5.);
#33568=CIRCLE('',#101139,10.1960538523774);
#33569=CIRCLE('',#101143,5.00000000000001);
#33570=CIRCLE('',#101145,3.);
#33571=CIRCLE('',#101146,2.28316188307923);
#33572=CIRCLE('',#101148,5.);
#33573=CIRCLE('',#101149,3.);
#33574=CIRCLE('',#101150,5.);
#33575=CIRCLE('',#101151,5.);
#33576=CIRCLE('',#101152,5.);
#33577=CIRCLE('',#101153,9.92561537912225);
#33578=CIRCLE('',#101155,0.75);
#33579=CIRCLE('',#101157,0.750000000000001);
#33580=CIRCLE('',#101159,0.750000000000001);
#33581=CIRCLE('',#101161,0.750000000000001);
#33582=CIRCLE('',#101163,0.750000000000001);
#33583=CIRCLE('',#101165,0.750000000000001);
#33584=CIRCLE('',#101167,0.75);
#33585=CIRCLE('',#101169,0.75);
#33586=CIRCLE('',#101171,0.75);
#33587=CIRCLE('',#101173,0.750000000000001);
#33588=CIRCLE('',#101175,0.750000000000001);
#33589=CIRCLE('',#101177,0.750000000000001);
#33590=CIRCLE('',#101179,0.750000000000001);
#33591=CIRCLE('',#101181,0.750000000000001);
#33592=CIRCLE('',#101183,0.750000000000001);
#33593=CIRCLE('',#101185,0.750000000000001);
#33594=CIRCLE('',#101187,0.75);
#33595=CIRCLE('',#101189,0.75);
#33596=CIRCLE('',#101191,0.75);
#33597=CIRCLE('',#101193,0.750000000000001);
#33598=CIRCLE('',#101195,0.750000000000001);
#33599=CIRCLE('',#101197,0.75);
#33600=CIRCLE('',#101199,0.750000000000001);
#33601=CIRCLE('',#101201,0.750000000000001);
#33602=CIRCLE('',#101203,0.750000000000001);
#33603=CIRCLE('',#101205,0.750000000000001);
#33604=CIRCLE('',#101207,0.750000000000001);
#33605=CIRCLE('',#101209,0.750000000000001);
#33606=CIRCLE('',#101211,0.750000000000001);
#33607=CIRCLE('',#101213,0.750000000000001);
#33608=CIRCLE('',#101215,0.750000000000001);
#33609=CIRCLE('',#101217,0.750000000000001);
#33610=CIRCLE('',#101219,0.750000000000001);
#33611=CIRCLE('',#101221,0.750000000000001);
#33612=CIRCLE('',#101223,0.75);
#33613=CIRCLE('',#101225,0.75);
#33614=CIRCLE('',#101227,0.750000000000001);
#33615=CIRCLE('',#101229,0.750000000000001);
#33616=CIRCLE('',#101231,0.750000000000001);
#33617=CIRCLE('',#101233,0.750000000000001);
#33618=CIRCLE('',#101235,0.750000000000001);
#33619=CIRCLE('',#101237,0.750000000000001);
#33620=CIRCLE('',#101239,0.750000000000001);
#33621=CIRCLE('',#101241,0.750000000000001);
#33622=CIRCLE('',#101243,0.75);
#33623=CIRCLE('',#101245,0.75);
#33624=CIRCLE('',#101247,0.750000000000001);
#33625=CIRCLE('',#101249,0.750000000000001);
#33626=CIRCLE('',#101251,0.750000000000001);
#33627=CIRCLE('',#101253,0.750000000000001);
#33628=CIRCLE('',#101255,0.750000000000001);
#33629=CIRCLE('',#101257,0.750000000000001);
#33630=CIRCLE('',#101259,0.750000000000001);
#33631=CIRCLE('',#101261,0.750000000000001);
#33632=CIRCLE('',#101263,0.750000000000001);
#33633=CIRCLE('',#101265,0.750000000000001);
#33634=CIRCLE('',#101267,0.750000000000001);
#33635=CIRCLE('',#101269,0.750000000000001);
#33636=CIRCLE('',#101271,0.750000000000001);
#33637=CIRCLE('',#101273,0.750000000000001);
#33638=CIRCLE('',#101275,0.750000000000001);
#33639=CIRCLE('',#101277,0.750000000000001);
#33640=CIRCLE('',#101279,0.750000000000001);
#33641=CIRCLE('',#101281,0.750000000000001);
#33642=CIRCLE('',#101283,0.750000000000001);
#33643=CIRCLE('',#101285,0.750000000000001);
#33644=CIRCLE('',#101287,0.750000000000001);
#33645=CIRCLE('',#101289,0.750000000000001);
#33646=CIRCLE('',#101291,0.750000000000001);
#33647=CIRCLE('',#101293,0.750000000000001);
#33648=CIRCLE('',#101295,0.750000000000001);
#33649=CIRCLE('',#101297,0.75);
#33650=CIRCLE('',#101299,0.750000000000001);
#33651=CIRCLE('',#101301,0.750000000000001);
#33652=CIRCLE('',#101303,0.75);
#33653=CIRCLE('',#101305,0.750000000000001);
#33654=CIRCLE('',#101307,0.75);
#33655=CIRCLE('',#101309,0.75);
#33656=CIRCLE('',#101311,0.750000000000001);
#33657=CIRCLE('',#101313,0.750000000000001);
#33658=CIRCLE('',#101315,0.750000000000001);
#33659=CIRCLE('',#101317,0.750000000000001);
#33660=CIRCLE('',#101319,0.750000000000001);
#33661=CIRCLE('',#101321,0.750000000000001);
#33662=CIRCLE('',#101323,0.750000000000001);
#33663=CIRCLE('',#101325,0.750000000000001);
#33664=CIRCLE('',#101327,0.750000000000001);
#33665=CIRCLE('',#101329,0.750000000000001);
#33666=CIRCLE('',#101331,0.750000000000001);
#33667=CIRCLE('',#101333,0.750000000000001);
#33668=CIRCLE('',#101335,0.750000000000001);
#33669=CIRCLE('',#101337,0.750000000000001);
#33670=CIRCLE('',#101339,0.750000000000001);
#33671=CIRCLE('',#101341,0.750000000000001);
#33672=CIRCLE('',#101343,0.750000000000001);
#33673=CIRCLE('',#101345,0.750000000000001);
#33674=CIRCLE('',#101347,0.750000000000001);
#33675=CIRCLE('',#101349,0.75);
#33676=CIRCLE('',#101351,0.75);
#33677=CIRCLE('',#101353,0.750000000000001);
#33678=CIRCLE('',#101355,0.750000000000001);
#33679=CIRCLE('',#101357,0.750000000000001);
#33680=CIRCLE('',#101359,0.750000000000001);
#33681=CIRCLE('',#101361,0.750000000000001);
#33682=CIRCLE('',#101363,0.750000000000001);
#33683=CIRCLE('',#101365,0.750000000000001);
#33684=CIRCLE('',#101367,0.750000000000001);
#33685=CIRCLE('',#101369,0.750000000000001);
#33686=CIRCLE('',#101371,0.750000000000001);
#33687=CIRCLE('',#101373,0.750000000000001);
#33688=CIRCLE('',#101375,0.750000000000001);
#33689=CIRCLE('',#101377,0.750000000000001);
#33690=CIRCLE('',#101379,0.750000000000001);
#33691=CIRCLE('',#101381,0.750000000000001);
#33692=CIRCLE('',#101383,0.750000000000001);
#33693=CIRCLE('',#101385,0.750000000000001);
#33694=CIRCLE('',#101387,0.750000000000001);
#33695=CIRCLE('',#101389,0.750000000000001);
#33696=CIRCLE('',#101391,0.750000000000001);
#33697=CIRCLE('',#101393,0.750000000000001);
#33698=CIRCLE('',#101395,0.750000000000001);
#33699=CIRCLE('',#101397,0.750000000000001);
#33700=CIRCLE('',#101399,0.750000000000001);
#33701=CIRCLE('',#101401,0.750000000000001);
#33702=CIRCLE('',#101403,0.750000000000001);
#33703=CIRCLE('',#101405,0.750000000000001);
#33704=CIRCLE('',#101407,0.750000000000001);
#33705=CIRCLE('',#101409,0.750000000000001);
#33706=CIRCLE('',#101411,0.750000000000001);
#33707=CIRCLE('',#101413,0.75);
#33708=CIRCLE('',#101415,0.75);
#33709=CIRCLE('',#101417,0.750000000000001);
#33710=CIRCLE('',#101419,0.750000000000001);
#33711=CIRCLE('',#101421,0.750000000000001);
#33712=CIRCLE('',#101423,10.);
#33713=CIRCLE('',#101425,10.);
#33714=CIRCLE('',#101427,10.);
#33715=CIRCLE('',#101429,10.);
#33716=CIRCLE('',#101431,4.62535);
#33717=CIRCLE('',#101435,13.1055395526668);
#33718=CIRCLE('',#101437,13.1055395526668);
#33719=CIRCLE('',#101439,8.10553955266685);
#33720=CIRCLE('',#101440,8.10553955266686);
#33721=CIRCLE('',#101441,8.10553955266685);
#33722=CIRCLE('',#101442,8.10553955266686);
#33723=CIRCLE('',#101443,8.10553955266685);
#33724=CIRCLE('',#101444,8.10553955266686);
#33725=CIRCLE('',#101445,8.10553955266685);
#33726=CIRCLE('',#101446,8.10553955266686);
#33727=CIRCLE('',#101447,8.10553955266685);
#33728=CIRCLE('',#101448,8.10553955266686);
#33729=CIRCLE('',#101449,8.10553955266685);
#33730=CIRCLE('',#101450,8.10553955266686);
#33731=CIRCLE('',#101451,8.10553955266685);
#33732=CIRCLE('',#101452,8.10553955266686);
#33733=CIRCLE('',#101453,8.10553955266685);
#33734=CIRCLE('',#101454,8.10553955266686);
#33735=CIRCLE('',#101455,8.10553955266685);
#33736=CIRCLE('',#101457,11.1055395526669);
#33737=CIRCLE('',#101461,11.1055395526669);
#33738=CIRCLE('',#101463,12.1055395526668);
#33739=CIRCLE('',#101465,11.1055395526669);
#33740=CIRCLE('',#101469,11.1055395526669);
#33741=CIRCLE('',#101471,12.1055395526668);
#33742=CIRCLE('',#101530,206.99569081556);
#33743=CIRCLE('',#101531,679.934816028482);
#33744=CIRCLE('',#101532,3.49999999999996);
#33745=CIRCLE('',#101533,50.5);
#33746=CIRCLE('',#101534,3.5);
#33747=CIRCLE('',#101535,679.934816028482);
#33748=CIRCLE('',#101536,3.5);
#33749=CIRCLE('',#101537,50.5);
#33750=CIRCLE('',#101538,3.5);
#33751=CIRCLE('',#101539,206.99569081556);
#33752=CIRCLE('',#101540,677.434816028482);
#33753=CIRCLE('',#101541,204.49569081556);
#33754=CIRCLE('',#101542,204.49569081556);
#33755=CIRCLE('',#101543,677.434816028482);
#33756=CIRCLE('',#101544,204.49569081556);
#33757=CIRCLE('',#101545,1.);
#33758=CIRCLE('',#101546,48.);
#33759=CIRCLE('',#101547,48.);
#33760=CIRCLE('',#101548,0.999999999999999);
#33761=CIRCLE('',#101549,677.434816028482);
#33762=CIRCLE('',#101550,677.434816028482);
#33763=CIRCLE('',#101551,677.434816028482);
#33764=CIRCLE('',#101552,677.434816028482);
#33765=CIRCLE('',#101553,677.434816028482);
#33766=CIRCLE('',#101554,48.);
#33767=CIRCLE('',#101555,677.434816028482);
#33768=CIRCLE('',#101556,1.);
#33769=CIRCLE('',#101557,48.);
#33770=CIRCLE('',#101558,48.);
#33771=CIRCLE('',#101559,0.999999999999959);
#33772=CIRCLE('',#101560,677.434816028482);
#33773=CIRCLE('',#101561,48.);
#33774=CIRCLE('',#101563,3.5);
#33775=CIRCLE('',#101565,50.5);
#33776=CIRCLE('',#101567,3.5);
#33777=CIRCLE('',#101569,679.934816028482);
#33778=CIRCLE('',#101571,3.5);
#33779=CIRCLE('',#101573,50.5);
#33780=CIRCLE('',#101575,3.49999999999996);
#33781=CIRCLE('',#101577,679.934816028482);
#33782=CIRCLE('',#101579,5.98129380707219);
#33783=CIRCLE('',#101582,5.9812938070714);
#33784=CIRCLE('',#101587,74.6139048513169);
#33785=CIRCLE('',#101588,74.6139048513169);
#33786=CIRCLE('',#101592,74.6139048513167);
#33787=CIRCLE('',#101593,74.6139048513167);
#33788=CIRCLE('',#101595,8.5);
#33789=CIRCLE('',#101596,8.5);
#33790=CIRCLE('',#101598,684.934816028482);
#33791=CIRCLE('',#101599,684.934816028482);
#33792=CIRCLE('',#101601,211.99569081556);
#33793=CIRCLE('',#101602,211.99569081556);
#33794=CIRCLE('',#101603,211.99569081556);
#33795=CIRCLE('',#101604,211.99569081556);
#33796=CIRCLE('',#101606,8.5);
#33797=CIRCLE('',#101607,8.5);
#33798=CIRCLE('',#101609,55.5);
#33799=CIRCLE('',#101610,55.5);
#33800=CIRCLE('',#101612,8.5);
#33801=CIRCLE('',#101613,8.5);
#33802=CIRCLE('',#101615,684.934816028482);
#33803=CIRCLE('',#101616,684.934816028482);
#33804=CIRCLE('',#101618,8.5);
#33805=CIRCLE('',#101619,8.5);
#33806=CIRCLE('',#101621,55.5);
#33807=CIRCLE('',#101622,55.5);
#33808=CIRCLE('',#101624,9.05766167355557);
#33809=CIRCLE('',#101626,74.7071616935275);
#33810=CIRCLE('',#101628,9.05766167355546);
#33811=CIRCLE('',#101629,6.68387219307026);
#33812=CIRCLE('',#101631,9.05766167355555);
#33813=CIRCLE('',#101632,6.41600556624483);
#33814=CIRCLE('',#101634,74.7071616935275);
#33815=CIRCLE('',#101636,9.05766167355558);
#33816=CIRCLE('',#101637,6.41130036340322);
#33817=CIRCLE('',#101639,1064.59466167355);
#33818=CIRCLE('',#101641,232.094661673555);
#33819=CIRCLE('',#101642,1067.09466167355);
#33820=CIRCLE('',#101643,11.5576616735556);
#33821=CIRCLE('',#101644,77.2071616935275);
#33822=CIRCLE('',#101645,11.5576616735555);
#33823=CIRCLE('',#101646,1067.09466167355);
#33824=CIRCLE('',#101647,11.5576616735555);
#33825=CIRCLE('',#101648,77.2071616935275);
#33826=CIRCLE('',#101649,11.5576616735556);
#33827=CIRCLE('',#101650,229.594661673555);
#33828=CIRCLE('',#101651,1064.59466167355);
#33829=CIRCLE('',#101653,1067.49961917989);
#33830=CIRCLE('',#101655,11.9626191798902);
#33831=CIRCLE('',#101657,77.6121191998622);
#33832=CIRCLE('',#101659,11.9626191798902);
#33833=CIRCLE('',#101661,232.49961917989);
#33834=CIRCLE('',#101663,1067.49961917989);
#33835=CIRCLE('',#101665,11.9626191798902);
#33836=CIRCLE('',#101667,77.6121191998622);
#33837=CIRCLE('',#101669,11.9626191798902);
#33838=CIRCLE('',#101671,211.167112167697);
#33839=CIRCLE('',#101674,684.934816028482);
#33840=CIRCLE('',#101675,684.934816028482);
#33841=CIRCLE('',#101676,705.368683747911);
#33842=CIRCLE('',#101678,5.80674315778922);
#33843=CIRCLE('',#101680,5.80674315779001);
#33844=CIRCLE('',#101685,684.934816028482);
#33845=CIRCLE('',#101687,684.934816028482);
#33846=CIRCLE('',#101689,684.934816028482);
#33847=CIRCLE('',#101692,684.934816028482);
#33848=CIRCLE('',#101694,5.9812938070714);
#33849=CIRCLE('',#101696,684.934816028482);
#33850=CIRCLE('',#101698,684.934816028482);
#33851=CIRCLE('',#101700,684.934816028482);
#33852=CIRCLE('',#101702,684.934816028482);
#33853=CIRCLE('',#101704,684.934816028482);
#33854=CIRCLE('',#101717,3.35);
#33855=CIRCLE('',#101720,3.35000000000079);
#33856=CIRCLE('',#101738,51.8);
#33857=CIRCLE('',#101740,4.8);
#33858=CIRCLE('',#101742,681.234816028482);
#33859=CIRCLE('',#101744,4.8);
#33860=CIRCLE('',#101746,51.8);
#33861=CIRCLE('',#101748,4.8);
#33862=CIRCLE('',#101750,681.234816028482);
#33863=CIRCLE('',#101752,208.295690815561);
#33864=CIRCLE('',#101754,4.8);
#33865=CIRCLE('',#101756,682.434816028482);
#33866=CIRCLE('',#101757,209.495690815561);
#33867=CIRCLE('',#101758,6.);
#33868=CIRCLE('',#101759,53.);
#33869=CIRCLE('',#101760,6.);
#33870=CIRCLE('',#101761,682.434816028482);
#33871=CIRCLE('',#101762,6.);
#33872=CIRCLE('',#101763,53.);
#33873=CIRCLE('',#101764,5.99999999999992);
#33874=CIRCLE('',#101782,235.);
#33875=CIRCLE('',#101783,1070.);
#33876=CIRCLE('',#101784,14.463);
#33877=CIRCLE('',#101785,80.1125000199719);
#33878=CIRCLE('',#101786,14.463);
#33879=CIRCLE('',#101787,1070.);
#33880=CIRCLE('',#101788,14.463);
#33881=CIRCLE('',#101789,80.1125000199719);
#33882=CIRCLE('',#101790,14.463);
#33883=CIRCLE('',#101824,206.99569081556);
#33884=CIRCLE('',#101826,206.99569081556);
#33885=CIRCLE('',#101887,1.73205080756888);
#33886=CIRCLE('',#101889,1.73205080756888);
#33887=CIRCLE('',#101891,1.73205080756888);
#33888=CIRCLE('',#101893,1.73205080756888);
#33889=CIRCLE('',#101895,1.73205080756888);
#33890=CIRCLE('',#101897,1.73205080756888);
#33891=CIRCLE('',#101899,3.);
#33892=CIRCLE('',#101900,0.25);
#33893=CIRCLE('',#101901,3.25);
#33894=CIRCLE('',#101902,3.25);
#33895=CIRCLE('',#101904,3.25);
#33896=CIRCLE('',#101908,5.);
#33897=CIRCLE('',#101909,5.);
#33898=CIRCLE('',#101910,5.);
#33899=CIRCLE('',#101911,5.);
#33900=CIRCLE('',#101912,5.);
#33901=CIRCLE('',#101913,5.);
#33902=CIRCLE('',#101921,5.);
#33903=CIRCLE('',#101922,5.);
#33904=CIRCLE('',#101923,5.);
#33905=CIRCLE('',#101924,5.);
#33906=CIRCLE('',#101925,5.);
#33907=CIRCLE('',#101926,5.);
#33908=CIRCLE('',#101940,5.);
#33909=CIRCLE('',#101941,5.);
#33910=CIRCLE('',#101942,5.);
#33911=CIRCLE('',#101943,5.);
#33912=CIRCLE('',#101944,5.);
#33913=CIRCLE('',#101945,5.);
#33914=CIRCLE('',#101953,5.);
#33915=CIRCLE('',#101954,5.);
#33916=CIRCLE('',#101955,5.);
#33917=CIRCLE('',#101956,5.);
#33918=CIRCLE('',#101957,5.);
#33919=CIRCLE('',#101958,5.);
#33920=CIRCLE('',#101979,1.73205080756888);
#33921=CIRCLE('',#101981,1.73205080756888);
#33922=CIRCLE('',#101983,1.73205080756888);
#33923=CIRCLE('',#101985,1.73205080756888);
#33924=CIRCLE('',#101987,1.73205080756888);
#33925=CIRCLE('',#101989,1.73205080756888);
#33926=CIRCLE('',#101991,3.);
#33927=CIRCLE('',#101992,0.25);
#33928=CIRCLE('',#101993,3.25);
#33929=CIRCLE('',#101994,3.25);
#33930=CIRCLE('',#101996,3.25);
#33931=CIRCLE('',#102000,8.65629040278471);
#33932=CIRCLE('',#102001,20.3599346995449);
#33933=CIRCLE('',#102002,20.3599346995449);
#33934=CIRCLE('',#102004,8.8);
#33935=CIRCLE('',#102005,8.8);
#33936=CIRCLE('',#102006,0.25);
#33937=CIRCLE('',#102008,8.55);
#33938=CIRCLE('',#102009,0.25);
#33939=CIRCLE('',#102010,8.8);
#33940=CIRCLE('',#102011,8.8);
#33941=CIRCLE('',#102013,0.750000000000001);
#33942=CIRCLE('',#102014,0.750000000000001);
#33943=CIRCLE('',#102020,7.8);
#33944=CIRCLE('',#102022,7.8);
#33945=CIRCLE('',#102026,2.);
#33946=CIRCLE('',#102027,1.47499999999998);
#33947=CIRCLE('',#102030,2.);
#33948=CIRCLE('',#102032,2.5);
#33949=CIRCLE('',#102034,2.5);
#33950=CIRCLE('',#102037,0.5);
#33951=CIRCLE('',#102038,6.50000000000001);
#33952=CIRCLE('',#102039,0.5);
#33953=CIRCLE('',#102040,7.00000000000001);
#33954=CIRCLE('',#102042,0.5);
#33955=CIRCLE('',#102044,0.5);
#33956=CIRCLE('',#102046,0.5);
#33957=CIRCLE('',#102047,7.00000000000001);
#33958=CIRCLE('',#102048,6.50000000000001);
#33959=CIRCLE('',#102050,0.5);
#33960=CIRCLE('',#102051,6.50000000000001);
#33961=CIRCLE('',#102052,7.00000000000001);
#33962=CIRCLE('',#102054,0.5);
#33963=CIRCLE('',#102056,0.5);
#33964=CIRCLE('',#102058,6.50000000000001);
#33965=CIRCLE('',#102059,7.00000000000001);
#33966=CIRCLE('',#102062,7.00000000000001);
#33967=CIRCLE('',#102064,7.00000000000001);
#33968=CIRCLE('',#102066,7.8);
#33969=CIRCLE('',#102067,7.8);
#33970=CIRCLE('',#102069,1.);
#33971=CIRCLE('',#102070,4.);
#33972=CIRCLE('',#102071,1.);
#33973=CIRCLE('',#102072,5.);
#33974=CIRCLE('',#102074,1.);
#33975=CIRCLE('',#102076,1.);
#33976=CIRCLE('',#102077,4.);
#33977=CIRCLE('',#102078,5.);
#33978=CIRCLE('',#102080,4.);
#33979=CIRCLE('',#102082,1.);
#33980=CIRCLE('',#102083,3.);
#33981=CIRCLE('',#102084,1.);
#33982=CIRCLE('',#102086,1.);
#33983=CIRCLE('',#102087,3.);
#33984=CIRCLE('',#102088,1.);
#33985=CIRCLE('',#102089,4.);
#33986=CIRCLE('',#102093,4.);
#33987=CIRCLE('',#102094,4.);
#33988=CIRCLE('',#102096,1.);
#33989=CIRCLE('',#102097,1.);
#33990=CIRCLE('',#102099,1.);
#33991=CIRCLE('',#102100,3.);
#33992=CIRCLE('',#102102,1.);
#33993=CIRCLE('',#102103,4.);
#33994=CIRCLE('',#102104,3.);
#33995=CIRCLE('',#102106,4.);
#33996=CIRCLE('',#102108,1.);
#33997=CIRCLE('',#102109,5.);
#33998=CIRCLE('',#102110,1.);
#33999=CIRCLE('',#102112,1.);
#34000=CIRCLE('',#102114,5.);
#34001=CIRCLE('',#102115,1.);
#34002=CIRCLE('',#102117,7.8);
#34003=CIRCLE('',#102118,7.8);
#34004=CIRCLE('',#102120,7.00000000000001);
#34005=CIRCLE('',#102122,7.00000000000001);
#34006=CIRCLE('',#102138,8.65629040278469);
#34007=CIRCLE('',#102139,20.3599346995449);
#34008=CIRCLE('',#102140,20.3599346995449);
#34009=CIRCLE('',#102142,8.8);
#34010=CIRCLE('',#102143,8.8);
#34011=CIRCLE('',#102144,0.25);
#34012=CIRCLE('',#102146,8.55);
#34013=CIRCLE('',#102147,0.25);
#34014=CIRCLE('',#102148,8.8);
#34015=CIRCLE('',#102149,8.8);
#34016=CIRCLE('',#102151,0.750000000000001);
#34017=CIRCLE('',#102152,0.750000000000001);
#34018=CIRCLE('',#102158,7.8);
#34019=CIRCLE('',#102160,7.8);
#34020=CIRCLE('',#102164,0.499999999999998);
#34021=CIRCLE('',#102166,0.5);
#34022=CIRCLE('',#102167,1.);
#34023=CIRCLE('',#102168,0.5);
#34024=CIRCLE('',#102170,0.5);
#34025=CIRCLE('',#102172,0.5);
#34026=CIRCLE('',#102173,1.);
#34027=CIRCLE('',#102174,0.5);
#34028=CIRCLE('',#102177,0.5);
#34029=CIRCLE('',#102178,0.5);
#34030=CIRCLE('',#102180,0.5);
#34031=CIRCLE('',#102181,1.);
#34032=CIRCLE('',#102182,0.5);
#34033=CIRCLE('',#102184,0.5);
#34034=CIRCLE('',#102186,0.499999999999998);
#34035=CIRCLE('',#102187,1.);
#34036=CIRCLE('',#102188,0.5);
#34037=CIRCLE('',#102191,0.5);
#34038=CIRCLE('',#102192,0.5);
#34039=CIRCLE('',#102194,0.5);
#34040=CIRCLE('',#102195,2.5);
#34041=CIRCLE('',#102196,3.);
#34042=CIRCLE('',#102198,0.5);
#34043=CIRCLE('',#102200,0.5);
#34044=CIRCLE('',#102201,0.5);
#34045=CIRCLE('',#102202,1.);
#34046=CIRCLE('',#102204,0.5);
#34047=CIRCLE('',#102206,0.5);
#34048=CIRCLE('',#102207,0.5);
#34049=CIRCLE('',#102208,1.);
#34050=CIRCLE('',#102210,0.5);
#34051=CIRCLE('',#102212,0.5);
#34052=CIRCLE('',#102213,2.5);
#34053=CIRCLE('',#102214,3.);
#34054=CIRCLE('',#102216,0.5);
#34055=CIRCLE('',#102218,0.5);
#34056=CIRCLE('',#102219,0.5);
#34057=CIRCLE('',#102221,0.5);
#34058=CIRCLE('',#102222,2.5);
#34059=CIRCLE('',#102223,3.);
#34060=CIRCLE('',#102225,0.5);
#34061=CIRCLE('',#102227,0.499999999999998);
#34062=CIRCLE('',#102228,0.5);
#34063=CIRCLE('',#102229,1.);
#34064=CIRCLE('',#102232,0.5);
#34065=CIRCLE('',#102233,0.5);
#34066=CIRCLE('',#102235,0.5);
#34067=CIRCLE('',#102236,2.5);
#34068=CIRCLE('',#102237,3.);
#34069=CIRCLE('',#102239,0.5);
#34070=CIRCLE('',#102241,0.500000000000003);
#34071=CIRCLE('',#102242,0.5);
#34072=CIRCLE('',#102243,1.);
#34073=CIRCLE('',#102245,0.5);
#34074=CIRCLE('',#102246,5.);
#34075=CIRCLE('',#102247,5.5);
#34076=CIRCLE('',#102249,0.5);
#34077=CIRCLE('',#102251,0.5);
#34078=CIRCLE('',#102252,0.5);
#34079=CIRCLE('',#102253,1.);
#34080=CIRCLE('',#102255,0.5);
#34081=CIRCLE('',#102257,0.5);
#34082=CIRCLE('',#102258,2.5);
#34083=CIRCLE('',#102259,3.);
#34084=CIRCLE('',#102261,0.5);
#34085=CIRCLE('',#102263,0.5);
#34086=CIRCLE('',#102264,0.5);
#34087=CIRCLE('',#102266,0.5);
#34088=CIRCLE('',#102267,2.5);
#34089=CIRCLE('',#102268,3.);
#34090=CIRCLE('',#102270,0.5);
#34091=CIRCLE('',#102272,0.499999999999998);
#34092=CIRCLE('',#102273,0.5);
#34093=CIRCLE('',#102274,0.999999999999998);
#34094=CIRCLE('',#102276,0.499999999999999);
#34095=CIRCLE('',#102277,58.5);
#34096=CIRCLE('',#102278,58.);
#34097=CIRCLE('',#102280,0.5);
#34098=CIRCLE('',#102281,0.5);
#34099=CIRCLE('',#102282,1.);
#34100=CIRCLE('',#102284,0.5);
#34101=CIRCLE('',#102286,0.5);
#34102=CIRCLE('',#102287,2.5);
#34103=CIRCLE('',#102288,3.);
#34104=CIRCLE('',#102290,0.5);
#34105=CIRCLE('',#102292,0.5);
#34106=CIRCLE('',#102293,0.5);
#34107=CIRCLE('',#102295,0.5);
#34108=CIRCLE('',#102296,2.5);
#34109=CIRCLE('',#102297,3.);
#34110=CIRCLE('',#102299,0.5);
#34111=CIRCLE('',#102301,0.500000000000002);
#34112=CIRCLE('',#102302,0.5);
#34113=CIRCLE('',#102303,1.);
#34114=CIRCLE('',#102305,0.500000000000001);
#34115=CIRCLE('',#102306,58.5);
#34116=CIRCLE('',#102307,58.);
#34117=CIRCLE('',#102309,0.5);
#34118=CIRCLE('',#102310,0.5);
#34119=CIRCLE('',#102311,1.);
#34120=CIRCLE('',#102313,0.5);
#34121=CIRCLE('',#102315,0.5);
#34122=CIRCLE('',#102316,2.5);
#34123=CIRCLE('',#102317,3.);
#34124=CIRCLE('',#102319,0.5);
#34125=CIRCLE('',#102321,0.5);
#34126=CIRCLE('',#102322,0.5);
#34127=CIRCLE('',#102324,0.5);
#34128=CIRCLE('',#102325,2.5);
#34129=CIRCLE('',#102326,3.);
#34130=CIRCLE('',#102328,0.5);
#34131=CIRCLE('',#102330,0.499999999999999);
#34132=CIRCLE('',#102331,0.5);
#34133=CIRCLE('',#102332,1.);
#34134=CIRCLE('',#102334,0.499999999999998);
#34135=CIRCLE('',#102335,58.5);
#34136=CIRCLE('',#102336,58.);
#34137=CIRCLE('',#102338,0.5);
#34138=CIRCLE('',#102339,0.5);
#34139=CIRCLE('',#102340,1.);
#34140=CIRCLE('',#102342,0.5);
#34141=CIRCLE('',#102344,0.5);
#34142=CIRCLE('',#102345,2.5);
#34143=CIRCLE('',#102346,3.);
#34144=CIRCLE('',#102348,0.5);
#34145=CIRCLE('',#102350,0.5);
#34146=CIRCLE('',#102351,0.5);
#34147=CIRCLE('',#102353,0.5);
#34148=CIRCLE('',#102354,2.5);
#34149=CIRCLE('',#102355,3.);
#34150=CIRCLE('',#102357,0.5);
#34151=CIRCLE('',#102359,0.499999999999997);
#34152=CIRCLE('',#102360,0.5);
#34153=CIRCLE('',#102361,1.);
#34154=CIRCLE('',#102363,0.500000000000002);
#34155=CIRCLE('',#102364,58.5);
#34156=CIRCLE('',#102365,58.);
#34157=CIRCLE('',#102367,0.5);
#34158=CIRCLE('',#102368,0.5);
#34159=CIRCLE('',#102369,0.999999999999999);
#34160=CIRCLE('',#102371,0.5);
#34161=CIRCLE('',#102373,0.5);
#34162=CIRCLE('',#102374,2.5);
#34163=CIRCLE('',#102375,3.);
#34164=CIRCLE('',#102377,0.5);
#34165=CIRCLE('',#102379,0.5);
#34166=CIRCLE('',#102380,0.5);
#34167=CIRCLE('',#102382,0.5);
#34168=CIRCLE('',#102383,2.5);
#34169=CIRCLE('',#102384,3.);
#34170=CIRCLE('',#102386,0.5);
#34171=CIRCLE('',#102388,0.500000000000002);
#34172=CIRCLE('',#102389,0.5);
#34173=CIRCLE('',#102390,1.);
#34174=CIRCLE('',#102392,0.499999999999997);
#34175=CIRCLE('',#102393,58.5);
#34176=CIRCLE('',#102394,58.);
#34177=CIRCLE('',#102396,0.5);
#34178=CIRCLE('',#102397,0.5);
#34179=CIRCLE('',#102398,1.);
#34180=CIRCLE('',#102400,0.5);
#34181=CIRCLE('',#102402,0.5);
#34182=CIRCLE('',#102403,2.5);
#34183=CIRCLE('',#102404,3.);
#34184=CIRCLE('',#102406,0.5);
#34185=CIRCLE('',#102408,0.5);
#34186=CIRCLE('',#102409,0.5);
#34187=CIRCLE('',#102411,0.5);
#34188=CIRCLE('',#102412,2.5);
#34189=CIRCLE('',#102413,3.);
#34190=CIRCLE('',#102415,0.5);
#34191=CIRCLE('',#102417,0.499999999999999);
#34192=CIRCLE('',#102418,0.5);
#34193=CIRCLE('',#102419,0.999999999999999);
#34194=CIRCLE('',#102421,0.499999999999999);
#34195=CIRCLE('',#102422,58.5);
#34196=CIRCLE('',#102423,58.);
#34197=CIRCLE('',#102425,0.5);
#34198=CIRCLE('',#102426,0.5);
#34199=CIRCLE('',#102427,1.);
#34200=CIRCLE('',#102429,0.5);
#34201=CIRCLE('',#102431,0.5);
#34202=CIRCLE('',#102432,2.5);
#34203=CIRCLE('',#102433,3.);
#34204=CIRCLE('',#102435,0.5);
#34205=CIRCLE('',#102437,0.5);
#34206=CIRCLE('',#102438,0.5);
#34207=CIRCLE('',#102440,0.5);
#34208=CIRCLE('',#102441,2.5);
#34209=CIRCLE('',#102442,3.);
#34210=CIRCLE('',#102444,0.5);
#34211=CIRCLE('',#102446,0.5);
#34212=CIRCLE('',#102447,0.5);
#34213=CIRCLE('',#102448,1.);
#34214=CIRCLE('',#102450,0.5);
#34215=CIRCLE('',#102452,0.500000000000003);
#34216=CIRCLE('',#102453,5.);
#34217=CIRCLE('',#102454,5.5);
#34218=CIRCLE('',#102456,0.5);
#34219=CIRCLE('',#102457,0.5);
#34220=CIRCLE('',#102458,0.999999999999999);
#34221=CIRCLE('',#102460,0.5);
#34222=CIRCLE('',#102462,0.5);
#34223=CIRCLE('',#102463,2.5);
#34224=CIRCLE('',#102464,3.);
#34225=CIRCLE('',#102466,0.5);
#34226=CIRCLE('',#102468,0.5);
#34227=CIRCLE('',#102469,0.5);
#34228=CIRCLE('',#102471,0.5);
#34229=CIRCLE('',#102472,2.5);
#34230=CIRCLE('',#102473,3.);
#34231=CIRCLE('',#102475,0.5);
#34232=CIRCLE('',#102477,0.5);
#34233=CIRCLE('',#102478,0.5);
#34234=CIRCLE('',#102479,1.);
#34235=CIRCLE('',#102481,0.5);
#34236=CIRCLE('',#102483,0.5);
#34237=CIRCLE('',#102484,0.5);
#34238=CIRCLE('',#102485,1.);
#34239=CIRCLE('',#102487,0.5);
#34240=CIRCLE('',#102489,0.5);
#34241=CIRCLE('',#102490,2.5);
#34242=CIRCLE('',#102491,3.);
#34243=CIRCLE('',#102493,0.5);
#34244=CIRCLE('',#102495,0.500000000000001);
#34245=CIRCLE('',#102497,0.5);
#34246=CIRCLE('',#102498,0.5);
#34247=CIRCLE('',#102499,1.);
#34248=CIRCLE('',#102501,0.5);
#34249=CIRCLE('',#102503,0.5);
#34250=CIRCLE('',#102504,2.5);
#34251=CIRCLE('',#102505,3.);
#34252=CIRCLE('',#102507,0.5);
#34253=CIRCLE('',#102509,0.5);
#34254=CIRCLE('',#102511,0.5);
#34255=CIRCLE('',#102513,0.5);
#34256=CIRCLE('',#102515,0.5);
#34257=CIRCLE('',#102517,0.5);
#34258=CIRCLE('',#102519,0.5);
#34259=CIRCLE('',#102521,0.5);
#34260=CIRCLE('',#102523,0.5);
#34261=CIRCLE('',#102525,0.5);
#34262=CIRCLE('',#102527,0.5);
#34263=CIRCLE('',#102529,0.5);
#34264=CIRCLE('',#102531,0.5);
#34265=CIRCLE('',#102533,0.5);
#34266=CIRCLE('',#102535,0.5);
#34267=CIRCLE('',#102537,0.5);
#34268=CIRCLE('',#102539,0.5);
#34269=CIRCLE('',#102541,0.5);
#34270=CIRCLE('',#102543,0.5);
#34271=CIRCLE('',#102545,0.5);
#34272=CIRCLE('',#102547,0.5);
#34273=CIRCLE('',#102549,0.5);
#34274=CIRCLE('',#102551,0.5);
#34275=CIRCLE('',#102553,0.5);
#34276=CIRCLE('',#102555,0.5);
#34277=CIRCLE('',#102557,0.5);
#34278=CIRCLE('',#102559,0.5);
#34279=CIRCLE('',#102561,77.1121191998622);
#34280=CIRCLE('',#102562,231.99961917989);
#34281=CIRCLE('',#102563,77.1121191998622);
#34282=CIRCLE('',#102566,231.99961917989);
#34283=CIRCLE('',#102583,58.5);
#34284=CIRCLE('',#102589,58.5);
#34285=CIRCLE('',#102595,58.5);
#34286=CIRCLE('',#102601,58.5);
#34287=CIRCLE('',#102608,5.);
#34288=CIRCLE('',#102611,5.);
#34289=CIRCLE('',#102614,58.5);
#34290=CIRCLE('',#102615,58.5);
#34291=CIRCLE('',#102616,77.1121191998622);
#34292=CIRCLE('',#102617,77.1121191998622);
#34293=CIRCLE('',#102646,5.);
#34294=CIRCLE('',#102647,5.);
#34295=CIRCLE('',#102648,5.);
#34296=CIRCLE('',#102649,5.);
#34297=CIRCLE('',#102650,5.);
#34298=CIRCLE('',#102651,5.);
#34299=CIRCLE('',#102659,5.);
#34300=CIRCLE('',#102660,5.);
#34301=CIRCLE('',#102661,5.);
#34302=CIRCLE('',#102662,5.);
#34303=CIRCLE('',#102663,5.);
#34304=CIRCLE('',#102664,5.);
#34305=CIRCLE('',#102678,5.);
#34306=CIRCLE('',#102679,5.);
#34307=CIRCLE('',#102680,5.);
#34308=CIRCLE('',#102681,5.);
#34309=CIRCLE('',#102682,5.);
#34310=CIRCLE('',#102683,5.);
#34311=CIRCLE('',#102691,5.);
#34312=CIRCLE('',#102692,5.);
#34313=CIRCLE('',#102693,5.);
#34314=CIRCLE('',#102694,5.);
#34315=CIRCLE('',#102695,5.);
#34316=CIRCLE('',#102696,5.);
#34317=CIRCLE('',#102717,1.73205080756888);
#34318=CIRCLE('',#102719,1.73205080756888);
#34319=CIRCLE('',#102721,1.73205080756888);
#34320=CIRCLE('',#102723,1.73205080756888);
#34321=CIRCLE('',#102725,1.73205080756888);
#34322=CIRCLE('',#102727,1.73205080756888);
#34323=CIRCLE('',#102729,3.);
#34324=CIRCLE('',#102730,0.25);
#34325=CIRCLE('',#102731,3.25);
#34326=CIRCLE('',#102732,3.25);
#34327=CIRCLE('',#102734,3.25);
#34328=CIRCLE('',#102742,0.75);
#34329=CIRCLE('',#102744,0.643324430555217);
#34330=CIRCLE('',#102745,0.750000000000001);
#34331=CIRCLE('',#102746,0.750000000000001);
#34332=CIRCLE('',#102748,0.750000000000001);
#34333=CIRCLE('',#102750,0.643324430555217);
#34334=CIRCLE('',#102751,0.749999999999999);
#34335=CIRCLE('',#102753,0.750000000000005);
#34336=CIRCLE('',#102754,0.750000000000001);
#34337=CIRCLE('',#102755,1.75);
#34338=CIRCLE('',#102757,0.750000000000001);
#34339=CIRCLE('',#102758,0.633028767237975);
#34340=CIRCLE('',#102760,493.060657452016);
#34341=CIRCLE('',#102762,0.750000000000007);
#34342=CIRCLE('',#102763,493.060657452016);
#34343=CIRCLE('',#102765,0.749999999999994);
#34344=CIRCLE('',#102766,0.633028767237989);
#34345=CIRCLE('',#102768,0.750000000000001);
#34346=CIRCLE('',#102769,1.75);
#34347=CIRCLE('',#102771,0.750000000000001);
#34348=CIRCLE('',#102772,1.75);
#34349=CIRCLE('',#102774,0.750000000000001);
#34350=CIRCLE('',#102775,1.75);
#34351=CIRCLE('',#102788,0.75);
#34352=CIRCLE('',#102791,0.750000000000001);
#34353=CIRCLE('',#102792,0.643324430555217);
#34354=CIRCLE('',#102793,0.750000000000001);
#34355=CIRCLE('',#102795,0.750000000000001);
#34356=CIRCLE('',#102797,0.749999999999999);
#34357=CIRCLE('',#102798,0.643324430555217);
#34358=CIRCLE('',#102800,0.750000000000001);
#34359=CIRCLE('',#102801,0.750000000000005);
#34360=CIRCLE('',#102802,1.75);
#34361=CIRCLE('',#102804,0.633028767237975);
#34362=CIRCLE('',#102805,0.750000000000001);
#34363=CIRCLE('',#102807,493.060657452016);
#34364=CIRCLE('',#102809,493.060657452016);
#34365=CIRCLE('',#102810,0.750000000000007);
#34366=CIRCLE('',#102812,0.633028767237989);
#34367=CIRCLE('',#102813,0.749999999999994);
#34368=CIRCLE('',#102815,0.750000000000001);
#34369=CIRCLE('',#102816,1.75);
#34370=CIRCLE('',#102818,1.75);
#34371=CIRCLE('',#102819,0.750000000000001);
#34372=CIRCLE('',#102821,0.750000000000001);
#34373=CIRCLE('',#102822,1.75);
#34374=CIRCLE('',#102834,0.750000000000001);
#34375=CIRCLE('',#102835,0.750000000000001);
#34376=CIRCLE('',#102837,0.750000000000001);
#34377=CIRCLE('',#102839,0.750000000000001);
#34378=CIRCLE('',#102840,7.00000000000001);
#34379=CIRCLE('',#102841,6.25000000000001);
#34380=CIRCLE('',#102844,0.750000000000001);
#34381=CIRCLE('',#102846,0.750000000000001);
#34382=CIRCLE('',#102847,6.25000000000001);
#34383=CIRCLE('',#102848,7.00000000000001);
#34384=CIRCLE('',#102851,7.00000000000001);
#34385=CIRCLE('',#102853,7.00000000000001);
#34386=CIRCLE('',#102855,7.00000000000001);
#34387=CIRCLE('',#102856,7.00000000000001);
#34388=CIRCLE('',#102858,0.750000000000001);
#34389=CIRCLE('',#102859,0.750000000000001);
#34390=CIRCLE('',#102862,0.750000000000001);
#34391=CIRCLE('',#102864,0.750000000000001);
#34392=CIRCLE('',#102865,6.25000000000001);
#34393=CIRCLE('',#102866,7.00000000000001);
#34394=CIRCLE('',#102869,0.750000000000001);
#34395=CIRCLE('',#102871,0.750000000000001);
#34396=CIRCLE('',#102872,7.00000000000001);
#34397=CIRCLE('',#102873,6.25000000000001);
#34398=CIRCLE('',#102881,2.);
#34399=CIRCLE('',#102901,2.);
#34400=CIRCLE('',#102939,1.66874528305244);
#34401=CIRCLE('',#102941,2.);
#34402=CIRCLE('',#102959,2.16001782903144);
#34403=CIRCLE('',#102979,1.66874528305248);
#34404=CIRCLE('',#102981,2.);
#34405=CIRCLE('',#103019,1.66874528305242);
#34406=CIRCLE('',#103039,1.66874528305242);
#34407=CIRCLE('',#103042,10.);
#34408=CIRCLE('',#103043,10.);
#34409=CIRCLE('',#103050,6.00000000000001);
#34410=CIRCLE('',#103051,6.00000000000001);
#34411=CIRCLE('',#103052,6.00000000000001);
#34412=CIRCLE('',#103053,6.);
#34413=CIRCLE('',#103054,55.3875000000282);
#34414=CIRCLE('',#103057,6.);
#34415=CIRCLE('',#103058,3.);
#34416=CIRCLE('',#103060,3.);
#34417=CIRCLE('',#103064,6.);
#34418=CIRCLE('',#103065,3.);
#34419=CIRCLE('',#103067,3.);
#34420=CIRCLE('',#103071,6.);
#34421=CIRCLE('',#103072,3.);
#34422=CIRCLE('',#103074,3.);
#34423=CIRCLE('',#103078,6.);
#34424=CIRCLE('',#103079,3.);
#34425=CIRCLE('',#103081,3.);
#34426=CIRCLE('',#103083,6.00000000000001);
#34427=CIRCLE('',#103084,6.00000000000001);
#34428=CIRCLE('',#103087,7.00000000000001);
#34429=CIRCLE('',#103088,7.00000000000001);
#34430=CIRCLE('',#103089,6.75);
#34431=CIRCLE('',#103091,5.89644660940673);
#34432=CIRCLE('',#103092,0.25);
#34433=CIRCLE('',#103093,6.07322330470337);
#34434=CIRCLE('',#103094,6.07322330470337);
#34435=CIRCLE('',#103096,6.92677669529664);
#34436=CIRCLE('',#103097,6.92677669529664);
#34437=CIRCLE('',#103098,0.25);
#34438=CIRCLE('',#103099,7.);
#34439=CIRCLE('',#103100,7.);
#34440=CIRCLE('',#103109,2.88675134594813);
#34441=CIRCLE('',#103111,2.88675134594813);
#34442=CIRCLE('',#103113,2.88675134594813);
#34443=CIRCLE('',#103115,2.88675134594813);
#34444=CIRCLE('',#103117,2.88675134594813);
#34445=CIRCLE('',#103119,2.88675134594813);
#34446=CIRCLE('',#103123,202.199982478859);
#34447=CIRCLE('',#103125,0.500000000000001);
#34448=CIRCLE('',#103126,0.499999999999999);
#34449=CIRCLE('',#103127,0.500000000000002);
#34450=CIRCLE('',#103130,0.499999999999998);
#34451=CIRCLE('',#103131,0.499999999999997);
#34452=CIRCLE('',#103132,0.999999999999999);
#34453=CIRCLE('',#103133,0.999999999999998);
#34454=CIRCLE('',#103134,0.999999999999999);
#34455=CIRCLE('',#103135,0.999999999999997);
#34456=CIRCLE('',#103136,1.);
#34457=CIRCLE('',#103139,0.999999999999997);
#34458=CIRCLE('',#103140,0.999999999999997);
#34459=CIRCLE('',#103141,0.999999999999997);
#34460=CIRCLE('',#103144,1.);
#34461=CIRCLE('',#103146,2.5626088159608);
#34462=CIRCLE('',#103147,1.);
#34463=CIRCLE('',#103148,1.);
#34464=CIRCLE('',#103149,7716.37708104352);
#34465=CIRCLE('',#103150,7759.01836682707);
#34466=CIRCLE('',#103152,1.);
#34467=CIRCLE('',#103153,0.999999999999999);
#34468=CIRCLE('',#103155,1.);
#34469=CIRCLE('',#103156,1.);
#34470=CIRCLE('',#103158,7824.7826781668);
#34471=CIRCLE('',#103159,7740.55951768335);
#34472=CIRCLE('',#103160,0.999999999999997);
#34473=CIRCLE('',#103162,0.999999999999999);
#34474=CIRCLE('',#103163,1.);
#34475=CIRCLE('',#103165,1.);
#34476=CIRCLE('',#103166,1.);
#34477=CIRCLE('',#103170,20.);
#34478=CIRCLE('',#103175,3.);
#34479=CIRCLE('',#103177,3.);
#34480=CIRCLE('',#103179,3.);
#34481=CIRCLE('',#103180,1.5);
#34482=CIRCLE('',#103181,1.5);
#34483=CIRCLE('',#103183,3.);
#34484=CIRCLE('',#103185,3.);
#34485=CIRCLE('',#103187,1.5);
#34486=CIRCLE('',#103188,1.5);
#34487=CIRCLE('',#103190,67.5);
#34488=CIRCLE('',#103191,67.5);
#34489=CIRCLE('',#103192,1.5);
#34490=CIRCLE('',#103193,1.5);
#34491=CIRCLE('',#103195,1.5);
#34492=CIRCLE('',#103196,1.5);
#34493=CIRCLE('',#103198,3.);
#34494=CIRCLE('',#103200,3.);
#34495=CIRCLE('',#103202,1.5);
#34496=CIRCLE('',#103203,1.5);
#34497=CIRCLE('',#103205,67.5);
#34498=CIRCLE('',#103206,67.5);
#34499=CIRCLE('',#103207,1.5);
#34500=CIRCLE('',#103208,1.5);
#34501=CIRCLE('',#103210,1.5);
#34502=CIRCLE('',#103211,1.5);
#34503=CIRCLE('',#103213,66.3628828433995);
#34504=CIRCLE('',#103215,66.3628828433995);
#34505=CIRCLE('',#103217,3.);
#34506=CIRCLE('',#103219,3.);
#34507=CIRCLE('',#103221,3.);
#34508=CIRCLE('',#103223,3.);
#34509=CIRCLE('',#103225,58.3875000000282);
#34510=CIRCLE('',#103226,58.3875000000282);
#34511=CIRCLE('',#103227,1.5);
#34512=CIRCLE('',#103228,1.5);
#34513=CIRCLE('',#103230,3.);
#34514=CIRCLE('',#103232,3.);
#34515=CIRCLE('',#103234,1.5);
#34516=CIRCLE('',#103235,1.5);
#34517=CIRCLE('',#103237,67.5);
#34518=CIRCLE('',#103238,67.5);
#34519=CIRCLE('',#103239,1.5);
#34520=CIRCLE('',#103240,1.5);
#34521=CIRCLE('',#103242,1.5);
#34522=CIRCLE('',#103243,1.5);
#34523=CIRCLE('',#103245,58.3875000000282);
#34524=CIRCLE('',#103246,58.3875000000282);
#34525=CIRCLE('',#103247,1.5);
#34526=CIRCLE('',#103248,1.5);
#34527=CIRCLE('',#103250,3.);
#34528=CIRCLE('',#103252,3.);
#34529=CIRCLE('',#103254,1.5);
#34530=CIRCLE('',#103255,1.5);
#34531=CIRCLE('',#103257,67.5);
#34532=CIRCLE('',#103258,67.5);
#34533=CIRCLE('',#103259,1.5);
#34534=CIRCLE('',#103260,1.5);
#34535=CIRCLE('',#103262,1.5);
#34536=CIRCLE('',#103263,1.5);
#34537=CIRCLE('',#103265,58.3875000000282);
#34538=CIRCLE('',#103266,58.3875000000282);
#34539=CIRCLE('',#103268,57.2503828434276);
#34540=CIRCLE('',#103270,54.6455781044285);
#34541=CIRCLE('',#103271,53.8875000000282);
#34542=CIRCLE('',#103273,53.8875000000282);
#34543=CIRCLE('',#103275,57.2503828434277);
#34544=CIRCLE('',#103277,57.2503828434277);
#34545=CIRCLE('',#103279,66.3628828433995);
#34546=CIRCLE('',#103281,66.3628828433995);
#34547=CIRCLE('',#103283,3.);
#34548=CIRCLE('',#103285,58.3875000000282);
#34549=CIRCLE('',#103286,58.3875000000282);
#34550=CIRCLE('',#103288,57.2503828434277);
#34551=CIRCLE('',#103290,2.12684354297908);
#34552=CIRCLE('',#103291,2.13919470072314);
#34553=CIRCLE('',#103298,2.16007343674245);
#34554=CIRCLE('',#103302,2.13474728493424);
#34555=CIRCLE('',#103303,2.14445192257171);
#34556=CIRCLE('',#103313,10.);
#34557=CIRCLE('',#103314,10.);
#34558=CIRCLE('',#103315,10.);
#34559=CIRCLE('',#103317,10.);
#34560=CIRCLE('',#103319,10.);
#34561=CIRCLE('',#103320,10.);
#34562=CIRCLE('',#103322,10.);
#34563=CIRCLE('',#103324,10.);
#34564=CIRCLE('',#103326,10.);
#35201=VERTEX_POINT('',#131310);
#35202=VERTEX_POINT('',#131312);
#35203=VERTEX_POINT('',#131317);
#35204=VERTEX_POINT('',#131321);
#35205=VERTEX_POINT('',#131324);
#35206=VERTEX_POINT('',#131329);
#35207=VERTEX_POINT('',#131331);
#35208=VERTEX_POINT('',#131336);
#35209=VERTEX_POINT('',#131340);
#35210=VERTEX_POINT('',#131343);
#35211=VERTEX_POINT('',#131348);
#35212=VERTEX_POINT('',#131349);
#35213=VERTEX_POINT('',#131351);
#35214=VERTEX_POINT('',#131353);
#35215=VERTEX_POINT('',#131355);
#35216=VERTEX_POINT('',#131363);
#35217=VERTEX_POINT('',#131370);
#35218=VERTEX_POINT('',#131371);
#35219=VERTEX_POINT('',#131373);
#35220=VERTEX_POINT('',#131375);
#35221=VERTEX_POINT('',#131377);
#35222=VERTEX_POINT('',#131384);
#35223=VERTEX_POINT('',#131386);
#35224=VERTEX_POINT('',#131401);
#35225=VERTEX_POINT('',#131414);
#35226=VERTEX_POINT('',#131415);
#35227=VERTEX_POINT('',#131417);
#35228=VERTEX_POINT('',#131419);
#35229=VERTEX_POINT('',#131423);
#35230=VERTEX_POINT('',#131424);
#35231=VERTEX_POINT('',#131426);
#35232=VERTEX_POINT('',#131428);
#35233=VERTEX_POINT('',#131436);
#35234=VERTEX_POINT('',#131438);
#35235=VERTEX_POINT('',#131446);
#35236=VERTEX_POINT('',#131448);
#35237=VERTEX_POINT('',#131450);
#35238=VERTEX_POINT('',#131470);
#35239=VERTEX_POINT('',#131510);
#35240=VERTEX_POINT('',#131512);
#35241=VERTEX_POINT('',#131514);
#35242=VERTEX_POINT('',#131522);
#35243=VERTEX_POINT('',#131524);
#35244=VERTEX_POINT('',#131534);
#35245=VERTEX_POINT('',#131536);
#35246=VERTEX_POINT('',#131540);
#35247=VERTEX_POINT('',#131541);
#35248=VERTEX_POINT('',#131543);
#35249=VERTEX_POINT('',#131545);
#35250=VERTEX_POINT('',#131552);
#35251=VERTEX_POINT('',#131554);
#35252=VERTEX_POINT('',#131558);
#35253=VERTEX_POINT('',#131559);
#35254=VERTEX_POINT('',#131579);
#35255=VERTEX_POINT('',#131581);
#35256=VERTEX_POINT('',#131583);
#35257=VERTEX_POINT('',#131591);
#35258=VERTEX_POINT('',#131593);
#35259=VERTEX_POINT('',#131601);
#35260=VERTEX_POINT('',#131603);
#35261=VERTEX_POINT('',#131605);
#35262=VERTEX_POINT('',#131607);
#35263=VERTEX_POINT('',#131615);
#35264=VERTEX_POINT('',#131617);
#35265=VERTEX_POINT('',#131625);
#35266=VERTEX_POINT('',#131629);
#35267=VERTEX_POINT('',#131656);
#35268=VERTEX_POINT('',#131657);
#35269=VERTEX_POINT('',#131659);
#35270=VERTEX_POINT('',#131668);
#35271=VERTEX_POINT('',#131679);
#35272=VERTEX_POINT('',#131680);
#35273=VERTEX_POINT('',#131685);
#35274=VERTEX_POINT('',#131686);
#35275=VERTEX_POINT('',#131689);
#35276=VERTEX_POINT('',#131693);
#35277=VERTEX_POINT('',#131694);
#35278=VERTEX_POINT('',#131696);
#35279=VERTEX_POINT('',#131698);
#35280=VERTEX_POINT('',#131701);
#35281=VERTEX_POINT('',#131734);
#35282=VERTEX_POINT('',#131781);
#35283=VERTEX_POINT('',#131805);
#35284=VERTEX_POINT('',#131807);
#35285=VERTEX_POINT('',#131840);
#35286=VERTEX_POINT('',#131878);
#35287=VERTEX_POINT('',#131891);
#35288=VERTEX_POINT('',#131892);
#35289=VERTEX_POINT('',#131897);
#35290=VERTEX_POINT('',#131898);
#35291=VERTEX_POINT('',#131901);
#35292=VERTEX_POINT('',#131905);
#35293=VERTEX_POINT('',#131906);
#35294=VERTEX_POINT('',#131908);
#35295=VERTEX_POINT('',#131910);
#35296=VERTEX_POINT('',#131932);
#35297=VERTEX_POINT('',#131939);
#35298=VERTEX_POINT('',#131948);
#35299=VERTEX_POINT('',#131950);
#35300=VERTEX_POINT('',#131983);
#35301=VERTEX_POINT('',#132027);
#35302=VERTEX_POINT('',#132067);
#35303=VERTEX_POINT('',#132068);
#35304=VERTEX_POINT('',#132073);
#35305=VERTEX_POINT('',#132074);
#35306=VERTEX_POINT('',#132077);
#35307=VERTEX_POINT('',#132081);
#35308=VERTEX_POINT('',#132082);
#35309=VERTEX_POINT('',#132084);
#35310=VERTEX_POINT('',#132118);
#35311=VERTEX_POINT('',#132162);
#35312=VERTEX_POINT('',#132178);
#35313=VERTEX_POINT('',#132179);
#35314=VERTEX_POINT('',#132181);
#35315=VERTEX_POINT('',#132183);
#35316=VERTEX_POINT('',#132205);
#35317=VERTEX_POINT('',#132206);
#35318=VERTEX_POINT('',#132209);
#35319=VERTEX_POINT('',#132216);
#35320=VERTEX_POINT('',#132217);
#35321=VERTEX_POINT('',#132219);
#35322=VERTEX_POINT('',#132241);
#35323=VERTEX_POINT('',#132242);
#35324=VERTEX_POINT('',#132257);
#35325=VERTEX_POINT('',#132258);
#35326=VERTEX_POINT('',#132292);
#35327=VERTEX_POINT('',#132293);
#35328=VERTEX_POINT('',#132352);
#35329=VERTEX_POINT('',#132354);
#35330=VERTEX_POINT('',#132358);
#35331=VERTEX_POINT('',#132359);
#35332=VERTEX_POINT('',#132362);
#35333=VERTEX_POINT('',#132366);
#35334=VERTEX_POINT('',#132367);
#35335=VERTEX_POINT('',#132369);
#35336=VERTEX_POINT('',#132403);
#35337=VERTEX_POINT('',#132404);
#35338=VERTEX_POINT('',#132471);
#35339=VERTEX_POINT('',#132472);
#35340=VERTEX_POINT('',#132494);
#35341=VERTEX_POINT('',#132495);
#35342=VERTEX_POINT('',#132510);
#35343=VERTEX_POINT('',#132511);
#35344=VERTEX_POINT('',#132516);
#35345=VERTEX_POINT('',#132517);
#35346=VERTEX_POINT('',#132520);
#35347=VERTEX_POINT('',#132524);
#35348=VERTEX_POINT('',#132525);
#35349=VERTEX_POINT('',#132527);
#35350=VERTEX_POINT('',#132561);
#35351=VERTEX_POINT('',#132562);
#35352=VERTEX_POINT('',#132598);
#35353=VERTEX_POINT('',#132599);
#35354=VERTEX_POINT('',#132639);
#35355=VERTEX_POINT('',#132640);
#35356=VERTEX_POINT('',#132698);
#35357=VERTEX_POINT('',#132699);
#35358=VERTEX_POINT('',#132715);
#35359=VERTEX_POINT('',#132717);
#35360=VERTEX_POINT('',#132724);
#35361=VERTEX_POINT('',#132739);
#35362=VERTEX_POINT('',#132752);
#35363=VERTEX_POINT('',#132753);
#35364=VERTEX_POINT('',#132755);
#35365=VERTEX_POINT('',#132757);
#35366=VERTEX_POINT('',#132759);
#35367=VERTEX_POINT('',#132766);
#35368=VERTEX_POINT('',#132771);
#35369=VERTEX_POINT('',#132780);
#35370=VERTEX_POINT('',#132782);
#35371=VERTEX_POINT('',#132784);
#35372=VERTEX_POINT('',#132786);
#35373=VERTEX_POINT('',#132830);
#35374=VERTEX_POINT('',#132832);
#35375=VERTEX_POINT('',#132839);
#35376=VERTEX_POINT('',#132841);
#35377=VERTEX_POINT('',#132843);
#35378=VERTEX_POINT('',#132845);
#35379=VERTEX_POINT('',#132854);
#35380=VERTEX_POINT('',#132856);
#35381=VERTEX_POINT('',#132909);
#35382=VERTEX_POINT('',#132911);
#35383=VERTEX_POINT('',#132913);
#35384=VERTEX_POINT('',#132915);
#35385=VERTEX_POINT('',#132926);
#35386=VERTEX_POINT('',#132928);
#35387=VERTEX_POINT('',#132951);
#35388=VERTEX_POINT('',#132953);
#35389=VERTEX_POINT('',#132955);
#35390=VERTEX_POINT('',#132957);
#35391=VERTEX_POINT('',#133001);
#35392=VERTEX_POINT('',#133003);
#35393=VERTEX_POINT('',#133050);
#35394=VERTEX_POINT('',#133052);
#35395=VERTEX_POINT('',#133054);
#35396=VERTEX_POINT('',#133056);
#35397=VERTEX_POINT('',#133100);
#35398=VERTEX_POINT('',#133102);
#35399=VERTEX_POINT('',#133111);
#35400=VERTEX_POINT('',#133113);
#35401=VERTEX_POINT('',#133115);
#35402=VERTEX_POINT('',#133135);
#35403=VERTEX_POINT('',#133137);
#35404=VERTEX_POINT('',#133144);
#35405=VERTEX_POINT('',#133165);
#35406=VERTEX_POINT('',#133174);
#35407=VERTEX_POINT('',#133175);
#35408=VERTEX_POINT('',#133177);
#35409=VERTEX_POINT('',#133179);
#35410=VERTEX_POINT('',#133183);
#35411=VERTEX_POINT('',#133184);
#35412=VERTEX_POINT('',#133186);
#35413=VERTEX_POINT('',#133188);
#35414=VERTEX_POINT('',#133196);
#35415=VERTEX_POINT('',#133198);
#35416=VERTEX_POINT('',#133206);
#35417=VERTEX_POINT('',#133208);
#35418=VERTEX_POINT('',#133210);
#35419=VERTEX_POINT('',#133230);
#35420=VERTEX_POINT('',#133234);
#35421=VERTEX_POINT('',#133236);
#35422=VERTEX_POINT('',#133238);
#35423=VERTEX_POINT('',#133246);
#35424=VERTEX_POINT('',#133248);
#35425=VERTEX_POINT('',#133258);
#35426=VERTEX_POINT('',#133260);
#35427=VERTEX_POINT('',#133264);
#35428=VERTEX_POINT('',#133265);
#35429=VERTEX_POINT('',#133267);
#35430=VERTEX_POINT('',#133269);
#35431=VERTEX_POINT('',#133276);
#35432=VERTEX_POINT('',#133278);
#35433=VERTEX_POINT('',#133282);
#35434=VERTEX_POINT('',#133283);
#35435=VERTEX_POINT('',#133285);
#35436=VERTEX_POINT('',#133287);
#35437=VERTEX_POINT('',#133295);
#35438=VERTEX_POINT('',#133297);
#35439=VERTEX_POINT('',#133305);
#35440=VERTEX_POINT('',#133309);
#35441=VERTEX_POINT('',#133326);
#35442=VERTEX_POINT('',#133328);
#35443=VERTEX_POINT('',#133336);
#35444=VERTEX_POINT('',#133338);
#35445=VERTEX_POINT('',#133365);
#35446=VERTEX_POINT('',#133374);
#35447=VERTEX_POINT('',#133378);
#35448=VERTEX_POINT('',#133379);
#35449=VERTEX_POINT('',#133384);
#35450=VERTEX_POINT('',#133386);
#35451=VERTEX_POINT('',#133413);
#35452=VERTEX_POINT('',#133424);
#35453=VERTEX_POINT('',#133457);
#35454=VERTEX_POINT('',#133470);
#35455=VERTEX_POINT('',#133474);
#35456=VERTEX_POINT('',#133475);
#35457=VERTEX_POINT('',#133480);
#35458=VERTEX_POINT('',#133482);
#35459=VERTEX_POINT('',#133515);
#35460=VERTEX_POINT('',#133539);
#35461=VERTEX_POINT('',#133578);
#35462=VERTEX_POINT('',#133630);
#35463=VERTEX_POINT('',#133634);
#35464=VERTEX_POINT('',#133635);
#35465=VERTEX_POINT('',#133640);
#35466=VERTEX_POINT('',#133642);
#35467=VERTEX_POINT('',#133675);
#35468=VERTEX_POINT('',#133738);
#35469=VERTEX_POINT('',#133771);
#35470=VERTEX_POINT('',#133823);
#35471=VERTEX_POINT('',#133827);
#35472=VERTEX_POINT('',#133828);
#35473=VERTEX_POINT('',#133833);
#35474=VERTEX_POINT('',#133835);
#35475=VERTEX_POINT('',#133868);
#35476=VERTEX_POINT('',#133892);
#35477=VERTEX_POINT('',#133919);
#35478=VERTEX_POINT('',#133930);
#35479=VERTEX_POINT('',#133934);
#35480=VERTEX_POINT('',#133935);
#35481=VERTEX_POINT('',#133940);
#35482=VERTEX_POINT('',#133942);
#35483=VERTEX_POINT('',#133963);
#35484=VERTEX_POINT('',#133972);
#35485=VERTEX_POINT('',#134005);
#35486=VERTEX_POINT('',#134045);
#35487=VERTEX_POINT('',#134049);
#35488=VERTEX_POINT('',#134050);
#35489=VERTEX_POINT('',#134055);
#35490=VERTEX_POINT('',#134057);
#35491=VERTEX_POINT('',#134093);
#35492=VERTEX_POINT('',#134094);
#35493=VERTEX_POINT('',#134117);
#35494=VERTEX_POINT('',#134119);
#35495=VERTEX_POINT('',#134140);
#35496=VERTEX_POINT('',#134149);
#35497=VERTEX_POINT('',#134170);
#35498=VERTEX_POINT('',#134179);
#35499=VERTEX_POINT('',#134183);
#35500=VERTEX_POINT('',#134213);
#35501=VERTEX_POINT('',#134222);
#35502=VERTEX_POINT('',#134243);
#35503=VERTEX_POINT('',#134245);
#35504=VERTEX_POINT('',#134259);
#35505=VERTEX_POINT('',#134272);
#35506=VERTEX_POINT('',#134274);
#35507=VERTEX_POINT('',#134295);
#35508=VERTEX_POINT('',#134304);
#35509=VERTEX_POINT('',#134325);
#35510=VERTEX_POINT('',#134334);
#35511=VERTEX_POINT('',#134357);
#35512=VERTEX_POINT('',#134366);
#35513=VERTEX_POINT('',#134367);
#35514=VERTEX_POINT('',#134390);
#35515=VERTEX_POINT('',#134392);
#35516=VERTEX_POINT('',#134413);
#35517=VERTEX_POINT('',#134422);
#35518=VERTEX_POINT('',#134443);
#35519=VERTEX_POINT('',#134452);
#35520=VERTEX_POINT('',#134473);
#35521=VERTEX_POINT('',#134493);
#35522=VERTEX_POINT('',#134506);
#35523=VERTEX_POINT('',#134508);
#35524=VERTEX_POINT('',#134529);
#35525=VERTEX_POINT('',#134538);
#35526=VERTEX_POINT('',#134559);
#35527=VERTEX_POINT('',#134568);
#35528=VERTEX_POINT('',#134574);
#35529=VERTEX_POINT('',#134575);
#35530=VERTEX_POINT('',#134598);
#35531=VERTEX_POINT('',#134600);
#35532=VERTEX_POINT('',#134621);
#35533=VERTEX_POINT('',#134630);
#35534=VERTEX_POINT('',#134651);
#35535=VERTEX_POINT('',#134660);
#35536=VERTEX_POINT('',#134664);
#35537=VERTEX_POINT('',#134688);
#35538=VERTEX_POINT('',#134692);
#35539=VERTEX_POINT('',#134713);
#35540=VERTEX_POINT('',#134715);
#35541=VERTEX_POINT('',#134722);
#35542=VERTEX_POINT('',#134738);
#35543=VERTEX_POINT('',#134751);
#35544=VERTEX_POINT('',#134753);
#35545=VERTEX_POINT('',#134774);
#35546=VERTEX_POINT('',#134783);
#35547=VERTEX_POINT('',#134804);
#35548=VERTEX_POINT('',#134813);
#35549=VERTEX_POINT('',#134834);
#35550=VERTEX_POINT('',#134835);
#35551=VERTEX_POINT('',#134850);
#35552=VERTEX_POINT('',#134852);
#35553=VERTEX_POINT('',#134869);
#35554=VERTEX_POINT('',#134882);
#35555=VERTEX_POINT('',#134884);
#35556=VERTEX_POINT('',#134905);
#35557=VERTEX_POINT('',#134914);
#35558=VERTEX_POINT('',#134935);
#35559=VERTEX_POINT('',#134944);
#35560=VERTEX_POINT('',#134948);
#35561=VERTEX_POINT('',#134949);
#35562=VERTEX_POINT('',#134972);
#35563=VERTEX_POINT('',#134974);
#35564=VERTEX_POINT('',#134995);
#35565=VERTEX_POINT('',#135004);
#35566=VERTEX_POINT('',#135025);
#35567=VERTEX_POINT('',#135027);
#35568=VERTEX_POINT('',#135036);
#35569=VERTEX_POINT('',#135038);
#35570=VERTEX_POINT('',#135042);
#35571=VERTEX_POINT('',#135055);
#35572=VERTEX_POINT('',#135057);
#35573=VERTEX_POINT('',#135059);
#35574=VERTEX_POINT('',#135061);
#35575=VERTEX_POINT('',#135063);
#35576=VERTEX_POINT('',#135065);
#35577=VERTEX_POINT('',#135069);
#35578=VERTEX_POINT('',#135071);
#35579=VERTEX_POINT('',#135073);
#35580=VERTEX_POINT('',#135077);
#35581=VERTEX_POINT('',#135079);
#35582=VERTEX_POINT('',#135083);
#35583=VERTEX_POINT('',#135098);
#35584=VERTEX_POINT('',#135099);
#35585=VERTEX_POINT('',#135115);
#35586=VERTEX_POINT('',#135120);
#35587=VERTEX_POINT('',#135168);
#35588=VERTEX_POINT('',#135209);
#35589=VERTEX_POINT('',#135224);
#35590=VERTEX_POINT('',#135233);
#35591=VERTEX_POINT('',#135234);
#35592=VERTEX_POINT('',#135236);
#35593=VERTEX_POINT('',#135238);
#35594=VERTEX_POINT('',#135242);
#35595=VERTEX_POINT('',#135244);
#35596=VERTEX_POINT('',#135248);
#35597=VERTEX_POINT('',#135249);
#35598=VERTEX_POINT('',#135256);
#35599=VERTEX_POINT('',#135263);
#35600=VERTEX_POINT('',#135268);
#35601=VERTEX_POINT('',#135280);
#35602=VERTEX_POINT('',#135282);
#35603=VERTEX_POINT('',#135284);
#35604=VERTEX_POINT('',#135288);
#35605=VERTEX_POINT('',#135290);
#35606=VERTEX_POINT('',#135294);
#35607=VERTEX_POINT('',#135296);
#35608=VERTEX_POINT('',#135300);
#35609=VERTEX_POINT('',#135302);
#35610=VERTEX_POINT('',#135306);
#35611=VERTEX_POINT('',#135308);
#35612=VERTEX_POINT('',#135312);
#35613=VERTEX_POINT('',#135314);
#35614=VERTEX_POINT('',#135318);
#35615=VERTEX_POINT('',#135319);
#35616=VERTEX_POINT('',#135321);
#35617=VERTEX_POINT('',#135323);
#35618=VERTEX_POINT('',#135337);
#35619=VERTEX_POINT('',#135383);
#35620=VERTEX_POINT('',#135385);
#35621=VERTEX_POINT('',#135387);
#35622=VERTEX_POINT('',#135391);
#35623=VERTEX_POINT('',#135393);
#35624=VERTEX_POINT('',#135397);
#35625=VERTEX_POINT('',#135399);
#35626=VERTEX_POINT('',#135403);
#35627=VERTEX_POINT('',#135405);
#35628=VERTEX_POINT('',#135409);
#35629=VERTEX_POINT('',#135411);
#35630=VERTEX_POINT('',#135415);
#35631=VERTEX_POINT('',#135417);
#35632=VERTEX_POINT('',#135438);
#35633=VERTEX_POINT('',#135445);
#35634=VERTEX_POINT('',#135447);
#35635=VERTEX_POINT('',#135465);
#35636=VERTEX_POINT('',#135467);
#35637=VERTEX_POINT('',#135471);
#35638=VERTEX_POINT('',#135473);
#35639=VERTEX_POINT('',#135475);
#35640=VERTEX_POINT('',#135479);
#35641=VERTEX_POINT('',#135481);
#35642=VERTEX_POINT('',#135485);
#35643=VERTEX_POINT('',#135487);
#35644=VERTEX_POINT('',#135491);
#35645=VERTEX_POINT('',#135493);
#35646=VERTEX_POINT('',#135497);
#35647=VERTEX_POINT('',#135499);
#35648=VERTEX_POINT('',#135503);
#35649=VERTEX_POINT('',#135505);
#35650=VERTEX_POINT('',#135507);
#35651=VERTEX_POINT('',#135511);
#35652=VERTEX_POINT('',#135513);
#35653=VERTEX_POINT('',#135515);
#35654=VERTEX_POINT('',#135519);
#35655=VERTEX_POINT('',#135521);
#35656=VERTEX_POINT('',#135525);
#35657=VERTEX_POINT('',#135527);
#35658=VERTEX_POINT('',#135531);
#35659=VERTEX_POINT('',#135533);
#35660=VERTEX_POINT('',#135537);
#35661=VERTEX_POINT('',#135539);
#35662=VERTEX_POINT('',#135543);
#35663=VERTEX_POINT('',#135545);
#35664=VERTEX_POINT('',#135547);
#35665=VERTEX_POINT('',#135551);
#35666=VERTEX_POINT('',#135556);
#35667=VERTEX_POINT('',#135558);
#35668=VERTEX_POINT('',#135560);
#35669=VERTEX_POINT('',#135562);
#35670=VERTEX_POINT('',#135564);
#35671=VERTEX_POINT('',#135575);
#35672=VERTEX_POINT('',#135577);
#35673=VERTEX_POINT('',#135611);
#35674=VERTEX_POINT('',#135613);
#35675=VERTEX_POINT('',#135626);
#35676=VERTEX_POINT('',#135627);
#35677=VERTEX_POINT('',#135629);
#35678=VERTEX_POINT('',#135631);
#35679=VERTEX_POINT('',#135635);
#35680=VERTEX_POINT('',#135640);
#35681=VERTEX_POINT('',#135642);
#35682=VERTEX_POINT('',#135646);
#35683=VERTEX_POINT('',#135648);
#35684=VERTEX_POINT('',#135652);
#35685=VERTEX_POINT('',#135653);
#35686=VERTEX_POINT('',#135658);
#35687=VERTEX_POINT('',#135659);
#35688=VERTEX_POINT('',#135664);
#35689=VERTEX_POINT('',#135665);
#35690=VERTEX_POINT('',#135670);
#35691=VERTEX_POINT('',#135671);
#35692=VERTEX_POINT('',#135676);
#35693=VERTEX_POINT('',#135677);
#35694=VERTEX_POINT('',#135682);
#35695=VERTEX_POINT('',#135683);
#35696=VERTEX_POINT('',#135688);
#35697=VERTEX_POINT('',#135689);
#35698=VERTEX_POINT('',#135694);
#35699=VERTEX_POINT('',#135695);
#35700=VERTEX_POINT('',#135700);
#35701=VERTEX_POINT('',#135701);
#35702=VERTEX_POINT('',#135706);
#35703=VERTEX_POINT('',#135707);
#35704=VERTEX_POINT('',#135712);
#35705=VERTEX_POINT('',#135713);
#35706=VERTEX_POINT('',#135718);
#35707=VERTEX_POINT('',#135719);
#35708=VERTEX_POINT('',#135724);
#35709=VERTEX_POINT('',#135725);
#35710=VERTEX_POINT('',#135730);
#35711=VERTEX_POINT('',#135731);
#35712=VERTEX_POINT('',#135736);
#35713=VERTEX_POINT('',#135737);
#35714=VERTEX_POINT('',#135764);
#35715=VERTEX_POINT('',#135766);
#35716=VERTEX_POINT('',#135769);
#35717=VERTEX_POINT('',#135771);
#35718=VERTEX_POINT('',#135792);
#35719=VERTEX_POINT('',#135793);
#35720=VERTEX_POINT('',#135795);
#35721=VERTEX_POINT('',#135804);
#35722=VERTEX_POINT('',#135807);
#35723=VERTEX_POINT('',#135816);
#35724=VERTEX_POINT('',#135866);
#35725=VERTEX_POINT('',#135867);
#35726=VERTEX_POINT('',#135869);
#35727=VERTEX_POINT('',#135880);
#35728=VERTEX_POINT('',#135926);
#35729=VERTEX_POINT('',#135928);
#35730=VERTEX_POINT('',#135932);
#35731=VERTEX_POINT('',#135934);
#35732=VERTEX_POINT('',#135936);
#35733=VERTEX_POINT('',#135940);
#35734=VERTEX_POINT('',#135941);
#35735=VERTEX_POINT('',#135943);
#35736=VERTEX_POINT('',#135977);
#35737=VERTEX_POINT('',#135978);
#35738=VERTEX_POINT('',#136064);
#35739=VERTEX_POINT('',#136065);
#35740=VERTEX_POINT('',#136087);
#35741=VERTEX_POINT('',#136094);
#35742=VERTEX_POINT('',#136103);
#35743=VERTEX_POINT('',#136105);
#35744=VERTEX_POINT('',#136109);
#35745=VERTEX_POINT('',#136111);
#35746=VERTEX_POINT('',#136113);
#35747=VERTEX_POINT('',#136117);
#35748=VERTEX_POINT('',#136118);
#35749=VERTEX_POINT('',#136120);
#35750=VERTEX_POINT('',#136148);
#35751=VERTEX_POINT('',#136149);
#35752=VERTEX_POINT('',#136179);
#35753=VERTEX_POINT('',#136180);
#35754=VERTEX_POINT('',#136214);
#35755=VERTEX_POINT('',#136267);
#35756=VERTEX_POINT('',#136280);
#35757=VERTEX_POINT('',#136282);
#35758=VERTEX_POINT('',#136286);
#35759=VERTEX_POINT('',#136288);
#35760=VERTEX_POINT('',#136290);
#35761=VERTEX_POINT('',#136294);
#35762=VERTEX_POINT('',#136295);
#35763=VERTEX_POINT('',#136297);
#35764=VERTEX_POINT('',#136331);
#35765=VERTEX_POINT('',#136332);
#35766=VERTEX_POINT('',#136394);
#35767=VERTEX_POINT('',#136395);
#35768=VERTEX_POINT('',#136397);
#35769=VERTEX_POINT('',#136403);
#35770=VERTEX_POINT('',#136423);
#35771=VERTEX_POINT('',#136424);
#35772=VERTEX_POINT('',#136426);
#35773=VERTEX_POINT('',#136469);
#35774=VERTEX_POINT('',#136480);
#35775=VERTEX_POINT('',#136511);
#35776=VERTEX_POINT('',#136513);
#35777=VERTEX_POINT('',#136613);
#35778=VERTEX_POINT('',#136617);
#35779=VERTEX_POINT('',#136622);
#35780=VERTEX_POINT('',#136624);
#35781=VERTEX_POINT('',#136626);
#35782=VERTEX_POINT('',#136628);
#35783=VERTEX_POINT('',#136635);
#35784=VERTEX_POINT('',#136636);
#35785=VERTEX_POINT('',#136672);
#35786=VERTEX_POINT('',#136676);
#35787=VERTEX_POINT('',#136714);
#35788=VERTEX_POINT('',#136753);
#35789=VERTEX_POINT('',#136755);
#35790=VERTEX_POINT('',#136760);
#35791=VERTEX_POINT('',#136774);
#35792=VERTEX_POINT('',#136776);
#35793=VERTEX_POINT('',#136836);
#35794=VERTEX_POINT('',#136864);
#35795=VERTEX_POINT('',#136917);
#35796=VERTEX_POINT('',#136977);
#35797=VERTEX_POINT('',#136981);
#35798=VERTEX_POINT('',#137032);
#35799=VERTEX_POINT('',#137037);
#35800=VERTEX_POINT('',#137051);
#35801=VERTEX_POINT('',#137053);
#35802=VERTEX_POINT('',#137067);
#35803=VERTEX_POINT('',#137074);
#35804=VERTEX_POINT('',#137075);
#35805=VERTEX_POINT('',#137102);
#35806=VERTEX_POINT('',#137106);
#35807=VERTEX_POINT('',#137108);
#35808=VERTEX_POINT('',#137110);
#35809=VERTEX_POINT('',#137112);
#35810=VERTEX_POINT('',#137115);
#35811=VERTEX_POINT('',#137117);
#35812=VERTEX_POINT('',#137122);
#35813=VERTEX_POINT('',#137139);
#35814=VERTEX_POINT('',#137141);
#35815=VERTEX_POINT('',#137160);
#35816=VERTEX_POINT('',#137164);
#35817=VERTEX_POINT('',#137168);
#35818=VERTEX_POINT('',#137183);
#35819=VERTEX_POINT('',#137187);
#35820=VERTEX_POINT('',#137189);
#35821=VERTEX_POINT('',#137191);
#35822=VERTEX_POINT('',#137194);
#35823=VERTEX_POINT('',#137199);
#35824=VERTEX_POINT('',#137216);
#35825=VERTEX_POINT('',#137218);
#35826=VERTEX_POINT('',#137232);
#35827=VERTEX_POINT('',#137239);
#35828=VERTEX_POINT('',#137240);
#35829=VERTEX_POINT('',#137268);
#35830=VERTEX_POINT('',#137272);
#35831=VERTEX_POINT('',#137274);
#35832=VERTEX_POINT('',#137276);
#35833=VERTEX_POINT('',#137278);
#35834=VERTEX_POINT('',#137281);
#35835=VERTEX_POINT('',#137283);
#35836=VERTEX_POINT('',#137288);
#35837=VERTEX_POINT('',#137314);
#35838=VERTEX_POINT('',#137316);
#35839=VERTEX_POINT('',#137343);
#35840=VERTEX_POINT('',#137344);
#35841=VERTEX_POINT('',#137367);
#35842=VERTEX_POINT('',#137371);
#35843=VERTEX_POINT('',#137373);
#35844=VERTEX_POINT('',#137376);
#35845=VERTEX_POINT('',#137378);
#35846=VERTEX_POINT('',#137380);
#35847=VERTEX_POINT('',#137397);
#35848=VERTEX_POINT('',#137404);
#35849=VERTEX_POINT('',#137408);
#35850=VERTEX_POINT('',#137412);
#35851=VERTEX_POINT('',#137416);
#35852=VERTEX_POINT('',#137418);
#35853=VERTEX_POINT('',#137423);
#35854=VERTEX_POINT('',#137432);
#35855=VERTEX_POINT('',#137435);
#35856=VERTEX_POINT('',#137452);
#35857=VERTEX_POINT('',#137453);
#35858=VERTEX_POINT('',#137480);
#35859=VERTEX_POINT('',#137484);
#35860=VERTEX_POINT('',#137550);
#35861=VERTEX_POINT('',#137552);
#35862=VERTEX_POINT('',#137587);
#35863=VERTEX_POINT('',#137638);
#35864=VERTEX_POINT('',#137666);
#35865=VERTEX_POINT('',#137716);
#35866=VERTEX_POINT('',#137791);
#35867=VERTEX_POINT('',#137795);
#35868=VERTEX_POINT('',#137856);
#35869=VERTEX_POINT('',#137860);
#35870=VERTEX_POINT('',#137893);
#35871=VERTEX_POINT('',#137940);
#35872=VERTEX_POINT('',#137966);
#35873=VERTEX_POINT('',#138011);
#35874=VERTEX_POINT('',#138044);
#35875=VERTEX_POINT('',#138046);
#35876=VERTEX_POINT('',#138050);
#35877=VERTEX_POINT('',#138054);
#35878=VERTEX_POINT('',#138058);
#35879=VERTEX_POINT('',#138060);
#35880=VERTEX_POINT('',#138064);
#35881=VERTEX_POINT('',#138068);
#35882=VERTEX_POINT('',#138072);
#35883=VERTEX_POINT('',#138073);
#35884=VERTEX_POINT('',#138075);
#35885=VERTEX_POINT('',#138077);
#35886=VERTEX_POINT('',#138080);
#35887=VERTEX_POINT('',#138082);
#35888=VERTEX_POINT('',#138090);
#35889=VERTEX_POINT('',#138116);
#35890=VERTEX_POINT('',#138118);
#35891=VERTEX_POINT('',#138141);
#35892=VERTEX_POINT('',#138149);
#35893=VERTEX_POINT('',#138166);
#35894=VERTEX_POINT('',#138167);
#35895=VERTEX_POINT('',#138199);
#35896=VERTEX_POINT('',#138203);
#35897=VERTEX_POINT('',#138205);
#35898=VERTEX_POINT('',#138207);
#35899=VERTEX_POINT('',#138209);
#35900=VERTEX_POINT('',#138211);
#35901=VERTEX_POINT('',#138213);
#35902=VERTEX_POINT('',#138215);
#35903=VERTEX_POINT('',#138217);
#35904=VERTEX_POINT('',#138225);
#35905=VERTEX_POINT('',#138234);
#35906=VERTEX_POINT('',#138236);
#35907=VERTEX_POINT('',#138261);
#35908=VERTEX_POINT('',#138265);
#35909=VERTEX_POINT('',#138269);
#35910=VERTEX_POINT('',#138284);
#35911=VERTEX_POINT('',#138288);
#35912=VERTEX_POINT('',#138296);
#35913=VERTEX_POINT('',#138313);
#35914=VERTEX_POINT('',#138315);
#35915=VERTEX_POINT('',#138329);
#35916=VERTEX_POINT('',#138337);
#35917=VERTEX_POINT('',#138339);
#35918=VERTEX_POINT('',#138341);
#35919=VERTEX_POINT('',#138343);
#35920=VERTEX_POINT('',#138347);
#35921=VERTEX_POINT('',#138348);
#35922=VERTEX_POINT('',#138381);
#35923=VERTEX_POINT('',#138385);
#35924=VERTEX_POINT('',#138438);
#35925=VERTEX_POINT('',#138440);
#35926=VERTEX_POINT('',#138478);
#35927=VERTEX_POINT('',#138480);
#35928=VERTEX_POINT('',#138482);
#35929=VERTEX_POINT('',#138487);
#35930=VERTEX_POINT('',#138501);
#35931=VERTEX_POINT('',#138503);
#35932=VERTEX_POINT('',#138563);
#35933=VERTEX_POINT('',#138591);
#35934=VERTEX_POINT('',#138652);
#35935=VERTEX_POINT('',#138703);
#35936=VERTEX_POINT('',#138707);
#35937=VERTEX_POINT('',#138708);
#35938=VERTEX_POINT('',#138744);
#35939=VERTEX_POINT('',#138749);
#35940=VERTEX_POINT('',#138763);
#35941=VERTEX_POINT('',#138765);
#35942=VERTEX_POINT('',#138779);
#35943=VERTEX_POINT('',#138784);
#35944=VERTEX_POINT('',#138788);
#35945=VERTEX_POINT('',#138789);
#35946=VERTEX_POINT('',#138816);
#35947=VERTEX_POINT('',#138820);
#35948=VERTEX_POINT('',#138849);
#35949=VERTEX_POINT('',#138851);
#35950=VERTEX_POINT('',#138877);
#35951=VERTEX_POINT('',#138879);
#35952=VERTEX_POINT('',#138881);
#35953=VERTEX_POINT('',#138886);
#35954=VERTEX_POINT('',#138888);
#35955=VERTEX_POINT('',#138890);
#35956=VERTEX_POINT('',#138926);
#35957=VERTEX_POINT('',#138950);
#35958=VERTEX_POINT('',#138992);
#35959=VERTEX_POINT('',#139034);
#35960=VERTEX_POINT('',#139038);
#35961=VERTEX_POINT('',#139043);
#35962=VERTEX_POINT('',#139045);
#35963=VERTEX_POINT('',#139047);
#35964=VERTEX_POINT('',#139049);
#35965=VERTEX_POINT('',#139054);
#35966=VERTEX_POINT('',#139056);
#35967=VERTEX_POINT('',#139058);
#35968=VERTEX_POINT('',#139086);
#35969=VERTEX_POINT('',#139087);
#35970=VERTEX_POINT('',#139116);
#35971=VERTEX_POINT('',#139120);
#35972=VERTEX_POINT('',#139158);
#35973=VERTEX_POINT('',#139160);
#35974=VERTEX_POINT('',#139198);
#35975=VERTEX_POINT('',#139200);
#35976=VERTEX_POINT('',#139202);
#35977=VERTEX_POINT('',#139207);
#35978=VERTEX_POINT('',#139221);
#35979=VERTEX_POINT('',#139223);
#35980=VERTEX_POINT('',#139283);
#35981=VERTEX_POINT('',#139311);
#35982=VERTEX_POINT('',#139372);
#35983=VERTEX_POINT('',#139423);
#35984=VERTEX_POINT('',#139427);
#35985=VERTEX_POINT('',#139432);
#35986=VERTEX_POINT('',#139446);
#35987=VERTEX_POINT('',#139448);
#35988=VERTEX_POINT('',#139462);
#35989=VERTEX_POINT('',#139467);
#35990=VERTEX_POINT('',#139469);
#35991=VERTEX_POINT('',#139471);
#35992=VERTEX_POINT('',#139514);
#35993=VERTEX_POINT('',#139515);
#35994=VERTEX_POINT('',#139546);
#35995=VERTEX_POINT('',#139550);
#35996=VERTEX_POINT('',#139552);
#35997=VERTEX_POINT('',#139554);
#35998=VERTEX_POINT('',#139556);
#35999=VERTEX_POINT('',#139558);
#36000=VERTEX_POINT('',#139560);
#36001=VERTEX_POINT('',#139562);
#36002=VERTEX_POINT('',#139570);
#36003=VERTEX_POINT('',#139587);
#36004=VERTEX_POINT('',#139589);
#36005=VERTEX_POINT('',#139611);
#36006=VERTEX_POINT('',#139615);
#36007=VERTEX_POINT('',#139619);
#36008=VERTEX_POINT('',#139634);
#36009=VERTEX_POINT('',#139638);
#36010=VERTEX_POINT('',#139646);
#36011=VERTEX_POINT('',#139655);
#36012=VERTEX_POINT('',#139657);
#36013=VERTEX_POINT('',#139674);
#36014=VERTEX_POINT('',#139682);
#36015=VERTEX_POINT('',#139684);
#36016=VERTEX_POINT('',#139686);
#36017=VERTEX_POINT('',#139688);
#36018=VERTEX_POINT('',#139690);
#36019=VERTEX_POINT('',#139694);
#36020=VERTEX_POINT('',#139695);
#36021=VERTEX_POINT('',#139727);
#36022=VERTEX_POINT('',#139731);
#36023=VERTEX_POINT('',#139732);
#36024=VERTEX_POINT('',#139734);
#36025=VERTEX_POINT('',#139742);
#36026=VERTEX_POINT('',#139768);
#36027=VERTEX_POINT('',#139770);
#36028=VERTEX_POINT('',#139800);
#36029=VERTEX_POINT('',#139802);
#36030=VERTEX_POINT('',#139804);
#36031=VERTEX_POINT('',#139806);
#36032=VERTEX_POINT('',#139810);
#36033=VERTEX_POINT('',#139811);
#36034=VERTEX_POINT('',#139816);
#36035=VERTEX_POINT('',#139850);
#36036=VERTEX_POINT('',#139892);
#36037=VERTEX_POINT('',#139905);
#36038=VERTEX_POINT('',#139906);
#36039=VERTEX_POINT('',#139917);
#36040=VERTEX_POINT('',#139919);
#36041=VERTEX_POINT('',#139924);
#36042=VERTEX_POINT('',#139950);
#36043=VERTEX_POINT('',#139967);
#36044=VERTEX_POINT('',#139969);
#36045=VERTEX_POINT('',#139983);
#36046=VERTEX_POINT('',#140004);
#36047=VERTEX_POINT('',#140006);
#36048=VERTEX_POINT('',#140008);
#36049=VERTEX_POINT('',#140010);
#36050=VERTEX_POINT('',#140012);
#36051=VERTEX_POINT('',#140016);
#36052=VERTEX_POINT('',#140020);
#36053=VERTEX_POINT('',#140024);
#36054=VERTEX_POINT('',#140028);
#36055=VERTEX_POINT('',#140029);
#36056=VERTEX_POINT('',#140061);
#36057=VERTEX_POINT('',#140063);
#36058=VERTEX_POINT('',#140074);
#36059=VERTEX_POINT('',#140076);
#36060=VERTEX_POINT('',#140078);
#36061=VERTEX_POINT('',#140080);
#36062=VERTEX_POINT('',#140083);
#36063=VERTEX_POINT('',#140094);
#36064=VERTEX_POINT('',#140096);
#36065=VERTEX_POINT('',#140134);
#36066=VERTEX_POINT('',#140136);
#36067=VERTEX_POINT('',#140188);
#36068=VERTEX_POINT('',#140222);
#36069=VERTEX_POINT('',#140223);
#36070=VERTEX_POINT('',#140225);
#36071=VERTEX_POINT('',#140227);
#36072=VERTEX_POINT('',#140230);
#36073=VERTEX_POINT('',#140232);
#36074=VERTEX_POINT('',#140237);
#36075=VERTEX_POINT('',#140251);
#36076=VERTEX_POINT('',#140253);
#36077=VERTEX_POINT('',#140276);
#36078=VERTEX_POINT('',#140281);
#36079=VERTEX_POINT('',#140286);
#36080=VERTEX_POINT('',#140302);
#36081=VERTEX_POINT('',#140303);
#36082=VERTEX_POINT('',#140306);
#36083=VERTEX_POINT('',#140348);
#36084=VERTEX_POINT('',#140361);
#36085=VERTEX_POINT('',#140363);
#36086=VERTEX_POINT('',#140365);
#36087=VERTEX_POINT('',#140367);
#36088=VERTEX_POINT('',#140369);
#36089=VERTEX_POINT('',#140371);
#36090=VERTEX_POINT('',#140373);
#36091=VERTEX_POINT('',#140384);
#36092=VERTEX_POINT('',#140386);
#36093=VERTEX_POINT('',#140406);
#36094=VERTEX_POINT('',#140411);
#36095=VERTEX_POINT('',#140428);
#36096=VERTEX_POINT('',#140430);
#36097=VERTEX_POINT('',#140444);
#36098=VERTEX_POINT('',#140449);
#36099=VERTEX_POINT('',#140465);
#36100=VERTEX_POINT('',#140469);
#36101=VERTEX_POINT('',#140473);
#36102=VERTEX_POINT('',#140477);
#36103=VERTEX_POINT('',#140478);
#36104=VERTEX_POINT('',#140480);
#36105=VERTEX_POINT('',#140482);
#36106=VERTEX_POINT('',#140485);
#36107=VERTEX_POINT('',#140487);
#36108=VERTEX_POINT('',#140510);
#36109=VERTEX_POINT('',#140515);
#36110=VERTEX_POINT('',#140541);
#36111=VERTEX_POINT('',#140543);
#36112=VERTEX_POINT('',#140560);
#36113=VERTEX_POINT('',#140565);
#36114=VERTEX_POINT('',#140582);
#36115=VERTEX_POINT('',#140584);
#36116=VERTEX_POINT('',#140597);
#36117=VERTEX_POINT('',#140598);
#36118=VERTEX_POINT('',#140632);
#36119=VERTEX_POINT('',#140674);
#36120=VERTEX_POINT('',#140687);
#36121=VERTEX_POINT('',#140689);
#36122=VERTEX_POINT('',#140692);
#36123=VERTEX_POINT('',#140694);
#36124=VERTEX_POINT('',#140696);
#36125=VERTEX_POINT('',#140710);
#36126=VERTEX_POINT('',#140715);
#36127=VERTEX_POINT('',#140737);
#36128=VERTEX_POINT('',#140741);
#36129=VERTEX_POINT('',#140745);
#36130=VERTEX_POINT('',#140749);
#36131=VERTEX_POINT('',#140790);
#36132=VERTEX_POINT('',#140810);
#36133=VERTEX_POINT('',#140815);
#36134=VERTEX_POINT('',#140829);
#36135=VERTEX_POINT('',#140832);
#36136=VERTEX_POINT('',#140902);
#36137=VERTEX_POINT('',#140918);
#36138=VERTEX_POINT('',#140919);
#36139=VERTEX_POINT('',#140922);
#36140=VERTEX_POINT('',#140924);
#36141=VERTEX_POINT('',#140926);
#36142=VERTEX_POINT('',#140930);
#36143=VERTEX_POINT('',#140934);
#36144=VERTEX_POINT('',#140938);
#36145=VERTEX_POINT('',#140942);
#36146=VERTEX_POINT('',#140945);
#36147=VERTEX_POINT('',#140947);
#36148=VERTEX_POINT('',#140967);
#36149=VERTEX_POINT('',#140972);
#36150=VERTEX_POINT('',#140989);
#36151=VERTEX_POINT('',#140993);
#36152=VERTEX_POINT('',#140994);
#36153=VERTEX_POINT('',#141028);
#36154=VERTEX_POINT('',#141070);
#36155=VERTEX_POINT('',#141083);
#36156=VERTEX_POINT('',#141084);
#36157=VERTEX_POINT('',#141095);
#36158=VERTEX_POINT('',#141097);
#36159=VERTEX_POINT('',#141117);
#36160=VERTEX_POINT('',#141122);
#36161=VERTEX_POINT('',#141142);
#36162=VERTEX_POINT('',#141144);
#36163=VERTEX_POINT('',#141161);
#36164=VERTEX_POINT('',#141166);
#36165=VERTEX_POINT('',#141181);
#36166=VERTEX_POINT('',#141183);
#36167=VERTEX_POINT('',#141185);
#36168=VERTEX_POINT('',#141187);
#36169=VERTEX_POINT('',#141189);
#36170=VERTEX_POINT('',#141193);
#36171=VERTEX_POINT('',#141197);
#36172=VERTEX_POINT('',#141201);
#36173=VERTEX_POINT('',#141234);
#36174=VERTEX_POINT('',#141247);
#36175=VERTEX_POINT('',#141248);
#36176=VERTEX_POINT('',#141250);
#36177=VERTEX_POINT('',#141252);
#36178=VERTEX_POINT('',#141272);
#36179=VERTEX_POINT('',#141274);
#36180=VERTEX_POINT('',#141285);
#36181=VERTEX_POINT('',#141287);
#36182=VERTEX_POINT('',#141289);
#36183=VERTEX_POINT('',#141291);
#36184=VERTEX_POINT('',#141294);
#36185=VERTEX_POINT('',#141296);
#36186=VERTEX_POINT('',#141316);
#36187=VERTEX_POINT('',#141318);
#36188=VERTEX_POINT('',#141322);
#36189=VERTEX_POINT('',#141323);
#36190=VERTEX_POINT('',#141325);
#36191=VERTEX_POINT('',#141327);
#36192=VERTEX_POINT('',#141330);
#36193=VERTEX_POINT('',#141332);
#36194=VERTEX_POINT('',#141334);
#36195=VERTEX_POINT('',#141336);
#36196=VERTEX_POINT('',#141344);
#36197=VERTEX_POINT('',#141361);
#36198=VERTEX_POINT('',#141363);
#36199=VERTEX_POINT('',#141389);
#36200=VERTEX_POINT('',#141397);
#36201=VERTEX_POINT('',#141402);
#36202=VERTEX_POINT('',#141442);
#36203=VERTEX_POINT('',#141452);
#36204=VERTEX_POINT('',#141453);
#36205=VERTEX_POINT('',#141456);
#36206=VERTEX_POINT('',#141498);
#36207=VERTEX_POINT('',#141511);
#36208=VERTEX_POINT('',#141513);
#36209=VERTEX_POINT('',#141515);
#36210=VERTEX_POINT('',#141517);
#36211=VERTEX_POINT('',#141519);
#36212=VERTEX_POINT('',#141521);
#36213=VERTEX_POINT('',#141523);
#36214=VERTEX_POINT('',#141534);
#36215=VERTEX_POINT('',#141536);
#36216=VERTEX_POINT('',#141556);
#36217=VERTEX_POINT('',#141561);
#36218=VERTEX_POINT('',#141578);
#36219=VERTEX_POINT('',#141580);
#36220=VERTEX_POINT('',#141597);
#36221=VERTEX_POINT('',#141602);
#36222=VERTEX_POINT('',#141618);
#36223=VERTEX_POINT('',#141622);
#36224=VERTEX_POINT('',#141626);
#36225=VERTEX_POINT('',#141630);
#36226=VERTEX_POINT('',#141631);
#36227=VERTEX_POINT('',#141633);
#36228=VERTEX_POINT('',#141635);
#36229=VERTEX_POINT('',#141638);
#36230=VERTEX_POINT('',#141640);
#36231=VERTEX_POINT('',#141663);
#36232=VERTEX_POINT('',#141668);
#36233=VERTEX_POINT('',#141688);
#36234=VERTEX_POINT('',#141690);
#36235=VERTEX_POINT('',#141707);
#36236=VERTEX_POINT('',#141712);
#36237=VERTEX_POINT('',#141729);
#36238=VERTEX_POINT('',#141731);
#36239=VERTEX_POINT('',#141744);
#36240=VERTEX_POINT('',#141745);
#36241=VERTEX_POINT('',#141747);
#36242=VERTEX_POINT('',#141778);
#36243=VERTEX_POINT('',#141812);
#36244=VERTEX_POINT('',#141813);
#36245=VERTEX_POINT('',#141827);
#36246=VERTEX_POINT('',#141832);
#36247=VERTEX_POINT('',#141840);
#36248=VERTEX_POINT('',#141857);
#36249=VERTEX_POINT('',#141859);
#36250=VERTEX_POINT('',#141885);
#36251=VERTEX_POINT('',#141894);
#36252=VERTEX_POINT('',#141896);
#36253=VERTEX_POINT('',#141898);
#36254=VERTEX_POINT('',#141900);
#36255=VERTEX_POINT('',#141933);
#36256=VERTEX_POINT('',#141946);
#36257=VERTEX_POINT('',#141947);
#36258=VERTEX_POINT('',#141958);
#36259=VERTEX_POINT('',#141960);
#36260=VERTEX_POINT('',#141992);
#36261=VERTEX_POINT('',#141994);
#36262=VERTEX_POINT('',#141996);
#36263=VERTEX_POINT('',#141998);
#36264=VERTEX_POINT('',#142028);
#36265=VERTEX_POINT('',#142030);
#36266=VERTEX_POINT('',#142032);
#36267=VERTEX_POINT('',#142034);
#36268=VERTEX_POINT('',#142036);
#36269=VERTEX_POINT('',#142040);
#36270=VERTEX_POINT('',#142044);
#36271=VERTEX_POINT('',#142048);
#36272=VERTEX_POINT('',#142052);
#36273=VERTEX_POINT('',#142053);
#36274=VERTEX_POINT('',#142055);
#36275=VERTEX_POINT('',#142057);
#36276=VERTEX_POINT('',#142060);
#36277=VERTEX_POINT('',#142071);
#36278=VERTEX_POINT('',#142073);
#36279=VERTEX_POINT('',#142093);
#36280=VERTEX_POINT('',#142098);
#36281=VERTEX_POINT('',#142118);
#36282=VERTEX_POINT('',#142120);
#36283=VERTEX_POINT('',#142137);
#36284=VERTEX_POINT('',#142142);
#36285=VERTEX_POINT('',#142156);
#36286=VERTEX_POINT('',#142158);
#36287=VERTEX_POINT('',#142202);
#36288=VERTEX_POINT('',#142203);
#36289=VERTEX_POINT('',#142237);
#36290=VERTEX_POINT('',#142253);
#36291=VERTEX_POINT('',#142255);
#36292=VERTEX_POINT('',#142257);
#36293=VERTEX_POINT('',#142259);
#36294=VERTEX_POINT('',#142261);
#36295=VERTEX_POINT('',#142263);
#36296=VERTEX_POINT('',#142265);
#36297=VERTEX_POINT('',#142276);
#36298=VERTEX_POINT('',#142278);
#36299=VERTEX_POINT('',#142301);
#36300=VERTEX_POINT('',#142306);
#36301=VERTEX_POINT('',#142326);
#36302=VERTEX_POINT('',#142328);
#36303=VERTEX_POINT('',#142345);
#36304=VERTEX_POINT('',#142350);
#36305=VERTEX_POINT('',#142369);
#36306=VERTEX_POINT('',#142373);
#36307=VERTEX_POINT('',#142377);
#36308=VERTEX_POINT('',#142410);
#36309=VERTEX_POINT('',#142423);
#36310=VERTEX_POINT('',#142424);
#36311=VERTEX_POINT('',#142426);
#36312=VERTEX_POINT('',#142428);
#36313=VERTEX_POINT('',#142431);
#36314=VERTEX_POINT('',#142433);
#36315=VERTEX_POINT('',#142453);
#36316=VERTEX_POINT('',#142458);
#36317=VERTEX_POINT('',#142487);
#36318=VERTEX_POINT('',#142489);
#36319=VERTEX_POINT('',#142506);
#36320=VERTEX_POINT('',#142511);
#36321=VERTEX_POINT('',#142525);
#36322=VERTEX_POINT('',#142527);
#36323=VERTEX_POINT('',#142544);
#36324=VERTEX_POINT('',#142546);
#36325=VERTEX_POINT('',#142550);
#36326=VERTEX_POINT('',#142553);
#36327=VERTEX_POINT('',#142583);
#36328=VERTEX_POINT('',#142587);
#36329=VERTEX_POINT('',#142605);
#36330=VERTEX_POINT('',#142607);
#36331=VERTEX_POINT('',#142611);
#36332=VERTEX_POINT('',#142615);
#36333=VERTEX_POINT('',#142642);
#36334=VERTEX_POINT('',#142665);
#36335=VERTEX_POINT('',#142667);
#36336=VERTEX_POINT('',#142673);
#36337=VERTEX_POINT('',#142677);
#36338=VERTEX_POINT('',#142739);
#36339=VERTEX_POINT('',#142764);
#36340=VERTEX_POINT('',#142940);
#36341=VERTEX_POINT('',#142984);
#36342=VERTEX_POINT('',#142988);
#36343=VERTEX_POINT('',#143004);
#36344=VERTEX_POINT('',#143006);
#36345=VERTEX_POINT('',#143035);
#36346=VERTEX_POINT('',#143039);
#36347=VERTEX_POINT('',#143055);
#36348=VERTEX_POINT('',#143057);
#36349=VERTEX_POINT('',#143085);
#36350=VERTEX_POINT('',#143121);
#36351=VERTEX_POINT('',#143154);
#36352=VERTEX_POINT('',#143167);
#36353=VERTEX_POINT('',#143214);
#36354=VERTEX_POINT('',#143218);
#36355=VERTEX_POINT('',#143222);
#36356=VERTEX_POINT('',#143226);
#36357=VERTEX_POINT('',#143230);
#36358=VERTEX_POINT('',#143232);
#36359=VERTEX_POINT('',#143234);
#36360=VERTEX_POINT('',#143248);
#36361=VERTEX_POINT('',#143250);
#36362=VERTEX_POINT('',#143252);
#36363=VERTEX_POINT('',#143260);
#36364=VERTEX_POINT('',#143262);
#36365=VERTEX_POINT('',#143270);
#36366=VERTEX_POINT('',#143272);
#36367=VERTEX_POINT('',#143274);
#36368=VERTEX_POINT('',#143276);
#36369=VERTEX_POINT('',#143284);
#36370=VERTEX_POINT('',#143286);
#36371=VERTEX_POINT('',#143296);
#36372=VERTEX_POINT('',#143297);
#36373=VERTEX_POINT('',#143303);
#36374=VERTEX_POINT('',#143312);
#36375=VERTEX_POINT('',#143314);
#36376=VERTEX_POINT('',#143316);
#36377=VERTEX_POINT('',#143318);
#36378=VERTEX_POINT('',#143365);
#36379=VERTEX_POINT('',#143367);
#36380=VERTEX_POINT('',#143369);
#36381=VERTEX_POINT('',#143371);
#36382=VERTEX_POINT('',#143380);
#36383=VERTEX_POINT('',#143382);
#36384=VERTEX_POINT('',#143389);
#36385=VERTEX_POINT('',#143391);
#36386=VERTEX_POINT('',#143393);
#36387=VERTEX_POINT('',#143395);
#36388=VERTEX_POINT('',#143397);
#36389=VERTEX_POINT('',#143441);
#36390=VERTEX_POINT('',#143443);
#36391=VERTEX_POINT('',#143452);
#36392=VERTEX_POINT('',#143454);
#36393=VERTEX_POINT('',#143456);
#36394=VERTEX_POINT('',#143458);
#36395=VERTEX_POINT('',#143467);
#36396=VERTEX_POINT('',#143469);
#36397=VERTEX_POINT('',#143510);
#36398=VERTEX_POINT('',#143512);
#36399=VERTEX_POINT('',#143514);
#36400=VERTEX_POINT('',#143516);
#36401=VERTEX_POINT('',#143566);
#36402=VERTEX_POINT('',#143568);
#36403=VERTEX_POINT('',#143575);
#36404=VERTEX_POINT('',#143577);
#36405=VERTEX_POINT('',#143579);
#36406=VERTEX_POINT('',#143581);
#36407=VERTEX_POINT('',#143586);
#36408=VERTEX_POINT('',#143591);
#36409=VERTEX_POINT('',#143593);
#36410=VERTEX_POINT('',#143640);
#36411=VERTEX_POINT('',#143642);
#36412=VERTEX_POINT('',#143644);
#36413=VERTEX_POINT('',#143646);
#36414=VERTEX_POINT('',#143690);
#36415=VERTEX_POINT('',#143697);
#36416=VERTEX_POINT('',#143699);
#36417=VERTEX_POINT('',#143704);
#36418=VERTEX_POINT('',#143713);
#36419=VERTEX_POINT('',#143714);
#36420=VERTEX_POINT('',#143716);
#36421=VERTEX_POINT('',#143718);
#36422=VERTEX_POINT('',#143726);
#36423=VERTEX_POINT('',#143728);
#36424=VERTEX_POINT('',#143736);
#36425=VERTEX_POINT('',#143738);
#36426=VERTEX_POINT('',#143753);
#36427=VERTEX_POINT('',#143755);
#36428=VERTEX_POINT('',#143757);
#36429=VERTEX_POINT('',#143759);
#36430=VERTEX_POINT('',#143767);
#36431=VERTEX_POINT('',#143769);
#36432=VERTEX_POINT('',#143779);
#36433=VERTEX_POINT('',#143783);
#36434=VERTEX_POINT('',#143787);
#36435=VERTEX_POINT('',#143791);
#36436=VERTEX_POINT('',#143793);
#36437=VERTEX_POINT('',#143807);
#36438=VERTEX_POINT('',#143809);
#36439=VERTEX_POINT('',#143811);
#36440=VERTEX_POINT('',#143819);
#36441=VERTEX_POINT('',#143821);
#36442=VERTEX_POINT('',#143829);
#36443=VERTEX_POINT('',#143831);
#36444=VERTEX_POINT('',#143833);
#36445=VERTEX_POINT('',#143835);
#36446=VERTEX_POINT('',#143843);
#36447=VERTEX_POINT('',#143845);
#36448=VERTEX_POINT('',#143887);
#36449=VERTEX_POINT('',#143888);
#36450=VERTEX_POINT('',#143890);
#36451=VERTEX_POINT('',#143892);
#36452=VERTEX_POINT('',#143894);
#36453=VERTEX_POINT('',#143896);
#36454=VERTEX_POINT('',#143933);
#36455=VERTEX_POINT('',#143935);
#36456=VERTEX_POINT('',#143971);
#36457=VERTEX_POINT('',#143973);
#36458=VERTEX_POINT('',#143975);
#36459=VERTEX_POINT('',#143977);
#36460=VERTEX_POINT('',#143979);
#36461=VERTEX_POINT('',#143985);
#36462=VERTEX_POINT('',#144002);
#36463=VERTEX_POINT('',#144007);
#36464=VERTEX_POINT('',#144033);
#36465=VERTEX_POINT('',#144037);
#36466=VERTEX_POINT('',#144056);
#36467=VERTEX_POINT('',#144061);
#36468=VERTEX_POINT('',#144127);
#36469=VERTEX_POINT('',#144155);
#36470=VERTEX_POINT('',#144231);
#36471=VERTEX_POINT('',#144244);
#36472=VERTEX_POINT('',#144309);
#36473=VERTEX_POINT('',#144310);
#36474=VERTEX_POINT('',#144323);
#36475=VERTEX_POINT('',#144366);
#36476=VERTEX_POINT('',#144370);
#36477=VERTEX_POINT('',#144404);
#36478=VERTEX_POINT('',#144470);
#36479=VERTEX_POINT('',#144578);
#36480=VERTEX_POINT('',#144606);
#36481=VERTEX_POINT('',#144651);
#36482=VERTEX_POINT('',#144707);
#36483=VERTEX_POINT('',#144770);
#36484=VERTEX_POINT('',#144774);
#36485=VERTEX_POINT('',#144780);
#36486=VERTEX_POINT('',#144829);
#36487=VERTEX_POINT('',#144860);
#36488=VERTEX_POINT('',#144888);
#36489=VERTEX_POINT('',#144911);
#36490=VERTEX_POINT('',#144967);
#36491=VERTEX_POINT('',#145033);
#36492=VERTEX_POINT('',#145041);
#36493=VERTEX_POINT('',#145042);
#36494=VERTEX_POINT('',#145248);
#36495=VERTEX_POINT('',#145252);
#36496=VERTEX_POINT('',#145258);
#36497=VERTEX_POINT('',#145262);
#36498=VERTEX_POINT('',#145268);
#36499=VERTEX_POINT('',#145269);
#36500=VERTEX_POINT('',#145297);
#36501=VERTEX_POINT('',#145318);
#36502=VERTEX_POINT('',#145344);
#36503=VERTEX_POINT('',#145353);
#36504=VERTEX_POINT('',#145425);
#36505=VERTEX_POINT('',#145448);
#36506=VERTEX_POINT('',#145538);
#36507=VERTEX_POINT('',#145559);
#36508=VERTEX_POINT('',#145585);
#36509=VERTEX_POINT('',#145610);
#36510=VERTEX_POINT('',#145612);
#36511=VERTEX_POINT('',#145623);
#36512=VERTEX_POINT('',#145627);
#36513=VERTEX_POINT('',#145633);
#36514=VERTEX_POINT('',#145658);
#36515=VERTEX_POINT('',#145662);
#36516=VERTEX_POINT('',#145663);
#36517=VERTEX_POINT('',#145685);
#36518=VERTEX_POINT('',#145706);
#36519=VERTEX_POINT('',#145732);
#36520=VERTEX_POINT('',#145741);
#36521=VERTEX_POINT('',#145814);
#36522=VERTEX_POINT('',#145892);
#36523=VERTEX_POINT('',#145913);
#36524=VERTEX_POINT('',#145933);
#36525=VERTEX_POINT('',#145997);
#36526=VERTEX_POINT('',#145999);
#36527=VERTEX_POINT('',#146027);
#36528=VERTEX_POINT('',#146090);
#36529=VERTEX_POINT('',#146163);
#36530=VERTEX_POINT('',#146178);
#36531=VERTEX_POINT('',#146202);
#36532=VERTEX_POINT('',#146212);
#36533=VERTEX_POINT('',#146276);
#36534=VERTEX_POINT('',#146327);
#36535=VERTEX_POINT('',#146342);
#36536=VERTEX_POINT('',#146357);
#36537=VERTEX_POINT('',#146409);
#36538=VERTEX_POINT('',#146411);
#36539=VERTEX_POINT('',#146471);
#36540=VERTEX_POINT('',#146519);
#36541=VERTEX_POINT('',#146557);
#36542=VERTEX_POINT('',#146572);
#36543=VERTEX_POINT('',#146590);
#36544=VERTEX_POINT('',#146594);
#36545=VERTEX_POINT('',#146634);
#36546=VERTEX_POINT('',#146700);
#36547=VERTEX_POINT('',#146721);
#36548=VERTEX_POINT('',#146760);
#36549=VERTEX_POINT('',#146824);
#36550=VERTEX_POINT('',#146826);
#36551=VERTEX_POINT('',#146887);
#36552=VERTEX_POINT('',#146950);
#36553=VERTEX_POINT('',#146986);
#36554=VERTEX_POINT('',#147001);
#36555=VERTEX_POINT('',#147025);
#36556=VERTEX_POINT('',#147053);
#36557=VERTEX_POINT('',#147104);
#36558=VERTEX_POINT('',#147169);
#36559=VERTEX_POINT('',#147190);
#36560=VERTEX_POINT('',#147238);
#36561=VERTEX_POINT('',#147263);
#36562=VERTEX_POINT('',#147265);
#36563=VERTEX_POINT('',#147267);
#36564=VERTEX_POINT('',#147274);
#36565=VERTEX_POINT('',#147280);
#36566=VERTEX_POINT('',#147305);
#36567=VERTEX_POINT('',#147309);
#36568=VERTEX_POINT('',#147313);
#36569=VERTEX_POINT('',#147367);
#36570=VERTEX_POINT('',#147388);
#36571=VERTEX_POINT('',#147414);
#36572=VERTEX_POINT('',#147445);
#36573=VERTEX_POINT('',#147491);
#36574=VERTEX_POINT('',#147548);
#36575=VERTEX_POINT('',#147555);
#36576=VERTEX_POINT('',#147557);
#36577=VERTEX_POINT('',#147570);
#36578=VERTEX_POINT('',#147595);
#36579=VERTEX_POINT('',#147616);
#36580=VERTEX_POINT('',#147685);
#36581=VERTEX_POINT('',#147686);
#36582=VERTEX_POINT('',#147707);
#36583=VERTEX_POINT('',#147745);
#36584=VERTEX_POINT('',#147747);
#36585=VERTEX_POINT('',#147763);
#36586=VERTEX_POINT('',#147765);
#36587=VERTEX_POINT('',#147774);
#36588=VERTEX_POINT('',#147778);
#36589=VERTEX_POINT('',#147838);
#36590=VERTEX_POINT('',#147851);
#36591=VERTEX_POINT('',#147884);
#36592=VERTEX_POINT('',#147947);
#36593=VERTEX_POINT('',#147967);
#36594=VERTEX_POINT('',#147973);
#36595=VERTEX_POINT('',#147985);
#36596=VERTEX_POINT('',#148019);
#36597=VERTEX_POINT('',#148023);
#36598=VERTEX_POINT('',#148027);
#36599=VERTEX_POINT('',#148124);
#36600=VERTEX_POINT('',#148139);
#36601=VERTEX_POINT('',#148163);
#36602=VERTEX_POINT('',#148197);
#36603=VERTEX_POINT('',#148224);
#36604=VERTEX_POINT('',#148251);
#36605=VERTEX_POINT('',#148257);
#36606=VERTEX_POINT('',#148330);
#36607=VERTEX_POINT('',#148343);
#36608=VERTEX_POINT('',#148376);
#36609=VERTEX_POINT('',#148430);
#36610=VERTEX_POINT('',#148466);
#36611=VERTEX_POINT('',#148479);
#36612=VERTEX_POINT('',#148526);
#36613=VERTEX_POINT('',#148528);
#36614=VERTEX_POINT('',#148537);
#36615=VERTEX_POINT('',#148541);
#36616=VERTEX_POINT('',#148547);
#36617=VERTEX_POINT('',#148553);
#36618=VERTEX_POINT('',#148554);
#36619=VERTEX_POINT('',#148596);
#36620=VERTEX_POINT('',#148609);
#36621=VERTEX_POINT('',#148630);
#36622=VERTEX_POINT('',#148650);
#36623=VERTEX_POINT('',#148680);
#36624=VERTEX_POINT('',#148723);
#36625=VERTEX_POINT('',#148750);
#36626=VERTEX_POINT('',#148796);
#36627=VERTEX_POINT('',#148802);
#36628=VERTEX_POINT('',#148803);
#36629=VERTEX_POINT('',#148854);
#36630=VERTEX_POINT('',#149051);
#36631=VERTEX_POINT('',#149103);
#36632=VERTEX_POINT('',#149104);
#36633=VERTEX_POINT('',#149156);
#36634=VERTEX_POINT('',#149158);
#36635=VERTEX_POINT('',#149174);
#36636=VERTEX_POINT('',#149176);
#36637=VERTEX_POINT('',#149185);
#36638=VERTEX_POINT('',#149189);
#36639=VERTEX_POINT('',#149237);
#36640=VERTEX_POINT('',#149273);
#36641=VERTEX_POINT('',#149325);
#36642=VERTEX_POINT('',#149364);
#36643=VERTEX_POINT('',#149427);
#36644=VERTEX_POINT('',#149457);
#36645=VERTEX_POINT('',#149470);
#36646=VERTEX_POINT('',#149508);
#36647=VERTEX_POINT('',#149512);
#36648=VERTEX_POINT('',#149516);
#36649=VERTEX_POINT('',#149572);
#36650=VERTEX_POINT('',#149573);
#36651=VERTEX_POINT('',#149584);
#36652=VERTEX_POINT('',#149614);
#36653=VERTEX_POINT('',#149653);
#36654=VERTEX_POINT('',#149674);
#36655=VERTEX_POINT('',#149700);
#36656=VERTEX_POINT('',#149740);
#36657=VERTEX_POINT('',#149767);
#36658=VERTEX_POINT('',#149830);
#36659=VERTEX_POINT('',#149836);
#36660=VERTEX_POINT('',#149912);
#36661=VERTEX_POINT('',#149925);
#36662=VERTEX_POINT('',#149958);
#36663=VERTEX_POINT('',#149982);
#36664=VERTEX_POINT('',#150018);
#36665=VERTEX_POINT('',#150031);
#36666=VERTEX_POINT('',#150078);
#36667=VERTEX_POINT('',#150080);
#36668=VERTEX_POINT('',#150089);
#36669=VERTEX_POINT('',#150093);
#36670=VERTEX_POINT('',#150099);
#36671=VERTEX_POINT('',#150105);
#36672=VERTEX_POINT('',#150106);
#36673=VERTEX_POINT('',#150148);
#36674=VERTEX_POINT('',#150161);
#36675=VERTEX_POINT('',#150182);
#36676=VERTEX_POINT('',#150202);
#36677=VERTEX_POINT('',#150232);
#36678=VERTEX_POINT('',#150275);
#36679=VERTEX_POINT('',#150302);
#36680=VERTEX_POINT('',#150386);
#36681=VERTEX_POINT('',#150392);
#36682=VERTEX_POINT('',#150393);
#36683=VERTEX_POINT('',#150474);
#36684=VERTEX_POINT('',#150486);
#36685=VERTEX_POINT('',#150493);
#36686=VERTEX_POINT('',#150495);
#36687=VERTEX_POINT('',#150499);
#36688=VERTEX_POINT('',#150541);
#36689=VERTEX_POINT('',#150581);
#36690=VERTEX_POINT('',#150608);
#36691=VERTEX_POINT('',#150638);
#36692=VERTEX_POINT('',#150704);
#36693=VERTEX_POINT('',#150706);
#36694=VERTEX_POINT('',#150715);
#36695=VERTEX_POINT('',#150719);
#36696=VERTEX_POINT('',#150756);
#36697=VERTEX_POINT('',#150763);
#36698=VERTEX_POINT('',#150769);
#36699=VERTEX_POINT('',#150770);
#36700=VERTEX_POINT('',#150780);
#36701=VERTEX_POINT('',#150814);
#36702=VERTEX_POINT('',#150827);
#36703=VERTEX_POINT('',#150860);
#36704=VERTEX_POINT('',#150884);
#36705=VERTEX_POINT('',#150920);
#36706=VERTEX_POINT('',#150972);
#36707=VERTEX_POINT('',#151011);
#36708=VERTEX_POINT('',#151074);
#36709=VERTEX_POINT('',#151115);
#36710=VERTEX_POINT('',#151121);
#36711=VERTEX_POINT('',#151162);
#36712=VERTEX_POINT('',#151192);
#36713=VERTEX_POINT('',#151238);
#36714=VERTEX_POINT('',#151265);
#36715=VERTEX_POINT('',#151325);
#36716=VERTEX_POINT('',#151349);
#36717=VERTEX_POINT('',#151358);
#36718=VERTEX_POINT('',#151405);
#36719=VERTEX_POINT('',#151407);
#36720=VERTEX_POINT('',#151416);
#36721=VERTEX_POINT('',#151420);
#36722=VERTEX_POINT('',#151426);
#36723=VERTEX_POINT('',#151433);
#36724=VERTEX_POINT('',#151434);
#36725=VERTEX_POINT('',#151444);
#36726=VERTEX_POINT('',#151478);
#36727=VERTEX_POINT('',#151491);
#36728=VERTEX_POINT('',#151518);
#36729=VERTEX_POINT('',#151540);
#36730=VERTEX_POINT('',#151570);
#36731=VERTEX_POINT('',#151583);
#36732=VERTEX_POINT('',#151667);
#36733=VERTEX_POINT('',#151813);
#36734=VERTEX_POINT('',#151834);
#36735=VERTEX_POINT('',#151957);
#36736=VERTEX_POINT('',#152235);
#36737=VERTEX_POINT('',#152349);
#36738=VERTEX_POINT('',#152417);
#36739=VERTEX_POINT('',#152557);
#36740=VERTEX_POINT('',#153125);
#36741=VERTEX_POINT('',#153468);
#36742=VERTEX_POINT('',#153469);
#36743=VERTEX_POINT('',#153471);
#36744=VERTEX_POINT('',#153475);
#36745=VERTEX_POINT('',#153476);
#36746=VERTEX_POINT('',#153478);
#36747=VERTEX_POINT('',#153480);
#36748=VERTEX_POINT('',#153484);
#36749=VERTEX_POINT('',#153486);
#36750=VERTEX_POINT('',#153490);
#36751=VERTEX_POINT('',#153492);
#36752=VERTEX_POINT('',#153496);
#36753=VERTEX_POINT('',#153497);
#36754=VERTEX_POINT('',#153514);
#36755=VERTEX_POINT('',#153531);
#36756=VERTEX_POINT('',#153549);
#36757=VERTEX_POINT('',#153550);
#36758=VERTEX_POINT('',#153792);
#36759=VERTEX_POINT('',#153793);
#36760=VERTEX_POINT('',#153812);
#36761=VERTEX_POINT('',#153813);
#36762=VERTEX_POINT('',#154067);
#36763=VERTEX_POINT('',#154068);
#36764=VERTEX_POINT('',#154091);
#36765=VERTEX_POINT('',#154092);
#36766=VERTEX_POINT('',#154229);
#36767=VERTEX_POINT('',#154230);
#36768=VERTEX_POINT('',#154235);
#36769=VERTEX_POINT('',#154236);
#36770=VERTEX_POINT('',#154238);
#36771=VERTEX_POINT('',#154240);
#36772=VERTEX_POINT('',#154244);
#36773=VERTEX_POINT('',#154246);
#36774=VERTEX_POINT('',#154250);
#36775=VERTEX_POINT('',#154252);
#36776=VERTEX_POINT('',#154256);
#36777=VERTEX_POINT('',#154257);
#36778=VERTEX_POINT('',#154271);
#36779=VERTEX_POINT('',#154273);
#36780=VERTEX_POINT('',#154369);
#36781=VERTEX_POINT('',#154398);
#36782=VERTEX_POINT('',#154452);
#36783=VERTEX_POINT('',#154508);
#36784=VERTEX_POINT('',#154602);
#36785=VERTEX_POINT('',#154604);
#36786=VERTEX_POINT('',#154637);
#36787=VERTEX_POINT('',#154723);
#36788=VERTEX_POINT('',#154808);
#36789=VERTEX_POINT('',#154809);
#36790=VERTEX_POINT('',#154811);
#36791=VERTEX_POINT('',#154813);
#36792=VERTEX_POINT('',#154817);
#36793=VERTEX_POINT('',#154819);
#36794=VERTEX_POINT('',#154823);
#36795=VERTEX_POINT('',#154825);
#36796=VERTEX_POINT('',#154829);
#36797=VERTEX_POINT('',#154830);
#36798=VERTEX_POINT('',#154832);
#36799=VERTEX_POINT('',#154853);
#36800=VERTEX_POINT('',#154854);
#36801=VERTEX_POINT('',#154868);
#36802=VERTEX_POINT('',#154945);
#36803=VERTEX_POINT('',#154982);
#36804=VERTEX_POINT('',#154983);
#36805=VERTEX_POINT('',#155017);
#36806=VERTEX_POINT('',#155018);
#36807=VERTEX_POINT('',#155239);
#36808=VERTEX_POINT('',#155240);
#36809=VERTEX_POINT('',#155306);
#36810=VERTEX_POINT('',#155308);
#36811=VERTEX_POINT('',#155369);
#36812=VERTEX_POINT('',#155370);
#36813=VERTEX_POINT('',#155372);
#36814=VERTEX_POINT('',#155374);
#36815=VERTEX_POINT('',#155378);
#36816=VERTEX_POINT('',#155449);
#36817=VERTEX_POINT('',#155519);
#36818=VERTEX_POINT('',#155524);
#36819=VERTEX_POINT('',#155569);
#36820=VERTEX_POINT('',#155673);
#36821=VERTEX_POINT('',#155809);
#36822=VERTEX_POINT('',#155811);
#36823=VERTEX_POINT('',#155829);
#36824=VERTEX_POINT('',#155951);
#36825=VERTEX_POINT('',#156126);
#36826=VERTEX_POINT('',#156127);
#36827=VERTEX_POINT('',#156129);
#36828=VERTEX_POINT('',#156131);
#36829=VERTEX_POINT('',#156135);
#36830=VERTEX_POINT('',#156136);
#36831=VERTEX_POINT('',#156141);
#36832=VERTEX_POINT('',#156143);
#36833=VERTEX_POINT('',#156147);
#36834=VERTEX_POINT('',#156152);
#36835=VERTEX_POINT('',#156171);
#36836=VERTEX_POINT('',#156172);
#36837=VERTEX_POINT('',#156189);
#36838=VERTEX_POINT('',#156203);
#36839=VERTEX_POINT('',#156210);
#36840=VERTEX_POINT('',#156211);
#36841=VERTEX_POINT('',#156225);
#36842=VERTEX_POINT('',#156238);
#36843=VERTEX_POINT('',#156239);
#36844=VERTEX_POINT('',#156241);
#36845=VERTEX_POINT('',#156243);
#36846=VERTEX_POINT('',#156247);
#36847=VERTEX_POINT('',#156249);
#36848=VERTEX_POINT('',#156253);
#36849=VERTEX_POINT('',#156255);
#36850=VERTEX_POINT('',#156259);
#36851=VERTEX_POINT('',#156260);
#36852=VERTEX_POINT('',#156262);
#36853=VERTEX_POINT('',#156277);
#36854=VERTEX_POINT('',#156278);
#36855=VERTEX_POINT('',#156283);
#36856=VERTEX_POINT('',#156357);
#36857=VERTEX_POINT('',#156421);
#36858=VERTEX_POINT('',#156422);
#36859=VERTEX_POINT('',#156441);
#36860=VERTEX_POINT('',#156442);
#36861=VERTEX_POINT('',#156657);
#36862=VERTEX_POINT('',#156658);
#36863=VERTEX_POINT('',#156698);
#36864=VERTEX_POINT('',#156699);
#36865=VERTEX_POINT('',#156701);
#36866=VERTEX_POINT('',#156703);
#36867=VERTEX_POINT('',#156707);
#36868=VERTEX_POINT('',#156708);
#36869=VERTEX_POINT('',#156710);
#36870=VERTEX_POINT('',#156712);
#36871=VERTEX_POINT('',#156716);
#36872=VERTEX_POINT('',#156798);
#36873=VERTEX_POINT('',#156864);
#36874=VERTEX_POINT('',#156956);
#36875=VERTEX_POINT('',#157089);
#36876=VERTEX_POINT('',#157091);
#36877=VERTEX_POINT('',#157098);
#36878=VERTEX_POINT('',#157099);
#36879=VERTEX_POINT('',#157101);
#36880=VERTEX_POINT('',#157103);
#36881=VERTEX_POINT('',#157107);
#36882=VERTEX_POINT('',#157108);
#36883=VERTEX_POINT('',#157113);
#36884=VERTEX_POINT('',#157115);
#36885=VERTEX_POINT('',#157119);
#36886=VERTEX_POINT('',#157120);
#36887=VERTEX_POINT('',#157122);
#36888=VERTEX_POINT('',#157158);
#36889=VERTEX_POINT('',#157342);
#36890=VERTEX_POINT('',#157343);
#36891=VERTEX_POINT('',#157345);
#36892=VERTEX_POINT('',#157347);
#36893=VERTEX_POINT('',#157351);
#36894=VERTEX_POINT('',#157353);
#36895=VERTEX_POINT('',#157357);
#36896=VERTEX_POINT('',#157358);
#36897=VERTEX_POINT('',#157378);
#36898=VERTEX_POINT('',#157380);
#36899=VERTEX_POINT('',#157419);
#36900=VERTEX_POINT('',#157420);
#36901=VERTEX_POINT('',#157570);
#36902=VERTEX_POINT('',#157571);
#36903=VERTEX_POINT('',#157645);
#36904=VERTEX_POINT('',#157646);
#36905=VERTEX_POINT('',#157648);
#36906=VERTEX_POINT('',#157650);
#36907=VERTEX_POINT('',#157654);
#36908=VERTEX_POINT('',#157655);
#36909=VERTEX_POINT('',#157657);
#36910=VERTEX_POINT('',#157659);
#36911=VERTEX_POINT('',#157666);
#36912=VERTEX_POINT('',#157700);
#36913=VERTEX_POINT('',#157701);
#36914=VERTEX_POINT('',#157721);
#36915=VERTEX_POINT('',#157723);
#36916=VERTEX_POINT('',#157768);
#36917=VERTEX_POINT('',#157769);
#36918=VERTEX_POINT('',#157936);
#36919=VERTEX_POINT('',#157937);
#36920=VERTEX_POINT('',#158010);
#36921=VERTEX_POINT('',#158011);
#36922=VERTEX_POINT('',#158124);
#36923=VERTEX_POINT('',#158126);
#36924=VERTEX_POINT('',#158232);
#36925=VERTEX_POINT('',#158233);
#36926=VERTEX_POINT('',#158253);
#36927=VERTEX_POINT('',#158255);
#36928=VERTEX_POINT('',#158300);
#36929=VERTEX_POINT('',#158301);
#36930=VERTEX_POINT('',#158393);
#36931=VERTEX_POINT('',#158394);
#36932=VERTEX_POINT('',#158433);
#36933=VERTEX_POINT('',#158434);
#36934=VERTEX_POINT('',#158496);
#36935=VERTEX_POINT('',#158498);
#36936=VERTEX_POINT('',#158541);
#36937=VERTEX_POINT('',#158542);
#36938=VERTEX_POINT('',#158568);
#36939=VERTEX_POINT('',#158570);
#36940=VERTEX_POINT('',#158618);
#36941=VERTEX_POINT('',#158619);
#36942=VERTEX_POINT('',#158726);
#36943=VERTEX_POINT('',#158727);
#36944=VERTEX_POINT('',#158785);
#36945=VERTEX_POINT('',#158786);
#36946=VERTEX_POINT('',#158817);
#36947=VERTEX_POINT('',#158819);
#36948=VERTEX_POINT('',#158955);
#36949=VERTEX_POINT('',#158956);
#36950=VERTEX_POINT('',#158973);
#36951=VERTEX_POINT('',#158975);
#36952=VERTEX_POINT('',#159014);
#36953=VERTEX_POINT('',#159015);
#36954=VERTEX_POINT('',#159212);
#36955=VERTEX_POINT('',#159213);
#36956=VERTEX_POINT('',#159248);
#36957=VERTEX_POINT('',#159249);
#36958=VERTEX_POINT('',#159251);
#36959=VERTEX_POINT('',#159268);
#36960=VERTEX_POINT('',#159269);
#36961=VERTEX_POINT('',#159271);
#36962=VERTEX_POINT('',#159273);
#36963=VERTEX_POINT('',#159277);
#36964=VERTEX_POINT('',#159282);
#36965=VERTEX_POINT('',#159286);
#36966=VERTEX_POINT('',#159287);
#36967=VERTEX_POINT('',#159289);
#36968=VERTEX_POINT('',#159291);
#36969=VERTEX_POINT('',#159295);
#36970=VERTEX_POINT('',#159296);
#36971=VERTEX_POINT('',#159316);
#36972=VERTEX_POINT('',#159318);
#36973=VERTEX_POINT('',#159357);
#36974=VERTEX_POINT('',#159358);
#36975=VERTEX_POINT('',#159501);
#36976=VERTEX_POINT('',#159502);
#36977=VERTEX_POINT('',#159552);
#36978=VERTEX_POINT('',#159554);
#36979=VERTEX_POINT('',#159558);
#36980=VERTEX_POINT('',#159559);
#36981=VERTEX_POINT('',#159564);
#36982=VERTEX_POINT('',#159565);
#36983=VERTEX_POINT('',#159570);
#36984=VERTEX_POINT('',#159571);
#36985=VERTEX_POINT('',#159591);
#36986=VERTEX_POINT('',#159593);
#36987=VERTEX_POINT('',#159612);
#36988=VERTEX_POINT('',#159613);
#36989=VERTEX_POINT('',#159615);
#36990=VERTEX_POINT('',#159617);
#36991=VERTEX_POINT('',#159621);
#36992=VERTEX_POINT('',#159622);
#36993=VERTEX_POINT('',#159639);
#36994=VERTEX_POINT('',#159641);
#36995=VERTEX_POINT('',#159660);
#36996=VERTEX_POINT('',#159661);
#36997=VERTEX_POINT('',#159687);
#36998=VERTEX_POINT('',#159689);
#36999=VERTEX_POINT('',#159717);
#37000=VERTEX_POINT('',#159718);
#37001=VERTEX_POINT('',#159720);
#37002=VERTEX_POINT('',#159722);
#37003=VERTEX_POINT('',#159742);
#37004=VERTEX_POINT('',#159744);
#37005=VERTEX_POINT('',#159831);
#37006=VERTEX_POINT('',#159832);
#37007=VERTEX_POINT('',#159928);
#37008=VERTEX_POINT('',#159929);
#37009=VERTEX_POINT('',#160102);
#37010=VERTEX_POINT('',#160104);
#37011=VERTEX_POINT('',#160125);
#37012=VERTEX_POINT('',#160126);
#37013=VERTEX_POINT('',#160364);
#37014=VERTEX_POINT('',#160365);
#37015=VERTEX_POINT('',#160367);
#37016=VERTEX_POINT('',#160369);
#37017=VERTEX_POINT('',#160396);
#37018=VERTEX_POINT('',#160398);
#37019=VERTEX_POINT('',#160414);
#37020=VERTEX_POINT('',#160507);
#37021=VERTEX_POINT('',#160509);
#37022=VERTEX_POINT('',#160565);
#37023=VERTEX_POINT('',#160575);
#37024=VERTEX_POINT('',#160596);
#37025=VERTEX_POINT('',#160604);
#37026=VERTEX_POINT('',#160653);
#37027=VERTEX_POINT('',#160654);
#37028=VERTEX_POINT('',#160817);
#37029=VERTEX_POINT('',#160818);
#37030=VERTEX_POINT('',#160820);
#37031=VERTEX_POINT('',#160885);
#37032=VERTEX_POINT('',#160906);
#37033=VERTEX_POINT('',#160914);
#37034=VERTEX_POINT('',#160963);
#37035=VERTEX_POINT('',#160964);
#37036=VERTEX_POINT('',#160966);
#37037=VERTEX_POINT('',#161037);
#37038=VERTEX_POINT('',#161041);
#37039=VERTEX_POINT('',#161043);
#37040=VERTEX_POINT('',#161047);
#37041=VERTEX_POINT('',#161049);
#37042=VERTEX_POINT('',#161053);
#37043=VERTEX_POINT('',#161055);
#37044=VERTEX_POINT('',#161076);
#37045=VERTEX_POINT('',#161078);
#37046=VERTEX_POINT('',#161128);
#37047=VERTEX_POINT('',#161138);
#37048=VERTEX_POINT('',#161159);
#37049=VERTEX_POINT('',#161167);
#37050=VERTEX_POINT('',#161222);
#37051=VERTEX_POINT('',#161299);
#37052=VERTEX_POINT('',#161320);
#37053=VERTEX_POINT('',#161336);
#37054=VERTEX_POINT('',#161338);
#37055=VERTEX_POINT('',#161428);
#37056=VERTEX_POINT('',#161429);
#37057=VERTEX_POINT('',#161431);
#37058=VERTEX_POINT('',#161490);
#37059=VERTEX_POINT('',#161511);
#37060=VERTEX_POINT('',#161519);
#37061=VERTEX_POINT('',#161574);
#37062=VERTEX_POINT('',#161575);
#37063=VERTEX_POINT('',#161735);
#37064=VERTEX_POINT('',#161825);
#37065=VERTEX_POINT('',#161826);
#37066=VERTEX_POINT('',#161828);
#37067=VERTEX_POINT('',#161843);
#37068=VERTEX_POINT('',#161885);
#37069=VERTEX_POINT('',#161890);
#37070=VERTEX_POINT('',#161923);
#37071=VERTEX_POINT('',#161924);
#37072=VERTEX_POINT('',#162034);
#37073=VERTEX_POINT('',#162035);
#37074=VERTEX_POINT('',#162063);
#37075=VERTEX_POINT('',#162065);
#37076=VERTEX_POINT('',#162139);
#37077=VERTEX_POINT('',#162152);
#37078=VERTEX_POINT('',#162173);
#37079=VERTEX_POINT('',#162218);
#37080=VERTEX_POINT('',#162219);
#37081=VERTEX_POINT('',#162233);
#37082=VERTEX_POINT('',#162234);
#37083=VERTEX_POINT('',#162268);
#37084=VERTEX_POINT('',#162270);
#37085=VERTEX_POINT('',#162335);
#37086=VERTEX_POINT('',#162392);
#37087=VERTEX_POINT('',#162419);
#37088=VERTEX_POINT('',#162502);
#37089=VERTEX_POINT('',#162520);
#37090=VERTEX_POINT('',#162521);
#37091=VERTEX_POINT('',#162549);
#37092=VERTEX_POINT('',#162551);
#37093=VERTEX_POINT('',#162628);
#37094=VERTEX_POINT('',#162659);
#37095=VERTEX_POINT('',#162698);
#37096=VERTEX_POINT('',#162739);
#37097=VERTEX_POINT('',#162830);
#37098=VERTEX_POINT('',#162831);
#37099=VERTEX_POINT('',#162865);
#37100=VERTEX_POINT('',#162867);
#37101=VERTEX_POINT('',#162938);
#37102=VERTEX_POINT('',#163001);
#37103=VERTEX_POINT('',#163022);
#37104=VERTEX_POINT('',#163051);
#37105=VERTEX_POINT('',#163103);
#37106=VERTEX_POINT('',#163104);
#37107=VERTEX_POINT('',#163120);
#37108=VERTEX_POINT('',#163122);
#37109=VERTEX_POINT('',#163129);
#37110=VERTEX_POINT('',#163180);
#37111=VERTEX_POINT('',#163211);
#37112=VERTEX_POINT('',#163244);
#37113=VERTEX_POINT('',#163245);
#37114=VERTEX_POINT('',#163310);
#37115=VERTEX_POINT('',#163311);
#37116=VERTEX_POINT('',#163345);
#37117=VERTEX_POINT('',#163346);
#37118=VERTEX_POINT('',#163348);
#37119=VERTEX_POINT('',#163464);
#37120=VERTEX_POINT('',#163479);
#37121=VERTEX_POINT('',#163487);
#37122=VERTEX_POINT('',#163538);
#37123=VERTEX_POINT('',#163573);
#37124=VERTEX_POINT('',#163630);
#37125=VERTEX_POINT('',#163631);
#37126=VERTEX_POINT('',#163669);
#37127=VERTEX_POINT('',#163685);
#37128=VERTEX_POINT('',#163778);
#37129=VERTEX_POINT('',#163780);
#37130=VERTEX_POINT('',#163836);
#37131=VERTEX_POINT('',#163846);
#37132=VERTEX_POINT('',#163867);
#37133=VERTEX_POINT('',#163875);
#37134=VERTEX_POINT('',#163924);
#37135=VERTEX_POINT('',#163925);
#37136=VERTEX_POINT('',#164088);
#37137=VERTEX_POINT('',#164089);
#37138=VERTEX_POINT('',#164091);
#37139=VERTEX_POINT('',#164156);
#37140=VERTEX_POINT('',#164177);
#37141=VERTEX_POINT('',#164185);
#37142=VERTEX_POINT('',#164234);
#37143=VERTEX_POINT('',#164235);
#37144=VERTEX_POINT('',#164237);
#37145=VERTEX_POINT('',#164308);
#37146=VERTEX_POINT('',#164312);
#37147=VERTEX_POINT('',#164314);
#37148=VERTEX_POINT('',#164318);
#37149=VERTEX_POINT('',#164320);
#37150=VERTEX_POINT('',#164324);
#37151=VERTEX_POINT('',#164326);
#37152=VERTEX_POINT('',#164330);
#37153=VERTEX_POINT('',#164332);
#37154=VERTEX_POINT('',#164405);
#37155=VERTEX_POINT('',#164406);
#37156=VERTEX_POINT('',#164408);
#37157=VERTEX_POINT('',#164429);
#37158=VERTEX_POINT('',#164430);
#37159=VERTEX_POINT('',#164659);
#37160=VERTEX_POINT('',#164660);
#37161=VERTEX_POINT('',#164677);
#37162=VERTEX_POINT('',#164784);
#37163=VERTEX_POINT('',#164890);
#37164=VERTEX_POINT('',#164891);
#37165=VERTEX_POINT('',#164896);
#37166=VERTEX_POINT('',#164897);
#37167=VERTEX_POINT('',#164899);
#37168=VERTEX_POINT('',#164940);
#37169=VERTEX_POINT('',#164944);
#37170=VERTEX_POINT('',#164945);
#37171=VERTEX_POINT('',#164950);
#37172=VERTEX_POINT('',#164952);
#37173=VERTEX_POINT('',#164956);
#37174=VERTEX_POINT('',#164971);
#37175=VERTEX_POINT('',#164973);
#37176=VERTEX_POINT('',#164990);
#37177=VERTEX_POINT('',#165020);
#37178=VERTEX_POINT('',#165051);
#37179=VERTEX_POINT('',#165078);
#37180=VERTEX_POINT('',#165108);
#37181=VERTEX_POINT('',#165138);
#37182=VERTEX_POINT('',#165154);
#37183=VERTEX_POINT('',#165187);
#37184=VERTEX_POINT('',#165188);
#37185=VERTEX_POINT('',#165207);
#37186=VERTEX_POINT('',#165208);
#37187=VERTEX_POINT('',#165210);
#37188=VERTEX_POINT('',#165212);
#37189=VERTEX_POINT('',#165216);
#37190=VERTEX_POINT('',#165218);
#37191=VERTEX_POINT('',#165222);
#37192=VERTEX_POINT('',#165226);
#37193=VERTEX_POINT('',#165228);
#37194=VERTEX_POINT('',#165232);
#37195=VERTEX_POINT('',#165236);
#37196=VERTEX_POINT('',#165242);
#37197=VERTEX_POINT('',#165276);
#37198=VERTEX_POINT('',#165289);
#37199=VERTEX_POINT('',#165310);
#37200=VERTEX_POINT('',#165346);
#37201=VERTEX_POINT('',#165376);
#37202=VERTEX_POINT('',#165398);
#37203=VERTEX_POINT('',#165425);
#37204=VERTEX_POINT('',#165455);
#37205=VERTEX_POINT('',#165479);
#37206=VERTEX_POINT('',#165496);
#37207=VERTEX_POINT('',#165575);
#37208=VERTEX_POINT('',#165577);
#37209=VERTEX_POINT('',#165581);
#37210=VERTEX_POINT('',#165654);
#37211=VERTEX_POINT('',#165656);
#37212=VERTEX_POINT('',#165660);
#37213=VERTEX_POINT('',#165664);
#37214=VERTEX_POINT('',#165665);
#37215=VERTEX_POINT('',#165667);
#37216=VERTEX_POINT('',#165695);
#37217=VERTEX_POINT('',#165728);
#37218=VERTEX_POINT('',#165770);
#37219=VERTEX_POINT('',#165792);
#37220=VERTEX_POINT('',#165825);
#37221=VERTEX_POINT('',#165855);
#37222=VERTEX_POINT('',#165891);
#37223=VERTEX_POINT('',#165907);
#37224=VERTEX_POINT('',#165940);
#37225=VERTEX_POINT('',#165941);
#37226=VERTEX_POINT('',#165960);
#37227=VERTEX_POINT('',#165962);
#37228=VERTEX_POINT('',#165966);
#37229=VERTEX_POINT('',#165970);
#37230=VERTEX_POINT('',#165971);
#37231=VERTEX_POINT('',#165974);
#37232=VERTEX_POINT('',#165978);
#37233=VERTEX_POINT('',#165980);
#37234=VERTEX_POINT('',#165984);
#37235=VERTEX_POINT('',#166017);
#37236=VERTEX_POINT('',#166046);
#37237=VERTEX_POINT('',#166075);
#37238=VERTEX_POINT('',#166077);
#37239=VERTEX_POINT('',#166081);
#37240=VERTEX_POINT('',#166085);
#37241=VERTEX_POINT('',#166091);
#37242=VERTEX_POINT('',#166147);
#37243=VERTEX_POINT('',#166149);
#37244=VERTEX_POINT('',#166173);
#37245=VERTEX_POINT('',#166206);
#37246=VERTEX_POINT('',#166225);
#37247=VERTEX_POINT('',#166246);
#37248=VERTEX_POINT('',#166291);
#37249=VERTEX_POINT('',#166292);
#37250=VERTEX_POINT('',#166330);
#37251=VERTEX_POINT('',#166332);
#37252=VERTEX_POINT('',#166336);
#37253=VERTEX_POINT('',#166342);
#37254=VERTEX_POINT('',#166454);
#37255=VERTEX_POINT('',#166455);
#37256=VERTEX_POINT('',#166462);
#37257=VERTEX_POINT('',#166464);
#37258=VERTEX_POINT('',#166468);
#37259=VERTEX_POINT('',#166489);
#37260=VERTEX_POINT('',#166491);
#37261=VERTEX_POINT('',#166547);
#37262=VERTEX_POINT('',#166583);
#37263=VERTEX_POINT('',#166613);
#37264=VERTEX_POINT('',#166635);
#37265=VERTEX_POINT('',#166662);
#37266=VERTEX_POINT('',#166692);
#37267=VERTEX_POINT('',#166716);
#37268=VERTEX_POINT('',#166735);
#37269=VERTEX_POINT('',#166768);
#37270=VERTEX_POINT('',#166786);
#37271=VERTEX_POINT('',#166788);
#37272=VERTEX_POINT('',#166792);
#37273=VERTEX_POINT('',#166796);
#37274=VERTEX_POINT('',#166798);
#37275=VERTEX_POINT('',#166802);
#37276=VERTEX_POINT('',#166806);
#37277=VERTEX_POINT('',#166812);
#37278=VERTEX_POINT('',#166846);
#37279=VERTEX_POINT('',#166859);
#37280=VERTEX_POINT('',#166892);
#37281=VERTEX_POINT('',#166925);
#37282=VERTEX_POINT('',#166961);
#37283=VERTEX_POINT('',#166980);
#37284=VERTEX_POINT('',#167007);
#37285=VERTEX_POINT('',#167037);
#37286=VERTEX_POINT('',#167042);
#37287=VERTEX_POINT('',#167064);
#37288=VERTEX_POINT('',#167065);
#37289=VERTEX_POINT('',#167067);
#37290=VERTEX_POINT('',#167069);
#37291=VERTEX_POINT('',#167186);
#37292=VERTEX_POINT('',#167217);
#37293=VERTEX_POINT('',#167219);
#37294=VERTEX_POINT('',#167223);
#37295=VERTEX_POINT('',#167238);
#37296=VERTEX_POINT('',#167239);
#37297=VERTEX_POINT('',#167241);
#37298=VERTEX_POINT('',#167243);
#37299=VERTEX_POINT('',#167270);
#37300=VERTEX_POINT('',#167292);
#37301=VERTEX_POINT('',#167325);
#37302=VERTEX_POINT('',#167344);
#37303=VERTEX_POINT('',#167365);
#37304=VERTEX_POINT('',#167410);
#37305=VERTEX_POINT('',#167431);
#37306=VERTEX_POINT('',#167455);
#37307=VERTEX_POINT('',#167476);
#37308=VERTEX_POINT('',#167478);
#37309=VERTEX_POINT('',#167482);
#37310=VERTEX_POINT('',#167484);
#37311=VERTEX_POINT('',#167486);
#37312=VERTEX_POINT('',#167519);
#37313=VERTEX_POINT('',#167535);
#37314=VERTEX_POINT('',#167539);
#37315=VERTEX_POINT('',#167543);
#37316=VERTEX_POINT('',#167576);
#37317=VERTEX_POINT('',#167577);
#37318=VERTEX_POINT('',#167579);
#37319=VERTEX_POINT('',#167599);
#37320=VERTEX_POINT('',#167601);
#37321=VERTEX_POINT('',#167619);
#37322=VERTEX_POINT('',#167620);
#37323=VERTEX_POINT('',#167661);
#37324=VERTEX_POINT('',#167663);
#37325=VERTEX_POINT('',#167667);
#37326=VERTEX_POINT('',#167671);
#37327=VERTEX_POINT('',#167673);
#37328=VERTEX_POINT('',#167700);
#37329=VERTEX_POINT('',#167733);
#37330=VERTEX_POINT('',#167775);
#37331=VERTEX_POINT('',#167797);
#37332=VERTEX_POINT('',#167830);
#37333=VERTEX_POINT('',#167860);
#37334=VERTEX_POINT('',#167896);
#37335=VERTEX_POINT('',#167897);
#37336=VERTEX_POINT('',#167992);
#37337=VERTEX_POINT('',#167994);
#37338=VERTEX_POINT('',#167998);
#37339=VERTEX_POINT('',#168002);
#37340=VERTEX_POINT('',#168008);
#37341=VERTEX_POINT('',#168011);
#37342=VERTEX_POINT('',#168055);
#37343=VERTEX_POINT('',#168057);
#37344=VERTEX_POINT('',#168061);
#37345=VERTEX_POINT('',#168062);
#37346=VERTEX_POINT('',#168092);
#37347=VERTEX_POINT('',#168093);
#37348=VERTEX_POINT('',#168095);
#37349=VERTEX_POINT('',#168201);
#37350=VERTEX_POINT('',#168231);
#37351=VERTEX_POINT('',#168250);
#37352=VERTEX_POINT('',#168252);
#37353=VERTEX_POINT('',#168256);
#37354=VERTEX_POINT('',#168257);
#37355=VERTEX_POINT('',#168259);
#37356=VERTEX_POINT('',#168261);
#37357=VERTEX_POINT('',#168265);
#37358=VERTEX_POINT('',#168267);
#37359=VERTEX_POINT('',#168271);
#37360=VERTEX_POINT('',#168273);
#37361=VERTEX_POINT('',#168277);
#37362=VERTEX_POINT('',#168279);
#37363=VERTEX_POINT('',#168376);
#37364=VERTEX_POINT('',#168396);
#37365=VERTEX_POINT('',#168411);
#37366=VERTEX_POINT('',#168412);
#37367=VERTEX_POINT('',#168414);
#37368=VERTEX_POINT('',#168466);
#37369=VERTEX_POINT('',#168482);
#37370=VERTEX_POINT('',#168484);
#37371=VERTEX_POINT('',#168488);
#37372=VERTEX_POINT('',#168489);
#37373=VERTEX_POINT('',#168491);
#37374=VERTEX_POINT('',#168493);
#37375=VERTEX_POINT('',#168497);
#37376=VERTEX_POINT('',#168499);
#37377=VERTEX_POINT('',#168503);
#37378=VERTEX_POINT('',#168505);
#37379=VERTEX_POINT('',#168509);
#37380=VERTEX_POINT('',#168511);
#37381=VERTEX_POINT('',#168513);
#37382=VERTEX_POINT('',#168540);
#37383=VERTEX_POINT('',#168567);
#37384=VERTEX_POINT('',#168591);
#37385=VERTEX_POINT('',#168592);
#37386=VERTEX_POINT('',#168690);
#37387=VERTEX_POINT('',#168691);
#37388=VERTEX_POINT('',#168696);
#37389=VERTEX_POINT('',#168697);
#37390=VERTEX_POINT('',#168704);
#37391=VERTEX_POINT('',#168706);
#37392=VERTEX_POINT('',#168710);
#37393=VERTEX_POINT('',#168731);
#37394=VERTEX_POINT('',#168733);
#37395=VERTEX_POINT('',#168789);
#37396=VERTEX_POINT('',#168825);
#37397=VERTEX_POINT('',#168855);
#37398=VERTEX_POINT('',#168883);
#37399=VERTEX_POINT('',#168910);
#37400=VERTEX_POINT('',#168940);
#37401=VERTEX_POINT('',#168964);
#37402=VERTEX_POINT('',#168983);
#37403=VERTEX_POINT('',#169016);
#37404=VERTEX_POINT('',#169034);
#37405=VERTEX_POINT('',#169036);
#37406=VERTEX_POINT('',#169040);
#37407=VERTEX_POINT('',#169044);
#37408=VERTEX_POINT('',#169046);
#37409=VERTEX_POINT('',#169050);
#37410=VERTEX_POINT('',#169054);
#37411=VERTEX_POINT('',#169060);
#37412=VERTEX_POINT('',#169094);
#37413=VERTEX_POINT('',#169107);
#37414=VERTEX_POINT('',#169140);
#37415=VERTEX_POINT('',#169173);
#37416=VERTEX_POINT('',#169209);
#37417=VERTEX_POINT('',#169228);
#37418=VERTEX_POINT('',#169255);
#37419=VERTEX_POINT('',#169282);
#37420=VERTEX_POINT('',#169287);
#37421=VERTEX_POINT('',#169303);
#37422=VERTEX_POINT('',#169304);
#37423=VERTEX_POINT('',#169306);
#37424=VERTEX_POINT('',#169308);
#37425=VERTEX_POINT('',#169425);
#37426=VERTEX_POINT('',#169444);
#37427=VERTEX_POINT('',#169446);
#37428=VERTEX_POINT('',#169450);
#37429=VERTEX_POINT('',#169465);
#37430=VERTEX_POINT('',#169467);
#37431=VERTEX_POINT('',#169497);
#37432=VERTEX_POINT('',#169513);
#37433=VERTEX_POINT('',#169534);
#37434=VERTEX_POINT('',#169570);
#37435=VERTEX_POINT('',#169588);
#37436=VERTEX_POINT('',#169612);
#37437=VERTEX_POINT('',#169613);
#37438=VERTEX_POINT('',#169674);
#37439=VERTEX_POINT('',#169688);
#37440=VERTEX_POINT('',#169692);
#37441=VERTEX_POINT('',#169694);
#37442=VERTEX_POINT('',#169696);
#37443=VERTEX_POINT('',#169729);
#37444=VERTEX_POINT('',#169745);
#37445=VERTEX_POINT('',#169749);
#37446=VERTEX_POINT('',#169753);
#37447=VERTEX_POINT('',#169786);
#37448=VERTEX_POINT('',#169787);
#37449=VERTEX_POINT('',#169789);
#37450=VERTEX_POINT('',#169852);
#37451=VERTEX_POINT('',#169853);
#37452=VERTEX_POINT('',#169858);
#37453=VERTEX_POINT('',#169859);
#37454=VERTEX_POINT('',#169864);
#37455=VERTEX_POINT('',#169868);
#37456=VERTEX_POINT('',#169870);
#37457=VERTEX_POINT('',#169885);
#37458=VERTEX_POINT('',#169909);
#37459=VERTEX_POINT('',#169966);
#37460=VERTEX_POINT('',#169985);
#37461=VERTEX_POINT('',#170012);
#37462=VERTEX_POINT('',#170057);
#37463=VERTEX_POINT('',#170077);
#37464=VERTEX_POINT('',#170105);
#37465=VERTEX_POINT('',#170107);
#37466=VERTEX_POINT('',#170111);
#37467=VERTEX_POINT('',#170115);
#37468=VERTEX_POINT('',#170121);
#37469=VERTEX_POINT('',#170124);
#37470=VERTEX_POINT('',#170168);
#37471=VERTEX_POINT('',#170172);
#37472=VERTEX_POINT('',#170174);
#37473=VERTEX_POINT('',#170178);
#37474=VERTEX_POINT('',#170180);
#37475=VERTEX_POINT('',#170217);
#37476=VERTEX_POINT('',#170219);
#37477=VERTEX_POINT('',#170246);
#37478=VERTEX_POINT('',#170274);
#37479=VERTEX_POINT('',#170295);
#37480=VERTEX_POINT('',#170296);
#37481=VERTEX_POINT('',#170360);
#37482=VERTEX_POINT('',#170362);
#37483=VERTEX_POINT('',#170366);
#37484=VERTEX_POINT('',#170372);
#37485=VERTEX_POINT('',#170407);
#37486=VERTEX_POINT('',#170408);
#37487=VERTEX_POINT('',#170451);
#37488=VERTEX_POINT('',#170568);
#37489=VERTEX_POINT('',#170570);
#37490=VERTEX_POINT('',#170581);
#37491=VERTEX_POINT('',#170602);
#37492=VERTEX_POINT('',#170638);
#37493=VERTEX_POINT('',#170659);
#37494=VERTEX_POINT('',#170666);
#37495=VERTEX_POINT('',#170670);
#37496=VERTEX_POINT('',#170674);
#37497=VERTEX_POINT('',#170695);
#37498=VERTEX_POINT('',#170727);
#37499=VERTEX_POINT('',#170737);
#37500=VERTEX_POINT('',#170739);
#37501=VERTEX_POINT('',#170743);
#37502=VERTEX_POINT('',#170747);
#37503=VERTEX_POINT('',#170749);
#37504=VERTEX_POINT('',#170753);
#37505=VERTEX_POINT('',#170759);
#37506=VERTEX_POINT('',#170775);
#37507=VERTEX_POINT('',#170796);
#37508=VERTEX_POINT('',#170823);
#37509=VERTEX_POINT('',#170842);
#37510=VERTEX_POINT('',#170863);
#37511=VERTEX_POINT('',#170864);
#37512=VERTEX_POINT('',#171000);
#37513=VERTEX_POINT('',#171001);
#37514=VERTEX_POINT('',#171050);
#37515=VERTEX_POINT('',#171173);
#37516=VERTEX_POINT('',#171175);
#37517=VERTEX_POINT('',#171191);
#37518=VERTEX_POINT('',#171212);
#37519=VERTEX_POINT('',#171239);
#37520=VERTEX_POINT('',#171257);
#37521=VERTEX_POINT('',#171305);
#37522=VERTEX_POINT('',#171359);
#37523=VERTEX_POINT('',#171376);
#37524=VERTEX_POINT('',#171383);
#37525=VERTEX_POINT('',#171384);
#37526=VERTEX_POINT('',#171389);
#37527=VERTEX_POINT('',#171396);
#37528=VERTEX_POINT('',#171398);
#37529=VERTEX_POINT('',#171481);
#37530=VERTEX_POINT('',#171497);
#37531=VERTEX_POINT('',#171512);
#37532=VERTEX_POINT('',#171536);
#37533=VERTEX_POINT('',#171552);
#37534=VERTEX_POINT('',#171573);
#37535=VERTEX_POINT('',#171587);
#37536=VERTEX_POINT('',#171665);
#37537=VERTEX_POINT('',#171670);
#37538=VERTEX_POINT('',#171712);
#37539=VERTEX_POINT('',#171766);
#37540=VERTEX_POINT('',#171768);
#37541=VERTEX_POINT('',#171772);
#37542=VERTEX_POINT('',#171787);
#37543=VERTEX_POINT('',#171802);
#37544=VERTEX_POINT('',#171820);
#37545=VERTEX_POINT('',#171856);
#37546=VERTEX_POINT('',#171895);
#37547=VERTEX_POINT('',#171906);
#37548=VERTEX_POINT('',#171913);
#37549=VERTEX_POINT('',#171914);
#37550=VERTEX_POINT('',#171919);
#37551=VERTEX_POINT('',#171923);
#37552=VERTEX_POINT('',#171925);
#37553=VERTEX_POINT('',#171984);
#37554=VERTEX_POINT('',#172000);
#37555=VERTEX_POINT('',#172015);
#37556=VERTEX_POINT('',#172033);
#37557=VERTEX_POINT('',#172037);
#37558=VERTEX_POINT('',#172052);
#37559=VERTEX_POINT('',#172054);
#37560=VERTEX_POINT('',#172069);
#37561=VERTEX_POINT('',#172074);
#37562=VERTEX_POINT('',#172119);
#37563=VERTEX_POINT('',#172227);
#37564=VERTEX_POINT('',#172229);
#37565=VERTEX_POINT('',#172245);
#37566=VERTEX_POINT('',#172266);
#37567=VERTEX_POINT('',#172293);
#37568=VERTEX_POINT('',#172311);
#37569=VERTEX_POINT('',#172359);
#37570=VERTEX_POINT('',#172407);
#37571=VERTEX_POINT('',#172423);
#37572=VERTEX_POINT('',#172430);
#37573=VERTEX_POINT('',#172432);
#37574=VERTEX_POINT('',#172436);
#37575=VERTEX_POINT('',#172443);
#37576=VERTEX_POINT('',#172445);
#37577=VERTEX_POINT('',#172528);
#37578=VERTEX_POINT('',#172544);
#37579=VERTEX_POINT('',#172559);
#37580=VERTEX_POINT('',#172583);
#37581=VERTEX_POINT('',#172599);
#37582=VERTEX_POINT('',#172620);
#37583=VERTEX_POINT('',#172634);
#37584=VERTEX_POINT('',#172712);
#37585=VERTEX_POINT('',#172717);
#37586=VERTEX_POINT('',#172759);
#37587=VERTEX_POINT('',#172882);
#37588=VERTEX_POINT('',#172884);
#37589=VERTEX_POINT('',#172903);
#37590=VERTEX_POINT('',#172924);
#37591=VERTEX_POINT('',#172957);
#37592=VERTEX_POINT('',#172978);
#37593=VERTEX_POINT('',#172985);
#37594=VERTEX_POINT('',#172989);
#37595=VERTEX_POINT('',#173010);
#37596=VERTEX_POINT('',#173054);
#37597=VERTEX_POINT('',#173064);
#37598=VERTEX_POINT('',#173066);
#37599=VERTEX_POINT('',#173070);
#37600=VERTEX_POINT('',#173074);
#37601=VERTEX_POINT('',#173076);
#37602=VERTEX_POINT('',#173080);
#37603=VERTEX_POINT('',#173084);
#37604=VERTEX_POINT('',#173090);
#37605=VERTEX_POINT('',#173106);
#37606=VERTEX_POINT('',#173127);
#37607=VERTEX_POINT('',#173154);
#37608=VERTEX_POINT('',#173165);
#37609=VERTEX_POINT('',#173186);
#37610=VERTEX_POINT('',#173187);
#37611=VERTEX_POINT('',#173320);
#37612=VERTEX_POINT('',#173321);
#37613=VERTEX_POINT('',#173379);
#37614=VERTEX_POINT('',#173503);
#37615=VERTEX_POINT('',#173505);
#37616=VERTEX_POINT('',#173509);
#37617=VERTEX_POINT('',#173530);
#37618=VERTEX_POINT('',#173531);
#37619=VERTEX_POINT('',#173533);
#37620=VERTEX_POINT('',#173600);
#37621=VERTEX_POINT('',#173628);
#37622=VERTEX_POINT('',#173649);
#37623=VERTEX_POINT('',#173691);
#37624=VERTEX_POINT('',#173712);
#37625=VERTEX_POINT('',#173721);
#37626=VERTEX_POINT('',#173723);
#37627=VERTEX_POINT('',#173727);
#37628=VERTEX_POINT('',#173731);
#37629=VERTEX_POINT('',#173735);
#37630=VERTEX_POINT('',#173737);
#37631=VERTEX_POINT('',#173741);
#37632=VERTEX_POINT('',#173745);
#37633=VERTEX_POINT('',#173760);
#37634=VERTEX_POINT('',#173761);
#37635=VERTEX_POINT('',#173763);
#37636=VERTEX_POINT('',#173778);
#37637=VERTEX_POINT('',#173796);
#37638=VERTEX_POINT('',#173797);
#37639=VERTEX_POINT('',#173799);
#37640=VERTEX_POINT('',#173804);
#37641=VERTEX_POINT('',#173832);
#37642=VERTEX_POINT('',#173833);
#37643=VERTEX_POINT('',#173835);
#37644=VERTEX_POINT('',#173837);
#37645=VERTEX_POINT('',#173855);
#37646=VERTEX_POINT('',#173856);
#37647=VERTEX_POINT('',#173893);
#37648=VERTEX_POINT('',#173894);
#37649=VERTEX_POINT('',#173896);
#37650=VERTEX_POINT('',#173901);
#37651=VERTEX_POINT('',#173940);
#37652=VERTEX_POINT('',#173949);
#37653=VERTEX_POINT('',#174055);
#37654=VERTEX_POINT('',#174057);
#37655=VERTEX_POINT('',#174061);
#37656=VERTEX_POINT('',#174062);
#37657=VERTEX_POINT('',#174064);
#37658=VERTEX_POINT('',#174066);
#37659=VERTEX_POINT('',#174070);
#37660=VERTEX_POINT('',#174072);
#37661=VERTEX_POINT('',#174076);
#37662=VERTEX_POINT('',#174078);
#37663=VERTEX_POINT('',#174082);
#37664=VERTEX_POINT('',#174084);
#37665=VERTEX_POINT('',#174086);
#37666=VERTEX_POINT('',#174107);
#37667=VERTEX_POINT('',#174137);
#37668=VERTEX_POINT('',#174138);
#37669=VERTEX_POINT('',#174187);
#37670=VERTEX_POINT('',#174188);
#37671=VERTEX_POINT('',#174276);
#37672=VERTEX_POINT('',#174277);
#37673=VERTEX_POINT('',#174284);
#37674=VERTEX_POINT('',#174285);
#37675=VERTEX_POINT('',#174287);
#37676=VERTEX_POINT('',#174292);
#37677=VERTEX_POINT('',#174296);
#37678=VERTEX_POINT('',#174311);
#37679=VERTEX_POINT('',#174312);
#37680=VERTEX_POINT('',#174314);
#37681=VERTEX_POINT('',#174357);
#37682=VERTEX_POINT('',#174385);
#37683=VERTEX_POINT('',#174406);
#37684=VERTEX_POINT('',#174426);
#37685=VERTEX_POINT('',#174479);
#37686=VERTEX_POINT('',#174484);
#37687=VERTEX_POINT('',#174523);
#37688=VERTEX_POINT('',#174580);
#37689=VERTEX_POINT('',#174582);
#37690=VERTEX_POINT('',#174586);
#37691=VERTEX_POINT('',#174607);
#37692=VERTEX_POINT('',#174609);
#37693=VERTEX_POINT('',#174628);
#37694=VERTEX_POINT('',#174649);
#37695=VERTEX_POINT('',#174676);
#37696=VERTEX_POINT('',#174677);
#37697=VERTEX_POINT('',#174714);
#37698=VERTEX_POINT('',#174734);
#37699=VERTEX_POINT('',#174741);
#37700=VERTEX_POINT('',#174743);
#37701=VERTEX_POINT('',#174747);
#37702=VERTEX_POINT('',#174751);
#37703=VERTEX_POINT('',#174753);
#37704=VERTEX_POINT('',#174757);
#37705=VERTEX_POINT('',#174761);
#37706=VERTEX_POINT('',#174776);
#37707=VERTEX_POINT('',#174777);
#37708=VERTEX_POINT('',#174779);
#37709=VERTEX_POINT('',#174822);
#37710=VERTEX_POINT('',#174841);
#37711=VERTEX_POINT('',#174862);
#37712=VERTEX_POINT('',#174876);
#37713=VERTEX_POINT('',#174987);
#37714=VERTEX_POINT('',#174992);
#37715=VERTEX_POINT('',#175031);
#37716=VERTEX_POINT('',#175151);
#37717=VERTEX_POINT('',#175153);
#37718=VERTEX_POINT('',#175169);
#37719=VERTEX_POINT('',#175190);
#37720=VERTEX_POINT('',#175217);
#37721=VERTEX_POINT('',#175218);
#37722=VERTEX_POINT('',#175252);
#37723=VERTEX_POINT('',#175268);
#37724=VERTEX_POINT('',#175275);
#37725=VERTEX_POINT('',#175276);
#37726=VERTEX_POINT('',#175278);
#37727=VERTEX_POINT('',#175280);
#37728=VERTEX_POINT('',#175284);
#37729=VERTEX_POINT('',#175289);
#37730=VERTEX_POINT('',#175296);
#37731=VERTEX_POINT('',#175298);
#37732=VERTEX_POINT('',#175313);
#37733=VERTEX_POINT('',#175314);
#37734=VERTEX_POINT('',#175316);
#37735=VERTEX_POINT('',#175354);
#37736=VERTEX_POINT('',#175370);
#37737=VERTEX_POINT('',#175391);
#37738=VERTEX_POINT('',#175405);
#37739=VERTEX_POINT('',#175489);
#37740=VERTEX_POINT('',#175494);
#37741=VERTEX_POINT('',#175572);
#37742=VERTEX_POINT('',#175599);
#37743=VERTEX_POINT('',#175601);
#37744=VERTEX_POINT('',#175605);
#37745=VERTEX_POINT('',#175620);
#37746=VERTEX_POINT('',#175635);
#37747=VERTEX_POINT('',#175636);
#37748=VERTEX_POINT('',#175666);
#37749=VERTEX_POINT('',#175679);
#37750=VERTEX_POINT('',#175686);
#37751=VERTEX_POINT('',#175688);
#37752=VERTEX_POINT('',#175692);
#37753=VERTEX_POINT('',#175739);
#37754=VERTEX_POINT('',#175788);
#37755=VERTEX_POINT('',#175790);
#37756=VERTEX_POINT('',#175819);
#37757=VERTEX_POINT('',#175820);
#37758=VERTEX_POINT('',#175838);
#37759=VERTEX_POINT('',#175839);
#37760=VERTEX_POINT('',#175885);
#37761=VERTEX_POINT('',#175923);
#37762=VERTEX_POINT('',#176036);
#37763=VERTEX_POINT('',#176112);
#37764=VERTEX_POINT('',#176223);
#37765=VERTEX_POINT('',#176224);
#37766=VERTEX_POINT('',#176242);
#37767=VERTEX_POINT('',#176243);
#37768=VERTEX_POINT('',#176248);
#37769=VERTEX_POINT('',#176250);
#37770=VERTEX_POINT('',#176269);
#37771=VERTEX_POINT('',#176273);
#37772=VERTEX_POINT('',#176303);
#37773=VERTEX_POINT('',#176304);
#37774=VERTEX_POINT('',#176322);
#37775=VERTEX_POINT('',#176323);
#37776=VERTEX_POINT('',#176328);
#37777=VERTEX_POINT('',#176401);
#37778=VERTEX_POINT('',#176405);
#37779=VERTEX_POINT('',#176438);
#37780=VERTEX_POINT('',#176564);
#37781=VERTEX_POINT('',#176647);
#37782=VERTEX_POINT('',#176649);
#37783=VERTEX_POINT('',#176653);
#37784=VERTEX_POINT('',#176657);
#37785=VERTEX_POINT('',#176661);
#37786=VERTEX_POINT('',#176665);
#37787=VERTEX_POINT('',#176669);
#37788=VERTEX_POINT('',#176673);
#37789=VERTEX_POINT('',#176677);
#37790=VERTEX_POINT('',#176681);
#37791=VERTEX_POINT('',#176685);
#37792=VERTEX_POINT('',#176689);
#37793=VERTEX_POINT('',#176693);
#37794=VERTEX_POINT('',#176697);
#37795=VERTEX_POINT('',#176698);
#37796=VERTEX_POINT('',#176700);
#37797=VERTEX_POINT('',#176702);
#37798=VERTEX_POINT('',#176748);
#37799=VERTEX_POINT('',#176750);
#37800=VERTEX_POINT('',#176847);
#37801=VERTEX_POINT('',#176880);
#37802=VERTEX_POINT('',#176893);
#37803=VERTEX_POINT('',#176926);
#37804=VERTEX_POINT('',#176980);
#37805=VERTEX_POINT('',#176982);
#37806=VERTEX_POINT('',#176994);
#37807=VERTEX_POINT('',#176996);
#37808=VERTEX_POINT('',#177010);
#37809=VERTEX_POINT('',#177012);
#37810=VERTEX_POINT('',#177016);
#37811=VERTEX_POINT('',#177018);
#37812=VERTEX_POINT('',#177022);
#37813=VERTEX_POINT('',#177026);
#37814=VERTEX_POINT('',#177038);
#37815=VERTEX_POINT('',#177040);
#37816=VERTEX_POINT('',#177054);
#37817=VERTEX_POINT('',#177056);
#37818=VERTEX_POINT('',#177060);
#37819=VERTEX_POINT('',#177062);
#37820=VERTEX_POINT('',#177066);
#37821=VERTEX_POINT('',#177070);
#37822=VERTEX_POINT('',#177082);
#37823=VERTEX_POINT('',#177084);
#37824=VERTEX_POINT('',#177088);
#37825=VERTEX_POINT('',#177210);
#37826=VERTEX_POINT('',#177311);
#37827=VERTEX_POINT('',#177359);
#37828=VERTEX_POINT('',#177360);
#37829=VERTEX_POINT('',#177365);
#37830=VERTEX_POINT('',#177366);
#37831=VERTEX_POINT('',#177368);
#37832=VERTEX_POINT('',#177370);
#37833=VERTEX_POINT('',#177374);
#37834=VERTEX_POINT('',#177376);
#37835=VERTEX_POINT('',#177380);
#37836=VERTEX_POINT('',#177382);
#37837=VERTEX_POINT('',#177421);
#37838=VERTEX_POINT('',#177456);
#37839=VERTEX_POINT('',#177458);
#37840=VERTEX_POINT('',#177514);
#37841=VERTEX_POINT('',#177516);
#37842=VERTEX_POINT('',#177578);
#37843=VERTEX_POINT('',#177587);
#37844=VERTEX_POINT('',#177588);
#37845=VERTEX_POINT('',#177590);
#37846=VERTEX_POINT('',#177592);
#37847=VERTEX_POINT('',#177596);
#37848=VERTEX_POINT('',#177598);
#37849=VERTEX_POINT('',#177605);
#37850=VERTEX_POINT('',#177607);
#37851=VERTEX_POINT('',#177628);
#37852=VERTEX_POINT('',#177630);
#37853=VERTEX_POINT('',#177690);
#37854=VERTEX_POINT('',#177727);
#37855=VERTEX_POINT('',#177732);
#37856=VERTEX_POINT('',#177818);
#37857=VERTEX_POINT('',#177837);
#37858=VERTEX_POINT('',#177841);
#37859=VERTEX_POINT('',#177845);
#37860=VERTEX_POINT('',#177847);
#37861=VERTEX_POINT('',#177853);
#37862=VERTEX_POINT('',#177855);
#37863=VERTEX_POINT('',#177859);
#37864=VERTEX_POINT('',#177861);
#37865=VERTEX_POINT('',#177866);
#37866=VERTEX_POINT('',#177869);
#37867=VERTEX_POINT('',#177873);
#37868=VERTEX_POINT('',#177874);
#37869=VERTEX_POINT('',#177879);
#37870=VERTEX_POINT('',#177881);
#37871=VERTEX_POINT('',#177883);
#37872=VERTEX_POINT('',#177895);
#37873=VERTEX_POINT('',#177899);
#37874=VERTEX_POINT('',#177911);
#37875=VERTEX_POINT('',#177918);
#37876=VERTEX_POINT('',#177923);
#37877=VERTEX_POINT('',#177926);
#37878=VERTEX_POINT('',#177930);
#37879=VERTEX_POINT('',#177932);
#37880=VERTEX_POINT('',#177936);
#37881=VERTEX_POINT('',#177940);
#37882=VERTEX_POINT('',#177951);
#37883=VERTEX_POINT('',#177984);
#37884=VERTEX_POINT('',#178058);
#37885=VERTEX_POINT('',#178062);
#37886=VERTEX_POINT('',#178120);
#37887=VERTEX_POINT('',#178124);
#37888=VERTEX_POINT('',#178173);
#37889=VERTEX_POINT('',#178218);
#37890=VERTEX_POINT('',#178322);
#37891=VERTEX_POINT('',#178323);
#37892=VERTEX_POINT('',#178409);
#37893=VERTEX_POINT('',#178413);
#37894=VERTEX_POINT('',#178471);
#37895=VERTEX_POINT('',#178475);
#37896=VERTEX_POINT('',#178524);
#37897=VERTEX_POINT('',#178566);
#37898=VERTEX_POINT('',#178639);
#37899=VERTEX_POINT('',#178641);
#37900=VERTEX_POINT('',#178692);
#37901=VERTEX_POINT('',#178821);
#37902=VERTEX_POINT('',#178832);
#37903=VERTEX_POINT('',#178836);
#37904=VERTEX_POINT('',#178888);
#37905=VERTEX_POINT('',#178892);
#37906=VERTEX_POINT('',#178947);
#37907=VERTEX_POINT('',#178989);
#37908=VERTEX_POINT('',#179068);
#37909=VERTEX_POINT('',#179072);
#37910=VERTEX_POINT('',#179123);
#37911=VERTEX_POINT('',#179124);
#37912=VERTEX_POINT('',#179171);
#37913=VERTEX_POINT('',#179175);
#37914=VERTEX_POINT('',#179186);
#37915=VERTEX_POINT('',#179219);
#37916=VERTEX_POINT('',#179292);
#37917=VERTEX_POINT('',#179344);
#37918=VERTEX_POINT('',#179348);
#37919=VERTEX_POINT('',#179403);
#37920=VERTEX_POINT('',#179445);
#37921=VERTEX_POINT('',#179547);
#37922=VERTEX_POINT('',#179629);
#37923=VERTEX_POINT('',#179640);
#37924=VERTEX_POINT('',#179644);
#37925=VERTEX_POINT('',#179702);
#37926=VERTEX_POINT('',#179706);
#37927=VERTEX_POINT('',#179755);
#37928=VERTEX_POINT('',#179800);
#37929=VERTEX_POINT('',#179908);
#37930=VERTEX_POINT('',#179909);
#37931=VERTEX_POINT('',#180022);
#37932=VERTEX_POINT('',#180027);
#37933=VERTEX_POINT('',#180085);
#37934=VERTEX_POINT('',#180089);
#37935=VERTEX_POINT('',#180138);
#37936=VERTEX_POINT('',#180181);
#37937=VERTEX_POINT('',#180286);
#37938=VERTEX_POINT('',#180361);
#37939=VERTEX_POINT('',#180372);
#37940=VERTEX_POINT('',#180376);
#37941=VERTEX_POINT('',#180428);
#37942=VERTEX_POINT('',#180432);
#37943=VERTEX_POINT('',#180487);
#37944=VERTEX_POINT('',#180529);
#37945=VERTEX_POINT('',#180608);
#37946=VERTEX_POINT('',#180634);
#37947=VERTEX_POINT('',#180666);
#37948=VERTEX_POINT('',#180687);
#37949=VERTEX_POINT('',#180735);
#37950=VERTEX_POINT('',#180736);
#37951=VERTEX_POINT('',#180819);
#37952=VERTEX_POINT('',#180823);
#37953=VERTEX_POINT('',#180875);
#37954=VERTEX_POINT('',#180879);
#37955=VERTEX_POINT('',#180934);
#37956=VERTEX_POINT('',#180976);
#37957=VERTEX_POINT('',#181078);
#37958=VERTEX_POINT('',#181159);
#37959=VERTEX_POINT('',#181161);
#37960=VERTEX_POINT('',#181176);
#37961=VERTEX_POINT('',#181182);
#37962=VERTEX_POINT('',#181184);
#37963=VERTEX_POINT('',#181199);
#37964=VERTEX_POINT('',#181203);
#37965=VERTEX_POINT('',#181224);
#37966=VERTEX_POINT('',#181228);
#37967=VERTEX_POINT('',#181283);
#37968=VERTEX_POINT('',#181298);
#37969=VERTEX_POINT('',#181304);
#37970=VERTEX_POINT('',#181306);
#37971=VERTEX_POINT('',#181357);
#37972=VERTEX_POINT('',#181402);
#37973=VERTEX_POINT('',#181459);
#37974=VERTEX_POINT('',#181633);
#37975=VERTEX_POINT('',#181730);
#37976=VERTEX_POINT('',#181745);
#37977=VERTEX_POINT('',#181751);
#37978=VERTEX_POINT('',#181753);
#37979=VERTEX_POINT('',#181795);
#37980=VERTEX_POINT('',#181828);
#37981=VERTEX_POINT('',#181954);
#37982=VERTEX_POINT('',#182047);
#37983=VERTEX_POINT('',#182147);
#37984=VERTEX_POINT('',#182162);
#37985=VERTEX_POINT('',#182168);
#37986=VERTEX_POINT('',#182170);
#37987=VERTEX_POINT('',#182221);
#37988=VERTEX_POINT('',#182266);
#37989=VERTEX_POINT('',#182385);
#37990=VERTEX_POINT('',#182461);
#37991=VERTEX_POINT('',#182579);
#37992=VERTEX_POINT('',#182594);
#37993=VERTEX_POINT('',#182600);
#37994=VERTEX_POINT('',#182602);
#37995=VERTEX_POINT('',#182617);
#37996=VERTEX_POINT('',#182621);
#37997=VERTEX_POINT('',#182673);
#37998=VERTEX_POINT('',#182677);
#37999=VERTEX_POINT('',#182756);
#38000=VERTEX_POINT('',#182771);
#38001=VERTEX_POINT('',#182788);
#38002=VERTEX_POINT('',#182789);
#38003=VERTEX_POINT('',#182806);
#38004=VERTEX_POINT('',#182810);
#38005=VERTEX_POINT('',#182854);
#38006=VERTEX_POINT('',#182861);
#38007=VERTEX_POINT('',#182865);
#38008=VERTEX_POINT('',#182881);
#38009=VERTEX_POINT('',#182883);
#38010=VERTEX_POINT('',#182920);
#38011=VERTEX_POINT('',#182924);
#38012=VERTEX_POINT('',#182979);
#38013=VERTEX_POINT('',#182980);
#38014=VERTEX_POINT('',#182982);
#38015=VERTEX_POINT('',#183012);
#38016=VERTEX_POINT('',#183014);
#38017=VERTEX_POINT('',#183055);
#38018=VERTEX_POINT('',#183223);
#38019=VERTEX_POINT('',#183355);
#38020=VERTEX_POINT('',#183458);
#38021=VERTEX_POINT('',#183474);
#38022=VERTEX_POINT('',#183481);
#38023=VERTEX_POINT('',#183483);
#38024=VERTEX_POINT('',#183559);
#38025=VERTEX_POINT('',#183598);
#38026=VERTEX_POINT('',#183781);
#38027=VERTEX_POINT('',#183907);
#38028=VERTEX_POINT('',#184037);
#38029=VERTEX_POINT('',#184053);
#38030=VERTEX_POINT('',#184070);
#38031=VERTEX_POINT('',#184071);
#38032=VERTEX_POINT('',#184076);
#38033=VERTEX_POINT('',#184081);
#38034=VERTEX_POINT('',#184166);
#38035=VERTEX_POINT('',#184170);
#38036=VERTEX_POINT('',#184189);
#38037=VERTEX_POINT('',#184205);
#38038=VERTEX_POINT('',#184224);
#38039=VERTEX_POINT('',#184226);
#38040=VERTEX_POINT('',#184293);
#38041=VERTEX_POINT('',#184295);
#38042=VERTEX_POINT('',#184368);
#38043=VERTEX_POINT('',#184384);
#38044=VERTEX_POINT('',#184391);
#38045=VERTEX_POINT('',#184393);
#38046=VERTEX_POINT('',#184408);
#38047=VERTEX_POINT('',#184412);
#38048=VERTEX_POINT('',#184433);
#38049=VERTEX_POINT('',#184437);
#38050=VERTEX_POINT('',#184492);
#38051=VERTEX_POINT('',#184508);
#38052=VERTEX_POINT('',#184510);
#38053=VERTEX_POINT('',#184517);
#38054=VERTEX_POINT('',#184519);
#38055=VERTEX_POINT('',#184579);
#38056=VERTEX_POINT('',#184618);
#38057=VERTEX_POINT('',#184777);
#38058=VERTEX_POINT('',#184909);
#38059=VERTEX_POINT('',#185012);
#38060=VERTEX_POINT('',#185028);
#38061=VERTEX_POINT('',#185030);
#38062=VERTEX_POINT('',#185036);
#38063=VERTEX_POINT('',#185037);
#38064=VERTEX_POINT('',#185067);
#38065=VERTEX_POINT('',#185069);
#38066=VERTEX_POINT('',#185071);
#38067=VERTEX_POINT('',#185122);
#38068=VERTEX_POINT('',#185161);
#38069=VERTEX_POINT('',#185226);
#38070=VERTEX_POINT('',#185272);
#38071=VERTEX_POINT('',#185305);
#38072=VERTEX_POINT('',#185420);
#38073=VERTEX_POINT('',#185422);
#38074=VERTEX_POINT('',#185469);
#38075=VERTEX_POINT('',#185502);
#38076=VERTEX_POINT('',#185504);
#38077=VERTEX_POINT('',#185529);
#38078=VERTEX_POINT('',#185562);
#38079=VERTEX_POINT('',#185628);
#38080=VERTEX_POINT('',#185655);
#38081=VERTEX_POINT('',#185687);
#38082=VERTEX_POINT('',#185708);
#38083=VERTEX_POINT('',#185733);
#38084=VERTEX_POINT('',#185766);
#38085=VERTEX_POINT('',#185819);
#38086=VERTEX_POINT('',#185896);
#38087=VERTEX_POINT('',#185900);
#38088=VERTEX_POINT('',#185904);
#38089=VERTEX_POINT('',#185906);
#38090=VERTEX_POINT('',#185910);
#38091=VERTEX_POINT('',#185914);
#38092=VERTEX_POINT('',#185918);
#38093=VERTEX_POINT('',#185922);
#38094=VERTEX_POINT('',#185926);
#38095=VERTEX_POINT('',#185930);
#38096=VERTEX_POINT('',#185934);
#38097=VERTEX_POINT('',#185938);
#38098=VERTEX_POINT('',#185942);
#38099=VERTEX_POINT('',#185946);
#38100=VERTEX_POINT('',#185950);
#38101=VERTEX_POINT('',#185954);
#38102=VERTEX_POINT('',#185958);
#38103=VERTEX_POINT('',#185962);
#38104=VERTEX_POINT('',#185964);
#38105=VERTEX_POINT('',#185968);
#38106=VERTEX_POINT('',#185972);
#38107=VERTEX_POINT('',#185976);
#38108=VERTEX_POINT('',#185980);
#38109=VERTEX_POINT('',#185982);
#38110=VERTEX_POINT('',#185986);
#38111=VERTEX_POINT('',#185990);
#38112=VERTEX_POINT('',#185996);
#38113=VERTEX_POINT('',#186000);
#38114=VERTEX_POINT('',#186004);
#38115=VERTEX_POINT('',#186008);
#38116=VERTEX_POINT('',#186016);
#38117=VERTEX_POINT('',#186020);
#38118=VERTEX_POINT('',#186024);
#38119=VERTEX_POINT('',#186028);
#38120=VERTEX_POINT('',#186034);
#38121=VERTEX_POINT('',#186055);
#38122=VERTEX_POINT('',#186066);
#38123=VERTEX_POINT('',#186070);
#38124=VERTEX_POINT('',#186074);
#38125=VERTEX_POINT('',#186078);
#38126=VERTEX_POINT('',#186086);
#38127=VERTEX_POINT('',#186090);
#38128=VERTEX_POINT('',#186094);
#38129=VERTEX_POINT('',#186098);
#38130=VERTEX_POINT('',#186102);
#38131=VERTEX_POINT('',#186106);
#38132=VERTEX_POINT('',#186110);
#38133=VERTEX_POINT('',#186157);
#38134=VERTEX_POINT('',#186159);
#38135=VERTEX_POINT('',#186246);
#38136=VERTEX_POINT('',#186270);
#38137=VERTEX_POINT('',#186274);
#38138=VERTEX_POINT('',#186312);
#38139=VERTEX_POINT('',#186328);
#38140=VERTEX_POINT('',#186332);
#38141=VERTEX_POINT('',#186334);
#38142=VERTEX_POINT('',#186336);
#38143=VERTEX_POINT('',#186338);
#38144=VERTEX_POINT('',#186342);
#38145=VERTEX_POINT('',#186344);
#38146=VERTEX_POINT('',#186346);
#38147=VERTEX_POINT('',#186348);
#38148=VERTEX_POINT('',#186352);
#38149=VERTEX_POINT('',#186356);
#38150=VERTEX_POINT('',#186358);
#38151=VERTEX_POINT('',#186379);
#38152=VERTEX_POINT('',#186389);
#38153=VERTEX_POINT('',#186410);
#38154=VERTEX_POINT('',#186424);
#38155=VERTEX_POINT('',#186445);
#38156=VERTEX_POINT('',#186455);
#38157=VERTEX_POINT('',#186476);
#38158=VERTEX_POINT('',#186488);
#38159=VERTEX_POINT('',#186503);
#38160=VERTEX_POINT('',#186505);
#38161=VERTEX_POINT('',#186548);
#38162=VERTEX_POINT('',#186569);
#38163=VERTEX_POINT('',#186579);
#38164=VERTEX_POINT('',#186600);
#38165=VERTEX_POINT('',#186612);
#38166=VERTEX_POINT('',#186653);
#38167=VERTEX_POINT('',#186668);
#38168=VERTEX_POINT('',#186672);
#38169=VERTEX_POINT('',#186676);
#38170=VERTEX_POINT('',#186697);
#38171=VERTEX_POINT('',#186707);
#38172=VERTEX_POINT('',#186728);
#38173=VERTEX_POINT('',#186742);
#38174=VERTEX_POINT('',#186744);
#38175=VERTEX_POINT('',#186748);
#38176=VERTEX_POINT('',#186769);
#38177=VERTEX_POINT('',#186779);
#38178=VERTEX_POINT('',#186800);
#38179=VERTEX_POINT('',#186812);
#38180=VERTEX_POINT('',#186833);
#38181=VERTEX_POINT('',#186852);
#38182=VERTEX_POINT('',#186873);
#38183=VERTEX_POINT('',#186883);
#38184=VERTEX_POINT('',#186904);
#38185=VERTEX_POINT('',#186935);
#38186=VERTEX_POINT('',#186996);
#38187=VERTEX_POINT('',#186998);
#38188=VERTEX_POINT('',#187002);
#38189=VERTEX_POINT('',#187023);
#38190=VERTEX_POINT('',#187033);
#38191=VERTEX_POINT('',#187054);
#38192=VERTEX_POINT('',#187066);
#38193=VERTEX_POINT('',#187107);
#38194=VERTEX_POINT('',#187128);
#38195=VERTEX_POINT('',#187168);
#38196=VERTEX_POINT('',#187172);
#38197=VERTEX_POINT('',#187193);
#38198=VERTEX_POINT('',#187203);
#38199=VERTEX_POINT('',#187224);
#38200=VERTEX_POINT('',#187261);
#38201=VERTEX_POINT('',#187263);
#38202=VERTEX_POINT('',#187337);
#38203=VERTEX_POINT('',#187370);
#38204=VERTEX_POINT('',#187416);
#38205=VERTEX_POINT('',#187437);
#38206=VERTEX_POINT('',#187463);
#38207=VERTEX_POINT('',#187490);
#38208=VERTEX_POINT('',#187532);
#38209=VERTEX_POINT('',#187565);
#38210=VERTEX_POINT('',#187624);
#38211=VERTEX_POINT('',#187657);
#38212=VERTEX_POINT('',#187688);
#38213=VERTEX_POINT('',#187721);
#38214=VERTEX_POINT('',#187750);
#38215=VERTEX_POINT('',#187789);
#38216=VERTEX_POINT('',#187846);
#38217=VERTEX_POINT('',#187879);
#38218=VERTEX_POINT('',#187932);
#38219=VERTEX_POINT('',#187965);
#38220=VERTEX_POINT('',#188011);
#38221=VERTEX_POINT('',#188038);
#38222=VERTEX_POINT('',#188106);
#38223=VERTEX_POINT('',#188127);
#38224=VERTEX_POINT('',#188182);
#38225=VERTEX_POINT('',#188184);
#38226=VERTEX_POINT('',#188190);
#38227=VERTEX_POINT('',#188192);
#38228=VERTEX_POINT('',#188200);
#38229=VERTEX_POINT('',#188202);
#38230=VERTEX_POINT('',#188225);
#38231=VERTEX_POINT('',#188239);
#38232=VERTEX_POINT('',#188256);
#38233=VERTEX_POINT('',#188257);
#38234=VERTEX_POINT('',#188275);
#38235=VERTEX_POINT('',#188285);
#38236=VERTEX_POINT('',#188332);
#38237=VERTEX_POINT('',#188371);
#38238=VERTEX_POINT('',#188428);
#38239=VERTEX_POINT('',#188461);
#38240=VERTEX_POINT('',#188480);
#38241=VERTEX_POINT('',#188501);
#38242=VERTEX_POINT('',#188527);
#38243=VERTEX_POINT('',#188560);
#38244=VERTEX_POINT('',#188610);
#38245=VERTEX_POINT('',#188643);
#38246=VERTEX_POINT('',#188692);
#38247=VERTEX_POINT('',#188713);
#38248=VERTEX_POINT('',#188734);
#38249=VERTEX_POINT('',#188738);
#38250=VERTEX_POINT('',#188740);
#38251=VERTEX_POINT('',#188773);
#38252=VERTEX_POINT('',#188823);
#38253=VERTEX_POINT('',#188856);
#38254=VERTEX_POINT('',#188902);
#38255=VERTEX_POINT('',#188923);
#38256=VERTEX_POINT('',#188949);
#38257=VERTEX_POINT('',#188982);
#38258=VERTEX_POINT('',#189033);
#38259=VERTEX_POINT('',#189066);
#38260=VERTEX_POINT('',#189067);
#38261=VERTEX_POINT('',#189121);
#38262=VERTEX_POINT('',#189148);
#38263=VERTEX_POINT('',#189166);
#38264=VERTEX_POINT('',#189171);
#38265=VERTEX_POINT('',#189173);
#38266=VERTEX_POINT('',#189179);
#38267=VERTEX_POINT('',#189181);
#38268=VERTEX_POINT('',#189189);
#38269=VERTEX_POINT('',#189191);
#38270=VERTEX_POINT('',#189208);
#38271=VERTEX_POINT('',#189311);
#38272=VERTEX_POINT('',#189312);
#38273=VERTEX_POINT('',#189314);
#38274=VERTEX_POINT('',#189318);
#38275=VERTEX_POINT('',#189324);
#38276=VERTEX_POINT('',#189325);
#38277=VERTEX_POINT('',#189334);
#38278=VERTEX_POINT('',#189335);
#38279=VERTEX_POINT('',#189344);
#38280=VERTEX_POINT('',#189345);
#38281=VERTEX_POINT('',#189354);
#38282=VERTEX_POINT('',#189355);
#38283=VERTEX_POINT('',#189371);
#38284=VERTEX_POINT('',#189386);
#38285=VERTEX_POINT('',#189388);
#38286=VERTEX_POINT('',#189390);
#38287=VERTEX_POINT('',#189394);
#38288=VERTEX_POINT('',#189400);
#38289=VERTEX_POINT('',#189402);
#38290=VERTEX_POINT('',#189407);
#38291=VERTEX_POINT('',#189411);
#38292=VERTEX_POINT('',#189414);
#38293=VERTEX_POINT('',#189436);
#38294=VERTEX_POINT('',#189437);
#38295=VERTEX_POINT('',#189439);
#38296=VERTEX_POINT('',#189446);
#38297=VERTEX_POINT('',#189455);
#38298=VERTEX_POINT('',#189457);
#38299=VERTEX_POINT('',#189459);
#38300=VERTEX_POINT('',#189492);
#38301=VERTEX_POINT('',#189493);
#38302=VERTEX_POINT('',#189495);
#38303=VERTEX_POINT('',#189527);
#38304=VERTEX_POINT('',#189551);
#38305=VERTEX_POINT('',#189552);
#38306=VERTEX_POINT('',#189578);
#38307=VERTEX_POINT('',#189611);
#38308=VERTEX_POINT('',#189612);
#38309=VERTEX_POINT('',#189677);
#38310=VERTEX_POINT('',#189678);
#38311=VERTEX_POINT('',#189700);
#38312=VERTEX_POINT('',#189701);
#38313=VERTEX_POINT('',#189717);
#38314=VERTEX_POINT('',#189718);
#38315=VERTEX_POINT('',#189752);
#38316=VERTEX_POINT('',#189753);
#38317=VERTEX_POINT('',#189815);
#38318=VERTEX_POINT('',#189816);
#38319=VERTEX_POINT('',#189832);
#38320=VERTEX_POINT('',#189833);
#38321=VERTEX_POINT('',#189855);
#38322=VERTEX_POINT('',#189856);
#38323=VERTEX_POINT('',#189884);
#38324=VERTEX_POINT('',#189886);
#38325=VERTEX_POINT('',#189957);
#38326=VERTEX_POINT('',#189958);
#38327=VERTEX_POINT('',#189960);
#38328=VERTEX_POINT('',#189973);
#38329=VERTEX_POINT('',#190042);
#38330=VERTEX_POINT('',#190043);
#38331=VERTEX_POINT('',#190080);
#38332=VERTEX_POINT('',#190081);
#38333=VERTEX_POINT('',#190133);
#38334=VERTEX_POINT('',#190134);
#38335=VERTEX_POINT('',#190178);
#38336=VERTEX_POINT('',#190179);
#38337=VERTEX_POINT('',#190244);
#38338=VERTEX_POINT('',#190259);
#38339=VERTEX_POINT('',#190260);
#38340=VERTEX_POINT('',#190297);
#38341=VERTEX_POINT('',#190298);
#38342=VERTEX_POINT('',#190332);
#38343=VERTEX_POINT('',#190333);
#38344=VERTEX_POINT('',#190352);
#38345=VERTEX_POINT('',#190353);
#38346=VERTEX_POINT('',#190358);
#38347=VERTEX_POINT('',#190362);
#38348=VERTEX_POINT('',#190363);
#38349=VERTEX_POINT('',#190379);
#38350=VERTEX_POINT('',#190380);
#38351=VERTEX_POINT('',#190394);
#38352=VERTEX_POINT('',#190395);
#38353=VERTEX_POINT('',#190397);
#38354=VERTEX_POINT('',#190399);
#38355=VERTEX_POINT('',#190403);
#38356=VERTEX_POINT('',#190404);
#38357=VERTEX_POINT('',#190409);
#38358=VERTEX_POINT('',#190410);
#38359=VERTEX_POINT('',#190415);
#38360=VERTEX_POINT('',#190416);
#38361=VERTEX_POINT('',#190421);
#38362=VERTEX_POINT('',#190422);
#38363=VERTEX_POINT('',#190427);
#38364=VERTEX_POINT('',#190428);
#38365=VERTEX_POINT('',#190433);
#38366=VERTEX_POINT('',#190434);
#38367=VERTEX_POINT('',#190450);
#38368=VERTEX_POINT('',#190452);
#38369=VERTEX_POINT('',#190467);
#38370=VERTEX_POINT('',#190468);
#38371=VERTEX_POINT('',#190511);
#38372=VERTEX_POINT('',#190524);
#38373=VERTEX_POINT('',#190574);
#38374=VERTEX_POINT('',#190575);
#38375=VERTEX_POINT('',#190635);
#38376=VERTEX_POINT('',#190636);
#38377=VERTEX_POINT('',#190652);
#38378=VERTEX_POINT('',#190653);
#38379=VERTEX_POINT('',#190669);
#38380=VERTEX_POINT('',#190670);
#38381=VERTEX_POINT('',#190707);
#38382=VERTEX_POINT('',#190708);
#38383=VERTEX_POINT('',#190757);
#38384=VERTEX_POINT('',#190758);
#38385=VERTEX_POINT('',#190800);
#38386=VERTEX_POINT('',#190801);
#38387=VERTEX_POINT('',#190873);
#38388=VERTEX_POINT('',#190874);
#38389=VERTEX_POINT('',#190966);
#38390=VERTEX_POINT('',#190967);
#38391=VERTEX_POINT('',#191069);
#38392=VERTEX_POINT('',#191070);
#38393=VERTEX_POINT('',#191072);
#38394=VERTEX_POINT('',#191091);
#38395=VERTEX_POINT('',#191112);
#38396=VERTEX_POINT('',#191113);
#38397=VERTEX_POINT('',#191141);
#38398=VERTEX_POINT('',#191142);
#38399=VERTEX_POINT('',#191214);
#38400=VERTEX_POINT('',#191215);
#38401=VERTEX_POINT('',#191272);
#38402=VERTEX_POINT('',#191273);
#38403=VERTEX_POINT('',#191319);
#38404=VERTEX_POINT('',#191320);
#38405=VERTEX_POINT('',#191322);
#38406=VERTEX_POINT('',#191360);
#38407=VERTEX_POINT('',#191361);
#38408=VERTEX_POINT('',#191377);
#38409=VERTEX_POINT('',#191378);
#38410=VERTEX_POINT('',#191549);
#38411=VERTEX_POINT('',#191550);
#38412=VERTEX_POINT('',#191637);
#38413=VERTEX_POINT('',#191639);
#38414=VERTEX_POINT('',#191651);
#38415=VERTEX_POINT('',#191653);
#38416=VERTEX_POINT('',#191657);
#38417=VERTEX_POINT('',#191659);
#38418=VERTEX_POINT('',#191672);
#38419=VERTEX_POINT('',#191673);
#38420=VERTEX_POINT('',#191681);
#38421=VERTEX_POINT('',#191683);
#38422=VERTEX_POINT('',#191695);
#38423=VERTEX_POINT('',#191697);
#38424=VERTEX_POINT('',#191701);
#38425=VERTEX_POINT('',#191702);
#38426=VERTEX_POINT('',#191715);
#38427=VERTEX_POINT('',#191716);
#38428=VERTEX_POINT('',#191724);
#38429=VERTEX_POINT('',#191726);
#38430=VERTEX_POINT('',#191738);
#38431=VERTEX_POINT('',#191739);
#38432=VERTEX_POINT('',#191744);
#38433=VERTEX_POINT('',#191745);
#38434=VERTEX_POINT('',#191758);
#38435=VERTEX_POINT('',#191760);
#38436=VERTEX_POINT('',#191767);
#38437=VERTEX_POINT('',#191769);
#38438=VERTEX_POINT('',#191781);
#38439=VERTEX_POINT('',#191782);
#38440=VERTEX_POINT('',#191787);
#38441=VERTEX_POINT('',#191788);
#38442=VERTEX_POINT('',#191801);
#38443=VERTEX_POINT('',#191803);
#38444=VERTEX_POINT('',#191834);
#38445=VERTEX_POINT('',#191835);
#38446=VERTEX_POINT('',#191837);
#38447=VERTEX_POINT('',#191839);
#38448=VERTEX_POINT('',#191843);
#38449=VERTEX_POINT('',#191844);
#38450=VERTEX_POINT('',#191849);
#38451=VERTEX_POINT('',#191850);
#38452=VERTEX_POINT('',#191855);
#38453=VERTEX_POINT('',#191856);
#38454=VERTEX_POINT('',#191861);
#38455=VERTEX_POINT('',#191862);
#38456=VERTEX_POINT('',#191867);
#38457=VERTEX_POINT('',#191868);
#38458=VERTEX_POINT('',#191873);
#38459=VERTEX_POINT('',#191874);
#38460=VERTEX_POINT('',#191879);
#38461=VERTEX_POINT('',#191880);
#38462=VERTEX_POINT('',#191885);
#38463=VERTEX_POINT('',#191886);
#38464=VERTEX_POINT('',#191894);
#38465=VERTEX_POINT('',#191895);
#38466=VERTEX_POINT('',#191897);
#38467=VERTEX_POINT('',#191899);
#38468=VERTEX_POINT('',#191903);
#38469=VERTEX_POINT('',#191904);
#38470=VERTEX_POINT('',#191909);
#38471=VERTEX_POINT('',#191910);
#38472=VERTEX_POINT('',#191915);
#38473=VERTEX_POINT('',#191916);
#38474=VERTEX_POINT('',#191921);
#38475=VERTEX_POINT('',#191922);
#38476=VERTEX_POINT('',#191927);
#38477=VERTEX_POINT('',#191928);
#38478=VERTEX_POINT('',#191933);
#38479=VERTEX_POINT('',#191934);
#38480=VERTEX_POINT('',#191942);
#38481=VERTEX_POINT('',#191943);
#38482=VERTEX_POINT('',#191945);
#38483=VERTEX_POINT('',#191947);
#38484=VERTEX_POINT('',#191951);
#38485=VERTEX_POINT('',#191952);
#38486=VERTEX_POINT('',#191957);
#38487=VERTEX_POINT('',#191958);
#38488=VERTEX_POINT('',#191963);
#38489=VERTEX_POINT('',#191964);
#38490=VERTEX_POINT('',#191969);
#38491=VERTEX_POINT('',#191970);
#38492=VERTEX_POINT('',#191975);
#38493=VERTEX_POINT('',#191976);
#38494=VERTEX_POINT('',#191981);
#38495=VERTEX_POINT('',#191982);
#38496=VERTEX_POINT('',#191990);
#38497=VERTEX_POINT('',#191991);
#38498=VERTEX_POINT('',#191993);
#38499=VERTEX_POINT('',#191995);
#38500=VERTEX_POINT('',#191999);
#38501=VERTEX_POINT('',#192000);
#38502=VERTEX_POINT('',#192005);
#38503=VERTEX_POINT('',#192006);
#38504=VERTEX_POINT('',#192011);
#38505=VERTEX_POINT('',#192012);
#38506=VERTEX_POINT('',#192017);
#38507=VERTEX_POINT('',#192018);
#38508=VERTEX_POINT('',#192023);
#38509=VERTEX_POINT('',#192024);
#38510=VERTEX_POINT('',#192029);
#38511=VERTEX_POINT('',#192030);
#38512=VERTEX_POINT('',#192038);
#38513=VERTEX_POINT('',#192039);
#38514=VERTEX_POINT('',#192041);
#38515=VERTEX_POINT('',#192043);
#38516=VERTEX_POINT('',#192047);
#38517=VERTEX_POINT('',#192048);
#38518=VERTEX_POINT('',#192053);
#38519=VERTEX_POINT('',#192054);
#38520=VERTEX_POINT('',#192059);
#38521=VERTEX_POINT('',#192060);
#38522=VERTEX_POINT('',#192065);
#38523=VERTEX_POINT('',#192066);
#38524=VERTEX_POINT('',#192071);
#38525=VERTEX_POINT('',#192072);
#38526=VERTEX_POINT('',#192077);
#38527=VERTEX_POINT('',#192078);
#38528=VERTEX_POINT('',#192083);
#38529=VERTEX_POINT('',#192084);
#38530=VERTEX_POINT('',#192092);
#38531=VERTEX_POINT('',#192093);
#38532=VERTEX_POINT('',#192095);
#38533=VERTEX_POINT('',#192097);
#38534=VERTEX_POINT('',#192101);
#38535=VERTEX_POINT('',#192102);
#38536=VERTEX_POINT('',#192107);
#38537=VERTEX_POINT('',#192108);
#38538=VERTEX_POINT('',#192113);
#38539=VERTEX_POINT('',#192114);
#38540=VERTEX_POINT('',#192119);
#38541=VERTEX_POINT('',#192120);
#38542=VERTEX_POINT('',#192125);
#38543=VERTEX_POINT('',#192126);
#38544=VERTEX_POINT('',#192131);
#38545=VERTEX_POINT('',#192132);
#38546=VERTEX_POINT('',#192140);
#38547=VERTEX_POINT('',#192141);
#38548=VERTEX_POINT('',#192143);
#38549=VERTEX_POINT('',#192145);
#38550=VERTEX_POINT('',#192149);
#38551=VERTEX_POINT('',#192150);
#38552=VERTEX_POINT('',#192155);
#38553=VERTEX_POINT('',#192156);
#38554=VERTEX_POINT('',#192161);
#38555=VERTEX_POINT('',#192162);
#38556=VERTEX_POINT('',#192167);
#38557=VERTEX_POINT('',#192168);
#38558=VERTEX_POINT('',#192173);
#38559=VERTEX_POINT('',#192174);
#38560=VERTEX_POINT('',#192179);
#38561=VERTEX_POINT('',#192180);
#38562=VERTEX_POINT('',#192188);
#38563=VERTEX_POINT('',#192189);
#38564=VERTEX_POINT('',#192191);
#38565=VERTEX_POINT('',#192193);
#38566=VERTEX_POINT('',#192197);
#38567=VERTEX_POINT('',#192198);
#38568=VERTEX_POINT('',#192203);
#38569=VERTEX_POINT('',#192204);
#38570=VERTEX_POINT('',#192209);
#38571=VERTEX_POINT('',#192210);
#38572=VERTEX_POINT('',#192215);
#38573=VERTEX_POINT('',#192216);
#38574=VERTEX_POINT('',#192221);
#38575=VERTEX_POINT('',#192222);
#38576=VERTEX_POINT('',#192227);
#38577=VERTEX_POINT('',#192228);
#38578=VERTEX_POINT('',#192236);
#38579=VERTEX_POINT('',#192237);
#38580=VERTEX_POINT('',#192239);
#38581=VERTEX_POINT('',#192241);
#38582=VERTEX_POINT('',#192245);
#38583=VERTEX_POINT('',#192246);
#38584=VERTEX_POINT('',#192251);
#38585=VERTEX_POINT('',#192252);
#38586=VERTEX_POINT('',#192257);
#38587=VERTEX_POINT('',#192258);
#38588=VERTEX_POINT('',#192263);
#38589=VERTEX_POINT('',#192264);
#38590=VERTEX_POINT('',#192269);
#38591=VERTEX_POINT('',#192270);
#38592=VERTEX_POINT('',#192275);
#38593=VERTEX_POINT('',#192276);
#38594=VERTEX_POINT('',#192284);
#38595=VERTEX_POINT('',#192285);
#38596=VERTEX_POINT('',#192287);
#38597=VERTEX_POINT('',#192289);
#38598=VERTEX_POINT('',#192293);
#38599=VERTEX_POINT('',#192294);
#38600=VERTEX_POINT('',#192299);
#38601=VERTEX_POINT('',#192300);
#38602=VERTEX_POINT('',#192305);
#38603=VERTEX_POINT('',#192306);
#38604=VERTEX_POINT('',#192311);
#38605=VERTEX_POINT('',#192312);
#38606=VERTEX_POINT('',#192317);
#38607=VERTEX_POINT('',#192318);
#38608=VERTEX_POINT('',#192323);
#38609=VERTEX_POINT('',#192324);
#38610=VERTEX_POINT('',#192332);
#38611=VERTEX_POINT('',#192333);
#38612=VERTEX_POINT('',#192335);
#38613=VERTEX_POINT('',#192337);
#38614=VERTEX_POINT('',#192341);
#38615=VERTEX_POINT('',#192342);
#38616=VERTEX_POINT('',#192347);
#38617=VERTEX_POINT('',#192348);
#38618=VERTEX_POINT('',#192353);
#38619=VERTEX_POINT('',#192354);
#38620=VERTEX_POINT('',#192359);
#38621=VERTEX_POINT('',#192360);
#38622=VERTEX_POINT('',#192365);
#38623=VERTEX_POINT('',#192366);
#38624=VERTEX_POINT('',#192371);
#38625=VERTEX_POINT('',#192372);
#38626=VERTEX_POINT('',#192377);
#38627=VERTEX_POINT('',#192378);
#38628=VERTEX_POINT('',#192383);
#38629=VERTEX_POINT('',#192384);
#38630=VERTEX_POINT('',#192392);
#38631=VERTEX_POINT('',#192393);
#38632=VERTEX_POINT('',#192395);
#38633=VERTEX_POINT('',#192397);
#38634=VERTEX_POINT('',#192401);
#38635=VERTEX_POINT('',#192402);
#38636=VERTEX_POINT('',#192407);
#38637=VERTEX_POINT('',#192408);
#38638=VERTEX_POINT('',#192413);
#38639=VERTEX_POINT('',#192414);
#38640=VERTEX_POINT('',#192419);
#38641=VERTEX_POINT('',#192420);
#38642=VERTEX_POINT('',#192425);
#38643=VERTEX_POINT('',#192426);
#38644=VERTEX_POINT('',#192431);
#38645=VERTEX_POINT('',#192432);
#38646=VERTEX_POINT('',#192440);
#38647=VERTEX_POINT('',#192441);
#38648=VERTEX_POINT('',#192443);
#38649=VERTEX_POINT('',#192445);
#38650=VERTEX_POINT('',#192449);
#38651=VERTEX_POINT('',#192450);
#38652=VERTEX_POINT('',#192455);
#38653=VERTEX_POINT('',#192456);
#38654=VERTEX_POINT('',#192461);
#38655=VERTEX_POINT('',#192462);
#38656=VERTEX_POINT('',#192467);
#38657=VERTEX_POINT('',#192468);
#38658=VERTEX_POINT('',#192473);
#38659=VERTEX_POINT('',#192474);
#38660=VERTEX_POINT('',#192479);
#38661=VERTEX_POINT('',#192480);
#38662=VERTEX_POINT('',#192488);
#38663=VERTEX_POINT('',#192489);
#38664=VERTEX_POINT('',#192491);
#38665=VERTEX_POINT('',#192493);
#38666=VERTEX_POINT('',#192497);
#38667=VERTEX_POINT('',#192498);
#38668=VERTEX_POINT('',#192503);
#38669=VERTEX_POINT('',#192504);
#38670=VERTEX_POINT('',#192509);
#38671=VERTEX_POINT('',#192510);
#38672=VERTEX_POINT('',#192515);
#38673=VERTEX_POINT('',#192516);
#38674=VERTEX_POINT('',#192521);
#38675=VERTEX_POINT('',#192522);
#38676=VERTEX_POINT('',#192527);
#38677=VERTEX_POINT('',#192528);
#38678=VERTEX_POINT('',#192533);
#38679=VERTEX_POINT('',#192534);
#38680=VERTEX_POINT('',#192539);
#38681=VERTEX_POINT('',#192540);
#38682=VERTEX_POINT('',#192548);
#38683=VERTEX_POINT('',#192549);
#38684=VERTEX_POINT('',#192551);
#38685=VERTEX_POINT('',#192553);
#38686=VERTEX_POINT('',#192557);
#38687=VERTEX_POINT('',#192558);
#38688=VERTEX_POINT('',#192563);
#38689=VERTEX_POINT('',#192564);
#38690=VERTEX_POINT('',#192569);
#38691=VERTEX_POINT('',#192570);
#38692=VERTEX_POINT('',#192575);
#38693=VERTEX_POINT('',#192576);
#38694=VERTEX_POINT('',#192581);
#38695=VERTEX_POINT('',#192582);
#38696=VERTEX_POINT('',#192587);
#38697=VERTEX_POINT('',#192588);
#38698=VERTEX_POINT('',#192593);
#38699=VERTEX_POINT('',#192594);
#38700=VERTEX_POINT('',#192599);
#38701=VERTEX_POINT('',#192600);
#38702=VERTEX_POINT('',#192608);
#38703=VERTEX_POINT('',#192609);
#38704=VERTEX_POINT('',#192611);
#38705=VERTEX_POINT('',#192613);
#38706=VERTEX_POINT('',#192617);
#38707=VERTEX_POINT('',#192618);
#38708=VERTEX_POINT('',#192623);
#38709=VERTEX_POINT('',#192624);
#38710=VERTEX_POINT('',#192629);
#38711=VERTEX_POINT('',#192630);
#38712=VERTEX_POINT('',#192635);
#38713=VERTEX_POINT('',#192636);
#38714=VERTEX_POINT('',#192641);
#38715=VERTEX_POINT('',#192642);
#38716=VERTEX_POINT('',#192647);
#38717=VERTEX_POINT('',#192648);
#38718=VERTEX_POINT('',#192656);
#38719=VERTEX_POINT('',#192657);
#38720=VERTEX_POINT('',#192659);
#38721=VERTEX_POINT('',#192661);
#38722=VERTEX_POINT('',#192665);
#38723=VERTEX_POINT('',#192666);
#38724=VERTEX_POINT('',#192671);
#38725=VERTEX_POINT('',#192672);
#38726=VERTEX_POINT('',#192677);
#38727=VERTEX_POINT('',#192678);
#38728=VERTEX_POINT('',#192683);
#38729=VERTEX_POINT('',#192684);
#38730=VERTEX_POINT('',#192689);
#38731=VERTEX_POINT('',#192690);
#38732=VERTEX_POINT('',#192695);
#38733=VERTEX_POINT('',#192696);
#38734=VERTEX_POINT('',#192704);
#38735=VERTEX_POINT('',#192705);
#38736=VERTEX_POINT('',#192707);
#38737=VERTEX_POINT('',#192709);
#38738=VERTEX_POINT('',#192713);
#38739=VERTEX_POINT('',#192714);
#38740=VERTEX_POINT('',#192719);
#38741=VERTEX_POINT('',#192720);
#38742=VERTEX_POINT('',#192725);
#38743=VERTEX_POINT('',#192726);
#38744=VERTEX_POINT('',#192731);
#38745=VERTEX_POINT('',#192732);
#38746=VERTEX_POINT('',#192737);
#38747=VERTEX_POINT('',#192738);
#38748=VERTEX_POINT('',#192743);
#38749=VERTEX_POINT('',#192744);
#38750=VERTEX_POINT('',#192752);
#38751=VERTEX_POINT('',#192753);
#38752=VERTEX_POINT('',#192755);
#38753=VERTEX_POINT('',#192757);
#38754=VERTEX_POINT('',#192761);
#38755=VERTEX_POINT('',#192762);
#38756=VERTEX_POINT('',#192767);
#38757=VERTEX_POINT('',#192768);
#38758=VERTEX_POINT('',#192773);
#38759=VERTEX_POINT('',#192774);
#38760=VERTEX_POINT('',#192779);
#38761=VERTEX_POINT('',#192780);
#38762=VERTEX_POINT('',#192785);
#38763=VERTEX_POINT('',#192786);
#38764=VERTEX_POINT('',#192791);
#38765=VERTEX_POINT('',#192792);
#38766=VERTEX_POINT('',#192800);
#38767=VERTEX_POINT('',#192801);
#38768=VERTEX_POINT('',#192803);
#38769=VERTEX_POINT('',#192805);
#38770=VERTEX_POINT('',#192809);
#38771=VERTEX_POINT('',#192810);
#38772=VERTEX_POINT('',#192815);
#38773=VERTEX_POINT('',#192816);
#38774=VERTEX_POINT('',#192821);
#38775=VERTEX_POINT('',#192822);
#38776=VERTEX_POINT('',#192827);
#38777=VERTEX_POINT('',#192828);
#38778=VERTEX_POINT('',#192833);
#38779=VERTEX_POINT('',#192834);
#38780=VERTEX_POINT('',#192839);
#38781=VERTEX_POINT('',#192840);
#38782=VERTEX_POINT('',#192845);
#38783=VERTEX_POINT('',#192847);
#38784=VERTEX_POINT('',#192854);
#38785=VERTEX_POINT('',#192855);
#38786=VERTEX_POINT('',#192857);
#38787=VERTEX_POINT('',#192859);
#38788=VERTEX_POINT('',#192863);
#38789=VERTEX_POINT('',#192864);
#38790=VERTEX_POINT('',#192869);
#38791=VERTEX_POINT('',#192870);
#38792=VERTEX_POINT('',#192875);
#38793=VERTEX_POINT('',#192876);
#38794=VERTEX_POINT('',#192881);
#38795=VERTEX_POINT('',#192882);
#38796=VERTEX_POINT('',#192887);
#38797=VERTEX_POINT('',#192888);
#38798=VERTEX_POINT('',#192893);
#38799=VERTEX_POINT('',#192894);
#38800=VERTEX_POINT('',#192902);
#38801=VERTEX_POINT('',#192903);
#38802=VERTEX_POINT('',#192905);
#38803=VERTEX_POINT('',#192907);
#38804=VERTEX_POINT('',#192911);
#38805=VERTEX_POINT('',#192912);
#38806=VERTEX_POINT('',#192917);
#38807=VERTEX_POINT('',#192918);
#38808=VERTEX_POINT('',#192923);
#38809=VERTEX_POINT('',#192924);
#38810=VERTEX_POINT('',#192929);
#38811=VERTEX_POINT('',#192930);
#38812=VERTEX_POINT('',#192935);
#38813=VERTEX_POINT('',#192936);
#38814=VERTEX_POINT('',#192941);
#38815=VERTEX_POINT('',#192942);
#38816=VERTEX_POINT('',#192947);
#38817=VERTEX_POINT('',#192948);
#38818=VERTEX_POINT('',#192953);
#38819=VERTEX_POINT('',#192954);
#38820=VERTEX_POINT('',#192962);
#38821=VERTEX_POINT('',#192963);
#38822=VERTEX_POINT('',#192965);
#38823=VERTEX_POINT('',#192967);
#38824=VERTEX_POINT('',#192971);
#38825=VERTEX_POINT('',#192972);
#38826=VERTEX_POINT('',#192977);
#38827=VERTEX_POINT('',#192978);
#38828=VERTEX_POINT('',#192983);
#38829=VERTEX_POINT('',#192984);
#38830=VERTEX_POINT('',#192989);
#38831=VERTEX_POINT('',#192990);
#38832=VERTEX_POINT('',#192995);
#38833=VERTEX_POINT('',#192996);
#38834=VERTEX_POINT('',#193001);
#38835=VERTEX_POINT('',#193002);
#38836=VERTEX_POINT('',#193010);
#38837=VERTEX_POINT('',#193011);
#38838=VERTEX_POINT('',#193013);
#38839=VERTEX_POINT('',#193015);
#38840=VERTEX_POINT('',#193019);
#38841=VERTEX_POINT('',#193020);
#38842=VERTEX_POINT('',#193025);
#38843=VERTEX_POINT('',#193026);
#38844=VERTEX_POINT('',#193031);
#38845=VERTEX_POINT('',#193032);
#38846=VERTEX_POINT('',#193037);
#38847=VERTEX_POINT('',#193038);
#38848=VERTEX_POINT('',#193043);
#38849=VERTEX_POINT('',#193044);
#38850=VERTEX_POINT('',#193049);
#38851=VERTEX_POINT('',#193050);
#38852=VERTEX_POINT('',#193055);
#38853=VERTEX_POINT('',#193056);
#38854=VERTEX_POINT('',#193061);
#38855=VERTEX_POINT('',#193062);
#38856=VERTEX_POINT('',#193070);
#38857=VERTEX_POINT('',#193071);
#38858=VERTEX_POINT('',#193073);
#38859=VERTEX_POINT('',#193075);
#38860=VERTEX_POINT('',#193079);
#38861=VERTEX_POINT('',#193080);
#38862=VERTEX_POINT('',#193085);
#38863=VERTEX_POINT('',#193086);
#38864=VERTEX_POINT('',#193091);
#38865=VERTEX_POINT('',#193092);
#38866=VERTEX_POINT('',#193097);
#38867=VERTEX_POINT('',#193098);
#38868=VERTEX_POINT('',#193103);
#38869=VERTEX_POINT('',#193104);
#38870=VERTEX_POINT('',#193109);
#38871=VERTEX_POINT('',#193110);
#38872=VERTEX_POINT('',#193118);
#38873=VERTEX_POINT('',#193119);
#38874=VERTEX_POINT('',#193121);
#38875=VERTEX_POINT('',#193123);
#38876=VERTEX_POINT('',#193127);
#38877=VERTEX_POINT('',#193128);
#38878=VERTEX_POINT('',#193133);
#38879=VERTEX_POINT('',#193134);
#38880=VERTEX_POINT('',#193139);
#38881=VERTEX_POINT('',#193140);
#38882=VERTEX_POINT('',#193145);
#38883=VERTEX_POINT('',#193146);
#38884=VERTEX_POINT('',#193151);
#38885=VERTEX_POINT('',#193152);
#38886=VERTEX_POINT('',#193157);
#38887=VERTEX_POINT('',#193158);
#38888=VERTEX_POINT('',#193166);
#38889=VERTEX_POINT('',#193167);
#38890=VERTEX_POINT('',#193169);
#38891=VERTEX_POINT('',#193171);
#38892=VERTEX_POINT('',#193175);
#38893=VERTEX_POINT('',#193176);
#38894=VERTEX_POINT('',#193181);
#38895=VERTEX_POINT('',#193182);
#38896=VERTEX_POINT('',#193187);
#38897=VERTEX_POINT('',#193188);
#38898=VERTEX_POINT('',#193193);
#38899=VERTEX_POINT('',#193194);
#38900=VERTEX_POINT('',#193199);
#38901=VERTEX_POINT('',#193200);
#38902=VERTEX_POINT('',#193205);
#38903=VERTEX_POINT('',#193206);
#38904=VERTEX_POINT('',#193214);
#38905=VERTEX_POINT('',#193215);
#38906=VERTEX_POINT('',#193217);
#38907=VERTEX_POINT('',#193219);
#38908=VERTEX_POINT('',#193223);
#38909=VERTEX_POINT('',#193224);
#38910=VERTEX_POINT('',#193229);
#38911=VERTEX_POINT('',#193230);
#38912=VERTEX_POINT('',#193235);
#38913=VERTEX_POINT('',#193236);
#38914=VERTEX_POINT('',#193241);
#38915=VERTEX_POINT('',#193242);
#38916=VERTEX_POINT('',#193247);
#38917=VERTEX_POINT('',#193248);
#38918=VERTEX_POINT('',#193253);
#38919=VERTEX_POINT('',#193254);
#38920=VERTEX_POINT('',#193262);
#38921=VERTEX_POINT('',#193263);
#38922=VERTEX_POINT('',#193265);
#38923=VERTEX_POINT('',#193267);
#38924=VERTEX_POINT('',#193271);
#38925=VERTEX_POINT('',#193272);
#38926=VERTEX_POINT('',#193277);
#38927=VERTEX_POINT('',#193278);
#38928=VERTEX_POINT('',#193283);
#38929=VERTEX_POINT('',#193284);
#38930=VERTEX_POINT('',#193289);
#38931=VERTEX_POINT('',#193290);
#38932=VERTEX_POINT('',#193298);
#38933=VERTEX_POINT('',#193299);
#38934=VERTEX_POINT('',#193301);
#38935=VERTEX_POINT('',#193303);
#38936=VERTEX_POINT('',#193307);
#38937=VERTEX_POINT('',#193308);
#38938=VERTEX_POINT('',#193313);
#38939=VERTEX_POINT('',#193314);
#38940=VERTEX_POINT('',#193319);
#38941=VERTEX_POINT('',#193320);
#38942=VERTEX_POINT('',#193325);
#38943=VERTEX_POINT('',#193326);
#38944=VERTEX_POINT('',#193334);
#38945=VERTEX_POINT('',#193335);
#38946=VERTEX_POINT('',#193337);
#38947=VERTEX_POINT('',#193339);
#38948=VERTEX_POINT('',#193343);
#38949=VERTEX_POINT('',#193344);
#38950=VERTEX_POINT('',#193349);
#38951=VERTEX_POINT('',#193350);
#38952=VERTEX_POINT('',#193355);
#38953=VERTEX_POINT('',#193356);
#38954=VERTEX_POINT('',#193361);
#38955=VERTEX_POINT('',#193362);
#38956=VERTEX_POINT('',#193367);
#38957=VERTEX_POINT('',#193368);
#38958=VERTEX_POINT('',#193373);
#38959=VERTEX_POINT('',#193374);
#38960=VERTEX_POINT('',#193379);
#38961=VERTEX_POINT('',#193380);
#38962=VERTEX_POINT('',#193382);
#38963=VERTEX_POINT('',#193384);
#38964=VERTEX_POINT('',#193388);
#38965=VERTEX_POINT('',#193389);
#38966=VERTEX_POINT('',#193394);
#38967=VERTEX_POINT('',#193395);
#38968=VERTEX_POINT('',#193400);
#38969=VERTEX_POINT('',#193401);
#38970=VERTEX_POINT('',#193406);
#38971=VERTEX_POINT('',#193407);
#38972=VERTEX_POINT('',#193412);
#38973=VERTEX_POINT('',#193413);
#38974=VERTEX_POINT('',#193418);
#38975=VERTEX_POINT('',#193419);
#38976=VERTEX_POINT('',#193424);
#38977=VERTEX_POINT('',#193425);
#38978=VERTEX_POINT('',#193427);
#38979=VERTEX_POINT('',#193429);
#38980=VERTEX_POINT('',#193442);
#38981=VERTEX_POINT('',#193443);
#38982=VERTEX_POINT('',#193448);
#38983=VERTEX_POINT('',#193450);
#38984=VERTEX_POINT('',#193454);
#38985=VERTEX_POINT('',#193455);
#38986=VERTEX_POINT('',#193460);
#38987=VERTEX_POINT('',#193461);
#38988=VERTEX_POINT('',#193466);
#38989=VERTEX_POINT('',#193467);
#38990=VERTEX_POINT('',#193472);
#38991=VERTEX_POINT('',#193473);
#38992=VERTEX_POINT('',#193487);
#38993=VERTEX_POINT('',#193488);
#38994=VERTEX_POINT('',#193490);
#38995=VERTEX_POINT('',#193492);
#38996=VERTEX_POINT('',#193505);
#38997=VERTEX_POINT('',#193506);
#38998=VERTEX_POINT('',#193511);
#38999=VERTEX_POINT('',#193512);
#39000=VERTEX_POINT('',#193517);
#39001=VERTEX_POINT('',#193518);
#39002=VERTEX_POINT('',#193523);
#39003=VERTEX_POINT('',#193524);
#39004=VERTEX_POINT('',#193529);
#39005=VERTEX_POINT('',#193530);
#39006=VERTEX_POINT('',#193535);
#39007=VERTEX_POINT('',#193536);
#39008=VERTEX_POINT('',#193550);
#39009=VERTEX_POINT('',#193551);
#39010=VERTEX_POINT('',#193553);
#39011=VERTEX_POINT('',#193555);
#39012=VERTEX_POINT('',#193568);
#39013=VERTEX_POINT('',#193569);
#39014=VERTEX_POINT('',#193574);
#39015=VERTEX_POINT('',#193576);
#39016=VERTEX_POINT('',#193580);
#39017=VERTEX_POINT('',#193581);
#39018=VERTEX_POINT('',#193586);
#39019=VERTEX_POINT('',#193587);
#39020=VERTEX_POINT('',#193592);
#39021=VERTEX_POINT('',#193593);
#39022=VERTEX_POINT('',#193598);
#39023=VERTEX_POINT('',#193599);
#39024=VERTEX_POINT('',#193613);
#39025=VERTEX_POINT('',#193614);
#39026=VERTEX_POINT('',#193625);
#39027=VERTEX_POINT('',#193627);
#39028=VERTEX_POINT('',#193631);
#39029=VERTEX_POINT('',#193632);
#39030=VERTEX_POINT('',#193637);
#39031=VERTEX_POINT('',#193638);
#39032=VERTEX_POINT('',#193643);
#39033=VERTEX_POINT('',#193644);
#39034=VERTEX_POINT('',#193649);
#39035=VERTEX_POINT('',#193650);
#39036=VERTEX_POINT('',#193655);
#39037=VERTEX_POINT('',#193656);
#39038=VERTEX_POINT('',#193661);
#39039=VERTEX_POINT('',#193662);
#39040=VERTEX_POINT('',#193676);
#39041=VERTEX_POINT('',#193677);
#39042=VERTEX_POINT('',#193679);
#39043=VERTEX_POINT('',#193681);
#39044=VERTEX_POINT('',#193685);
#39045=VERTEX_POINT('',#193686);
#39046=VERTEX_POINT('',#193691);
#39047=VERTEX_POINT('',#193692);
#39048=VERTEX_POINT('',#193697);
#39049=VERTEX_POINT('',#193698);
#39050=VERTEX_POINT('',#193703);
#39051=VERTEX_POINT('',#193704);
#39052=VERTEX_POINT('',#193709);
#39053=VERTEX_POINT('',#193710);
#39054=VERTEX_POINT('',#193715);
#39055=VERTEX_POINT('',#193716);
#39056=VERTEX_POINT('',#193864);
#39057=VERTEX_POINT('',#193865);
#39058=VERTEX_POINT('',#193888);
#39059=VERTEX_POINT('',#193915);
#39060=VERTEX_POINT('',#193917);
#39061=VERTEX_POINT('',#194030);
#39062=VERTEX_POINT('',#194055);
#39063=VERTEX_POINT('',#194056);
#39064=VERTEX_POINT('',#194078);
#39065=VERTEX_POINT('',#194079);
#39066=VERTEX_POINT('',#194161);
#39067=VERTEX_POINT('',#194162);
#39068=VERTEX_POINT('',#194263);
#39069=VERTEX_POINT('',#194264);
#39070=VERTEX_POINT('',#194469);
#39071=VERTEX_POINT('',#194470);
#39072=VERTEX_POINT('',#194567);
#39073=VERTEX_POINT('',#194568);
#39074=VERTEX_POINT('',#194584);
#39075=VERTEX_POINT('',#194585);
#39076=VERTEX_POINT('',#194907);
#39077=VERTEX_POINT('',#194908);
#39078=VERTEX_POINT('',#194910);
#39079=VERTEX_POINT('',#194963);
#39080=VERTEX_POINT('',#195004);
#39081=VERTEX_POINT('',#195049);
#39082=VERTEX_POINT('',#195066);
#39083=VERTEX_POINT('',#195310);
#39084=VERTEX_POINT('',#195311);
#39085=VERTEX_POINT('',#195333);
#39086=VERTEX_POINT('',#195334);
#39087=VERTEX_POINT('',#195434);
#39088=VERTEX_POINT('',#195435);
#39089=VERTEX_POINT('',#195551);
#39090=VERTEX_POINT('',#195552);
#39091=VERTEX_POINT('',#195766);
#39092=VERTEX_POINT('',#195767);
#39093=VERTEX_POINT('',#195864);
#39094=VERTEX_POINT('',#195865);
#39095=VERTEX_POINT('',#195881);
#39096=VERTEX_POINT('',#195882);
#39097=VERTEX_POINT('',#195904);
#39098=VERTEX_POINT('',#195909);
#39099=VERTEX_POINT('',#195924);
#39100=VERTEX_POINT('',#195925);
#39101=VERTEX_POINT('',#196007);
#39102=VERTEX_POINT('',#196008);
#39103=VERTEX_POINT('',#196086);
#39104=VERTEX_POINT('',#196087);
#39105=VERTEX_POINT('',#196147);
#39106=VERTEX_POINT('',#196148);
#39107=VERTEX_POINT('',#196155);
#39108=VERTEX_POINT('',#196174);
#39109=VERTEX_POINT('',#196175);
#39110=VERTEX_POINT('',#196666);
#39111=VERTEX_POINT('',#196667);
#39112=VERTEX_POINT('',#196693);
#39113=VERTEX_POINT('',#196737);
#39114=VERTEX_POINT('',#196766);
#39115=VERTEX_POINT('',#196787);
#39116=VERTEX_POINT('',#196817);
#39117=VERTEX_POINT('',#196843);
#39118=VERTEX_POINT('',#197287);
#39119=VERTEX_POINT('',#197315);
#39120=VERTEX_POINT('',#197316);
#39121=VERTEX_POINT('',#197341);
#39122=VERTEX_POINT('',#197343);
#39123=VERTEX_POINT('',#197364);
#39124=VERTEX_POINT('',#197365);
#39125=VERTEX_POINT('',#197458);
#39126=VERTEX_POINT('',#197459);
#39127=VERTEX_POINT('',#197632);
#39128=VERTEX_POINT('',#197633);
#39129=VERTEX_POINT('',#197666);
#39130=VERTEX_POINT('',#197667);
#39131=VERTEX_POINT('',#197669);
#39132=VERTEX_POINT('',#197747);
#39133=VERTEX_POINT('',#197748);
#39134=VERTEX_POINT('',#197764);
#39135=VERTEX_POINT('',#197766);
#39136=VERTEX_POINT('',#197799);
#39137=VERTEX_POINT('',#197800);
#39138=VERTEX_POINT('',#197903);
#39139=VERTEX_POINT('',#197904);
#39140=VERTEX_POINT('',#197970);
#39141=VERTEX_POINT('',#197971);
#39142=VERTEX_POINT('',#198002);
#39143=VERTEX_POINT('',#198003);
#39144=VERTEX_POINT('',#198005);
#39145=VERTEX_POINT('',#198007);
#39146=VERTEX_POINT('',#198196);
#39147=VERTEX_POINT('',#198197);
#39148=VERTEX_POINT('',#198221);
#39149=VERTEX_POINT('',#198256);
#39150=VERTEX_POINT('',#198275);
#39151=VERTEX_POINT('',#198498);
#39152=VERTEX_POINT('',#198543);
#39153=VERTEX_POINT('',#198544);
#39154=VERTEX_POINT('',#198549);
#39155=VERTEX_POINT('',#198565);
#39156=VERTEX_POINT('',#198604);
#39157=VERTEX_POINT('',#198605);
#39158=VERTEX_POINT('',#198762);
#39159=VERTEX_POINT('',#198763);
#39160=VERTEX_POINT('',#198924);
#39161=VERTEX_POINT('',#198925);
#39162=VERTEX_POINT('',#199109);
#39163=VERTEX_POINT('',#199110);
#39164=VERTEX_POINT('',#199115);
#39165=VERTEX_POINT('',#199117);
#39166=VERTEX_POINT('',#199121);
#39167=VERTEX_POINT('',#199123);
#39168=VERTEX_POINT('',#199127);
#39169=VERTEX_POINT('',#199129);
#39170=VERTEX_POINT('',#199133);
#39171=VERTEX_POINT('',#199135);
#39172=VERTEX_POINT('',#199139);
#39173=VERTEX_POINT('',#199141);
#39174=VERTEX_POINT('',#199145);
#39175=VERTEX_POINT('',#199147);
#39176=VERTEX_POINT('',#199151);
#39177=VERTEX_POINT('',#199153);
#39178=VERTEX_POINT('',#199157);
#39179=VERTEX_POINT('',#199159);
#39180=VERTEX_POINT('',#199163);
#39181=VERTEX_POINT('',#199164);
#39182=VERTEX_POINT('',#199169);
#39183=VERTEX_POINT('',#199171);
#39184=VERTEX_POINT('',#199175);
#39185=VERTEX_POINT('',#199177);
#39186=VERTEX_POINT('',#199181);
#39187=VERTEX_POINT('',#199183);
#39188=VERTEX_POINT('',#199187);
#39189=VERTEX_POINT('',#199189);
#39190=VERTEX_POINT('',#199193);
#39191=VERTEX_POINT('',#199195);
#39192=VERTEX_POINT('',#199199);
#39193=VERTEX_POINT('',#199201);
#39194=VERTEX_POINT('',#199205);
#39195=VERTEX_POINT('',#199207);
#39196=VERTEX_POINT('',#199211);
#39197=VERTEX_POINT('',#199213);
#39198=VERTEX_POINT('',#199217);
#39199=VERTEX_POINT('',#199219);
#39200=VERTEX_POINT('',#199223);
#39201=VERTEX_POINT('',#199225);
#39202=VERTEX_POINT('',#199229);
#39203=VERTEX_POINT('',#199231);
#39204=VERTEX_POINT('',#199235);
#39205=VERTEX_POINT('',#199237);
#39206=VERTEX_POINT('',#199241);
#39207=VERTEX_POINT('',#199243);
#39208=VERTEX_POINT('',#199247);
#39209=VERTEX_POINT('',#199249);
#39210=VERTEX_POINT('',#199253);
#39211=VERTEX_POINT('',#199255);
#39212=VERTEX_POINT('',#199259);
#39213=VERTEX_POINT('',#199261);
#39214=VERTEX_POINT('',#199265);
#39215=VERTEX_POINT('',#199267);
#39216=VERTEX_POINT('',#199271);
#39217=VERTEX_POINT('',#199272);
#39218=VERTEX_POINT('',#199277);
#39219=VERTEX_POINT('',#199279);
#39220=VERTEX_POINT('',#199283);
#39221=VERTEX_POINT('',#199285);
#39222=VERTEX_POINT('',#199289);
#39223=VERTEX_POINT('',#199291);
#39224=VERTEX_POINT('',#199295);
#39225=VERTEX_POINT('',#199297);
#39226=VERTEX_POINT('',#199301);
#39227=VERTEX_POINT('',#199303);
#39228=VERTEX_POINT('',#199307);
#39229=VERTEX_POINT('',#199309);
#39230=VERTEX_POINT('',#199313);
#39231=VERTEX_POINT('',#199315);
#39232=VERTEX_POINT('',#199319);
#39233=VERTEX_POINT('',#199321);
#39234=VERTEX_POINT('',#199325);
#39235=VERTEX_POINT('',#199327);
#39236=VERTEX_POINT('',#199331);
#39237=VERTEX_POINT('',#199333);
#39238=VERTEX_POINT('',#199337);
#39239=VERTEX_POINT('',#199339);
#39240=VERTEX_POINT('',#199343);
#39241=VERTEX_POINT('',#199345);
#39242=VERTEX_POINT('',#199349);
#39243=VERTEX_POINT('',#199351);
#39244=VERTEX_POINT('',#199355);
#39245=VERTEX_POINT('',#199357);
#39246=VERTEX_POINT('',#199361);
#39247=VERTEX_POINT('',#199363);
#39248=VERTEX_POINT('',#199367);
#39249=VERTEX_POINT('',#199369);
#39250=VERTEX_POINT('',#199373);
#39251=VERTEX_POINT('',#199375);
#39252=VERTEX_POINT('',#199379);
#39253=VERTEX_POINT('',#199381);
#39254=VERTEX_POINT('',#199385);
#39255=VERTEX_POINT('',#199387);
#39256=VERTEX_POINT('',#199391);
#39257=VERTEX_POINT('',#199393);
#39258=VERTEX_POINT('',#199397);
#39259=VERTEX_POINT('',#199399);
#39260=VERTEX_POINT('',#199403);
#39261=VERTEX_POINT('',#199405);
#39262=VERTEX_POINT('',#199409);
#39263=VERTEX_POINT('',#199411);
#39264=VERTEX_POINT('',#199415);
#39265=VERTEX_POINT('',#199417);
#39266=VERTEX_POINT('',#199421);
#39267=VERTEX_POINT('',#199423);
#39268=VERTEX_POINT('',#199427);
#39269=VERTEX_POINT('',#199429);
#39270=VERTEX_POINT('',#199433);
#39271=VERTEX_POINT('',#199435);
#39272=VERTEX_POINT('',#199439);
#39273=VERTEX_POINT('',#199441);
#39274=VERTEX_POINT('',#199445);
#39275=VERTEX_POINT('',#199447);
#39276=VERTEX_POINT('',#199451);
#39277=VERTEX_POINT('',#199453);
#39278=VERTEX_POINT('',#199457);
#39279=VERTEX_POINT('',#199459);
#39280=VERTEX_POINT('',#199463);
#39281=VERTEX_POINT('',#199465);
#39282=VERTEX_POINT('',#199469);
#39283=VERTEX_POINT('',#199471);
#39284=VERTEX_POINT('',#199475);
#39285=VERTEX_POINT('',#199477);
#39286=VERTEX_POINT('',#199481);
#39287=VERTEX_POINT('',#199483);
#39288=VERTEX_POINT('',#199487);
#39289=VERTEX_POINT('',#199489);
#39290=VERTEX_POINT('',#199493);
#39291=VERTEX_POINT('',#199495);
#39292=VERTEX_POINT('',#199499);
#39293=VERTEX_POINT('',#199501);
#39294=VERTEX_POINT('',#199505);
#39295=VERTEX_POINT('',#199507);
#39296=VERTEX_POINT('',#199511);
#39297=VERTEX_POINT('',#199513);
#39298=VERTEX_POINT('',#199517);
#39299=VERTEX_POINT('',#199519);
#39300=VERTEX_POINT('',#199523);
#39301=VERTEX_POINT('',#199525);
#39302=VERTEX_POINT('',#199529);
#39303=VERTEX_POINT('',#199531);
#39304=VERTEX_POINT('',#199535);
#39305=VERTEX_POINT('',#199537);
#39306=VERTEX_POINT('',#199541);
#39307=VERTEX_POINT('',#199543);
#39308=VERTEX_POINT('',#199547);
#39309=VERTEX_POINT('',#199549);
#39310=VERTEX_POINT('',#199553);
#39311=VERTEX_POINT('',#199555);
#39312=VERTEX_POINT('',#199559);
#39313=VERTEX_POINT('',#199561);
#39314=VERTEX_POINT('',#199565);
#39315=VERTEX_POINT('',#199567);
#39316=VERTEX_POINT('',#199571);
#39317=VERTEX_POINT('',#199573);
#39318=VERTEX_POINT('',#199577);
#39319=VERTEX_POINT('',#199579);
#39320=VERTEX_POINT('',#199583);
#39321=VERTEX_POINT('',#199585);
#39322=VERTEX_POINT('',#199589);
#39323=VERTEX_POINT('',#199591);
#39324=VERTEX_POINT('',#199595);
#39325=VERTEX_POINT('',#199597);
#39326=VERTEX_POINT('',#199601);
#39327=VERTEX_POINT('',#199603);
#39328=VERTEX_POINT('',#199607);
#39329=VERTEX_POINT('',#199609);
#39330=VERTEX_POINT('',#199613);
#39331=VERTEX_POINT('',#199615);
#39332=VERTEX_POINT('',#199619);
#39333=VERTEX_POINT('',#199620);
#39334=VERTEX_POINT('',#199625);
#39335=VERTEX_POINT('',#199627);
#39336=VERTEX_POINT('',#199631);
#39337=VERTEX_POINT('',#199633);
#39338=VERTEX_POINT('',#199637);
#39339=VERTEX_POINT('',#199639);
#39340=VERTEX_POINT('',#199643);
#39341=VERTEX_POINT('',#199645);
#39342=VERTEX_POINT('',#199649);
#39343=VERTEX_POINT('',#199651);
#39344=VERTEX_POINT('',#199655);
#39345=VERTEX_POINT('',#199657);
#39346=VERTEX_POINT('',#199661);
#39347=VERTEX_POINT('',#199663);
#39348=VERTEX_POINT('',#199667);
#39349=VERTEX_POINT('',#199669);
#39350=VERTEX_POINT('',#199673);
#39351=VERTEX_POINT('',#199675);
#39352=VERTEX_POINT('',#199679);
#39353=VERTEX_POINT('',#199681);
#39354=VERTEX_POINT('',#199685);
#39355=VERTEX_POINT('',#199687);
#39356=VERTEX_POINT('',#199691);
#39357=VERTEX_POINT('',#199693);
#39358=VERTEX_POINT('',#199697);
#39359=VERTEX_POINT('',#199699);
#39360=VERTEX_POINT('',#199703);
#39361=VERTEX_POINT('',#199705);
#39362=VERTEX_POINT('',#199709);
#39363=VERTEX_POINT('',#199711);
#39364=VERTEX_POINT('',#199715);
#39365=VERTEX_POINT('',#199717);
#39366=VERTEX_POINT('',#199721);
#39367=VERTEX_POINT('',#199723);
#39368=VERTEX_POINT('',#199727);
#39369=VERTEX_POINT('',#199729);
#39370=VERTEX_POINT('',#199733);
#39371=VERTEX_POINT('',#199735);
#39372=VERTEX_POINT('',#199739);
#39373=VERTEX_POINT('',#199741);
#39374=VERTEX_POINT('',#199745);
#39375=VERTEX_POINT('',#199747);
#39376=VERTEX_POINT('',#199751);
#39377=VERTEX_POINT('',#199753);
#39378=VERTEX_POINT('',#199757);
#39379=VERTEX_POINT('',#199759);
#39380=VERTEX_POINT('',#199763);
#39381=VERTEX_POINT('',#199764);
#39382=VERTEX_POINT('',#199769);
#39383=VERTEX_POINT('',#199771);
#39384=VERTEX_POINT('',#199775);
#39385=VERTEX_POINT('',#199777);
#39386=VERTEX_POINT('',#199781);
#39387=VERTEX_POINT('',#199783);
#39388=VERTEX_POINT('',#199787);
#39389=VERTEX_POINT('',#199789);
#39390=VERTEX_POINT('',#199793);
#39391=VERTEX_POINT('',#199795);
#39392=VERTEX_POINT('',#199799);
#39393=VERTEX_POINT('',#199801);
#39394=VERTEX_POINT('',#199805);
#39395=VERTEX_POINT('',#199807);
#39396=VERTEX_POINT('',#199811);
#39397=VERTEX_POINT('',#199813);
#39398=VERTEX_POINT('',#199817);
#39399=VERTEX_POINT('',#199819);
#39400=VERTEX_POINT('',#199823);
#39401=VERTEX_POINT('',#199825);
#39402=VERTEX_POINT('',#199829);
#39403=VERTEX_POINT('',#199831);
#39404=VERTEX_POINT('',#199835);
#39405=VERTEX_POINT('',#199837);
#39406=VERTEX_POINT('',#199841);
#39407=VERTEX_POINT('',#199843);
#39408=VERTEX_POINT('',#199847);
#39409=VERTEX_POINT('',#199849);
#39410=VERTEX_POINT('',#199853);
#39411=VERTEX_POINT('',#199855);
#39412=VERTEX_POINT('',#199859);
#39413=VERTEX_POINT('',#199860);
#39414=VERTEX_POINT('',#199865);
#39415=VERTEX_POINT('',#199867);
#39416=VERTEX_POINT('',#199871);
#39417=VERTEX_POINT('',#199873);
#39418=VERTEX_POINT('',#199877);
#39419=VERTEX_POINT('',#199879);
#39420=VERTEX_POINT('',#199883);
#39421=VERTEX_POINT('',#199885);
#39422=VERTEX_POINT('',#199889);
#39423=VERTEX_POINT('',#199890);
#39424=VERTEX_POINT('',#199895);
#39425=VERTEX_POINT('',#199897);
#39426=VERTEX_POINT('',#199901);
#39427=VERTEX_POINT('',#199902);
#39428=VERTEX_POINT('',#199907);
#39429=VERTEX_POINT('',#199909);
#39430=VERTEX_POINT('',#199913);
#39431=VERTEX_POINT('',#199915);
#39432=VERTEX_POINT('',#199919);
#39433=VERTEX_POINT('',#199921);
#39434=VERTEX_POINT('',#199925);
#39435=VERTEX_POINT('',#199929);
#39436=VERTEX_POINT('',#200021);
#39437=VERTEX_POINT('',#200022);
#39438=VERTEX_POINT('',#200024);
#39439=VERTEX_POINT('',#200026);
#39440=VERTEX_POINT('',#200030);
#39441=VERTEX_POINT('',#200031);
#39442=VERTEX_POINT('',#200036);
#39443=VERTEX_POINT('',#200038);
#39444=VERTEX_POINT('',#200086);
#39445=VERTEX_POINT('',#200087);
#39446=VERTEX_POINT('',#200089);
#39447=VERTEX_POINT('',#200091);
#39448=VERTEX_POINT('',#200095);
#39449=VERTEX_POINT('',#200097);
#39450=VERTEX_POINT('',#200101);
#39451=VERTEX_POINT('',#200103);
#39452=VERTEX_POINT('',#200107);
#39453=VERTEX_POINT('',#200109);
#39454=VERTEX_POINT('',#200113);
#39455=VERTEX_POINT('',#200115);
#39456=VERTEX_POINT('',#200119);
#39457=VERTEX_POINT('',#200121);
#39458=VERTEX_POINT('',#200125);
#39459=VERTEX_POINT('',#200127);
#39460=VERTEX_POINT('',#200131);
#39461=VERTEX_POINT('',#200132);
#39462=VERTEX_POINT('',#200134);
#39463=VERTEX_POINT('',#200136);
#39464=VERTEX_POINT('',#200145);
#39465=VERTEX_POINT('',#200154);
#39466=VERTEX_POINT('',#200155);
#39467=VERTEX_POINT('',#200157);
#39468=VERTEX_POINT('',#200166);
#39469=VERTEX_POINT('',#200175);
#39470=VERTEX_POINT('',#200176);
#39471=VERTEX_POINT('',#200180);
#39472=VERTEX_POINT('',#200182);
#39473=VERTEX_POINT('',#200191);
#39474=VERTEX_POINT('',#200192);
#39475=VERTEX_POINT('',#200196);
#39476=VERTEX_POINT('',#200203);
#39477=VERTEX_POINT('',#200210);
#39478=VERTEX_POINT('',#200211);
#39479=VERTEX_POINT('',#200215);
#39480=VERTEX_POINT('',#200222);
#39481=VERTEX_POINT('',#200226);
#39482=VERTEX_POINT('',#200227);
#39483=VERTEX_POINT('',#200231);
#39484=VERTEX_POINT('',#200233);
#39485=VERTEX_POINT('',#200245);
#39486=VERTEX_POINT('',#200246);
#39487=VERTEX_POINT('',#200248);
#39488=VERTEX_POINT('',#200250);
#39489=VERTEX_POINT('',#200254);
#39490=VERTEX_POINT('',#200255);
#39491=VERTEX_POINT('',#200257);
#39492=VERTEX_POINT('',#200259);
#39493=VERTEX_POINT('',#200263);
#39494=VERTEX_POINT('',#200265);
#39495=VERTEX_POINT('',#200269);
#39496=VERTEX_POINT('',#200271);
#39497=VERTEX_POINT('',#200275);
#39498=VERTEX_POINT('',#200276);
#39499=VERTEX_POINT('',#200286);
#39500=VERTEX_POINT('',#200287);
#39501=VERTEX_POINT('',#200289);
#39502=VERTEX_POINT('',#200291);
#39503=VERTEX_POINT('',#200661);
#39504=VERTEX_POINT('',#200662);
#39505=VERTEX_POINT('',#200683);
#39506=VERTEX_POINT('',#200688);
#39507=VERTEX_POINT('',#200695);
#39508=VERTEX_POINT('',#201283);
#39509=VERTEX_POINT('',#201284);
#39510=VERTEX_POINT('',#201309);
#39511=VERTEX_POINT('',#201320);
#39512=VERTEX_POINT('',#201345);
#39513=VERTEX_POINT('',#201724);
#39514=VERTEX_POINT('',#201725);
#39515=VERTEX_POINT('',#201744);
#39516=VERTEX_POINT('',#201758);
#39517=VERTEX_POINT('',#201765);
#39518=VERTEX_POINT('',#202316);
#39519=VERTEX_POINT('',#202317);
#39520=VERTEX_POINT('',#202334);
#39521=VERTEX_POINT('',#202342);
#39522=VERTEX_POINT('',#202369);
#39523=VERTEX_POINT('',#202383);
#39524=VERTEX_POINT('',#202384);
#39525=VERTEX_POINT('',#202387);
#39526=VERTEX_POINT('',#202404);
#39527=VERTEX_POINT('',#202411);
#39528=VERTEX_POINT('',#202415);
#39529=VERTEX_POINT('',#202420);
#39530=VERTEX_POINT('',#202421);
#39531=VERTEX_POINT('',#202424);
#39532=VERTEX_POINT('',#202428);
#39533=VERTEX_POINT('',#202437);
#39534=VERTEX_POINT('',#202449);
#39535=VERTEX_POINT('',#202454);
#39536=VERTEX_POINT('',#202455);
#39537=VERTEX_POINT('',#202457);
#39538=VERTEX_POINT('',#202459);
#39539=VERTEX_POINT('',#202463);
#39540=VERTEX_POINT('',#202465);
#39541=VERTEX_POINT('',#202469);
#39542=VERTEX_POINT('',#202471);
#39543=VERTEX_POINT('',#202475);
#39544=VERTEX_POINT('',#202477);
#39545=VERTEX_POINT('',#202481);
#39546=VERTEX_POINT('',#202482);
#39547=VERTEX_POINT('',#202484);
#39548=VERTEX_POINT('',#202486);
#39549=VERTEX_POINT('',#202490);
#39550=VERTEX_POINT('',#202492);
#39551=VERTEX_POINT('',#202514);
#39552=VERTEX_POINT('',#202521);
#39553=VERTEX_POINT('',#202550);
#39554=VERTEX_POINT('',#202557);
#39555=VERTEX_POINT('',#202769);
#39556=VERTEX_POINT('',#202771);
#39557=VERTEX_POINT('',#202855);
#39558=VERTEX_POINT('',#202879);
#39559=VERTEX_POINT('',#202881);
#39560=VERTEX_POINT('',#202905);
#39561=VERTEX_POINT('',#202953);
#39562=VERTEX_POINT('',#202960);
#39563=VERTEX_POINT('',#203164);
#39564=VERTEX_POINT('',#203209);
#39565=VERTEX_POINT('',#203216);
#39566=VERTEX_POINT('',#203230);
#39567=VERTEX_POINT('',#203237);
#39568=VERTEX_POINT('',#203525);
#39569=VERTEX_POINT('',#203563);
#39570=VERTEX_POINT('',#203564);
#39571=VERTEX_POINT('',#203579);
#39572=VERTEX_POINT('',#203588);
#39573=VERTEX_POINT('',#203589);
#39574=VERTEX_POINT('',#203598);
#39575=VERTEX_POINT('',#203599);
#39576=VERTEX_POINT('',#203608);
#39577=VERTEX_POINT('',#203609);
#39578=VERTEX_POINT('',#203618);
#39579=VERTEX_POINT('',#203619);
#39580=VERTEX_POINT('',#203628);
#39581=VERTEX_POINT('',#203632);
#39582=VERTEX_POINT('',#203641);
#39583=VERTEX_POINT('',#203652);
#39584=VERTEX_POINT('',#203653);
#39585=VERTEX_POINT('',#203670);
#39586=VERTEX_POINT('',#203679);
#39587=VERTEX_POINT('',#203680);
#39588=VERTEX_POINT('',#203719);
#39589=VERTEX_POINT('',#204831);
#39590=VERTEX_POINT('',#204842);
#39591=VERTEX_POINT('',#204867);
#39592=VERTEX_POINT('',#204869);
#39593=VERTEX_POINT('',#204873);
#39594=VERTEX_POINT('',#204877);
#39595=VERTEX_POINT('',#204883);
#39596=VERTEX_POINT('',#204885);
#39597=VERTEX_POINT('',#204891);
#39598=VERTEX_POINT('',#204893);
#39599=VERTEX_POINT('',#204897);
#39600=VERTEX_POINT('',#204900);
#39601=VERTEX_POINT('',#204905);
#39602=VERTEX_POINT('',#205009);
#39603=VERTEX_POINT('',#205011);
#39604=VERTEX_POINT('',#205015);
#39605=VERTEX_POINT('',#205019);
#39606=VERTEX_POINT('',#205023);
#39607=VERTEX_POINT('',#205027);
#39608=VERTEX_POINT('',#205031);
#39609=VERTEX_POINT('',#205035);
#39610=VERTEX_POINT('',#205039);
#39611=VERTEX_POINT('',#205041);
#39612=VERTEX_POINT('',#205045);
#39613=VERTEX_POINT('',#205047);
#39614=VERTEX_POINT('',#205051);
#39615=VERTEX_POINT('',#205055);
#39616=VERTEX_POINT('',#205059);
#39617=VERTEX_POINT('',#205063);
#39618=VERTEX_POINT('',#205474);
#39619=VERTEX_POINT('',#205476);
#39620=VERTEX_POINT('',#205480);
#39621=VERTEX_POINT('',#205484);
#39622=VERTEX_POINT('',#205488);
#39623=VERTEX_POINT('',#205492);
#39624=VERTEX_POINT('',#205494);
#39625=VERTEX_POINT('',#205498);
#39626=VERTEX_POINT('',#207116);
#39627=VERTEX_POINT('',#207117);
#39628=VERTEX_POINT('',#207119);
#39629=VERTEX_POINT('',#207172);
#39630=VERTEX_POINT('',#207201);
#39631=VERTEX_POINT('',#207205);
#39632=VERTEX_POINT('',#207207);
#39633=VERTEX_POINT('',#207209);
#39634=VERTEX_POINT('',#207242);
#39635=VERTEX_POINT('',#207243);
#39636=VERTEX_POINT('',#207245);
#39637=VERTEX_POINT('',#207325);
#39638=VERTEX_POINT('',#207370);
#39639=VERTEX_POINT('',#207371);
#39640=VERTEX_POINT('',#207424);
#39641=VERTEX_POINT('',#207457);
#39642=VERTEX_POINT('',#207458);
#39643=VERTEX_POINT('',#207524);
#39644=VERTEX_POINT('',#207525);
#39645=VERTEX_POINT('',#207547);
#39646=VERTEX_POINT('',#207548);
#39647=VERTEX_POINT('',#207583);
#39648=VERTEX_POINT('',#207584);
#39649=VERTEX_POINT('',#207618);
#39650=VERTEX_POINT('',#207619);
#39651=VERTEX_POINT('',#207744);
#39652=VERTEX_POINT('',#207745);
#39653=VERTEX_POINT('',#207761);
#39654=VERTEX_POINT('',#207762);
#39655=VERTEX_POINT('',#207795);
#39656=VERTEX_POINT('',#207796);
#39657=VERTEX_POINT('',#207854);
#39658=VERTEX_POINT('',#207905);
#39659=VERTEX_POINT('',#208000);
#39660=VERTEX_POINT('',#208001);
#39661=VERTEX_POINT('',#208003);
#39662=VERTEX_POINT('',#208038);
#39663=VERTEX_POINT('',#208079);
#39664=VERTEX_POINT('',#208080);
#39665=VERTEX_POINT('',#208108);
#39666=VERTEX_POINT('',#208109);
#39667=VERTEX_POINT('',#208158);
#39668=VERTEX_POINT('',#208159);
#39669=VERTEX_POINT('',#208331);
#39670=VERTEX_POINT('',#208332);
#39671=VERTEX_POINT('',#208398);
#39672=VERTEX_POINT('',#208413);
#39673=VERTEX_POINT('',#208414);
#39674=VERTEX_POINT('',#208447);
#39675=VERTEX_POINT('',#208448);
#39676=VERTEX_POINT('',#208482);
#39677=VERTEX_POINT('',#208483);
#39678=VERTEX_POINT('',#208590);
#39679=VERTEX_POINT('',#208591);
#39680=VERTEX_POINT('',#208596);
#39681=VERTEX_POINT('',#208600);
#39682=VERTEX_POINT('',#208601);
#39683=VERTEX_POINT('',#208617);
#39684=VERTEX_POINT('',#208618);
#39685=VERTEX_POINT('',#208632);
#39686=VERTEX_POINT('',#208634);
#39687=VERTEX_POINT('',#208638);
#39688=VERTEX_POINT('',#208639);
#39689=VERTEX_POINT('',#208644);
#39690=VERTEX_POINT('',#208645);
#39691=VERTEX_POINT('',#208650);
#39692=VERTEX_POINT('',#208651);
#39693=VERTEX_POINT('',#208656);
#39694=VERTEX_POINT('',#208657);
#39695=VERTEX_POINT('',#208662);
#39696=VERTEX_POINT('',#208663);
#39697=VERTEX_POINT('',#208668);
#39698=VERTEX_POINT('',#208669);
#39699=VERTEX_POINT('',#208674);
#39700=VERTEX_POINT('',#208675);
#39701=VERTEX_POINT('',#208694);
#39702=VERTEX_POINT('',#208696);
#39703=VERTEX_POINT('',#208711);
#39704=VERTEX_POINT('',#208712);
#39705=VERTEX_POINT('',#208755);
#39706=VERTEX_POINT('',#208788);
#39707=VERTEX_POINT('',#208849);
#39708=VERTEX_POINT('',#208850);
#39709=VERTEX_POINT('',#209011);
#39710=VERTEX_POINT('',#209012);
#39711=VERTEX_POINT('',#209028);
#39712=VERTEX_POINT('',#209029);
#39713=VERTEX_POINT('',#209045);
#39714=VERTEX_POINT('',#209046);
#39715=VERTEX_POINT('',#209119);
#39716=VERTEX_POINT('',#209120);
#39717=VERTEX_POINT('',#209208);
#39718=VERTEX_POINT('',#209209);
#39719=VERTEX_POINT('',#209377);
#39720=VERTEX_POINT('',#209378);
#39721=VERTEX_POINT('',#209563);
#39722=VERTEX_POINT('',#209564);
#39723=VERTEX_POINT('',#209735);
#39724=VERTEX_POINT('',#209736);
#39725=VERTEX_POINT('',#209914);
#39726=VERTEX_POINT('',#209915);
#39727=VERTEX_POINT('',#209917);
#39728=VERTEX_POINT('',#210015);
#39729=VERTEX_POINT('',#210036);
#39730=VERTEX_POINT('',#210037);
#39731=VERTEX_POINT('',#210065);
#39732=VERTEX_POINT('',#210066);
#39733=VERTEX_POINT('',#210257);
#39734=VERTEX_POINT('',#210258);
#39735=VERTEX_POINT('',#210391);
#39736=VERTEX_POINT('',#210392);
#39737=VERTEX_POINT('',#210471);
#39738=VERTEX_POINT('',#210472);
#39739=VERTEX_POINT('',#210509);
#39740=VERTEX_POINT('',#210554);
#39741=VERTEX_POINT('',#210555);
#39742=VERTEX_POINT('',#210571);
#39743=VERTEX_POINT('',#210572);
#39744=VERTEX_POINT('',#210732);
#39745=VERTEX_POINT('',#210733);
#39746=VERTEX_POINT('',#210830);
#39747=VERTEX_POINT('',#210832);
#39748=VERTEX_POINT('',#210844);
#39749=VERTEX_POINT('',#210846);
#39750=VERTEX_POINT('',#210850);
#39751=VERTEX_POINT('',#210853);
#39752=VERTEX_POINT('',#210865);
#39753=VERTEX_POINT('',#210866);
#39754=VERTEX_POINT('',#210874);
#39755=VERTEX_POINT('',#210876);
#39756=VERTEX_POINT('',#210888);
#39757=VERTEX_POINT('',#210890);
#39758=VERTEX_POINT('',#210894);
#39759=VERTEX_POINT('',#210895);
#39760=VERTEX_POINT('',#210908);
#39761=VERTEX_POINT('',#210909);
#39762=VERTEX_POINT('',#210917);
#39763=VERTEX_POINT('',#210919);
#39764=VERTEX_POINT('',#210931);
#39765=VERTEX_POINT('',#210932);
#39766=VERTEX_POINT('',#210937);
#39767=VERTEX_POINT('',#210938);
#39768=VERTEX_POINT('',#210951);
#39769=VERTEX_POINT('',#210953);
#39770=VERTEX_POINT('',#210960);
#39771=VERTEX_POINT('',#210962);
#39772=VERTEX_POINT('',#210974);
#39773=VERTEX_POINT('',#210975);
#39774=VERTEX_POINT('',#210980);
#39775=VERTEX_POINT('',#210981);
#39776=VERTEX_POINT('',#210994);
#39777=VERTEX_POINT('',#210996);
#39778=VERTEX_POINT('',#211027);
#39779=VERTEX_POINT('',#211028);
#39780=VERTEX_POINT('',#211030);
#39781=VERTEX_POINT('',#211032);
#39782=VERTEX_POINT('',#211036);
#39783=VERTEX_POINT('',#211037);
#39784=VERTEX_POINT('',#211042);
#39785=VERTEX_POINT('',#211043);
#39786=VERTEX_POINT('',#211048);
#39787=VERTEX_POINT('',#211049);
#39788=VERTEX_POINT('',#211054);
#39789=VERTEX_POINT('',#211055);
#39790=VERTEX_POINT('',#211060);
#39791=VERTEX_POINT('',#211061);
#39792=VERTEX_POINT('',#211066);
#39793=VERTEX_POINT('',#211067);
#39794=VERTEX_POINT('',#211072);
#39795=VERTEX_POINT('',#211073);
#39796=VERTEX_POINT('',#211078);
#39797=VERTEX_POINT('',#211079);
#39798=VERTEX_POINT('',#211087);
#39799=VERTEX_POINT('',#211088);
#39800=VERTEX_POINT('',#211090);
#39801=VERTEX_POINT('',#211092);
#39802=VERTEX_POINT('',#211096);
#39803=VERTEX_POINT('',#211097);
#39804=VERTEX_POINT('',#211102);
#39805=VERTEX_POINT('',#211103);
#39806=VERTEX_POINT('',#211108);
#39807=VERTEX_POINT('',#211109);
#39808=VERTEX_POINT('',#211114);
#39809=VERTEX_POINT('',#211115);
#39810=VERTEX_POINT('',#211120);
#39811=VERTEX_POINT('',#211121);
#39812=VERTEX_POINT('',#211126);
#39813=VERTEX_POINT('',#211127);
#39814=VERTEX_POINT('',#211135);
#39815=VERTEX_POINT('',#211136);
#39816=VERTEX_POINT('',#211138);
#39817=VERTEX_POINT('',#211140);
#39818=VERTEX_POINT('',#211144);
#39819=VERTEX_POINT('',#211145);
#39820=VERTEX_POINT('',#211150);
#39821=VERTEX_POINT('',#211151);
#39822=VERTEX_POINT('',#211156);
#39823=VERTEX_POINT('',#211157);
#39824=VERTEX_POINT('',#211162);
#39825=VERTEX_POINT('',#211163);
#39826=VERTEX_POINT('',#211168);
#39827=VERTEX_POINT('',#211169);
#39828=VERTEX_POINT('',#211174);
#39829=VERTEX_POINT('',#211175);
#39830=VERTEX_POINT('',#211183);
#39831=VERTEX_POINT('',#211184);
#39832=VERTEX_POINT('',#211186);
#39833=VERTEX_POINT('',#211188);
#39834=VERTEX_POINT('',#211192);
#39835=VERTEX_POINT('',#211193);
#39836=VERTEX_POINT('',#211198);
#39837=VERTEX_POINT('',#211199);
#39838=VERTEX_POINT('',#211204);
#39839=VERTEX_POINT('',#211205);
#39840=VERTEX_POINT('',#211210);
#39841=VERTEX_POINT('',#211211);
#39842=VERTEX_POINT('',#211216);
#39843=VERTEX_POINT('',#211217);
#39844=VERTEX_POINT('',#211222);
#39845=VERTEX_POINT('',#211223);
#39846=VERTEX_POINT('',#211231);
#39847=VERTEX_POINT('',#211232);
#39848=VERTEX_POINT('',#211234);
#39849=VERTEX_POINT('',#211236);
#39850=VERTEX_POINT('',#211240);
#39851=VERTEX_POINT('',#211241);
#39852=VERTEX_POINT('',#211246);
#39853=VERTEX_POINT('',#211247);
#39854=VERTEX_POINT('',#211252);
#39855=VERTEX_POINT('',#211253);
#39856=VERTEX_POINT('',#211258);
#39857=VERTEX_POINT('',#211259);
#39858=VERTEX_POINT('',#211264);
#39859=VERTEX_POINT('',#211265);
#39860=VERTEX_POINT('',#211270);
#39861=VERTEX_POINT('',#211271);
#39862=VERTEX_POINT('',#211276);
#39863=VERTEX_POINT('',#211277);
#39864=VERTEX_POINT('',#211285);
#39865=VERTEX_POINT('',#211286);
#39866=VERTEX_POINT('',#211288);
#39867=VERTEX_POINT('',#211290);
#39868=VERTEX_POINT('',#211294);
#39869=VERTEX_POINT('',#211295);
#39870=VERTEX_POINT('',#211300);
#39871=VERTEX_POINT('',#211301);
#39872=VERTEX_POINT('',#211306);
#39873=VERTEX_POINT('',#211307);
#39874=VERTEX_POINT('',#211312);
#39875=VERTEX_POINT('',#211313);
#39876=VERTEX_POINT('',#211318);
#39877=VERTEX_POINT('',#211319);
#39878=VERTEX_POINT('',#211324);
#39879=VERTEX_POINT('',#211325);
#39880=VERTEX_POINT('',#211333);
#39881=VERTEX_POINT('',#211334);
#39882=VERTEX_POINT('',#211336);
#39883=VERTEX_POINT('',#211338);
#39884=VERTEX_POINT('',#211342);
#39885=VERTEX_POINT('',#211343);
#39886=VERTEX_POINT('',#211348);
#39887=VERTEX_POINT('',#211349);
#39888=VERTEX_POINT('',#211354);
#39889=VERTEX_POINT('',#211355);
#39890=VERTEX_POINT('',#211360);
#39891=VERTEX_POINT('',#211361);
#39892=VERTEX_POINT('',#211366);
#39893=VERTEX_POINT('',#211367);
#39894=VERTEX_POINT('',#211372);
#39895=VERTEX_POINT('',#211373);
#39896=VERTEX_POINT('',#211381);
#39897=VERTEX_POINT('',#211382);
#39898=VERTEX_POINT('',#211384);
#39899=VERTEX_POINT('',#211386);
#39900=VERTEX_POINT('',#211390);
#39901=VERTEX_POINT('',#211391);
#39902=VERTEX_POINT('',#211396);
#39903=VERTEX_POINT('',#211397);
#39904=VERTEX_POINT('',#211402);
#39905=VERTEX_POINT('',#211403);
#39906=VERTEX_POINT('',#211408);
#39907=VERTEX_POINT('',#211409);
#39908=VERTEX_POINT('',#211414);
#39909=VERTEX_POINT('',#211415);
#39910=VERTEX_POINT('',#211420);
#39911=VERTEX_POINT('',#211421);
#39912=VERTEX_POINT('',#211429);
#39913=VERTEX_POINT('',#211430);
#39914=VERTEX_POINT('',#211432);
#39915=VERTEX_POINT('',#211434);
#39916=VERTEX_POINT('',#211438);
#39917=VERTEX_POINT('',#211439);
#39918=VERTEX_POINT('',#211444);
#39919=VERTEX_POINT('',#211445);
#39920=VERTEX_POINT('',#211450);
#39921=VERTEX_POINT('',#211451);
#39922=VERTEX_POINT('',#211456);
#39923=VERTEX_POINT('',#211457);
#39924=VERTEX_POINT('',#211462);
#39925=VERTEX_POINT('',#211463);
#39926=VERTEX_POINT('',#211468);
#39927=VERTEX_POINT('',#211469);
#39928=VERTEX_POINT('',#211477);
#39929=VERTEX_POINT('',#211478);
#39930=VERTEX_POINT('',#211480);
#39931=VERTEX_POINT('',#211482);
#39932=VERTEX_POINT('',#211486);
#39933=VERTEX_POINT('',#211487);
#39934=VERTEX_POINT('',#211492);
#39935=VERTEX_POINT('',#211493);
#39936=VERTEX_POINT('',#211498);
#39937=VERTEX_POINT('',#211499);
#39938=VERTEX_POINT('',#211504);
#39939=VERTEX_POINT('',#211505);
#39940=VERTEX_POINT('',#211510);
#39941=VERTEX_POINT('',#211511);
#39942=VERTEX_POINT('',#211516);
#39943=VERTEX_POINT('',#211517);
#39944=VERTEX_POINT('',#211525);
#39945=VERTEX_POINT('',#211526);
#39946=VERTEX_POINT('',#211528);
#39947=VERTEX_POINT('',#211530);
#39948=VERTEX_POINT('',#211534);
#39949=VERTEX_POINT('',#211535);
#39950=VERTEX_POINT('',#211540);
#39951=VERTEX_POINT('',#211541);
#39952=VERTEX_POINT('',#211546);
#39953=VERTEX_POINT('',#211547);
#39954=VERTEX_POINT('',#211552);
#39955=VERTEX_POINT('',#211553);
#39956=VERTEX_POINT('',#211558);
#39957=VERTEX_POINT('',#211559);
#39958=VERTEX_POINT('',#211564);
#39959=VERTEX_POINT('',#211565);
#39960=VERTEX_POINT('',#211570);
#39961=VERTEX_POINT('',#211571);
#39962=VERTEX_POINT('',#211576);
#39963=VERTEX_POINT('',#211577);
#39964=VERTEX_POINT('',#211585);
#39965=VERTEX_POINT('',#211586);
#39966=VERTEX_POINT('',#211588);
#39967=VERTEX_POINT('',#211590);
#39968=VERTEX_POINT('',#211594);
#39969=VERTEX_POINT('',#211595);
#39970=VERTEX_POINT('',#211600);
#39971=VERTEX_POINT('',#211601);
#39972=VERTEX_POINT('',#211606);
#39973=VERTEX_POINT('',#211607);
#39974=VERTEX_POINT('',#211612);
#39975=VERTEX_POINT('',#211613);
#39976=VERTEX_POINT('',#211618);
#39977=VERTEX_POINT('',#211619);
#39978=VERTEX_POINT('',#211624);
#39979=VERTEX_POINT('',#211625);
#39980=VERTEX_POINT('',#211633);
#39981=VERTEX_POINT('',#211634);
#39982=VERTEX_POINT('',#211636);
#39983=VERTEX_POINT('',#211638);
#39984=VERTEX_POINT('',#211642);
#39985=VERTEX_POINT('',#211643);
#39986=VERTEX_POINT('',#211648);
#39987=VERTEX_POINT('',#211649);
#39988=VERTEX_POINT('',#211654);
#39989=VERTEX_POINT('',#211655);
#39990=VERTEX_POINT('',#211660);
#39991=VERTEX_POINT('',#211661);
#39992=VERTEX_POINT('',#211666);
#39993=VERTEX_POINT('',#211667);
#39994=VERTEX_POINT('',#211672);
#39995=VERTEX_POINT('',#211673);
#39996=VERTEX_POINT('',#211681);
#39997=VERTEX_POINT('',#211682);
#39998=VERTEX_POINT('',#211684);
#39999=VERTEX_POINT('',#211686);
#40000=VERTEX_POINT('',#211690);
#40001=VERTEX_POINT('',#211691);
#40002=VERTEX_POINT('',#211696);
#40003=VERTEX_POINT('',#211697);
#40004=VERTEX_POINT('',#211702);
#40005=VERTEX_POINT('',#211703);
#40006=VERTEX_POINT('',#211708);
#40007=VERTEX_POINT('',#211709);
#40008=VERTEX_POINT('',#211714);
#40009=VERTEX_POINT('',#211715);
#40010=VERTEX_POINT('',#211720);
#40011=VERTEX_POINT('',#211721);
#40012=VERTEX_POINT('',#211726);
#40013=VERTEX_POINT('',#211727);
#40014=VERTEX_POINT('',#211732);
#40015=VERTEX_POINT('',#211733);
#40016=VERTEX_POINT('',#211741);
#40017=VERTEX_POINT('',#211742);
#40018=VERTEX_POINT('',#211744);
#40019=VERTEX_POINT('',#211746);
#40020=VERTEX_POINT('',#211750);
#40021=VERTEX_POINT('',#211751);
#40022=VERTEX_POINT('',#211756);
#40023=VERTEX_POINT('',#211757);
#40024=VERTEX_POINT('',#211762);
#40025=VERTEX_POINT('',#211763);
#40026=VERTEX_POINT('',#211768);
#40027=VERTEX_POINT('',#211769);
#40028=VERTEX_POINT('',#211774);
#40029=VERTEX_POINT('',#211775);
#40030=VERTEX_POINT('',#211780);
#40031=VERTEX_POINT('',#211781);
#40032=VERTEX_POINT('',#211786);
#40033=VERTEX_POINT('',#211787);
#40034=VERTEX_POINT('',#211792);
#40035=VERTEX_POINT('',#211793);
#40036=VERTEX_POINT('',#211801);
#40037=VERTEX_POINT('',#211802);
#40038=VERTEX_POINT('',#211804);
#40039=VERTEX_POINT('',#211806);
#40040=VERTEX_POINT('',#211810);
#40041=VERTEX_POINT('',#211811);
#40042=VERTEX_POINT('',#211816);
#40043=VERTEX_POINT('',#211817);
#40044=VERTEX_POINT('',#211822);
#40045=VERTEX_POINT('',#211823);
#40046=VERTEX_POINT('',#211828);
#40047=VERTEX_POINT('',#211829);
#40048=VERTEX_POINT('',#211834);
#40049=VERTEX_POINT('',#211835);
#40050=VERTEX_POINT('',#211840);
#40051=VERTEX_POINT('',#211841);
#40052=VERTEX_POINT('',#211849);
#40053=VERTEX_POINT('',#211850);
#40054=VERTEX_POINT('',#211852);
#40055=VERTEX_POINT('',#211854);
#40056=VERTEX_POINT('',#211858);
#40057=VERTEX_POINT('',#211859);
#40058=VERTEX_POINT('',#211864);
#40059=VERTEX_POINT('',#211865);
#40060=VERTEX_POINT('',#211870);
#40061=VERTEX_POINT('',#211871);
#40062=VERTEX_POINT('',#211876);
#40063=VERTEX_POINT('',#211877);
#40064=VERTEX_POINT('',#211882);
#40065=VERTEX_POINT('',#211883);
#40066=VERTEX_POINT('',#211888);
#40067=VERTEX_POINT('',#211889);
#40068=VERTEX_POINT('',#211897);
#40069=VERTEX_POINT('',#211898);
#40070=VERTEX_POINT('',#211900);
#40071=VERTEX_POINT('',#211902);
#40072=VERTEX_POINT('',#211906);
#40073=VERTEX_POINT('',#211907);
#40074=VERTEX_POINT('',#211912);
#40075=VERTEX_POINT('',#211913);
#40076=VERTEX_POINT('',#211918);
#40077=VERTEX_POINT('',#211919);
#40078=VERTEX_POINT('',#211924);
#40079=VERTEX_POINT('',#211925);
#40080=VERTEX_POINT('',#211930);
#40081=VERTEX_POINT('',#211931);
#40082=VERTEX_POINT('',#211936);
#40083=VERTEX_POINT('',#211937);
#40084=VERTEX_POINT('',#211945);
#40085=VERTEX_POINT('',#211946);
#40086=VERTEX_POINT('',#211948);
#40087=VERTEX_POINT('',#211950);
#40088=VERTEX_POINT('',#211954);
#40089=VERTEX_POINT('',#211955);
#40090=VERTEX_POINT('',#211960);
#40091=VERTEX_POINT('',#211961);
#40092=VERTEX_POINT('',#211966);
#40093=VERTEX_POINT('',#211967);
#40094=VERTEX_POINT('',#211972);
#40095=VERTEX_POINT('',#211973);
#40096=VERTEX_POINT('',#211978);
#40097=VERTEX_POINT('',#211979);
#40098=VERTEX_POINT('',#211984);
#40099=VERTEX_POINT('',#211985);
#40100=VERTEX_POINT('',#211993);
#40101=VERTEX_POINT('',#211994);
#40102=VERTEX_POINT('',#211996);
#40103=VERTEX_POINT('',#211998);
#40104=VERTEX_POINT('',#212002);
#40105=VERTEX_POINT('',#212003);
#40106=VERTEX_POINT('',#212008);
#40107=VERTEX_POINT('',#212009);
#40108=VERTEX_POINT('',#212014);
#40109=VERTEX_POINT('',#212015);
#40110=VERTEX_POINT('',#212020);
#40111=VERTEX_POINT('',#212021);
#40112=VERTEX_POINT('',#212026);
#40113=VERTEX_POINT('',#212027);
#40114=VERTEX_POINT('',#212032);
#40115=VERTEX_POINT('',#212033);
#40116=VERTEX_POINT('',#212038);
#40117=VERTEX_POINT('',#212040);
#40118=VERTEX_POINT('',#212047);
#40119=VERTEX_POINT('',#212048);
#40120=VERTEX_POINT('',#212050);
#40121=VERTEX_POINT('',#212052);
#40122=VERTEX_POINT('',#212056);
#40123=VERTEX_POINT('',#212057);
#40124=VERTEX_POINT('',#212062);
#40125=VERTEX_POINT('',#212063);
#40126=VERTEX_POINT('',#212068);
#40127=VERTEX_POINT('',#212069);
#40128=VERTEX_POINT('',#212074);
#40129=VERTEX_POINT('',#212075);
#40130=VERTEX_POINT('',#212080);
#40131=VERTEX_POINT('',#212081);
#40132=VERTEX_POINT('',#212086);
#40133=VERTEX_POINT('',#212087);
#40134=VERTEX_POINT('',#212095);
#40135=VERTEX_POINT('',#212096);
#40136=VERTEX_POINT('',#212098);
#40137=VERTEX_POINT('',#212100);
#40138=VERTEX_POINT('',#212104);
#40139=VERTEX_POINT('',#212105);
#40140=VERTEX_POINT('',#212110);
#40141=VERTEX_POINT('',#212111);
#40142=VERTEX_POINT('',#212116);
#40143=VERTEX_POINT('',#212117);
#40144=VERTEX_POINT('',#212122);
#40145=VERTEX_POINT('',#212123);
#40146=VERTEX_POINT('',#212128);
#40147=VERTEX_POINT('',#212129);
#40148=VERTEX_POINT('',#212134);
#40149=VERTEX_POINT('',#212135);
#40150=VERTEX_POINT('',#212140);
#40151=VERTEX_POINT('',#212141);
#40152=VERTEX_POINT('',#212146);
#40153=VERTEX_POINT('',#212147);
#40154=VERTEX_POINT('',#212155);
#40155=VERTEX_POINT('',#212156);
#40156=VERTEX_POINT('',#212158);
#40157=VERTEX_POINT('',#212160);
#40158=VERTEX_POINT('',#212164);
#40159=VERTEX_POINT('',#212165);
#40160=VERTEX_POINT('',#212170);
#40161=VERTEX_POINT('',#212171);
#40162=VERTEX_POINT('',#212176);
#40163=VERTEX_POINT('',#212177);
#40164=VERTEX_POINT('',#212182);
#40165=VERTEX_POINT('',#212183);
#40166=VERTEX_POINT('',#212188);
#40167=VERTEX_POINT('',#212189);
#40168=VERTEX_POINT('',#212194);
#40169=VERTEX_POINT('',#212195);
#40170=VERTEX_POINT('',#212203);
#40171=VERTEX_POINT('',#212204);
#40172=VERTEX_POINT('',#212206);
#40173=VERTEX_POINT('',#212208);
#40174=VERTEX_POINT('',#212212);
#40175=VERTEX_POINT('',#212213);
#40176=VERTEX_POINT('',#212218);
#40177=VERTEX_POINT('',#212219);
#40178=VERTEX_POINT('',#212224);
#40179=VERTEX_POINT('',#212225);
#40180=VERTEX_POINT('',#212230);
#40181=VERTEX_POINT('',#212231);
#40182=VERTEX_POINT('',#212236);
#40183=VERTEX_POINT('',#212237);
#40184=VERTEX_POINT('',#212242);
#40185=VERTEX_POINT('',#212243);
#40186=VERTEX_POINT('',#212248);
#40187=VERTEX_POINT('',#212249);
#40188=VERTEX_POINT('',#212254);
#40189=VERTEX_POINT('',#212255);
#40190=VERTEX_POINT('',#212263);
#40191=VERTEX_POINT('',#212264);
#40192=VERTEX_POINT('',#212266);
#40193=VERTEX_POINT('',#212268);
#40194=VERTEX_POINT('',#212272);
#40195=VERTEX_POINT('',#212273);
#40196=VERTEX_POINT('',#212278);
#40197=VERTEX_POINT('',#212279);
#40198=VERTEX_POINT('',#212284);
#40199=VERTEX_POINT('',#212285);
#40200=VERTEX_POINT('',#212290);
#40201=VERTEX_POINT('',#212291);
#40202=VERTEX_POINT('',#212296);
#40203=VERTEX_POINT('',#212297);
#40204=VERTEX_POINT('',#212302);
#40205=VERTEX_POINT('',#212303);
#40206=VERTEX_POINT('',#212311);
#40207=VERTEX_POINT('',#212312);
#40208=VERTEX_POINT('',#212314);
#40209=VERTEX_POINT('',#212316);
#40210=VERTEX_POINT('',#212320);
#40211=VERTEX_POINT('',#212321);
#40212=VERTEX_POINT('',#212326);
#40213=VERTEX_POINT('',#212327);
#40214=VERTEX_POINT('',#212332);
#40215=VERTEX_POINT('',#212333);
#40216=VERTEX_POINT('',#212338);
#40217=VERTEX_POINT('',#212339);
#40218=VERTEX_POINT('',#212344);
#40219=VERTEX_POINT('',#212345);
#40220=VERTEX_POINT('',#212350);
#40221=VERTEX_POINT('',#212351);
#40222=VERTEX_POINT('',#212359);
#40223=VERTEX_POINT('',#212360);
#40224=VERTEX_POINT('',#212362);
#40225=VERTEX_POINT('',#212364);
#40226=VERTEX_POINT('',#212368);
#40227=VERTEX_POINT('',#212369);
#40228=VERTEX_POINT('',#212374);
#40229=VERTEX_POINT('',#212375);
#40230=VERTEX_POINT('',#212380);
#40231=VERTEX_POINT('',#212381);
#40232=VERTEX_POINT('',#212386);
#40233=VERTEX_POINT('',#212387);
#40234=VERTEX_POINT('',#212392);
#40235=VERTEX_POINT('',#212393);
#40236=VERTEX_POINT('',#212398);
#40237=VERTEX_POINT('',#212399);
#40238=VERTEX_POINT('',#212407);
#40239=VERTEX_POINT('',#212408);
#40240=VERTEX_POINT('',#212410);
#40241=VERTEX_POINT('',#212412);
#40242=VERTEX_POINT('',#212416);
#40243=VERTEX_POINT('',#212417);
#40244=VERTEX_POINT('',#212422);
#40245=VERTEX_POINT('',#212423);
#40246=VERTEX_POINT('',#212428);
#40247=VERTEX_POINT('',#212429);
#40248=VERTEX_POINT('',#212434);
#40249=VERTEX_POINT('',#212435);
#40250=VERTEX_POINT('',#212440);
#40251=VERTEX_POINT('',#212441);
#40252=VERTEX_POINT('',#212446);
#40253=VERTEX_POINT('',#212447);
#40254=VERTEX_POINT('',#212455);
#40255=VERTEX_POINT('',#212456);
#40256=VERTEX_POINT('',#212458);
#40257=VERTEX_POINT('',#212460);
#40258=VERTEX_POINT('',#212464);
#40259=VERTEX_POINT('',#212465);
#40260=VERTEX_POINT('',#212470);
#40261=VERTEX_POINT('',#212471);
#40262=VERTEX_POINT('',#212476);
#40263=VERTEX_POINT('',#212477);
#40264=VERTEX_POINT('',#212482);
#40265=VERTEX_POINT('',#212483);
#40266=VERTEX_POINT('',#212491);
#40267=VERTEX_POINT('',#212492);
#40268=VERTEX_POINT('',#212494);
#40269=VERTEX_POINT('',#212496);
#40270=VERTEX_POINT('',#212500);
#40271=VERTEX_POINT('',#212501);
#40272=VERTEX_POINT('',#212506);
#40273=VERTEX_POINT('',#212507);
#40274=VERTEX_POINT('',#212512);
#40275=VERTEX_POINT('',#212513);
#40276=VERTEX_POINT('',#212518);
#40277=VERTEX_POINT('',#212519);
#40278=VERTEX_POINT('',#212527);
#40279=VERTEX_POINT('',#212529);
#40280=VERTEX_POINT('',#212533);
#40281=VERTEX_POINT('',#212535);
#40282=VERTEX_POINT('',#212539);
#40283=VERTEX_POINT('',#212540);
#40284=VERTEX_POINT('',#212545);
#40285=VERTEX_POINT('',#212546);
#40286=VERTEX_POINT('',#212551);
#40287=VERTEX_POINT('',#212552);
#40288=VERTEX_POINT('',#212557);
#40289=VERTEX_POINT('',#212558);
#40290=VERTEX_POINT('',#212563);
#40291=VERTEX_POINT('',#212564);
#40292=VERTEX_POINT('',#212569);
#40293=VERTEX_POINT('',#212570);
#40294=VERTEX_POINT('',#212575);
#40295=VERTEX_POINT('',#212576);
#40296=VERTEX_POINT('',#212581);
#40297=VERTEX_POINT('',#212582);
#40298=VERTEX_POINT('',#212590);
#40299=VERTEX_POINT('',#212591);
#40300=VERTEX_POINT('',#212596);
#40301=VERTEX_POINT('',#212597);
#40302=VERTEX_POINT('',#212602);
#40303=VERTEX_POINT('',#212603);
#40304=VERTEX_POINT('',#212608);
#40305=VERTEX_POINT('',#212609);
#40306=VERTEX_POINT('',#212614);
#40307=VERTEX_POINT('',#212615);
#40308=VERTEX_POINT('',#212620);
#40309=VERTEX_POINT('',#212621);
#40310=VERTEX_POINT('',#212626);
#40311=VERTEX_POINT('',#212627);
#40312=VERTEX_POINT('',#212632);
#40313=VERTEX_POINT('',#212633);
#40314=VERTEX_POINT('',#212641);
#40315=VERTEX_POINT('',#212642);
#40316=VERTEX_POINT('',#212644);
#40317=VERTEX_POINT('',#212646);
#40318=VERTEX_POINT('',#212659);
#40319=VERTEX_POINT('',#212660);
#40320=VERTEX_POINT('',#212665);
#40321=VERTEX_POINT('',#212667);
#40322=VERTEX_POINT('',#212671);
#40323=VERTEX_POINT('',#212672);
#40324=VERTEX_POINT('',#212677);
#40325=VERTEX_POINT('',#212678);
#40326=VERTEX_POINT('',#212683);
#40327=VERTEX_POINT('',#212684);
#40328=VERTEX_POINT('',#212689);
#40329=VERTEX_POINT('',#212690);
#40330=VERTEX_POINT('',#212704);
#40331=VERTEX_POINT('',#212705);
#40332=VERTEX_POINT('',#212707);
#40333=VERTEX_POINT('',#212709);
#40334=VERTEX_POINT('',#212722);
#40335=VERTEX_POINT('',#212723);
#40336=VERTEX_POINT('',#212728);
#40337=VERTEX_POINT('',#212729);
#40338=VERTEX_POINT('',#212734);
#40339=VERTEX_POINT('',#212735);
#40340=VERTEX_POINT('',#212740);
#40341=VERTEX_POINT('',#212741);
#40342=VERTEX_POINT('',#212746);
#40343=VERTEX_POINT('',#212747);
#40344=VERTEX_POINT('',#212752);
#40345=VERTEX_POINT('',#212753);
#40346=VERTEX_POINT('',#212767);
#40347=VERTEX_POINT('',#212768);
#40348=VERTEX_POINT('',#212770);
#40349=VERTEX_POINT('',#212772);
#40350=VERTEX_POINT('',#212785);
#40351=VERTEX_POINT('',#212786);
#40352=VERTEX_POINT('',#212791);
#40353=VERTEX_POINT('',#212793);
#40354=VERTEX_POINT('',#212797);
#40355=VERTEX_POINT('',#212798);
#40356=VERTEX_POINT('',#212803);
#40357=VERTEX_POINT('',#212804);
#40358=VERTEX_POINT('',#212809);
#40359=VERTEX_POINT('',#212810);
#40360=VERTEX_POINT('',#212815);
#40361=VERTEX_POINT('',#212816);
#40362=VERTEX_POINT('',#212830);
#40363=VERTEX_POINT('',#212831);
#40364=VERTEX_POINT('',#212842);
#40365=VERTEX_POINT('',#212844);
#40366=VERTEX_POINT('',#212848);
#40367=VERTEX_POINT('',#212849);
#40368=VERTEX_POINT('',#212854);
#40369=VERTEX_POINT('',#212855);
#40370=VERTEX_POINT('',#212860);
#40371=VERTEX_POINT('',#212861);
#40372=VERTEX_POINT('',#212866);
#40373=VERTEX_POINT('',#212867);
#40374=VERTEX_POINT('',#212872);
#40375=VERTEX_POINT('',#212873);
#40376=VERTEX_POINT('',#212878);
#40377=VERTEX_POINT('',#212879);
#40378=VERTEX_POINT('',#212893);
#40379=VERTEX_POINT('',#212895);
#40380=VERTEX_POINT('',#212899);
#40381=VERTEX_POINT('',#212900);
#40382=VERTEX_POINT('',#212905);
#40383=VERTEX_POINT('',#212906);
#40384=VERTEX_POINT('',#212911);
#40385=VERTEX_POINT('',#212912);
#40386=VERTEX_POINT('',#212917);
#40387=VERTEX_POINT('',#212918);
#40388=VERTEX_POINT('',#212923);
#40389=VERTEX_POINT('',#212924);
#40390=VERTEX_POINT('',#212929);
#40391=VERTEX_POINT('',#212930);
#40392=VERTEX_POINT('',#212935);
#40393=VERTEX_POINT('',#212936);
#40394=VERTEX_POINT('',#213087);
#40395=VERTEX_POINT('',#213088);
#40396=VERTEX_POINT('',#213141);
#40397=VERTEX_POINT('',#213176);
#40398=VERTEX_POINT('',#213408);
#40399=VERTEX_POINT('',#213409);
#40400=VERTEX_POINT('',#213428);
#40401=VERTEX_POINT('',#213429);
#40402=VERTEX_POINT('',#213511);
#40403=VERTEX_POINT('',#213512);
#40404=VERTEX_POINT('',#213662);
#40405=VERTEX_POINT('',#213663);
#40406=VERTEX_POINT('',#213895);
#40407=VERTEX_POINT('',#213896);
#40408=VERTEX_POINT('',#214052);
#40409=VERTEX_POINT('',#214053);
#40410=VERTEX_POINT('',#214069);
#40411=VERTEX_POINT('',#214070);
#40412=VERTEX_POINT('',#214401);
#40413=VERTEX_POINT('',#214402);
#40414=VERTEX_POINT('',#214558);
#40415=VERTEX_POINT('',#214593);
#40416=VERTEX_POINT('',#214600);
#40417=VERTEX_POINT('',#214626);
#40418=VERTEX_POINT('',#214802);
#40419=VERTEX_POINT('',#214925);
#40420=VERTEX_POINT('',#214926);
#40421=VERTEX_POINT('',#214960);
#40422=VERTEX_POINT('',#214961);
#40423=VERTEX_POINT('',#215061);
#40424=VERTEX_POINT('',#215062);
#40425=VERTEX_POINT('',#215390);
#40426=VERTEX_POINT('',#215391);
#40427=VERTEX_POINT('',#215635);
#40428=VERTEX_POINT('',#215636);
#40429=VERTEX_POINT('',#215773);
#40430=VERTEX_POINT('',#215774);
#40431=VERTEX_POINT('',#215790);
#40432=VERTEX_POINT('',#215791);
#40433=VERTEX_POINT('',#216122);
#40434=VERTEX_POINT('',#216123);
#40435=VERTEX_POINT('',#216224);
#40436=VERTEX_POINT('',#216271);
#40437=VERTEX_POINT('',#216604);
#40438=VERTEX_POINT('',#216739);
#40439=VERTEX_POINT('',#216762);
#40440=VERTEX_POINT('',#216777);
#40441=VERTEX_POINT('',#216778);
#40442=VERTEX_POINT('',#216860);
#40443=VERTEX_POINT('',#216861);
#40444=VERTEX_POINT('',#217213);
#40445=VERTEX_POINT('',#217214);
#40446=VERTEX_POINT('',#217260);
#40447=VERTEX_POINT('',#217261);
#40448=VERTEX_POINT('',#217278);
#40449=VERTEX_POINT('',#217293);
#40450=VERTEX_POINT('',#217294);
#40451=VERTEX_POINT('',#217752);
#40452=VERTEX_POINT('',#217753);
#40453=VERTEX_POINT('',#218158);
#40454=VERTEX_POINT('',#218238);
#40455=VERTEX_POINT('',#218306);
#40456=VERTEX_POINT('',#218345);
#40457=VERTEX_POINT('',#218378);
#40458=VERTEX_POINT('',#218503);
#40459=VERTEX_POINT('',#218571);
#40460=VERTEX_POINT('',#218591);
#40461=VERTEX_POINT('',#218592);
#40462=VERTEX_POINT('',#218617);
#40463=VERTEX_POINT('',#218619);
#40464=VERTEX_POINT('',#218640);
#40465=VERTEX_POINT('',#218641);
#40466=VERTEX_POINT('',#218741);
#40467=VERTEX_POINT('',#218742);
#40468=VERTEX_POINT('',#219016);
#40469=VERTEX_POINT('',#219017);
#40470=VERTEX_POINT('',#219446);
#40471=VERTEX_POINT('',#219447);
#40472=VERTEX_POINT('',#219462);
#40473=VERTEX_POINT('',#219479);
#40474=VERTEX_POINT('',#219826);
#40475=VERTEX_POINT('',#219841);
#40476=VERTEX_POINT('',#219867);
#40477=VERTEX_POINT('',#219932);
#40478=VERTEX_POINT('',#219967);
#40479=VERTEX_POINT('',#220114);
#40480=VERTEX_POINT('',#220129);
#40481=VERTEX_POINT('',#220130);
#40482=VERTEX_POINT('',#220146);
#40483=VERTEX_POINT('',#220148);
#40484=VERTEX_POINT('',#220181);
#40485=VERTEX_POINT('',#220182);
#40486=VERTEX_POINT('',#220396);
#40487=VERTEX_POINT('',#220397);
#40488=VERTEX_POINT('',#220606);
#40489=VERTEX_POINT('',#220607);
#40490=VERTEX_POINT('',#220644);
#40491=VERTEX_POINT('',#220646);
#40492=VERTEX_POINT('',#220835);
#40493=VERTEX_POINT('',#220836);
#40494=VERTEX_POINT('',#220881);
#40495=VERTEX_POINT('',#221048);
#40496=VERTEX_POINT('',#221113);
#40497=VERTEX_POINT('',#221287);
#40498=VERTEX_POINT('',#221329);
#40499=VERTEX_POINT('',#221330);
#40500=VERTEX_POINT('',#221342);
#40501=VERTEX_POINT('',#221357);
#40502=VERTEX_POINT('',#221396);
#40503=VERTEX_POINT('',#221397);
#40504=VERTEX_POINT('',#221499);
#40505=VERTEX_POINT('',#221500);
#40506=VERTEX_POINT('',#221825);
#40507=VERTEX_POINT('',#221826);
#40508=VERTEX_POINT('',#222189);
#40509=VERTEX_POINT('',#222190);
#40510=VERTEX_POINT('',#222195);
#40511=VERTEX_POINT('',#222197);
#40512=VERTEX_POINT('',#222201);
#40513=VERTEX_POINT('',#222203);
#40514=VERTEX_POINT('',#222207);
#40515=VERTEX_POINT('',#222209);
#40516=VERTEX_POINT('',#222213);
#40517=VERTEX_POINT('',#222215);
#40518=VERTEX_POINT('',#222219);
#40519=VERTEX_POINT('',#222221);
#40520=VERTEX_POINT('',#222225);
#40521=VERTEX_POINT('',#222227);
#40522=VERTEX_POINT('',#222231);
#40523=VERTEX_POINT('',#222233);
#40524=VERTEX_POINT('',#222237);
#40525=VERTEX_POINT('',#222239);
#40526=VERTEX_POINT('',#222243);
#40527=VERTEX_POINT('',#222244);
#40528=VERTEX_POINT('',#222249);
#40529=VERTEX_POINT('',#222251);
#40530=VERTEX_POINT('',#222255);
#40531=VERTEX_POINT('',#222257);
#40532=VERTEX_POINT('',#222261);
#40533=VERTEX_POINT('',#222263);
#40534=VERTEX_POINT('',#222267);
#40535=VERTEX_POINT('',#222269);
#40536=VERTEX_POINT('',#222273);
#40537=VERTEX_POINT('',#222275);
#40538=VERTEX_POINT('',#222279);
#40539=VERTEX_POINT('',#222281);
#40540=VERTEX_POINT('',#222285);
#40541=VERTEX_POINT('',#222287);
#40542=VERTEX_POINT('',#222291);
#40543=VERTEX_POINT('',#222293);
#40544=VERTEX_POINT('',#222297);
#40545=VERTEX_POINT('',#222299);
#40546=VERTEX_POINT('',#222303);
#40547=VERTEX_POINT('',#222305);
#40548=VERTEX_POINT('',#222309);
#40549=VERTEX_POINT('',#222311);
#40550=VERTEX_POINT('',#222315);
#40551=VERTEX_POINT('',#222317);
#40552=VERTEX_POINT('',#222321);
#40553=VERTEX_POINT('',#222323);
#40554=VERTEX_POINT('',#222327);
#40555=VERTEX_POINT('',#222329);
#40556=VERTEX_POINT('',#222333);
#40557=VERTEX_POINT('',#222335);
#40558=VERTEX_POINT('',#222339);
#40559=VERTEX_POINT('',#222341);
#40560=VERTEX_POINT('',#222345);
#40561=VERTEX_POINT('',#222347);
#40562=VERTEX_POINT('',#222351);
#40563=VERTEX_POINT('',#222352);
#40564=VERTEX_POINT('',#222357);
#40565=VERTEX_POINT('',#222359);
#40566=VERTEX_POINT('',#222363);
#40567=VERTEX_POINT('',#222365);
#40568=VERTEX_POINT('',#222369);
#40569=VERTEX_POINT('',#222371);
#40570=VERTEX_POINT('',#222375);
#40571=VERTEX_POINT('',#222377);
#40572=VERTEX_POINT('',#222381);
#40573=VERTEX_POINT('',#222383);
#40574=VERTEX_POINT('',#222387);
#40575=VERTEX_POINT('',#222389);
#40576=VERTEX_POINT('',#222393);
#40577=VERTEX_POINT('',#222395);
#40578=VERTEX_POINT('',#222399);
#40579=VERTEX_POINT('',#222401);
#40580=VERTEX_POINT('',#222405);
#40581=VERTEX_POINT('',#222407);
#40582=VERTEX_POINT('',#222411);
#40583=VERTEX_POINT('',#222413);
#40584=VERTEX_POINT('',#222417);
#40585=VERTEX_POINT('',#222419);
#40586=VERTEX_POINT('',#222423);
#40587=VERTEX_POINT('',#222425);
#40588=VERTEX_POINT('',#222429);
#40589=VERTEX_POINT('',#222431);
#40590=VERTEX_POINT('',#222435);
#40591=VERTEX_POINT('',#222437);
#40592=VERTEX_POINT('',#222441);
#40593=VERTEX_POINT('',#222443);
#40594=VERTEX_POINT('',#222447);
#40595=VERTEX_POINT('',#222449);
#40596=VERTEX_POINT('',#222453);
#40597=VERTEX_POINT('',#222455);
#40598=VERTEX_POINT('',#222459);
#40599=VERTEX_POINT('',#222461);
#40600=VERTEX_POINT('',#222465);
#40601=VERTEX_POINT('',#222467);
#40602=VERTEX_POINT('',#222471);
#40603=VERTEX_POINT('',#222473);
#40604=VERTEX_POINT('',#222477);
#40605=VERTEX_POINT('',#222479);
#40606=VERTEX_POINT('',#222483);
#40607=VERTEX_POINT('',#222485);
#40608=VERTEX_POINT('',#222489);
#40609=VERTEX_POINT('',#222491);
#40610=VERTEX_POINT('',#222495);
#40611=VERTEX_POINT('',#222497);
#40612=VERTEX_POINT('',#222501);
#40613=VERTEX_POINT('',#222503);
#40614=VERTEX_POINT('',#222507);
#40615=VERTEX_POINT('',#222509);
#40616=VERTEX_POINT('',#222513);
#40617=VERTEX_POINT('',#222515);
#40618=VERTEX_POINT('',#222519);
#40619=VERTEX_POINT('',#222521);
#40620=VERTEX_POINT('',#222525);
#40621=VERTEX_POINT('',#222527);
#40622=VERTEX_POINT('',#222531);
#40623=VERTEX_POINT('',#222533);
#40624=VERTEX_POINT('',#222537);
#40625=VERTEX_POINT('',#222539);
#40626=VERTEX_POINT('',#222543);
#40627=VERTEX_POINT('',#222545);
#40628=VERTEX_POINT('',#222549);
#40629=VERTEX_POINT('',#222551);
#40630=VERTEX_POINT('',#222555);
#40631=VERTEX_POINT('',#222557);
#40632=VERTEX_POINT('',#222561);
#40633=VERTEX_POINT('',#222563);
#40634=VERTEX_POINT('',#222567);
#40635=VERTEX_POINT('',#222569);
#40636=VERTEX_POINT('',#222573);
#40637=VERTEX_POINT('',#222575);
#40638=VERTEX_POINT('',#222579);
#40639=VERTEX_POINT('',#222581);
#40640=VERTEX_POINT('',#222585);
#40641=VERTEX_POINT('',#222587);
#40642=VERTEX_POINT('',#222591);
#40643=VERTEX_POINT('',#222593);
#40644=VERTEX_POINT('',#222597);
#40645=VERTEX_POINT('',#222599);
#40646=VERTEX_POINT('',#222603);
#40647=VERTEX_POINT('',#222605);
#40648=VERTEX_POINT('',#222609);
#40649=VERTEX_POINT('',#222611);
#40650=VERTEX_POINT('',#222615);
#40651=VERTEX_POINT('',#222617);
#40652=VERTEX_POINT('',#222621);
#40653=VERTEX_POINT('',#222623);
#40654=VERTEX_POINT('',#222627);
#40655=VERTEX_POINT('',#222629);
#40656=VERTEX_POINT('',#222633);
#40657=VERTEX_POINT('',#222635);
#40658=VERTEX_POINT('',#222639);
#40659=VERTEX_POINT('',#222641);
#40660=VERTEX_POINT('',#222645);
#40661=VERTEX_POINT('',#222647);
#40662=VERTEX_POINT('',#222651);
#40663=VERTEX_POINT('',#222653);
#40664=VERTEX_POINT('',#222657);
#40665=VERTEX_POINT('',#222659);
#40666=VERTEX_POINT('',#222663);
#40667=VERTEX_POINT('',#222665);
#40668=VERTEX_POINT('',#222669);
#40669=VERTEX_POINT('',#222671);
#40670=VERTEX_POINT('',#222675);
#40671=VERTEX_POINT('',#222677);
#40672=VERTEX_POINT('',#222681);
#40673=VERTEX_POINT('',#222683);
#40674=VERTEX_POINT('',#222687);
#40675=VERTEX_POINT('',#222689);
#40676=VERTEX_POINT('',#222693);
#40677=VERTEX_POINT('',#222695);
#40678=VERTEX_POINT('',#222699);
#40679=VERTEX_POINT('',#222700);
#40680=VERTEX_POINT('',#222705);
#40681=VERTEX_POINT('',#222707);
#40682=VERTEX_POINT('',#222711);
#40683=VERTEX_POINT('',#222713);
#40684=VERTEX_POINT('',#222717);
#40685=VERTEX_POINT('',#222719);
#40686=VERTEX_POINT('',#222723);
#40687=VERTEX_POINT('',#222725);
#40688=VERTEX_POINT('',#222729);
#40689=VERTEX_POINT('',#222731);
#40690=VERTEX_POINT('',#222735);
#40691=VERTEX_POINT('',#222737);
#40692=VERTEX_POINT('',#222741);
#40693=VERTEX_POINT('',#222743);
#40694=VERTEX_POINT('',#222747);
#40695=VERTEX_POINT('',#222749);
#40696=VERTEX_POINT('',#222753);
#40697=VERTEX_POINT('',#222755);
#40698=VERTEX_POINT('',#222759);
#40699=VERTEX_POINT('',#222761);
#40700=VERTEX_POINT('',#222765);
#40701=VERTEX_POINT('',#222767);
#40702=VERTEX_POINT('',#222771);
#40703=VERTEX_POINT('',#222773);
#40704=VERTEX_POINT('',#222777);
#40705=VERTEX_POINT('',#222779);
#40706=VERTEX_POINT('',#222783);
#40707=VERTEX_POINT('',#222785);
#40708=VERTEX_POINT('',#222789);
#40709=VERTEX_POINT('',#222791);
#40710=VERTEX_POINT('',#222795);
#40711=VERTEX_POINT('',#222797);
#40712=VERTEX_POINT('',#222801);
#40713=VERTEX_POINT('',#222803);
#40714=VERTEX_POINT('',#222807);
#40715=VERTEX_POINT('',#222809);
#40716=VERTEX_POINT('',#222813);
#40717=VERTEX_POINT('',#222815);
#40718=VERTEX_POINT('',#222819);
#40719=VERTEX_POINT('',#222821);
#40720=VERTEX_POINT('',#222825);
#40721=VERTEX_POINT('',#222827);
#40722=VERTEX_POINT('',#222831);
#40723=VERTEX_POINT('',#222833);
#40724=VERTEX_POINT('',#222837);
#40725=VERTEX_POINT('',#222839);
#40726=VERTEX_POINT('',#222843);
#40727=VERTEX_POINT('',#222844);
#40728=VERTEX_POINT('',#222849);
#40729=VERTEX_POINT('',#222851);
#40730=VERTEX_POINT('',#222855);
#40731=VERTEX_POINT('',#222857);
#40732=VERTEX_POINT('',#222861);
#40733=VERTEX_POINT('',#222863);
#40734=VERTEX_POINT('',#222867);
#40735=VERTEX_POINT('',#222869);
#40736=VERTEX_POINT('',#222873);
#40737=VERTEX_POINT('',#222875);
#40738=VERTEX_POINT('',#222879);
#40739=VERTEX_POINT('',#222881);
#40740=VERTEX_POINT('',#222885);
#40741=VERTEX_POINT('',#222887);
#40742=VERTEX_POINT('',#222891);
#40743=VERTEX_POINT('',#222893);
#40744=VERTEX_POINT('',#222897);
#40745=VERTEX_POINT('',#222899);
#40746=VERTEX_POINT('',#222903);
#40747=VERTEX_POINT('',#222905);
#40748=VERTEX_POINT('',#222909);
#40749=VERTEX_POINT('',#222911);
#40750=VERTEX_POINT('',#222915);
#40751=VERTEX_POINT('',#222917);
#40752=VERTEX_POINT('',#222921);
#40753=VERTEX_POINT('',#222923);
#40754=VERTEX_POINT('',#222927);
#40755=VERTEX_POINT('',#222929);
#40756=VERTEX_POINT('',#222933);
#40757=VERTEX_POINT('',#222935);
#40758=VERTEX_POINT('',#222939);
#40759=VERTEX_POINT('',#222940);
#40760=VERTEX_POINT('',#222945);
#40761=VERTEX_POINT('',#222947);
#40762=VERTEX_POINT('',#222951);
#40763=VERTEX_POINT('',#222953);
#40764=VERTEX_POINT('',#222957);
#40765=VERTEX_POINT('',#222959);
#40766=VERTEX_POINT('',#222963);
#40767=VERTEX_POINT('',#222965);
#40768=VERTEX_POINT('',#222969);
#40769=VERTEX_POINT('',#222970);
#40770=VERTEX_POINT('',#222975);
#40771=VERTEX_POINT('',#222977);
#40772=VERTEX_POINT('',#222981);
#40773=VERTEX_POINT('',#222982);
#40774=VERTEX_POINT('',#222987);
#40775=VERTEX_POINT('',#222989);
#40776=VERTEX_POINT('',#222993);
#40777=VERTEX_POINT('',#222995);
#40778=VERTEX_POINT('',#222999);
#40779=VERTEX_POINT('',#223001);
#40780=VERTEX_POINT('',#223005);
#40781=VERTEX_POINT('',#223009);
#40782=VERTEX_POINT('',#223013);
#40783=VERTEX_POINT('',#223023);
#40784=VERTEX_POINT('',#223127);
#40785=VERTEX_POINT('',#223128);
#40786=VERTEX_POINT('',#223130);
#40787=VERTEX_POINT('',#223132);
#40788=VERTEX_POINT('',#223136);
#40789=VERTEX_POINT('',#223137);
#40790=VERTEX_POINT('',#223142);
#40791=VERTEX_POINT('',#223144);
#40792=VERTEX_POINT('',#223193);
#40793=VERTEX_POINT('',#223195);
#40794=VERTEX_POINT('',#223197);
#40795=VERTEX_POINT('',#223199);
#40796=VERTEX_POINT('',#223201);
#40797=VERTEX_POINT('',#223203);
#40798=VERTEX_POINT('',#223205);
#40799=VERTEX_POINT('',#223207);
#40800=VERTEX_POINT('',#223231);
#40801=VERTEX_POINT('',#223233);
#40802=VERTEX_POINT('',#223238);
#40803=VERTEX_POINT('',#223240);
#40804=VERTEX_POINT('',#223267);
#40805=VERTEX_POINT('',#223269);
#40806=VERTEX_POINT('',#223273);
#40807=VERTEX_POINT('',#223275);
#40808=VERTEX_POINT('',#223293);
#40809=VERTEX_POINT('',#223295);
#40810=VERTEX_POINT('',#223299);
#40811=VERTEX_POINT('',#223303);
#40812=VERTEX_POINT('',#223307);
#40813=VERTEX_POINT('',#223311);
#40814=VERTEX_POINT('',#223315);
#40815=VERTEX_POINT('',#223319);
#40816=VERTEX_POINT('',#223325);
#40817=VERTEX_POINT('',#223326);
#40818=VERTEX_POINT('',#223328);
#40819=VERTEX_POINT('',#223335);
#40820=VERTEX_POINT('',#223339);
#40821=VERTEX_POINT('',#223343);
#40822=VERTEX_POINT('',#223344);
#40823=VERTEX_POINT('',#223346);
#40824=VERTEX_POINT('',#223355);
#40825=VERTEX_POINT('',#223364);
#40826=VERTEX_POINT('',#223365);
#40827=VERTEX_POINT('',#223369);
#40828=VERTEX_POINT('',#223376);
#40829=VERTEX_POINT('',#223380);
#40830=VERTEX_POINT('',#223381);
#40831=VERTEX_POINT('',#223385);
#40832=VERTEX_POINT('',#223387);
#40833=VERTEX_POINT('',#223399);
#40834=VERTEX_POINT('',#223400);
#40835=VERTEX_POINT('',#223404);
#40836=VERTEX_POINT('',#223406);
#40837=VERTEX_POINT('',#223415);
#40838=VERTEX_POINT('',#223416);
#40839=VERTEX_POINT('',#223420);
#40840=VERTEX_POINT('',#223427);
#40841=VERTEX_POINT('',#224658);
#40842=VERTEX_POINT('',#224659);
#40843=VERTEX_POINT('',#224674);
#40844=VERTEX_POINT('',#224681);
#40845=VERTEX_POINT('',#224702);
#40846=VERTEX_POINT('',#224899);
#40847=VERTEX_POINT('',#224940);
#40848=VERTEX_POINT('',#224947);
#40849=VERTEX_POINT('',#224968);
#40850=VERTEX_POINT('',#224975);
#40851=VERTEX_POINT('',#225592);
#40852=VERTEX_POINT('',#225593);
#40853=VERTEX_POINT('',#225600);
#40854=VERTEX_POINT('',#225862);
#40855=VERTEX_POINT('',#225873);
#40856=VERTEX_POINT('',#225880);
#40857=VERTEX_POINT('',#225891);
#40858=VERTEX_POINT('',#225924);
#40859=VERTEX_POINT('',#225925);
#40860=VERTEX_POINT('',#225927);
#40861=VERTEX_POINT('',#225929);
#40862=VERTEX_POINT('',#225936);
#40863=VERTEX_POINT('',#225938);
#40864=VERTEX_POINT('',#225944);
#40865=VERTEX_POINT('',#225946);
#40866=VERTEX_POINT('',#225950);
#40867=VERTEX_POINT('',#225952);
#40868=VERTEX_POINT('',#225956);
#40869=VERTEX_POINT('',#225958);
#40870=VERTEX_POINT('',#225962);
#40871=VERTEX_POINT('',#225964);
#40872=VERTEX_POINT('',#225973);
#40873=VERTEX_POINT('',#225974);
#40874=VERTEX_POINT('',#225976);
#40875=VERTEX_POINT('',#225978);
#40876=VERTEX_POINT('',#226348);
#40877=VERTEX_POINT('',#226349);
#40878=VERTEX_POINT('',#226370);
#40879=VERTEX_POINT('',#226384);
#40880=VERTEX_POINT('',#226407);
#40881=VERTEX_POINT('',#226977);
#40882=VERTEX_POINT('',#226978);
#40883=VERTEX_POINT('',#227001);
#40884=VERTEX_POINT('',#227006);
#40885=VERTEX_POINT('',#227017);
#40886=VERTEX_POINT('',#227419);
#40887=VERTEX_POINT('',#227420);
#40888=VERTEX_POINT('',#227441);
#40889=VERTEX_POINT('',#227455);
#40890=VERTEX_POINT('',#227480);
#40891=VERTEX_POINT('',#228011);
#40892=VERTEX_POINT('',#228012);
#40893=VERTEX_POINT('',#228029);
#40894=VERTEX_POINT('',#228034);
#40895=VERTEX_POINT('',#228043);
#40896=VERTEX_POINT('',#228077);
#40897=VERTEX_POINT('',#228078);
#40898=VERTEX_POINT('',#228080);
#40899=VERTEX_POINT('',#228098);
#40900=VERTEX_POINT('',#228100);
#40901=VERTEX_POINT('',#228109);
#40902=VERTEX_POINT('',#228114);
#40903=VERTEX_POINT('',#228115);
#40904=VERTEX_POINT('',#228117);
#40905=VERTEX_POINT('',#228128);
#40906=VERTEX_POINT('',#228130);
#40907=VERTEX_POINT('',#228141);
#40908=VERTEX_POINT('',#228154);
#40909=VERTEX_POINT('',#228156);
#40910=VERTEX_POINT('',#228158);
#40911=VERTEX_POINT('',#228160);
#40912=VERTEX_POINT('',#228162);
#40913=VERTEX_POINT('',#228164);
#40914=VERTEX_POINT('',#228166);
#40915=VERTEX_POINT('',#228168);
#40916=VERTEX_POINT('',#228174);
#40917=VERTEX_POINT('',#228175);
#40918=VERTEX_POINT('',#228180);
#40919=VERTEX_POINT('',#228184);
#40920=VERTEX_POINT('',#228188);
#40921=VERTEX_POINT('',#228194);
#40922=VERTEX_POINT('',#228198);
#40923=VERTEX_POINT('',#228202);
#40924=VERTEX_POINT('',#228223);
#40925=VERTEX_POINT('',#228230);
#40926=VERTEX_POINT('',#228259);
#40927=VERTEX_POINT('',#228266);
#40928=VERTEX_POINT('',#228486);
#40929=VERTEX_POINT('',#228529);
#40930=VERTEX_POINT('',#228536);
#40931=VERTEX_POINT('',#228740);
#40932=VERTEX_POINT('',#228755);
#40933=VERTEX_POINT('',#228762);
#40934=VERTEX_POINT('',#228806);
#40935=VERTEX_POINT('',#228813);
#40936=VERTEX_POINT('',#229101);
#40937=VERTEX_POINT('',#229148);
#40938=VERTEX_POINT('',#229149);
#40939=VERTEX_POINT('',#229158);
#40940=VERTEX_POINT('',#229159);
#40941=VERTEX_POINT('',#229168);
#40942=VERTEX_POINT('',#229169);
#40943=VERTEX_POINT('',#229181);
#40944=VERTEX_POINT('',#229185);
#40945=VERTEX_POINT('',#229194);
#40946=VERTEX_POINT('',#229205);
#40947=VERTEX_POINT('',#229206);
#40948=VERTEX_POINT('',#229223);
#40949=VERTEX_POINT('',#229232);
#40950=VERTEX_POINT('',#229233);
#40951=VERTEX_POINT('',#230357);
#40952=VERTEX_POINT('',#230376);
#40953=VERTEX_POINT('',#230408);
#40954=VERTEX_POINT('',#230413);
#40955=VERTEX_POINT('',#230769);
#40956=VERTEX_POINT('',#230771);
#40957=VERTEX_POINT('',#230775);
#40958=VERTEX_POINT('',#230779);
#40959=VERTEX_POINT('',#230783);
#40960=VERTEX_POINT('',#230787);
#40961=VERTEX_POINT('',#230791);
#40962=VERTEX_POINT('',#230797);
#40963=VERTEX_POINT('',#230803);
#40964=VERTEX_POINT('',#230805);
#40965=VERTEX_POINT('',#230807);
#40966=VERTEX_POINT('',#230809);
#40967=VERTEX_POINT('',#230811);
#40968=VERTEX_POINT('',#230813);
#40969=VERTEX_POINT('',#230815);
#40970=VERTEX_POINT('',#230817);
#40971=VERTEX_POINT('',#231244);
#40972=VERTEX_POINT('',#231246);
#40973=VERTEX_POINT('',#231248);
#40974=VERTEX_POINT('',#231250);
#40975=VERTEX_POINT('',#231252);
#40976=VERTEX_POINT('',#231254);
#40977=VERTEX_POINT('',#231256);
#40978=VERTEX_POINT('',#231258);
#40979=VERTEX_POINT('',#232813);
#40980=VERTEX_POINT('',#232814);
#40981=VERTEX_POINT('',#232816);
#40982=VERTEX_POINT('',#232820);
#40983=VERTEX_POINT('',#232826);
#40984=VERTEX_POINT('',#232827);
#40985=VERTEX_POINT('',#232836);
#40986=VERTEX_POINT('',#232837);
#40987=VERTEX_POINT('',#232846);
#40988=VERTEX_POINT('',#232847);
#40989=VERTEX_POINT('',#232856);
#40990=VERTEX_POINT('',#232857);
#40991=VERTEX_POINT('',#232873);
#40992=VERTEX_POINT('',#232888);
#40993=VERTEX_POINT('',#232890);
#40994=VERTEX_POINT('',#232892);
#40995=VERTEX_POINT('',#232896);
#40996=VERTEX_POINT('',#232902);
#40997=VERTEX_POINT('',#232903);
#40998=VERTEX_POINT('',#232905);
#40999=VERTEX_POINT('',#232907);
#41000=VERTEX_POINT('',#232909);
#41001=VERTEX_POINT('',#232911);
#41002=VERTEX_POINT('',#232915);
#41003=VERTEX_POINT('',#232923);
#41004=VERTEX_POINT('',#232931);
#41005=VERTEX_POINT('',#232939);
#41006=VERTEX_POINT('',#232947);
#41007=VERTEX_POINT('',#232955);
#41008=VERTEX_POINT('',#232963);
#41009=VERTEX_POINT('',#232964);
#41010=VERTEX_POINT('',#232966);
#41011=VERTEX_POINT('',#232968);
#41012=VERTEX_POINT('',#232970);
#41013=VERTEX_POINT('',#232972);
#41014=VERTEX_POINT('',#232976);
#41015=VERTEX_POINT('',#232984);
#41016=VERTEX_POINT('',#232992);
#41017=VERTEX_POINT('',#233000);
#41018=VERTEX_POINT('',#233008);
#41019=VERTEX_POINT('',#233016);
#41020=VERTEX_POINT('',#233036);
#41021=VERTEX_POINT('',#233037);
#41022=VERTEX_POINT('',#233039);
#41023=VERTEX_POINT('',#233041);
#41024=VERTEX_POINT('',#233043);
#41025=VERTEX_POINT('',#233045);
#41026=VERTEX_POINT('',#233049);
#41027=VERTEX_POINT('',#233057);
#41028=VERTEX_POINT('',#233065);
#41029=VERTEX_POINT('',#233073);
#41030=VERTEX_POINT('',#233081);
#41031=VERTEX_POINT('',#233089);
#41032=VERTEX_POINT('',#233097);
#41033=VERTEX_POINT('',#233098);
#41034=VERTEX_POINT('',#233100);
#41035=VERTEX_POINT('',#233102);
#41036=VERTEX_POINT('',#233104);
#41037=VERTEX_POINT('',#233106);
#41038=VERTEX_POINT('',#233110);
#41039=VERTEX_POINT('',#233118);
#41040=VERTEX_POINT('',#233126);
#41041=VERTEX_POINT('',#233134);
#41042=VERTEX_POINT('',#233142);
#41043=VERTEX_POINT('',#233150);
#41044=VERTEX_POINT('',#233170);
#41045=VERTEX_POINT('',#233171);
#41046=VERTEX_POINT('',#233173);
#41047=VERTEX_POINT('',#233177);
#41048=VERTEX_POINT('',#233183);
#41049=VERTEX_POINT('',#233184);
#41050=VERTEX_POINT('',#233193);
#41051=VERTEX_POINT('',#233194);
#41052=VERTEX_POINT('',#233203);
#41053=VERTEX_POINT('',#233204);
#41054=VERTEX_POINT('',#233213);
#41055=VERTEX_POINT('',#233214);
#41056=VERTEX_POINT('',#233230);
#41057=VERTEX_POINT('',#233245);
#41058=VERTEX_POINT('',#233247);
#41059=VERTEX_POINT('',#233249);
#41060=VERTEX_POINT('',#233253);
#41061=VERTEX_POINT('',#233259);
#41062=VERTEX_POINT('',#233261);
#41063=VERTEX_POINT('',#233262);
#41064=VERTEX_POINT('',#233264);
#41065=VERTEX_POINT('',#233283);
#41066=VERTEX_POINT('',#233304);
#41067=VERTEX_POINT('',#233305);
#41068=VERTEX_POINT('',#233310);
#41069=VERTEX_POINT('',#233312);
#41070=VERTEX_POINT('',#233314);
#41071=VERTEX_POINT('',#233318);
#41072=VERTEX_POINT('',#233319);
#41073=VERTEX_POINT('',#233321);
#41074=VERTEX_POINT('',#233323);
#41075=VERTEX_POINT('',#233335);
#41076=VERTEX_POINT('',#233338);
#41077=VERTEX_POINT('',#233345);
#41078=VERTEX_POINT('',#233347);
#41079=VERTEX_POINT('',#233352);
#41080=VERTEX_POINT('',#233356);
#41081=VERTEX_POINT('',#233359);
#41082=VERTEX_POINT('',#233364);
#41083=VERTEX_POINT('',#233365);
#41084=VERTEX_POINT('',#233367);
#41085=VERTEX_POINT('',#233369);
#41086=VERTEX_POINT('',#233373);
#41087=VERTEX_POINT('',#233374);
#41088=VERTEX_POINT('',#233379);
#41089=VERTEX_POINT('',#233380);
#41090=VERTEX_POINT('',#233385);
#41091=VERTEX_POINT('',#233386);
#41092=VERTEX_POINT('',#233391);
#41093=VERTEX_POINT('',#233392);
#41094=VERTEX_POINT('',#233397);
#41095=VERTEX_POINT('',#233398);
#41096=VERTEX_POINT('',#233403);
#41097=VERTEX_POINT('',#233404);
#41098=VERTEX_POINT('',#233412);
#41099=VERTEX_POINT('',#233414);
#41100=VERTEX_POINT('',#233418);
#41101=VERTEX_POINT('',#233422);
#41102=VERTEX_POINT('',#233426);
#41103=VERTEX_POINT('',#233427);
#41104=VERTEX_POINT('',#233429);
#41105=VERTEX_POINT('',#233431);
#41106=VERTEX_POINT('',#233434);
#41107=VERTEX_POINT('',#233436);
#41108=VERTEX_POINT('',#233439);
#41109=VERTEX_POINT('',#233441);
#41110=VERTEX_POINT('',#233443);
#41111=VERTEX_POINT('',#233447);
#41112=VERTEX_POINT('',#233451);
#41113=VERTEX_POINT('',#233452);
#41114=VERTEX_POINT('',#233457);
#41115=VERTEX_POINT('',#233461);
#41116=VERTEX_POINT('',#233463);
#41117=VERTEX_POINT('',#233467);
#41118=VERTEX_POINT('',#233469);
#41119=VERTEX_POINT('',#233471);
#41120=VERTEX_POINT('',#233479);
#41121=VERTEX_POINT('',#233480);
#41122=VERTEX_POINT('',#233482);
#41123=VERTEX_POINT('',#233484);
#41124=VERTEX_POINT('',#233488);
#41125=VERTEX_POINT('',#233489);
#41126=VERTEX_POINT('',#233492);
#41127=VERTEX_POINT('',#233496);
#41128=VERTEX_POINT('',#233500);
#41129=VERTEX_POINT('',#233501);
#41130=VERTEX_POINT('',#233506);
#41131=VERTEX_POINT('',#233508);
#41132=VERTEX_POINT('',#233512);
#41133=VERTEX_POINT('',#233514);
#41134=VERTEX_POINT('',#233518);
#41135=VERTEX_POINT('',#233523);
#41136=VERTEX_POINT('',#233527);
#41137=VERTEX_POINT('',#233529);
#41138=VERTEX_POINT('',#233532);
#41139=VERTEX_POINT('',#233534);
#41140=VERTEX_POINT('',#233538);
#41141=VERTEX_POINT('',#233540);
#41142=VERTEX_POINT('',#233571);
#41143=VERTEX_POINT('',#233573);
#41144=VERTEX_POINT('',#233574);
#41145=VERTEX_POINT('',#233576);
#41146=VERTEX_POINT('',#233595);
#41147=VERTEX_POINT('',#233616);
#41148=VERTEX_POINT('',#233617);
#41149=VERTEX_POINT('',#233622);
#41150=VERTEX_POINT('',#233624);
#41151=VERTEX_POINT('',#233626);
#41152=VERTEX_POINT('',#233630);
#41153=VERTEX_POINT('',#233631);
#41154=VERTEX_POINT('',#233633);
#41155=VERTEX_POINT('',#233635);
#41156=VERTEX_POINT('',#233647);
#41157=VERTEX_POINT('',#233650);
#41158=VERTEX_POINT('',#233657);
#41159=VERTEX_POINT('',#233658);
#41160=VERTEX_POINT('',#233660);
#41161=VERTEX_POINT('',#233662);
#41162=VERTEX_POINT('',#233675);
#41163=VERTEX_POINT('',#233676);
#41164=VERTEX_POINT('',#233681);
#41165=VERTEX_POINT('',#233682);
#41166=VERTEX_POINT('',#233687);
#41167=VERTEX_POINT('',#233688);
#41168=VERTEX_POINT('',#233693);
#41169=VERTEX_POINT('',#233694);
#41170=VERTEX_POINT('',#233708);
#41171=VERTEX_POINT('',#233709);
#41172=VERTEX_POINT('',#233711);
#41173=VERTEX_POINT('',#233713);
#41174=VERTEX_POINT('',#233717);
#41175=VERTEX_POINT('',#233718);
#41176=VERTEX_POINT('',#233723);
#41177=VERTEX_POINT('',#233724);
#41178=VERTEX_POINT('',#233729);
#41179=VERTEX_POINT('',#233730);
#41180=VERTEX_POINT('',#233735);
#41181=VERTEX_POINT('',#233736);
#41182=VERTEX_POINT('',#233750);
#41183=VERTEX_POINT('',#233751);
#41184=VERTEX_POINT('',#233753);
#41185=VERTEX_POINT('',#233755);
#41186=VERTEX_POINT('',#233759);
#41187=VERTEX_POINT('',#233760);
#41188=VERTEX_POINT('',#233765);
#41189=VERTEX_POINT('',#233766);
#41190=VERTEX_POINT('',#233771);
#41191=VERTEX_POINT('',#233772);
#41192=VERTEX_POINT('',#233777);
#41193=VERTEX_POINT('',#233778);
#41194=VERTEX_POINT('',#233783);
#41195=VERTEX_POINT('',#233784);
#41196=VERTEX_POINT('',#233789);
#41197=VERTEX_POINT('',#233790);
#41198=VERTEX_POINT('',#233795);
#41199=VERTEX_POINT('',#233796);
#41200=VERTEX_POINT('',#233801);
#41201=VERTEX_POINT('',#233802);
#41202=VERTEX_POINT('',#233807);
#41203=VERTEX_POINT('',#233808);
#41204=VERTEX_POINT('',#233810);
#41205=VERTEX_POINT('',#233812);
#41206=VERTEX_POINT('',#233816);
#41207=VERTEX_POINT('',#233817);
#41208=VERTEX_POINT('',#233822);
#41209=VERTEX_POINT('',#233823);
#41210=VERTEX_POINT('',#233828);
#41211=VERTEX_POINT('',#233829);
#41212=VERTEX_POINT('',#233834);
#41213=VERTEX_POINT('',#233835);
#41214=VERTEX_POINT('',#233849);
#41215=VERTEX_POINT('',#233850);
#41216=VERTEX_POINT('',#233852);
#41217=VERTEX_POINT('',#233854);
#41218=VERTEX_POINT('',#233858);
#41219=VERTEX_POINT('',#233859);
#41220=VERTEX_POINT('',#233864);
#41221=VERTEX_POINT('',#233865);
#41222=VERTEX_POINT('',#233870);
#41223=VERTEX_POINT('',#233871);
#41224=VERTEX_POINT('',#233876);
#41225=VERTEX_POINT('',#233877);
#41226=VERTEX_POINT('',#233882);
#41227=VERTEX_POINT('',#233883);
#41228=VERTEX_POINT('',#233888);
#41229=VERTEX_POINT('',#233889);
#41230=VERTEX_POINT('',#233894);
#41231=VERTEX_POINT('',#233895);
#41232=VERTEX_POINT('',#233900);
#41233=VERTEX_POINT('',#233901);
#41234=VERTEX_POINT('',#233906);
#41235=VERTEX_POINT('',#233907);
#41236=VERTEX_POINT('',#233912);
#41237=VERTEX_POINT('',#233913);
#41238=VERTEX_POINT('',#233915);
#41239=VERTEX_POINT('',#233917);
#41240=VERTEX_POINT('',#233921);
#41241=VERTEX_POINT('',#233922);
#41242=VERTEX_POINT('',#233927);
#41243=VERTEX_POINT('',#233928);
#41244=VERTEX_POINT('',#233933);
#41245=VERTEX_POINT('',#233934);
#41246=VERTEX_POINT('',#233939);
#41247=VERTEX_POINT('',#233940);
#41248=VERTEX_POINT('',#233945);
#41249=VERTEX_POINT('',#233946);
#41250=VERTEX_POINT('',#233951);
#41251=VERTEX_POINT('',#233952);
#41252=VERTEX_POINT('',#233957);
#41253=VERTEX_POINT('',#233958);
#41254=VERTEX_POINT('',#233963);
#41255=VERTEX_POINT('',#233964);
#41256=VERTEX_POINT('',#233969);
#41257=VERTEX_POINT('',#233970);
#41258=VERTEX_POINT('',#233972);
#41259=VERTEX_POINT('',#233974);
#41260=VERTEX_POINT('',#233978);
#41261=VERTEX_POINT('',#233979);
#41262=VERTEX_POINT('',#233984);
#41263=VERTEX_POINT('',#233985);
#41264=VERTEX_POINT('',#233990);
#41265=VERTEX_POINT('',#233991);
#41266=VERTEX_POINT('',#233996);
#41267=VERTEX_POINT('',#233997);
#41268=VERTEX_POINT('',#234002);
#41269=VERTEX_POINT('',#234003);
#41270=VERTEX_POINT('',#234008);
#41271=VERTEX_POINT('',#234009);
#41272=VERTEX_POINT('',#234014);
#41273=VERTEX_POINT('',#234015);
#41274=VERTEX_POINT('',#234020);
#41275=VERTEX_POINT('',#234021);
#41276=VERTEX_POINT('',#234026);
#41277=VERTEX_POINT('',#234027);
#41278=VERTEX_POINT('',#234029);
#41279=VERTEX_POINT('',#234031);
#41280=VERTEX_POINT('',#234035);
#41281=VERTEX_POINT('',#234036);
#41282=VERTEX_POINT('',#234041);
#41283=VERTEX_POINT('',#234042);
#41284=VERTEX_POINT('',#234047);
#41285=VERTEX_POINT('',#234048);
#41286=VERTEX_POINT('',#234053);
#41287=VERTEX_POINT('',#234054);
#41288=VERTEX_POINT('',#234059);
#41289=VERTEX_POINT('',#234060);
#41290=VERTEX_POINT('',#234065);
#41291=VERTEX_POINT('',#234066);
#41292=VERTEX_POINT('',#234071);
#41293=VERTEX_POINT('',#234072);
#41294=VERTEX_POINT('',#234077);
#41295=VERTEX_POINT('',#234078);
#41296=VERTEX_POINT('',#234083);
#41297=VERTEX_POINT('',#234084);
#41298=VERTEX_POINT('',#234086);
#41299=VERTEX_POINT('',#234088);
#41300=VERTEX_POINT('',#234092);
#41301=VERTEX_POINT('',#234093);
#41302=VERTEX_POINT('',#234098);
#41303=VERTEX_POINT('',#234099);
#41304=VERTEX_POINT('',#234104);
#41305=VERTEX_POINT('',#234105);
#41306=VERTEX_POINT('',#234110);
#41307=VERTEX_POINT('',#234111);
#41308=VERTEX_POINT('',#234116);
#41309=VERTEX_POINT('',#234117);
#41310=VERTEX_POINT('',#234122);
#41311=VERTEX_POINT('',#234123);
#41312=VERTEX_POINT('',#234128);
#41313=VERTEX_POINT('',#234129);
#41314=VERTEX_POINT('',#234134);
#41315=VERTEX_POINT('',#234135);
#41316=VERTEX_POINT('',#234140);
#41317=VERTEX_POINT('',#234141);
#41318=VERTEX_POINT('',#234143);
#41319=VERTEX_POINT('',#234145);
#41320=VERTEX_POINT('',#234149);
#41321=VERTEX_POINT('',#234150);
#41322=VERTEX_POINT('',#234155);
#41323=VERTEX_POINT('',#234156);
#41324=VERTEX_POINT('',#234161);
#41325=VERTEX_POINT('',#234162);
#41326=VERTEX_POINT('',#234167);
#41327=VERTEX_POINT('',#234168);
#41328=VERTEX_POINT('',#234173);
#41329=VERTEX_POINT('',#234174);
#41330=VERTEX_POINT('',#234179);
#41331=VERTEX_POINT('',#234180);
#41332=VERTEX_POINT('',#234185);
#41333=VERTEX_POINT('',#234186);
#41334=VERTEX_POINT('',#234191);
#41335=VERTEX_POINT('',#234192);
#41336=VERTEX_POINT('',#234197);
#41337=VERTEX_POINT('',#234198);
#41338=VERTEX_POINT('',#234200);
#41339=VERTEX_POINT('',#234202);
#41340=VERTEX_POINT('',#234206);
#41341=VERTEX_POINT('',#234207);
#41342=VERTEX_POINT('',#234212);
#41343=VERTEX_POINT('',#234213);
#41344=VERTEX_POINT('',#234218);
#41345=VERTEX_POINT('',#234219);
#41346=VERTEX_POINT('',#234224);
#41347=VERTEX_POINT('',#234225);
#41348=VERTEX_POINT('',#234230);
#41349=VERTEX_POINT('',#234231);
#41350=VERTEX_POINT('',#234236);
#41351=VERTEX_POINT('',#234237);
#41352=VERTEX_POINT('',#234242);
#41353=VERTEX_POINT('',#234243);
#41354=VERTEX_POINT('',#234248);
#41355=VERTEX_POINT('',#234249);
#41356=VERTEX_POINT('',#234254);
#41357=VERTEX_POINT('',#234255);
#41358=VERTEX_POINT('',#234257);
#41359=VERTEX_POINT('',#234259);
#41360=VERTEX_POINT('',#234263);
#41361=VERTEX_POINT('',#234264);
#41362=VERTEX_POINT('',#234269);
#41363=VERTEX_POINT('',#234270);
#41364=VERTEX_POINT('',#234275);
#41365=VERTEX_POINT('',#234276);
#41366=VERTEX_POINT('',#234281);
#41367=VERTEX_POINT('',#234282);
#41368=VERTEX_POINT('',#234287);
#41369=VERTEX_POINT('',#234288);
#41370=VERTEX_POINT('',#234293);
#41371=VERTEX_POINT('',#234294);
#41372=VERTEX_POINT('',#234299);
#41373=VERTEX_POINT('',#234300);
#41374=VERTEX_POINT('',#234305);
#41375=VERTEX_POINT('',#234306);
#41376=VERTEX_POINT('',#234311);
#41377=VERTEX_POINT('',#234312);
#41378=VERTEX_POINT('',#234317);
#41379=VERTEX_POINT('',#234318);
#41380=VERTEX_POINT('',#234320);
#41381=VERTEX_POINT('',#234322);
#41382=VERTEX_POINT('',#234326);
#41383=VERTEX_POINT('',#234327);
#41384=VERTEX_POINT('',#234332);
#41385=VERTEX_POINT('',#234333);
#41386=VERTEX_POINT('',#234338);
#41387=VERTEX_POINT('',#234339);
#41388=VERTEX_POINT('',#234344);
#41389=VERTEX_POINT('',#234345);
#41390=VERTEX_POINT('',#234350);
#41391=VERTEX_POINT('',#234351);
#41392=VERTEX_POINT('',#234356);
#41393=VERTEX_POINT('',#234357);
#41394=VERTEX_POINT('',#234362);
#41395=VERTEX_POINT('',#234363);
#41396=VERTEX_POINT('',#234368);
#41397=VERTEX_POINT('',#234369);
#41398=VERTEX_POINT('',#234374);
#41399=VERTEX_POINT('',#234375);
#41400=VERTEX_POINT('',#234386);
#41401=VERTEX_POINT('',#234388);
#41402=VERTEX_POINT('',#234392);
#41403=VERTEX_POINT('',#234393);
#41404=VERTEX_POINT('',#234398);
#41405=VERTEX_POINT('',#234399);
#41406=VERTEX_POINT('',#234404);
#41407=VERTEX_POINT('',#234405);
#41408=VERTEX_POINT('',#234410);
#41409=VERTEX_POINT('',#234411);
#41410=VERTEX_POINT('',#234416);
#41411=VERTEX_POINT('',#234418);
#41412=VERTEX_POINT('',#234422);
#41413=VERTEX_POINT('',#234424);
#41414=VERTEX_POINT('',#234428);
#41415=VERTEX_POINT('',#234430);
#41416=VERTEX_POINT('',#234434);
#41417=VERTEX_POINT('',#234436);
#41418=VERTEX_POINT('',#234440);
#41419=VERTEX_POINT('',#234442);
#41420=VERTEX_POINT('',#234446);
#41421=VERTEX_POINT('',#234448);
#41422=VERTEX_POINT('',#234452);
#41423=VERTEX_POINT('',#234454);
#41424=VERTEX_POINT('',#234458);
#41425=VERTEX_POINT('',#234460);
#41426=VERTEX_POINT('',#234464);
#41427=VERTEX_POINT('',#234466);
#41428=VERTEX_POINT('',#234470);
#41429=VERTEX_POINT('',#234472);
#41430=VERTEX_POINT('',#234476);
#41431=VERTEX_POINT('',#234478);
#41432=VERTEX_POINT('',#234482);
#41433=VERTEX_POINT('',#234484);
#41434=VERTEX_POINT('',#234488);
#41435=VERTEX_POINT('',#234490);
#41436=VERTEX_POINT('',#234494);
#41437=VERTEX_POINT('',#234496);
#41438=VERTEX_POINT('',#234500);
#41439=VERTEX_POINT('',#234502);
#41440=VERTEX_POINT('',#234506);
#41441=VERTEX_POINT('',#234508);
#41442=VERTEX_POINT('',#234512);
#41443=VERTEX_POINT('',#234514);
#41444=VERTEX_POINT('',#234518);
#41445=VERTEX_POINT('',#234520);
#41446=VERTEX_POINT('',#234524);
#41447=VERTEX_POINT('',#234526);
#41448=VERTEX_POINT('',#234530);
#41449=VERTEX_POINT('',#234532);
#41450=VERTEX_POINT('',#234536);
#41451=VERTEX_POINT('',#234538);
#41452=VERTEX_POINT('',#234542);
#41453=VERTEX_POINT('',#234544);
#41454=VERTEX_POINT('',#234548);
#41455=VERTEX_POINT('',#234550);
#41456=VERTEX_POINT('',#234554);
#41457=VERTEX_POINT('',#234556);
#41458=VERTEX_POINT('',#234560);
#41459=VERTEX_POINT('',#234562);
#41460=VERTEX_POINT('',#234566);
#41461=VERTEX_POINT('',#234568);
#41462=VERTEX_POINT('',#234573);
#41463=VERTEX_POINT('',#234575);
#41464=VERTEX_POINT('',#234593);
#41465=VERTEX_POINT('',#234595);
#41466=VERTEX_POINT('',#234603);
#41467=VERTEX_POINT('',#234673);
#41468=VERTEX_POINT('',#234679);
#41469=VERTEX_POINT('',#234697);
#41470=VERTEX_POINT('',#234699);
#41471=VERTEX_POINT('',#234702);
#41472=VERTEX_POINT('',#234706);
#41473=VERTEX_POINT('',#234708);
#41474=VERTEX_POINT('',#234750);
#41475=VERTEX_POINT('',#234751);
#41476=VERTEX_POINT('',#234753);
#41477=VERTEX_POINT('',#234755);
#41478=VERTEX_POINT('',#234757);
#41479=VERTEX_POINT('',#234759);
#41480=VERTEX_POINT('',#234763);
#41481=VERTEX_POINT('',#234771);
#41482=VERTEX_POINT('',#234779);
#41483=VERTEX_POINT('',#234787);
#41484=VERTEX_POINT('',#234795);
#41485=VERTEX_POINT('',#234803);
#41486=VERTEX_POINT('',#234811);
#41487=VERTEX_POINT('',#234812);
#41488=VERTEX_POINT('',#234814);
#41489=VERTEX_POINT('',#234816);
#41490=VERTEX_POINT('',#234818);
#41491=VERTEX_POINT('',#234820);
#41492=VERTEX_POINT('',#234824);
#41493=VERTEX_POINT('',#234832);
#41494=VERTEX_POINT('',#234840);
#41495=VERTEX_POINT('',#234848);
#41496=VERTEX_POINT('',#234856);
#41497=VERTEX_POINT('',#234864);
#41498=VERTEX_POINT('',#234884);
#41499=VERTEX_POINT('',#234885);
#41500=VERTEX_POINT('',#234887);
#41501=VERTEX_POINT('',#234889);
#41502=VERTEX_POINT('',#234891);
#41503=VERTEX_POINT('',#234893);
#41504=VERTEX_POINT('',#234897);
#41505=VERTEX_POINT('',#234905);
#41506=VERTEX_POINT('',#234913);
#41507=VERTEX_POINT('',#234921);
#41508=VERTEX_POINT('',#234929);
#41509=VERTEX_POINT('',#234937);
#41510=VERTEX_POINT('',#234945);
#41511=VERTEX_POINT('',#234946);
#41512=VERTEX_POINT('',#234948);
#41513=VERTEX_POINT('',#234950);
#41514=VERTEX_POINT('',#234952);
#41515=VERTEX_POINT('',#234954);
#41516=VERTEX_POINT('',#234958);
#41517=VERTEX_POINT('',#234966);
#41518=VERTEX_POINT('',#234974);
#41519=VERTEX_POINT('',#234982);
#41520=VERTEX_POINT('',#234990);
#41521=VERTEX_POINT('',#234998);
#41522=VERTEX_POINT('',#235018);
#41523=VERTEX_POINT('',#235019);
#41524=VERTEX_POINT('',#235021);
#41525=VERTEX_POINT('',#235025);
#41526=VERTEX_POINT('',#235031);
#41527=VERTEX_POINT('',#235032);
#41528=VERTEX_POINT('',#235041);
#41529=VERTEX_POINT('',#235042);
#41530=VERTEX_POINT('',#235051);
#41531=VERTEX_POINT('',#235052);
#41532=VERTEX_POINT('',#235061);
#41533=VERTEX_POINT('',#235062);
#41534=VERTEX_POINT('',#235078);
#41535=VERTEX_POINT('',#235093);
#41536=VERTEX_POINT('',#235095);
#41537=VERTEX_POINT('',#235097);
#41538=VERTEX_POINT('',#235101);
#41539=VERTEX_POINT('',#235107);
#41540=VERTEX_POINT('',#235108);
#41541=VERTEX_POINT('',#235110);
#41542=VERTEX_POINT('',#235114);
#41543=VERTEX_POINT('',#235115);
#41544=VERTEX_POINT('',#235117);
#41545=VERTEX_POINT('',#235121);
#41546=VERTEX_POINT('',#235123);
#41547=VERTEX_POINT('',#235127);
#41548=VERTEX_POINT('',#235129);
#41549=VERTEX_POINT('',#235133);
#41550=VERTEX_POINT('',#235137);
#41551=VERTEX_POINT('',#235138);
#41552=VERTEX_POINT('',#235140);
#41553=VERTEX_POINT('',#235145);
#41554=VERTEX_POINT('',#235149);
#41555=VERTEX_POINT('',#235153);
#41556=VERTEX_POINT('',#235162);
#41557=VERTEX_POINT('',#235163);
#41558=VERTEX_POINT('',#235165);
#41559=VERTEX_POINT('',#235174);
#41560=VERTEX_POINT('',#235178);
#41561=VERTEX_POINT('',#235179);
#41562=VERTEX_POINT('',#235187);
#41563=VERTEX_POINT('',#235188);
#41564=VERTEX_POINT('',#235190);
#41565=VERTEX_POINT('',#235199);
#41566=VERTEX_POINT('',#235204);
#41567=VERTEX_POINT('',#235208);
#41568=VERTEX_POINT('',#235209);
#41569=VERTEX_POINT('',#235211);
#41570=VERTEX_POINT('',#235213);
#41571=VERTEX_POINT('',#235217);
#41572=VERTEX_POINT('',#235218);
#41573=VERTEX_POINT('',#235220);
#41574=VERTEX_POINT('',#235222);
#41575=VERTEX_POINT('',#235242);
#41576=VERTEX_POINT('',#235244);
#41577=VERTEX_POINT('',#235246);
#41578=VERTEX_POINT('',#235248);
#41579=VERTEX_POINT('',#235252);
#41580=VERTEX_POINT('',#235253);
#41581=VERTEX_POINT('',#235255);
#41582=VERTEX_POINT('',#235259);
#41583=VERTEX_POINT('',#235260);
#41584=VERTEX_POINT('',#235262);
#41585=VERTEX_POINT('',#235266);
#41586=VERTEX_POINT('',#235267);
#41587=VERTEX_POINT('',#235272);
#41588=VERTEX_POINT('',#235273);
#41589=VERTEX_POINT('',#235278);
#41590=VERTEX_POINT('',#235282);
#41591=VERTEX_POINT('',#235283);
#41592=VERTEX_POINT('',#235285);
#41593=VERTEX_POINT('',#235290);
#41594=VERTEX_POINT('',#235294);
#41595=VERTEX_POINT('',#235298);
#41596=VERTEX_POINT('',#235307);
#41597=VERTEX_POINT('',#235308);
#41598=VERTEX_POINT('',#235310);
#41599=VERTEX_POINT('',#235319);
#41600=VERTEX_POINT('',#235323);
#41601=VERTEX_POINT('',#235328);
#41602=VERTEX_POINT('',#235332);
#41603=VERTEX_POINT('',#235333);
#41604=VERTEX_POINT('',#235335);
#41605=VERTEX_POINT('',#235344);
#41606=VERTEX_POINT('',#235345);
#41607=VERTEX_POINT('',#235353);
#41608=VERTEX_POINT('',#235354);
#41609=VERTEX_POINT('',#235356);
#41610=VERTEX_POINT('',#235358);
#41611=VERTEX_POINT('',#235362);
#41612=VERTEX_POINT('',#235363);
#41613=VERTEX_POINT('',#235365);
#41614=VERTEX_POINT('',#235367);
#41615=VERTEX_POINT('',#235459);
#41616=VERTEX_POINT('',#235461);
#41617=VERTEX_POINT('',#235463);
#41618=VERTEX_POINT('',#235465);
#41619=VERTEX_POINT('',#235469);
#41620=VERTEX_POINT('',#235502);
#41621=VERTEX_POINT('',#235515);
#41622=VERTEX_POINT('',#235519);
#41623=VERTEX_POINT('',#235520);
#41624=VERTEX_POINT('',#235528);
#41625=VERTEX_POINT('',#235532);
#41626=VERTEX_POINT('',#235533);
#41627=VERTEX_POINT('',#235541);
#41628=VERTEX_POINT('',#235545);
#41629=VERTEX_POINT('',#235549);
#41630=VERTEX_POINT('',#235552);
#41631=VERTEX_POINT('',#235556);
#41632=VERTEX_POINT('',#235589);
#41633=VERTEX_POINT('',#235604);
#41634=VERTEX_POINT('',#235608);
#41635=VERTEX_POINT('',#235609);
#41636=VERTEX_POINT('',#235617);
#41637=VERTEX_POINT('',#235621);
#41638=VERTEX_POINT('',#235622);
#41639=VERTEX_POINT('',#235639);
#41640=VERTEX_POINT('',#235640);
#41641=VERTEX_POINT('',#235642);
#41642=VERTEX_POINT('',#235663);
#41643=VERTEX_POINT('',#235694);
#41644=VERTEX_POINT('',#235695);
#41645=VERTEX_POINT('',#235770);
#41646=VERTEX_POINT('',#235771);
#41647=VERTEX_POINT('',#235848);
#41648=VERTEX_POINT('',#235849);
#41649=VERTEX_POINT('',#235926);
#41650=VERTEX_POINT('',#235927);
#41651=VERTEX_POINT('',#236002);
#41652=VERTEX_POINT('',#236003);
#41653=VERTEX_POINT('',#236078);
#41654=VERTEX_POINT('',#236079);
#41655=VERTEX_POINT('',#236154);
#41656=VERTEX_POINT('',#236155);
#41657=VERTEX_POINT('',#236230);
#41658=VERTEX_POINT('',#236231);
#41659=VERTEX_POINT('',#236308);
#41660=VERTEX_POINT('',#236309);
#41661=VERTEX_POINT('',#236386);
#41662=VERTEX_POINT('',#236387);
#41663=VERTEX_POINT('',#236462);
#41664=VERTEX_POINT('',#236463);
#41665=VERTEX_POINT('',#236538);
#41666=VERTEX_POINT('',#236539);
#41667=VERTEX_POINT('',#236614);
#41668=VERTEX_POINT('',#236615);
#41669=VERTEX_POINT('',#236690);
#41670=VERTEX_POINT('',#236691);
#41671=VERTEX_POINT('',#236766);
#41672=VERTEX_POINT('',#236767);
#41673=VERTEX_POINT('',#236844);
#41674=VERTEX_POINT('',#236845);
#41675=VERTEX_POINT('',#236922);
#41676=VERTEX_POINT('',#236923);
#41677=VERTEX_POINT('',#236998);
#41678=VERTEX_POINT('',#236999);
#41679=VERTEX_POINT('',#237001);
#41680=VERTEX_POINT('',#237010);
#41681=VERTEX_POINT('',#237026);
#41682=VERTEX_POINT('',#237027);
#41683=VERTEX_POINT('',#237029);
#41684=VERTEX_POINT('',#237042);
#41685=VERTEX_POINT('',#237063);
#41686=VERTEX_POINT('',#237064);
#41687=VERTEX_POINT('',#237139);
#41688=VERTEX_POINT('',#237140);
#41689=VERTEX_POINT('',#237217);
#41690=VERTEX_POINT('',#237218);
#41691=VERTEX_POINT('',#237293);
#41692=VERTEX_POINT('',#237294);
#41693=VERTEX_POINT('',#237369);
#41694=VERTEX_POINT('',#237370);
#41695=VERTEX_POINT('',#237445);
#41696=VERTEX_POINT('',#237446);
#41697=VERTEX_POINT('',#237521);
#41698=VERTEX_POINT('',#237522);
#41699=VERTEX_POINT('',#237599);
#41700=VERTEX_POINT('',#237600);
#41701=VERTEX_POINT('',#237675);
#41702=VERTEX_POINT('',#237676);
#41703=VERTEX_POINT('',#237753);
#41704=VERTEX_POINT('',#237754);
#41705=VERTEX_POINT('',#237829);
#41706=VERTEX_POINT('',#237830);
#41707=VERTEX_POINT('',#237905);
#41708=VERTEX_POINT('',#237906);
#41709=VERTEX_POINT('',#237981);
#41710=VERTEX_POINT('',#237982);
#41711=VERTEX_POINT('',#238057);
#41712=VERTEX_POINT('',#238058);
#41713=VERTEX_POINT('',#238135);
#41714=VERTEX_POINT('',#238136);
#41715=VERTEX_POINT('',#238211);
#41716=VERTEX_POINT('',#238212);
#41717=VERTEX_POINT('',#238289);
#41718=VERTEX_POINT('',#238290);
#41719=VERTEX_POINT('',#238365);
#41720=VERTEX_POINT('',#238366);
#41721=VERTEX_POINT('',#238368);
#41722=VERTEX_POINT('',#238385);
#41723=VERTEX_POINT('',#238411);
#41724=VERTEX_POINT('',#238412);
#41725=VERTEX_POINT('',#238414);
#41726=VERTEX_POINT('',#238418);
#41727=VERTEX_POINT('',#238429);
#41728=VERTEX_POINT('',#238430);
#41729=VERTEX_POINT('',#238432);
#41730=VERTEX_POINT('',#238440);
#41731=VERTEX_POINT('',#238474);
#41732=VERTEX_POINT('',#238475);
#41733=VERTEX_POINT('',#238504);
#41734=VERTEX_POINT('',#238505);
#41735=VERTEX_POINT('',#238534);
#41736=VERTEX_POINT('',#238535);
#41737=VERTEX_POINT('',#238564);
#41738=VERTEX_POINT('',#238565);
#41739=VERTEX_POINT('',#238594);
#41740=VERTEX_POINT('',#238595);
#41741=VERTEX_POINT('',#238624);
#41742=VERTEX_POINT('',#238625);
#41743=VERTEX_POINT('',#238654);
#41744=VERTEX_POINT('',#238655);
#41745=VERTEX_POINT('',#238684);
#41746=VERTEX_POINT('',#238685);
#41747=VERTEX_POINT('',#238714);
#41748=VERTEX_POINT('',#238715);
#41749=VERTEX_POINT('',#238744);
#41750=VERTEX_POINT('',#238745);
#41751=VERTEX_POINT('',#238774);
#41752=VERTEX_POINT('',#238775);
#41753=VERTEX_POINT('',#238804);
#41754=VERTEX_POINT('',#238805);
#41755=VERTEX_POINT('',#238834);
#41756=VERTEX_POINT('',#238835);
#41757=VERTEX_POINT('',#238864);
#41758=VERTEX_POINT('',#238865);
#41759=VERTEX_POINT('',#238894);
#41760=VERTEX_POINT('',#238895);
#41761=VERTEX_POINT('',#238924);
#41762=VERTEX_POINT('',#238925);
#41763=VERTEX_POINT('',#238954);
#41764=VERTEX_POINT('',#238955);
#41765=VERTEX_POINT('',#238957);
#41766=VERTEX_POINT('',#238965);
#41767=VERTEX_POINT('',#238966);
#41768=VERTEX_POINT('',#238968);
#41769=VERTEX_POINT('',#238997);
#41770=VERTEX_POINT('',#239036);
#41771=VERTEX_POINT('',#239037);
#41772=VERTEX_POINT('',#239112);
#41773=VERTEX_POINT('',#239113);
#41774=VERTEX_POINT('',#239188);
#41775=VERTEX_POINT('',#239189);
#41776=VERTEX_POINT('',#239266);
#41777=VERTEX_POINT('',#239267);
#41778=VERTEX_POINT('',#239342);
#41779=VERTEX_POINT('',#239343);
#41780=VERTEX_POINT('',#239418);
#41781=VERTEX_POINT('',#239419);
#41782=VERTEX_POINT('',#239496);
#41783=VERTEX_POINT('',#239497);
#41784=VERTEX_POINT('',#239572);
#41785=VERTEX_POINT('',#239573);
#41786=VERTEX_POINT('',#239648);
#41787=VERTEX_POINT('',#239649);
#41788=VERTEX_POINT('',#239724);
#41789=VERTEX_POINT('',#239725);
#41790=VERTEX_POINT('',#239802);
#41791=VERTEX_POINT('',#239803);
#41792=VERTEX_POINT('',#239878);
#41793=VERTEX_POINT('',#239879);
#41794=VERTEX_POINT('',#239954);
#41795=VERTEX_POINT('',#239955);
#41796=VERTEX_POINT('',#240032);
#41797=VERTEX_POINT('',#240033);
#41798=VERTEX_POINT('',#240108);
#41799=VERTEX_POINT('',#240109);
#41800=VERTEX_POINT('',#240184);
#41801=VERTEX_POINT('',#240185);
#41802=VERTEX_POINT('',#240260);
#41803=VERTEX_POINT('',#240261);
#41804=VERTEX_POINT('',#240263);
#41805=VERTEX_POINT('',#240270);
#41806=VERTEX_POINT('',#240281);
#41807=VERTEX_POINT('',#240308);
#41808=VERTEX_POINT('',#240345);
#41809=VERTEX_POINT('',#240346);
#41810=VERTEX_POINT('',#240348);
#41811=VERTEX_POINT('',#240352);
#41812=VERTEX_POINT('',#240373);
#41813=VERTEX_POINT('',#240374);
#41814=VERTEX_POINT('',#240376);
#41815=VERTEX_POINT('',#240384);
#41816=VERTEX_POINT('',#240418);
#41817=VERTEX_POINT('',#240419);
#41818=VERTEX_POINT('',#240448);
#41819=VERTEX_POINT('',#240449);
#41820=VERTEX_POINT('',#240478);
#41821=VERTEX_POINT('',#240479);
#41822=VERTEX_POINT('',#240508);
#41823=VERTEX_POINT('',#240509);
#41824=VERTEX_POINT('',#240538);
#41825=VERTEX_POINT('',#240539);
#41826=VERTEX_POINT('',#240568);
#41827=VERTEX_POINT('',#240569);
#41828=VERTEX_POINT('',#240598);
#41829=VERTEX_POINT('',#240599);
#41830=VERTEX_POINT('',#240628);
#41831=VERTEX_POINT('',#240629);
#41832=VERTEX_POINT('',#240658);
#41833=VERTEX_POINT('',#240659);
#41834=VERTEX_POINT('',#240688);
#41835=VERTEX_POINT('',#240689);
#41836=VERTEX_POINT('',#240718);
#41837=VERTEX_POINT('',#240719);
#41838=VERTEX_POINT('',#240748);
#41839=VERTEX_POINT('',#240749);
#41840=VERTEX_POINT('',#240778);
#41841=VERTEX_POINT('',#240779);
#41842=VERTEX_POINT('',#240808);
#41843=VERTEX_POINT('',#240809);
#41844=VERTEX_POINT('',#240838);
#41845=VERTEX_POINT('',#240839);
#41846=VERTEX_POINT('',#240868);
#41847=VERTEX_POINT('',#240869);
#41848=VERTEX_POINT('',#240898);
#41849=VERTEX_POINT('',#240899);
#41850=VERTEX_POINT('',#240901);
#41851=VERTEX_POINT('',#240909);
#41852=VERTEX_POINT('',#240910);
#41853=VERTEX_POINT('',#240912);
#41854=VERTEX_POINT('',#240925);
#41855=VERTEX_POINT('',#240926);
#41856=VERTEX_POINT('',#241003);
#41857=VERTEX_POINT('',#241004);
#41858=VERTEX_POINT('',#241079);
#41859=VERTEX_POINT('',#241080);
#41860=VERTEX_POINT('',#241155);
#41861=VERTEX_POINT('',#241156);
#41862=VERTEX_POINT('',#241231);
#41863=VERTEX_POINT('',#241232);
#41864=VERTEX_POINT('',#241307);
#41865=VERTEX_POINT('',#241308);
#41866=VERTEX_POINT('',#241383);
#41867=VERTEX_POINT('',#241384);
#41868=VERTEX_POINT('',#241461);
#41869=VERTEX_POINT('',#241462);
#41870=VERTEX_POINT('',#241539);
#41871=VERTEX_POINT('',#241540);
#41872=VERTEX_POINT('',#241615);
#41873=VERTEX_POINT('',#241616);
#41874=VERTEX_POINT('',#241691);
#41875=VERTEX_POINT('',#241692);
#41876=VERTEX_POINT('',#241767);
#41877=VERTEX_POINT('',#241768);
#41878=VERTEX_POINT('',#241843);
#41879=VERTEX_POINT('',#241844);
#41880=VERTEX_POINT('',#241919);
#41881=VERTEX_POINT('',#241920);
#41882=VERTEX_POINT('',#241999);
#41883=VERTEX_POINT('',#242000);
#41884=VERTEX_POINT('',#242075);
#41885=VERTEX_POINT('',#242076);
#41886=VERTEX_POINT('',#242151);
#41887=VERTEX_POINT('',#242152);
#41888=VERTEX_POINT('',#242227);
#41889=VERTEX_POINT('',#242228);
#41890=VERTEX_POINT('',#242230);
#41891=VERTEX_POINT('',#242257);
#41892=VERTEX_POINT('',#242291);
#41893=VERTEX_POINT('',#242292);
#41894=VERTEX_POINT('',#242294);
#41895=VERTEX_POINT('',#242298);
#41896=VERTEX_POINT('',#242309);
#41897=VERTEX_POINT('',#242310);
#41898=VERTEX_POINT('',#242312);
#41899=VERTEX_POINT('',#242320);
#41900=VERTEX_POINT('',#242354);
#41901=VERTEX_POINT('',#242355);
#41902=VERTEX_POINT('',#242384);
#41903=VERTEX_POINT('',#242385);
#41904=VERTEX_POINT('',#242414);
#41905=VERTEX_POINT('',#242415);
#41906=VERTEX_POINT('',#242444);
#41907=VERTEX_POINT('',#242445);
#41908=VERTEX_POINT('',#242474);
#41909=VERTEX_POINT('',#242475);
#41910=VERTEX_POINT('',#242504);
#41911=VERTEX_POINT('',#242505);
#41912=VERTEX_POINT('',#242534);
#41913=VERTEX_POINT('',#242535);
#41914=VERTEX_POINT('',#242564);
#41915=VERTEX_POINT('',#242565);
#41916=VERTEX_POINT('',#242594);
#41917=VERTEX_POINT('',#242595);
#41918=VERTEX_POINT('',#242624);
#41919=VERTEX_POINT('',#242625);
#41920=VERTEX_POINT('',#242654);
#41921=VERTEX_POINT('',#242655);
#41922=VERTEX_POINT('',#242684);
#41923=VERTEX_POINT('',#242685);
#41924=VERTEX_POINT('',#242714);
#41925=VERTEX_POINT('',#242715);
#41926=VERTEX_POINT('',#242744);
#41927=VERTEX_POINT('',#242745);
#41928=VERTEX_POINT('',#242774);
#41929=VERTEX_POINT('',#242775);
#41930=VERTEX_POINT('',#242804);
#41931=VERTEX_POINT('',#242805);
#41932=VERTEX_POINT('',#242834);
#41933=VERTEX_POINT('',#242835);
#41934=VERTEX_POINT('',#242837);
#41935=VERTEX_POINT('',#242845);
#41936=VERTEX_POINT('',#242846);
#41937=VERTEX_POINT('',#242848);
#41938=VERTEX_POINT('',#242852);
#41939=VERTEX_POINT('',#242863);
#41940=VERTEX_POINT('',#242864);
#41941=VERTEX_POINT('',#242866);
#41942=VERTEX_POINT('',#242874);
#41943=VERTEX_POINT('',#242908);
#41944=VERTEX_POINT('',#242909);
#41945=VERTEX_POINT('',#242938);
#41946=VERTEX_POINT('',#242939);
#41947=VERTEX_POINT('',#242968);
#41948=VERTEX_POINT('',#242969);
#41949=VERTEX_POINT('',#242998);
#41950=VERTEX_POINT('',#242999);
#41951=VERTEX_POINT('',#243028);
#41952=VERTEX_POINT('',#243029);
#41953=VERTEX_POINT('',#243058);
#41954=VERTEX_POINT('',#243059);
#41955=VERTEX_POINT('',#243088);
#41956=VERTEX_POINT('',#243089);
#41957=VERTEX_POINT('',#243118);
#41958=VERTEX_POINT('',#243119);
#41959=VERTEX_POINT('',#243148);
#41960=VERTEX_POINT('',#243149);
#41961=VERTEX_POINT('',#243178);
#41962=VERTEX_POINT('',#243179);
#41963=VERTEX_POINT('',#243208);
#41964=VERTEX_POINT('',#243209);
#41965=VERTEX_POINT('',#243238);
#41966=VERTEX_POINT('',#243239);
#41967=VERTEX_POINT('',#243268);
#41968=VERTEX_POINT('',#243269);
#41969=VERTEX_POINT('',#243298);
#41970=VERTEX_POINT('',#243299);
#41971=VERTEX_POINT('',#243328);
#41972=VERTEX_POINT('',#243329);
#41973=VERTEX_POINT('',#243358);
#41974=VERTEX_POINT('',#243359);
#41975=VERTEX_POINT('',#243388);
#41976=VERTEX_POINT('',#243389);
#41977=VERTEX_POINT('',#243391);
#41978=VERTEX_POINT('',#243399);
#41979=VERTEX_POINT('',#243400);
#41980=VERTEX_POINT('',#243402);
#41981=VERTEX_POINT('',#243404);
#41982=VERTEX_POINT('',#243406);
#41983=VERTEX_POINT('',#243408);
#41984=VERTEX_POINT('',#243410);
#41985=VERTEX_POINT('',#243412);
#41986=VERTEX_POINT('',#243416);
#41987=VERTEX_POINT('',#243417);
#41988=VERTEX_POINT('',#243419);
#41989=VERTEX_POINT('',#243422);
#41990=VERTEX_POINT('',#243426);
#41991=VERTEX_POINT('',#243427);
#41992=VERTEX_POINT('',#243469);
#41993=VERTEX_POINT('',#243471);
#41994=VERTEX_POINT('',#243473);
#41995=VERTEX_POINT('',#243519);
#41996=VERTEX_POINT('',#243520);
#41997=VERTEX_POINT('',#243522);
#41998=VERTEX_POINT('',#243524);
#41999=VERTEX_POINT('',#243528);
#42000=VERTEX_POINT('',#243530);
#42001=VERTEX_POINT('',#243534);
#42002=VERTEX_POINT('',#243536);
#42003=VERTEX_POINT('',#243543);
#42004=VERTEX_POINT('',#243545);
#42005=VERTEX_POINT('',#243547);
#42006=VERTEX_POINT('',#243549);
#42007=VERTEX_POINT('',#243551);
#42008=VERTEX_POINT('',#243554);
#42009=VERTEX_POINT('',#243556);
#42010=VERTEX_POINT('',#243558);
#42011=VERTEX_POINT('',#243559);
#42012=VERTEX_POINT('',#243574);
#42013=VERTEX_POINT('',#243576);
#42014=VERTEX_POINT('',#243583);
#42015=VERTEX_POINT('',#243590);
#42016=VERTEX_POINT('',#243724);
#42017=VERTEX_POINT('',#243726);
#42018=VERTEX_POINT('',#243728);
#42019=VERTEX_POINT('',#243730);
#42020=VERTEX_POINT('',#243801);
#42021=VERTEX_POINT('',#243808);
#42022=VERTEX_POINT('',#243815);
#42023=VERTEX_POINT('',#243817);
#42024=VERTEX_POINT('',#243834);
#42025=VERTEX_POINT('',#243836);
#42026=VERTEX_POINT('',#243839);
#42027=VERTEX_POINT('',#243846);
#42028=VERTEX_POINT('',#243848);
#42029=VERTEX_POINT('',#243851);
#42030=VERTEX_POINT('',#243858);
#42031=VERTEX_POINT('',#243860);
#42032=VERTEX_POINT('',#243863);
#42033=VERTEX_POINT('',#243867);
#42034=VERTEX_POINT('',#243907);
#42035=VERTEX_POINT('',#243909);
#42036=VERTEX_POINT('',#243912);
#42037=VERTEX_POINT('',#243916);
#42038=VERTEX_POINT('',#243922);
#42039=VERTEX_POINT('',#243927);
#42040=VERTEX_POINT('',#243929);
#42041=VERTEX_POINT('',#243931);
#42042=VERTEX_POINT('',#243935);
#42043=VERTEX_POINT('',#243936);
#42044=VERTEX_POINT('',#243939);
#42045=VERTEX_POINT('',#243941);
#42046=VERTEX_POINT('',#243945);
#42047=VERTEX_POINT('',#243946);
#42048=VERTEX_POINT('',#243948);
#42049=VERTEX_POINT('',#243952);
#42050=VERTEX_POINT('',#243958);
#42051=VERTEX_POINT('',#243959);
#42052=VERTEX_POINT('',#243968);
#42053=VERTEX_POINT('',#243969);
#42054=VERTEX_POINT('',#243978);
#42055=VERTEX_POINT('',#243979);
#42056=VERTEX_POINT('',#243988);
#42057=VERTEX_POINT('',#243989);
#42058=VERTEX_POINT('',#244005);
#42059=VERTEX_POINT('',#244374);
#42060=VERTEX_POINT('',#244375);
#42061=VERTEX_POINT('',#245374);
#42062=VERTEX_POINT('',#245375);
#42063=VERTEX_POINT('',#246033);
#42064=VERTEX_POINT('',#246034);
#42065=VERTEX_POINT('',#246036);
#42066=VERTEX_POINT('',#246081);
#42067=VERTEX_POINT('',#246082);
#42068=VERTEX_POINT('',#246175);
#42069=VERTEX_POINT('',#246202);
#42070=VERTEX_POINT('',#246248);
#42071=VERTEX_POINT('',#246249);
#42072=VERTEX_POINT('',#246265);
#42073=VERTEX_POINT('',#246266);
#42074=VERTEX_POINT('',#246327);
#42075=VERTEX_POINT('',#246328);
#42076=VERTEX_POINT('',#246461);
#42077=VERTEX_POINT('',#246462);
#42078=VERTEX_POINT('',#246500);
#42079=VERTEX_POINT('',#246583);
#42080=VERTEX_POINT('',#246619);
#42081=VERTEX_POINT('',#246701);
#42082=VERTEX_POINT('',#246722);
#42083=VERTEX_POINT('',#246864);
#42084=VERTEX_POINT('',#246869);
#42085=VERTEX_POINT('',#246876);
#42086=VERTEX_POINT('',#246926);
#42087=VERTEX_POINT('',#246927);
#42088=VERTEX_POINT('',#246929);
#42089=VERTEX_POINT('',#247111);
#42090=VERTEX_POINT('',#247112);
#42091=VERTEX_POINT('',#247115);
#42092=VERTEX_POINT('',#247291);
#42093=VERTEX_POINT('',#247368);
#42094=VERTEX_POINT('',#247475);
#42095=VERTEX_POINT('',#247477);
#42096=VERTEX_POINT('',#247486);
#42097=VERTEX_POINT('',#247487);
#42098=VERTEX_POINT('',#247643);
#42099=VERTEX_POINT('',#247645);
#42100=VERTEX_POINT('',#247660);
#42101=VERTEX_POINT('',#247661);
#42102=VERTEX_POINT('',#247666);
#42103=VERTEX_POINT('',#247670);
#42104=VERTEX_POINT('',#247671);
#42105=VERTEX_POINT('',#247711);
#42106=VERTEX_POINT('',#247852);
#42107=VERTEX_POINT('',#247854);
#42108=VERTEX_POINT('',#247858);
#42109=VERTEX_POINT('',#247862);
#42110=VERTEX_POINT('',#247863);
#42111=VERTEX_POINT('',#247903);
#42112=VERTEX_POINT('',#247973);
#42113=VERTEX_POINT('',#247974);
#42114=VERTEX_POINT('',#247976);
#42115=VERTEX_POINT('',#247978);
#42116=VERTEX_POINT('',#247997);
#42117=VERTEX_POINT('',#247998);
#42118=VERTEX_POINT('',#248000);
#42119=VERTEX_POINT('',#248002);
#42120=VERTEX_POINT('',#248021);
#42121=VERTEX_POINT('',#248022);
#42122=VERTEX_POINT('',#248024);
#42123=VERTEX_POINT('',#248026);
#42124=VERTEX_POINT('',#248056);
#42125=VERTEX_POINT('',#248058);
#42126=VERTEX_POINT('',#248074);
#42127=VERTEX_POINT('',#248075);
#42128=VERTEX_POINT('',#248077);
#42129=VERTEX_POINT('',#248079);
#42130=VERTEX_POINT('',#248088);
#42131=VERTEX_POINT('',#248089);
#42132=VERTEX_POINT('',#248091);
#42133=VERTEX_POINT('',#248093);
#42134=VERTEX_POINT('',#248125);
#42135=VERTEX_POINT('',#248127);
#42136=VERTEX_POINT('',#248166);
#42137=VERTEX_POINT('',#248168);
#42138=VERTEX_POINT('',#248204);
#42139=VERTEX_POINT('',#248206);
#42140=VERTEX_POINT('',#248222);
#42141=VERTEX_POINT('',#248223);
#42142=VERTEX_POINT('',#248225);
#42143=VERTEX_POINT('',#248227);
#42144=VERTEX_POINT('',#248236);
#42145=VERTEX_POINT('',#248237);
#42146=VERTEX_POINT('',#248239);
#42147=VERTEX_POINT('',#248241);
#42148=VERTEX_POINT('',#248254);
#42149=VERTEX_POINT('',#248275);
#42150=VERTEX_POINT('',#248277);
#42151=VERTEX_POINT('',#248316);
#42152=VERTEX_POINT('',#248318);
#42153=VERTEX_POINT('',#248354);
#42154=VERTEX_POINT('',#248356);
#42155=VERTEX_POINT('',#248496);
#42156=VERTEX_POINT('',#248497);
#42157=VERTEX_POINT('',#248499);
#42158=VERTEX_POINT('',#248519);
#42159=VERTEX_POINT('',#248523);
#42160=VERTEX_POINT('',#248524);
#42161=VERTEX_POINT('',#248526);
#42162=VERTEX_POINT('',#248546);
#42163=VERTEX_POINT('',#248550);
#42164=VERTEX_POINT('',#248551);
#42165=VERTEX_POINT('',#248553);
#42166=VERTEX_POINT('',#248573);
#42167=VERTEX_POINT('',#248577);
#42168=VERTEX_POINT('',#248578);
#42169=VERTEX_POINT('',#248580);
#42170=VERTEX_POINT('',#248600);
#42171=VERTEX_POINT('',#248618);
#42172=VERTEX_POINT('',#248620);
#42173=VERTEX_POINT('',#248636);
#42174=VERTEX_POINT('',#248637);
#42175=VERTEX_POINT('',#248639);
#42176=VERTEX_POINT('',#248662);
#42177=VERTEX_POINT('',#248666);
#42178=VERTEX_POINT('',#248667);
#42179=VERTEX_POINT('',#248669);
#42180=VERTEX_POINT('',#248692);
#42181=VERTEX_POINT('',#248719);
#42182=VERTEX_POINT('',#248721);
#42183=VERTEX_POINT('',#248760);
#42184=VERTEX_POINT('',#248762);
#42185=VERTEX_POINT('',#248798);
#42186=VERTEX_POINT('',#248800);
#42187=VERTEX_POINT('',#248830);
#42188=VERTEX_POINT('',#248832);
#42189=VERTEX_POINT('',#248848);
#42190=VERTEX_POINT('',#248849);
#42191=VERTEX_POINT('',#248851);
#42192=VERTEX_POINT('',#248874);
#42193=VERTEX_POINT('',#248878);
#42194=VERTEX_POINT('',#248879);
#42195=VERTEX_POINT('',#248881);
#42196=VERTEX_POINT('',#248904);
#42197=VERTEX_POINT('',#248931);
#42198=VERTEX_POINT('',#248933);
#42199=VERTEX_POINT('',#248972);
#42200=VERTEX_POINT('',#248974);
#42201=VERTEX_POINT('',#249010);
#42202=VERTEX_POINT('',#249012);
#42203=VERTEX_POINT('',#249164);
#42204=VERTEX_POINT('',#249546);
#42205=VERTEX_POINT('',#249547);
#42206=VERTEX_POINT('',#250188);
#42207=VERTEX_POINT('',#250220);
#42208=VERTEX_POINT('',#251062);
#42209=VERTEX_POINT('',#251063);
#42210=VERTEX_POINT('',#251065);
#42211=VERTEX_POINT('',#251464);
#42212=VERTEX_POINT('',#251465);
#42213=VERTEX_POINT('',#252013);
#42214=VERTEX_POINT('',#252015);
#42215=VERTEX_POINT('',#253783);
#42216=VERTEX_POINT('',#254405);
#42217=VERTEX_POINT('',#254406);
#42218=VERTEX_POINT('',#255306);
#42219=VERTEX_POINT('',#255716);
#42220=VERTEX_POINT('',#255717);
#42221=VERTEX_POINT('',#255958);
#42222=VERTEX_POINT('',#255960);
#42223=VERTEX_POINT('',#256077);
#42224=VERTEX_POINT('',#256079);
#42225=VERTEX_POINT('',#257914);
#42226=VERTEX_POINT('',#258538);
#42227=VERTEX_POINT('',#258559);
#42228=VERTEX_POINT('',#258689);
#42229=VERTEX_POINT('',#258720);
#42230=VERTEX_POINT('',#259886);
#42231=VERTEX_POINT('',#259887);
#42232=VERTEX_POINT('',#260124);
#42233=VERTEX_POINT('',#260126);
#42234=VERTEX_POINT('',#260241);
#42235=VERTEX_POINT('',#262002);
#42236=VERTEX_POINT('',#262606);
#42237=VERTEX_POINT('',#262615);
#42238=VERTEX_POINT('',#263457);
#42239=VERTEX_POINT('',#263458);
#42240=VERTEX_POINT('',#263851);
#42241=VERTEX_POINT('',#263852);
#42242=VERTEX_POINT('',#264374);
#42243=VERTEX_POINT('',#264376);
#42244=VERTEX_POINT('',#271076);
#43752=EDGE_CURVE('',#35201,#35201,#29239,.T.);
#43753=EDGE_CURVE('',#35201,#35202,#20561,.T.);
#43754=EDGE_CURVE('',#35202,#35202,#29240,.T.);
#43755=EDGE_CURVE('',#35203,#35203,#29241,.T.);
#43756=EDGE_CURVE('',#35203,#35201,#20562,.T.);
#43757=EDGE_CURVE('',#35204,#35204,#29242,.T.);
#43758=EDGE_CURVE('',#35205,#35205,#29243,.T.);
#43759=EDGE_CURVE('',#35205,#35204,#20563,.T.);
#43760=EDGE_CURVE('',#35206,#35206,#29244,.T.);
#43761=EDGE_CURVE('',#35206,#35207,#20564,.T.);
#43762=EDGE_CURVE('',#35207,#35207,#29245,.T.);
#43763=EDGE_CURVE('',#35208,#35208,#29246,.T.);
#43764=EDGE_CURVE('',#35208,#35206,#20565,.T.);
#43765=EDGE_CURVE('',#35209,#35209,#29247,.T.);
#43766=EDGE_CURVE('',#35210,#35210,#29248,.T.);
#43767=EDGE_CURVE('',#35210,#35209,#20566,.T.);
#43768=EDGE_CURVE('',#35211,#35212,#20567,.T.);
#43769=EDGE_CURVE('',#35212,#35213,#29249,.T.);
#43770=EDGE_CURVE('',#35213,#35214,#20568,.T.);
#43771=EDGE_CURVE('',#35215,#35214,#4127,.T.);
#43772=EDGE_CURVE('',#35216,#35215,#29250,.T.);
#43773=EDGE_CURVE('',#35211,#35216,#4128,.T.);
#43774=EDGE_CURVE('',#35217,#35218,#29251,.T.);
#43775=EDGE_CURVE('',#35217,#35219,#20569,.T.);
#43776=EDGE_CURVE('',#35219,#35220,#29252,.T.);
#43777=EDGE_CURVE('',#35220,#35221,#20570,.T.);
#43778=EDGE_CURVE('',#35218,#35221,#4129,.T.);
#43779=EDGE_CURVE('',#35217,#35222,#29253,.T.);
#43780=EDGE_CURVE('',#35218,#35223,#29254,.T.);
#43781=EDGE_CURVE('',#35223,#35222,#29255,.T.);
#43782=EDGE_CURVE('',#35221,#35224,#29256,.T.);
#43783=EDGE_CURVE('',#35224,#35223,#4130,.T.);
#43784=EDGE_CURVE('',#35225,#35226,#20571,.T.);
#43785=EDGE_CURVE('',#35226,#35227,#29257,.T.);
#43786=EDGE_CURVE('',#35227,#35228,#20572,.T.);
#43787=EDGE_CURVE('',#35225,#35228,#29258,.T.);
#43788=EDGE_CURVE('',#35229,#35230,#20573,.T.);
#43789=EDGE_CURVE('',#35231,#35229,#20574,.T.);
#43790=EDGE_CURVE('',#35232,#35231,#4131,.T.);
#43791=EDGE_CURVE('',#35233,#35232,#20575,.T.);
#43792=EDGE_CURVE('',#35234,#35233,#4132,.T.);
#43793=EDGE_CURVE('',#35235,#35234,#20576,.T.);
#43794=EDGE_CURVE('',#35236,#35235,#20577,.T.);
#43795=EDGE_CURVE('',#35237,#35236,#4133,.T.);
#43796=EDGE_CURVE('',#35238,#35237,#20578,.T.);
#43797=EDGE_CURVE('',#35221,#35238,#4134,.T.);
#43798=EDGE_CURVE('',#35226,#35220,#20579,.T.);
#43799=EDGE_CURVE('',#35239,#35225,#20580,.T.);
#43800=EDGE_CURVE('',#35240,#35239,#20581,.T.);
#43801=EDGE_CURVE('',#35241,#35240,#4135,.T.);
#43802=EDGE_CURVE('',#35242,#35241,#20582,.T.);
#43803=EDGE_CURVE('',#35243,#35242,#4136,.T.);
#43804=EDGE_CURVE('',#35230,#35243,#20583,.T.);
#43805=EDGE_CURVE('',#35225,#35244,#29259,.T.);
#43806=EDGE_CURVE('',#35228,#35245,#29260,.T.);
#43807=EDGE_CURVE('',#35245,#35244,#29261,.T.);
#43808=EDGE_CURVE('',#35246,#35247,#20584,.T.);
#43809=EDGE_CURVE('',#35247,#35248,#29262,.T.);
#43810=EDGE_CURVE('',#35248,#35249,#20585,.T.);
#43811=EDGE_CURVE('',#35246,#35249,#29263,.T.);
#43812=EDGE_CURVE('',#35247,#35227,#20586,.T.);
#43813=EDGE_CURVE('',#35228,#35246,#20587,.T.);
#43814=EDGE_CURVE('',#35246,#35250,#29264,.T.);
#43815=EDGE_CURVE('',#35249,#35251,#29265,.T.);
#43816=EDGE_CURVE('',#35251,#35250,#29266,.T.);
#43817=EDGE_CURVE('',#35252,#35253,#4137,.T.);
#43818=EDGE_CURVE('',#35254,#35252,#20588,.T.);
#43819=EDGE_CURVE('',#35255,#35254,#20589,.T.);
#43820=EDGE_CURVE('',#35256,#35255,#4138,.T.);
#43821=EDGE_CURVE('',#35257,#35256,#20590,.T.);
#43822=EDGE_CURVE('',#35258,#35257,#4139,.T.);
#43823=EDGE_CURVE('',#35259,#35258,#20591,.T.);
#43824=EDGE_CURVE('',#35260,#35259,#20592,.T.);
#43825=EDGE_CURVE('',#35261,#35260,#20593,.T.);
#43826=EDGE_CURVE('',#35262,#35261,#4140,.T.);
#43827=EDGE_CURVE('',#35263,#35262,#20594,.T.);
#43828=EDGE_CURVE('',#35264,#35263,#4141,.T.);
#43829=EDGE_CURVE('',#35265,#35264,#20595,.T.);
#43830=EDGE_CURVE('',#35249,#35265,#20596,.T.);
#43831=EDGE_CURVE('',#35212,#35248,#20597,.T.);
#43832=EDGE_CURVE('',#35266,#35211,#1771,.T.);
#43833=EDGE_CURVE('',#35253,#35266,#20598,.T.);
#43834=EDGE_CURVE('',#35267,#35268,#29267,.T.);
#43835=EDGE_CURVE('',#35267,#35269,#4142,.T.);
#43836=EDGE_CURVE('',#35269,#35270,#29268,.T.);
#43837=EDGE_CURVE('',#35270,#35268,#4143,.T.);
#43838=EDGE_CURVE('',#35271,#35272,#29269,.T.);
#43839=EDGE_CURVE('',#35271,#35267,#20599,.T.);
#43840=EDGE_CURVE('',#35268,#35272,#20600,.T.);
#43841=EDGE_CURVE('',#35273,#35274,#29270,.T.);
#43842=EDGE_CURVE('',#35272,#35274,#29271,.T.);
#43843=EDGE_CURVE('',#35272,#35275,#29272,.T.);
#43844=EDGE_CURVE('',#35273,#35275,#1772,.T.);
#43845=EDGE_CURVE('',#35276,#35277,#29273,.T.);
#43846=EDGE_CURVE('',#35277,#35278,#20601,.T.);
#43847=EDGE_CURVE('',#35279,#35278,#29274,.T.);
#43848=EDGE_CURVE('',#35275,#35279,#29275,.T.);
#43849=EDGE_CURVE('',#35275,#35280,#20602,.T.);
#43850=EDGE_CURVE('',#35280,#35276,#29276,.T.);
#43851=EDGE_CURVE('',#35280,#35281,#4144,.T.);
#43852=EDGE_CURVE('',#35281,#35282,#29277,.T.);
#43853=EDGE_CURVE('',#35282,#35277,#4145,.T.);
#43854=EDGE_CURVE('',#35281,#35283,#29278,.T.);
#43855=EDGE_CURVE('',#35283,#35284,#29279,.T.);
#43856=EDGE_CURVE('',#35284,#35282,#29280,.T.);
#43857=EDGE_CURVE('',#35283,#35285,#4146,.T.);
#43858=EDGE_CURVE('',#35286,#35285,#29281,.T.);
#43859=EDGE_CURVE('',#35286,#35284,#4147,.T.);
#43860=EDGE_CURVE('',#35287,#35288,#29282,.T.);
#43861=EDGE_CURVE('',#35287,#35286,#20603,.T.);
#43862=EDGE_CURVE('',#35285,#35288,#20604,.T.);
#43863=EDGE_CURVE('',#35289,#35290,#29283,.T.);
#43864=EDGE_CURVE('',#35288,#35290,#1773,.T.);
#43865=EDGE_CURVE('',#35288,#35291,#29284,.T.);
#43866=EDGE_CURVE('',#35289,#35291,#1774,.T.);
#43867=EDGE_CURVE('',#35292,#35293,#29285,.T.);
#43868=EDGE_CURVE('',#35293,#35294,#20605,.T.);
#43869=EDGE_CURVE('',#35295,#35294,#29286,.T.);
#43870=EDGE_CURVE('',#35291,#35295,#29287,.T.);
#43871=EDGE_CURVE('',#35291,#35292,#20606,.T.);
#43872=EDGE_CURVE('',#35292,#35296,#4148,.T.);
#43873=EDGE_CURVE('',#35296,#35297,#29288,.T.);
#43874=EDGE_CURVE('',#35297,#35293,#4149,.T.);
#43875=EDGE_CURVE('',#35296,#35298,#29289,.T.);
#43876=EDGE_CURVE('',#35298,#35299,#29290,.T.);
#43877=EDGE_CURVE('',#35299,#35297,#29291,.T.);
#43878=EDGE_CURVE('',#35298,#35300,#4150,.T.);
#43879=EDGE_CURVE('',#35301,#35300,#29292,.T.);
#43880=EDGE_CURVE('',#35301,#35299,#4151,.T.);
#43881=EDGE_CURVE('',#35302,#35303,#29293,.T.);
#43882=EDGE_CURVE('',#35302,#35301,#20607,.T.);
#43883=EDGE_CURVE('',#35300,#35303,#20608,.T.);
#43884=EDGE_CURVE('',#35304,#35305,#29294,.T.);
#43885=EDGE_CURVE('',#35303,#35305,#1775,.T.);
#43886=EDGE_CURVE('',#35303,#35306,#29295,.T.);
#43887=EDGE_CURVE('',#35304,#35306,#1776,.T.);
#43888=EDGE_CURVE('',#35307,#35308,#29296,.T.);
#43889=EDGE_CURVE('',#35308,#35309,#20609,.T.);
#43890=EDGE_CURVE('',#35306,#35309,#29297,.T.);
#43891=EDGE_CURVE('',#35306,#35307,#20610,.T.);
#43892=EDGE_CURVE('',#35307,#35310,#4152,.T.);
#43893=EDGE_CURVE('',#35310,#35311,#29298,.T.);
#43894=EDGE_CURVE('',#35311,#35308,#4153,.T.);
#43895=EDGE_CURVE('',#35310,#35217,#29299,.T.);
#43896=EDGE_CURVE('',#35222,#35311,#29300,.T.);
#43897=EDGE_CURVE('',#35312,#35313,#20611,.T.);
#43898=EDGE_CURVE('',#35313,#35314,#29301,.T.);
#43899=EDGE_CURVE('',#35314,#35315,#20612,.T.);
#43900=EDGE_CURVE('',#35312,#35315,#4154,.T.);
#43901=EDGE_CURVE('',#35316,#35317,#29302,.T.);
#43902=EDGE_CURVE('',#35315,#35317,#29303,.T.);
#43903=EDGE_CURVE('',#35315,#35318,#29304,.T.);
#43904=EDGE_CURVE('',#35316,#35318,#4155,.T.);
#43905=EDGE_CURVE('',#35319,#35320,#29305,.T.);
#43906=EDGE_CURVE('',#35319,#35321,#20613,.T.);
#43907=EDGE_CURVE('',#35321,#35318,#29306,.T.);
#43908=EDGE_CURVE('',#35318,#35320,#20614,.T.);
#43909=EDGE_CURVE('',#35322,#35323,#29307,.T.);
#43910=EDGE_CURVE('',#35322,#35319,#4156,.T.);
#43911=EDGE_CURVE('',#35320,#35323,#4157,.T.);
#43912=EDGE_CURVE('',#35324,#35325,#29308,.T.);
#43913=EDGE_CURVE('',#35324,#35322,#29309,.T.);
#43914=EDGE_CURVE('',#35323,#35325,#29310,.T.);
#43915=EDGE_CURVE('',#35326,#35327,#29311,.T.);
#43916=EDGE_CURVE('',#35326,#35324,#4158,.T.);
#43917=EDGE_CURVE('',#35325,#35327,#4159,.T.);
#43918=EDGE_CURVE('',#35327,#35328,#20615,.T.);
#43919=EDGE_CURVE('',#35328,#35329,#29312,.T.);
#43920=EDGE_CURVE('',#35329,#35326,#20616,.T.);
#43921=EDGE_CURVE('',#35330,#35331,#29313,.T.);
#43922=EDGE_CURVE('',#35328,#35331,#1777,.T.);
#43923=EDGE_CURVE('',#35328,#35332,#29314,.T.);
#43924=EDGE_CURVE('',#35330,#35332,#1778,.T.);
#43925=EDGE_CURVE('',#35333,#35334,#29315,.T.);
#43926=EDGE_CURVE('',#35333,#35335,#20617,.T.);
#43927=EDGE_CURVE('',#35335,#35332,#29316,.T.);
#43928=EDGE_CURVE('',#35332,#35334,#20618,.T.);
#43929=EDGE_CURVE('',#35336,#35337,#29317,.T.);
#43930=EDGE_CURVE('',#35336,#35333,#4160,.T.);
#43931=EDGE_CURVE('',#35334,#35337,#4161,.T.);
#43932=EDGE_CURVE('',#35338,#35339,#29318,.T.);
#43933=EDGE_CURVE('',#35338,#35336,#29319,.T.);
#43934=EDGE_CURVE('',#35337,#35339,#29320,.T.);
#43935=EDGE_CURVE('',#35340,#35341,#29321,.T.);
#43936=EDGE_CURVE('',#35340,#35338,#4162,.T.);
#43937=EDGE_CURVE('',#35339,#35341,#4163,.T.);
#43938=EDGE_CURVE('',#35342,#35343,#29322,.T.);
#43939=EDGE_CURVE('',#35342,#35340,#20619,.T.);
#43940=EDGE_CURVE('',#35341,#35343,#20620,.T.);
#43941=EDGE_CURVE('',#35344,#35345,#29323,.T.);
#43942=EDGE_CURVE('',#35343,#35345,#1779,.T.);
#43943=EDGE_CURVE('',#35343,#35346,#29324,.T.);
#43944=EDGE_CURVE('',#35344,#35346,#29325,.T.);
#43945=EDGE_CURVE('',#35347,#35348,#29326,.T.);
#43946=EDGE_CURVE('',#35347,#35349,#20621,.T.);
#43947=EDGE_CURVE('',#35349,#35346,#29327,.T.);
#43948=EDGE_CURVE('',#35346,#35348,#20622,.T.);
#43949=EDGE_CURVE('',#35350,#35351,#29328,.T.);
#43950=EDGE_CURVE('',#35350,#35347,#4164,.T.);
#43951=EDGE_CURVE('',#35348,#35351,#4165,.T.);
#43952=EDGE_CURVE('',#35352,#35353,#29329,.T.);
#43953=EDGE_CURVE('',#35352,#35350,#29330,.T.);
#43954=EDGE_CURVE('',#35351,#35353,#29331,.T.);
#43955=EDGE_CURVE('',#35354,#35355,#29332,.T.);
#43956=EDGE_CURVE('',#35354,#35352,#4166,.T.);
#43957=EDGE_CURVE('',#35353,#35355,#4167,.T.);
#43958=EDGE_CURVE('',#35356,#35357,#29333,.T.);
#43959=EDGE_CURVE('',#35356,#35354,#20623,.T.);
#43960=EDGE_CURVE('',#35355,#35357,#20624,.T.);
#43961=EDGE_CURVE('',#35211,#35358,#29334,.T.);
#43962=EDGE_CURVE('',#35216,#35359,#29335,.T.);
#43963=EDGE_CURVE('',#35359,#35358,#4168,.T.);
#43964=EDGE_CURVE('',#35215,#35360,#29336,.T.);
#43965=EDGE_CURVE('',#35360,#35359,#29337,.T.);
#43966=EDGE_CURVE('',#35214,#35361,#29338,.T.);
#43967=EDGE_CURVE('',#35361,#35360,#4169,.T.);
#43968=EDGE_CURVE('',#35362,#35363,#20625,.T.);
#43969=EDGE_CURVE('',#35363,#35364,#29339,.T.);
#43970=EDGE_CURVE('',#35364,#35365,#20626,.T.);
#43971=EDGE_CURVE('',#35366,#35365,#4170,.T.);
#43972=EDGE_CURVE('',#35367,#35366,#29340,.T.);
#43973=EDGE_CURVE('',#35362,#35367,#29341,.T.);
#43974=EDGE_CURVE('',#35213,#35363,#29342,.T.);
#43975=EDGE_CURVE('',#35368,#35362,#4171,.T.);
#43976=EDGE_CURVE('',#35369,#35368,#20627,.T.);
#43977=EDGE_CURVE('',#35370,#35369,#29343,.T.);
#43978=EDGE_CURVE('',#35371,#35370,#20628,.T.);
#43979=EDGE_CURVE('',#35372,#35371,#4172,.T.);
#43980=EDGE_CURVE('',#35373,#35372,#29344,.T.);
#43981=EDGE_CURVE('',#35374,#35373,#4173,.T.);
#43982=EDGE_CURVE('',#35375,#35374,#20629,.T.);
#43983=EDGE_CURVE('',#35376,#35375,#29345,.T.);
#43984=EDGE_CURVE('',#35377,#35376,#20630,.T.);
#43985=EDGE_CURVE('',#35378,#35377,#4174,.T.);
#43986=EDGE_CURVE('',#35379,#35378,#29346,.T.);
#43987=EDGE_CURVE('',#35380,#35379,#4175,.T.);
#43988=EDGE_CURVE('',#35381,#35380,#20631,.T.);
#43989=EDGE_CURVE('',#35382,#35381,#29347,.T.);
#43990=EDGE_CURVE('',#35383,#35382,#20632,.T.);
#43991=EDGE_CURVE('',#35384,#35383,#4176,.T.);
#43992=EDGE_CURVE('',#35385,#35384,#29348,.T.);
#43993=EDGE_CURVE('',#35386,#35385,#4177,.T.);
#43994=EDGE_CURVE('',#35387,#35386,#20633,.T.);
#43995=EDGE_CURVE('',#35388,#35387,#29349,.T.);
#43996=EDGE_CURVE('',#35389,#35388,#20634,.T.);
#43997=EDGE_CURVE('',#35390,#35389,#4178,.T.);
#43998=EDGE_CURVE('',#35391,#35390,#29350,.T.);
#43999=EDGE_CURVE('',#35392,#35391,#4179,.T.);
#44000=EDGE_CURVE('',#35393,#35392,#20635,.T.);
#44001=EDGE_CURVE('',#35394,#35393,#29351,.T.);
#44002=EDGE_CURVE('',#35395,#35394,#20636,.T.);
#44003=EDGE_CURVE('',#35396,#35395,#4180,.T.);
#44004=EDGE_CURVE('',#35397,#35396,#29352,.T.);
#44005=EDGE_CURVE('',#35398,#35397,#4181,.T.);
#44006=EDGE_CURVE('',#35399,#35398,#20637,.T.);
#44007=EDGE_CURVE('',#35400,#35399,#29353,.T.);
#44008=EDGE_CURVE('',#35401,#35400,#20638,.T.);
#44009=EDGE_CURVE('',#35214,#35401,#4182,.T.);
#44010=EDGE_CURVE('',#35402,#35367,#29354,.T.);
#44011=EDGE_CURVE('',#35402,#35403,#4183,.T.);
#44012=EDGE_CURVE('',#35403,#35362,#29355,.T.);
#44013=EDGE_CURVE('',#35366,#35404,#29356,.T.);
#44014=EDGE_CURVE('',#35404,#35402,#29357,.T.);
#44015=EDGE_CURVE('',#35365,#35405,#29358,.T.);
#44016=EDGE_CURVE('',#35405,#35404,#4184,.T.);
#44017=EDGE_CURVE('',#35406,#35407,#20639,.T.);
#44018=EDGE_CURVE('',#35407,#35408,#29359,.T.);
#44019=EDGE_CURVE('',#35408,#35409,#20640,.T.);
#44020=EDGE_CURVE('',#35406,#35409,#29360,.T.);
#44021=EDGE_CURVE('',#35410,#35411,#20641,.T.);
#44022=EDGE_CURVE('',#35412,#35410,#20642,.T.);
#44023=EDGE_CURVE('',#35413,#35412,#4185,.T.);
#44024=EDGE_CURVE('',#35414,#35413,#20643,.T.);
#44025=EDGE_CURVE('',#35415,#35414,#4186,.T.);
#44026=EDGE_CURVE('',#35416,#35415,#20644,.T.);
#44027=EDGE_CURVE('',#35417,#35416,#20645,.T.);
#44028=EDGE_CURVE('',#35418,#35417,#4187,.T.);
#44029=EDGE_CURVE('',#35419,#35418,#20646,.T.);
#44030=EDGE_CURVE('',#35365,#35419,#1780,.T.);
#44031=EDGE_CURVE('',#35407,#35364,#20647,.T.);
#44032=EDGE_CURVE('',#35420,#35406,#20648,.T.);
#44033=EDGE_CURVE('',#35421,#35420,#20649,.T.);
#44034=EDGE_CURVE('',#35422,#35421,#4188,.T.);
#44035=EDGE_CURVE('',#35423,#35422,#20650,.T.);
#44036=EDGE_CURVE('',#35424,#35423,#4189,.T.);
#44037=EDGE_CURVE('',#35411,#35424,#20651,.T.);
#44038=EDGE_CURVE('',#35406,#35425,#29361,.T.);
#44039=EDGE_CURVE('',#35409,#35426,#29362,.T.);
#44040=EDGE_CURVE('',#35426,#35425,#29363,.T.);
#44041=EDGE_CURVE('',#35427,#35428,#20652,.T.);
#44042=EDGE_CURVE('',#35428,#35429,#29364,.T.);
#44043=EDGE_CURVE('',#35429,#35430,#20653,.T.);
#44044=EDGE_CURVE('',#35427,#35430,#29365,.T.);
#44045=EDGE_CURVE('',#35428,#35408,#20654,.T.);
#44046=EDGE_CURVE('',#35409,#35427,#20655,.T.);
#44047=EDGE_CURVE('',#35427,#35431,#29366,.T.);
#44048=EDGE_CURVE('',#35430,#35432,#29367,.T.);
#44049=EDGE_CURVE('',#35432,#35431,#29368,.T.);
#44050=EDGE_CURVE('',#35433,#35434,#20656,.T.);
#44051=EDGE_CURVE('',#35435,#35433,#20657,.T.);
#44052=EDGE_CURVE('',#35436,#35435,#4190,.T.);
#44053=EDGE_CURVE('',#35437,#35436,#20658,.T.);
#44054=EDGE_CURVE('',#35438,#35437,#4191,.T.);
#44055=EDGE_CURVE('',#35439,#35438,#20659,.T.);
#44056=EDGE_CURVE('',#35430,#35439,#20660,.T.);
#44057=EDGE_CURVE('',#35313,#35429,#20661,.T.);
#44058=EDGE_CURVE('',#35440,#35312,#4192,.T.);
#44059=EDGE_CURVE('',#35441,#35440,#20662,.T.);
#44060=EDGE_CURVE('',#35442,#35441,#4193,.T.);
#44061=EDGE_CURVE('',#35443,#35442,#20663,.T.);
#44062=EDGE_CURVE('',#35444,#35443,#4194,.T.);
#44063=EDGE_CURVE('',#35434,#35444,#20664,.T.);
#44064=EDGE_CURVE('',#35401,#35445,#29369,.T.);
#44065=EDGE_CURVE('',#35445,#35361,#4195,.T.);
#44066=EDGE_CURVE('',#35400,#35446,#29370,.T.);
#44067=EDGE_CURVE('',#35446,#35445,#20665,.T.);
#44068=EDGE_CURVE('',#35447,#35448,#29371,.T.);
#44069=EDGE_CURVE('',#35400,#35448,#1781,.T.);
#44070=EDGE_CURVE('',#35447,#35399,#1782,.T.);
#44071=EDGE_CURVE('',#35449,#35398,#29372,.T.);
#44072=EDGE_CURVE('',#35449,#35450,#20666,.T.);
#44073=EDGE_CURVE('',#35450,#35399,#29373,.T.);
#44074=EDGE_CURVE('',#35451,#35397,#29374,.T.);
#44075=EDGE_CURVE('',#35451,#35449,#4196,.T.);
#44076=EDGE_CURVE('',#35452,#35396,#29375,.T.);
#44077=EDGE_CURVE('',#35452,#35451,#29376,.T.);
#44078=EDGE_CURVE('',#35453,#35395,#29377,.T.);
#44079=EDGE_CURVE('',#35453,#35452,#4197,.T.);
#44080=EDGE_CURVE('',#35454,#35394,#29378,.T.);
#44081=EDGE_CURVE('',#35454,#35453,#20667,.T.);
#44082=EDGE_CURVE('',#35455,#35456,#29379,.T.);
#44083=EDGE_CURVE('',#35394,#35456,#1783,.T.);
#44084=EDGE_CURVE('',#35455,#35393,#1784,.T.);
#44085=EDGE_CURVE('',#35393,#35457,#29380,.T.);
#44086=EDGE_CURVE('',#35392,#35458,#29381,.T.);
#44087=EDGE_CURVE('',#35458,#35457,#20668,.T.);
#44088=EDGE_CURVE('',#35391,#35459,#29382,.T.);
#44089=EDGE_CURVE('',#35459,#35458,#4198,.T.);
#44090=EDGE_CURVE('',#35390,#35460,#29383,.T.);
#44091=EDGE_CURVE('',#35460,#35459,#29384,.T.);
#44092=EDGE_CURVE('',#35461,#35389,#29385,.T.);
#44093=EDGE_CURVE('',#35461,#35460,#4199,.T.);
#44094=EDGE_CURVE('',#35462,#35388,#29386,.T.);
#44095=EDGE_CURVE('',#35462,#35461,#20669,.T.);
#44096=EDGE_CURVE('',#35463,#35464,#29387,.T.);
#44097=EDGE_CURVE('',#35388,#35464,#1785,.T.);
#44098=EDGE_CURVE('',#35463,#35387,#29388,.T.);
#44099=EDGE_CURVE('',#35387,#35465,#29389,.T.);
#44100=EDGE_CURVE('',#35386,#35466,#29390,.T.);
#44101=EDGE_CURVE('',#35466,#35465,#20670,.T.);
#44102=EDGE_CURVE('',#35385,#35467,#29391,.T.);
#44103=EDGE_CURVE('',#35467,#35466,#4200,.T.);
#44104=EDGE_CURVE('',#35384,#35468,#29392,.T.);
#44105=EDGE_CURVE('',#35468,#35467,#29393,.T.);
#44106=EDGE_CURVE('',#35469,#35383,#29394,.T.);
#44107=EDGE_CURVE('',#35469,#35468,#4201,.T.);
#44108=EDGE_CURVE('',#35470,#35382,#29395,.T.);
#44109=EDGE_CURVE('',#35470,#35469,#20671,.T.);
#44110=EDGE_CURVE('',#35471,#35472,#29396,.T.);
#44111=EDGE_CURVE('',#35382,#35472,#29397,.T.);
#44112=EDGE_CURVE('',#35471,#35381,#1786,.T.);
#44113=EDGE_CURVE('',#35381,#35473,#29398,.T.);
#44114=EDGE_CURVE('',#35380,#35474,#29399,.T.);
#44115=EDGE_CURVE('',#35474,#35473,#20672,.T.);
#44116=EDGE_CURVE('',#35379,#35475,#29400,.T.);
#44117=EDGE_CURVE('',#35475,#35474,#4202,.T.);
#44118=EDGE_CURVE('',#35378,#35476,#29401,.T.);
#44119=EDGE_CURVE('',#35476,#35475,#29402,.T.);
#44120=EDGE_CURVE('',#35477,#35377,#29403,.T.);
#44121=EDGE_CURVE('',#35477,#35476,#4203,.T.);
#44122=EDGE_CURVE('',#35478,#35376,#29404,.T.);
#44123=EDGE_CURVE('',#35478,#35477,#20673,.T.);
#44124=EDGE_CURVE('',#35479,#35480,#29405,.T.);
#44125=EDGE_CURVE('',#35376,#35480,#1787,.T.);
#44126=EDGE_CURVE('',#35479,#35375,#1788,.T.);
#44127=EDGE_CURVE('',#35481,#35374,#29406,.T.);
#44128=EDGE_CURVE('',#35481,#35482,#20674,.T.);
#44129=EDGE_CURVE('',#35482,#35375,#29407,.T.);
#44130=EDGE_CURVE('',#35483,#35373,#29408,.T.);
#44131=EDGE_CURVE('',#35483,#35481,#4204,.T.);
#44132=EDGE_CURVE('',#35484,#35372,#29409,.T.);
#44133=EDGE_CURVE('',#35484,#35483,#29410,.T.);
#44134=EDGE_CURVE('',#35485,#35371,#29411,.T.);
#44135=EDGE_CURVE('',#35485,#35484,#4205,.T.);
#44136=EDGE_CURVE('',#35486,#35370,#29412,.T.);
#44137=EDGE_CURVE('',#35486,#35485,#20675,.T.);
#44138=EDGE_CURVE('',#35487,#35488,#29413,.T.);
#44139=EDGE_CURVE('',#35370,#35488,#1789,.T.);
#44140=EDGE_CURVE('',#35487,#35369,#1790,.T.);
#44141=EDGE_CURVE('',#35489,#35368,#29414,.T.);
#44142=EDGE_CURVE('',#35489,#35490,#20676,.T.);
#44143=EDGE_CURVE('',#35490,#35369,#29415,.T.);
#44144=EDGE_CURVE('',#35403,#35489,#4206,.T.);
#44145=EDGE_CURVE('',#35491,#35492,#20677,.T.);
#44146=EDGE_CURVE('',#35229,#35492,#4207,.T.);
#44147=EDGE_CURVE('',#35491,#35230,#4208,.T.);
#44148=EDGE_CURVE('',#35230,#35493,#29416,.T.);
#44149=EDGE_CURVE('',#35243,#35494,#29417,.T.);
#44150=EDGE_CURVE('',#35494,#35493,#20678,.T.);
#44151=EDGE_CURVE('',#35242,#35495,#29418,.T.);
#44152=EDGE_CURVE('',#35495,#35494,#4209,.T.);
#44153=EDGE_CURVE('',#35241,#35496,#29419,.T.);
#44154=EDGE_CURVE('',#35496,#35495,#20679,.T.);
#44155=EDGE_CURVE('',#35240,#35497,#29420,.T.);
#44156=EDGE_CURVE('',#35497,#35496,#4210,.T.);
#44157=EDGE_CURVE('',#35239,#35498,#29421,.T.);
#44158=EDGE_CURVE('',#35498,#35497,#20680,.T.);
#44159=EDGE_CURVE('',#35244,#35499,#20681,.T.);
#44160=EDGE_CURVE('',#35239,#35499,#4211,.T.);
#44161=EDGE_CURVE('',#35500,#35238,#29422,.T.);
#44162=EDGE_CURVE('',#35500,#35224,#4212,.T.);
#44163=EDGE_CURVE('',#35501,#35237,#29423,.T.);
#44164=EDGE_CURVE('',#35501,#35500,#20682,.T.);
#44165=EDGE_CURVE('',#35502,#35236,#29424,.T.);
#44166=EDGE_CURVE('',#35502,#35503,#4213,.T.);
#44167=EDGE_CURVE('',#35237,#35503,#4214,.T.);
#44168=EDGE_CURVE('',#35504,#35502,#20683,.T.);
#44169=EDGE_CURVE('',#35504,#35235,#4215,.T.);
#44170=EDGE_CURVE('',#35235,#35505,#29425,.T.);
#44171=EDGE_CURVE('',#35234,#35506,#29426,.T.);
#44172=EDGE_CURVE('',#35506,#35505,#20684,.T.);
#44173=EDGE_CURVE('',#35233,#35507,#29427,.T.);
#44174=EDGE_CURVE('',#35507,#35506,#4216,.T.);
#44175=EDGE_CURVE('',#35232,#35508,#29428,.T.);
#44176=EDGE_CURVE('',#35508,#35507,#20685,.T.);
#44177=EDGE_CURVE('',#35509,#35231,#29429,.T.);
#44178=EDGE_CURVE('',#35509,#35508,#4217,.T.);
#44179=EDGE_CURVE('',#35510,#35229,#29430,.T.);
#44180=EDGE_CURVE('',#35510,#35509,#20686,.T.);
#44181=EDGE_CURVE('',#35250,#35245,#20687,.T.);
#44182=EDGE_CURVE('',#35312,#35511,#29431,.T.);
#44183=EDGE_CURVE('',#35317,#35511,#4218,.T.);
#44184=EDGE_CURVE('',#35512,#35513,#20688,.T.);
#44185=EDGE_CURVE('',#35433,#35513,#4219,.T.);
#44186=EDGE_CURVE('',#35512,#35434,#4220,.T.);
#44187=EDGE_CURVE('',#35514,#35444,#29432,.T.);
#44188=EDGE_CURVE('',#35514,#35515,#20689,.T.);
#44189=EDGE_CURVE('',#35515,#35434,#29433,.T.);
#44190=EDGE_CURVE('',#35516,#35443,#29434,.T.);
#44191=EDGE_CURVE('',#35516,#35514,#4221,.T.);
#44192=EDGE_CURVE('',#35517,#35442,#29435,.T.);
#44193=EDGE_CURVE('',#35517,#35516,#20690,.T.);
#44194=EDGE_CURVE('',#35518,#35441,#29436,.T.);
#44195=EDGE_CURVE('',#35518,#35517,#4222,.T.);
#44196=EDGE_CURVE('',#35440,#35519,#29437,.T.);
#44197=EDGE_CURVE('',#35519,#35518,#20691,.T.);
#44198=EDGE_CURVE('',#35511,#35520,#4223,.T.);
#44199=EDGE_CURVE('',#35440,#35520,#4224,.T.);
#44200=EDGE_CURVE('',#35521,#35432,#20692,.T.);
#44201=EDGE_CURVE('',#35521,#35439,#4225,.T.);
#44202=EDGE_CURVE('',#35439,#35522,#29438,.T.);
#44203=EDGE_CURVE('',#35438,#35523,#29439,.T.);
#44204=EDGE_CURVE('',#35523,#35522,#20693,.T.);
#44205=EDGE_CURVE('',#35437,#35524,#29440,.T.);
#44206=EDGE_CURVE('',#35524,#35523,#4226,.T.);
#44207=EDGE_CURVE('',#35436,#35525,#29441,.T.);
#44208=EDGE_CURVE('',#35525,#35524,#20694,.T.);
#44209=EDGE_CURVE('',#35435,#35526,#29442,.T.);
#44210=EDGE_CURVE('',#35526,#35525,#4227,.T.);
#44211=EDGE_CURVE('',#35433,#35527,#29443,.T.);
#44212=EDGE_CURVE('',#35527,#35526,#20695,.T.);
#44213=EDGE_CURVE('',#35431,#35426,#20696,.T.);
#44214=EDGE_CURVE('',#35528,#35529,#20697,.T.);
#44215=EDGE_CURVE('',#35410,#35529,#4228,.T.);
#44216=EDGE_CURVE('',#35528,#35411,#4229,.T.);
#44217=EDGE_CURVE('',#35530,#35424,#29444,.T.);
#44218=EDGE_CURVE('',#35530,#35531,#20698,.T.);
#44219=EDGE_CURVE('',#35531,#35411,#29445,.T.);
#44220=EDGE_CURVE('',#35532,#35423,#29446,.T.);
#44221=EDGE_CURVE('',#35532,#35530,#4230,.T.);
#44222=EDGE_CURVE('',#35533,#35422,#29447,.T.);
#44223=EDGE_CURVE('',#35533,#35532,#20699,.T.);
#44224=EDGE_CURVE('',#35534,#35421,#29448,.T.);
#44225=EDGE_CURVE('',#35534,#35533,#4231,.T.);
#44226=EDGE_CURVE('',#35535,#35420,#29449,.T.);
#44227=EDGE_CURVE('',#35535,#35534,#20700,.T.);
#44228=EDGE_CURVE('',#35425,#35536,#20701,.T.);
#44229=EDGE_CURVE('',#35420,#35536,#4232,.T.);
#44230=EDGE_CURVE('',#35419,#35537,#29450,.T.);
#44231=EDGE_CURVE('',#35537,#35405,#1791,.T.);
#44232=EDGE_CURVE('',#35418,#35538,#29451,.T.);
#44233=EDGE_CURVE('',#35538,#35537,#20702,.T.);
#44234=EDGE_CURVE('',#35539,#35417,#29452,.T.);
#44235=EDGE_CURVE('',#35539,#35540,#1068,.T.);
#44236=EDGE_CURVE('',#35540,#35541,#29453,.T.);
#44237=EDGE_CURVE('',#35418,#35541,#4233,.T.);
#44238=EDGE_CURVE('',#35542,#35539,#20703,.T.);
#44239=EDGE_CURVE('',#35542,#35416,#4234,.T.);
#44240=EDGE_CURVE('',#35416,#35543,#29454,.T.);
#44241=EDGE_CURVE('',#35415,#35544,#29455,.T.);
#44242=EDGE_CURVE('',#35544,#35543,#20704,.T.);
#44243=EDGE_CURVE('',#35414,#35545,#29456,.T.);
#44244=EDGE_CURVE('',#35545,#35544,#4235,.T.);
#44245=EDGE_CURVE('',#35413,#35546,#29457,.T.);
#44246=EDGE_CURVE('',#35546,#35545,#20705,.T.);
#44247=EDGE_CURVE('',#35547,#35412,#29458,.T.);
#44248=EDGE_CURVE('',#35547,#35546,#4236,.T.);
#44249=EDGE_CURVE('',#35548,#35410,#29459,.T.);
#44250=EDGE_CURVE('',#35548,#35547,#20706,.T.);
#44251=EDGE_CURVE('',#35549,#35550,#4237,.T.);
#44252=EDGE_CURVE('',#35252,#35550,#29460,.T.);
#44253=EDGE_CURVE('',#35549,#35253,#4238,.T.);
#44254=EDGE_CURVE('',#35551,#35266,#29461,.T.);
#44255=EDGE_CURVE('',#35551,#35552,#20707,.T.);
#44256=EDGE_CURVE('',#35552,#35253,#29462,.T.);
#44257=EDGE_CURVE('',#35358,#35551,#1792,.T.);
#44258=EDGE_CURVE('',#35553,#35251,#20708,.T.);
#44259=EDGE_CURVE('',#35553,#35265,#4239,.T.);
#44260=EDGE_CURVE('',#35265,#35554,#29463,.T.);
#44261=EDGE_CURVE('',#35264,#35555,#29464,.T.);
#44262=EDGE_CURVE('',#35555,#35554,#20709,.T.);
#44263=EDGE_CURVE('',#35263,#35556,#29465,.T.);
#44264=EDGE_CURVE('',#35556,#35555,#4240,.T.);
#44265=EDGE_CURVE('',#35262,#35557,#29466,.T.);
#44266=EDGE_CURVE('',#35557,#35556,#20710,.T.);
#44267=EDGE_CURVE('',#35261,#35558,#29467,.T.);
#44268=EDGE_CURVE('',#35558,#35557,#4241,.T.);
#44269=EDGE_CURVE('',#35260,#35559,#29468,.T.);
#44270=EDGE_CURVE('',#35559,#35558,#20711,.T.);
#44271=EDGE_CURVE('',#35560,#35561,#20712,.T.);
#44272=EDGE_CURVE('',#35260,#35561,#4242,.T.);
#44273=EDGE_CURVE('',#35560,#35259,#4243,.T.);
#44274=EDGE_CURVE('',#35259,#35562,#29469,.T.);
#44275=EDGE_CURVE('',#35258,#35563,#29470,.T.);
#44276=EDGE_CURVE('',#35563,#35562,#20713,.T.);
#44277=EDGE_CURVE('',#35257,#35564,#29471,.T.);
#44278=EDGE_CURVE('',#35564,#35563,#4244,.T.);
#44279=EDGE_CURVE('',#35256,#35565,#29472,.T.);
#44280=EDGE_CURVE('',#35565,#35564,#20714,.T.);
#44281=EDGE_CURVE('',#35566,#35255,#29473,.T.);
#44282=EDGE_CURVE('',#35567,#35566,#29474,.T.);
#44283=EDGE_CURVE('',#35567,#35565,#4245,.T.);
#44284=EDGE_CURVE('',#35568,#35254,#29475,.T.);
#44285=EDGE_CURVE('',#35569,#35568,#29476,.T.);
#44286=EDGE_CURVE('',#35569,#35567,#20715,.T.);
#44287=EDGE_CURVE('',#35550,#35570,#20716,.T.);
#44288=EDGE_CURVE('',#35254,#35570,#4246,.T.);
#44289=EDGE_CURVE('',#35571,#35521,#20717,.T.);
#44290=EDGE_CURVE('',#35572,#35571,#29477,.T.);
#44291=EDGE_CURVE('',#35573,#35572,#29478,.T.);
#44292=EDGE_CURVE('',#35574,#35573,#29479,.T.);
#44293=EDGE_CURVE('',#35575,#35574,#20718,.T.);
#44294=EDGE_CURVE('',#35575,#35576,#29480,.T.);
#44295=EDGE_CURVE('',#35536,#35576,#20719,.T.);
#44296=EDGE_CURVE('',#35577,#35553,#20720,.T.);
#44297=EDGE_CURVE('',#35577,#35578,#29481,.T.);
#44298=EDGE_CURVE('',#35578,#35579,#29482,.T.);
#44299=EDGE_CURVE('',#35499,#35579,#20721,.T.);
#44300=EDGE_CURVE('',#35580,#35223,#20722,.T.);
#44301=EDGE_CURVE('',#35581,#35580,#20723,.T.);
#44302=EDGE_CURVE('',#35311,#35581,#20724,.T.);
#44303=EDGE_CURVE('',#35500,#35582,#20725,.T.);
#44304=EDGE_CURVE('',#35580,#35582,#29483,.T.);
#44305=EDGE_CURVE('',#35583,#35584,#29484,.T.);
#44306=EDGE_CURVE('',#35584,#35356,#1793,.T.);
#44307=EDGE_CURVE('',#35357,#35583,#1794,.T.);
#44308=EDGE_CURVE('',#35583,#35585,#4247,.T.);
#44309=EDGE_CURVE('',#35585,#35586,#29485,.T.);
#44310=EDGE_CURVE('',#35586,#35584,#4248,.T.);
#44311=EDGE_CURVE('',#35585,#35587,#4249,.T.);
#44312=EDGE_CURVE('',#35587,#35588,#1069,.T.);
#44313=EDGE_CURVE('',#35588,#35589,#29486,.T.);
#44314=EDGE_CURVE('',#35589,#35586,#4250,.T.);
#44315=EDGE_CURVE('',#35590,#35591,#29487,.T.);
#44316=EDGE_CURVE('',#35590,#35592,#29488,.T.);
#44317=EDGE_CURVE('',#35592,#35593,#29489,.T.);
#44318=EDGE_CURVE('',#35593,#35591,#29490,.T.);
#44319=EDGE_CURVE('',#35592,#35594,#20726,.T.);
#44320=EDGE_CURVE('',#35594,#35595,#29491,.T.);
#44321=EDGE_CURVE('',#35595,#35593,#20727,.T.);
#44322=EDGE_CURVE('',#35596,#35597,#4251,.T.);
#44323=EDGE_CURVE('',#35598,#35596,#4252,.T.);
#44324=EDGE_CURVE('',#35599,#35598,#4253,.T.);
#44325=EDGE_CURVE('',#35600,#35599,#20728,.T.);
#44326=EDGE_CURVE('',#35594,#35600,#4254,.T.);
#44327=EDGE_CURVE('',#35594,#35601,#20729,.T.);
#44328=EDGE_CURVE('',#35601,#35602,#29492,.T.);
#44329=EDGE_CURVE('',#35602,#35603,#20730,.T.);
#44330=EDGE_CURVE('',#35597,#35603,#29493,.T.);
#44331=EDGE_CURVE('',#35588,#35604,#20731,.T.);
#44332=EDGE_CURVE('',#35604,#35605,#29494,.T.);
#44333=EDGE_CURVE('',#35605,#35589,#20732,.T.);
#44334=EDGE_CURVE('',#35604,#35606,#29495,.T.);
#44335=EDGE_CURVE('',#35606,#35607,#29496,.T.);
#44336=EDGE_CURVE('',#35607,#35605,#29497,.T.);
#44337=EDGE_CURVE('',#35606,#35608,#20733,.T.);
#44338=EDGE_CURVE('',#35608,#35609,#29498,.T.);
#44339=EDGE_CURVE('',#35609,#35607,#20734,.T.);
#44340=EDGE_CURVE('',#35608,#35610,#29499,.T.);
#44341=EDGE_CURVE('',#35610,#35611,#29500,.T.);
#44342=EDGE_CURVE('',#35611,#35609,#29501,.T.);
#44343=EDGE_CURVE('',#35610,#35612,#20735,.T.);
#44344=EDGE_CURVE('',#35612,#35613,#29502,.T.);
#44345=EDGE_CURVE('',#35613,#35611,#20736,.T.);
#44346=EDGE_CURVE('',#35614,#35615,#1795,.T.);
#44347=EDGE_CURVE('',#35614,#35616,#29503,.T.);
#44348=EDGE_CURVE('',#35617,#35616,#1796,.T.);
#44349=EDGE_CURVE('',#35612,#35617,#4255,.T.);
#44350=EDGE_CURVE('',#35612,#35618,#29504,.T.);
#44351=EDGE_CURVE('',#35615,#35618,#4256,.T.);
#44352=EDGE_CURVE('',#35618,#35619,#29505,.T.);
#44353=EDGE_CURVE('',#35618,#35620,#20737,.T.);
#44354=EDGE_CURVE('',#35620,#35621,#29506,.T.);
#44355=EDGE_CURVE('',#35621,#35619,#20738,.T.);
#44356=EDGE_CURVE('',#35620,#35622,#29507,.T.);
#44357=EDGE_CURVE('',#35622,#35623,#29508,.T.);
#44358=EDGE_CURVE('',#35623,#35621,#29509,.T.);
#44359=EDGE_CURVE('',#35622,#35624,#20739,.T.);
#44360=EDGE_CURVE('',#35624,#35625,#29510,.T.);
#44361=EDGE_CURVE('',#35625,#35623,#20740,.T.);
#44362=EDGE_CURVE('',#35624,#35626,#29511,.T.);
#44363=EDGE_CURVE('',#35626,#35627,#29512,.T.);
#44364=EDGE_CURVE('',#35627,#35625,#29513,.T.);
#44365=EDGE_CURVE('',#35626,#35628,#20741,.T.);
#44366=EDGE_CURVE('',#35628,#35629,#29514,.T.);
#44367=EDGE_CURVE('',#35629,#35627,#20742,.T.);
#44368=EDGE_CURVE('',#35628,#35630,#29515,.T.);
#44369=EDGE_CURVE('',#35631,#35630,#29516,.T.);
#44370=EDGE_CURVE('',#35628,#35631,#29517,.T.);
#44371=EDGE_CURVE('',#35630,#35632,#4257,.T.);
#44372=EDGE_CURVE('',#35633,#35632,#29518,.T.);
#44373=EDGE_CURVE('',#35633,#35634,#4258,.T.);
#44374=EDGE_CURVE('',#35631,#35634,#4259,.T.);
#44375=EDGE_CURVE('',#35635,#35633,#20743,.T.);
#44376=EDGE_CURVE('',#35632,#35636,#20744,.T.);
#44377=EDGE_CURVE('',#35635,#35636,#29519,.T.);
#44378=EDGE_CURVE('',#35636,#35637,#29520,.T.);
#44379=EDGE_CURVE('',#35636,#35638,#20745,.T.);
#44380=EDGE_CURVE('',#35638,#35639,#29521,.T.);
#44381=EDGE_CURVE('',#35639,#35637,#20746,.T.);
#44382=EDGE_CURVE('',#35638,#35640,#29522,.T.);
#44383=EDGE_CURVE('',#35640,#35641,#29523,.T.);
#44384=EDGE_CURVE('',#35641,#35639,#29524,.T.);
#44385=EDGE_CURVE('',#35640,#35642,#20747,.T.);
#44386=EDGE_CURVE('',#35642,#35643,#29525,.T.);
#44387=EDGE_CURVE('',#35643,#35641,#20748,.T.);
#44388=EDGE_CURVE('',#35642,#35644,#29526,.T.);
#44389=EDGE_CURVE('',#35644,#35645,#29527,.T.);
#44390=EDGE_CURVE('',#35645,#35643,#29528,.T.);
#44391=EDGE_CURVE('',#35644,#35646,#20749,.T.);
#44392=EDGE_CURVE('',#35646,#35647,#29529,.T.);
#44393=EDGE_CURVE('',#35647,#35645,#20750,.T.);
#44394=EDGE_CURVE('',#35646,#35648,#20751,.T.);
#44395=EDGE_CURVE('',#35649,#35648,#29530,.T.);
#44396=EDGE_CURVE('',#35649,#35650,#20752,.T.);
#44397=EDGE_CURVE('',#35646,#35650,#29531,.T.);
#44398=EDGE_CURVE('',#35648,#35651,#29532,.T.);
#44399=EDGE_CURVE('',#35648,#35652,#20753,.T.);
#44400=EDGE_CURVE('',#35652,#35653,#29533,.T.);
#44401=EDGE_CURVE('',#35653,#35651,#20754,.T.);
#44402=EDGE_CURVE('',#35652,#35654,#29534,.T.);
#44403=EDGE_CURVE('',#35654,#35655,#29535,.T.);
#44404=EDGE_CURVE('',#35655,#35653,#29536,.T.);
#44405=EDGE_CURVE('',#35654,#35656,#20755,.T.);
#44406=EDGE_CURVE('',#35656,#35657,#29537,.T.);
#44407=EDGE_CURVE('',#35657,#35655,#20756,.T.);
#44408=EDGE_CURVE('',#35656,#35658,#29538,.T.);
#44409=EDGE_CURVE('',#35658,#35659,#29539,.T.);
#44410=EDGE_CURVE('',#35659,#35657,#29540,.T.);
#44411=EDGE_CURVE('',#35658,#35660,#20757,.T.);
#44412=EDGE_CURVE('',#35660,#35661,#29541,.T.);
#44413=EDGE_CURVE('',#35661,#35659,#20758,.T.);
#44414=EDGE_CURVE('',#35660,#35662,#20759,.T.);
#44415=EDGE_CURVE('',#35663,#35662,#29542,.T.);
#44416=EDGE_CURVE('',#35663,#35664,#20760,.T.);
#44417=EDGE_CURVE('',#35660,#35664,#29543,.T.);
#44418=EDGE_CURVE('',#35662,#35665,#29544,.T.);
#44419=EDGE_CURVE('',#35662,#35590,#20761,.T.);
#44420=EDGE_CURVE('',#35591,#35665,#20762,.T.);
#44421=EDGE_CURVE('',#35603,#35666,#20763,.T.);
#44422=EDGE_CURVE('',#35602,#35667,#20764,.T.);
#44423=EDGE_CURVE('',#35668,#35667,#20765,.T.);
#44424=EDGE_CURVE('',#35669,#35668,#20766,.T.);
#44425=EDGE_CURVE('',#35670,#35669,#1070,.T.);
#44426=EDGE_CURVE('',#35671,#35670,#20767,.T.);
#44427=EDGE_CURVE('',#35672,#35671,#4260,.T.);
#44428=EDGE_CURVE('',#35666,#35672,#20768,.T.);
#44429=EDGE_CURVE('',#35667,#35673,#29545,.T.);
#44430=EDGE_CURVE('',#35673,#35674,#20769,.T.);
#44431=EDGE_CURVE('',#35668,#35674,#4261,.T.);
#44432=EDGE_CURVE('',#35675,#35676,#29546,.T.);
#44433=EDGE_CURVE('',#35675,#35677,#29547,.T.);
#44434=EDGE_CURVE('',#35677,#35678,#29548,.T.);
#44435=EDGE_CURVE('',#35678,#35676,#29549,.T.);
#44436=EDGE_CURVE('',#35674,#35679,#29550,.T.);
#44437=EDGE_CURVE('',#35674,#35675,#20770,.T.);
#44438=EDGE_CURVE('',#35676,#35679,#20771,.T.);
#44439=EDGE_CURVE('',#35678,#35680,#20772,.T.);
#44440=EDGE_CURVE('',#35681,#35680,#29551,.T.);
#44441=EDGE_CURVE('',#35681,#35676,#20773,.T.);
#44442=EDGE_CURVE('',#35681,#35682,#29552,.T.);
#44443=EDGE_CURVE('',#35680,#35683,#29553,.T.);
#44444=EDGE_CURVE('',#35683,#35682,#29554,.T.);
#44445=EDGE_CURVE('',#35684,#35685,#29555,.T.);
#44446=EDGE_CURVE('',#35684,#35681,#20774,.T.);
#44447=EDGE_CURVE('',#35682,#35685,#20775,.T.);
#44448=EDGE_CURVE('',#35686,#35687,#29556,.T.);
#44449=EDGE_CURVE('',#35686,#35684,#29557,.T.);
#44450=EDGE_CURVE('',#35685,#35687,#29558,.T.);
#44451=EDGE_CURVE('',#35688,#35689,#29559,.T.);
#44452=EDGE_CURVE('',#35688,#35686,#29560,.T.);
#44453=EDGE_CURVE('',#35687,#35689,#29561,.T.);
#44454=EDGE_CURVE('',#35690,#35691,#29562,.T.);
#44455=EDGE_CURVE('',#35690,#35688,#29563,.T.);
#44456=EDGE_CURVE('',#35689,#35691,#29564,.T.);
#44457=EDGE_CURVE('',#35692,#35693,#29565,.T.);
#44458=EDGE_CURVE('',#35692,#35690,#20776,.T.);
#44459=EDGE_CURVE('',#35691,#35693,#20777,.T.);
#44460=EDGE_CURVE('',#35694,#35695,#29566,.T.);
#44461=EDGE_CURVE('',#35694,#35692,#29567,.T.);
#44462=EDGE_CURVE('',#35693,#35695,#29568,.T.);
#44463=EDGE_CURVE('',#35696,#35697,#29569,.T.);
#44464=EDGE_CURVE('',#35696,#35694,#29570,.T.);
#44465=EDGE_CURVE('',#35695,#35697,#29571,.T.);
#44466=EDGE_CURVE('',#35698,#35699,#29572,.T.);
#44467=EDGE_CURVE('',#35698,#35696,#29573,.T.);
#44468=EDGE_CURVE('',#35697,#35699,#29574,.T.);
#44469=EDGE_CURVE('',#35700,#35701,#29575,.T.);
#44470=EDGE_CURVE('',#35700,#35698,#20778,.T.);
#44471=EDGE_CURVE('',#35699,#35701,#20779,.T.);
#44472=EDGE_CURVE('',#35702,#35703,#29576,.T.);
#44473=EDGE_CURVE('',#35702,#35700,#29577,.T.);
#44474=EDGE_CURVE('',#35701,#35703,#29578,.T.);
#44475=EDGE_CURVE('',#35704,#35705,#29579,.T.);
#44476=EDGE_CURVE('',#35704,#35702,#29580,.T.);
#44477=EDGE_CURVE('',#35703,#35705,#29581,.T.);
#44478=EDGE_CURVE('',#35706,#35707,#29582,.T.);
#44479=EDGE_CURVE('',#35706,#35704,#29583,.T.);
#44480=EDGE_CURVE('',#35705,#35707,#29584,.T.);
#44481=EDGE_CURVE('',#35708,#35709,#29585,.T.);
#44482=EDGE_CURVE('',#35708,#35706,#20780,.T.);
#44483=EDGE_CURVE('',#35707,#35709,#20781,.T.);
#44484=EDGE_CURVE('',#35710,#35711,#29586,.T.);
#44485=EDGE_CURVE('',#35710,#35708,#29587,.T.);
#44486=EDGE_CURVE('',#35709,#35711,#29588,.T.);
#44487=EDGE_CURVE('',#35712,#35713,#4262,.F.);
#44488=EDGE_CURVE('',#35713,#35714,#29589,.T.);
#44489=EDGE_CURVE('',#35714,#35715,#20782,.T.);
#44490=EDGE_CURVE('',#35715,#35715,#29590,.T.);
#44491=EDGE_CURVE('',#35714,#35716,#29591,.T.);
#44492=EDGE_CURVE('',#35716,#35717,#4263,.T.);
#44493=EDGE_CURVE('',#35717,#35712,#29592,.T.);
#44494=EDGE_CURVE('',#35718,#35719,#29593,.T.);
#44495=EDGE_CURVE('',#35719,#35720,#4264,.T.);
#44496=EDGE_CURVE('',#35720,#35721,#20783,.T.);
#44497=EDGE_CURVE('',#35721,#35721,#29594,.T.);
#44498=EDGE_CURVE('',#35720,#35722,#4265,.T.);
#44499=EDGE_CURVE('',#35722,#35723,#29595,.T.);
#44500=EDGE_CURVE('',#35723,#35718,#4266,.T.);
#44501=EDGE_CURVE('',#35724,#35725,#29596,.T.);
#44502=EDGE_CURVE('',#35725,#35726,#4267,.T.);
#44503=EDGE_CURVE('',#35726,#35727,#29597,.T.);
#44504=EDGE_CURVE('',#35727,#35724,#4268,.T.);
#44505=EDGE_CURVE('',#35724,#35728,#20784,.T.);
#44506=EDGE_CURVE('',#35728,#35729,#29598,.T.);
#44507=EDGE_CURVE('',#35729,#35725,#20785,.T.);
#44508=EDGE_CURVE('',#35728,#35730,#29599,.T.);
#44509=EDGE_CURVE('',#35731,#35730,#1797,.T.);
#44510=EDGE_CURVE('',#35731,#35732,#29600,.T.);
#44511=EDGE_CURVE('',#35728,#35732,#1798,.T.);
#44512=EDGE_CURVE('',#35733,#35734,#29601,.T.);
#44513=EDGE_CURVE('',#35733,#35735,#20786,.T.);
#44514=EDGE_CURVE('',#35735,#35730,#29602,.T.);
#44515=EDGE_CURVE('',#35730,#35734,#20787,.T.);
#44516=EDGE_CURVE('',#35736,#35737,#29603,.T.);
#44517=EDGE_CURVE('',#35736,#35733,#4269,.T.);
#44518=EDGE_CURVE('',#35734,#35737,#4270,.T.);
#44519=EDGE_CURVE('',#35738,#35739,#29604,.T.);
#44520=EDGE_CURVE('',#35738,#35736,#29605,.T.);
#44521=EDGE_CURVE('',#35737,#35739,#29606,.T.);
#44522=EDGE_CURVE('',#35739,#35740,#4271,.T.);
#44523=EDGE_CURVE('',#35740,#35741,#29607,.T.);
#44524=EDGE_CURVE('',#35741,#35738,#4272,.T.);
#44525=EDGE_CURVE('',#35740,#35742,#20788,.T.);
#44526=EDGE_CURVE('',#35742,#35743,#29608,.T.);
#44527=EDGE_CURVE('',#35743,#35741,#20789,.T.);
#44528=EDGE_CURVE('',#35742,#35744,#29609,.T.);
#44529=EDGE_CURVE('',#35745,#35744,#1799,.T.);
#44530=EDGE_CURVE('',#35745,#35746,#29610,.T.);
#44531=EDGE_CURVE('',#35742,#35746,#1800,.T.);
#44532=EDGE_CURVE('',#35747,#35748,#29611,.T.);
#44533=EDGE_CURVE('',#35747,#35749,#20790,.T.);
#44534=EDGE_CURVE('',#35749,#35744,#29612,.T.);
#44535=EDGE_CURVE('',#35744,#35748,#20791,.T.);
#44536=EDGE_CURVE('',#35750,#35751,#29613,.T.);
#44537=EDGE_CURVE('',#35750,#35747,#4273,.T.);
#44538=EDGE_CURVE('',#35748,#35751,#4274,.T.);
#44539=EDGE_CURVE('',#35752,#35753,#29614,.T.);
#44540=EDGE_CURVE('',#35752,#35750,#29615,.T.);
#44541=EDGE_CURVE('',#35751,#35753,#29616,.T.);
#44542=EDGE_CURVE('',#35753,#35754,#4275,.T.);
#44543=EDGE_CURVE('',#35754,#35755,#29617,.T.);
#44544=EDGE_CURVE('',#35755,#35752,#4276,.T.);
#44545=EDGE_CURVE('',#35754,#35756,#20792,.T.);
#44546=EDGE_CURVE('',#35756,#35757,#29618,.T.);
#44547=EDGE_CURVE('',#35757,#35755,#20793,.T.);
#44548=EDGE_CURVE('',#35756,#35758,#29619,.T.);
#44549=EDGE_CURVE('',#35759,#35758,#29620,.T.);
#44550=EDGE_CURVE('',#35759,#35760,#29621,.T.);
#44551=EDGE_CURVE('',#35756,#35760,#1801,.T.);
#44552=EDGE_CURVE('',#35761,#35762,#29622,.T.);
#44553=EDGE_CURVE('',#35761,#35763,#20794,.T.);
#44554=EDGE_CURVE('',#35763,#35758,#29623,.T.);
#44555=EDGE_CURVE('',#35758,#35762,#20795,.T.);
#44556=EDGE_CURVE('',#35764,#35765,#29624,.T.);
#44557=EDGE_CURVE('',#35764,#35761,#4277,.T.);
#44558=EDGE_CURVE('',#35762,#35765,#4278,.T.);
#44559=EDGE_CURVE('',#35766,#35767,#20796,.T.);
#44560=EDGE_CURVE('',#35768,#35766,#4279,.T.);
#44561=EDGE_CURVE('',#35768,#35708,#20797,.T.);
#44562=EDGE_CURVE('',#35710,#35769,#20798,.T.);
#44563=EDGE_CURVE('',#35767,#35769,#4280,.T.);
#44564=EDGE_CURVE('',#35770,#35771,#29625,.T.);
#44565=EDGE_CURVE('',#35770,#35772,#4281,.T.);
#44566=EDGE_CURVE('',#35772,#35769,#29626,.T.);
#44567=EDGE_CURVE('',#35769,#35771,#4282,.T.);
#44568=EDGE_CURVE('',#35726,#35770,#29627,.T.);
#44569=EDGE_CURVE('',#35771,#35727,#29628,.T.);
#44570=EDGE_CURVE('',#35764,#35773,#1071,.T.);
#44571=EDGE_CURVE('',#35773,#35774,#29629,.T.);
#44572=EDGE_CURVE('',#35774,#35761,#4283,.T.);
#44573=EDGE_CURVE('',#35773,#35775,#20799,.T.);
#44574=EDGE_CURVE('',#35775,#35776,#29630,.T.);
#44575=EDGE_CURVE('',#35776,#35774,#20800,.T.);
#44576=EDGE_CURVE('',#35267,#35776,#4284,.T.);
#44577=EDGE_CURVE('',#35775,#35269,#4285,.T.);
#44578=EDGE_CURVE('',#35777,#35274,#29631,.T.);
#44579=EDGE_CURVE('',#35777,#35271,#1802,.T.);
#44580=EDGE_CURVE('',#35778,#35777,#1072,.T.);
#44581=EDGE_CURVE('',#35779,#35778,#1803,.T.);
#44582=EDGE_CURVE('',#35780,#35779,#20801,.T.);
#44583=EDGE_CURVE('',#35781,#35780,#1804,.T.);
#44584=EDGE_CURVE('',#35782,#35781,#1073,.T.);
#44585=EDGE_CURVE('',#35763,#35782,#1805,.T.);
#44586=EDGE_CURVE('',#35783,#35784,#4286,.T.);
#44587=EDGE_CURVE('',#35274,#35783,#4287,.T.);
#44588=EDGE_CURVE('',#35784,#35273,#4288,.T.);
#44589=EDGE_CURVE('',#35273,#35785,#29632,.T.);
#44590=EDGE_CURVE('',#35278,#35785,#1806,.T.);
#44591=EDGE_CURVE('',#35786,#35277,#4289,.T.);
#44592=EDGE_CURVE('',#35787,#35786,#20802,.T.);
#44593=EDGE_CURVE('',#35755,#35787,#4290,.T.);
#44594=EDGE_CURVE('',#35788,#35757,#1807,.T.);
#44595=EDGE_CURVE('',#35789,#35788,#1074,.T.);
#44596=EDGE_CURVE('',#35790,#35789,#4291,.T.);
#44597=EDGE_CURVE('',#35791,#35790,#20803,.T.);
#44598=EDGE_CURVE('',#35792,#35791,#4292,.T.);
#44599=EDGE_CURVE('',#35785,#35792,#1075,.T.);
#44600=EDGE_CURVE('',#35282,#35793,#1076,.T.);
#44601=EDGE_CURVE('',#35793,#35786,#29633,.T.);
#44602=EDGE_CURVE('',#35794,#35284,#4293,.T.);
#44603=EDGE_CURVE('',#35794,#35793,#4294,.T.);
#44604=EDGE_CURVE('',#35286,#35795,#4295,.T.);
#44605=EDGE_CURVE('',#35794,#35795,#29634,.T.);
#44606=EDGE_CURVE('',#35796,#35290,#29635,.T.);
#44607=EDGE_CURVE('',#35796,#35287,#1808,.T.);
#44608=EDGE_CURVE('',#35797,#35747,#4296,.T.);
#44609=EDGE_CURVE('',#35795,#35797,#20804,.T.);
#44610=EDGE_CURVE('',#35798,#35796,#1077,.T.);
#44611=EDGE_CURVE('',#35799,#35798,#4297,.T.);
#44612=EDGE_CURVE('',#35800,#35799,#20805,.T.);
#44613=EDGE_CURVE('',#35801,#35800,#4298,.T.);
#44614=EDGE_CURVE('',#35802,#35801,#1078,.T.);
#44615=EDGE_CURVE('',#35749,#35802,#1809,.T.);
#44616=EDGE_CURVE('',#35803,#35804,#4299,.T.);
#44617=EDGE_CURVE('',#35290,#35803,#1079,.T.);
#44618=EDGE_CURVE('',#35804,#35289,#4300,.T.);
#44619=EDGE_CURVE('',#35289,#35805,#29636,.T.);
#44620=EDGE_CURVE('',#35294,#35805,#1810,.T.);
#44621=EDGE_CURVE('',#35806,#35293,#20806,.T.);
#44622=EDGE_CURVE('',#35807,#35806,#29637,.T.);
#44623=EDGE_CURVE('',#35808,#35807,#20807,.T.);
#44624=EDGE_CURVE('',#35809,#35808,#29638,.T.);
#44625=EDGE_CURVE('',#35741,#35809,#20808,.T.);
#44626=EDGE_CURVE('',#35810,#35743,#1811,.T.);
#44627=EDGE_CURVE('',#35811,#35810,#4301,.T.);
#44628=EDGE_CURVE('',#35812,#35811,#4302,.T.);
#44629=EDGE_CURVE('',#35813,#35812,#20809,.T.);
#44630=EDGE_CURVE('',#35814,#35813,#4303,.T.);
#44631=EDGE_CURVE('',#35805,#35814,#4304,.T.);
#44632=EDGE_CURVE('',#35297,#35815,#20810,.T.);
#44633=EDGE_CURVE('',#35815,#35806,#29639,.T.);
#44634=EDGE_CURVE('',#35816,#35299,#20811,.T.);
#44635=EDGE_CURVE('',#35815,#35816,#20812,.T.);
#44636=EDGE_CURVE('',#35301,#35817,#20813,.T.);
#44637=EDGE_CURVE('',#35816,#35817,#29640,.T.);
#44638=EDGE_CURVE('',#35818,#35305,#29641,.T.);
#44639=EDGE_CURVE('',#35818,#35302,#1812,.T.);
#44640=EDGE_CURVE('',#35819,#35733,#20814,.T.);
#44641=EDGE_CURVE('',#35820,#35819,#29642,.T.);
#44642=EDGE_CURVE('',#35821,#35820,#20815,.T.);
#44643=EDGE_CURVE('',#35817,#35821,#29643,.T.);
#44644=EDGE_CURVE('',#35822,#35818,#4305,.T.);
#44645=EDGE_CURVE('',#35823,#35822,#4306,.T.);
#44646=EDGE_CURVE('',#35824,#35823,#20816,.T.);
#44647=EDGE_CURVE('',#35825,#35824,#4307,.T.);
#44648=EDGE_CURVE('',#35826,#35825,#4308,.T.);
#44649=EDGE_CURVE('',#35735,#35826,#1813,.T.);
#44650=EDGE_CURVE('',#35827,#35828,#4309,.T.);
#44651=EDGE_CURVE('',#35305,#35827,#1080,.T.);
#44652=EDGE_CURVE('',#35828,#35304,#4310,.T.);
#44653=EDGE_CURVE('',#35304,#35829,#29644,.T.);
#44654=EDGE_CURVE('',#35309,#35829,#1814,.T.);
#44655=EDGE_CURVE('',#35830,#35308,#20817,.T.);
#44656=EDGE_CURVE('',#35831,#35830,#29645,.T.);
#44657=EDGE_CURVE('',#35832,#35831,#20818,.T.);
#44658=EDGE_CURVE('',#35833,#35832,#29646,.T.);
#44659=EDGE_CURVE('',#35725,#35833,#20819,.T.);
#44660=EDGE_CURVE('',#35834,#35729,#1815,.T.);
#44661=EDGE_CURVE('',#35835,#35834,#4311,.T.);
#44662=EDGE_CURVE('',#35836,#35835,#4312,.T.);
#44663=EDGE_CURVE('',#35837,#35836,#20820,.T.);
#44664=EDGE_CURVE('',#35838,#35837,#4313,.T.);
#44665=EDGE_CURVE('',#35829,#35838,#4314,.T.);
#44666=EDGE_CURVE('',#35581,#35830,#29647,.T.);
#44667=EDGE_CURVE('',#35839,#35840,#29648,.T.);
#44668=EDGE_CURVE('',#35520,#35840,#4315,.T.);
#44669=EDGE_CURVE('',#35839,#35316,#29649,.T.);
#44670=EDGE_CURVE('',#35321,#35841,#1816,.T.);
#44671=EDGE_CURVE('',#35841,#35316,#29650,.T.);
#44672=EDGE_CURVE('',#35842,#35319,#20821,.T.);
#44673=EDGE_CURVE('',#35843,#35842,#29651,.T.);
#44674=EDGE_CURVE('',#35645,#35843,#20822,.T.);
#44675=EDGE_CURVE('',#35844,#35647,#29652,.T.);
#44676=EDGE_CURVE('',#35845,#35844,#20823,.T.);
#44677=EDGE_CURVE('',#35846,#35845,#4316,.T.);
#44678=EDGE_CURVE('',#35847,#35846,#4317,.T.);
#44679=EDGE_CURVE('',#35841,#35847,#29653,.T.);
#44680=EDGE_CURVE('',#35322,#35848,#20824,.T.);
#44681=EDGE_CURVE('',#35848,#35842,#29654,.T.);
#44682=EDGE_CURVE('',#35849,#35324,#20825,.T.);
#44683=EDGE_CURVE('',#35848,#35849,#20826,.T.);
#44684=EDGE_CURVE('',#35326,#35850,#20827,.T.);
#44685=EDGE_CURVE('',#35849,#35850,#29655,.T.);
#44686=EDGE_CURVE('',#35851,#35329,#1817,.T.);
#44687=EDGE_CURVE('',#35852,#35851,#4318,.T.);
#44688=EDGE_CURVE('',#35853,#35852,#4319,.T.);
#44689=EDGE_CURVE('',#35854,#35853,#20828,.T.);
#44690=EDGE_CURVE('',#35637,#35854,#29656,.T.);
#44691=EDGE_CURVE('',#35855,#35639,#20829,.T.);
#44692=EDGE_CURVE('',#35850,#35855,#29657,.T.);
#44693=EDGE_CURVE('',#35331,#35851,#29658,.T.);
#44694=EDGE_CURVE('',#35856,#35857,#4320,.T.);
#44695=EDGE_CURVE('',#35331,#35856,#4321,.T.);
#44696=EDGE_CURVE('',#35857,#35330,#1081,.T.);
#44697=EDGE_CURVE('',#35335,#35858,#1818,.T.);
#44698=EDGE_CURVE('',#35858,#35330,#29659,.T.);
#44699=EDGE_CURVE('',#35859,#35333,#4322,.T.);
#44700=EDGE_CURVE('',#35627,#35859,#20830,.T.);
#44701=EDGE_CURVE('',#35860,#35629,#29660,.T.);
#44702=EDGE_CURVE('',#35861,#35860,#4323,.T.);
#44703=EDGE_CURVE('',#35862,#35861,#4324,.T.);
#44704=EDGE_CURVE('',#35858,#35862,#4325,.T.);
#44705=EDGE_CURVE('',#35336,#35863,#4326,.T.);
#44706=EDGE_CURVE('',#35863,#35859,#29661,.T.);
#44707=EDGE_CURVE('',#35864,#35338,#4327,.T.);
#44708=EDGE_CURVE('',#35864,#35863,#29662,.T.);
#44709=EDGE_CURVE('',#35340,#35865,#4328,.T.);
#44710=EDGE_CURVE('',#35865,#35864,#29663,.T.);
#44711=EDGE_CURVE('',#35345,#35866,#29664,.T.);
#44712=EDGE_CURVE('',#35866,#35342,#1819,.T.);
#44713=EDGE_CURVE('',#35867,#35866,#4329,.T.);
#44714=EDGE_CURVE('',#35619,#35867,#4330,.T.);
#44715=EDGE_CURVE('',#35865,#35621,#20831,.T.);
#44716=EDGE_CURVE('',#35345,#35614,#4331,.T.);
#44717=EDGE_CURVE('',#35616,#35344,#4332,.T.);
#44718=EDGE_CURVE('',#35349,#35868,#1820,.T.);
#44719=EDGE_CURVE('',#35868,#35344,#29665,.T.);
#44720=EDGE_CURVE('',#35869,#35347,#4333,.T.);
#44721=EDGE_CURVE('',#35611,#35869,#20832,.T.);
#44722=EDGE_CURVE('',#35870,#35613,#4334,.T.);
#44723=EDGE_CURVE('',#35868,#35870,#1082,.T.);
#44724=EDGE_CURVE('',#35350,#35871,#1083,.T.);
#44725=EDGE_CURVE('',#35871,#35869,#29666,.T.);
#44726=EDGE_CURVE('',#35872,#35352,#4335,.T.);
#44727=EDGE_CURVE('',#35872,#35871,#4336,.T.);
#44728=EDGE_CURVE('',#35354,#35873,#4337,.T.);
#44729=EDGE_CURVE('',#35873,#35872,#29667,.T.);
#44730=EDGE_CURVE('',#35873,#35605,#20833,.T.);
#44731=EDGE_CURVE('',#35402,#35874,#20834,.T.);
#44732=EDGE_CURVE('',#35874,#35875,#29668,.T.);
#44733=EDGE_CURVE('',#35875,#35489,#20835,.T.);
#44734=EDGE_CURVE('',#35876,#35404,#20836,.T.);
#44735=EDGE_CURVE('',#35874,#35876,#20837,.T.);
#44736=EDGE_CURVE('',#35537,#35877,#20838,.T.);
#44737=EDGE_CURVE('',#35876,#35877,#29669,.T.);
#44738=EDGE_CURVE('',#35359,#35878,#20839,.T.);
#44739=EDGE_CURVE('',#35878,#35879,#29670,.T.);
#44740=EDGE_CURVE('',#35879,#35551,#20840,.T.);
#44741=EDGE_CURVE('',#35880,#35360,#20841,.T.);
#44742=EDGE_CURVE('',#35878,#35880,#20842,.T.);
#44743=EDGE_CURVE('',#35445,#35881,#20843,.T.);
#44744=EDGE_CURVE('',#35880,#35881,#29671,.T.);
#44745=EDGE_CURVE('',#35882,#35883,#20844,.T.);
#44746=EDGE_CURVE('',#35884,#35882,#29672,.T.);
#44747=EDGE_CURVE('',#35885,#35884,#20845,.T.);
#44748=EDGE_CURVE('',#35881,#35885,#29673,.T.);
#44749=EDGE_CURVE('',#35886,#35446,#1821,.T.);
#44750=EDGE_CURVE('',#35887,#35886,#4338,.T.);
#44751=EDGE_CURVE('',#35888,#35887,#4339,.T.);
#44752=EDGE_CURVE('',#35889,#35888,#20846,.T.);
#44753=EDGE_CURVE('',#35890,#35889,#4340,.T.);
#44754=EDGE_CURVE('',#35891,#35890,#4341,.T.);
#44755=EDGE_CURVE('',#35892,#35891,#1822,.T.);
#44756=EDGE_CURVE('',#35883,#35892,#20847,.T.);
#44757=EDGE_CURVE('',#35448,#35886,#29674,.T.);
#44758=EDGE_CURVE('',#35893,#35894,#4342,.T.);
#44759=EDGE_CURVE('',#35448,#35893,#1084,.T.);
#44760=EDGE_CURVE('',#35894,#35447,#4343,.T.);
#44761=EDGE_CURVE('',#35450,#35895,#1823,.T.);
#44762=EDGE_CURVE('',#35895,#35447,#29675,.T.);
#44763=EDGE_CURVE('',#35896,#35449,#20848,.T.);
#44764=EDGE_CURVE('',#35897,#35896,#29676,.T.);
#44765=EDGE_CURVE('',#35898,#35897,#20849,.T.);
#44766=EDGE_CURVE('',#35899,#35898,#29677,.T.);
#44767=EDGE_CURVE('',#35900,#35899,#20850,.T.);
#44768=EDGE_CURVE('',#35901,#35900,#20851,.T.);
#44769=EDGE_CURVE('',#35902,#35901,#1824,.T.);
#44770=EDGE_CURVE('',#35903,#35902,#4344,.T.);
#44771=EDGE_CURVE('',#35904,#35903,#4345,.T.);
#44772=EDGE_CURVE('',#35905,#35904,#20852,.T.);
#44773=EDGE_CURVE('',#35906,#35905,#4346,.T.);
#44774=EDGE_CURVE('',#35895,#35906,#4347,.T.);
#44775=EDGE_CURVE('',#35451,#35907,#20853,.T.);
#44776=EDGE_CURVE('',#35907,#35896,#29678,.T.);
#44777=EDGE_CURVE('',#35908,#35452,#20854,.T.);
#44778=EDGE_CURVE('',#35907,#35908,#20855,.T.);
#44779=EDGE_CURVE('',#35453,#35909,#20856,.T.);
#44780=EDGE_CURVE('',#35908,#35909,#29679,.T.);
#44781=EDGE_CURVE('',#35910,#35456,#29680,.T.);
#44782=EDGE_CURVE('',#35910,#35454,#1825,.T.);
#44783=EDGE_CURVE('',#35911,#35910,#4348,.T.);
#44784=EDGE_CURVE('',#35912,#35911,#4349,.T.);
#44785=EDGE_CURVE('',#35913,#35912,#20857,.T.);
#44786=EDGE_CURVE('',#35914,#35913,#4350,.T.);
#44787=EDGE_CURVE('',#35915,#35914,#4351,.T.);
#44788=EDGE_CURVE('',#35916,#35915,#1826,.T.);
#44789=EDGE_CURVE('',#35917,#35916,#20858,.T.);
#44790=EDGE_CURVE('',#35918,#35917,#29681,.T.);
#44791=EDGE_CURVE('',#35919,#35918,#20859,.T.);
#44792=EDGE_CURVE('',#35909,#35919,#29682,.T.);
#44793=EDGE_CURVE('',#35920,#35921,#4352,.T.);
#44794=EDGE_CURVE('',#35456,#35920,#4353,.T.);
#44795=EDGE_CURVE('',#35921,#35455,#1085,.T.);
#44796=EDGE_CURVE('',#35455,#35922,#29683,.T.);
#44797=EDGE_CURVE('',#35457,#35922,#1827,.T.);
#44798=EDGE_CURVE('',#35923,#35458,#4354,.T.);
#44799=EDGE_CURVE('',#35924,#35923,#20860,.T.);
#44800=EDGE_CURVE('',#35925,#35924,#4355,.T.);
#44801=EDGE_CURVE('',#35926,#35925,#20861,.T.);
#44802=EDGE_CURVE('',#35927,#35926,#1828,.T.);
#44803=EDGE_CURVE('',#35928,#35927,#4356,.T.);
#44804=EDGE_CURVE('',#35929,#35928,#4357,.T.);
#44805=EDGE_CURVE('',#35930,#35929,#20862,.T.);
#44806=EDGE_CURVE('',#35931,#35930,#4358,.T.);
#44807=EDGE_CURVE('',#35922,#35931,#4359,.T.);
#44808=EDGE_CURVE('',#35459,#35932,#4360,.T.);
#44809=EDGE_CURVE('',#35932,#35923,#29684,.T.);
#44810=EDGE_CURVE('',#35933,#35460,#4361,.T.);
#44811=EDGE_CURVE('',#35933,#35932,#4362,.T.);
#44812=EDGE_CURVE('',#35461,#35934,#4363,.T.);
#44813=EDGE_CURVE('',#35933,#35934,#29685,.T.);
#44814=EDGE_CURVE('',#35935,#35464,#29686,.T.);
#44815=EDGE_CURVE('',#35935,#35462,#1829,.T.);
#44816=EDGE_CURVE('',#35936,#35937,#4364,.T.);
#44817=EDGE_CURVE('',#35934,#35936,#20863,.T.);
#44818=EDGE_CURVE('',#35938,#35935,#1086,.T.);
#44819=EDGE_CURVE('',#35939,#35938,#4365,.T.);
#44820=EDGE_CURVE('',#35940,#35939,#20864,.T.);
#44821=EDGE_CURVE('',#35941,#35940,#4366,.T.);
#44822=EDGE_CURVE('',#35942,#35941,#1087,.T.);
#44823=EDGE_CURVE('',#35943,#35942,#1830,.T.);
#44824=EDGE_CURVE('',#35937,#35943,#20865,.T.);
#44825=EDGE_CURVE('',#35944,#35945,#4367,.T.);
#44826=EDGE_CURVE('',#35464,#35944,#1088,.T.);
#44827=EDGE_CURVE('',#35945,#35463,#4368,.T.);
#44828=EDGE_CURVE('',#35463,#35946,#29687,.T.);
#44829=EDGE_CURVE('',#35465,#35946,#1831,.T.);
#44830=EDGE_CURVE('',#35947,#35466,#4369,.T.);
#44831=EDGE_CURVE('',#35948,#35947,#20866,.T.);
#44832=EDGE_CURVE('',#35949,#35948,#4370,.T.);
#44833=EDGE_CURVE('',#35950,#35949,#20867,.T.);
#44834=EDGE_CURVE('',#35951,#35950,#1832,.T.);
#44835=EDGE_CURVE('',#35952,#35951,#1089,.T.);
#44836=EDGE_CURVE('',#35953,#35952,#1833,.T.);
#44837=EDGE_CURVE('',#35954,#35953,#20868,.T.);
#44838=EDGE_CURVE('',#35955,#35954,#1834,.T.);
#44839=EDGE_CURVE('',#35946,#35955,#1090,.T.);
#44840=EDGE_CURVE('',#35467,#35956,#1091,.T.);
#44841=EDGE_CURVE('',#35956,#35947,#29688,.T.);
#44842=EDGE_CURVE('',#35957,#35468,#1092,.T.);
#44843=EDGE_CURVE('',#35957,#35956,#29689,.T.);
#44844=EDGE_CURVE('',#35469,#35958,#4371,.T.);
#44845=EDGE_CURVE('',#35958,#35957,#29690,.T.);
#44846=EDGE_CURVE('',#35959,#35472,#29691,.T.);
#44847=EDGE_CURVE('',#35959,#35470,#1835,.T.);
#44848=EDGE_CURVE('',#35960,#35959,#1093,.T.);
#44849=EDGE_CURVE('',#35961,#35960,#1836,.T.);
#44850=EDGE_CURVE('',#35962,#35961,#20869,.T.);
#44851=EDGE_CURVE('',#35963,#35962,#1837,.T.);
#44852=EDGE_CURVE('',#35964,#35963,#4372,.T.);
#44853=EDGE_CURVE('',#35965,#35964,#1838,.T.);
#44854=EDGE_CURVE('',#35966,#35965,#20870,.T.);
#44855=EDGE_CURVE('',#35967,#35966,#4373,.T.);
#44856=EDGE_CURVE('',#35958,#35967,#20871,.T.);
#44857=EDGE_CURVE('',#35968,#35969,#1094,.T.);
#44858=EDGE_CURVE('',#35472,#35968,#4374,.T.);
#44859=EDGE_CURVE('',#35969,#35471,#1095,.T.);
#44860=EDGE_CURVE('',#35471,#35970,#29692,.T.);
#44861=EDGE_CURVE('',#35473,#35970,#1839,.T.);
#44862=EDGE_CURVE('',#35971,#35474,#4375,.T.);
#44863=EDGE_CURVE('',#35972,#35971,#20872,.T.);
#44864=EDGE_CURVE('',#35973,#35972,#4376,.T.);
#44865=EDGE_CURVE('',#35974,#35973,#20873,.T.);
#44866=EDGE_CURVE('',#35975,#35974,#1840,.T.);
#44867=EDGE_CURVE('',#35976,#35975,#1096,.T.);
#44868=EDGE_CURVE('',#35977,#35976,#4377,.T.);
#44869=EDGE_CURVE('',#35978,#35977,#20874,.T.);
#44870=EDGE_CURVE('',#35979,#35978,#4378,.T.);
#44871=EDGE_CURVE('',#35970,#35979,#1097,.T.);
#44872=EDGE_CURVE('',#35475,#35980,#1098,.T.);
#44873=EDGE_CURVE('',#35980,#35971,#29693,.T.);
#44874=EDGE_CURVE('',#35981,#35476,#4379,.T.);
#44875=EDGE_CURVE('',#35981,#35980,#4380,.T.);
#44876=EDGE_CURVE('',#35477,#35982,#4381,.T.);
#44877=EDGE_CURVE('',#35982,#35981,#29694,.T.);
#44878=EDGE_CURVE('',#35983,#35480,#29695,.T.);
#44879=EDGE_CURVE('',#35983,#35478,#1841,.T.);
#44880=EDGE_CURVE('',#35984,#35983,#4382,.T.);
#44881=EDGE_CURVE('',#35985,#35984,#4383,.T.);
#44882=EDGE_CURVE('',#35986,#35985,#20875,.T.);
#44883=EDGE_CURVE('',#35987,#35986,#4384,.T.);
#44884=EDGE_CURVE('',#35988,#35987,#4385,.T.);
#44885=EDGE_CURVE('',#35989,#35988,#1842,.T.);
#44886=EDGE_CURVE('',#35990,#35989,#20876,.T.);
#44887=EDGE_CURVE('',#35991,#35990,#4386,.T.);
#44888=EDGE_CURVE('',#35982,#35991,#20877,.T.);
#44889=EDGE_CURVE('',#35992,#35993,#4387,.T.);
#44890=EDGE_CURVE('',#35480,#35992,#1099,.T.);
#44891=EDGE_CURVE('',#35993,#35479,#4388,.T.);
#44892=EDGE_CURVE('',#35482,#35994,#1843,.T.);
#44893=EDGE_CURVE('',#35994,#35479,#29696,.T.);
#44894=EDGE_CURVE('',#35995,#35481,#20878,.T.);
#44895=EDGE_CURVE('',#35996,#35995,#29697,.T.);
#44896=EDGE_CURVE('',#35997,#35996,#20879,.T.);
#44897=EDGE_CURVE('',#35998,#35997,#29698,.T.);
#44898=EDGE_CURVE('',#35999,#35998,#20880,.T.);
#44899=EDGE_CURVE('',#36000,#35999,#1844,.T.);
#44900=EDGE_CURVE('',#36001,#36000,#4389,.T.);
#44901=EDGE_CURVE('',#36002,#36001,#4390,.T.);
#44902=EDGE_CURVE('',#36003,#36002,#20881,.T.);
#44903=EDGE_CURVE('',#36004,#36003,#4391,.T.);
#44904=EDGE_CURVE('',#35994,#36004,#4392,.T.);
#44905=EDGE_CURVE('',#35483,#36005,#20882,.T.);
#44906=EDGE_CURVE('',#36005,#35995,#29699,.T.);
#44907=EDGE_CURVE('',#36006,#35484,#20883,.T.);
#44908=EDGE_CURVE('',#36005,#36006,#20884,.T.);
#44909=EDGE_CURVE('',#35485,#36007,#20885,.T.);
#44910=EDGE_CURVE('',#36006,#36007,#29700,.T.);
#44911=EDGE_CURVE('',#36008,#35488,#29701,.T.);
#44912=EDGE_CURVE('',#36008,#35486,#1845,.T.);
#44913=EDGE_CURVE('',#36009,#36008,#4393,.T.);
#44914=EDGE_CURVE('',#36010,#36009,#4394,.T.);
#44915=EDGE_CURVE('',#36011,#36010,#20886,.T.);
#44916=EDGE_CURVE('',#36012,#36011,#4395,.T.);
#44917=EDGE_CURVE('',#36013,#36012,#4396,.T.);
#44918=EDGE_CURVE('',#36014,#36013,#1846,.T.);
#44919=EDGE_CURVE('',#36015,#36014,#20887,.T.);
#44920=EDGE_CURVE('',#36016,#36015,#20888,.T.);
#44921=EDGE_CURVE('',#36017,#36016,#29702,.T.);
#44922=EDGE_CURVE('',#36018,#36017,#20889,.T.);
#44923=EDGE_CURVE('',#36007,#36018,#29703,.T.);
#44924=EDGE_CURVE('',#36019,#36020,#4397,.T.);
#44925=EDGE_CURVE('',#35488,#36019,#1100,.T.);
#44926=EDGE_CURVE('',#36020,#35487,#1101,.T.);
#44927=EDGE_CURVE('',#35490,#36021,#1847,.T.);
#44928=EDGE_CURVE('',#36021,#35487,#29704,.T.);
#44929=EDGE_CURVE('',#36022,#36023,#1848,.T.);
#44930=EDGE_CURVE('',#36024,#36022,#4398,.T.);
#44931=EDGE_CURVE('',#36025,#36024,#4399,.T.);
#44932=EDGE_CURVE('',#36026,#36025,#20890,.T.);
#44933=EDGE_CURVE('',#36027,#36026,#4400,.T.);
#44934=EDGE_CURVE('',#36021,#36027,#4401,.T.);
#44935=EDGE_CURVE('',#36028,#35875,#29705,.T.);
#44936=EDGE_CURVE('',#36029,#36028,#20891,.T.);
#44937=EDGE_CURVE('',#36030,#36029,#29706,.T.);
#44938=EDGE_CURVE('',#36031,#36030,#20892,.T.);
#44939=EDGE_CURVE('',#36023,#36031,#20893,.T.);
#44940=EDGE_CURVE('',#36032,#36033,#4402,.T.);
#44941=EDGE_CURVE('',#36034,#36032,#29707,.T.);
#44942=EDGE_CURVE('',#35492,#36034,#20894,.T.);
#44943=EDGE_CURVE('',#36033,#35491,#20895,.T.);
#44944=EDGE_CURVE('',#35491,#36035,#29708,.T.);
#44945=EDGE_CURVE('',#35493,#36035,#1102,.T.);
#44946=EDGE_CURVE('',#36036,#35492,#29709,.T.);
#44947=EDGE_CURVE('',#36036,#35510,#1103,.T.);
#44948=EDGE_CURVE('',#36037,#36038,#1104,.T.);
#44949=EDGE_CURVE('',#36039,#36037,#20896,.T.);
#44950=EDGE_CURVE('',#36040,#36039,#4403,.T.);
#44951=EDGE_CURVE('',#36041,#36040,#4404,.T.);
#44952=EDGE_CURVE('',#36042,#36041,#4405,.T.);
#44953=EDGE_CURVE('',#36043,#36042,#20897,.T.);
#44954=EDGE_CURVE('',#36044,#36043,#4406,.T.);
#44955=EDGE_CURVE('',#36045,#36044,#4407,.T.);
#44956=EDGE_CURVE('',#36035,#36045,#20898,.T.);
#44957=EDGE_CURVE('',#36046,#35494,#20899,.T.);
#44958=EDGE_CURVE('',#36047,#36046,#29710,.T.);
#44959=EDGE_CURVE('',#36048,#36047,#20900,.T.);
#44960=EDGE_CURVE('',#36049,#36048,#29711,.T.);
#44961=EDGE_CURVE('',#36050,#36049,#20901,.T.);
#44962=EDGE_CURVE('',#36038,#36050,#20902,.T.);
#44963=EDGE_CURVE('',#35495,#36051,#20903,.T.);
#44964=EDGE_CURVE('',#36051,#36046,#29712,.T.);
#44965=EDGE_CURVE('',#36052,#35496,#20904,.T.);
#44966=EDGE_CURVE('',#36051,#36052,#20905,.T.);
#44967=EDGE_CURVE('',#35497,#36053,#20906,.T.);
#44968=EDGE_CURVE('',#36053,#36052,#29713,.T.);
#44969=EDGE_CURVE('',#36054,#36055,#4408,.T.);
#44970=EDGE_CURVE('',#36056,#36054,#20907,.T.);
#44971=EDGE_CURVE('',#36057,#36056,#1105,.T.);
#44972=EDGE_CURVE('',#36058,#36057,#20908,.T.);
#44973=EDGE_CURVE('',#36059,#36058,#20909,.T.);
#44974=EDGE_CURVE('',#36060,#36059,#29714,.T.);
#44975=EDGE_CURVE('',#36061,#36060,#20910,.T.);
#44976=EDGE_CURVE('',#36053,#36061,#29715,.T.);
#44977=EDGE_CURVE('',#36062,#35498,#1106,.T.);
#44978=EDGE_CURVE('',#36063,#36062,#20911,.T.);
#44979=EDGE_CURVE('',#36064,#36063,#4409,.T.);
#44980=EDGE_CURVE('',#36065,#36064,#20912,.T.);
#44981=EDGE_CURVE('',#36066,#36065,#20913,.T.);
#44982=EDGE_CURVE('',#36055,#36066,#20914,.T.);
#44983=EDGE_CURVE('',#35499,#36062,#29716,.T.);
#44984=EDGE_CURVE('',#36067,#35503,#29717,.T.);
#44985=EDGE_CURVE('',#36067,#35501,#4410,.T.);
#44986=EDGE_CURVE('',#36068,#36069,#20915,.T.);
#44987=EDGE_CURVE('',#36070,#36068,#29718,.T.);
#44988=EDGE_CURVE('',#36071,#36070,#20916,.T.);
#44989=EDGE_CURVE('',#35582,#36071,#29719,.T.);
#44990=EDGE_CURVE('',#36072,#36067,#1849,.T.);
#44991=EDGE_CURVE('',#36073,#36072,#4411,.T.);
#44992=EDGE_CURVE('',#36074,#36073,#4412,.T.);
#44993=EDGE_CURVE('',#36075,#36074,#20917,.T.);
#44994=EDGE_CURVE('',#36076,#36075,#4413,.T.);
#44995=EDGE_CURVE('',#36077,#36076,#4414,.T.);
#44996=EDGE_CURVE('',#36078,#36077,#4415,.T.);
#44997=EDGE_CURVE('',#36079,#36078,#4416,.T.);
#44998=EDGE_CURVE('',#36069,#36079,#20918,.T.);
#44999=EDGE_CURVE('',#36080,#36081,#29720,.T.);
#45000=EDGE_CURVE('',#35503,#36081,#1850,.T.);
#45001=EDGE_CURVE('',#35502,#36082,#29721,.T.);
#45002=EDGE_CURVE('',#36080,#36082,#4417,.T.);
#45003=EDGE_CURVE('',#36082,#35504,#20919,.T.);
#45004=EDGE_CURVE('',#35504,#36083,#29722,.T.);
#45005=EDGE_CURVE('',#35505,#36083,#1107,.T.);
#45006=EDGE_CURVE('',#36084,#35506,#20920,.T.);
#45007=EDGE_CURVE('',#36085,#36084,#29723,.T.);
#45008=EDGE_CURVE('',#36086,#36085,#20921,.T.);
#45009=EDGE_CURVE('',#36087,#36086,#29724,.T.);
#45010=EDGE_CURVE('',#36088,#36087,#20922,.T.);
#45011=EDGE_CURVE('',#36089,#36088,#20923,.T.);
#45012=EDGE_CURVE('',#36090,#36089,#1108,.T.);
#45013=EDGE_CURVE('',#36091,#36090,#20924,.T.);
#45014=EDGE_CURVE('',#36092,#36091,#4418,.T.);
#45015=EDGE_CURVE('',#36093,#36092,#4419,.T.);
#45016=EDGE_CURVE('',#36094,#36093,#4420,.T.);
#45017=EDGE_CURVE('',#36095,#36094,#20925,.T.);
#45018=EDGE_CURVE('',#36096,#36095,#4421,.T.);
#45019=EDGE_CURVE('',#36097,#36096,#4422,.T.);
#45020=EDGE_CURVE('',#36098,#36097,#4423,.T.);
#45021=EDGE_CURVE('',#36083,#36098,#20926,.T.);
#45022=EDGE_CURVE('',#35507,#36099,#20927,.T.);
#45023=EDGE_CURVE('',#36099,#36084,#29725,.T.);
#45024=EDGE_CURVE('',#36100,#35508,#20928,.T.);
#45025=EDGE_CURVE('',#36099,#36100,#20929,.T.);
#45026=EDGE_CURVE('',#35509,#36101,#20930,.T.);
#45027=EDGE_CURVE('',#36100,#36101,#29726,.T.);
#45028=EDGE_CURVE('',#36102,#36103,#20931,.T.);
#45029=EDGE_CURVE('',#36104,#36102,#29727,.T.);
#45030=EDGE_CURVE('',#36105,#36104,#20932,.T.);
#45031=EDGE_CURVE('',#36101,#36105,#29728,.T.);
#45032=EDGE_CURVE('',#36106,#36036,#20933,.T.);
#45033=EDGE_CURVE('',#36107,#36106,#4424,.T.);
#45034=EDGE_CURVE('',#36108,#36107,#4425,.T.);
#45035=EDGE_CURVE('',#36109,#36108,#4426,.T.);
#45036=EDGE_CURVE('',#36110,#36109,#20934,.T.);
#45037=EDGE_CURVE('',#36111,#36110,#4427,.T.);
#45038=EDGE_CURVE('',#36112,#36111,#4428,.T.);
#45039=EDGE_CURVE('',#36113,#36112,#4429,.T.);
#45040=EDGE_CURVE('',#36114,#36113,#20935,.T.);
#45041=EDGE_CURVE('',#36115,#36114,#1109,.T.);
#45042=EDGE_CURVE('',#36103,#36115,#20936,.T.);
#45043=EDGE_CURVE('',#36116,#36117,#29729,.T.);
#45044=EDGE_CURVE('',#35513,#36116,#20937,.T.);
#45045=EDGE_CURVE('',#36117,#35512,#20938,.T.);
#45046=EDGE_CURVE('',#35515,#36118,#1110,.T.);
#45047=EDGE_CURVE('',#36118,#35512,#29730,.T.);
#45048=EDGE_CURVE('',#35513,#36119,#29731,.T.);
#45049=EDGE_CURVE('',#36119,#35527,#1111,.T.);
#45050=EDGE_CURVE('',#36120,#35514,#20939,.T.);
#45051=EDGE_CURVE('',#36121,#36120,#29732,.T.);
#45052=EDGE_CURVE('',#35659,#36121,#20940,.T.);
#45053=EDGE_CURVE('',#36122,#35661,#29733,.T.);
#45054=EDGE_CURVE('',#36123,#36122,#20941,.T.);
#45055=EDGE_CURVE('',#36124,#36123,#4430,.T.);
#45056=EDGE_CURVE('',#36125,#36124,#4431,.T.);
#45057=EDGE_CURVE('',#36126,#36125,#4432,.T.);
#45058=EDGE_CURVE('',#36118,#36126,#20942,.T.);
#45059=EDGE_CURVE('',#35516,#36127,#20943,.T.);
#45060=EDGE_CURVE('',#36127,#36120,#29734,.T.);
#45061=EDGE_CURVE('',#36128,#35517,#20944,.T.);
#45062=EDGE_CURVE('',#36127,#36128,#20945,.T.);
#45063=EDGE_CURVE('',#35518,#36129,#20946,.T.);
#45064=EDGE_CURVE('',#36128,#36129,#29735,.T.);
#45065=EDGE_CURVE('',#36130,#35519,#4433,.T.);
#45066=EDGE_CURVE('',#36131,#36130,#4434,.T.);
#45067=EDGE_CURVE('',#36132,#36131,#4435,.T.);
#45068=EDGE_CURVE('',#36133,#36132,#4436,.T.);
#45069=EDGE_CURVE('',#36134,#36133,#20947,.T.);
#45070=EDGE_CURVE('',#35651,#36134,#29736,.T.);
#45071=EDGE_CURVE('',#36135,#35653,#20948,.T.);
#45072=EDGE_CURVE('',#36129,#36135,#29737,.T.);
#45073=EDGE_CURVE('',#35520,#36130,#29738,.T.);
#45074=EDGE_CURVE('',#35521,#36136,#29739,.T.);
#45075=EDGE_CURVE('',#35522,#36136,#4437,.T.);
#45076=EDGE_CURVE('',#36137,#36138,#20949,.T.);
#45077=EDGE_CURVE('',#36136,#36137,#20950,.T.);
#45078=EDGE_CURVE('',#36139,#35523,#20951,.T.);
#45079=EDGE_CURVE('',#36140,#36139,#29740,.T.);
#45080=EDGE_CURVE('',#36141,#36140,#20952,.T.);
#45081=EDGE_CURVE('',#36138,#36141,#20953,.T.);
#45082=EDGE_CURVE('',#35524,#36142,#20954,.T.);
#45083=EDGE_CURVE('',#36142,#36139,#29741,.T.);
#45084=EDGE_CURVE('',#36143,#35525,#20955,.T.);
#45085=EDGE_CURVE('',#36142,#36143,#20956,.T.);
#45086=EDGE_CURVE('',#35526,#36144,#20957,.T.);
#45087=EDGE_CURVE('',#36143,#36144,#29742,.T.);
#45088=EDGE_CURVE('',#36145,#35591,#20958,.T.);
#45089=EDGE_CURVE('',#36144,#36145,#29743,.T.);
#45090=EDGE_CURVE('',#36146,#36119,#20959,.T.);
#45091=EDGE_CURVE('',#36147,#36146,#4438,.T.);
#45092=EDGE_CURVE('',#36148,#36147,#1112,.T.);
#45093=EDGE_CURVE('',#36149,#36148,#4439,.T.);
#45094=EDGE_CURVE('',#36150,#36149,#20960,.T.);
#45095=EDGE_CURVE('',#35665,#36150,#29744,.T.);
#45096=EDGE_CURVE('',#36151,#36152,#29745,.T.);
#45097=EDGE_CURVE('',#35529,#36151,#20961,.T.);
#45098=EDGE_CURVE('',#36152,#35528,#20962,.T.);
#45099=EDGE_CURVE('',#35531,#36153,#1113,.T.);
#45100=EDGE_CURVE('',#36153,#35528,#29746,.T.);
#45101=EDGE_CURVE('',#36154,#35529,#29747,.T.);
#45102=EDGE_CURVE('',#36154,#35548,#1114,.T.);
#45103=EDGE_CURVE('',#36155,#36156,#1115,.T.);
#45104=EDGE_CURVE('',#36157,#36155,#20963,.T.);
#45105=EDGE_CURVE('',#36158,#36157,#4440,.T.);
#45106=EDGE_CURVE('',#36159,#36158,#1116,.T.);
#45107=EDGE_CURVE('',#36160,#36159,#4441,.T.);
#45108=EDGE_CURVE('',#36161,#36160,#20964,.T.);
#45109=EDGE_CURVE('',#36162,#36161,#4442,.T.);
#45110=EDGE_CURVE('',#36163,#36162,#1117,.T.);
#45111=EDGE_CURVE('',#36164,#36163,#4443,.T.);
#45112=EDGE_CURVE('',#36153,#36164,#20965,.T.);
#45113=EDGE_CURVE('',#36165,#35530,#20966,.T.);
#45114=EDGE_CURVE('',#36166,#36165,#29748,.T.);
#45115=EDGE_CURVE('',#36167,#36166,#20967,.T.);
#45116=EDGE_CURVE('',#36168,#36167,#29749,.T.);
#45117=EDGE_CURVE('',#36169,#36168,#20968,.T.);
#45118=EDGE_CURVE('',#36156,#36169,#20969,.T.);
#45119=EDGE_CURVE('',#35532,#36170,#20970,.T.);
#45120=EDGE_CURVE('',#36170,#36165,#29750,.T.);
#45121=EDGE_CURVE('',#36171,#35533,#20971,.T.);
#45122=EDGE_CURVE('',#36170,#36171,#20972,.T.);
#45123=EDGE_CURVE('',#35534,#36172,#20973,.T.);
#45124=EDGE_CURVE('',#36171,#36172,#29751,.T.);
#45125=EDGE_CURVE('',#36173,#35536,#29752,.T.);
#45126=EDGE_CURVE('',#36173,#35535,#1118,.T.);
#45127=EDGE_CURVE('',#36174,#36175,#20974,.T.);
#45128=EDGE_CURVE('',#36176,#36174,#20975,.T.);
#45129=EDGE_CURVE('',#36177,#36176,#4444,.T.);
#45130=EDGE_CURVE('',#36178,#36177,#20976,.T.);
#45131=EDGE_CURVE('',#36179,#36178,#1119,.T.);
#45132=EDGE_CURVE('',#36180,#36179,#20977,.T.);
#45133=EDGE_CURVE('',#36181,#36180,#20978,.T.);
#45134=EDGE_CURVE('',#36182,#36181,#29753,.T.);
#45135=EDGE_CURVE('',#36183,#36182,#20979,.T.);
#45136=EDGE_CURVE('',#36172,#36183,#29754,.T.);
#45137=EDGE_CURVE('',#36184,#36173,#20980,.T.);
#45138=EDGE_CURVE('',#36185,#36184,#4445,.T.);
#45139=EDGE_CURVE('',#36186,#36185,#20981,.T.);
#45140=EDGE_CURVE('',#36187,#36186,#20982,.T.);
#45141=EDGE_CURVE('',#36175,#36187,#29755,.T.);
#45142=EDGE_CURVE('',#36188,#36189,#20983,.T.);
#45143=EDGE_CURVE('',#36190,#36188,#29756,.T.);
#45144=EDGE_CURVE('',#36191,#36190,#20984,.T.);
#45145=EDGE_CURVE('',#35877,#36191,#29757,.T.);
#45146=EDGE_CURVE('',#36192,#35538,#1851,.T.);
#45147=EDGE_CURVE('',#36193,#36192,#1852,.T.);
#45148=EDGE_CURVE('',#36194,#36193,#1853,.T.);
#45149=EDGE_CURVE('',#36195,#36194,#4446,.T.);
#45150=EDGE_CURVE('',#36196,#36195,#4447,.T.);
#45151=EDGE_CURVE('',#36197,#36196,#20985,.T.);
#45152=EDGE_CURVE('',#36198,#36197,#4448,.T.);
#45153=EDGE_CURVE('',#36199,#36198,#4449,.T.);
#45154=EDGE_CURVE('',#36200,#36199,#4450,.T.);
#45155=EDGE_CURVE('',#36201,#36200,#4451,.T.);
#45156=EDGE_CURVE('',#36189,#36201,#20986,.T.);
#45157=EDGE_CURVE('',#35541,#36192,#29758,.T.);
#45158=EDGE_CURVE('',#35540,#36202,#4452,.T.);
#45159=EDGE_CURVE('',#35541,#36202,#4453,.T.);
#45160=EDGE_CURVE('',#36203,#36204,#29759,.T.);
#45161=EDGE_CURVE('',#36202,#36204,#1854,.T.);
#45162=EDGE_CURVE('',#35539,#36205,#29760,.T.);
#45163=EDGE_CURVE('',#36203,#36205,#4454,.T.);
#45164=EDGE_CURVE('',#36205,#35542,#20987,.T.);
#45165=EDGE_CURVE('',#35542,#36206,#29761,.T.);
#45166=EDGE_CURVE('',#35543,#36206,#1120,.T.);
#45167=EDGE_CURVE('',#36207,#35544,#20988,.T.);
#45168=EDGE_CURVE('',#36208,#36207,#29762,.T.);
#45169=EDGE_CURVE('',#36209,#36208,#20989,.T.);
#45170=EDGE_CURVE('',#36210,#36209,#29763,.T.);
#45171=EDGE_CURVE('',#36211,#36210,#20990,.T.);
#45172=EDGE_CURVE('',#36212,#36211,#20991,.T.);
#45173=EDGE_CURVE('',#36213,#36212,#1121,.T.);
#45174=EDGE_CURVE('',#36214,#36213,#20992,.T.);
#45175=EDGE_CURVE('',#36215,#36214,#4455,.T.);
#45176=EDGE_CURVE('',#36216,#36215,#4456,.T.);
#45177=EDGE_CURVE('',#36217,#36216,#4457,.T.);
#45178=EDGE_CURVE('',#36218,#36217,#20993,.T.);
#45179=EDGE_CURVE('',#36219,#36218,#4458,.T.);
#45180=EDGE_CURVE('',#36220,#36219,#4459,.T.);
#45181=EDGE_CURVE('',#36221,#36220,#4460,.T.);
#45182=EDGE_CURVE('',#36206,#36221,#20994,.T.);
#45183=EDGE_CURVE('',#35545,#36222,#20995,.T.);
#45184=EDGE_CURVE('',#36222,#36207,#29764,.T.);
#45185=EDGE_CURVE('',#36223,#35546,#20996,.T.);
#45186=EDGE_CURVE('',#36222,#36223,#20997,.T.);
#45187=EDGE_CURVE('',#35547,#36224,#20998,.T.);
#45188=EDGE_CURVE('',#36223,#36224,#29765,.T.);
#45189=EDGE_CURVE('',#36225,#36226,#20999,.T.);
#45190=EDGE_CURVE('',#36227,#36225,#29766,.T.);
#45191=EDGE_CURVE('',#36228,#36227,#21000,.T.);
#45192=EDGE_CURVE('',#36224,#36228,#29767,.T.);
#45193=EDGE_CURVE('',#36229,#36154,#21001,.T.);
#45194=EDGE_CURVE('',#36230,#36229,#4461,.T.);
#45195=EDGE_CURVE('',#36231,#36230,#4462,.T.);
#45196=EDGE_CURVE('',#36232,#36231,#4463,.T.);
#45197=EDGE_CURVE('',#36233,#36232,#21002,.T.);
#45198=EDGE_CURVE('',#36234,#36233,#4464,.T.);
#45199=EDGE_CURVE('',#36235,#36234,#4465,.T.);
#45200=EDGE_CURVE('',#36236,#36235,#4466,.T.);
#45201=EDGE_CURVE('',#36237,#36236,#21003,.T.);
#45202=EDGE_CURVE('',#36238,#36237,#1122,.T.);
#45203=EDGE_CURVE('',#36226,#36238,#21004,.T.);
#45204=EDGE_CURVE('',#36239,#36240,#29768,.T.);
#45205=EDGE_CURVE('',#36241,#36240,#4467,.T.);
#45206=EDGE_CURVE('',#36241,#35550,#29769,.T.);
#45207=EDGE_CURVE('',#36239,#35549,#1855,.T.);
#45208=EDGE_CURVE('',#35552,#36242,#4468,.T.);
#45209=EDGE_CURVE('',#36242,#35549,#29770,.T.);
#45210=EDGE_CURVE('',#36243,#36244,#4469,.T.);
#45211=EDGE_CURVE('',#36245,#36243,#4470,.T.);
#45212=EDGE_CURVE('',#36246,#36245,#4471,.T.);
#45213=EDGE_CURVE('',#36247,#36246,#4472,.T.);
#45214=EDGE_CURVE('',#36248,#36247,#21005,.T.);
#45215=EDGE_CURVE('',#36249,#36248,#4473,.T.);
#45216=EDGE_CURVE('',#36250,#36249,#4474,.T.);
#45217=EDGE_CURVE('',#36242,#36250,#1856,.T.);
#45218=EDGE_CURVE('',#36251,#35879,#29771,.T.);
#45219=EDGE_CURVE('',#36252,#36251,#21006,.T.);
#45220=EDGE_CURVE('',#36253,#36252,#29772,.T.);
#45221=EDGE_CURVE('',#36254,#36253,#21007,.T.);
#45222=EDGE_CURVE('',#36244,#36254,#21008,.T.);
#45223=EDGE_CURVE('',#35553,#36255,#29773,.T.);
#45224=EDGE_CURVE('',#35554,#36255,#1123,.T.);
#45225=EDGE_CURVE('',#36256,#36257,#1124,.T.);
#45226=EDGE_CURVE('',#36258,#36256,#21009,.T.);
#45227=EDGE_CURVE('',#36259,#36258,#4475,.T.);
#45228=EDGE_CURVE('',#36260,#36259,#21010,.T.);
#45229=EDGE_CURVE('',#36261,#36260,#21011,.T.);
#45230=EDGE_CURVE('',#36262,#36261,#21012,.T.);
#45231=EDGE_CURVE('',#36263,#36262,#4476,.T.);
#45232=EDGE_CURVE('',#36255,#36263,#21013,.T.);
#45233=EDGE_CURVE('',#36264,#35555,#21014,.T.);
#45234=EDGE_CURVE('',#36265,#36264,#29774,.T.);
#45235=EDGE_CURVE('',#36266,#36265,#21015,.T.);
#45236=EDGE_CURVE('',#36267,#36266,#29775,.T.);
#45237=EDGE_CURVE('',#36268,#36267,#21016,.T.);
#45238=EDGE_CURVE('',#36257,#36268,#21017,.T.);
#45239=EDGE_CURVE('',#35556,#36269,#21018,.T.);
#45240=EDGE_CURVE('',#36264,#36269,#29776,.T.);
#45241=EDGE_CURVE('',#36270,#35557,#21019,.T.);
#45242=EDGE_CURVE('',#36269,#36270,#21020,.T.);
#45243=EDGE_CURVE('',#35558,#36271,#21021,.T.);
#45244=EDGE_CURVE('',#36270,#36271,#29777,.T.);
#45245=EDGE_CURVE('',#36272,#36273,#21022,.T.);
#45246=EDGE_CURVE('',#36274,#36272,#29778,.T.);
#45247=EDGE_CURVE('',#36275,#36274,#21023,.T.);
#45248=EDGE_CURVE('',#36271,#36275,#29779,.T.);
#45249=EDGE_CURVE('',#36276,#35559,#1125,.T.);
#45250=EDGE_CURVE('',#36277,#36276,#21024,.T.);
#45251=EDGE_CURVE('',#36278,#36277,#4477,.T.);
#45252=EDGE_CURVE('',#36279,#36278,#1126,.T.);
#45253=EDGE_CURVE('',#36280,#36279,#4478,.T.);
#45254=EDGE_CURVE('',#36281,#36280,#21025,.T.);
#45255=EDGE_CURVE('',#36282,#36281,#4479,.T.);
#45256=EDGE_CURVE('',#36283,#36282,#1127,.T.);
#45257=EDGE_CURVE('',#36284,#36283,#4480,.T.);
#45258=EDGE_CURVE('',#36285,#36284,#21026,.T.);
#45259=EDGE_CURVE('',#36286,#36285,#1128,.T.);
#45260=EDGE_CURVE('',#36273,#36286,#21027,.T.);
#45261=EDGE_CURVE('',#35561,#36276,#29780,.T.);
#45262=EDGE_CURVE('',#36287,#36288,#29781,.T.);
#45263=EDGE_CURVE('',#35561,#36287,#21028,.T.);
#45264=EDGE_CURVE('',#36288,#35560,#21029,.T.);
#45265=EDGE_CURVE('',#35560,#36289,#29782,.T.);
#45266=EDGE_CURVE('',#35562,#36289,#4481,.T.);
#45267=EDGE_CURVE('',#36290,#35563,#21030,.T.);
#45268=EDGE_CURVE('',#36291,#36290,#29783,.T.);
#45269=EDGE_CURVE('',#36292,#36291,#21031,.T.);
#45270=EDGE_CURVE('',#36293,#36292,#29784,.T.);
#45271=EDGE_CURVE('',#36294,#36293,#21032,.T.);
#45272=EDGE_CURVE('',#36295,#36294,#21033,.T.);
#45273=EDGE_CURVE('',#36296,#36295,#1129,.T.);
#45274=EDGE_CURVE('',#36297,#36296,#21034,.T.);
#45275=EDGE_CURVE('',#36298,#36297,#4482,.T.);
#45276=EDGE_CURVE('',#36299,#36298,#4483,.T.);
#45277=EDGE_CURVE('',#36300,#36299,#4484,.T.);
#45278=EDGE_CURVE('',#36301,#36300,#21035,.T.);
#45279=EDGE_CURVE('',#36302,#36301,#4485,.T.);
#45280=EDGE_CURVE('',#36303,#36302,#4486,.T.);
#45281=EDGE_CURVE('',#36304,#36303,#4487,.T.);
#45282=EDGE_CURVE('',#36289,#36304,#21036,.T.);
#45283=EDGE_CURVE('',#35564,#36305,#21037,.T.);
#45284=EDGE_CURVE('',#36305,#36290,#29785,.T.);
#45285=EDGE_CURVE('',#36306,#35565,#21038,.T.);
#45286=EDGE_CURVE('',#36305,#36306,#21039,.T.);
#45287=EDGE_CURVE('',#35567,#36307,#21040,.T.);
#45288=EDGE_CURVE('',#36306,#36307,#29786,.T.);
#45289=EDGE_CURVE('',#36308,#35570,#29787,.T.);
#45290=EDGE_CURVE('',#36308,#35569,#1130,.T.);
#45291=EDGE_CURVE('',#36309,#36310,#21041,.T.);
#45292=EDGE_CURVE('',#36311,#36309,#29788,.T.);
#45293=EDGE_CURVE('',#36312,#36311,#21042,.T.);
#45294=EDGE_CURVE('',#36307,#36312,#29789,.T.);
#45295=EDGE_CURVE('',#36313,#36308,#21043,.T.);
#45296=EDGE_CURVE('',#36314,#36313,#4488,.T.);
#45297=EDGE_CURVE('',#36315,#36314,#4489,.T.);
#45298=EDGE_CURVE('',#36316,#36315,#4490,.T.);
#45299=EDGE_CURVE('',#36317,#36316,#21044,.T.);
#45300=EDGE_CURVE('',#36318,#36317,#4491,.T.);
#45301=EDGE_CURVE('',#36319,#36318,#4492,.T.);
#45302=EDGE_CURVE('',#36320,#36319,#4493,.T.);
#45303=EDGE_CURVE('',#36321,#36320,#21045,.T.);
#45304=EDGE_CURVE('',#36322,#36321,#1131,.T.);
#45305=EDGE_CURVE('',#36310,#36322,#21046,.T.);
#45306=EDGE_CURVE('',#35570,#36241,#21047,.T.);
#45307=EDGE_CURVE('',#36184,#35576,#29790,.T.);
#45308=EDGE_CURVE('',#36323,#36323,#29791,.T.);
#45309=EDGE_CURVE('',#36323,#36324,#21048,.T.);
#45310=EDGE_CURVE('',#36324,#36324,#29792,.T.);
#45311=EDGE_CURVE('',#36325,#36325,#29793,.T.);
#45312=EDGE_CURVE('',#36325,#36326,#21049,.T.);
#45313=EDGE_CURVE('',#35576,#36326,#4494,.F.);
#45314=EDGE_CURVE('',#36326,#35575,#4495,.F.);
#45315=EDGE_CURVE('',#35575,#36185,#29794,.T.);
#45316=EDGE_CURVE('',#35574,#36186,#29795,.T.);
#45317=EDGE_CURVE('',#35573,#36327,#29796,.T.);
#45318=EDGE_CURVE('',#36327,#36186,#29797,.T.);
#45319=EDGE_CURVE('',#35572,#36328,#29798,.T.);
#45320=EDGE_CURVE('',#36328,#36327,#29799,.T.);
#45321=EDGE_CURVE('',#35571,#36137,#29800,.T.);
#45322=EDGE_CURVE('',#36137,#36328,#29801,.T.);
#45323=EDGE_CURVE('',#35579,#36063,#29802,.T.);
#45324=EDGE_CURVE('',#36329,#36329,#29803,.T.);
#45325=EDGE_CURVE('',#36329,#36330,#21050,.T.);
#45326=EDGE_CURVE('',#36330,#36330,#29804,.T.);
#45327=EDGE_CURVE('',#36331,#36331,#29805,.T.);
#45328=EDGE_CURVE('',#36331,#35578,#21051,.T.);
#45329=EDGE_CURVE('',#36332,#35577,#4496,.T.);
#45330=EDGE_CURVE('',#36333,#36332,#29806,.T.);
#45331=EDGE_CURVE('',#35579,#36333,#4497,.T.);
#45332=EDGE_CURVE('',#35577,#36263,#29807,.T.);
#45333=EDGE_CURVE('',#36334,#35580,#29808,.T.);
#45334=EDGE_CURVE('',#36334,#36335,#21052,.T.);
#45335=EDGE_CURVE('',#35581,#36335,#29809,.T.);
#45336=EDGE_CURVE('',#36334,#36071,#29810,.T.);
#45337=EDGE_CURVE('',#35593,#36336,#21053,.T.);
#45338=EDGE_CURVE('',#36336,#36145,#29811,.T.);
#45339=EDGE_CURVE('',#36337,#35595,#21054,.T.);
#45340=EDGE_CURVE('',#36336,#36337,#21055,.T.);
#45341=EDGE_CURVE('',#35600,#36141,#29812,.T.);
#45342=EDGE_CURVE('',#36141,#35595,#4498,.T.);
#45343=EDGE_CURVE('',#35596,#36338,#29813,.T.);
#45344=EDGE_CURVE('',#35597,#36187,#29814,.T.);
#45345=EDGE_CURVE('',#36187,#36338,#4499,.T.);
#45346=EDGE_CURVE('',#35603,#36175,#29815,.T.);
#45347=EDGE_CURVE('',#35599,#36138,#29816,.T.);
#45348=EDGE_CURVE('',#35598,#36339,#29817,.T.);
#45349=EDGE_CURVE('',#36339,#36138,#4500,.T.);
#45350=EDGE_CURVE('',#36338,#36339,#4501,.T.);
#45351=EDGE_CURVE('',#35607,#35872,#21056,.T.);
#45352=EDGE_CURVE('',#35871,#35609,#21057,.T.);
#45353=EDGE_CURVE('',#35870,#35616,#29818,.T.);
#45354=EDGE_CURVE('',#35614,#35867,#29819,.T.);
#45355=EDGE_CURVE('',#35623,#35864,#21058,.T.);
#45356=EDGE_CURVE('',#35863,#35625,#21059,.T.);
#45357=EDGE_CURVE('',#35631,#35860,#29820,.T.);
#45358=EDGE_CURVE('',#35861,#35634,#29821,.T.);
#45359=EDGE_CURVE('',#35633,#36340,#1857,.T.);
#45360=EDGE_CURVE('',#35856,#36340,#4502,.T.);
#45361=EDGE_CURVE('',#35634,#35857,#1858,.T.);
#45362=EDGE_CURVE('',#36340,#35635,#21060,.T.);
#45363=EDGE_CURVE('',#35635,#35854,#29822,.T.);
#45364=EDGE_CURVE('',#35641,#36341,#21061,.T.);
#45365=EDGE_CURVE('',#36341,#35855,#29823,.T.);
#45366=EDGE_CURVE('',#36342,#35643,#21062,.T.);
#45367=EDGE_CURVE('',#36341,#36342,#21063,.T.);
#45368=EDGE_CURVE('',#36342,#35843,#29824,.T.);
#45369=EDGE_CURVE('',#35844,#35650,#29825,.T.);
#45370=EDGE_CURVE('',#36343,#35649,#21064,.T.);
#45371=EDGE_CURVE('',#36344,#36343,#4503,.T.);
#45372=EDGE_CURVE('',#35650,#36344,#21065,.T.);
#45373=EDGE_CURVE('',#35649,#36134,#29826,.T.);
#45374=EDGE_CURVE('',#35655,#36345,#21066,.T.);
#45375=EDGE_CURVE('',#36345,#36135,#29827,.T.);
#45376=EDGE_CURVE('',#36346,#35657,#21067,.T.);
#45377=EDGE_CURVE('',#36345,#36346,#21068,.T.);
#45378=EDGE_CURVE('',#36346,#36121,#29828,.T.);
#45379=EDGE_CURVE('',#36122,#35664,#29829,.T.);
#45380=EDGE_CURVE('',#36347,#35663,#21069,.T.);
#45381=EDGE_CURVE('',#36348,#36347,#4504,.T.);
#45382=EDGE_CURVE('',#35664,#36348,#21070,.T.);
#45383=EDGE_CURVE('',#35663,#36150,#29830,.T.);
#45384=EDGE_CURVE('',#36174,#35666,#29831,.T.);
#45385=EDGE_CURVE('',#35666,#36349,#29832,.T.);
#45386=EDGE_CURVE('',#35672,#35723,#29833,.T.);
#45387=EDGE_CURVE('',#35723,#36349,#21071,.T.);
#45388=EDGE_CURVE('',#35671,#35718,#29834,.T.);
#45389=EDGE_CURVE('',#35670,#36350,#29835,.T.);
#45390=EDGE_CURVE('',#36350,#35718,#21072,.T.);
#45391=EDGE_CURVE('',#35669,#36351,#29836,.T.);
#45392=EDGE_CURVE('',#36351,#36350,#4505,.T.);
#45393=EDGE_CURVE('',#35668,#36352,#29837,.T.);
#45394=EDGE_CURVE('',#36352,#36351,#21073,.T.);
#45395=EDGE_CURVE('',#35679,#36352,#4506,.T.);
#45396=EDGE_CURVE('',#36353,#35684,#21074,.T.);
#45397=EDGE_CURVE('',#36351,#36353,#21075,.T.);
#45398=EDGE_CURVE('',#35686,#36354,#21076,.T.);
#45399=EDGE_CURVE('',#36353,#36354,#29838,.T.);
#45400=EDGE_CURVE('',#36355,#35688,#21077,.T.);
#45401=EDGE_CURVE('',#36354,#36355,#29839,.T.);
#45402=EDGE_CURVE('',#35690,#36356,#21078,.T.);
#45403=EDGE_CURVE('',#36355,#36356,#29840,.T.);
#45404=EDGE_CURVE('',#36356,#36357,#21079,.T.);
#45405=EDGE_CURVE('',#36358,#35692,#21080,.T.);
#45406=EDGE_CURVE('',#36359,#36358,#4507,.T.);
#45407=EDGE_CURVE('',#36360,#36359,#21081,.T.);
#45408=EDGE_CURVE('',#36361,#36360,#21082,.T.);
#45409=EDGE_CURVE('',#36362,#36361,#4508,.T.);
#45410=EDGE_CURVE('',#36363,#36362,#21083,.T.);
#45411=EDGE_CURVE('',#36364,#36363,#4509,.T.);
#45412=EDGE_CURVE('',#36365,#36364,#21084,.T.);
#45413=EDGE_CURVE('',#36366,#36365,#21085,.T.);
#45414=EDGE_CURVE('',#36367,#36366,#21086,.T.);
#45415=EDGE_CURVE('',#36368,#36367,#4510,.T.);
#45416=EDGE_CURVE('',#36369,#36368,#21087,.T.);
#45417=EDGE_CURVE('',#36370,#36369,#4511,.T.);
#45418=EDGE_CURVE('',#36357,#36370,#21088,.T.);
#45419=EDGE_CURVE('',#36371,#36372,#21089,.T.);
#45420=EDGE_CURVE('',#36358,#36371,#4512,.T.);
#45421=EDGE_CURVE('',#35694,#36373,#21090,.T.);
#45422=EDGE_CURVE('',#36372,#36373,#4513,.T.);
#45423=EDGE_CURVE('',#36374,#35696,#21091,.T.);
#45424=EDGE_CURVE('',#36375,#36374,#1859,.T.);
#45425=EDGE_CURVE('',#36376,#36375,#29841,.T.);
#45426=EDGE_CURVE('',#36377,#36376,#4514,.T.);
#45427=EDGE_CURVE('',#36378,#36377,#21092,.T.);
#45428=EDGE_CURVE('',#36379,#36378,#29842,.T.);
#45429=EDGE_CURVE('',#36380,#36379,#21093,.T.);
#45430=EDGE_CURVE('',#36381,#36380,#4515,.T.);
#45431=EDGE_CURVE('',#36382,#36381,#29843,.T.);
#45432=EDGE_CURVE('',#36383,#36382,#4516,.T.);
#45433=EDGE_CURVE('',#36384,#36383,#1860,.T.);
#45434=EDGE_CURVE('',#36385,#36384,#21094,.T.);
#45435=EDGE_CURVE('',#36386,#36385,#29844,.T.);
#45436=EDGE_CURVE('',#36387,#36386,#21095,.T.);
#45437=EDGE_CURVE('',#36388,#36387,#4517,.T.);
#45438=EDGE_CURVE('',#36389,#36388,#29845,.T.);
#45439=EDGE_CURVE('',#36390,#36389,#4518,.T.);
#45440=EDGE_CURVE('',#36391,#36390,#21096,.T.);
#45441=EDGE_CURVE('',#36392,#36391,#29846,.T.);
#45442=EDGE_CURVE('',#36393,#36392,#21097,.T.);
#45443=EDGE_CURVE('',#36394,#36393,#4519,.T.);
#45444=EDGE_CURVE('',#36395,#36394,#29847,.T.);
#45445=EDGE_CURVE('',#36396,#36395,#4520,.T.);
#45446=EDGE_CURVE('',#36397,#36396,#21098,.T.);
#45447=EDGE_CURVE('',#36398,#36397,#29848,.T.);
#45448=EDGE_CURVE('',#36399,#36398,#21099,.T.);
#45449=EDGE_CURVE('',#36400,#36399,#4521,.T.);
#45450=EDGE_CURVE('',#36401,#36400,#29849,.T.);
#45451=EDGE_CURVE('',#36402,#36401,#4522,.T.);
#45452=EDGE_CURVE('',#36403,#36402,#21100,.T.);
#45453=EDGE_CURVE('',#36404,#36403,#29850,.T.);
#45454=EDGE_CURVE('',#36405,#36404,#21101,.T.);
#45455=EDGE_CURVE('',#36406,#36405,#4523,.T.);
#45456=EDGE_CURVE('',#36407,#36406,#4524,.T.);
#45457=EDGE_CURVE('',#36408,#36407,#29851,.T.);
#45458=EDGE_CURVE('',#36409,#36408,#4525,.T.);
#45459=EDGE_CURVE('',#36410,#36409,#21102,.T.);
#45460=EDGE_CURVE('',#36411,#36410,#29852,.T.);
#45461=EDGE_CURVE('',#36412,#36411,#21103,.T.);
#45462=EDGE_CURVE('',#36413,#36412,#4526,.T.);
#45463=EDGE_CURVE('',#36414,#36413,#29853,.T.);
#45464=EDGE_CURVE('',#36373,#36414,#4527,.T.);
#45465=EDGE_CURVE('',#35698,#36415,#21104,.T.);
#45466=EDGE_CURVE('',#36416,#36415,#4528,.T.);
#45467=EDGE_CURVE('',#36417,#36416,#21105,.T.);
#45468=EDGE_CURVE('',#36374,#36417,#4529,.T.);
#45469=EDGE_CURVE('',#36418,#36419,#21106,.T.);
#45470=EDGE_CURVE('',#36420,#36418,#21107,.T.);
#45471=EDGE_CURVE('',#36421,#36420,#4530,.T.);
#45472=EDGE_CURVE('',#36422,#36421,#21108,.T.);
#45473=EDGE_CURVE('',#36423,#36422,#4531,.T.);
#45474=EDGE_CURVE('',#36424,#36423,#21109,.T.);
#45475=EDGE_CURVE('',#36425,#36424,#21110,.T.);
#45476=EDGE_CURVE('',#36415,#36425,#4532,.T.);
#45477=EDGE_CURVE('',#36426,#35700,#21111,.T.);
#45478=EDGE_CURVE('',#36427,#36426,#21112,.T.);
#45479=EDGE_CURVE('',#36428,#36427,#21113,.T.);
#45480=EDGE_CURVE('',#36429,#36428,#4533,.T.);
#45481=EDGE_CURVE('',#36430,#36429,#21114,.T.);
#45482=EDGE_CURVE('',#36431,#36430,#4534,.T.);
#45483=EDGE_CURVE('',#36419,#36431,#21115,.T.);
#45484=EDGE_CURVE('',#35702,#36432,#21116,.T.);
#45485=EDGE_CURVE('',#36426,#36432,#29854,.T.);
#45486=EDGE_CURVE('',#36433,#35704,#21117,.T.);
#45487=EDGE_CURVE('',#36432,#36433,#29855,.T.);
#45488=EDGE_CURVE('',#35706,#36434,#21118,.T.);
#45489=EDGE_CURVE('',#36433,#36434,#29856,.T.);
#45490=EDGE_CURVE('',#36434,#36435,#21119,.T.);
#45491=EDGE_CURVE('',#36436,#35768,#4535,.T.);
#45492=EDGE_CURVE('',#36437,#36436,#21120,.T.);
#45493=EDGE_CURVE('',#36438,#36437,#21121,.T.);
#45494=EDGE_CURVE('',#36439,#36438,#4536,.T.);
#45495=EDGE_CURVE('',#36440,#36439,#21122,.T.);
#45496=EDGE_CURVE('',#36441,#36440,#4537,.T.);
#45497=EDGE_CURVE('',#36442,#36441,#21123,.T.);
#45498=EDGE_CURVE('',#36443,#36442,#21124,.T.);
#45499=EDGE_CURVE('',#36444,#36443,#21125,.T.);
#45500=EDGE_CURVE('',#36445,#36444,#4538,.T.);
#45501=EDGE_CURVE('',#36446,#36445,#21126,.T.);
#45502=EDGE_CURVE('',#36447,#36446,#4539,.T.);
#45503=EDGE_CURVE('',#36435,#36447,#21127,.T.);
#45504=EDGE_CURVE('',#36054,#35716,#29857,.T.);
#45505=EDGE_CURVE('',#36055,#35717,#29858,.T.);
#45506=EDGE_CURVE('',#36448,#36449,#21128,.T.);
#45507=EDGE_CURVE('',#36450,#36448,#29859,.T.);
#45508=EDGE_CURVE('',#36451,#36450,#29860,.T.);
#45509=EDGE_CURVE('',#36452,#36451,#29861,.T.);
#45510=EDGE_CURVE('',#36453,#36452,#21129,.T.);
#45511=EDGE_CURVE('',#35716,#36453,#21130,.T.);
#45512=EDGE_CURVE('',#36449,#35713,#21131,.T.);
#45513=EDGE_CURVE('',#36259,#35712,#29862,.T.);
#45514=EDGE_CURVE('',#36258,#35713,#29863,.T.);
#45515=EDGE_CURVE('',#36454,#35717,#21132,.T.);
#45516=EDGE_CURVE('',#36455,#36454,#29864,.T.);
#45517=EDGE_CURVE('',#35712,#36455,#21133,.T.);
#45518=EDGE_CURVE('',#36177,#35719,#29865,.T.);
#45519=EDGE_CURVE('',#36176,#35722,#29866,.T.);
#45520=EDGE_CURVE('',#36456,#36350,#21134,.T.);
#45521=EDGE_CURVE('',#36457,#36456,#29867,.T.);
#45522=EDGE_CURVE('',#36458,#36457,#29868,.T.);
#45523=EDGE_CURVE('',#36459,#36458,#29869,.T.);
#45524=EDGE_CURVE('',#36460,#36459,#21135,.T.);
#45525=EDGE_CURVE('',#35719,#36460,#21136,.T.);
#45526=EDGE_CURVE('',#36349,#35722,#21137,.T.);
#45527=EDGE_CURVE('',#36461,#35833,#29870,.T.);
#45528=EDGE_CURVE('',#36461,#35726,#21138,.T.);
#45529=EDGE_CURVE('',#35732,#35834,#29871,.T.);
#45530=EDGE_CURVE('',#36462,#35731,#1132,.T.);
#45531=EDGE_CURVE('',#36463,#36462,#4540,.T.);
#45532=EDGE_CURVE('',#35732,#36463,#4541,.T.);
#45533=EDGE_CURVE('',#35826,#35731,#29872,.T.);
#45534=EDGE_CURVE('',#35736,#36464,#21139,.T.);
#45535=EDGE_CURVE('',#36464,#35819,#29873,.T.);
#45536=EDGE_CURVE('',#36465,#35738,#21140,.T.);
#45537=EDGE_CURVE('',#36464,#36465,#21141,.T.);
#45538=EDGE_CURVE('',#36465,#35809,#29874,.T.);
#45539=EDGE_CURVE('',#35746,#35810,#29875,.T.);
#45540=EDGE_CURVE('',#36466,#35745,#1133,.T.);
#45541=EDGE_CURVE('',#36467,#36466,#4542,.T.);
#45542=EDGE_CURVE('',#35746,#36467,#4543,.T.);
#45543=EDGE_CURVE('',#35802,#35745,#29876,.T.);
#45544=EDGE_CURVE('',#35750,#36468,#4544,.T.);
#45545=EDGE_CURVE('',#36468,#35797,#29877,.T.);
#45546=EDGE_CURVE('',#36469,#35752,#4545,.T.);
#45547=EDGE_CURVE('',#36469,#36468,#4546,.T.);
#45548=EDGE_CURVE('',#36469,#35787,#29878,.T.);
#45549=EDGE_CURVE('',#35760,#35788,#29879,.T.);
#45550=EDGE_CURVE('',#36470,#35759,#4547,.T.);
#45551=EDGE_CURVE('',#36471,#36470,#4548,.T.);
#45552=EDGE_CURVE('',#35760,#36471,#1134,.T.);
#45553=EDGE_CURVE('',#35782,#35759,#29880,.T.);
#45554=EDGE_CURVE('',#36069,#35767,#29881,.T.);
#45555=EDGE_CURVE('',#36079,#35766,#29882,.T.);
#45556=EDGE_CURVE('',#35772,#36069,#4549,.T.);
#45557=EDGE_CURVE('',#36472,#36473,#1135,.T.);
#45558=EDGE_CURVE('',#35768,#36473,#29883,.T.);
#45559=EDGE_CURVE('',#36472,#35766,#4550,.T.);
#45560=EDGE_CURVE('',#35770,#36474,#21142,.T.);
#45561=EDGE_CURVE('',#36474,#36068,#29884,.T.);
#45562=EDGE_CURVE('',#36474,#36461,#21143,.T.);
#45563=EDGE_CURVE('',#35778,#35783,#29885,.T.);
#45564=EDGE_CURVE('',#35781,#36470,#29886,.T.);
#45565=EDGE_CURVE('',#35780,#36475,#29887,.T.);
#45566=EDGE_CURVE('',#36475,#36470,#1861,.T.);
#45567=EDGE_CURVE('',#35779,#36476,#29888,.T.);
#45568=EDGE_CURVE('',#36476,#36475,#21144,.T.);
#45569=EDGE_CURVE('',#35783,#36476,#1862,.T.);
#45570=EDGE_CURVE('',#36477,#36476,#4551,.T.);
#45571=EDGE_CURVE('',#36477,#35784,#4552,.T.);
#45572=EDGE_CURVE('',#35784,#35792,#29889,.T.);
#45573=EDGE_CURVE('',#36477,#35791,#29890,.T.);
#45574=EDGE_CURVE('',#36478,#35790,#29891,.T.);
#45575=EDGE_CURVE('',#36478,#36477,#21145,.T.);
#45576=EDGE_CURVE('',#36471,#35789,#29892,.T.);
#45577=EDGE_CURVE('',#36471,#36478,#4553,.T.);
#45578=EDGE_CURVE('',#35793,#36469,#21146,.T.);
#45579=EDGE_CURVE('',#36468,#35794,#21147,.T.);
#45580=EDGE_CURVE('',#35798,#35803,#29893,.T.);
#45581=EDGE_CURVE('',#35801,#36466,#29894,.T.);
#45582=EDGE_CURVE('',#35800,#36479,#29895,.T.);
#45583=EDGE_CURVE('',#36479,#36466,#4554,.T.);
#45584=EDGE_CURVE('',#35799,#36480,#29896,.T.);
#45585=EDGE_CURVE('',#36480,#36479,#21148,.T.);
#45586=EDGE_CURVE('',#35803,#36480,#4555,.T.);
#45587=EDGE_CURVE('',#36481,#36480,#4556,.T.);
#45588=EDGE_CURVE('',#36481,#35804,#1136,.T.);
#45589=EDGE_CURVE('',#35804,#35814,#29897,.T.);
#45590=EDGE_CURVE('',#36481,#35813,#29898,.T.);
#45591=EDGE_CURVE('',#36482,#35812,#29899,.T.);
#45592=EDGE_CURVE('',#36482,#36481,#21149,.T.);
#45593=EDGE_CURVE('',#36467,#35811,#29900,.T.);
#45594=EDGE_CURVE('',#36467,#36482,#4557,.T.);
#45595=EDGE_CURVE('',#36483,#35808,#29901,.T.);
#45596=EDGE_CURVE('',#36483,#36465,#29902,.T.);
#45597=EDGE_CURVE('',#36484,#35807,#29903,.T.);
#45598=EDGE_CURVE('',#36484,#36483,#21150,.T.);
#45599=EDGE_CURVE('',#35815,#36484,#29904,.T.);
#45600=EDGE_CURVE('',#36485,#35816,#29905,.T.);
#45601=EDGE_CURVE('',#36485,#36484,#21151,.T.);
#45602=EDGE_CURVE('',#36485,#35821,#29906,.T.);
#45603=EDGE_CURVE('',#35822,#35827,#29907,.T.);
#45604=EDGE_CURVE('',#35825,#36462,#29908,.T.);
#45605=EDGE_CURVE('',#35824,#36486,#29909,.T.);
#45606=EDGE_CURVE('',#36486,#36462,#4558,.T.);
#45607=EDGE_CURVE('',#35823,#36487,#29910,.T.);
#45608=EDGE_CURVE('',#36487,#36486,#21152,.T.);
#45609=EDGE_CURVE('',#35827,#36487,#4559,.T.);
#45610=EDGE_CURVE('',#36488,#35820,#29911,.T.);
#45611=EDGE_CURVE('',#36488,#36485,#21153,.T.);
#45612=EDGE_CURVE('',#36464,#36488,#29912,.T.);
#45613=EDGE_CURVE('',#36489,#36487,#4560,.T.);
#45614=EDGE_CURVE('',#36489,#35828,#1137,.T.);
#45615=EDGE_CURVE('',#35828,#35838,#29913,.T.);
#45616=EDGE_CURVE('',#36489,#35837,#29914,.T.);
#45617=EDGE_CURVE('',#36490,#35836,#29915,.T.);
#45618=EDGE_CURVE('',#36490,#36489,#21154,.T.);
#45619=EDGE_CURVE('',#36463,#35835,#29916,.T.);
#45620=EDGE_CURVE('',#36463,#36490,#4561,.T.);
#45621=EDGE_CURVE('',#36491,#35832,#29917,.T.);
#45622=EDGE_CURVE('',#36491,#36461,#29918,.T.);
#45623=EDGE_CURVE('',#36335,#35831,#29919,.T.);
#45624=EDGE_CURVE('',#36335,#36491,#21155,.T.);
#45625=EDGE_CURVE('',#36492,#36493,#4562,.T.);
#45626=EDGE_CURVE('',#35840,#36492,#4563,.T.);
#45627=EDGE_CURVE('',#36493,#35839,#1138,.T.);
#45628=EDGE_CURVE('',#35847,#35839,#29920,.T.);
#45629=EDGE_CURVE('',#35840,#36131,#29921,.T.);
#45630=EDGE_CURVE('',#35846,#36493,#29922,.T.);
#45631=EDGE_CURVE('',#35845,#36344,#29923,.T.);
#45632=EDGE_CURVE('',#36344,#36493,#4564,.T.);
#45633=EDGE_CURVE('',#35848,#36342,#29924,.T.);
#45634=EDGE_CURVE('',#36341,#35849,#29925,.T.);
#45635=EDGE_CURVE('',#36340,#35853,#29926,.T.);
#45636=EDGE_CURVE('',#35856,#35852,#29927,.T.);
#45637=EDGE_CURVE('',#35862,#35857,#29928,.T.);
#45638=EDGE_CURVE('',#35874,#36494,#29929,.T.);
#45639=EDGE_CURVE('',#36494,#36028,#29930,.T.);
#45640=EDGE_CURVE('',#36495,#35876,#29931,.T.);
#45641=EDGE_CURVE('',#36495,#36494,#21156,.T.);
#45642=EDGE_CURVE('',#36495,#36191,#29932,.T.);
#45643=EDGE_CURVE('',#35878,#36496,#29933,.T.);
#45644=EDGE_CURVE('',#36496,#36251,#29934,.T.);
#45645=EDGE_CURVE('',#36497,#35880,#29935,.T.);
#45646=EDGE_CURVE('',#36497,#36496,#21157,.T.);
#45647=EDGE_CURVE('',#36497,#35885,#29936,.T.);
#45648=EDGE_CURVE('',#36498,#36499,#21158,.T.);
#45649=EDGE_CURVE('',#36499,#35882,#29937,.T.);
#45650=EDGE_CURVE('',#36498,#35883,#4565,.T.);
#45651=EDGE_CURVE('',#36378,#35892,#29938,.T.);
#45652=EDGE_CURVE('',#36377,#35883,#29939,.T.);
#45653=EDGE_CURVE('',#36500,#35891,#29940,.T.);
#45654=EDGE_CURVE('',#36500,#36378,#1863,.T.);
#45655=EDGE_CURVE('',#36501,#35890,#29941,.T.);
#45656=EDGE_CURVE('',#36501,#36500,#4566,.T.);
#45657=EDGE_CURVE('',#36502,#35889,#29942,.T.);
#45658=EDGE_CURVE('',#36502,#36501,#4567,.T.);
#45659=EDGE_CURVE('',#36503,#35888,#29943,.T.);
#45660=EDGE_CURVE('',#36503,#36502,#21159,.T.);
#45661=EDGE_CURVE('',#35893,#35887,#29944,.T.);
#45662=EDGE_CURVE('',#35893,#36503,#4568,.T.);
#45663=EDGE_CURVE('',#36504,#35884,#29945,.T.);
#45664=EDGE_CURVE('',#36504,#36497,#21160,.T.);
#45665=EDGE_CURVE('',#36499,#36504,#29946,.T.);
#45666=EDGE_CURVE('',#36505,#36503,#4569,.T.);
#45667=EDGE_CURVE('',#36505,#35894,#4570,.T.);
#45668=EDGE_CURVE('',#35906,#35894,#29947,.T.);
#45669=EDGE_CURVE('',#36505,#35905,#29948,.T.);
#45670=EDGE_CURVE('',#36506,#35904,#29949,.T.);
#45671=EDGE_CURVE('',#36506,#36505,#21161,.T.);
#45672=EDGE_CURVE('',#36507,#35903,#29950,.T.);
#45673=EDGE_CURVE('',#36507,#36506,#4571,.T.);
#45674=EDGE_CURVE('',#36508,#35902,#29951,.T.);
#45675=EDGE_CURVE('',#36508,#36507,#4572,.T.);
#45676=EDGE_CURVE('',#36379,#35901,#29952,.T.);
#45677=EDGE_CURVE('',#36379,#36508,#1864,.T.);
#45678=EDGE_CURVE('',#36380,#35900,#29953,.T.);
#45679=EDGE_CURVE('',#36509,#35899,#29954,.T.);
#45680=EDGE_CURVE('',#36509,#36510,#21162,.T.);
#45681=EDGE_CURVE('',#35900,#36510,#4573,.T.);
#45682=EDGE_CURVE('',#36511,#35898,#29955,.T.);
#45683=EDGE_CURVE('',#36511,#36509,#29956,.T.);
#45684=EDGE_CURVE('',#36512,#35897,#29957,.T.);
#45685=EDGE_CURVE('',#36512,#36511,#21163,.T.);
#45686=EDGE_CURVE('',#35907,#36512,#29958,.T.);
#45687=EDGE_CURVE('',#36513,#35908,#29959,.T.);
#45688=EDGE_CURVE('',#36513,#36512,#21164,.T.);
#45689=EDGE_CURVE('',#36513,#35919,#29960,.T.);
#45690=EDGE_CURVE('',#35911,#35920,#29961,.T.);
#45691=EDGE_CURVE('',#36514,#35918,#29962,.T.);
#45692=EDGE_CURVE('',#36514,#36513,#21165,.T.);
#45693=EDGE_CURVE('',#36515,#36516,#29963,.T.);
#45694=EDGE_CURVE('',#36515,#36514,#29964,.T.);
#45695=EDGE_CURVE('',#36516,#35917,#4574,.T.);
#45696=EDGE_CURVE('',#36385,#35916,#29965,.T.);
#45697=EDGE_CURVE('',#36384,#35917,#29966,.T.);
#45698=EDGE_CURVE('',#36517,#35915,#29967,.T.);
#45699=EDGE_CURVE('',#36517,#36385,#1865,.T.);
#45700=EDGE_CURVE('',#36518,#35914,#29968,.T.);
#45701=EDGE_CURVE('',#36518,#36517,#1139,.T.);
#45702=EDGE_CURVE('',#35913,#36519,#29969,.T.);
#45703=EDGE_CURVE('',#36519,#36518,#1140,.T.);
#45704=EDGE_CURVE('',#35912,#36520,#29970,.T.);
#45705=EDGE_CURVE('',#36520,#36519,#21166,.T.);
#45706=EDGE_CURVE('',#35920,#36520,#4575,.T.);
#45707=EDGE_CURVE('',#36521,#36520,#4576,.T.);
#45708=EDGE_CURVE('',#36521,#35921,#4577,.T.);
#45709=EDGE_CURVE('',#35921,#35931,#29971,.T.);
#45710=EDGE_CURVE('',#36521,#35930,#29972,.T.);
#45711=EDGE_CURVE('',#36522,#35929,#29973,.T.);
#45712=EDGE_CURVE('',#36522,#36521,#21167,.T.);
#45713=EDGE_CURVE('',#36523,#35928,#29974,.T.);
#45714=EDGE_CURVE('',#36523,#36522,#4578,.T.);
#45715=EDGE_CURVE('',#36524,#35927,#29975,.T.);
#45716=EDGE_CURVE('',#36524,#36523,#1141,.T.);
#45717=EDGE_CURVE('',#36386,#35926,#29976,.T.);
#45718=EDGE_CURVE('',#36386,#36524,#1866,.T.);
#45719=EDGE_CURVE('',#36387,#35925,#29977,.T.);
#45720=EDGE_CURVE('',#36525,#35924,#29978,.T.);
#45721=EDGE_CURVE('',#36525,#36526,#4579,.T.);
#45722=EDGE_CURVE('',#35925,#36526,#4580,.T.);
#45723=EDGE_CURVE('',#35932,#36525,#21168,.T.);
#45724=EDGE_CURVE('',#36527,#35933,#21169,.T.);
#45725=EDGE_CURVE('',#36525,#36527,#4581,.T.);
#45726=EDGE_CURVE('',#36527,#35936,#29979,.T.);
#45727=EDGE_CURVE('',#35938,#35944,#29980,.T.);
#45728=EDGE_CURVE('',#36528,#36527,#1142,.T.);
#45729=EDGE_CURVE('',#36528,#35937,#4582,.T.);
#45730=EDGE_CURVE('',#35937,#36390,#29981,.T.);
#45731=EDGE_CURVE('',#35943,#36391,#29982,.T.);
#45732=EDGE_CURVE('',#35942,#36529,#29983,.T.);
#45733=EDGE_CURVE('',#36529,#36391,#1867,.T.);
#45734=EDGE_CURVE('',#35941,#36530,#29984,.T.);
#45735=EDGE_CURVE('',#36530,#36529,#1143,.T.);
#45736=EDGE_CURVE('',#35940,#36531,#29985,.T.);
#45737=EDGE_CURVE('',#36531,#36530,#4583,.T.);
#45738=EDGE_CURVE('',#35939,#36532,#29986,.T.);
#45739=EDGE_CURVE('',#36532,#36531,#21170,.T.);
#45740=EDGE_CURVE('',#35944,#36532,#4584,.T.);
#45741=EDGE_CURVE('',#36533,#36532,#4585,.T.);
#45742=EDGE_CURVE('',#36533,#35945,#1868,.T.);
#45743=EDGE_CURVE('',#35945,#35955,#29987,.T.);
#45744=EDGE_CURVE('',#36533,#35954,#29988,.T.);
#45745=EDGE_CURVE('',#36534,#35953,#29989,.T.);
#45746=EDGE_CURVE('',#36534,#36533,#21171,.T.);
#45747=EDGE_CURVE('',#36535,#35952,#29990,.T.);
#45748=EDGE_CURVE('',#36535,#36534,#1869,.T.);
#45749=EDGE_CURVE('',#36536,#35951,#29991,.T.);
#45750=EDGE_CURVE('',#36536,#36535,#4586,.T.);
#45751=EDGE_CURVE('',#36392,#35950,#29992,.T.);
#45752=EDGE_CURVE('',#36392,#36536,#29993,.T.);
#45753=EDGE_CURVE('',#36393,#35949,#29994,.T.);
#45754=EDGE_CURVE('',#36537,#35948,#29995,.T.);
#45755=EDGE_CURVE('',#36537,#36538,#1144,.T.);
#45756=EDGE_CURVE('',#35949,#36538,#4587,.T.);
#45757=EDGE_CURVE('',#35956,#36537,#21172,.T.);
#45758=EDGE_CURVE('',#36539,#35957,#21173,.T.);
#45759=EDGE_CURVE('',#36537,#36539,#29996,.T.);
#45760=EDGE_CURVE('',#35967,#36539,#29997,.T.);
#45761=EDGE_CURVE('',#35960,#35968,#29998,.T.);
#45762=EDGE_CURVE('',#36540,#36539,#1145,.T.);
#45763=EDGE_CURVE('',#36540,#35966,#4588,.T.);
#45764=EDGE_CURVE('',#35966,#36396,#29999,.T.);
#45765=EDGE_CURVE('',#35965,#36397,#30000,.T.);
#45766=EDGE_CURVE('',#35964,#36541,#30001,.T.);
#45767=EDGE_CURVE('',#36541,#36397,#30002,.T.);
#45768=EDGE_CURVE('',#35963,#36542,#30003,.T.);
#45769=EDGE_CURVE('',#36542,#36541,#4589,.T.);
#45770=EDGE_CURVE('',#35962,#36543,#30004,.T.);
#45771=EDGE_CURVE('',#36543,#36542,#1870,.T.);
#45772=EDGE_CURVE('',#35961,#36544,#30005,.T.);
#45773=EDGE_CURVE('',#36544,#36543,#21174,.T.);
#45774=EDGE_CURVE('',#35968,#36544,#1871,.T.);
#45775=EDGE_CURVE('',#36545,#36544,#4590,.T.);
#45776=EDGE_CURVE('',#36545,#35969,#4591,.T.);
#45777=EDGE_CURVE('',#35969,#35979,#30006,.T.);
#45778=EDGE_CURVE('',#36545,#35978,#30007,.T.);
#45779=EDGE_CURVE('',#36546,#35977,#30008,.T.);
#45780=EDGE_CURVE('',#36546,#36545,#21175,.T.);
#45781=EDGE_CURVE('',#36547,#35976,#30009,.T.);
#45782=EDGE_CURVE('',#36547,#36546,#4592,.T.);
#45783=EDGE_CURVE('',#36548,#35975,#30010,.T.);
#45784=EDGE_CURVE('',#36548,#36547,#1146,.T.);
#45785=EDGE_CURVE('',#36398,#35974,#30011,.T.);
#45786=EDGE_CURVE('',#36398,#36548,#1872,.T.);
#45787=EDGE_CURVE('',#36399,#35973,#30012,.T.);
#45788=EDGE_CURVE('',#36549,#35972,#30013,.T.);
#45789=EDGE_CURVE('',#36549,#36550,#4593,.T.);
#45790=EDGE_CURVE('',#35973,#36550,#4594,.T.);
#45791=EDGE_CURVE('',#35980,#36549,#21176,.T.);
#45792=EDGE_CURVE('',#36551,#35981,#21177,.T.);
#45793=EDGE_CURVE('',#36549,#36551,#4595,.T.);
#45794=EDGE_CURVE('',#35991,#36551,#30014,.T.);
#45795=EDGE_CURVE('',#35984,#35992,#30015,.T.);
#45796=EDGE_CURVE('',#36552,#36551,#4596,.T.);
#45797=EDGE_CURVE('',#36552,#35990,#4597,.T.);
#45798=EDGE_CURVE('',#35990,#36402,#30016,.T.);
#45799=EDGE_CURVE('',#35989,#36403,#30017,.T.);
#45800=EDGE_CURVE('',#35988,#36553,#30018,.T.);
#45801=EDGE_CURVE('',#36553,#36403,#1873,.T.);
#45802=EDGE_CURVE('',#35987,#36554,#30019,.T.);
#45803=EDGE_CURVE('',#36554,#36553,#1147,.T.);
#45804=EDGE_CURVE('',#35986,#36555,#30020,.T.);
#45805=EDGE_CURVE('',#36555,#36554,#4598,.T.);
#45806=EDGE_CURVE('',#35985,#36556,#30021,.T.);
#45807=EDGE_CURVE('',#36556,#36555,#21178,.T.);
#45808=EDGE_CURVE('',#35992,#36556,#4599,.T.);
#45809=EDGE_CURVE('',#36557,#36556,#4600,.T.);
#45810=EDGE_CURVE('',#36557,#35993,#1148,.T.);
#45811=EDGE_CURVE('',#36004,#35993,#30022,.T.);
#45812=EDGE_CURVE('',#36557,#36003,#30023,.T.);
#45813=EDGE_CURVE('',#36558,#36002,#30024,.T.);
#45814=EDGE_CURVE('',#36558,#36557,#21179,.T.);
#45815=EDGE_CURVE('',#36559,#36001,#30025,.T.);
#45816=EDGE_CURVE('',#36559,#36558,#4601,.T.);
#45817=EDGE_CURVE('',#36560,#36000,#30026,.T.);
#45818=EDGE_CURVE('',#36560,#36559,#4602,.T.);
#45819=EDGE_CURVE('',#36404,#35999,#30027,.T.);
#45820=EDGE_CURVE('',#36404,#36560,#1874,.T.);
#45821=EDGE_CURVE('',#36405,#35998,#30028,.T.);
#45822=EDGE_CURVE('',#36561,#35997,#30029,.T.);
#45823=EDGE_CURVE('',#36561,#36562,#30030,.T.);
#45824=EDGE_CURVE('',#36562,#36563,#30031,.T.);
#45825=EDGE_CURVE('',#35998,#36563,#4603,.T.);
#45826=EDGE_CURVE('',#36564,#35996,#30032,.T.);
#45827=EDGE_CURVE('',#36564,#36561,#21180,.T.);
#45828=EDGE_CURVE('',#36005,#36564,#30033,.T.);
#45829=EDGE_CURVE('',#36565,#36006,#30034,.T.);
#45830=EDGE_CURVE('',#36565,#36564,#21181,.T.);
#45831=EDGE_CURVE('',#36565,#36018,#30035,.T.);
#45832=EDGE_CURVE('',#36009,#36019,#30036,.T.);
#45833=EDGE_CURVE('',#36566,#36017,#30037,.T.);
#45834=EDGE_CURVE('',#36566,#36565,#21182,.T.);
#45835=EDGE_CURVE('',#36567,#36016,#30038,.T.);
#45836=EDGE_CURVE('',#36567,#36566,#30039,.T.);
#45837=EDGE_CURVE('',#36568,#36567,#21183,.T.);
#45838=EDGE_CURVE('',#36568,#36015,#4604,.T.);
#45839=EDGE_CURVE('',#36410,#36014,#30040,.T.);
#45840=EDGE_CURVE('',#36409,#36015,#30041,.T.);
#45841=EDGE_CURVE('',#36569,#36013,#30042,.T.);
#45842=EDGE_CURVE('',#36569,#36410,#1875,.T.);
#45843=EDGE_CURVE('',#36570,#36012,#30043,.T.);
#45844=EDGE_CURVE('',#36570,#36569,#4605,.T.);
#45845=EDGE_CURVE('',#36011,#36571,#30044,.T.);
#45846=EDGE_CURVE('',#36571,#36570,#4606,.T.);
#45847=EDGE_CURVE('',#36010,#36572,#30045,.T.);
#45848=EDGE_CURVE('',#36572,#36571,#21184,.T.);
#45849=EDGE_CURVE('',#36019,#36572,#4607,.T.);
#45850=EDGE_CURVE('',#36573,#36572,#4608,.T.);
#45851=EDGE_CURVE('',#36573,#36020,#4609,.T.);
#45852=EDGE_CURVE('',#36027,#36020,#30046,.T.);
#45853=EDGE_CURVE('',#36022,#36574,#30047,.T.);
#45854=EDGE_CURVE('',#36023,#36411,#30048,.T.);
#45855=EDGE_CURVE('',#36411,#36574,#1876,.T.);
#45856=EDGE_CURVE('',#36031,#36412,#30049,.T.);
#45857=EDGE_CURVE('',#36575,#36030,#30050,.T.);
#45858=EDGE_CURVE('',#36575,#36576,#21185,.T.);
#45859=EDGE_CURVE('',#36031,#36576,#4610,.T.);
#45860=EDGE_CURVE('',#36577,#36029,#30051,.T.);
#45861=EDGE_CURVE('',#36577,#36575,#30052,.T.);
#45862=EDGE_CURVE('',#36494,#36577,#21186,.T.);
#45863=EDGE_CURVE('',#36026,#36573,#30053,.T.);
#45864=EDGE_CURVE('',#36025,#36578,#30054,.T.);
#45865=EDGE_CURVE('',#36578,#36573,#21187,.T.);
#45866=EDGE_CURVE('',#36024,#36579,#30055,.T.);
#45867=EDGE_CURVE('',#36579,#36578,#4611,.T.);
#45868=EDGE_CURVE('',#36574,#36579,#4612,.T.);
#45869=EDGE_CURVE('',#36580,#36581,#4613,.T.);
#45870=EDGE_CURVE('',#36032,#36581,#30056,.T.);
#45871=EDGE_CURVE('',#36580,#36033,#4614,.T.);
#45872=EDGE_CURVE('',#36033,#36045,#30057,.T.);
#45873=EDGE_CURVE('',#36106,#36034,#30058,.T.);
#45874=EDGE_CURVE('',#36581,#36582,#30059,.T.);
#45875=EDGE_CURVE('',#36034,#36582,#4615,.T.);
#45876=EDGE_CURVE('',#36037,#36583,#30060,.T.);
#45877=EDGE_CURVE('',#36038,#36584,#30061,.T.);
#45878=EDGE_CURVE('',#36584,#36443,#30062,.T.);
#45879=EDGE_CURVE('',#36443,#36583,#4616,.T.);
#45880=EDGE_CURVE('',#36050,#36444,#30063,.T.);
#45881=EDGE_CURVE('',#36585,#36049,#30064,.T.);
#45882=EDGE_CURVE('',#36585,#36586,#21188,.T.);
#45883=EDGE_CURVE('',#36050,#36586,#4617,.T.);
#45884=EDGE_CURVE('',#36587,#36048,#30065,.T.);
#45885=EDGE_CURVE('',#36587,#36585,#30066,.T.);
#45886=EDGE_CURVE('',#36588,#36047,#30067,.T.);
#45887=EDGE_CURVE('',#36588,#36587,#21189,.T.);
#45888=EDGE_CURVE('',#36051,#36588,#30068,.T.);
#45889=EDGE_CURVE('',#36580,#36044,#30069,.T.);
#45890=EDGE_CURVE('',#36589,#36043,#30070,.T.);
#45891=EDGE_CURVE('',#36589,#36580,#4618,.T.);
#45892=EDGE_CURVE('',#36042,#36590,#30071,.T.);
#45893=EDGE_CURVE('',#36590,#36589,#21190,.T.);
#45894=EDGE_CURVE('',#36041,#36591,#30072,.T.);
#45895=EDGE_CURVE('',#36591,#36590,#4619,.T.);
#45896=EDGE_CURVE('',#36040,#36592,#30073,.T.);
#45897=EDGE_CURVE('',#36592,#36591,#4620,.T.);
#45898=EDGE_CURVE('',#36039,#36593,#30074,.T.);
#45899=EDGE_CURVE('',#36593,#36592,#1877,.T.);
#45900=EDGE_CURVE('',#36583,#36593,#21191,.T.);
#45901=EDGE_CURVE('',#36594,#36588,#21192,.T.);
#45902=EDGE_CURVE('',#36594,#36052,#30075,.T.);
#45903=EDGE_CURVE('',#36061,#36594,#30076,.T.);
#45904=EDGE_CURVE('',#36066,#36454,#30077,.T.);
#45905=EDGE_CURVE('',#36261,#36065,#30078,.T.);
#45906=EDGE_CURVE('',#36066,#36260,#30079,.T.);
#45907=EDGE_CURVE('',#36333,#36064,#30080,.T.);
#45908=EDGE_CURVE('',#36333,#36595,#21193,.T.);
#45909=EDGE_CURVE('',#36595,#36065,#30081,.T.);
#45910=EDGE_CURVE('',#36060,#36596,#30082,.T.);
#45911=EDGE_CURVE('',#36596,#36594,#21194,.T.);
#45912=EDGE_CURVE('',#36059,#36597,#30083,.T.);
#45913=EDGE_CURVE('',#36597,#36596,#30084,.T.);
#45914=EDGE_CURVE('',#36598,#36597,#21195,.T.);
#45915=EDGE_CURVE('',#36598,#36058,#4621,.T.);
#45916=EDGE_CURVE('',#36058,#36447,#30085,.T.);
#45917=EDGE_CURVE('',#36057,#36435,#30086,.T.);
#45918=EDGE_CURVE('',#36056,#36453,#30087,.T.);
#45919=EDGE_CURVE('',#36453,#36435,#4622,.T.);
#45920=EDGE_CURVE('',#36072,#36081,#30088,.T.);
#45921=EDGE_CURVE('',#36078,#36472,#30089,.T.);
#45922=EDGE_CURVE('',#36077,#36599,#30090,.T.);
#45923=EDGE_CURVE('',#36599,#36472,#30091,.T.);
#45924=EDGE_CURVE('',#36076,#36600,#30092,.T.);
#45925=EDGE_CURVE('',#36600,#36599,#1149,.T.);
#45926=EDGE_CURVE('',#36075,#36601,#30093,.T.);
#45927=EDGE_CURVE('',#36601,#36600,#4623,.T.);
#45928=EDGE_CURVE('',#36074,#36602,#30094,.T.);
#45929=EDGE_CURVE('',#36602,#36601,#21196,.T.);
#45930=EDGE_CURVE('',#36073,#36603,#30095,.T.);
#45931=EDGE_CURVE('',#36603,#36602,#4624,.T.);
#45932=EDGE_CURVE('',#36081,#36603,#1150,.T.);
#45933=EDGE_CURVE('',#36604,#36070,#30096,.T.);
#45934=EDGE_CURVE('',#36604,#36334,#21197,.T.);
#45935=EDGE_CURVE('',#36474,#36604,#30097,.T.);
#45936=EDGE_CURVE('',#36603,#36605,#4625,.T.);
#45937=EDGE_CURVE('',#36605,#36080,#1151,.T.);
#45938=EDGE_CURVE('',#36080,#36097,#30098,.T.);
#45939=EDGE_CURVE('',#36082,#36098,#30099,.T.);
#45940=EDGE_CURVE('',#36605,#36096,#30100,.T.);
#45941=EDGE_CURVE('',#36606,#36095,#30101,.T.);
#45942=EDGE_CURVE('',#36606,#36605,#4626,.T.);
#45943=EDGE_CURVE('',#36607,#36094,#30102,.T.);
#45944=EDGE_CURVE('',#36607,#36606,#21198,.T.);
#45945=EDGE_CURVE('',#36608,#36093,#30103,.T.);
#45946=EDGE_CURVE('',#36608,#36607,#4627,.T.);
#45947=EDGE_CURVE('',#36609,#36092,#30104,.T.);
#45948=EDGE_CURVE('',#36609,#36608,#1152,.T.);
#45949=EDGE_CURVE('',#36610,#36091,#30105,.T.);
#45950=EDGE_CURVE('',#36610,#36609,#4628,.T.);
#45951=EDGE_CURVE('',#36611,#36090,#30106,.T.);
#45952=EDGE_CURVE('',#36611,#36610,#21199,.T.);
#45953=EDGE_CURVE('',#36437,#36089,#30107,.T.);
#45954=EDGE_CURVE('',#36437,#36611,#4629,.T.);
#45955=EDGE_CURVE('',#36438,#36088,#30108,.T.);
#45956=EDGE_CURVE('',#36612,#36087,#30109,.T.);
#45957=EDGE_CURVE('',#36612,#36613,#21200,.T.);
#45958=EDGE_CURVE('',#36088,#36613,#4630,.T.);
#45959=EDGE_CURVE('',#36614,#36086,#30110,.T.);
#45960=EDGE_CURVE('',#36614,#36612,#30111,.T.);
#45961=EDGE_CURVE('',#36615,#36085,#30112,.T.);
#45962=EDGE_CURVE('',#36615,#36614,#21201,.T.);
#45963=EDGE_CURVE('',#36099,#36615,#30113,.T.);
#45964=EDGE_CURVE('',#36616,#36100,#30114,.T.);
#45965=EDGE_CURVE('',#36616,#36615,#21202,.T.);
#45966=EDGE_CURVE('',#36616,#36105,#30115,.T.);
#45967=EDGE_CURVE('',#36617,#36618,#21203,.T.);
#45968=EDGE_CURVE('',#36618,#36102,#30116,.T.);
#45969=EDGE_CURVE('',#36617,#36103,#4631,.T.);
#45970=EDGE_CURVE('',#36103,#36441,#30117,.T.);
#45971=EDGE_CURVE('',#36115,#36442,#30118,.T.);
#45972=EDGE_CURVE('',#36114,#36619,#30119,.T.);
#45973=EDGE_CURVE('',#36619,#36442,#4632,.T.);
#45974=EDGE_CURVE('',#36113,#36620,#30120,.T.);
#45975=EDGE_CURVE('',#36620,#36619,#21204,.T.);
#45976=EDGE_CURVE('',#36112,#36621,#30121,.T.);
#45977=EDGE_CURVE('',#36621,#36620,#4633,.T.);
#45978=EDGE_CURVE('',#36111,#36622,#30122,.T.);
#45979=EDGE_CURVE('',#36622,#36621,#4634,.T.);
#45980=EDGE_CURVE('',#36110,#36623,#30123,.T.);
#45981=EDGE_CURVE('',#36623,#36622,#4635,.T.);
#45982=EDGE_CURVE('',#36109,#36624,#30124,.T.);
#45983=EDGE_CURVE('',#36624,#36623,#21205,.T.);
#45984=EDGE_CURVE('',#36108,#36625,#30125,.T.);
#45985=EDGE_CURVE('',#36625,#36624,#4636,.T.);
#45986=EDGE_CURVE('',#36107,#36582,#30126,.T.);
#45987=EDGE_CURVE('',#36582,#36625,#4637,.T.);
#45988=EDGE_CURVE('',#36626,#36104,#30127,.T.);
#45989=EDGE_CURVE('',#36626,#36616,#21206,.T.);
#45990=EDGE_CURVE('',#36618,#36626,#30128,.T.);
#45991=EDGE_CURVE('',#36627,#36628,#30129,.T.);
#45992=EDGE_CURVE('',#36116,#36628,#4638,.T.);
#45993=EDGE_CURVE('',#36627,#36117,#4639,.T.);
#45994=EDGE_CURVE('',#36126,#36117,#30130,.T.);
#45995=EDGE_CURVE('',#36116,#36146,#30131,.T.);
#45996=EDGE_CURVE('',#36125,#36627,#30132,.T.);
#45997=EDGE_CURVE('',#36124,#36629,#30133,.T.);
#45998=EDGE_CURVE('',#36629,#36627,#4640,.T.);
#45999=EDGE_CURVE('',#36123,#36348,#30134,.T.);
#46000=EDGE_CURVE('',#36348,#36629,#4641,.T.);
#46001=EDGE_CURVE('',#36127,#36346,#30135,.T.);
#46002=EDGE_CURVE('',#36345,#36128,#30136,.T.);
#46003=EDGE_CURVE('',#36343,#36133,#30137,.T.);
#46004=EDGE_CURVE('',#36492,#36132,#30138,.T.);
#46005=EDGE_CURVE('',#36492,#36343,#4642,.T.);
#46006=EDGE_CURVE('',#36339,#36328,#21207,.T.);
#46007=EDGE_CURVE('',#36337,#36140,#30139,.T.);
#46008=EDGE_CURVE('',#36142,#36337,#30140,.T.);
#46009=EDGE_CURVE('',#36336,#36143,#30141,.T.);
#46010=EDGE_CURVE('',#36347,#36149,#30142,.T.);
#46011=EDGE_CURVE('',#36630,#36148,#30143,.T.);
#46012=EDGE_CURVE('',#36630,#36347,#4643,.T.);
#46013=EDGE_CURVE('',#36628,#36147,#30144,.T.);
#46014=EDGE_CURVE('',#36628,#36630,#4644,.T.);
#46015=EDGE_CURVE('',#36631,#36632,#30145,.T.);
#46016=EDGE_CURVE('',#36151,#36632,#4645,.T.);
#46017=EDGE_CURVE('',#36631,#36152,#4646,.T.);
#46018=EDGE_CURVE('',#36164,#36152,#30146,.T.);
#46019=EDGE_CURVE('',#36229,#36151,#30147,.T.);
#46020=EDGE_CURVE('',#36155,#36633,#30148,.T.);
#46021=EDGE_CURVE('',#36156,#36634,#30149,.T.);
#46022=EDGE_CURVE('',#36634,#36366,#30150,.T.);
#46023=EDGE_CURVE('',#36366,#36633,#4647,.T.);
#46024=EDGE_CURVE('',#36169,#36367,#30151,.T.);
#46025=EDGE_CURVE('',#36635,#36168,#30152,.T.);
#46026=EDGE_CURVE('',#36635,#36636,#21208,.T.);
#46027=EDGE_CURVE('',#36169,#36636,#4648,.T.);
#46028=EDGE_CURVE('',#36637,#36167,#30153,.T.);
#46029=EDGE_CURVE('',#36637,#36635,#30154,.T.);
#46030=EDGE_CURVE('',#36638,#36166,#30155,.T.);
#46031=EDGE_CURVE('',#36638,#36637,#21209,.T.);
#46032=EDGE_CURVE('',#36170,#36638,#30156,.T.);
#46033=EDGE_CURVE('',#36163,#36631,#30157,.T.);
#46034=EDGE_CURVE('',#36162,#36639,#30158,.T.);
#46035=EDGE_CURVE('',#36639,#36631,#4649,.T.);
#46036=EDGE_CURVE('',#36161,#36640,#30159,.T.);
#46037=EDGE_CURVE('',#36640,#36639,#4650,.T.);
#46038=EDGE_CURVE('',#36160,#36641,#30160,.T.);
#46039=EDGE_CURVE('',#36641,#36640,#21210,.T.);
#46040=EDGE_CURVE('',#36159,#36642,#30161,.T.);
#46041=EDGE_CURVE('',#36642,#36641,#4651,.T.);
#46042=EDGE_CURVE('',#36158,#36643,#30162,.T.);
#46043=EDGE_CURVE('',#36643,#36642,#4652,.T.);
#46044=EDGE_CURVE('',#36157,#36644,#30163,.T.);
#46045=EDGE_CURVE('',#36644,#36643,#4653,.T.);
#46046=EDGE_CURVE('',#36633,#36644,#21211,.T.);
#46047=EDGE_CURVE('',#36645,#36638,#21212,.T.);
#46048=EDGE_CURVE('',#36645,#36171,#30164,.T.);
#46049=EDGE_CURVE('',#36645,#36183,#30165,.T.);
#46050=EDGE_CURVE('',#36327,#36338,#21213,.T.);
#46051=EDGE_CURVE('',#36646,#36182,#30166,.T.);
#46052=EDGE_CURVE('',#36646,#36645,#21214,.T.);
#46053=EDGE_CURVE('',#36647,#36181,#30167,.T.);
#46054=EDGE_CURVE('',#36647,#36646,#30168,.T.);
#46055=EDGE_CURVE('',#36648,#36647,#21215,.T.);
#46056=EDGE_CURVE('',#36648,#36180,#4654,.T.);
#46057=EDGE_CURVE('',#36180,#36370,#30169,.T.);
#46058=EDGE_CURVE('',#36179,#36357,#30170,.T.);
#46059=EDGE_CURVE('',#36178,#36460,#30171,.T.);
#46060=EDGE_CURVE('',#36460,#36357,#4655,.T.);
#46061=EDGE_CURVE('',#36349,#36174,#30172,.T.);
#46062=EDGE_CURVE('',#36649,#36650,#4656,.T.);
#46063=EDGE_CURVE('',#36649,#36651,#21216,.T.);
#46064=EDGE_CURVE('',#36651,#36188,#30173,.T.);
#46065=EDGE_CURVE('',#36650,#36189,#4657,.T.);
#46066=EDGE_CURVE('',#36371,#36201,#30174,.T.);
#46067=EDGE_CURVE('',#36372,#36189,#30175,.T.);
#46068=EDGE_CURVE('',#36652,#36200,#30176,.T.);
#46069=EDGE_CURVE('',#36652,#36371,#4658,.T.);
#46070=EDGE_CURVE('',#36653,#36199,#30177,.T.);
#46071=EDGE_CURVE('',#36653,#36652,#30178,.T.);
#46072=EDGE_CURVE('',#36654,#36198,#30179,.T.);
#46073=EDGE_CURVE('',#36654,#36653,#4659,.T.);
#46074=EDGE_CURVE('',#36655,#36197,#30180,.T.);
#46075=EDGE_CURVE('',#36655,#36654,#4660,.T.);
#46076=EDGE_CURVE('',#36656,#36196,#30181,.T.);
#46077=EDGE_CURVE('',#36656,#36655,#21217,.T.);
#46078=EDGE_CURVE('',#36657,#36195,#30182,.T.);
#46079=EDGE_CURVE('',#36657,#36656,#4661,.T.);
#46080=EDGE_CURVE('',#36204,#36194,#30183,.T.);
#46081=EDGE_CURVE('',#36204,#36657,#1153,.T.);
#46082=EDGE_CURVE('',#36202,#36193,#30184,.T.);
#46083=EDGE_CURVE('',#36658,#36190,#30185,.T.);
#46084=EDGE_CURVE('',#36658,#36495,#21218,.T.);
#46085=EDGE_CURVE('',#36651,#36658,#30186,.T.);
#46086=EDGE_CURVE('',#36657,#36659,#4662,.T.);
#46087=EDGE_CURVE('',#36659,#36203,#4663,.T.);
#46088=EDGE_CURVE('',#36203,#36220,#30187,.T.);
#46089=EDGE_CURVE('',#36205,#36221,#30188,.T.);
#46090=EDGE_CURVE('',#36659,#36219,#30189,.T.);
#46091=EDGE_CURVE('',#36660,#36218,#30190,.T.);
#46092=EDGE_CURVE('',#36660,#36659,#4664,.T.);
#46093=EDGE_CURVE('',#36661,#36217,#30191,.T.);
#46094=EDGE_CURVE('',#36661,#36660,#21219,.T.);
#46095=EDGE_CURVE('',#36662,#36216,#30192,.T.);
#46096=EDGE_CURVE('',#36662,#36661,#4665,.T.);
#46097=EDGE_CURVE('',#36663,#36215,#30193,.T.);
#46098=EDGE_CURVE('',#36663,#36662,#4666,.T.);
#46099=EDGE_CURVE('',#36664,#36214,#30194,.T.);
#46100=EDGE_CURVE('',#36664,#36663,#4667,.T.);
#46101=EDGE_CURVE('',#36665,#36213,#30195,.T.);
#46102=EDGE_CURVE('',#36665,#36664,#21220,.T.);
#46103=EDGE_CURVE('',#36360,#36212,#30196,.T.);
#46104=EDGE_CURVE('',#36360,#36665,#4668,.T.);
#46105=EDGE_CURVE('',#36361,#36211,#30197,.T.);
#46106=EDGE_CURVE('',#36666,#36210,#30198,.T.);
#46107=EDGE_CURVE('',#36666,#36667,#21221,.T.);
#46108=EDGE_CURVE('',#36211,#36667,#4669,.T.);
#46109=EDGE_CURVE('',#36668,#36209,#30199,.T.);
#46110=EDGE_CURVE('',#36668,#36666,#30200,.T.);
#46111=EDGE_CURVE('',#36669,#36208,#30201,.T.);
#46112=EDGE_CURVE('',#36669,#36668,#21222,.T.);
#46113=EDGE_CURVE('',#36222,#36669,#30202,.T.);
#46114=EDGE_CURVE('',#36670,#36223,#30203,.T.);
#46115=EDGE_CURVE('',#36670,#36669,#21223,.T.);
#46116=EDGE_CURVE('',#36670,#36228,#30204,.T.);
#46117=EDGE_CURVE('',#36671,#36672,#21224,.T.);
#46118=EDGE_CURVE('',#36672,#36225,#30205,.T.);
#46119=EDGE_CURVE('',#36671,#36226,#4670,.T.);
#46120=EDGE_CURVE('',#36226,#36364,#30206,.T.);
#46121=EDGE_CURVE('',#36238,#36365,#30207,.T.);
#46122=EDGE_CURVE('',#36237,#36673,#30208,.T.);
#46123=EDGE_CURVE('',#36673,#36365,#4671,.T.);
#46124=EDGE_CURVE('',#36236,#36674,#30209,.T.);
#46125=EDGE_CURVE('',#36674,#36673,#21225,.T.);
#46126=EDGE_CURVE('',#36235,#36675,#30210,.T.);
#46127=EDGE_CURVE('',#36675,#36674,#4672,.T.);
#46128=EDGE_CURVE('',#36234,#36676,#30211,.T.);
#46129=EDGE_CURVE('',#36676,#36675,#4673,.T.);
#46130=EDGE_CURVE('',#36233,#36677,#30212,.T.);
#46131=EDGE_CURVE('',#36677,#36676,#4674,.T.);
#46132=EDGE_CURVE('',#36232,#36678,#30213,.T.);
#46133=EDGE_CURVE('',#36678,#36677,#21226,.T.);
#46134=EDGE_CURVE('',#36231,#36679,#30214,.T.);
#46135=EDGE_CURVE('',#36679,#36678,#4675,.T.);
#46136=EDGE_CURVE('',#36230,#36632,#30215,.T.);
#46137=EDGE_CURVE('',#36632,#36679,#4676,.T.);
#46138=EDGE_CURVE('',#36680,#36227,#30216,.T.);
#46139=EDGE_CURVE('',#36680,#36670,#21227,.T.);
#46140=EDGE_CURVE('',#36672,#36680,#30217,.T.);
#46141=EDGE_CURVE('',#36681,#36682,#4677,.T.);
#46142=EDGE_CURVE('',#36240,#36681,#4678,.T.);
#46143=EDGE_CURVE('',#36682,#36239,#4679,.T.);
#46144=EDGE_CURVE('',#36250,#36239,#30218,.T.);
#46145=EDGE_CURVE('',#36314,#36240,#30219,.T.);
#46146=EDGE_CURVE('',#36313,#36241,#30220,.T.);
#46147=EDGE_CURVE('',#36243,#36683,#30221,.T.);
#46148=EDGE_CURVE('',#36244,#36416,#30222,.T.);
#46149=EDGE_CURVE('',#36416,#36683,#4680,.T.);
#46150=EDGE_CURVE('',#36254,#36417,#30223,.T.);
#46151=EDGE_CURVE('',#36254,#36684,#4681,.T.);
#46152=EDGE_CURVE('',#36685,#36253,#30224,.T.);
#46153=EDGE_CURVE('',#36685,#36686,#21228,.T.);
#46154=EDGE_CURVE('',#36684,#36686,#1878,.T.);
#46155=EDGE_CURVE('',#36687,#36252,#30225,.T.);
#46156=EDGE_CURVE('',#36687,#36685,#30226,.T.);
#46157=EDGE_CURVE('',#36496,#36687,#21229,.T.);
#46158=EDGE_CURVE('',#36249,#36682,#30227,.T.);
#46159=EDGE_CURVE('',#36248,#36688,#30228,.T.);
#46160=EDGE_CURVE('',#36688,#36682,#4682,.T.);
#46161=EDGE_CURVE('',#36247,#36689,#30229,.T.);
#46162=EDGE_CURVE('',#36689,#36688,#21230,.T.);
#46163=EDGE_CURVE('',#36246,#36690,#30230,.T.);
#46164=EDGE_CURVE('',#36690,#36689,#4683,.T.);
#46165=EDGE_CURVE('',#36245,#36691,#30231,.T.);
#46166=EDGE_CURVE('',#36691,#36690,#1154,.T.);
#46167=EDGE_CURVE('',#36683,#36691,#1879,.T.);
#46168=EDGE_CURVE('',#36256,#36449,#30232,.T.);
#46169=EDGE_CURVE('',#36257,#36427,#30233,.T.);
#46170=EDGE_CURVE('',#36427,#36449,#4684,.T.);
#46171=EDGE_CURVE('',#36268,#36428,#30234,.T.);
#46172=EDGE_CURVE('',#36267,#36692,#30235,.T.);
#46173=EDGE_CURVE('',#36692,#36693,#21231,.T.);
#46174=EDGE_CURVE('',#36268,#36693,#4685,.T.);
#46175=EDGE_CURVE('',#36266,#36694,#30236,.T.);
#46176=EDGE_CURVE('',#36694,#36692,#30237,.T.);
#46177=EDGE_CURVE('',#36265,#36695,#30238,.T.);
#46178=EDGE_CURVE('',#36695,#36694,#21232,.T.);
#46179=EDGE_CURVE('',#36269,#36695,#30239,.T.);
#46180=EDGE_CURVE('',#36332,#36262,#30240,.T.);
#46181=EDGE_CURVE('',#36696,#36261,#30241,.T.);
#46182=EDGE_CURVE('',#36696,#36332,#21233,.T.);
#46183=EDGE_CURVE('',#36260,#36455,#30242,.T.);
#46184=EDGE_CURVE('',#36697,#36270,#30243,.T.);
#46185=EDGE_CURVE('',#36697,#36695,#21234,.T.);
#46186=EDGE_CURVE('',#36697,#36275,#30244,.T.);
#46187=EDGE_CURVE('',#36698,#36699,#21235,.T.);
#46188=EDGE_CURVE('',#36699,#36272,#30245,.T.);
#46189=EDGE_CURVE('',#36698,#36273,#4686,.T.);
#46190=EDGE_CURVE('',#36700,#36419,#30246,.T.);
#46191=EDGE_CURVE('',#36273,#36431,#30247,.T.);
#46192=EDGE_CURVE('',#36286,#36700,#30248,.T.);
#46193=EDGE_CURVE('',#36285,#36701,#30249,.T.);
#46194=EDGE_CURVE('',#36701,#36419,#4687,.T.);
#46195=EDGE_CURVE('',#36284,#36702,#30250,.T.);
#46196=EDGE_CURVE('',#36702,#36701,#21236,.T.);
#46197=EDGE_CURVE('',#36283,#36703,#30251,.T.);
#46198=EDGE_CURVE('',#36703,#36702,#4688,.T.);
#46199=EDGE_CURVE('',#36282,#36704,#30252,.T.);
#46200=EDGE_CURVE('',#36704,#36703,#4689,.T.);
#46201=EDGE_CURVE('',#36705,#36281,#30253,.T.);
#46202=EDGE_CURVE('',#36705,#36704,#4690,.T.);
#46203=EDGE_CURVE('',#36706,#36280,#30254,.T.);
#46204=EDGE_CURVE('',#36706,#36705,#21237,.T.);
#46205=EDGE_CURVE('',#36707,#36279,#30255,.T.);
#46206=EDGE_CURVE('',#36707,#36706,#4691,.T.);
#46207=EDGE_CURVE('',#36708,#36278,#30256,.T.);
#46208=EDGE_CURVE('',#36708,#36707,#4692,.T.);
#46209=EDGE_CURVE('',#36287,#36277,#30257,.T.);
#46210=EDGE_CURVE('',#36287,#36708,#4693,.T.);
#46211=EDGE_CURVE('',#36709,#36274,#30258,.T.);
#46212=EDGE_CURVE('',#36709,#36697,#21238,.T.);
#46213=EDGE_CURVE('',#36699,#36709,#30259,.T.);
#46214=EDGE_CURVE('',#36710,#36708,#30260,.T.);
#46215=EDGE_CURVE('',#36710,#36288,#4694,.T.);
#46216=EDGE_CURVE('',#36288,#36304,#30261,.T.);
#46217=EDGE_CURVE('',#36710,#36303,#30262,.T.);
#46218=EDGE_CURVE('',#36711,#36302,#30263,.T.);
#46219=EDGE_CURVE('',#36711,#36710,#4695,.T.);
#46220=EDGE_CURVE('',#36712,#36301,#30264,.T.);
#46221=EDGE_CURVE('',#36712,#36711,#4696,.T.);
#46222=EDGE_CURVE('',#36713,#36300,#30265,.T.);
#46223=EDGE_CURVE('',#36713,#36712,#21239,.T.);
#46224=EDGE_CURVE('',#36714,#36299,#30266,.T.);
#46225=EDGE_CURVE('',#36714,#36713,#4697,.T.);
#46226=EDGE_CURVE('',#36715,#36298,#30267,.T.);
#46227=EDGE_CURVE('',#36715,#36714,#4698,.T.);
#46228=EDGE_CURVE('',#36716,#36297,#30268,.T.);
#46229=EDGE_CURVE('',#36716,#36715,#4699,.T.);
#46230=EDGE_CURVE('',#36717,#36296,#30269,.T.);
#46231=EDGE_CURVE('',#36717,#36716,#21240,.T.);
#46232=EDGE_CURVE('',#36418,#36295,#30270,.T.);
#46233=EDGE_CURVE('',#36418,#36717,#4700,.T.);
#46234=EDGE_CURVE('',#36420,#36294,#30271,.T.);
#46235=EDGE_CURVE('',#36718,#36293,#30272,.T.);
#46236=EDGE_CURVE('',#36718,#36719,#21241,.T.);
#46237=EDGE_CURVE('',#36294,#36719,#4701,.T.);
#46238=EDGE_CURVE('',#36720,#36292,#30273,.T.);
#46239=EDGE_CURVE('',#36720,#36718,#30274,.T.);
#46240=EDGE_CURVE('',#36721,#36291,#30275,.T.);
#46241=EDGE_CURVE('',#36721,#36720,#21242,.T.);
#46242=EDGE_CURVE('',#36305,#36721,#30276,.T.);
#46243=EDGE_CURVE('',#36722,#36306,#30277,.T.);
#46244=EDGE_CURVE('',#36722,#36721,#21243,.T.);
#46245=EDGE_CURVE('',#36722,#36312,#30278,.T.);
#46246=EDGE_CURVE('',#36723,#36724,#21244,.T.);
#46247=EDGE_CURVE('',#36724,#36309,#30279,.T.);
#46248=EDGE_CURVE('',#36723,#36310,#4702,.T.);
#46249=EDGE_CURVE('',#36725,#36424,#30280,.T.);
#46250=EDGE_CURVE('',#36310,#36423,#30281,.T.);
#46251=EDGE_CURVE('',#36322,#36725,#30282,.T.);
#46252=EDGE_CURVE('',#36321,#36726,#30283,.T.);
#46253=EDGE_CURVE('',#36726,#36424,#4703,.T.);
#46254=EDGE_CURVE('',#36320,#36727,#30284,.T.);
#46255=EDGE_CURVE('',#36727,#36726,#21245,.T.);
#46256=EDGE_CURVE('',#36319,#36728,#30285,.T.);
#46257=EDGE_CURVE('',#36728,#36727,#4704,.T.);
#46258=EDGE_CURVE('',#36318,#36729,#30286,.T.);
#46259=EDGE_CURVE('',#36729,#36728,#4705,.T.);
#46260=EDGE_CURVE('',#36317,#36730,#30287,.T.);
#46261=EDGE_CURVE('',#36730,#36729,#4706,.T.);
#46262=EDGE_CURVE('',#36316,#36731,#30288,.T.);
#46263=EDGE_CURVE('',#36731,#36730,#21246,.T.);
#46264=EDGE_CURVE('',#36315,#36681,#30289,.T.);
#46265=EDGE_CURVE('',#36681,#36731,#4707,.T.);
#46266=EDGE_CURVE('',#36732,#36311,#30290,.T.);
#46267=EDGE_CURVE('',#36732,#36722,#21247,.T.);
#46268=EDGE_CURVE('',#36724,#36732,#30291,.T.);
#46269=EDGE_CURVE('',#36595,#36696,#30292,.T.);
#46270=EDGE_CURVE('',#36491,#36604,#21248,.T.);
#46271=EDGE_CURVE('',#36630,#36629,#4708,.T.);
#46272=EDGE_CURVE('',#36456,#36353,#30293,.T.);
#46273=EDGE_CURVE('',#36457,#36354,#30294,.T.);
#46274=EDGE_CURVE('',#36458,#36355,#30295,.T.);
#46275=EDGE_CURVE('',#36459,#36356,#30296,.T.);
#46276=EDGE_CURVE('',#36648,#36369,#30297,.T.);
#46277=EDGE_CURVE('',#36636,#36368,#30298,.T.);
#46278=EDGE_CURVE('',#36636,#36648,#21249,.T.);
#46279=EDGE_CURVE('',#36673,#36633,#21250,.T.);
#46280=EDGE_CURVE('',#36671,#36363,#30299,.T.);
#46281=EDGE_CURVE('',#36667,#36362,#30300,.T.);
#46282=EDGE_CURVE('',#36667,#36671,#21251,.T.);
#46283=EDGE_CURVE('',#36359,#36733,#30301,.T.);
#46284=EDGE_CURVE('',#36733,#36665,#21252,.T.);
#46285=EDGE_CURVE('',#36358,#36734,#30302,.T.);
#46286=EDGE_CURVE('',#36734,#36733,#1155,.T.);
#46287=EDGE_CURVE('',#36650,#36373,#30303,.T.);
#46288=EDGE_CURVE('',#36652,#36734,#1156,.T.);
#46289=EDGE_CURVE('',#36649,#36414,#30304,.T.);
#46290=EDGE_CURVE('',#36576,#36413,#30305,.T.);
#46291=EDGE_CURVE('',#36576,#36649,#30306,.T.);
#46292=EDGE_CURVE('',#36569,#36574,#30307,.T.);
#46293=EDGE_CURVE('',#36408,#36568,#30308,.T.);
#46294=EDGE_CURVE('',#36407,#36735,#30309,.T.);
#46295=EDGE_CURVE('',#36735,#36568,#30310,.T.);
#46296=EDGE_CURVE('',#36406,#36563,#30311,.T.);
#46297=EDGE_CURVE('',#36563,#36735,#4709,.T.);
#46298=EDGE_CURVE('',#36553,#36560,#30312,.T.);
#46299=EDGE_CURVE('',#36552,#36401,#30313,.T.);
#46300=EDGE_CURVE('',#36550,#36400,#30314,.T.);
#46301=EDGE_CURVE('',#36550,#36552,#30315,.T.);
#46302=EDGE_CURVE('',#36541,#36548,#30316,.T.);
#46303=EDGE_CURVE('',#36540,#36395,#30317,.T.);
#46304=EDGE_CURVE('',#36538,#36394,#30318,.T.);
#46305=EDGE_CURVE('',#36538,#36540,#30319,.T.);
#46306=EDGE_CURVE('',#36529,#36536,#30320,.T.);
#46307=EDGE_CURVE('',#36528,#36389,#30321,.T.);
#46308=EDGE_CURVE('',#36526,#36388,#30322,.T.);
#46309=EDGE_CURVE('',#36526,#36528,#30323,.T.);
#46310=EDGE_CURVE('',#36517,#36524,#30324,.T.);
#46311=EDGE_CURVE('',#36383,#36516,#30325,.T.);
#46312=EDGE_CURVE('',#36382,#36736,#30326,.T.);
#46313=EDGE_CURVE('',#36736,#36516,#4710,.T.);
#46314=EDGE_CURVE('',#36381,#36510,#30327,.T.);
#46315=EDGE_CURVE('',#36510,#36736,#30328,.T.);
#46316=EDGE_CURVE('',#36500,#36508,#30329,.T.);
#46317=EDGE_CURVE('',#36498,#36376,#30330,.T.);
#46318=EDGE_CURVE('',#36686,#36375,#30331,.T.);
#46319=EDGE_CURVE('',#36686,#36498,#30332,.T.);
#46320=EDGE_CURVE('',#36684,#36374,#30333,.T.);
#46321=EDGE_CURVE('',#36737,#36415,#30334,.T.);
#46322=EDGE_CURVE('',#36737,#36683,#4711,.T.);
#46323=EDGE_CURVE('',#36701,#36717,#21253,.T.);
#46324=EDGE_CURVE('',#36698,#36430,#30335,.T.);
#46325=EDGE_CURVE('',#36693,#36429,#30336,.T.);
#46326=EDGE_CURVE('',#36693,#36698,#21254,.T.);
#46327=EDGE_CURVE('',#36448,#36426,#30337,.T.);
#46328=EDGE_CURVE('',#36738,#36425,#30338,.T.);
#46329=EDGE_CURVE('',#36738,#36737,#1157,.T.);
#46330=EDGE_CURVE('',#36726,#36738,#21255,.T.);
#46331=EDGE_CURVE('',#36723,#36422,#30339,.T.);
#46332=EDGE_CURVE('',#36719,#36421,#30340,.T.);
#46333=EDGE_CURVE('',#36719,#36723,#21256,.T.);
#46334=EDGE_CURVE('',#36450,#36432,#30341,.T.);
#46335=EDGE_CURVE('',#36451,#36433,#30342,.T.);
#46336=EDGE_CURVE('',#36452,#36434,#30343,.T.);
#46337=EDGE_CURVE('',#36598,#36446,#30344,.T.);
#46338=EDGE_CURVE('',#36586,#36445,#30345,.T.);
#46339=EDGE_CURVE('',#36586,#36598,#21257,.T.);
#46340=EDGE_CURVE('',#36619,#36583,#21258,.T.);
#46341=EDGE_CURVE('',#36617,#36440,#30346,.T.);
#46342=EDGE_CURVE('',#36613,#36439,#30347,.T.);
#46343=EDGE_CURVE('',#36613,#36617,#21259,.T.);
#46344=EDGE_CURVE('',#36436,#36739,#30348,.T.);
#46345=EDGE_CURVE('',#36739,#36611,#21260,.T.);
#46346=EDGE_CURVE('',#36473,#36739,#4712,.T.);
#46347=EDGE_CURVE('',#36486,#36490,#4713,.T.);
#46348=EDGE_CURVE('',#36483,#36488,#21261,.T.);
#46349=EDGE_CURVE('',#36479,#36482,#4714,.T.);
#46350=EDGE_CURVE('',#36475,#36478,#4715,.T.);
#46351=EDGE_CURVE('',#36610,#36739,#30349,.T.);
#46352=EDGE_CURVE('',#36599,#36609,#30350,.T.);
#46353=EDGE_CURVE('',#36577,#36658,#21262,.T.);
#46354=EDGE_CURVE('',#36687,#36504,#21263,.T.);
#46355=EDGE_CURVE('',#36499,#36685,#21264,.T.);
#46356=EDGE_CURVE('',#36507,#36501,#4716,.T.);
#46357=EDGE_CURVE('',#36502,#36506,#4717,.T.);
#46358=EDGE_CURVE('',#36515,#36509,#21265,.T.);
#46359=EDGE_CURVE('',#36736,#36515,#21266,.T.);
#46360=EDGE_CURVE('',#36511,#36514,#21267,.T.);
#46361=EDGE_CURVE('',#36523,#36518,#4718,.T.);
#46362=EDGE_CURVE('',#36519,#36522,#4719,.T.);
#46363=EDGE_CURVE('',#36535,#36530,#1158,.T.);
#46364=EDGE_CURVE('',#36531,#36534,#4720,.T.);
#46365=EDGE_CURVE('',#36547,#36542,#4721,.T.);
#46366=EDGE_CURVE('',#36543,#36546,#4722,.T.);
#46367=EDGE_CURVE('',#36559,#36554,#4723,.T.);
#46368=EDGE_CURVE('',#36555,#36558,#4724,.T.);
#46369=EDGE_CURVE('',#36562,#36735,#21268,.T.);
#46370=EDGE_CURVE('',#36561,#36566,#21269,.T.);
#46371=EDGE_CURVE('',#36567,#36562,#21270,.T.);
#46372=EDGE_CURVE('',#36579,#36570,#4725,.T.);
#46373=EDGE_CURVE('',#36571,#36578,#4726,.T.);
#46374=EDGE_CURVE('',#36651,#36575,#21271,.T.);
#46375=EDGE_CURVE('',#36589,#36624,#4727,.T.);
#46376=EDGE_CURVE('',#36625,#36581,#4728,.T.);
#46377=EDGE_CURVE('',#36597,#36585,#21272,.T.);
#46378=EDGE_CURVE('',#36587,#36596,#21273,.T.);
#46379=EDGE_CURVE('',#36623,#36590,#4729,.T.);
#46380=EDGE_CURVE('',#36740,#36591,#30351,.T.);
#46381=EDGE_CURVE('',#36740,#36622,#4730,.T.);
#46382=EDGE_CURVE('',#36740,#36592,#30352,.T.);
#46383=EDGE_CURVE('',#36593,#36620,#30353,.T.);
#46384=EDGE_CURVE('',#36621,#36740,#30354,.T.);
#46385=EDGE_CURVE('',#36608,#36600,#4731,.T.);
#46386=EDGE_CURVE('',#36601,#36607,#4732,.T.);
#46387=EDGE_CURVE('',#36606,#36602,#4733,.T.);
#46388=EDGE_CURVE('',#36618,#36612,#21274,.T.);
#46389=EDGE_CURVE('',#36614,#36626,#21275,.T.);
#46390=EDGE_CURVE('',#36679,#36639,#4734,.T.);
#46391=EDGE_CURVE('',#36647,#36635,#21276,.T.);
#46392=EDGE_CURVE('',#36637,#36646,#21277,.T.);
#46393=EDGE_CURVE('',#36640,#36678,#4735,.T.);
#46394=EDGE_CURVE('',#36677,#36641,#4736,.T.);
#46395=EDGE_CURVE('',#36642,#36676,#4737,.T.);
#46396=EDGE_CURVE('',#36675,#36643,#30355,.T.);
#46397=EDGE_CURVE('',#36644,#36674,#30356,.T.);
#46398=EDGE_CURVE('',#36664,#36733,#30357,.T.);
#46399=EDGE_CURVE('',#36653,#36663,#30358,.T.);
#46400=EDGE_CURVE('',#36662,#36654,#4738,.T.);
#46401=EDGE_CURVE('',#36655,#36661,#4739,.T.);
#46402=EDGE_CURVE('',#36660,#36656,#4740,.T.);
#46403=EDGE_CURVE('',#36672,#36666,#21278,.T.);
#46404=EDGE_CURVE('',#36668,#36680,#21279,.T.);
#46405=EDGE_CURVE('',#36688,#36731,#4741,.T.);
#46406=EDGE_CURVE('',#36730,#36689,#4742,.T.);
#46407=EDGE_CURVE('',#36690,#36729,#4743,.T.);
#46408=EDGE_CURVE('',#36728,#36691,#30359,.T.);
#46409=EDGE_CURVE('',#36738,#36727,#30360,.T.);
#46410=EDGE_CURVE('',#36699,#36692,#21280,.T.);
#46411=EDGE_CURVE('',#36694,#36709,#21281,.T.);
#46412=EDGE_CURVE('',#36716,#36702,#30361,.T.);
#46413=EDGE_CURVE('',#36703,#36715,#30362,.T.);
#46414=EDGE_CURVE('',#36714,#36704,#4744,.T.);
#46415=EDGE_CURVE('',#36705,#36713,#4745,.T.);
#46416=EDGE_CURVE('',#36712,#36706,#4746,.T.);
#46417=EDGE_CURVE('',#36707,#36711,#4747,.T.);
#46418=EDGE_CURVE('',#36724,#36718,#21282,.T.);
#46419=EDGE_CURVE('',#36720,#36732,#21283,.T.);
#46420=EDGE_CURVE('',#36741,#36742,#30363,.T.);
#46421=EDGE_CURVE('',#36742,#36743,#21284,.T.);
#46422=EDGE_CURVE('',#36743,#36741,#21285,.T.);
#46423=EDGE_CURVE('',#36744,#36745,#21286,.T.);
#46424=EDGE_CURVE('',#36745,#36746,#21287,.T.);
#46425=EDGE_CURVE('',#36746,#36747,#21288,.T.);
#46426=EDGE_CURVE('',#36747,#36744,#21289,.T.);
#46427=EDGE_CURVE('',#36746,#36748,#30364,.T.);
#46428=EDGE_CURVE('',#36749,#36748,#21290,.T.);
#46429=EDGE_CURVE('',#36749,#36747,#30365,.T.);
#46430=EDGE_CURVE('',#36748,#36750,#21291,.T.);
#46431=EDGE_CURVE('',#36750,#36751,#21292,.T.);
#46432=EDGE_CURVE('',#36751,#36749,#21293,.T.);
#46433=EDGE_CURVE('',#36752,#36753,#4748,.T.);
#46434=EDGE_CURVE('',#36753,#36754,#4749,.T.);
#46435=EDGE_CURVE('',#36754,#36755,#30366,.T.);
#46436=EDGE_CURVE('',#36755,#36752,#4750,.T.);
#46437=EDGE_CURVE('',#36756,#36757,#4751,.T.);
#46438=EDGE_CURVE('',#36756,#36753,#4752,.T.);
#46439=EDGE_CURVE('',#36752,#36757,#4753,.T.);
#46440=EDGE_CURVE('',#36758,#36759,#4754,.T.);
#46441=EDGE_CURVE('',#36759,#36756,#21294,.T.);
#46442=EDGE_CURVE('',#36757,#36758,#21295,.T.);
#46443=EDGE_CURVE('',#36760,#36761,#4755,.T.);
#46444=EDGE_CURVE('',#36760,#36759,#4756,.T.);
#46445=EDGE_CURVE('',#36758,#36761,#4757,.T.);
#46446=EDGE_CURVE('',#36762,#36763,#30367,.T.);
#46447=EDGE_CURVE('',#36763,#36760,#4758,.T.);
#46448=EDGE_CURVE('',#36761,#36762,#4759,.T.);
#46449=EDGE_CURVE('',#36764,#36765,#30368,.T.);
#46450=EDGE_CURVE('',#36764,#36763,#4760,.T.);
#46451=EDGE_CURVE('',#36762,#36765,#4761,.T.);
#46452=EDGE_CURVE('',#36766,#36767,#21296,.T.);
#46453=EDGE_CURVE('',#36767,#36764,#21297,.T.);
#46454=EDGE_CURVE('',#36765,#36766,#21298,.T.);
#46455=EDGE_CURVE('',#36768,#36769,#21299,.T.);
#46456=EDGE_CURVE('',#36769,#36770,#21300,.T.);
#46457=EDGE_CURVE('',#36770,#36771,#21301,.T.);
#46458=EDGE_CURVE('',#36771,#36768,#21302,.T.);
#46459=EDGE_CURVE('',#36770,#36772,#30369,.T.);
#46460=EDGE_CURVE('',#36773,#36772,#21303,.T.);
#46461=EDGE_CURVE('',#36773,#36771,#30370,.T.);
#46462=EDGE_CURVE('',#36772,#36774,#21304,.T.);
#46463=EDGE_CURVE('',#36774,#36775,#21305,.T.);
#46464=EDGE_CURVE('',#36775,#36773,#21306,.T.);
#46465=EDGE_CURVE('',#36776,#36777,#4762,.T.);
#46466=EDGE_CURVE('',#36777,#36778,#30371,.T.);
#46467=EDGE_CURVE('',#36779,#36778,#30372,.T.);
#46468=EDGE_CURVE('',#36779,#36742,#4763,.T.);
#46469=EDGE_CURVE('',#36741,#36776,#4764,.T.);
#46470=EDGE_CURVE('',#36778,#36780,#4765,.T.);
#46471=EDGE_CURVE('',#36780,#36781,#4766,.T.);
#46472=EDGE_CURVE('',#36781,#36779,#4767,.T.);
#46473=EDGE_CURVE('',#36780,#36782,#4768,.T.);
#46474=EDGE_CURVE('',#36783,#36782,#4769,.T.);
#46475=EDGE_CURVE('',#36783,#36781,#4770,.T.);
#46476=EDGE_CURVE('',#36782,#36784,#21307,.T.);
#46477=EDGE_CURVE('',#36784,#36785,#4771,.T.);
#46478=EDGE_CURVE('',#36785,#36783,#21308,.T.);
#46479=EDGE_CURVE('',#36784,#36786,#4772,.T.);
#46480=EDGE_CURVE('',#36787,#36786,#4773,.T.);
#46481=EDGE_CURVE('',#36787,#36785,#4774,.T.);
#46482=EDGE_CURVE('',#36788,#36789,#21309,.T.);
#46483=EDGE_CURVE('',#36789,#36790,#21310,.T.);
#46484=EDGE_CURVE('',#36790,#36791,#21311,.T.);
#46485=EDGE_CURVE('',#36791,#36788,#21312,.T.);
#46486=EDGE_CURVE('',#36790,#36792,#30373,.T.);
#46487=EDGE_CURVE('',#36793,#36792,#21313,.T.);
#46488=EDGE_CURVE('',#36793,#36791,#30374,.T.);
#46489=EDGE_CURVE('',#36792,#36794,#21314,.T.);
#46490=EDGE_CURVE('',#36794,#36795,#21315,.T.);
#46491=EDGE_CURVE('',#36795,#36793,#21316,.T.);
#46492=EDGE_CURVE('',#36796,#36797,#21317,.T.);
#46493=EDGE_CURVE('',#36797,#36798,#21318,.T.);
#46494=EDGE_CURVE('',#36798,#36796,#30375,.T.);
#46495=EDGE_CURVE('',#36799,#36800,#4775,.T.);
#46496=EDGE_CURVE('',#36799,#36801,#4776,.T.);
#46497=EDGE_CURVE('',#36802,#36801,#4777,.T.);
#46498=EDGE_CURVE('',#36802,#36800,#4778,.T.);
#46499=EDGE_CURVE('',#36803,#36804,#4779,.T.);
#46500=EDGE_CURVE('',#36804,#36799,#21319,.T.);
#46501=EDGE_CURVE('',#36800,#36803,#21320,.T.);
#46502=EDGE_CURVE('',#36805,#36806,#4780,.T.);
#46503=EDGE_CURVE('',#36805,#36804,#4781,.T.);
#46504=EDGE_CURVE('',#36803,#36806,#4782,.T.);
#46505=EDGE_CURVE('',#36807,#36808,#30376,.T.);
#46506=EDGE_CURVE('',#36808,#36805,#4783,.T.);
#46507=EDGE_CURVE('',#36806,#36807,#4784,.T.);
#46508=EDGE_CURVE('',#36798,#36808,#4785,.T.);
#46509=EDGE_CURVE('',#36807,#36809,#30377,.T.);
#46510=EDGE_CURVE('',#36809,#36810,#4786,.T.);
#46511=EDGE_CURVE('',#36810,#36796,#4787,.T.);
#46512=EDGE_CURVE('',#36811,#36812,#21321,.T.);
#46513=EDGE_CURVE('',#36812,#36813,#21322,.T.);
#46514=EDGE_CURVE('',#36813,#36814,#30378,.T.);
#46515=EDGE_CURVE('',#36814,#36811,#21323,.T.);
#46516=EDGE_CURVE('',#36813,#36815,#4788,.T.);
#46517=EDGE_CURVE('',#36816,#36815,#30379,.T.);
#46518=EDGE_CURVE('',#36816,#36814,#4789,.T.);
#46519=EDGE_CURVE('',#36815,#36817,#4790,.T.);
#46520=EDGE_CURVE('',#36817,#36818,#4791,.T.);
#46521=EDGE_CURVE('',#36818,#36816,#4792,.T.);
#46522=EDGE_CURVE('',#36817,#36819,#4793,.T.);
#46523=EDGE_CURVE('',#36820,#36819,#4794,.T.);
#46524=EDGE_CURVE('',#36820,#36818,#4795,.T.);
#46525=EDGE_CURVE('',#36819,#36821,#21324,.T.);
#46526=EDGE_CURVE('',#36821,#36822,#4796,.T.);
#46527=EDGE_CURVE('',#36822,#36820,#21325,.T.);
#46528=EDGE_CURVE('',#36821,#36823,#4797,.T.);
#46529=EDGE_CURVE('',#36824,#36823,#4798,.T.);
#46530=EDGE_CURVE('',#36824,#36822,#4799,.T.);
#46531=EDGE_CURVE('',#36825,#36826,#21326,.T.);
#46532=EDGE_CURVE('',#36826,#36827,#21327,.T.);
#46533=EDGE_CURVE('',#36827,#36828,#21328,.T.);
#46534=EDGE_CURVE('',#36828,#36825,#21329,.T.);
#46535=EDGE_CURVE('',#36829,#36830,#21330,.T.);
#46536=EDGE_CURVE('',#36829,#36826,#30380,.T.);
#46537=EDGE_CURVE('',#36825,#36830,#30381,.T.);
#46538=EDGE_CURVE('',#36830,#36831,#21331,.T.);
#46539=EDGE_CURVE('',#36831,#36832,#21332,.T.);
#46540=EDGE_CURVE('',#36832,#36829,#21333,.T.);
#46541=EDGE_CURVE('',#36823,#36833,#4800,.T.);
#46542=EDGE_CURVE('',#36833,#36834,#30382,.T.);
#46543=EDGE_CURVE('',#36834,#36824,#4801,.T.);
#46544=EDGE_CURVE('',#36835,#36836,#4802,.T.);
#46545=EDGE_CURVE('',#36836,#36837,#4803,.T.);
#46546=EDGE_CURVE('',#36837,#36838,#30383,.T.);
#46547=EDGE_CURVE('',#36838,#36835,#4804,.T.);
#46548=EDGE_CURVE('',#36839,#36840,#4805,.T.);
#46549=EDGE_CURVE('',#36840,#36841,#4806,.T.);
#46550=EDGE_CURVE('',#36841,#36839,#30384,.T.);
#46551=EDGE_CURVE('',#36842,#36843,#21334,.T.);
#46552=EDGE_CURVE('',#36843,#36844,#21335,.T.);
#46553=EDGE_CURVE('',#36844,#36845,#21336,.T.);
#46554=EDGE_CURVE('',#36845,#36842,#21337,.T.);
#46555=EDGE_CURVE('',#36844,#36846,#30385,.T.);
#46556=EDGE_CURVE('',#36847,#36846,#21338,.T.);
#46557=EDGE_CURVE('',#36847,#36845,#30386,.T.);
#46558=EDGE_CURVE('',#36846,#36848,#21339,.T.);
#46559=EDGE_CURVE('',#36848,#36849,#21340,.T.);
#46560=EDGE_CURVE('',#36849,#36847,#21341,.T.);
#46561=EDGE_CURVE('',#36850,#36851,#21342,.T.);
#46562=EDGE_CURVE('',#36851,#36852,#21343,.T.);
#46563=EDGE_CURVE('',#36852,#36850,#30387,.T.);
#46564=EDGE_CURVE('',#36853,#36854,#4807,.T.);
#46565=EDGE_CURVE('',#36853,#36855,#4808,.T.);
#46566=EDGE_CURVE('',#36856,#36855,#4809,.T.);
#46567=EDGE_CURVE('',#36856,#36854,#4810,.T.);
#46568=EDGE_CURVE('',#36857,#36858,#4811,.T.);
#46569=EDGE_CURVE('',#36858,#36853,#21344,.T.);
#46570=EDGE_CURVE('',#36854,#36857,#21345,.T.);
#46571=EDGE_CURVE('',#36859,#36860,#4812,.T.);
#46572=EDGE_CURVE('',#36859,#36858,#4813,.T.);
#46573=EDGE_CURVE('',#36857,#36860,#4814,.T.);
#46574=EDGE_CURVE('',#36861,#36862,#30388,.T.);
#46575=EDGE_CURVE('',#36862,#36859,#4815,.T.);
#46576=EDGE_CURVE('',#36860,#36861,#4816,.T.);
#46577=EDGE_CURVE('',#36863,#36864,#30389,.T.);
#46578=EDGE_CURVE('',#36865,#36864,#30390,.T.);
#46579=EDGE_CURVE('',#36866,#36865,#30391,.T.);
#46580=EDGE_CURVE('',#36863,#36866,#30392,.T.);
#46581=EDGE_CURVE('',#36867,#36868,#21346,.T.);
#46582=EDGE_CURVE('',#36868,#36869,#21347,.T.);
#46583=EDGE_CURVE('',#36869,#36870,#30393,.T.);
#46584=EDGE_CURVE('',#36870,#36867,#21348,.T.);
#46585=EDGE_CURVE('',#36869,#36871,#1880,.T.);
#46586=EDGE_CURVE('',#36839,#36871,#30394,.T.);
#46587=EDGE_CURVE('',#36841,#36870,#4817,.T.);
#46588=EDGE_CURVE('',#36871,#36872,#4818,.T.);
#46589=EDGE_CURVE('',#36839,#36872,#30395,.T.);
#46590=EDGE_CURVE('',#36872,#36873,#4819,.T.);
#46591=EDGE_CURVE('',#36874,#36873,#4820,.T.);
#46592=EDGE_CURVE('',#36874,#36840,#4821,.T.);
#46593=EDGE_CURVE('',#36873,#36875,#21349,.T.);
#46594=EDGE_CURVE('',#36875,#36876,#4822,.T.);
#46595=EDGE_CURVE('',#36876,#36874,#21350,.T.);
#46596=EDGE_CURVE('',#36877,#36878,#21351,.T.);
#46597=EDGE_CURVE('',#36878,#36879,#21352,.T.);
#46598=EDGE_CURVE('',#36879,#36880,#21353,.T.);
#46599=EDGE_CURVE('',#36880,#36877,#21354,.T.);
#46600=EDGE_CURVE('',#36881,#36882,#21355,.T.);
#46601=EDGE_CURVE('',#36881,#36878,#30396,.T.);
#46602=EDGE_CURVE('',#36877,#36882,#30397,.T.);
#46603=EDGE_CURVE('',#36882,#36883,#21356,.T.);
#46604=EDGE_CURVE('',#36883,#36884,#21357,.T.);
#46605=EDGE_CURVE('',#36884,#36881,#21358,.T.);
#46606=EDGE_CURVE('',#36885,#36886,#30398,.T.);
#46607=EDGE_CURVE('',#36886,#36887,#4823,.T.);
#46608=EDGE_CURVE('',#36887,#36885,#4824,.T.);
#46609=EDGE_CURVE('',#36875,#36888,#4825,.T.);
#46610=EDGE_CURVE('',#36888,#36885,#4826,.T.);
#46611=EDGE_CURVE('',#36887,#36876,#4827,.T.);
#46612=EDGE_CURVE('',#36889,#36890,#21359,.T.);
#46613=EDGE_CURVE('',#36889,#36891,#30399,.T.);
#46614=EDGE_CURVE('',#36892,#36891,#21360,.T.);
#46615=EDGE_CURVE('',#36892,#36890,#30400,.T.);
#46616=EDGE_CURVE('',#36891,#36893,#21361,.T.);
#46617=EDGE_CURVE('',#36893,#36894,#30401,.T.);
#46618=EDGE_CURVE('',#36894,#36892,#21362,.T.);
#46619=EDGE_CURVE('',#36895,#36896,#4828,.T.);
#46620=EDGE_CURVE('',#36896,#36897,#21363,.T.);
#46621=EDGE_CURVE('',#36897,#36898,#4829,.T.);
#46622=EDGE_CURVE('',#36898,#36895,#21364,.T.);
#46623=EDGE_CURVE('',#36899,#36900,#4830,.T.);
#46624=EDGE_CURVE('',#36899,#36896,#4831,.T.);
#46625=EDGE_CURVE('',#36895,#36900,#4832,.T.);
#46626=EDGE_CURVE('',#36901,#36902,#30402,.T.);
#46627=EDGE_CURVE('',#36902,#36899,#4833,.T.);
#46628=EDGE_CURVE('',#36900,#36901,#4834,.T.);
#46629=EDGE_CURVE('',#36903,#36904,#21365,.T.);
#46630=EDGE_CURVE('',#36904,#36905,#30403,.T.);
#46631=EDGE_CURVE('',#36905,#36906,#21366,.T.);
#46632=EDGE_CURVE('',#36906,#36903,#21367,.T.);
#46633=EDGE_CURVE('',#36907,#36908,#21368,.T.);
#46634=EDGE_CURVE('',#36908,#36909,#21369,.T.);
#46635=EDGE_CURVE('',#36909,#36910,#21370,.T.);
#46636=EDGE_CURVE('',#36910,#36907,#21371,.T.);
#46637=EDGE_CURVE('',#36909,#36903,#30404,.T.);
#46638=EDGE_CURVE('',#36906,#36910,#30405,.T.);
#46639=EDGE_CURVE('',#36903,#36911,#30406,.T.);
#46640=EDGE_CURVE('',#36911,#36904,#4835,.T.);
#46641=EDGE_CURVE('',#36912,#36913,#4836,.T.);
#46642=EDGE_CURVE('',#36913,#36914,#21372,.T.);
#46643=EDGE_CURVE('',#36914,#36915,#4837,.T.);
#46644=EDGE_CURVE('',#36915,#36912,#21373,.T.);
#46645=EDGE_CURVE('',#36916,#36917,#4838,.T.);
#46646=EDGE_CURVE('',#36916,#36915,#4839,.T.);
#46647=EDGE_CURVE('',#36914,#36917,#4840,.T.);
#46648=EDGE_CURVE('',#36918,#36919,#30407,.T.);
#46649=EDGE_CURVE('',#36919,#36916,#4841,.T.);
#46650=EDGE_CURVE('',#36917,#36918,#4842,.T.);
#46651=EDGE_CURVE('',#36920,#36921,#4843,.T.);
#46652=EDGE_CURVE('',#36921,#36922,#30408,.T.);
#46653=EDGE_CURVE('',#36922,#36923,#4844,.T.);
#46654=EDGE_CURVE('',#36920,#36923,#4845,.T.);
#46655=EDGE_CURVE('',#36924,#36925,#4846,.T.);
#46656=EDGE_CURVE('',#36925,#36926,#21374,.T.);
#46657=EDGE_CURVE('',#36926,#36927,#4847,.T.);
#46658=EDGE_CURVE('',#36927,#36924,#21375,.T.);
#46659=EDGE_CURVE('',#36928,#36929,#4848,.T.);
#46660=EDGE_CURVE('',#36928,#36925,#4849,.T.);
#46661=EDGE_CURVE('',#36924,#36929,#1881,.T.);
#46662=EDGE_CURVE('',#36930,#36931,#30409,.T.);
#46663=EDGE_CURVE('',#36931,#36928,#4850,.T.);
#46664=EDGE_CURVE('',#36929,#36930,#4851,.T.);
#46665=EDGE_CURVE('',#36932,#36933,#4852,.T.);
#46666=EDGE_CURVE('',#36933,#36934,#30410,.T.);
#46667=EDGE_CURVE('',#36934,#36935,#4853,.T.);
#46668=EDGE_CURVE('',#36932,#36935,#30411,.T.);
#46669=EDGE_CURVE('',#36936,#36937,#4854,.T.);
#46670=EDGE_CURVE('',#36937,#36938,#21376,.T.);
#46671=EDGE_CURVE('',#36938,#36939,#4855,.T.);
#46672=EDGE_CURVE('',#36939,#36936,#21377,.T.);
#46673=EDGE_CURVE('',#36940,#36941,#4856,.T.);
#46674=EDGE_CURVE('',#36940,#36937,#1882,.T.);
#46675=EDGE_CURVE('',#36936,#36941,#4857,.T.);
#46676=EDGE_CURVE('',#36942,#36943,#30412,.T.);
#46677=EDGE_CURVE('',#36943,#36940,#4858,.T.);
#46678=EDGE_CURVE('',#36941,#36942,#4859,.T.);
#46679=EDGE_CURVE('',#36944,#36945,#4860,.T.);
#46680=EDGE_CURVE('',#36945,#36946,#30413,.T.);
#46681=EDGE_CURVE('',#36946,#36947,#4861,.T.);
#46682=EDGE_CURVE('',#36944,#36947,#4862,.T.);
#46683=EDGE_CURVE('',#36948,#36949,#4863,.T.);
#46684=EDGE_CURVE('',#36949,#36950,#21378,.T.);
#46685=EDGE_CURVE('',#36950,#36951,#4864,.T.);
#46686=EDGE_CURVE('',#36951,#36948,#21379,.T.);
#46687=EDGE_CURVE('',#36952,#36953,#4865,.T.);
#46688=EDGE_CURVE('',#36952,#36949,#4866,.T.);
#46689=EDGE_CURVE('',#36948,#36953,#4867,.T.);
#46690=EDGE_CURVE('',#36954,#36955,#30414,.T.);
#46691=EDGE_CURVE('',#36955,#36952,#4868,.T.);
#46692=EDGE_CURVE('',#36953,#36954,#4869,.T.);
#46693=EDGE_CURVE('',#36956,#36957,#21380,.T.);
#46694=EDGE_CURVE('',#36956,#36958,#4870,.T.);
#46695=EDGE_CURVE('',#36957,#36958,#30415,.T.);
#46696=EDGE_CURVE('',#36959,#36960,#21381,.T.);
#46697=EDGE_CURVE('',#36960,#36961,#21382,.T.);
#46698=EDGE_CURVE('',#36961,#36962,#21383,.T.);
#46699=EDGE_CURVE('',#36962,#36959,#21384,.T.);
#46700=EDGE_CURVE('',#36961,#36963,#30416,.T.);
#46701=EDGE_CURVE('',#36957,#36963,#21385,.T.);
#46702=EDGE_CURVE('',#36957,#36962,#30417,.T.);
#46703=EDGE_CURVE('',#36963,#36964,#21386,.T.);
#46704=EDGE_CURVE('',#36964,#36956,#30418,.T.);
#46705=EDGE_CURVE('',#36965,#36966,#21387,.T.);
#46706=EDGE_CURVE('',#36965,#36967,#30419,.T.);
#46707=EDGE_CURVE('',#36968,#36967,#21388,.T.);
#46708=EDGE_CURVE('',#36968,#36966,#30420,.T.);
#46709=EDGE_CURVE('',#36969,#36970,#4871,.T.);
#46710=EDGE_CURVE('',#36970,#36971,#21389,.T.);
#46711=EDGE_CURVE('',#36971,#36972,#4872,.T.);
#46712=EDGE_CURVE('',#36972,#36969,#21390,.T.);
#46713=EDGE_CURVE('',#36973,#36974,#4873,.T.);
#46714=EDGE_CURVE('',#36973,#36972,#4874,.T.);
#46715=EDGE_CURVE('',#36971,#36974,#4875,.T.);
#46716=EDGE_CURVE('',#36975,#36976,#30421,.T.);
#46717=EDGE_CURVE('',#36976,#36973,#4876,.T.);
#46718=EDGE_CURVE('',#36974,#36975,#4877,.T.);
#46719=EDGE_CURVE('',#36967,#36977,#21391,.T.);
#46720=EDGE_CURVE('',#36977,#36978,#30422,.T.);
#46721=EDGE_CURVE('',#36978,#36968,#21392,.T.);
#46722=EDGE_CURVE('',#36979,#36980,#21393,.T.);
#46723=EDGE_CURVE('',#36980,#36965,#21394,.T.);
#46724=EDGE_CURVE('',#36966,#36979,#21395,.T.);
#46725=EDGE_CURVE('',#36981,#36982,#21396,.T.);
#46726=EDGE_CURVE('',#36982,#36889,#21397,.T.);
#46727=EDGE_CURVE('',#36890,#36981,#21398,.T.);
#46728=EDGE_CURVE('',#36983,#36984,#4878,.T.);
#46729=EDGE_CURVE('',#36984,#36985,#21399,.T.);
#46730=EDGE_CURVE('',#36985,#36986,#4879,.T.);
#46731=EDGE_CURVE('',#36986,#36983,#21400,.T.);
#46732=EDGE_CURVE('',#36987,#36988,#21401,.T.);
#46733=EDGE_CURVE('',#36988,#36989,#21402,.T.);
#46734=EDGE_CURVE('',#36989,#36990,#21403,.T.);
#46735=EDGE_CURVE('',#36990,#36987,#21404,.T.);
#46736=EDGE_CURVE('',#36991,#36992,#4880,.T.);
#46737=EDGE_CURVE('',#36992,#36993,#21405,.T.);
#46738=EDGE_CURVE('',#36993,#36994,#4881,.T.);
#46739=EDGE_CURVE('',#36994,#36991,#21406,.T.);
#46740=EDGE_CURVE('',#36995,#36996,#4882,.T.);
#46741=EDGE_CURVE('',#36996,#36997,#21407,.T.);
#46742=EDGE_CURVE('',#36997,#36998,#4883,.T.);
#46743=EDGE_CURVE('',#36998,#36995,#21408,.T.);
#46744=EDGE_CURVE('',#36999,#37000,#21409,.T.);
#46745=EDGE_CURVE('',#36999,#37001,#30423,.T.);
#46746=EDGE_CURVE('',#37002,#37001,#21410,.T.);
#46747=EDGE_CURVE('',#37002,#37000,#30424,.T.);
#46748=EDGE_CURVE('',#36852,#36862,#4884,.T.);
#46749=EDGE_CURVE('',#36861,#37003,#30425,.T.);
#46750=EDGE_CURVE('',#37003,#37004,#4885,.T.);
#46751=EDGE_CURVE('',#37004,#36850,#4886,.T.);
#46752=EDGE_CURVE('',#37005,#37006,#4887,.T.);
#46753=EDGE_CURVE('',#37005,#36996,#4888,.T.);
#46754=EDGE_CURVE('',#36995,#37006,#1883,.T.);
#46755=EDGE_CURVE('',#37007,#37008,#4889,.T.);
#46756=EDGE_CURVE('',#37007,#36992,#4890,.T.);
#46757=EDGE_CURVE('',#36991,#37008,#4891,.T.);
#46758=EDGE_CURVE('',#36989,#37009,#30426,.T.);
#46759=EDGE_CURVE('',#37010,#37009,#21411,.T.);
#46760=EDGE_CURVE('',#37010,#36990,#30427,.T.);
#46761=EDGE_CURVE('',#37011,#37012,#4892,.T.);
#46762=EDGE_CURVE('',#37011,#36984,#4893,.T.);
#46763=EDGE_CURVE('',#36983,#37012,#4894,.T.);
#46764=EDGE_CURVE('',#37013,#37014,#30428,.T.);
#46765=EDGE_CURVE('',#37015,#37014,#30429,.T.);
#46766=EDGE_CURVE('',#37016,#37015,#30430,.T.);
#46767=EDGE_CURVE('',#37013,#37016,#30431,.T.);
#46768=EDGE_CURVE('',#37017,#36850,#30432,.T.);
#46769=EDGE_CURVE('',#37018,#37004,#30433,.T.);
#46770=EDGE_CURVE('',#37017,#37018,#4895,.T.);
#46771=EDGE_CURVE('',#37019,#37017,#21412,.T.);
#46772=EDGE_CURVE('',#37019,#36851,#4896,.T.);
#46773=EDGE_CURVE('',#36848,#37020,#30434,.T.);
#46774=EDGE_CURVE('',#37021,#36848,#4897,.T.);
#46775=EDGE_CURVE('',#37022,#37021,#30435,.T.);
#46776=EDGE_CURVE('',#37020,#37022,#4898,.T.);
#46777=EDGE_CURVE('',#37023,#37020,#21413,.T.);
#46778=EDGE_CURVE('',#36849,#37023,#30436,.T.);
#46779=EDGE_CURVE('',#37024,#37023,#4899,.T.);
#46780=EDGE_CURVE('',#37025,#37024,#30437,.T.);
#46781=EDGE_CURVE('',#36849,#37025,#4900,.T.);
#46782=EDGE_CURVE('',#37026,#37027,#21414,.T.);
#46783=EDGE_CURVE('',#37026,#36868,#4901,.T.);
#46784=EDGE_CURVE('',#36867,#37027,#4902,.T.);
#46785=EDGE_CURVE('',#37028,#37029,#30438,.T.);
#46786=EDGE_CURVE('',#37030,#37029,#4903,.T.);
#46787=EDGE_CURVE('',#36883,#37030,#30439,.T.);
#46788=EDGE_CURVE('',#37028,#36883,#4904,.T.);
#46789=EDGE_CURVE('',#37031,#37030,#21415,.T.);
#46790=EDGE_CURVE('',#36884,#37031,#30440,.T.);
#46791=EDGE_CURVE('',#37032,#37031,#4905,.T.);
#46792=EDGE_CURVE('',#37033,#37032,#30441,.T.);
#46793=EDGE_CURVE('',#36884,#37033,#4906,.T.);
#46794=EDGE_CURVE('',#37034,#37035,#21416,.T.);
#46795=EDGE_CURVE('',#37034,#37036,#4907,.T.);
#46796=EDGE_CURVE('',#37037,#37036,#21417,.T.);
#46797=EDGE_CURVE('',#37035,#37037,#30442,.T.);
#46798=EDGE_CURVE('',#37038,#37037,#30443,.T.);
#46799=EDGE_CURVE('',#37039,#37038,#30444,.T.);
#46800=EDGE_CURVE('',#37035,#37039,#30445,.T.);
#46801=EDGE_CURVE('',#37040,#37038,#30446,.T.);
#46802=EDGE_CURVE('',#37041,#37040,#30447,.T.);
#46803=EDGE_CURVE('',#37039,#37041,#30448,.T.);
#46804=EDGE_CURVE('',#37042,#37040,#30449,.T.);
#46805=EDGE_CURVE('',#37043,#37042,#30450,.T.);
#46806=EDGE_CURVE('',#37041,#37043,#30451,.T.);
#46807=EDGE_CURVE('',#36750,#37044,#30452,.T.);
#46808=EDGE_CURVE('',#37045,#36750,#4908,.T.);
#46809=EDGE_CURVE('',#37046,#37045,#30453,.T.);
#46810=EDGE_CURVE('',#37044,#37046,#4909,.T.);
#46811=EDGE_CURVE('',#37047,#37044,#21418,.T.);
#46812=EDGE_CURVE('',#36751,#37047,#30454,.T.);
#46813=EDGE_CURVE('',#37048,#37047,#4910,.T.);
#46814=EDGE_CURVE('',#37049,#37048,#30455,.T.);
#46815=EDGE_CURVE('',#36751,#37049,#4911,.T.);
#46816=EDGE_CURVE('',#36743,#37050,#4912,.T.);
#46817=EDGE_CURVE('',#37051,#37050,#21419,.T.);
#46818=EDGE_CURVE('',#36741,#37051,#30456,.T.);
#46819=EDGE_CURVE('',#37052,#37051,#4913,.T.);
#46820=EDGE_CURVE('',#36776,#37052,#30457,.T.);
#46821=EDGE_CURVE('',#37053,#37042,#21420,.T.);
#46822=EDGE_CURVE('',#37053,#37054,#4914,.T.);
#46823=EDGE_CURVE('',#37043,#37054,#21421,.T.);
#46824=EDGE_CURVE('',#37055,#37056,#30458,.T.);
#46825=EDGE_CURVE('',#37057,#37056,#4915,.T.);
#46826=EDGE_CURVE('',#36774,#37057,#30459,.T.);
#46827=EDGE_CURVE('',#37055,#36774,#4916,.T.);
#46828=EDGE_CURVE('',#37058,#37057,#21422,.T.);
#46829=EDGE_CURVE('',#36775,#37058,#30460,.T.);
#46830=EDGE_CURVE('',#37059,#37058,#4917,.T.);
#46831=EDGE_CURVE('',#37060,#37059,#30461,.T.);
#46832=EDGE_CURVE('',#36775,#37060,#4918,.T.);
#46833=EDGE_CURVE('',#37061,#37062,#21423,.T.);
#46834=EDGE_CURVE('',#37061,#36767,#4919,.T.);
#46835=EDGE_CURVE('',#36766,#37062,#4920,.T.);
#46836=EDGE_CURVE('',#37063,#37052,#4921,.T.);
#46837=EDGE_CURVE('',#37063,#36777,#4922,.T.);
#46838=EDGE_CURVE('',#37064,#37065,#30462,.T.);
#46839=EDGE_CURVE('',#37066,#37065,#4923,.T.);
#46840=EDGE_CURVE('',#37067,#37066,#30463,.T.);
#46841=EDGE_CURVE('',#37064,#37067,#4924,.T.);
#46842=EDGE_CURVE('',#37068,#37066,#1884,.T.);
#46843=EDGE_CURVE('',#36977,#37068,#30464,.T.);
#46844=EDGE_CURVE('',#37067,#36977,#1885,.T.);
#46845=EDGE_CURVE('',#37069,#37068,#30465,.T.);
#46846=EDGE_CURVE('',#36978,#37069,#30466,.T.);
#46847=EDGE_CURVE('',#37070,#37071,#30467,.T.);
#46848=EDGE_CURVE('',#36978,#37071,#4925,.T.);
#46849=EDGE_CURVE('',#37070,#37069,#4926,.T.);
#46850=EDGE_CURVE('',#37072,#37073,#30468,.T.);
#46851=EDGE_CURVE('',#37072,#36976,#1886,.T.);
#46852=EDGE_CURVE('',#36975,#37073,#1887,.T.);
#46853=EDGE_CURVE('',#37074,#36964,#30469,.T.);
#46854=EDGE_CURVE('',#37075,#36964,#4927,.T.);
#46855=EDGE_CURVE('',#37076,#37075,#30470,.T.);
#46856=EDGE_CURVE('',#37074,#37076,#4928,.T.);
#46857=EDGE_CURVE('',#37077,#36956,#30471,.T.);
#46858=EDGE_CURVE('',#37077,#37074,#30472,.T.);
#46859=EDGE_CURVE('',#37078,#36958,#30473,.T.);
#46860=EDGE_CURVE('',#37078,#37077,#4929,.T.);
#46861=EDGE_CURVE('',#37079,#37080,#30474,.T.);
#46862=EDGE_CURVE('',#36958,#37080,#4930,.T.);
#46863=EDGE_CURVE('',#37079,#37078,#1888,.T.);
#46864=EDGE_CURVE('',#37081,#37082,#30475,.T.);
#46865=EDGE_CURVE('',#37081,#36955,#1889,.T.);
#46866=EDGE_CURVE('',#36954,#37082,#1890,.T.);
#46867=EDGE_CURVE('',#36945,#37083,#30476,.T.);
#46868=EDGE_CURVE('',#37084,#36945,#4931,.T.);
#46869=EDGE_CURVE('',#37085,#37084,#30477,.T.);
#46870=EDGE_CURVE('',#37083,#37085,#4932,.T.);
#46871=EDGE_CURVE('',#37086,#37083,#30478,.T.);
#46872=EDGE_CURVE('',#36946,#37086,#30479,.T.);
#46873=EDGE_CURVE('',#37087,#37086,#4933,.T.);
#46874=EDGE_CURVE('',#37088,#37087,#30480,.T.);
#46875=EDGE_CURVE('',#36946,#37088,#4934,.T.);
#46876=EDGE_CURVE('',#37089,#37090,#30481,.T.);
#46877=EDGE_CURVE('',#37089,#36943,#1891,.T.);
#46878=EDGE_CURVE('',#36942,#37090,#1892,.T.);
#46879=EDGE_CURVE('',#36933,#37091,#30482,.T.);
#46880=EDGE_CURVE('',#37092,#36933,#4935,.T.);
#46881=EDGE_CURVE('',#37093,#37092,#30483,.T.);
#46882=EDGE_CURVE('',#37091,#37093,#4936,.T.);
#46883=EDGE_CURVE('',#37094,#37091,#30484,.T.);
#46884=EDGE_CURVE('',#36934,#37094,#30485,.T.);
#46885=EDGE_CURVE('',#37095,#37094,#4937,.T.);
#46886=EDGE_CURVE('',#37096,#37095,#30486,.T.);
#46887=EDGE_CURVE('',#36934,#37096,#4938,.T.);
#46888=EDGE_CURVE('',#37097,#37098,#30487,.T.);
#46889=EDGE_CURVE('',#37097,#36931,#1893,.T.);
#46890=EDGE_CURVE('',#36930,#37098,#1894,.T.);
#46891=EDGE_CURVE('',#36921,#37099,#30488,.T.);
#46892=EDGE_CURVE('',#37100,#36921,#4939,.T.);
#46893=EDGE_CURVE('',#37101,#37100,#30489,.T.);
#46894=EDGE_CURVE('',#37099,#37101,#4940,.T.);
#46895=EDGE_CURVE('',#37102,#37099,#30490,.T.);
#46896=EDGE_CURVE('',#36922,#37102,#30491,.T.);
#46897=EDGE_CURVE('',#37103,#37102,#4941,.T.);
#46898=EDGE_CURVE('',#37104,#37103,#30492,.T.);
#46899=EDGE_CURVE('',#36922,#37104,#4942,.T.);
#46900=EDGE_CURVE('',#37105,#37106,#30493,.T.);
#46901=EDGE_CURVE('',#37105,#36919,#1895,.T.);
#46902=EDGE_CURVE('',#36918,#37106,#1896,.T.);
#46903=EDGE_CURVE('',#37107,#36911,#30494,.T.);
#46904=EDGE_CURVE('',#37108,#36911,#4943,.T.);
#46905=EDGE_CURVE('',#37109,#37108,#30495,.T.);
#46906=EDGE_CURVE('',#37107,#37109,#4944,.T.);
#46907=EDGE_CURVE('',#37110,#36904,#30496,.T.);
#46908=EDGE_CURVE('',#37110,#37107,#4945,.T.);
#46909=EDGE_CURVE('',#37111,#36905,#30497,.T.);
#46910=EDGE_CURVE('',#37111,#37110,#30498,.T.);
#46911=EDGE_CURVE('',#37112,#37113,#30499,.T.);
#46912=EDGE_CURVE('',#36905,#37113,#4946,.T.);
#46913=EDGE_CURVE('',#37112,#37111,#4947,.T.);
#46914=EDGE_CURVE('',#37114,#37115,#30500,.T.);
#46915=EDGE_CURVE('',#37114,#36902,#1897,.T.);
#46916=EDGE_CURVE('',#36901,#37115,#1898,.T.);
#46917=EDGE_CURVE('',#37116,#37117,#30501,.T.);
#46918=EDGE_CURVE('',#37118,#37117,#4948,.T.);
#46919=EDGE_CURVE('',#36893,#37118,#30502,.T.);
#46920=EDGE_CURVE('',#37116,#36893,#4949,.T.);
#46921=EDGE_CURVE('',#37119,#37118,#30503,.T.);
#46922=EDGE_CURVE('',#36894,#37119,#30504,.T.);
#46923=EDGE_CURVE('',#37120,#37119,#4950,.T.);
#46924=EDGE_CURVE('',#37121,#37120,#30505,.T.);
#46925=EDGE_CURVE('',#36894,#37121,#4951,.T.);
#46926=EDGE_CURVE('',#36809,#37122,#4952,.T.);
#46927=EDGE_CURVE('',#37123,#37122,#4953,.T.);
#46928=EDGE_CURVE('',#37123,#36810,#30506,.T.);
#46929=EDGE_CURVE('',#37124,#37125,#30507,.T.);
#46930=EDGE_CURVE('',#37121,#37125,#4954,.T.);
#46931=EDGE_CURVE('',#37124,#37120,#4955,.T.);
#46932=EDGE_CURVE('',#37126,#36796,#30508,.T.);
#46933=EDGE_CURVE('',#37126,#37123,#4956,.T.);
#46934=EDGE_CURVE('',#37127,#37126,#21424,.T.);
#46935=EDGE_CURVE('',#37127,#36797,#4957,.T.);
#46936=EDGE_CURVE('',#36794,#37128,#30509,.T.);
#46937=EDGE_CURVE('',#37129,#36794,#4958,.T.);
#46938=EDGE_CURVE('',#37130,#37129,#30510,.T.);
#46939=EDGE_CURVE('',#37128,#37130,#4959,.T.);
#46940=EDGE_CURVE('',#37131,#37128,#21425,.T.);
#46941=EDGE_CURVE('',#36795,#37131,#30511,.T.);
#46942=EDGE_CURVE('',#37132,#37131,#4960,.T.);
#46943=EDGE_CURVE('',#37133,#37132,#30512,.T.);
#46944=EDGE_CURVE('',#36795,#37133,#4961,.T.);
#46945=EDGE_CURVE('',#37134,#37135,#21426,.T.);
#46946=EDGE_CURVE('',#37134,#36812,#4962,.T.);
#46947=EDGE_CURVE('',#36811,#37135,#4963,.T.);
#46948=EDGE_CURVE('',#37136,#37137,#30513,.T.);
#46949=EDGE_CURVE('',#37138,#37137,#4964,.T.);
#46950=EDGE_CURVE('',#36831,#37138,#30514,.T.);
#46951=EDGE_CURVE('',#37136,#36831,#4965,.T.);
#46952=EDGE_CURVE('',#37139,#37138,#21427,.T.);
#46953=EDGE_CURVE('',#36832,#37139,#30515,.T.);
#46954=EDGE_CURVE('',#37140,#37139,#4966,.T.);
#46955=EDGE_CURVE('',#37141,#37140,#30516,.T.);
#46956=EDGE_CURVE('',#36832,#37141,#4967,.T.);
#46957=EDGE_CURVE('',#37142,#37143,#21428,.T.);
#46958=EDGE_CURVE('',#37142,#37144,#4968,.T.);
#46959=EDGE_CURVE('',#37145,#37144,#21429,.T.);
#46960=EDGE_CURVE('',#37143,#37145,#30517,.T.);
#46961=EDGE_CURVE('',#37146,#37145,#30518,.T.);
#46962=EDGE_CURVE('',#37147,#37146,#30519,.T.);
#46963=EDGE_CURVE('',#37143,#37147,#30520,.T.);
#46964=EDGE_CURVE('',#37148,#37146,#30521,.T.);
#46965=EDGE_CURVE('',#37149,#37148,#30522,.T.);
#46966=EDGE_CURVE('',#37147,#37149,#30523,.T.);
#46967=EDGE_CURVE('',#37150,#37148,#30524,.T.);
#46968=EDGE_CURVE('',#37151,#37150,#30525,.T.);
#46969=EDGE_CURVE('',#37149,#37151,#30526,.T.);
#46970=EDGE_CURVE('',#37152,#37150,#21430,.T.);
#46971=EDGE_CURVE('',#37152,#37153,#4969,.T.);
#46972=EDGE_CURVE('',#37151,#37153,#21431,.T.);
#46973=EDGE_CURVE('',#37154,#37155,#30527,.T.);
#46974=EDGE_CURVE('',#37156,#37154,#30528,.T.);
#46975=EDGE_CURVE('',#37155,#37156,#30529,.T.);
#46976=EDGE_CURVE('',#37157,#37158,#4970,.T.);
#46977=EDGE_CURVE('',#37157,#36836,#4971,.T.);
#46978=EDGE_CURVE('',#36835,#37158,#4972,.T.);
#46979=EDGE_CURVE('',#37159,#37160,#4973,.T.);
#46980=EDGE_CURVE('',#37159,#37161,#4974,.T.);
#46981=EDGE_CURVE('',#37162,#37161,#4975,.T.);
#46982=EDGE_CURVE('',#37162,#37160,#4976,.T.);
#46983=EDGE_CURVE('',#37163,#37164,#21432,.T.);
#46984=EDGE_CURVE('',#37164,#36999,#21433,.T.);
#46985=EDGE_CURVE('',#37000,#37163,#21434,.T.);
#46986=EDGE_CURVE('',#37165,#37166,#21435,.T.);
#46987=EDGE_CURVE('',#37166,#37167,#4977,.T.);
#46988=EDGE_CURVE('',#37167,#37168,#21436,.T.);
#46989=EDGE_CURVE('',#37168,#37165,#30530,.T.);
#46990=EDGE_CURVE('',#37169,#37170,#30531,.T.);
#46991=EDGE_CURVE('',#37169,#36863,#21437,.T.);
#46992=EDGE_CURVE('',#36866,#37170,#21438,.T.);
#46993=EDGE_CURVE('',#36749,#37171,#30532,.T.);
#46994=EDGE_CURVE('',#37172,#37171,#30533,.T.);
#46995=EDGE_CURVE('',#36747,#37172,#30534,.T.);
#46996=EDGE_CURVE('',#37173,#37172,#21439,.T.);
#46997=EDGE_CURVE('',#36744,#37173,#30535,.T.);
#46998=EDGE_CURVE('',#37174,#36787,#30536,.T.);
#46999=EDGE_CURVE('',#37175,#36787,#4978,.T.);
#47000=EDGE_CURVE('',#37176,#37175,#30537,.T.);
#47001=EDGE_CURVE('',#37174,#37176,#4979,.T.);
#47002=EDGE_CURVE('',#37177,#36785,#30538,.T.);
#47003=EDGE_CURVE('',#37177,#37174,#4980,.T.);
#47004=EDGE_CURVE('',#37178,#36783,#30539,.T.);
#47005=EDGE_CURVE('',#37178,#37177,#21440,.T.);
#47006=EDGE_CURVE('',#37179,#36781,#30540,.T.);
#47007=EDGE_CURVE('',#37179,#37178,#4981,.T.);
#47008=EDGE_CURVE('',#37180,#36779,#30541,.T.);
#47009=EDGE_CURVE('',#37180,#37179,#4982,.T.);
#47010=EDGE_CURVE('',#37181,#36742,#30542,.T.);
#47011=EDGE_CURVE('',#37181,#37180,#4983,.T.);
#47012=EDGE_CURVE('',#37182,#36743,#30543,.T.);
#47013=EDGE_CURVE('',#37182,#37181,#21441,.T.);
#47014=EDGE_CURVE('',#37183,#37184,#30544,.T.);
#47015=EDGE_CURVE('',#37184,#37050,#30545,.T.);
#47016=EDGE_CURVE('',#37183,#37182,#1159,.T.);
#47017=EDGE_CURVE('',#37049,#37183,#21442,.T.);
#47018=EDGE_CURVE('',#37050,#37048,#21443,.T.);
#47019=EDGE_CURVE('',#37171,#37049,#21444,.T.);
#47020=EDGE_CURVE('',#37185,#37186,#30546,.T.);
#47021=EDGE_CURVE('',#37187,#37186,#21445,.T.);
#47022=EDGE_CURVE('',#37188,#37187,#30547,.T.);
#47023=EDGE_CURVE('',#37185,#37188,#21446,.T.);
#47024=EDGE_CURVE('',#37189,#37173,#30548,.T.);
#47025=EDGE_CURVE('',#37190,#37189,#30549,.T.);
#47026=EDGE_CURVE('',#36744,#37190,#30550,.T.);
#47027=EDGE_CURVE('',#37191,#37190,#21447,.T.);
#47028=EDGE_CURVE('',#37191,#36745,#30551,.T.);
#47029=EDGE_CURVE('',#37191,#37192,#30552,.T.);
#47030=EDGE_CURVE('',#37193,#37192,#30553,.T.);
#47031=EDGE_CURVE('',#36745,#37193,#30554,.T.);
#47032=EDGE_CURVE('',#37194,#37193,#21448,.T.);
#47033=EDGE_CURVE('',#36746,#37194,#30555,.T.);
#47034=EDGE_CURVE('',#37195,#37194,#30556,.T.);
#47035=EDGE_CURVE('',#36748,#37195,#30557,.T.);
#47036=EDGE_CURVE('',#37045,#37195,#21449,.T.);
#47037=EDGE_CURVE('',#37196,#37045,#21450,.T.);
#47038=EDGE_CURVE('',#37061,#37196,#30558,.T.);
#47039=EDGE_CURVE('',#37046,#37061,#21451,.T.);
#47040=EDGE_CURVE('',#37197,#37196,#1160,.T.);
#47041=EDGE_CURVE('',#36767,#37197,#30559,.T.);
#47042=EDGE_CURVE('',#37198,#37197,#21452,.T.);
#47043=EDGE_CURVE('',#36764,#37198,#30560,.T.);
#47044=EDGE_CURVE('',#37199,#37198,#4984,.T.);
#47045=EDGE_CURVE('',#36763,#37199,#30561,.T.);
#47046=EDGE_CURVE('',#37200,#37199,#4985,.T.);
#47047=EDGE_CURVE('',#36760,#37200,#30562,.T.);
#47048=EDGE_CURVE('',#37201,#37200,#4986,.T.);
#47049=EDGE_CURVE('',#36759,#37201,#30563,.T.);
#47050=EDGE_CURVE('',#37202,#37201,#21453,.T.);
#47051=EDGE_CURVE('',#36756,#37202,#30564,.T.);
#47052=EDGE_CURVE('',#37203,#37202,#4987,.T.);
#47053=EDGE_CURVE('',#36753,#37203,#30565,.T.);
#47054=EDGE_CURVE('',#37204,#37203,#4988,.T.);
#47055=EDGE_CURVE('',#36754,#37204,#30566,.T.);
#47056=EDGE_CURVE('',#37205,#37204,#4989,.T.);
#47057=EDGE_CURVE('',#37206,#37205,#30567,.T.);
#47058=EDGE_CURVE('',#36754,#37206,#4990,.T.);
#47059=EDGE_CURVE('',#37207,#37205,#21454,.T.);
#47060=EDGE_CURVE('',#37208,#37207,#30568,.T.);
#47061=EDGE_CURVE('',#37206,#37208,#21455,.T.);
#47062=EDGE_CURVE('',#37209,#37206,#30569,.T.);
#47063=EDGE_CURVE('',#37209,#36755,#4991,.T.);
#47064=EDGE_CURVE('',#36773,#37210,#30570,.T.);
#47065=EDGE_CURVE('',#37211,#37210,#30571,.T.);
#47066=EDGE_CURVE('',#36771,#37211,#30572,.T.);
#47067=EDGE_CURVE('',#37212,#37211,#21456,.T.);
#47068=EDGE_CURVE('',#36768,#37212,#30573,.T.);
#47069=EDGE_CURVE('',#37213,#37214,#30574,.T.);
#47070=EDGE_CURVE('',#37215,#37214,#21457,.T.);
#47071=EDGE_CURVE('',#37209,#37215,#30575,.T.);
#47072=EDGE_CURVE('',#37213,#37209,#21458,.T.);
#47073=EDGE_CURVE('',#37216,#37215,#4992,.T.);
#47074=EDGE_CURVE('',#36755,#37216,#30576,.T.);
#47075=EDGE_CURVE('',#37217,#37216,#1161,.T.);
#47076=EDGE_CURVE('',#36752,#37217,#30577,.T.);
#47077=EDGE_CURVE('',#37218,#37217,#4993,.T.);
#47078=EDGE_CURVE('',#36757,#37218,#30578,.T.);
#47079=EDGE_CURVE('',#37219,#37218,#21459,.T.);
#47080=EDGE_CURVE('',#36758,#37219,#30579,.T.);
#47081=EDGE_CURVE('',#37220,#36761,#30580,.T.);
#47082=EDGE_CURVE('',#37220,#37219,#4994,.T.);
#47083=EDGE_CURVE('',#37221,#36762,#30581,.T.);
#47084=EDGE_CURVE('',#37221,#37220,#1162,.T.);
#47085=EDGE_CURVE('',#37222,#36765,#30582,.T.);
#47086=EDGE_CURVE('',#37222,#37221,#4995,.T.);
#47087=EDGE_CURVE('',#37223,#36766,#30583,.T.);
#47088=EDGE_CURVE('',#37223,#37222,#21460,.T.);
#47089=EDGE_CURVE('',#37224,#37225,#30584,.T.);
#47090=EDGE_CURVE('',#37225,#37062,#30585,.T.);
#47091=EDGE_CURVE('',#37224,#37223,#1163,.T.);
#47092=EDGE_CURVE('',#37060,#37224,#21461,.T.);
#47093=EDGE_CURVE('',#37062,#37059,#21462,.T.);
#47094=EDGE_CURVE('',#37210,#37060,#21463,.T.);
#47095=EDGE_CURVE('',#37226,#37212,#30586,.T.);
#47096=EDGE_CURVE('',#37227,#37226,#30587,.T.);
#47097=EDGE_CURVE('',#36768,#37227,#30588,.T.);
#47098=EDGE_CURVE('',#37228,#37227,#21464,.T.);
#47099=EDGE_CURVE('',#37228,#36769,#30589,.T.);
#47100=EDGE_CURVE('',#37229,#37230,#30590,.T.);
#47101=EDGE_CURVE('',#37054,#37230,#21465,.T.);
#47102=EDGE_CURVE('',#37231,#37054,#30591,.T.);
#47103=EDGE_CURVE('',#37229,#37231,#21466,.T.);
#47104=EDGE_CURVE('',#37232,#37015,#21467,.T.);
#47105=EDGE_CURVE('',#37233,#37232,#30592,.T.);
#47106=EDGE_CURVE('',#37016,#37233,#21468,.T.);
#47107=EDGE_CURVE('',#37234,#36865,#21469,.T.);
#47108=EDGE_CURVE('',#37170,#37234,#30593,.T.);
#47109=EDGE_CURVE('',#37235,#37234,#4996,.T.);
#47110=EDGE_CURVE('',#37236,#37235,#30594,.T.);
#47111=EDGE_CURVE('',#37170,#37236,#4997,.F.);
#47112=EDGE_CURVE('',#37237,#36769,#30595,.T.);
#47113=EDGE_CURVE('',#37238,#37228,#30596,.T.);
#47114=EDGE_CURVE('',#37237,#37238,#30597,.T.);
#47115=EDGE_CURVE('',#37239,#36770,#30598,.T.);
#47116=EDGE_CURVE('',#37239,#37237,#21470,.T.);
#47117=EDGE_CURVE('',#37240,#36772,#30599,.T.);
#47118=EDGE_CURVE('',#37240,#37239,#30600,.T.);
#47119=EDGE_CURVE('',#37055,#37240,#21471,.T.);
#47120=EDGE_CURVE('',#37241,#37053,#30601,.T.);
#47121=EDGE_CURVE('',#37056,#37053,#21472,.T.);
#47122=EDGE_CURVE('',#37241,#37055,#21473,.T.);
#47123=EDGE_CURVE('',#37231,#37241,#1164,.T.);
#47124=EDGE_CURVE('',#37242,#36778,#30602,.T.);
#47125=EDGE_CURVE('',#37243,#36777,#30603,.T.);
#47126=EDGE_CURVE('',#37242,#37243,#4998,.T.);
#47127=EDGE_CURVE('',#37244,#36780,#30604,.T.);
#47128=EDGE_CURVE('',#37244,#37242,#4999,.T.);
#47129=EDGE_CURVE('',#37245,#36782,#30605,.T.);
#47130=EDGE_CURVE('',#37245,#37244,#5000,.T.);
#47131=EDGE_CURVE('',#37246,#36784,#30606,.T.);
#47132=EDGE_CURVE('',#37246,#37245,#21474,.T.);
#47133=EDGE_CURVE('',#37247,#36786,#30607,.T.);
#47134=EDGE_CURVE('',#37247,#37246,#5001,.T.);
#47135=EDGE_CURVE('',#37248,#37249,#30608,.T.);
#47136=EDGE_CURVE('',#36786,#37249,#5002,.T.);
#47137=EDGE_CURVE('',#37248,#37247,#5003,.T.);
#47138=EDGE_CURVE('',#36980,#37250,#30609,.T.);
#47139=EDGE_CURVE('',#37251,#37250,#21475,.T.);
#47140=EDGE_CURVE('',#36965,#37251,#30610,.T.);
#47141=EDGE_CURVE('',#37252,#37251,#30611,.T.);
#47142=EDGE_CURVE('',#36967,#37252,#30612,.T.);
#47143=EDGE_CURVE('',#37064,#37252,#21476,.T.);
#47144=EDGE_CURVE('',#37253,#37063,#30613,.T.);
#47145=EDGE_CURVE('',#37065,#37063,#21477,.T.);
#47146=EDGE_CURVE('',#37253,#37064,#21478,.T.);
#47147=EDGE_CURVE('',#37243,#37253,#5004,.T.);
#47148=EDGE_CURVE('',#37186,#37175,#5005,.T.);
#47149=EDGE_CURVE('',#37176,#37185,#5006,.T.);
#47150=EDGE_CURVE('',#37254,#37255,#30614,.T.);
#47151=EDGE_CURVE('',#37249,#37255,#1899,.T.);
#47152=EDGE_CURVE('',#37254,#37248,#1900,.T.);
#47153=EDGE_CURVE('',#37249,#37175,#30615,.T.);
#47154=EDGE_CURVE('',#36793,#37256,#30616,.T.);
#47155=EDGE_CURVE('',#37257,#37256,#30617,.T.);
#47156=EDGE_CURVE('',#36791,#37257,#30618,.T.);
#47157=EDGE_CURVE('',#37258,#37257,#21479,.T.);
#47158=EDGE_CURVE('',#36788,#37258,#30619,.T.);
#47159=EDGE_CURVE('',#37259,#36834,#30620,.T.);
#47160=EDGE_CURVE('',#37260,#36834,#5007,.T.);
#47161=EDGE_CURVE('',#37261,#37260,#30621,.T.);
#47162=EDGE_CURVE('',#37259,#37261,#5008,.T.);
#47163=EDGE_CURVE('',#37262,#36824,#30622,.T.);
#47164=EDGE_CURVE('',#37262,#37259,#5009,.T.);
#47165=EDGE_CURVE('',#37263,#36822,#30623,.T.);
#47166=EDGE_CURVE('',#37263,#37262,#5010,.T.);
#47167=EDGE_CURVE('',#37264,#36820,#30624,.T.);
#47168=EDGE_CURVE('',#37264,#37263,#21480,.T.);
#47169=EDGE_CURVE('',#37265,#36818,#30625,.T.);
#47170=EDGE_CURVE('',#37265,#37264,#5011,.T.);
#47171=EDGE_CURVE('',#37266,#36816,#30626,.T.);
#47172=EDGE_CURVE('',#37266,#37265,#5012,.T.);
#47173=EDGE_CURVE('',#37267,#36814,#30627,.T.);
#47174=EDGE_CURVE('',#37267,#37266,#5013,.T.);
#47175=EDGE_CURVE('',#37268,#36811,#30628,.T.);
#47176=EDGE_CURVE('',#37268,#37267,#21481,.T.);
#47177=EDGE_CURVE('',#37269,#37135,#30629,.T.);
#47178=EDGE_CURVE('',#37269,#37268,#1165,.T.);
#47179=EDGE_CURVE('',#37135,#37132,#21482,.T.);
#47180=EDGE_CURVE('',#37133,#37269,#21483,.T.);
#47181=EDGE_CURVE('',#37256,#37133,#21484,.T.);
#47182=EDGE_CURVE('',#37270,#37258,#30630,.T.);
#47183=EDGE_CURVE('',#37271,#37270,#30631,.T.);
#47184=EDGE_CURVE('',#36788,#37271,#30632,.T.);
#47185=EDGE_CURVE('',#37272,#37271,#21485,.T.);
#47186=EDGE_CURVE('',#37272,#36789,#30633,.T.);
#47187=EDGE_CURVE('',#37272,#37273,#30634,.T.);
#47188=EDGE_CURVE('',#37274,#37273,#30635,.T.);
#47189=EDGE_CURVE('',#36789,#37274,#30636,.T.);
#47190=EDGE_CURVE('',#37275,#37274,#21486,.T.);
#47191=EDGE_CURVE('',#36790,#37275,#30637,.T.);
#47192=EDGE_CURVE('',#37276,#37275,#30638,.T.);
#47193=EDGE_CURVE('',#36792,#37276,#30639,.T.);
#47194=EDGE_CURVE('',#37129,#37276,#21487,.T.);
#47195=EDGE_CURVE('',#37277,#37129,#21488,.T.);
#47196=EDGE_CURVE('',#37127,#37277,#30640,.T.);
#47197=EDGE_CURVE('',#37130,#37127,#21489,.T.);
#47198=EDGE_CURVE('',#37278,#37277,#1166,.T.);
#47199=EDGE_CURVE('',#36797,#37278,#30641,.T.);
#47200=EDGE_CURVE('',#37279,#37278,#21490,.T.);
#47201=EDGE_CURVE('',#36798,#37279,#30642,.T.);
#47202=EDGE_CURVE('',#37280,#37279,#5014,.T.);
#47203=EDGE_CURVE('',#36808,#37280,#30643,.T.);
#47204=EDGE_CURVE('',#37281,#37280,#5015,.T.);
#47205=EDGE_CURVE('',#36805,#37281,#30644,.T.);
#47206=EDGE_CURVE('',#37282,#37281,#5016,.T.);
#47207=EDGE_CURVE('',#36804,#37282,#30645,.T.);
#47208=EDGE_CURVE('',#37283,#37282,#21491,.T.);
#47209=EDGE_CURVE('',#36799,#37283,#30646,.T.);
#47210=EDGE_CURVE('',#37284,#37283,#5017,.T.);
#47211=EDGE_CURVE('',#36801,#37284,#30647,.T.);
#47212=EDGE_CURVE('',#37285,#37284,#5018,.T.);
#47213=EDGE_CURVE('',#37286,#37285,#30648,.T.);
#47214=EDGE_CURVE('',#36801,#37286,#5019,.T.);
#47215=EDGE_CURVE('',#37287,#37288,#30649,.T.);
#47216=EDGE_CURVE('',#37289,#37288,#21492,.T.);
#47217=EDGE_CURVE('',#37290,#37289,#30650,.T.);
#47218=EDGE_CURVE('',#37287,#37290,#21493,.T.);
#47219=EDGE_CURVE('',#37288,#37285,#5020,.T.);
#47220=EDGE_CURVE('',#37286,#37287,#5021,.T.);
#47221=EDGE_CURVE('',#37286,#37291,#30651,.T.);
#47222=EDGE_CURVE('',#37291,#36802,#5022,.T.);
#47223=EDGE_CURVE('',#36892,#37292,#30652,.T.);
#47224=EDGE_CURVE('',#37293,#37292,#30653,.T.);
#47225=EDGE_CURVE('',#36890,#37293,#30654,.T.);
#47226=EDGE_CURVE('',#37294,#37293,#21494,.T.);
#47227=EDGE_CURVE('',#36981,#37294,#30655,.T.);
#47228=EDGE_CURVE('',#37295,#37296,#30656,.T.);
#47229=EDGE_CURVE('',#37297,#37296,#1901,.T.);
#47230=EDGE_CURVE('',#37298,#37297,#30657,.T.);
#47231=EDGE_CURVE('',#37295,#37298,#5023,.T.);
#47232=EDGE_CURVE('',#37299,#37297,#1902,.T.);
#47233=EDGE_CURVE('',#37291,#37299,#30658,.T.);
#47234=EDGE_CURVE('',#37298,#37291,#1903,.T.);
#47235=EDGE_CURVE('',#37300,#37299,#5024,.T.);
#47236=EDGE_CURVE('',#36802,#37300,#30659,.T.);
#47237=EDGE_CURVE('',#37301,#37300,#5025,.T.);
#47238=EDGE_CURVE('',#36800,#37301,#30660,.T.);
#47239=EDGE_CURVE('',#37302,#37301,#21495,.T.);
#47240=EDGE_CURVE('',#36803,#37302,#30661,.T.);
#47241=EDGE_CURVE('',#37303,#37302,#5026,.T.);
#47242=EDGE_CURVE('',#36806,#37303,#30662,.T.);
#47243=EDGE_CURVE('',#37304,#37303,#5027,.T.);
#47244=EDGE_CURVE('',#36807,#37304,#30663,.T.);
#47245=EDGE_CURVE('',#37305,#37304,#5028,.T.);
#47246=EDGE_CURVE('',#36809,#37305,#30664,.T.);
#47247=EDGE_CURVE('',#37306,#37305,#5029,.T.);
#47248=EDGE_CURVE('',#37122,#37306,#30665,.T.);
#47249=EDGE_CURVE('',#37125,#37306,#21496,.T.);
#47250=EDGE_CURVE('',#37122,#37124,#21497,.T.);
#47251=EDGE_CURVE('',#37292,#37125,#21498,.T.);
#47252=EDGE_CURVE('',#37156,#37307,#21499,.T.);
#47253=EDGE_CURVE('',#37308,#37154,#21500,.T.);
#47254=EDGE_CURVE('',#37308,#37307,#30666,.T.);
#47255=EDGE_CURVE('',#37309,#37142,#30667,.T.);
#47256=EDGE_CURVE('',#37310,#37142,#21501,.T.);
#47257=EDGE_CURVE('',#37311,#37310,#30668,.T.);
#47258=EDGE_CURVE('',#37309,#37311,#21502,.T.);
#47259=EDGE_CURVE('',#37312,#37144,#30669,.T.);
#47260=EDGE_CURVE('',#37312,#37309,#1167,.T.);
#47261=EDGE_CURVE('',#37144,#37140,#21503,.T.);
#47262=EDGE_CURVE('',#37141,#37312,#21504,.T.);
#47263=EDGE_CURVE('',#37313,#37141,#21505,.T.);
#47264=EDGE_CURVE('',#36829,#37313,#30670,.T.);
#47265=EDGE_CURVE('',#37314,#37313,#30671,.T.);
#47266=EDGE_CURVE('',#36826,#37314,#30672,.T.);
#47267=EDGE_CURVE('',#37315,#37314,#21506,.T.);
#47268=EDGE_CURVE('',#36827,#37315,#30673,.T.);
#47269=EDGE_CURVE('',#37316,#37317,#30674,.T.);
#47270=EDGE_CURVE('',#37318,#37316,#5030,.T.);
#47271=EDGE_CURVE('',#37319,#37318,#30675,.T.);
#47272=EDGE_CURVE('',#37320,#37319,#5031,.F.);
#47273=EDGE_CURVE('',#37317,#37320,#5032,.F.);
#47274=EDGE_CURVE('',#37321,#37322,#21507,.T.);
#47275=EDGE_CURVE('',#37321,#37166,#5033,.T.);
#47276=EDGE_CURVE('',#37165,#37322,#30676,.T.);
#47277=EDGE_CURVE('',#37323,#37315,#30677,.T.);
#47278=EDGE_CURVE('',#37324,#37323,#30678,.T.);
#47279=EDGE_CURVE('',#36827,#37324,#30679,.T.);
#47280=EDGE_CURVE('',#37325,#37324,#21508,.T.);
#47281=EDGE_CURVE('',#37325,#36828,#30680,.T.);
#47282=EDGE_CURVE('',#37326,#36813,#30681,.T.);
#47283=EDGE_CURVE('',#37327,#36812,#30682,.T.);
#47284=EDGE_CURVE('',#37326,#37327,#21509,.T.);
#47285=EDGE_CURVE('',#37328,#36815,#30683,.T.);
#47286=EDGE_CURVE('',#37328,#37326,#5034,.T.);
#47287=EDGE_CURVE('',#37329,#36817,#30684,.T.);
#47288=EDGE_CURVE('',#37329,#37328,#1168,.T.);
#47289=EDGE_CURVE('',#37330,#36819,#30685,.T.);
#47290=EDGE_CURVE('',#37330,#37329,#5035,.T.);
#47291=EDGE_CURVE('',#37331,#36821,#30686,.T.);
#47292=EDGE_CURVE('',#37331,#37330,#21510,.T.);
#47293=EDGE_CURVE('',#37332,#36823,#30687,.T.);
#47294=EDGE_CURVE('',#37332,#37331,#5036,.T.);
#47295=EDGE_CURVE('',#37333,#36833,#30688,.T.);
#47296=EDGE_CURVE('',#37333,#37332,#1169,.T.);
#47297=EDGE_CURVE('',#37334,#37335,#30689,.T.);
#47298=EDGE_CURVE('',#36833,#37335,#5037,.T.);
#47299=EDGE_CURVE('',#37334,#37333,#5038,.T.);
#47300=EDGE_CURVE('',#37325,#37336,#30690,.T.);
#47301=EDGE_CURVE('',#37337,#37336,#30691,.T.);
#47302=EDGE_CURVE('',#36828,#37337,#30692,.T.);
#47303=EDGE_CURVE('',#37338,#37337,#21511,.T.);
#47304=EDGE_CURVE('',#36825,#37338,#30693,.T.);
#47305=EDGE_CURVE('',#37339,#37338,#30694,.T.);
#47306=EDGE_CURVE('',#36830,#37339,#30695,.T.);
#47307=EDGE_CURVE('',#37136,#37339,#21512,.T.);
#47308=EDGE_CURVE('',#37340,#37134,#30696,.T.);
#47309=EDGE_CURVE('',#37137,#37134,#21513,.T.);
#47310=EDGE_CURVE('',#37341,#37136,#21514,.T.);
#47311=EDGE_CURVE('',#37341,#37340,#30697,.T.);
#47312=EDGE_CURVE('',#37327,#37341,#1170,.T.);
#47313=EDGE_CURVE('',#37342,#37260,#21515,.T.);
#47314=EDGE_CURVE('',#37343,#37342,#30698,.T.);
#47315=EDGE_CURVE('',#37261,#37343,#21516,.T.);
#47316=EDGE_CURVE('',#37344,#37345,#30699,.T.);
#47317=EDGE_CURVE('',#37335,#37345,#21517,.T.);
#47318=EDGE_CURVE('',#37344,#37334,#21518,.T.);
#47319=EDGE_CURVE('',#37260,#37335,#30700,.T.);
#47320=EDGE_CURVE('',#37346,#37347,#30701,.T.);
#47321=EDGE_CURVE('',#37348,#37347,#5039,.T.);
#47322=EDGE_CURVE('',#36838,#37348,#30702,.T.);
#47323=EDGE_CURVE('',#37346,#36838,#5040,.T.);
#47324=EDGE_CURVE('',#37349,#37348,#1171,.T.);
#47325=EDGE_CURVE('',#36835,#37349,#30703,.T.);
#47326=EDGE_CURVE('',#37350,#37349,#5041,.T.);
#47327=EDGE_CURVE('',#37158,#37350,#30704,.T.);
#47328=EDGE_CURVE('',#37351,#37350,#21519,.T.);
#47329=EDGE_CURVE('',#37352,#37351,#30705,.T.);
#47330=EDGE_CURVE('',#37158,#37352,#21520,.T.);
#47331=EDGE_CURVE('',#37353,#37354,#30706,.T.);
#47332=EDGE_CURVE('',#37355,#37354,#30707,.T.);
#47333=EDGE_CURVE('',#37356,#37355,#30708,.T.);
#47334=EDGE_CURVE('',#37353,#37356,#30709,.T.);
#47335=EDGE_CURVE('',#37357,#37356,#21521,.T.);
#47336=EDGE_CURVE('',#37357,#37358,#30710,.T.);
#47337=EDGE_CURVE('',#37353,#37358,#21522,.T.);
#47338=EDGE_CURVE('',#37357,#37359,#30711,.T.);
#47339=EDGE_CURVE('',#37360,#37359,#30712,.T.);
#47340=EDGE_CURVE('',#37358,#37360,#30713,.T.);
#47341=EDGE_CURVE('',#37361,#37360,#21523,.T.);
#47342=EDGE_CURVE('',#37361,#37362,#5042,.T.);
#47343=EDGE_CURVE('',#37358,#37362,#21524,.T.);
#47344=EDGE_CURVE('',#37167,#37363,#5043,.T.);
#47345=EDGE_CURVE('',#37364,#37363,#21525,.T.);
#47346=EDGE_CURVE('',#37364,#37168,#30714,.T.);
#47347=EDGE_CURVE('',#37365,#37366,#30715,.T.);
#47348=EDGE_CURVE('',#37367,#37366,#5044,.T.);
#47349=EDGE_CURVE('',#37162,#37367,#30716,.T.);
#47350=EDGE_CURVE('',#37365,#37162,#5045,.T.);
#47351=EDGE_CURVE('',#37368,#37367,#5046,.T.);
#47352=EDGE_CURVE('',#37160,#37368,#30717,.T.);
#47353=EDGE_CURVE('',#37369,#37368,#21526,.T.);
#47354=EDGE_CURVE('',#37370,#37369,#30718,.T.);
#47355=EDGE_CURVE('',#37160,#37370,#21527,.T.);
#47356=EDGE_CURVE('',#37371,#37372,#30719,.T.);
#47357=EDGE_CURVE('',#37373,#37372,#30720,.T.);
#47358=EDGE_CURVE('',#37374,#37373,#30721,.T.);
#47359=EDGE_CURVE('',#37371,#37374,#30722,.T.);
#47360=EDGE_CURVE('',#37371,#37375,#21528,.T.);
#47361=EDGE_CURVE('',#37376,#37374,#21529,.T.);
#47362=EDGE_CURVE('',#37376,#37375,#30723,.T.);
#47363=EDGE_CURVE('',#37376,#37377,#30724,.T.);
#47364=EDGE_CURVE('',#37378,#37377,#30725,.T.);
#47365=EDGE_CURVE('',#37375,#37378,#30726,.T.);
#47366=EDGE_CURVE('',#37379,#37157,#30727,.T.);
#47367=EDGE_CURVE('',#37380,#37157,#21530,.T.);
#47368=EDGE_CURVE('',#37381,#37380,#30728,.T.);
#47369=EDGE_CURVE('',#37379,#37381,#21531,.T.);
#47370=EDGE_CURVE('',#37382,#36836,#30729,.T.);
#47371=EDGE_CURVE('',#37382,#37379,#5047,.T.);
#47372=EDGE_CURVE('',#37383,#36837,#30730,.T.);
#47373=EDGE_CURVE('',#37383,#37382,#5048,.T.);
#47374=EDGE_CURVE('',#37384,#37385,#30731,.T.);
#47375=EDGE_CURVE('',#36837,#37385,#5049,.T.);
#47376=EDGE_CURVE('',#37384,#37383,#5050,.T.);
#47377=EDGE_CURVE('',#37386,#37387,#30732,.T.);
#47378=EDGE_CURVE('',#37347,#37387,#21532,.T.);
#47379=EDGE_CURVE('',#37386,#37346,#21533,.T.);
#47380=EDGE_CURVE('',#37388,#37389,#30733,.T.);
#47381=EDGE_CURVE('',#37385,#37389,#21534,.T.);
#47382=EDGE_CURVE('',#37388,#37384,#21535,.T.);
#47383=EDGE_CURVE('',#37346,#37385,#30734,.T.);
#47384=EDGE_CURVE('',#36847,#37390,#30735,.T.);
#47385=EDGE_CURVE('',#37391,#37390,#30736,.T.);
#47386=EDGE_CURVE('',#36845,#37391,#30737,.T.);
#47387=EDGE_CURVE('',#37392,#37391,#21536,.T.);
#47388=EDGE_CURVE('',#36842,#37392,#30738,.T.);
#47389=EDGE_CURVE('',#37393,#36886,#30739,.T.);
#47390=EDGE_CURVE('',#37394,#36886,#5051,.T.);
#47391=EDGE_CURVE('',#37395,#37394,#30740,.T.);
#47392=EDGE_CURVE('',#37393,#37395,#5052,.T.);
#47393=EDGE_CURVE('',#37396,#36887,#30741,.T.);
#47394=EDGE_CURVE('',#37396,#37393,#5053,.T.);
#47395=EDGE_CURVE('',#37397,#36876,#30742,.T.);
#47396=EDGE_CURVE('',#37397,#37396,#5054,.T.);
#47397=EDGE_CURVE('',#37398,#36874,#30743,.T.);
#47398=EDGE_CURVE('',#37398,#37397,#21537,.T.);
#47399=EDGE_CURVE('',#37399,#36840,#30744,.T.);
#47400=EDGE_CURVE('',#37399,#37398,#5055,.T.);
#47401=EDGE_CURVE('',#37400,#36841,#30745,.T.);
#47402=EDGE_CURVE('',#37400,#37399,#5056,.T.);
#47403=EDGE_CURVE('',#37401,#36870,#30746,.T.);
#47404=EDGE_CURVE('',#37401,#37400,#5057,.T.);
#47405=EDGE_CURVE('',#37402,#36867,#30747,.T.);
#47406=EDGE_CURVE('',#37402,#37401,#21538,.T.);
#47407=EDGE_CURVE('',#37403,#37027,#30748,.T.);
#47408=EDGE_CURVE('',#37403,#37402,#1172,.T.);
#47409=EDGE_CURVE('',#37027,#37024,#21539,.T.);
#47410=EDGE_CURVE('',#37025,#37403,#21540,.T.);
#47411=EDGE_CURVE('',#37390,#37025,#21541,.T.);
#47412=EDGE_CURVE('',#37404,#37392,#30749,.T.);
#47413=EDGE_CURVE('',#37405,#37404,#30750,.T.);
#47414=EDGE_CURVE('',#36842,#37405,#30751,.T.);
#47415=EDGE_CURVE('',#37406,#37405,#21542,.T.);
#47416=EDGE_CURVE('',#37406,#36843,#30752,.T.);
#47417=EDGE_CURVE('',#37406,#37407,#30753,.T.);
#47418=EDGE_CURVE('',#37408,#37407,#30754,.T.);
#47419=EDGE_CURVE('',#36843,#37408,#30755,.T.);
#47420=EDGE_CURVE('',#37409,#37408,#21543,.T.);
#47421=EDGE_CURVE('',#36844,#37409,#30756,.T.);
#47422=EDGE_CURVE('',#37410,#37409,#30757,.T.);
#47423=EDGE_CURVE('',#36846,#37410,#30758,.T.);
#47424=EDGE_CURVE('',#37021,#37410,#21544,.T.);
#47425=EDGE_CURVE('',#37411,#37021,#21545,.T.);
#47426=EDGE_CURVE('',#37019,#37411,#30759,.T.);
#47427=EDGE_CURVE('',#37022,#37019,#21546,.T.);
#47428=EDGE_CURVE('',#37412,#37411,#1173,.T.);
#47429=EDGE_CURVE('',#36851,#37412,#30760,.T.);
#47430=EDGE_CURVE('',#37413,#37412,#21547,.T.);
#47431=EDGE_CURVE('',#36852,#37413,#30761,.T.);
#47432=EDGE_CURVE('',#37414,#37413,#5058,.T.);
#47433=EDGE_CURVE('',#36862,#37414,#30762,.T.);
#47434=EDGE_CURVE('',#37415,#37414,#5059,.T.);
#47435=EDGE_CURVE('',#36859,#37415,#30763,.T.);
#47436=EDGE_CURVE('',#37416,#37415,#5060,.T.);
#47437=EDGE_CURVE('',#36858,#37416,#30764,.T.);
#47438=EDGE_CURVE('',#37417,#37416,#21548,.T.);
#47439=EDGE_CURVE('',#36853,#37417,#30765,.T.);
#47440=EDGE_CURVE('',#37418,#37417,#5061,.T.);
#47441=EDGE_CURVE('',#36855,#37418,#30766,.T.);
#47442=EDGE_CURVE('',#37419,#37418,#5062,.T.);
#47443=EDGE_CURVE('',#37420,#37419,#30767,.T.);
#47444=EDGE_CURVE('',#36855,#37420,#5063,.T.);
#47445=EDGE_CURVE('',#37421,#37422,#30768,.T.);
#47446=EDGE_CURVE('',#37423,#37422,#21549,.T.);
#47447=EDGE_CURVE('',#37424,#37423,#30769,.T.);
#47448=EDGE_CURVE('',#37421,#37424,#21550,.T.);
#47449=EDGE_CURVE('',#37422,#37419,#5064,.T.);
#47450=EDGE_CURVE('',#37420,#37421,#5065,.T.);
#47451=EDGE_CURVE('',#37420,#37425,#30770,.T.);
#47452=EDGE_CURVE('',#37425,#36856,#5066,.T.);
#47453=EDGE_CURVE('',#37002,#37426,#30771,.T.);
#47454=EDGE_CURVE('',#37427,#37426,#30772,.T.);
#47455=EDGE_CURVE('',#37000,#37427,#30773,.T.);
#47456=EDGE_CURVE('',#37428,#37427,#21551,.T.);
#47457=EDGE_CURVE('',#37163,#37428,#30774,.T.);
#47458=EDGE_CURVE('',#37429,#36856,#30775,.T.);
#47459=EDGE_CURVE('',#37430,#37425,#30776,.T.);
#47460=EDGE_CURVE('',#37429,#37430,#5067,.T.);
#47461=EDGE_CURVE('',#37431,#36854,#30777,.T.);
#47462=EDGE_CURVE('',#37431,#37429,#5068,.T.);
#47463=EDGE_CURVE('',#37432,#36857,#30778,.T.);
#47464=EDGE_CURVE('',#37432,#37431,#21552,.T.);
#47465=EDGE_CURVE('',#37433,#36860,#30779,.T.);
#47466=EDGE_CURVE('',#37433,#37432,#5069,.T.);
#47467=EDGE_CURVE('',#37434,#36861,#30780,.T.);
#47468=EDGE_CURVE('',#37434,#37433,#5070,.T.);
#47469=EDGE_CURVE('',#37435,#37003,#30781,.T.);
#47470=EDGE_CURVE('',#37435,#37434,#5071,.T.);
#47471=EDGE_CURVE('',#37436,#37437,#30782,.T.);
#47472=EDGE_CURVE('',#37003,#37437,#5072,.T.);
#47473=EDGE_CURVE('',#37436,#37435,#5073,.T.);
#47474=EDGE_CURVE('',#37438,#37425,#5074,.T.);
#47475=EDGE_CURVE('',#37439,#37438,#30783,.T.);
#47476=EDGE_CURVE('',#37430,#37439,#1904,.T.);
#47477=EDGE_CURVE('',#37440,#37034,#30784,.T.);
#47478=EDGE_CURVE('',#37441,#37034,#21553,.T.);
#47479=EDGE_CURVE('',#37442,#37441,#30785,.T.);
#47480=EDGE_CURVE('',#37440,#37442,#21554,.T.);
#47481=EDGE_CURVE('',#37443,#37036,#30786,.T.);
#47482=EDGE_CURVE('',#37443,#37440,#1174,.T.);
#47483=EDGE_CURVE('',#37036,#37032,#21555,.T.);
#47484=EDGE_CURVE('',#37033,#37443,#21556,.T.);
#47485=EDGE_CURVE('',#37444,#37033,#21557,.T.);
#47486=EDGE_CURVE('',#37444,#36881,#30787,.T.);
#47487=EDGE_CURVE('',#37445,#36878,#30788,.T.);
#47488=EDGE_CURVE('',#37445,#37444,#30789,.T.);
#47489=EDGE_CURVE('',#37446,#36879,#30790,.T.);
#47490=EDGE_CURVE('',#37446,#37445,#21558,.T.);
#47491=EDGE_CURVE('',#37447,#37448,#30791,.T.);
#47492=EDGE_CURVE('',#37449,#37448,#5075,.T.);
#47493=EDGE_CURVE('',#37169,#37449,#30792,.T.);
#47494=EDGE_CURVE('',#37447,#37169,#5076,.T.);
#47495=EDGE_CURVE('',#36864,#37449,#21559,.T.);
#47496=EDGE_CURVE('',#37013,#36864,#21560,.T.);
#47497=EDGE_CURVE('',#36865,#37016,#21561,.T.);
#47498=EDGE_CURVE('',#37450,#37451,#30793,.T.);
#47499=EDGE_CURVE('',#37014,#37451,#21562,.T.);
#47500=EDGE_CURVE('',#37450,#37013,#21563,.T.);
#47501=EDGE_CURVE('',#37452,#37453,#30794,.T.);
#47502=EDGE_CURVE('',#36879,#37453,#30795,.T.);
#47503=EDGE_CURVE('',#37452,#37446,#30796,.T.);
#47504=EDGE_CURVE('',#37454,#37453,#21564,.T.);
#47505=EDGE_CURVE('',#37454,#36880,#30797,.T.);
#47506=EDGE_CURVE('',#37455,#36869,#30798,.T.);
#47507=EDGE_CURVE('',#37456,#36868,#30799,.T.);
#47508=EDGE_CURVE('',#37455,#37456,#21565,.T.);
#47509=EDGE_CURVE('',#37457,#36871,#30800,.T.);
#47510=EDGE_CURVE('',#37457,#37455,#5077,.T.);
#47511=EDGE_CURVE('',#37458,#36872,#30801,.T.);
#47512=EDGE_CURVE('',#37458,#37457,#5078,.T.);
#47513=EDGE_CURVE('',#37459,#36873,#30802,.T.);
#47514=EDGE_CURVE('',#37459,#37458,#5079,.T.);
#47515=EDGE_CURVE('',#37460,#37459,#21566,.T.);
#47516=EDGE_CURVE('',#36875,#37460,#30803,.T.);
#47517=EDGE_CURVE('',#37461,#37460,#5080,.T.);
#47518=EDGE_CURVE('',#36888,#37461,#30804,.T.);
#47519=EDGE_CURVE('',#37462,#37461,#5081,.T.);
#47520=EDGE_CURVE('',#37463,#37462,#30805,.T.);
#47521=EDGE_CURVE('',#36888,#37463,#5082,.T.);
#47522=EDGE_CURVE('',#37454,#37464,#30806,.T.);
#47523=EDGE_CURVE('',#37465,#37464,#30807,.T.);
#47524=EDGE_CURVE('',#36880,#37465,#30808,.T.);
#47525=EDGE_CURVE('',#37466,#37465,#21567,.T.);
#47526=EDGE_CURVE('',#36877,#37466,#30809,.T.);
#47527=EDGE_CURVE('',#37467,#37466,#30810,.T.);
#47528=EDGE_CURVE('',#36882,#37467,#30811,.T.);
#47529=EDGE_CURVE('',#37028,#37467,#21568,.T.);
#47530=EDGE_CURVE('',#37468,#37026,#30812,.T.);
#47531=EDGE_CURVE('',#37029,#37026,#21569,.T.);
#47532=EDGE_CURVE('',#37469,#37028,#21570,.T.);
#47533=EDGE_CURVE('',#37469,#37468,#30813,.T.);
#47534=EDGE_CURVE('',#37456,#37469,#1175,.T.);
#47535=EDGE_CURVE('',#37394,#37470,#30814,.T.);
#47536=EDGE_CURVE('',#37470,#36885,#30815,.T.);
#47537=EDGE_CURVE('',#37471,#37394,#21571,.T.);
#47538=EDGE_CURVE('',#37472,#37471,#30816,.T.);
#47539=EDGE_CURVE('',#37395,#37472,#21572,.T.);
#47540=EDGE_CURVE('',#37473,#37462,#21573,.T.);
#47541=EDGE_CURVE('',#37474,#37473,#30817,.T.);
#47542=EDGE_CURVE('',#37463,#37474,#21574,.T.);
#47543=EDGE_CURVE('',#37470,#37463,#5083,.T.);
#47544=EDGE_CURVE('',#37475,#36899,#30818,.T.);
#47545=EDGE_CURVE('',#37476,#36902,#30819,.T.);
#47546=EDGE_CURVE('',#37475,#37476,#5084,.T.);
#47547=EDGE_CURVE('',#37477,#36896,#30820,.T.);
#47548=EDGE_CURVE('',#37477,#37475,#5085,.T.);
#47549=EDGE_CURVE('',#37478,#36897,#30821,.T.);
#47550=EDGE_CURVE('',#37478,#37477,#21575,.T.);
#47551=EDGE_CURVE('',#37479,#37480,#30822,.T.);
#47552=EDGE_CURVE('',#36897,#37480,#5086,.T.);
#47553=EDGE_CURVE('',#37479,#37478,#5087,.T.);
#47554=EDGE_CURVE('',#36982,#37481,#30823,.T.);
#47555=EDGE_CURVE('',#37482,#37481,#21576,.T.);
#47556=EDGE_CURVE('',#36889,#37482,#30824,.T.);
#47557=EDGE_CURVE('',#37483,#37482,#30825,.T.);
#47558=EDGE_CURVE('',#36891,#37483,#30826,.T.);
#47559=EDGE_CURVE('',#37116,#37483,#21577,.T.);
#47560=EDGE_CURVE('',#37484,#37114,#30827,.T.);
#47561=EDGE_CURVE('',#37117,#37114,#21578,.T.);
#47562=EDGE_CURVE('',#37484,#37116,#21579,.T.);
#47563=EDGE_CURVE('',#37476,#37484,#1905,.T.);
#47564=EDGE_CURVE('',#37485,#37486,#30828,.T.);
#47565=EDGE_CURVE('',#37480,#37486,#5088,.T.);
#47566=EDGE_CURVE('',#37485,#37479,#5089,.T.);
#47567=EDGE_CURVE('',#37487,#37480,#5090,.T.);
#47568=EDGE_CURVE('',#37487,#36898,#5091,.T.);
#47569=EDGE_CURVE('',#37488,#36898,#30829,.T.);
#47570=EDGE_CURVE('',#37489,#37487,#30830,.T.);
#47571=EDGE_CURVE('',#37488,#37489,#5092,.T.);
#47572=EDGE_CURVE('',#37490,#36895,#30831,.T.);
#47573=EDGE_CURVE('',#37490,#37488,#21580,.T.);
#47574=EDGE_CURVE('',#37491,#37490,#5093,.T.);
#47575=EDGE_CURVE('',#36900,#37491,#30832,.T.);
#47576=EDGE_CURVE('',#37492,#37491,#5094,.T.);
#47577=EDGE_CURVE('',#36901,#37492,#30833,.T.);
#47578=EDGE_CURVE('',#37493,#37492,#1906,.T.);
#47579=EDGE_CURVE('',#37115,#37493,#30834,.T.);
#47580=EDGE_CURVE('',#37113,#37493,#21581,.T.);
#47581=EDGE_CURVE('',#37115,#37112,#21582,.T.);
#47582=EDGE_CURVE('',#37494,#37113,#21583,.T.);
#47583=EDGE_CURVE('',#36906,#37494,#30835,.T.);
#47584=EDGE_CURVE('',#37495,#37494,#30836,.T.);
#47585=EDGE_CURVE('',#36910,#37495,#30837,.T.);
#47586=EDGE_CURVE('',#37496,#37495,#21584,.T.);
#47587=EDGE_CURVE('',#36907,#37496,#30838,.T.);
#47588=EDGE_CURVE('',#37497,#37487,#5095,.T.);
#47589=EDGE_CURVE('',#37498,#37497,#30839,.T.);
#47590=EDGE_CURVE('',#37489,#37498,#5096,.T.);
#47591=EDGE_CURVE('',#37499,#37496,#30840,.T.);
#47592=EDGE_CURVE('',#37500,#37499,#30841,.T.);
#47593=EDGE_CURVE('',#36907,#37500,#30842,.T.);
#47594=EDGE_CURVE('',#37501,#37500,#21585,.T.);
#47595=EDGE_CURVE('',#37501,#36908,#30843,.T.);
#47596=EDGE_CURVE('',#37501,#37502,#30844,.T.);
#47597=EDGE_CURVE('',#37503,#37502,#30845,.T.);
#47598=EDGE_CURVE('',#36908,#37503,#30846,.T.);
#47599=EDGE_CURVE('',#37504,#37503,#21586,.T.);
#47600=EDGE_CURVE('',#36909,#37504,#30847,.T.);
#47601=EDGE_CURVE('',#37108,#37504,#30848,.T.);
#47602=EDGE_CURVE('',#37505,#37108,#21587,.T.);
#47603=EDGE_CURVE('',#37105,#37505,#30849,.T.);
#47604=EDGE_CURVE('',#37109,#37105,#21588,.T.);
#47605=EDGE_CURVE('',#37506,#37505,#1907,.T.);
#47606=EDGE_CURVE('',#36919,#37506,#30850,.T.);
#47607=EDGE_CURVE('',#37507,#37506,#5097,.T.);
#47608=EDGE_CURVE('',#36916,#37507,#30851,.T.);
#47609=EDGE_CURVE('',#37508,#37507,#5098,.T.);
#47610=EDGE_CURVE('',#36915,#37508,#30852,.T.);
#47611=EDGE_CURVE('',#37509,#37508,#21589,.T.);
#47612=EDGE_CURVE('',#36912,#37509,#30853,.T.);
#47613=EDGE_CURVE('',#37510,#37511,#30854,.T.);
#47614=EDGE_CURVE('',#36912,#37511,#5099,.T.);
#47615=EDGE_CURVE('',#37510,#37509,#5100,.T.);
#47616=EDGE_CURVE('',#37512,#37513,#30855,.T.);
#47617=EDGE_CURVE('',#37511,#37513,#5101,.T.);
#47618=EDGE_CURVE('',#37512,#37510,#5102,.T.);
#47619=EDGE_CURVE('',#37514,#37511,#5103,.T.);
#47620=EDGE_CURVE('',#37514,#36913,#5104,.T.);
#47621=EDGE_CURVE('',#37515,#36913,#30856,.T.);
#47622=EDGE_CURVE('',#37516,#37514,#30857,.T.);
#47623=EDGE_CURVE('',#37515,#37516,#5105,.T.);
#47624=EDGE_CURVE('',#37517,#36914,#30858,.T.);
#47625=EDGE_CURVE('',#37517,#37515,#21590,.T.);
#47626=EDGE_CURVE('',#37518,#36917,#30859,.T.);
#47627=EDGE_CURVE('',#37518,#37517,#5106,.T.);
#47628=EDGE_CURVE('',#37519,#36918,#30860,.T.);
#47629=EDGE_CURVE('',#37519,#37518,#5107,.T.);
#47630=EDGE_CURVE('',#37520,#37106,#30861,.T.);
#47631=EDGE_CURVE('',#37520,#37519,#1908,.T.);
#47632=EDGE_CURVE('',#37106,#37103,#21591,.T.);
#47633=EDGE_CURVE('',#37104,#37520,#21592,.T.);
#47634=EDGE_CURVE('',#37521,#37104,#5108,.T.);
#47635=EDGE_CURVE('',#37521,#36923,#30862,.T.);
#47636=EDGE_CURVE('',#37522,#37514,#5109,.T.);
#47637=EDGE_CURVE('',#37523,#37522,#30863,.T.);
#47638=EDGE_CURVE('',#37516,#37523,#5110,.T.);
#47639=EDGE_CURVE('',#37524,#37525,#30864,.T.);
#47640=EDGE_CURVE('',#36923,#37525,#21593,.T.);
#47641=EDGE_CURVE('',#37524,#37521,#21594,.T.);
#47642=EDGE_CURVE('',#37525,#37526,#5111,.T.);
#47643=EDGE_CURVE('',#37526,#36920,#21595,.T.);
#47644=EDGE_CURVE('',#37526,#37527,#30865,.T.);
#47645=EDGE_CURVE('',#37528,#37527,#21596,.T.);
#47646=EDGE_CURVE('',#36920,#37528,#30866,.T.);
#47647=EDGE_CURVE('',#37100,#37528,#5112,.T.);
#47648=EDGE_CURVE('',#37529,#37100,#21597,.T.);
#47649=EDGE_CURVE('',#37097,#37529,#30867,.T.);
#47650=EDGE_CURVE('',#37101,#37097,#21598,.T.);
#47651=EDGE_CURVE('',#37530,#37529,#1909,.T.);
#47652=EDGE_CURVE('',#36931,#37530,#30868,.T.);
#47653=EDGE_CURVE('',#37531,#37530,#1176,.T.);
#47654=EDGE_CURVE('',#36928,#37531,#30869,.T.);
#47655=EDGE_CURVE('',#37532,#37531,#5113,.T.);
#47656=EDGE_CURVE('',#36925,#37532,#30870,.T.);
#47657=EDGE_CURVE('',#37533,#37532,#21599,.T.);
#47658=EDGE_CURVE('',#36926,#37533,#30871,.T.);
#47659=EDGE_CURVE('',#37534,#37533,#5114,.T.);
#47660=EDGE_CURVE('',#37535,#37534,#30872,.T.);
#47661=EDGE_CURVE('',#36926,#37535,#5115,.T.);
#47662=EDGE_CURVE('',#37536,#37534,#1177,.T.);
#47663=EDGE_CURVE('',#37537,#37536,#30873,.T.);
#47664=EDGE_CURVE('',#37535,#37537,#5116,.T.);
#47665=EDGE_CURVE('',#37538,#37535,#5117,.T.);
#47666=EDGE_CURVE('',#37538,#36927,#1910,.T.);
#47667=EDGE_CURVE('',#37539,#36927,#30874,.T.);
#47668=EDGE_CURVE('',#37540,#37538,#30875,.T.);
#47669=EDGE_CURVE('',#37539,#37540,#1911,.T.);
#47670=EDGE_CURVE('',#37541,#36924,#30876,.T.);
#47671=EDGE_CURVE('',#37541,#37539,#21600,.T.);
#47672=EDGE_CURVE('',#37542,#36929,#30877,.T.);
#47673=EDGE_CURVE('',#37542,#37541,#1912,.T.);
#47674=EDGE_CURVE('',#37543,#36930,#30878,.T.);
#47675=EDGE_CURVE('',#37543,#37542,#5118,.T.);
#47676=EDGE_CURVE('',#37544,#37098,#30879,.T.);
#47677=EDGE_CURVE('',#37544,#37543,#1913,.T.);
#47678=EDGE_CURVE('',#37098,#37095,#21601,.T.);
#47679=EDGE_CURVE('',#37096,#37544,#21602,.T.);
#47680=EDGE_CURVE('',#37545,#37096,#5119,.T.);
#47681=EDGE_CURVE('',#37545,#36935,#30880,.T.);
#47682=EDGE_CURVE('',#37546,#37538,#5120,.T.);
#47683=EDGE_CURVE('',#37547,#37546,#30881,.T.);
#47684=EDGE_CURVE('',#37540,#37547,#1178,.T.);
#47685=EDGE_CURVE('',#37548,#37549,#30882,.T.);
#47686=EDGE_CURVE('',#36935,#37549,#21603,.T.);
#47687=EDGE_CURVE('',#37548,#37545,#21604,.T.);
#47688=EDGE_CURVE('',#37549,#37550,#30883,.T.);
#47689=EDGE_CURVE('',#37550,#36932,#21605,.T.);
#47690=EDGE_CURVE('',#37550,#37551,#30884,.T.);
#47691=EDGE_CURVE('',#37552,#37551,#21606,.T.);
#47692=EDGE_CURVE('',#36932,#37552,#30885,.T.);
#47693=EDGE_CURVE('',#37092,#37552,#5121,.T.);
#47694=EDGE_CURVE('',#37553,#37092,#21607,.T.);
#47695=EDGE_CURVE('',#37089,#37553,#30886,.T.);
#47696=EDGE_CURVE('',#37093,#37089,#21608,.T.);
#47697=EDGE_CURVE('',#37554,#37553,#1914,.T.);
#47698=EDGE_CURVE('',#36943,#37554,#30887,.T.);
#47699=EDGE_CURVE('',#37555,#37554,#1179,.T.);
#47700=EDGE_CURVE('',#36940,#37555,#30888,.T.);
#47701=EDGE_CURVE('',#37556,#37555,#1915,.T.);
#47702=EDGE_CURVE('',#36937,#37556,#30889,.T.);
#47703=EDGE_CURVE('',#37557,#37556,#21609,.T.);
#47704=EDGE_CURVE('',#36938,#37557,#30890,.T.);
#47705=EDGE_CURVE('',#37558,#37557,#1916,.T.);
#47706=EDGE_CURVE('',#37559,#37558,#30891,.T.);
#47707=EDGE_CURVE('',#36938,#37559,#1917,.T.);
#47708=EDGE_CURVE('',#37560,#37558,#1180,.T.);
#47709=EDGE_CURVE('',#37561,#37560,#30892,.T.);
#47710=EDGE_CURVE('',#37559,#37561,#5122,.T.);
#47711=EDGE_CURVE('',#37562,#37559,#5123,.T.);
#47712=EDGE_CURVE('',#37562,#36939,#5124,.T.);
#47713=EDGE_CURVE('',#37563,#36939,#30893,.T.);
#47714=EDGE_CURVE('',#37564,#37562,#30894,.T.);
#47715=EDGE_CURVE('',#37563,#37564,#5125,.T.);
#47716=EDGE_CURVE('',#37565,#36936,#30895,.T.);
#47717=EDGE_CURVE('',#37565,#37563,#21610,.T.);
#47718=EDGE_CURVE('',#37566,#36941,#30896,.T.);
#47719=EDGE_CURVE('',#37566,#37565,#5126,.T.);
#47720=EDGE_CURVE('',#37567,#36942,#30897,.T.);
#47721=EDGE_CURVE('',#37567,#37566,#1181,.T.);
#47722=EDGE_CURVE('',#37568,#37090,#30898,.T.);
#47723=EDGE_CURVE('',#37568,#37567,#1918,.T.);
#47724=EDGE_CURVE('',#37090,#37087,#21611,.T.);
#47725=EDGE_CURVE('',#37088,#37568,#21612,.T.);
#47726=EDGE_CURVE('',#37569,#37088,#5127,.T.);
#47727=EDGE_CURVE('',#36947,#37569,#30899,.T.);
#47728=EDGE_CURVE('',#37570,#37562,#5128,.T.);
#47729=EDGE_CURVE('',#37571,#37570,#30900,.T.);
#47730=EDGE_CURVE('',#37564,#37571,#1182,.T.);
#47731=EDGE_CURVE('',#37572,#37569,#21613,.T.);
#47732=EDGE_CURVE('',#37573,#37572,#30901,.T.);
#47733=EDGE_CURVE('',#36947,#37573,#21614,.T.);
#47734=EDGE_CURVE('',#37573,#37574,#5129,.T.);
#47735=EDGE_CURVE('',#37574,#36944,#21615,.T.);
#47736=EDGE_CURVE('',#37574,#37575,#30902,.T.);
#47737=EDGE_CURVE('',#37576,#37575,#21616,.T.);
#47738=EDGE_CURVE('',#36944,#37576,#30903,.T.);
#47739=EDGE_CURVE('',#37084,#37576,#5130,.T.);
#47740=EDGE_CURVE('',#37577,#37084,#21617,.T.);
#47741=EDGE_CURVE('',#37081,#37577,#30904,.T.);
#47742=EDGE_CURVE('',#37085,#37081,#21618,.T.);
#47743=EDGE_CURVE('',#37578,#37577,#1919,.T.);
#47744=EDGE_CURVE('',#36955,#37578,#30905,.T.);
#47745=EDGE_CURVE('',#37579,#37578,#5131,.T.);
#47746=EDGE_CURVE('',#36952,#37579,#30906,.T.);
#47747=EDGE_CURVE('',#37580,#37579,#5132,.T.);
#47748=EDGE_CURVE('',#36949,#37580,#30907,.T.);
#47749=EDGE_CURVE('',#37581,#37580,#21619,.T.);
#47750=EDGE_CURVE('',#36950,#37581,#30908,.T.);
#47751=EDGE_CURVE('',#37582,#37581,#5133,.T.);
#47752=EDGE_CURVE('',#37583,#37582,#30909,.T.);
#47753=EDGE_CURVE('',#36950,#37583,#5134,.T.);
#47754=EDGE_CURVE('',#37584,#37582,#5135,.T.);
#47755=EDGE_CURVE('',#37585,#37584,#30910,.T.);
#47756=EDGE_CURVE('',#37583,#37585,#5136,.T.);
#47757=EDGE_CURVE('',#37586,#37583,#5137,.T.);
#47758=EDGE_CURVE('',#37586,#36951,#5138,.T.);
#47759=EDGE_CURVE('',#37587,#36951,#30911,.T.);
#47760=EDGE_CURVE('',#37588,#37586,#30912,.T.);
#47761=EDGE_CURVE('',#37587,#37588,#5139,.T.);
#47762=EDGE_CURVE('',#37589,#36948,#30913,.T.);
#47763=EDGE_CURVE('',#37589,#37587,#21620,.T.);
#47764=EDGE_CURVE('',#37590,#37589,#5140,.T.);
#47765=EDGE_CURVE('',#36953,#37590,#30914,.T.);
#47766=EDGE_CURVE('',#37591,#37590,#5141,.T.);
#47767=EDGE_CURVE('',#36954,#37591,#30915,.T.);
#47768=EDGE_CURVE('',#37592,#37591,#1920,.T.);
#47769=EDGE_CURVE('',#37082,#37592,#30916,.T.);
#47770=EDGE_CURVE('',#37080,#37592,#21621,.T.);
#47771=EDGE_CURVE('',#37082,#37079,#21622,.T.);
#47772=EDGE_CURVE('',#37593,#37080,#30917,.T.);
#47773=EDGE_CURVE('',#36962,#37593,#30918,.T.);
#47774=EDGE_CURVE('',#37594,#37593,#21623,.T.);
#47775=EDGE_CURVE('',#36959,#37594,#30919,.T.);
#47776=EDGE_CURVE('',#37595,#37586,#5142,.T.);
#47777=EDGE_CURVE('',#37596,#37595,#30920,.T.);
#47778=EDGE_CURVE('',#37588,#37596,#5143,.T.);
#47779=EDGE_CURVE('',#37597,#37594,#30921,.T.);
#47780=EDGE_CURVE('',#37598,#37597,#30922,.T.);
#47781=EDGE_CURVE('',#36959,#37598,#30923,.T.);
#47782=EDGE_CURVE('',#37599,#37598,#21624,.T.);
#47783=EDGE_CURVE('',#37599,#36960,#30924,.T.);
#47784=EDGE_CURVE('',#37599,#37600,#30925,.T.);
#47785=EDGE_CURVE('',#37601,#37600,#30926,.T.);
#47786=EDGE_CURVE('',#36960,#37601,#30927,.T.);
#47787=EDGE_CURVE('',#37602,#37601,#21625,.T.);
#47788=EDGE_CURVE('',#36961,#37602,#30928,.T.);
#47789=EDGE_CURVE('',#37603,#37602,#30929,.T.);
#47790=EDGE_CURVE('',#36963,#37603,#30930,.T.);
#47791=EDGE_CURVE('',#37075,#37603,#21626,.T.);
#47792=EDGE_CURVE('',#37604,#37075,#21627,.T.);
#47793=EDGE_CURVE('',#37072,#37604,#30931,.T.);
#47794=EDGE_CURVE('',#37076,#37072,#21628,.T.);
#47795=EDGE_CURVE('',#37605,#37604,#1921,.T.);
#47796=EDGE_CURVE('',#36976,#37605,#30932,.T.);
#47797=EDGE_CURVE('',#37606,#37605,#5144,.T.);
#47798=EDGE_CURVE('',#36973,#37606,#30933,.T.);
#47799=EDGE_CURVE('',#37607,#37606,#5145,.T.);
#47800=EDGE_CURVE('',#36972,#37607,#30934,.T.);
#47801=EDGE_CURVE('',#37608,#37607,#21629,.T.);
#47802=EDGE_CURVE('',#36969,#37608,#30935,.T.);
#47803=EDGE_CURVE('',#37609,#37610,#30936,.T.);
#47804=EDGE_CURVE('',#36969,#37610,#5146,.T.);
#47805=EDGE_CURVE('',#37609,#37608,#5147,.T.);
#47806=EDGE_CURVE('',#37611,#37612,#30937,.T.);
#47807=EDGE_CURVE('',#37610,#37612,#5148,.T.);
#47808=EDGE_CURVE('',#37611,#37609,#5149,.T.);
#47809=EDGE_CURVE('',#37613,#37610,#5150,.T.);
#47810=EDGE_CURVE('',#37613,#36970,#5151,.T.);
#47811=EDGE_CURVE('',#36968,#37614,#30938,.T.);
#47812=EDGE_CURVE('',#37615,#37614,#30939,.T.);
#47813=EDGE_CURVE('',#36966,#37615,#30940,.T.);
#47814=EDGE_CURVE('',#37616,#37615,#21630,.T.);
#47815=EDGE_CURVE('',#36979,#37616,#30941,.T.);
#47816=EDGE_CURVE('',#37617,#37618,#30942,.T.);
#47817=EDGE_CURVE('',#37619,#37618,#5152,.T.);
#47818=EDGE_CURVE('',#37613,#37619,#30943,.T.);
#47819=EDGE_CURVE('',#37617,#37613,#5153,.T.);
#47820=EDGE_CURVE('',#37620,#37619,#5154,.T.);
#47821=EDGE_CURVE('',#36970,#37620,#30944,.T.);
#47822=EDGE_CURVE('',#37621,#37620,#21631,.T.);
#47823=EDGE_CURVE('',#36971,#37621,#30945,.T.);
#47824=EDGE_CURVE('',#37622,#37621,#5155,.T.);
#47825=EDGE_CURVE('',#36974,#37622,#30946,.T.);
#47826=EDGE_CURVE('',#37623,#37622,#5156,.T.);
#47827=EDGE_CURVE('',#36975,#37623,#30947,.T.);
#47828=EDGE_CURVE('',#37624,#37623,#1922,.T.);
#47829=EDGE_CURVE('',#37073,#37624,#30948,.T.);
#47830=EDGE_CURVE('',#37071,#37624,#21632,.T.);
#47831=EDGE_CURVE('',#37073,#37070,#21633,.T.);
#47832=EDGE_CURVE('',#37614,#37071,#21634,.T.);
#47833=EDGE_CURVE('',#37625,#37616,#30949,.T.);
#47834=EDGE_CURVE('',#37626,#37625,#30950,.T.);
#47835=EDGE_CURVE('',#36979,#37626,#30951,.T.);
#47836=EDGE_CURVE('',#37627,#37626,#21635,.T.);
#47837=EDGE_CURVE('',#37627,#36980,#30952,.T.);
#47838=EDGE_CURVE('',#37627,#37628,#30953,.T.);
#47839=EDGE_CURVE('',#37250,#37628,#30954,.T.);
#47840=EDGE_CURVE('',#37629,#37294,#30955,.T.);
#47841=EDGE_CURVE('',#37630,#37629,#30956,.T.);
#47842=EDGE_CURVE('',#36981,#37630,#30957,.T.);
#47843=EDGE_CURVE('',#37631,#37630,#21636,.T.);
#47844=EDGE_CURVE('',#37631,#36982,#30958,.T.);
#47845=EDGE_CURVE('',#37631,#37632,#30959,.T.);
#47846=EDGE_CURVE('',#37481,#37632,#30960,.T.);
#47847=EDGE_CURVE('',#37633,#37634,#30961,.T.);
#47848=EDGE_CURVE('',#37635,#37634,#5157,.T.);
#47849=EDGE_CURVE('',#37636,#37635,#30962,.T.);
#47850=EDGE_CURVE('',#37633,#37636,#1183,.T.);
#47851=EDGE_CURVE('',#37637,#37638,#30963,.T.);
#47852=EDGE_CURVE('',#37639,#37638,#5158,.T.);
#47853=EDGE_CURVE('',#37640,#37639,#30964,.T.);
#47854=EDGE_CURVE('',#37637,#37640,#5159,.T.);
#47855=EDGE_CURVE('',#37641,#37642,#30965,.T.);
#47856=EDGE_CURVE('',#37643,#37642,#1923,.T.);
#47857=EDGE_CURVE('',#37644,#37643,#30966,.T.);
#47858=EDGE_CURVE('',#37641,#37644,#5160,.T.);
#47859=EDGE_CURVE('',#37645,#37646,#30967,.T.);
#47860=EDGE_CURVE('',#37642,#37646,#5161,.T.);
#47861=EDGE_CURVE('',#37645,#37641,#5162,.T.);
#47862=EDGE_CURVE('',#37647,#37648,#30968,.T.);
#47863=EDGE_CURVE('',#37649,#37648,#5163,.T.);
#47864=EDGE_CURVE('',#37650,#37649,#30969,.T.);
#47865=EDGE_CURVE('',#37647,#37650,#5164,.T.);
#47866=EDGE_CURVE('',#37651,#37649,#5165,.T.);
#47867=EDGE_CURVE('',#37652,#37651,#30970,.T.);
#47868=EDGE_CURVE('',#37650,#37652,#5166,.T.);
#47869=EDGE_CURVE('',#37653,#37651,#21637,.T.);
#47870=EDGE_CURVE('',#37654,#37653,#30971,.T.);
#47871=EDGE_CURVE('',#37652,#37654,#21638,.T.);
#47872=EDGE_CURVE('',#37655,#37656,#30972,.T.);
#47873=EDGE_CURVE('',#37657,#37656,#30973,.T.);
#47874=EDGE_CURVE('',#37658,#37657,#30974,.T.);
#47875=EDGE_CURVE('',#37655,#37658,#30975,.T.);
#47876=EDGE_CURVE('',#37655,#37659,#21639,.T.);
#47877=EDGE_CURVE('',#37660,#37658,#21640,.T.);
#47878=EDGE_CURVE('',#37660,#37659,#30976,.T.);
#47879=EDGE_CURVE('',#37660,#37661,#30977,.T.);
#47880=EDGE_CURVE('',#37662,#37661,#30978,.T.);
#47881=EDGE_CURVE('',#37659,#37662,#30979,.T.);
#47882=EDGE_CURVE('',#37663,#37159,#30980,.T.);
#47883=EDGE_CURVE('',#37664,#37159,#21641,.T.);
#47884=EDGE_CURVE('',#37665,#37664,#30981,.T.);
#47885=EDGE_CURVE('',#37663,#37665,#21642,.T.);
#47886=EDGE_CURVE('',#37666,#37161,#30982,.T.);
#47887=EDGE_CURVE('',#37666,#37663,#5167,.T.);
#47888=EDGE_CURVE('',#37667,#37668,#30983,.T.);
#47889=EDGE_CURVE('',#37161,#37668,#5168,.T.);
#47890=EDGE_CURVE('',#37667,#37666,#5169,.T.);
#47891=EDGE_CURVE('',#37669,#37670,#30984,.T.);
#47892=EDGE_CURVE('',#37366,#37670,#5170,.T.);
#47893=EDGE_CURVE('',#37669,#37365,#5171,.T.);
#47894=EDGE_CURVE('',#37671,#37672,#30985,.T.);
#47895=EDGE_CURVE('',#37668,#37672,#30986,.T.);
#47896=EDGE_CURVE('',#37671,#37667,#30987,.T.);
#47897=EDGE_CURVE('',#37668,#37365,#30988,.T.);
#47898=EDGE_CURVE('',#37673,#37674,#30989,.T.);
#47899=EDGE_CURVE('',#37675,#37674,#30990,.T.);
#47900=EDGE_CURVE('',#37164,#37675,#30991,.T.);
#47901=EDGE_CURVE('',#37673,#37164,#30992,.T.);
#47902=EDGE_CURVE('',#37676,#37675,#21643,.T.);
#47903=EDGE_CURVE('',#36999,#37676,#30993,.T.);
#47904=EDGE_CURVE('',#37677,#37676,#30994,.T.);
#47905=EDGE_CURVE('',#37001,#37677,#30995,.T.);
#47906=EDGE_CURVE('',#37678,#37679,#30996,.T.);
#47907=EDGE_CURVE('',#37680,#37679,#5172,.T.);
#47908=EDGE_CURVE('',#37011,#37680,#30997,.T.);
#47909=EDGE_CURVE('',#37678,#37011,#5173,.T.);
#47910=EDGE_CURVE('',#37681,#37680,#5174,.T.);
#47911=EDGE_CURVE('',#36984,#37681,#30998,.T.);
#47912=EDGE_CURVE('',#37682,#37681,#21644,.T.);
#47913=EDGE_CURVE('',#36985,#37682,#30999,.T.);
#47914=EDGE_CURVE('',#37683,#37682,#5175,.T.);
#47915=EDGE_CURVE('',#37684,#37683,#31000,.T.);
#47916=EDGE_CURVE('',#36985,#37684,#5176,.T.);
#47917=EDGE_CURVE('',#37685,#37683,#5177,.T.);
#47918=EDGE_CURVE('',#37686,#37685,#31001,.T.);
#47919=EDGE_CURVE('',#37684,#37686,#5178,.T.);
#47920=EDGE_CURVE('',#37687,#37684,#5179,.T.);
#47921=EDGE_CURVE('',#37687,#36986,#5180,.T.);
#47922=EDGE_CURVE('',#37010,#37688,#31002,.T.);
#47923=EDGE_CURVE('',#37689,#37688,#31003,.T.);
#47924=EDGE_CURVE('',#36990,#37689,#31004,.T.);
#47925=EDGE_CURVE('',#37690,#37689,#21645,.T.);
#47926=EDGE_CURVE('',#36987,#37690,#31005,.T.);
#47927=EDGE_CURVE('',#37691,#36986,#31006,.T.);
#47928=EDGE_CURVE('',#37692,#37687,#31007,.T.);
#47929=EDGE_CURVE('',#37691,#37692,#5181,.T.);
#47930=EDGE_CURVE('',#37693,#36983,#31008,.T.);
#47931=EDGE_CURVE('',#37693,#37691,#21646,.T.);
#47932=EDGE_CURVE('',#37694,#37012,#31009,.T.);
#47933=EDGE_CURVE('',#37694,#37693,#5182,.T.);
#47934=EDGE_CURVE('',#37695,#37696,#31010,.T.);
#47935=EDGE_CURVE('',#37012,#37696,#5183,.T.);
#47936=EDGE_CURVE('',#37695,#37694,#5184,.T.);
#47937=EDGE_CURVE('',#37697,#37687,#5185,.T.);
#47938=EDGE_CURVE('',#37698,#37697,#31011,.T.);
#47939=EDGE_CURVE('',#37692,#37698,#5186,.T.);
#47940=EDGE_CURVE('',#37699,#37690,#31012,.T.);
#47941=EDGE_CURVE('',#37700,#37699,#31013,.T.);
#47942=EDGE_CURVE('',#36987,#37700,#31014,.T.);
#47943=EDGE_CURVE('',#37701,#37700,#21647,.T.);
#47944=EDGE_CURVE('',#37701,#36988,#31015,.T.);
#47945=EDGE_CURVE('',#37701,#37702,#31016,.T.);
#47946=EDGE_CURVE('',#37703,#37702,#31017,.T.);
#47947=EDGE_CURVE('',#36988,#37703,#31018,.T.);
#47948=EDGE_CURVE('',#37704,#37703,#21648,.T.);
#47949=EDGE_CURVE('',#36989,#37704,#31019,.T.);
#47950=EDGE_CURVE('',#37705,#37704,#31020,.T.);
#47951=EDGE_CURVE('',#37009,#37705,#31021,.T.);
#47952=EDGE_CURVE('',#37706,#37707,#31022,.T.);
#47953=EDGE_CURVE('',#37708,#37707,#5187,.T.);
#47954=EDGE_CURVE('',#37007,#37708,#31023,.T.);
#47955=EDGE_CURVE('',#37706,#37007,#5188,.T.);
#47956=EDGE_CURVE('',#37709,#37708,#5189,.T.);
#47957=EDGE_CURVE('',#36992,#37709,#31024,.T.);
#47958=EDGE_CURVE('',#37710,#37709,#21649,.T.);
#47959=EDGE_CURVE('',#36993,#37710,#31025,.T.);
#47960=EDGE_CURVE('',#37711,#37710,#5190,.T.);
#47961=EDGE_CURVE('',#37712,#37711,#31026,.T.);
#47962=EDGE_CURVE('',#36993,#37712,#5191,.T.);
#47963=EDGE_CURVE('',#37713,#37711,#5192,.T.);
#47964=EDGE_CURVE('',#37714,#37713,#31027,.T.);
#47965=EDGE_CURVE('',#37712,#37714,#5193,.T.);
#47966=EDGE_CURVE('',#37715,#37712,#5194,.T.);
#47967=EDGE_CURVE('',#37715,#36994,#5195,.T.);
#47968=EDGE_CURVE('',#37716,#36994,#31028,.T.);
#47969=EDGE_CURVE('',#37717,#37715,#31029,.T.);
#47970=EDGE_CURVE('',#37716,#37717,#5196,.T.);
#47971=EDGE_CURVE('',#37718,#36991,#31030,.T.);
#47972=EDGE_CURVE('',#37718,#37716,#21650,.T.);
#47973=EDGE_CURVE('',#37719,#37008,#31031,.T.);
#47974=EDGE_CURVE('',#37719,#37718,#5197,.T.);
#47975=EDGE_CURVE('',#37720,#37721,#31032,.T.);
#47976=EDGE_CURVE('',#37008,#37721,#5198,.T.);
#47977=EDGE_CURVE('',#37720,#37719,#1184,.T.);
#47978=EDGE_CURVE('',#37722,#37715,#5199,.T.);
#47979=EDGE_CURVE('',#37723,#37722,#31033,.T.);
#47980=EDGE_CURVE('',#37717,#37723,#1185,.T.);
#47981=EDGE_CURVE('',#37724,#37725,#31034,.T.);
#47982=EDGE_CURVE('',#37726,#37725,#21651,.T.);
#47983=EDGE_CURVE('',#37727,#37726,#31035,.T.);
#47984=EDGE_CURVE('',#37724,#37727,#21652,.T.);
#47985=EDGE_CURVE('',#37727,#37728,#5200,.T.);
#47986=EDGE_CURVE('',#37728,#37729,#21653,.T.);
#47987=EDGE_CURVE('',#37729,#37724,#5201,.T.);
#47988=EDGE_CURVE('',#37728,#37730,#31036,.T.);
#47989=EDGE_CURVE('',#37731,#37730,#21654,.T.);
#47990=EDGE_CURVE('',#37729,#37731,#31037,.T.);
#47991=EDGE_CURVE('',#37732,#37733,#31038,.T.);
#47992=EDGE_CURVE('',#37734,#37733,#1186,.T.);
#47993=EDGE_CURVE('',#37005,#37734,#31039,.T.);
#47994=EDGE_CURVE('',#37732,#37005,#5202,.T.);
#47995=EDGE_CURVE('',#37735,#37734,#5203,.T.);
#47996=EDGE_CURVE('',#36996,#37735,#31040,.T.);
#47997=EDGE_CURVE('',#37736,#37735,#21655,.T.);
#47998=EDGE_CURVE('',#36997,#37736,#31041,.T.);
#47999=EDGE_CURVE('',#37737,#37736,#5204,.T.);
#48000=EDGE_CURVE('',#37738,#37737,#31042,.T.);
#48001=EDGE_CURVE('',#36997,#37738,#5205,.T.);
#48002=EDGE_CURVE('',#37739,#37737,#1187,.T.);
#48003=EDGE_CURVE('',#37740,#37739,#31043,.T.);
#48004=EDGE_CURVE('',#37738,#37740,#5206,.T.);
#48005=EDGE_CURVE('',#37741,#37738,#5207,.T.);
#48006=EDGE_CURVE('',#37741,#36998,#1924,.T.);
#48007=EDGE_CURVE('',#37742,#36998,#31044,.T.);
#48008=EDGE_CURVE('',#37743,#37741,#31045,.T.);
#48009=EDGE_CURVE('',#37742,#37743,#1925,.T.);
#48010=EDGE_CURVE('',#37744,#36995,#31046,.T.);
#48011=EDGE_CURVE('',#37744,#37742,#21656,.T.);
#48012=EDGE_CURVE('',#37745,#37006,#31047,.T.);
#48013=EDGE_CURVE('',#37745,#37744,#1926,.T.);
#48014=EDGE_CURVE('',#37746,#37747,#31048,.T.);
#48015=EDGE_CURVE('',#37006,#37747,#5208,.T.);
#48016=EDGE_CURVE('',#37746,#37745,#1188,.T.);
#48017=EDGE_CURVE('',#37748,#37741,#5209,.T.);
#48018=EDGE_CURVE('',#37749,#37748,#31049,.T.);
#48019=EDGE_CURVE('',#37743,#37749,#1189,.T.);
#48020=EDGE_CURVE('',#37001,#37750,#21657,.T.);
#48021=EDGE_CURVE('',#37750,#37751,#31050,.T.);
#48022=EDGE_CURVE('',#37751,#37002,#21658,.T.);
#48023=EDGE_CURVE('',#37751,#37752,#5210,.T.);
#48024=EDGE_CURVE('',#37752,#37753,#5211,.T.);
#48025=EDGE_CURVE('',#37426,#37753,#21659,.T.);
#48026=EDGE_CURVE('',#37018,#37437,#5212,.T.);
#48027=EDGE_CURVE('',#37752,#37754,#31051,.T.);
#48028=EDGE_CURVE('',#37755,#37754,#5213,.T.);
#48029=EDGE_CURVE('',#37753,#37755,#31052,.T.);
#48030=EDGE_CURVE('',#37437,#37755,#21660,.T.);
#48031=EDGE_CURVE('',#37753,#37436,#21661,.T.);
#48032=EDGE_CURVE('',#37756,#37757,#31053,.T.);
#48033=EDGE_CURVE('',#37747,#37757,#1927,.T.);
#48034=EDGE_CURVE('',#37756,#37746,#1928,.T.);
#48035=EDGE_CURVE('',#37747,#37732,#31054,.T.);
#48036=EDGE_CURVE('',#37758,#37759,#31055,.T.);
#48037=EDGE_CURVE('',#37733,#37759,#1929,.T.);
#48038=EDGE_CURVE('',#37758,#37732,#1930,.T.);
#48039=EDGE_CURVE('',#37760,#37731,#5214,.T.);
#48040=EDGE_CURVE('',#37760,#37761,#5215,.T.);
#48041=EDGE_CURVE('',#37729,#37761,#5216,.T.);
#48042=EDGE_CURVE('',#37761,#37762,#31056,.T.);
#48043=EDGE_CURVE('',#37762,#37724,#5217,.T.);
#48044=EDGE_CURVE('',#37762,#37763,#5218,.T.);
#48045=EDGE_CURVE('',#37725,#37763,#5219,.T.);
#48046=EDGE_CURVE('',#37764,#37765,#31057,.T.);
#48047=EDGE_CURVE('',#37721,#37765,#1931,.T.);
#48048=EDGE_CURVE('',#37764,#37720,#1932,.T.);
#48049=EDGE_CURVE('',#37721,#37706,#31058,.T.);
#48050=EDGE_CURVE('',#37766,#37767,#31059,.T.);
#48051=EDGE_CURVE('',#37707,#37767,#1933,.T.);
#48052=EDGE_CURVE('',#37766,#37706,#1934,.T.);
#48053=EDGE_CURVE('',#37768,#37705,#21662,.T.);
#48054=EDGE_CURVE('',#37768,#37769,#5220,.T.);
#48055=EDGE_CURVE('',#37009,#37769,#21663,.T.);
#48056=EDGE_CURVE('',#37769,#37770,#31060,.T.);
#48057=EDGE_CURVE('',#37770,#37010,#21664,.T.);
#48058=EDGE_CURVE('',#37770,#37771,#5221,.T.);
#48059=EDGE_CURVE('',#37688,#37771,#21665,.T.);
#48060=EDGE_CURVE('',#37772,#37773,#31061,.T.);
#48061=EDGE_CURVE('',#37696,#37773,#1935,.T.);
#48062=EDGE_CURVE('',#37772,#37695,#1936,.T.);
#48063=EDGE_CURVE('',#37696,#37678,#31062,.T.);
#48064=EDGE_CURVE('',#37774,#37775,#31063,.T.);
#48065=EDGE_CURVE('',#37679,#37775,#1937,.T.);
#48066=EDGE_CURVE('',#37774,#37678,#1938,.T.);
#48067=EDGE_CURVE('',#37776,#37677,#21666,.T.);
#48068=EDGE_CURVE('',#37776,#37750,#5222,.T.);
#48069=EDGE_CURVE('',#37307,#37777,#31064,.T.);
#48070=EDGE_CURVE('',#37777,#37156,#21667,.T.);
#48071=EDGE_CURVE('',#37153,#37778,#21668,.T.);
#48072=EDGE_CURVE('',#37778,#37310,#31065,.T.);
#48073=EDGE_CURVE('',#37310,#37779,#5223,.T.);
#48074=EDGE_CURVE('',#37779,#37307,#5224,.T.);
#48075=EDGE_CURVE('',#37311,#37308,#5225,.T.);
#48076=EDGE_CURVE('',#37451,#37232,#31066,.T.);
#48077=EDGE_CURVE('',#37232,#37230,#5226,.T.);
#48078=EDGE_CURVE('',#37233,#37229,#5227,.T.);
#48079=EDGE_CURVE('',#37230,#37780,#31067,.T.);
#48080=EDGE_CURVE('',#37780,#37441,#31068,.T.);
#48081=EDGE_CURVE('',#37441,#37451,#5228,.T.);
#48082=EDGE_CURVE('',#37442,#37450,#5229,.T.);
#48083=EDGE_CURVE('',#37018,#37781,#21669,.T.);
#48084=EDGE_CURVE('',#37781,#37782,#21670,.T.);
#48085=EDGE_CURVE('',#37782,#37037,#21671,.T.);
#48086=EDGE_CURVE('',#37782,#37783,#31069,.T.);
#48087=EDGE_CURVE('',#37038,#37783,#21672,.T.);
#48088=EDGE_CURVE('',#37783,#37784,#31070,.T.);
#48089=EDGE_CURVE('',#37784,#37040,#21673,.T.);
#48090=EDGE_CURVE('',#37784,#37785,#31071,.T.);
#48091=EDGE_CURVE('',#37042,#37785,#21674,.T.);
#48092=EDGE_CURVE('',#37785,#37786,#21675,.T.);
#48093=EDGE_CURVE('',#37786,#37052,#21676,.T.);
#48094=EDGE_CURVE('',#37066,#37787,#21677,.T.);
#48095=EDGE_CURVE('',#37786,#37787,#31072,.T.);
#48096=EDGE_CURVE('',#37788,#37120,#21678,.T.);
#48097=EDGE_CURVE('',#37787,#37788,#31073,.T.);
#48098=EDGE_CURVE('',#37788,#37789,#31074,.T.);
#48099=EDGE_CURVE('',#37123,#37789,#21679,.T.);
#48100=EDGE_CURVE('',#37789,#37790,#21680,.T.);
#48101=EDGE_CURVE('',#37790,#37145,#21681,.T.);
#48102=EDGE_CURVE('',#37790,#37791,#31075,.T.);
#48103=EDGE_CURVE('',#37146,#37791,#21682,.T.);
#48104=EDGE_CURVE('',#37791,#37792,#31076,.T.);
#48105=EDGE_CURVE('',#37792,#37148,#21683,.T.);
#48106=EDGE_CURVE('',#37792,#37793,#31077,.T.);
#48107=EDGE_CURVE('',#37150,#37793,#21684,.T.);
#48108=EDGE_CURVE('',#37794,#37795,#21685,.T.);
#48109=EDGE_CURVE('',#37795,#37796,#21686,.T.);
#48110=EDGE_CURVE('',#37796,#37797,#5230,.T.);
#48111=EDGE_CURVE('',#37797,#37152,#21687,.T.);
#48112=EDGE_CURVE('',#37793,#37794,#21688,.T.);
#48113=EDGE_CURVE('',#37798,#37797,#31078,.T.);
#48114=EDGE_CURVE('',#37799,#37796,#31079,.T.);
#48115=EDGE_CURVE('',#37798,#37799,#5231,.T.);
#48116=EDGE_CURVE('',#37800,#37152,#31080,.T.);
#48117=EDGE_CURVE('',#37800,#37798,#21689,.T.);
#48118=EDGE_CURVE('',#37801,#37153,#31081,.T.);
#48119=EDGE_CURVE('',#37801,#37800,#1190,.T.);
#48120=EDGE_CURVE('',#37802,#37778,#31082,.T.);
#48121=EDGE_CURVE('',#37802,#37801,#21690,.T.);
#48122=EDGE_CURVE('',#37803,#37777,#31083,.T.);
#48123=EDGE_CURVE('',#37777,#37778,#5232,.T.);
#48124=EDGE_CURVE('',#37803,#37802,#5233,.T.);
#48125=EDGE_CURVE('',#37155,#37803,#21691,.T.);
#48126=EDGE_CURVE('',#37154,#37804,#21692,.T.);
#48127=EDGE_CURVE('',#37805,#37155,#21693,.T.);
#48128=EDGE_CURVE('',#37805,#37804,#31084,.T.);
#48129=EDGE_CURVE('',#37806,#37351,#31085,.T.);
#48130=EDGE_CURVE('',#37807,#37806,#31086,.T.);
#48131=EDGE_CURVE('',#37352,#37807,#31087,.T.);
#48132=EDGE_CURVE('',#37352,#37380,#21694,.T.);
#48133=EDGE_CURVE('',#37808,#37380,#31088,.T.);
#48134=EDGE_CURVE('',#37808,#37809,#31089,.T.);
#48135=EDGE_CURVE('',#37381,#37809,#31090,.T.);
#48136=EDGE_CURVE('',#37810,#37378,#21695,.T.);
#48137=EDGE_CURVE('',#37810,#37811,#31091,.T.);
#48138=EDGE_CURVE('',#37375,#37811,#21696,.T.);
#48139=EDGE_CURVE('',#37811,#37812,#21697,.T.);
#48140=EDGE_CURVE('',#37812,#37371,#21698,.T.);
#48141=EDGE_CURVE('',#37812,#37813,#31092,.T.);
#48142=EDGE_CURVE('',#37372,#37813,#21699,.T.);
#48143=EDGE_CURVE('',#37814,#37369,#31093,.T.);
#48144=EDGE_CURVE('',#37815,#37814,#31094,.T.);
#48145=EDGE_CURVE('',#37370,#37815,#31095,.T.);
#48146=EDGE_CURVE('',#37370,#37664,#21700,.T.);
#48147=EDGE_CURVE('',#37816,#37664,#31096,.T.);
#48148=EDGE_CURVE('',#37816,#37817,#31097,.T.);
#48149=EDGE_CURVE('',#37665,#37817,#31098,.T.);
#48150=EDGE_CURVE('',#37818,#37662,#21701,.T.);
#48151=EDGE_CURVE('',#37818,#37819,#31099,.T.);
#48152=EDGE_CURVE('',#37659,#37819,#21702,.T.);
#48153=EDGE_CURVE('',#37819,#37820,#21703,.T.);
#48154=EDGE_CURVE('',#37820,#37655,#21704,.T.);
#48155=EDGE_CURVE('',#37820,#37821,#31100,.T.);
#48156=EDGE_CURVE('',#37656,#37821,#21705,.T.);
#48157=EDGE_CURVE('',#37822,#37653,#31101,.T.);
#48158=EDGE_CURVE('',#37823,#37822,#31102,.T.);
#48159=EDGE_CURVE('',#37654,#37823,#31103,.T.);
#48160=EDGE_CURVE('',#37824,#37652,#1939,.T.);
#48161=EDGE_CURVE('',#37654,#37824,#21706,.T.);
#48162=EDGE_CURVE('',#37824,#37643,#5234,.T.);
#48163=EDGE_CURVE('',#37650,#37642,#5235,.T.);
#48164=EDGE_CURVE('',#37825,#37643,#5236,.T.);
#48165=EDGE_CURVE('',#37825,#37826,#31104,.T.);
#48166=EDGE_CURVE('',#37644,#37826,#5237,.T.);
#48167=EDGE_CURVE('',#37827,#37828,#31105,.T.);
#48168=EDGE_CURVE('',#37826,#37828,#31106,.T.);
#48169=EDGE_CURVE('',#37827,#37825,#31107,.T.);
#48170=EDGE_CURVE('',#37829,#37830,#21707,.T.);
#48171=EDGE_CURVE('',#37829,#37831,#31108,.T.);
#48172=EDGE_CURVE('',#37832,#37831,#21708,.T.);
#48173=EDGE_CURVE('',#37832,#37830,#31109,.T.);
#48174=EDGE_CURVE('',#37831,#37833,#21709,.T.);
#48175=EDGE_CURVE('',#37833,#37834,#21710,.T.);
#48176=EDGE_CURVE('',#37834,#37832,#31110,.T.);
#48177=EDGE_CURVE('',#37833,#37835,#31111,.T.);
#48178=EDGE_CURVE('',#37836,#37835,#21711,.T.);
#48179=EDGE_CURVE('',#37836,#37834,#31112,.T.);
#48180=EDGE_CURVE('',#37837,#37639,#5238,.T.);
#48181=EDGE_CURVE('',#37838,#37837,#31113,.T.);
#48182=EDGE_CURVE('',#37839,#37838,#5239,.T.);
#48183=EDGE_CURVE('',#37640,#37839,#1940,.T.);
#48184=EDGE_CURVE('',#37840,#37635,#1941,.T.);
#48185=EDGE_CURVE('',#37841,#37840,#5240,.T.);
#48186=EDGE_CURVE('',#37841,#37842,#31114,.T.);
#48187=EDGE_CURVE('',#37636,#37842,#5241,.T.);
#48188=EDGE_CURVE('',#37843,#37844,#21712,.T.);
#48189=EDGE_CURVE('',#37843,#37845,#31115,.T.);
#48190=EDGE_CURVE('',#37846,#37845,#21713,.T.);
#48191=EDGE_CURVE('',#37846,#37844,#31116,.T.);
#48192=EDGE_CURVE('',#37845,#37847,#21714,.T.);
#48193=EDGE_CURVE('',#37847,#37848,#21715,.T.);
#48194=EDGE_CURVE('',#37848,#37846,#5242,.T.);
#48195=EDGE_CURVE('',#37847,#37849,#31117,.T.);
#48196=EDGE_CURVE('',#37850,#37849,#21716,.T.);
#48197=EDGE_CURVE('',#37850,#37848,#31118,.T.);
#48198=EDGE_CURVE('',#37851,#37167,#31119,.T.);
#48199=EDGE_CURVE('',#37852,#37166,#31120,.T.);
#48200=EDGE_CURVE('',#37851,#37852,#5243,.T.);
#48201=EDGE_CURVE('',#37853,#37363,#31121,.T.);
#48202=EDGE_CURVE('',#37853,#37851,#5244,.T.);
#48203=EDGE_CURVE('',#37854,#37361,#31122,.T.);
#48204=EDGE_CURVE('',#37363,#37361,#21717,.T.);
#48205=EDGE_CURVE('',#37854,#37853,#21718,.T.);
#48206=EDGE_CURVE('',#37855,#37321,#31123,.T.);
#48207=EDGE_CURVE('',#37804,#37321,#31124,.T.);
#48208=EDGE_CURVE('',#37855,#37805,#31125,.T.);
#48209=EDGE_CURVE('',#37852,#37855,#5245,.T.);
#48210=EDGE_CURVE('',#37856,#37362,#31126,.T.);
#48211=EDGE_CURVE('',#37856,#37854,#5246,.T.);
#48212=EDGE_CURVE('',#37362,#37857,#21719,.T.);
#48213=EDGE_CURVE('',#37857,#37353,#21720,.T.);
#48214=EDGE_CURVE('',#37857,#37858,#31127,.T.);
#48215=EDGE_CURVE('',#37354,#37858,#21721,.T.);
#48216=EDGE_CURVE('',#37859,#37428,#31128,.T.);
#48217=EDGE_CURVE('',#37860,#37859,#31129,.T.);
#48218=EDGE_CURVE('',#37163,#37860,#31130,.T.);
#48219=EDGE_CURVE('',#37673,#37860,#21722,.T.);
#48220=EDGE_CURVE('',#37861,#37235,#21723,.T.);
#48221=EDGE_CURVE('',#37862,#37861,#31131,.T.);
#48222=EDGE_CURVE('',#37236,#37862,#21724,.T.);
#48223=EDGE_CURVE('',#37863,#37863,#31132,.T.);
#48224=EDGE_CURVE('',#37863,#37864,#21725,.T.);
#48225=EDGE_CURVE('',#37864,#37447,#31133,.T.);
#48226=EDGE_CURVE('',#37236,#37864,#31134,.T.);
#48227=EDGE_CURVE('',#37865,#37865,#31135,.T.);
#48228=EDGE_CURVE('',#37866,#37866,#31136,.T.);
#48229=EDGE_CURVE('',#37866,#37865,#21726,.T.);
#48230=EDGE_CURVE('',#37867,#37868,#31137,.T.);
#48231=EDGE_CURVE('',#37448,#37868,#21727,.T.);
#48232=EDGE_CURVE('',#37867,#37447,#21728,.T.);
#48233=EDGE_CURVE('',#37869,#37364,#31138,.T.);
#48234=EDGE_CURVE('',#37870,#37364,#21729,.T.);
#48235=EDGE_CURVE('',#37871,#37870,#31139,.T.);
#48236=EDGE_CURVE('',#37869,#37871,#21730,.T.);
#48237=EDGE_CURVE('',#37872,#37168,#31140,.T.);
#48238=EDGE_CURVE('',#37872,#37869,#31141,.T.);
#48239=EDGE_CURVE('',#37873,#37165,#31142,.T.);
#48240=EDGE_CURVE('',#37873,#37872,#31143,.T.);
#48241=EDGE_CURVE('',#37874,#37322,#31144,.T.);
#48242=EDGE_CURVE('',#37874,#37873,#31145,.T.);
#48243=EDGE_CURVE('',#37322,#37318,#21731,.T.);
#48244=EDGE_CURVE('',#37319,#37874,#21732,.T.);
#48245=EDGE_CURVE('',#37875,#37875,#31146,.T.);
#48246=EDGE_CURVE('',#37875,#37320,#21733,.T.);
#48247=EDGE_CURVE('',#37319,#37317,#31147,.T.);
#48248=EDGE_CURVE('',#37876,#37876,#31148,.T.);
#48249=EDGE_CURVE('',#37877,#37877,#31149,.T.);
#48250=EDGE_CURVE('',#37877,#37876,#21734,.T.);
#48251=EDGE_CURVE('',#37878,#37317,#21735,.T.);
#48252=EDGE_CURVE('',#37879,#37878,#31150,.T.);
#48253=EDGE_CURVE('',#37316,#37879,#21736,.T.);
#48254=EDGE_CURVE('',#37880,#37187,#21737,.T.);
#48255=EDGE_CURVE('',#37186,#37880,#31151,.T.);
#48256=EDGE_CURVE('',#37188,#37881,#1191,.T.);
#48257=EDGE_CURVE('',#37881,#37882,#21738,.T.);
#48258=EDGE_CURVE('',#37882,#37189,#21739,.T.);
#48259=EDGE_CURVE('',#37883,#37187,#5247,.T.);
#48260=EDGE_CURVE('',#37884,#37883,#31152,.T.);
#48261=EDGE_CURVE('',#37881,#37884,#31153,.T.);
#48262=EDGE_CURVE('',#37882,#37885,#5248,.T.);
#48263=EDGE_CURVE('',#37190,#37885,#21740,.T.);
#48264=EDGE_CURVE('',#37885,#37886,#21741,.T.);
#48265=EDGE_CURVE('',#37886,#37191,#21742,.T.);
#48266=EDGE_CURVE('',#37886,#37887,#5249,.T.);
#48267=EDGE_CURVE('',#37192,#37887,#21743,.T.);
#48268=EDGE_CURVE('',#37887,#37888,#21744,.T.);
#48269=EDGE_CURVE('',#37888,#37207,#5250,.T.);
#48270=EDGE_CURVE('',#37889,#37888,#31154,.T.);
#48271=EDGE_CURVE('',#37208,#37889,#5251,.T.);
#48272=EDGE_CURVE('',#37208,#37213,#21745,.T.);
#48273=EDGE_CURVE('',#37890,#37891,#31155,.T.);
#48274=EDGE_CURVE('',#37214,#37891,#1192,.T.);
#48275=EDGE_CURVE('',#37890,#37213,#5252,.T.);
#48276=EDGE_CURVE('',#37891,#37892,#21746,.T.);
#48277=EDGE_CURVE('',#37892,#37226,#21747,.T.);
#48278=EDGE_CURVE('',#37892,#37893,#5253,.T.);
#48279=EDGE_CURVE('',#37227,#37893,#21748,.T.);
#48280=EDGE_CURVE('',#37893,#37894,#21749,.T.);
#48281=EDGE_CURVE('',#37894,#37228,#21750,.T.);
#48282=EDGE_CURVE('',#37894,#37895,#5254,.T.);
#48283=EDGE_CURVE('',#37238,#37895,#21751,.T.);
#48284=EDGE_CURVE('',#37895,#37896,#21752,.T.);
#48285=EDGE_CURVE('',#37896,#37861,#1193,.T.);
#48286=EDGE_CURVE('',#37897,#37896,#31156,.T.);
#48287=EDGE_CURVE('',#37862,#37897,#5255,.T.);
#48288=EDGE_CURVE('',#37628,#37898,#21753,.T.);
#48289=EDGE_CURVE('',#37898,#37899,#21754,.T.);
#48290=EDGE_CURVE('',#37899,#37254,#5256,.T.);
#48291=EDGE_CURVE('',#37899,#37900,#31157,.T.);
#48292=EDGE_CURVE('',#37255,#37900,#5257,.T.);
#48293=EDGE_CURVE('',#37255,#37880,#5258,.T.);
#48294=EDGE_CURVE('',#37343,#37901,#1194,.T.);
#48295=EDGE_CURVE('',#37901,#37902,#21755,.T.);
#48296=EDGE_CURVE('',#37902,#37270,#21756,.T.);
#48297=EDGE_CURVE('',#37902,#37903,#5259,.T.);
#48298=EDGE_CURVE('',#37271,#37903,#21757,.T.);
#48299=EDGE_CURVE('',#37903,#37904,#21758,.T.);
#48300=EDGE_CURVE('',#37904,#37272,#21759,.T.);
#48301=EDGE_CURVE('',#37904,#37905,#5260,.T.);
#48302=EDGE_CURVE('',#37273,#37905,#21760,.T.);
#48303=EDGE_CURVE('',#37905,#37906,#21761,.T.);
#48304=EDGE_CURVE('',#37906,#37289,#1195,.T.);
#48305=EDGE_CURVE('',#37907,#37906,#31158,.T.);
#48306=EDGE_CURVE('',#37290,#37907,#5261,.T.);
#48307=EDGE_CURVE('',#37908,#37287,#31159,.T.);
#48308=EDGE_CURVE('',#37290,#37908,#21762,.T.);
#48309=EDGE_CURVE('',#37908,#37909,#5262,.T.);
#48310=EDGE_CURVE('',#37909,#37298,#5263,.T.);
#48311=EDGE_CURVE('',#37909,#37295,#31160,.T.);
#48312=EDGE_CURVE('',#37910,#37911,#31161,.T.);
#48313=EDGE_CURVE('',#37296,#37911,#1942,.T.);
#48314=EDGE_CURVE('',#37910,#37295,#5264,.T.);
#48315=EDGE_CURVE('',#37911,#37912,#21763,.T.);
#48316=EDGE_CURVE('',#37912,#37629,#21764,.T.);
#48317=EDGE_CURVE('',#37879,#37913,#1196,.T.);
#48318=EDGE_CURVE('',#37913,#37914,#21765,.T.);
#48319=EDGE_CURVE('',#37914,#37323,#21766,.T.);
#48320=EDGE_CURVE('',#37915,#37878,#5265,.T.);
#48321=EDGE_CURVE('',#37913,#37915,#31162,.T.);
#48322=EDGE_CURVE('',#37914,#37916,#5266,.T.);
#48323=EDGE_CURVE('',#37324,#37916,#21767,.T.);
#48324=EDGE_CURVE('',#37916,#37917,#21768,.T.);
#48325=EDGE_CURVE('',#37917,#37325,#21769,.T.);
#48326=EDGE_CURVE('',#37917,#37918,#5267,.T.);
#48327=EDGE_CURVE('',#37336,#37918,#21770,.T.);
#48328=EDGE_CURVE('',#37918,#37919,#21771,.T.);
#48329=EDGE_CURVE('',#37919,#37344,#1197,.T.);
#48330=EDGE_CURVE('',#37920,#37342,#5268,.T.);
#48331=EDGE_CURVE('',#37901,#37920,#31163,.T.);
#48332=EDGE_CURVE('',#37919,#37921,#31164,.T.);
#48333=EDGE_CURVE('',#37345,#37921,#5269,.T.);
#48334=EDGE_CURVE('',#37345,#37342,#21772,.T.);
#48335=EDGE_CURVE('',#37858,#37806,#21773,.T.);
#48336=EDGE_CURVE('',#37387,#37922,#1198,.T.);
#48337=EDGE_CURVE('',#37922,#37923,#21774,.T.);
#48338=EDGE_CURVE('',#37923,#37355,#21775,.T.);
#48339=EDGE_CURVE('',#37923,#37924,#5270,.T.);
#48340=EDGE_CURVE('',#37356,#37924,#21776,.T.);
#48341=EDGE_CURVE('',#37924,#37925,#21777,.T.);
#48342=EDGE_CURVE('',#37925,#37357,#21778,.T.);
#48343=EDGE_CURVE('',#37925,#37926,#5271,.T.);
#48344=EDGE_CURVE('',#37359,#37926,#21779,.T.);
#48345=EDGE_CURVE('',#37926,#37927,#21780,.T.);
#48346=EDGE_CURVE('',#37927,#37870,#5272,.T.);
#48347=EDGE_CURVE('',#37928,#37927,#31165,.T.);
#48348=EDGE_CURVE('',#37871,#37928,#5273,.T.);
#48349=EDGE_CURVE('',#37929,#37930,#31166,.T.);
#48350=EDGE_CURVE('',#37670,#37930,#5274,.T.);
#48351=EDGE_CURVE('',#37929,#37669,#5275,.T.);
#48352=EDGE_CURVE('',#37930,#37931,#21781,.T.);
#48353=EDGE_CURVE('',#37931,#37373,#21782,.T.);
#48354=EDGE_CURVE('',#37813,#37814,#21783,.T.);
#48355=EDGE_CURVE('',#37931,#37932,#5276,.T.);
#48356=EDGE_CURVE('',#37374,#37932,#21784,.T.);
#48357=EDGE_CURVE('',#37932,#37933,#21785,.T.);
#48358=EDGE_CURVE('',#37933,#37376,#21786,.T.);
#48359=EDGE_CURVE('',#37933,#37934,#5277,.T.);
#48360=EDGE_CURVE('',#37377,#37934,#21787,.T.);
#48361=EDGE_CURVE('',#37934,#37935,#21788,.T.);
#48362=EDGE_CURVE('',#37935,#37388,#1199,.T.);
#48363=EDGE_CURVE('',#37809,#37810,#21789,.T.);
#48364=EDGE_CURVE('',#37936,#37922,#31167,.T.);
#48365=EDGE_CURVE('',#37936,#37386,#5278,.T.);
#48366=EDGE_CURVE('',#37935,#37937,#31168,.T.);
#48367=EDGE_CURVE('',#37389,#37937,#5279,.T.);
#48368=EDGE_CURVE('',#37389,#37386,#21790,.T.);
#48369=EDGE_CURVE('',#37472,#37938,#1200,.T.);
#48370=EDGE_CURVE('',#37938,#37939,#21791,.T.);
#48371=EDGE_CURVE('',#37939,#37404,#21792,.T.);
#48372=EDGE_CURVE('',#37939,#37940,#5280,.T.);
#48373=EDGE_CURVE('',#37405,#37940,#21793,.T.);
#48374=EDGE_CURVE('',#37940,#37941,#21794,.T.);
#48375=EDGE_CURVE('',#37941,#37406,#21795,.T.);
#48376=EDGE_CURVE('',#37941,#37942,#5281,.T.);
#48377=EDGE_CURVE('',#37407,#37942,#21796,.T.);
#48378=EDGE_CURVE('',#37942,#37943,#21797,.T.);
#48379=EDGE_CURVE('',#37943,#37423,#1201,.T.);
#48380=EDGE_CURVE('',#37944,#37943,#31169,.T.);
#48381=EDGE_CURVE('',#37424,#37944,#5282,.T.);
#48382=EDGE_CURVE('',#37945,#37421,#31170,.T.);
#48383=EDGE_CURVE('',#37424,#37945,#21798,.T.);
#48384=EDGE_CURVE('',#37945,#37438,#5283,.T.);
#48385=EDGE_CURVE('',#37439,#37946,#5284,.T.);
#48386=EDGE_CURVE('',#37946,#37947,#21799,.T.);
#48387=EDGE_CURVE('',#37947,#37859,#21800,.T.);
#48388=EDGE_CURVE('',#37948,#37438,#5285,.T.);
#48389=EDGE_CURVE('',#37946,#37948,#31171,.T.);
#48390=EDGE_CURVE('',#37949,#37950,#31172,.T.);
#48391=EDGE_CURVE('',#37868,#37950,#1202,.T.);
#48392=EDGE_CURVE('',#37949,#37867,#5286,.T.);
#48393=EDGE_CURVE('',#37950,#37951,#21801,.T.);
#48394=EDGE_CURVE('',#37951,#37452,#21802,.T.);
#48395=EDGE_CURVE('',#37951,#37952,#5287,.T.);
#48396=EDGE_CURVE('',#37453,#37952,#21803,.T.);
#48397=EDGE_CURVE('',#37952,#37953,#21804,.T.);
#48398=EDGE_CURVE('',#37953,#37454,#21805,.T.);
#48399=EDGE_CURVE('',#37953,#37954,#5288,.T.);
#48400=EDGE_CURVE('',#37464,#37954,#21806,.T.);
#48401=EDGE_CURVE('',#37954,#37955,#21807,.T.);
#48402=EDGE_CURVE('',#37955,#37473,#1203,.T.);
#48403=EDGE_CURVE('',#37956,#37471,#5289,.T.);
#48404=EDGE_CURVE('',#37938,#37956,#31173,.T.);
#48405=EDGE_CURVE('',#37957,#37955,#31174,.T.);
#48406=EDGE_CURVE('',#37474,#37957,#5290,.T.);
#48407=EDGE_CURVE('',#37474,#37471,#21808,.T.);
#48408=EDGE_CURVE('',#37632,#37958,#21809,.T.);
#48409=EDGE_CURVE('',#37958,#37959,#21810,.T.);
#48410=EDGE_CURVE('',#37959,#37485,#1943,.T.);
#48411=EDGE_CURVE('',#37959,#37960,#31175,.T.);
#48412=EDGE_CURVE('',#37486,#37960,#1944,.T.);
#48413=EDGE_CURVE('',#37486,#37497,#31176,.T.);
#48414=EDGE_CURVE('',#37498,#37961,#1945,.T.);
#48415=EDGE_CURVE('',#37961,#37962,#21811,.T.);
#48416=EDGE_CURVE('',#37962,#37499,#21812,.T.);
#48417=EDGE_CURVE('',#37963,#37497,#1946,.T.);
#48418=EDGE_CURVE('',#37961,#37963,#31177,.T.);
#48419=EDGE_CURVE('',#37962,#37964,#5291,.T.);
#48420=EDGE_CURVE('',#37500,#37964,#21813,.T.);
#48421=EDGE_CURVE('',#37964,#37965,#31178,.T.);
#48422=EDGE_CURVE('',#37965,#37501,#21814,.T.);
#48423=EDGE_CURVE('',#37965,#37966,#5292,.T.);
#48424=EDGE_CURVE('',#37502,#37966,#21815,.T.);
#48425=EDGE_CURVE('',#37966,#37967,#21816,.T.);
#48426=EDGE_CURVE('',#37967,#37512,#1947,.T.);
#48427=EDGE_CURVE('',#37967,#37968,#31179,.T.);
#48428=EDGE_CURVE('',#37513,#37968,#1948,.T.);
#48429=EDGE_CURVE('',#37513,#37522,#31180,.T.);
#48430=EDGE_CURVE('',#37523,#37969,#1949,.T.);
#48431=EDGE_CURVE('',#37969,#37970,#21817,.T.);
#48432=EDGE_CURVE('',#37970,#37524,#5293,.T.);
#48433=EDGE_CURVE('',#37971,#37522,#1950,.T.);
#48434=EDGE_CURVE('',#37969,#37971,#31181,.T.);
#48435=EDGE_CURVE('',#37970,#37972,#5294,.T.);
#48436=EDGE_CURVE('',#37525,#37972,#5295,.T.);
#48437=EDGE_CURVE('',#37972,#37973,#31182,.T.);
#48438=EDGE_CURVE('',#37973,#37526,#5296,.T.);
#48439=EDGE_CURVE('',#37973,#37974,#5297,.T.);
#48440=EDGE_CURVE('',#37527,#37974,#5298,.T.);
#48441=EDGE_CURVE('',#37974,#37975,#21818,.T.);
#48442=EDGE_CURVE('',#37975,#37536,#1951,.T.);
#48443=EDGE_CURVE('',#37976,#37975,#31183,.T.);
#48444=EDGE_CURVE('',#37537,#37976,#1952,.T.);
#48445=EDGE_CURVE('',#37537,#37546,#31184,.T.);
#48446=EDGE_CURVE('',#37547,#37977,#1953,.T.);
#48447=EDGE_CURVE('',#37977,#37978,#21819,.T.);
#48448=EDGE_CURVE('',#37978,#37548,#5299,.T.);
#48449=EDGE_CURVE('',#37979,#37546,#1954,.T.);
#48450=EDGE_CURVE('',#37977,#37979,#31185,.T.);
#48451=EDGE_CURVE('',#37978,#37980,#5300,.T.);
#48452=EDGE_CURVE('',#37549,#37980,#5301,.T.);
#48453=EDGE_CURVE('',#37980,#37981,#31186,.T.);
#48454=EDGE_CURVE('',#37981,#37550,#5302,.T.);
#48455=EDGE_CURVE('',#37981,#37982,#5303,.T.);
#48456=EDGE_CURVE('',#37551,#37982,#5304,.T.);
#48457=EDGE_CURVE('',#37982,#37983,#21820,.T.);
#48458=EDGE_CURVE('',#37983,#37560,#1955,.T.);
#48459=EDGE_CURVE('',#37984,#37983,#31187,.T.);
#48460=EDGE_CURVE('',#37561,#37984,#1956,.T.);
#48461=EDGE_CURVE('',#37561,#37570,#31188,.T.);
#48462=EDGE_CURVE('',#37571,#37985,#1957,.T.);
#48463=EDGE_CURVE('',#37985,#37986,#21821,.T.);
#48464=EDGE_CURVE('',#37986,#37572,#5305,.T.);
#48465=EDGE_CURVE('',#37987,#37570,#1958,.T.);
#48466=EDGE_CURVE('',#37985,#37987,#31189,.T.);
#48467=EDGE_CURVE('',#37986,#37988,#5306,.T.);
#48468=EDGE_CURVE('',#37573,#37988,#5307,.T.);
#48469=EDGE_CURVE('',#37988,#37989,#31190,.T.);
#48470=EDGE_CURVE('',#37989,#37574,#5308,.T.);
#48471=EDGE_CURVE('',#37989,#37990,#5309,.T.);
#48472=EDGE_CURVE('',#37575,#37990,#5310,.T.);
#48473=EDGE_CURVE('',#37990,#37991,#21822,.T.);
#48474=EDGE_CURVE('',#37991,#37584,#1959,.T.);
#48475=EDGE_CURVE('',#37992,#37991,#31191,.T.);
#48476=EDGE_CURVE('',#37585,#37992,#1960,.T.);
#48477=EDGE_CURVE('',#37585,#37595,#31192,.T.);
#48478=EDGE_CURVE('',#37596,#37993,#1961,.T.);
#48479=EDGE_CURVE('',#37993,#37994,#21823,.T.);
#48480=EDGE_CURVE('',#37994,#37597,#21824,.T.);
#48481=EDGE_CURVE('',#37995,#37595,#1962,.T.);
#48482=EDGE_CURVE('',#37993,#37995,#31193,.T.);
#48483=EDGE_CURVE('',#37994,#37996,#5311,.T.);
#48484=EDGE_CURVE('',#37598,#37996,#21825,.T.);
#48485=EDGE_CURVE('',#37996,#37997,#31194,.T.);
#48486=EDGE_CURVE('',#37997,#37599,#21826,.T.);
#48487=EDGE_CURVE('',#37997,#37998,#5312,.T.);
#48488=EDGE_CURVE('',#37600,#37998,#21827,.T.);
#48489=EDGE_CURVE('',#37998,#37999,#21828,.T.);
#48490=EDGE_CURVE('',#37999,#37611,#1963,.T.);
#48491=EDGE_CURVE('',#37999,#38000,#31195,.T.);
#48492=EDGE_CURVE('',#37612,#38000,#1964,.T.);
#48493=EDGE_CURVE('',#37612,#37617,#31196,.T.);
#48494=EDGE_CURVE('',#38001,#38002,#31197,.T.);
#48495=EDGE_CURVE('',#37618,#38002,#1965,.T.);
#48496=EDGE_CURVE('',#38001,#37617,#5313,.T.);
#48497=EDGE_CURVE('',#38002,#38003,#21829,.T.);
#48498=EDGE_CURVE('',#38003,#37625,#21830,.T.);
#48499=EDGE_CURVE('',#38003,#38004,#5314,.T.);
#48500=EDGE_CURVE('',#38004,#38005,#5315,.T.);
#48501=EDGE_CURVE('',#37626,#38005,#21831,.T.);
#48502=EDGE_CURVE('',#38005,#38006,#31198,.T.);
#48503=EDGE_CURVE('',#38006,#37627,#21832,.T.);
#48504=EDGE_CURVE('',#38006,#38007,#5316,.T.);
#48505=EDGE_CURVE('',#38007,#37898,#1966,.T.);
#48506=EDGE_CURVE('',#37912,#38008,#1967,.T.);
#48507=EDGE_CURVE('',#38008,#38009,#5317,.T.);
#48508=EDGE_CURVE('',#37630,#38009,#21833,.T.);
#48509=EDGE_CURVE('',#38009,#38010,#31199,.T.);
#48510=EDGE_CURVE('',#38010,#37631,#21834,.T.);
#48511=EDGE_CURVE('',#38010,#38011,#5318,.T.);
#48512=EDGE_CURVE('',#38011,#37958,#5319,.T.);
#48513=EDGE_CURVE('',#38012,#38013,#1968,.T.);
#48514=EDGE_CURVE('',#38013,#38014,#21835,.T.);
#48515=EDGE_CURVE('',#38014,#37850,#5320,.T.);
#48516=EDGE_CURVE('',#37849,#38015,#21836,.T.);
#48517=EDGE_CURVE('',#38015,#38016,#5321,.T.);
#48518=EDGE_CURVE('',#38016,#38012,#5322,.T.);
#48519=EDGE_CURVE('',#38014,#38017,#5323,.T.);
#48520=EDGE_CURVE('',#37848,#38017,#5324,.T.);
#48521=EDGE_CURVE('',#38017,#38018,#31200,.T.);
#48522=EDGE_CURVE('',#38018,#37846,#5325,.T.);
#48523=EDGE_CURVE('',#38018,#38019,#5326,.T.);
#48524=EDGE_CURVE('',#37844,#38019,#5327,.T.);
#48525=EDGE_CURVE('',#38019,#38020,#21837,.T.);
#48526=EDGE_CURVE('',#38020,#37633,#1969,.T.);
#48527=EDGE_CURVE('',#37842,#37843,#21838,.T.);
#48528=EDGE_CURVE('',#38020,#38021,#31201,.T.);
#48529=EDGE_CURVE('',#37634,#38021,#1970,.T.);
#48530=EDGE_CURVE('',#37640,#37635,#31202,.T.);
#48531=EDGE_CURVE('',#37634,#37637,#31203,.T.);
#48532=EDGE_CURVE('',#37638,#38022,#1971,.T.);
#48533=EDGE_CURVE('',#38022,#38023,#21839,.T.);
#48534=EDGE_CURVE('',#38023,#37836,#5328,.T.);
#48535=EDGE_CURVE('',#37835,#37837,#21840,.T.);
#48536=EDGE_CURVE('',#38024,#37637,#1972,.T.);
#48537=EDGE_CURVE('',#38022,#38024,#31204,.T.);
#48538=EDGE_CURVE('',#38023,#38025,#5329,.T.);
#48539=EDGE_CURVE('',#37834,#38025,#5330,.T.);
#48540=EDGE_CURVE('',#38025,#38026,#31205,.T.);
#48541=EDGE_CURVE('',#38026,#37832,#5331,.T.);
#48542=EDGE_CURVE('',#38026,#38027,#5332,.T.);
#48543=EDGE_CURVE('',#37830,#38027,#5333,.T.);
#48544=EDGE_CURVE('',#38027,#38028,#21841,.T.);
#48545=EDGE_CURVE('',#38028,#37645,#1973,.T.);
#48546=EDGE_CURVE('',#37828,#37829,#21842,.T.);
#48547=EDGE_CURVE('',#38028,#38029,#31206,.T.);
#48548=EDGE_CURVE('',#37646,#38029,#1974,.T.);
#48549=EDGE_CURVE('',#37646,#37647,#31207,.T.);
#48550=EDGE_CURVE('',#38030,#38031,#31208,.T.);
#48551=EDGE_CURVE('',#37648,#38031,#1975,.T.);
#48552=EDGE_CURVE('',#38030,#37647,#1976,.T.);
#48553=EDGE_CURVE('',#38031,#38032,#21843,.T.);
#48554=EDGE_CURVE('',#38032,#37657,#21844,.T.);
#48555=EDGE_CURVE('',#37821,#37822,#21845,.T.);
#48556=EDGE_CURVE('',#38032,#38033,#5334,.T.);
#48557=EDGE_CURVE('',#37658,#38033,#21846,.T.);
#48558=EDGE_CURVE('',#38033,#38034,#31209,.T.);
#48559=EDGE_CURVE('',#38034,#37660,#21847,.T.);
#48560=EDGE_CURVE('',#38034,#38035,#5335,.T.);
#48561=EDGE_CURVE('',#37661,#38035,#21848,.T.);
#48562=EDGE_CURVE('',#38035,#38036,#21849,.T.);
#48563=EDGE_CURVE('',#38036,#37671,#1977,.T.);
#48564=EDGE_CURVE('',#37817,#37818,#21850,.T.);
#48565=EDGE_CURVE('',#38036,#38037,#31210,.T.);
#48566=EDGE_CURVE('',#37672,#38037,#5336,.T.);
#48567=EDGE_CURVE('',#37672,#38038,#31211,.T.);
#48568=EDGE_CURVE('',#38038,#38039,#5337,.T.);
#48569=EDGE_CURVE('',#38039,#37669,#5338,.T.);
#48570=EDGE_CURVE('',#38040,#37673,#21851,.T.);
#48571=EDGE_CURVE('',#38040,#38041,#5339,.T.);
#48572=EDGE_CURVE('',#37674,#38041,#21852,.T.);
#48573=EDGE_CURVE('',#38041,#38042,#21853,.T.);
#48574=EDGE_CURVE('',#38042,#37685,#1978,.T.);
#48575=EDGE_CURVE('',#37775,#37776,#21854,.T.);
#48576=EDGE_CURVE('',#38043,#38042,#31212,.T.);
#48577=EDGE_CURVE('',#37686,#38043,#1979,.T.);
#48578=EDGE_CURVE('',#37686,#37697,#31213,.T.);
#48579=EDGE_CURVE('',#37771,#37772,#21855,.T.);
#48580=EDGE_CURVE('',#37698,#38044,#1980,.T.);
#48581=EDGE_CURVE('',#38044,#38045,#21856,.T.);
#48582=EDGE_CURVE('',#38045,#37699,#21857,.T.);
#48583=EDGE_CURVE('',#38046,#37697,#1981,.T.);
#48584=EDGE_CURVE('',#38044,#38046,#31214,.T.);
#48585=EDGE_CURVE('',#38045,#38047,#5340,.T.);
#48586=EDGE_CURVE('',#37700,#38047,#21858,.T.);
#48587=EDGE_CURVE('',#38047,#38048,#31215,.T.);
#48588=EDGE_CURVE('',#38048,#37701,#21859,.T.);
#48589=EDGE_CURVE('',#38048,#38049,#5341,.T.);
#48590=EDGE_CURVE('',#37702,#38049,#21860,.T.);
#48591=EDGE_CURVE('',#38049,#38050,#21861,.T.);
#48592=EDGE_CURVE('',#38050,#37713,#1982,.T.);
#48593=EDGE_CURVE('',#37767,#37768,#21862,.T.);
#48594=EDGE_CURVE('',#38051,#38050,#31216,.T.);
#48595=EDGE_CURVE('',#38052,#38051,#31217,.T.);
#48596=EDGE_CURVE('',#37714,#38052,#1983,.T.);
#48597=EDGE_CURVE('',#37714,#37722,#31218,.T.);
#48598=EDGE_CURVE('',#37763,#37764,#21863,.T.);
#48599=EDGE_CURVE('',#37723,#38053,#1984,.T.);
#48600=EDGE_CURVE('',#38053,#38054,#21864,.T.);
#48601=EDGE_CURVE('',#38054,#37726,#5342,.T.);
#48602=EDGE_CURVE('',#38055,#37722,#1985,.T.);
#48603=EDGE_CURVE('',#38053,#38055,#31219,.T.);
#48604=EDGE_CURVE('',#38054,#38056,#5343,.T.);
#48605=EDGE_CURVE('',#37727,#38056,#5344,.T.);
#48606=EDGE_CURVE('',#38056,#38057,#31220,.T.);
#48607=EDGE_CURVE('',#38057,#37728,#5345,.T.);
#48608=EDGE_CURVE('',#38057,#38058,#5346,.T.);
#48609=EDGE_CURVE('',#37730,#38058,#5347,.T.);
#48610=EDGE_CURVE('',#38058,#38059,#21865,.T.);
#48611=EDGE_CURVE('',#38059,#37739,#1986,.T.);
#48612=EDGE_CURVE('',#37759,#37760,#21866,.T.);
#48613=EDGE_CURVE('',#38060,#38059,#31221,.T.);
#48614=EDGE_CURVE('',#38061,#38060,#31222,.T.);
#48615=EDGE_CURVE('',#37740,#38061,#1987,.T.);
#48616=EDGE_CURVE('',#37740,#37748,#31223,.T.);
#48617=EDGE_CURVE('',#38062,#38063,#5348,.T.);
#48618=EDGE_CURVE('',#38063,#37756,#21867,.T.);
#48619=EDGE_CURVE('',#37749,#38064,#1988,.T.);
#48620=EDGE_CURVE('',#38064,#38065,#21868,.T.);
#48621=EDGE_CURVE('',#38065,#38066,#5349,.T.);
#48622=EDGE_CURVE('',#38066,#38062,#21869,.T.);
#48623=EDGE_CURVE('',#38067,#37748,#1989,.T.);
#48624=EDGE_CURVE('',#38064,#38067,#31224,.T.);
#48625=EDGE_CURVE('',#38065,#38068,#5350,.T.);
#48626=EDGE_CURVE('',#38069,#38068,#5351,.T.);
#48627=EDGE_CURVE('',#38069,#38066,#31225,.T.);
#48628=EDGE_CURVE('',#38070,#38062,#31226,.T.);
#48629=EDGE_CURVE('',#38070,#38069,#21870,.T.);
#48630=EDGE_CURVE('',#38071,#38070,#5352,.T.);
#48631=EDGE_CURVE('',#38071,#38063,#5353,.T.);
#48632=EDGE_CURVE('',#37750,#38072,#31227,.T.);
#48633=EDGE_CURVE('',#38073,#38072,#31228,.T.);
#48634=EDGE_CURVE('',#37751,#38073,#31229,.T.);
#48635=EDGE_CURVE('',#37754,#38073,#5354,.T.);
#48636=EDGE_CURVE('',#38074,#37754,#21871,.T.);
#48637=EDGE_CURVE('',#38074,#37781,#31230,.T.);
#48638=EDGE_CURVE('',#38071,#38075,#31231,.T.);
#48639=EDGE_CURVE('',#38076,#38075,#5355,.T.);
#48640=EDGE_CURVE('',#38063,#38076,#31232,.T.);
#48641=EDGE_CURVE('',#37757,#38076,#21872,.T.);
#48642=EDGE_CURVE('',#37758,#37757,#31233,.T.);
#48643=EDGE_CURVE('',#38077,#37760,#31234,.T.);
#48644=EDGE_CURVE('',#38077,#37758,#21873,.T.);
#48645=EDGE_CURVE('',#37761,#38078,#31235,.T.);
#48646=EDGE_CURVE('',#38078,#38077,#5356,.T.);
#48647=EDGE_CURVE('',#38079,#38078,#31236,.T.);
#48648=EDGE_CURVE('',#37762,#38079,#31237,.T.);
#48649=EDGE_CURVE('',#38080,#38079,#5357,.T.);
#48650=EDGE_CURVE('',#37763,#38080,#31238,.T.);
#48651=EDGE_CURVE('',#37765,#38080,#21874,.T.);
#48652=EDGE_CURVE('',#37766,#37765,#31239,.T.);
#48653=EDGE_CURVE('',#38081,#37768,#31240,.T.);
#48654=EDGE_CURVE('',#38081,#37766,#21875,.T.);
#48655=EDGE_CURVE('',#37769,#38082,#31241,.T.);
#48656=EDGE_CURVE('',#38082,#38081,#5358,.T.);
#48657=EDGE_CURVE('',#38083,#38082,#31242,.T.);
#48658=EDGE_CURVE('',#37770,#38083,#31243,.T.);
#48659=EDGE_CURVE('',#38084,#38083,#5359,.T.);
#48660=EDGE_CURVE('',#37771,#38084,#31244,.T.);
#48661=EDGE_CURVE('',#37773,#38084,#21876,.T.);
#48662=EDGE_CURVE('',#37774,#37773,#31245,.T.);
#48663=EDGE_CURVE('',#38085,#37776,#31246,.T.);
#48664=EDGE_CURVE('',#38085,#37774,#21877,.T.);
#48665=EDGE_CURVE('',#38072,#38085,#5360,.T.);
#48666=EDGE_CURVE('',#37779,#38086,#21878,.T.);
#48667=EDGE_CURVE('',#38086,#38086,#31247,.T.);
#48668=EDGE_CURVE('',#37780,#38087,#21879,.T.);
#48669=EDGE_CURVE('',#38087,#38087,#31248,.T.);
#48670=EDGE_CURVE('',#38074,#38088,#31249,.T.);
#48671=EDGE_CURVE('',#38089,#38088,#31250,.T.);
#48672=EDGE_CURVE('',#37781,#38089,#31251,.T.);
#48673=EDGE_CURVE('',#38090,#38089,#21880,.T.);
#48674=EDGE_CURVE('',#37782,#38090,#31252,.T.);
#48675=EDGE_CURVE('',#38091,#38090,#31253,.T.);
#48676=EDGE_CURVE('',#37783,#38091,#31254,.T.);
#48677=EDGE_CURVE('',#38092,#38091,#31255,.T.);
#48678=EDGE_CURVE('',#37784,#38092,#31256,.T.);
#48679=EDGE_CURVE('',#38093,#38092,#31257,.T.);
#48680=EDGE_CURVE('',#37785,#38093,#31258,.T.);
#48681=EDGE_CURVE('',#38094,#38093,#21881,.T.);
#48682=EDGE_CURVE('',#37786,#38094,#31259,.T.);
#48683=EDGE_CURVE('',#38095,#38094,#31260,.T.);
#48684=EDGE_CURVE('',#37787,#38095,#31261,.T.);
#48685=EDGE_CURVE('',#38096,#38095,#31262,.T.);
#48686=EDGE_CURVE('',#37788,#38096,#31263,.T.);
#48687=EDGE_CURVE('',#38097,#38096,#31264,.T.);
#48688=EDGE_CURVE('',#37789,#38097,#31265,.T.);
#48689=EDGE_CURVE('',#38098,#38097,#21882,.T.);
#48690=EDGE_CURVE('',#37790,#38098,#31266,.T.);
#48691=EDGE_CURVE('',#38099,#38098,#31267,.T.);
#48692=EDGE_CURVE('',#37791,#38099,#31268,.T.);
#48693=EDGE_CURVE('',#38100,#38099,#31269,.T.);
#48694=EDGE_CURVE('',#37792,#38100,#31270,.T.);
#48695=EDGE_CURVE('',#38101,#38100,#31271,.T.);
#48696=EDGE_CURVE('',#37793,#38101,#31272,.T.);
#48697=EDGE_CURVE('',#38102,#38101,#21883,.T.);
#48698=EDGE_CURVE('',#37794,#38102,#31273,.T.);
#48699=EDGE_CURVE('',#38103,#38102,#31274,.T.);
#48700=EDGE_CURVE('',#38104,#38103,#31275,.T.);
#48701=EDGE_CURVE('',#37794,#38104,#31276,.T.);
#48702=EDGE_CURVE('',#38105,#38104,#21884,.T.);
#48703=EDGE_CURVE('',#38105,#37795,#31277,.T.);
#48704=EDGE_CURVE('',#38106,#37795,#31278,.T.);
#48705=EDGE_CURVE('',#37799,#38106,#21885,.T.);
#48706=EDGE_CURVE('',#38107,#38105,#31279,.T.);
#48707=EDGE_CURVE('',#38106,#38107,#31280,.T.);
#48708=EDGE_CURVE('',#37798,#38108,#21886,.T.);
#48709=EDGE_CURVE('',#38109,#37799,#21887,.T.);
#48710=EDGE_CURVE('',#38108,#38109,#31281,.T.);
#48711=EDGE_CURVE('',#38110,#38108,#21888,.T.);
#48712=EDGE_CURVE('',#38110,#37805,#21889,.T.);
#48713=EDGE_CURVE('',#38111,#37858,#31282,.T.);
#48714=EDGE_CURVE('',#37807,#38111,#21890,.T.);
#48715=EDGE_CURVE('',#37808,#37807,#21891,.T.);
#48716=EDGE_CURVE('',#38112,#37810,#31283,.T.);
#48717=EDGE_CURVE('',#38112,#37808,#21892,.T.);
#48718=EDGE_CURVE('',#38113,#37811,#31284,.T.);
#48719=EDGE_CURVE('',#38113,#38112,#31285,.T.);
#48720=EDGE_CURVE('',#38114,#37812,#31286,.T.);
#48721=EDGE_CURVE('',#38114,#38113,#21893,.T.);
#48722=EDGE_CURVE('',#38115,#37813,#31287,.T.);
#48723=EDGE_CURVE('',#38115,#38114,#31288,.T.);
#48724=EDGE_CURVE('',#37815,#38115,#21894,.T.);
#48725=EDGE_CURVE('',#37816,#37815,#21895,.T.);
#48726=EDGE_CURVE('',#38116,#37818,#31289,.T.);
#48727=EDGE_CURVE('',#38116,#37816,#21896,.T.);
#48728=EDGE_CURVE('',#38117,#37819,#31290,.T.);
#48729=EDGE_CURVE('',#38117,#38116,#31291,.T.);
#48730=EDGE_CURVE('',#38118,#37820,#31292,.T.);
#48731=EDGE_CURVE('',#38118,#38117,#21897,.T.);
#48732=EDGE_CURVE('',#38119,#37821,#31293,.T.);
#48733=EDGE_CURVE('',#38119,#38118,#31294,.T.);
#48734=EDGE_CURVE('',#37823,#38119,#21898,.T.);
#48735=EDGE_CURVE('',#38120,#37823,#21899,.T.);
#48736=EDGE_CURVE('',#37824,#38120,#31295,.T.);
#48737=EDGE_CURVE('',#37825,#38121,#31296,.T.);
#48738=EDGE_CURVE('',#38121,#38120,#5361,.T.);
#48739=EDGE_CURVE('',#37827,#38121,#31297,.T.);
#48740=EDGE_CURVE('',#38122,#37829,#31298,.T.);
#48741=EDGE_CURVE('',#38122,#37827,#21900,.T.);
#48742=EDGE_CURVE('',#38123,#37831,#31299,.T.);
#48743=EDGE_CURVE('',#38123,#38122,#31300,.T.);
#48744=EDGE_CURVE('',#38124,#37833,#31301,.T.);
#48745=EDGE_CURVE('',#38124,#38123,#21901,.T.);
#48746=EDGE_CURVE('',#38125,#37835,#31302,.T.);
#48747=EDGE_CURVE('',#38125,#38124,#31303,.T.);
#48748=EDGE_CURVE('',#37838,#38125,#21902,.T.);
#48749=EDGE_CURVE('',#37841,#37838,#31304,.T.);
#48750=EDGE_CURVE('',#38126,#37843,#31305,.T.);
#48751=EDGE_CURVE('',#38126,#37841,#21903,.T.);
#48752=EDGE_CURVE('',#38127,#37845,#31306,.T.);
#48753=EDGE_CURVE('',#38127,#38126,#31307,.T.);
#48754=EDGE_CURVE('',#38128,#37847,#31308,.T.);
#48755=EDGE_CURVE('',#38128,#38127,#21904,.T.);
#48756=EDGE_CURVE('',#38129,#37849,#31309,.T.);
#48757=EDGE_CURVE('',#38129,#38128,#31310,.T.);
#48758=EDGE_CURVE('',#38130,#38015,#31311,.T.);
#48759=EDGE_CURVE('',#38130,#38129,#21905,.T.);
#48760=EDGE_CURVE('',#38131,#38110,#31312,.T.);
#48761=EDGE_CURVE('',#37856,#38131,#21906,.T.);
#48762=EDGE_CURVE('',#38132,#37857,#31313,.T.);
#48763=EDGE_CURVE('',#38132,#37856,#21907,.T.);
#48764=EDGE_CURVE('',#38111,#38132,#31314,.T.);
#48765=EDGE_CURVE('',#38133,#38016,#31315,.T.);
#48766=EDGE_CURVE('',#38134,#38130,#5362,.T.);
#48767=EDGE_CURVE('',#38133,#38134,#1990,.T.);
#48768=EDGE_CURVE('',#38135,#38012,#31316,.T.);
#48769=EDGE_CURVE('',#38135,#38133,#5363,.T.);
#48770=EDGE_CURVE('',#38136,#38135,#1991,.T.);
#48771=EDGE_CURVE('',#38013,#38136,#31317,.T.);
#48772=EDGE_CURVE('',#37947,#38137,#5364,.T.);
#48773=EDGE_CURVE('',#38137,#38138,#5365,.T.);
#48774=EDGE_CURVE('',#37860,#38138,#21908,.T.);
#48775=EDGE_CURVE('',#38138,#38139,#31318,.T.);
#48776=EDGE_CURVE('',#38139,#38040,#31319,.T.);
#48777=EDGE_CURVE('',#38140,#37867,#21909,.T.);
#48778=EDGE_CURVE('',#37862,#38141,#21910,.T.);
#48779=EDGE_CURVE('',#38141,#38142,#31320,.T.);
#48780=EDGE_CURVE('',#38142,#38143,#21911,.T.);
#48781=EDGE_CURVE('',#38143,#38140,#31321,.T.);
#48782=EDGE_CURVE('',#38144,#37878,#21912,.T.);
#48783=EDGE_CURVE('',#37871,#38145,#21913,.T.);
#48784=EDGE_CURVE('',#38145,#38146,#31322,.T.);
#48785=EDGE_CURVE('',#38146,#38147,#21914,.T.);
#48786=EDGE_CURVE('',#38147,#38144,#31323,.T.);
#48787=EDGE_CURVE('',#37883,#38148,#21915,.T.);
#48788=EDGE_CURVE('',#38148,#37880,#31324,.T.);
#48789=EDGE_CURVE('',#37882,#38149,#31325,.T.);
#48790=EDGE_CURVE('',#38150,#37883,#21916,.T.);
#48791=EDGE_CURVE('',#38149,#38150,#31326,.T.);
#48792=EDGE_CURVE('',#38151,#37885,#31327,.T.);
#48793=EDGE_CURVE('',#38151,#38150,#5366,.T.);
#48794=EDGE_CURVE('',#38152,#37886,#31328,.T.);
#48795=EDGE_CURVE('',#38152,#38151,#21917,.T.);
#48796=EDGE_CURVE('',#38153,#37887,#31329,.T.);
#48797=EDGE_CURVE('',#38153,#38152,#5367,.T.);
#48798=EDGE_CURVE('',#37889,#38153,#21918,.T.);
#48799=EDGE_CURVE('',#37890,#37889,#21919,.T.);
#48800=EDGE_CURVE('',#38154,#37892,#31330,.T.);
#48801=EDGE_CURVE('',#38154,#37890,#21920,.T.);
#48802=EDGE_CURVE('',#38155,#37893,#31331,.T.);
#48803=EDGE_CURVE('',#38155,#38154,#5368,.T.);
#48804=EDGE_CURVE('',#38156,#37894,#31332,.T.);
#48805=EDGE_CURVE('',#38156,#38155,#21921,.T.);
#48806=EDGE_CURVE('',#38157,#37895,#31333,.T.);
#48807=EDGE_CURVE('',#38157,#38156,#5369,.T.);
#48808=EDGE_CURVE('',#37897,#38157,#21922,.T.);
#48809=EDGE_CURVE('',#38158,#37897,#21923,.T.);
#48810=EDGE_CURVE('',#38158,#38141,#31334,.T.);
#48811=EDGE_CURVE('',#38159,#38007,#31335,.T.);
#48812=EDGE_CURVE('',#38160,#38159,#1992,.T.);
#48813=EDGE_CURVE('',#37898,#38160,#31336,.T.);
#48814=EDGE_CURVE('',#37900,#38160,#21924,.T.);
#48815=EDGE_CURVE('',#38148,#37900,#5370,.T.);
#48816=EDGE_CURVE('',#38161,#37920,#21925,.T.);
#48817=EDGE_CURVE('',#37902,#38161,#31337,.T.);
#48818=EDGE_CURVE('',#38162,#37903,#31338,.T.);
#48819=EDGE_CURVE('',#38162,#38161,#5371,.T.);
#48820=EDGE_CURVE('',#38163,#37904,#31339,.T.);
#48821=EDGE_CURVE('',#38163,#38162,#21926,.T.);
#48822=EDGE_CURVE('',#38164,#37905,#31340,.T.);
#48823=EDGE_CURVE('',#38164,#38163,#5372,.T.);
#48824=EDGE_CURVE('',#37907,#38164,#21927,.T.);
#48825=EDGE_CURVE('',#38165,#37907,#21928,.T.);
#48826=EDGE_CURVE('',#37908,#38165,#31341,.T.);
#48827=EDGE_CURVE('',#37910,#38165,#5373,.T.);
#48828=EDGE_CURVE('',#38166,#37912,#31342,.T.);
#48829=EDGE_CURVE('',#38166,#37910,#21929,.T.);
#48830=EDGE_CURVE('',#38167,#38008,#31343,.T.);
#48831=EDGE_CURVE('',#38167,#38166,#1993,.T.);
#48832=EDGE_CURVE('',#37915,#38168,#21930,.T.);
#48833=EDGE_CURVE('',#38168,#38144,#31344,.T.);
#48834=EDGE_CURVE('',#38169,#37915,#21931,.T.);
#48835=EDGE_CURVE('',#37914,#38169,#31345,.T.);
#48836=EDGE_CURVE('',#38170,#38169,#5374,.T.);
#48837=EDGE_CURVE('',#37916,#38170,#31346,.T.);
#48838=EDGE_CURVE('',#38171,#38170,#21932,.T.);
#48839=EDGE_CURVE('',#37917,#38171,#31347,.T.);
#48840=EDGE_CURVE('',#38172,#38171,#5375,.T.);
#48841=EDGE_CURVE('',#37918,#38172,#31348,.T.);
#48842=EDGE_CURVE('',#37921,#38172,#21933,.T.);
#48843=EDGE_CURVE('',#37920,#37921,#21934,.T.);
#48844=EDGE_CURVE('',#38173,#38147,#31349,.T.);
#48845=EDGE_CURVE('',#38174,#38146,#31350,.T.);
#48846=EDGE_CURVE('',#38173,#38174,#21935,.T.);
#48847=EDGE_CURVE('',#38175,#37923,#31351,.T.);
#48848=EDGE_CURVE('',#38175,#37936,#21936,.T.);
#48849=EDGE_CURVE('',#38176,#37924,#31352,.T.);
#48850=EDGE_CURVE('',#38176,#38175,#5376,.T.);
#48851=EDGE_CURVE('',#38177,#37925,#31353,.T.);
#48852=EDGE_CURVE('',#38177,#38176,#21937,.T.);
#48853=EDGE_CURVE('',#38178,#37926,#31354,.T.);
#48854=EDGE_CURVE('',#38178,#38177,#5377,.T.);
#48855=EDGE_CURVE('',#37928,#38178,#21938,.T.);
#48856=EDGE_CURVE('',#38179,#37928,#21939,.T.);
#48857=EDGE_CURVE('',#38179,#38145,#31355,.T.);
#48858=EDGE_CURVE('',#37929,#38180,#5378,.T.);
#48859=EDGE_CURVE('',#38180,#38039,#31356,.T.);
#48860=EDGE_CURVE('',#37931,#38181,#31357,.T.);
#48861=EDGE_CURVE('',#38181,#37929,#21940,.T.);
#48862=EDGE_CURVE('',#38182,#38181,#5379,.T.);
#48863=EDGE_CURVE('',#37932,#38182,#31358,.T.);
#48864=EDGE_CURVE('',#38183,#38182,#21941,.T.);
#48865=EDGE_CURVE('',#37933,#38183,#31359,.T.);
#48866=EDGE_CURVE('',#38184,#38183,#5380,.T.);
#48867=EDGE_CURVE('',#37934,#38184,#31360,.T.);
#48868=EDGE_CURVE('',#37937,#38184,#21942,.T.);
#48869=EDGE_CURVE('',#37936,#37937,#21943,.T.);
#48870=EDGE_CURVE('',#38185,#38038,#31361,.T.);
#48871=EDGE_CURVE('',#38180,#38185,#5381,.T.);
#48872=EDGE_CURVE('',#38186,#38143,#31362,.T.);
#48873=EDGE_CURVE('',#38187,#38142,#31363,.T.);
#48874=EDGE_CURVE('',#38186,#38187,#21944,.T.);
#48875=EDGE_CURVE('',#38188,#37956,#21945,.T.);
#48876=EDGE_CURVE('',#37939,#38188,#31364,.T.);
#48877=EDGE_CURVE('',#38189,#37940,#31365,.T.);
#48878=EDGE_CURVE('',#38189,#38188,#5382,.T.);
#48879=EDGE_CURVE('',#38190,#37941,#31366,.T.);
#48880=EDGE_CURVE('',#38190,#38189,#21946,.T.);
#48881=EDGE_CURVE('',#38191,#37942,#31367,.T.);
#48882=EDGE_CURVE('',#38191,#38190,#5383,.T.);
#48883=EDGE_CURVE('',#37944,#38191,#21947,.T.);
#48884=EDGE_CURVE('',#38192,#37944,#21948,.T.);
#48885=EDGE_CURVE('',#37945,#38192,#31368,.T.);
#48886=EDGE_CURVE('',#37948,#38192,#5384,.T.);
#48887=EDGE_CURVE('',#38193,#37948,#21949,.T.);
#48888=EDGE_CURVE('',#37947,#38193,#31369,.T.);
#48889=EDGE_CURVE('',#38194,#38137,#31370,.T.);
#48890=EDGE_CURVE('',#38194,#38193,#5385,.T.);
#48891=EDGE_CURVE('',#37949,#38195,#21950,.T.);
#48892=EDGE_CURVE('',#38195,#38140,#31371,.T.);
#48893=EDGE_CURVE('',#38196,#37951,#31372,.T.);
#48894=EDGE_CURVE('',#38196,#37949,#21951,.T.);
#48895=EDGE_CURVE('',#38197,#37952,#31373,.T.);
#48896=EDGE_CURVE('',#38197,#38196,#5386,.T.);
#48897=EDGE_CURVE('',#38198,#37953,#31374,.T.);
#48898=EDGE_CURVE('',#38198,#38197,#21952,.T.);
#48899=EDGE_CURVE('',#38199,#37954,#31375,.T.);
#48900=EDGE_CURVE('',#38199,#38198,#5387,.T.);
#48901=EDGE_CURVE('',#37957,#38199,#21953,.T.);
#48902=EDGE_CURVE('',#37956,#37957,#21954,.T.);
#48903=EDGE_CURVE('',#38011,#38200,#31376,.T.);
#48904=EDGE_CURVE('',#38201,#38200,#5388,.T.);
#48905=EDGE_CURVE('',#37958,#38201,#31377,.T.);
#48906=EDGE_CURVE('',#37960,#38201,#21955,.T.);
#48907=EDGE_CURVE('',#37963,#37960,#31378,.T.);
#48908=EDGE_CURVE('',#38202,#37963,#21956,.T.);
#48909=EDGE_CURVE('',#37962,#38202,#31379,.T.);
#48910=EDGE_CURVE('',#38203,#38202,#5389,.T.);
#48911=EDGE_CURVE('',#37964,#38203,#31380,.T.);
#48912=EDGE_CURVE('',#38204,#38203,#31381,.T.);
#48913=EDGE_CURVE('',#37965,#38204,#31382,.T.);
#48914=EDGE_CURVE('',#38205,#38204,#5390,.T.);
#48915=EDGE_CURVE('',#37966,#38205,#31383,.T.);
#48916=EDGE_CURVE('',#37968,#38205,#21957,.T.);
#48917=EDGE_CURVE('',#37971,#37968,#31384,.T.);
#48918=EDGE_CURVE('',#38206,#37971,#21958,.T.);
#48919=EDGE_CURVE('',#37970,#38206,#31385,.T.);
#48920=EDGE_CURVE('',#38207,#37972,#31386,.T.);
#48921=EDGE_CURVE('',#38207,#38206,#5391,.T.);
#48922=EDGE_CURVE('',#38208,#37973,#31387,.T.);
#48923=EDGE_CURVE('',#38208,#38207,#31388,.T.);
#48924=EDGE_CURVE('',#38209,#37974,#31389,.T.);
#48925=EDGE_CURVE('',#38209,#38208,#5392,.T.);
#48926=EDGE_CURVE('',#37976,#38209,#21959,.T.);
#48927=EDGE_CURVE('',#37979,#37976,#31390,.T.);
#48928=EDGE_CURVE('',#38210,#37979,#21960,.T.);
#48929=EDGE_CURVE('',#37978,#38210,#31391,.T.);
#48930=EDGE_CURVE('',#38211,#37980,#31392,.T.);
#48931=EDGE_CURVE('',#38211,#38210,#5393,.T.);
#48932=EDGE_CURVE('',#38212,#37981,#31393,.T.);
#48933=EDGE_CURVE('',#38212,#38211,#31394,.T.);
#48934=EDGE_CURVE('',#38213,#37982,#31395,.T.);
#48935=EDGE_CURVE('',#38213,#38212,#5394,.T.);
#48936=EDGE_CURVE('',#37984,#38213,#21961,.T.);
#48937=EDGE_CURVE('',#37987,#37984,#31396,.T.);
#48938=EDGE_CURVE('',#38214,#37987,#21962,.T.);
#48939=EDGE_CURVE('',#37986,#38214,#31397,.T.);
#48940=EDGE_CURVE('',#38215,#37988,#31398,.T.);
#48941=EDGE_CURVE('',#38215,#38214,#5395,.T.);
#48942=EDGE_CURVE('',#38216,#37989,#31399,.T.);
#48943=EDGE_CURVE('',#38216,#38215,#31400,.T.);
#48944=EDGE_CURVE('',#38217,#37990,#31401,.T.);
#48945=EDGE_CURVE('',#38217,#38216,#5396,.T.);
#48946=EDGE_CURVE('',#37992,#38217,#21963,.T.);
#48947=EDGE_CURVE('',#37995,#37992,#31402,.T.);
#48948=EDGE_CURVE('',#38218,#37995,#21964,.T.);
#48949=EDGE_CURVE('',#37994,#38218,#31403,.T.);
#48950=EDGE_CURVE('',#38219,#38218,#5397,.T.);
#48951=EDGE_CURVE('',#37996,#38219,#31404,.T.);
#48952=EDGE_CURVE('',#38220,#38219,#31405,.T.);
#48953=EDGE_CURVE('',#37997,#38220,#31406,.T.);
#48954=EDGE_CURVE('',#38221,#38220,#5398,.T.);
#48955=EDGE_CURVE('',#37998,#38221,#31407,.T.);
#48956=EDGE_CURVE('',#38000,#38221,#21965,.T.);
#48957=EDGE_CURVE('',#38001,#38000,#31408,.T.);
#48958=EDGE_CURVE('',#38222,#38003,#31409,.T.);
#48959=EDGE_CURVE('',#38222,#38001,#21966,.T.);
#48960=EDGE_CURVE('',#38223,#38004,#31410,.T.);
#48961=EDGE_CURVE('',#38223,#38222,#5399,.T.);
#48962=EDGE_CURVE('',#38180,#38224,#21967,.T.);
#48963=EDGE_CURVE('',#38224,#38225,#21968,.T.);
#48964=EDGE_CURVE('',#38225,#38179,#21969,.T.);
#48965=EDGE_CURVE('',#38174,#38179,#31411,.T.);
#48966=EDGE_CURVE('',#38226,#38173,#21970,.T.);
#48967=EDGE_CURVE('',#38174,#38227,#21971,.T.);
#48968=EDGE_CURVE('',#38227,#38226,#21972,.T.);
#48969=EDGE_CURVE('',#38227,#38225,#31412,.T.);
#48970=EDGE_CURVE('',#38168,#38173,#31413,.T.);
#48971=EDGE_CURVE('',#38168,#38228,#21973,.T.);
#48972=EDGE_CURVE('',#38228,#38229,#21974,.T.);
#48973=EDGE_CURVE('',#38229,#38167,#21975,.T.);
#48974=EDGE_CURVE('',#38228,#38226,#31414,.T.);
#48975=EDGE_CURVE('',#38230,#38009,#31415,.T.);
#48976=EDGE_CURVE('',#38230,#38167,#5400,.T.);
#48977=EDGE_CURVE('',#38010,#38231,#31416,.T.);
#48978=EDGE_CURVE('',#38231,#38230,#31417,.T.);
#48979=EDGE_CURVE('',#38200,#38231,#31418,.T.);
#48980=EDGE_CURVE('',#38232,#38233,#31419,.T.);
#48981=EDGE_CURVE('',#38232,#38223,#21976,.T.);
#48982=EDGE_CURVE('',#38200,#38233,#21977,.T.);
#48983=EDGE_CURVE('',#38233,#38229,#31420,.T.);
#48984=EDGE_CURVE('',#38234,#38005,#31421,.T.);
#48985=EDGE_CURVE('',#38234,#38223,#5401,.T.);
#48986=EDGE_CURVE('',#38235,#38006,#31422,.T.);
#48987=EDGE_CURVE('',#38235,#38234,#31423,.T.);
#48988=EDGE_CURVE('',#38159,#38235,#5402,.T.);
#48989=EDGE_CURVE('',#38236,#38136,#21978,.T.);
#48990=EDGE_CURVE('',#38014,#38236,#31424,.T.);
#48991=EDGE_CURVE('',#38237,#38236,#5403,.T.);
#48992=EDGE_CURVE('',#38017,#38237,#31425,.T.);
#48993=EDGE_CURVE('',#38238,#38237,#31426,.T.);
#48994=EDGE_CURVE('',#38018,#38238,#31427,.T.);
#48995=EDGE_CURVE('',#38239,#38238,#5404,.T.);
#48996=EDGE_CURVE('',#38019,#38239,#31428,.T.);
#48997=EDGE_CURVE('',#38021,#38239,#21979,.T.);
#48998=EDGE_CURVE('',#38024,#38021,#31429,.T.);
#48999=EDGE_CURVE('',#38240,#38024,#21980,.T.);
#49000=EDGE_CURVE('',#38023,#38240,#31430,.T.);
#49001=EDGE_CURVE('',#38241,#38240,#5405,.T.);
#49002=EDGE_CURVE('',#38025,#38241,#31431,.T.);
#49003=EDGE_CURVE('',#38242,#38241,#31432,.T.);
#49004=EDGE_CURVE('',#38026,#38242,#31433,.T.);
#49005=EDGE_CURVE('',#38243,#38242,#5406,.T.);
#49006=EDGE_CURVE('',#38027,#38243,#31434,.T.);
#49007=EDGE_CURVE('',#38029,#38243,#21981,.T.);
#49008=EDGE_CURVE('',#38030,#38029,#31435,.T.);
#49009=EDGE_CURVE('',#38032,#38244,#31436,.T.);
#49010=EDGE_CURVE('',#38244,#38030,#21982,.T.);
#49011=EDGE_CURVE('',#38245,#38244,#5407,.T.);
#49012=EDGE_CURVE('',#38033,#38245,#31437,.T.);
#49013=EDGE_CURVE('',#38246,#38245,#31438,.T.);
#49014=EDGE_CURVE('',#38034,#38246,#31439,.T.);
#49015=EDGE_CURVE('',#38247,#38246,#5408,.T.);
#49016=EDGE_CURVE('',#38035,#38247,#31440,.T.);
#49017=EDGE_CURVE('',#38037,#38247,#21983,.T.);
#49018=EDGE_CURVE('',#38185,#38037,#31441,.T.);
#49019=EDGE_CURVE('',#38248,#38185,#21984,.T.);
#49020=EDGE_CURVE('',#38224,#38248,#31442,.T.);
#49021=EDGE_CURVE('',#38249,#38040,#31443,.T.);
#49022=EDGE_CURVE('',#38250,#38139,#31444,.T.);
#49023=EDGE_CURVE('',#38249,#38250,#31445,.T.);
#49024=EDGE_CURVE('',#38251,#38041,#31446,.T.);
#49025=EDGE_CURVE('',#38251,#38249,#5409,.T.);
#49026=EDGE_CURVE('',#38043,#38251,#21985,.T.);
#49027=EDGE_CURVE('',#38046,#38043,#31447,.T.);
#49028=EDGE_CURVE('',#38252,#38046,#21986,.T.);
#49029=EDGE_CURVE('',#38045,#38252,#31448,.T.);
#49030=EDGE_CURVE('',#38253,#38047,#31449,.T.);
#49031=EDGE_CURVE('',#38253,#38252,#5410,.T.);
#49032=EDGE_CURVE('',#38254,#38048,#31450,.T.);
#49033=EDGE_CURVE('',#38254,#38253,#31451,.T.);
#49034=EDGE_CURVE('',#38255,#38049,#31452,.T.);
#49035=EDGE_CURVE('',#38255,#38254,#5411,.T.);
#49036=EDGE_CURVE('',#38052,#38255,#21987,.T.);
#49037=EDGE_CURVE('',#38055,#38052,#31453,.T.);
#49038=EDGE_CURVE('',#38256,#38055,#21988,.T.);
#49039=EDGE_CURVE('',#38054,#38256,#31454,.T.);
#49040=EDGE_CURVE('',#38257,#38056,#31455,.T.);
#49041=EDGE_CURVE('',#38257,#38256,#5412,.T.);
#49042=EDGE_CURVE('',#38258,#38057,#31456,.T.);
#49043=EDGE_CURVE('',#38258,#38257,#31457,.T.);
#49044=EDGE_CURVE('',#38259,#38260,#31458,.T.);
#49045=EDGE_CURVE('',#38260,#38058,#31459,.T.);
#49046=EDGE_CURVE('',#38259,#38258,#5413,.T.);
#49047=EDGE_CURVE('',#38061,#38259,#21989,.T.);
#49048=EDGE_CURVE('',#38067,#38061,#31460,.T.);
#49049=EDGE_CURVE('',#38261,#38067,#21990,.T.);
#49050=EDGE_CURVE('',#38065,#38261,#31461,.T.);
#49051=EDGE_CURVE('',#38262,#38261,#5414,.T.);
#49052=EDGE_CURVE('',#38068,#38262,#31462,.T.);
#49053=EDGE_CURVE('',#35219,#38263,#31463,.T.);
#49054=EDGE_CURVE('',#35270,#38262,#31464,.T.);
#49055=EDGE_CURVE('',#38250,#38263,#21991,.T.);
#49056=EDGE_CURVE('',#38159,#38264,#21992,.T.);
#49057=EDGE_CURVE('',#38264,#38265,#21993,.T.);
#49058=EDGE_CURVE('',#38265,#38158,#21994,.T.);
#49059=EDGE_CURVE('',#38187,#38158,#31465,.T.);
#49060=EDGE_CURVE('',#38266,#38186,#21995,.T.);
#49061=EDGE_CURVE('',#38187,#38267,#21996,.T.);
#49062=EDGE_CURVE('',#38267,#38266,#21997,.T.);
#49063=EDGE_CURVE('',#38267,#38265,#31466,.T.);
#49064=EDGE_CURVE('',#38195,#38186,#31467,.T.);
#49065=EDGE_CURVE('',#38195,#38268,#21998,.T.);
#49066=EDGE_CURVE('',#38268,#38269,#21999,.T.);
#49067=EDGE_CURVE('',#38269,#38194,#22000,.T.);
#49068=EDGE_CURVE('',#38268,#38266,#31468,.T.);
#49069=EDGE_CURVE('',#38270,#38138,#31469,.T.);
#49070=EDGE_CURVE('',#38270,#38194,#5415,.T.);
#49071=EDGE_CURVE('',#38250,#38270,#31470,.T.);
#49072=EDGE_CURVE('',#38263,#38269,#31471,.T.);
#49073=EDGE_CURVE('',#38068,#35269,#31472,.T.);
#49074=EDGE_CURVE('',#38069,#35775,#31473,.T.);
#49075=EDGE_CURVE('',#35773,#38070,#31474,.T.);
#49076=EDGE_CURVE('',#35764,#38071,#31475,.T.);
#49077=EDGE_CURVE('',#38075,#35765,#31476,.F.);
#49078=EDGE_CURVE('',#35710,#38074,#31477,.T.);
#49079=EDGE_CURVE('',#38088,#35711,#31478,.T.);
#49080=EDGE_CURVE('',#35683,#38103,#31479,.T.);
#49081=EDGE_CURVE('',#38104,#35680,#31480,.T.);
#49082=EDGE_CURVE('',#35678,#38105,#31481,.T.);
#49083=EDGE_CURVE('',#38107,#35677,#31482,.T.);
#49084=EDGE_CURVE('',#38109,#35673,#22001,.T.);
#49085=EDGE_CURVE('',#35601,#38131,#22002,.T.);
#49086=EDGE_CURVE('',#35588,#38130,#31483,.T.);
#49087=EDGE_CURVE('',#38133,#35585,#31484,.T.);
#49088=EDGE_CURVE('',#35583,#38135,#31485,.T.);
#49089=EDGE_CURVE('',#38136,#35357,#31486,.T.);
#49090=EDGE_CURVE('',#38248,#35314,#31487,.T.);
#49091=EDGE_CURVE('',#38264,#38232,#31488,.T.);
#49092=EDGE_CURVE('',#38271,#38272,#22003,.T.);
#49093=EDGE_CURVE('',#38272,#38273,#1204,.T.);
#49094=EDGE_CURVE('',#38274,#38273,#22004,.T.);
#49095=EDGE_CURVE('',#38274,#38271,#1205,.T.);
#49096=EDGE_CURVE('',#38275,#38276,#22005,.T.);
#49097=EDGE_CURVE('',#38276,#38272,#1206,.T.);
#49098=EDGE_CURVE('',#38271,#38275,#1207,.T.);
#49099=EDGE_CURVE('',#38277,#38278,#22006,.T.);
#49100=EDGE_CURVE('',#38278,#38276,#1208,.T.);
#49101=EDGE_CURVE('',#38275,#38277,#1209,.T.);
#49102=EDGE_CURVE('',#38279,#38280,#22007,.T.);
#49103=EDGE_CURVE('',#38280,#38278,#1210,.T.);
#49104=EDGE_CURVE('',#38277,#38279,#1211,.T.);
#49105=EDGE_CURVE('',#38281,#38282,#22008,.T.);
#49106=EDGE_CURVE('',#38282,#38280,#1212,.T.);
#49107=EDGE_CURVE('',#38279,#38281,#1213,.T.);
#49108=EDGE_CURVE('',#38273,#38282,#1214,.T.);
#49109=EDGE_CURVE('',#38281,#38274,#1215,.T.);
#49110=EDGE_CURVE('',#38283,#38277,#22009,.T.);
#49111=EDGE_CURVE('',#38272,#38273,#31489,.T.);
#49112=EDGE_CURVE('',#38276,#38272,#31490,.T.);
#49113=EDGE_CURVE('',#38278,#38276,#31491,.T.);
#49114=EDGE_CURVE('',#38280,#38278,#31492,.T.);
#49115=EDGE_CURVE('',#38282,#38280,#31493,.T.);
#49116=EDGE_CURVE('',#38273,#38282,#31494,.T.);
#49117=EDGE_CURVE('',#38284,#38284,#31495,.T.);
#49118=EDGE_CURVE('',#38284,#38285,#31496,.T.);
#49119=EDGE_CURVE('',#38286,#38285,#31497,.T.);
#49120=EDGE_CURVE('',#38285,#38286,#31498,.T.);
#49121=EDGE_CURVE('',#38287,#38287,#31499,.T.);
#49122=EDGE_CURVE('',#38287,#38286,#22010,.T.);
#49123=EDGE_CURVE('',#38288,#38288,#31500,.T.);
#49124=EDGE_CURVE('',#38288,#38289,#22011,.T.);
#49125=EDGE_CURVE('',#38289,#38289,#31501,.T.);
#49126=EDGE_CURVE('',#38290,#38290,#31502,.T.);
#49127=EDGE_CURVE('',#38290,#38288,#22012,.T.);
#49128=EDGE_CURVE('',#38291,#38291,#31503,.T.);
#49129=EDGE_CURVE('',#38292,#38292,#31504,.T.);
#49130=EDGE_CURVE('',#38292,#38291,#22013,.T.);
#49131=EDGE_CURVE('',#38293,#38294,#31505,.T.);
#49132=EDGE_CURVE('',#38293,#38295,#5416,.T.);
#49133=EDGE_CURVE('',#38296,#38295,#31506,.T.);
#49134=EDGE_CURVE('',#38296,#38294,#1216,.T.);
#49135=EDGE_CURVE('',#38297,#38297,#31507,.T.);
#49136=EDGE_CURVE('',#38297,#38298,#31508,.T.);
#49137=EDGE_CURVE('',#38298,#38299,#31509,.T.);
#49138=EDGE_CURVE('',#38299,#38298,#31510,.T.);
#49139=EDGE_CURVE('',#38300,#38301,#31511,.T.);
#49140=EDGE_CURVE('',#38300,#38302,#5417,.T.);
#49141=EDGE_CURVE('',#38303,#38302,#31512,.T.);
#49142=EDGE_CURVE('',#38303,#38301,#5418,.T.);
#49143=EDGE_CURVE('',#38304,#38305,#31513,.T.);
#49144=EDGE_CURVE('',#38304,#38303,#5419,.T.);
#49145=EDGE_CURVE('',#38302,#38305,#5420,.T.);
#49146=EDGE_CURVE('',#38306,#38300,#31514,.T.);
#49147=EDGE_CURVE('',#38306,#38301,#31515,.T.);
#49148=EDGE_CURVE('',#38307,#38308,#31516,.T.);
#49149=EDGE_CURVE('',#38307,#38304,#5421,.T.);
#49150=EDGE_CURVE('',#38305,#38308,#5422,.T.);
#49151=EDGE_CURVE('',#38309,#38310,#31517,.T.);
#49152=EDGE_CURVE('',#38309,#38306,#31518,.T.);
#49153=EDGE_CURVE('',#38301,#38310,#31519,.T.);
#49154=EDGE_CURVE('',#38311,#38312,#31520,.T.);
#49155=EDGE_CURVE('',#38311,#38307,#5423,.T.);
#49156=EDGE_CURVE('',#38308,#38312,#5424,.T.);
#49157=EDGE_CURVE('',#38313,#38314,#31521,.T.);
#49158=EDGE_CURVE('',#38313,#38309,#31522,.T.);
#49159=EDGE_CURVE('',#38310,#38314,#31523,.T.);
#49160=EDGE_CURVE('',#38315,#38316,#31524,.T.);
#49161=EDGE_CURVE('',#38315,#38311,#5425,.T.);
#49162=EDGE_CURVE('',#38312,#38316,#5426,.T.);
#49163=EDGE_CURVE('',#38317,#38318,#31525,.T.);
#49164=EDGE_CURVE('',#38317,#38313,#31526,.T.);
#49165=EDGE_CURVE('',#38314,#38318,#31527,.T.);
#49166=EDGE_CURVE('',#38319,#38320,#31528,.T.);
#49167=EDGE_CURVE('',#38319,#38315,#5427,.T.);
#49168=EDGE_CURVE('',#38316,#38320,#5428,.T.);
#49169=EDGE_CURVE('',#38321,#38322,#31529,.T.);
#49170=EDGE_CURVE('',#38321,#38317,#5429,.T.);
#49171=EDGE_CURVE('',#38318,#38322,#5430,.T.);
#49172=EDGE_CURVE('',#38322,#38323,#31530,.T.);
#49173=EDGE_CURVE('',#38322,#38324,#1994,.T.);
#49174=EDGE_CURVE('',#38324,#38319,#5431,.T.);
#49175=EDGE_CURVE('',#38320,#38323,#5432,.T.);
#49176=EDGE_CURVE('',#38323,#38321,#31531,.T.);
#49177=EDGE_CURVE('',#38325,#38326,#31532,.T.);
#49178=EDGE_CURVE('',#38325,#38327,#5433,.T.);
#49179=EDGE_CURVE('',#38328,#38327,#31533,.T.);
#49180=EDGE_CURVE('',#38328,#38326,#5434,.T.);
#49181=EDGE_CURVE('',#38329,#38330,#31534,.T.);
#49182=EDGE_CURVE('',#38329,#38328,#5435,.T.);
#49183=EDGE_CURVE('',#38327,#38330,#5436,.T.);
#49184=EDGE_CURVE('',#38331,#38332,#31535,.T.);
#49185=EDGE_CURVE('',#38331,#38325,#5437,.T.);
#49186=EDGE_CURVE('',#38326,#38332,#5438,.T.);
#49187=EDGE_CURVE('',#38333,#38334,#31536,.T.);
#49188=EDGE_CURVE('',#38333,#38329,#5439,.T.);
#49189=EDGE_CURVE('',#38330,#38334,#5440,.T.);
#49190=EDGE_CURVE('',#38335,#38336,#31537,.T.);
#49191=EDGE_CURVE('',#38335,#38331,#5441,.T.);
#49192=EDGE_CURVE('',#38332,#38336,#5442,.T.);
#49193=EDGE_CURVE('',#38333,#38337,#31538,.T.);
#49194=EDGE_CURVE('',#38334,#38337,#31539,.T.);
#49195=EDGE_CURVE('',#38338,#38339,#31540,.T.);
#49196=EDGE_CURVE('',#38338,#38335,#5443,.T.);
#49197=EDGE_CURVE('',#38336,#38339,#5444,.T.);
#49198=EDGE_CURVE('',#38340,#38341,#31541,.T.);
#49199=EDGE_CURVE('',#38340,#38333,#5445,.T.);
#49200=EDGE_CURVE('',#38337,#38341,#5446,.T.);
#49201=EDGE_CURVE('',#38342,#38343,#31542,.T.);
#49202=EDGE_CURVE('',#38342,#38338,#5447,.T.);
#49203=EDGE_CURVE('',#38339,#38343,#5448,.T.);
#49204=EDGE_CURVE('',#38344,#38345,#31543,.T.);
#49205=EDGE_CURVE('',#38344,#38340,#31544,.T.);
#49206=EDGE_CURVE('',#38341,#38345,#31545,.T.);
#49207=EDGE_CURVE('',#38346,#38342,#31546,.T.);
#49208=EDGE_CURVE('',#38346,#38343,#31547,.T.);
#49209=EDGE_CURVE('',#38347,#38348,#31548,.T.);
#49210=EDGE_CURVE('',#38347,#38344,#31549,.T.);
#49211=EDGE_CURVE('',#38345,#38348,#31550,.T.);
#49212=EDGE_CURVE('',#38349,#38350,#31551,.T.);
#49213=EDGE_CURVE('',#38349,#38346,#5449,.T.);
#49214=EDGE_CURVE('',#38343,#38350,#5450,.T.);
#49215=EDGE_CURVE('',#38348,#38349,#31552,.T.);
#49216=EDGE_CURVE('',#38350,#38347,#31553,.T.);
#49217=EDGE_CURVE('',#38351,#38352,#31554,.T.);
#49218=EDGE_CURVE('',#38351,#38353,#31555,.T.);
#49219=EDGE_CURVE('',#38353,#38354,#31556,.T.);
#49220=EDGE_CURVE('',#38354,#38352,#31557,.T.);
#49221=EDGE_CURVE('',#38355,#38356,#31558,.T.);
#49222=EDGE_CURVE('',#38355,#38351,#31559,.T.);
#49223=EDGE_CURVE('',#38352,#38356,#31560,.T.);
#49224=EDGE_CURVE('',#38357,#38358,#31561,.T.);
#49225=EDGE_CURVE('',#38357,#38355,#31562,.T.);
#49226=EDGE_CURVE('',#38356,#38358,#31563,.T.);
#49227=EDGE_CURVE('',#38359,#38360,#31564,.T.);
#49228=EDGE_CURVE('',#38359,#38357,#31565,.T.);
#49229=EDGE_CURVE('',#38358,#38360,#31566,.T.);
#49230=EDGE_CURVE('',#38361,#38362,#31567,.T.);
#49231=EDGE_CURVE('',#38361,#38359,#31568,.T.);
#49232=EDGE_CURVE('',#38360,#38362,#31569,.T.);
#49233=EDGE_CURVE('',#38363,#38364,#31570,.T.);
#49234=EDGE_CURVE('',#38363,#38361,#31571,.T.);
#49235=EDGE_CURVE('',#38362,#38364,#31572,.T.);
#49236=EDGE_CURVE('',#38365,#38366,#31573,.T.);
#49237=EDGE_CURVE('',#38365,#38363,#31574,.T.);
#49238=EDGE_CURVE('',#38364,#38366,#31575,.T.);
#49239=EDGE_CURVE('',#38306,#38367,#31576,.T.);
#49240=EDGE_CURVE('',#38368,#38367,#31577,.T.);
#49241=EDGE_CURVE('',#38368,#38300,#31578,.T.);
#49242=EDGE_CURVE('',#38369,#38370,#31579,.T.);
#49243=EDGE_CURVE('',#38369,#38368,#1995,.T.);
#49244=EDGE_CURVE('',#38367,#38370,#5451,.T.);
#49245=EDGE_CURVE('',#38323,#38371,#5452,.T.);
#49246=EDGE_CURVE('',#38372,#38371,#31580,.T.);
#49247=EDGE_CURVE('',#38372,#38321,#5453,.T.);
#49248=EDGE_CURVE('',#38373,#38374,#31581,.T.);
#49249=EDGE_CURVE('',#38373,#38369,#5454,.T.);
#49250=EDGE_CURVE('',#38370,#38374,#5455,.T.);
#49251=EDGE_CURVE('',#38375,#38376,#31582,.T.);
#49252=EDGE_CURVE('',#38375,#38372,#31583,.T.);
#49253=EDGE_CURVE('',#38371,#38376,#31584,.T.);
#49254=EDGE_CURVE('',#38377,#38378,#31585,.T.);
#49255=EDGE_CURVE('',#38377,#38373,#31586,.T.);
#49256=EDGE_CURVE('',#38374,#38378,#31587,.T.);
#49257=EDGE_CURVE('',#38379,#38380,#31588,.T.);
#49258=EDGE_CURVE('',#38379,#38375,#5456,.T.);
#49259=EDGE_CURVE('',#38376,#38380,#5457,.T.);
#49260=EDGE_CURVE('',#38381,#38382,#31589,.T.);
#49261=EDGE_CURVE('',#38381,#38377,#5458,.T.);
#49262=EDGE_CURVE('',#38378,#38382,#5459,.T.);
#49263=EDGE_CURVE('',#38383,#38384,#31590,.T.);
#49264=EDGE_CURVE('',#38383,#38379,#5460,.T.);
#49265=EDGE_CURVE('',#38380,#38384,#5461,.T.);
#49266=EDGE_CURVE('',#38385,#38386,#31591,.T.);
#49267=EDGE_CURVE('',#38385,#38381,#5462,.T.);
#49268=EDGE_CURVE('',#38382,#38386,#5463,.T.);
#49269=EDGE_CURVE('',#38387,#38388,#31592,.T.);
#49270=EDGE_CURVE('',#38387,#38383,#5464,.T.);
#49271=EDGE_CURVE('',#38384,#38388,#5465,.T.);
#49272=EDGE_CURVE('',#38389,#38390,#31593,.T.);
#49273=EDGE_CURVE('',#38389,#38385,#5466,.T.);
#49274=EDGE_CURVE('',#38386,#38390,#5467,.T.);
#49275=EDGE_CURVE('',#38388,#38389,#31594,.T.);
#49276=EDGE_CURVE('',#38390,#38387,#31595,.T.);
#49277=EDGE_CURVE('',#38391,#38392,#31596,.T.);
#49278=EDGE_CURVE('',#38391,#38393,#5468,.T.);
#49279=EDGE_CURVE('',#38394,#38393,#31597,.T.);
#49280=EDGE_CURVE('',#38394,#38392,#5469,.T.);
#49281=EDGE_CURVE('',#38395,#38396,#31598,.T.);
#49282=EDGE_CURVE('',#38395,#38394,#31599,.T.);
#49283=EDGE_CURVE('',#38393,#38396,#31600,.T.);
#49284=EDGE_CURVE('',#38397,#38398,#31601,.T.);
#49285=EDGE_CURVE('',#38397,#38391,#5470,.T.);
#49286=EDGE_CURVE('',#38392,#38398,#5471,.T.);
#49287=EDGE_CURVE('',#38399,#38400,#31602,.T.);
#49288=EDGE_CURVE('',#38399,#38395,#5472,.T.);
#49289=EDGE_CURVE('',#38396,#38400,#5473,.T.);
#49290=EDGE_CURVE('',#38401,#38402,#31603,.T.);
#49291=EDGE_CURVE('',#38401,#38397,#5474,.T.);
#49292=EDGE_CURVE('',#38398,#38402,#5475,.T.);
#49293=EDGE_CURVE('',#38403,#38404,#31604,.T.);
#49294=EDGE_CURVE('',#38403,#38405,#5476,.T.);
#49295=EDGE_CURVE('',#38405,#38399,#5477,.T.);
#49296=EDGE_CURVE('',#38400,#38404,#5478,.T.);
#49297=EDGE_CURVE('',#38406,#38407,#31605,.T.);
#49298=EDGE_CURVE('',#38406,#38401,#31606,.T.);
#49299=EDGE_CURVE('',#38402,#38407,#31607,.T.);
#49300=EDGE_CURVE('',#38408,#38409,#31608,.T.);
#49301=EDGE_CURVE('',#38408,#38403,#5479,.T.);
#49302=EDGE_CURVE('',#38404,#38409,#5480,.T.);
#49303=EDGE_CURVE('',#38334,#38406,#5481,.T.);
#49304=EDGE_CURVE('',#38407,#38337,#5482,.T.);
#49305=EDGE_CURVE('',#38410,#38411,#31609,.T.);
#49306=EDGE_CURVE('',#38410,#38408,#31610,.T.);
#49307=EDGE_CURVE('',#38409,#38411,#31611,.T.);
#49308=EDGE_CURVE('',#38346,#38410,#5483,.T.);
#49309=EDGE_CURVE('',#38411,#38342,#5484,.T.);
#49310=EDGE_CURVE('',#38332,#38412,#22014,.T.);
#49311=EDGE_CURVE('',#38413,#38412,#31612,.T.);
#49312=EDGE_CURVE('',#38413,#38336,#22015,.T.);
#49313=EDGE_CURVE('',#38414,#38413,#31613,.T.);
#49314=EDGE_CURVE('',#38412,#38415,#31614,.T.);
#49315=EDGE_CURVE('',#38414,#38415,#31615,.T.);
#49316=EDGE_CURVE('',#38293,#38416,#31616,.T.);
#49317=EDGE_CURVE('',#38417,#38416,#31617,.T.);
#49318=EDGE_CURVE('',#38417,#38414,#31618,.T.);
#49319=EDGE_CURVE('',#38415,#38295,#31619,.T.);
#49320=EDGE_CURVE('',#38418,#38419,#31620,.T.);
#49321=EDGE_CURVE('',#38418,#38417,#31621,.T.);
#49322=EDGE_CURVE('',#38416,#38419,#31622,.T.);
#49323=EDGE_CURVE('',#38328,#38418,#22016,.T.);
#49324=EDGE_CURVE('',#38419,#38326,#22017,.T.);
#49325=EDGE_CURVE('',#38349,#38420,#22018,.T.);
#49326=EDGE_CURVE('',#38421,#38420,#31623,.T.);
#49327=EDGE_CURVE('',#38421,#38410,#22019,.T.);
#49328=EDGE_CURVE('',#38422,#38421,#31624,.T.);
#49329=EDGE_CURVE('',#38420,#38423,#31625,.T.);
#49330=EDGE_CURVE('',#38422,#38423,#31626,.T.);
#49331=EDGE_CURVE('',#38424,#38425,#31627,.T.);
#49332=EDGE_CURVE('',#38424,#38422,#31628,.T.);
#49333=EDGE_CURVE('',#38423,#38425,#31629,.T.);
#49334=EDGE_CURVE('',#38426,#38427,#31630,.T.);
#49335=EDGE_CURVE('',#38426,#38424,#31631,.T.);
#49336=EDGE_CURVE('',#38425,#38427,#31632,.T.);
#49337=EDGE_CURVE('',#38407,#38426,#22020,.T.);
#49338=EDGE_CURVE('',#38427,#38341,#22021,.T.);
#49339=EDGE_CURVE('',#38370,#38428,#22022,.T.);
#49340=EDGE_CURVE('',#38429,#38428,#31633,.T.);
#49341=EDGE_CURVE('',#38429,#38374,#22023,.T.);
#49342=EDGE_CURVE('',#38430,#38431,#31634,.T.);
#49343=EDGE_CURVE('',#38430,#38429,#31635,.T.);
#49344=EDGE_CURVE('',#38428,#38431,#31636,.T.);
#49345=EDGE_CURVE('',#38432,#38433,#31637,.T.);
#49346=EDGE_CURVE('',#38432,#38430,#31638,.T.);
#49347=EDGE_CURVE('',#38431,#38433,#31639,.T.);
#49348=EDGE_CURVE('',#38433,#38434,#31640,.T.);
#49349=EDGE_CURVE('',#38435,#38434,#31641,.T.);
#49350=EDGE_CURVE('',#38435,#38432,#31642,.T.);
#49351=EDGE_CURVE('',#38372,#38435,#22024,.T.);
#49352=EDGE_CURVE('',#38434,#38317,#22025,.T.);
#49353=EDGE_CURVE('',#38307,#38436,#22026,.T.);
#49354=EDGE_CURVE('',#38437,#38436,#31643,.T.);
#49355=EDGE_CURVE('',#38437,#38304,#22027,.T.);
#49356=EDGE_CURVE('',#38438,#38439,#31644,.T.);
#49357=EDGE_CURVE('',#38438,#38437,#31645,.T.);
#49358=EDGE_CURVE('',#38436,#38439,#31646,.T.);
#49359=EDGE_CURVE('',#38440,#38441,#31647,.T.);
#49360=EDGE_CURVE('',#38440,#38438,#31648,.T.);
#49361=EDGE_CURVE('',#38439,#38441,#31649,.T.);
#49362=EDGE_CURVE('',#38441,#38442,#31650,.T.);
#49363=EDGE_CURVE('',#38443,#38442,#31651,.T.);
#49364=EDGE_CURVE('',#38443,#38440,#31652,.T.);
#49365=EDGE_CURVE('',#38315,#38443,#22028,.T.);
#49366=EDGE_CURVE('',#38442,#38311,#22029,.T.);
#49367=EDGE_CURVE('',#38394,#38424,#22030,.T.);
#49368=EDGE_CURVE('',#38426,#38398,#22031,.T.);
#49369=EDGE_CURVE('',#38403,#38421,#22032,.T.);
#49370=EDGE_CURVE('',#38422,#38395,#22033,.T.);
#49371=EDGE_CURVE('',#38344,#38417,#22034,.T.);
#49372=EDGE_CURVE('',#38418,#38329,#22035,.T.);
#49373=EDGE_CURVE('',#38339,#38413,#22036,.T.);
#49374=EDGE_CURVE('',#38414,#38347,#22037,.T.);
#49375=EDGE_CURVE('',#38303,#38437,#22038,.T.);
#49376=EDGE_CURVE('',#38438,#38310,#22039,.T.);
#49377=EDGE_CURVE('',#38443,#38319,#22040,.T.);
#49378=EDGE_CURVE('',#38314,#38440,#22041,.T.);
#49379=EDGE_CURVE('',#38387,#38432,#22042,.T.);
#49380=EDGE_CURVE('',#38435,#38379,#22043,.T.);
#49381=EDGE_CURVE('',#38382,#38429,#22044,.T.);
#49382=EDGE_CURVE('',#38430,#38390,#22045,.T.);
#49383=EDGE_CURVE('',#38444,#38445,#31653,.T.);
#49384=EDGE_CURVE('',#38446,#38445,#31654,.T.);
#49385=EDGE_CURVE('',#38446,#38447,#31655,.T.);
#49386=EDGE_CURVE('',#38444,#38447,#31656,.T.);
#49387=EDGE_CURVE('',#38448,#38449,#31657,.T.);
#49388=EDGE_CURVE('',#38448,#38446,#22046,.T.);
#49389=EDGE_CURVE('',#38445,#38449,#22047,.T.);
#49390=EDGE_CURVE('',#38450,#38451,#31658,.T.);
#49391=EDGE_CURVE('',#38450,#38444,#31659,.T.);
#49392=EDGE_CURVE('',#38447,#38451,#31660,.T.);
#49393=EDGE_CURVE('',#38452,#38453,#31661,.T.);
#49394=EDGE_CURVE('',#38452,#38448,#31662,.T.);
#49395=EDGE_CURVE('',#38449,#38453,#31663,.T.);
#49396=EDGE_CURVE('',#38454,#38455,#31664,.T.);
#49397=EDGE_CURVE('',#38454,#38450,#31665,.T.);
#49398=EDGE_CURVE('',#38451,#38455,#31666,.T.);
#49399=EDGE_CURVE('',#38456,#38457,#31667,.T.);
#49400=EDGE_CURVE('',#38456,#38452,#22048,.T.);
#49401=EDGE_CURVE('',#38453,#38457,#22049,.T.);
#49402=EDGE_CURVE('',#38458,#38459,#31668,.T.);
#49403=EDGE_CURVE('',#38458,#38454,#31669,.T.);
#49404=EDGE_CURVE('',#38455,#38459,#31670,.T.);
#49405=EDGE_CURVE('',#38460,#38461,#31671,.T.);
#49406=EDGE_CURVE('',#38460,#38456,#31672,.T.);
#49407=EDGE_CURVE('',#38457,#38461,#31673,.T.);
#49408=EDGE_CURVE('',#38462,#38463,#31674,.T.);
#49409=EDGE_CURVE('',#38462,#38458,#31675,.T.);
#49410=EDGE_CURVE('',#38459,#38463,#31676,.T.);
#49411=EDGE_CURVE('',#38461,#38462,#22050,.T.);
#49412=EDGE_CURVE('',#38463,#38460,#22051,.T.);
#49413=EDGE_CURVE('',#38464,#38465,#31677,.T.);
#49414=EDGE_CURVE('',#38466,#38465,#31678,.T.);
#49415=EDGE_CURVE('',#38466,#38467,#31679,.T.);
#49416=EDGE_CURVE('',#38464,#38467,#31680,.T.);
#49417=EDGE_CURVE('',#38468,#38469,#31681,.T.);
#49418=EDGE_CURVE('',#38468,#38466,#22052,.T.);
#49419=EDGE_CURVE('',#38465,#38469,#22053,.T.);
#49420=EDGE_CURVE('',#38470,#38471,#31682,.T.);
#49421=EDGE_CURVE('',#38470,#38464,#31683,.T.);
#49422=EDGE_CURVE('',#38467,#38471,#31684,.T.);
#49423=EDGE_CURVE('',#38472,#38473,#31685,.T.);
#49424=EDGE_CURVE('',#38472,#38468,#31686,.T.);
#49425=EDGE_CURVE('',#38469,#38473,#31687,.T.);
#49426=EDGE_CURVE('',#38474,#38475,#31688,.T.);
#49427=EDGE_CURVE('',#38474,#38470,#31689,.T.);
#49428=EDGE_CURVE('',#38471,#38475,#31690,.T.);
#49429=EDGE_CURVE('',#38476,#38477,#31691,.T.);
#49430=EDGE_CURVE('',#38476,#38472,#22054,.T.);
#49431=EDGE_CURVE('',#38473,#38477,#22055,.T.);
#49432=EDGE_CURVE('',#38478,#38479,#31692,.T.);
#49433=EDGE_CURVE('',#38478,#38474,#22056,.T.);
#49434=EDGE_CURVE('',#38475,#38479,#22057,.T.);
#49435=EDGE_CURVE('',#38477,#38478,#31693,.T.);
#49436=EDGE_CURVE('',#38479,#38476,#31694,.T.);
#49437=EDGE_CURVE('',#38480,#38481,#31695,.T.);
#49438=EDGE_CURVE('',#38482,#38481,#31696,.T.);
#49439=EDGE_CURVE('',#38482,#38483,#31697,.T.);
#49440=EDGE_CURVE('',#38480,#38483,#31698,.T.);
#49441=EDGE_CURVE('',#38484,#38485,#31699,.T.);
#49442=EDGE_CURVE('',#38484,#38482,#22058,.T.);
#49443=EDGE_CURVE('',#38481,#38485,#22059,.T.);
#49444=EDGE_CURVE('',#38486,#38487,#31700,.T.);
#49445=EDGE_CURVE('',#38486,#38480,#31701,.T.);
#49446=EDGE_CURVE('',#38483,#38487,#31702,.T.);
#49447=EDGE_CURVE('',#38488,#38489,#31703,.T.);
#49448=EDGE_CURVE('',#38488,#38484,#31704,.T.);
#49449=EDGE_CURVE('',#38485,#38489,#31705,.T.);
#49450=EDGE_CURVE('',#38490,#38491,#31706,.T.);
#49451=EDGE_CURVE('',#38490,#38486,#31707,.T.);
#49452=EDGE_CURVE('',#38487,#38491,#31708,.T.);
#49453=EDGE_CURVE('',#38492,#38493,#31709,.T.);
#49454=EDGE_CURVE('',#38492,#38488,#22060,.T.);
#49455=EDGE_CURVE('',#38489,#38493,#22061,.T.);
#49456=EDGE_CURVE('',#38494,#38495,#31710,.T.);
#49457=EDGE_CURVE('',#38494,#38490,#22062,.T.);
#49458=EDGE_CURVE('',#38491,#38495,#22063,.T.);
#49459=EDGE_CURVE('',#38493,#38494,#31711,.T.);
#49460=EDGE_CURVE('',#38495,#38492,#31712,.T.);
#49461=EDGE_CURVE('',#38496,#38497,#31713,.T.);
#49462=EDGE_CURVE('',#38496,#38498,#31714,.T.);
#49463=EDGE_CURVE('',#38499,#38498,#31715,.T.);
#49464=EDGE_CURVE('',#38499,#38497,#31716,.T.);
#49465=EDGE_CURVE('',#38500,#38501,#31717,.T.);
#49466=EDGE_CURVE('',#38500,#38499,#22064,.T.);
#49467=EDGE_CURVE('',#38498,#38501,#22065,.T.);
#49468=EDGE_CURVE('',#38502,#38503,#31718,.T.);
#49469=EDGE_CURVE('',#38502,#38496,#22066,.T.);
#49470=EDGE_CURVE('',#38497,#38503,#22067,.T.);
#49471=EDGE_CURVE('',#38504,#38505,#31719,.T.);
#49472=EDGE_CURVE('',#38504,#38500,#31720,.T.);
#49473=EDGE_CURVE('',#38501,#38505,#31721,.T.);
#49474=EDGE_CURVE('',#38506,#38507,#31722,.T.);
#49475=EDGE_CURVE('',#38506,#38502,#31723,.T.);
#49476=EDGE_CURVE('',#38503,#38507,#31724,.T.);
#49477=EDGE_CURVE('',#38508,#38509,#31725,.T.);
#49478=EDGE_CURVE('',#38508,#38504,#22068,.T.);
#49479=EDGE_CURVE('',#38505,#38509,#22069,.T.);
#49480=EDGE_CURVE('',#38510,#38511,#31726,.T.);
#49481=EDGE_CURVE('',#38510,#38506,#22070,.T.);
#49482=EDGE_CURVE('',#38507,#38511,#22071,.T.);
#49483=EDGE_CURVE('',#38509,#38510,#31727,.T.);
#49484=EDGE_CURVE('',#38511,#38508,#31728,.T.);
#49485=EDGE_CURVE('',#38512,#38513,#31729,.T.);
#49486=EDGE_CURVE('',#38512,#38514,#31730,.T.);
#49487=EDGE_CURVE('',#38515,#38514,#31731,.T.);
#49488=EDGE_CURVE('',#38515,#38513,#31732,.T.);
#49489=EDGE_CURVE('',#38516,#38517,#31733,.T.);
#49490=EDGE_CURVE('',#38516,#38515,#22072,.T.);
#49491=EDGE_CURVE('',#38514,#38517,#22073,.T.);
#49492=EDGE_CURVE('',#38518,#38519,#31734,.T.);
#49493=EDGE_CURVE('',#38518,#38512,#22074,.T.);
#49494=EDGE_CURVE('',#38513,#38519,#22075,.T.);
#49495=EDGE_CURVE('',#38520,#38521,#31735,.T.);
#49496=EDGE_CURVE('',#38520,#38516,#31736,.T.);
#49497=EDGE_CURVE('',#38517,#38521,#31737,.T.);
#49498=EDGE_CURVE('',#38522,#38523,#31738,.T.);
#49499=EDGE_CURVE('',#38522,#38518,#31739,.T.);
#49500=EDGE_CURVE('',#38519,#38523,#31740,.T.);
#49501=EDGE_CURVE('',#38524,#38525,#31741,.T.);
#49502=EDGE_CURVE('',#38524,#38520,#31742,.T.);
#49503=EDGE_CURVE('',#38521,#38525,#31743,.T.);
#49504=EDGE_CURVE('',#38526,#38527,#31744,.T.);
#49505=EDGE_CURVE('',#38526,#38522,#22076,.T.);
#49506=EDGE_CURVE('',#38523,#38527,#22077,.T.);
#49507=EDGE_CURVE('',#38528,#38529,#31745,.T.);
#49508=EDGE_CURVE('',#38528,#38524,#31746,.T.);
#49509=EDGE_CURVE('',#38525,#38529,#31747,.T.);
#49510=EDGE_CURVE('',#38527,#38528,#31748,.T.);
#49511=EDGE_CURVE('',#38529,#38526,#31749,.T.);
#49512=EDGE_CURVE('',#38530,#38531,#31750,.T.);
#49513=EDGE_CURVE('',#38530,#38532,#31751,.T.);
#49514=EDGE_CURVE('',#38533,#38532,#31752,.T.);
#49515=EDGE_CURVE('',#38533,#38531,#31753,.T.);
#49516=EDGE_CURVE('',#38534,#38535,#31754,.T.);
#49517=EDGE_CURVE('',#38534,#38533,#22078,.T.);
#49518=EDGE_CURVE('',#38532,#38535,#22079,.T.);
#49519=EDGE_CURVE('',#38536,#38537,#31755,.T.);
#49520=EDGE_CURVE('',#38536,#38530,#22080,.T.);
#49521=EDGE_CURVE('',#38531,#38537,#22081,.T.);
#49522=EDGE_CURVE('',#38538,#38539,#31756,.T.);
#49523=EDGE_CURVE('',#38538,#38534,#31757,.T.);
#49524=EDGE_CURVE('',#38535,#38539,#31758,.T.);
#49525=EDGE_CURVE('',#38540,#38541,#31759,.T.);
#49526=EDGE_CURVE('',#38540,#38536,#31760,.T.);
#49527=EDGE_CURVE('',#38537,#38541,#31761,.T.);
#49528=EDGE_CURVE('',#38542,#38543,#31762,.T.);
#49529=EDGE_CURVE('',#38542,#38538,#22082,.T.);
#49530=EDGE_CURVE('',#38539,#38543,#22083,.T.);
#49531=EDGE_CURVE('',#38544,#38545,#31763,.T.);
#49532=EDGE_CURVE('',#38544,#38540,#22084,.T.);
#49533=EDGE_CURVE('',#38541,#38545,#22085,.T.);
#49534=EDGE_CURVE('',#38543,#38544,#31764,.T.);
#49535=EDGE_CURVE('',#38545,#38542,#31765,.T.);
#49536=EDGE_CURVE('',#38546,#38547,#31766,.T.);
#49537=EDGE_CURVE('',#38546,#38548,#31767,.T.);
#49538=EDGE_CURVE('',#38549,#38548,#31768,.T.);
#49539=EDGE_CURVE('',#38549,#38547,#31769,.T.);
#49540=EDGE_CURVE('',#38550,#38551,#31770,.T.);
#49541=EDGE_CURVE('',#38550,#38549,#22086,.T.);
#49542=EDGE_CURVE('',#38548,#38551,#22087,.T.);
#49543=EDGE_CURVE('',#38552,#38553,#31771,.T.);
#49544=EDGE_CURVE('',#38552,#38546,#22088,.T.);
#49545=EDGE_CURVE('',#38547,#38553,#22089,.T.);
#49546=EDGE_CURVE('',#38554,#38555,#31772,.T.);
#49547=EDGE_CURVE('',#38554,#38550,#31773,.T.);
#49548=EDGE_CURVE('',#38551,#38555,#31774,.T.);
#49549=EDGE_CURVE('',#38556,#38557,#31775,.T.);
#49550=EDGE_CURVE('',#38556,#38552,#31776,.T.);
#49551=EDGE_CURVE('',#38553,#38557,#31777,.T.);
#49552=EDGE_CURVE('',#38558,#38559,#31778,.T.);
#49553=EDGE_CURVE('',#38558,#38554,#22090,.T.);
#49554=EDGE_CURVE('',#38555,#38559,#22091,.T.);
#49555=EDGE_CURVE('',#38560,#38561,#31779,.T.);
#49556=EDGE_CURVE('',#38560,#38556,#22092,.T.);
#49557=EDGE_CURVE('',#38557,#38561,#22093,.T.);
#49558=EDGE_CURVE('',#38559,#38560,#31780,.T.);
#49559=EDGE_CURVE('',#38561,#38558,#31781,.T.);
#49560=EDGE_CURVE('',#38562,#38563,#31782,.T.);
#49561=EDGE_CURVE('',#38562,#38564,#31783,.T.);
#49562=EDGE_CURVE('',#38565,#38564,#31784,.T.);
#49563=EDGE_CURVE('',#38565,#38563,#31785,.T.);
#49564=EDGE_CURVE('',#38566,#38567,#31786,.T.);
#49565=EDGE_CURVE('',#38566,#38565,#22094,.T.);
#49566=EDGE_CURVE('',#38564,#38567,#22095,.T.);
#49567=EDGE_CURVE('',#38568,#38569,#31787,.T.);
#49568=EDGE_CURVE('',#38568,#38562,#22096,.T.);
#49569=EDGE_CURVE('',#38563,#38569,#22097,.T.);
#49570=EDGE_CURVE('',#38570,#38571,#31788,.T.);
#49571=EDGE_CURVE('',#38570,#38566,#31789,.T.);
#49572=EDGE_CURVE('',#38567,#38571,#31790,.T.);
#49573=EDGE_CURVE('',#38572,#38573,#31791,.T.);
#49574=EDGE_CURVE('',#38572,#38568,#31792,.T.);
#49575=EDGE_CURVE('',#38569,#38573,#31793,.T.);
#49576=EDGE_CURVE('',#38574,#38575,#31794,.T.);
#49577=EDGE_CURVE('',#38574,#38570,#22098,.T.);
#49578=EDGE_CURVE('',#38571,#38575,#22099,.T.);
#49579=EDGE_CURVE('',#38576,#38577,#31795,.T.);
#49580=EDGE_CURVE('',#38576,#38572,#22100,.T.);
#49581=EDGE_CURVE('',#38573,#38577,#22101,.T.);
#49582=EDGE_CURVE('',#38575,#38576,#31796,.T.);
#49583=EDGE_CURVE('',#38577,#38574,#31797,.T.);
#49584=EDGE_CURVE('',#38578,#38579,#31798,.T.);
#49585=EDGE_CURVE('',#38578,#38580,#31799,.T.);
#49586=EDGE_CURVE('',#38581,#38580,#31800,.T.);
#49587=EDGE_CURVE('',#38581,#38579,#31801,.T.);
#49588=EDGE_CURVE('',#38582,#38583,#31802,.T.);
#49589=EDGE_CURVE('',#38582,#38581,#22102,.T.);
#49590=EDGE_CURVE('',#38580,#38583,#22103,.T.);
#49591=EDGE_CURVE('',#38584,#38585,#31803,.T.);
#49592=EDGE_CURVE('',#38584,#38578,#22104,.T.);
#49593=EDGE_CURVE('',#38579,#38585,#22105,.T.);
#49594=EDGE_CURVE('',#38586,#38587,#31804,.T.);
#49595=EDGE_CURVE('',#38586,#38582,#31805,.T.);
#49596=EDGE_CURVE('',#38583,#38587,#31806,.T.);
#49597=EDGE_CURVE('',#38588,#38589,#31807,.T.);
#49598=EDGE_CURVE('',#38588,#38584,#31808,.T.);
#49599=EDGE_CURVE('',#38585,#38589,#31809,.T.);
#49600=EDGE_CURVE('',#38590,#38591,#31810,.T.);
#49601=EDGE_CURVE('',#38590,#38586,#22106,.T.);
#49602=EDGE_CURVE('',#38587,#38591,#22107,.T.);
#49603=EDGE_CURVE('',#38592,#38593,#31811,.T.);
#49604=EDGE_CURVE('',#38592,#38588,#22108,.T.);
#49605=EDGE_CURVE('',#38589,#38593,#22109,.T.);
#49606=EDGE_CURVE('',#38591,#38592,#31812,.T.);
#49607=EDGE_CURVE('',#38593,#38590,#31813,.T.);
#49608=EDGE_CURVE('',#38594,#38595,#31814,.T.);
#49609=EDGE_CURVE('',#38594,#38596,#31815,.T.);
#49610=EDGE_CURVE('',#38597,#38596,#31816,.T.);
#49611=EDGE_CURVE('',#38597,#38595,#31817,.T.);
#49612=EDGE_CURVE('',#38598,#38599,#31818,.T.);
#49613=EDGE_CURVE('',#38598,#38597,#22110,.T.);
#49614=EDGE_CURVE('',#38596,#38599,#22111,.T.);
#49615=EDGE_CURVE('',#38600,#38601,#31819,.T.);
#49616=EDGE_CURVE('',#38600,#38594,#22112,.T.);
#49617=EDGE_CURVE('',#38595,#38601,#22113,.T.);
#49618=EDGE_CURVE('',#38602,#38603,#31820,.T.);
#49619=EDGE_CURVE('',#38602,#38598,#31821,.T.);
#49620=EDGE_CURVE('',#38599,#38603,#31822,.T.);
#49621=EDGE_CURVE('',#38604,#38605,#31823,.T.);
#49622=EDGE_CURVE('',#38604,#38600,#31824,.T.);
#49623=EDGE_CURVE('',#38601,#38605,#31825,.T.);
#49624=EDGE_CURVE('',#38606,#38607,#31826,.T.);
#49625=EDGE_CURVE('',#38606,#38602,#22114,.T.);
#49626=EDGE_CURVE('',#38603,#38607,#22115,.T.);
#49627=EDGE_CURVE('',#38608,#38609,#31827,.T.);
#49628=EDGE_CURVE('',#38608,#38604,#31828,.T.);
#49629=EDGE_CURVE('',#38605,#38609,#31829,.T.);
#49630=EDGE_CURVE('',#38607,#38608,#31830,.T.);
#49631=EDGE_CURVE('',#38609,#38606,#31831,.T.);
#49632=EDGE_CURVE('',#38610,#38611,#31832,.T.);
#49633=EDGE_CURVE('',#38610,#38612,#31833,.T.);
#49634=EDGE_CURVE('',#38613,#38612,#31834,.T.);
#49635=EDGE_CURVE('',#38613,#38611,#31835,.T.);
#49636=EDGE_CURVE('',#38614,#38615,#31836,.T.);
#49637=EDGE_CURVE('',#38614,#38613,#22116,.T.);
#49638=EDGE_CURVE('',#38612,#38615,#22117,.T.);
#49639=EDGE_CURVE('',#38616,#38617,#31837,.T.);
#49640=EDGE_CURVE('',#38616,#38610,#22118,.T.);
#49641=EDGE_CURVE('',#38611,#38617,#22119,.T.);
#49642=EDGE_CURVE('',#38618,#38619,#31838,.T.);
#49643=EDGE_CURVE('',#38618,#38614,#31839,.T.);
#49644=EDGE_CURVE('',#38615,#38619,#31840,.T.);
#49645=EDGE_CURVE('',#38620,#38621,#31841,.T.);
#49646=EDGE_CURVE('',#38620,#38616,#31842,.T.);
#49647=EDGE_CURVE('',#38617,#38621,#31843,.T.);
#49648=EDGE_CURVE('',#38622,#38623,#31844,.T.);
#49649=EDGE_CURVE('',#38622,#38618,#22120,.T.);
#49650=EDGE_CURVE('',#38619,#38623,#22121,.T.);
#49651=EDGE_CURVE('',#38624,#38625,#31845,.T.);
#49652=EDGE_CURVE('',#38624,#38620,#31846,.T.);
#49653=EDGE_CURVE('',#38621,#38625,#31847,.T.);
#49654=EDGE_CURVE('',#38626,#38627,#31848,.T.);
#49655=EDGE_CURVE('',#38626,#38622,#31849,.T.);
#49656=EDGE_CURVE('',#38623,#38627,#31850,.T.);
#49657=EDGE_CURVE('',#38628,#38629,#31851,.T.);
#49658=EDGE_CURVE('',#38628,#38624,#31852,.T.);
#49659=EDGE_CURVE('',#38625,#38629,#31853,.T.);
#49660=EDGE_CURVE('',#38627,#38628,#31854,.T.);
#49661=EDGE_CURVE('',#38629,#38626,#31855,.T.);
#49662=EDGE_CURVE('',#38630,#38631,#31856,.T.);
#49663=EDGE_CURVE('',#38630,#38632,#31857,.T.);
#49664=EDGE_CURVE('',#38633,#38632,#31858,.T.);
#49665=EDGE_CURVE('',#38633,#38631,#31859,.T.);
#49666=EDGE_CURVE('',#38634,#38635,#31860,.T.);
#49667=EDGE_CURVE('',#38634,#38633,#22122,.T.);
#49668=EDGE_CURVE('',#38632,#38635,#22123,.T.);
#49669=EDGE_CURVE('',#38636,#38637,#31861,.T.);
#49670=EDGE_CURVE('',#38636,#38630,#22124,.T.);
#49671=EDGE_CURVE('',#38631,#38637,#22125,.T.);
#49672=EDGE_CURVE('',#38638,#38639,#31862,.T.);
#49673=EDGE_CURVE('',#38638,#38634,#31863,.T.);
#49674=EDGE_CURVE('',#38635,#38639,#31864,.T.);
#49675=EDGE_CURVE('',#38640,#38641,#31865,.T.);
#49676=EDGE_CURVE('',#38640,#38636,#31866,.T.);
#49677=EDGE_CURVE('',#38637,#38641,#31867,.T.);
#49678=EDGE_CURVE('',#38642,#38643,#31868,.T.);
#49679=EDGE_CURVE('',#38642,#38638,#22126,.T.);
#49680=EDGE_CURVE('',#38639,#38643,#22127,.T.);
#49681=EDGE_CURVE('',#38644,#38645,#31869,.T.);
#49682=EDGE_CURVE('',#38644,#38640,#31870,.T.);
#49683=EDGE_CURVE('',#38641,#38645,#31871,.T.);
#49684=EDGE_CURVE('',#38643,#38644,#31872,.T.);
#49685=EDGE_CURVE('',#38645,#38642,#31873,.T.);
#49686=EDGE_CURVE('',#38646,#38647,#31874,.T.);
#49687=EDGE_CURVE('',#38646,#38648,#31875,.T.);
#49688=EDGE_CURVE('',#38649,#38648,#31876,.T.);
#49689=EDGE_CURVE('',#38649,#38647,#31877,.T.);
#49690=EDGE_CURVE('',#38650,#38651,#31878,.T.);
#49691=EDGE_CURVE('',#38650,#38649,#22128,.T.);
#49692=EDGE_CURVE('',#38648,#38651,#22129,.T.);
#49693=EDGE_CURVE('',#38652,#38653,#31879,.T.);
#49694=EDGE_CURVE('',#38652,#38646,#22130,.T.);
#49695=EDGE_CURVE('',#38647,#38653,#22131,.T.);
#49696=EDGE_CURVE('',#38654,#38655,#31880,.T.);
#49697=EDGE_CURVE('',#38654,#38650,#31881,.T.);
#49698=EDGE_CURVE('',#38651,#38655,#31882,.T.);
#49699=EDGE_CURVE('',#38656,#38657,#31883,.T.);
#49700=EDGE_CURVE('',#38656,#38652,#31884,.T.);
#49701=EDGE_CURVE('',#38653,#38657,#31885,.T.);
#49702=EDGE_CURVE('',#38658,#38659,#31886,.T.);
#49703=EDGE_CURVE('',#38658,#38654,#22132,.T.);
#49704=EDGE_CURVE('',#38655,#38659,#22133,.T.);
#49705=EDGE_CURVE('',#38660,#38661,#31887,.T.);
#49706=EDGE_CURVE('',#38660,#38656,#22134,.T.);
#49707=EDGE_CURVE('',#38657,#38661,#22135,.T.);
#49708=EDGE_CURVE('',#38659,#38660,#31888,.T.);
#49709=EDGE_CURVE('',#38661,#38658,#31889,.T.);
#49710=EDGE_CURVE('',#38662,#38663,#31890,.T.);
#49711=EDGE_CURVE('',#38662,#38664,#31891,.T.);
#49712=EDGE_CURVE('',#38665,#38664,#31892,.T.);
#49713=EDGE_CURVE('',#38665,#38663,#31893,.T.);
#49714=EDGE_CURVE('',#38666,#38667,#31894,.T.);
#49715=EDGE_CURVE('',#38666,#38665,#22136,.T.);
#49716=EDGE_CURVE('',#38664,#38667,#22137,.T.);
#49717=EDGE_CURVE('',#38668,#38669,#31895,.T.);
#49718=EDGE_CURVE('',#38668,#38662,#31896,.T.);
#49719=EDGE_CURVE('',#38663,#38669,#31897,.T.);
#49720=EDGE_CURVE('',#38670,#38671,#31898,.T.);
#49721=EDGE_CURVE('',#38670,#38666,#31899,.T.);
#49722=EDGE_CURVE('',#38667,#38671,#31900,.T.);
#49723=EDGE_CURVE('',#38672,#38673,#31901,.T.);
#49724=EDGE_CURVE('',#38672,#38668,#31902,.T.);
#49725=EDGE_CURVE('',#38669,#38673,#31903,.T.);
#49726=EDGE_CURVE('',#38674,#38675,#31904,.T.);
#49727=EDGE_CURVE('',#38674,#38670,#22138,.T.);
#49728=EDGE_CURVE('',#38671,#38675,#22139,.T.);
#49729=EDGE_CURVE('',#38676,#38677,#31905,.T.);
#49730=EDGE_CURVE('',#38676,#38672,#22140,.T.);
#49731=EDGE_CURVE('',#38673,#38677,#22141,.T.);
#49732=EDGE_CURVE('',#38678,#38679,#31906,.T.);
#49733=EDGE_CURVE('',#38678,#38674,#31907,.T.);
#49734=EDGE_CURVE('',#38675,#38679,#31908,.T.);
#49735=EDGE_CURVE('',#38680,#38681,#31909,.T.);
#49736=EDGE_CURVE('',#38680,#38676,#31910,.T.);
#49737=EDGE_CURVE('',#38677,#38681,#31911,.T.);
#49738=EDGE_CURVE('',#38679,#38680,#22142,.T.);
#49739=EDGE_CURVE('',#38681,#38678,#22143,.T.);
#49740=EDGE_CURVE('',#38682,#38683,#31912,.T.);
#49741=EDGE_CURVE('',#38682,#38684,#31913,.T.);
#49742=EDGE_CURVE('',#38685,#38684,#31914,.T.);
#49743=EDGE_CURVE('',#38685,#38683,#31915,.T.);
#49744=EDGE_CURVE('',#38686,#38687,#31916,.T.);
#49745=EDGE_CURVE('',#38686,#38685,#22144,.T.);
#49746=EDGE_CURVE('',#38684,#38687,#22145,.T.);
#49747=EDGE_CURVE('',#38688,#38689,#31917,.T.);
#49748=EDGE_CURVE('',#38688,#38682,#22146,.T.);
#49749=EDGE_CURVE('',#38683,#38689,#22147,.T.);
#49750=EDGE_CURVE('',#38690,#38691,#31918,.T.);
#49751=EDGE_CURVE('',#38690,#38686,#31919,.T.);
#49752=EDGE_CURVE('',#38687,#38691,#31920,.T.);
#49753=EDGE_CURVE('',#38692,#38693,#31921,.T.);
#49754=EDGE_CURVE('',#38692,#38688,#31922,.T.);
#49755=EDGE_CURVE('',#38689,#38693,#31923,.T.);
#49756=EDGE_CURVE('',#38694,#38695,#31924,.T.);
#49757=EDGE_CURVE('',#38694,#38690,#22148,.T.);
#49758=EDGE_CURVE('',#38691,#38695,#22149,.T.);
#49759=EDGE_CURVE('',#38696,#38697,#31925,.T.);
#49760=EDGE_CURVE('',#38696,#38692,#31926,.T.);
#49761=EDGE_CURVE('',#38693,#38697,#31927,.T.);
#49762=EDGE_CURVE('',#38698,#38699,#31928,.T.);
#49763=EDGE_CURVE('',#38698,#38694,#31929,.T.);
#49764=EDGE_CURVE('',#38695,#38699,#31930,.T.);
#49765=EDGE_CURVE('',#38700,#38701,#31931,.T.);
#49766=EDGE_CURVE('',#38700,#38696,#31932,.T.);
#49767=EDGE_CURVE('',#38697,#38701,#31933,.T.);
#49768=EDGE_CURVE('',#38699,#38700,#22150,.T.);
#49769=EDGE_CURVE('',#38701,#38698,#22151,.T.);
#49770=EDGE_CURVE('',#38702,#38703,#31934,.T.);
#49771=EDGE_CURVE('',#38702,#38704,#31935,.T.);
#49772=EDGE_CURVE('',#38705,#38704,#31936,.T.);
#49773=EDGE_CURVE('',#38705,#38703,#31937,.T.);
#49774=EDGE_CURVE('',#38706,#38707,#31938,.T.);
#49775=EDGE_CURVE('',#38706,#38705,#22152,.T.);
#49776=EDGE_CURVE('',#38704,#38707,#22153,.T.);
#49777=EDGE_CURVE('',#38708,#38709,#31939,.T.);
#49778=EDGE_CURVE('',#38708,#38702,#22154,.T.);
#49779=EDGE_CURVE('',#38703,#38709,#22155,.T.);
#49780=EDGE_CURVE('',#38710,#38711,#31940,.T.);
#49781=EDGE_CURVE('',#38710,#38706,#31941,.T.);
#49782=EDGE_CURVE('',#38707,#38711,#31942,.T.);
#49783=EDGE_CURVE('',#38712,#38713,#31943,.T.);
#49784=EDGE_CURVE('',#38712,#38708,#31944,.T.);
#49785=EDGE_CURVE('',#38709,#38713,#31945,.T.);
#49786=EDGE_CURVE('',#38714,#38715,#31946,.T.);
#49787=EDGE_CURVE('',#38714,#38710,#22156,.T.);
#49788=EDGE_CURVE('',#38711,#38715,#22157,.T.);
#49789=EDGE_CURVE('',#38716,#38717,#31947,.T.);
#49790=EDGE_CURVE('',#38716,#38712,#22158,.T.);
#49791=EDGE_CURVE('',#38713,#38717,#22159,.T.);
#49792=EDGE_CURVE('',#38715,#38716,#31948,.T.);
#49793=EDGE_CURVE('',#38717,#38714,#31949,.T.);
#49794=EDGE_CURVE('',#38718,#38719,#31950,.T.);
#49795=EDGE_CURVE('',#38718,#38720,#31951,.T.);
#49796=EDGE_CURVE('',#38721,#38720,#31952,.T.);
#49797=EDGE_CURVE('',#38721,#38719,#31953,.T.);
#49798=EDGE_CURVE('',#38722,#38723,#31954,.T.);
#49799=EDGE_CURVE('',#38722,#38721,#22160,.T.);
#49800=EDGE_CURVE('',#38720,#38723,#22161,.T.);
#49801=EDGE_CURVE('',#38724,#38725,#31955,.T.);
#49802=EDGE_CURVE('',#38724,#38718,#22162,.T.);
#49803=EDGE_CURVE('',#38719,#38725,#22163,.T.);
#49804=EDGE_CURVE('',#38726,#38727,#31956,.T.);
#49805=EDGE_CURVE('',#38726,#38722,#31957,.T.);
#49806=EDGE_CURVE('',#38723,#38727,#31958,.T.);
#49807=EDGE_CURVE('',#38728,#38729,#31959,.T.);
#49808=EDGE_CURVE('',#38728,#38724,#31960,.T.);
#49809=EDGE_CURVE('',#38725,#38729,#31961,.T.);
#49810=EDGE_CURVE('',#38730,#38731,#31962,.T.);
#49811=EDGE_CURVE('',#38730,#38726,#31963,.T.);
#49812=EDGE_CURVE('',#38727,#38731,#31964,.T.);
#49813=EDGE_CURVE('',#38732,#38733,#31965,.T.);
#49814=EDGE_CURVE('',#38732,#38728,#22164,.T.);
#49815=EDGE_CURVE('',#38729,#38733,#22165,.T.);
#49816=EDGE_CURVE('',#38731,#38732,#31966,.T.);
#49817=EDGE_CURVE('',#38733,#38730,#31967,.T.);
#49818=EDGE_CURVE('',#38734,#38735,#31968,.T.);
#49819=EDGE_CURVE('',#38734,#38736,#31969,.T.);
#49820=EDGE_CURVE('',#38737,#38736,#31970,.T.);
#49821=EDGE_CURVE('',#38737,#38735,#31971,.T.);
#49822=EDGE_CURVE('',#38738,#38739,#31972,.T.);
#49823=EDGE_CURVE('',#38738,#38737,#22166,.T.);
#49824=EDGE_CURVE('',#38736,#38739,#22167,.T.);
#49825=EDGE_CURVE('',#38740,#38741,#31973,.T.);
#49826=EDGE_CURVE('',#38740,#38734,#22168,.T.);
#49827=EDGE_CURVE('',#38735,#38741,#22169,.T.);
#49828=EDGE_CURVE('',#38742,#38743,#31974,.T.);
#49829=EDGE_CURVE('',#38742,#38738,#31975,.T.);
#49830=EDGE_CURVE('',#38739,#38743,#31976,.T.);
#49831=EDGE_CURVE('',#38744,#38745,#31977,.T.);
#49832=EDGE_CURVE('',#38744,#38740,#31978,.T.);
#49833=EDGE_CURVE('',#38741,#38745,#31979,.T.);
#49834=EDGE_CURVE('',#38746,#38747,#31980,.T.);
#49835=EDGE_CURVE('',#38746,#38742,#22170,.T.);
#49836=EDGE_CURVE('',#38743,#38747,#22171,.T.);
#49837=EDGE_CURVE('',#38748,#38749,#31981,.T.);
#49838=EDGE_CURVE('',#38748,#38744,#22172,.T.);
#49839=EDGE_CURVE('',#38745,#38749,#22173,.T.);
#49840=EDGE_CURVE('',#38747,#38748,#31982,.T.);
#49841=EDGE_CURVE('',#38749,#38746,#31983,.T.);
#49842=EDGE_CURVE('',#38750,#38751,#31984,.T.);
#49843=EDGE_CURVE('',#38750,#38752,#31985,.T.);
#49844=EDGE_CURVE('',#38753,#38752,#31986,.T.);
#49845=EDGE_CURVE('',#38753,#38751,#31987,.T.);
#49846=EDGE_CURVE('',#38754,#38755,#31988,.T.);
#49847=EDGE_CURVE('',#38754,#38753,#22174,.T.);
#49848=EDGE_CURVE('',#38752,#38755,#22175,.T.);
#49849=EDGE_CURVE('',#38756,#38757,#31989,.T.);
#49850=EDGE_CURVE('',#38756,#38750,#22176,.T.);
#49851=EDGE_CURVE('',#38751,#38757,#22177,.T.);
#49852=EDGE_CURVE('',#38758,#38759,#31990,.T.);
#49853=EDGE_CURVE('',#38758,#38754,#31991,.T.);
#49854=EDGE_CURVE('',#38755,#38759,#31992,.T.);
#49855=EDGE_CURVE('',#38760,#38761,#31993,.T.);
#49856=EDGE_CURVE('',#38760,#38756,#31994,.T.);
#49857=EDGE_CURVE('',#38757,#38761,#31995,.T.);
#49858=EDGE_CURVE('',#38762,#38763,#31996,.T.);
#49859=EDGE_CURVE('',#38762,#38758,#22178,.T.);
#49860=EDGE_CURVE('',#38759,#38763,#22179,.T.);
#49861=EDGE_CURVE('',#38764,#38765,#31997,.T.);
#49862=EDGE_CURVE('',#38764,#38760,#22180,.T.);
#49863=EDGE_CURVE('',#38761,#38765,#22181,.T.);
#49864=EDGE_CURVE('',#38763,#38764,#31998,.T.);
#49865=EDGE_CURVE('',#38765,#38762,#31999,.T.);
#49866=EDGE_CURVE('',#38766,#38767,#32000,.T.);
#49867=EDGE_CURVE('',#38766,#38768,#32001,.T.);
#49868=EDGE_CURVE('',#38769,#38768,#32002,.T.);
#49869=EDGE_CURVE('',#38769,#38767,#32003,.T.);
#49870=EDGE_CURVE('',#38770,#38771,#32004,.T.);
#49871=EDGE_CURVE('',#38770,#38769,#22182,.T.);
#49872=EDGE_CURVE('',#38768,#38771,#22183,.T.);
#49873=EDGE_CURVE('',#38772,#38773,#32005,.T.);
#49874=EDGE_CURVE('',#38772,#38766,#22184,.T.);
#49875=EDGE_CURVE('',#38767,#38773,#22185,.T.);
#49876=EDGE_CURVE('',#38774,#38775,#32006,.T.);
#49877=EDGE_CURVE('',#38774,#38770,#32007,.T.);
#49878=EDGE_CURVE('',#38771,#38775,#32008,.T.);
#49879=EDGE_CURVE('',#38776,#38777,#32009,.T.);
#49880=EDGE_CURVE('',#38776,#38772,#32010,.T.);
#49881=EDGE_CURVE('',#38773,#38777,#32011,.T.);
#49882=EDGE_CURVE('',#38778,#38779,#32012,.T.);
#49883=EDGE_CURVE('',#38778,#38774,#22186,.T.);
#49884=EDGE_CURVE('',#38775,#38779,#22187,.T.);
#49885=EDGE_CURVE('',#38780,#38781,#32013,.T.);
#49886=EDGE_CURVE('',#38780,#38776,#32014,.T.);
#49887=EDGE_CURVE('',#38777,#38781,#32015,.T.);
#49888=EDGE_CURVE('',#38779,#38782,#32016,.T.);
#49889=EDGE_CURVE('',#38783,#38782,#32017,.T.);
#49890=EDGE_CURVE('',#38783,#38778,#32018,.T.);
#49891=EDGE_CURVE('',#38781,#38783,#32019,.T.);
#49892=EDGE_CURVE('',#38782,#38780,#32020,.T.);
#49893=EDGE_CURVE('',#38784,#38785,#32021,.T.);
#49894=EDGE_CURVE('',#38784,#38786,#32022,.T.);
#49895=EDGE_CURVE('',#38787,#38786,#32023,.T.);
#49896=EDGE_CURVE('',#38787,#38785,#32024,.T.);
#49897=EDGE_CURVE('',#38788,#38789,#32025,.T.);
#49898=EDGE_CURVE('',#38788,#38787,#22188,.T.);
#49899=EDGE_CURVE('',#38786,#38789,#22189,.T.);
#49900=EDGE_CURVE('',#38790,#38791,#32026,.T.);
#49901=EDGE_CURVE('',#38790,#38784,#22190,.T.);
#49902=EDGE_CURVE('',#38785,#38791,#22191,.T.);
#49903=EDGE_CURVE('',#38792,#38793,#32027,.T.);
#49904=EDGE_CURVE('',#38792,#38788,#32028,.T.);
#49905=EDGE_CURVE('',#38789,#38793,#32029,.T.);
#49906=EDGE_CURVE('',#38794,#38795,#32030,.T.);
#49907=EDGE_CURVE('',#38794,#38790,#32031,.T.);
#49908=EDGE_CURVE('',#38791,#38795,#32032,.T.);
#49909=EDGE_CURVE('',#38796,#38797,#32033,.T.);
#49910=EDGE_CURVE('',#38796,#38792,#32034,.T.);
#49911=EDGE_CURVE('',#38793,#38797,#32035,.T.);
#49912=EDGE_CURVE('',#38798,#38799,#32036,.T.);
#49913=EDGE_CURVE('',#38798,#38794,#22192,.T.);
#49914=EDGE_CURVE('',#38795,#38799,#22193,.T.);
#49915=EDGE_CURVE('',#38797,#38798,#32037,.T.);
#49916=EDGE_CURVE('',#38799,#38796,#32038,.T.);
#49917=EDGE_CURVE('',#38800,#38801,#32039,.T.);
#49918=EDGE_CURVE('',#38800,#38802,#32040,.T.);
#49919=EDGE_CURVE('',#38803,#38802,#32041,.T.);
#49920=EDGE_CURVE('',#38803,#38801,#32042,.T.);
#49921=EDGE_CURVE('',#38804,#38805,#32043,.T.);
#49922=EDGE_CURVE('',#38804,#38803,#22194,.T.);
#49923=EDGE_CURVE('',#38802,#38805,#22195,.T.);
#49924=EDGE_CURVE('',#38806,#38807,#32044,.T.);
#49925=EDGE_CURVE('',#38806,#38800,#22196,.T.);
#49926=EDGE_CURVE('',#38801,#38807,#22197,.T.);
#49927=EDGE_CURVE('',#38808,#38809,#32045,.T.);
#49928=EDGE_CURVE('',#38808,#38804,#32046,.T.);
#49929=EDGE_CURVE('',#38805,#38809,#32047,.T.);
#49930=EDGE_CURVE('',#38810,#38811,#32048,.T.);
#49931=EDGE_CURVE('',#38810,#38806,#32049,.T.);
#49932=EDGE_CURVE('',#38807,#38811,#32050,.T.);
#49933=EDGE_CURVE('',#38812,#38813,#32051,.T.);
#49934=EDGE_CURVE('',#38812,#38808,#32052,.T.);
#49935=EDGE_CURVE('',#38809,#38813,#32053,.T.);
#49936=EDGE_CURVE('',#38814,#38815,#32054,.T.);
#49937=EDGE_CURVE('',#38814,#38810,#22198,.T.);
#49938=EDGE_CURVE('',#38811,#38815,#22199,.T.);
#49939=EDGE_CURVE('',#38816,#38817,#32055,.T.);
#49940=EDGE_CURVE('',#38816,#38812,#32056,.T.);
#49941=EDGE_CURVE('',#38813,#38817,#32057,.T.);
#49942=EDGE_CURVE('',#38818,#38819,#32058,.T.);
#49943=EDGE_CURVE('',#38818,#38814,#32059,.T.);
#49944=EDGE_CURVE('',#38815,#38819,#32060,.T.);
#49945=EDGE_CURVE('',#38817,#38818,#32061,.T.);
#49946=EDGE_CURVE('',#38819,#38816,#32062,.T.);
#49947=EDGE_CURVE('',#38820,#38821,#32063,.T.);
#49948=EDGE_CURVE('',#38820,#38822,#32064,.T.);
#49949=EDGE_CURVE('',#38823,#38822,#32065,.T.);
#49950=EDGE_CURVE('',#38823,#38821,#32066,.T.);
#49951=EDGE_CURVE('',#38824,#38825,#32067,.T.);
#49952=EDGE_CURVE('',#38824,#38823,#22200,.T.);
#49953=EDGE_CURVE('',#38822,#38825,#22201,.T.);
#49954=EDGE_CURVE('',#38826,#38827,#32068,.T.);
#49955=EDGE_CURVE('',#38826,#38820,#22202,.T.);
#49956=EDGE_CURVE('',#38821,#38827,#22203,.T.);
#49957=EDGE_CURVE('',#38828,#38829,#32069,.T.);
#49958=EDGE_CURVE('',#38828,#38824,#32070,.T.);
#49959=EDGE_CURVE('',#38825,#38829,#32071,.T.);
#49960=EDGE_CURVE('',#38830,#38831,#32072,.T.);
#49961=EDGE_CURVE('',#38830,#38826,#32073,.T.);
#49962=EDGE_CURVE('',#38827,#38831,#32074,.T.);
#49963=EDGE_CURVE('',#38832,#38833,#32075,.T.);
#49964=EDGE_CURVE('',#38832,#38828,#22204,.T.);
#49965=EDGE_CURVE('',#38829,#38833,#22205,.T.);
#49966=EDGE_CURVE('',#38834,#38835,#32076,.T.);
#49967=EDGE_CURVE('',#38834,#38830,#22206,.T.);
#49968=EDGE_CURVE('',#38831,#38835,#22207,.T.);
#49969=EDGE_CURVE('',#38833,#38834,#32077,.T.);
#49970=EDGE_CURVE('',#38835,#38832,#32078,.T.);
#49971=EDGE_CURVE('',#38836,#38837,#32079,.T.);
#49972=EDGE_CURVE('',#38836,#38838,#32080,.T.);
#49973=EDGE_CURVE('',#38839,#38838,#32081,.T.);
#49974=EDGE_CURVE('',#38839,#38837,#32082,.T.);
#49975=EDGE_CURVE('',#38840,#38841,#32083,.T.);
#49976=EDGE_CURVE('',#38840,#38839,#22208,.T.);
#49977=EDGE_CURVE('',#38838,#38841,#22209,.T.);
#49978=EDGE_CURVE('',#38842,#38843,#32084,.T.);
#49979=EDGE_CURVE('',#38842,#38836,#22210,.T.);
#49980=EDGE_CURVE('',#38837,#38843,#22211,.T.);
#49981=EDGE_CURVE('',#38844,#38845,#32085,.T.);
#49982=EDGE_CURVE('',#38844,#38840,#32086,.T.);
#49983=EDGE_CURVE('',#38841,#38845,#32087,.T.);
#49984=EDGE_CURVE('',#38846,#38847,#32088,.T.);
#49985=EDGE_CURVE('',#38846,#38842,#32089,.T.);
#49986=EDGE_CURVE('',#38843,#38847,#32090,.T.);
#49987=EDGE_CURVE('',#38848,#38849,#32091,.T.);
#49988=EDGE_CURVE('',#38848,#38844,#22212,.T.);
#49989=EDGE_CURVE('',#38845,#38849,#22213,.T.);
#49990=EDGE_CURVE('',#38850,#38851,#32092,.T.);
#49991=EDGE_CURVE('',#38850,#38846,#32093,.T.);
#49992=EDGE_CURVE('',#38847,#38851,#32094,.T.);
#49993=EDGE_CURVE('',#38852,#38853,#32095,.T.);
#49994=EDGE_CURVE('',#38852,#38848,#32096,.T.);
#49995=EDGE_CURVE('',#38849,#38853,#32097,.T.);
#49996=EDGE_CURVE('',#38854,#38855,#32098,.T.);
#49997=EDGE_CURVE('',#38854,#38850,#32099,.T.);
#49998=EDGE_CURVE('',#38851,#38855,#32100,.T.);
#49999=EDGE_CURVE('',#38853,#38854,#32101,.T.);
#50000=EDGE_CURVE('',#38855,#38852,#32102,.T.);
#50001=EDGE_CURVE('',#38856,#38857,#32103,.T.);
#50002=EDGE_CURVE('',#38856,#38858,#32104,.T.);
#50003=EDGE_CURVE('',#38859,#38858,#32105,.T.);
#50004=EDGE_CURVE('',#38859,#38857,#32106,.T.);
#50005=EDGE_CURVE('',#38860,#38861,#32107,.T.);
#50006=EDGE_CURVE('',#38860,#38859,#22214,.T.);
#50007=EDGE_CURVE('',#38858,#38861,#22215,.T.);
#50008=EDGE_CURVE('',#38862,#38863,#32108,.T.);
#50009=EDGE_CURVE('',#38862,#38856,#22216,.T.);
#50010=EDGE_CURVE('',#38857,#38863,#22217,.T.);
#50011=EDGE_CURVE('',#38864,#38865,#32109,.T.);
#50012=EDGE_CURVE('',#38864,#38860,#32110,.T.);
#50013=EDGE_CURVE('',#38861,#38865,#32111,.T.);
#50014=EDGE_CURVE('',#38866,#38867,#32112,.T.);
#50015=EDGE_CURVE('',#38866,#38862,#32113,.T.);
#50016=EDGE_CURVE('',#38863,#38867,#32114,.T.);
#50017=EDGE_CURVE('',#38868,#38869,#32115,.T.);
#50018=EDGE_CURVE('',#38868,#38864,#22218,.T.);
#50019=EDGE_CURVE('',#38865,#38869,#22219,.T.);
#50020=EDGE_CURVE('',#38870,#38871,#32116,.T.);
#50021=EDGE_CURVE('',#38870,#38866,#32117,.T.);
#50022=EDGE_CURVE('',#38867,#38871,#32118,.T.);
#50023=EDGE_CURVE('',#38869,#38870,#32119,.T.);
#50024=EDGE_CURVE('',#38871,#38868,#32120,.T.);
#50025=EDGE_CURVE('',#38872,#38873,#32121,.T.);
#50026=EDGE_CURVE('',#38872,#38874,#32122,.T.);
#50027=EDGE_CURVE('',#38875,#38874,#32123,.T.);
#50028=EDGE_CURVE('',#38875,#38873,#32124,.T.);
#50029=EDGE_CURVE('',#38876,#38877,#32125,.T.);
#50030=EDGE_CURVE('',#38876,#38875,#22220,.T.);
#50031=EDGE_CURVE('',#38874,#38877,#22221,.T.);
#50032=EDGE_CURVE('',#38878,#38879,#32126,.T.);
#50033=EDGE_CURVE('',#38878,#38872,#22222,.T.);
#50034=EDGE_CURVE('',#38873,#38879,#22223,.T.);
#50035=EDGE_CURVE('',#38880,#38881,#32127,.T.);
#50036=EDGE_CURVE('',#38880,#38876,#32128,.T.);
#50037=EDGE_CURVE('',#38877,#38881,#32129,.T.);
#50038=EDGE_CURVE('',#38882,#38883,#32130,.T.);
#50039=EDGE_CURVE('',#38882,#38878,#32131,.T.);
#50040=EDGE_CURVE('',#38879,#38883,#32132,.T.);
#50041=EDGE_CURVE('',#38884,#38885,#32133,.T.);
#50042=EDGE_CURVE('',#38884,#38880,#22224,.T.);
#50043=EDGE_CURVE('',#38881,#38885,#22225,.T.);
#50044=EDGE_CURVE('',#38886,#38887,#32134,.T.);
#50045=EDGE_CURVE('',#38886,#38882,#22226,.T.);
#50046=EDGE_CURVE('',#38883,#38887,#22227,.T.);
#50047=EDGE_CURVE('',#38885,#38886,#32135,.T.);
#50048=EDGE_CURVE('',#38887,#38884,#32136,.T.);
#50049=EDGE_CURVE('',#38888,#38889,#32137,.T.);
#50050=EDGE_CURVE('',#38888,#38890,#32138,.T.);
#50051=EDGE_CURVE('',#38891,#38890,#32139,.T.);
#50052=EDGE_CURVE('',#38891,#38889,#32140,.T.);
#50053=EDGE_CURVE('',#38892,#38893,#32141,.T.);
#50054=EDGE_CURVE('',#38892,#38891,#22228,.T.);
#50055=EDGE_CURVE('',#38890,#38893,#22229,.T.);
#50056=EDGE_CURVE('',#38894,#38895,#32142,.T.);
#50057=EDGE_CURVE('',#38894,#38888,#22230,.T.);
#50058=EDGE_CURVE('',#38889,#38895,#22231,.T.);
#50059=EDGE_CURVE('',#38896,#38897,#32143,.T.);
#50060=EDGE_CURVE('',#38896,#38892,#32144,.T.);
#50061=EDGE_CURVE('',#38893,#38897,#32145,.T.);
#50062=EDGE_CURVE('',#38898,#38899,#32146,.T.);
#50063=EDGE_CURVE('',#38898,#38894,#32147,.T.);
#50064=EDGE_CURVE('',#38895,#38899,#32148,.T.);
#50065=EDGE_CURVE('',#38900,#38901,#32149,.T.);
#50066=EDGE_CURVE('',#38900,#38896,#22232,.T.);
#50067=EDGE_CURVE('',#38897,#38901,#22233,.T.);
#50068=EDGE_CURVE('',#38902,#38903,#32150,.T.);
#50069=EDGE_CURVE('',#38902,#38898,#32151,.T.);
#50070=EDGE_CURVE('',#38899,#38903,#32152,.T.);
#50071=EDGE_CURVE('',#38901,#38902,#32153,.T.);
#50072=EDGE_CURVE('',#38903,#38900,#32154,.T.);
#50073=EDGE_CURVE('',#38904,#38905,#32155,.T.);
#50074=EDGE_CURVE('',#38904,#38906,#32156,.T.);
#50075=EDGE_CURVE('',#38907,#38906,#32157,.T.);
#50076=EDGE_CURVE('',#38907,#38905,#32158,.T.);
#50077=EDGE_CURVE('',#38908,#38909,#32159,.T.);
#50078=EDGE_CURVE('',#38908,#38907,#22234,.T.);
#50079=EDGE_CURVE('',#38906,#38909,#22235,.T.);
#50080=EDGE_CURVE('',#38910,#38911,#32160,.T.);
#50081=EDGE_CURVE('',#38910,#38904,#22236,.T.);
#50082=EDGE_CURVE('',#38905,#38911,#22237,.T.);
#50083=EDGE_CURVE('',#38912,#38913,#32161,.T.);
#50084=EDGE_CURVE('',#38912,#38908,#32162,.T.);
#50085=EDGE_CURVE('',#38909,#38913,#32163,.T.);
#50086=EDGE_CURVE('',#38914,#38915,#32164,.T.);
#50087=EDGE_CURVE('',#38914,#38910,#32165,.T.);
#50088=EDGE_CURVE('',#38911,#38915,#32166,.T.);
#50089=EDGE_CURVE('',#38916,#38917,#32167,.T.);
#50090=EDGE_CURVE('',#38916,#38912,#22238,.T.);
#50091=EDGE_CURVE('',#38913,#38917,#22239,.T.);
#50092=EDGE_CURVE('',#38918,#38919,#32168,.T.);
#50093=EDGE_CURVE('',#38918,#38914,#22240,.T.);
#50094=EDGE_CURVE('',#38915,#38919,#22241,.T.);
#50095=EDGE_CURVE('',#38917,#38918,#32169,.T.);
#50096=EDGE_CURVE('',#38919,#38916,#32170,.T.);
#50097=EDGE_CURVE('',#38920,#38921,#32171,.T.);
#50098=EDGE_CURVE('',#38920,#38922,#32172,.T.);
#50099=EDGE_CURVE('',#38923,#38922,#32173,.T.);
#50100=EDGE_CURVE('',#38923,#38921,#32174,.T.);
#50101=EDGE_CURVE('',#38924,#38925,#32175,.T.);
#50102=EDGE_CURVE('',#38924,#38923,#22242,.T.);
#50103=EDGE_CURVE('',#38922,#38925,#22243,.T.);
#50104=EDGE_CURVE('',#38926,#38927,#32176,.T.);
#50105=EDGE_CURVE('',#38926,#38920,#32177,.T.);
#50106=EDGE_CURVE('',#38921,#38927,#32178,.T.);
#50107=EDGE_CURVE('',#38928,#38929,#32179,.T.);
#50108=EDGE_CURVE('',#38928,#38924,#32180,.T.);
#50109=EDGE_CURVE('',#38925,#38929,#32181,.T.);
#50110=EDGE_CURVE('',#38930,#38931,#32182,.T.);
#50111=EDGE_CURVE('',#38930,#38926,#32183,.T.);
#50112=EDGE_CURVE('',#38927,#38931,#32184,.T.);
#50113=EDGE_CURVE('',#38929,#38930,#22244,.T.);
#50114=EDGE_CURVE('',#38931,#38928,#22245,.T.);
#50115=EDGE_CURVE('',#38932,#38933,#32185,.T.);
#50116=EDGE_CURVE('',#38934,#38933,#32186,.T.);
#50117=EDGE_CURVE('',#38934,#38935,#32187,.T.);
#50118=EDGE_CURVE('',#38932,#38935,#32188,.T.);
#50119=EDGE_CURVE('',#38936,#38937,#32189,.T.);
#50120=EDGE_CURVE('',#38936,#38934,#22246,.T.);
#50121=EDGE_CURVE('',#38933,#38937,#22247,.T.);
#50122=EDGE_CURVE('',#38938,#38939,#32190,.T.);
#50123=EDGE_CURVE('',#38938,#38932,#32191,.T.);
#50124=EDGE_CURVE('',#38935,#38939,#32192,.T.);
#50125=EDGE_CURVE('',#38940,#38941,#32193,.T.);
#50126=EDGE_CURVE('',#38940,#38936,#32194,.T.);
#50127=EDGE_CURVE('',#38937,#38941,#32195,.T.);
#50128=EDGE_CURVE('',#38942,#38943,#32196,.T.);
#50129=EDGE_CURVE('',#38942,#38938,#32197,.T.);
#50130=EDGE_CURVE('',#38939,#38943,#32198,.T.);
#50131=EDGE_CURVE('',#38941,#38942,#22248,.T.);
#50132=EDGE_CURVE('',#38943,#38940,#22249,.T.);
#50133=EDGE_CURVE('',#38944,#38945,#32199,.T.);
#50134=EDGE_CURVE('',#38944,#38946,#32200,.T.);
#50135=EDGE_CURVE('',#38946,#38947,#32201,.T.);
#50136=EDGE_CURVE('',#38947,#38945,#32202,.T.);
#50137=EDGE_CURVE('',#38948,#38949,#32203,.T.);
#50138=EDGE_CURVE('',#38948,#38944,#32204,.T.);
#50139=EDGE_CURVE('',#38945,#38949,#32205,.T.);
#50140=EDGE_CURVE('',#38950,#38951,#32206,.T.);
#50141=EDGE_CURVE('',#38950,#38948,#32207,.T.);
#50142=EDGE_CURVE('',#38949,#38951,#32208,.T.);
#50143=EDGE_CURVE('',#38952,#38953,#32209,.T.);
#50144=EDGE_CURVE('',#38952,#38950,#32210,.T.);
#50145=EDGE_CURVE('',#38951,#38953,#32211,.T.);
#50146=EDGE_CURVE('',#38954,#38955,#32212,.T.);
#50147=EDGE_CURVE('',#38954,#38952,#32213,.T.);
#50148=EDGE_CURVE('',#38953,#38955,#32214,.T.);
#50149=EDGE_CURVE('',#38956,#38957,#32215,.T.);
#50150=EDGE_CURVE('',#38956,#38954,#32216,.T.);
#50151=EDGE_CURVE('',#38955,#38957,#32217,.T.);
#50152=EDGE_CURVE('',#38958,#38959,#32218,.T.);
#50153=EDGE_CURVE('',#38958,#38956,#32219,.T.);
#50154=EDGE_CURVE('',#38957,#38959,#32220,.T.);
#50155=EDGE_CURVE('',#38960,#38961,#32221,.T.);
#50156=EDGE_CURVE('',#38960,#38962,#32222,.T.);
#50157=EDGE_CURVE('',#38962,#38963,#32223,.T.);
#50158=EDGE_CURVE('',#38963,#38961,#32224,.T.);
#50159=EDGE_CURVE('',#38964,#38965,#32225,.T.);
#50160=EDGE_CURVE('',#38964,#38960,#32226,.T.);
#50161=EDGE_CURVE('',#38961,#38965,#32227,.T.);
#50162=EDGE_CURVE('',#38966,#38967,#32228,.T.);
#50163=EDGE_CURVE('',#38966,#38964,#32229,.T.);
#50164=EDGE_CURVE('',#38965,#38967,#32230,.T.);
#50165=EDGE_CURVE('',#38968,#38969,#32231,.T.);
#50166=EDGE_CURVE('',#38968,#38966,#32232,.T.);
#50167=EDGE_CURVE('',#38967,#38969,#32233,.T.);
#50168=EDGE_CURVE('',#38970,#38971,#32234,.T.);
#50169=EDGE_CURVE('',#38970,#38968,#32235,.T.);
#50170=EDGE_CURVE('',#38969,#38971,#32236,.T.);
#50171=EDGE_CURVE('',#38972,#38973,#32237,.T.);
#50172=EDGE_CURVE('',#38972,#38970,#32238,.T.);
#50173=EDGE_CURVE('',#38971,#38973,#32239,.T.);
#50174=EDGE_CURVE('',#38974,#38975,#32240,.T.);
#50175=EDGE_CURVE('',#38974,#38972,#32241,.T.);
#50176=EDGE_CURVE('',#38973,#38975,#32242,.T.);
#50177=EDGE_CURVE('',#38976,#38977,#32243,.T.);
#50178=EDGE_CURVE('',#38976,#38978,#32244,.T.);
#50179=EDGE_CURVE('',#38978,#38979,#5485,.T.);
#50180=EDGE_CURVE('',#38979,#38977,#32245,.T.);
#50181=EDGE_CURVE('',#38980,#38981,#32246,.T.);
#50182=EDGE_CURVE('',#38980,#38976,#22250,.T.);
#50183=EDGE_CURVE('',#38977,#38981,#22251,.T.);
#50184=EDGE_CURVE('',#38982,#38980,#32247,.T.);
#50185=EDGE_CURVE('',#38981,#38983,#32248,.T.);
#50186=EDGE_CURVE('',#38982,#38983,#32249,.T.);
#50187=EDGE_CURVE('',#38984,#38985,#32250,.T.);
#50188=EDGE_CURVE('',#38984,#38982,#32251,.T.);
#50189=EDGE_CURVE('',#38983,#38985,#32252,.T.);
#50190=EDGE_CURVE('',#38986,#38987,#32253,.T.);
#50191=EDGE_CURVE('',#38986,#38984,#32254,.T.);
#50192=EDGE_CURVE('',#38985,#38987,#32255,.T.);
#50193=EDGE_CURVE('',#38988,#38989,#32256,.T.);
#50194=EDGE_CURVE('',#38988,#38986,#22252,.T.);
#50195=EDGE_CURVE('',#38987,#38989,#22253,.T.);
#50196=EDGE_CURVE('',#38990,#38991,#5486,.T.);
#50197=EDGE_CURVE('',#38991,#38988,#32257,.T.);
#50198=EDGE_CURVE('',#38989,#38990,#32258,.T.);
#50199=EDGE_CURVE('',#38992,#38993,#32259,.T.);
#50200=EDGE_CURVE('',#38992,#38994,#32260,.T.);
#50201=EDGE_CURVE('',#38994,#38995,#5487,.T.);
#50202=EDGE_CURVE('',#38995,#38993,#32261,.T.);
#50203=EDGE_CURVE('',#38996,#38997,#32262,.T.);
#50204=EDGE_CURVE('',#38996,#38992,#22254,.T.);
#50205=EDGE_CURVE('',#38993,#38997,#22255,.T.);
#50206=EDGE_CURVE('',#38998,#38999,#32263,.T.);
#50207=EDGE_CURVE('',#38998,#38996,#32264,.T.);
#50208=EDGE_CURVE('',#38997,#38999,#32265,.T.);
#50209=EDGE_CURVE('',#39000,#39001,#32266,.T.);
#50210=EDGE_CURVE('',#39000,#38998,#32267,.T.);
#50211=EDGE_CURVE('',#38999,#39001,#32268,.T.);
#50212=EDGE_CURVE('',#39002,#39003,#32269,.T.);
#50213=EDGE_CURVE('',#39002,#39000,#32270,.T.);
#50214=EDGE_CURVE('',#39001,#39003,#32271,.T.);
#50215=EDGE_CURVE('',#39004,#39005,#32272,.T.);
#50216=EDGE_CURVE('',#39004,#39002,#22256,.T.);
#50217=EDGE_CURVE('',#39003,#39005,#22257,.T.);
#50218=EDGE_CURVE('',#39006,#39007,#5488,.T.);
#50219=EDGE_CURVE('',#39007,#39004,#32273,.T.);
#50220=EDGE_CURVE('',#39005,#39006,#32274,.T.);
#50221=EDGE_CURVE('',#39008,#39009,#32275,.T.);
#50222=EDGE_CURVE('',#39008,#39010,#32276,.T.);
#50223=EDGE_CURVE('',#39010,#39011,#5489,.T.);
#50224=EDGE_CURVE('',#39011,#39009,#32277,.T.);
#50225=EDGE_CURVE('',#39012,#39013,#32278,.T.);
#50226=EDGE_CURVE('',#39012,#39008,#22258,.T.);
#50227=EDGE_CURVE('',#39009,#39013,#22259,.T.);
#50228=EDGE_CURVE('',#39014,#39012,#32279,.T.);
#50229=EDGE_CURVE('',#39013,#39015,#32280,.T.);
#50230=EDGE_CURVE('',#39014,#39015,#32281,.T.);
#50231=EDGE_CURVE('',#39016,#39017,#32282,.T.);
#50232=EDGE_CURVE('',#39016,#39014,#32283,.T.);
#50233=EDGE_CURVE('',#39015,#39017,#32284,.T.);
#50234=EDGE_CURVE('',#39018,#39019,#32285,.T.);
#50235=EDGE_CURVE('',#39018,#39016,#32286,.T.);
#50236=EDGE_CURVE('',#39017,#39019,#32287,.T.);
#50237=EDGE_CURVE('',#39020,#39021,#32288,.T.);
#50238=EDGE_CURVE('',#39020,#39018,#22260,.T.);
#50239=EDGE_CURVE('',#39019,#39021,#22261,.T.);
#50240=EDGE_CURVE('',#39022,#39023,#5490,.T.);
#50241=EDGE_CURVE('',#39023,#39020,#32289,.T.);
#50242=EDGE_CURVE('',#39021,#39022,#32290,.T.);
#50243=EDGE_CURVE('',#39024,#39025,#5491,.F.);
#50244=EDGE_CURVE('',#39025,#39026,#32291,.T.);
#50245=EDGE_CURVE('',#39027,#39026,#32292,.T.);
#50246=EDGE_CURVE('',#39027,#39024,#32293,.T.);
#50247=EDGE_CURVE('',#39028,#39029,#32294,.T.);
#50248=EDGE_CURVE('',#39028,#39027,#22262,.T.);
#50249=EDGE_CURVE('',#39026,#39029,#22263,.T.);
#50250=EDGE_CURVE('',#39030,#39031,#32295,.T.);
#50251=EDGE_CURVE('',#39030,#39028,#32296,.T.);
#50252=EDGE_CURVE('',#39029,#39031,#32297,.T.);
#50253=EDGE_CURVE('',#39032,#39033,#32298,.T.);
#50254=EDGE_CURVE('',#39032,#39030,#32299,.T.);
#50255=EDGE_CURVE('',#39031,#39033,#32300,.T.);
#50256=EDGE_CURVE('',#39034,#39035,#32301,.T.);
#50257=EDGE_CURVE('',#39034,#39032,#32302,.T.);
#50258=EDGE_CURVE('',#39033,#39035,#32303,.T.);
#50259=EDGE_CURVE('',#39036,#39037,#32304,.T.);
#50260=EDGE_CURVE('',#39036,#39034,#22264,.T.);
#50261=EDGE_CURVE('',#39035,#39037,#22265,.T.);
#50262=EDGE_CURVE('',#39038,#39039,#5492,.T.);
#50263=EDGE_CURVE('',#39039,#39036,#32305,.T.);
#50264=EDGE_CURVE('',#39037,#39038,#32306,.T.);
#50265=EDGE_CURVE('',#39040,#39041,#32307,.T.);
#50266=EDGE_CURVE('',#39040,#39042,#32308,.T.);
#50267=EDGE_CURVE('',#39042,#39043,#32309,.T.);
#50268=EDGE_CURVE('',#39043,#39041,#32310,.T.);
#50269=EDGE_CURVE('',#39044,#39045,#32311,.T.);
#50270=EDGE_CURVE('',#39044,#39040,#32312,.T.);
#50271=EDGE_CURVE('',#39041,#39045,#32313,.T.);
#50272=EDGE_CURVE('',#39046,#39047,#32314,.T.);
#50273=EDGE_CURVE('',#39046,#39044,#32315,.T.);
#50274=EDGE_CURVE('',#39045,#39047,#32316,.T.);
#50275=EDGE_CURVE('',#39048,#39049,#32317,.T.);
#50276=EDGE_CURVE('',#39048,#39046,#32318,.T.);
#50277=EDGE_CURVE('',#39047,#39049,#32319,.T.);
#50278=EDGE_CURVE('',#39050,#39051,#32320,.T.);
#50279=EDGE_CURVE('',#39050,#39048,#32321,.T.);
#50280=EDGE_CURVE('',#39049,#39051,#32322,.T.);
#50281=EDGE_CURVE('',#39052,#39053,#32323,.T.);
#50282=EDGE_CURVE('',#39052,#39050,#32324,.T.);
#50283=EDGE_CURVE('',#39051,#39053,#32325,.T.);
#50284=EDGE_CURVE('',#39054,#39055,#32326,.T.);
#50285=EDGE_CURVE('',#39054,#39052,#32327,.T.);
#50286=EDGE_CURVE('',#39053,#39055,#32328,.T.);
#50287=EDGE_CURVE('',#39056,#39057,#5493,.T.);
#50288=EDGE_CURVE('',#39057,#39058,#5494,.T.);
#50289=EDGE_CURVE('',#39058,#39059,#32329,.T.);
#50290=EDGE_CURVE('',#39059,#39060,#5495,.T.);
#50291=EDGE_CURVE('',#39061,#39060,#32330,.T.);
#50292=EDGE_CURVE('',#39061,#39056,#5496,.T.);
#50293=EDGE_CURVE('',#39062,#39063,#32331,.T.);
#50294=EDGE_CURVE('',#39062,#39061,#5497,.T.);
#50295=EDGE_CURVE('',#39060,#39063,#5498,.T.);
#50296=EDGE_CURVE('',#39064,#39065,#32332,.T.);
#50297=EDGE_CURVE('',#39064,#39062,#32333,.T.);
#50298=EDGE_CURVE('',#39063,#39065,#32334,.T.);
#50299=EDGE_CURVE('',#39066,#39067,#32335,.T.);
#50300=EDGE_CURVE('',#39066,#39064,#5499,.T.);
#50301=EDGE_CURVE('',#39065,#39067,#5500,.T.);
#50302=EDGE_CURVE('',#39068,#39069,#32336,.T.);
#50303=EDGE_CURVE('',#39068,#39066,#5501,.T.);
#50304=EDGE_CURVE('',#39067,#39069,#5502,.T.);
#50305=EDGE_CURVE('',#39070,#39071,#32337,.T.);
#50306=EDGE_CURVE('',#39070,#39068,#5503,.T.);
#50307=EDGE_CURVE('',#39069,#39071,#5504,.T.);
#50308=EDGE_CURVE('',#39072,#39073,#32338,.T.);
#50309=EDGE_CURVE('',#39072,#39070,#32339,.T.);
#50310=EDGE_CURVE('',#39071,#39073,#32340,.T.);
#50311=EDGE_CURVE('',#39074,#39075,#32341,.T.);
#50312=EDGE_CURVE('',#39074,#39072,#5505,.T.);
#50313=EDGE_CURVE('',#39073,#39075,#5506,.T.);
#50314=EDGE_CURVE('',#39076,#39077,#32342,.T.);
#50315=EDGE_CURVE('',#39076,#39078,#5507,.T.);
#50316=EDGE_CURVE('',#39078,#39079,#5508,.T.);
#50317=EDGE_CURVE('',#39079,#39080,#5509,.T.);
#50318=EDGE_CURVE('',#39080,#39081,#5510,.T.);
#50319=EDGE_CURVE('',#39081,#39082,#5511,.T.);
#50320=EDGE_CURVE('',#39082,#39074,#5512,.T.);
#50321=EDGE_CURVE('',#39075,#39077,#5513,.T.);
#50322=EDGE_CURVE('',#39083,#39084,#32343,.T.);
#50323=EDGE_CURVE('',#39083,#39076,#5514,.T.);
#50324=EDGE_CURVE('',#39077,#39084,#5515,.T.);
#50325=EDGE_CURVE('',#39085,#39086,#32344,.T.);
#50326=EDGE_CURVE('',#39085,#39083,#32345,.T.);
#50327=EDGE_CURVE('',#39084,#39086,#32346,.T.);
#50328=EDGE_CURVE('',#39087,#39088,#32347,.T.);
#50329=EDGE_CURVE('',#39087,#39085,#5516,.T.);
#50330=EDGE_CURVE('',#39086,#39088,#5517,.T.);
#50331=EDGE_CURVE('',#39089,#39090,#32348,.T.);
#50332=EDGE_CURVE('',#39089,#39087,#5518,.T.);
#50333=EDGE_CURVE('',#39088,#39090,#5519,.T.);
#50334=EDGE_CURVE('',#39091,#39092,#32349,.T.);
#50335=EDGE_CURVE('',#39091,#39089,#5520,.T.);
#50336=EDGE_CURVE('',#39090,#39092,#5521,.T.);
#50337=EDGE_CURVE('',#39093,#39094,#32350,.T.);
#50338=EDGE_CURVE('',#39093,#39091,#32351,.T.);
#50339=EDGE_CURVE('',#39092,#39094,#32352,.T.);
#50340=EDGE_CURVE('',#39095,#39096,#32353,.T.);
#50341=EDGE_CURVE('',#39095,#39093,#5522,.T.);
#50342=EDGE_CURVE('',#39094,#39096,#5523,.T.);
#50343=EDGE_CURVE('',#38385,#39097,#1217,.T.);
#50344=EDGE_CURVE('',#39098,#39097,#32354,.T.);
#50345=EDGE_CURVE('',#39098,#38377,#32355,.T.);
#50346=EDGE_CURVE('',#39099,#39100,#32356,.T.);
#50347=EDGE_CURVE('',#39099,#39098,#32357,.T.);
#50348=EDGE_CURVE('',#39097,#39100,#32358,.T.);
#50349=EDGE_CURVE('',#39101,#39102,#32359,.T.);
#50350=EDGE_CURVE('',#39101,#39099,#5524,.T.);
#50351=EDGE_CURVE('',#39100,#39102,#5525,.T.);
#50352=EDGE_CURVE('',#39103,#39104,#32360,.T.);
#50353=EDGE_CURVE('',#39103,#39101,#5526,.T.);
#50354=EDGE_CURVE('',#39102,#39104,#5527,.T.);
#50355=EDGE_CURVE('',#39105,#39106,#5528,.T.);
#50356=EDGE_CURVE('',#39107,#39105,#5529,.T.);
#50357=EDGE_CURVE('',#39107,#39103,#32361,.T.);
#50358=EDGE_CURVE('',#39104,#39106,#32362,.T.);
#50359=EDGE_CURVE('',#39108,#39109,#5530,.T.);
#50360=EDGE_CURVE('',#39109,#39107,#32363,.T.);
#50361=EDGE_CURVE('',#39108,#39105,#32364,.T.);
#50362=EDGE_CURVE('',#39108,#39106,#5531,.T.);
#50363=EDGE_CURVE('',#39110,#39111,#5532,.T.);
#50364=EDGE_CURVE('',#39110,#39112,#5533,.T.);
#50365=EDGE_CURVE('',#39112,#39113,#5534,.T.);
#50366=EDGE_CURVE('',#39113,#39114,#5535,.T.);
#50367=EDGE_CURVE('',#39114,#39115,#5536,.T.);
#50368=EDGE_CURVE('',#39115,#39116,#5537,.T.);
#50369=EDGE_CURVE('',#39116,#39117,#5538,.T.);
#50370=EDGE_CURVE('',#39117,#39108,#5539,.T.);
#50371=EDGE_CURVE('',#39106,#39111,#5540,.T.);
#50372=EDGE_CURVE('',#39110,#39118,#32365,.T.);
#50373=EDGE_CURVE('',#39118,#39111,#5541,.T.);
#50374=EDGE_CURVE('',#39119,#39120,#32366,.T.);
#50375=EDGE_CURVE('',#39120,#39110,#5542,.T.);
#50376=EDGE_CURVE('',#39119,#39118,#5543,.T.);
#50377=EDGE_CURVE('',#39111,#39121,#32367,.T.);
#50378=EDGE_CURVE('',#39122,#39121,#32368,.T.);
#50379=EDGE_CURVE('',#39122,#39119,#32369,.T.);
#50380=EDGE_CURVE('',#39123,#39124,#32370,.T.);
#50381=EDGE_CURVE('',#39123,#39122,#5544,.T.);
#50382=EDGE_CURVE('',#39121,#39124,#5545,.T.);
#50383=EDGE_CURVE('',#39125,#39126,#32371,.T.);
#50384=EDGE_CURVE('',#39125,#39123,#5546,.T.);
#50385=EDGE_CURVE('',#39124,#39126,#5547,.T.);
#50386=EDGE_CURVE('',#39127,#39128,#32372,.T.);
#50387=EDGE_CURVE('',#39127,#39125,#32373,.T.);
#50388=EDGE_CURVE('',#39126,#39128,#32374,.T.);
#50389=EDGE_CURVE('',#38401,#39127,#1996,.T.);
#50390=EDGE_CURVE('',#39128,#38391,#5548,.T.);
#50391=EDGE_CURVE('',#39129,#39130,#32375,.T.);
#50392=EDGE_CURVE('',#39129,#39131,#5549,.T.);
#50393=EDGE_CURVE('',#39130,#39131,#5550,.T.);
#50394=EDGE_CURVE('',#39132,#39133,#32376,.T.);
#50395=EDGE_CURVE('',#39133,#39129,#1997,.T.);
#50396=EDGE_CURVE('',#39132,#39130,#1998,.T.);
#50397=EDGE_CURVE('',#39131,#39134,#32377,.T.);
#50398=EDGE_CURVE('',#39135,#39134,#32378,.T.);
#50399=EDGE_CURVE('',#39135,#39132,#32379,.T.);
#50400=EDGE_CURVE('',#39136,#39137,#32380,.T.);
#50401=EDGE_CURVE('',#39136,#39135,#5551,.T.);
#50402=EDGE_CURVE('',#39134,#39137,#5552,.T.);
#50403=EDGE_CURVE('',#39138,#39139,#32381,.T.);
#50404=EDGE_CURVE('',#39138,#39136,#5553,.T.);
#50405=EDGE_CURVE('',#39137,#39139,#5554,.T.);
#50406=EDGE_CURVE('',#39140,#39141,#32382,.T.);
#50407=EDGE_CURVE('',#39140,#39138,#5555,.T.);
#50408=EDGE_CURVE('',#39139,#39141,#32383,.T.);
#50409=EDGE_CURVE('',#38376,#39140,#1999,.T.);
#50410=EDGE_CURVE('',#39141,#38384,#5556,.T.);
#50411=EDGE_CURVE('',#39142,#39143,#32384,.T.);
#50412=EDGE_CURVE('',#39143,#39144,#2000,.T.);
#50413=EDGE_CURVE('',#39145,#39144,#32385,.T.);
#50414=EDGE_CURVE('',#39145,#39142,#2001,.T.);
#50415=EDGE_CURVE('',#39146,#39147,#5557,.T.);
#50416=EDGE_CURVE('',#39147,#39148,#5558,.T.);
#50417=EDGE_CURVE('',#39148,#39149,#5559,.T.);
#50418=EDGE_CURVE('',#39150,#39149,#5560,.T.);
#50419=EDGE_CURVE('',#39150,#39145,#5561,.T.);
#50420=EDGE_CURVE('',#39144,#39146,#5562,.T.);
#50421=EDGE_CURVE('',#39150,#39151,#5563,.T.);
#50422=EDGE_CURVE('',#39151,#39149,#32386,.T.);
#50423=EDGE_CURVE('',#39152,#39153,#1218,.T.);
#50424=EDGE_CURVE('',#39154,#39153,#32387,.T.);
#50425=EDGE_CURVE('',#39154,#39150,#2002,.T.);
#50426=EDGE_CURVE('',#39152,#39151,#32388,.T.);
#50427=EDGE_CURVE('',#39149,#39155,#5564,.T.);
#50428=EDGE_CURVE('',#39155,#39152,#32389,.T.);
#50429=EDGE_CURVE('',#39156,#39157,#32390,.T.);
#50430=EDGE_CURVE('',#39156,#39154,#5565,.T.);
#50431=EDGE_CURVE('',#39153,#39157,#5566,.T.);
#50432=EDGE_CURVE('',#39158,#39159,#32391,.T.);
#50433=EDGE_CURVE('',#39158,#39156,#1219,.T.);
#50434=EDGE_CURVE('',#39157,#39159,#5567,.T.);
#50435=EDGE_CURVE('',#39160,#39161,#32392,.T.);
#50436=EDGE_CURVE('',#39160,#39158,#32393,.T.);
#50437=EDGE_CURVE('',#39159,#39161,#32394,.T.);
#50438=EDGE_CURVE('',#38400,#39160,#1220,.T.);
#50439=EDGE_CURVE('',#39161,#38409,#5568,.T.);
#50440=EDGE_CURVE('',#39095,#39133,#5569,.T.);
#50441=EDGE_CURVE('',#39132,#39093,#5570,.T.);
#50442=EDGE_CURVE('',#39083,#39107,#5571,.T.);
#50443=EDGE_CURVE('',#39109,#39076,#5572,.T.);
#50444=EDGE_CURVE('',#39074,#39120,#5573,.T.);
#50445=EDGE_CURVE('',#39119,#39072,#5574,.T.);
#50446=EDGE_CURVE('',#39062,#39152,#1221,.T.);
#50447=EDGE_CURVE('',#39155,#39061,#5575,.T.);
#50448=EDGE_CURVE('',#39162,#39163,#32395,.T.);
#50449=EDGE_CURVE('',#39163,#38983,#22266,.T.);
#50450=EDGE_CURVE('',#38981,#39162,#22267,.T.);
#50451=EDGE_CURVE('',#39037,#39164,#22268,.T.);
#50452=EDGE_CURVE('',#39164,#39165,#32396,.T.);
#50453=EDGE_CURVE('',#39165,#39038,#22269,.T.);
#50454=EDGE_CURVE('',#38997,#39166,#22270,.T.);
#50455=EDGE_CURVE('',#39166,#39167,#32397,.T.);
#50456=EDGE_CURVE('',#39167,#38999,#22271,.T.);
#50457=EDGE_CURVE('',#38995,#39168,#22272,.T.);
#50458=EDGE_CURVE('',#39168,#39169,#32398,.T.);
#50459=EDGE_CURVE('',#39169,#38993,#22273,.T.);
#50460=EDGE_CURVE('',#38989,#39170,#22274,.T.);
#50461=EDGE_CURVE('',#39170,#39171,#32399,.T.);
#50462=EDGE_CURVE('',#39171,#38990,#22275,.T.);
#50463=EDGE_CURVE('',#38985,#39172,#22276,.T.);
#50464=EDGE_CURVE('',#39172,#39173,#32400,.T.);
#50465=EDGE_CURVE('',#39173,#38987,#22277,.T.);
#50466=EDGE_CURVE('',#38979,#39174,#22278,.T.);
#50467=EDGE_CURVE('',#39174,#39175,#32401,.T.);
#50468=EDGE_CURVE('',#39175,#38977,#22279,.T.);
#50469=EDGE_CURVE('',#39021,#39176,#22280,.T.);
#50470=EDGE_CURVE('',#39176,#39177,#32402,.T.);
#50471=EDGE_CURVE('',#39177,#39022,#22281,.T.);
#50472=EDGE_CURVE('',#39011,#39178,#22282,.T.);
#50473=EDGE_CURVE('',#39178,#39179,#32403,.T.);
#50474=EDGE_CURVE('',#39179,#39009,#22283,.T.);
#50475=EDGE_CURVE('',#39180,#39181,#32404,.T.);
#50476=EDGE_CURVE('',#39181,#38778,#22284,.T.);
#50477=EDGE_CURVE('',#38783,#39180,#22285,.T.);
#50478=EDGE_CURVE('',#38697,#39182,#22286,.T.);
#50479=EDGE_CURVE('',#39182,#39183,#32405,.T.);
#50480=EDGE_CURVE('',#39183,#38701,#22287,.T.);
#50481=EDGE_CURVE('',#38685,#39184,#22288,.T.);
#50482=EDGE_CURVE('',#39184,#39185,#32406,.T.);
#50483=EDGE_CURVE('',#39185,#38683,#22289,.T.);
#50484=EDGE_CURVE('',#38690,#39186,#22290,.T.);
#50485=EDGE_CURVE('',#39186,#39187,#32407,.T.);
#50486=EDGE_CURVE('',#39187,#38686,#22291,.T.);
#50487=EDGE_CURVE('',#38698,#39188,#22292,.T.);
#50488=EDGE_CURVE('',#39188,#39189,#32408,.T.);
#50489=EDGE_CURVE('',#39189,#38694,#22293,.T.);
#50490=EDGE_CURVE('',#38665,#39190,#22294,.T.);
#50491=EDGE_CURVE('',#39190,#39191,#32409,.T.);
#50492=EDGE_CURVE('',#39191,#38663,#22295,.T.);
#50493=EDGE_CURVE('',#38670,#39192,#22296,.T.);
#50494=EDGE_CURVE('',#39192,#39193,#32410,.T.);
#50495=EDGE_CURVE('',#39193,#38666,#22297,.T.);
#50496=EDGE_CURVE('',#38678,#39194,#22298,.T.);
#50497=EDGE_CURVE('',#39194,#39195,#32411,.T.);
#50498=EDGE_CURVE('',#39195,#38674,#22299,.T.);
#50499=EDGE_CURVE('',#38677,#39196,#22300,.T.);
#50500=EDGE_CURVE('',#39196,#39197,#32412,.T.);
#50501=EDGE_CURVE('',#39197,#38681,#22301,.T.);
#50502=EDGE_CURVE('',#38527,#39198,#22302,.T.);
#50503=EDGE_CURVE('',#39198,#39199,#32413,.T.);
#50504=EDGE_CURVE('',#39199,#38528,#22303,.T.);
#50505=EDGE_CURVE('',#38519,#39200,#22304,.T.);
#50506=EDGE_CURVE('',#39200,#39201,#32414,.T.);
#50507=EDGE_CURVE('',#39201,#38523,#22305,.T.);
#50508=EDGE_CURVE('',#38515,#39202,#22306,.T.);
#50509=EDGE_CURVE('',#39202,#39203,#32415,.T.);
#50510=EDGE_CURVE('',#39203,#38513,#22307,.T.);
#50511=EDGE_CURVE('',#38520,#39204,#22308,.T.);
#50512=EDGE_CURVE('',#39204,#39205,#32416,.T.);
#50513=EDGE_CURVE('',#39205,#38516,#22309,.T.);
#50514=EDGE_CURVE('',#38773,#39206,#22310,.T.);
#50515=EDGE_CURVE('',#39206,#39207,#32417,.T.);
#50516=EDGE_CURVE('',#39207,#38777,#22311,.T.);
#50517=EDGE_CURVE('',#38769,#39208,#22312,.T.);
#50518=EDGE_CURVE('',#39208,#39209,#32418,.T.);
#50519=EDGE_CURVE('',#39209,#38767,#22313,.T.);
#50520=EDGE_CURVE('',#38774,#39210,#22314,.T.);
#50521=EDGE_CURVE('',#39210,#39211,#32419,.T.);
#50522=EDGE_CURVE('',#39211,#38770,#22315,.T.);
#50523=EDGE_CURVE('',#38940,#39212,#22316,.T.);
#50524=EDGE_CURVE('',#39212,#39213,#32420,.T.);
#50525=EDGE_CURVE('',#39213,#38936,#22317,.T.);
#50526=EDGE_CURVE('',#38939,#39214,#22318,.T.);
#50527=EDGE_CURVE('',#39214,#39215,#32421,.T.);
#50528=EDGE_CURVE('',#39215,#38943,#22319,.T.);
#50529=EDGE_CURVE('',#39216,#39217,#32422,.T.);
#50530=EDGE_CURVE('',#39217,#38935,#22320,.T.);
#50531=EDGE_CURVE('',#38934,#39216,#22321,.T.);
#50532=EDGE_CURVE('',#38569,#39218,#22322,.T.);
#50533=EDGE_CURVE('',#39218,#39219,#32423,.T.);
#50534=EDGE_CURVE('',#39219,#38573,#22323,.T.);
#50535=EDGE_CURVE('',#38565,#39220,#22324,.T.);
#50536=EDGE_CURVE('',#39220,#39221,#32424,.T.);
#50537=EDGE_CURVE('',#39221,#38563,#22325,.T.);
#50538=EDGE_CURVE('',#38570,#39222,#22326,.T.);
#50539=EDGE_CURVE('',#39222,#39223,#32425,.T.);
#50540=EDGE_CURVE('',#39223,#38566,#22327,.T.);
#50541=EDGE_CURVE('',#38577,#39224,#22328,.T.);
#50542=EDGE_CURVE('',#39224,#39225,#32426,.T.);
#50543=EDGE_CURVE('',#39225,#38574,#22329,.T.);
#50544=EDGE_CURVE('',#38585,#39226,#22330,.T.);
#50545=EDGE_CURVE('',#39226,#39227,#32427,.T.);
#50546=EDGE_CURVE('',#39227,#38589,#22331,.T.);
#50547=EDGE_CURVE('',#38581,#39228,#22332,.T.);
#50548=EDGE_CURVE('',#39228,#39229,#32428,.T.);
#50549=EDGE_CURVE('',#39229,#38579,#22333,.T.);
#50550=EDGE_CURVE('',#38586,#39230,#22334,.T.);
#50551=EDGE_CURVE('',#39230,#39231,#32429,.T.);
#50552=EDGE_CURVE('',#39231,#38582,#22335,.T.);
#50553=EDGE_CURVE('',#38593,#39232,#22336,.T.);
#50554=EDGE_CURVE('',#39232,#39233,#32430,.T.);
#50555=EDGE_CURVE('',#39233,#38590,#22337,.T.);
#50556=EDGE_CURVE('',#38839,#39234,#22338,.T.);
#50557=EDGE_CURVE('',#39234,#39235,#32431,.T.);
#50558=EDGE_CURVE('',#39235,#38837,#22339,.T.);
#50559=EDGE_CURVE('',#38844,#39236,#22340,.T.);
#50560=EDGE_CURVE('',#39236,#39237,#32432,.T.);
#50561=EDGE_CURVE('',#39237,#38840,#22341,.T.);
#50562=EDGE_CURVE('',#38852,#39238,#22342,.T.);
#50563=EDGE_CURVE('',#39238,#39239,#32433,.T.);
#50564=EDGE_CURVE('',#39239,#38848,#22343,.T.);
#50565=EDGE_CURVE('',#38843,#39240,#22344,.T.);
#50566=EDGE_CURVE('',#39240,#39241,#32434,.T.);
#50567=EDGE_CURVE('',#39241,#38847,#22345,.T.);
#50568=EDGE_CURVE('',#38803,#39242,#22346,.T.);
#50569=EDGE_CURVE('',#39242,#39243,#32435,.T.);
#50570=EDGE_CURVE('',#39243,#38801,#22347,.T.);
#50571=EDGE_CURVE('',#38808,#39244,#22348,.T.);
#50572=EDGE_CURVE('',#39244,#39245,#32436,.T.);
#50573=EDGE_CURVE('',#39245,#38804,#22349,.T.);
#50574=EDGE_CURVE('',#38815,#39246,#22350,.T.);
#50575=EDGE_CURVE('',#39246,#39247,#32437,.T.);
#50576=EDGE_CURVE('',#39247,#38819,#22351,.T.);
#50577=EDGE_CURVE('',#38807,#39248,#22352,.T.);
#50578=EDGE_CURVE('',#39248,#39249,#32438,.T.);
#50579=EDGE_CURVE('',#39249,#38811,#22353,.T.);
#50580=EDGE_CURVE('',#38653,#39250,#22354,.T.);
#50581=EDGE_CURVE('',#39250,#39251,#32439,.T.);
#50582=EDGE_CURVE('',#39251,#38657,#22355,.T.);
#50583=EDGE_CURVE('',#38649,#39252,#22356,.T.);
#50584=EDGE_CURVE('',#39252,#39253,#32440,.T.);
#50585=EDGE_CURVE('',#39253,#38647,#22357,.T.);
#50586=EDGE_CURVE('',#38654,#39254,#22358,.T.);
#50587=EDGE_CURVE('',#39254,#39255,#32441,.T.);
#50588=EDGE_CURVE('',#39255,#38650,#22359,.T.);
#50589=EDGE_CURVE('',#38661,#39256,#22360,.T.);
#50590=EDGE_CURVE('',#39256,#39257,#32442,.T.);
#50591=EDGE_CURVE('',#39257,#38658,#22361,.T.);
#50592=EDGE_CURVE('',#38717,#39258,#22362,.T.);
#50593=EDGE_CURVE('',#39258,#39259,#32443,.T.);
#50594=EDGE_CURVE('',#39259,#38714,#22363,.T.);
#50595=EDGE_CURVE('',#38709,#39260,#22364,.T.);
#50596=EDGE_CURVE('',#39260,#39261,#32444,.T.);
#50597=EDGE_CURVE('',#39261,#38713,#22365,.T.);
#50598=EDGE_CURVE('',#38705,#39262,#22366,.T.);
#50599=EDGE_CURVE('',#39262,#39263,#32445,.T.);
#50600=EDGE_CURVE('',#39263,#38703,#22367,.T.);
#50601=EDGE_CURVE('',#38710,#39264,#22368,.T.);
#50602=EDGE_CURVE('',#39264,#39265,#32446,.T.);
#50603=EDGE_CURVE('',#39265,#38706,#22369,.T.);
#50604=EDGE_CURVE('',#38737,#39266,#22370,.T.);
#50605=EDGE_CURVE('',#39266,#39267,#32447,.T.);
#50606=EDGE_CURVE('',#39267,#38735,#22371,.T.);
#50607=EDGE_CURVE('',#38742,#39268,#22372,.T.);
#50608=EDGE_CURVE('',#39268,#39269,#32448,.T.);
#50609=EDGE_CURVE('',#39269,#38738,#22373,.T.);
#50610=EDGE_CURVE('',#38749,#39270,#22374,.T.);
#50611=EDGE_CURVE('',#39270,#39271,#32449,.T.);
#50612=EDGE_CURVE('',#39271,#38746,#22375,.T.);
#50613=EDGE_CURVE('',#38741,#39272,#22376,.T.);
#50614=EDGE_CURVE('',#39272,#39273,#32450,.T.);
#50615=EDGE_CURVE('',#39273,#38745,#22377,.T.);
#50616=EDGE_CURVE('',#38928,#39274,#22378,.T.);
#50617=EDGE_CURVE('',#39274,#39275,#32451,.T.);
#50618=EDGE_CURVE('',#39275,#38924,#22379,.T.);
#50619=EDGE_CURVE('',#38927,#39276,#22380,.T.);
#50620=EDGE_CURVE('',#39276,#39277,#32452,.T.);
#50621=EDGE_CURVE('',#39277,#38931,#22381,.T.);
#50622=EDGE_CURVE('',#38923,#39278,#22382,.T.);
#50623=EDGE_CURVE('',#39278,#39279,#32453,.T.);
#50624=EDGE_CURVE('',#39279,#38921,#22383,.T.);
#50625=EDGE_CURVE('',#38828,#39280,#22384,.T.);
#50626=EDGE_CURVE('',#39280,#39281,#32454,.T.);
#50627=EDGE_CURVE('',#39281,#38824,#22385,.T.);
#50628=EDGE_CURVE('',#38835,#39282,#22386,.T.);
#50629=EDGE_CURVE('',#39282,#39283,#32455,.T.);
#50630=EDGE_CURVE('',#39283,#38832,#22387,.T.);
#50631=EDGE_CURVE('',#38827,#39284,#22388,.T.);
#50632=EDGE_CURVE('',#39284,#39285,#32456,.T.);
#50633=EDGE_CURVE('',#39285,#38831,#22389,.T.);
#50634=EDGE_CURVE('',#38823,#39286,#22390,.T.);
#50635=EDGE_CURVE('',#39286,#39287,#32457,.T.);
#50636=EDGE_CURVE('',#39287,#38821,#22391,.T.);
#50637=EDGE_CURVE('',#38791,#39288,#22392,.T.);
#50638=EDGE_CURVE('',#39288,#39289,#32458,.T.);
#50639=EDGE_CURVE('',#39289,#38795,#22393,.T.);
#50640=EDGE_CURVE('',#38787,#39290,#22394,.T.);
#50641=EDGE_CURVE('',#39290,#39291,#32459,.T.);
#50642=EDGE_CURVE('',#39291,#38785,#22395,.T.);
#50643=EDGE_CURVE('',#38792,#39292,#22396,.T.);
#50644=EDGE_CURVE('',#39292,#39293,#32460,.T.);
#50645=EDGE_CURVE('',#39293,#38788,#22397,.T.);
#50646=EDGE_CURVE('',#38799,#39294,#22398,.T.);
#50647=EDGE_CURVE('',#39294,#39295,#32461,.T.);
#50648=EDGE_CURVE('',#39295,#38796,#22399,.T.);
#50649=EDGE_CURVE('',#38725,#39296,#22400,.T.);
#50650=EDGE_CURVE('',#39296,#39297,#32462,.T.);
#50651=EDGE_CURVE('',#39297,#38729,#22401,.T.);
#50652=EDGE_CURVE('',#38721,#39298,#22402,.T.);
#50653=EDGE_CURVE('',#39298,#39299,#32463,.T.);
#50654=EDGE_CURVE('',#39299,#38719,#22403,.T.);
#50655=EDGE_CURVE('',#38726,#39300,#22404,.T.);
#50656=EDGE_CURVE('',#39300,#39301,#32464,.T.);
#50657=EDGE_CURVE('',#39301,#38722,#22405,.T.);
#50658=EDGE_CURVE('',#38733,#39302,#22406,.T.);
#50659=EDGE_CURVE('',#39302,#39303,#32465,.T.);
#50660=EDGE_CURVE('',#39303,#38730,#22407,.T.);
#50661=EDGE_CURVE('',#38633,#39304,#22408,.T.);
#50662=EDGE_CURVE('',#39304,#39305,#32466,.T.);
#50663=EDGE_CURVE('',#39305,#38631,#22409,.T.);
#50664=EDGE_CURVE('',#38638,#39306,#22410,.T.);
#50665=EDGE_CURVE('',#39306,#39307,#32467,.T.);
#50666=EDGE_CURVE('',#39307,#38634,#22411,.T.);
#50667=EDGE_CURVE('',#38645,#39308,#22412,.T.);
#50668=EDGE_CURVE('',#39308,#39309,#32468,.T.);
#50669=EDGE_CURVE('',#39309,#38642,#22413,.T.);
#50670=EDGE_CURVE('',#38637,#39310,#22414,.T.);
#50671=EDGE_CURVE('',#39310,#39311,#32469,.T.);
#50672=EDGE_CURVE('',#39311,#38641,#22415,.T.);
#50673=EDGE_CURVE('',#38597,#39312,#22416,.T.);
#50674=EDGE_CURVE('',#39312,#39313,#32470,.T.);
#50675=EDGE_CURVE('',#39313,#38595,#22417,.T.);
#50676=EDGE_CURVE('',#38602,#39314,#22418,.T.);
#50677=EDGE_CURVE('',#39314,#39315,#32471,.T.);
#50678=EDGE_CURVE('',#39315,#38598,#22419,.T.);
#50679=EDGE_CURVE('',#38609,#39316,#22420,.T.);
#50680=EDGE_CURVE('',#39316,#39317,#32472,.T.);
#50681=EDGE_CURVE('',#39317,#38606,#22421,.T.);
#50682=EDGE_CURVE('',#38601,#39318,#22422,.T.);
#50683=EDGE_CURVE('',#39318,#39319,#32473,.T.);
#50684=EDGE_CURVE('',#39319,#38605,#22423,.T.);
#50685=EDGE_CURVE('',#38613,#39320,#22424,.T.);
#50686=EDGE_CURVE('',#39320,#39321,#32474,.T.);
#50687=EDGE_CURVE('',#39321,#38611,#22425,.T.);
#50688=EDGE_CURVE('',#38618,#39322,#22426,.T.);
#50689=EDGE_CURVE('',#39322,#39323,#32475,.T.);
#50690=EDGE_CURVE('',#39323,#38614,#22427,.T.);
#50691=EDGE_CURVE('',#38626,#39324,#22428,.T.);
#50692=EDGE_CURVE('',#39324,#39325,#32476,.T.);
#50693=EDGE_CURVE('',#39325,#38622,#22429,.T.);
#50694=EDGE_CURVE('',#38617,#39326,#22430,.T.);
#50695=EDGE_CURVE('',#39326,#39327,#32477,.T.);
#50696=EDGE_CURVE('',#39327,#38621,#22431,.T.);
#50697=EDGE_CURVE('',#38460,#39328,#22432,.T.);
#50698=EDGE_CURVE('',#39328,#39329,#32478,.T.);
#50699=EDGE_CURVE('',#39329,#38456,#22433,.T.);
#50700=EDGE_CURVE('',#38459,#39330,#22434,.T.);
#50701=EDGE_CURVE('',#39330,#39331,#32479,.T.);
#50702=EDGE_CURVE('',#39331,#38463,#22435,.T.);
#50703=EDGE_CURVE('',#39332,#39333,#32480,.T.);
#50704=EDGE_CURVE('',#39333,#38447,#22436,.T.);
#50705=EDGE_CURVE('',#38446,#39332,#22437,.T.);
#50706=EDGE_CURVE('',#38452,#39334,#22438,.T.);
#50707=EDGE_CURVE('',#39334,#39335,#32481,.T.);
#50708=EDGE_CURVE('',#39335,#38448,#22439,.T.);
#50709=EDGE_CURVE('',#38863,#39336,#22440,.T.);
#50710=EDGE_CURVE('',#39336,#39337,#32482,.T.);
#50711=EDGE_CURVE('',#39337,#38867,#22441,.T.);
#50712=EDGE_CURVE('',#38859,#39338,#22442,.T.);
#50713=EDGE_CURVE('',#39338,#39339,#32483,.T.);
#50714=EDGE_CURVE('',#39339,#38857,#22443,.T.);
#50715=EDGE_CURVE('',#38864,#39340,#22444,.T.);
#50716=EDGE_CURVE('',#39340,#39341,#32484,.T.);
#50717=EDGE_CURVE('',#39341,#38860,#22445,.T.);
#50718=EDGE_CURVE('',#38871,#39342,#22446,.T.);
#50719=EDGE_CURVE('',#39342,#39343,#32485,.T.);
#50720=EDGE_CURVE('',#39343,#38868,#22447,.T.);
#50721=EDGE_CURVE('',#38553,#39344,#22448,.T.);
#50722=EDGE_CURVE('',#39344,#39345,#32486,.T.);
#50723=EDGE_CURVE('',#39345,#38557,#22449,.T.);
#50724=EDGE_CURVE('',#38549,#39346,#22450,.T.);
#50725=EDGE_CURVE('',#39346,#39347,#32487,.T.);
#50726=EDGE_CURVE('',#39347,#38547,#22451,.T.);
#50727=EDGE_CURVE('',#38554,#39348,#22452,.T.);
#50728=EDGE_CURVE('',#39348,#39349,#32488,.T.);
#50729=EDGE_CURVE('',#39349,#38550,#22453,.T.);
#50730=EDGE_CURVE('',#38561,#39350,#22454,.T.);
#50731=EDGE_CURVE('',#39350,#39351,#32489,.T.);
#50732=EDGE_CURVE('',#39351,#38558,#22455,.T.);
#50733=EDGE_CURVE('',#38537,#39352,#22456,.T.);
#50734=EDGE_CURVE('',#39352,#39353,#32490,.T.);
#50735=EDGE_CURVE('',#39353,#38541,#22457,.T.);
#50736=EDGE_CURVE('',#38533,#39354,#22458,.T.);
#50737=EDGE_CURVE('',#39354,#39355,#32491,.T.);
#50738=EDGE_CURVE('',#39355,#38531,#22459,.T.);
#50739=EDGE_CURVE('',#38538,#39356,#22460,.T.);
#50740=EDGE_CURVE('',#39356,#39357,#32492,.T.);
#50741=EDGE_CURVE('',#39357,#38534,#22461,.T.);
#50742=EDGE_CURVE('',#38545,#39358,#22462,.T.);
#50743=EDGE_CURVE('',#39358,#39359,#32493,.T.);
#50744=EDGE_CURVE('',#39359,#38542,#22463,.T.);
#50745=EDGE_CURVE('',#38753,#39360,#22464,.T.);
#50746=EDGE_CURVE('',#39360,#39361,#32494,.T.);
#50747=EDGE_CURVE('',#39361,#38751,#22465,.T.);
#50748=EDGE_CURVE('',#38758,#39362,#22466,.T.);
#50749=EDGE_CURVE('',#39362,#39363,#32495,.T.);
#50750=EDGE_CURVE('',#39363,#38754,#22467,.T.);
#50751=EDGE_CURVE('',#38765,#39364,#22468,.T.);
#50752=EDGE_CURVE('',#39364,#39365,#32496,.T.);
#50753=EDGE_CURVE('',#39365,#38762,#22469,.T.);
#50754=EDGE_CURVE('',#38757,#39366,#22470,.T.);
#50755=EDGE_CURVE('',#39366,#39367,#32497,.T.);
#50756=EDGE_CURVE('',#39367,#38761,#22471,.T.);
#50757=EDGE_CURVE('',#38880,#39368,#22472,.T.);
#50758=EDGE_CURVE('',#39368,#39369,#32498,.T.);
#50759=EDGE_CURVE('',#39369,#38876,#22473,.T.);
#50760=EDGE_CURVE('',#38887,#39370,#22474,.T.);
#50761=EDGE_CURVE('',#39370,#39371,#32499,.T.);
#50762=EDGE_CURVE('',#39371,#38884,#22475,.T.);
#50763=EDGE_CURVE('',#38879,#39372,#22476,.T.);
#50764=EDGE_CURVE('',#39372,#39373,#32500,.T.);
#50765=EDGE_CURVE('',#39373,#38883,#22477,.T.);
#50766=EDGE_CURVE('',#38875,#39374,#22478,.T.);
#50767=EDGE_CURVE('',#39374,#39375,#32501,.T.);
#50768=EDGE_CURVE('',#39375,#38873,#22479,.T.);
#50769=EDGE_CURVE('',#38479,#39376,#22480,.T.);
#50770=EDGE_CURVE('',#39376,#39377,#32502,.T.);
#50771=EDGE_CURVE('',#39377,#38476,#22481,.T.);
#50772=EDGE_CURVE('',#38471,#39378,#22482,.T.);
#50773=EDGE_CURVE('',#39378,#39379,#32503,.T.);
#50774=EDGE_CURVE('',#39379,#38475,#22483,.T.);
#50775=EDGE_CURVE('',#39380,#39381,#32504,.T.);
#50776=EDGE_CURVE('',#39381,#38467,#22484,.T.);
#50777=EDGE_CURVE('',#38466,#39380,#22485,.T.);
#50778=EDGE_CURVE('',#38472,#39382,#22486,.T.);
#50779=EDGE_CURVE('',#39382,#39383,#32505,.T.);
#50780=EDGE_CURVE('',#39383,#38468,#22487,.T.);
#50781=EDGE_CURVE('',#38895,#39384,#22488,.T.);
#50782=EDGE_CURVE('',#39384,#39385,#32506,.T.);
#50783=EDGE_CURVE('',#39385,#38899,#22489,.T.);
#50784=EDGE_CURVE('',#38891,#39386,#22490,.T.);
#50785=EDGE_CURVE('',#39386,#39387,#32507,.T.);
#50786=EDGE_CURVE('',#39387,#38889,#22491,.T.);
#50787=EDGE_CURVE('',#38896,#39388,#22492,.T.);
#50788=EDGE_CURVE('',#39388,#39389,#32508,.T.);
#50789=EDGE_CURVE('',#39389,#38892,#22493,.T.);
#50790=EDGE_CURVE('',#38903,#39390,#22494,.T.);
#50791=EDGE_CURVE('',#39390,#39391,#32509,.T.);
#50792=EDGE_CURVE('',#39391,#38900,#22495,.T.);
#50793=EDGE_CURVE('',#38503,#39392,#22496,.T.);
#50794=EDGE_CURVE('',#39392,#39393,#32510,.T.);
#50795=EDGE_CURVE('',#39393,#38507,#22497,.T.);
#50796=EDGE_CURVE('',#38499,#39394,#22498,.T.);
#50797=EDGE_CURVE('',#39394,#39395,#32511,.T.);
#50798=EDGE_CURVE('',#39395,#38497,#22499,.T.);
#50799=EDGE_CURVE('',#38504,#39396,#22500,.T.);
#50800=EDGE_CURVE('',#39396,#39397,#32512,.T.);
#50801=EDGE_CURVE('',#39397,#38500,#22501,.T.);
#50802=EDGE_CURVE('',#38511,#39398,#22502,.T.);
#50803=EDGE_CURVE('',#39398,#39399,#32513,.T.);
#50804=EDGE_CURVE('',#39399,#38508,#22503,.T.);
#50805=EDGE_CURVE('',#38912,#39400,#22504,.T.);
#50806=EDGE_CURVE('',#39400,#39401,#32514,.T.);
#50807=EDGE_CURVE('',#39401,#38908,#22505,.T.);
#50808=EDGE_CURVE('',#38919,#39402,#22506,.T.);
#50809=EDGE_CURVE('',#39402,#39403,#32515,.T.);
#50810=EDGE_CURVE('',#39403,#38916,#22507,.T.);
#50811=EDGE_CURVE('',#38911,#39404,#22508,.T.);
#50812=EDGE_CURVE('',#39404,#39405,#32516,.T.);
#50813=EDGE_CURVE('',#39405,#38915,#22509,.T.);
#50814=EDGE_CURVE('',#38907,#39406,#22510,.T.);
#50815=EDGE_CURVE('',#39406,#39407,#32517,.T.);
#50816=EDGE_CURVE('',#39407,#38905,#22511,.T.);
#50817=EDGE_CURVE('',#38495,#39408,#22512,.T.);
#50818=EDGE_CURVE('',#39408,#39409,#32518,.T.);
#50819=EDGE_CURVE('',#39409,#38492,#22513,.T.);
#50820=EDGE_CURVE('',#38487,#39410,#22514,.T.);
#50821=EDGE_CURVE('',#39410,#39411,#32519,.T.);
#50822=EDGE_CURVE('',#39411,#38491,#22515,.T.);
#50823=EDGE_CURVE('',#39412,#39413,#32520,.T.);
#50824=EDGE_CURVE('',#39413,#38483,#22516,.T.);
#50825=EDGE_CURVE('',#38482,#39412,#22517,.T.);
#50826=EDGE_CURVE('',#38488,#39414,#22518,.T.);
#50827=EDGE_CURVE('',#39414,#39415,#32521,.T.);
#50828=EDGE_CURVE('',#39415,#38484,#22519,.T.);
#50829=EDGE_CURVE('',#39001,#39416,#22520,.T.);
#50830=EDGE_CURVE('',#39416,#39417,#32522,.T.);
#50831=EDGE_CURVE('',#39417,#39003,#22521,.T.);
#50832=EDGE_CURVE('',#39029,#39418,#22522,.T.);
#50833=EDGE_CURVE('',#39418,#39419,#32523,.T.);
#50834=EDGE_CURVE('',#39419,#39031,#22523,.T.);
#50835=EDGE_CURVE('',#39017,#39420,#22524,.T.);
#50836=EDGE_CURVE('',#39420,#39421,#32524,.T.);
#50837=EDGE_CURVE('',#39421,#39019,#22525,.T.);
#50838=EDGE_CURVE('',#39422,#39423,#32525,.T.);
#50839=EDGE_CURVE('',#39423,#39015,#22526,.T.);
#50840=EDGE_CURVE('',#39013,#39422,#22527,.T.);
#50841=EDGE_CURVE('',#39033,#39424,#22528,.T.);
#50842=EDGE_CURVE('',#39424,#39425,#32526,.T.);
#50843=EDGE_CURVE('',#39425,#39035,#22529,.T.);
#50844=EDGE_CURVE('',#39426,#39427,#32527,.T.);
#50845=EDGE_CURVE('',#39427,#39026,#22530,.T.);
#50846=EDGE_CURVE('',#39025,#39426,#22531,.T.);
#50847=EDGE_CURVE('',#39005,#39428,#22532,.T.);
#50848=EDGE_CURVE('',#39428,#39429,#32528,.T.);
#50849=EDGE_CURVE('',#39429,#39006,#22533,.T.);
#50850=EDGE_CURVE('',#38669,#39430,#22534,.T.);
#50851=EDGE_CURVE('',#39430,#39431,#32529,.T.);
#50852=EDGE_CURVE('',#39431,#38673,#22535,.T.);
#50853=EDGE_CURVE('',#38689,#39432,#22536,.T.);
#50854=EDGE_CURVE('',#39432,#39433,#32530,.T.);
#50855=EDGE_CURVE('',#39433,#38693,#22537,.T.);
#50856=EDGE_CURVE('',#38781,#39434,#22538,.T.);
#50857=EDGE_CURVE('',#39434,#39180,#32531,.T.);
#50858=EDGE_CURVE('',#39199,#39435,#32532,.T.);
#50859=EDGE_CURVE('',#39435,#38524,#22539,.T.);
#50860=EDGE_CURVE('',#39207,#39434,#32533,.T.);
#50861=EDGE_CURVE('',#39435,#39204,#32534,.T.);
#50862=EDGE_CURVE('',#39424,#39419,#32535,.T.);
#50863=EDGE_CURVE('',#39418,#39427,#22540,.T.);
#50864=EDGE_CURVE('',#39428,#39417,#22541,.T.);
#50865=EDGE_CURVE('',#39416,#39167,#32536,.T.);
#50866=EDGE_CURVE('',#39433,#39182,#32537,.T.);
#50867=EDGE_CURVE('',#39420,#39423,#32538,.T.);
#50868=EDGE_CURVE('',#39421,#39176,#22542,.T.);
#50869=EDGE_CURVE('',#39175,#39162,#22543,.T.);
#50870=EDGE_CURVE('',#39172,#39163,#32539,.T.);
#50871=EDGE_CURVE('',#39191,#39430,#32540,.T.);
#50872=EDGE_CURVE('',#39224,#39219,#22544,.T.);
#50873=EDGE_CURVE('',#39320,#39323,#22545,.T.);
#50874=EDGE_CURVE('',#39312,#39315,#22546,.T.);
#50875=EDGE_CURVE('',#39232,#39227,#22547,.T.);
#50876=EDGE_CURVE('',#39304,#39307,#22548,.T.);
#50877=EDGE_CURVE('',#39256,#39251,#22549,.T.);
#50878=EDGE_CURVE('',#39296,#39299,#22550,.T.);
#50879=EDGE_CURVE('',#39264,#39259,#22551,.T.);
#50880=EDGE_CURVE('',#39248,#39243,#22552,.T.);
#50881=EDGE_CURVE('',#39280,#39283,#22553,.T.);
#50882=EDGE_CURVE('',#39288,#39291,#22554,.T.);
#50883=EDGE_CURVE('',#39272,#39267,#22555,.T.);
#50884=EDGE_CURVE('',#39274,#39277,#22556,.T.);
#50885=EDGE_CURVE('',#39240,#39235,#22557,.T.);
#50886=EDGE_CURVE('',#39216,#39213,#22558,.T.);
#50887=EDGE_CURVE('',#39328,#39331,#22559,.T.);
#50888=EDGE_CURVE('',#39376,#39379,#22560,.T.);
#50889=EDGE_CURVE('',#39332,#39335,#22561,.T.);
#50890=EDGE_CURVE('',#39220,#39223,#22562,.T.);
#50891=EDGE_CURVE('',#39350,#39345,#22563,.T.);
#50892=EDGE_CURVE('',#39236,#39239,#22564,.T.);
#50893=EDGE_CURVE('',#39336,#39339,#22565,.T.);
#50894=EDGE_CURVE('',#39228,#39231,#22566,.T.);
#50895=EDGE_CURVE('',#39358,#39353,#22567,.T.);
#50896=EDGE_CURVE('',#39252,#39255,#22568,.T.);
#50897=EDGE_CURVE('',#39192,#39195,#22569,.T.);
#50898=EDGE_CURVE('',#39260,#39263,#22570,.T.);
#50899=EDGE_CURVE('',#39186,#39189,#22571,.T.);
#50900=EDGE_CURVE('',#39284,#39287,#22572,.T.);
#50901=EDGE_CURVE('',#39368,#39371,#22573,.T.);
#50902=EDGE_CURVE('',#39268,#39271,#22574,.T.);
#50903=EDGE_CURVE('',#39366,#39361,#22575,.T.);
#50904=EDGE_CURVE('',#39436,#39437,#22576,.T.);
#50905=EDGE_CURVE('',#39438,#39437,#22577,.T.);
#50906=EDGE_CURVE('',#39439,#39438,#22578,.T.);
#50907=EDGE_CURVE('',#39436,#39439,#22579,.T.);
#50908=EDGE_CURVE('',#39440,#39441,#22580,.T.);
#50909=EDGE_CURVE('',#39437,#39441,#22581,.T.);
#50910=EDGE_CURVE('',#39440,#39436,#22582,.T.);
#50911=EDGE_CURVE('',#39442,#39438,#22583,.T.);
#50912=EDGE_CURVE('',#39442,#39443,#22584,.T.);
#50913=EDGE_CURVE('',#39439,#39443,#22585,.T.);
#50914=EDGE_CURVE('',#39408,#39411,#22586,.T.);
#50915=EDGE_CURVE('',#39380,#39383,#22587,.T.);
#50916=EDGE_CURVE('',#39346,#39349,#22588,.T.);
#50917=EDGE_CURVE('',#39398,#39393,#22589,.T.);
#50918=EDGE_CURVE('',#39340,#39343,#22590,.T.);
#50919=EDGE_CURVE('',#39384,#39387,#22591,.T.);
#50920=EDGE_CURVE('',#39354,#39357,#22592,.T.);
#50921=EDGE_CURVE('',#39198,#39201,#22593,.T.);
#50922=EDGE_CURVE('',#39196,#39431,#22594,.T.);
#50923=EDGE_CURVE('',#39432,#39185,#22595,.T.);
#50924=EDGE_CURVE('',#39372,#39375,#22596,.T.);
#50925=EDGE_CURVE('',#39400,#39403,#22597,.T.);
#50926=EDGE_CURVE('',#39362,#39365,#22598,.T.);
#50927=EDGE_CURVE('',#39210,#39181,#22599,.T.);
#50928=EDGE_CURVE('',#39202,#39205,#22600,.T.);
#50929=EDGE_CURVE('',#39404,#39407,#22601,.T.);
#50930=EDGE_CURVE('',#39206,#39209,#22602,.T.);
#50931=EDGE_CURVE('',#39164,#39425,#22603,.T.);
#50932=EDGE_CURVE('',#39422,#39179,#22604,.T.);
#50933=EDGE_CURVE('',#39394,#39397,#22605,.T.);
#50934=EDGE_CURVE('',#39412,#39415,#22606,.T.);
#50935=EDGE_CURVE('',#39388,#39391,#22607,.T.);
#50936=EDGE_CURVE('',#39444,#39445,#22608,.T.);
#50937=EDGE_CURVE('',#39445,#39446,#32541,.T.);
#50938=EDGE_CURVE('',#39447,#39446,#22609,.T.);
#50939=EDGE_CURVE('',#39444,#39447,#32542,.T.);
#50940=EDGE_CURVE('',#39448,#39446,#32543,.T.);
#50941=EDGE_CURVE('',#39449,#39448,#22610,.T.);
#50942=EDGE_CURVE('',#39447,#39449,#32544,.T.);
#50943=EDGE_CURVE('',#39448,#39450,#32545,.T.);
#50944=EDGE_CURVE('',#39451,#39450,#22611,.T.);
#50945=EDGE_CURVE('',#39449,#39451,#32546,.T.);
#50946=EDGE_CURVE('',#39450,#39452,#32547,.T.);
#50947=EDGE_CURVE('',#39453,#39452,#22612,.T.);
#50948=EDGE_CURVE('',#39451,#39453,#32548,.T.);
#50949=EDGE_CURVE('',#39452,#39454,#32549,.T.);
#50950=EDGE_CURVE('',#39455,#39454,#22613,.T.);
#50951=EDGE_CURVE('',#39453,#39455,#32550,.T.);
#50952=EDGE_CURVE('',#39456,#39454,#32551,.T.);
#50953=EDGE_CURVE('',#39457,#39456,#22614,.T.);
#50954=EDGE_CURVE('',#39455,#39457,#32552,.T.);
#50955=EDGE_CURVE('',#39456,#39458,#32553,.T.);
#50956=EDGE_CURVE('',#39459,#39458,#22615,.T.);
#50957=EDGE_CURVE('',#39457,#39459,#32554,.T.);
#50958=EDGE_CURVE('',#39460,#39461,#22616,.T.);
#50959=EDGE_CURVE('',#39462,#39461,#32555,.T.);
#50960=EDGE_CURVE('',#39462,#39463,#22617,.T.);
#50961=EDGE_CURVE('',#39460,#39463,#5576,.T.);
#50962=EDGE_CURVE('',#39464,#39460,#5577,.T.);
#50963=EDGE_CURVE('',#39464,#39461,#22618,.T.);
#50964=EDGE_CURVE('',#39465,#39466,#32556,.T.);
#50965=EDGE_CURVE('',#39466,#39467,#5578,.T.);
#50966=EDGE_CURVE('',#39467,#39465,#22619,.T.);
#50967=EDGE_CURVE('',#39468,#39467,#5579,.T.);
#50968=EDGE_CURVE('',#39468,#39465,#22620,.T.);
#50969=EDGE_CURVE('',#39469,#39470,#1222,.T.);
#50970=EDGE_CURVE('',#39469,#39471,#22621,.T.);
#50971=EDGE_CURVE('',#39472,#39471,#22622,.T.);
#50972=EDGE_CURVE('',#39472,#39470,#5580,.T.);
#50973=EDGE_CURVE('',#39473,#39474,#1223,.T.);
#50974=EDGE_CURVE('',#39473,#39475,#5581,.T.);
#50975=EDGE_CURVE('',#39476,#39475,#22623,.T.);
#50976=EDGE_CURVE('',#39474,#39476,#22624,.T.);
#50977=EDGE_CURVE('',#39474,#39469,#32557,.T.);
#50978=EDGE_CURVE('',#39471,#39476,#32558,.T.);
#50979=EDGE_CURVE('',#39477,#39478,#1224,.T.);
#50980=EDGE_CURVE('',#39477,#39479,#5582,.T.);
#50981=EDGE_CURVE('',#39480,#39479,#22625,.T.);
#50982=EDGE_CURVE('',#39478,#39480,#22626,.T.);
#50983=EDGE_CURVE('',#39481,#39482,#1225,.T.);
#50984=EDGE_CURVE('',#39481,#39483,#22627,.T.);
#50985=EDGE_CURVE('',#39484,#39483,#22628,.T.);
#50986=EDGE_CURVE('',#39484,#39482,#5583,.T.);
#50987=EDGE_CURVE('',#39478,#39481,#32559,.T.);
#50988=EDGE_CURVE('',#39483,#39480,#32560,.T.);
#50989=EDGE_CURVE('',#39485,#39486,#32561,.T.);
#50990=EDGE_CURVE('',#39487,#39486,#22629,.T.);
#50991=EDGE_CURVE('',#39488,#39487,#32562,.T.);
#50992=EDGE_CURVE('',#39488,#39485,#22630,.T.);
#50993=EDGE_CURVE('',#39489,#39490,#32563,.T.);
#50994=EDGE_CURVE('',#39491,#39490,#22631,.T.);
#50995=EDGE_CURVE('',#39492,#39491,#32564,.T.);
#50996=EDGE_CURVE('',#39492,#39489,#22632,.T.);
#50997=EDGE_CURVE('',#39490,#39493,#32565,.T.);
#50998=EDGE_CURVE('',#39494,#39493,#22633,.T.);
#50999=EDGE_CURVE('',#39491,#39494,#32566,.T.);
#51000=EDGE_CURVE('',#39493,#39495,#32567,.T.);
#51001=EDGE_CURVE('',#39496,#39495,#22634,.T.);
#51002=EDGE_CURVE('',#39494,#39496,#32568,.T.);
#51003=EDGE_CURVE('',#39497,#39498,#5584,.T.);
#51004=EDGE_CURVE('',#39496,#39497,#32569,.T.);
#51005=EDGE_CURVE('',#39495,#39498,#32570,.T.);
#51006=EDGE_CURVE('',#39499,#39500,#32571,.T.);
#51007=EDGE_CURVE('',#39501,#39500,#22635,.T.);
#51008=EDGE_CURVE('',#39502,#39501,#32572,.T.);
#51009=EDGE_CURVE('',#39502,#39499,#22636,.T.);
#51010=EDGE_CURVE('',#39500,#39485,#32573,.T.);
#51011=EDGE_CURVE('',#39501,#39488,#32574,.T.);
#51012=EDGE_CURVE('',#39503,#39504,#5585,.T.);
#51013=EDGE_CURVE('',#39503,#39505,#5586,.T.);
#51014=EDGE_CURVE('',#39506,#39505,#5587,.T.);
#51015=EDGE_CURVE('',#39506,#39507,#5588,.T.);
#51016=EDGE_CURVE('',#39504,#39507,#5589,.T.);
#51017=EDGE_CURVE('',#39508,#39509,#5590,.T.);
#51018=EDGE_CURVE('',#39508,#39510,#5591,.T.);
#51019=EDGE_CURVE('',#39510,#39511,#5592,.T.);
#51020=EDGE_CURVE('',#39511,#39512,#5593,.T.);
#51021=EDGE_CURVE('',#39509,#39512,#5594,.T.);
#51022=EDGE_CURVE('',#39513,#39514,#5595,.T.);
#51023=EDGE_CURVE('',#39513,#39515,#5596,.T.);
#51024=EDGE_CURVE('',#39516,#39515,#5597,.T.);
#51025=EDGE_CURVE('',#39516,#39517,#5598,.T.);
#51026=EDGE_CURVE('',#39514,#39517,#5599,.T.);
#51027=EDGE_CURVE('',#39518,#39519,#5600,.T.);
#51028=EDGE_CURVE('',#39518,#39520,#5601,.T.);
#51029=EDGE_CURVE('',#39520,#39521,#5602,.T.);
#51030=EDGE_CURVE('',#39521,#39522,#5603,.T.);
#51031=EDGE_CURVE('',#39522,#39519,#5604,.T.);
#51032=EDGE_CURVE('',#39523,#39524,#32575,.T.);
#51033=EDGE_CURVE('',#39511,#39524,#22637,.T.);
#51034=EDGE_CURVE('',#39525,#39510,#5605,.T.);
#51035=EDGE_CURVE('',#39525,#39523,#22638,.T.);
#51036=EDGE_CURVE('',#39473,#39525,#5606,.T.);
#51037=EDGE_CURVE('',#39526,#39470,#5607,.T.);
#51038=EDGE_CURVE('',#39526,#39527,#22639,.T.);
#51039=EDGE_CURVE('',#39527,#39523,#32576,.T.);
#51040=EDGE_CURVE('',#39528,#39527,#32577,.T.);
#51041=EDGE_CURVE('',#39526,#39507,#32578,.T.);
#51042=EDGE_CURVE('',#39506,#39528,#22640,.T.);
#51043=EDGE_CURVE('',#39529,#39530,#32579,.T.);
#51044=EDGE_CURVE('',#39521,#39530,#22641,.T.);
#51045=EDGE_CURVE('',#39531,#39520,#32580,.T.);
#51046=EDGE_CURVE('',#39531,#39529,#22642,.T.);
#51047=EDGE_CURVE('',#39532,#39482,#5608,.T.);
#51048=EDGE_CURVE('',#39532,#39533,#22643,.T.);
#51049=EDGE_CURVE('',#39533,#39529,#32581,.T.);
#51050=EDGE_CURVE('',#39477,#39531,#5609,.T.);
#51051=EDGE_CURVE('',#39534,#39533,#32582,.T.);
#51052=EDGE_CURVE('',#39532,#39517,#32583,.T.);
#51053=EDGE_CURVE('',#39516,#39534,#22644,.T.);
#51054=EDGE_CURVE('',#39535,#39536,#32584,.T.);
#51055=EDGE_CURVE('',#39537,#39536,#22645,.T.);
#51056=EDGE_CURVE('',#39538,#39537,#32585,.T.);
#51057=EDGE_CURVE('',#39538,#39535,#22646,.T.);
#51058=EDGE_CURVE('',#39539,#39535,#32586,.T.);
#51059=EDGE_CURVE('',#39540,#39538,#32587,.T.);
#51060=EDGE_CURVE('',#39540,#39539,#22647,.T.);
#51061=EDGE_CURVE('',#39541,#39539,#32588,.T.);
#51062=EDGE_CURVE('',#39542,#39540,#32589,.T.);
#51063=EDGE_CURVE('',#39542,#39541,#22648,.T.);
#51064=EDGE_CURVE('',#39543,#39541,#32590,.T.);
#51065=EDGE_CURVE('',#39544,#39542,#32591,.T.);
#51066=EDGE_CURVE('',#39544,#39543,#22649,.T.);
#51067=EDGE_CURVE('',#39545,#39546,#32592,.T.);
#51068=EDGE_CURVE('',#39547,#39546,#22650,.T.);
#51069=EDGE_CURVE('',#39548,#39547,#32593,.T.);
#51070=EDGE_CURVE('',#39548,#39545,#22651,.T.);
#51071=EDGE_CURVE('',#39549,#39545,#32594,.T.);
#51072=EDGE_CURVE('',#39550,#39548,#32595,.T.);
#51073=EDGE_CURVE('',#39550,#39549,#22652,.T.);
#51074=EDGE_CURVE('',#39536,#39549,#32596,.T.);
#51075=EDGE_CURVE('',#39537,#39550,#32597,.T.);
#51076=EDGE_CURVE('',#39551,#39503,#5610,.T.);
#51077=EDGE_CURVE('',#39551,#39552,#5611,.T.);
#51078=EDGE_CURVE('',#39552,#39505,#5612,.T.);
#51079=EDGE_CURVE('',#39522,#39553,#5613,.T.);
#51080=EDGE_CURVE('',#39553,#39554,#5614,.T.);
#51081=EDGE_CURVE('',#39519,#39554,#5615,.T.);
#51082=EDGE_CURVE('',#39553,#39552,#5616,.T.);
#51083=EDGE_CURVE('',#39530,#39528,#32598,.T.);
#51084=EDGE_CURVE('',#39555,#39513,#32599,.T.);
#51085=EDGE_CURVE('',#39555,#39556,#5617,.T.);
#51086=EDGE_CURVE('',#39556,#39515,#5618,.T.);
#51087=EDGE_CURVE('',#39557,#39499,#32600,.T.);
#51088=EDGE_CURVE('',#39557,#39551,#5619,.T.);
#51089=EDGE_CURVE('',#39504,#39508,#5620,.T.);
#51090=EDGE_CURVE('',#39509,#39558,#32601,.T.);
#51091=EDGE_CURVE('',#39559,#39558,#5621,.T.);
#51092=EDGE_CURVE('',#39486,#39559,#32602,.T.);
#51093=EDGE_CURVE('',#39558,#39560,#5622,.T.);
#51094=EDGE_CURVE('',#39512,#39560,#5623,.T.);
#51095=EDGE_CURVE('',#39484,#39561,#5624,.T.);
#51096=EDGE_CURVE('',#39562,#39479,#5625,.T.);
#51097=EDGE_CURVE('',#39562,#39561,#32603,.T.);
#51098=EDGE_CURVE('',#39562,#39563,#5626,.T.);
#51099=EDGE_CURVE('',#39514,#39518,#5627,.T.);
#51100=EDGE_CURVE('',#39561,#39468,#5628,.T.);
#51101=EDGE_CURVE('',#39564,#39466,#5629,.T.);
#51102=EDGE_CURVE('',#39565,#39564,#5630,.T.);
#51103=EDGE_CURVE('',#39565,#39563,#5631,.T.);
#51104=EDGE_CURVE('',#39566,#39475,#5632,.T.);
#51105=EDGE_CURVE('',#39566,#39567,#32604,.T.);
#51106=EDGE_CURVE('',#39472,#39567,#5633,.T.);
#51107=EDGE_CURVE('',#39566,#39568,#5634,.T.);
#51108=EDGE_CURVE('',#39464,#39567,#5635,.F.);
#51109=EDGE_CURVE('',#39463,#39568,#5636,.T.);
#51110=EDGE_CURVE('',#39569,#39570,#32605,.T.);
#51111=EDGE_CURVE('',#39569,#39570,#5637,.T.);
#51112=EDGE_CURVE('',#39554,#39498,#5638,.T.);
#51113=EDGE_CURVE('',#39571,#39489,#32606,.T.);
#51114=EDGE_CURVE('',#39571,#39555,#5639,.T.);
#51115=EDGE_CURVE('',#39572,#39573,#32607,.T.);
#51116=EDGE_CURVE('',#39572,#39573,#5640,.T.);
#51117=EDGE_CURVE('',#39574,#39575,#32608,.T.);
#51118=EDGE_CURVE('',#39574,#39575,#5641,.T.);
#51119=EDGE_CURVE('',#39576,#39577,#32609,.T.);
#51120=EDGE_CURVE('',#39576,#39577,#5642,.T.);
#51121=EDGE_CURVE('',#39578,#39579,#5643,.T.);
#51122=EDGE_CURVE('',#39579,#39578,#32610,.T.);
#51123=EDGE_CURVE('',#39564,#39580,#32611,.T.);
#51124=EDGE_CURVE('',#39580,#39565,#22653,.T.);
#51125=EDGE_CURVE('',#39581,#39575,#5644,.T.);
#51126=EDGE_CURVE('',#39582,#39581,#32612,.T.);
#51127=EDGE_CURVE('',#39582,#39574,#5645,.T.);
#51128=EDGE_CURVE('',#39583,#39584,#32613,.T.);
#51129=EDGE_CURVE('',#39583,#39572,#5646,.T.);
#51130=EDGE_CURVE('',#39573,#39584,#5647,.T.);
#51131=EDGE_CURVE('',#39585,#39502,#32614,.T.);
#51132=EDGE_CURVE('',#39585,#39557,#5648,.T.);
#51133=EDGE_CURVE('',#39586,#39587,#32615,.T.);
#51134=EDGE_CURVE('',#39586,#39576,#5649,.T.);
#51135=EDGE_CURVE('',#39577,#39587,#5650,.T.);
#51136=EDGE_CURVE('',#39579,#39559,#5651,.T.);
#51137=EDGE_CURVE('',#39578,#39588,#5652,.T.);
#51138=EDGE_CURVE('',#39487,#39588,#32616,.T.);
#51139=EDGE_CURVE('',#39462,#39568,#22654,.T.);
#51140=EDGE_CURVE('',#39580,#39563,#22655,.T.);
#51141=EDGE_CURVE('',#39589,#39583,#5653,.T.);
#51142=EDGE_CURVE('',#39589,#39497,#5654,.T.);
#51143=EDGE_CURVE('',#39590,#39585,#5655,.T.);
#51144=EDGE_CURVE('',#39587,#39590,#5656,.T.);
#51145=EDGE_CURVE('',#39581,#39586,#5657,.T.);
#51146=EDGE_CURVE('',#39584,#39582,#5658,.T.);
#51147=EDGE_CURVE('',#39591,#38451,#22656,.T.);
#51148=EDGE_CURVE('',#39591,#39592,#32617,.T.);
#51149=EDGE_CURVE('',#39592,#38455,#22657,.T.);
#51150=EDGE_CURVE('',#39327,#39593,#32618,.T.);
#51151=EDGE_CURVE('',#39593,#38625,#22658,.T.);
#51152=EDGE_CURVE('',#39593,#39594,#32619,.T.);
#51153=EDGE_CURVE('',#39594,#38629,#22659,.T.);
#51154=EDGE_CURVE('',#39319,#39316,#32620,.T.);
#51155=EDGE_CURVE('',#39595,#38816,#22660,.T.);
#51156=EDGE_CURVE('',#39595,#39596,#32621,.T.);
#51157=EDGE_CURVE('',#39596,#38812,#22661,.T.);
#51158=EDGE_CURVE('',#39596,#39244,#32622,.T.);
#51159=EDGE_CURVE('',#39597,#38851,#22662,.T.);
#51160=EDGE_CURVE('',#39597,#39598,#32623,.T.);
#51161=EDGE_CURVE('',#39598,#38855,#22663,.T.);
#51162=EDGE_CURVE('',#39599,#39599,#32624,.T.);
#51163=EDGE_CURVE('',#39599,#39600,#22664,.T.);
#51164=EDGE_CURVE('',#38294,#39600,#32625,.T.);
#51165=EDGE_CURVE('',#39600,#38296,#32626,.T.);
#51166=EDGE_CURVE('',#39601,#39601,#32627,.T.);
#51167=EDGE_CURVE('',#39601,#38299,#22665,.T.);
#51168=EDGE_CURVE('',#38295,#38293,#32628,.T.);
#51169=EDGE_CURVE('',#39602,#38971,#22666,.T.);
#51170=EDGE_CURVE('',#39603,#39602,#32629,.T.);
#51171=EDGE_CURVE('',#39603,#38973,#22667,.T.);
#51172=EDGE_CURVE('',#39604,#38969,#22668,.T.);
#51173=EDGE_CURVE('',#39602,#39604,#32630,.T.);
#51174=EDGE_CURVE('',#39605,#38967,#22669,.T.);
#51175=EDGE_CURVE('',#39604,#39605,#32631,.T.);
#51176=EDGE_CURVE('',#39606,#38965,#22670,.T.);
#51177=EDGE_CURVE('',#39605,#39606,#32632,.T.);
#51178=EDGE_CURVE('',#39607,#38961,#22671,.T.);
#51179=EDGE_CURVE('',#39606,#39607,#32633,.T.);
#51180=EDGE_CURVE('',#39608,#38963,#22672,.T.);
#51181=EDGE_CURVE('',#39607,#39608,#32634,.T.);
#51182=EDGE_CURVE('',#39609,#39603,#32635,.T.);
#51183=EDGE_CURVE('',#39609,#38975,#22673,.T.);
#51184=EDGE_CURVE('',#39610,#38944,#22674,.T.);
#51185=EDGE_CURVE('',#39610,#39611,#32636,.T.);
#51186=EDGE_CURVE('',#39611,#38946,#22675,.T.);
#51187=EDGE_CURVE('',#39612,#38958,#22676,.T.);
#51188=EDGE_CURVE('',#39612,#39613,#32637,.T.);
#51189=EDGE_CURVE('',#39613,#38956,#22677,.T.);
#51190=EDGE_CURVE('',#39613,#39614,#32638,.T.);
#51191=EDGE_CURVE('',#39614,#38954,#22678,.T.);
#51192=EDGE_CURVE('',#39614,#39615,#32639,.T.);
#51193=EDGE_CURVE('',#39615,#38952,#22679,.T.);
#51194=EDGE_CURVE('',#39615,#39616,#32640,.T.);
#51195=EDGE_CURVE('',#39616,#38950,#22680,.T.);
#51196=EDGE_CURVE('',#39616,#39617,#32641,.T.);
#51197=EDGE_CURVE('',#39617,#38948,#22681,.T.);
#51198=EDGE_CURVE('',#39617,#39610,#32642,.T.);
#51199=EDGE_CURVE('',#39087,#39099,#5659,.T.);
#51200=EDGE_CURVE('',#39085,#39103,#22682,.T.);
#51201=EDGE_CURVE('',#39091,#39135,#22683,.T.);
#51202=EDGE_CURVE('',#39089,#39138,#5660,.T.);
#51203=EDGE_CURVE('',#39066,#39159,#5661,.T.);
#51204=EDGE_CURVE('',#39064,#39153,#22684,.T.);
#51205=EDGE_CURVE('',#39122,#39070,#22685,.T.);
#51206=EDGE_CURVE('',#39068,#39125,#5662,.T.);
#51207=EDGE_CURVE('',#39141,#38364,#22686,.T.);
#51208=EDGE_CURVE('',#39137,#38366,#22687,.T.);
#51209=EDGE_CURVE('',#39097,#38362,#22688,.T.);
#51210=EDGE_CURVE('',#39102,#38360,#22689,.T.);
#51211=EDGE_CURVE('',#39128,#38356,#22690,.T.);
#51212=EDGE_CURVE('',#39124,#38358,#22691,.T.);
#51213=EDGE_CURVE('',#39160,#38352,#22692,.T.);
#51214=EDGE_CURVE('',#39156,#38354,#22693,.T.);
#51215=EDGE_CURVE('',#39048,#39618,#22694,.T.);
#51216=EDGE_CURVE('',#39619,#39618,#32643,.T.);
#51217=EDGE_CURVE('',#39046,#39619,#22695,.T.);
#51218=EDGE_CURVE('',#39620,#39619,#32644,.T.);
#51219=EDGE_CURVE('',#39044,#39620,#22696,.T.);
#51220=EDGE_CURVE('',#39621,#39620,#32645,.T.);
#51221=EDGE_CURVE('',#39040,#39621,#22697,.T.);
#51222=EDGE_CURVE('',#39622,#39621,#32646,.T.);
#51223=EDGE_CURVE('',#39042,#39622,#22698,.T.);
#51224=EDGE_CURVE('',#39054,#39623,#22699,.T.);
#51225=EDGE_CURVE('',#39624,#39623,#32647,.T.);
#51226=EDGE_CURVE('',#39052,#39624,#22700,.T.);
#51227=EDGE_CURVE('',#39625,#39624,#32648,.T.);
#51228=EDGE_CURVE('',#39050,#39625,#22701,.T.);
#51229=EDGE_CURVE('',#39618,#39625,#32649,.T.);
#51230=EDGE_CURVE('',#39594,#39324,#32650,.T.);
#51231=EDGE_CURVE('',#39311,#39308,#32651,.T.);
#51232=EDGE_CURVE('',#39303,#39300,#32652,.T.);
#51233=EDGE_CURVE('',#39295,#39292,#32653,.T.);
#51234=EDGE_CURVE('',#39247,#39595,#32654,.T.);
#51235=EDGE_CURVE('',#39208,#39211,#22702,.T.);
#51236=EDGE_CURVE('',#39402,#39405,#22703,.T.);
#51237=EDGE_CURVE('',#39170,#39173,#22704,.T.);
#51238=EDGE_CURVE('',#39166,#39169,#22705,.T.);
#51239=EDGE_CURVE('',#39406,#39401,#22706,.T.);
#51240=EDGE_CURVE('',#39386,#39389,#22707,.T.);
#51241=EDGE_CURVE('',#39200,#39203,#22708,.T.);
#51242=EDGE_CURVE('',#39396,#39399,#22709,.T.);
#51243=EDGE_CURVE('',#39392,#39395,#22710,.T.);
#51244=EDGE_CURVE('',#39414,#39409,#22711,.T.);
#51245=EDGE_CURVE('',#39413,#39410,#32655,.T.);
#51246=EDGE_CURVE('',#39385,#39390,#32656,.T.);
#51247=EDGE_CURVE('',#39445,#39440,#32657,.T.);
#51248=EDGE_CURVE('',#39441,#39444,#32658,.T.);
#51249=EDGE_CURVE('',#39364,#39367,#22712,.T.);
#51250=EDGE_CURVE('',#39370,#39373,#22713,.T.);
#51251=EDGE_CURVE('',#39184,#39187,#22714,.T.);
#51252=EDGE_CURVE('',#39360,#39363,#22715,.T.);
#51253=EDGE_CURVE('',#39190,#39193,#22716,.T.);
#51254=EDGE_CURVE('',#39188,#39183,#22717,.T.);
#51255=EDGE_CURVE('',#39356,#39359,#22718,.T.);
#51256=EDGE_CURVE('',#39194,#39197,#22719,.T.);
#51257=EDGE_CURVE('',#39374,#39369,#22720,.T.);
#51258=EDGE_CURVE('',#39338,#39341,#22721,.T.);
#51259=EDGE_CURVE('',#39352,#39355,#22722,.T.);
#51260=EDGE_CURVE('',#39348,#39351,#22723,.T.);
#51261=EDGE_CURVE('',#39344,#39347,#22724,.T.);
#51262=EDGE_CURVE('',#39382,#39377,#22725,.T.);
#51263=EDGE_CURVE('',#39381,#39378,#32659,.T.);
#51264=EDGE_CURVE('',#39333,#39591,#32660,.T.);
#51265=EDGE_CURVE('',#39337,#39342,#32661,.T.);
#51266=EDGE_CURVE('',#39598,#39238,#32662,.T.);
#51267=EDGE_CURVE('',#39592,#39330,#32663,.T.);
#51268=EDGE_CURVE('',#39217,#39214,#32664,.T.);
#51269=EDGE_CURVE('',#39241,#39597,#32665,.T.);
#51270=EDGE_CURVE('',#39279,#39276,#32666,.T.);
#51271=EDGE_CURVE('',#39270,#39273,#22726,.T.);
#51272=EDGE_CURVE('',#39290,#39293,#22727,.T.);
#51273=EDGE_CURVE('',#39282,#39285,#22728,.T.);
#51274=EDGE_CURVE('',#39246,#39249,#22729,.T.);
#51275=EDGE_CURVE('',#39262,#39265,#22730,.T.);
#51276=EDGE_CURVE('',#39298,#39301,#22731,.T.);
#51277=EDGE_CURVE('',#39266,#39269,#22732,.T.);
#51278=EDGE_CURVE('',#39294,#39289,#22733,.T.);
#51279=EDGE_CURVE('',#39254,#39257,#22734,.T.);
#51280=EDGE_CURVE('',#39306,#39309,#22735,.T.);
#51281=EDGE_CURVE('',#39258,#39261,#22736,.T.);
#51282=EDGE_CURVE('',#39302,#39297,#22737,.T.);
#51283=EDGE_CURVE('',#39230,#39233,#22738,.T.);
#51284=EDGE_CURVE('',#39314,#39317,#22739,.T.);
#51285=EDGE_CURVE('',#39250,#39253,#22740,.T.);
#51286=EDGE_CURVE('',#39310,#39305,#22741,.T.);
#51287=EDGE_CURVE('',#39286,#39281,#22742,.T.);
#51288=EDGE_CURVE('',#39242,#39245,#22743,.T.);
#51289=EDGE_CURVE('',#39234,#39237,#22744,.T.);
#51290=EDGE_CURVE('',#39278,#39275,#22745,.T.);
#51291=EDGE_CURVE('',#39226,#39229,#22746,.T.);
#51292=EDGE_CURVE('',#39318,#39313,#22747,.T.);
#51293=EDGE_CURVE('',#39222,#39225,#22748,.T.);
#51294=EDGE_CURVE('',#39322,#39325,#22749,.T.);
#51295=EDGE_CURVE('',#39218,#39221,#22750,.T.);
#51296=EDGE_CURVE('',#39326,#39321,#22751,.T.);
#51297=EDGE_CURVE('',#39334,#39329,#22752,.T.);
#51298=EDGE_CURVE('',#39212,#39215,#22753,.T.);
#51299=EDGE_CURVE('',#39626,#39627,#32667,.T.);
#51300=EDGE_CURVE('',#39628,#39627,#5663,.T.);
#51301=EDGE_CURVE('',#39628,#39629,#32668,.T.);
#51302=EDGE_CURVE('',#39626,#39629,#5664,.T.);
#51303=EDGE_CURVE('',#39629,#39626,#32669,.T.);
#51304=EDGE_CURVE('',#39630,#39628,#32670,.T.);
#51305=EDGE_CURVE('',#39627,#39630,#32671,.T.);
#51306=EDGE_CURVE('',#39631,#39631,#32672,.T.);
#51307=EDGE_CURVE('',#39631,#39632,#32673,.T.);
#51308=EDGE_CURVE('',#39633,#39632,#32674,.T.);
#51309=EDGE_CURVE('',#39632,#39633,#32675,.T.);
#51310=EDGE_CURVE('',#39634,#39635,#32676,.T.);
#51311=EDGE_CURVE('',#39636,#39635,#5665,.T.);
#51312=EDGE_CURVE('',#39636,#39637,#32677,.T.);
#51313=EDGE_CURVE('',#39634,#39637,#5666,.T.);
#51314=EDGE_CURVE('',#39638,#39639,#32678,.T.);
#51315=EDGE_CURVE('',#39637,#39639,#5667,.T.);
#51316=EDGE_CURVE('',#39638,#39636,#5668,.T.);
#51317=EDGE_CURVE('',#39640,#39634,#32679,.T.);
#51318=EDGE_CURVE('',#39640,#39635,#32680,.T.);
#51319=EDGE_CURVE('',#39641,#39642,#32681,.T.);
#51320=EDGE_CURVE('',#39639,#39642,#5669,.T.);
#51321=EDGE_CURVE('',#39641,#39638,#5670,.T.);
#51322=EDGE_CURVE('',#39643,#39644,#32682,.T.);
#51323=EDGE_CURVE('',#39635,#39644,#32683,.T.);
#51324=EDGE_CURVE('',#39643,#39640,#32684,.T.);
#51325=EDGE_CURVE('',#39645,#39646,#32685,.T.);
#51326=EDGE_CURVE('',#39642,#39646,#5671,.T.);
#51327=EDGE_CURVE('',#39645,#39641,#5672,.T.);
#51328=EDGE_CURVE('',#39647,#39648,#32686,.T.);
#51329=EDGE_CURVE('',#39644,#39648,#32687,.T.);
#51330=EDGE_CURVE('',#39647,#39643,#32688,.T.);
#51331=EDGE_CURVE('',#39649,#39650,#32689,.T.);
#51332=EDGE_CURVE('',#39646,#39650,#5673,.T.);
#51333=EDGE_CURVE('',#39649,#39645,#5674,.T.);
#51334=EDGE_CURVE('',#39651,#39652,#32690,.T.);
#51335=EDGE_CURVE('',#39648,#39652,#32691,.T.);
#51336=EDGE_CURVE('',#39651,#39647,#32692,.T.);
#51337=EDGE_CURVE('',#39653,#39654,#32693,.T.);
#51338=EDGE_CURVE('',#39650,#39654,#5675,.T.);
#51339=EDGE_CURVE('',#39653,#39649,#5676,.T.);
#51340=EDGE_CURVE('',#39655,#39656,#32694,.T.);
#51341=EDGE_CURVE('',#39652,#39656,#5677,.T.);
#51342=EDGE_CURVE('',#39655,#39651,#5678,.T.);
#51343=EDGE_CURVE('',#39656,#39657,#32695,.T.);
#51344=EDGE_CURVE('',#39654,#39657,#5679,.T.);
#51345=EDGE_CURVE('',#39658,#39653,#5680,.T.);
#51346=EDGE_CURVE('',#39656,#39658,#2003,.T.);
#51347=EDGE_CURVE('',#39657,#39655,#32696,.T.);
#51348=EDGE_CURVE('',#39659,#39660,#32697,.T.);
#51349=EDGE_CURVE('',#39661,#39660,#5681,.T.);
#51350=EDGE_CURVE('',#39661,#39662,#32698,.T.);
#51351=EDGE_CURVE('',#39659,#39662,#5682,.T.);
#51352=EDGE_CURVE('',#39663,#39664,#32699,.T.);
#51353=EDGE_CURVE('',#39662,#39664,#5683,.T.);
#51354=EDGE_CURVE('',#39663,#39661,#5684,.T.);
#51355=EDGE_CURVE('',#39665,#39666,#32700,.T.);
#51356=EDGE_CURVE('',#39660,#39666,#5685,.T.);
#51357=EDGE_CURVE('',#39665,#39659,#5686,.T.);
#51358=EDGE_CURVE('',#39667,#39668,#32701,.T.);
#51359=EDGE_CURVE('',#39664,#39668,#5687,.T.);
#51360=EDGE_CURVE('',#39667,#39663,#5688,.T.);
#51361=EDGE_CURVE('',#39669,#39670,#32702,.T.);
#51362=EDGE_CURVE('',#39666,#39670,#5689,.T.);
#51363=EDGE_CURVE('',#39669,#39665,#5690,.T.);
#51364=EDGE_CURVE('',#39667,#39671,#32703,.T.);
#51365=EDGE_CURVE('',#39668,#39671,#32704,.T.);
#51366=EDGE_CURVE('',#39672,#39673,#32705,.T.);
#51367=EDGE_CURVE('',#39670,#39673,#5691,.T.);
#51368=EDGE_CURVE('',#39672,#39669,#5692,.T.);
#51369=EDGE_CURVE('',#39674,#39675,#32706,.T.);
#51370=EDGE_CURVE('',#39671,#39675,#5693,.T.);
#51371=EDGE_CURVE('',#39674,#39667,#5694,.T.);
#51372=EDGE_CURVE('',#39676,#39677,#32707,.T.);
#51373=EDGE_CURVE('',#39673,#39677,#5695,.T.);
#51374=EDGE_CURVE('',#39676,#39672,#5696,.T.);
#51375=EDGE_CURVE('',#39678,#39679,#32708,.T.);
#51376=EDGE_CURVE('',#39675,#39679,#32709,.T.);
#51377=EDGE_CURVE('',#39678,#39674,#32710,.T.);
#51378=EDGE_CURVE('',#39680,#39676,#32711,.T.);
#51379=EDGE_CURVE('',#39680,#39677,#32712,.T.);
#51380=EDGE_CURVE('',#39681,#39682,#32713,.T.);
#51381=EDGE_CURVE('',#39679,#39682,#32714,.T.);
#51382=EDGE_CURVE('',#39681,#39678,#32715,.T.);
#51383=EDGE_CURVE('',#39683,#39684,#32716,.T.);
#51384=EDGE_CURVE('',#39677,#39684,#5697,.T.);
#51385=EDGE_CURVE('',#39683,#39680,#5698,.T.);
#51386=EDGE_CURVE('',#39684,#39681,#32717,.T.);
#51387=EDGE_CURVE('',#39682,#39683,#32718,.T.);
#51388=EDGE_CURVE('',#38354,#39685,#32719,.T.);
#51389=EDGE_CURVE('',#39686,#38353,#32720,.T.);
#51390=EDGE_CURVE('',#39686,#39685,#32721,.T.);
#51391=EDGE_CURVE('',#39687,#39688,#32722,.T.);
#51392=EDGE_CURVE('',#39685,#39688,#32723,.T.);
#51393=EDGE_CURVE('',#39687,#39686,#32724,.T.);
#51394=EDGE_CURVE('',#39689,#39690,#32725,.T.);
#51395=EDGE_CURVE('',#39688,#39690,#32726,.T.);
#51396=EDGE_CURVE('',#39689,#39687,#32727,.T.);
#51397=EDGE_CURVE('',#39691,#39692,#32728,.T.);
#51398=EDGE_CURVE('',#39690,#39692,#32729,.T.);
#51399=EDGE_CURVE('',#39691,#39689,#32730,.T.);
#51400=EDGE_CURVE('',#39693,#39694,#32731,.T.);
#51401=EDGE_CURVE('',#39692,#39694,#32732,.T.);
#51402=EDGE_CURVE('',#39693,#39691,#32733,.T.);
#51403=EDGE_CURVE('',#39695,#39696,#32734,.T.);
#51404=EDGE_CURVE('',#39694,#39696,#32735,.T.);
#51405=EDGE_CURVE('',#39695,#39693,#32736,.T.);
#51406=EDGE_CURVE('',#39697,#39698,#32737,.T.);
#51407=EDGE_CURVE('',#39696,#39698,#32738,.T.);
#51408=EDGE_CURVE('',#39697,#39695,#32739,.T.);
#51409=EDGE_CURVE('',#39699,#39700,#32740,.T.);
#51410=EDGE_CURVE('',#39698,#39700,#32741,.T.);
#51411=EDGE_CURVE('',#39699,#39697,#32742,.T.);
#51412=EDGE_CURVE('',#38365,#39699,#32743,.T.);
#51413=EDGE_CURVE('',#39700,#38366,#32744,.T.);
#51414=EDGE_CURVE('',#39640,#39701,#32745,.T.);
#51415=EDGE_CURVE('',#39702,#39634,#32746,.T.);
#51416=EDGE_CURVE('',#39702,#39701,#32747,.T.);
#51417=EDGE_CURVE('',#39703,#39704,#32748,.T.);
#51418=EDGE_CURVE('',#39701,#39704,#5699,.T.);
#51419=EDGE_CURVE('',#39703,#39702,#2004,.T.);
#51420=EDGE_CURVE('',#39657,#39705,#5700,.T.);
#51421=EDGE_CURVE('',#39706,#39655,#5701,.T.);
#51422=EDGE_CURVE('',#39706,#39705,#32749,.T.);
#51423=EDGE_CURVE('',#39707,#39708,#32750,.T.);
#51424=EDGE_CURVE('',#39704,#39708,#5702,.T.);
#51425=EDGE_CURVE('',#39707,#39703,#5703,.T.);
#51426=EDGE_CURVE('',#39709,#39710,#32751,.T.);
#51427=EDGE_CURVE('',#39705,#39710,#32752,.T.);
#51428=EDGE_CURVE('',#39709,#39706,#32753,.T.);
#51429=EDGE_CURVE('',#39711,#39712,#32754,.T.);
#51430=EDGE_CURVE('',#39708,#39712,#32755,.T.);
#51431=EDGE_CURVE('',#39711,#39707,#32756,.T.);
#51432=EDGE_CURVE('',#39713,#39714,#32757,.T.);
#51433=EDGE_CURVE('',#39710,#39714,#5704,.T.);
#51434=EDGE_CURVE('',#39713,#39709,#5705,.T.);
#51435=EDGE_CURVE('',#39715,#39716,#32758,.T.);
#51436=EDGE_CURVE('',#39712,#39716,#5706,.T.);
#51437=EDGE_CURVE('',#39715,#39711,#5707,.T.);
#51438=EDGE_CURVE('',#39717,#39718,#32759,.T.);
#51439=EDGE_CURVE('',#39714,#39718,#5708,.T.);
#51440=EDGE_CURVE('',#39717,#39713,#5709,.T.);
#51441=EDGE_CURVE('',#39719,#39720,#32760,.T.);
#51442=EDGE_CURVE('',#39716,#39720,#5710,.T.);
#51443=EDGE_CURVE('',#39719,#39715,#5711,.T.);
#51444=EDGE_CURVE('',#39721,#39722,#32761,.T.);
#51445=EDGE_CURVE('',#39718,#39722,#5712,.T.);
#51446=EDGE_CURVE('',#39721,#39717,#5713,.T.);
#51447=EDGE_CURVE('',#39723,#39724,#32762,.T.);
#51448=EDGE_CURVE('',#39720,#39724,#5714,.T.);
#51449=EDGE_CURVE('',#39723,#39719,#5715,.T.);
#51450=EDGE_CURVE('',#39724,#39721,#32763,.T.);
#51451=EDGE_CURVE('',#39722,#39723,#32764,.T.);
#51452=EDGE_CURVE('',#39725,#39726,#32765,.T.);
#51453=EDGE_CURVE('',#39727,#39726,#5716,.T.);
#51454=EDGE_CURVE('',#39727,#39728,#32766,.T.);
#51455=EDGE_CURVE('',#39725,#39728,#5717,.T.);
#51456=EDGE_CURVE('',#39729,#39730,#32767,.T.);
#51457=EDGE_CURVE('',#39728,#39730,#32768,.T.);
#51458=EDGE_CURVE('',#39729,#39727,#32769,.T.);
#51459=EDGE_CURVE('',#39731,#39732,#32770,.T.);
#51460=EDGE_CURVE('',#39726,#39732,#5718,.T.);
#51461=EDGE_CURVE('',#39731,#39725,#5719,.T.);
#51462=EDGE_CURVE('',#39733,#39734,#32771,.T.);
#51463=EDGE_CURVE('',#39730,#39734,#5720,.T.);
#51464=EDGE_CURVE('',#39733,#39729,#5721,.T.);
#51465=EDGE_CURVE('',#39735,#39736,#32772,.T.);
#51466=EDGE_CURVE('',#39732,#39736,#5722,.T.);
#51467=EDGE_CURVE('',#39735,#39731,#5723,.T.);
#51468=EDGE_CURVE('',#39737,#39738,#32773,.T.);
#51469=EDGE_CURVE('',#39734,#39738,#5724,.T.);
#51470=EDGE_CURVE('',#39739,#39733,#5725,.T.);
#51471=EDGE_CURVE('',#39737,#39739,#5726,.T.);
#51472=EDGE_CURVE('',#39740,#39741,#32774,.T.);
#51473=EDGE_CURVE('',#39736,#39741,#32775,.T.);
#51474=EDGE_CURVE('',#39740,#39735,#32776,.T.);
#51475=EDGE_CURVE('',#39742,#39743,#32777,.T.);
#51476=EDGE_CURVE('',#39738,#39743,#5727,.T.);
#51477=EDGE_CURVE('',#39742,#39737,#5728,.T.);
#51478=EDGE_CURVE('',#39668,#39740,#5729,.T.);
#51479=EDGE_CURVE('',#39741,#39671,#5730,.T.);
#51480=EDGE_CURVE('',#39744,#39745,#32778,.T.);
#51481=EDGE_CURVE('',#39743,#39745,#32779,.T.);
#51482=EDGE_CURVE('',#39744,#39742,#32780,.T.);
#51483=EDGE_CURVE('',#39680,#39744,#5731,.T.);
#51484=EDGE_CURVE('',#39745,#39676,#5732,.T.);
#51485=EDGE_CURVE('',#39666,#39746,#22754,.T.);
#51486=EDGE_CURVE('',#39747,#39670,#22755,.T.);
#51487=EDGE_CURVE('',#39747,#39746,#32781,.T.);
#51488=EDGE_CURVE('',#39748,#39747,#32782,.T.);
#51489=EDGE_CURVE('',#39748,#39749,#32783,.T.);
#51490=EDGE_CURVE('',#39746,#39749,#32784,.T.);
#51491=EDGE_CURVE('',#39626,#39750,#32785,.T.);
#51492=EDGE_CURVE('',#39749,#39629,#32786,.T.);
#51493=EDGE_CURVE('',#39751,#39748,#32787,.T.);
#51494=EDGE_CURVE('',#39751,#39750,#32788,.T.);
#51495=EDGE_CURVE('',#39752,#39753,#32789,.T.);
#51496=EDGE_CURVE('',#39750,#39753,#32790,.T.);
#51497=EDGE_CURVE('',#39752,#39751,#32791,.T.);
#51498=EDGE_CURVE('',#39661,#39752,#22756,.T.);
#51499=EDGE_CURVE('',#39753,#39660,#22757,.T.);
#51500=EDGE_CURVE('',#39683,#39754,#22758,.T.);
#51501=EDGE_CURVE('',#39755,#39744,#22759,.T.);
#51502=EDGE_CURVE('',#39755,#39754,#32792,.T.);
#51503=EDGE_CURVE('',#39756,#39755,#32793,.T.);
#51504=EDGE_CURVE('',#39756,#39757,#32794,.T.);
#51505=EDGE_CURVE('',#39754,#39757,#32795,.T.);
#51506=EDGE_CURVE('',#39758,#39759,#32796,.T.);
#51507=EDGE_CURVE('',#39757,#39759,#32797,.T.);
#51508=EDGE_CURVE('',#39758,#39756,#32798,.T.);
#51509=EDGE_CURVE('',#39760,#39761,#32799,.T.);
#51510=EDGE_CURVE('',#39759,#39761,#32800,.T.);
#51511=EDGE_CURVE('',#39760,#39758,#32801,.T.);
#51512=EDGE_CURVE('',#39761,#39675,#22760,.T.);
#51513=EDGE_CURVE('',#39741,#39760,#22761,.T.);
#51514=EDGE_CURVE('',#39704,#39762,#22762,.T.);
#51515=EDGE_CURVE('',#39763,#39708,#22763,.T.);
#51516=EDGE_CURVE('',#39763,#39762,#32802,.T.);
#51517=EDGE_CURVE('',#39764,#39765,#32803,.T.);
#51518=EDGE_CURVE('',#39762,#39765,#32804,.T.);
#51519=EDGE_CURVE('',#39764,#39763,#32805,.T.);
#51520=EDGE_CURVE('',#39766,#39767,#32806,.T.);
#51521=EDGE_CURVE('',#39765,#39767,#32807,.T.);
#51522=EDGE_CURVE('',#39766,#39764,#32808,.T.);
#51523=EDGE_CURVE('',#39767,#39768,#32809,.T.);
#51524=EDGE_CURVE('',#39769,#39766,#32810,.T.);
#51525=EDGE_CURVE('',#39769,#39768,#32811,.T.);
#51526=EDGE_CURVE('',#39768,#39651,#22764,.T.);
#51527=EDGE_CURVE('',#39706,#39769,#22765,.T.);
#51528=EDGE_CURVE('',#39641,#39770,#22766,.T.);
#51529=EDGE_CURVE('',#39771,#39638,#22767,.T.);
#51530=EDGE_CURVE('',#39771,#39770,#32812,.T.);
#51531=EDGE_CURVE('',#39772,#39773,#32813,.T.);
#51532=EDGE_CURVE('',#39770,#39773,#32814,.T.);
#51533=EDGE_CURVE('',#39772,#39771,#32815,.T.);
#51534=EDGE_CURVE('',#39774,#39775,#32816,.T.);
#51535=EDGE_CURVE('',#39773,#39775,#32817,.T.);
#51536=EDGE_CURVE('',#39774,#39772,#32818,.T.);
#51537=EDGE_CURVE('',#39775,#39776,#32819,.T.);
#51538=EDGE_CURVE('',#39777,#39774,#32820,.T.);
#51539=EDGE_CURVE('',#39777,#39776,#32821,.T.);
#51540=EDGE_CURVE('',#39649,#39777,#22768,.T.);
#51541=EDGE_CURVE('',#39776,#39645,#22769,.T.);
#51542=EDGE_CURVE('',#39727,#39758,#22770,.T.);
#51543=EDGE_CURVE('',#39760,#39732,#22771,.T.);
#51544=EDGE_CURVE('',#39756,#39729,#22772,.T.);
#51545=EDGE_CURVE('',#39737,#39755,#22773,.T.);
#51546=EDGE_CURVE('',#39678,#39751,#22774,.T.);
#51547=EDGE_CURVE('',#39752,#39663,#22775,.T.);
#51548=EDGE_CURVE('',#39673,#39747,#22776,.T.);
#51549=EDGE_CURVE('',#39748,#39681,#22777,.T.);
#51550=EDGE_CURVE('',#39636,#39771,#22778,.T.);
#51551=EDGE_CURVE('',#39772,#39644,#22779,.T.);
#51552=EDGE_CURVE('',#39648,#39774,#22780,.T.);
#51553=EDGE_CURVE('',#39777,#39653,#22781,.T.);
#51554=EDGE_CURVE('',#39769,#39713,#22782,.T.);
#51555=EDGE_CURVE('',#39721,#39766,#22783,.T.);
#51556=EDGE_CURVE('',#39764,#39724,#22784,.T.);
#51557=EDGE_CURVE('',#39716,#39763,#22785,.T.);
#51558=EDGE_CURVE('',#39778,#39779,#32822,.T.);
#51559=EDGE_CURVE('',#39778,#39780,#32823,.T.);
#51560=EDGE_CURVE('',#39781,#39780,#32824,.T.);
#51561=EDGE_CURVE('',#39781,#39779,#32825,.T.);
#51562=EDGE_CURVE('',#39782,#39783,#32826,.T.);
#51563=EDGE_CURVE('',#39779,#39783,#22786,.T.);
#51564=EDGE_CURVE('',#39782,#39781,#22787,.T.);
#51565=EDGE_CURVE('',#39784,#39785,#32827,.T.);
#51566=EDGE_CURVE('',#39780,#39785,#32828,.T.);
#51567=EDGE_CURVE('',#39784,#39778,#32829,.T.);
#51568=EDGE_CURVE('',#39786,#39787,#32830,.T.);
#51569=EDGE_CURVE('',#39783,#39787,#32831,.T.);
#51570=EDGE_CURVE('',#39786,#39782,#32832,.T.);
#51571=EDGE_CURVE('',#39788,#39789,#32833,.T.);
#51572=EDGE_CURVE('',#39785,#39789,#32834,.T.);
#51573=EDGE_CURVE('',#39788,#39784,#32835,.T.);
#51574=EDGE_CURVE('',#39790,#39791,#32836,.T.);
#51575=EDGE_CURVE('',#39787,#39791,#22788,.T.);
#51576=EDGE_CURVE('',#39790,#39786,#22789,.T.);
#51577=EDGE_CURVE('',#39792,#39793,#32837,.T.);
#51578=EDGE_CURVE('',#39789,#39793,#32838,.T.);
#51579=EDGE_CURVE('',#39792,#39788,#32839,.T.);
#51580=EDGE_CURVE('',#39794,#39795,#32840,.T.);
#51581=EDGE_CURVE('',#39791,#39795,#32841,.T.);
#51582=EDGE_CURVE('',#39794,#39790,#32842,.T.);
#51583=EDGE_CURVE('',#39796,#39797,#32843,.T.);
#51584=EDGE_CURVE('',#39793,#39797,#32844,.T.);
#51585=EDGE_CURVE('',#39796,#39792,#32845,.T.);
#51586=EDGE_CURVE('',#39797,#39794,#22790,.T.);
#51587=EDGE_CURVE('',#39795,#39796,#22791,.T.);
#51588=EDGE_CURVE('',#39798,#39799,#32846,.T.);
#51589=EDGE_CURVE('',#39798,#39800,#32847,.T.);
#51590=EDGE_CURVE('',#39801,#39800,#32848,.T.);
#51591=EDGE_CURVE('',#39801,#39799,#32849,.T.);
#51592=EDGE_CURVE('',#39802,#39803,#32850,.T.);
#51593=EDGE_CURVE('',#39799,#39803,#22792,.T.);
#51594=EDGE_CURVE('',#39802,#39801,#22793,.T.);
#51595=EDGE_CURVE('',#39804,#39805,#32851,.T.);
#51596=EDGE_CURVE('',#39800,#39805,#32852,.T.);
#51597=EDGE_CURVE('',#39804,#39798,#32853,.T.);
#51598=EDGE_CURVE('',#39806,#39807,#32854,.T.);
#51599=EDGE_CURVE('',#39803,#39807,#32855,.T.);
#51600=EDGE_CURVE('',#39806,#39802,#32856,.T.);
#51601=EDGE_CURVE('',#39808,#39809,#32857,.T.);
#51602=EDGE_CURVE('',#39805,#39809,#32858,.T.);
#51603=EDGE_CURVE('',#39808,#39804,#32859,.T.);
#51604=EDGE_CURVE('',#39810,#39811,#32860,.T.);
#51605=EDGE_CURVE('',#39807,#39811,#22794,.T.);
#51606=EDGE_CURVE('',#39810,#39806,#22795,.T.);
#51607=EDGE_CURVE('',#39812,#39813,#32861,.T.);
#51608=EDGE_CURVE('',#39809,#39813,#22796,.T.);
#51609=EDGE_CURVE('',#39812,#39808,#22797,.T.);
#51610=EDGE_CURVE('',#39813,#39810,#32862,.T.);
#51611=EDGE_CURVE('',#39811,#39812,#32863,.T.);
#51612=EDGE_CURVE('',#39814,#39815,#32864,.T.);
#51613=EDGE_CURVE('',#39814,#39816,#32865,.T.);
#51614=EDGE_CURVE('',#39817,#39816,#32866,.T.);
#51615=EDGE_CURVE('',#39817,#39815,#32867,.T.);
#51616=EDGE_CURVE('',#39818,#39819,#32868,.T.);
#51617=EDGE_CURVE('',#39815,#39819,#22798,.T.);
#51618=EDGE_CURVE('',#39818,#39817,#22799,.T.);
#51619=EDGE_CURVE('',#39820,#39821,#32869,.T.);
#51620=EDGE_CURVE('',#39816,#39821,#32870,.T.);
#51621=EDGE_CURVE('',#39820,#39814,#32871,.T.);
#51622=EDGE_CURVE('',#39822,#39823,#32872,.T.);
#51623=EDGE_CURVE('',#39819,#39823,#32873,.T.);
#51624=EDGE_CURVE('',#39822,#39818,#32874,.T.);
#51625=EDGE_CURVE('',#39824,#39825,#32875,.T.);
#51626=EDGE_CURVE('',#39821,#39825,#32876,.T.);
#51627=EDGE_CURVE('',#39824,#39820,#32877,.T.);
#51628=EDGE_CURVE('',#39826,#39827,#32878,.T.);
#51629=EDGE_CURVE('',#39823,#39827,#22800,.T.);
#51630=EDGE_CURVE('',#39826,#39822,#22801,.T.);
#51631=EDGE_CURVE('',#39828,#39829,#32879,.T.);
#51632=EDGE_CURVE('',#39825,#39829,#22802,.T.);
#51633=EDGE_CURVE('',#39828,#39824,#22803,.T.);
#51634=EDGE_CURVE('',#39829,#39826,#32880,.T.);
#51635=EDGE_CURVE('',#39827,#39828,#32881,.T.);
#51636=EDGE_CURVE('',#39830,#39831,#32882,.T.);
#51637=EDGE_CURVE('',#39832,#39831,#32883,.T.);
#51638=EDGE_CURVE('',#39832,#39833,#32884,.T.);
#51639=EDGE_CURVE('',#39830,#39833,#32885,.T.);
#51640=EDGE_CURVE('',#39834,#39835,#32886,.T.);
#51641=EDGE_CURVE('',#39833,#39835,#22804,.T.);
#51642=EDGE_CURVE('',#39834,#39832,#22805,.T.);
#51643=EDGE_CURVE('',#39836,#39837,#32887,.T.);
#51644=EDGE_CURVE('',#39831,#39837,#22806,.T.);
#51645=EDGE_CURVE('',#39836,#39830,#22807,.T.);
#51646=EDGE_CURVE('',#39838,#39839,#32888,.T.);
#51647=EDGE_CURVE('',#39835,#39839,#32889,.T.);
#51648=EDGE_CURVE('',#39838,#39834,#32890,.T.);
#51649=EDGE_CURVE('',#39840,#39841,#32891,.T.);
#51650=EDGE_CURVE('',#39837,#39841,#32892,.T.);
#51651=EDGE_CURVE('',#39840,#39836,#32893,.T.);
#51652=EDGE_CURVE('',#39842,#39843,#32894,.T.);
#51653=EDGE_CURVE('',#39839,#39843,#22808,.T.);
#51654=EDGE_CURVE('',#39842,#39838,#22809,.T.);
#51655=EDGE_CURVE('',#39844,#39845,#32895,.T.);
#51656=EDGE_CURVE('',#39841,#39845,#22810,.T.);
#51657=EDGE_CURVE('',#39844,#39840,#22811,.T.);
#51658=EDGE_CURVE('',#39845,#39842,#32896,.T.);
#51659=EDGE_CURVE('',#39843,#39844,#32897,.T.);
#51660=EDGE_CURVE('',#39846,#39847,#32898,.T.);
#51661=EDGE_CURVE('',#39848,#39847,#32899,.T.);
#51662=EDGE_CURVE('',#39848,#39849,#32900,.T.);
#51663=EDGE_CURVE('',#39846,#39849,#32901,.T.);
#51664=EDGE_CURVE('',#39850,#39851,#32902,.T.);
#51665=EDGE_CURVE('',#39849,#39851,#22812,.T.);
#51666=EDGE_CURVE('',#39850,#39848,#22813,.T.);
#51667=EDGE_CURVE('',#39852,#39853,#32903,.T.);
#51668=EDGE_CURVE('',#39847,#39853,#22814,.T.);
#51669=EDGE_CURVE('',#39852,#39846,#22815,.T.);
#51670=EDGE_CURVE('',#39854,#39855,#32904,.T.);
#51671=EDGE_CURVE('',#39851,#39855,#32905,.T.);
#51672=EDGE_CURVE('',#39854,#39850,#32906,.T.);
#51673=EDGE_CURVE('',#39856,#39857,#32907,.T.);
#51674=EDGE_CURVE('',#39853,#39857,#32908,.T.);
#51675=EDGE_CURVE('',#39856,#39852,#32909,.T.);
#51676=EDGE_CURVE('',#39858,#39859,#32910,.T.);
#51677=EDGE_CURVE('',#39855,#39859,#32911,.T.);
#51678=EDGE_CURVE('',#39858,#39854,#32912,.T.);
#51679=EDGE_CURVE('',#39860,#39861,#32913,.T.);
#51680=EDGE_CURVE('',#39857,#39861,#22816,.T.);
#51681=EDGE_CURVE('',#39860,#39856,#22817,.T.);
#51682=EDGE_CURVE('',#39862,#39863,#32914,.T.);
#51683=EDGE_CURVE('',#39859,#39863,#32915,.T.);
#51684=EDGE_CURVE('',#39862,#39858,#32916,.T.);
#51685=EDGE_CURVE('',#39863,#39860,#32917,.T.);
#51686=EDGE_CURVE('',#39861,#39862,#32918,.T.);
#51687=EDGE_CURVE('',#39864,#39865,#32919,.T.);
#51688=EDGE_CURVE('',#39866,#39865,#32920,.T.);
#51689=EDGE_CURVE('',#39866,#39867,#32921,.T.);
#51690=EDGE_CURVE('',#39864,#39867,#32922,.T.);
#51691=EDGE_CURVE('',#39868,#39869,#32923,.T.);
#51692=EDGE_CURVE('',#39867,#39869,#22818,.T.);
#51693=EDGE_CURVE('',#39868,#39866,#22819,.T.);
#51694=EDGE_CURVE('',#39870,#39871,#32924,.T.);
#51695=EDGE_CURVE('',#39865,#39871,#22820,.T.);
#51696=EDGE_CURVE('',#39870,#39864,#22821,.T.);
#51697=EDGE_CURVE('',#39872,#39873,#32925,.T.);
#51698=EDGE_CURVE('',#39869,#39873,#32926,.T.);
#51699=EDGE_CURVE('',#39872,#39868,#32927,.T.);
#51700=EDGE_CURVE('',#39874,#39875,#32928,.T.);
#51701=EDGE_CURVE('',#39871,#39875,#32929,.T.);
#51702=EDGE_CURVE('',#39874,#39870,#32930,.T.);
#51703=EDGE_CURVE('',#39876,#39877,#32931,.T.);
#51704=EDGE_CURVE('',#39873,#39877,#22822,.T.);
#51705=EDGE_CURVE('',#39876,#39872,#22823,.T.);
#51706=EDGE_CURVE('',#39878,#39879,#32932,.T.);
#51707=EDGE_CURVE('',#39875,#39879,#22824,.T.);
#51708=EDGE_CURVE('',#39878,#39874,#22825,.T.);
#51709=EDGE_CURVE('',#39879,#39876,#32933,.T.);
#51710=EDGE_CURVE('',#39877,#39878,#32934,.T.);
#51711=EDGE_CURVE('',#39880,#39881,#32935,.T.);
#51712=EDGE_CURVE('',#39882,#39881,#32936,.T.);
#51713=EDGE_CURVE('',#39882,#39883,#32937,.T.);
#51714=EDGE_CURVE('',#39880,#39883,#32938,.T.);
#51715=EDGE_CURVE('',#39884,#39885,#32939,.T.);
#51716=EDGE_CURVE('',#39883,#39885,#22826,.T.);
#51717=EDGE_CURVE('',#39884,#39882,#22827,.T.);
#51718=EDGE_CURVE('',#39886,#39887,#32940,.T.);
#51719=EDGE_CURVE('',#39881,#39887,#22828,.T.);
#51720=EDGE_CURVE('',#39886,#39880,#22829,.T.);
#51721=EDGE_CURVE('',#39888,#39889,#32941,.T.);
#51722=EDGE_CURVE('',#39885,#39889,#32942,.T.);
#51723=EDGE_CURVE('',#39888,#39884,#32943,.T.);
#51724=EDGE_CURVE('',#39890,#39891,#32944,.T.);
#51725=EDGE_CURVE('',#39887,#39891,#32945,.T.);
#51726=EDGE_CURVE('',#39890,#39886,#32946,.T.);
#51727=EDGE_CURVE('',#39892,#39893,#32947,.T.);
#51728=EDGE_CURVE('',#39889,#39893,#22830,.T.);
#51729=EDGE_CURVE('',#39892,#39888,#22831,.T.);
#51730=EDGE_CURVE('',#39894,#39895,#32948,.T.);
#51731=EDGE_CURVE('',#39891,#39895,#22832,.T.);
#51732=EDGE_CURVE('',#39894,#39890,#22833,.T.);
#51733=EDGE_CURVE('',#39895,#39892,#32949,.T.);
#51734=EDGE_CURVE('',#39893,#39894,#32950,.T.);
#51735=EDGE_CURVE('',#39896,#39897,#32951,.T.);
#51736=EDGE_CURVE('',#39898,#39897,#32952,.T.);
#51737=EDGE_CURVE('',#39898,#39899,#32953,.T.);
#51738=EDGE_CURVE('',#39896,#39899,#32954,.T.);
#51739=EDGE_CURVE('',#39900,#39901,#32955,.T.);
#51740=EDGE_CURVE('',#39899,#39901,#22834,.T.);
#51741=EDGE_CURVE('',#39900,#39898,#22835,.T.);
#51742=EDGE_CURVE('',#39902,#39903,#32956,.T.);
#51743=EDGE_CURVE('',#39897,#39903,#22836,.T.);
#51744=EDGE_CURVE('',#39902,#39896,#22837,.T.);
#51745=EDGE_CURVE('',#39904,#39905,#32957,.T.);
#51746=EDGE_CURVE('',#39901,#39905,#32958,.T.);
#51747=EDGE_CURVE('',#39904,#39900,#32959,.T.);
#51748=EDGE_CURVE('',#39906,#39907,#32960,.T.);
#51749=EDGE_CURVE('',#39903,#39907,#32961,.T.);
#51750=EDGE_CURVE('',#39906,#39902,#32962,.T.);
#51751=EDGE_CURVE('',#39908,#39909,#32963,.T.);
#51752=EDGE_CURVE('',#39905,#39909,#22838,.T.);
#51753=EDGE_CURVE('',#39908,#39904,#22839,.T.);
#51754=EDGE_CURVE('',#39910,#39911,#32964,.T.);
#51755=EDGE_CURVE('',#39907,#39911,#22840,.T.);
#51756=EDGE_CURVE('',#39910,#39906,#22841,.T.);
#51757=EDGE_CURVE('',#39911,#39908,#32965,.T.);
#51758=EDGE_CURVE('',#39909,#39910,#32966,.T.);
#51759=EDGE_CURVE('',#39912,#39913,#32967,.T.);
#51760=EDGE_CURVE('',#39914,#39913,#32968,.T.);
#51761=EDGE_CURVE('',#39914,#39915,#32969,.T.);
#51762=EDGE_CURVE('',#39912,#39915,#32970,.T.);
#51763=EDGE_CURVE('',#39916,#39917,#32971,.T.);
#51764=EDGE_CURVE('',#39915,#39917,#22842,.T.);
#51765=EDGE_CURVE('',#39916,#39914,#22843,.T.);
#51766=EDGE_CURVE('',#39918,#39919,#32972,.T.);
#51767=EDGE_CURVE('',#39913,#39919,#22844,.T.);
#51768=EDGE_CURVE('',#39918,#39912,#22845,.T.);
#51769=EDGE_CURVE('',#39920,#39921,#32973,.T.);
#51770=EDGE_CURVE('',#39917,#39921,#32974,.T.);
#51771=EDGE_CURVE('',#39920,#39916,#32975,.T.);
#51772=EDGE_CURVE('',#39922,#39923,#32976,.T.);
#51773=EDGE_CURVE('',#39919,#39923,#32977,.T.);
#51774=EDGE_CURVE('',#39922,#39918,#32978,.T.);
#51775=EDGE_CURVE('',#39924,#39925,#32979,.T.);
#51776=EDGE_CURVE('',#39921,#39925,#22846,.T.);
#51777=EDGE_CURVE('',#39924,#39920,#22847,.T.);
#51778=EDGE_CURVE('',#39926,#39927,#32980,.T.);
#51779=EDGE_CURVE('',#39923,#39927,#22848,.T.);
#51780=EDGE_CURVE('',#39926,#39922,#22849,.T.);
#51781=EDGE_CURVE('',#39927,#39924,#32981,.T.);
#51782=EDGE_CURVE('',#39925,#39926,#32982,.T.);
#51783=EDGE_CURVE('',#39928,#39929,#32983,.T.);
#51784=EDGE_CURVE('',#39930,#39929,#32984,.T.);
#51785=EDGE_CURVE('',#39930,#39931,#32985,.T.);
#51786=EDGE_CURVE('',#39928,#39931,#32986,.T.);
#51787=EDGE_CURVE('',#39932,#39933,#32987,.T.);
#51788=EDGE_CURVE('',#39931,#39933,#22850,.T.);
#51789=EDGE_CURVE('',#39932,#39930,#22851,.T.);
#51790=EDGE_CURVE('',#39934,#39935,#32988,.T.);
#51791=EDGE_CURVE('',#39929,#39935,#22852,.T.);
#51792=EDGE_CURVE('',#39934,#39928,#22853,.T.);
#51793=EDGE_CURVE('',#39936,#39937,#32989,.T.);
#51794=EDGE_CURVE('',#39933,#39937,#32990,.T.);
#51795=EDGE_CURVE('',#39936,#39932,#32991,.T.);
#51796=EDGE_CURVE('',#39938,#39939,#32992,.T.);
#51797=EDGE_CURVE('',#39935,#39939,#32993,.T.);
#51798=EDGE_CURVE('',#39938,#39934,#32994,.T.);
#51799=EDGE_CURVE('',#39940,#39941,#32995,.T.);
#51800=EDGE_CURVE('',#39937,#39941,#22854,.T.);
#51801=EDGE_CURVE('',#39940,#39936,#22855,.T.);
#51802=EDGE_CURVE('',#39942,#39943,#32996,.T.);
#51803=EDGE_CURVE('',#39939,#39943,#32997,.T.);
#51804=EDGE_CURVE('',#39942,#39938,#32998,.T.);
#51805=EDGE_CURVE('',#39943,#39940,#32999,.T.);
#51806=EDGE_CURVE('',#39941,#39942,#33000,.T.);
#51807=EDGE_CURVE('',#39944,#39945,#33001,.T.);
#51808=EDGE_CURVE('',#39946,#39945,#33002,.T.);
#51809=EDGE_CURVE('',#39946,#39947,#33003,.T.);
#51810=EDGE_CURVE('',#39944,#39947,#33004,.T.);
#51811=EDGE_CURVE('',#39948,#39949,#33005,.T.);
#51812=EDGE_CURVE('',#39947,#39949,#22856,.T.);
#51813=EDGE_CURVE('',#39948,#39946,#22857,.T.);
#51814=EDGE_CURVE('',#39950,#39951,#33006,.T.);
#51815=EDGE_CURVE('',#39945,#39951,#22858,.T.);
#51816=EDGE_CURVE('',#39950,#39944,#22859,.T.);
#51817=EDGE_CURVE('',#39952,#39953,#33007,.T.);
#51818=EDGE_CURVE('',#39949,#39953,#33008,.T.);
#51819=EDGE_CURVE('',#39952,#39948,#33009,.T.);
#51820=EDGE_CURVE('',#39954,#39955,#33010,.T.);
#51821=EDGE_CURVE('',#39951,#39955,#33011,.T.);
#51822=EDGE_CURVE('',#39954,#39950,#33012,.T.);
#51823=EDGE_CURVE('',#39956,#39957,#33013,.T.);
#51824=EDGE_CURVE('',#39953,#39957,#22860,.T.);
#51825=EDGE_CURVE('',#39956,#39952,#22861,.T.);
#51826=EDGE_CURVE('',#39958,#39959,#33014,.T.);
#51827=EDGE_CURVE('',#39955,#39959,#33015,.T.);
#51828=EDGE_CURVE('',#39958,#39954,#33016,.T.);
#51829=EDGE_CURVE('',#39960,#39961,#33017,.T.);
#51830=EDGE_CURVE('',#39957,#39961,#33018,.T.);
#51831=EDGE_CURVE('',#39960,#39956,#33019,.T.);
#51832=EDGE_CURVE('',#39962,#39963,#33020,.T.);
#51833=EDGE_CURVE('',#39959,#39963,#33021,.T.);
#51834=EDGE_CURVE('',#39962,#39958,#33022,.T.);
#51835=EDGE_CURVE('',#39963,#39960,#33023,.T.);
#51836=EDGE_CURVE('',#39961,#39962,#33024,.T.);
#51837=EDGE_CURVE('',#39964,#39965,#33025,.T.);
#51838=EDGE_CURVE('',#39966,#39965,#33026,.T.);
#51839=EDGE_CURVE('',#39966,#39967,#33027,.T.);
#51840=EDGE_CURVE('',#39964,#39967,#33028,.T.);
#51841=EDGE_CURVE('',#39968,#39969,#33029,.T.);
#51842=EDGE_CURVE('',#39967,#39969,#22862,.T.);
#51843=EDGE_CURVE('',#39968,#39966,#22863,.T.);
#51844=EDGE_CURVE('',#39970,#39971,#33030,.T.);
#51845=EDGE_CURVE('',#39965,#39971,#22864,.T.);
#51846=EDGE_CURVE('',#39970,#39964,#22865,.T.);
#51847=EDGE_CURVE('',#39972,#39973,#33031,.T.);
#51848=EDGE_CURVE('',#39969,#39973,#33032,.T.);
#51849=EDGE_CURVE('',#39972,#39968,#33033,.T.);
#51850=EDGE_CURVE('',#39974,#39975,#33034,.T.);
#51851=EDGE_CURVE('',#39971,#39975,#33035,.T.);
#51852=EDGE_CURVE('',#39974,#39970,#33036,.T.);
#51853=EDGE_CURVE('',#39976,#39977,#33037,.T.);
#51854=EDGE_CURVE('',#39973,#39977,#22866,.T.);
#51855=EDGE_CURVE('',#39976,#39972,#22867,.T.);
#51856=EDGE_CURVE('',#39978,#39979,#33038,.T.);
#51857=EDGE_CURVE('',#39975,#39979,#33039,.T.);
#51858=EDGE_CURVE('',#39978,#39974,#33040,.T.);
#51859=EDGE_CURVE('',#39979,#39976,#33041,.T.);
#51860=EDGE_CURVE('',#39977,#39978,#33042,.T.);
#51861=EDGE_CURVE('',#39980,#39981,#33043,.T.);
#51862=EDGE_CURVE('',#39982,#39981,#33044,.T.);
#51863=EDGE_CURVE('',#39982,#39983,#33045,.T.);
#51864=EDGE_CURVE('',#39980,#39983,#33046,.T.);
#51865=EDGE_CURVE('',#39984,#39985,#33047,.T.);
#51866=EDGE_CURVE('',#39983,#39985,#22868,.T.);
#51867=EDGE_CURVE('',#39984,#39982,#22869,.T.);
#51868=EDGE_CURVE('',#39986,#39987,#33048,.T.);
#51869=EDGE_CURVE('',#39981,#39987,#22870,.T.);
#51870=EDGE_CURVE('',#39986,#39980,#22871,.T.);
#51871=EDGE_CURVE('',#39988,#39989,#33049,.T.);
#51872=EDGE_CURVE('',#39985,#39989,#33050,.T.);
#51873=EDGE_CURVE('',#39988,#39984,#33051,.T.);
#51874=EDGE_CURVE('',#39990,#39991,#33052,.T.);
#51875=EDGE_CURVE('',#39987,#39991,#33053,.T.);
#51876=EDGE_CURVE('',#39990,#39986,#33054,.T.);
#51877=EDGE_CURVE('',#39992,#39993,#33055,.T.);
#51878=EDGE_CURVE('',#39989,#39993,#22872,.T.);
#51879=EDGE_CURVE('',#39992,#39988,#22873,.T.);
#51880=EDGE_CURVE('',#39994,#39995,#33056,.T.);
#51881=EDGE_CURVE('',#39991,#39995,#22874,.T.);
#51882=EDGE_CURVE('',#39994,#39990,#22875,.T.);
#51883=EDGE_CURVE('',#39995,#39992,#33057,.T.);
#51884=EDGE_CURVE('',#39993,#39994,#33058,.T.);
#51885=EDGE_CURVE('',#39996,#39997,#33059,.T.);
#51886=EDGE_CURVE('',#39998,#39997,#33060,.T.);
#51887=EDGE_CURVE('',#39998,#39999,#33061,.T.);
#51888=EDGE_CURVE('',#39996,#39999,#33062,.T.);
#51889=EDGE_CURVE('',#40000,#40001,#33063,.T.);
#51890=EDGE_CURVE('',#39999,#40001,#22876,.T.);
#51891=EDGE_CURVE('',#40000,#39998,#22877,.T.);
#51892=EDGE_CURVE('',#40002,#40003,#33064,.T.);
#51893=EDGE_CURVE('',#39997,#40003,#33065,.T.);
#51894=EDGE_CURVE('',#40002,#39996,#33066,.T.);
#51895=EDGE_CURVE('',#40004,#40005,#33067,.T.);
#51896=EDGE_CURVE('',#40001,#40005,#33068,.T.);
#51897=EDGE_CURVE('',#40004,#40000,#33069,.T.);
#51898=EDGE_CURVE('',#40006,#40007,#33070,.T.);
#51899=EDGE_CURVE('',#40003,#40007,#33071,.T.);
#51900=EDGE_CURVE('',#40006,#40002,#33072,.T.);
#51901=EDGE_CURVE('',#40008,#40009,#33073,.T.);
#51902=EDGE_CURVE('',#40005,#40009,#22878,.T.);
#51903=EDGE_CURVE('',#40008,#40004,#22879,.T.);
#51904=EDGE_CURVE('',#40010,#40011,#33074,.T.);
#51905=EDGE_CURVE('',#40007,#40011,#22880,.T.);
#51906=EDGE_CURVE('',#40010,#40006,#22881,.T.);
#51907=EDGE_CURVE('',#40012,#40013,#33075,.T.);
#51908=EDGE_CURVE('',#40009,#40013,#33076,.T.);
#51909=EDGE_CURVE('',#40012,#40008,#33077,.T.);
#51910=EDGE_CURVE('',#40014,#40015,#33078,.T.);
#51911=EDGE_CURVE('',#40011,#40015,#33079,.T.);
#51912=EDGE_CURVE('',#40014,#40010,#33080,.T.);
#51913=EDGE_CURVE('',#40015,#40012,#22882,.T.);
#51914=EDGE_CURVE('',#40013,#40014,#22883,.T.);
#51915=EDGE_CURVE('',#40016,#40017,#33081,.T.);
#51916=EDGE_CURVE('',#40018,#40017,#33082,.T.);
#51917=EDGE_CURVE('',#40018,#40019,#33083,.T.);
#51918=EDGE_CURVE('',#40016,#40019,#33084,.T.);
#51919=EDGE_CURVE('',#40020,#40021,#33085,.T.);
#51920=EDGE_CURVE('',#40019,#40021,#22884,.T.);
#51921=EDGE_CURVE('',#40020,#40018,#22885,.T.);
#51922=EDGE_CURVE('',#40022,#40023,#33086,.T.);
#51923=EDGE_CURVE('',#40017,#40023,#22886,.T.);
#51924=EDGE_CURVE('',#40022,#40016,#22887,.T.);
#51925=EDGE_CURVE('',#40024,#40025,#33087,.T.);
#51926=EDGE_CURVE('',#40021,#40025,#33088,.T.);
#51927=EDGE_CURVE('',#40024,#40020,#33089,.T.);
#51928=EDGE_CURVE('',#40026,#40027,#33090,.T.);
#51929=EDGE_CURVE('',#40023,#40027,#33091,.T.);
#51930=EDGE_CURVE('',#40026,#40022,#33092,.T.);
#51931=EDGE_CURVE('',#40028,#40029,#33093,.T.);
#51932=EDGE_CURVE('',#40025,#40029,#22888,.T.);
#51933=EDGE_CURVE('',#40028,#40024,#22889,.T.);
#51934=EDGE_CURVE('',#40030,#40031,#33094,.T.);
#51935=EDGE_CURVE('',#40027,#40031,#33095,.T.);
#51936=EDGE_CURVE('',#40030,#40026,#33096,.T.);
#51937=EDGE_CURVE('',#40032,#40033,#33097,.T.);
#51938=EDGE_CURVE('',#40029,#40033,#33098,.T.);
#51939=EDGE_CURVE('',#40032,#40028,#33099,.T.);
#51940=EDGE_CURVE('',#40034,#40035,#33100,.T.);
#51941=EDGE_CURVE('',#40031,#40035,#33101,.T.);
#51942=EDGE_CURVE('',#40034,#40030,#33102,.T.);
#51943=EDGE_CURVE('',#40035,#40032,#22890,.T.);
#51944=EDGE_CURVE('',#40033,#40034,#22891,.T.);
#51945=EDGE_CURVE('',#40036,#40037,#33103,.T.);
#51946=EDGE_CURVE('',#40038,#40037,#33104,.T.);
#51947=EDGE_CURVE('',#40038,#40039,#33105,.T.);
#51948=EDGE_CURVE('',#40036,#40039,#33106,.T.);
#51949=EDGE_CURVE('',#40040,#40041,#33107,.T.);
#51950=EDGE_CURVE('',#40039,#40041,#22892,.T.);
#51951=EDGE_CURVE('',#40040,#40038,#22893,.T.);
#51952=EDGE_CURVE('',#40042,#40043,#33108,.T.);
#51953=EDGE_CURVE('',#40037,#40043,#22894,.T.);
#51954=EDGE_CURVE('',#40042,#40036,#22895,.T.);
#51955=EDGE_CURVE('',#40044,#40045,#33109,.T.);
#51956=EDGE_CURVE('',#40041,#40045,#33110,.T.);
#51957=EDGE_CURVE('',#40044,#40040,#33111,.T.);
#51958=EDGE_CURVE('',#40046,#40047,#33112,.T.);
#51959=EDGE_CURVE('',#40043,#40047,#33113,.T.);
#51960=EDGE_CURVE('',#40046,#40042,#33114,.T.);
#51961=EDGE_CURVE('',#40048,#40049,#33115,.T.);
#51962=EDGE_CURVE('',#40045,#40049,#22896,.T.);
#51963=EDGE_CURVE('',#40048,#40044,#22897,.T.);
#51964=EDGE_CURVE('',#40050,#40051,#33116,.T.);
#51965=EDGE_CURVE('',#40047,#40051,#22898,.T.);
#51966=EDGE_CURVE('',#40050,#40046,#22899,.T.);
#51967=EDGE_CURVE('',#40051,#40048,#33117,.T.);
#51968=EDGE_CURVE('',#40049,#40050,#33118,.T.);
#51969=EDGE_CURVE('',#40052,#40053,#33119,.T.);
#51970=EDGE_CURVE('',#40054,#40053,#33120,.T.);
#51971=EDGE_CURVE('',#40054,#40055,#33121,.T.);
#51972=EDGE_CURVE('',#40052,#40055,#33122,.T.);
#51973=EDGE_CURVE('',#40056,#40057,#33123,.T.);
#51974=EDGE_CURVE('',#40055,#40057,#22900,.T.);
#51975=EDGE_CURVE('',#40056,#40054,#22901,.T.);
#51976=EDGE_CURVE('',#40058,#40059,#33124,.T.);
#51977=EDGE_CURVE('',#40053,#40059,#22902,.T.);
#51978=EDGE_CURVE('',#40058,#40052,#22903,.T.);
#51979=EDGE_CURVE('',#40060,#40061,#33125,.T.);
#51980=EDGE_CURVE('',#40057,#40061,#33126,.T.);
#51981=EDGE_CURVE('',#40060,#40056,#33127,.T.);
#51982=EDGE_CURVE('',#40062,#40063,#33128,.T.);
#51983=EDGE_CURVE('',#40059,#40063,#33129,.T.);
#51984=EDGE_CURVE('',#40062,#40058,#33130,.T.);
#51985=EDGE_CURVE('',#40064,#40065,#33131,.T.);
#51986=EDGE_CURVE('',#40061,#40065,#33132,.T.);
#51987=EDGE_CURVE('',#40064,#40060,#33133,.T.);
#51988=EDGE_CURVE('',#40066,#40067,#33134,.T.);
#51989=EDGE_CURVE('',#40063,#40067,#22904,.T.);
#51990=EDGE_CURVE('',#40066,#40062,#22905,.T.);
#51991=EDGE_CURVE('',#40067,#40064,#33135,.T.);
#51992=EDGE_CURVE('',#40065,#40066,#33136,.T.);
#51993=EDGE_CURVE('',#40068,#40069,#33137,.T.);
#51994=EDGE_CURVE('',#40070,#40069,#33138,.T.);
#51995=EDGE_CURVE('',#40070,#40071,#33139,.T.);
#51996=EDGE_CURVE('',#40068,#40071,#33140,.T.);
#51997=EDGE_CURVE('',#40072,#40073,#33141,.T.);
#51998=EDGE_CURVE('',#40071,#40073,#22906,.T.);
#51999=EDGE_CURVE('',#40072,#40070,#22907,.T.);
#52000=EDGE_CURVE('',#40074,#40075,#33142,.T.);
#52001=EDGE_CURVE('',#40069,#40075,#22908,.T.);
#52002=EDGE_CURVE('',#40074,#40068,#22909,.T.);
#52003=EDGE_CURVE('',#40076,#40077,#33143,.T.);
#52004=EDGE_CURVE('',#40073,#40077,#33144,.T.);
#52005=EDGE_CURVE('',#40076,#40072,#33145,.T.);
#52006=EDGE_CURVE('',#40078,#40079,#33146,.T.);
#52007=EDGE_CURVE('',#40075,#40079,#33147,.T.);
#52008=EDGE_CURVE('',#40078,#40074,#33148,.T.);
#52009=EDGE_CURVE('',#40080,#40081,#33149,.T.);
#52010=EDGE_CURVE('',#40077,#40081,#22910,.T.);
#52011=EDGE_CURVE('',#40080,#40076,#22911,.T.);
#52012=EDGE_CURVE('',#40082,#40083,#33150,.T.);
#52013=EDGE_CURVE('',#40079,#40083,#22912,.T.);
#52014=EDGE_CURVE('',#40082,#40078,#22913,.T.);
#52015=EDGE_CURVE('',#40083,#40080,#33151,.T.);
#52016=EDGE_CURVE('',#40081,#40082,#33152,.T.);
#52017=EDGE_CURVE('',#40084,#40085,#33153,.T.);
#52018=EDGE_CURVE('',#40086,#40085,#33154,.T.);
#52019=EDGE_CURVE('',#40086,#40087,#33155,.T.);
#52020=EDGE_CURVE('',#40084,#40087,#33156,.T.);
#52021=EDGE_CURVE('',#40088,#40089,#33157,.T.);
#52022=EDGE_CURVE('',#40087,#40089,#22914,.T.);
#52023=EDGE_CURVE('',#40088,#40086,#22915,.T.);
#52024=EDGE_CURVE('',#40090,#40091,#33158,.T.);
#52025=EDGE_CURVE('',#40085,#40091,#22916,.T.);
#52026=EDGE_CURVE('',#40090,#40084,#22917,.T.);
#52027=EDGE_CURVE('',#40092,#40093,#33159,.T.);
#52028=EDGE_CURVE('',#40089,#40093,#33160,.T.);
#52029=EDGE_CURVE('',#40092,#40088,#33161,.T.);
#52030=EDGE_CURVE('',#40094,#40095,#33162,.T.);
#52031=EDGE_CURVE('',#40091,#40095,#33163,.T.);
#52032=EDGE_CURVE('',#40094,#40090,#33164,.T.);
#52033=EDGE_CURVE('',#40096,#40097,#33165,.T.);
#52034=EDGE_CURVE('',#40093,#40097,#22918,.T.);
#52035=EDGE_CURVE('',#40096,#40092,#22919,.T.);
#52036=EDGE_CURVE('',#40098,#40099,#33166,.T.);
#52037=EDGE_CURVE('',#40095,#40099,#22920,.T.);
#52038=EDGE_CURVE('',#40098,#40094,#22921,.T.);
#52039=EDGE_CURVE('',#40099,#40096,#33167,.T.);
#52040=EDGE_CURVE('',#40097,#40098,#33168,.T.);
#52041=EDGE_CURVE('',#40100,#40101,#33169,.T.);
#52042=EDGE_CURVE('',#40102,#40101,#33170,.T.);
#52043=EDGE_CURVE('',#40102,#40103,#33171,.T.);
#52044=EDGE_CURVE('',#40100,#40103,#33172,.T.);
#52045=EDGE_CURVE('',#40104,#40105,#33173,.T.);
#52046=EDGE_CURVE('',#40103,#40105,#22922,.T.);
#52047=EDGE_CURVE('',#40104,#40102,#22923,.T.);
#52048=EDGE_CURVE('',#40106,#40107,#33174,.T.);
#52049=EDGE_CURVE('',#40101,#40107,#22924,.T.);
#52050=EDGE_CURVE('',#40106,#40100,#22925,.T.);
#52051=EDGE_CURVE('',#40108,#40109,#33175,.T.);
#52052=EDGE_CURVE('',#40105,#40109,#33176,.T.);
#52053=EDGE_CURVE('',#40108,#40104,#33177,.T.);
#52054=EDGE_CURVE('',#40110,#40111,#33178,.T.);
#52055=EDGE_CURVE('',#40107,#40111,#33179,.T.);
#52056=EDGE_CURVE('',#40110,#40106,#33180,.T.);
#52057=EDGE_CURVE('',#40112,#40113,#33181,.T.);
#52058=EDGE_CURVE('',#40109,#40113,#22926,.T.);
#52059=EDGE_CURVE('',#40112,#40108,#22927,.T.);
#52060=EDGE_CURVE('',#40114,#40115,#33182,.T.);
#52061=EDGE_CURVE('',#40111,#40115,#33183,.T.);
#52062=EDGE_CURVE('',#40114,#40110,#33184,.T.);
#52063=EDGE_CURVE('',#40113,#40116,#33185,.T.);
#52064=EDGE_CURVE('',#40117,#40112,#33186,.T.);
#52065=EDGE_CURVE('',#40117,#40116,#33187,.T.);
#52066=EDGE_CURVE('',#40116,#40114,#33188,.T.);
#52067=EDGE_CURVE('',#40115,#40117,#33189,.T.);
#52068=EDGE_CURVE('',#40118,#40119,#33190,.T.);
#52069=EDGE_CURVE('',#40120,#40119,#33191,.T.);
#52070=EDGE_CURVE('',#40120,#40121,#33192,.T.);
#52071=EDGE_CURVE('',#40118,#40121,#33193,.T.);
#52072=EDGE_CURVE('',#40122,#40123,#33194,.T.);
#52073=EDGE_CURVE('',#40121,#40123,#22928,.T.);
#52074=EDGE_CURVE('',#40122,#40120,#22929,.T.);
#52075=EDGE_CURVE('',#40124,#40125,#33195,.T.);
#52076=EDGE_CURVE('',#40119,#40125,#22930,.T.);
#52077=EDGE_CURVE('',#40124,#40118,#22931,.T.);
#52078=EDGE_CURVE('',#40126,#40127,#33196,.T.);
#52079=EDGE_CURVE('',#40123,#40127,#33197,.T.);
#52080=EDGE_CURVE('',#40126,#40122,#33198,.T.);
#52081=EDGE_CURVE('',#40128,#40129,#33199,.T.);
#52082=EDGE_CURVE('',#40125,#40129,#33200,.T.);
#52083=EDGE_CURVE('',#40128,#40124,#33201,.T.);
#52084=EDGE_CURVE('',#40130,#40131,#33202,.T.);
#52085=EDGE_CURVE('',#40127,#40131,#33203,.T.);
#52086=EDGE_CURVE('',#40130,#40126,#33204,.T.);
#52087=EDGE_CURVE('',#40132,#40133,#33205,.T.);
#52088=EDGE_CURVE('',#40129,#40133,#22932,.T.);
#52089=EDGE_CURVE('',#40132,#40128,#22933,.T.);
#52090=EDGE_CURVE('',#40133,#40130,#33206,.T.);
#52091=EDGE_CURVE('',#40131,#40132,#33207,.T.);
#52092=EDGE_CURVE('',#40134,#40135,#33208,.T.);
#52093=EDGE_CURVE('',#40136,#40135,#33209,.T.);
#52094=EDGE_CURVE('',#40136,#40137,#33210,.T.);
#52095=EDGE_CURVE('',#40134,#40137,#33211,.T.);
#52096=EDGE_CURVE('',#40138,#40139,#33212,.T.);
#52097=EDGE_CURVE('',#40137,#40139,#22934,.T.);
#52098=EDGE_CURVE('',#40138,#40136,#22935,.T.);
#52099=EDGE_CURVE('',#40140,#40141,#33213,.T.);
#52100=EDGE_CURVE('',#40135,#40141,#22936,.T.);
#52101=EDGE_CURVE('',#40140,#40134,#22937,.T.);
#52102=EDGE_CURVE('',#40142,#40143,#33214,.T.);
#52103=EDGE_CURVE('',#40139,#40143,#33215,.T.);
#52104=EDGE_CURVE('',#40142,#40138,#33216,.T.);
#52105=EDGE_CURVE('',#40144,#40145,#33217,.T.);
#52106=EDGE_CURVE('',#40141,#40145,#33218,.T.);
#52107=EDGE_CURVE('',#40144,#40140,#33219,.T.);
#52108=EDGE_CURVE('',#40146,#40147,#33220,.T.);
#52109=EDGE_CURVE('',#40143,#40147,#33221,.T.);
#52110=EDGE_CURVE('',#40146,#40142,#33222,.T.);
#52111=EDGE_CURVE('',#40148,#40149,#33223,.T.);
#52112=EDGE_CURVE('',#40145,#40149,#22938,.T.);
#52113=EDGE_CURVE('',#40148,#40144,#22939,.T.);
#52114=EDGE_CURVE('',#40150,#40151,#33224,.T.);
#52115=EDGE_CURVE('',#40147,#40151,#33225,.T.);
#52116=EDGE_CURVE('',#40150,#40146,#33226,.T.);
#52117=EDGE_CURVE('',#40152,#40153,#33227,.T.);
#52118=EDGE_CURVE('',#40149,#40153,#33228,.T.);
#52119=EDGE_CURVE('',#40152,#40148,#33229,.T.);
#52120=EDGE_CURVE('',#40153,#40150,#33230,.T.);
#52121=EDGE_CURVE('',#40151,#40152,#33231,.T.);
#52122=EDGE_CURVE('',#40154,#40155,#33232,.T.);
#52123=EDGE_CURVE('',#40156,#40155,#33233,.T.);
#52124=EDGE_CURVE('',#40156,#40157,#33234,.T.);
#52125=EDGE_CURVE('',#40154,#40157,#33235,.T.);
#52126=EDGE_CURVE('',#40158,#40159,#33236,.T.);
#52127=EDGE_CURVE('',#40157,#40159,#22940,.T.);
#52128=EDGE_CURVE('',#40158,#40156,#22941,.T.);
#52129=EDGE_CURVE('',#40160,#40161,#33237,.T.);
#52130=EDGE_CURVE('',#40155,#40161,#22942,.T.);
#52131=EDGE_CURVE('',#40160,#40154,#22943,.T.);
#52132=EDGE_CURVE('',#40162,#40163,#33238,.T.);
#52133=EDGE_CURVE('',#40159,#40163,#33239,.T.);
#52134=EDGE_CURVE('',#40162,#40158,#33240,.T.);
#52135=EDGE_CURVE('',#40164,#40165,#33241,.T.);
#52136=EDGE_CURVE('',#40161,#40165,#33242,.T.);
#52137=EDGE_CURVE('',#40164,#40160,#33243,.T.);
#52138=EDGE_CURVE('',#40166,#40167,#33244,.T.);
#52139=EDGE_CURVE('',#40163,#40167,#22944,.T.);
#52140=EDGE_CURVE('',#40166,#40162,#22945,.T.);
#52141=EDGE_CURVE('',#40168,#40169,#33245,.T.);
#52142=EDGE_CURVE('',#40165,#40169,#22946,.T.);
#52143=EDGE_CURVE('',#40168,#40164,#22947,.T.);
#52144=EDGE_CURVE('',#40169,#40166,#33246,.T.);
#52145=EDGE_CURVE('',#40167,#40168,#33247,.T.);
#52146=EDGE_CURVE('',#40170,#40171,#33248,.T.);
#52147=EDGE_CURVE('',#40172,#40171,#33249,.T.);
#52148=EDGE_CURVE('',#40172,#40173,#33250,.T.);
#52149=EDGE_CURVE('',#40170,#40173,#33251,.T.);
#52150=EDGE_CURVE('',#40174,#40175,#33252,.T.);
#52151=EDGE_CURVE('',#40173,#40175,#22948,.T.);
#52152=EDGE_CURVE('',#40174,#40172,#22949,.T.);
#52153=EDGE_CURVE('',#40176,#40177,#33253,.T.);
#52154=EDGE_CURVE('',#40171,#40177,#22950,.T.);
#52155=EDGE_CURVE('',#40176,#40170,#22951,.T.);
#52156=EDGE_CURVE('',#40178,#40179,#33254,.T.);
#52157=EDGE_CURVE('',#40175,#40179,#33255,.T.);
#52158=EDGE_CURVE('',#40178,#40174,#33256,.T.);
#52159=EDGE_CURVE('',#40180,#40181,#33257,.T.);
#52160=EDGE_CURVE('',#40177,#40181,#33258,.T.);
#52161=EDGE_CURVE('',#40180,#40176,#33259,.T.);
#52162=EDGE_CURVE('',#40182,#40183,#33260,.T.);
#52163=EDGE_CURVE('',#40179,#40183,#22952,.T.);
#52164=EDGE_CURVE('',#40182,#40178,#22953,.T.);
#52165=EDGE_CURVE('',#40184,#40185,#33261,.T.);
#52166=EDGE_CURVE('',#40181,#40185,#33262,.T.);
#52167=EDGE_CURVE('',#40184,#40180,#33263,.T.);
#52168=EDGE_CURVE('',#40186,#40187,#33264,.T.);
#52169=EDGE_CURVE('',#40183,#40187,#33265,.T.);
#52170=EDGE_CURVE('',#40186,#40182,#33266,.T.);
#52171=EDGE_CURVE('',#40188,#40189,#33267,.T.);
#52172=EDGE_CURVE('',#40185,#40189,#33268,.T.);
#52173=EDGE_CURVE('',#40188,#40184,#33269,.T.);
#52174=EDGE_CURVE('',#40189,#40186,#33270,.T.);
#52175=EDGE_CURVE('',#40187,#40188,#33271,.T.);
#52176=EDGE_CURVE('',#40190,#40191,#33272,.T.);
#52177=EDGE_CURVE('',#40192,#40191,#33273,.T.);
#52178=EDGE_CURVE('',#40192,#40193,#33274,.T.);
#52179=EDGE_CURVE('',#40190,#40193,#33275,.T.);
#52180=EDGE_CURVE('',#40194,#40195,#33276,.T.);
#52181=EDGE_CURVE('',#40193,#40195,#22954,.T.);
#52182=EDGE_CURVE('',#40194,#40192,#22955,.T.);
#52183=EDGE_CURVE('',#40196,#40197,#33277,.T.);
#52184=EDGE_CURVE('',#40191,#40197,#22956,.T.);
#52185=EDGE_CURVE('',#40196,#40190,#22957,.T.);
#52186=EDGE_CURVE('',#40198,#40199,#33278,.T.);
#52187=EDGE_CURVE('',#40195,#40199,#33279,.T.);
#52188=EDGE_CURVE('',#40198,#40194,#33280,.T.);
#52189=EDGE_CURVE('',#40200,#40201,#33281,.T.);
#52190=EDGE_CURVE('',#40197,#40201,#33282,.T.);
#52191=EDGE_CURVE('',#40200,#40196,#33283,.T.);
#52192=EDGE_CURVE('',#40202,#40203,#33284,.T.);
#52193=EDGE_CURVE('',#40199,#40203,#22958,.T.);
#52194=EDGE_CURVE('',#40202,#40198,#22959,.T.);
#52195=EDGE_CURVE('',#40204,#40205,#33285,.T.);
#52196=EDGE_CURVE('',#40201,#40205,#33286,.T.);
#52197=EDGE_CURVE('',#40204,#40200,#33287,.T.);
#52198=EDGE_CURVE('',#40205,#40202,#33288,.T.);
#52199=EDGE_CURVE('',#40203,#40204,#33289,.T.);
#52200=EDGE_CURVE('',#40206,#40207,#33290,.T.);
#52201=EDGE_CURVE('',#40208,#40207,#33291,.T.);
#52202=EDGE_CURVE('',#40208,#40209,#33292,.T.);
#52203=EDGE_CURVE('',#40206,#40209,#33293,.T.);
#52204=EDGE_CURVE('',#40210,#40211,#33294,.T.);
#52205=EDGE_CURVE('',#40209,#40211,#22960,.T.);
#52206=EDGE_CURVE('',#40210,#40208,#22961,.T.);
#52207=EDGE_CURVE('',#40212,#40213,#33295,.T.);
#52208=EDGE_CURVE('',#40207,#40213,#22962,.T.);
#52209=EDGE_CURVE('',#40212,#40206,#22963,.T.);
#52210=EDGE_CURVE('',#40214,#40215,#33296,.T.);
#52211=EDGE_CURVE('',#40211,#40215,#33297,.T.);
#52212=EDGE_CURVE('',#40214,#40210,#33298,.T.);
#52213=EDGE_CURVE('',#40216,#40217,#33299,.T.);
#52214=EDGE_CURVE('',#40213,#40217,#33300,.T.);
#52215=EDGE_CURVE('',#40216,#40212,#33301,.T.);
#52216=EDGE_CURVE('',#40218,#40219,#33302,.T.);
#52217=EDGE_CURVE('',#40215,#40219,#22964,.T.);
#52218=EDGE_CURVE('',#40218,#40214,#22965,.T.);
#52219=EDGE_CURVE('',#40220,#40221,#33303,.T.);
#52220=EDGE_CURVE('',#40217,#40221,#22966,.T.);
#52221=EDGE_CURVE('',#40220,#40216,#22967,.T.);
#52222=EDGE_CURVE('',#40221,#40218,#33304,.T.);
#52223=EDGE_CURVE('',#40219,#40220,#33305,.T.);
#52224=EDGE_CURVE('',#40222,#40223,#33306,.T.);
#52225=EDGE_CURVE('',#40224,#40223,#33307,.T.);
#52226=EDGE_CURVE('',#40224,#40225,#33308,.T.);
#52227=EDGE_CURVE('',#40222,#40225,#33309,.T.);
#52228=EDGE_CURVE('',#40226,#40227,#33310,.T.);
#52229=EDGE_CURVE('',#40225,#40227,#22968,.T.);
#52230=EDGE_CURVE('',#40226,#40224,#22969,.T.);
#52231=EDGE_CURVE('',#40228,#40229,#33311,.T.);
#52232=EDGE_CURVE('',#40223,#40229,#22970,.T.);
#52233=EDGE_CURVE('',#40228,#40222,#22971,.T.);
#52234=EDGE_CURVE('',#40230,#40231,#33312,.T.);
#52235=EDGE_CURVE('',#40227,#40231,#33313,.T.);
#52236=EDGE_CURVE('',#40230,#40226,#33314,.T.);
#52237=EDGE_CURVE('',#40232,#40233,#33315,.T.);
#52238=EDGE_CURVE('',#40229,#40233,#33316,.T.);
#52239=EDGE_CURVE('',#40232,#40228,#33317,.T.);
#52240=EDGE_CURVE('',#40234,#40235,#33318,.T.);
#52241=EDGE_CURVE('',#40231,#40235,#22972,.T.);
#52242=EDGE_CURVE('',#40234,#40230,#22973,.T.);
#52243=EDGE_CURVE('',#40236,#40237,#33319,.T.);
#52244=EDGE_CURVE('',#40233,#40237,#33320,.T.);
#52245=EDGE_CURVE('',#40236,#40232,#33321,.T.);
#52246=EDGE_CURVE('',#40237,#40234,#33322,.T.);
#52247=EDGE_CURVE('',#40235,#40236,#33323,.T.);
#52248=EDGE_CURVE('',#40238,#40239,#33324,.T.);
#52249=EDGE_CURVE('',#40240,#40239,#33325,.T.);
#52250=EDGE_CURVE('',#40240,#40241,#33326,.T.);
#52251=EDGE_CURVE('',#40238,#40241,#33327,.T.);
#52252=EDGE_CURVE('',#40242,#40243,#33328,.T.);
#52253=EDGE_CURVE('',#40241,#40243,#22974,.T.);
#52254=EDGE_CURVE('',#40242,#40240,#22975,.T.);
#52255=EDGE_CURVE('',#40244,#40245,#33329,.T.);
#52256=EDGE_CURVE('',#40239,#40245,#22976,.T.);
#52257=EDGE_CURVE('',#40244,#40238,#22977,.T.);
#52258=EDGE_CURVE('',#40246,#40247,#33330,.T.);
#52259=EDGE_CURVE('',#40243,#40247,#33331,.T.);
#52260=EDGE_CURVE('',#40246,#40242,#33332,.T.);
#52261=EDGE_CURVE('',#40248,#40249,#33333,.T.);
#52262=EDGE_CURVE('',#40245,#40249,#33334,.T.);
#52263=EDGE_CURVE('',#40248,#40244,#33335,.T.);
#52264=EDGE_CURVE('',#40250,#40251,#33336,.T.);
#52265=EDGE_CURVE('',#40247,#40251,#22978,.T.);
#52266=EDGE_CURVE('',#40250,#40246,#22979,.T.);
#52267=EDGE_CURVE('',#40252,#40253,#33337,.T.);
#52268=EDGE_CURVE('',#40249,#40253,#22980,.T.);
#52269=EDGE_CURVE('',#40252,#40248,#22981,.T.);
#52270=EDGE_CURVE('',#40253,#40250,#33338,.T.);
#52271=EDGE_CURVE('',#40251,#40252,#33339,.T.);
#52272=EDGE_CURVE('',#40254,#40255,#33340,.T.);
#52273=EDGE_CURVE('',#40256,#40255,#33341,.T.);
#52274=EDGE_CURVE('',#40256,#40257,#33342,.T.);
#52275=EDGE_CURVE('',#40254,#40257,#33343,.T.);
#52276=EDGE_CURVE('',#40258,#40259,#33344,.T.);
#52277=EDGE_CURVE('',#40257,#40259,#22982,.T.);
#52278=EDGE_CURVE('',#40258,#40256,#22983,.T.);
#52279=EDGE_CURVE('',#40260,#40261,#33345,.T.);
#52280=EDGE_CURVE('',#40255,#40261,#33346,.T.);
#52281=EDGE_CURVE('',#40260,#40254,#33347,.T.);
#52282=EDGE_CURVE('',#40262,#40263,#33348,.T.);
#52283=EDGE_CURVE('',#40259,#40263,#33349,.T.);
#52284=EDGE_CURVE('',#40262,#40258,#33350,.T.);
#52285=EDGE_CURVE('',#40264,#40265,#33351,.T.);
#52286=EDGE_CURVE('',#40261,#40265,#33352,.T.);
#52287=EDGE_CURVE('',#40264,#40260,#33353,.T.);
#52288=EDGE_CURVE('',#40265,#40262,#22984,.T.);
#52289=EDGE_CURVE('',#40263,#40264,#22985,.T.);
#52290=EDGE_CURVE('',#40266,#40267,#33354,.T.);
#52291=EDGE_CURVE('',#40266,#40268,#33355,.T.);
#52292=EDGE_CURVE('',#40269,#40268,#33356,.T.);
#52293=EDGE_CURVE('',#40269,#40267,#33357,.T.);
#52294=EDGE_CURVE('',#40270,#40271,#33358,.T.);
#52295=EDGE_CURVE('',#40267,#40271,#22986,.T.);
#52296=EDGE_CURVE('',#40270,#40269,#22987,.T.);
#52297=EDGE_CURVE('',#40272,#40273,#33359,.T.);
#52298=EDGE_CURVE('',#40268,#40273,#33360,.T.);
#52299=EDGE_CURVE('',#40272,#40266,#33361,.T.);
#52300=EDGE_CURVE('',#40274,#40275,#33362,.T.);
#52301=EDGE_CURVE('',#40271,#40275,#33363,.T.);
#52302=EDGE_CURVE('',#40274,#40270,#33364,.T.);
#52303=EDGE_CURVE('',#40276,#40277,#33365,.T.);
#52304=EDGE_CURVE('',#40273,#40277,#33366,.T.);
#52305=EDGE_CURVE('',#40276,#40272,#33367,.T.);
#52306=EDGE_CURVE('',#40277,#40274,#22988,.T.);
#52307=EDGE_CURVE('',#40275,#40276,#22989,.T.);
#52308=EDGE_CURVE('',#40278,#40278,#33368,.T.);
#52309=EDGE_CURVE('',#40278,#40279,#33369,.T.);
#52310=EDGE_CURVE('',#40279,#40279,#33370,.T.);
#52311=EDGE_CURVE('',#40280,#40280,#33371,.T.);
#52312=EDGE_CURVE('',#40280,#40281,#33372,.T.);
#52313=EDGE_CURVE('',#40281,#40281,#33373,.T.);
#52314=EDGE_CURVE('',#40282,#40283,#33374,.T.);
#52315=EDGE_CURVE('',#38947,#40283,#33375,.T.);
#52316=EDGE_CURVE('',#40282,#38946,#33376,.T.);
#52317=EDGE_CURVE('',#40284,#40285,#33377,.T.);
#52318=EDGE_CURVE('',#40283,#40285,#33378,.T.);
#52319=EDGE_CURVE('',#40284,#40282,#33379,.T.);
#52320=EDGE_CURVE('',#40286,#40287,#33380,.T.);
#52321=EDGE_CURVE('',#40285,#40287,#33381,.T.);
#52322=EDGE_CURVE('',#40286,#40284,#33382,.T.);
#52323=EDGE_CURVE('',#40288,#40289,#33383,.T.);
#52324=EDGE_CURVE('',#40287,#40289,#33384,.T.);
#52325=EDGE_CURVE('',#40288,#40286,#33385,.T.);
#52326=EDGE_CURVE('',#40290,#40291,#33386,.T.);
#52327=EDGE_CURVE('',#40289,#40291,#33387,.T.);
#52328=EDGE_CURVE('',#40290,#40288,#33388,.T.);
#52329=EDGE_CURVE('',#40292,#40293,#33389,.T.);
#52330=EDGE_CURVE('',#40291,#40293,#33390,.T.);
#52331=EDGE_CURVE('',#40292,#40290,#33391,.T.);
#52332=EDGE_CURVE('',#40294,#40295,#33392,.T.);
#52333=EDGE_CURVE('',#40293,#40295,#33393,.T.);
#52334=EDGE_CURVE('',#40294,#40292,#33394,.T.);
#52335=EDGE_CURVE('',#40296,#40297,#33395,.T.);
#52336=EDGE_CURVE('',#40295,#40297,#33396,.T.);
#52337=EDGE_CURVE('',#40296,#40294,#33397,.T.);
#52338=EDGE_CURVE('',#40297,#38959,#33398,.T.);
#52339=EDGE_CURVE('',#38958,#40296,#33399,.T.);
#52340=EDGE_CURVE('',#40298,#40299,#33400,.T.);
#52341=EDGE_CURVE('',#38963,#40299,#33401,.T.);
#52342=EDGE_CURVE('',#40298,#38962,#33402,.T.);
#52343=EDGE_CURVE('',#40300,#40301,#33403,.T.);
#52344=EDGE_CURVE('',#40299,#40301,#33404,.T.);
#52345=EDGE_CURVE('',#40300,#40298,#33405,.T.);
#52346=EDGE_CURVE('',#40302,#40303,#33406,.T.);
#52347=EDGE_CURVE('',#40301,#40303,#33407,.T.);
#52348=EDGE_CURVE('',#40302,#40300,#33408,.T.);
#52349=EDGE_CURVE('',#40304,#40305,#33409,.T.);
#52350=EDGE_CURVE('',#40303,#40305,#33410,.T.);
#52351=EDGE_CURVE('',#40304,#40302,#33411,.T.);
#52352=EDGE_CURVE('',#40306,#40307,#33412,.T.);
#52353=EDGE_CURVE('',#40305,#40307,#33413,.T.);
#52354=EDGE_CURVE('',#40306,#40304,#33414,.T.);
#52355=EDGE_CURVE('',#40308,#40309,#33415,.T.);
#52356=EDGE_CURVE('',#40307,#40309,#33416,.T.);
#52357=EDGE_CURVE('',#40308,#40306,#33417,.T.);
#52358=EDGE_CURVE('',#40310,#40311,#33418,.T.);
#52359=EDGE_CURVE('',#40309,#40311,#33419,.T.);
#52360=EDGE_CURVE('',#40310,#40308,#33420,.T.);
#52361=EDGE_CURVE('',#40312,#40313,#33421,.T.);
#52362=EDGE_CURVE('',#40311,#40313,#33422,.T.);
#52363=EDGE_CURVE('',#40312,#40310,#33423,.T.);
#52364=EDGE_CURVE('',#40313,#38975,#33424,.T.);
#52365=EDGE_CURVE('',#38974,#40312,#33425,.T.);
#52366=EDGE_CURVE('',#40314,#40315,#33426,.T.);
#52367=EDGE_CURVE('',#40316,#40315,#33427,.T.);
#52368=EDGE_CURVE('',#40317,#40316,#5733,.T.);
#52369=EDGE_CURVE('',#40314,#40317,#33428,.T.);
#52370=EDGE_CURVE('',#40318,#40319,#33429,.T.);
#52371=EDGE_CURVE('',#40315,#40319,#22990,.T.);
#52372=EDGE_CURVE('',#40318,#40314,#22991,.T.);
#52373=EDGE_CURVE('',#40320,#40318,#33430,.T.);
#52374=EDGE_CURVE('',#40320,#40321,#33431,.T.);
#52375=EDGE_CURVE('',#40319,#40321,#33432,.T.);
#52376=EDGE_CURVE('',#40322,#40323,#33433,.T.);
#52377=EDGE_CURVE('',#40321,#40323,#33434,.T.);
#52378=EDGE_CURVE('',#40322,#40320,#33435,.T.);
#52379=EDGE_CURVE('',#40324,#40325,#33436,.T.);
#52380=EDGE_CURVE('',#40323,#40325,#33437,.T.);
#52381=EDGE_CURVE('',#40324,#40322,#33438,.T.);
#52382=EDGE_CURVE('',#40326,#40327,#33439,.T.);
#52383=EDGE_CURVE('',#40325,#40327,#22992,.T.);
#52384=EDGE_CURVE('',#40326,#40324,#22993,.T.);
#52385=EDGE_CURVE('',#40328,#40329,#5734,.T.);
#52386=EDGE_CURVE('',#40327,#40328,#33440,.T.);
#52387=EDGE_CURVE('',#40329,#40326,#33441,.T.);
#52388=EDGE_CURVE('',#40330,#40331,#33442,.T.);
#52389=EDGE_CURVE('',#40332,#40331,#33443,.T.);
#52390=EDGE_CURVE('',#40333,#40332,#5735,.T.);
#52391=EDGE_CURVE('',#40330,#40333,#33444,.T.);
#52392=EDGE_CURVE('',#40334,#40335,#33445,.T.);
#52393=EDGE_CURVE('',#40331,#40335,#22994,.T.);
#52394=EDGE_CURVE('',#40334,#40330,#22995,.T.);
#52395=EDGE_CURVE('',#40336,#40337,#33446,.T.);
#52396=EDGE_CURVE('',#40335,#40337,#33447,.T.);
#52397=EDGE_CURVE('',#40336,#40334,#33448,.T.);
#52398=EDGE_CURVE('',#40338,#40339,#33449,.T.);
#52399=EDGE_CURVE('',#40337,#40339,#33450,.T.);
#52400=EDGE_CURVE('',#40338,#40336,#33451,.T.);
#52401=EDGE_CURVE('',#40340,#40341,#33452,.T.);
#52402=EDGE_CURVE('',#40339,#40341,#33453,.T.);
#52403=EDGE_CURVE('',#40340,#40338,#33454,.T.);
#52404=EDGE_CURVE('',#40342,#40343,#33455,.T.);
#52405=EDGE_CURVE('',#40341,#40343,#22996,.T.);
#52406=EDGE_CURVE('',#40342,#40340,#22997,.T.);
#52407=EDGE_CURVE('',#40344,#40345,#5736,.T.);
#52408=EDGE_CURVE('',#40343,#40344,#33456,.T.);
#52409=EDGE_CURVE('',#40345,#40342,#33457,.T.);
#52410=EDGE_CURVE('',#40346,#40347,#33458,.T.);
#52411=EDGE_CURVE('',#40348,#40347,#33459,.T.);
#52412=EDGE_CURVE('',#40349,#40348,#5737,.T.);
#52413=EDGE_CURVE('',#40346,#40349,#33460,.T.);
#52414=EDGE_CURVE('',#40350,#40351,#33461,.T.);
#52415=EDGE_CURVE('',#40347,#40351,#22998,.T.);
#52416=EDGE_CURVE('',#40350,#40346,#22999,.T.);
#52417=EDGE_CURVE('',#40352,#40350,#33462,.T.);
#52418=EDGE_CURVE('',#40352,#40353,#33463,.T.);
#52419=EDGE_CURVE('',#40351,#40353,#33464,.T.);
#52420=EDGE_CURVE('',#40354,#40355,#33465,.T.);
#52421=EDGE_CURVE('',#40353,#40355,#33466,.T.);
#52422=EDGE_CURVE('',#40354,#40352,#33467,.T.);
#52423=EDGE_CURVE('',#40356,#40357,#33468,.T.);
#52424=EDGE_CURVE('',#40355,#40357,#33469,.T.);
#52425=EDGE_CURVE('',#40356,#40354,#33470,.T.);
#52426=EDGE_CURVE('',#40358,#40359,#33471,.T.);
#52427=EDGE_CURVE('',#40357,#40359,#23000,.T.);
#52428=EDGE_CURVE('',#40358,#40356,#23001,.T.);
#52429=EDGE_CURVE('',#40360,#40361,#5738,.T.);
#52430=EDGE_CURVE('',#40359,#40360,#33472,.T.);
#52431=EDGE_CURVE('',#40361,#40358,#33473,.T.);
#52432=EDGE_CURVE('',#40362,#40363,#5739,.T.);
#52433=EDGE_CURVE('',#40364,#40362,#33474,.T.);
#52434=EDGE_CURVE('',#40364,#40365,#33475,.T.);
#52435=EDGE_CURVE('',#40363,#40365,#33476,.T.);
#52436=EDGE_CURVE('',#40366,#40367,#33477,.T.);
#52437=EDGE_CURVE('',#40365,#40367,#23002,.T.);
#52438=EDGE_CURVE('',#40366,#40364,#23003,.T.);
#52439=EDGE_CURVE('',#40368,#40369,#33478,.T.);
#52440=EDGE_CURVE('',#40367,#40369,#33479,.T.);
#52441=EDGE_CURVE('',#40368,#40366,#33480,.T.);
#52442=EDGE_CURVE('',#40370,#40371,#33481,.T.);
#52443=EDGE_CURVE('',#40369,#40371,#33482,.T.);
#52444=EDGE_CURVE('',#40370,#40368,#33483,.T.);
#52445=EDGE_CURVE('',#40372,#40373,#33484,.T.);
#52446=EDGE_CURVE('',#40371,#40373,#33485,.T.);
#52447=EDGE_CURVE('',#40372,#40370,#33486,.T.);
#52448=EDGE_CURVE('',#40374,#40375,#33487,.T.);
#52449=EDGE_CURVE('',#40373,#40375,#23004,.T.);
#52450=EDGE_CURVE('',#40374,#40372,#23005,.T.);
#52451=EDGE_CURVE('',#40376,#40377,#5740,.T.);
#52452=EDGE_CURVE('',#40375,#40376,#33488,.T.);
#52453=EDGE_CURVE('',#40377,#40374,#33489,.T.);
#52454=EDGE_CURVE('',#39043,#40378,#33490,.T.);
#52455=EDGE_CURVE('',#40379,#39042,#33491,.T.);
#52456=EDGE_CURVE('',#40379,#40378,#33492,.T.);
#52457=EDGE_CURVE('',#40380,#40381,#33493,.T.);
#52458=EDGE_CURVE('',#40378,#40381,#33494,.T.);
#52459=EDGE_CURVE('',#40380,#40379,#33495,.T.);
#52460=EDGE_CURVE('',#40382,#40383,#33496,.T.);
#52461=EDGE_CURVE('',#40381,#40383,#33497,.T.);
#52462=EDGE_CURVE('',#40382,#40380,#33498,.T.);
#52463=EDGE_CURVE('',#40384,#40385,#33499,.T.);
#52464=EDGE_CURVE('',#40383,#40385,#33500,.T.);
#52465=EDGE_CURVE('',#40384,#40382,#33501,.T.);
#52466=EDGE_CURVE('',#40386,#40387,#33502,.T.);
#52467=EDGE_CURVE('',#40385,#40387,#33503,.T.);
#52468=EDGE_CURVE('',#40386,#40384,#33504,.T.);
#52469=EDGE_CURVE('',#40388,#40389,#33505,.T.);
#52470=EDGE_CURVE('',#40387,#40389,#33506,.T.);
#52471=EDGE_CURVE('',#40388,#40386,#33507,.T.);
#52472=EDGE_CURVE('',#40390,#40391,#33508,.T.);
#52473=EDGE_CURVE('',#40389,#40391,#33509,.T.);
#52474=EDGE_CURVE('',#40390,#40388,#33510,.T.);
#52475=EDGE_CURVE('',#40392,#40393,#33511,.T.);
#52476=EDGE_CURVE('',#40391,#40393,#33512,.T.);
#52477=EDGE_CURVE('',#40392,#40390,#33513,.T.);
#52478=EDGE_CURVE('',#40393,#39055,#33514,.T.);
#52479=EDGE_CURVE('',#39054,#40392,#33515,.T.);
#52480=EDGE_CURVE('',#40394,#40395,#5741,.T.);
#52481=EDGE_CURVE('',#40396,#40394,#5742,.T.);
#52482=EDGE_CURVE('',#40396,#40397,#33516,.T.);
#52483=EDGE_CURVE('',#39059,#40397,#5743,.T.);
#52484=EDGE_CURVE('',#40395,#39058,#5744,.T.);
#52485=EDGE_CURVE('',#40398,#40399,#33517,.T.);
#52486=EDGE_CURVE('',#40397,#40399,#5745,.T.);
#52487=EDGE_CURVE('',#40398,#40396,#2005,.T.);
#52488=EDGE_CURVE('',#40400,#40401,#33518,.T.);
#52489=EDGE_CURVE('',#40399,#40401,#33519,.T.);
#52490=EDGE_CURVE('',#40400,#40398,#33520,.T.);
#52491=EDGE_CURVE('',#40402,#40403,#33521,.T.);
#52492=EDGE_CURVE('',#40401,#40403,#5746,.T.);
#52493=EDGE_CURVE('',#40402,#40400,#5747,.T.);
#52494=EDGE_CURVE('',#40404,#40405,#33522,.T.);
#52495=EDGE_CURVE('',#40403,#40405,#5748,.T.);
#52496=EDGE_CURVE('',#40404,#40402,#5749,.T.);
#52497=EDGE_CURVE('',#40406,#40407,#33523,.T.);
#52498=EDGE_CURVE('',#40405,#40407,#5750,.T.);
#52499=EDGE_CURVE('',#40406,#40404,#5751,.T.);
#52500=EDGE_CURVE('',#40408,#40409,#33524,.T.);
#52501=EDGE_CURVE('',#40407,#40409,#33525,.T.);
#52502=EDGE_CURVE('',#40408,#40406,#33526,.T.);
#52503=EDGE_CURVE('',#40410,#40411,#33527,.T.);
#52504=EDGE_CURVE('',#40409,#40411,#5752,.T.);
#52505=EDGE_CURVE('',#40410,#40408,#5753,.T.);
#52506=EDGE_CURVE('',#40412,#40413,#33528,.T.);
#52507=EDGE_CURVE('',#40411,#40413,#5754,.T.);
#52508=EDGE_CURVE('',#40414,#40410,#5755,.T.);
#52509=EDGE_CURVE('',#40415,#40414,#5756,.T.);
#52510=EDGE_CURVE('',#40416,#40415,#5757,.T.);
#52511=EDGE_CURVE('',#40417,#40416,#5758,.T.);
#52512=EDGE_CURVE('',#40418,#40417,#5759,.T.);
#52513=EDGE_CURVE('',#40412,#40418,#5760,.T.);
#52514=EDGE_CURVE('',#40419,#40420,#33529,.T.);
#52515=EDGE_CURVE('',#40413,#40420,#5761,.T.);
#52516=EDGE_CURVE('',#40419,#40412,#5762,.T.);
#52517=EDGE_CURVE('',#40421,#40422,#33530,.T.);
#52518=EDGE_CURVE('',#40420,#40422,#33531,.T.);
#52519=EDGE_CURVE('',#40421,#40419,#33532,.T.);
#52520=EDGE_CURVE('',#40423,#40424,#33533,.T.);
#52521=EDGE_CURVE('',#40422,#40424,#5763,.T.);
#52522=EDGE_CURVE('',#40423,#40421,#5764,.T.);
#52523=EDGE_CURVE('',#40425,#40426,#33534,.T.);
#52524=EDGE_CURVE('',#40424,#40426,#5765,.T.);
#52525=EDGE_CURVE('',#40425,#40423,#5766,.T.);
#52526=EDGE_CURVE('',#40427,#40428,#33535,.T.);
#52527=EDGE_CURVE('',#40426,#40428,#5767,.T.);
#52528=EDGE_CURVE('',#40427,#40425,#5768,.T.);
#52529=EDGE_CURVE('',#40429,#40430,#33536,.T.);
#52530=EDGE_CURVE('',#40428,#40430,#33537,.T.);
#52531=EDGE_CURVE('',#40429,#40427,#33538,.T.);
#52532=EDGE_CURVE('',#40431,#40432,#33539,.T.);
#52533=EDGE_CURVE('',#40430,#40432,#5769,.T.);
#52534=EDGE_CURVE('',#40431,#40429,#5770,.T.);
#52535=EDGE_CURVE('',#40433,#40434,#5771,.T.);
#52536=EDGE_CURVE('',#40433,#40435,#5772,.T.);
#52537=EDGE_CURVE('',#40435,#40436,#5773,.T.);
#52538=EDGE_CURVE('',#40436,#39095,#5774,.T.);
#52539=EDGE_CURVE('',#40432,#39096,#5775,.T.);
#52540=EDGE_CURVE('',#40437,#40431,#5776,.T.);
#52541=EDGE_CURVE('',#40434,#40437,#5777,.T.);
#52542=EDGE_CURVE('',#39719,#40438,#5778,.T.);
#52543=EDGE_CURVE('',#40439,#39711,#33540,.T.);
#52544=EDGE_CURVE('',#40439,#40438,#33541,.T.);
#52545=EDGE_CURVE('',#40440,#40441,#33542,.T.);
#52546=EDGE_CURVE('',#40438,#40441,#33543,.T.);
#52547=EDGE_CURVE('',#40440,#40439,#2006,.T.);
#52548=EDGE_CURVE('',#40442,#40443,#33544,.T.);
#52549=EDGE_CURVE('',#40441,#40443,#5779,.T.);
#52550=EDGE_CURVE('',#40442,#40440,#5780,.T.);
#52551=EDGE_CURVE('',#40444,#40445,#33545,.T.);
#52552=EDGE_CURVE('',#40443,#40445,#5781,.T.);
#52553=EDGE_CURVE('',#40444,#40442,#5782,.T.);
#52554=EDGE_CURVE('',#40446,#40447,#5783,.T.);
#52555=EDGE_CURVE('',#40445,#40447,#33546,.T.);
#52556=EDGE_CURVE('',#40448,#40444,#33547,.T.);
#52557=EDGE_CURVE('',#40448,#40446,#2007,.T.);
#52558=EDGE_CURVE('',#40449,#40450,#5784,.T.);
#52559=EDGE_CURVE('',#40449,#40446,#33548,.T.);
#52560=EDGE_CURVE('',#40450,#40448,#33549,.T.);
#52561=EDGE_CURVE('',#40449,#40447,#5785,.T.);
#52562=EDGE_CURVE('',#40451,#40452,#5786,.T.);
#52563=EDGE_CURVE('',#40447,#40452,#5787,.T.);
#52564=EDGE_CURVE('',#40453,#40449,#5788,.T.);
#52565=EDGE_CURVE('',#40454,#40453,#5789,.T.);
#52566=EDGE_CURVE('',#40455,#40454,#5790,.T.);
#52567=EDGE_CURVE('',#40456,#40455,#5791,.T.);
#52568=EDGE_CURVE('',#40457,#40456,#5792,.T.);
#52569=EDGE_CURVE('',#40458,#40457,#5793,.T.);
#52570=EDGE_CURVE('',#40451,#40458,#5794,.T.);
#52571=EDGE_CURVE('',#40451,#40459,#33550,.T.);
#52572=EDGE_CURVE('',#40459,#40452,#5795,.T.);
#52573=EDGE_CURVE('',#40460,#40461,#33551,.T.);
#52574=EDGE_CURVE('',#40460,#40459,#5796,.T.);
#52575=EDGE_CURVE('',#40461,#40451,#5797,.T.);
#52576=EDGE_CURVE('',#40462,#40460,#33552,.T.);
#52577=EDGE_CURVE('',#40462,#40463,#33553,.T.);
#52578=EDGE_CURVE('',#40452,#40463,#33554,.T.);
#52579=EDGE_CURVE('',#40464,#40465,#33555,.T.);
#52580=EDGE_CURVE('',#40463,#40465,#5798,.T.);
#52581=EDGE_CURVE('',#40464,#40462,#5799,.T.);
#52582=EDGE_CURVE('',#40466,#40467,#33556,.T.);
#52583=EDGE_CURVE('',#40465,#40467,#5800,.T.);
#52584=EDGE_CURVE('',#40466,#40464,#5801,.T.);
#52585=EDGE_CURVE('',#40468,#40469,#33557,.T.);
#52586=EDGE_CURVE('',#40467,#40469,#33558,.T.);
#52587=EDGE_CURVE('',#40468,#40466,#33559,.T.);
#52588=EDGE_CURVE('',#40469,#39725,#5802,.T.);
#52589=EDGE_CURVE('',#39735,#40468,#2008,.T.);
#52590=EDGE_CURVE('',#40470,#40471,#5803,.T.);
#52591=EDGE_CURVE('',#40472,#40470,#5804,.T.);
#52592=EDGE_CURVE('',#40472,#40473,#5805,.T.);
#52593=EDGE_CURVE('',#39131,#40473,#5806,.T.);
#52594=EDGE_CURVE('',#39129,#40474,#5807,.T.);
#52595=EDGE_CURVE('',#40474,#40475,#5808,.T.);
#52596=EDGE_CURVE('',#40475,#40476,#5809,.T.);
#52597=EDGE_CURVE('',#40476,#40477,#5810,.T.);
#52598=EDGE_CURVE('',#40478,#40477,#5811,.T.);
#52599=EDGE_CURVE('',#40471,#40478,#5812,.T.);
#52600=EDGE_CURVE('',#40472,#40479,#33560,.T.);
#52601=EDGE_CURVE('',#40479,#40473,#2009,.T.);
#52602=EDGE_CURVE('',#40480,#40481,#33561,.T.);
#52603=EDGE_CURVE('',#40480,#40479,#2010,.T.);
#52604=EDGE_CURVE('',#40481,#40472,#2011,.T.);
#52605=EDGE_CURVE('',#40482,#40480,#33562,.T.);
#52606=EDGE_CURVE('',#40482,#40483,#33563,.T.);
#52607=EDGE_CURVE('',#40473,#40483,#33564,.T.);
#52608=EDGE_CURVE('',#40484,#40485,#33565,.T.);
#52609=EDGE_CURVE('',#40483,#40485,#5813,.T.);
#52610=EDGE_CURVE('',#40484,#40482,#5814,.T.);
#52611=EDGE_CURVE('',#40486,#40487,#33566,.T.);
#52612=EDGE_CURVE('',#40485,#40487,#5815,.T.);
#52613=EDGE_CURVE('',#40486,#40484,#5816,.T.);
#52614=EDGE_CURVE('',#40488,#40489,#33567,.T.);
#52615=EDGE_CURVE('',#40487,#40489,#33568,.T.);
#52616=EDGE_CURVE('',#40488,#40486,#5817,.T.);
#52617=EDGE_CURVE('',#39710,#40488,#2012,.T.);
#52618=EDGE_CURVE('',#40489,#39718,#5818,.T.);
#52619=EDGE_CURVE('',#40490,#39142,#2013,.T.);
#52620=EDGE_CURVE('',#40490,#40491,#33569,.T.);
#52621=EDGE_CURVE('',#39143,#40491,#2014,.T.);
#52622=EDGE_CURVE('',#40492,#40493,#5819,.T.);
#52623=EDGE_CURVE('',#40491,#40492,#5820,.T.);
#52624=EDGE_CURVE('',#40494,#40490,#5821,.T.);
#52625=EDGE_CURVE('',#40494,#40495,#5822,.T.);
#52626=EDGE_CURVE('',#40496,#40495,#5823,.T.);
#52627=EDGE_CURVE('',#40493,#40496,#5824,.T.);
#52628=EDGE_CURVE('',#40494,#40497,#5825,.T.);
#52629=EDGE_CURVE('',#40497,#40495,#33570,.T.);
#52630=EDGE_CURVE('',#40498,#40499,#5826,.T.);
#52631=EDGE_CURVE('',#40498,#40497,#33571,.T.);
#52632=EDGE_CURVE('',#40500,#40494,#2015,.T.);
#52633=EDGE_CURVE('',#40500,#40499,#33572,.T.);
#52634=EDGE_CURVE('',#40501,#40498,#33573,.T.);
#52635=EDGE_CURVE('',#40495,#40501,#5827,.T.);
#52636=EDGE_CURVE('',#40502,#40503,#33574,.T.);
#52637=EDGE_CURVE('',#40499,#40503,#5828,.T.);
#52638=EDGE_CURVE('',#40502,#40500,#5829,.T.);
#52639=EDGE_CURVE('',#40504,#40505,#33575,.T.);
#52640=EDGE_CURVE('',#40503,#40505,#5830,.T.);
#52641=EDGE_CURVE('',#40504,#40502,#5831,.T.);
#52642=EDGE_CURVE('',#40506,#40507,#33576,.T.);
#52643=EDGE_CURVE('',#40505,#40507,#5832,.T.);
#52644=EDGE_CURVE('',#40506,#40504,#33577,.T.);
#52645=EDGE_CURVE('',#40507,#39743,#5833,.T.);
#52646=EDGE_CURVE('',#39734,#40506,#5834,.T.);
#52647=EDGE_CURVE('',#40431,#40481,#5835,.T.);
#52648=EDGE_CURVE('',#40480,#40429,#5836,.T.);
#52649=EDGE_CURVE('',#40419,#40448,#5837,.T.);
#52650=EDGE_CURVE('',#40450,#40412,#5838,.T.);
#52651=EDGE_CURVE('',#40410,#40461,#5839,.T.);
#52652=EDGE_CURVE('',#40460,#40408,#5840,.T.);
#52653=EDGE_CURVE('',#40398,#40498,#5841,.T.);
#52654=EDGE_CURVE('',#40501,#40396,#5842,.T.);
#52655=EDGE_CURVE('',#40508,#40509,#33578,.T.);
#52656=EDGE_CURVE('',#40319,#40508,#23006,.T.);
#52657=EDGE_CURVE('',#40509,#40321,#23007,.T.);
#52658=EDGE_CURVE('',#40375,#40510,#23008,.T.);
#52659=EDGE_CURVE('',#40511,#40376,#23009,.T.);
#52660=EDGE_CURVE('',#40510,#40511,#33579,.T.);
#52661=EDGE_CURVE('',#40335,#40512,#23010,.T.);
#52662=EDGE_CURVE('',#40513,#40337,#23011,.T.);
#52663=EDGE_CURVE('',#40512,#40513,#33580,.T.);
#52664=EDGE_CURVE('',#40332,#40514,#23012,.T.);
#52665=EDGE_CURVE('',#40515,#40331,#23013,.T.);
#52666=EDGE_CURVE('',#40514,#40515,#33581,.T.);
#52667=EDGE_CURVE('',#40327,#40516,#23014,.T.);
#52668=EDGE_CURVE('',#40517,#40328,#23015,.T.);
#52669=EDGE_CURVE('',#40516,#40517,#33582,.T.);
#52670=EDGE_CURVE('',#40323,#40518,#23016,.T.);
#52671=EDGE_CURVE('',#40519,#40325,#23017,.T.);
#52672=EDGE_CURVE('',#40518,#40519,#33583,.T.);
#52673=EDGE_CURVE('',#40316,#40520,#23018,.T.);
#52674=EDGE_CURVE('',#40521,#40315,#23019,.T.);
#52675=EDGE_CURVE('',#40520,#40521,#33584,.T.);
#52676=EDGE_CURVE('',#40359,#40522,#23020,.T.);
#52677=EDGE_CURVE('',#40523,#40360,#23021,.T.);
#52678=EDGE_CURVE('',#40522,#40523,#33585,.T.);
#52679=EDGE_CURVE('',#40348,#40524,#23022,.T.);
#52680=EDGE_CURVE('',#40525,#40347,#23023,.T.);
#52681=EDGE_CURVE('',#40524,#40525,#33586,.T.);
#52682=EDGE_CURVE('',#40526,#40527,#33587,.T.);
#52683=EDGE_CURVE('',#40117,#40526,#23024,.T.);
#52684=EDGE_CURVE('',#40527,#40112,#23025,.T.);
#52685=EDGE_CURVE('',#40031,#40528,#23026,.T.);
#52686=EDGE_CURVE('',#40529,#40035,#23027,.T.);
#52687=EDGE_CURVE('',#40528,#40529,#33588,.T.);
#52688=EDGE_CURVE('',#40018,#40530,#23028,.T.);
#52689=EDGE_CURVE('',#40531,#40017,#23029,.T.);
#52690=EDGE_CURVE('',#40530,#40531,#33589,.T.);
#52691=EDGE_CURVE('',#40024,#40532,#23030,.T.);
#52692=EDGE_CURVE('',#40533,#40020,#23031,.T.);
#52693=EDGE_CURVE('',#40532,#40533,#33590,.T.);
#52694=EDGE_CURVE('',#40032,#40534,#23032,.T.);
#52695=EDGE_CURVE('',#40535,#40028,#23033,.T.);
#52696=EDGE_CURVE('',#40534,#40535,#33591,.T.);
#52697=EDGE_CURVE('',#39998,#40536,#23034,.T.);
#52698=EDGE_CURVE('',#40537,#39997,#23035,.T.);
#52699=EDGE_CURVE('',#40536,#40537,#33592,.T.);
#52700=EDGE_CURVE('',#40004,#40538,#23036,.T.);
#52701=EDGE_CURVE('',#40539,#40000,#23037,.T.);
#52702=EDGE_CURVE('',#40538,#40539,#33593,.T.);
#52703=EDGE_CURVE('',#40012,#40540,#23038,.T.);
#52704=EDGE_CURVE('',#40541,#40008,#23039,.T.);
#52705=EDGE_CURVE('',#40540,#40541,#33594,.T.);
#52706=EDGE_CURVE('',#40011,#40542,#23040,.T.);
#52707=EDGE_CURVE('',#40543,#40015,#23041,.T.);
#52708=EDGE_CURVE('',#40542,#40543,#33595,.T.);
#52709=EDGE_CURVE('',#39861,#40544,#23042,.T.);
#52710=EDGE_CURVE('',#40545,#39862,#23043,.T.);
#52711=EDGE_CURVE('',#40544,#40545,#33596,.T.);
#52712=EDGE_CURVE('',#39853,#40546,#23044,.T.);
#52713=EDGE_CURVE('',#40547,#39857,#23045,.T.);
#52714=EDGE_CURVE('',#40546,#40547,#33597,.T.);
#52715=EDGE_CURVE('',#39848,#40548,#23046,.T.);
#52716=EDGE_CURVE('',#40549,#39847,#23047,.T.);
#52717=EDGE_CURVE('',#40548,#40549,#33598,.T.);
#52718=EDGE_CURVE('',#39854,#40550,#23048,.T.);
#52719=EDGE_CURVE('',#40551,#39850,#23049,.T.);
#52720=EDGE_CURVE('',#40550,#40551,#33599,.T.);
#52721=EDGE_CURVE('',#40107,#40552,#23050,.T.);
#52722=EDGE_CURVE('',#40553,#40111,#23051,.T.);
#52723=EDGE_CURVE('',#40552,#40553,#33600,.T.);
#52724=EDGE_CURVE('',#40102,#40554,#23052,.T.);
#52725=EDGE_CURVE('',#40555,#40101,#23053,.T.);
#52726=EDGE_CURVE('',#40554,#40555,#33601,.T.);
#52727=EDGE_CURVE('',#40108,#40556,#23054,.T.);
#52728=EDGE_CURVE('',#40557,#40104,#23055,.T.);
#52729=EDGE_CURVE('',#40556,#40557,#33602,.T.);
#52730=EDGE_CURVE('',#40274,#40558,#23056,.T.);
#52731=EDGE_CURVE('',#40559,#40270,#23057,.T.);
#52732=EDGE_CURVE('',#40558,#40559,#33603,.T.);
#52733=EDGE_CURVE('',#40273,#40560,#23058,.T.);
#52734=EDGE_CURVE('',#40561,#40277,#23059,.T.);
#52735=EDGE_CURVE('',#40560,#40561,#33604,.T.);
#52736=EDGE_CURVE('',#40562,#40563,#33605,.T.);
#52737=EDGE_CURVE('',#40269,#40562,#23060,.T.);
#52738=EDGE_CURVE('',#40563,#40268,#23061,.T.);
#52739=EDGE_CURVE('',#39903,#40564,#23062,.T.);
#52740=EDGE_CURVE('',#40565,#39907,#23063,.T.);
#52741=EDGE_CURVE('',#40564,#40565,#33606,.T.);
#52742=EDGE_CURVE('',#39898,#40566,#23064,.T.);
#52743=EDGE_CURVE('',#40567,#39897,#23065,.T.);
#52744=EDGE_CURVE('',#40566,#40567,#33607,.T.);
#52745=EDGE_CURVE('',#39904,#40568,#23066,.T.);
#52746=EDGE_CURVE('',#40569,#39900,#23067,.T.);
#52747=EDGE_CURVE('',#40568,#40569,#33608,.T.);
#52748=EDGE_CURVE('',#39911,#40570,#23068,.T.);
#52749=EDGE_CURVE('',#40571,#39908,#23069,.T.);
#52750=EDGE_CURVE('',#40570,#40571,#33609,.T.);
#52751=EDGE_CURVE('',#39919,#40572,#23070,.T.);
#52752=EDGE_CURVE('',#40573,#39923,#23071,.T.);
#52753=EDGE_CURVE('',#40572,#40573,#33610,.T.);
#52754=EDGE_CURVE('',#39914,#40574,#23072,.T.);
#52755=EDGE_CURVE('',#40575,#39913,#23073,.T.);
#52756=EDGE_CURVE('',#40574,#40575,#33611,.T.);
#52757=EDGE_CURVE('',#39920,#40576,#23074,.T.);
#52758=EDGE_CURVE('',#40577,#39916,#23075,.T.);
#52759=EDGE_CURVE('',#40576,#40577,#33612,.T.);
#52760=EDGE_CURVE('',#39927,#40578,#23076,.T.);
#52761=EDGE_CURVE('',#40579,#39924,#23077,.T.);
#52762=EDGE_CURVE('',#40578,#40579,#33613,.T.);
#52763=EDGE_CURVE('',#40172,#40580,#23078,.T.);
#52764=EDGE_CURVE('',#40581,#40171,#23079,.T.);
#52765=EDGE_CURVE('',#40580,#40581,#33614,.T.);
#52766=EDGE_CURVE('',#40178,#40582,#23080,.T.);
#52767=EDGE_CURVE('',#40583,#40174,#23081,.T.);
#52768=EDGE_CURVE('',#40582,#40583,#33615,.T.);
#52769=EDGE_CURVE('',#40186,#40584,#23082,.T.);
#52770=EDGE_CURVE('',#40585,#40182,#23083,.T.);
#52771=EDGE_CURVE('',#40584,#40585,#33616,.T.);
#52772=EDGE_CURVE('',#40177,#40586,#23084,.T.);
#52773=EDGE_CURVE('',#40587,#40181,#23085,.T.);
#52774=EDGE_CURVE('',#40586,#40587,#33617,.T.);
#52775=EDGE_CURVE('',#40136,#40588,#23086,.T.);
#52776=EDGE_CURVE('',#40589,#40135,#23087,.T.);
#52777=EDGE_CURVE('',#40588,#40589,#33618,.T.);
#52778=EDGE_CURVE('',#40142,#40590,#23088,.T.);
#52779=EDGE_CURVE('',#40591,#40138,#23089,.T.);
#52780=EDGE_CURVE('',#40590,#40591,#33619,.T.);
#52781=EDGE_CURVE('',#40149,#40592,#23090,.T.);
#52782=EDGE_CURVE('',#40593,#40153,#23091,.T.);
#52783=EDGE_CURVE('',#40592,#40593,#33620,.T.);
#52784=EDGE_CURVE('',#40141,#40594,#23092,.T.);
#52785=EDGE_CURVE('',#40595,#40145,#23093,.T.);
#52786=EDGE_CURVE('',#40594,#40595,#33621,.T.);
#52787=EDGE_CURVE('',#39987,#40596,#23094,.T.);
#52788=EDGE_CURVE('',#40597,#39991,#23095,.T.);
#52789=EDGE_CURVE('',#40596,#40597,#33622,.T.);
#52790=EDGE_CURVE('',#39982,#40598,#23096,.T.);
#52791=EDGE_CURVE('',#40599,#39981,#23097,.T.);
#52792=EDGE_CURVE('',#40598,#40599,#33623,.T.);
#52793=EDGE_CURVE('',#39988,#40600,#23098,.T.);
#52794=EDGE_CURVE('',#40601,#39984,#23099,.T.);
#52795=EDGE_CURVE('',#40600,#40601,#33624,.T.);
#52796=EDGE_CURVE('',#39995,#40602,#23100,.T.);
#52797=EDGE_CURVE('',#40603,#39992,#23101,.T.);
#52798=EDGE_CURVE('',#40602,#40603,#33625,.T.);
#52799=EDGE_CURVE('',#40051,#40604,#23102,.T.);
#52800=EDGE_CURVE('',#40605,#40048,#23103,.T.);
#52801=EDGE_CURVE('',#40604,#40605,#33626,.T.);
#52802=EDGE_CURVE('',#40043,#40606,#23104,.T.);
#52803=EDGE_CURVE('',#40607,#40047,#23105,.T.);
#52804=EDGE_CURVE('',#40606,#40607,#33627,.T.);
#52805=EDGE_CURVE('',#40038,#40608,#23106,.T.);
#52806=EDGE_CURVE('',#40609,#40037,#23107,.T.);
#52807=EDGE_CURVE('',#40608,#40609,#33628,.T.);
#52808=EDGE_CURVE('',#40044,#40610,#23108,.T.);
#52809=EDGE_CURVE('',#40611,#40040,#23109,.T.);
#52810=EDGE_CURVE('',#40610,#40611,#33629,.T.);
#52811=EDGE_CURVE('',#40070,#40612,#23110,.T.);
#52812=EDGE_CURVE('',#40613,#40069,#23111,.T.);
#52813=EDGE_CURVE('',#40612,#40613,#33630,.T.);
#52814=EDGE_CURVE('',#40076,#40614,#23112,.T.);
#52815=EDGE_CURVE('',#40615,#40072,#23113,.T.);
#52816=EDGE_CURVE('',#40614,#40615,#33631,.T.);
#52817=EDGE_CURVE('',#40083,#40616,#23114,.T.);
#52818=EDGE_CURVE('',#40617,#40080,#23115,.T.);
#52819=EDGE_CURVE('',#40616,#40617,#33632,.T.);
#52820=EDGE_CURVE('',#40075,#40618,#23116,.T.);
#52821=EDGE_CURVE('',#40619,#40079,#23117,.T.);
#52822=EDGE_CURVE('',#40618,#40619,#33633,.T.);
#52823=EDGE_CURVE('',#40262,#40620,#23118,.T.);
#52824=EDGE_CURVE('',#40621,#40258,#23119,.T.);
#52825=EDGE_CURVE('',#40620,#40621,#33634,.T.);
#52826=EDGE_CURVE('',#40261,#40622,#23120,.T.);
#52827=EDGE_CURVE('',#40623,#40265,#23121,.T.);
#52828=EDGE_CURVE('',#40622,#40623,#33635,.T.);
#52829=EDGE_CURVE('',#40256,#40624,#23122,.T.);
#52830=EDGE_CURVE('',#40625,#40255,#23123,.T.);
#52831=EDGE_CURVE('',#40624,#40625,#33636,.T.);
#52832=EDGE_CURVE('',#40162,#40626,#23124,.T.);
#52833=EDGE_CURVE('',#40627,#40158,#23125,.T.);
#52834=EDGE_CURVE('',#40626,#40627,#33637,.T.);
#52835=EDGE_CURVE('',#40169,#40628,#23126,.T.);
#52836=EDGE_CURVE('',#40629,#40166,#23127,.T.);
#52837=EDGE_CURVE('',#40628,#40629,#33638,.T.);
#52838=EDGE_CURVE('',#40161,#40630,#23128,.T.);
#52839=EDGE_CURVE('',#40631,#40165,#23129,.T.);
#52840=EDGE_CURVE('',#40630,#40631,#33639,.T.);
#52841=EDGE_CURVE('',#40156,#40632,#23130,.T.);
#52842=EDGE_CURVE('',#40633,#40155,#23131,.T.);
#52843=EDGE_CURVE('',#40632,#40633,#33640,.T.);
#52844=EDGE_CURVE('',#40125,#40634,#23132,.T.);
#52845=EDGE_CURVE('',#40635,#40129,#23133,.T.);
#52846=EDGE_CURVE('',#40634,#40635,#33641,.T.);
#52847=EDGE_CURVE('',#40120,#40636,#23134,.T.);
#52848=EDGE_CURVE('',#40637,#40119,#23135,.T.);
#52849=EDGE_CURVE('',#40636,#40637,#33642,.T.);
#52850=EDGE_CURVE('',#40126,#40638,#23136,.T.);
#52851=EDGE_CURVE('',#40639,#40122,#23137,.T.);
#52852=EDGE_CURVE('',#40638,#40639,#33643,.T.);
#52853=EDGE_CURVE('',#40133,#40640,#23138,.T.);
#52854=EDGE_CURVE('',#40641,#40130,#23139,.T.);
#52855=EDGE_CURVE('',#40640,#40641,#33644,.T.);
#52856=EDGE_CURVE('',#40059,#40642,#23140,.T.);
#52857=EDGE_CURVE('',#40643,#40063,#23141,.T.);
#52858=EDGE_CURVE('',#40642,#40643,#33645,.T.);
#52859=EDGE_CURVE('',#40054,#40644,#23142,.T.);
#52860=EDGE_CURVE('',#40645,#40053,#23143,.T.);
#52861=EDGE_CURVE('',#40644,#40645,#33646,.T.);
#52862=EDGE_CURVE('',#40060,#40646,#23144,.T.);
#52863=EDGE_CURVE('',#40647,#40056,#23145,.T.);
#52864=EDGE_CURVE('',#40646,#40647,#33647,.T.);
#52865=EDGE_CURVE('',#40067,#40648,#23146,.T.);
#52866=EDGE_CURVE('',#40649,#40064,#23147,.T.);
#52867=EDGE_CURVE('',#40648,#40649,#33648,.T.);
#52868=EDGE_CURVE('',#39966,#40650,#23148,.T.);
#52869=EDGE_CURVE('',#40651,#39965,#23149,.T.);
#52870=EDGE_CURVE('',#40650,#40651,#33649,.T.);
#52871=EDGE_CURVE('',#39972,#40652,#23150,.T.);
#52872=EDGE_CURVE('',#40653,#39968,#23151,.T.);
#52873=EDGE_CURVE('',#40652,#40653,#33650,.T.);
#52874=EDGE_CURVE('',#39979,#40654,#23152,.T.);
#52875=EDGE_CURVE('',#40655,#39976,#23153,.T.);
#52876=EDGE_CURVE('',#40654,#40655,#33651,.T.);
#52877=EDGE_CURVE('',#39971,#40656,#23154,.T.);
#52878=EDGE_CURVE('',#40657,#39975,#23155,.T.);
#52879=EDGE_CURVE('',#40656,#40657,#33652,.T.);
#52880=EDGE_CURVE('',#39930,#40658,#23156,.T.);
#52881=EDGE_CURVE('',#40659,#39929,#23157,.T.);
#52882=EDGE_CURVE('',#40658,#40659,#33653,.T.);
#52883=EDGE_CURVE('',#39936,#40660,#23158,.T.);
#52884=EDGE_CURVE('',#40661,#39932,#23159,.T.);
#52885=EDGE_CURVE('',#40660,#40661,#33654,.T.);
#52886=EDGE_CURVE('',#39943,#40662,#23160,.T.);
#52887=EDGE_CURVE('',#40663,#39940,#23161,.T.);
#52888=EDGE_CURVE('',#40662,#40663,#33655,.T.);
#52889=EDGE_CURVE('',#39935,#40664,#23162,.T.);
#52890=EDGE_CURVE('',#40665,#39939,#23163,.T.);
#52891=EDGE_CURVE('',#40664,#40665,#33656,.T.);
#52892=EDGE_CURVE('',#39946,#40666,#23164,.T.);
#52893=EDGE_CURVE('',#40667,#39945,#23165,.T.);
#52894=EDGE_CURVE('',#40666,#40667,#33657,.T.);
#52895=EDGE_CURVE('',#39952,#40668,#23166,.T.);
#52896=EDGE_CURVE('',#40669,#39948,#23167,.T.);
#52897=EDGE_CURVE('',#40668,#40669,#33658,.T.);
#52898=EDGE_CURVE('',#39960,#40670,#23168,.T.);
#52899=EDGE_CURVE('',#40671,#39956,#23169,.T.);
#52900=EDGE_CURVE('',#40670,#40671,#33659,.T.);
#52901=EDGE_CURVE('',#39951,#40672,#23170,.T.);
#52902=EDGE_CURVE('',#40673,#39955,#23171,.T.);
#52903=EDGE_CURVE('',#40672,#40673,#33660,.T.);
#52904=EDGE_CURVE('',#39794,#40674,#23172,.T.);
#52905=EDGE_CURVE('',#40675,#39790,#23173,.T.);
#52906=EDGE_CURVE('',#40674,#40675,#33661,.T.);
#52907=EDGE_CURVE('',#39793,#40676,#23174,.T.);
#52908=EDGE_CURVE('',#40677,#39797,#23175,.T.);
#52909=EDGE_CURVE('',#40676,#40677,#33662,.T.);
#52910=EDGE_CURVE('',#40678,#40679,#33663,.T.);
#52911=EDGE_CURVE('',#39781,#40678,#23176,.T.);
#52912=EDGE_CURVE('',#40679,#39780,#23177,.T.);
#52913=EDGE_CURVE('',#39786,#40680,#23178,.T.);
#52914=EDGE_CURVE('',#40681,#39782,#23179,.T.);
#52915=EDGE_CURVE('',#40680,#40681,#33664,.T.);
#52916=EDGE_CURVE('',#40197,#40682,#23180,.T.);
#52917=EDGE_CURVE('',#40683,#40201,#23181,.T.);
#52918=EDGE_CURVE('',#40682,#40683,#33665,.T.);
#52919=EDGE_CURVE('',#40192,#40684,#23182,.T.);
#52920=EDGE_CURVE('',#40685,#40191,#23183,.T.);
#52921=EDGE_CURVE('',#40684,#40685,#33666,.T.);
#52922=EDGE_CURVE('',#40198,#40686,#23184,.T.);
#52923=EDGE_CURVE('',#40687,#40194,#23185,.T.);
#52924=EDGE_CURVE('',#40686,#40687,#33667,.T.);
#52925=EDGE_CURVE('',#40205,#40688,#23186,.T.);
#52926=EDGE_CURVE('',#40689,#40202,#23187,.T.);
#52927=EDGE_CURVE('',#40688,#40689,#33668,.T.);
#52928=EDGE_CURVE('',#39887,#40690,#23188,.T.);
#52929=EDGE_CURVE('',#40691,#39891,#23189,.T.);
#52930=EDGE_CURVE('',#40690,#40691,#33669,.T.);
#52931=EDGE_CURVE('',#39882,#40692,#23190,.T.);
#52932=EDGE_CURVE('',#40693,#39881,#23191,.T.);
#52933=EDGE_CURVE('',#40692,#40693,#33670,.T.);
#52934=EDGE_CURVE('',#39888,#40694,#23192,.T.);
#52935=EDGE_CURVE('',#40695,#39884,#23193,.T.);
#52936=EDGE_CURVE('',#40694,#40695,#33671,.T.);
#52937=EDGE_CURVE('',#39895,#40696,#23194,.T.);
#52938=EDGE_CURVE('',#40697,#39892,#23195,.T.);
#52939=EDGE_CURVE('',#40696,#40697,#33672,.T.);
#52940=EDGE_CURVE('',#39871,#40698,#23196,.T.);
#52941=EDGE_CURVE('',#40699,#39875,#23197,.T.);
#52942=EDGE_CURVE('',#40698,#40699,#33673,.T.);
#52943=EDGE_CURVE('',#39866,#40700,#23198,.T.);
#52944=EDGE_CURVE('',#40701,#39865,#23199,.T.);
#52945=EDGE_CURVE('',#40700,#40701,#33674,.T.);
#52946=EDGE_CURVE('',#39872,#40702,#23200,.T.);
#52947=EDGE_CURVE('',#40703,#39868,#23201,.T.);
#52948=EDGE_CURVE('',#40702,#40703,#33675,.T.);
#52949=EDGE_CURVE('',#39879,#40704,#23202,.T.);
#52950=EDGE_CURVE('',#40705,#39876,#23203,.T.);
#52951=EDGE_CURVE('',#40704,#40705,#33676,.T.);
#52952=EDGE_CURVE('',#40086,#40706,#23204,.T.);
#52953=EDGE_CURVE('',#40707,#40085,#23205,.T.);
#52954=EDGE_CURVE('',#40706,#40707,#33677,.T.);
#52955=EDGE_CURVE('',#40092,#40708,#23206,.T.);
#52956=EDGE_CURVE('',#40709,#40088,#23207,.T.);
#52957=EDGE_CURVE('',#40708,#40709,#33678,.T.);
#52958=EDGE_CURVE('',#40099,#40710,#23208,.T.);
#52959=EDGE_CURVE('',#40711,#40096,#23209,.T.);
#52960=EDGE_CURVE('',#40710,#40711,#33679,.T.);
#52961=EDGE_CURVE('',#40091,#40712,#23210,.T.);
#52962=EDGE_CURVE('',#40713,#40095,#23211,.T.);
#52963=EDGE_CURVE('',#40712,#40713,#33680,.T.);
#52964=EDGE_CURVE('',#40214,#40714,#23212,.T.);
#52965=EDGE_CURVE('',#40715,#40210,#23213,.T.);
#52966=EDGE_CURVE('',#40714,#40715,#33681,.T.);
#52967=EDGE_CURVE('',#40221,#40716,#23214,.T.);
#52968=EDGE_CURVE('',#40717,#40218,#23215,.T.);
#52969=EDGE_CURVE('',#40716,#40717,#33682,.T.);
#52970=EDGE_CURVE('',#40213,#40718,#23216,.T.);
#52971=EDGE_CURVE('',#40719,#40217,#23217,.T.);
#52972=EDGE_CURVE('',#40718,#40719,#33683,.T.);
#52973=EDGE_CURVE('',#40208,#40720,#23218,.T.);
#52974=EDGE_CURVE('',#40721,#40207,#23219,.T.);
#52975=EDGE_CURVE('',#40720,#40721,#33684,.T.);
#52976=EDGE_CURVE('',#39813,#40722,#23220,.T.);
#52977=EDGE_CURVE('',#40723,#39810,#23221,.T.);
#52978=EDGE_CURVE('',#40722,#40723,#33685,.T.);
#52979=EDGE_CURVE('',#39805,#40724,#23222,.T.);
#52980=EDGE_CURVE('',#40725,#39809,#23223,.T.);
#52981=EDGE_CURVE('',#40724,#40725,#33686,.T.);
#52982=EDGE_CURVE('',#40726,#40727,#33687,.T.);
#52983=EDGE_CURVE('',#39801,#40726,#23224,.T.);
#52984=EDGE_CURVE('',#40727,#39800,#23225,.T.);
#52985=EDGE_CURVE('',#39806,#40728,#23226,.T.);
#52986=EDGE_CURVE('',#40729,#39802,#23227,.T.);
#52987=EDGE_CURVE('',#40728,#40729,#33688,.T.);
#52988=EDGE_CURVE('',#40229,#40730,#23228,.T.);
#52989=EDGE_CURVE('',#40731,#40233,#23229,.T.);
#52990=EDGE_CURVE('',#40730,#40731,#33689,.T.);
#52991=EDGE_CURVE('',#40224,#40732,#23230,.T.);
#52992=EDGE_CURVE('',#40733,#40223,#23231,.T.);
#52993=EDGE_CURVE('',#40732,#40733,#33690,.T.);
#52994=EDGE_CURVE('',#40230,#40734,#23232,.T.);
#52995=EDGE_CURVE('',#40735,#40226,#23233,.T.);
#52996=EDGE_CURVE('',#40734,#40735,#33691,.T.);
#52997=EDGE_CURVE('',#40237,#40736,#23234,.T.);
#52998=EDGE_CURVE('',#40737,#40234,#23235,.T.);
#52999=EDGE_CURVE('',#40736,#40737,#33692,.T.);
#53000=EDGE_CURVE('',#39837,#40738,#23236,.T.);
#53001=EDGE_CURVE('',#40739,#39841,#23237,.T.);
#53002=EDGE_CURVE('',#40738,#40739,#33693,.T.);
#53003=EDGE_CURVE('',#39832,#40740,#23238,.T.);
#53004=EDGE_CURVE('',#40741,#39831,#23239,.T.);
#53005=EDGE_CURVE('',#40740,#40741,#33694,.T.);
#53006=EDGE_CURVE('',#39838,#40742,#23240,.T.);
#53007=EDGE_CURVE('',#40743,#39834,#23241,.T.);
#53008=EDGE_CURVE('',#40742,#40743,#33695,.T.);
#53009=EDGE_CURVE('',#39845,#40744,#23242,.T.);
#53010=EDGE_CURVE('',#40745,#39842,#23243,.T.);
#53011=EDGE_CURVE('',#40744,#40745,#33696,.T.);
#53012=EDGE_CURVE('',#40246,#40746,#23244,.T.);
#53013=EDGE_CURVE('',#40747,#40242,#23245,.T.);
#53014=EDGE_CURVE('',#40746,#40747,#33697,.T.);
#53015=EDGE_CURVE('',#40253,#40748,#23246,.T.);
#53016=EDGE_CURVE('',#40749,#40250,#23247,.T.);
#53017=EDGE_CURVE('',#40748,#40749,#33698,.T.);
#53018=EDGE_CURVE('',#40245,#40750,#23248,.T.);
#53019=EDGE_CURVE('',#40751,#40249,#23249,.T.);
#53020=EDGE_CURVE('',#40750,#40751,#33699,.T.);
#53021=EDGE_CURVE('',#40240,#40752,#23250,.T.);
#53022=EDGE_CURVE('',#40753,#40239,#23251,.T.);
#53023=EDGE_CURVE('',#40752,#40753,#33700,.T.);
#53024=EDGE_CURVE('',#39829,#40754,#23252,.T.);
#53025=EDGE_CURVE('',#40755,#39826,#23253,.T.);
#53026=EDGE_CURVE('',#40754,#40755,#33701,.T.);
#53027=EDGE_CURVE('',#39821,#40756,#23254,.T.);
#53028=EDGE_CURVE('',#40757,#39825,#23255,.T.);
#53029=EDGE_CURVE('',#40756,#40757,#33702,.T.);
#53030=EDGE_CURVE('',#40758,#40759,#33703,.T.);
#53031=EDGE_CURVE('',#39817,#40758,#23256,.T.);
#53032=EDGE_CURVE('',#40759,#39816,#23257,.T.);
#53033=EDGE_CURVE('',#39822,#40760,#23258,.T.);
#53034=EDGE_CURVE('',#40761,#39818,#23259,.T.);
#53035=EDGE_CURVE('',#40760,#40761,#33704,.T.);
#53036=EDGE_CURVE('',#40339,#40762,#23260,.T.);
#53037=EDGE_CURVE('',#40763,#40341,#23261,.T.);
#53038=EDGE_CURVE('',#40762,#40763,#33705,.T.);
#53039=EDGE_CURVE('',#40367,#40764,#23262,.T.);
#53040=EDGE_CURVE('',#40765,#40369,#23263,.T.);
#53041=EDGE_CURVE('',#40764,#40765,#33706,.T.);
#53042=EDGE_CURVE('',#40355,#40766,#23264,.T.);
#53043=EDGE_CURVE('',#40767,#40357,#23265,.T.);
#53044=EDGE_CURVE('',#40766,#40767,#33707,.T.);
#53045=EDGE_CURVE('',#40768,#40769,#33708,.T.);
#53046=EDGE_CURVE('',#40351,#40768,#23266,.T.);
#53047=EDGE_CURVE('',#40769,#40353,#23267,.T.);
#53048=EDGE_CURVE('',#40371,#40770,#23268,.T.);
#53049=EDGE_CURVE('',#40771,#40373,#23269,.T.);
#53050=EDGE_CURVE('',#40770,#40771,#33709,.T.);
#53051=EDGE_CURVE('',#40772,#40773,#33710,.T.);
#53052=EDGE_CURVE('',#40363,#40772,#23270,.T.);
#53053=EDGE_CURVE('',#40773,#40365,#23271,.T.);
#53054=EDGE_CURVE('',#40343,#40774,#23272,.T.);
#53055=EDGE_CURVE('',#40775,#40344,#23273,.T.);
#53056=EDGE_CURVE('',#40774,#40775,#33711,.T.);
#53057=EDGE_CURVE('',#40003,#40776,#23274,.T.);
#53058=EDGE_CURVE('',#40777,#40007,#23275,.T.);
#53059=EDGE_CURVE('',#40776,#40777,#33712,.T.);
#53060=EDGE_CURVE('',#40023,#40778,#23276,.T.);
#53061=EDGE_CURVE('',#40779,#40027,#23277,.T.);
#53062=EDGE_CURVE('',#40778,#40779,#33713,.T.);
#53063=EDGE_CURVE('',#40115,#40780,#23278,.T.);
#53064=EDGE_CURVE('',#40780,#40526,#33714,.T.);
#53065=EDGE_CURVE('',#40781,#39858,#23279,.T.);
#53066=EDGE_CURVE('',#40545,#40781,#33715,.T.);
#53067=EDGE_CURVE('',#40782,#40782,#33716,.T.);
#53068=EDGE_CURVE('',#40782,#40280,#23280,.T.);
#53069=EDGE_CURVE('',#40553,#40780,#33717,.T.);
#53070=EDGE_CURVE('',#40781,#40550,#33718,.T.);
#53071=EDGE_CURVE('',#40279,#40783,#23281,.T.);
#53072=EDGE_CURVE('',#40783,#39039,#33719,.T.);
#53073=EDGE_CURVE('',#39165,#39426,#33720,.T.);
#53074=EDGE_CURVE('',#39007,#39024,#33721,.T.);
#53075=EDGE_CURVE('',#39429,#39168,#33722,.T.);
#53076=EDGE_CURVE('',#38991,#38994,#33723,.T.);
#53077=EDGE_CURVE('',#39171,#39174,#33724,.T.);
#53078=EDGE_CURVE('',#39023,#38978,#33725,.T.);
#53079=EDGE_CURVE('',#39177,#39178,#33726,.T.);
#53080=EDGE_CURVE('',#39010,#40349,#33727,.T.);
#53081=EDGE_CURVE('',#40523,#40524,#33728,.T.);
#53082=EDGE_CURVE('',#40361,#40317,#33729,.T.);
#53083=EDGE_CURVE('',#40517,#40520,#33730,.T.);
#53084=EDGE_CURVE('',#40329,#40333,#33731,.T.);
#53085=EDGE_CURVE('',#40775,#40514,#33732,.T.);
#53086=EDGE_CURVE('',#40345,#40362,#33733,.T.);
#53087=EDGE_CURVE('',#40511,#40772,#33734,.T.);
#53088=EDGE_CURVE('',#40377,#40783,#33735,.T.);
#53089=EDGE_CURVE('',#40770,#40765,#33736,.T.);
#53090=EDGE_CURVE('',#40764,#40773,#23282,.T.);
#53091=EDGE_CURVE('',#40774,#40763,#23283,.T.);
#53092=EDGE_CURVE('',#40762,#40513,#33737,.T.);
#53093=EDGE_CURVE('',#40779,#40528,#33738,.T.);
#53094=EDGE_CURVE('',#40766,#40769,#33739,.T.);
#53095=EDGE_CURVE('',#40767,#40522,#23284,.T.);
#53096=EDGE_CURVE('',#40521,#40508,#23285,.T.);
#53097=EDGE_CURVE('',#40518,#40509,#33740,.T.);
#53098=EDGE_CURVE('',#40537,#40776,#33741,.T.);
#53099=EDGE_CURVE('',#40570,#40565,#23286,.T.);
#53100=EDGE_CURVE('',#40666,#40669,#23287,.T.);
#53101=EDGE_CURVE('',#40658,#40661,#23288,.T.);
#53102=EDGE_CURVE('',#40578,#40573,#23289,.T.);
#53103=EDGE_CURVE('',#40650,#40653,#23290,.T.);
#53104=EDGE_CURVE('',#40602,#40597,#23291,.T.);
#53105=EDGE_CURVE('',#40642,#40645,#23292,.T.);
#53106=EDGE_CURVE('',#40610,#40605,#23293,.T.);
#53107=EDGE_CURVE('',#40594,#40589,#23294,.T.);
#53108=EDGE_CURVE('',#40626,#40629,#23295,.T.);
#53109=EDGE_CURVE('',#40634,#40637,#23296,.T.);
#53110=EDGE_CURVE('',#40618,#40613,#23297,.T.);
#53111=EDGE_CURVE('',#40620,#40623,#23298,.T.);
#53112=EDGE_CURVE('',#40586,#40581,#23299,.T.);
#53113=EDGE_CURVE('',#40562,#40559,#23300,.T.);
#53114=EDGE_CURVE('',#40674,#40677,#23301,.T.);
#53115=EDGE_CURVE('',#40722,#40725,#23302,.T.);
#53116=EDGE_CURVE('',#40678,#40681,#23303,.T.);
#53117=EDGE_CURVE('',#40566,#40569,#23304,.T.);
#53118=EDGE_CURVE('',#40696,#40691,#23305,.T.);
#53119=EDGE_CURVE('',#40582,#40585,#23306,.T.);
#53120=EDGE_CURVE('',#40682,#40685,#23307,.T.);
#53121=EDGE_CURVE('',#40574,#40577,#23308,.T.);
#53122=EDGE_CURVE('',#40704,#40699,#23309,.T.);
#53123=EDGE_CURVE('',#40598,#40601,#23310,.T.);
#53124=EDGE_CURVE('',#40538,#40541,#23311,.T.);
#53125=EDGE_CURVE('',#40606,#40609,#23312,.T.);
#53126=EDGE_CURVE('',#40532,#40535,#23313,.T.);
#53127=EDGE_CURVE('',#40630,#40633,#23314,.T.);
#53128=EDGE_CURVE('',#40714,#40717,#23315,.T.);
#53129=EDGE_CURVE('',#40614,#40617,#23316,.T.);
#53130=EDGE_CURVE('',#40712,#40707,#23317,.T.);
#53131=EDGE_CURVE('',#40784,#40785,#23318,.T.);
#53132=EDGE_CURVE('',#40784,#40786,#23319,.T.);
#53133=EDGE_CURVE('',#40786,#40787,#23320,.T.);
#53134=EDGE_CURVE('',#40787,#40785,#23321,.T.);
#53135=EDGE_CURVE('',#40788,#40789,#23322,.T.);
#53136=EDGE_CURVE('',#40788,#40784,#23323,.T.);
#53137=EDGE_CURVE('',#40785,#40789,#23324,.T.);
#53138=EDGE_CURVE('',#40786,#40790,#23325,.T.);
#53139=EDGE_CURVE('',#40791,#40790,#23326,.T.);
#53140=EDGE_CURVE('',#40791,#40787,#23327,.T.);
#53141=EDGE_CURVE('',#40754,#40757,#23328,.T.);
#53142=EDGE_CURVE('',#40726,#40729,#23329,.T.);
#53143=EDGE_CURVE('',#40692,#40695,#23330,.T.);
#53144=EDGE_CURVE('',#40744,#40739,#23331,.T.);
#53145=EDGE_CURVE('',#40686,#40689,#23332,.T.);
#53146=EDGE_CURVE('',#40730,#40733,#23333,.T.);
#53147=EDGE_CURVE('',#40700,#40703,#23334,.T.);
#53148=EDGE_CURVE('',#40544,#40547,#23335,.T.);
#53149=EDGE_CURVE('',#40542,#40777,#23336,.T.);
#53150=EDGE_CURVE('',#40778,#40531,#23337,.T.);
#53151=EDGE_CURVE('',#40718,#40721,#23338,.T.);
#53152=EDGE_CURVE('',#40746,#40749,#23339,.T.);
#53153=EDGE_CURVE('',#40708,#40711,#23340,.T.);
#53154=EDGE_CURVE('',#40556,#40527,#23341,.T.);
#53155=EDGE_CURVE('',#40548,#40551,#23342,.T.);
#53156=EDGE_CURVE('',#40750,#40753,#23343,.T.);
#53157=EDGE_CURVE('',#40552,#40555,#23344,.T.);
#53158=EDGE_CURVE('',#40510,#40771,#23345,.T.);
#53159=EDGE_CURVE('',#40768,#40525,#23346,.T.);
#53160=EDGE_CURVE('',#40740,#40743,#23347,.T.);
#53161=EDGE_CURVE('',#40758,#40761,#23348,.T.);
#53162=EDGE_CURVE('',#40734,#40737,#23349,.T.);
#53163=EDGE_CURVE('',#39442,#40791,#33742,.T.);
#53164=EDGE_CURVE('',#40792,#39459,#33743,.T.);
#53165=EDGE_CURVE('',#40793,#40792,#33744,.T.);
#53166=EDGE_CURVE('',#40794,#40793,#33745,.T.);
#53167=EDGE_CURVE('',#40795,#40794,#33746,.T.);
#53168=EDGE_CURVE('',#40796,#40795,#33747,.T.);
#53169=EDGE_CURVE('',#40797,#40796,#33748,.T.);
#53170=EDGE_CURVE('',#40798,#40797,#33749,.T.);
#53171=EDGE_CURVE('',#40799,#40798,#33750,.T.);
#53172=EDGE_CURVE('',#40789,#40799,#33751,.T.);
#53173=EDGE_CURVE('',#40683,#40688,#33752,.T.);
#53174=EDGE_CURVE('',#40684,#40687,#23350,.T.);
#53175=EDGE_CURVE('',#40690,#40693,#23351,.T.);
#53176=EDGE_CURVE('',#40694,#40697,#23352,.T.);
#53177=EDGE_CURVE('',#40698,#40701,#23353,.T.);
#53178=EDGE_CURVE('',#40702,#40705,#23354,.T.);
#53179=EDGE_CURVE('',#40706,#40709,#23355,.T.);
#53180=EDGE_CURVE('',#40710,#40713,#23356,.T.);
#53181=EDGE_CURVE('',#40720,#40715,#23357,.T.);
#53182=EDGE_CURVE('',#40716,#40719,#23358,.T.);
#53183=EDGE_CURVE('',#40727,#40724,#33753,.T.);
#53184=EDGE_CURVE('',#40728,#40723,#23359,.T.);
#53185=EDGE_CURVE('',#40759,#40756,#33754,.T.);
#53186=EDGE_CURVE('',#40760,#40755,#23360,.T.);
#53187=EDGE_CURVE('',#40752,#40747,#23361,.T.);
#53188=EDGE_CURVE('',#40748,#40751,#23362,.T.);
#53189=EDGE_CURVE('',#40738,#40741,#23363,.T.);
#53190=EDGE_CURVE('',#40742,#40745,#23364,.T.);
#53191=EDGE_CURVE('',#40731,#40736,#33755,.T.);
#53192=EDGE_CURVE('',#40732,#40735,#23365,.T.);
#53193=EDGE_CURVE('',#40680,#40675,#23366,.T.);
#53194=EDGE_CURVE('',#40679,#40800,#33756,.T.);
#53195=EDGE_CURVE('',#40800,#40801,#33757,.T.);
#53196=EDGE_CURVE('',#40801,#40676,#33758,.T.);
#53197=EDGE_CURVE('',#40668,#40671,#23367,.T.);
#53198=EDGE_CURVE('',#40672,#40667,#23368,.T.);
#53199=EDGE_CURVE('',#40673,#40802,#33759,.T.);
#53200=EDGE_CURVE('',#40802,#40803,#33760,.T.);
#53201=EDGE_CURVE('',#40803,#40670,#33761,.T.);
#53202=EDGE_CURVE('',#40660,#40663,#23369,.T.);
#53203=EDGE_CURVE('',#40664,#40659,#23370,.T.);
#53204=EDGE_CURVE('',#40665,#40662,#33762,.T.);
#53205=EDGE_CURVE('',#40652,#40655,#23371,.T.);
#53206=EDGE_CURVE('',#40656,#40651,#23372,.T.);
#53207=EDGE_CURVE('',#40657,#40654,#33763,.T.);
#53208=EDGE_CURVE('',#40644,#40647,#23373,.T.);
#53209=EDGE_CURVE('',#40648,#40643,#23374,.T.);
#53210=EDGE_CURVE('',#40649,#40646,#33764,.T.);
#53211=EDGE_CURVE('',#40636,#40639,#23375,.T.);
#53212=EDGE_CURVE('',#40640,#40635,#23376,.T.);
#53213=EDGE_CURVE('',#40641,#40638,#33765,.T.);
#53214=EDGE_CURVE('',#40632,#40627,#23377,.T.);
#53215=EDGE_CURVE('',#40628,#40631,#23378,.T.);
#53216=EDGE_CURVE('',#40624,#40621,#23379,.T.);
#53217=EDGE_CURVE('',#40625,#40622,#33766,.T.);
#53218=EDGE_CURVE('',#40612,#40615,#23380,.T.);
#53219=EDGE_CURVE('',#40616,#40619,#23381,.T.);
#53220=EDGE_CURVE('',#40604,#40607,#23382,.T.);
#53221=EDGE_CURVE('',#40608,#40611,#23383,.T.);
#53222=EDGE_CURVE('',#40596,#40599,#23384,.T.);
#53223=EDGE_CURVE('',#40600,#40603,#23385,.T.);
#53224=EDGE_CURVE('',#40588,#40591,#23386,.T.);
#53225=EDGE_CURVE('',#40592,#40595,#23387,.T.);
#53226=EDGE_CURVE('',#40593,#40804,#33767,.T.);
#53227=EDGE_CURVE('',#40804,#40805,#33768,.T.);
#53228=EDGE_CURVE('',#40805,#40590,#33769,.T.);
#53229=EDGE_CURVE('',#40580,#40583,#23388,.T.);
#53230=EDGE_CURVE('',#40587,#40806,#33770,.T.);
#53231=EDGE_CURVE('',#40806,#40807,#33771,.T.);
#53232=EDGE_CURVE('',#40807,#40584,#33772,.T.);
#53233=EDGE_CURVE('',#40572,#40575,#23389,.T.);
#53234=EDGE_CURVE('',#40576,#40579,#23390,.T.);
#53235=EDGE_CURVE('',#40564,#40567,#23391,.T.);
#53236=EDGE_CURVE('',#40568,#40571,#23392,.T.);
#53237=EDGE_CURVE('',#40558,#40561,#23393,.T.);
#53238=EDGE_CURVE('',#40563,#40560,#33773,.T.);
#53239=EDGE_CURVE('',#40536,#40539,#23394,.T.);
#53240=EDGE_CURVE('',#40540,#40543,#23395,.T.);
#53241=EDGE_CURVE('',#40554,#40557,#23396,.T.);
#53242=EDGE_CURVE('',#40512,#40515,#23397,.T.);
#53243=EDGE_CURVE('',#40546,#40549,#23398,.T.);
#53244=EDGE_CURVE('',#40516,#40519,#23399,.T.);
#53245=EDGE_CURVE('',#40534,#40529,#23400,.T.);
#53246=EDGE_CURVE('',#40530,#40533,#23401,.T.);
#53247=EDGE_CURVE('',#40799,#40808,#23402,.T.);
#53248=EDGE_CURVE('',#40798,#40809,#23403,.T.);
#53249=EDGE_CURVE('',#40808,#40809,#33774,.T.);
#53250=EDGE_CURVE('',#40810,#40809,#33775,.T.);
#53251=EDGE_CURVE('',#40797,#40810,#23404,.T.);
#53252=EDGE_CURVE('',#40796,#40811,#23405,.T.);
#53253=EDGE_CURVE('',#40810,#40811,#33776,.T.);
#53254=EDGE_CURVE('',#40795,#40812,#23406,.T.);
#53255=EDGE_CURVE('',#40811,#40812,#33777,.T.);
#53256=EDGE_CURVE('',#40794,#40813,#23407,.T.);
#53257=EDGE_CURVE('',#40812,#40813,#33778,.T.);
#53258=EDGE_CURVE('',#40814,#40813,#33779,.T.);
#53259=EDGE_CURVE('',#40793,#40814,#23408,.T.);
#53260=EDGE_CURVE('',#40792,#40815,#23409,.T.);
#53261=EDGE_CURVE('',#40814,#40815,#33780,.T.);
#53262=EDGE_CURVE('',#40815,#39458,#33781,.T.);
#53263=EDGE_CURVE('',#40816,#40817,#23410,.T.);
#53264=EDGE_CURVE('',#40816,#40818,#5843,.T.);
#53265=EDGE_CURVE('',#40819,#40818,#23411,.T.);
#53266=EDGE_CURVE('',#40819,#40817,#33782,.T.);
#53267=EDGE_CURVE('',#40820,#40816,#23412,.T.);
#53268=EDGE_CURVE('',#40820,#40817,#23413,.T.);
#53269=EDGE_CURVE('',#40821,#40822,#33783,.T.);
#53270=EDGE_CURVE('',#40823,#40821,#23414,.T.);
#53271=EDGE_CURVE('',#40822,#40823,#5844,.T.);
#53272=EDGE_CURVE('',#40824,#40823,#5845,.T.);
#53273=EDGE_CURVE('',#40824,#40821,#23415,.T.);
#53274=EDGE_CURVE('',#40825,#40826,#1226,.T.);
#53275=EDGE_CURVE('',#40827,#40826,#5846,.T.);
#53276=EDGE_CURVE('',#40827,#40828,#23416,.T.);
#53277=EDGE_CURVE('',#40825,#40828,#23417,.T.);
#53278=EDGE_CURVE('',#40829,#40830,#1227,.T.);
#53279=EDGE_CURVE('',#40830,#40831,#23418,.T.);
#53280=EDGE_CURVE('',#40831,#40832,#23419,.T.);
#53281=EDGE_CURVE('',#40829,#40832,#5847,.T.);
#53282=EDGE_CURVE('',#40830,#40825,#33784,.T.);
#53283=EDGE_CURVE('',#40828,#40831,#33785,.T.);
#53284=EDGE_CURVE('',#40833,#40834,#1228,.T.);
#53285=EDGE_CURVE('',#40834,#40835,#23420,.T.);
#53286=EDGE_CURVE('',#40835,#40836,#23421,.T.);
#53287=EDGE_CURVE('',#40833,#40836,#5848,.T.);
#53288=EDGE_CURVE('',#40837,#40838,#1229,.T.);
#53289=EDGE_CURVE('',#40839,#40838,#5849,.T.);
#53290=EDGE_CURVE('',#40839,#40840,#23422,.T.);
#53291=EDGE_CURVE('',#40837,#40840,#23423,.T.);
#53292=EDGE_CURVE('',#40834,#40837,#33786,.T.);
#53293=EDGE_CURVE('',#40840,#40835,#33787,.T.);
#53294=EDGE_CURVE('',#40841,#40842,#5850,.T.);
#53295=EDGE_CURVE('',#40843,#40841,#5851,.T.);
#53296=EDGE_CURVE('',#40843,#40844,#5852,.T.);
#53297=EDGE_CURVE('',#40844,#39588,#5853,.T.);
#53298=EDGE_CURVE('',#39560,#40845,#5854,.T.);
#53299=EDGE_CURVE('',#40846,#40845,#5855,.T.);
#53300=EDGE_CURVE('',#40847,#40846,#5856,.T.);
#53301=EDGE_CURVE('',#40848,#40847,#5857,.T.);
#53302=EDGE_CURVE('',#40849,#40848,#5858,.T.);
#53303=EDGE_CURVE('',#40849,#40850,#5859,.T.);
#53304=EDGE_CURVE('',#40842,#40850,#5860,.T.);
#53305=EDGE_CURVE('',#40851,#40852,#5861,.T.);
#53306=EDGE_CURVE('',#40852,#40853,#5862,.T.);
#53307=EDGE_CURVE('',#39556,#40853,#5863,.F.);
#53308=EDGE_CURVE('',#39571,#39570,#5864,.T.);
#53309=EDGE_CURVE('',#39569,#40854,#5865,.T.);
#53310=EDGE_CURVE('',#40855,#40854,#5866,.F.);
#53311=EDGE_CURVE('',#40856,#40855,#5867,.T.);
#53312=EDGE_CURVE('',#40856,#40857,#5868,.T.);
#53313=EDGE_CURVE('',#40851,#40857,#5869,.T.);
#53314=EDGE_CURVE('',#40858,#40859,#33788,.T.);
#53315=EDGE_CURVE('',#40860,#40858,#23424,.T.);
#53316=EDGE_CURVE('',#40860,#40861,#33789,.T.);
#53317=EDGE_CURVE('',#40861,#40859,#23425,.T.);
#53318=EDGE_CURVE('',#40842,#40844,#33790,.T.);
#53319=EDGE_CURVE('',#40841,#40843,#33791,.T.);
#53320=EDGE_CURVE('',#39492,#40862,#33792,.T.);
#53321=EDGE_CURVE('',#40862,#40863,#23426,.T.);
#53322=EDGE_CURVE('',#40851,#40863,#33793,.T.);
#53323=EDGE_CURVE('',#40856,#40857,#33794,.T.);
#53324=EDGE_CURVE('',#40854,#40855,#33795,.T.);
#53325=EDGE_CURVE('',#40863,#40864,#33796,.T.);
#53326=EDGE_CURVE('',#40862,#40865,#33797,.T.);
#53327=EDGE_CURVE('',#40865,#40864,#23427,.T.);
#53328=EDGE_CURVE('',#40864,#40866,#33798,.T.);
#53329=EDGE_CURVE('',#40865,#40867,#33799,.T.);
#53330=EDGE_CURVE('',#40867,#40866,#23428,.T.);
#53331=EDGE_CURVE('',#40866,#40868,#33800,.T.);
#53332=EDGE_CURVE('',#40867,#40869,#33801,.T.);
#53333=EDGE_CURVE('',#40869,#40868,#23429,.T.);
#53334=EDGE_CURVE('',#40869,#40870,#33802,.T.);
#53335=EDGE_CURVE('',#40870,#40871,#5870,.T.);
#53336=EDGE_CURVE('',#40868,#40871,#33803,.T.);
#53337=EDGE_CURVE('',#40872,#40873,#33804,.T.);
#53338=EDGE_CURVE('',#40874,#40872,#23430,.T.);
#53339=EDGE_CURVE('',#40874,#40875,#33805,.T.);
#53340=EDGE_CURVE('',#40875,#40873,#23431,.T.);
#53341=EDGE_CURVE('',#40873,#40858,#33806,.T.);
#53342=EDGE_CURVE('',#40875,#40860,#33807,.T.);
#53343=EDGE_CURVE('',#40876,#40877,#5871,.T.);
#53344=EDGE_CURVE('',#40877,#40878,#5872,.T.);
#53345=EDGE_CURVE('',#40879,#40878,#5873,.T.);
#53346=EDGE_CURVE('',#40879,#40880,#5874,.T.);
#53347=EDGE_CURVE('',#40876,#40880,#5875,.T.);
#53348=EDGE_CURVE('',#40881,#40882,#5876,.T.);
#53349=EDGE_CURVE('',#40882,#40883,#5877,.T.);
#53350=EDGE_CURVE('',#40884,#40883,#5878,.T.);
#53351=EDGE_CURVE('',#40885,#40884,#5879,.T.);
#53352=EDGE_CURVE('',#40881,#40885,#5880,.T.);
#53353=EDGE_CURVE('',#40886,#40887,#5881,.T.);
#53354=EDGE_CURVE('',#40887,#40888,#5882,.T.);
#53355=EDGE_CURVE('',#40889,#40888,#5883,.T.);
#53356=EDGE_CURVE('',#40889,#40890,#5884,.T.);
#53357=EDGE_CURVE('',#40886,#40890,#5885,.T.);
#53358=EDGE_CURVE('',#40891,#40892,#5886,.T.);
#53359=EDGE_CURVE('',#40893,#40892,#5887,.T.);
#53360=EDGE_CURVE('',#40894,#40893,#5888,.T.);
#53361=EDGE_CURVE('',#40895,#40894,#5889,.T.);
#53362=EDGE_CURVE('',#40891,#40895,#5890,.T.);
#53363=EDGE_CURVE('',#40896,#40897,#33808,.T.);
#53364=EDGE_CURVE('',#40898,#40896,#23432,.T.);
#53365=EDGE_CURVE('',#40898,#40885,#5891,.T.);
#53366=EDGE_CURVE('',#40884,#40897,#23433,.T.);
#53367=EDGE_CURVE('',#40829,#40898,#5892,.T.);
#53368=EDGE_CURVE('',#40899,#40896,#33809,.T.);
#53369=EDGE_CURVE('',#40900,#40899,#23434,.T.);
#53370=EDGE_CURVE('',#40900,#40826,#5893,.T.);
#53371=EDGE_CURVE('',#40901,#40899,#33810,.T.);
#53372=EDGE_CURVE('',#40879,#40901,#23435,.T.);
#53373=EDGE_CURVE('',#40900,#40878,#33811,.T.);
#53374=EDGE_CURVE('',#40902,#40903,#33812,.T.);
#53375=EDGE_CURVE('',#40904,#40902,#23436,.T.);
#53376=EDGE_CURVE('',#40904,#40895,#33813,.T.);
#53377=EDGE_CURVE('',#40894,#40903,#23437,.T.);
#53378=EDGE_CURVE('',#40833,#40904,#5894,.T.);
#53379=EDGE_CURVE('',#40905,#40902,#33814,.T.);
#53380=EDGE_CURVE('',#40906,#40905,#23438,.T.);
#53381=EDGE_CURVE('',#40906,#40838,#5895,.T.);
#53382=EDGE_CURVE('',#40907,#40905,#33815,.T.);
#53383=EDGE_CURVE('',#40889,#40907,#23439,.T.);
#53384=EDGE_CURVE('',#40906,#40888,#33816,.T.);
#53385=EDGE_CURVE('',#40897,#39524,#33817,.T.);
#53386=EDGE_CURVE('',#40883,#40845,#5896,.T.);
#53387=EDGE_CURVE('',#39544,#40908,#33818,.T.);
#53388=EDGE_CURVE('',#40909,#39547,#33819,.T.);
#53389=EDGE_CURVE('',#40910,#40909,#33820,.T.);
#53390=EDGE_CURVE('',#40911,#40910,#33821,.T.);
#53391=EDGE_CURVE('',#40912,#40911,#33822,.T.);
#53392=EDGE_CURVE('',#40913,#40912,#33823,.T.);
#53393=EDGE_CURVE('',#40914,#40913,#33824,.T.);
#53394=EDGE_CURVE('',#40915,#40914,#33825,.T.);
#53395=EDGE_CURVE('',#40908,#40915,#33826,.T.);
#53396=EDGE_CURVE('',#39534,#40907,#33827,.T.);
#53397=EDGE_CURVE('',#40903,#40901,#33828,.T.);
#53398=EDGE_CURVE('',#40916,#40917,#33829,.T.);
#53399=EDGE_CURVE('',#40913,#40916,#23440,.T.);
#53400=EDGE_CURVE('',#40912,#40917,#23441,.T.);
#53401=EDGE_CURVE('',#40918,#40916,#33830,.T.);
#53402=EDGE_CURVE('',#40914,#40918,#23442,.T.);
#53403=EDGE_CURVE('',#40919,#40918,#33831,.T.);
#53404=EDGE_CURVE('',#40915,#40919,#23443,.T.);
#53405=EDGE_CURVE('',#40920,#40919,#33832,.T.);
#53406=EDGE_CURVE('',#40908,#40920,#23444,.T.);
#53407=EDGE_CURVE('',#39543,#40920,#33833,.T.);
#53408=EDGE_CURVE('',#40921,#39546,#33834,.T.);
#53409=EDGE_CURVE('',#40909,#40921,#23445,.T.);
#53410=EDGE_CURVE('',#40922,#40921,#33835,.T.);
#53411=EDGE_CURVE('',#40910,#40922,#23446,.T.);
#53412=EDGE_CURVE('',#40923,#40922,#33836,.T.);
#53413=EDGE_CURVE('',#40911,#40923,#23447,.T.);
#53414=EDGE_CURVE('',#40917,#40923,#33837,.T.);
#53415=EDGE_CURVE('',#40924,#40876,#5897,.T.);
#53416=EDGE_CURVE('',#40925,#40880,#5898,.T.);
#53417=EDGE_CURVE('',#40924,#40925,#5899,.T.);
#53418=EDGE_CURVE('',#40893,#40926,#5900,.T.);
#53419=EDGE_CURVE('',#40892,#40927,#5901,.T.);
#53420=EDGE_CURVE('',#40926,#40927,#5902,.T.);
#53421=EDGE_CURVE('',#40926,#40925,#5903,.T.);
#53422=EDGE_CURVE('',#40852,#40886,#33838,.T.);
#53423=EDGE_CURVE('',#40853,#40890,#5904,.T.);
#53424=EDGE_CURVE('',#40928,#40872,#33839,.T.);
#53425=EDGE_CURVE('',#40859,#40847,#33840,.T.);
#53426=EDGE_CURVE('',#40882,#40846,#33841,.T.);
#53427=EDGE_CURVE('',#40877,#40881,#5905,.T.);
#53428=EDGE_CURVE('',#40928,#40924,#5906,.T.);
#53429=EDGE_CURVE('',#40839,#40929,#5907,.T.);
#53430=EDGE_CURVE('',#40930,#40929,#33842,.T.);
#53431=EDGE_CURVE('',#40930,#40836,#5908,.T.);
#53432=EDGE_CURVE('',#40930,#40931,#5909,.T.);
#53433=EDGE_CURVE('',#40932,#40931,#5910,.T.);
#53434=EDGE_CURVE('',#40932,#40933,#5911,.T.);
#53435=EDGE_CURVE('',#40933,#40822,#5912,.T.);
#53436=EDGE_CURVE('',#40929,#40824,#5913,.T.);
#53437=EDGE_CURVE('',#40887,#40891,#5914,.T.);
#53438=EDGE_CURVE('',#40827,#40934,#5915,.T.);
#53439=EDGE_CURVE('',#40935,#40934,#33843,.T.);
#53440=EDGE_CURVE('',#40935,#40832,#5916,.T.);
#53441=EDGE_CURVE('',#40935,#40936,#5917,.T.);
#53442=EDGE_CURVE('',#40818,#40936,#5918,.T.);
#53443=EDGE_CURVE('',#40820,#40934,#5919,.T.);
#53444=EDGE_CURVE('',#40927,#40871,#5920,.T.);
#53445=EDGE_CURVE('',#40937,#40938,#33844,.T.);
#53446=EDGE_CURVE('',#40937,#40938,#5921,.T.);
#53447=EDGE_CURVE('',#40939,#40940,#33845,.T.);
#53448=EDGE_CURVE('',#40939,#40940,#5922,.T.);
#53449=EDGE_CURVE('',#40941,#40942,#33846,.T.);
#53450=EDGE_CURVE('',#40941,#40942,#5923,.T.);
#53451=EDGE_CURVE('',#40848,#40849,#33847,.T.);
#53452=EDGE_CURVE('',#40943,#40932,#23448,.T.);
#53453=EDGE_CURVE('',#40933,#40943,#33848,.T.);
#53454=EDGE_CURVE('',#40944,#40940,#5924,.T.);
#53455=EDGE_CURVE('',#40945,#40939,#5925,.T.);
#53456=EDGE_CURVE('',#40945,#40944,#33849,.T.);
#53457=EDGE_CURVE('',#40946,#40947,#33850,.T.);
#53458=EDGE_CURVE('',#40938,#40947,#5926,.T.);
#53459=EDGE_CURVE('',#40946,#40937,#5927,.T.);
#53460=EDGE_CURVE('',#40948,#40928,#5928,.T.);
#53461=EDGE_CURVE('',#40948,#40874,#33851,.T.);
#53462=EDGE_CURVE('',#40949,#40950,#33852,.T.);
#53463=EDGE_CURVE('',#40942,#40950,#5929,.T.);
#53464=EDGE_CURVE('',#40949,#40941,#5930,.T.);
#53465=EDGE_CURVE('',#40861,#40850,#33853,.T.);
#53466=EDGE_CURVE('',#40819,#40936,#23449,.T.);
#53467=EDGE_CURVE('',#40943,#40931,#23450,.T.);
#53468=EDGE_CURVE('',#40951,#40946,#5931,.T.);
#53469=EDGE_CURVE('',#40947,#40945,#5932,.T.);
#53470=EDGE_CURVE('',#40944,#40949,#5933,.T.);
#53471=EDGE_CURVE('',#40950,#40952,#5934,.T.);
#53472=EDGE_CURVE('',#40952,#40948,#5935,.T.);
#53473=EDGE_CURVE('',#40870,#40951,#5936,.T.);
#53474=EDGE_CURVE('',#40800,#39785,#23451,.T.);
#53475=EDGE_CURVE('',#40801,#39789,#23452,.T.);
#53476=EDGE_CURVE('',#40802,#39959,#23453,.T.);
#53477=EDGE_CURVE('',#40803,#39963,#23454,.T.);
#53478=EDGE_CURVE('',#40804,#40150,#23455,.T.);
#53479=EDGE_CURVE('',#40805,#40146,#23456,.T.);
#53480=EDGE_CURVE('',#40806,#40185,#23457,.T.);
#53481=EDGE_CURVE('',#40807,#40189,#23458,.T.);
#53482=EDGE_CURVE('',#40953,#40953,#33854,.T.);
#53483=EDGE_CURVE('',#40953,#39630,#23459,.T.);
#53484=EDGE_CURVE('',#40954,#40954,#33855,.T.);
#53485=EDGE_CURVE('',#40954,#39633,#23460,.T.);
#53486=EDGE_CURVE('',#40955,#40309,#23461,.T.);
#53487=EDGE_CURVE('',#40956,#40311,#23462,.T.);
#53488=EDGE_CURVE('',#40956,#40955,#33856,.T.);
#53489=EDGE_CURVE('',#40957,#40307,#23463,.T.);
#53490=EDGE_CURVE('',#40955,#40957,#33857,.T.);
#53491=EDGE_CURVE('',#40958,#40305,#23464,.T.);
#53492=EDGE_CURVE('',#40957,#40958,#33858,.T.);
#53493=EDGE_CURVE('',#40959,#40303,#23465,.T.);
#53494=EDGE_CURVE('',#40958,#40959,#33859,.T.);
#53495=EDGE_CURVE('',#40960,#40301,#23466,.T.);
#53496=EDGE_CURVE('',#40959,#40960,#33860,.T.);
#53497=EDGE_CURVE('',#40961,#40299,#23467,.T.);
#53498=EDGE_CURVE('',#40960,#40961,#33861,.T.);
#53499=EDGE_CURVE('',#40961,#39608,#33862,.T.);
#53500=EDGE_CURVE('',#39609,#40962,#33863,.T.);
#53501=EDGE_CURVE('',#40962,#40313,#23468,.T.);
#53502=EDGE_CURVE('',#40962,#40956,#33864,.T.);
#53503=EDGE_CURVE('',#40963,#39611,#33865,.T.);
#53504=EDGE_CURVE('',#39612,#40964,#33866,.T.);
#53505=EDGE_CURVE('',#40964,#40965,#33867,.T.);
#53506=EDGE_CURVE('',#40965,#40966,#33868,.T.);
#53507=EDGE_CURVE('',#40966,#40967,#33869,.T.);
#53508=EDGE_CURVE('',#40967,#40968,#33870,.T.);
#53509=EDGE_CURVE('',#40968,#40969,#33871,.T.);
#53510=EDGE_CURVE('',#40969,#40970,#33872,.T.);
#53511=EDGE_CURVE('',#40970,#40963,#33873,.T.);
#53512=EDGE_CURVE('',#40970,#40284,#23469,.T.);
#53513=EDGE_CURVE('',#40963,#40282,#23470,.T.);
#53514=EDGE_CURVE('',#40964,#40296,#23471,.T.);
#53515=EDGE_CURVE('',#40965,#40294,#23472,.T.);
#53516=EDGE_CURVE('',#40966,#40292,#23473,.T.);
#53517=EDGE_CURVE('',#40967,#40290,#23474,.T.);
#53518=EDGE_CURVE('',#40968,#40288,#23475,.T.);
#53519=EDGE_CURVE('',#40969,#40286,#23476,.T.);
#53520=EDGE_CURVE('',#40423,#40440,#5937,.T.);
#53521=EDGE_CURVE('',#40421,#40444,#23477,.T.);
#53522=EDGE_CURVE('',#40427,#40482,#23478,.T.);
#53523=EDGE_CURVE('',#40425,#40486,#5938,.T.);
#53524=EDGE_CURVE('',#40402,#40505,#5939,.T.);
#53525=EDGE_CURVE('',#40400,#40499,#23479,.T.);
#53526=EDGE_CURVE('',#40462,#40406,#23480,.T.);
#53527=EDGE_CURVE('',#40404,#40466,#5940,.T.);
#53528=EDGE_CURVE('',#40489,#39698,#23481,.T.);
#53529=EDGE_CURVE('',#40485,#39700,#23482,.T.);
#53530=EDGE_CURVE('',#40438,#39696,#23483,.T.);
#53531=EDGE_CURVE('',#40443,#39694,#23484,.T.);
#53532=EDGE_CURVE('',#40469,#39690,#23485,.T.);
#53533=EDGE_CURVE('',#40465,#39692,#23486,.T.);
#53534=EDGE_CURVE('',#40506,#39688,#23487,.T.);
#53535=EDGE_CURVE('',#40502,#39685,#23488,.T.);
#53536=EDGE_CURVE('',#39622,#40971,#33874,.T.);
#53537=EDGE_CURVE('',#40972,#39623,#33875,.T.);
#53538=EDGE_CURVE('',#40973,#40972,#33876,.T.);
#53539=EDGE_CURVE('',#40974,#40973,#33877,.T.);
#53540=EDGE_CURVE('',#40975,#40974,#33878,.T.);
#53541=EDGE_CURVE('',#40976,#40975,#33879,.T.);
#53542=EDGE_CURVE('',#40977,#40976,#33880,.T.);
#53543=EDGE_CURVE('',#40978,#40977,#33881,.T.);
#53544=EDGE_CURVE('',#40971,#40978,#33882,.T.);
#53545=EDGE_CURVE('',#40386,#40975,#23489,.T.);
#53546=EDGE_CURVE('',#40384,#40976,#23490,.T.);
#53547=EDGE_CURVE('',#40382,#40977,#23491,.T.);
#53548=EDGE_CURVE('',#40380,#40978,#23492,.T.);
#53549=EDGE_CURVE('',#40379,#40971,#23493,.T.);
#53550=EDGE_CURVE('',#40392,#40972,#23494,.T.);
#53551=EDGE_CURVE('',#40390,#40973,#23495,.T.);
#53552=EDGE_CURVE('',#40388,#40974,#23496,.T.);
#53553=EDGE_CURVE('',#40790,#39443,#33883,.T.);
#53554=EDGE_CURVE('',#40808,#40788,#33884,.T.);
#53555=EDGE_CURVE('',#40979,#40980,#23497,.T.);
#53556=EDGE_CURVE('',#40981,#40979,#1230,.T.);
#53557=EDGE_CURVE('',#40981,#40982,#23498,.T.);
#53558=EDGE_CURVE('',#40980,#40982,#1231,.T.);
#53559=EDGE_CURVE('',#40983,#40984,#23499,.T.);
#53560=EDGE_CURVE('',#40979,#40983,#1232,.T.);
#53561=EDGE_CURVE('',#40984,#40980,#1233,.T.);
#53562=EDGE_CURVE('',#40985,#40986,#23500,.T.);
#53563=EDGE_CURVE('',#40983,#40985,#1234,.T.);
#53564=EDGE_CURVE('',#40986,#40984,#1235,.T.);
#53565=EDGE_CURVE('',#40987,#40988,#23501,.T.);
#53566=EDGE_CURVE('',#40985,#40987,#1236,.T.);
#53567=EDGE_CURVE('',#40988,#40986,#1237,.T.);
#53568=EDGE_CURVE('',#40989,#40990,#23502,.T.);
#53569=EDGE_CURVE('',#40987,#40989,#1238,.T.);
#53570=EDGE_CURVE('',#40990,#40988,#1239,.T.);
#53571=EDGE_CURVE('',#40989,#40981,#1240,.T.);
#53572=EDGE_CURVE('',#40982,#40990,#1241,.T.);
#53573=EDGE_CURVE('',#40991,#40985,#23503,.T.);
#53574=EDGE_CURVE('',#40980,#40982,#33885,.T.);
#53575=EDGE_CURVE('',#40984,#40980,#33886,.T.);
#53576=EDGE_CURVE('',#40986,#40984,#33887,.T.);
#53577=EDGE_CURVE('',#40988,#40986,#33888,.T.);
#53578=EDGE_CURVE('',#40990,#40988,#33889,.T.);
#53579=EDGE_CURVE('',#40982,#40990,#33890,.T.);
#53580=EDGE_CURVE('',#40992,#40992,#33891,.T.);
#53581=EDGE_CURVE('',#40992,#40993,#33892,.T.);
#53582=EDGE_CURVE('',#40993,#40994,#33893,.T.);
#53583=EDGE_CURVE('',#40994,#40993,#33894,.T.);
#53584=EDGE_CURVE('',#40995,#40995,#33895,.T.);
#53585=EDGE_CURVE('',#40995,#40994,#23504,.T.);
#53586=EDGE_CURVE('',#40996,#40997,#33896,.T.);
#53587=EDGE_CURVE('',#40997,#40998,#33897,.T.);
#53588=EDGE_CURVE('',#40998,#40999,#33898,.T.);
#53589=EDGE_CURVE('',#40999,#41000,#33899,.T.);
#53590=EDGE_CURVE('',#41000,#41001,#33900,.T.);
#53591=EDGE_CURVE('',#41001,#40996,#33901,.T.);
#53592=EDGE_CURVE('',#41002,#40998,#1242,.T.);
#53593=EDGE_CURVE('',#40997,#41002,#1243,.T.);
#53594=EDGE_CURVE('',#40998,#41003,#1244,.T.);
#53595=EDGE_CURVE('',#41003,#40999,#1245,.T.);
#53596=EDGE_CURVE('',#40999,#41004,#1246,.T.);
#53597=EDGE_CURVE('',#41004,#41000,#1247,.T.);
#53598=EDGE_CURVE('',#41000,#41005,#1248,.T.);
#53599=EDGE_CURVE('',#41005,#41001,#1249,.T.);
#53600=EDGE_CURVE('',#41001,#41006,#1250,.T.);
#53601=EDGE_CURVE('',#41006,#40996,#1251,.T.);
#53602=EDGE_CURVE('',#40996,#41007,#1252,.T.);
#53603=EDGE_CURVE('',#41007,#40997,#1253,.T.);
#53604=EDGE_CURVE('',#41008,#41009,#33902,.T.);
#53605=EDGE_CURVE('',#41008,#41010,#33903,.T.);
#53606=EDGE_CURVE('',#41010,#41011,#33904,.T.);
#53607=EDGE_CURVE('',#41011,#41012,#33905,.T.);
#53608=EDGE_CURVE('',#41012,#41013,#33906,.T.);
#53609=EDGE_CURVE('',#41013,#41009,#33907,.T.);
#53610=EDGE_CURVE('',#41014,#41008,#1254,.T.);
#53611=EDGE_CURVE('',#41010,#41014,#1255,.T.);
#53612=EDGE_CURVE('',#41015,#41010,#1256,.T.);
#53613=EDGE_CURVE('',#41011,#41015,#1257,.T.);
#53614=EDGE_CURVE('',#41016,#41011,#1258,.T.);
#53615=EDGE_CURVE('',#41012,#41016,#1259,.T.);
#53616=EDGE_CURVE('',#41017,#41012,#1260,.T.);
#53617=EDGE_CURVE('',#41013,#41017,#1261,.T.);
#53618=EDGE_CURVE('',#41018,#41013,#1262,.T.);
#53619=EDGE_CURVE('',#41009,#41018,#1263,.T.);
#53620=EDGE_CURVE('',#41008,#41019,#1264,.T.);
#53621=EDGE_CURVE('',#41019,#41009,#1265,.T.);
#53622=EDGE_CURVE('',#41007,#41014,#23505,.T.);
#53623=EDGE_CURVE('',#41002,#41019,#23506,.T.);
#53624=EDGE_CURVE('',#41006,#41015,#23507,.T.);
#53625=EDGE_CURVE('',#41005,#41016,#23508,.T.);
#53626=EDGE_CURVE('',#41004,#41017,#23509,.T.);
#53627=EDGE_CURVE('',#41003,#41018,#23510,.T.);
#53628=EDGE_CURVE('',#41020,#41021,#33908,.T.);
#53629=EDGE_CURVE('',#41021,#41022,#33909,.T.);
#53630=EDGE_CURVE('',#41022,#41023,#33910,.T.);
#53631=EDGE_CURVE('',#41023,#41024,#33911,.T.);
#53632=EDGE_CURVE('',#41024,#41025,#33912,.T.);
#53633=EDGE_CURVE('',#41025,#41020,#33913,.T.);
#53634=EDGE_CURVE('',#41026,#41022,#1266,.T.);
#53635=EDGE_CURVE('',#41021,#41026,#1267,.T.);
#53636=EDGE_CURVE('',#41022,#41027,#1268,.T.);
#53637=EDGE_CURVE('',#41027,#41023,#1269,.T.);
#53638=EDGE_CURVE('',#41023,#41028,#1270,.T.);
#53639=EDGE_CURVE('',#41028,#41024,#1271,.T.);
#53640=EDGE_CURVE('',#41024,#41029,#1272,.T.);
#53641=EDGE_CURVE('',#41029,#41025,#1273,.T.);
#53642=EDGE_CURVE('',#41025,#41030,#1274,.T.);
#53643=EDGE_CURVE('',#41030,#41020,#1275,.T.);
#53644=EDGE_CURVE('',#41020,#41031,#1276,.T.);
#53645=EDGE_CURVE('',#41031,#41021,#1277,.T.);
#53646=EDGE_CURVE('',#41032,#41033,#33914,.T.);
#53647=EDGE_CURVE('',#41032,#41034,#33915,.T.);
#53648=EDGE_CURVE('',#41034,#41035,#33916,.T.);
#53649=EDGE_CURVE('',#41035,#41036,#33917,.T.);
#53650=EDGE_CURVE('',#41036,#41037,#33918,.T.);
#53651=EDGE_CURVE('',#41037,#41033,#33919,.T.);
#53652=EDGE_CURVE('',#41038,#41032,#1278,.T.);
#53653=EDGE_CURVE('',#41034,#41038,#1279,.T.);
#53654=EDGE_CURVE('',#41039,#41034,#1280,.T.);
#53655=EDGE_CURVE('',#41035,#41039,#1281,.T.);
#53656=EDGE_CURVE('',#41040,#41035,#1282,.T.);
#53657=EDGE_CURVE('',#41036,#41040,#1283,.T.);
#53658=EDGE_CURVE('',#41041,#41036,#1284,.T.);
#53659=EDGE_CURVE('',#41037,#41041,#1285,.T.);
#53660=EDGE_CURVE('',#41042,#41037,#1286,.T.);
#53661=EDGE_CURVE('',#41033,#41042,#1287,.T.);
#53662=EDGE_CURVE('',#41032,#41043,#1288,.T.);
#53663=EDGE_CURVE('',#41043,#41033,#1289,.T.);
#53664=EDGE_CURVE('',#41031,#41038,#23511,.T.);
#53665=EDGE_CURVE('',#41026,#41043,#23512,.T.);
#53666=EDGE_CURVE('',#41030,#41039,#23513,.T.);
#53667=EDGE_CURVE('',#41029,#41040,#23514,.T.);
#53668=EDGE_CURVE('',#41028,#41041,#23515,.T.);
#53669=EDGE_CURVE('',#41027,#41042,#23516,.T.);
#53670=EDGE_CURVE('',#41044,#41045,#23517,.T.);
#53671=EDGE_CURVE('',#41045,#41046,#1290,.T.);
#53672=EDGE_CURVE('',#41047,#41046,#23518,.T.);
#53673=EDGE_CURVE('',#41047,#41044,#1291,.T.);
#53674=EDGE_CURVE('',#41048,#41049,#23519,.T.);
#53675=EDGE_CURVE('',#41049,#41045,#1292,.T.);
#53676=EDGE_CURVE('',#41044,#41048,#1293,.T.);
#53677=EDGE_CURVE('',#41050,#41051,#23520,.T.);
#53678=EDGE_CURVE('',#41051,#41049,#1294,.T.);
#53679=EDGE_CURVE('',#41048,#41050,#1295,.T.);
#53680=EDGE_CURVE('',#41052,#41053,#23521,.T.);
#53681=EDGE_CURVE('',#41053,#41051,#1296,.T.);
#53682=EDGE_CURVE('',#41050,#41052,#1297,.T.);
#53683=EDGE_CURVE('',#41054,#41055,#23522,.T.);
#53684=EDGE_CURVE('',#41055,#41053,#1298,.T.);
#53685=EDGE_CURVE('',#41052,#41054,#1299,.T.);
#53686=EDGE_CURVE('',#41046,#41055,#1300,.T.);
#53687=EDGE_CURVE('',#41054,#41047,#1301,.T.);
#53688=EDGE_CURVE('',#41056,#41050,#23523,.T.);
#53689=EDGE_CURVE('',#41045,#41046,#33920,.T.);
#53690=EDGE_CURVE('',#41049,#41045,#33921,.T.);
#53691=EDGE_CURVE('',#41051,#41049,#33922,.T.);
#53692=EDGE_CURVE('',#41053,#41051,#33923,.T.);
#53693=EDGE_CURVE('',#41055,#41053,#33924,.T.);
#53694=EDGE_CURVE('',#41046,#41055,#33925,.T.);
#53695=EDGE_CURVE('',#41057,#41057,#33926,.T.);
#53696=EDGE_CURVE('',#41057,#41058,#33927,.T.);
#53697=EDGE_CURVE('',#41059,#41058,#33928,.T.);
#53698=EDGE_CURVE('',#41058,#41059,#33929,.T.);
#53699=EDGE_CURVE('',#41060,#41060,#33930,.T.);
#53700=EDGE_CURVE('',#41060,#41059,#23524,.T.);
#53701=EDGE_CURVE('',#41061,#41061,#33931,.T.);
#53702=EDGE_CURVE('',#41062,#41063,#33932,.T.);
#53703=EDGE_CURVE('',#41064,#41062,#5941,.F.);
#53704=EDGE_CURVE('',#41065,#41064,#33933,.T.);
#53705=EDGE_CURVE('',#41063,#41065,#5942,.F.);
#53706=EDGE_CURVE('',#41066,#41067,#33934,.T.);
#53707=EDGE_CURVE('',#41067,#41066,#33935,.T.);
#53708=EDGE_CURVE('',#41067,#41061,#33936,.T.);
#53709=EDGE_CURVE('',#41068,#41068,#33937,.T.);
#53710=EDGE_CURVE('',#41068,#41069,#33938,.T.);
#53711=EDGE_CURVE('',#41070,#41069,#33939,.T.);
#53712=EDGE_CURVE('',#41069,#41070,#33940,.T.);
#53713=EDGE_CURVE('',#41071,#41072,#33941,.T.);
#53714=EDGE_CURVE('',#41073,#41071,#23525,.T.);
#53715=EDGE_CURVE('',#41074,#41073,#33942,.T.);
#53716=EDGE_CURVE('',#41072,#41074,#23526,.T.);
#53717=EDGE_CURVE('',#41063,#41072,#23527,.T.);
#53718=EDGE_CURVE('',#41062,#41074,#23528,.T.);
#53719=EDGE_CURVE('',#41064,#41073,#23529,.T.);
#53720=EDGE_CURVE('',#41065,#41071,#23530,.T.);
#53721=EDGE_CURVE('',#41075,#41075,#33943,.T.);
#53722=EDGE_CURVE('',#41076,#41076,#33944,.T.);
#53723=EDGE_CURVE('',#41076,#41075,#23531,.T.);
#53724=EDGE_CURVE('',#41066,#41070,#23532,.T.);
#53725=EDGE_CURVE('',#41077,#41077,#33945,.T.);
#53726=EDGE_CURVE('',#41077,#41078,#23533,.T.);
#53727=EDGE_CURVE('',#41078,#41078,#33946,.T.);
#53728=EDGE_CURVE('',#41079,#41079,#33947,.T.);
#53729=EDGE_CURVE('',#41079,#41077,#23534,.T.);
#53730=EDGE_CURVE('',#41080,#41080,#33948,.T.);
#53731=EDGE_CURVE('',#41081,#41081,#33949,.T.);
#53732=EDGE_CURVE('',#41081,#41080,#23535,.T.);
#53733=EDGE_CURVE('',#41082,#41083,#33950,.T.);
#53734=EDGE_CURVE('',#41084,#41083,#33951,.T.);
#53735=EDGE_CURVE('',#41084,#41085,#33952,.T.);
#53736=EDGE_CURVE('',#41082,#41085,#33953,.T.);
#53737=EDGE_CURVE('',#41086,#41087,#33954,.T.);
#53738=EDGE_CURVE('',#41085,#41087,#23536,.T.);
#53739=EDGE_CURVE('',#41086,#41084,#23537,.T.);
#53740=EDGE_CURVE('',#41088,#41089,#33955,.T.);
#53741=EDGE_CURVE('',#41083,#41089,#23538,.T.);
#53742=EDGE_CURVE('',#41088,#41082,#23539,.T.);
#53743=EDGE_CURVE('',#41090,#41091,#33956,.T.);
#53744=EDGE_CURVE('',#41087,#41091,#33957,.T.);
#53745=EDGE_CURVE('',#41090,#41086,#33958,.T.);
#53746=EDGE_CURVE('',#41092,#41093,#33959,.T.);
#53747=EDGE_CURVE('',#41089,#41093,#33960,.T.);
#53748=EDGE_CURVE('',#41092,#41088,#33961,.T.);
#53749=EDGE_CURVE('',#41094,#41095,#33962,.T.);
#53750=EDGE_CURVE('',#41091,#41095,#23540,.T.);
#53751=EDGE_CURVE('',#41094,#41090,#23541,.T.);
#53752=EDGE_CURVE('',#41096,#41097,#33963,.T.);
#53753=EDGE_CURVE('',#41093,#41097,#23542,.T.);
#53754=EDGE_CURVE('',#41096,#41092,#23543,.T.);
#53755=EDGE_CURVE('',#41097,#41094,#33964,.T.);
#53756=EDGE_CURVE('',#41095,#41096,#33965,.T.);
#53757=EDGE_CURVE('',#41098,#41096,#23544,.T.);
#53758=EDGE_CURVE('',#41099,#41092,#23545,.T.);
#53759=EDGE_CURVE('',#41098,#41099,#23546,.T.);
#53760=EDGE_CURVE('',#41100,#41095,#23547,.T.);
#53761=EDGE_CURVE('',#41100,#41098,#33966,.T.);
#53762=EDGE_CURVE('',#41101,#41088,#23548,.T.);
#53763=EDGE_CURVE('',#41099,#41101,#33967,.T.);
#53764=EDGE_CURVE('',#41102,#41103,#23549,.T.);
#53765=EDGE_CURVE('',#41104,#41102,#23550,.T.);
#53766=EDGE_CURVE('',#41105,#41104,#23551,.T.);
#53767=EDGE_CURVE('',#41103,#41105,#23552,.T.);
#53768=EDGE_CURVE('',#41106,#41106,#33968,.T.);
#53769=EDGE_CURVE('',#41107,#41107,#33969,.T.);
#53770=EDGE_CURVE('',#41102,#41108,#33970,.T.);
#53771=EDGE_CURVE('',#41102,#41109,#33971,.T.);
#53772=EDGE_CURVE('',#41109,#41110,#33972,.T.);
#53773=EDGE_CURVE('',#41110,#41108,#33973,.T.);
#53774=EDGE_CURVE('',#41104,#41111,#33974,.T.);
#53775=EDGE_CURVE('',#41108,#41111,#23553,.T.);
#53776=EDGE_CURVE('',#41112,#41113,#33975,.T.);
#53777=EDGE_CURVE('',#41112,#41104,#33976,.T.);
#53778=EDGE_CURVE('',#41111,#41113,#33977,.T.);
#53779=EDGE_CURVE('',#41112,#41114,#23554,.T.);
#53780=EDGE_CURVE('',#41105,#41114,#33978,.T.);
#53781=EDGE_CURVE('',#41115,#41114,#33979,.T.);
#53782=EDGE_CURVE('',#41115,#41116,#33980,.T.);
#53783=EDGE_CURVE('',#41116,#41105,#33981,.T.);
#53784=EDGE_CURVE('',#41117,#41103,#33982,.T.);
#53785=EDGE_CURVE('',#41117,#41118,#33983,.T.);
#53786=EDGE_CURVE('',#41118,#41119,#33984,.T.);
#53787=EDGE_CURVE('',#41119,#41103,#33985,.T.);
#53788=EDGE_CURVE('',#41116,#41117,#23555,.T.);
#53789=EDGE_CURVE('',#41119,#41109,#23556,.T.);
#53790=EDGE_CURVE('',#41120,#41121,#23557,.T.);
#53791=EDGE_CURVE('',#41120,#41122,#33986,.T.);
#53792=EDGE_CURVE('',#41123,#41122,#23558,.T.);
#53793=EDGE_CURVE('',#41123,#41121,#33987,.T.);
#53794=EDGE_CURVE('',#41124,#41125,#33988,.T.);
#53795=EDGE_CURVE('',#41122,#41125,#23559,.T.);
#53796=EDGE_CURVE('',#41126,#41122,#33989,.T.);
#53797=EDGE_CURVE('',#41124,#41126,#23560,.T.);
#53798=EDGE_CURVE('',#41127,#41120,#33990,.T.);
#53799=EDGE_CURVE('',#41126,#41127,#33991,.T.);
#53800=EDGE_CURVE('',#41128,#41129,#33992,.T.);
#53801=EDGE_CURVE('',#41125,#41129,#33993,.T.);
#53802=EDGE_CURVE('',#41128,#41124,#33994,.T.);
#53803=EDGE_CURVE('',#41125,#41130,#23561,.T.);
#53804=EDGE_CURVE('',#41131,#41129,#23562,.T.);
#53805=EDGE_CURVE('',#41131,#41130,#33995,.T.);
#53806=EDGE_CURVE('',#41131,#41132,#33996,.T.);
#53807=EDGE_CURVE('',#41133,#41132,#33997,.T.);
#53808=EDGE_CURVE('',#41130,#41133,#33998,.T.);
#53809=EDGE_CURVE('',#41134,#41133,#23563,.T.);
#53810=EDGE_CURVE('',#41123,#41134,#33999,.T.);
#53811=EDGE_CURVE('',#41130,#41123,#23564,.T.);
#53812=EDGE_CURVE('',#41135,#41134,#34000,.T.);
#53813=EDGE_CURVE('',#41121,#41135,#34001,.T.);
#53814=EDGE_CURVE('',#41136,#41136,#34002,.T.);
#53815=EDGE_CURVE('',#41137,#41137,#34003,.T.);
#53816=EDGE_CURVE('',#41138,#41082,#23565,.T.);
#53817=EDGE_CURVE('',#41139,#41085,#23566,.T.);
#53818=EDGE_CURVE('',#41139,#41138,#34004,.T.);
#53819=EDGE_CURVE('',#41140,#41087,#23567,.T.);
#53820=EDGE_CURVE('',#41141,#41091,#23568,.T.);
#53821=EDGE_CURVE('',#41141,#41140,#34005,.T.);
#53822=EDGE_CURVE('',#41110,#41135,#23569,.T.);
#53823=EDGE_CURVE('',#41121,#41109,#23570,.T.);
#53824=EDGE_CURVE('',#41119,#41120,#23571,.T.);
#53825=EDGE_CURVE('',#41127,#41118,#23572,.T.);
#53826=EDGE_CURVE('',#41115,#41128,#23573,.T.);
#53827=EDGE_CURVE('',#41129,#41114,#23574,.T.);
#53828=EDGE_CURVE('',#41112,#41131,#23575,.T.);
#53829=EDGE_CURVE('',#41132,#41113,#23576,.T.);
#53830=EDGE_CURVE('',#41100,#41141,#23577,.T.);
#53831=EDGE_CURVE('',#41138,#41101,#23578,.T.);
#53832=EDGE_CURVE('',#41136,#41106,#23579,.T.);
#53833=EDGE_CURVE('',#41137,#41107,#23580,.T.);
#53834=EDGE_CURVE('',#41140,#41139,#23581,.T.);
#53835=EDGE_CURVE('',#41142,#41142,#34006,.T.);
#53836=EDGE_CURVE('',#41143,#41144,#34007,.T.);
#53837=EDGE_CURVE('',#41145,#41143,#5943,.F.);
#53838=EDGE_CURVE('',#41146,#41145,#34008,.T.);
#53839=EDGE_CURVE('',#41144,#41146,#5944,.F.);
#53840=EDGE_CURVE('',#41147,#41148,#34009,.T.);
#53841=EDGE_CURVE('',#41148,#41147,#34010,.T.);
#53842=EDGE_CURVE('',#41148,#41142,#34011,.T.);
#53843=EDGE_CURVE('',#41149,#41149,#34012,.T.);
#53844=EDGE_CURVE('',#41149,#41150,#34013,.T.);
#53845=EDGE_CURVE('',#41151,#41150,#34014,.T.);
#53846=EDGE_CURVE('',#41150,#41151,#34015,.T.);
#53847=EDGE_CURVE('',#41152,#41153,#34016,.T.);
#53848=EDGE_CURVE('',#41154,#41152,#23582,.T.);
#53849=EDGE_CURVE('',#41155,#41154,#34017,.T.);
#53850=EDGE_CURVE('',#41153,#41155,#23583,.T.);
#53851=EDGE_CURVE('',#41144,#41153,#23584,.T.);
#53852=EDGE_CURVE('',#41143,#41155,#23585,.T.);
#53853=EDGE_CURVE('',#41145,#41154,#23586,.T.);
#53854=EDGE_CURVE('',#41146,#41152,#23587,.T.);
#53855=EDGE_CURVE('',#41156,#41156,#34018,.T.);
#53856=EDGE_CURVE('',#41157,#41157,#34019,.T.);
#53857=EDGE_CURVE('',#41157,#41156,#23588,.T.);
#53858=EDGE_CURVE('',#41147,#41151,#23589,.T.);
#53859=EDGE_CURVE('',#41158,#41159,#34020,.T.);
#53860=EDGE_CURVE('',#41160,#41159,#23590,.T.);
#53861=EDGE_CURVE('',#41161,#41160,#5945,.T.);
#53862=EDGE_CURVE('',#41158,#41161,#23591,.T.);
#53863=EDGE_CURVE('',#41162,#41163,#34021,.T.);
#53864=EDGE_CURVE('',#41159,#41163,#34022,.T.);
#53865=EDGE_CURVE('',#41162,#41158,#34023,.T.);
#53866=EDGE_CURVE('',#41164,#41165,#34024,.T.);
#53867=EDGE_CURVE('',#41163,#41165,#23592,.T.);
#53868=EDGE_CURVE('',#41164,#41162,#23593,.T.);
#53869=EDGE_CURVE('',#41166,#41167,#34025,.T.);
#53870=EDGE_CURVE('',#41165,#41167,#34026,.T.);
#53871=EDGE_CURVE('',#41166,#41164,#34027,.T.);
#53872=EDGE_CURVE('',#41168,#41169,#5946,.T.);
#53873=EDGE_CURVE('',#41167,#41168,#23594,.T.);
#53874=EDGE_CURVE('',#41169,#41166,#23595,.T.);
#53875=EDGE_CURVE('',#41170,#41171,#34028,.T.);
#53876=EDGE_CURVE('',#41172,#41171,#23596,.T.);
#53877=EDGE_CURVE('',#41173,#41172,#34029,.T.);
#53878=EDGE_CURVE('',#41170,#41173,#23597,.T.);
#53879=EDGE_CURVE('',#41174,#41175,#34030,.T.);
#53880=EDGE_CURVE('',#41171,#41175,#34031,.T.);
#53881=EDGE_CURVE('',#41174,#41170,#34032,.T.);
#53882=EDGE_CURVE('',#41176,#41177,#34033,.T.);
#53883=EDGE_CURVE('',#41175,#41177,#23598,.T.);
#53884=EDGE_CURVE('',#41176,#41174,#23599,.T.);
#53885=EDGE_CURVE('',#41178,#41179,#34034,.T.);
#53886=EDGE_CURVE('',#41177,#41179,#34035,.T.);
#53887=EDGE_CURVE('',#41178,#41176,#34036,.T.);
#53888=EDGE_CURVE('',#41180,#41181,#5947,.T.);
#53889=EDGE_CURVE('',#41179,#41180,#23600,.T.);
#53890=EDGE_CURVE('',#41181,#41178,#23601,.T.);
#53891=EDGE_CURVE('',#41182,#41183,#34037,.T.);
#53892=EDGE_CURVE('',#41184,#41183,#23602,.T.);
#53893=EDGE_CURVE('',#41185,#41184,#34038,.T.);
#53894=EDGE_CURVE('',#41182,#41185,#23603,.T.);
#53895=EDGE_CURVE('',#41186,#41187,#34039,.T.);
#53896=EDGE_CURVE('',#41183,#41187,#34040,.T.);
#53897=EDGE_CURVE('',#41186,#41182,#34041,.T.);
#53898=EDGE_CURVE('',#41188,#41189,#34042,.T.);
#53899=EDGE_CURVE('',#41187,#41189,#23604,.T.);
#53900=EDGE_CURVE('',#41188,#41186,#23605,.T.);
#53901=EDGE_CURVE('',#41190,#41191,#34043,.T.);
#53902=EDGE_CURVE('',#41189,#41191,#34044,.T.);
#53903=EDGE_CURVE('',#41190,#41188,#34045,.T.);
#53904=EDGE_CURVE('',#41192,#41193,#34046,.T.);
#53905=EDGE_CURVE('',#41191,#41193,#23606,.T.);
#53906=EDGE_CURVE('',#41192,#41190,#23607,.T.);
#53907=EDGE_CURVE('',#41194,#41195,#34047,.T.);
#53908=EDGE_CURVE('',#41193,#41195,#34048,.T.);
#53909=EDGE_CURVE('',#41194,#41192,#34049,.T.);
#53910=EDGE_CURVE('',#41196,#41197,#34050,.T.);
#53911=EDGE_CURVE('',#41195,#41197,#23608,.T.);
#53912=EDGE_CURVE('',#41196,#41194,#23609,.T.);
#53913=EDGE_CURVE('',#41198,#41199,#34051,.T.);
#53914=EDGE_CURVE('',#41197,#41199,#34052,.T.);
#53915=EDGE_CURVE('',#41198,#41196,#34053,.T.);
#53916=EDGE_CURVE('',#41200,#41201,#34054,.T.);
#53917=EDGE_CURVE('',#41199,#41200,#23610,.T.);
#53918=EDGE_CURVE('',#41201,#41198,#23611,.T.);
#53919=EDGE_CURVE('',#41202,#41203,#34055,.T.);
#53920=EDGE_CURVE('',#41204,#41202,#23612,.T.);
#53921=EDGE_CURVE('',#41204,#41205,#34056,.T.);
#53922=EDGE_CURVE('',#41203,#41205,#23613,.T.);
#53923=EDGE_CURVE('',#41206,#41207,#34057,.T.);
#53924=EDGE_CURVE('',#41205,#41207,#34058,.T.);
#53925=EDGE_CURVE('',#41206,#41204,#34059,.T.);
#53926=EDGE_CURVE('',#41208,#41209,#34060,.T.);
#53927=EDGE_CURVE('',#41207,#41209,#23614,.T.);
#53928=EDGE_CURVE('',#41208,#41206,#23615,.T.);
#53929=EDGE_CURVE('',#41210,#41211,#34061,.T.);
#53930=EDGE_CURVE('',#41209,#41211,#34062,.T.);
#53931=EDGE_CURVE('',#41210,#41208,#34063,.T.);
#53932=EDGE_CURVE('',#41212,#41213,#5948,.T.);
#53933=EDGE_CURVE('',#41211,#41212,#23616,.T.);
#53934=EDGE_CURVE('',#41213,#41210,#23617,.T.);
#53935=EDGE_CURVE('',#41214,#41215,#34064,.T.);
#53936=EDGE_CURVE('',#41216,#41215,#23618,.T.);
#53937=EDGE_CURVE('',#41217,#41216,#34065,.T.);
#53938=EDGE_CURVE('',#41214,#41217,#23619,.T.);
#53939=EDGE_CURVE('',#41218,#41219,#34066,.T.);
#53940=EDGE_CURVE('',#41215,#41219,#34067,.T.);
#53941=EDGE_CURVE('',#41218,#41214,#34068,.T.);
#53942=EDGE_CURVE('',#41220,#41221,#34069,.T.);
#53943=EDGE_CURVE('',#41219,#41221,#23620,.T.);
#53944=EDGE_CURVE('',#41220,#41218,#23621,.T.);
#53945=EDGE_CURVE('',#41222,#41223,#34070,.T.);
#53946=EDGE_CURVE('',#41221,#41223,#34071,.T.);
#53947=EDGE_CURVE('',#41222,#41220,#34072,.T.);
#53948=EDGE_CURVE('',#41224,#41225,#34073,.T.);
#53949=EDGE_CURVE('',#41223,#41225,#34074,.T.);
#53950=EDGE_CURVE('',#41224,#41222,#34075,.T.);
#53951=EDGE_CURVE('',#41226,#41227,#34076,.T.);
#53952=EDGE_CURVE('',#41225,#41227,#23622,.T.);
#53953=EDGE_CURVE('',#41226,#41224,#23623,.T.);
#53954=EDGE_CURVE('',#41228,#41229,#34077,.T.);
#53955=EDGE_CURVE('',#41227,#41229,#34078,.T.);
#53956=EDGE_CURVE('',#41228,#41226,#34079,.T.);
#53957=EDGE_CURVE('',#41230,#41231,#34080,.T.);
#53958=EDGE_CURVE('',#41229,#41231,#23624,.T.);
#53959=EDGE_CURVE('',#41230,#41228,#23625,.T.);
#53960=EDGE_CURVE('',#41232,#41233,#34081,.T.);
#53961=EDGE_CURVE('',#41231,#41233,#34082,.T.);
#53962=EDGE_CURVE('',#41232,#41230,#34083,.T.);
#53963=EDGE_CURVE('',#41234,#41235,#34084,.T.);
#53964=EDGE_CURVE('',#41233,#41234,#23626,.T.);
#53965=EDGE_CURVE('',#41235,#41232,#23627,.T.);
#53966=EDGE_CURVE('',#41236,#41237,#34085,.T.);
#53967=EDGE_CURVE('',#41238,#41237,#23628,.T.);
#53968=EDGE_CURVE('',#41239,#41238,#34086,.T.);
#53969=EDGE_CURVE('',#41236,#41239,#23629,.T.);
#53970=EDGE_CURVE('',#41240,#41241,#34087,.T.);
#53971=EDGE_CURVE('',#41237,#41241,#34088,.T.);
#53972=EDGE_CURVE('',#41240,#41236,#34089,.T.);
#53973=EDGE_CURVE('',#41242,#41243,#34090,.T.);
#53974=EDGE_CURVE('',#41241,#41243,#23630,.T.);
#53975=EDGE_CURVE('',#41242,#41240,#23631,.T.);
#53976=EDGE_CURVE('',#41244,#41245,#34091,.T.);
#53977=EDGE_CURVE('',#41243,#41245,#34092,.T.);
#53978=EDGE_CURVE('',#41244,#41242,#34093,.T.);
#53979=EDGE_CURVE('',#41246,#41247,#34094,.T.);
#53980=EDGE_CURVE('',#41245,#41247,#34095,.T.);
#53981=EDGE_CURVE('',#41246,#41244,#34096,.T.);
#53982=EDGE_CURVE('',#41248,#41249,#34097,.T.);
#53983=EDGE_CURVE('',#41247,#41249,#34098,.T.);
#53984=EDGE_CURVE('',#41248,#41246,#34099,.T.);
#53985=EDGE_CURVE('',#41250,#41251,#34100,.T.);
#53986=EDGE_CURVE('',#41249,#41251,#23632,.T.);
#53987=EDGE_CURVE('',#41250,#41248,#23633,.T.);
#53988=EDGE_CURVE('',#41252,#41253,#34101,.T.);
#53989=EDGE_CURVE('',#41251,#41253,#34102,.T.);
#53990=EDGE_CURVE('',#41252,#41250,#34103,.T.);
#53991=EDGE_CURVE('',#41254,#41255,#34104,.T.);
#53992=EDGE_CURVE('',#41253,#41254,#23634,.T.);
#53993=EDGE_CURVE('',#41255,#41252,#23635,.T.);
#53994=EDGE_CURVE('',#41256,#41257,#34105,.T.);
#53995=EDGE_CURVE('',#41258,#41257,#23636,.T.);
#53996=EDGE_CURVE('',#41259,#41258,#34106,.T.);
#53997=EDGE_CURVE('',#41256,#41259,#23637,.T.);
#53998=EDGE_CURVE('',#41260,#41261,#34107,.T.);
#53999=EDGE_CURVE('',#41257,#41261,#34108,.T.);
#54000=EDGE_CURVE('',#41260,#41256,#34109,.T.);
#54001=EDGE_CURVE('',#41262,#41263,#34110,.T.);
#54002=EDGE_CURVE('',#41261,#41263,#23638,.T.);
#54003=EDGE_CURVE('',#41262,#41260,#23639,.T.);
#54004=EDGE_CURVE('',#41264,#41265,#34111,.T.);
#54005=EDGE_CURVE('',#41263,#41265,#34112,.T.);
#54006=EDGE_CURVE('',#41264,#41262,#34113,.T.);
#54007=EDGE_CURVE('',#41266,#41267,#34114,.T.);
#54008=EDGE_CURVE('',#41265,#41267,#34115,.T.);
#54009=EDGE_CURVE('',#41266,#41264,#34116,.T.);
#54010=EDGE_CURVE('',#41268,#41269,#34117,.T.);
#54011=EDGE_CURVE('',#41267,#41269,#34118,.T.);
#54012=EDGE_CURVE('',#41268,#41266,#34119,.T.);
#54013=EDGE_CURVE('',#41270,#41271,#34120,.T.);
#54014=EDGE_CURVE('',#41269,#41271,#23640,.T.);
#54015=EDGE_CURVE('',#41270,#41268,#23641,.T.);
#54016=EDGE_CURVE('',#41272,#41273,#34121,.T.);
#54017=EDGE_CURVE('',#41271,#41273,#34122,.T.);
#54018=EDGE_CURVE('',#41272,#41270,#34123,.T.);
#54019=EDGE_CURVE('',#41274,#41275,#34124,.T.);
#54020=EDGE_CURVE('',#41273,#41274,#23642,.T.);
#54021=EDGE_CURVE('',#41275,#41272,#23643,.T.);
#54022=EDGE_CURVE('',#41276,#41277,#34125,.T.);
#54023=EDGE_CURVE('',#41278,#41277,#23644,.T.);
#54024=EDGE_CURVE('',#41279,#41278,#34126,.T.);
#54025=EDGE_CURVE('',#41276,#41279,#23645,.T.);
#54026=EDGE_CURVE('',#41280,#41281,#34127,.T.);
#54027=EDGE_CURVE('',#41277,#41281,#34128,.T.);
#54028=EDGE_CURVE('',#41280,#41276,#34129,.T.);
#54029=EDGE_CURVE('',#41282,#41283,#34130,.T.);
#54030=EDGE_CURVE('',#41281,#41283,#23646,.T.);
#54031=EDGE_CURVE('',#41282,#41280,#23647,.T.);
#54032=EDGE_CURVE('',#41284,#41285,#34131,.T.);
#54033=EDGE_CURVE('',#41283,#41285,#34132,.T.);
#54034=EDGE_CURVE('',#41284,#41282,#34133,.T.);
#54035=EDGE_CURVE('',#41286,#41287,#34134,.T.);
#54036=EDGE_CURVE('',#41285,#41287,#34135,.T.);
#54037=EDGE_CURVE('',#41286,#41284,#34136,.T.);
#54038=EDGE_CURVE('',#41288,#41289,#34137,.T.);
#54039=EDGE_CURVE('',#41287,#41289,#34138,.T.);
#54040=EDGE_CURVE('',#41288,#41286,#34139,.T.);
#54041=EDGE_CURVE('',#41290,#41291,#34140,.T.);
#54042=EDGE_CURVE('',#41289,#41291,#23648,.T.);
#54043=EDGE_CURVE('',#41290,#41288,#23649,.T.);
#54044=EDGE_CURVE('',#41292,#41293,#34141,.T.);
#54045=EDGE_CURVE('',#41291,#41293,#34142,.T.);
#54046=EDGE_CURVE('',#41292,#41290,#34143,.T.);
#54047=EDGE_CURVE('',#41294,#41295,#34144,.T.);
#54048=EDGE_CURVE('',#41293,#41294,#23650,.T.);
#54049=EDGE_CURVE('',#41295,#41292,#23651,.T.);
#54050=EDGE_CURVE('',#41296,#41297,#34145,.T.);
#54051=EDGE_CURVE('',#41298,#41297,#23652,.T.);
#54052=EDGE_CURVE('',#41299,#41298,#34146,.T.);
#54053=EDGE_CURVE('',#41296,#41299,#23653,.T.);
#54054=EDGE_CURVE('',#41300,#41301,#34147,.T.);
#54055=EDGE_CURVE('',#41297,#41301,#34148,.T.);
#54056=EDGE_CURVE('',#41300,#41296,#34149,.T.);
#54057=EDGE_CURVE('',#41302,#41303,#34150,.T.);
#54058=EDGE_CURVE('',#41301,#41303,#23654,.T.);
#54059=EDGE_CURVE('',#41302,#41300,#23655,.T.);
#54060=EDGE_CURVE('',#41304,#41305,#34151,.T.);
#54061=EDGE_CURVE('',#41303,#41305,#34152,.T.);
#54062=EDGE_CURVE('',#41304,#41302,#34153,.T.);
#54063=EDGE_CURVE('',#41306,#41307,#34154,.T.);
#54064=EDGE_CURVE('',#41305,#41307,#34155,.T.);
#54065=EDGE_CURVE('',#41306,#41304,#34156,.T.);
#54066=EDGE_CURVE('',#41308,#41309,#34157,.T.);
#54067=EDGE_CURVE('',#41307,#41309,#34158,.T.);
#54068=EDGE_CURVE('',#41308,#41306,#34159,.T.);
#54069=EDGE_CURVE('',#41310,#41311,#34160,.T.);
#54070=EDGE_CURVE('',#41309,#41311,#23656,.T.);
#54071=EDGE_CURVE('',#41310,#41308,#23657,.T.);
#54072=EDGE_CURVE('',#41312,#41313,#34161,.T.);
#54073=EDGE_CURVE('',#41311,#41313,#34162,.T.);
#54074=EDGE_CURVE('',#41312,#41310,#34163,.T.);
#54075=EDGE_CURVE('',#41314,#41315,#34164,.T.);
#54076=EDGE_CURVE('',#41313,#41314,#23658,.T.);
#54077=EDGE_CURVE('',#41315,#41312,#23659,.T.);
#54078=EDGE_CURVE('',#41316,#41317,#34165,.T.);
#54079=EDGE_CURVE('',#41318,#41317,#23660,.T.);
#54080=EDGE_CURVE('',#41319,#41318,#34166,.T.);
#54081=EDGE_CURVE('',#41316,#41319,#23661,.T.);
#54082=EDGE_CURVE('',#41320,#41321,#34167,.T.);
#54083=EDGE_CURVE('',#41317,#41321,#34168,.T.);
#54084=EDGE_CURVE('',#41320,#41316,#34169,.T.);
#54085=EDGE_CURVE('',#41322,#41323,#34170,.T.);
#54086=EDGE_CURVE('',#41321,#41323,#23662,.T.);
#54087=EDGE_CURVE('',#41322,#41320,#23663,.T.);
#54088=EDGE_CURVE('',#41324,#41325,#34171,.T.);
#54089=EDGE_CURVE('',#41323,#41325,#34172,.T.);
#54090=EDGE_CURVE('',#41324,#41322,#34173,.T.);
#54091=EDGE_CURVE('',#41326,#41327,#34174,.T.);
#54092=EDGE_CURVE('',#41325,#41327,#34175,.T.);
#54093=EDGE_CURVE('',#41326,#41324,#34176,.T.);
#54094=EDGE_CURVE('',#41328,#41329,#34177,.T.);
#54095=EDGE_CURVE('',#41327,#41329,#34178,.T.);
#54096=EDGE_CURVE('',#41328,#41326,#34179,.T.);
#54097=EDGE_CURVE('',#41330,#41331,#34180,.T.);
#54098=EDGE_CURVE('',#41329,#41331,#23664,.T.);
#54099=EDGE_CURVE('',#41330,#41328,#23665,.T.);
#54100=EDGE_CURVE('',#41332,#41333,#34181,.T.);
#54101=EDGE_CURVE('',#41331,#41333,#34182,.T.);
#54102=EDGE_CURVE('',#41332,#41330,#34183,.T.);
#54103=EDGE_CURVE('',#41334,#41335,#34184,.T.);
#54104=EDGE_CURVE('',#41333,#41334,#23666,.T.);
#54105=EDGE_CURVE('',#41335,#41332,#23667,.T.);
#54106=EDGE_CURVE('',#41336,#41337,#34185,.T.);
#54107=EDGE_CURVE('',#41338,#41337,#23668,.T.);
#54108=EDGE_CURVE('',#41339,#41338,#34186,.T.);
#54109=EDGE_CURVE('',#41336,#41339,#23669,.T.);
#54110=EDGE_CURVE('',#41340,#41341,#34187,.T.);
#54111=EDGE_CURVE('',#41337,#41341,#34188,.T.);
#54112=EDGE_CURVE('',#41340,#41336,#34189,.T.);
#54113=EDGE_CURVE('',#41342,#41343,#34190,.T.);
#54114=EDGE_CURVE('',#41341,#41343,#23670,.T.);
#54115=EDGE_CURVE('',#41342,#41340,#23671,.T.);
#54116=EDGE_CURVE('',#41344,#41345,#34191,.T.);
#54117=EDGE_CURVE('',#41343,#41345,#34192,.T.);
#54118=EDGE_CURVE('',#41344,#41342,#34193,.T.);
#54119=EDGE_CURVE('',#41346,#41347,#34194,.T.);
#54120=EDGE_CURVE('',#41345,#41347,#34195,.T.);
#54121=EDGE_CURVE('',#41346,#41344,#34196,.T.);
#54122=EDGE_CURVE('',#41348,#41349,#34197,.T.);
#54123=EDGE_CURVE('',#41347,#41349,#34198,.T.);
#54124=EDGE_CURVE('',#41348,#41346,#34199,.T.);
#54125=EDGE_CURVE('',#41350,#41351,#34200,.T.);
#54126=EDGE_CURVE('',#41349,#41351,#23672,.T.);
#54127=EDGE_CURVE('',#41350,#41348,#23673,.T.);
#54128=EDGE_CURVE('',#41352,#41353,#34201,.T.);
#54129=EDGE_CURVE('',#41351,#41353,#34202,.T.);
#54130=EDGE_CURVE('',#41352,#41350,#34203,.T.);
#54131=EDGE_CURVE('',#41354,#41355,#34204,.T.);
#54132=EDGE_CURVE('',#41353,#41354,#23674,.T.);
#54133=EDGE_CURVE('',#41355,#41352,#23675,.T.);
#54134=EDGE_CURVE('',#41356,#41357,#34205,.T.);
#54135=EDGE_CURVE('',#41358,#41357,#23676,.T.);
#54136=EDGE_CURVE('',#41359,#41358,#34206,.T.);
#54137=EDGE_CURVE('',#41356,#41359,#23677,.T.);
#54138=EDGE_CURVE('',#41360,#41361,#34207,.T.);
#54139=EDGE_CURVE('',#41357,#41361,#34208,.T.);
#54140=EDGE_CURVE('',#41360,#41356,#34209,.T.);
#54141=EDGE_CURVE('',#41362,#41363,#34210,.T.);
#54142=EDGE_CURVE('',#41361,#41363,#23678,.T.);
#54143=EDGE_CURVE('',#41362,#41360,#23679,.T.);
#54144=EDGE_CURVE('',#41364,#41365,#34211,.T.);
#54145=EDGE_CURVE('',#41363,#41365,#34212,.T.);
#54146=EDGE_CURVE('',#41364,#41362,#34213,.T.);
#54147=EDGE_CURVE('',#41366,#41367,#34214,.T.);
#54148=EDGE_CURVE('',#41365,#41367,#23680,.T.);
#54149=EDGE_CURVE('',#41366,#41364,#23681,.T.);
#54150=EDGE_CURVE('',#41368,#41369,#34215,.T.);
#54151=EDGE_CURVE('',#41367,#41369,#34216,.T.);
#54152=EDGE_CURVE('',#41368,#41366,#34217,.T.);
#54153=EDGE_CURVE('',#41370,#41371,#34218,.T.);
#54154=EDGE_CURVE('',#41369,#41371,#34219,.T.);
#54155=EDGE_CURVE('',#41370,#41368,#34220,.T.);
#54156=EDGE_CURVE('',#41372,#41373,#34221,.T.);
#54157=EDGE_CURVE('',#41371,#41373,#23682,.T.);
#54158=EDGE_CURVE('',#41372,#41370,#23683,.T.);
#54159=EDGE_CURVE('',#41374,#41375,#34222,.T.);
#54160=EDGE_CURVE('',#41373,#41375,#34223,.T.);
#54161=EDGE_CURVE('',#41374,#41372,#34224,.T.);
#54162=EDGE_CURVE('',#41376,#41377,#34225,.T.);
#54163=EDGE_CURVE('',#41375,#41376,#23684,.T.);
#54164=EDGE_CURVE('',#41377,#41374,#23685,.T.);
#54165=EDGE_CURVE('',#41378,#41379,#34226,.T.);
#54166=EDGE_CURVE('',#41380,#41379,#23686,.T.);
#54167=EDGE_CURVE('',#41381,#41380,#34227,.T.);
#54168=EDGE_CURVE('',#41378,#41381,#23687,.T.);
#54169=EDGE_CURVE('',#41382,#41383,#34228,.T.);
#54170=EDGE_CURVE('',#41379,#41383,#34229,.T.);
#54171=EDGE_CURVE('',#41382,#41378,#34230,.T.);
#54172=EDGE_CURVE('',#41384,#41385,#34231,.T.);
#54173=EDGE_CURVE('',#41383,#41385,#23688,.T.);
#54174=EDGE_CURVE('',#41384,#41382,#23689,.T.);
#54175=EDGE_CURVE('',#41386,#41387,#34232,.T.);
#54176=EDGE_CURVE('',#41385,#41387,#34233,.T.);
#54177=EDGE_CURVE('',#41386,#41384,#34234,.T.);
#54178=EDGE_CURVE('',#41388,#41389,#34235,.T.);
#54179=EDGE_CURVE('',#41387,#41389,#23690,.T.);
#54180=EDGE_CURVE('',#41388,#41386,#23691,.T.);
#54181=EDGE_CURVE('',#41390,#41391,#34236,.T.);
#54182=EDGE_CURVE('',#41389,#41391,#34237,.T.);
#54183=EDGE_CURVE('',#41390,#41388,#34238,.T.);
#54184=EDGE_CURVE('',#41392,#41393,#34239,.T.);
#54185=EDGE_CURVE('',#41391,#41393,#23692,.T.);
#54186=EDGE_CURVE('',#41392,#41390,#23693,.T.);
#54187=EDGE_CURVE('',#41394,#41395,#34240,.T.);
#54188=EDGE_CURVE('',#41393,#41395,#34241,.T.);
#54189=EDGE_CURVE('',#41394,#41392,#34242,.T.);
#54190=EDGE_CURVE('',#41396,#41397,#34243,.T.);
#54191=EDGE_CURVE('',#41395,#41396,#23694,.T.);
#54192=EDGE_CURVE('',#41397,#41394,#23695,.T.);
#54193=EDGE_CURVE('',#41398,#41399,#5949,.T.);
#54194=EDGE_CURVE('',#41400,#41398,#23696,.T.);
#54195=EDGE_CURVE('',#41400,#41401,#34244,.T.);
#54196=EDGE_CURVE('',#41399,#41401,#23697,.T.);
#54197=EDGE_CURVE('',#41402,#41403,#34245,.T.);
#54198=EDGE_CURVE('',#41401,#41403,#34246,.T.);
#54199=EDGE_CURVE('',#41402,#41400,#34247,.T.);
#54200=EDGE_CURVE('',#41404,#41405,#34248,.T.);
#54201=EDGE_CURVE('',#41403,#41405,#23698,.T.);
#54202=EDGE_CURVE('',#41404,#41402,#23699,.T.);
#54203=EDGE_CURVE('',#41406,#41407,#34249,.T.);
#54204=EDGE_CURVE('',#41405,#41407,#34250,.T.);
#54205=EDGE_CURVE('',#41406,#41404,#34251,.T.);
#54206=EDGE_CURVE('',#41408,#41409,#34252,.T.);
#54207=EDGE_CURVE('',#41407,#41408,#23700,.T.);
#54208=EDGE_CURVE('',#41409,#41406,#23701,.T.);
#54209=EDGE_CURVE('',#41209,#41410,#23702,.T.);
#54210=EDGE_CURVE('',#41411,#41211,#23703,.T.);
#54211=EDGE_CURVE('',#41410,#41411,#34253,.T.);
#54212=EDGE_CURVE('',#41178,#41412,#23704,.T.);
#54213=EDGE_CURVE('',#41413,#41176,#23705,.T.);
#54214=EDGE_CURVE('',#41412,#41413,#34254,.T.);
#54215=EDGE_CURVE('',#41401,#41414,#23706,.T.);
#54216=EDGE_CURVE('',#41415,#41403,#23707,.T.);
#54217=EDGE_CURVE('',#41414,#41415,#34255,.T.);
#54218=EDGE_CURVE('',#41162,#41416,#23708,.T.);
#54219=EDGE_CURVE('',#41417,#41158,#23709,.T.);
#54220=EDGE_CURVE('',#41416,#41417,#34256,.T.);
#54221=EDGE_CURVE('',#41166,#41418,#23710,.T.);
#54222=EDGE_CURVE('',#41419,#41164,#23711,.T.);
#54223=EDGE_CURVE('',#41418,#41419,#34257,.T.);
#54224=EDGE_CURVE('',#41385,#41420,#23712,.T.);
#54225=EDGE_CURVE('',#41421,#41387,#23713,.T.);
#54226=EDGE_CURVE('',#41420,#41421,#34258,.T.);
#54227=EDGE_CURVE('',#41363,#41422,#23714,.T.);
#54228=EDGE_CURVE('',#41423,#41365,#23715,.T.);
#54229=EDGE_CURVE('',#41422,#41423,#34259,.T.);
#54230=EDGE_CURVE('',#41343,#41424,#23716,.T.);
#54231=EDGE_CURVE('',#41425,#41345,#23717,.T.);
#54232=EDGE_CURVE('',#41424,#41425,#34260,.T.);
#54233=EDGE_CURVE('',#41323,#41426,#23718,.T.);
#54234=EDGE_CURVE('',#41427,#41325,#23719,.T.);
#54235=EDGE_CURVE('',#41426,#41427,#34261,.T.);
#54236=EDGE_CURVE('',#41303,#41428,#23720,.T.);
#54237=EDGE_CURVE('',#41429,#41305,#23721,.T.);
#54238=EDGE_CURVE('',#41428,#41429,#34262,.T.);
#54239=EDGE_CURVE('',#41283,#41430,#23722,.T.);
#54240=EDGE_CURVE('',#41431,#41285,#23723,.T.);
#54241=EDGE_CURVE('',#41430,#41431,#34263,.T.);
#54242=EDGE_CURVE('',#41307,#41432,#23724,.T.);
#54243=EDGE_CURVE('',#41433,#41309,#23725,.T.);
#54244=EDGE_CURVE('',#41432,#41433,#34264,.T.);
#54245=EDGE_CURVE('',#41327,#41434,#23726,.T.);
#54246=EDGE_CURVE('',#41435,#41329,#23727,.T.);
#54247=EDGE_CURVE('',#41434,#41435,#34265,.T.);
#54248=EDGE_CURVE('',#41347,#41436,#23728,.T.);
#54249=EDGE_CURVE('',#41437,#41349,#23729,.T.);
#54250=EDGE_CURVE('',#41436,#41437,#34266,.T.);
#54251=EDGE_CURVE('',#41369,#41438,#23730,.T.);
#54252=EDGE_CURVE('',#41439,#41371,#23731,.T.);
#54253=EDGE_CURVE('',#41438,#41439,#34267,.T.);
#54254=EDGE_CURVE('',#41389,#41440,#23732,.T.);
#54255=EDGE_CURVE('',#41441,#41391,#23733,.T.);
#54256=EDGE_CURVE('',#41440,#41441,#34268,.T.);
#54257=EDGE_CURVE('',#41287,#41442,#23734,.T.);
#54258=EDGE_CURVE('',#41443,#41289,#23735,.T.);
#54259=EDGE_CURVE('',#41442,#41443,#34269,.T.);
#54260=EDGE_CURVE('',#41263,#41444,#23736,.T.);
#54261=EDGE_CURVE('',#41445,#41265,#23737,.T.);
#54262=EDGE_CURVE('',#41444,#41445,#34270,.T.);
#54263=EDGE_CURVE('',#41267,#41446,#23738,.T.);
#54264=EDGE_CURVE('',#41447,#41269,#23739,.T.);
#54265=EDGE_CURVE('',#41446,#41447,#34271,.T.);
#54266=EDGE_CURVE('',#41243,#41448,#23740,.T.);
#54267=EDGE_CURVE('',#41449,#41245,#23741,.T.);
#54268=EDGE_CURVE('',#41448,#41449,#34272,.T.);
#54269=EDGE_CURVE('',#41221,#41450,#23742,.T.);
#54270=EDGE_CURVE('',#41451,#41223,#23743,.T.);
#54271=EDGE_CURVE('',#41450,#41451,#34273,.T.);
#54272=EDGE_CURVE('',#41247,#41452,#23744,.T.);
#54273=EDGE_CURVE('',#41453,#41249,#23745,.T.);
#54274=EDGE_CURVE('',#41452,#41453,#34274,.T.);
#54275=EDGE_CURVE('',#41227,#41454,#23746,.T.);
#54276=EDGE_CURVE('',#41455,#41229,#23747,.T.);
#54277=EDGE_CURVE('',#41454,#41455,#34275,.T.);
#54278=EDGE_CURVE('',#41189,#41456,#23748,.T.);
#54279=EDGE_CURVE('',#41457,#41191,#23749,.T.);
#54280=EDGE_CURVE('',#41456,#41457,#34276,.T.);
#54281=EDGE_CURVE('',#41193,#41458,#23750,.T.);
#54282=EDGE_CURVE('',#41459,#41195,#23751,.T.);
#54283=EDGE_CURVE('',#41458,#41459,#34277,.T.);
#54284=EDGE_CURVE('',#41174,#41460,#23752,.T.);
#54285=EDGE_CURVE('',#41461,#41170,#23753,.T.);
#54286=EDGE_CURVE('',#41460,#41461,#34278,.T.);
#54287=EDGE_CURVE('',#41160,#41398,#34279,.T.);
#54288=EDGE_CURVE('',#41462,#41168,#34280,.T.);
#54289=EDGE_CURVE('',#41463,#41462,#23754,.T.);
#54290=EDGE_CURVE('',#41172,#41463,#23755,.T.);
#54291=EDGE_CURVE('',#41213,#41180,#34281,.T.);
#54292=EDGE_CURVE('',#41206,#41196,#23756,.T.);
#54293=EDGE_CURVE('',#41186,#41230,#23757,.T.);
#54294=EDGE_CURVE('',#41218,#41250,#23758,.T.);
#54295=EDGE_CURVE('',#41240,#41270,#23759,.T.);
#54296=EDGE_CURVE('',#41260,#41290,#23760,.T.);
#54297=EDGE_CURVE('',#41280,#41310,#23761,.T.);
#54298=EDGE_CURVE('',#41300,#41330,#23762,.T.);
#54299=EDGE_CURVE('',#41320,#41350,#23763,.T.);
#54300=EDGE_CURVE('',#41340,#41372,#23764,.T.);
#54301=EDGE_CURVE('',#41360,#41392,#23765,.T.);
#54302=EDGE_CURVE('',#41382,#41404,#23766,.T.);
#54303=EDGE_CURVE('',#41203,#41410,#23767,.T.);
#54304=EDGE_CURVE('',#41464,#41169,#23768,.T.);
#54305=EDGE_CURVE('',#41465,#41464,#34282,.T.);
#54306=EDGE_CURVE('',#41465,#41462,#23769,.T.);
#54307=EDGE_CURVE('',#41464,#41418,#23770,.T.);
#54308=EDGE_CURVE('',#41413,#41460,#23771,.T.);
#54309=EDGE_CURVE('',#41466,#41173,#23772,.T.);
#54310=EDGE_CURVE('',#41461,#41466,#23773,.T.);
#54311=EDGE_CURVE('',#41459,#41200,#23774,.T.);
#54312=EDGE_CURVE('',#41184,#41456,#23775,.T.);
#54313=EDGE_CURVE('',#41435,#41334,#23776,.T.);
#54314=EDGE_CURVE('',#41318,#41426,#23777,.T.);
#54315=EDGE_CURVE('',#41437,#41354,#23778,.T.);
#54316=EDGE_CURVE('',#41338,#41424,#23779,.T.);
#54317=EDGE_CURVE('',#41358,#41422,#23780,.T.);
#54318=EDGE_CURVE('',#41455,#41234,#23781,.T.);
#54319=EDGE_CURVE('',#41433,#41314,#23782,.T.);
#54320=EDGE_CURVE('',#41298,#41428,#23783,.T.);
#54321=EDGE_CURVE('',#41335,#41299,#23784,.T.);
#54322=EDGE_CURVE('',#41332,#41296,#23785,.T.);
#54323=EDGE_CURVE('',#41429,#41432,#34283,.T.);
#54324=EDGE_CURVE('',#41443,#41294,#23786,.T.);
#54325=EDGE_CURVE('',#41278,#41430,#23787,.T.);
#54326=EDGE_CURVE('',#41315,#41279,#23788,.T.);
#54327=EDGE_CURVE('',#41312,#41276,#23789,.T.);
#54328=EDGE_CURVE('',#41431,#41442,#34284,.T.);
#54329=EDGE_CURVE('',#41447,#41274,#23790,.T.);
#54330=EDGE_CURVE('',#41258,#41444,#23791,.T.);
#54331=EDGE_CURVE('',#41295,#41259,#23792,.T.);
#54332=EDGE_CURVE('',#41292,#41256,#23793,.T.);
#54333=EDGE_CURVE('',#41445,#41446,#34285,.T.);
#54334=EDGE_CURVE('',#41453,#41254,#23794,.T.);
#54335=EDGE_CURVE('',#41238,#41448,#23795,.T.);
#54336=EDGE_CURVE('',#41275,#41239,#23796,.T.);
#54337=EDGE_CURVE('',#41272,#41236,#23797,.T.);
#54338=EDGE_CURVE('',#41449,#41452,#34286,.T.);
#54339=EDGE_CURVE('',#41441,#41396,#23798,.T.);
#54340=EDGE_CURVE('',#41380,#41420,#23799,.T.);
#54341=EDGE_CURVE('',#41409,#41381,#23800,.T.);
#54342=EDGE_CURVE('',#41406,#41378,#23801,.T.);
#54343=EDGE_CURVE('',#41421,#41440,#23802,.T.);
#54344=EDGE_CURVE('',#41467,#41225,#23803,.T.);
#54345=EDGE_CURVE('',#41451,#41467,#34287,.T.);
#54346=EDGE_CURVE('',#41467,#41454,#23804,.T.);
#54347=EDGE_CURVE('',#41367,#41468,#23805,.T.);
#54348=EDGE_CURVE('',#41468,#41438,#34288,.T.);
#54349=EDGE_CURVE('',#41439,#41376,#23806,.T.);
#54350=EDGE_CURVE('',#41415,#41408,#23807,.T.);
#54351=EDGE_CURVE('',#41397,#41359,#23808,.T.);
#54352=EDGE_CURVE('',#41423,#41468,#23809,.T.);
#54353=EDGE_CURVE('',#41377,#41339,#23810,.T.);
#54354=EDGE_CURVE('',#41425,#41436,#34289,.T.);
#54355=EDGE_CURVE('',#41355,#41319,#23811,.T.);
#54356=EDGE_CURVE('',#41427,#41434,#34290,.T.);
#54357=EDGE_CURVE('',#41255,#41217,#23812,.T.);
#54358=EDGE_CURVE('',#41216,#41450,#23813,.T.);
#54359=EDGE_CURVE('',#41235,#41185,#23814,.T.);
#54360=EDGE_CURVE('',#41457,#41458,#23815,.T.);
#54361=EDGE_CURVE('',#41201,#41202,#23816,.T.);
#54362=EDGE_CURVE('',#41411,#41469,#23817,.T.);
#54363=EDGE_CURVE('',#41469,#41470,#34291,.T.);
#54364=EDGE_CURVE('',#41470,#41412,#23818,.T.);
#54365=EDGE_CURVE('',#41466,#41471,#23819,.T.);
#54366=EDGE_CURVE('',#41471,#41465,#23820,.T.);
#54367=EDGE_CURVE('',#41419,#41416,#23821,.T.);
#54368=EDGE_CURVE('',#41417,#41472,#23822,.T.);
#54369=EDGE_CURVE('',#41472,#41473,#34292,.T.);
#54370=EDGE_CURVE('',#41473,#41414,#23823,.T.);
#54371=EDGE_CURVE('',#41394,#41356,#23824,.T.);
#54372=EDGE_CURVE('',#41252,#41214,#23825,.T.);
#54373=EDGE_CURVE('',#41232,#41182,#23826,.T.);
#54374=EDGE_CURVE('',#41374,#41336,#23827,.T.);
#54375=EDGE_CURVE('',#41352,#41316,#23828,.T.);
#54376=EDGE_CURVE('',#41198,#41204,#23829,.T.);
#54377=EDGE_CURVE('',#41470,#41181,#23830,.T.);
#54378=EDGE_CURVE('',#41471,#41463,#23831,.T.);
#54379=EDGE_CURVE('',#41472,#41161,#23832,.T.);
#54380=EDGE_CURVE('',#41473,#41399,#23833,.T.);
#54381=EDGE_CURVE('',#41469,#41212,#23834,.T.);
#54382=EDGE_CURVE('',#41474,#41475,#34293,.T.);
#54383=EDGE_CURVE('',#41475,#41476,#34294,.T.);
#54384=EDGE_CURVE('',#41476,#41477,#34295,.T.);
#54385=EDGE_CURVE('',#41477,#41478,#34296,.T.);
#54386=EDGE_CURVE('',#41478,#41479,#34297,.T.);
#54387=EDGE_CURVE('',#41479,#41474,#34298,.T.);
#54388=EDGE_CURVE('',#41480,#41476,#1302,.T.);
#54389=EDGE_CURVE('',#41475,#41480,#1303,.T.);
#54390=EDGE_CURVE('',#41476,#41481,#1304,.T.);
#54391=EDGE_CURVE('',#41481,#41477,#1305,.T.);
#54392=EDGE_CURVE('',#41477,#41482,#1306,.T.);
#54393=EDGE_CURVE('',#41482,#41478,#1307,.T.);
#54394=EDGE_CURVE('',#41478,#41483,#1308,.T.);
#54395=EDGE_CURVE('',#41483,#41479,#1309,.T.);
#54396=EDGE_CURVE('',#41479,#41484,#1310,.T.);
#54397=EDGE_CURVE('',#41484,#41474,#1311,.T.);
#54398=EDGE_CURVE('',#41474,#41485,#1312,.T.);
#54399=EDGE_CURVE('',#41485,#41475,#1313,.T.);
#54400=EDGE_CURVE('',#41486,#41487,#34299,.T.);
#54401=EDGE_CURVE('',#41486,#41488,#34300,.T.);
#54402=EDGE_CURVE('',#41488,#41489,#34301,.T.);
#54403=EDGE_CURVE('',#41489,#41490,#34302,.T.);
#54404=EDGE_CURVE('',#41490,#41491,#34303,.T.);
#54405=EDGE_CURVE('',#41491,#41487,#34304,.T.);
#54406=EDGE_CURVE('',#41492,#41486,#1314,.T.);
#54407=EDGE_CURVE('',#41488,#41492,#1315,.T.);
#54408=EDGE_CURVE('',#41493,#41488,#1316,.T.);
#54409=EDGE_CURVE('',#41489,#41493,#1317,.T.);
#54410=EDGE_CURVE('',#41494,#41489,#1318,.T.);
#54411=EDGE_CURVE('',#41490,#41494,#1319,.T.);
#54412=EDGE_CURVE('',#41495,#41490,#1320,.T.);
#54413=EDGE_CURVE('',#41491,#41495,#1321,.T.);
#54414=EDGE_CURVE('',#41496,#41491,#1322,.T.);
#54415=EDGE_CURVE('',#41487,#41496,#1323,.T.);
#54416=EDGE_CURVE('',#41486,#41497,#1324,.T.);
#54417=EDGE_CURVE('',#41497,#41487,#1325,.T.);
#54418=EDGE_CURVE('',#41485,#41492,#23835,.T.);
#54419=EDGE_CURVE('',#41480,#41497,#23836,.T.);
#54420=EDGE_CURVE('',#41484,#41493,#23837,.T.);
#54421=EDGE_CURVE('',#41483,#41494,#23838,.T.);
#54422=EDGE_CURVE('',#41482,#41495,#23839,.T.);
#54423=EDGE_CURVE('',#41481,#41496,#23840,.T.);
#54424=EDGE_CURVE('',#41498,#41499,#34305,.T.);
#54425=EDGE_CURVE('',#41499,#41500,#34306,.T.);
#54426=EDGE_CURVE('',#41500,#41501,#34307,.T.);
#54427=EDGE_CURVE('',#41501,#41502,#34308,.T.);
#54428=EDGE_CURVE('',#41502,#41503,#34309,.T.);
#54429=EDGE_CURVE('',#41503,#41498,#34310,.T.);
#54430=EDGE_CURVE('',#41504,#41500,#1326,.T.);
#54431=EDGE_CURVE('',#41499,#41504,#1327,.T.);
#54432=EDGE_CURVE('',#41500,#41505,#1328,.T.);
#54433=EDGE_CURVE('',#41505,#41501,#1329,.T.);
#54434=EDGE_CURVE('',#41501,#41506,#1330,.T.);
#54435=EDGE_CURVE('',#41506,#41502,#1331,.T.);
#54436=EDGE_CURVE('',#41502,#41507,#1332,.T.);
#54437=EDGE_CURVE('',#41507,#41503,#1333,.T.);
#54438=EDGE_CURVE('',#41503,#41508,#1334,.T.);
#54439=EDGE_CURVE('',#41508,#41498,#1335,.T.);
#54440=EDGE_CURVE('',#41498,#41509,#1336,.T.);
#54441=EDGE_CURVE('',#41509,#41499,#1337,.T.);
#54442=EDGE_CURVE('',#41510,#41511,#34311,.T.);
#54443=EDGE_CURVE('',#41510,#41512,#34312,.T.);
#54444=EDGE_CURVE('',#41512,#41513,#34313,.T.);
#54445=EDGE_CURVE('',#41513,#41514,#34314,.T.);
#54446=EDGE_CURVE('',#41514,#41515,#34315,.T.);
#54447=EDGE_CURVE('',#41515,#41511,#34316,.T.);
#54448=EDGE_CURVE('',#41516,#41510,#1338,.T.);
#54449=EDGE_CURVE('',#41512,#41516,#1339,.T.);
#54450=EDGE_CURVE('',#41517,#41512,#1340,.T.);
#54451=EDGE_CURVE('',#41513,#41517,#1341,.T.);
#54452=EDGE_CURVE('',#41518,#41513,#1342,.T.);
#54453=EDGE_CURVE('',#41514,#41518,#1343,.T.);
#54454=EDGE_CURVE('',#41519,#41514,#1344,.T.);
#54455=EDGE_CURVE('',#41515,#41519,#1345,.T.);
#54456=EDGE_CURVE('',#41520,#41515,#1346,.T.);
#54457=EDGE_CURVE('',#41511,#41520,#1347,.T.);
#54458=EDGE_CURVE('',#41510,#41521,#1348,.T.);
#54459=EDGE_CURVE('',#41521,#41511,#1349,.T.);
#54460=EDGE_CURVE('',#41509,#41516,#23841,.T.);
#54461=EDGE_CURVE('',#41504,#41521,#23842,.T.);
#54462=EDGE_CURVE('',#41508,#41517,#23843,.T.);
#54463=EDGE_CURVE('',#41507,#41518,#23844,.T.);
#54464=EDGE_CURVE('',#41506,#41519,#23845,.T.);
#54465=EDGE_CURVE('',#41505,#41520,#23846,.T.);
#54466=EDGE_CURVE('',#41522,#41523,#23847,.T.);
#54467=EDGE_CURVE('',#41524,#41522,#1350,.T.);
#54468=EDGE_CURVE('',#41524,#41525,#23848,.T.);
#54469=EDGE_CURVE('',#41523,#41525,#1351,.T.);
#54470=EDGE_CURVE('',#41526,#41527,#23849,.T.);
#54471=EDGE_CURVE('',#41522,#41526,#1352,.T.);
#54472=EDGE_CURVE('',#41527,#41523,#1353,.T.);
#54473=EDGE_CURVE('',#41528,#41529,#23850,.T.);
#54474=EDGE_CURVE('',#41526,#41528,#1354,.T.);
#54475=EDGE_CURVE('',#41529,#41527,#1355,.T.);
#54476=EDGE_CURVE('',#41530,#41531,#23851,.T.);
#54477=EDGE_CURVE('',#41528,#41530,#1356,.T.);
#54478=EDGE_CURVE('',#41531,#41529,#1357,.T.);
#54479=EDGE_CURVE('',#41532,#41533,#23852,.T.);
#54480=EDGE_CURVE('',#41530,#41532,#1358,.T.);
#54481=EDGE_CURVE('',#41533,#41531,#1359,.T.);
#54482=EDGE_CURVE('',#41532,#41524,#1360,.T.);
#54483=EDGE_CURVE('',#41525,#41533,#1361,.T.);
#54484=EDGE_CURVE('',#41534,#41528,#23853,.T.);
#54485=EDGE_CURVE('',#41523,#41525,#34317,.T.);
#54486=EDGE_CURVE('',#41527,#41523,#34318,.T.);
#54487=EDGE_CURVE('',#41529,#41527,#34319,.T.);
#54488=EDGE_CURVE('',#41531,#41529,#34320,.T.);
#54489=EDGE_CURVE('',#41533,#41531,#34321,.T.);
#54490=EDGE_CURVE('',#41525,#41533,#34322,.T.);
#54491=EDGE_CURVE('',#41535,#41535,#34323,.T.);
#54492=EDGE_CURVE('',#41535,#41536,#34324,.T.);
#54493=EDGE_CURVE('',#41536,#41537,#34325,.T.);
#54494=EDGE_CURVE('',#41537,#41536,#34326,.T.);
#54495=EDGE_CURVE('',#41538,#41538,#34327,.T.);
#54496=EDGE_CURVE('',#41538,#41537,#23854,.T.);
#54497=EDGE_CURVE('',#41539,#41540,#2016,.T.);
#54498=EDGE_CURVE('',#41540,#41541,#2017,.T.);
#54499=EDGE_CURVE('',#41541,#41539,#23855,.T.);
#54500=EDGE_CURVE('',#41542,#41543,#23856,.T.);
#54501=EDGE_CURVE('',#41543,#41544,#2018,.T.);
#54502=EDGE_CURVE('',#41542,#41544,#34328,.T.);
#54503=EDGE_CURVE('',#41544,#41545,#34329,.T.);
#54504=EDGE_CURVE('',#41546,#41545,#34330,.T.);
#54505=EDGE_CURVE('',#41542,#41546,#34331,.T.);
#54506=EDGE_CURVE('',#41545,#41547,#23857,.T.);
#54507=EDGE_CURVE('',#41548,#41547,#34332,.T.);
#54508=EDGE_CURVE('',#41548,#41546,#23858,.T.);
#54509=EDGE_CURVE('',#41547,#41549,#34333,.T.);
#54510=EDGE_CURVE('',#41549,#41548,#34334,.T.);
#54511=EDGE_CURVE('',#41550,#41551,#34335,.T.);
#54512=EDGE_CURVE('',#41550,#41552,#5950,.T.);
#54513=EDGE_CURVE('',#41553,#41552,#34336,.T.);
#54514=EDGE_CURVE('',#41553,#41551,#34337,.T.);
#54515=EDGE_CURVE('',#41554,#41551,#34338,.T.);
#54516=EDGE_CURVE('',#41554,#41550,#34339,.T.);
#54517=EDGE_CURVE('',#41551,#41555,#34340,.T.);
#54518=EDGE_CURVE('',#41555,#41554,#5951,.T.);
#54519=EDGE_CURVE('',#41556,#41557,#34341,.T.);
#54520=EDGE_CURVE('',#41556,#41558,#5952,.T.);
#54521=EDGE_CURVE('',#41558,#41557,#34342,.T.);
#54522=EDGE_CURVE('',#41559,#41557,#34343,.T.);
#54523=EDGE_CURVE('',#41559,#41556,#34344,.T.);
#54524=EDGE_CURVE('',#41560,#41561,#34345,.T.);
#54525=EDGE_CURVE('',#41560,#41559,#5953,.T.);
#54526=EDGE_CURVE('',#41557,#41561,#34346,.T.);
#54527=EDGE_CURVE('',#41562,#41563,#34347,.T.);
#54528=EDGE_CURVE('',#41563,#41564,#5954,.T.);
#54529=EDGE_CURVE('',#41564,#41562,#34348,.T.);
#54530=EDGE_CURVE('',#41549,#41565,#5955,.T.);
#54531=EDGE_CURVE('',#41565,#41566,#34349,.T.);
#54532=EDGE_CURVE('',#41566,#41548,#34350,.T.);
#54533=EDGE_CURVE('',#41567,#41568,#2019,.T.);
#54534=EDGE_CURVE('',#41567,#41569,#23859,.T.);
#54535=EDGE_CURVE('',#41569,#41570,#2020,.T.);
#54536=EDGE_CURVE('',#41570,#41568,#23860,.T.);
#54537=EDGE_CURVE('',#41571,#41572,#2021,.T.);
#54538=EDGE_CURVE('',#41571,#41573,#23861,.T.);
#54539=EDGE_CURVE('',#41574,#41573,#5956,.T.);
#54540=EDGE_CURVE('',#41574,#41572,#23862,.T.);
#54541=EDGE_CURVE('',#41543,#41571,#23863,.T.);
#54542=EDGE_CURVE('',#41573,#41542,#23864,.T.);
#54543=EDGE_CURVE('',#41568,#41541,#23865,.T.);
#54544=EDGE_CURVE('',#41570,#41539,#23866,.T.);
#54545=EDGE_CURVE('',#41555,#41558,#23867,.T.);
#54546=EDGE_CURVE('',#41575,#41553,#23868,.T.);
#54547=EDGE_CURVE('',#41575,#41576,#23869,.T.);
#54548=EDGE_CURVE('',#41576,#41577,#23870,.T.);
#54549=EDGE_CURVE('',#41578,#41577,#23871,.T.);
#54550=EDGE_CURVE('',#41561,#41578,#23872,.T.);
#54551=EDGE_CURVE('',#41579,#41580,#23873,.T.);
#54552=EDGE_CURVE('',#41579,#41581,#2022,.T.);
#54553=EDGE_CURVE('',#41580,#41581,#2023,.T.);
#54554=EDGE_CURVE('',#41582,#41583,#34351,.T.);
#54555=EDGE_CURVE('',#41583,#41584,#2024,.T.);
#54556=EDGE_CURVE('',#41582,#41584,#23874,.T.);
#54557=EDGE_CURVE('',#41585,#41586,#34352,.T.);
#54558=EDGE_CURVE('',#41586,#41583,#34353,.T.);
#54559=EDGE_CURVE('',#41582,#41585,#34354,.T.);
#54560=EDGE_CURVE('',#41587,#41588,#34355,.T.);
#54561=EDGE_CURVE('',#41588,#41586,#23875,.T.);
#54562=EDGE_CURVE('',#41587,#41585,#23876,.T.);
#54563=EDGE_CURVE('',#41589,#41587,#34356,.T.);
#54564=EDGE_CURVE('',#41589,#41588,#34357,.T.);
#54565=EDGE_CURVE('',#41590,#41591,#34358,.T.);
#54566=EDGE_CURVE('',#41591,#41592,#5957,.T.);
#54567=EDGE_CURVE('',#41592,#41593,#34359,.T.);
#54568=EDGE_CURVE('',#41590,#41593,#34360,.T.);
#54569=EDGE_CURVE('',#41592,#41594,#34361,.T.);
#54570=EDGE_CURVE('',#41594,#41593,#34362,.T.);
#54571=EDGE_CURVE('',#41594,#41595,#5958,.T.);
#54572=EDGE_CURVE('',#41593,#41595,#34363,.T.);
#54573=EDGE_CURVE('',#41596,#41597,#34364,.T.);
#54574=EDGE_CURVE('',#41596,#41598,#5959,.T.);
#54575=EDGE_CURVE('',#41598,#41597,#34365,.T.);
#54576=EDGE_CURVE('',#41598,#41599,#34366,.T.);
#54577=EDGE_CURVE('',#41599,#41597,#34367,.T.);
#54578=EDGE_CURVE('',#41599,#41600,#5960,.T.);
#54579=EDGE_CURVE('',#41600,#41601,#34368,.T.);
#54580=EDGE_CURVE('',#41597,#41601,#34369,.T.);
#54581=EDGE_CURVE('',#41602,#41603,#34370,.T.);
#54582=EDGE_CURVE('',#41602,#41604,#5961,.T.);
#54583=EDGE_CURVE('',#41603,#41604,#34371,.T.);
#54584=EDGE_CURVE('',#41605,#41606,#34372,.T.);
#54585=EDGE_CURVE('',#41605,#41589,#5962,.T.);
#54586=EDGE_CURVE('',#41606,#41587,#34373,.T.);
#54587=EDGE_CURVE('',#41607,#41608,#2025,.T.);
#54588=EDGE_CURVE('',#41609,#41607,#23877,.T.);
#54589=EDGE_CURVE('',#41610,#41609,#2026,.T.);
#54590=EDGE_CURVE('',#41608,#41610,#23878,.T.);
#54591=EDGE_CURVE('',#41611,#41612,#2027,.T.);
#54592=EDGE_CURVE('',#41613,#41611,#23879,.T.);
#54593=EDGE_CURVE('',#41613,#41614,#5963,.T.);
#54594=EDGE_CURVE('',#41612,#41614,#23880,.T.);
#54595=EDGE_CURVE('',#41579,#41607,#23881,.T.);
#54596=EDGE_CURVE('',#41609,#41580,#23882,.T.);
#54597=EDGE_CURVE('',#41612,#41584,#23883,.T.);
#54598=EDGE_CURVE('',#41614,#41582,#23884,.T.);
#54599=EDGE_CURVE('',#41567,#41608,#23885,.T.);
#54600=EDGE_CURVE('',#41610,#41569,#23886,.T.);
#54601=EDGE_CURVE('',#41611,#41572,#23887,.T.);
#54602=EDGE_CURVE('',#41574,#41613,#23888,.T.);
#54603=EDGE_CURVE('',#41596,#41595,#23889,.T.);
#54604=EDGE_CURVE('',#41601,#41615,#23890,.T.);
#54605=EDGE_CURVE('',#41615,#41616,#23891,.T.);
#54606=EDGE_CURVE('',#41617,#41616,#23892,.T.);
#54607=EDGE_CURVE('',#41618,#41617,#23893,.T.);
#54608=EDGE_CURVE('',#41618,#41590,#23894,.T.);
#54609=EDGE_CURVE('',#41573,#41619,#34374,.T.);
#54610=EDGE_CURVE('',#41546,#41619,#23895,.T.);
#54611=EDGE_CURVE('',#41574,#41620,#34375,.T.);
#54612=EDGE_CURVE('',#41619,#41620,#1362,.T.);
#54613=EDGE_CURVE('',#41575,#41621,#34376,.T.);
#54614=EDGE_CURVE('',#41552,#41621,#23896,.T.);
#54615=EDGE_CURVE('',#41622,#41623,#34377,.T.);
#54616=EDGE_CURVE('',#41622,#41575,#34378,.T.);
#54617=EDGE_CURVE('',#41621,#41623,#34379,.T.);
#54618=EDGE_CURVE('',#41562,#41622,#23897,.T.);
#54619=EDGE_CURVE('',#41623,#41563,#23898,.T.);
#54620=EDGE_CURVE('',#41624,#41578,#34380,.T.);
#54621=EDGE_CURVE('',#41624,#41560,#23899,.T.);
#54622=EDGE_CURVE('',#41625,#41626,#34381,.T.);
#54623=EDGE_CURVE('',#41625,#41624,#34382,.T.);
#54624=EDGE_CURVE('',#41578,#41626,#34383,.T.);
#54625=EDGE_CURVE('',#41565,#41625,#23900,.T.);
#54626=EDGE_CURVE('',#41626,#41566,#23901,.T.);
#54627=EDGE_CURVE('',#41577,#41627,#34384,.T.);
#54628=EDGE_CURVE('',#41626,#41627,#23902,.T.);
#54629=EDGE_CURVE('',#41628,#41576,#34385,.T.);
#54630=EDGE_CURVE('',#41622,#41628,#23903,.T.);
#54631=EDGE_CURVE('',#41628,#41629,#23904,.T.);
#54632=EDGE_CURVE('',#41629,#41617,#34386,.T.);
#54633=EDGE_CURVE('',#41616,#41630,#34387,.T.);
#54634=EDGE_CURVE('',#41630,#41627,#23905,.T.);
#54635=EDGE_CURVE('',#41614,#41631,#34388,.T.);
#54636=EDGE_CURVE('',#41585,#41631,#23906,.T.);
#54637=EDGE_CURVE('',#41613,#41632,#34389,.T.);
#54638=EDGE_CURVE('',#41631,#41632,#1363,.T.);
#54639=EDGE_CURVE('',#41632,#41620,#23907,.T.);
#54640=EDGE_CURVE('',#41618,#41633,#34390,.T.);
#54641=EDGE_CURVE('',#41591,#41633,#23908,.T.);
#54642=EDGE_CURVE('',#41634,#41635,#34391,.T.);
#54643=EDGE_CURVE('',#41633,#41635,#34392,.T.);
#54644=EDGE_CURVE('',#41634,#41618,#34393,.T.);
#54645=EDGE_CURVE('',#41635,#41604,#23909,.T.);
#54646=EDGE_CURVE('',#41603,#41634,#23910,.T.);
#54647=EDGE_CURVE('',#41636,#41615,#34394,.T.);
#54648=EDGE_CURVE('',#41636,#41600,#23911,.T.);
#54649=EDGE_CURVE('',#41637,#41638,#34395,.T.);
#54650=EDGE_CURVE('',#41615,#41638,#34396,.T.);
#54651=EDGE_CURVE('',#41637,#41636,#34397,.T.);
#54652=EDGE_CURVE('',#41638,#41606,#23912,.T.);
#54653=EDGE_CURVE('',#41605,#41637,#23913,.T.);
#54654=EDGE_CURVE('',#41581,#41602,#23914,.T.);
#54655=EDGE_CURVE('',#41540,#41564,#23915,.T.);
#54656=EDGE_CURVE('',#41634,#41629,#23916,.T.);
#54657=EDGE_CURVE('',#41638,#41630,#23917,.T.);
#54658=EDGE_CURVE('',#41639,#41640,#23918,.T.);
#54659=EDGE_CURVE('',#41640,#41641,#5964,.F.);
#54660=EDGE_CURVE('',#41642,#41641,#34398,.T.);
#54661=EDGE_CURVE('',#41642,#41639,#5965,.F.);
#54662=EDGE_CURVE('',#41643,#41644,#23919,.T.);
#54663=EDGE_CURVE('',#41644,#41640,#5966,.F.);
#54664=EDGE_CURVE('',#41639,#41643,#5967,.F.);
#54665=EDGE_CURVE('',#41645,#41646,#23920,.T.);
#54666=EDGE_CURVE('',#41646,#41644,#5968,.F.);
#54667=EDGE_CURVE('',#41643,#41645,#5969,.F.);
#54668=EDGE_CURVE('',#41647,#41648,#23921,.T.);
#54669=EDGE_CURVE('',#41648,#41646,#5970,.F.);
#54670=EDGE_CURVE('',#41645,#41647,#5971,.F.);
#54671=EDGE_CURVE('',#41649,#41650,#23922,.T.);
#54672=EDGE_CURVE('',#41650,#41648,#5972,.F.);
#54673=EDGE_CURVE('',#41647,#41649,#5973,.F.);
#54674=EDGE_CURVE('',#41651,#41652,#23923,.T.);
#54675=EDGE_CURVE('',#41652,#41650,#5974,.F.);
#54676=EDGE_CURVE('',#41649,#41651,#5975,.F.);
#54677=EDGE_CURVE('',#41653,#41654,#23924,.T.);
#54678=EDGE_CURVE('',#41654,#41652,#5976,.F.);
#54679=EDGE_CURVE('',#41651,#41653,#5977,.F.);
#54680=EDGE_CURVE('',#41655,#41656,#23925,.T.);
#54681=EDGE_CURVE('',#41656,#41654,#5978,.F.);
#54682=EDGE_CURVE('',#41653,#41655,#5979,.F.);
#54683=EDGE_CURVE('',#41657,#41658,#23926,.T.);
#54684=EDGE_CURVE('',#41658,#41656,#5980,.F.);
#54685=EDGE_CURVE('',#41655,#41657,#5981,.F.);
#54686=EDGE_CURVE('',#41659,#41660,#23927,.T.);
#54687=EDGE_CURVE('',#41660,#41658,#5982,.F.);
#54688=EDGE_CURVE('',#41657,#41659,#5983,.F.);
#54689=EDGE_CURVE('',#41661,#41662,#23928,.T.);
#54690=EDGE_CURVE('',#41662,#41660,#5984,.F.);
#54691=EDGE_CURVE('',#41659,#41661,#5985,.F.);
#54692=EDGE_CURVE('',#41663,#41664,#23929,.T.);
#54693=EDGE_CURVE('',#41664,#41662,#5986,.F.);
#54694=EDGE_CURVE('',#41661,#41663,#5987,.F.);
#54695=EDGE_CURVE('',#41665,#41666,#23930,.T.);
#54696=EDGE_CURVE('',#41666,#41664,#5988,.F.);
#54697=EDGE_CURVE('',#41663,#41665,#5989,.F.);
#54698=EDGE_CURVE('',#41667,#41668,#23931,.T.);
#54699=EDGE_CURVE('',#41668,#41666,#5990,.F.);
#54700=EDGE_CURVE('',#41665,#41667,#5991,.F.);
#54701=EDGE_CURVE('',#41669,#41670,#23932,.T.);
#54702=EDGE_CURVE('',#41670,#41668,#5992,.F.);
#54703=EDGE_CURVE('',#41667,#41669,#5993,.F.);
#54704=EDGE_CURVE('',#41671,#41672,#23933,.T.);
#54705=EDGE_CURVE('',#41672,#41670,#5994,.F.);
#54706=EDGE_CURVE('',#41669,#41671,#5995,.F.);
#54707=EDGE_CURVE('',#41673,#41674,#23934,.T.);
#54708=EDGE_CURVE('',#41674,#41672,#5996,.F.);
#54709=EDGE_CURVE('',#41671,#41673,#5997,.F.);
#54710=EDGE_CURVE('',#41675,#41676,#23935,.T.);
#54711=EDGE_CURVE('',#41676,#41674,#5998,.F.);
#54712=EDGE_CURVE('',#41673,#41675,#5999,.F.);
#54713=EDGE_CURVE('',#41677,#41678,#23936,.T.);
#54714=EDGE_CURVE('',#41677,#41679,#6000,.F.);
#54715=EDGE_CURVE('',#41679,#41680,#6001,.T.);
#54716=EDGE_CURVE('',#41680,#41678,#6002,.F.);
#54717=EDGE_CURVE('',#41681,#41682,#23937,.T.);
#54718=EDGE_CURVE('',#41682,#41683,#6003,.F.);
#54719=EDGE_CURVE('',#41683,#41684,#34399,.T.);
#54720=EDGE_CURVE('',#41684,#41681,#6004,.F.);
#54721=EDGE_CURVE('',#41685,#41686,#23938,.T.);
#54722=EDGE_CURVE('',#41686,#41682,#6005,.F.);
#54723=EDGE_CURVE('',#41681,#41685,#6006,.F.);
#54724=EDGE_CURVE('',#41687,#41688,#23939,.T.);
#54725=EDGE_CURVE('',#41688,#41686,#6007,.F.);
#54726=EDGE_CURVE('',#41685,#41687,#6008,.F.);
#54727=EDGE_CURVE('',#41689,#41690,#23940,.T.);
#54728=EDGE_CURVE('',#41690,#41688,#6009,.F.);
#54729=EDGE_CURVE('',#41687,#41689,#6010,.F.);
#54730=EDGE_CURVE('',#41691,#41692,#23941,.T.);
#54731=EDGE_CURVE('',#41692,#41690,#6011,.F.);
#54732=EDGE_CURVE('',#41689,#41691,#6012,.F.);
#54733=EDGE_CURVE('',#41693,#41694,#23942,.T.);
#54734=EDGE_CURVE('',#41694,#41692,#6013,.F.);
#54735=EDGE_CURVE('',#41691,#41693,#6014,.F.);
#54736=EDGE_CURVE('',#41695,#41696,#23943,.T.);
#54737=EDGE_CURVE('',#41696,#41694,#6015,.F.);
#54738=EDGE_CURVE('',#41693,#41695,#6016,.F.);
#54739=EDGE_CURVE('',#41697,#41698,#23944,.T.);
#54740=EDGE_CURVE('',#41698,#41696,#6017,.F.);
#54741=EDGE_CURVE('',#41695,#41697,#6018,.F.);
#54742=EDGE_CURVE('',#41699,#41700,#23945,.T.);
#54743=EDGE_CURVE('',#41700,#41698,#6019,.F.);
#54744=EDGE_CURVE('',#41697,#41699,#6020,.F.);
#54745=EDGE_CURVE('',#41701,#41702,#23946,.T.);
#54746=EDGE_CURVE('',#41702,#41700,#6021,.F.);
#54747=EDGE_CURVE('',#41699,#41701,#6022,.F.);
#54748=EDGE_CURVE('',#41703,#41704,#23947,.T.);
#54749=EDGE_CURVE('',#41704,#41702,#6023,.F.);
#54750=EDGE_CURVE('',#41701,#41703,#6024,.F.);
#54751=EDGE_CURVE('',#41705,#41706,#23948,.T.);
#54752=EDGE_CURVE('',#41706,#41704,#6025,.F.);
#54753=EDGE_CURVE('',#41703,#41705,#6026,.F.);
#54754=EDGE_CURVE('',#41707,#41708,#23949,.T.);
#54755=EDGE_CURVE('',#41708,#41706,#6027,.F.);
#54756=EDGE_CURVE('',#41705,#41707,#6028,.F.);
#54757=EDGE_CURVE('',#41709,#41710,#23950,.T.);
#54758=EDGE_CURVE('',#41710,#41708,#6029,.F.);
#54759=EDGE_CURVE('',#41707,#41709,#6030,.F.);
#54760=EDGE_CURVE('',#41711,#41712,#23951,.T.);
#54761=EDGE_CURVE('',#41712,#41710,#6031,.F.);
#54762=EDGE_CURVE('',#41709,#41711,#6032,.F.);
#54763=EDGE_CURVE('',#41713,#41714,#23952,.T.);
#54764=EDGE_CURVE('',#41714,#41712,#6033,.F.);
#54765=EDGE_CURVE('',#41711,#41713,#6034,.F.);
#54766=EDGE_CURVE('',#41715,#41716,#23953,.T.);
#54767=EDGE_CURVE('',#41716,#41714,#6035,.F.);
#54768=EDGE_CURVE('',#41713,#41715,#6036,.F.);
#54769=EDGE_CURVE('',#41717,#41718,#23954,.T.);
#54770=EDGE_CURVE('',#41718,#41716,#6037,.F.);
#54771=EDGE_CURVE('',#41715,#41717,#6038,.F.);
#54772=EDGE_CURVE('',#41719,#41720,#23955,.T.);
#54773=EDGE_CURVE('',#41719,#41721,#6039,.T.);
#54774=EDGE_CURVE('',#41722,#41721,#6040,.T.);
#54775=EDGE_CURVE('',#41722,#41720,#6041,.F.);
#54776=EDGE_CURVE('',#41723,#41724,#23956,.T.);
#54777=EDGE_CURVE('',#41724,#41725,#1364,.T.);
#54778=EDGE_CURVE('',#41726,#41725,#6042,.T.);
#54779=EDGE_CURVE('',#41723,#41726,#1365,.T.);
#54780=EDGE_CURVE('',#41727,#41728,#23957,.T.);
#54781=EDGE_CURVE('',#41728,#41729,#1366,.T.);
#54782=EDGE_CURVE('',#41730,#41729,#6043,.T.);
#54783=EDGE_CURVE('',#41730,#41724,#1367,.T.);
#54784=EDGE_CURVE('',#41727,#41723,#1368,.T.);
#54785=EDGE_CURVE('',#41731,#41732,#23958,.T.);
#54786=EDGE_CURVE('',#41732,#41728,#1369,.T.);
#54787=EDGE_CURVE('',#41731,#41727,#1370,.T.);
#54788=EDGE_CURVE('',#41733,#41734,#23959,.T.);
#54789=EDGE_CURVE('',#41734,#41732,#1371,.T.);
#54790=EDGE_CURVE('',#41733,#41731,#1372,.T.);
#54791=EDGE_CURVE('',#41735,#41736,#23960,.T.);
#54792=EDGE_CURVE('',#41736,#41734,#1373,.T.);
#54793=EDGE_CURVE('',#41735,#41733,#1374,.T.);
#54794=EDGE_CURVE('',#41737,#41738,#23961,.T.);
#54795=EDGE_CURVE('',#41738,#41736,#1375,.T.);
#54796=EDGE_CURVE('',#41737,#41735,#1376,.T.);
#54797=EDGE_CURVE('',#41739,#41740,#23962,.T.);
#54798=EDGE_CURVE('',#41740,#41738,#1377,.T.);
#54799=EDGE_CURVE('',#41739,#41737,#1378,.T.);
#54800=EDGE_CURVE('',#41741,#41742,#23963,.T.);
#54801=EDGE_CURVE('',#41742,#41740,#1379,.T.);
#54802=EDGE_CURVE('',#41741,#41739,#1380,.T.);
#54803=EDGE_CURVE('',#41743,#41744,#23964,.T.);
#54804=EDGE_CURVE('',#41744,#41742,#1381,.T.);
#54805=EDGE_CURVE('',#41743,#41741,#1382,.T.);
#54806=EDGE_CURVE('',#41745,#41746,#23965,.T.);
#54807=EDGE_CURVE('',#41746,#41744,#1383,.T.);
#54808=EDGE_CURVE('',#41745,#41743,#1384,.T.);
#54809=EDGE_CURVE('',#41747,#41748,#23966,.T.);
#54810=EDGE_CURVE('',#41748,#41746,#1385,.T.);
#54811=EDGE_CURVE('',#41747,#41745,#1386,.T.);
#54812=EDGE_CURVE('',#41749,#41750,#23967,.T.);
#54813=EDGE_CURVE('',#41750,#41748,#1387,.T.);
#54814=EDGE_CURVE('',#41749,#41747,#1388,.T.);
#54815=EDGE_CURVE('',#41751,#41752,#23968,.T.);
#54816=EDGE_CURVE('',#41752,#41750,#1389,.T.);
#54817=EDGE_CURVE('',#41751,#41749,#1390,.T.);
#54818=EDGE_CURVE('',#41753,#41754,#23969,.T.);
#54819=EDGE_CURVE('',#41754,#41752,#1391,.T.);
#54820=EDGE_CURVE('',#41753,#41751,#1392,.T.);
#54821=EDGE_CURVE('',#41755,#41756,#23970,.T.);
#54822=EDGE_CURVE('',#41756,#41754,#1393,.T.);
#54823=EDGE_CURVE('',#41755,#41753,#1394,.T.);
#54824=EDGE_CURVE('',#41757,#41758,#23971,.T.);
#54825=EDGE_CURVE('',#41758,#41756,#1395,.T.);
#54826=EDGE_CURVE('',#41757,#41755,#1396,.T.);
#54827=EDGE_CURVE('',#41759,#41760,#23972,.T.);
#54828=EDGE_CURVE('',#41760,#41758,#1397,.T.);
#54829=EDGE_CURVE('',#41759,#41757,#1398,.T.);
#54830=EDGE_CURVE('',#41761,#41762,#23973,.T.);
#54831=EDGE_CURVE('',#41762,#41760,#1399,.T.);
#54832=EDGE_CURVE('',#41761,#41759,#1400,.T.);
#54833=EDGE_CURVE('',#41763,#41764,#23974,.T.);
#54834=EDGE_CURVE('',#41765,#41763,#34400,.T.);
#54835=EDGE_CURVE('',#41765,#41764,#1401,.T.);
#54836=EDGE_CURVE('',#41766,#41767,#23975,.T.);
#54837=EDGE_CURVE('',#41767,#41768,#6044,.T.);
#54838=EDGE_CURVE('',#41769,#41768,#34401,.T.);
#54839=EDGE_CURVE('',#41769,#41766,#6045,.T.);
#54840=EDGE_CURVE('',#41770,#41771,#23976,.T.);
#54841=EDGE_CURVE('',#41771,#41767,#6046,.T.);
#54842=EDGE_CURVE('',#41766,#41770,#6047,.T.);
#54843=EDGE_CURVE('',#41772,#41773,#23977,.T.);
#54844=EDGE_CURVE('',#41773,#41771,#6048,.T.);
#54845=EDGE_CURVE('',#41770,#41772,#6049,.T.);
#54846=EDGE_CURVE('',#41774,#41775,#23978,.T.);
#54847=EDGE_CURVE('',#41775,#41773,#6050,.T.);
#54848=EDGE_CURVE('',#41772,#41774,#6051,.T.);
#54849=EDGE_CURVE('',#41776,#41777,#23979,.T.);
#54850=EDGE_CURVE('',#41777,#41775,#6052,.T.);
#54851=EDGE_CURVE('',#41774,#41776,#6053,.T.);
#54852=EDGE_CURVE('',#41778,#41779,#23980,.T.);
#54853=EDGE_CURVE('',#41779,#41777,#6054,.T.);
#54854=EDGE_CURVE('',#41776,#41778,#6055,.T.);
#54855=EDGE_CURVE('',#41780,#41781,#23981,.T.);
#54856=EDGE_CURVE('',#41781,#41779,#6056,.T.);
#54857=EDGE_CURVE('',#41778,#41780,#6057,.T.);
#54858=EDGE_CURVE('',#41782,#41783,#23982,.T.);
#54859=EDGE_CURVE('',#41783,#41781,#6058,.T.);
#54860=EDGE_CURVE('',#41780,#41782,#6059,.T.);
#54861=EDGE_CURVE('',#41784,#41785,#23983,.T.);
#54862=EDGE_CURVE('',#41785,#41783,#6060,.T.);
#54863=EDGE_CURVE('',#41782,#41784,#6061,.T.);
#54864=EDGE_CURVE('',#41786,#41787,#23984,.T.);
#54865=EDGE_CURVE('',#41787,#41785,#6062,.T.);
#54866=EDGE_CURVE('',#41784,#41786,#6063,.T.);
#54867=EDGE_CURVE('',#41788,#41789,#23985,.T.);
#54868=EDGE_CURVE('',#41789,#41787,#6064,.T.);
#54869=EDGE_CURVE('',#41786,#41788,#6065,.T.);
#54870=EDGE_CURVE('',#41790,#41791,#23986,.T.);
#54871=EDGE_CURVE('',#41791,#41789,#6066,.T.);
#54872=EDGE_CURVE('',#41788,#41790,#6067,.T.);
#54873=EDGE_CURVE('',#41792,#41793,#23987,.T.);
#54874=EDGE_CURVE('',#41793,#41791,#6068,.T.);
#54875=EDGE_CURVE('',#41790,#41792,#6069,.T.);
#54876=EDGE_CURVE('',#41794,#41795,#23988,.T.);
#54877=EDGE_CURVE('',#41795,#41793,#6070,.T.);
#54878=EDGE_CURVE('',#41792,#41794,#6071,.T.);
#54879=EDGE_CURVE('',#41796,#41797,#23989,.T.);
#54880=EDGE_CURVE('',#41797,#41795,#6072,.T.);
#54881=EDGE_CURVE('',#41794,#41796,#6073,.T.);
#54882=EDGE_CURVE('',#41798,#41799,#23990,.T.);
#54883=EDGE_CURVE('',#41799,#41797,#6074,.T.);
#54884=EDGE_CURVE('',#41796,#41798,#6075,.T.);
#54885=EDGE_CURVE('',#41800,#41801,#23991,.T.);
#54886=EDGE_CURVE('',#41801,#41799,#6076,.T.);
#54887=EDGE_CURVE('',#41798,#41800,#6077,.T.);
#54888=EDGE_CURVE('',#41802,#41803,#23992,.T.);
#54889=EDGE_CURVE('',#41802,#41804,#6078,.T.);
#54890=EDGE_CURVE('',#41804,#41805,#6079,.T.);
#54891=EDGE_CURVE('',#41805,#41806,#6080,.F.);
#54892=EDGE_CURVE('',#41806,#41807,#34402,.T.);
#54893=EDGE_CURVE('',#41807,#41803,#6081,.T.);
#54894=EDGE_CURVE('',#41808,#41809,#23993,.T.);
#54895=EDGE_CURVE('',#41809,#41810,#1402,.T.);
#54896=EDGE_CURVE('',#41811,#41810,#6082,.T.);
#54897=EDGE_CURVE('',#41808,#41811,#1403,.T.);
#54898=EDGE_CURVE('',#41812,#41813,#23994,.T.);
#54899=EDGE_CURVE('',#41813,#41814,#1404,.T.);
#54900=EDGE_CURVE('',#41815,#41814,#6083,.T.);
#54901=EDGE_CURVE('',#41815,#41809,#1405,.T.);
#54902=EDGE_CURVE('',#41812,#41808,#1406,.T.);
#54903=EDGE_CURVE('',#41816,#41817,#23995,.T.);
#54904=EDGE_CURVE('',#41817,#41813,#1407,.T.);
#54905=EDGE_CURVE('',#41816,#41812,#1408,.T.);
#54906=EDGE_CURVE('',#41818,#41819,#23996,.T.);
#54907=EDGE_CURVE('',#41819,#41817,#1409,.T.);
#54908=EDGE_CURVE('',#41818,#41816,#1410,.T.);
#54909=EDGE_CURVE('',#41820,#41821,#23997,.T.);
#54910=EDGE_CURVE('',#41821,#41819,#1411,.T.);
#54911=EDGE_CURVE('',#41820,#41818,#1412,.T.);
#54912=EDGE_CURVE('',#41822,#41823,#23998,.T.);
#54913=EDGE_CURVE('',#41823,#41821,#1413,.T.);
#54914=EDGE_CURVE('',#41822,#41820,#1414,.T.);
#54915=EDGE_CURVE('',#41824,#41825,#23999,.T.);
#54916=EDGE_CURVE('',#41825,#41823,#1415,.T.);
#54917=EDGE_CURVE('',#41824,#41822,#1416,.T.);
#54918=EDGE_CURVE('',#41826,#41827,#24000,.T.);
#54919=EDGE_CURVE('',#41827,#41825,#1417,.T.);
#54920=EDGE_CURVE('',#41826,#41824,#1418,.T.);
#54921=EDGE_CURVE('',#41828,#41829,#24001,.T.);
#54922=EDGE_CURVE('',#41829,#41827,#1419,.T.);
#54923=EDGE_CURVE('',#41828,#41826,#1420,.T.);
#54924=EDGE_CURVE('',#41830,#41831,#24002,.T.);
#54925=EDGE_CURVE('',#41831,#41829,#1421,.T.);
#54926=EDGE_CURVE('',#41830,#41828,#1422,.T.);
#54927=EDGE_CURVE('',#41832,#41833,#24003,.T.);
#54928=EDGE_CURVE('',#41833,#41831,#1423,.T.);
#54929=EDGE_CURVE('',#41832,#41830,#1424,.T.);
#54930=EDGE_CURVE('',#41834,#41835,#24004,.T.);
#54931=EDGE_CURVE('',#41835,#41833,#1425,.T.);
#54932=EDGE_CURVE('',#41834,#41832,#1426,.T.);
#54933=EDGE_CURVE('',#41836,#41837,#24005,.T.);
#54934=EDGE_CURVE('',#41837,#41835,#1427,.T.);
#54935=EDGE_CURVE('',#41836,#41834,#1428,.T.);
#54936=EDGE_CURVE('',#41838,#41839,#24006,.T.);
#54937=EDGE_CURVE('',#41839,#41837,#1429,.T.);
#54938=EDGE_CURVE('',#41838,#41836,#1430,.T.);
#54939=EDGE_CURVE('',#41840,#41841,#24007,.T.);
#54940=EDGE_CURVE('',#41841,#41839,#1431,.T.);
#54941=EDGE_CURVE('',#41840,#41838,#1432,.T.);
#54942=EDGE_CURVE('',#41842,#41843,#24008,.T.);
#54943=EDGE_CURVE('',#41843,#41841,#1433,.T.);
#54944=EDGE_CURVE('',#41842,#41840,#1434,.T.);
#54945=EDGE_CURVE('',#41844,#41845,#24009,.T.);
#54946=EDGE_CURVE('',#41845,#41843,#1435,.T.);
#54947=EDGE_CURVE('',#41844,#41842,#1436,.T.);
#54948=EDGE_CURVE('',#41846,#41847,#24010,.T.);
#54949=EDGE_CURVE('',#41847,#41845,#1437,.T.);
#54950=EDGE_CURVE('',#41846,#41844,#1438,.T.);
#54951=EDGE_CURVE('',#41848,#41849,#24011,.T.);
#54952=EDGE_CURVE('',#41850,#41848,#34403,.T.);
#54953=EDGE_CURVE('',#41850,#41849,#1439,.T.);
#54954=EDGE_CURVE('',#41851,#41852,#24012,.T.);
#54955=EDGE_CURVE('',#41852,#41853,#34404,.T.);
#54956=EDGE_CURVE('',#41853,#41851,#6084,.T.);
#54957=EDGE_CURVE('',#41854,#41855,#24013,.T.);
#54958=EDGE_CURVE('',#41855,#41852,#6085,.T.);
#54959=EDGE_CURVE('',#41851,#41854,#6086,.T.);
#54960=EDGE_CURVE('',#41856,#41857,#24014,.T.);
#54961=EDGE_CURVE('',#41857,#41855,#6087,.T.);
#54962=EDGE_CURVE('',#41854,#41856,#6088,.T.);
#54963=EDGE_CURVE('',#41858,#41859,#24015,.T.);
#54964=EDGE_CURVE('',#41859,#41857,#6089,.T.);
#54965=EDGE_CURVE('',#41856,#41858,#6090,.T.);
#54966=EDGE_CURVE('',#41860,#41861,#24016,.T.);
#54967=EDGE_CURVE('',#41861,#41859,#6091,.T.);
#54968=EDGE_CURVE('',#41858,#41860,#6092,.T.);
#54969=EDGE_CURVE('',#41862,#41863,#24017,.T.);
#54970=EDGE_CURVE('',#41863,#41861,#6093,.T.);
#54971=EDGE_CURVE('',#41860,#41862,#6094,.T.);
#54972=EDGE_CURVE('',#41864,#41865,#24018,.T.);
#54973=EDGE_CURVE('',#41865,#41863,#6095,.T.);
#54974=EDGE_CURVE('',#41862,#41864,#6096,.T.);
#54975=EDGE_CURVE('',#41866,#41867,#24019,.T.);
#54976=EDGE_CURVE('',#41867,#41865,#6097,.T.);
#54977=EDGE_CURVE('',#41864,#41866,#6098,.T.);
#54978=EDGE_CURVE('',#41868,#41869,#24020,.T.);
#54979=EDGE_CURVE('',#41869,#41867,#6099,.T.);
#54980=EDGE_CURVE('',#41866,#41868,#6100,.T.);
#54981=EDGE_CURVE('',#41870,#41871,#24021,.T.);
#54982=EDGE_CURVE('',#41871,#41869,#6101,.T.);
#54983=EDGE_CURVE('',#41868,#41870,#6102,.T.);
#54984=EDGE_CURVE('',#41872,#41873,#24022,.T.);
#54985=EDGE_CURVE('',#41873,#41871,#6103,.T.);
#54986=EDGE_CURVE('',#41870,#41872,#6104,.T.);
#54987=EDGE_CURVE('',#41874,#41875,#24023,.T.);
#54988=EDGE_CURVE('',#41875,#41873,#6105,.T.);
#54989=EDGE_CURVE('',#41872,#41874,#6106,.T.);
#54990=EDGE_CURVE('',#41876,#41877,#24024,.T.);
#54991=EDGE_CURVE('',#41877,#41875,#6107,.T.);
#54992=EDGE_CURVE('',#41874,#41876,#6108,.T.);
#54993=EDGE_CURVE('',#41878,#41879,#24025,.T.);
#54994=EDGE_CURVE('',#41879,#41877,#6109,.T.);
#54995=EDGE_CURVE('',#41876,#41878,#6110,.T.);
#54996=EDGE_CURVE('',#41880,#41881,#24026,.T.);
#54997=EDGE_CURVE('',#41881,#41879,#6111,.T.);
#54998=EDGE_CURVE('',#41878,#41880,#6112,.T.);
#54999=EDGE_CURVE('',#41882,#41883,#24027,.T.);
#55000=EDGE_CURVE('',#41883,#41881,#6113,.T.);
#55001=EDGE_CURVE('',#41880,#41882,#6114,.T.);
#55002=EDGE_CURVE('',#41884,#41885,#24028,.T.);
#55003=EDGE_CURVE('',#41885,#41883,#6115,.T.);
#55004=EDGE_CURVE('',#41882,#41884,#6116,.T.);
#55005=EDGE_CURVE('',#41886,#41887,#24029,.T.);
#55006=EDGE_CURVE('',#41887,#41885,#6117,.T.);
#55007=EDGE_CURVE('',#41884,#41886,#6118,.T.);
#55008=EDGE_CURVE('',#41888,#41889,#24030,.T.);
#55009=EDGE_CURVE('',#41888,#41890,#6119,.T.);
#55010=EDGE_CURVE('',#41891,#41890,#6120,.T.);
#55011=EDGE_CURVE('',#41891,#41889,#6121,.T.);
#55012=EDGE_CURVE('',#41892,#41893,#24031,.T.);
#55013=EDGE_CURVE('',#41893,#41894,#1440,.T.);
#55014=EDGE_CURVE('',#41895,#41894,#6122,.T.);
#55015=EDGE_CURVE('',#41892,#41895,#1441,.T.);
#55016=EDGE_CURVE('',#41896,#41897,#24032,.T.);
#55017=EDGE_CURVE('',#41897,#41898,#1442,.T.);
#55018=EDGE_CURVE('',#41899,#41898,#6123,.T.);
#55019=EDGE_CURVE('',#41899,#41893,#1443,.T.);
#55020=EDGE_CURVE('',#41896,#41892,#1444,.T.);
#55021=EDGE_CURVE('',#41900,#41901,#24033,.T.);
#55022=EDGE_CURVE('',#41901,#41897,#1445,.T.);
#55023=EDGE_CURVE('',#41900,#41896,#1446,.T.);
#55024=EDGE_CURVE('',#41902,#41903,#24034,.T.);
#55025=EDGE_CURVE('',#41903,#41901,#1447,.T.);
#55026=EDGE_CURVE('',#41902,#41900,#1448,.T.);
#55027=EDGE_CURVE('',#41904,#41905,#24035,.T.);
#55028=EDGE_CURVE('',#41905,#41903,#1449,.T.);
#55029=EDGE_CURVE('',#41904,#41902,#1450,.T.);
#55030=EDGE_CURVE('',#41906,#41907,#24036,.T.);
#55031=EDGE_CURVE('',#41907,#41905,#1451,.T.);
#55032=EDGE_CURVE('',#41906,#41904,#1452,.T.);
#55033=EDGE_CURVE('',#41908,#41909,#24037,.T.);
#55034=EDGE_CURVE('',#41909,#41907,#1453,.T.);
#55035=EDGE_CURVE('',#41908,#41906,#1454,.T.);
#55036=EDGE_CURVE('',#41910,#41911,#24038,.T.);
#55037=EDGE_CURVE('',#41911,#41909,#1455,.T.);
#55038=EDGE_CURVE('',#41910,#41908,#1456,.T.);
#55039=EDGE_CURVE('',#41912,#41913,#24039,.T.);
#55040=EDGE_CURVE('',#41913,#41911,#1457,.T.);
#55041=EDGE_CURVE('',#41912,#41910,#1458,.T.);
#55042=EDGE_CURVE('',#41914,#41915,#24040,.T.);
#55043=EDGE_CURVE('',#41915,#41913,#1459,.T.);
#55044=EDGE_CURVE('',#41914,#41912,#1460,.T.);
#55045=EDGE_CURVE('',#41916,#41917,#24041,.T.);
#55046=EDGE_CURVE('',#41917,#41915,#1461,.T.);
#55047=EDGE_CURVE('',#41916,#41914,#1462,.T.);
#55048=EDGE_CURVE('',#41918,#41919,#24042,.T.);
#55049=EDGE_CURVE('',#41919,#41917,#1463,.T.);
#55050=EDGE_CURVE('',#41918,#41916,#1464,.T.);
#55051=EDGE_CURVE('',#41920,#41921,#24043,.T.);
#55052=EDGE_CURVE('',#41921,#41919,#1465,.T.);
#55053=EDGE_CURVE('',#41920,#41918,#1466,.T.);
#55054=EDGE_CURVE('',#41922,#41923,#24044,.T.);
#55055=EDGE_CURVE('',#41923,#41921,#1467,.T.);
#55056=EDGE_CURVE('',#41922,#41920,#1468,.T.);
#55057=EDGE_CURVE('',#41924,#41925,#24045,.T.);
#55058=EDGE_CURVE('',#41925,#41923,#1469,.T.);
#55059=EDGE_CURVE('',#41924,#41922,#1470,.T.);
#55060=EDGE_CURVE('',#41926,#41927,#24046,.T.);
#55061=EDGE_CURVE('',#41927,#41925,#1471,.T.);
#55062=EDGE_CURVE('',#41926,#41924,#1472,.T.);
#55063=EDGE_CURVE('',#41928,#41929,#24047,.T.);
#55064=EDGE_CURVE('',#41929,#41927,#1473,.T.);
#55065=EDGE_CURVE('',#41928,#41926,#1474,.T.);
#55066=EDGE_CURVE('',#41930,#41931,#24048,.T.);
#55067=EDGE_CURVE('',#41931,#41929,#1475,.T.);
#55068=EDGE_CURVE('',#41930,#41928,#1476,.T.);
#55069=EDGE_CURVE('',#41932,#41933,#24049,.T.);
#55070=EDGE_CURVE('',#41934,#41932,#34405,.T.);
#55071=EDGE_CURVE('',#41934,#41933,#1477,.T.);
#55072=EDGE_CURVE('',#41935,#41936,#24050,.T.);
#55073=EDGE_CURVE('',#41936,#41937,#1478,.T.);
#55074=EDGE_CURVE('',#41938,#41937,#6124,.T.);
#55075=EDGE_CURVE('',#41935,#41938,#1479,.T.);
#55076=EDGE_CURVE('',#41939,#41940,#24051,.T.);
#55077=EDGE_CURVE('',#41940,#41941,#1480,.T.);
#55078=EDGE_CURVE('',#41942,#41941,#6125,.T.);
#55079=EDGE_CURVE('',#41942,#41936,#1481,.T.);
#55080=EDGE_CURVE('',#41939,#41935,#1482,.T.);
#55081=EDGE_CURVE('',#41943,#41944,#24052,.T.);
#55082=EDGE_CURVE('',#41944,#41940,#1483,.T.);
#55083=EDGE_CURVE('',#41943,#41939,#1484,.T.);
#55084=EDGE_CURVE('',#41945,#41946,#24053,.T.);
#55085=EDGE_CURVE('',#41946,#41944,#1485,.T.);
#55086=EDGE_CURVE('',#41945,#41943,#1486,.T.);
#55087=EDGE_CURVE('',#41947,#41948,#24054,.T.);
#55088=EDGE_CURVE('',#41948,#41946,#1487,.T.);
#55089=EDGE_CURVE('',#41947,#41945,#1488,.T.);
#55090=EDGE_CURVE('',#41949,#41950,#24055,.T.);
#55091=EDGE_CURVE('',#41950,#41948,#1489,.T.);
#55092=EDGE_CURVE('',#41949,#41947,#1490,.T.);
#55093=EDGE_CURVE('',#41951,#41952,#24056,.T.);
#55094=EDGE_CURVE('',#41952,#41950,#1491,.T.);
#55095=EDGE_CURVE('',#41951,#41949,#1492,.T.);
#55096=EDGE_CURVE('',#41953,#41954,#24057,.T.);
#55097=EDGE_CURVE('',#41954,#41952,#1493,.T.);
#55098=EDGE_CURVE('',#41953,#41951,#1494,.T.);
#55099=EDGE_CURVE('',#41955,#41956,#24058,.T.);
#55100=EDGE_CURVE('',#41956,#41954,#1495,.T.);
#55101=EDGE_CURVE('',#41955,#41953,#1496,.T.);
#55102=EDGE_CURVE('',#41957,#41958,#24059,.T.);
#55103=EDGE_CURVE('',#41958,#41956,#1497,.T.);
#55104=EDGE_CURVE('',#41957,#41955,#1498,.T.);
#55105=EDGE_CURVE('',#41959,#41960,#24060,.T.);
#55106=EDGE_CURVE('',#41960,#41958,#1499,.T.);
#55107=EDGE_CURVE('',#41959,#41957,#1500,.T.);
#55108=EDGE_CURVE('',#41961,#41962,#24061,.T.);
#55109=EDGE_CURVE('',#41962,#41960,#1501,.T.);
#55110=EDGE_CURVE('',#41961,#41959,#1502,.T.);
#55111=EDGE_CURVE('',#41963,#41964,#24062,.T.);
#55112=EDGE_CURVE('',#41964,#41962,#1503,.T.);
#55113=EDGE_CURVE('',#41963,#41961,#1504,.T.);
#55114=EDGE_CURVE('',#41965,#41966,#24063,.T.);
#55115=EDGE_CURVE('',#41966,#41964,#1505,.T.);
#55116=EDGE_CURVE('',#41965,#41963,#1506,.T.);
#55117=EDGE_CURVE('',#41967,#41968,#24064,.T.);
#55118=EDGE_CURVE('',#41968,#41966,#1507,.T.);
#55119=EDGE_CURVE('',#41967,#41965,#1508,.T.);
#55120=EDGE_CURVE('',#41969,#41970,#24065,.T.);
#55121=EDGE_CURVE('',#41970,#41968,#1509,.T.);
#55122=EDGE_CURVE('',#41969,#41967,#1510,.T.);
#55123=EDGE_CURVE('',#41971,#41972,#24066,.T.);
#55124=EDGE_CURVE('',#41972,#41970,#1511,.T.);
#55125=EDGE_CURVE('',#41971,#41969,#1512,.T.);
#55126=EDGE_CURVE('',#41973,#41974,#24067,.T.);
#55127=EDGE_CURVE('',#41974,#41972,#1513,.T.);
#55128=EDGE_CURVE('',#41973,#41971,#1514,.T.);
#55129=EDGE_CURVE('',#41975,#41976,#24068,.T.);
#55130=EDGE_CURVE('',#41977,#41975,#34406,.T.);
#55131=EDGE_CURVE('',#41977,#41976,#1515,.T.);
#55132=EDGE_CURVE('',#41978,#41979,#24069,.T.);
#55133=EDGE_CURVE('',#41979,#41980,#24070,.T.);
#55134=EDGE_CURVE('',#41981,#41980,#24071,.T.);
#55135=EDGE_CURVE('',#41982,#41981,#24072,.T.);
#55136=EDGE_CURVE('',#41983,#41982,#24073,.T.);
#55137=EDGE_CURVE('',#41984,#41983,#24074,.T.);
#55138=EDGE_CURVE('',#41985,#41984,#24075,.T.);
#55139=EDGE_CURVE('',#41985,#41978,#24076,.T.);
#55140=EDGE_CURVE('',#41986,#41987,#24077,.T.);
#55141=EDGE_CURVE('',#41987,#41988,#34407,.T.);
#55142=EDGE_CURVE('',#41988,#41978,#24078,.T.);
#55143=EDGE_CURVE('',#41989,#41985,#24079,.T.);
#55144=EDGE_CURVE('',#41989,#41986,#34408,.T.);
#55145=EDGE_CURVE('',#41990,#41991,#6126,.T.);
#55146=EDGE_CURVE('',#41991,#41987,#24080,.T.);
#55147=EDGE_CURVE('',#41986,#41992,#24081,.T.);
#55148=EDGE_CURVE('',#41992,#41993,#24082,.T.);
#55149=EDGE_CURVE('',#41993,#41994,#24083,.T.);
#55150=EDGE_CURVE('',#41994,#41990,#6127,.T.);
#55151=EDGE_CURVE('',#41995,#41996,#24084,.T.);
#55152=EDGE_CURVE('',#41996,#41997,#24085,.T.);
#55153=EDGE_CURVE('',#41997,#41998,#24086,.T.);
#55154=EDGE_CURVE('',#41998,#41995,#24087,.T.);
#55155=EDGE_CURVE('',#41999,#41981,#24088,.T.);
#55156=EDGE_CURVE('',#42000,#41999,#24089,.T.);
#55157=EDGE_CURVE('',#42000,#41982,#24090,.T.);
#55158=EDGE_CURVE('',#41984,#42001,#24091,.T.);
#55159=EDGE_CURVE('',#42002,#41983,#24092,.T.);
#55160=EDGE_CURVE('',#42001,#42002,#24093,.T.);
#55161=EDGE_CURVE('',#42001,#41999,#24094,.T.);
#55162=EDGE_CURVE('',#42002,#42000,#24095,.T.);
#55163=EDGE_CURVE('',#41988,#42003,#24096,.T.);
#55164=EDGE_CURVE('',#42004,#42003,#34409,.T.);
#55165=EDGE_CURVE('',#42004,#42005,#24097,.T.);
#55166=EDGE_CURVE('',#42005,#42006,#24098,.T.);
#55167=EDGE_CURVE('',#42007,#42006,#34410,.T.);
#55168=EDGE_CURVE('',#42007,#41979,#24099,.T.);
#55169=EDGE_CURVE('',#42008,#42008,#34411,.T.);
#55170=EDGE_CURVE('',#42009,#42009,#34412,.T.);
#55171=EDGE_CURVE('',#42010,#42011,#6128,.T.);
#55172=EDGE_CURVE('',#42012,#42011,#24100,.T.);
#55173=EDGE_CURVE('',#42013,#42012,#6129,.T.);
#55174=EDGE_CURVE('',#42014,#42013,#6130,.T.);
#55175=EDGE_CURVE('',#42015,#42014,#6131,.T.);
#55176=EDGE_CURVE('',#42015,#42016,#24101,.T.);
#55177=EDGE_CURVE('',#42016,#42017,#34413,.T.);
#55178=EDGE_CURVE('',#42017,#42018,#24102,.T.);
#55179=EDGE_CURVE('',#42019,#42018,#6132,.T.);
#55180=EDGE_CURVE('',#42020,#42019,#6133,.T.);
#55181=EDGE_CURVE('',#42021,#42020,#6134,.T.);
#55182=EDGE_CURVE('',#42022,#42021,#24103,.T.);
#55183=EDGE_CURVE('',#42022,#42023,#6135,.T.);
#55184=EDGE_CURVE('',#42023,#42010,#2028,.T.);
#55185=EDGE_CURVE('',#42024,#42024,#34414,.T.);
#55186=EDGE_CURVE('',#42025,#42025,#34415,.T.);
#55187=EDGE_CURVE('',#42025,#42026,#24104,.T.);
#55188=EDGE_CURVE('',#42026,#42026,#34416,.T.);
#55189=EDGE_CURVE('',#42009,#42024,#24105,.T.);
#55190=EDGE_CURVE('',#42027,#42027,#34417,.T.);
#55191=EDGE_CURVE('',#42028,#42028,#34418,.T.);
#55192=EDGE_CURVE('',#42028,#42029,#24106,.T.);
#55193=EDGE_CURVE('',#42029,#42029,#34419,.T.);
#55194=EDGE_CURVE('',#42008,#42027,#24107,.T.);
#55195=EDGE_CURVE('',#42030,#42030,#34420,.T.);
#55196=EDGE_CURVE('',#42031,#42031,#34421,.T.);
#55197=EDGE_CURVE('',#42031,#42032,#24108,.T.);
#55198=EDGE_CURVE('',#42032,#42032,#34422,.T.);
#55199=EDGE_CURVE('',#42006,#42033,#6136,.T.);
#55200=EDGE_CURVE('',#42033,#42030,#24109,.T.);
#55201=EDGE_CURVE('',#42033,#42007,#6137,.T.);
#55202=EDGE_CURVE('',#42034,#42034,#34423,.T.);
#55203=EDGE_CURVE('',#42035,#42035,#34424,.T.);
#55204=EDGE_CURVE('',#42035,#42036,#24110,.T.);
#55205=EDGE_CURVE('',#42036,#42036,#34425,.T.);
#55206=EDGE_CURVE('',#42003,#42037,#34426,.T.);
#55207=EDGE_CURVE('',#42037,#42034,#24111,.T.);
#55208=EDGE_CURVE('',#42037,#42004,#34427,.T.);
#55209=EDGE_CURVE('',#42038,#42010,#34428,.T.);
#55210=EDGE_CURVE('',#42023,#42038,#34429,.T.);
#55211=EDGE_CURVE('',#42011,#42022,#34430,.T.);
#55212=EDGE_CURVE('',#42039,#42039,#34431,.T.);
#55213=EDGE_CURVE('',#42039,#42040,#34432,.T.);
#55214=EDGE_CURVE('',#42041,#42040,#34433,.T.);
#55215=EDGE_CURVE('',#42040,#42041,#34434,.T.);
#55216=EDGE_CURVE('',#42042,#42043,#34435,.T.);
#55217=EDGE_CURVE('',#42043,#42042,#34436,.T.);
#55218=EDGE_CURVE('',#42043,#42044,#34437,.T.);
#55219=EDGE_CURVE('',#42045,#42044,#34438,.T.);
#55220=EDGE_CURVE('',#42044,#42045,#34439,.T.);
#55221=EDGE_CURVE('',#42046,#42047,#24112,.T.);
#55222=EDGE_CURVE('',#42047,#42048,#1516,.T.);
#55223=EDGE_CURVE('',#42049,#42048,#24113,.T.);
#55224=EDGE_CURVE('',#42049,#42046,#1517,.T.);
#55225=EDGE_CURVE('',#42050,#42051,#24114,.T.);
#55226=EDGE_CURVE('',#42051,#42047,#1518,.T.);
#55227=EDGE_CURVE('',#42046,#42050,#1519,.T.);
#55228=EDGE_CURVE('',#42052,#42053,#24115,.T.);
#55229=EDGE_CURVE('',#42053,#42051,#1520,.T.);
#55230=EDGE_CURVE('',#42050,#42052,#1521,.T.);
#55231=EDGE_CURVE('',#42054,#42055,#24116,.T.);
#55232=EDGE_CURVE('',#42055,#42053,#1522,.T.);
#55233=EDGE_CURVE('',#42052,#42054,#1523,.T.);
#55234=EDGE_CURVE('',#42056,#42057,#24117,.T.);
#55235=EDGE_CURVE('',#42057,#42055,#1524,.T.);
#55236=EDGE_CURVE('',#42054,#42056,#1525,.T.);
#55237=EDGE_CURVE('',#42048,#42057,#1526,.T.);
#55238=EDGE_CURVE('',#42056,#42049,#1527,.T.);
#55239=EDGE_CURVE('',#42058,#42049,#24118,.T.);
#55240=EDGE_CURVE('',#42047,#42048,#34440,.T.);
#55241=EDGE_CURVE('',#42051,#42047,#34441,.T.);
#55242=EDGE_CURVE('',#42053,#42051,#34442,.T.);
#55243=EDGE_CURVE('',#42055,#42053,#34443,.T.);
#55244=EDGE_CURVE('',#42057,#42055,#34444,.T.);
#55245=EDGE_CURVE('',#42048,#42057,#34445,.T.);
#55246=EDGE_CURVE('',#42042,#42041,#24119,.T.);
#55247=EDGE_CURVE('',#42038,#42045,#24120,.T.);
#55248=EDGE_CURVE('',#42059,#42060,#6138,.T.);
#55249=EDGE_CURVE('',#42059,#42060,#6139,.T.);
#55250=EDGE_CURVE('',#42059,#42060,#6140,.T.);
#55251=EDGE_CURVE('',#42061,#42062,#6141,.T.);
#55252=EDGE_CURVE('',#42062,#42061,#6142,.T.);
#55253=EDGE_CURVE('',#42062,#42061,#6143,.T.);
#55254=EDGE_CURVE('',#42063,#42064,#34446,.T.);
#55255=EDGE_CURVE('',#42065,#42063,#2029,.T.);
#55256=EDGE_CURVE('',#42065,#42064,#34447,.T.);
#55257=EDGE_CURVE('',#42066,#42067,#34448,.T.);
#55258=EDGE_CURVE('',#42064,#42067,#6144,.T.);
#55259=EDGE_CURVE('',#42068,#42065,#6145,.T.);
#55260=EDGE_CURVE('',#42069,#42068,#6146,.T.);
#55261=EDGE_CURVE('',#42066,#42069,#6147,.T.);
#55262=EDGE_CURVE('',#42070,#42071,#34449,.T.);
#55263=EDGE_CURVE('',#42067,#42071,#2030,.T.);
#55264=EDGE_CURVE('',#42070,#42066,#2031,.T.);
#55265=EDGE_CURVE('',#42072,#42073,#34450,.T.);
#55266=EDGE_CURVE('',#42071,#42073,#6148,.T.);
#55267=EDGE_CURVE('',#42072,#42070,#6149,.T.);
#55268=EDGE_CURVE('',#42074,#42075,#34451,.T.);
#55269=EDGE_CURVE('',#42073,#42075,#6150,.T.);
#55270=EDGE_CURVE('',#42074,#42072,#6151,.T.);
#55271=EDGE_CURVE('',#42076,#42077,#6152,.T.);
#55272=EDGE_CURVE('',#42075,#42076,#6153,.T.);
#55273=EDGE_CURVE('',#42078,#42074,#6154,.T.);
#55274=EDGE_CURVE('',#42077,#42078,#6155,.T.);
#55275=EDGE_CURVE('',#42015,#42079,#6156,.T.);
#55276=EDGE_CURVE('',#42014,#42079,#34452,.T.);
#55277=EDGE_CURVE('',#42013,#42080,#34453,.T.);
#55278=EDGE_CURVE('',#42079,#42080,#6157,.T.);
#55279=EDGE_CURVE('',#42080,#42012,#24121,.T.);
#55280=EDGE_CURVE('',#42021,#42081,#24122,.T.);
#55281=EDGE_CURVE('',#42020,#42081,#34454,.T.);
#55282=EDGE_CURVE('',#42019,#42082,#34455,.T.);
#55283=EDGE_CURVE('',#42081,#42082,#6158,.T.);
#55284=EDGE_CURVE('',#42082,#42018,#6159,.T.);
#55285=EDGE_CURVE('',#42069,#42083,#6160,.T.);
#55286=EDGE_CURVE('',#42084,#42068,#6161,.T.);
#55287=EDGE_CURVE('',#42085,#42084,#24123,.T.);
#55288=EDGE_CURVE('',#42083,#42085,#6162,.T.);
#55289=EDGE_CURVE('',#42086,#42087,#34456,.T.);
#55290=EDGE_CURVE('',#42088,#42087,#6163,.T.);
#55291=EDGE_CURVE('',#42076,#42088,#6164,.T.);
#55292=EDGE_CURVE('',#42086,#42077,#2032,.T.);
#55293=EDGE_CURVE('',#42089,#42090,#34457,.T.);
#55294=EDGE_CURVE('',#42087,#42090,#24124,.T.);
#55295=EDGE_CURVE('',#42091,#42086,#24125,.T.);
#55296=EDGE_CURVE('',#42091,#42089,#34458,.T.);
#55297=EDGE_CURVE('',#42081,#42091,#6165,.T.);
#55298=EDGE_CURVE('',#42090,#42018,#6166,.T.);
#55299=EDGE_CURVE('',#42092,#42085,#6167,.T.);
#55300=EDGE_CURVE('',#42093,#42092,#6168,.T.);
#55301=EDGE_CURVE('',#42093,#42094,#34459,.T.);
#55302=EDGE_CURVE('',#42095,#42094,#2033,.T.);
#55303=EDGE_CURVE('',#42083,#42095,#6169,.T.);
#55304=EDGE_CURVE('',#42096,#42097,#34460,.T.);
#55305=EDGE_CURVE('',#42094,#42097,#24126,.T.);
#55306=EDGE_CURVE('',#42096,#42093,#24127,.T.);
#55307=EDGE_CURVE('',#42015,#42096,#6170,.T.);
#55308=EDGE_CURVE('',#42097,#42080,#6171,.T.);
#55309=EDGE_CURVE('',#42088,#42098,#2034,.T.);
#55310=EDGE_CURVE('',#42099,#42087,#34461,.T.);
#55311=EDGE_CURVE('',#42099,#42098,#34462,.T.);
#55312=EDGE_CURVE('',#42100,#42101,#34463,.T.);
#55313=EDGE_CURVE('',#42098,#42101,#34464,.T.);
#55314=EDGE_CURVE('',#42100,#42099,#34465,.T.);
#55315=EDGE_CURVE('',#42100,#42102,#34466,.T.);
#55316=EDGE_CURVE('',#42101,#42102,#34467,.T.);
#55317=EDGE_CURVE('',#42103,#42104,#34468,.T.);
#55318=EDGE_CURVE('',#42102,#42104,#24128,.T.);
#55319=EDGE_CURVE('',#42103,#42100,#24129,.T.);
#55320=EDGE_CURVE('',#42105,#42017,#34469,.T.);
#55321=EDGE_CURVE('',#42104,#42017,#6172,.T.);
#55322=EDGE_CURVE('',#42105,#42103,#6173,.T.);
#55323=EDGE_CURVE('',#42090,#42105,#24130,.T.);
#55324=EDGE_CURVE('',#42093,#42106,#34470,.T.);
#55325=EDGE_CURVE('',#42107,#42092,#34471,.T.);
#55326=EDGE_CURVE('',#42107,#42106,#34472,.T.);
#55327=EDGE_CURVE('',#42108,#42107,#34473,.T.);
#55328=EDGE_CURVE('',#42108,#42106,#34474,.T.);
#55329=EDGE_CURVE('',#42109,#42110,#34475,.T.);
#55330=EDGE_CURVE('',#42106,#42110,#24131,.T.);
#55331=EDGE_CURVE('',#42109,#42108,#24132,.T.);
#55332=EDGE_CURVE('',#42016,#42111,#34476,.T.);
#55333=EDGE_CURVE('',#42110,#42111,#6174,.T.);
#55334=EDGE_CURVE('',#42016,#42109,#6175,.T.);
#55335=EDGE_CURVE('',#42111,#42096,#24133,.T.);
#55336=EDGE_CURVE('',#42084,#42063,#1528,.T.);
#55337=EDGE_CURVE('',#42078,#42095,#34477,.T.);
#55338=EDGE_CURVE('',#42112,#42113,#24134,.T.);
#55339=EDGE_CURVE('',#42113,#42114,#34478,.T.);
#55340=EDGE_CURVE('',#42114,#42115,#24135,.T.);
#55341=EDGE_CURVE('',#42112,#42115,#6176,.T.);
#55342=EDGE_CURVE('',#42116,#42117,#24136,.T.);
#55343=EDGE_CURVE('',#42117,#42118,#34479,.T.);
#55344=EDGE_CURVE('',#42118,#42119,#24137,.T.);
#55345=EDGE_CURVE('',#42116,#42119,#6177,.T.);
#55346=EDGE_CURVE('',#42120,#42121,#24138,.T.);
#55347=EDGE_CURVE('',#42121,#42122,#34480,.T.);
#55348=EDGE_CURVE('',#42122,#42123,#24139,.T.);
#55349=EDGE_CURVE('',#42120,#42123,#6178,.T.);
#55350=EDGE_CURVE('',#42120,#42124,#34481,.T.);
#55351=EDGE_CURVE('',#42123,#42125,#34482,.T.);
#55352=EDGE_CURVE('',#42125,#42124,#6179,.T.);
#55353=EDGE_CURVE('',#42126,#42127,#24140,.T.);
#55354=EDGE_CURVE('',#42127,#42128,#34483,.T.);
#55355=EDGE_CURVE('',#42128,#42129,#24141,.T.);
#55356=EDGE_CURVE('',#42126,#42129,#6180,.T.);
#55357=EDGE_CURVE('',#42130,#42131,#24142,.T.);
#55358=EDGE_CURVE('',#42131,#42132,#34484,.T.);
#55359=EDGE_CURVE('',#42132,#42133,#24143,.T.);
#55360=EDGE_CURVE('',#42130,#42133,#1529,.T.);
#55361=EDGE_CURVE('',#42131,#42122,#24144,.T.);
#55362=EDGE_CURVE('',#42123,#42130,#6181,.T.);
#55363=EDGE_CURVE('',#42130,#42134,#34485,.T.);
#55364=EDGE_CURVE('',#42133,#42135,#34486,.T.);
#55365=EDGE_CURVE('',#42135,#42134,#6182,.T.);
#55366=EDGE_CURVE('',#42127,#42132,#34487,.T.);
#55367=EDGE_CURVE('',#42133,#42126,#34488,.T.);
#55368=EDGE_CURVE('',#42126,#42136,#34489,.T.);
#55369=EDGE_CURVE('',#42129,#42137,#34490,.T.);
#55370=EDGE_CURVE('',#42137,#42136,#6183,.T.);
#55371=EDGE_CURVE('',#42117,#42128,#24145,.T.);
#55372=EDGE_CURVE('',#42129,#42116,#6184,.T.);
#55373=EDGE_CURVE('',#42116,#42138,#34491,.T.);
#55374=EDGE_CURVE('',#42119,#42139,#34492,.T.);
#55375=EDGE_CURVE('',#42139,#42138,#6185,.T.);
#55376=EDGE_CURVE('',#42140,#42141,#24146,.T.);
#55377=EDGE_CURVE('',#42141,#42142,#34493,.T.);
#55378=EDGE_CURVE('',#42142,#42143,#24147,.T.);
#55379=EDGE_CURVE('',#42140,#42143,#6186,.T.);
#55380=EDGE_CURVE('',#42144,#42145,#24148,.T.);
#55381=EDGE_CURVE('',#42145,#42146,#34494,.T.);
#55382=EDGE_CURVE('',#42146,#42147,#24149,.T.);
#55383=EDGE_CURVE('',#42144,#42147,#1530,.T.);
#55384=EDGE_CURVE('',#42067,#42144,#6187,.T.);
#55385=EDGE_CURVE('',#42148,#42071,#24150,.T.);
#55386=EDGE_CURVE('',#42145,#42148,#24151,.T.);
#55387=EDGE_CURVE('',#42144,#42149,#34495,.T.);
#55388=EDGE_CURVE('',#42147,#42150,#34496,.T.);
#55389=EDGE_CURVE('',#42150,#42149,#6188,.T.);
#55390=EDGE_CURVE('',#42141,#42146,#34497,.T.);
#55391=EDGE_CURVE('',#42147,#42140,#34498,.T.);
#55392=EDGE_CURVE('',#42140,#42151,#34499,.T.);
#55393=EDGE_CURVE('',#42143,#42152,#34500,.T.);
#55394=EDGE_CURVE('',#42152,#42151,#6189,.T.);
#55395=EDGE_CURVE('',#42113,#42142,#24152,.T.);
#55396=EDGE_CURVE('',#42143,#42112,#6190,.T.);
#55397=EDGE_CURVE('',#42112,#42153,#34501,.T.);
#55398=EDGE_CURVE('',#42115,#42154,#34502,.T.);
#55399=EDGE_CURVE('',#42154,#42153,#6191,.T.);
#55400=EDGE_CURVE('',#42153,#42152,#6192,.T.);
#55401=EDGE_CURVE('',#42151,#42150,#34503,.T.);
#55402=EDGE_CURVE('',#42138,#42137,#6193,.T.);
#55403=EDGE_CURVE('',#42136,#42135,#34504,.T.);
#55404=EDGE_CURVE('',#42134,#42125,#6194,.T.);
#55405=EDGE_CURVE('',#42155,#42156,#24153,.T.);
#55406=EDGE_CURVE('',#42155,#42157,#6195,.T.);
#55407=EDGE_CURVE('',#42158,#42157,#24154,.T.);
#55408=EDGE_CURVE('',#42156,#42158,#34505,.T.);
#55409=EDGE_CURVE('',#42159,#42160,#24155,.T.);
#55410=EDGE_CURVE('',#42159,#42161,#6196,.T.);
#55411=EDGE_CURVE('',#42162,#42161,#24156,.T.);
#55412=EDGE_CURVE('',#42160,#42162,#34506,.T.);
#55413=EDGE_CURVE('',#42163,#42164,#24157,.T.);
#55414=EDGE_CURVE('',#42163,#42165,#6197,.T.);
#55415=EDGE_CURVE('',#42166,#42165,#24158,.T.);
#55416=EDGE_CURVE('',#42164,#42166,#34507,.T.);
#55417=EDGE_CURVE('',#42167,#42168,#24159,.T.);
#55418=EDGE_CURVE('',#42167,#42169,#6198,.T.);
#55419=EDGE_CURVE('',#42170,#42169,#24160,.T.);
#55420=EDGE_CURVE('',#42168,#42170,#34508,.T.);
#55421=EDGE_CURVE('',#42120,#42167,#34509,.T.);
#55422=EDGE_CURVE('',#42168,#42121,#34510,.T.);
#55423=EDGE_CURVE('',#42167,#42171,#34511,.T.);
#55424=EDGE_CURVE('',#42172,#42171,#6199,.T.);
#55425=EDGE_CURVE('',#42169,#42172,#34512,.T.);
#55426=EDGE_CURVE('',#42173,#42174,#24161,.T.);
#55427=EDGE_CURVE('',#42173,#42175,#6200,.T.);
#55428=EDGE_CURVE('',#42176,#42175,#24162,.T.);
#55429=EDGE_CURVE('',#42174,#42176,#34513,.T.);
#55430=EDGE_CURVE('',#42177,#42178,#24163,.T.);
#55431=EDGE_CURVE('',#42177,#42179,#6201,.T.);
#55432=EDGE_CURVE('',#42180,#42179,#24164,.T.);
#55433=EDGE_CURVE('',#42178,#42180,#34514,.T.);
#55434=EDGE_CURVE('',#42169,#42177,#6202,.T.);
#55435=EDGE_CURVE('',#42178,#42170,#24165,.T.);
#55436=EDGE_CURVE('',#42177,#42181,#34515,.T.);
#55437=EDGE_CURVE('',#42182,#42181,#6203,.T.);
#55438=EDGE_CURVE('',#42179,#42182,#34516,.T.);
#55439=EDGE_CURVE('',#42179,#42173,#34517,.T.);
#55440=EDGE_CURVE('',#42174,#42180,#34518,.T.);
#55441=EDGE_CURVE('',#42173,#42183,#34519,.T.);
#55442=EDGE_CURVE('',#42184,#42183,#6204,.T.);
#55443=EDGE_CURVE('',#42175,#42184,#34520,.T.);
#55444=EDGE_CURVE('',#42175,#42163,#6205,.T.);
#55445=EDGE_CURVE('',#42164,#42176,#24166,.T.);
#55446=EDGE_CURVE('',#42163,#42185,#34521,.T.);
#55447=EDGE_CURVE('',#42186,#42185,#6206,.T.);
#55448=EDGE_CURVE('',#42165,#42186,#34522,.T.);
#55449=EDGE_CURVE('',#42160,#42166,#34523,.T.);
#55450=EDGE_CURVE('',#42165,#42159,#34524,.T.);
#55451=EDGE_CURVE('',#42159,#42187,#34525,.T.);
#55452=EDGE_CURVE('',#42188,#42187,#6207,.T.);
#55453=EDGE_CURVE('',#42161,#42188,#34526,.T.);
#55454=EDGE_CURVE('',#42189,#42190,#24167,.T.);
#55455=EDGE_CURVE('',#42189,#42191,#6208,.T.);
#55456=EDGE_CURVE('',#42192,#42191,#24168,.T.);
#55457=EDGE_CURVE('',#42190,#42192,#34527,.T.);
#55458=EDGE_CURVE('',#42193,#42194,#24169,.T.);
#55459=EDGE_CURVE('',#42193,#42195,#6209,.T.);
#55460=EDGE_CURVE('',#42196,#42195,#24170,.T.);
#55461=EDGE_CURVE('',#42194,#42196,#34528,.T.);
#55462=EDGE_CURVE('',#42161,#42193,#6210,.T.);
#55463=EDGE_CURVE('',#42194,#42162,#24171,.T.);
#55464=EDGE_CURVE('',#42193,#42197,#34529,.T.);
#55465=EDGE_CURVE('',#42198,#42197,#6211,.T.);
#55466=EDGE_CURVE('',#42195,#42198,#34530,.T.);
#55467=EDGE_CURVE('',#42195,#42189,#34531,.T.);
#55468=EDGE_CURVE('',#42190,#42196,#34532,.T.);
#55469=EDGE_CURVE('',#42189,#42199,#34533,.T.);
#55470=EDGE_CURVE('',#42200,#42199,#6212,.T.);
#55471=EDGE_CURVE('',#42191,#42200,#34534,.T.);
#55472=EDGE_CURVE('',#42191,#42155,#6213,.T.);
#55473=EDGE_CURVE('',#42156,#42192,#24172,.T.);
#55474=EDGE_CURVE('',#42155,#42201,#34535,.T.);
#55475=EDGE_CURVE('',#42202,#42201,#6214,.T.);
#55476=EDGE_CURVE('',#42157,#42202,#34536,.T.);
#55477=EDGE_CURVE('',#42157,#42115,#34537,.T.);
#55478=EDGE_CURVE('',#42114,#42158,#34538,.T.);
#55479=EDGE_CURVE('',#42154,#42202,#34539,.T.);
#55480=EDGE_CURVE('',#42101,#42107,#34540,.T.);
#55481=EDGE_CURVE('',#42108,#42102,#34541,.T.);
#55482=EDGE_CURVE('',#42104,#42109,#34542,.T.);
#55483=EDGE_CURVE('',#42171,#42124,#34543,.T.);
#55484=EDGE_CURVE('',#42187,#42186,#34544,.T.);
#55485=EDGE_CURVE('',#42201,#42200,#6215,.T.);
#55486=EDGE_CURVE('',#42199,#42198,#34545,.T.);
#55487=EDGE_CURVE('',#42197,#42188,#6216,.T.);
#55488=EDGE_CURVE('',#42185,#42184,#6217,.T.);
#55489=EDGE_CURVE('',#42183,#42182,#34546,.T.);
#55490=EDGE_CURVE('',#42181,#42172,#6218,.T.);
#55491=EDGE_CURVE('',#42073,#42203,#24173,.T.);
#55492=EDGE_CURVE('',#42203,#42148,#34547,.T.);
#55493=EDGE_CURVE('',#42119,#42075,#34548,.T.);
#55494=EDGE_CURVE('',#42203,#42118,#34549,.T.);
#55495=EDGE_CURVE('',#42098,#42139,#34550,.T.);
#55496=EDGE_CURVE('',#42149,#42064,#6219,.T.);
#55497=EDGE_CURVE('',#42204,#42205,#6220,.T.);
#55498=EDGE_CURVE('',#42205,#42204,#6221,.T.);
#55499=EDGE_CURVE('',#42204,#42205,#6222,.T.);
#55500=EDGE_CURVE('',#42205,#42206,#6223,.T.);
#55501=EDGE_CURVE('',#42206,#42207,#6224,.T.);
#55502=EDGE_CURVE('',#42207,#42204,#6225,.T.);
#55503=EDGE_CURVE('',#41941,#41942,#6226,.T.);
#55504=EDGE_CURVE('',#42208,#42209,#24174,.T.);
#55505=EDGE_CURVE('',#42208,#42210,#6227,.T.);
#55506=EDGE_CURVE('',#42210,#42209,#6228,.T.);
#55507=EDGE_CURVE('',#42211,#42212,#24175,.T.);
#55508=EDGE_CURVE('',#42211,#42207,#34551,.T.);
#55509=EDGE_CURVE('',#42207,#42206,#6229,.T.);
#55510=EDGE_CURVE('',#42206,#41679,#6230,.T.);
#55511=EDGE_CURVE('',#41679,#42212,#6231,.T.);
#55512=EDGE_CURVE('',#42213,#42211,#24176,.T.);
#55513=EDGE_CURVE('',#42214,#42213,#6232,.T.);
#55514=EDGE_CURVE('',#42214,#42208,#24177,.T.);
#55515=EDGE_CURVE('',#41680,#42208,#34552,.T.);
#55516=EDGE_CURVE('',#41976,#41974,#1531,.T.);
#55517=EDGE_CURVE('',#41975,#41973,#1532,.T.);
#55518=EDGE_CURVE('',#41937,#41680,#6233,.T.);
#55519=EDGE_CURVE('',#41641,#41977,#6234,.T.);
#55520=EDGE_CURVE('',#41678,#41676,#6235,.F.);
#55521=EDGE_CURVE('',#42215,#41677,#6236,.F.);
#55522=EDGE_CURVE('',#42212,#42215,#6237,.T.);
#55523=EDGE_CURVE('',#41975,#41642,#6238,.T.);
#55524=EDGE_CURVE('',#42209,#41938,#6239,.T.);
#55525=EDGE_CURVE('',#41675,#42210,#6240,.F.);
#55526=EDGE_CURVE('',#42216,#42217,#6241,.T.);
#55527=EDGE_CURVE('',#42216,#42217,#6242,.T.);
#55528=EDGE_CURVE('',#41898,#41899,#6243,.T.);
#55529=EDGE_CURVE('',#41722,#42218,#6244,.T.);
#55530=EDGE_CURVE('',#42218,#41895,#6245,.T.);
#55531=EDGE_CURVE('',#41894,#41722,#6246,.T.);
#55532=EDGE_CURVE('',#42219,#42220,#24178,.T.);
#55533=EDGE_CURVE('',#42219,#41721,#2035,.T.);
#55534=EDGE_CURVE('',#41721,#42220,#6247,.T.);
#55535=EDGE_CURVE('',#42221,#42219,#24179,.T.);
#55536=EDGE_CURVE('',#42221,#42222,#6248,.T.);
#55537=EDGE_CURVE('',#42222,#42223,#24180,.T.);
#55538=EDGE_CURVE('',#42224,#42223,#6249,.T.);
#55539=EDGE_CURVE('',#42224,#42218,#6250,.T.);
#55540=EDGE_CURVE('',#41933,#41931,#1533,.T.);
#55541=EDGE_CURVE('',#41932,#41930,#1534,.T.);
#55542=EDGE_CURVE('',#42217,#42216,#6251,.T.);
#55543=EDGE_CURVE('',#41683,#41934,#6252,.T.);
#55544=EDGE_CURVE('',#41720,#41718,#6253,.F.);
#55545=EDGE_CURVE('',#42224,#41719,#6254,.T.);
#55546=EDGE_CURVE('',#42225,#42224,#6255,.T.);
#55547=EDGE_CURVE('',#42220,#42225,#6256,.T.);
#55548=EDGE_CURVE('',#41932,#41684,#6257,.T.);
#55549=EDGE_CURVE('',#41717,#42218,#6258,.F.);
#55550=EDGE_CURVE('',#42226,#42059,#6259,.T.);
#55551=EDGE_CURVE('',#42226,#42227,#6260,.T.);
#55552=EDGE_CURVE('',#42060,#42227,#6261,.T.);
#55553=EDGE_CURVE('',#41889,#41887,#6262,.T.);
#55554=EDGE_CURVE('',#41886,#42228,#6263,.T.);
#55555=EDGE_CURVE('',#42229,#42228,#6264,.T.);
#55556=EDGE_CURVE('',#42229,#41888,#6265,.T.);
#55557=EDGE_CURVE('',#41814,#41815,#6266,.T.);
#55558=EDGE_CURVE('',#41891,#42228,#6267,.T.);
#55559=EDGE_CURVE('',#42228,#41811,#6268,.T.);
#55560=EDGE_CURVE('',#41810,#41891,#6269,.T.);
#55561=EDGE_CURVE('',#42230,#42231,#24181,.T.);
#55562=EDGE_CURVE('',#42230,#41890,#34553,.T.);
#55563=EDGE_CURVE('',#41890,#42231,#6270,.T.);
#55564=EDGE_CURVE('',#42232,#42230,#24182,.T.);
#55565=EDGE_CURVE('',#42232,#42233,#6271,.T.);
#55566=EDGE_CURVE('',#42233,#42234,#24183,.T.);
#55567=EDGE_CURVE('',#42229,#42234,#6272,.T.);
#55568=EDGE_CURVE('',#41849,#41847,#1535,.T.);
#55569=EDGE_CURVE('',#41848,#41846,#1536,.T.);
#55570=EDGE_CURVE('',#42227,#42226,#6273,.T.);
#55571=EDGE_CURVE('',#41852,#41850,#6274,.T.);
#55572=EDGE_CURVE('',#42235,#42229,#6275,.T.);
#55573=EDGE_CURVE('',#42231,#42235,#6276,.T.);
#55574=EDGE_CURVE('',#41848,#41853,#6277,.T.);
#55575=EDGE_CURVE('',#42236,#42061,#6278,.F.);
#55576=EDGE_CURVE('',#42062,#42237,#6279,.T.);
#55577=EDGE_CURVE('',#42237,#42236,#6280,.T.);
#55578=EDGE_CURVE('',#41803,#41801,#6281,.T.);
#55579=EDGE_CURVE('',#41800,#41802,#6282,.T.);
#55580=EDGE_CURVE('',#41729,#41730,#6283,.T.);
#55581=EDGE_CURVE('',#42238,#42239,#24184,.T.);
#55582=EDGE_CURVE('',#42238,#41804,#6284,.T.);
#55583=EDGE_CURVE('',#41804,#42239,#6285,.T.);
#55584=EDGE_CURVE('',#42240,#42241,#24185,.T.);
#55585=EDGE_CURVE('',#42240,#42236,#34554,.T.);
#55586=EDGE_CURVE('',#42236,#42237,#6286,.T.);
#55587=EDGE_CURVE('',#42237,#41806,#6287,.T.);
#55588=EDGE_CURVE('',#41806,#42241,#6288,.T.);
#55589=EDGE_CURVE('',#42242,#42240,#24186,.T.);
#55590=EDGE_CURVE('',#42243,#42242,#6289,.T.);
#55591=EDGE_CURVE('',#42243,#42238,#24187,.T.);
#55592=EDGE_CURVE('',#41807,#42238,#34555,.T.);
#55593=EDGE_CURVE('',#41763,#41769,#6290,.T.);
#55594=EDGE_CURVE('',#41768,#41765,#6291,.T.);
#55595=EDGE_CURVE('',#41764,#41762,#1537,.T.);
#55596=EDGE_CURVE('',#41763,#41761,#1538,.T.);
#55597=EDGE_CURVE('',#41725,#41807,#6292,.T.);
#55598=EDGE_CURVE('',#42241,#41805,#6293,.T.);
#55599=EDGE_CURVE('',#42239,#41726,#6294,.T.);
#55600=EDGE_CURVE('',#42210,#42215,#6295,.T.);
#55601=EDGE_CURVE('',#42233,#42232,#6296,.T.);
#55602=EDGE_CURVE('',#42242,#42243,#6297,.T.);
#55603=EDGE_CURVE('',#42213,#42214,#6298,.T.);
#55604=EDGE_CURVE('',#42222,#42221,#6299,.T.);
#55605=EDGE_CURVE('',#41805,#42240,#6300,.T.);
#55606=EDGE_CURVE('',#42226,#42230,#6301,.T.);
#55607=EDGE_CURVE('',#42234,#42227,#6302,.T.);
#55608=EDGE_CURVE('',#42234,#42235,#24188,.T.);
#55609=EDGE_CURVE('',#42216,#42219,#6303,.T.);
#55610=EDGE_CURVE('',#42223,#42217,#6304,.T.);
#55611=EDGE_CURVE('',#42223,#42225,#24189,.T.);
#55612=EDGE_CURVE('',#42215,#42211,#6305,.T.);
#55613=EDGE_CURVE('',#41980,#42244,#24190,.T.);
#55614=EDGE_CURVE('',#42244,#41989,#24191,.T.);
#55615=EDGE_CURVE('',#42003,#41991,#34556,.T.);
#55616=EDGE_CURVE('',#42037,#41990,#34557,.T.);
#55617=EDGE_CURVE('',#42004,#41994,#34558,.T.);
#55618=EDGE_CURVE('',#41992,#42244,#34559,.T.);
#55619=EDGE_CURVE('',#41993,#41998,#34560,.T.);
#55620=EDGE_CURVE('',#41995,#41992,#34561,.T.);
#55621=EDGE_CURVE('',#42005,#41993,#34562,.T.);
#55622=EDGE_CURVE('',#41995,#42244,#34563,.T.);
#55623=EDGE_CURVE('',#42005,#41998,#34564,.T.);
#55624=EDGE_CURVE('',#41996,#41980,#2036,.T.);
#55625=EDGE_CURVE('',#41979,#41997,#2037,.T.);
#57945=ORIENTED_EDGE('',*,*,#43752,.T.);
#57946=ORIENTED_EDGE('',*,*,#43753,.T.);
#57947=ORIENTED_EDGE('',*,*,#43754,.T.);
#57948=ORIENTED_EDGE('',*,*,#43753,.F.);
#57949=ORIENTED_EDGE('',*,*,#43754,.F.);
#57950=ORIENTED_EDGE('',*,*,#43755,.F.);
#57951=ORIENTED_EDGE('',*,*,#43756,.T.);
#57952=ORIENTED_EDGE('',*,*,#43752,.F.);
#57953=ORIENTED_EDGE('',*,*,#43756,.F.);
#57954=ORIENTED_EDGE('',*,*,#43757,.T.);
#57955=ORIENTED_EDGE('',*,*,#43755,.T.);
#57956=ORIENTED_EDGE('',*,*,#43758,.F.);
#57957=ORIENTED_EDGE('',*,*,#43759,.T.);
#57958=ORIENTED_EDGE('',*,*,#43757,.F.);
#57959=ORIENTED_EDGE('',*,*,#43759,.F.);
#57960=ORIENTED_EDGE('',*,*,#43758,.T.);
#57961=ORIENTED_EDGE('',*,*,#43760,.F.);
#57962=ORIENTED_EDGE('',*,*,#43761,.T.);
#57963=ORIENTED_EDGE('',*,*,#43762,.F.);
#57964=ORIENTED_EDGE('',*,*,#43761,.F.);
#57965=ORIENTED_EDGE('',*,*,#43762,.T.);
#57966=ORIENTED_EDGE('',*,*,#43763,.T.);
#57967=ORIENTED_EDGE('',*,*,#43764,.T.);
#57968=ORIENTED_EDGE('',*,*,#43760,.T.);
#57969=ORIENTED_EDGE('',*,*,#43764,.F.);
#57970=ORIENTED_EDGE('',*,*,#43765,.F.);
#57971=ORIENTED_EDGE('',*,*,#43763,.F.);
#57972=ORIENTED_EDGE('',*,*,#43766,.T.);
#57973=ORIENTED_EDGE('',*,*,#43767,.T.);
#57974=ORIENTED_EDGE('',*,*,#43765,.T.);
#57975=ORIENTED_EDGE('',*,*,#43767,.F.);
#57976=ORIENTED_EDGE('',*,*,#43766,.F.);
#57977=ORIENTED_EDGE('',*,*,#43768,.T.);
#57978=ORIENTED_EDGE('',*,*,#43769,.T.);
#57979=ORIENTED_EDGE('',*,*,#43770,.T.);
#57980=ORIENTED_EDGE('',*,*,#43771,.F.);
#57981=ORIENTED_EDGE('',*,*,#43772,.F.);
#57982=ORIENTED_EDGE('',*,*,#43773,.F.);
#57983=ORIENTED_EDGE('',*,*,#43774,.F.);
#57984=ORIENTED_EDGE('',*,*,#43775,.T.);
#57985=ORIENTED_EDGE('',*,*,#43776,.T.);
#57986=ORIENTED_EDGE('',*,*,#43777,.T.);
#57987=ORIENTED_EDGE('',*,*,#43778,.F.);
#57988=ORIENTED_EDGE('',*,*,#43779,.F.);
#57989=ORIENTED_EDGE('',*,*,#43774,.T.);
#57990=ORIENTED_EDGE('',*,*,#43780,.T.);
#57991=ORIENTED_EDGE('',*,*,#43781,.T.);
#57992=ORIENTED_EDGE('',*,*,#43780,.F.);
#57993=ORIENTED_EDGE('',*,*,#43778,.T.);
#57994=ORIENTED_EDGE('',*,*,#43782,.T.);
#57995=ORIENTED_EDGE('',*,*,#43783,.T.);
#57996=ORIENTED_EDGE('',*,*,#43784,.T.);
#57997=ORIENTED_EDGE('',*,*,#43785,.T.);
#57998=ORIENTED_EDGE('',*,*,#43786,.T.);
#57999=ORIENTED_EDGE('',*,*,#43787,.F.);
#58000=ORIENTED_EDGE('',*,*,#43788,.F.);
#58001=ORIENTED_EDGE('',*,*,#43789,.F.);
#58002=ORIENTED_EDGE('',*,*,#43790,.F.);
#58003=ORIENTED_EDGE('',*,*,#43791,.F.);
#58004=ORIENTED_EDGE('',*,*,#43792,.F.);
#58005=ORIENTED_EDGE('',*,*,#43793,.F.);
#58006=ORIENTED_EDGE('',*,*,#43794,.F.);
#58007=ORIENTED_EDGE('',*,*,#43795,.F.);
#58008=ORIENTED_EDGE('',*,*,#43796,.F.);
#58009=ORIENTED_EDGE('',*,*,#43797,.F.);
#58010=ORIENTED_EDGE('',*,*,#43777,.F.);
#58011=ORIENTED_EDGE('',*,*,#43798,.F.);
#58012=ORIENTED_EDGE('',*,*,#43784,.F.);
#58013=ORIENTED_EDGE('',*,*,#43799,.F.);
#58014=ORIENTED_EDGE('',*,*,#43800,.F.);
#58015=ORIENTED_EDGE('',*,*,#43801,.F.);
#58016=ORIENTED_EDGE('',*,*,#43802,.F.);
#58017=ORIENTED_EDGE('',*,*,#43803,.F.);
#58018=ORIENTED_EDGE('',*,*,#43804,.F.);
#58019=ORIENTED_EDGE('',*,*,#43805,.F.);
#58020=ORIENTED_EDGE('',*,*,#43787,.T.);
#58021=ORIENTED_EDGE('',*,*,#43806,.T.);
#58022=ORIENTED_EDGE('',*,*,#43807,.T.);
#58023=ORIENTED_EDGE('',*,*,#43808,.T.);
#58024=ORIENTED_EDGE('',*,*,#43809,.T.);
#58025=ORIENTED_EDGE('',*,*,#43810,.T.);
#58026=ORIENTED_EDGE('',*,*,#43811,.F.);
#58027=ORIENTED_EDGE('',*,*,#43786,.F.);
#58028=ORIENTED_EDGE('',*,*,#43812,.F.);
#58029=ORIENTED_EDGE('',*,*,#43808,.F.);
#58030=ORIENTED_EDGE('',*,*,#43813,.F.);
#58031=ORIENTED_EDGE('',*,*,#43814,.F.);
#58032=ORIENTED_EDGE('',*,*,#43811,.T.);
#58033=ORIENTED_EDGE('',*,*,#43815,.T.);
#58034=ORIENTED_EDGE('',*,*,#43816,.T.);
#58035=ORIENTED_EDGE('',*,*,#43817,.F.);
#58036=ORIENTED_EDGE('',*,*,#43818,.F.);
#58037=ORIENTED_EDGE('',*,*,#43819,.F.);
#58038=ORIENTED_EDGE('',*,*,#43820,.F.);
#58039=ORIENTED_EDGE('',*,*,#43821,.F.);
#58040=ORIENTED_EDGE('',*,*,#43822,.F.);
#58041=ORIENTED_EDGE('',*,*,#43823,.F.);
#58042=ORIENTED_EDGE('',*,*,#43824,.F.);
#58043=ORIENTED_EDGE('',*,*,#43825,.F.);
#58044=ORIENTED_EDGE('',*,*,#43826,.F.);
#58045=ORIENTED_EDGE('',*,*,#43827,.F.);
#58046=ORIENTED_EDGE('',*,*,#43828,.F.);
#58047=ORIENTED_EDGE('',*,*,#43829,.F.);
#58048=ORIENTED_EDGE('',*,*,#43830,.F.);
#58049=ORIENTED_EDGE('',*,*,#43810,.F.);
#58050=ORIENTED_EDGE('',*,*,#43831,.F.);
#58051=ORIENTED_EDGE('',*,*,#43768,.F.);
#58052=ORIENTED_EDGE('',*,*,#43832,.F.);
#58053=ORIENTED_EDGE('',*,*,#43833,.F.);
#58054=ORIENTED_EDGE('',*,*,#43834,.F.);
#58055=ORIENTED_EDGE('',*,*,#43835,.T.);
#58056=ORIENTED_EDGE('',*,*,#43836,.T.);
#58057=ORIENTED_EDGE('',*,*,#43837,.T.);
#58058=ORIENTED_EDGE('',*,*,#43838,.F.);
#58059=ORIENTED_EDGE('',*,*,#43839,.T.);
#58060=ORIENTED_EDGE('',*,*,#43834,.T.);
#58061=ORIENTED_EDGE('',*,*,#43840,.T.);
#58062=ORIENTED_EDGE('',*,*,#43841,.T.);
#58063=ORIENTED_EDGE('',*,*,#43842,.F.);
#58064=ORIENTED_EDGE('',*,*,#43843,.T.);
#58065=ORIENTED_EDGE('',*,*,#43844,.F.);
#58066=ORIENTED_EDGE('',*,*,#43845,.T.);
#58067=ORIENTED_EDGE('',*,*,#43846,.T.);
#58068=ORIENTED_EDGE('',*,*,#43847,.F.);
#58069=ORIENTED_EDGE('',*,*,#43848,.F.);
#58070=ORIENTED_EDGE('',*,*,#43849,.T.);
#58071=ORIENTED_EDGE('',*,*,#43850,.T.);
#58072=ORIENTED_EDGE('',*,*,#43850,.F.);
#58073=ORIENTED_EDGE('',*,*,#43851,.T.);
#58074=ORIENTED_EDGE('',*,*,#43852,.T.);
#58075=ORIENTED_EDGE('',*,*,#43853,.T.);
#58076=ORIENTED_EDGE('',*,*,#43845,.F.);
#58077=ORIENTED_EDGE('',*,*,#43852,.F.);
#58078=ORIENTED_EDGE('',*,*,#43854,.T.);
#58079=ORIENTED_EDGE('',*,*,#43855,.T.);
#58080=ORIENTED_EDGE('',*,*,#43856,.T.);
#58081=ORIENTED_EDGE('',*,*,#43855,.F.);
#58082=ORIENTED_EDGE('',*,*,#43857,.T.);
#58083=ORIENTED_EDGE('',*,*,#43858,.F.);
#58084=ORIENTED_EDGE('',*,*,#43859,.T.);
#58085=ORIENTED_EDGE('',*,*,#43860,.F.);
#58086=ORIENTED_EDGE('',*,*,#43861,.T.);
#58087=ORIENTED_EDGE('',*,*,#43858,.T.);
#58088=ORIENTED_EDGE('',*,*,#43862,.T.);
#58089=ORIENTED_EDGE('',*,*,#43863,.T.);
#58090=ORIENTED_EDGE('',*,*,#43864,.F.);
#58091=ORIENTED_EDGE('',*,*,#43865,.T.);
#58092=ORIENTED_EDGE('',*,*,#43866,.F.);
#58093=ORIENTED_EDGE('',*,*,#43867,.T.);
#58094=ORIENTED_EDGE('',*,*,#43868,.T.);
#58095=ORIENTED_EDGE('',*,*,#43869,.F.);
#58096=ORIENTED_EDGE('',*,*,#43870,.F.);
#58097=ORIENTED_EDGE('',*,*,#43871,.T.);
#58098=ORIENTED_EDGE('',*,*,#43867,.F.);
#58099=ORIENTED_EDGE('',*,*,#43872,.T.);
#58100=ORIENTED_EDGE('',*,*,#43873,.T.);
#58101=ORIENTED_EDGE('',*,*,#43874,.T.);
#58102=ORIENTED_EDGE('',*,*,#43873,.F.);
#58103=ORIENTED_EDGE('',*,*,#43875,.T.);
#58104=ORIENTED_EDGE('',*,*,#43876,.T.);
#58105=ORIENTED_EDGE('',*,*,#43877,.T.);
#58106=ORIENTED_EDGE('',*,*,#43876,.F.);
#58107=ORIENTED_EDGE('',*,*,#43878,.T.);
#58108=ORIENTED_EDGE('',*,*,#43879,.F.);
#58109=ORIENTED_EDGE('',*,*,#43880,.T.);
#58110=ORIENTED_EDGE('',*,*,#43881,.F.);
#58111=ORIENTED_EDGE('',*,*,#43882,.T.);
#58112=ORIENTED_EDGE('',*,*,#43879,.T.);
#58113=ORIENTED_EDGE('',*,*,#43883,.T.);
#58114=ORIENTED_EDGE('',*,*,#43884,.T.);
#58115=ORIENTED_EDGE('',*,*,#43885,.F.);
#58116=ORIENTED_EDGE('',*,*,#43886,.T.);
#58117=ORIENTED_EDGE('',*,*,#43887,.F.);
#58118=ORIENTED_EDGE('',*,*,#43888,.T.);
#58119=ORIENTED_EDGE('',*,*,#43889,.T.);
#58120=ORIENTED_EDGE('',*,*,#43890,.F.);
#58121=ORIENTED_EDGE('',*,*,#43891,.T.);
#58122=ORIENTED_EDGE('',*,*,#43888,.F.);
#58123=ORIENTED_EDGE('',*,*,#43892,.T.);
#58124=ORIENTED_EDGE('',*,*,#43893,.T.);
#58125=ORIENTED_EDGE('',*,*,#43894,.T.);
#58126=ORIENTED_EDGE('',*,*,#43893,.F.);
#58127=ORIENTED_EDGE('',*,*,#43895,.T.);
#58128=ORIENTED_EDGE('',*,*,#43779,.T.);
#58129=ORIENTED_EDGE('',*,*,#43896,.T.);
#58130=ORIENTED_EDGE('',*,*,#43897,.T.);
#58131=ORIENTED_EDGE('',*,*,#43898,.T.);
#58132=ORIENTED_EDGE('',*,*,#43899,.T.);
#58133=ORIENTED_EDGE('',*,*,#43900,.F.);
#58134=ORIENTED_EDGE('',*,*,#43901,.T.);
#58135=ORIENTED_EDGE('',*,*,#43902,.F.);
#58136=ORIENTED_EDGE('',*,*,#43903,.T.);
#58137=ORIENTED_EDGE('',*,*,#43904,.F.);
#58138=ORIENTED_EDGE('',*,*,#43905,.F.);
#58139=ORIENTED_EDGE('',*,*,#43906,.T.);
#58140=ORIENTED_EDGE('',*,*,#43907,.T.);
#58141=ORIENTED_EDGE('',*,*,#43908,.T.);
#58142=ORIENTED_EDGE('',*,*,#43909,.F.);
#58143=ORIENTED_EDGE('',*,*,#43910,.T.);
#58144=ORIENTED_EDGE('',*,*,#43905,.T.);
#58145=ORIENTED_EDGE('',*,*,#43911,.T.);
#58146=ORIENTED_EDGE('',*,*,#43912,.F.);
#58147=ORIENTED_EDGE('',*,*,#43913,.T.);
#58148=ORIENTED_EDGE('',*,*,#43909,.T.);
#58149=ORIENTED_EDGE('',*,*,#43914,.T.);
#58150=ORIENTED_EDGE('',*,*,#43915,.F.);
#58151=ORIENTED_EDGE('',*,*,#43916,.T.);
#58152=ORIENTED_EDGE('',*,*,#43912,.T.);
#58153=ORIENTED_EDGE('',*,*,#43917,.T.);
#58154=ORIENTED_EDGE('',*,*,#43915,.T.);
#58155=ORIENTED_EDGE('',*,*,#43918,.T.);
#58156=ORIENTED_EDGE('',*,*,#43919,.T.);
#58157=ORIENTED_EDGE('',*,*,#43920,.T.);
#58158=ORIENTED_EDGE('',*,*,#43921,.T.);
#58159=ORIENTED_EDGE('',*,*,#43922,.F.);
#58160=ORIENTED_EDGE('',*,*,#43923,.T.);
#58161=ORIENTED_EDGE('',*,*,#43924,.F.);
#58162=ORIENTED_EDGE('',*,*,#43925,.F.);
#58163=ORIENTED_EDGE('',*,*,#43926,.T.);
#58164=ORIENTED_EDGE('',*,*,#43927,.T.);
#58165=ORIENTED_EDGE('',*,*,#43928,.T.);
#58166=ORIENTED_EDGE('',*,*,#43929,.F.);
#58167=ORIENTED_EDGE('',*,*,#43930,.T.);
#58168=ORIENTED_EDGE('',*,*,#43925,.T.);
#58169=ORIENTED_EDGE('',*,*,#43931,.T.);
#58170=ORIENTED_EDGE('',*,*,#43932,.F.);
#58171=ORIENTED_EDGE('',*,*,#43933,.T.);
#58172=ORIENTED_EDGE('',*,*,#43929,.T.);
#58173=ORIENTED_EDGE('',*,*,#43934,.T.);
#58174=ORIENTED_EDGE('',*,*,#43935,.F.);
#58175=ORIENTED_EDGE('',*,*,#43936,.T.);
#58176=ORIENTED_EDGE('',*,*,#43932,.T.);
#58177=ORIENTED_EDGE('',*,*,#43937,.T.);
#58178=ORIENTED_EDGE('',*,*,#43938,.F.);
#58179=ORIENTED_EDGE('',*,*,#43939,.T.);
#58180=ORIENTED_EDGE('',*,*,#43935,.T.);
#58181=ORIENTED_EDGE('',*,*,#43940,.T.);
#58182=ORIENTED_EDGE('',*,*,#43941,.T.);
#58183=ORIENTED_EDGE('',*,*,#43942,.F.);
#58184=ORIENTED_EDGE('',*,*,#43943,.T.);
#58185=ORIENTED_EDGE('',*,*,#43944,.F.);
#58186=ORIENTED_EDGE('',*,*,#43945,.F.);
#58187=ORIENTED_EDGE('',*,*,#43946,.T.);
#58188=ORIENTED_EDGE('',*,*,#43947,.T.);
#58189=ORIENTED_EDGE('',*,*,#43948,.T.);
#58190=ORIENTED_EDGE('',*,*,#43949,.F.);
#58191=ORIENTED_EDGE('',*,*,#43950,.T.);
#58192=ORIENTED_EDGE('',*,*,#43945,.T.);
#58193=ORIENTED_EDGE('',*,*,#43951,.T.);
#58194=ORIENTED_EDGE('',*,*,#43952,.F.);
#58195=ORIENTED_EDGE('',*,*,#43953,.T.);
#58196=ORIENTED_EDGE('',*,*,#43949,.T.);
#58197=ORIENTED_EDGE('',*,*,#43954,.T.);
#58198=ORIENTED_EDGE('',*,*,#43955,.F.);
#58199=ORIENTED_EDGE('',*,*,#43956,.T.);
#58200=ORIENTED_EDGE('',*,*,#43952,.T.);
#58201=ORIENTED_EDGE('',*,*,#43957,.T.);
#58202=ORIENTED_EDGE('',*,*,#43958,.F.);
#58203=ORIENTED_EDGE('',*,*,#43959,.T.);
#58204=ORIENTED_EDGE('',*,*,#43955,.T.);
#58205=ORIENTED_EDGE('',*,*,#43960,.T.);
#58206=ORIENTED_EDGE('',*,*,#43961,.F.);
#58207=ORIENTED_EDGE('',*,*,#43773,.T.);
#58208=ORIENTED_EDGE('',*,*,#43962,.T.);
#58209=ORIENTED_EDGE('',*,*,#43963,.T.);
#58210=ORIENTED_EDGE('',*,*,#43962,.F.);
#58211=ORIENTED_EDGE('',*,*,#43772,.T.);
#58212=ORIENTED_EDGE('',*,*,#43964,.T.);
#58213=ORIENTED_EDGE('',*,*,#43965,.T.);
#58214=ORIENTED_EDGE('',*,*,#43964,.F.);
#58215=ORIENTED_EDGE('',*,*,#43771,.T.);
#58216=ORIENTED_EDGE('',*,*,#43966,.T.);
#58217=ORIENTED_EDGE('',*,*,#43967,.T.);
#58218=ORIENTED_EDGE('',*,*,#43968,.T.);
#58219=ORIENTED_EDGE('',*,*,#43969,.T.);
#58220=ORIENTED_EDGE('',*,*,#43970,.T.);
#58221=ORIENTED_EDGE('',*,*,#43971,.F.);
#58222=ORIENTED_EDGE('',*,*,#43972,.F.);
#58223=ORIENTED_EDGE('',*,*,#43973,.F.);
#58224=ORIENTED_EDGE('',*,*,#43974,.T.);
#58225=ORIENTED_EDGE('',*,*,#43968,.F.);
#58226=ORIENTED_EDGE('',*,*,#43975,.F.);
#58227=ORIENTED_EDGE('',*,*,#43976,.F.);
#58228=ORIENTED_EDGE('',*,*,#43977,.F.);
#58229=ORIENTED_EDGE('',*,*,#43978,.F.);
#58230=ORIENTED_EDGE('',*,*,#43979,.F.);
#58231=ORIENTED_EDGE('',*,*,#43980,.F.);
#58232=ORIENTED_EDGE('',*,*,#43981,.F.);
#58233=ORIENTED_EDGE('',*,*,#43982,.F.);
#58234=ORIENTED_EDGE('',*,*,#43983,.F.);
#58235=ORIENTED_EDGE('',*,*,#43984,.F.);
#58236=ORIENTED_EDGE('',*,*,#43985,.F.);
#58237=ORIENTED_EDGE('',*,*,#43986,.F.);
#58238=ORIENTED_EDGE('',*,*,#43987,.F.);
#58239=ORIENTED_EDGE('',*,*,#43988,.F.);
#58240=ORIENTED_EDGE('',*,*,#43989,.F.);
#58241=ORIENTED_EDGE('',*,*,#43990,.F.);
#58242=ORIENTED_EDGE('',*,*,#43991,.F.);
#58243=ORIENTED_EDGE('',*,*,#43992,.F.);
#58244=ORIENTED_EDGE('',*,*,#43993,.F.);
#58245=ORIENTED_EDGE('',*,*,#43994,.F.);
#58246=ORIENTED_EDGE('',*,*,#43995,.F.);
#58247=ORIENTED_EDGE('',*,*,#43996,.F.);
#58248=ORIENTED_EDGE('',*,*,#43997,.F.);
#58249=ORIENTED_EDGE('',*,*,#43998,.F.);
#58250=ORIENTED_EDGE('',*,*,#43999,.F.);
#58251=ORIENTED_EDGE('',*,*,#44000,.F.);
#58252=ORIENTED_EDGE('',*,*,#44001,.F.);
#58253=ORIENTED_EDGE('',*,*,#44002,.F.);
#58254=ORIENTED_EDGE('',*,*,#44003,.F.);
#58255=ORIENTED_EDGE('',*,*,#44004,.F.);
#58256=ORIENTED_EDGE('',*,*,#44005,.F.);
#58257=ORIENTED_EDGE('',*,*,#44006,.F.);
#58258=ORIENTED_EDGE('',*,*,#44007,.F.);
#58259=ORIENTED_EDGE('',*,*,#44008,.F.);
#58260=ORIENTED_EDGE('',*,*,#44009,.F.);
#58261=ORIENTED_EDGE('',*,*,#43770,.F.);
#58262=ORIENTED_EDGE('',*,*,#44010,.F.);
#58263=ORIENTED_EDGE('',*,*,#44011,.T.);
#58264=ORIENTED_EDGE('',*,*,#44012,.T.);
#58265=ORIENTED_EDGE('',*,*,#43973,.T.);
#58266=ORIENTED_EDGE('',*,*,#44010,.T.);
#58267=ORIENTED_EDGE('',*,*,#43972,.T.);
#58268=ORIENTED_EDGE('',*,*,#44013,.T.);
#58269=ORIENTED_EDGE('',*,*,#44014,.T.);
#58270=ORIENTED_EDGE('',*,*,#44013,.F.);
#58271=ORIENTED_EDGE('',*,*,#43971,.T.);
#58272=ORIENTED_EDGE('',*,*,#44015,.T.);
#58273=ORIENTED_EDGE('',*,*,#44016,.T.);
#58274=ORIENTED_EDGE('',*,*,#44017,.T.);
#58275=ORIENTED_EDGE('',*,*,#44018,.T.);
#58276=ORIENTED_EDGE('',*,*,#44019,.T.);
#58277=ORIENTED_EDGE('',*,*,#44020,.F.);
#58278=ORIENTED_EDGE('',*,*,#44021,.F.);
#58279=ORIENTED_EDGE('',*,*,#44022,.F.);
#58280=ORIENTED_EDGE('',*,*,#44023,.F.);
#58281=ORIENTED_EDGE('',*,*,#44024,.F.);
#58282=ORIENTED_EDGE('',*,*,#44025,.F.);
#58283=ORIENTED_EDGE('',*,*,#44026,.F.);
#58284=ORIENTED_EDGE('',*,*,#44027,.F.);
#58285=ORIENTED_EDGE('',*,*,#44028,.F.);
#58286=ORIENTED_EDGE('',*,*,#44029,.F.);
#58287=ORIENTED_EDGE('',*,*,#44030,.F.);
#58288=ORIENTED_EDGE('',*,*,#43970,.F.);
#58289=ORIENTED_EDGE('',*,*,#44031,.F.);
#58290=ORIENTED_EDGE('',*,*,#44017,.F.);
#58291=ORIENTED_EDGE('',*,*,#44032,.F.);
#58292=ORIENTED_EDGE('',*,*,#44033,.F.);
#58293=ORIENTED_EDGE('',*,*,#44034,.F.);
#58294=ORIENTED_EDGE('',*,*,#44035,.F.);
#58295=ORIENTED_EDGE('',*,*,#44036,.F.);
#58296=ORIENTED_EDGE('',*,*,#44037,.F.);
#58297=ORIENTED_EDGE('',*,*,#44038,.F.);
#58298=ORIENTED_EDGE('',*,*,#44020,.T.);
#58299=ORIENTED_EDGE('',*,*,#44039,.T.);
#58300=ORIENTED_EDGE('',*,*,#44040,.T.);
#58301=ORIENTED_EDGE('',*,*,#44041,.T.);
#58302=ORIENTED_EDGE('',*,*,#44042,.T.);
#58303=ORIENTED_EDGE('',*,*,#44043,.T.);
#58304=ORIENTED_EDGE('',*,*,#44044,.F.);
#58305=ORIENTED_EDGE('',*,*,#44019,.F.);
#58306=ORIENTED_EDGE('',*,*,#44045,.F.);
#58307=ORIENTED_EDGE('',*,*,#44041,.F.);
#58308=ORIENTED_EDGE('',*,*,#44046,.F.);
#58309=ORIENTED_EDGE('',*,*,#44047,.F.);
#58310=ORIENTED_EDGE('',*,*,#44044,.T.);
#58311=ORIENTED_EDGE('',*,*,#44048,.T.);
#58312=ORIENTED_EDGE('',*,*,#44049,.T.);
#58313=ORIENTED_EDGE('',*,*,#44050,.F.);
#58314=ORIENTED_EDGE('',*,*,#44051,.F.);
#58315=ORIENTED_EDGE('',*,*,#44052,.F.);
#58316=ORIENTED_EDGE('',*,*,#44053,.F.);
#58317=ORIENTED_EDGE('',*,*,#44054,.F.);
#58318=ORIENTED_EDGE('',*,*,#44055,.F.);
#58319=ORIENTED_EDGE('',*,*,#44056,.F.);
#58320=ORIENTED_EDGE('',*,*,#44043,.F.);
#58321=ORIENTED_EDGE('',*,*,#44057,.F.);
#58322=ORIENTED_EDGE('',*,*,#43897,.F.);
#58323=ORIENTED_EDGE('',*,*,#44058,.F.);
#58324=ORIENTED_EDGE('',*,*,#44059,.F.);
#58325=ORIENTED_EDGE('',*,*,#44060,.F.);
#58326=ORIENTED_EDGE('',*,*,#44061,.F.);
#58327=ORIENTED_EDGE('',*,*,#44062,.F.);
#58328=ORIENTED_EDGE('',*,*,#44063,.F.);
#58329=ORIENTED_EDGE('',*,*,#43966,.F.);
#58330=ORIENTED_EDGE('',*,*,#44009,.T.);
#58331=ORIENTED_EDGE('',*,*,#44064,.T.);
#58332=ORIENTED_EDGE('',*,*,#44065,.T.);
#58333=ORIENTED_EDGE('',*,*,#44064,.F.);
#58334=ORIENTED_EDGE('',*,*,#44008,.T.);
#58335=ORIENTED_EDGE('',*,*,#44066,.T.);
#58336=ORIENTED_EDGE('',*,*,#44067,.T.);
#58337=ORIENTED_EDGE('',*,*,#44068,.T.);
#58338=ORIENTED_EDGE('',*,*,#44069,.F.);
#58339=ORIENTED_EDGE('',*,*,#44007,.T.);
#58340=ORIENTED_EDGE('',*,*,#44070,.F.);
#58341=ORIENTED_EDGE('',*,*,#44071,.F.);
#58342=ORIENTED_EDGE('',*,*,#44072,.T.);
#58343=ORIENTED_EDGE('',*,*,#44073,.T.);
#58344=ORIENTED_EDGE('',*,*,#44006,.T.);
#58345=ORIENTED_EDGE('',*,*,#44074,.F.);
#58346=ORIENTED_EDGE('',*,*,#44075,.T.);
#58347=ORIENTED_EDGE('',*,*,#44071,.T.);
#58348=ORIENTED_EDGE('',*,*,#44005,.T.);
#58349=ORIENTED_EDGE('',*,*,#44076,.F.);
#58350=ORIENTED_EDGE('',*,*,#44077,.T.);
#58351=ORIENTED_EDGE('',*,*,#44074,.T.);
#58352=ORIENTED_EDGE('',*,*,#44004,.T.);
#58353=ORIENTED_EDGE('',*,*,#44078,.F.);
#58354=ORIENTED_EDGE('',*,*,#44079,.T.);
#58355=ORIENTED_EDGE('',*,*,#44076,.T.);
#58356=ORIENTED_EDGE('',*,*,#44003,.T.);
#58357=ORIENTED_EDGE('',*,*,#44080,.F.);
#58358=ORIENTED_EDGE('',*,*,#44081,.T.);
#58359=ORIENTED_EDGE('',*,*,#44078,.T.);
#58360=ORIENTED_EDGE('',*,*,#44002,.T.);
#58361=ORIENTED_EDGE('',*,*,#44082,.T.);
#58362=ORIENTED_EDGE('',*,*,#44083,.F.);
#58363=ORIENTED_EDGE('',*,*,#44001,.T.);
#58364=ORIENTED_EDGE('',*,*,#44084,.F.);
#58365=ORIENTED_EDGE('',*,*,#44085,.F.);
#58366=ORIENTED_EDGE('',*,*,#44000,.T.);
#58367=ORIENTED_EDGE('',*,*,#44086,.T.);
#58368=ORIENTED_EDGE('',*,*,#44087,.T.);
#58369=ORIENTED_EDGE('',*,*,#44086,.F.);
#58370=ORIENTED_EDGE('',*,*,#43999,.T.);
#58371=ORIENTED_EDGE('',*,*,#44088,.T.);
#58372=ORIENTED_EDGE('',*,*,#44089,.T.);
#58373=ORIENTED_EDGE('',*,*,#44088,.F.);
#58374=ORIENTED_EDGE('',*,*,#43998,.T.);
#58375=ORIENTED_EDGE('',*,*,#44090,.T.);
#58376=ORIENTED_EDGE('',*,*,#44091,.T.);
#58377=ORIENTED_EDGE('',*,*,#44090,.F.);
#58378=ORIENTED_EDGE('',*,*,#43997,.T.);
#58379=ORIENTED_EDGE('',*,*,#44092,.F.);
#58380=ORIENTED_EDGE('',*,*,#44093,.T.);
#58381=ORIENTED_EDGE('',*,*,#44094,.F.);
#58382=ORIENTED_EDGE('',*,*,#44095,.T.);
#58383=ORIENTED_EDGE('',*,*,#44092,.T.);
#58384=ORIENTED_EDGE('',*,*,#43996,.T.);
#58385=ORIENTED_EDGE('',*,*,#44096,.T.);
#58386=ORIENTED_EDGE('',*,*,#44097,.F.);
#58387=ORIENTED_EDGE('',*,*,#43995,.T.);
#58388=ORIENTED_EDGE('',*,*,#44098,.F.);
#58389=ORIENTED_EDGE('',*,*,#44099,.F.);
#58390=ORIENTED_EDGE('',*,*,#43994,.T.);
#58391=ORIENTED_EDGE('',*,*,#44100,.T.);
#58392=ORIENTED_EDGE('',*,*,#44101,.T.);
#58393=ORIENTED_EDGE('',*,*,#44100,.F.);
#58394=ORIENTED_EDGE('',*,*,#43993,.T.);
#58395=ORIENTED_EDGE('',*,*,#44102,.T.);
#58396=ORIENTED_EDGE('',*,*,#44103,.T.);
#58397=ORIENTED_EDGE('',*,*,#44102,.F.);
#58398=ORIENTED_EDGE('',*,*,#43992,.T.);
#58399=ORIENTED_EDGE('',*,*,#44104,.T.);
#58400=ORIENTED_EDGE('',*,*,#44105,.T.);
#58401=ORIENTED_EDGE('',*,*,#44104,.F.);
#58402=ORIENTED_EDGE('',*,*,#43991,.T.);
#58403=ORIENTED_EDGE('',*,*,#44106,.F.);
#58404=ORIENTED_EDGE('',*,*,#44107,.T.);
#58405=ORIENTED_EDGE('',*,*,#44108,.F.);
#58406=ORIENTED_EDGE('',*,*,#44109,.T.);
#58407=ORIENTED_EDGE('',*,*,#44106,.T.);
#58408=ORIENTED_EDGE('',*,*,#43990,.T.);
#58409=ORIENTED_EDGE('',*,*,#44110,.T.);
#58410=ORIENTED_EDGE('',*,*,#44111,.F.);
#58411=ORIENTED_EDGE('',*,*,#43989,.T.);
#58412=ORIENTED_EDGE('',*,*,#44112,.F.);
#58413=ORIENTED_EDGE('',*,*,#44113,.F.);
#58414=ORIENTED_EDGE('',*,*,#43988,.T.);
#58415=ORIENTED_EDGE('',*,*,#44114,.T.);
#58416=ORIENTED_EDGE('',*,*,#44115,.T.);
#58417=ORIENTED_EDGE('',*,*,#44114,.F.);
#58418=ORIENTED_EDGE('',*,*,#43987,.T.);
#58419=ORIENTED_EDGE('',*,*,#44116,.T.);
#58420=ORIENTED_EDGE('',*,*,#44117,.T.);
#58421=ORIENTED_EDGE('',*,*,#44116,.F.);
#58422=ORIENTED_EDGE('',*,*,#43986,.T.);
#58423=ORIENTED_EDGE('',*,*,#44118,.T.);
#58424=ORIENTED_EDGE('',*,*,#44119,.T.);
#58425=ORIENTED_EDGE('',*,*,#44118,.F.);
#58426=ORIENTED_EDGE('',*,*,#43985,.T.);
#58427=ORIENTED_EDGE('',*,*,#44120,.F.);
#58428=ORIENTED_EDGE('',*,*,#44121,.T.);
#58429=ORIENTED_EDGE('',*,*,#44122,.F.);
#58430=ORIENTED_EDGE('',*,*,#44123,.T.);
#58431=ORIENTED_EDGE('',*,*,#44120,.T.);
#58432=ORIENTED_EDGE('',*,*,#43984,.T.);
#58433=ORIENTED_EDGE('',*,*,#44124,.T.);
#58434=ORIENTED_EDGE('',*,*,#44125,.F.);
#58435=ORIENTED_EDGE('',*,*,#43983,.T.);
#58436=ORIENTED_EDGE('',*,*,#44126,.F.);
#58437=ORIENTED_EDGE('',*,*,#44127,.F.);
#58438=ORIENTED_EDGE('',*,*,#44128,.T.);
#58439=ORIENTED_EDGE('',*,*,#44129,.T.);
#58440=ORIENTED_EDGE('',*,*,#43982,.T.);
#58441=ORIENTED_EDGE('',*,*,#44130,.F.);
#58442=ORIENTED_EDGE('',*,*,#44131,.T.);
#58443=ORIENTED_EDGE('',*,*,#44127,.T.);
#58444=ORIENTED_EDGE('',*,*,#43981,.T.);
#58445=ORIENTED_EDGE('',*,*,#44132,.F.);
#58446=ORIENTED_EDGE('',*,*,#44133,.T.);
#58447=ORIENTED_EDGE('',*,*,#44130,.T.);
#58448=ORIENTED_EDGE('',*,*,#43980,.T.);
#58449=ORIENTED_EDGE('',*,*,#44134,.F.);
#58450=ORIENTED_EDGE('',*,*,#44135,.T.);
#58451=ORIENTED_EDGE('',*,*,#44132,.T.);
#58452=ORIENTED_EDGE('',*,*,#43979,.T.);
#58453=ORIENTED_EDGE('',*,*,#44136,.F.);
#58454=ORIENTED_EDGE('',*,*,#44137,.T.);
#58455=ORIENTED_EDGE('',*,*,#44134,.T.);
#58456=ORIENTED_EDGE('',*,*,#43978,.T.);
#58457=ORIENTED_EDGE('',*,*,#44138,.T.);
#58458=ORIENTED_EDGE('',*,*,#44139,.F.);
#58459=ORIENTED_EDGE('',*,*,#43977,.T.);
#58460=ORIENTED_EDGE('',*,*,#44140,.F.);
#58461=ORIENTED_EDGE('',*,*,#44141,.F.);
#58462=ORIENTED_EDGE('',*,*,#44142,.T.);
#58463=ORIENTED_EDGE('',*,*,#44143,.T.);
#58464=ORIENTED_EDGE('',*,*,#43976,.T.);
#58465=ORIENTED_EDGE('',*,*,#44012,.F.);
#58466=ORIENTED_EDGE('',*,*,#44144,.T.);
#58467=ORIENTED_EDGE('',*,*,#44141,.T.);
#58468=ORIENTED_EDGE('',*,*,#43975,.T.);
#58469=ORIENTED_EDGE('',*,*,#44145,.T.);
#58470=ORIENTED_EDGE('',*,*,#44146,.F.);
#58471=ORIENTED_EDGE('',*,*,#43788,.T.);
#58472=ORIENTED_EDGE('',*,*,#44147,.F.);
#58473=ORIENTED_EDGE('',*,*,#44148,.F.);
#58474=ORIENTED_EDGE('',*,*,#43804,.T.);
#58475=ORIENTED_EDGE('',*,*,#44149,.T.);
#58476=ORIENTED_EDGE('',*,*,#44150,.T.);
#58477=ORIENTED_EDGE('',*,*,#44149,.F.);
#58478=ORIENTED_EDGE('',*,*,#43803,.T.);
#58479=ORIENTED_EDGE('',*,*,#44151,.T.);
#58480=ORIENTED_EDGE('',*,*,#44152,.T.);
#58481=ORIENTED_EDGE('',*,*,#44151,.F.);
#58482=ORIENTED_EDGE('',*,*,#43802,.T.);
#58483=ORIENTED_EDGE('',*,*,#44153,.T.);
#58484=ORIENTED_EDGE('',*,*,#44154,.T.);
#58485=ORIENTED_EDGE('',*,*,#44153,.F.);
#58486=ORIENTED_EDGE('',*,*,#43801,.T.);
#58487=ORIENTED_EDGE('',*,*,#44155,.T.);
#58488=ORIENTED_EDGE('',*,*,#44156,.T.);
#58489=ORIENTED_EDGE('',*,*,#44155,.F.);
#58490=ORIENTED_EDGE('',*,*,#43800,.T.);
#58491=ORIENTED_EDGE('',*,*,#44157,.T.);
#58492=ORIENTED_EDGE('',*,*,#44158,.T.);
#58493=ORIENTED_EDGE('',*,*,#43799,.T.);
#58494=ORIENTED_EDGE('',*,*,#43805,.T.);
#58495=ORIENTED_EDGE('',*,*,#44159,.T.);
#58496=ORIENTED_EDGE('',*,*,#44160,.F.);
#58497=ORIENTED_EDGE('',*,*,#43782,.F.);
#58498=ORIENTED_EDGE('',*,*,#43797,.T.);
#58499=ORIENTED_EDGE('',*,*,#44161,.F.);
#58500=ORIENTED_EDGE('',*,*,#44162,.T.);
#58501=ORIENTED_EDGE('',*,*,#44163,.F.);
#58502=ORIENTED_EDGE('',*,*,#44164,.T.);
#58503=ORIENTED_EDGE('',*,*,#44161,.T.);
#58504=ORIENTED_EDGE('',*,*,#43796,.T.);
#58505=ORIENTED_EDGE('',*,*,#43795,.T.);
#58506=ORIENTED_EDGE('',*,*,#44165,.F.);
#58507=ORIENTED_EDGE('',*,*,#44166,.T.);
#58508=ORIENTED_EDGE('',*,*,#44167,.F.);
#58509=ORIENTED_EDGE('',*,*,#44168,.T.);
#58510=ORIENTED_EDGE('',*,*,#44165,.T.);
#58511=ORIENTED_EDGE('',*,*,#43794,.T.);
#58512=ORIENTED_EDGE('',*,*,#44169,.F.);
#58513=ORIENTED_EDGE('',*,*,#44170,.F.);
#58514=ORIENTED_EDGE('',*,*,#43793,.T.);
#58515=ORIENTED_EDGE('',*,*,#44171,.T.);
#58516=ORIENTED_EDGE('',*,*,#44172,.T.);
#58517=ORIENTED_EDGE('',*,*,#44171,.F.);
#58518=ORIENTED_EDGE('',*,*,#43792,.T.);
#58519=ORIENTED_EDGE('',*,*,#44173,.T.);
#58520=ORIENTED_EDGE('',*,*,#44174,.T.);
#58521=ORIENTED_EDGE('',*,*,#44173,.F.);
#58522=ORIENTED_EDGE('',*,*,#43791,.T.);
#58523=ORIENTED_EDGE('',*,*,#44175,.T.);
#58524=ORIENTED_EDGE('',*,*,#44176,.T.);
#58525=ORIENTED_EDGE('',*,*,#44175,.F.);
#58526=ORIENTED_EDGE('',*,*,#43790,.T.);
#58527=ORIENTED_EDGE('',*,*,#44177,.F.);
#58528=ORIENTED_EDGE('',*,*,#44178,.T.);
#58529=ORIENTED_EDGE('',*,*,#44179,.F.);
#58530=ORIENTED_EDGE('',*,*,#44180,.T.);
#58531=ORIENTED_EDGE('',*,*,#44177,.T.);
#58532=ORIENTED_EDGE('',*,*,#43789,.T.);
#58533=ORIENTED_EDGE('',*,*,#43806,.F.);
#58534=ORIENTED_EDGE('',*,*,#43813,.T.);
#58535=ORIENTED_EDGE('',*,*,#43814,.T.);
#58536=ORIENTED_EDGE('',*,*,#44181,.T.);
#58537=ORIENTED_EDGE('',*,*,#44182,.F.);
#58538=ORIENTED_EDGE('',*,*,#43900,.T.);
#58539=ORIENTED_EDGE('',*,*,#43902,.T.);
#58540=ORIENTED_EDGE('',*,*,#44183,.T.);
#58541=ORIENTED_EDGE('',*,*,#44184,.T.);
#58542=ORIENTED_EDGE('',*,*,#44185,.F.);
#58543=ORIENTED_EDGE('',*,*,#44050,.T.);
#58544=ORIENTED_EDGE('',*,*,#44186,.F.);
#58545=ORIENTED_EDGE('',*,*,#44187,.F.);
#58546=ORIENTED_EDGE('',*,*,#44188,.T.);
#58547=ORIENTED_EDGE('',*,*,#44189,.T.);
#58548=ORIENTED_EDGE('',*,*,#44063,.T.);
#58549=ORIENTED_EDGE('',*,*,#44190,.F.);
#58550=ORIENTED_EDGE('',*,*,#44191,.T.);
#58551=ORIENTED_EDGE('',*,*,#44187,.T.);
#58552=ORIENTED_EDGE('',*,*,#44062,.T.);
#58553=ORIENTED_EDGE('',*,*,#44192,.F.);
#58554=ORIENTED_EDGE('',*,*,#44193,.T.);
#58555=ORIENTED_EDGE('',*,*,#44190,.T.);
#58556=ORIENTED_EDGE('',*,*,#44061,.T.);
#58557=ORIENTED_EDGE('',*,*,#44194,.F.);
#58558=ORIENTED_EDGE('',*,*,#44195,.T.);
#58559=ORIENTED_EDGE('',*,*,#44192,.T.);
#58560=ORIENTED_EDGE('',*,*,#44060,.T.);
#58561=ORIENTED_EDGE('',*,*,#44194,.T.);
#58562=ORIENTED_EDGE('',*,*,#44059,.T.);
#58563=ORIENTED_EDGE('',*,*,#44196,.T.);
#58564=ORIENTED_EDGE('',*,*,#44197,.T.);
#58565=ORIENTED_EDGE('',*,*,#44058,.T.);
#58566=ORIENTED_EDGE('',*,*,#44182,.T.);
#58567=ORIENTED_EDGE('',*,*,#44198,.T.);
#58568=ORIENTED_EDGE('',*,*,#44199,.F.);
#58569=ORIENTED_EDGE('',*,*,#44200,.T.);
#58570=ORIENTED_EDGE('',*,*,#44048,.F.);
#58571=ORIENTED_EDGE('',*,*,#44056,.T.);
#58572=ORIENTED_EDGE('',*,*,#44201,.F.);
#58573=ORIENTED_EDGE('',*,*,#44202,.F.);
#58574=ORIENTED_EDGE('',*,*,#44055,.T.);
#58575=ORIENTED_EDGE('',*,*,#44203,.T.);
#58576=ORIENTED_EDGE('',*,*,#44204,.T.);
#58577=ORIENTED_EDGE('',*,*,#44203,.F.);
#58578=ORIENTED_EDGE('',*,*,#44054,.T.);
#58579=ORIENTED_EDGE('',*,*,#44205,.T.);
#58580=ORIENTED_EDGE('',*,*,#44206,.T.);
#58581=ORIENTED_EDGE('',*,*,#44205,.F.);
#58582=ORIENTED_EDGE('',*,*,#44053,.T.);
#58583=ORIENTED_EDGE('',*,*,#44207,.T.);
#58584=ORIENTED_EDGE('',*,*,#44208,.T.);
#58585=ORIENTED_EDGE('',*,*,#44207,.F.);
#58586=ORIENTED_EDGE('',*,*,#44052,.T.);
#58587=ORIENTED_EDGE('',*,*,#44209,.T.);
#58588=ORIENTED_EDGE('',*,*,#44210,.T.);
#58589=ORIENTED_EDGE('',*,*,#44209,.F.);
#58590=ORIENTED_EDGE('',*,*,#44051,.T.);
#58591=ORIENTED_EDGE('',*,*,#44211,.T.);
#58592=ORIENTED_EDGE('',*,*,#44212,.T.);
#58593=ORIENTED_EDGE('',*,*,#44039,.F.);
#58594=ORIENTED_EDGE('',*,*,#44046,.T.);
#58595=ORIENTED_EDGE('',*,*,#44047,.T.);
#58596=ORIENTED_EDGE('',*,*,#44213,.T.);
#58597=ORIENTED_EDGE('',*,*,#44214,.T.);
#58598=ORIENTED_EDGE('',*,*,#44215,.F.);
#58599=ORIENTED_EDGE('',*,*,#44021,.T.);
#58600=ORIENTED_EDGE('',*,*,#44216,.F.);
#58601=ORIENTED_EDGE('',*,*,#44217,.F.);
#58602=ORIENTED_EDGE('',*,*,#44218,.T.);
#58603=ORIENTED_EDGE('',*,*,#44219,.T.);
#58604=ORIENTED_EDGE('',*,*,#44037,.T.);
#58605=ORIENTED_EDGE('',*,*,#44220,.F.);
#58606=ORIENTED_EDGE('',*,*,#44221,.T.);
#58607=ORIENTED_EDGE('',*,*,#44217,.T.);
#58608=ORIENTED_EDGE('',*,*,#44036,.T.);
#58609=ORIENTED_EDGE('',*,*,#44222,.F.);
#58610=ORIENTED_EDGE('',*,*,#44223,.T.);
#58611=ORIENTED_EDGE('',*,*,#44220,.T.);
#58612=ORIENTED_EDGE('',*,*,#44035,.T.);
#58613=ORIENTED_EDGE('',*,*,#44224,.F.);
#58614=ORIENTED_EDGE('',*,*,#44225,.T.);
#58615=ORIENTED_EDGE('',*,*,#44222,.T.);
#58616=ORIENTED_EDGE('',*,*,#44034,.T.);
#58617=ORIENTED_EDGE('',*,*,#44226,.F.);
#58618=ORIENTED_EDGE('',*,*,#44227,.T.);
#58619=ORIENTED_EDGE('',*,*,#44224,.T.);
#58620=ORIENTED_EDGE('',*,*,#44033,.T.);
#58621=ORIENTED_EDGE('',*,*,#44032,.T.);
#58622=ORIENTED_EDGE('',*,*,#44038,.T.);
#58623=ORIENTED_EDGE('',*,*,#44228,.T.);
#58624=ORIENTED_EDGE('',*,*,#44229,.F.);
#58625=ORIENTED_EDGE('',*,*,#44015,.F.);
#58626=ORIENTED_EDGE('',*,*,#44030,.T.);
#58627=ORIENTED_EDGE('',*,*,#44230,.T.);
#58628=ORIENTED_EDGE('',*,*,#44231,.T.);
#58629=ORIENTED_EDGE('',*,*,#44230,.F.);
#58630=ORIENTED_EDGE('',*,*,#44029,.T.);
#58631=ORIENTED_EDGE('',*,*,#44232,.T.);
#58632=ORIENTED_EDGE('',*,*,#44233,.T.);
#58633=ORIENTED_EDGE('',*,*,#44028,.T.);
#58634=ORIENTED_EDGE('',*,*,#44234,.F.);
#58635=ORIENTED_EDGE('',*,*,#44235,.T.);
#58636=ORIENTED_EDGE('',*,*,#44236,.T.);
#58637=ORIENTED_EDGE('',*,*,#44237,.F.);
#58638=ORIENTED_EDGE('',*,*,#44238,.T.);
#58639=ORIENTED_EDGE('',*,*,#44234,.T.);
#58640=ORIENTED_EDGE('',*,*,#44027,.T.);
#58641=ORIENTED_EDGE('',*,*,#44239,.F.);
#58642=ORIENTED_EDGE('',*,*,#44240,.F.);
#58643=ORIENTED_EDGE('',*,*,#44026,.T.);
#58644=ORIENTED_EDGE('',*,*,#44241,.T.);
#58645=ORIENTED_EDGE('',*,*,#44242,.T.);
#58646=ORIENTED_EDGE('',*,*,#44241,.F.);
#58647=ORIENTED_EDGE('',*,*,#44025,.T.);
#58648=ORIENTED_EDGE('',*,*,#44243,.T.);
#58649=ORIENTED_EDGE('',*,*,#44244,.T.);
#58650=ORIENTED_EDGE('',*,*,#44243,.F.);
#58651=ORIENTED_EDGE('',*,*,#44024,.T.);
#58652=ORIENTED_EDGE('',*,*,#44245,.T.);
#58653=ORIENTED_EDGE('',*,*,#44246,.T.);
#58654=ORIENTED_EDGE('',*,*,#44245,.F.);
#58655=ORIENTED_EDGE('',*,*,#44023,.T.);
#58656=ORIENTED_EDGE('',*,*,#44247,.F.);
#58657=ORIENTED_EDGE('',*,*,#44248,.T.);
#58658=ORIENTED_EDGE('',*,*,#44249,.F.);
#58659=ORIENTED_EDGE('',*,*,#44250,.T.);
#58660=ORIENTED_EDGE('',*,*,#44247,.T.);
#58661=ORIENTED_EDGE('',*,*,#44022,.T.);
#58662=ORIENTED_EDGE('',*,*,#44251,.T.);
#58663=ORIENTED_EDGE('',*,*,#44252,.F.);
#58664=ORIENTED_EDGE('',*,*,#43817,.T.);
#58665=ORIENTED_EDGE('',*,*,#44253,.F.);
#58666=ORIENTED_EDGE('',*,*,#44254,.F.);
#58667=ORIENTED_EDGE('',*,*,#44255,.T.);
#58668=ORIENTED_EDGE('',*,*,#44256,.T.);
#58669=ORIENTED_EDGE('',*,*,#43833,.T.);
#58670=ORIENTED_EDGE('',*,*,#43961,.T.);
#58671=ORIENTED_EDGE('',*,*,#44257,.T.);
#58672=ORIENTED_EDGE('',*,*,#44254,.T.);
#58673=ORIENTED_EDGE('',*,*,#43832,.T.);
#58674=ORIENTED_EDGE('',*,*,#44258,.T.);
#58675=ORIENTED_EDGE('',*,*,#43815,.F.);
#58676=ORIENTED_EDGE('',*,*,#43830,.T.);
#58677=ORIENTED_EDGE('',*,*,#44259,.F.);
#58678=ORIENTED_EDGE('',*,*,#44260,.F.);
#58679=ORIENTED_EDGE('',*,*,#43829,.T.);
#58680=ORIENTED_EDGE('',*,*,#44261,.T.);
#58681=ORIENTED_EDGE('',*,*,#44262,.T.);
#58682=ORIENTED_EDGE('',*,*,#44261,.F.);
#58683=ORIENTED_EDGE('',*,*,#43828,.T.);
#58684=ORIENTED_EDGE('',*,*,#44263,.T.);
#58685=ORIENTED_EDGE('',*,*,#44264,.T.);
#58686=ORIENTED_EDGE('',*,*,#44263,.F.);
#58687=ORIENTED_EDGE('',*,*,#43827,.T.);
#58688=ORIENTED_EDGE('',*,*,#44265,.T.);
#58689=ORIENTED_EDGE('',*,*,#44266,.T.);
#58690=ORIENTED_EDGE('',*,*,#44265,.F.);
#58691=ORIENTED_EDGE('',*,*,#43826,.T.);
#58692=ORIENTED_EDGE('',*,*,#44267,.T.);
#58693=ORIENTED_EDGE('',*,*,#44268,.T.);
#58694=ORIENTED_EDGE('',*,*,#44267,.F.);
#58695=ORIENTED_EDGE('',*,*,#43825,.T.);
#58696=ORIENTED_EDGE('',*,*,#44269,.T.);
#58697=ORIENTED_EDGE('',*,*,#44270,.T.);
#58698=ORIENTED_EDGE('',*,*,#44271,.T.);
#58699=ORIENTED_EDGE('',*,*,#44272,.F.);
#58700=ORIENTED_EDGE('',*,*,#43824,.T.);
#58701=ORIENTED_EDGE('',*,*,#44273,.F.);
#58702=ORIENTED_EDGE('',*,*,#44274,.F.);
#58703=ORIENTED_EDGE('',*,*,#43823,.T.);
#58704=ORIENTED_EDGE('',*,*,#44275,.T.);
#58705=ORIENTED_EDGE('',*,*,#44276,.T.);
#58706=ORIENTED_EDGE('',*,*,#44275,.F.);
#58707=ORIENTED_EDGE('',*,*,#43822,.T.);
#58708=ORIENTED_EDGE('',*,*,#44277,.T.);
#58709=ORIENTED_EDGE('',*,*,#44278,.T.);
#58710=ORIENTED_EDGE('',*,*,#44277,.F.);
#58711=ORIENTED_EDGE('',*,*,#43821,.T.);
#58712=ORIENTED_EDGE('',*,*,#44279,.T.);
#58713=ORIENTED_EDGE('',*,*,#44280,.T.);
#58714=ORIENTED_EDGE('',*,*,#44279,.F.);
#58715=ORIENTED_EDGE('',*,*,#43820,.T.);
#58716=ORIENTED_EDGE('',*,*,#44281,.F.);
#58717=ORIENTED_EDGE('',*,*,#44282,.F.);
#58718=ORIENTED_EDGE('',*,*,#44283,.T.);
#58719=ORIENTED_EDGE('',*,*,#44281,.T.);
#58720=ORIENTED_EDGE('',*,*,#43819,.T.);
#58721=ORIENTED_EDGE('',*,*,#44284,.F.);
#58722=ORIENTED_EDGE('',*,*,#44285,.F.);
#58723=ORIENTED_EDGE('',*,*,#44286,.T.);
#58724=ORIENTED_EDGE('',*,*,#44282,.T.);
#58725=ORIENTED_EDGE('',*,*,#43818,.T.);
#58726=ORIENTED_EDGE('',*,*,#44252,.T.);
#58727=ORIENTED_EDGE('',*,*,#44287,.T.);
#58728=ORIENTED_EDGE('',*,*,#44288,.F.);
#58729=ORIENTED_EDGE('',*,*,#44228,.F.);
#58730=ORIENTED_EDGE('',*,*,#44040,.F.);
#58731=ORIENTED_EDGE('',*,*,#44213,.F.);
#58732=ORIENTED_EDGE('',*,*,#44049,.F.);
#58733=ORIENTED_EDGE('',*,*,#44200,.F.);
#58734=ORIENTED_EDGE('',*,*,#44289,.F.);
#58735=ORIENTED_EDGE('',*,*,#44290,.F.);
#58736=ORIENTED_EDGE('',*,*,#44291,.F.);
#58737=ORIENTED_EDGE('',*,*,#44292,.F.);
#58738=ORIENTED_EDGE('',*,*,#44293,.F.);
#58739=ORIENTED_EDGE('',*,*,#44294,.T.);
#58740=ORIENTED_EDGE('',*,*,#44295,.F.);
#58741=ORIENTED_EDGE('',*,*,#44159,.F.);
#58742=ORIENTED_EDGE('',*,*,#43807,.F.);
#58743=ORIENTED_EDGE('',*,*,#44181,.F.);
#58744=ORIENTED_EDGE('',*,*,#43816,.F.);
#58745=ORIENTED_EDGE('',*,*,#44258,.F.);
#58746=ORIENTED_EDGE('',*,*,#44296,.F.);
#58747=ORIENTED_EDGE('',*,*,#44297,.T.);
#58748=ORIENTED_EDGE('',*,*,#44298,.T.);
#58749=ORIENTED_EDGE('',*,*,#44299,.F.);
#58750=ORIENTED_EDGE('',*,*,#44300,.F.);
#58751=ORIENTED_EDGE('',*,*,#44301,.F.);
#58752=ORIENTED_EDGE('',*,*,#44302,.F.);
#58753=ORIENTED_EDGE('',*,*,#43896,.F.);
#58754=ORIENTED_EDGE('',*,*,#43781,.F.);
#58755=ORIENTED_EDGE('',*,*,#44303,.T.);
#58756=ORIENTED_EDGE('',*,*,#44304,.F.);
#58757=ORIENTED_EDGE('',*,*,#44300,.T.);
#58758=ORIENTED_EDGE('',*,*,#43783,.F.);
#58759=ORIENTED_EDGE('',*,*,#44162,.F.);
#58760=ORIENTED_EDGE('',*,*,#44305,.T.);
#58761=ORIENTED_EDGE('',*,*,#44306,.T.);
#58762=ORIENTED_EDGE('',*,*,#43958,.T.);
#58763=ORIENTED_EDGE('',*,*,#44307,.T.);
#58764=ORIENTED_EDGE('',*,*,#44305,.F.);
#58765=ORIENTED_EDGE('',*,*,#44308,.T.);
#58766=ORIENTED_EDGE('',*,*,#44309,.T.);
#58767=ORIENTED_EDGE('',*,*,#44310,.T.);
#58768=ORIENTED_EDGE('',*,*,#44309,.F.);
#58769=ORIENTED_EDGE('',*,*,#44311,.T.);
#58770=ORIENTED_EDGE('',*,*,#44312,.T.);
#58771=ORIENTED_EDGE('',*,*,#44313,.T.);
#58772=ORIENTED_EDGE('',*,*,#44314,.T.);
#58773=ORIENTED_EDGE('',*,*,#44315,.F.);
#58774=ORIENTED_EDGE('',*,*,#44316,.T.);
#58775=ORIENTED_EDGE('',*,*,#44317,.T.);
#58776=ORIENTED_EDGE('',*,*,#44318,.T.);
#58777=ORIENTED_EDGE('',*,*,#44317,.F.);
#58778=ORIENTED_EDGE('',*,*,#44319,.T.);
#58779=ORIENTED_EDGE('',*,*,#44320,.T.);
#58780=ORIENTED_EDGE('',*,*,#44321,.T.);
#58781=ORIENTED_EDGE('',*,*,#44322,.F.);
#58782=ORIENTED_EDGE('',*,*,#44323,.F.);
#58783=ORIENTED_EDGE('',*,*,#44324,.F.);
#58784=ORIENTED_EDGE('',*,*,#44325,.F.);
#58785=ORIENTED_EDGE('',*,*,#44326,.F.);
#58786=ORIENTED_EDGE('',*,*,#44327,.T.);
#58787=ORIENTED_EDGE('',*,*,#44328,.T.);
#58788=ORIENTED_EDGE('',*,*,#44329,.T.);
#58789=ORIENTED_EDGE('',*,*,#44330,.F.);
#58790=ORIENTED_EDGE('',*,*,#44313,.F.);
#58791=ORIENTED_EDGE('',*,*,#44331,.T.);
#58792=ORIENTED_EDGE('',*,*,#44332,.T.);
#58793=ORIENTED_EDGE('',*,*,#44333,.T.);
#58794=ORIENTED_EDGE('',*,*,#44332,.F.);
#58795=ORIENTED_EDGE('',*,*,#44334,.T.);
#58796=ORIENTED_EDGE('',*,*,#44335,.T.);
#58797=ORIENTED_EDGE('',*,*,#44336,.T.);
#58798=ORIENTED_EDGE('',*,*,#44335,.F.);
#58799=ORIENTED_EDGE('',*,*,#44337,.T.);
#58800=ORIENTED_EDGE('',*,*,#44338,.T.);
#58801=ORIENTED_EDGE('',*,*,#44339,.T.);
#58802=ORIENTED_EDGE('',*,*,#44338,.F.);
#58803=ORIENTED_EDGE('',*,*,#44340,.T.);
#58804=ORIENTED_EDGE('',*,*,#44341,.T.);
#58805=ORIENTED_EDGE('',*,*,#44342,.T.);
#58806=ORIENTED_EDGE('',*,*,#44341,.F.);
#58807=ORIENTED_EDGE('',*,*,#44343,.T.);
#58808=ORIENTED_EDGE('',*,*,#44344,.T.);
#58809=ORIENTED_EDGE('',*,*,#44345,.T.);
#58810=ORIENTED_EDGE('',*,*,#44346,.F.);
#58811=ORIENTED_EDGE('',*,*,#44347,.T.);
#58812=ORIENTED_EDGE('',*,*,#44348,.F.);
#58813=ORIENTED_EDGE('',*,*,#44349,.F.);
#58814=ORIENTED_EDGE('',*,*,#44350,.T.);
#58815=ORIENTED_EDGE('',*,*,#44351,.F.);
#58816=ORIENTED_EDGE('',*,*,#44352,.F.);
#58817=ORIENTED_EDGE('',*,*,#44353,.T.);
#58818=ORIENTED_EDGE('',*,*,#44354,.T.);
#58819=ORIENTED_EDGE('',*,*,#44355,.T.);
#58820=ORIENTED_EDGE('',*,*,#44354,.F.);
#58821=ORIENTED_EDGE('',*,*,#44356,.T.);
#58822=ORIENTED_EDGE('',*,*,#44357,.T.);
#58823=ORIENTED_EDGE('',*,*,#44358,.T.);
#58824=ORIENTED_EDGE('',*,*,#44357,.F.);
#58825=ORIENTED_EDGE('',*,*,#44359,.T.);
#58826=ORIENTED_EDGE('',*,*,#44360,.T.);
#58827=ORIENTED_EDGE('',*,*,#44361,.T.);
#58828=ORIENTED_EDGE('',*,*,#44360,.F.);
#58829=ORIENTED_EDGE('',*,*,#44362,.T.);
#58830=ORIENTED_EDGE('',*,*,#44363,.T.);
#58831=ORIENTED_EDGE('',*,*,#44364,.T.);
#58832=ORIENTED_EDGE('',*,*,#44363,.F.);
#58833=ORIENTED_EDGE('',*,*,#44365,.T.);
#58834=ORIENTED_EDGE('',*,*,#44366,.T.);
#58835=ORIENTED_EDGE('',*,*,#44367,.T.);
#58836=ORIENTED_EDGE('',*,*,#44368,.T.);
#58837=ORIENTED_EDGE('',*,*,#44369,.F.);
#58838=ORIENTED_EDGE('',*,*,#44370,.F.);
#58839=ORIENTED_EDGE('',*,*,#44369,.T.);
#58840=ORIENTED_EDGE('',*,*,#44371,.T.);
#58841=ORIENTED_EDGE('',*,*,#44372,.F.);
#58842=ORIENTED_EDGE('',*,*,#44373,.T.);
#58843=ORIENTED_EDGE('',*,*,#44374,.F.);
#58844=ORIENTED_EDGE('',*,*,#44375,.T.);
#58845=ORIENTED_EDGE('',*,*,#44372,.T.);
#58846=ORIENTED_EDGE('',*,*,#44376,.T.);
#58847=ORIENTED_EDGE('',*,*,#44377,.F.);
#58848=ORIENTED_EDGE('',*,*,#44378,.F.);
#58849=ORIENTED_EDGE('',*,*,#44379,.T.);
#58850=ORIENTED_EDGE('',*,*,#44380,.T.);
#58851=ORIENTED_EDGE('',*,*,#44381,.T.);
#58852=ORIENTED_EDGE('',*,*,#44380,.F.);
#58853=ORIENTED_EDGE('',*,*,#44382,.T.);
#58854=ORIENTED_EDGE('',*,*,#44383,.T.);
#58855=ORIENTED_EDGE('',*,*,#44384,.T.);
#58856=ORIENTED_EDGE('',*,*,#44383,.F.);
#58857=ORIENTED_EDGE('',*,*,#44385,.T.);
#58858=ORIENTED_EDGE('',*,*,#44386,.T.);
#58859=ORIENTED_EDGE('',*,*,#44387,.T.);
#58860=ORIENTED_EDGE('',*,*,#44386,.F.);
#58861=ORIENTED_EDGE('',*,*,#44388,.T.);
#58862=ORIENTED_EDGE('',*,*,#44389,.T.);
#58863=ORIENTED_EDGE('',*,*,#44390,.T.);
#58864=ORIENTED_EDGE('',*,*,#44389,.F.);
#58865=ORIENTED_EDGE('',*,*,#44391,.T.);
#58866=ORIENTED_EDGE('',*,*,#44392,.T.);
#58867=ORIENTED_EDGE('',*,*,#44393,.T.);
#58868=ORIENTED_EDGE('',*,*,#44394,.T.);
#58869=ORIENTED_EDGE('',*,*,#44395,.F.);
#58870=ORIENTED_EDGE('',*,*,#44396,.T.);
#58871=ORIENTED_EDGE('',*,*,#44397,.F.);
#58872=ORIENTED_EDGE('',*,*,#44398,.F.);
#58873=ORIENTED_EDGE('',*,*,#44399,.T.);
#58874=ORIENTED_EDGE('',*,*,#44400,.T.);
#58875=ORIENTED_EDGE('',*,*,#44401,.T.);
#58876=ORIENTED_EDGE('',*,*,#44400,.F.);
#58877=ORIENTED_EDGE('',*,*,#44402,.T.);
#58878=ORIENTED_EDGE('',*,*,#44403,.T.);
#58879=ORIENTED_EDGE('',*,*,#44404,.T.);
#58880=ORIENTED_EDGE('',*,*,#44403,.F.);
#58881=ORIENTED_EDGE('',*,*,#44405,.T.);
#58882=ORIENTED_EDGE('',*,*,#44406,.T.);
#58883=ORIENTED_EDGE('',*,*,#44407,.T.);
#58884=ORIENTED_EDGE('',*,*,#44406,.F.);
#58885=ORIENTED_EDGE('',*,*,#44408,.T.);
#58886=ORIENTED_EDGE('',*,*,#44409,.T.);
#58887=ORIENTED_EDGE('',*,*,#44410,.T.);
#58888=ORIENTED_EDGE('',*,*,#44409,.F.);
#58889=ORIENTED_EDGE('',*,*,#44411,.T.);
#58890=ORIENTED_EDGE('',*,*,#44412,.T.);
#58891=ORIENTED_EDGE('',*,*,#44413,.T.);
#58892=ORIENTED_EDGE('',*,*,#44414,.T.);
#58893=ORIENTED_EDGE('',*,*,#44415,.F.);
#58894=ORIENTED_EDGE('',*,*,#44416,.T.);
#58895=ORIENTED_EDGE('',*,*,#44417,.F.);
#58896=ORIENTED_EDGE('',*,*,#44418,.F.);
#58897=ORIENTED_EDGE('',*,*,#44419,.T.);
#58898=ORIENTED_EDGE('',*,*,#44315,.T.);
#58899=ORIENTED_EDGE('',*,*,#44420,.T.);
#58900=ORIENTED_EDGE('',*,*,#44421,.F.);
#58901=ORIENTED_EDGE('',*,*,#44329,.F.);
#58902=ORIENTED_EDGE('',*,*,#44422,.T.);
#58903=ORIENTED_EDGE('',*,*,#44423,.F.);
#58904=ORIENTED_EDGE('',*,*,#44424,.F.);
#58905=ORIENTED_EDGE('',*,*,#44425,.F.);
#58906=ORIENTED_EDGE('',*,*,#44426,.F.);
#58907=ORIENTED_EDGE('',*,*,#44427,.F.);
#58908=ORIENTED_EDGE('',*,*,#44428,.F.);
#58909=ORIENTED_EDGE('',*,*,#44423,.T.);
#58910=ORIENTED_EDGE('',*,*,#44429,.T.);
#58911=ORIENTED_EDGE('',*,*,#44430,.T.);
#58912=ORIENTED_EDGE('',*,*,#44431,.F.);
#58913=ORIENTED_EDGE('',*,*,#44432,.F.);
#58914=ORIENTED_EDGE('',*,*,#44433,.T.);
#58915=ORIENTED_EDGE('',*,*,#44434,.T.);
#58916=ORIENTED_EDGE('',*,*,#44435,.T.);
#58917=ORIENTED_EDGE('',*,*,#44436,.F.);
#58918=ORIENTED_EDGE('',*,*,#44437,.T.);
#58919=ORIENTED_EDGE('',*,*,#44432,.T.);
#58920=ORIENTED_EDGE('',*,*,#44438,.T.);
#58921=ORIENTED_EDGE('',*,*,#44439,.T.);
#58922=ORIENTED_EDGE('',*,*,#44440,.F.);
#58923=ORIENTED_EDGE('',*,*,#44441,.T.);
#58924=ORIENTED_EDGE('',*,*,#44435,.F.);
#58925=ORIENTED_EDGE('',*,*,#44442,.F.);
#58926=ORIENTED_EDGE('',*,*,#44440,.T.);
#58927=ORIENTED_EDGE('',*,*,#44443,.T.);
#58928=ORIENTED_EDGE('',*,*,#44444,.T.);
#58929=ORIENTED_EDGE('',*,*,#44445,.F.);
#58930=ORIENTED_EDGE('',*,*,#44446,.T.);
#58931=ORIENTED_EDGE('',*,*,#44442,.T.);
#58932=ORIENTED_EDGE('',*,*,#44447,.T.);
#58933=ORIENTED_EDGE('',*,*,#44448,.F.);
#58934=ORIENTED_EDGE('',*,*,#44449,.T.);
#58935=ORIENTED_EDGE('',*,*,#44445,.T.);
#58936=ORIENTED_EDGE('',*,*,#44450,.T.);
#58937=ORIENTED_EDGE('',*,*,#44451,.F.);
#58938=ORIENTED_EDGE('',*,*,#44452,.T.);
#58939=ORIENTED_EDGE('',*,*,#44448,.T.);
#58940=ORIENTED_EDGE('',*,*,#44453,.T.);
#58941=ORIENTED_EDGE('',*,*,#44454,.F.);
#58942=ORIENTED_EDGE('',*,*,#44455,.T.);
#58943=ORIENTED_EDGE('',*,*,#44451,.T.);
#58944=ORIENTED_EDGE('',*,*,#44456,.T.);
#58945=ORIENTED_EDGE('',*,*,#44457,.F.);
#58946=ORIENTED_EDGE('',*,*,#44458,.T.);
#58947=ORIENTED_EDGE('',*,*,#44454,.T.);
#58948=ORIENTED_EDGE('',*,*,#44459,.T.);
#58949=ORIENTED_EDGE('',*,*,#44460,.F.);
#58950=ORIENTED_EDGE('',*,*,#44461,.T.);
#58951=ORIENTED_EDGE('',*,*,#44457,.T.);
#58952=ORIENTED_EDGE('',*,*,#44462,.T.);
#58953=ORIENTED_EDGE('',*,*,#44463,.F.);
#58954=ORIENTED_EDGE('',*,*,#44464,.T.);
#58955=ORIENTED_EDGE('',*,*,#44460,.T.);
#58956=ORIENTED_EDGE('',*,*,#44465,.T.);
#58957=ORIENTED_EDGE('',*,*,#44466,.F.);
#58958=ORIENTED_EDGE('',*,*,#44467,.T.);
#58959=ORIENTED_EDGE('',*,*,#44463,.T.);
#58960=ORIENTED_EDGE('',*,*,#44468,.T.);
#58961=ORIENTED_EDGE('',*,*,#44469,.F.);
#58962=ORIENTED_EDGE('',*,*,#44470,.T.);
#58963=ORIENTED_EDGE('',*,*,#44466,.T.);
#58964=ORIENTED_EDGE('',*,*,#44471,.T.);
#58965=ORIENTED_EDGE('',*,*,#44472,.F.);
#58966=ORIENTED_EDGE('',*,*,#44473,.T.);
#58967=ORIENTED_EDGE('',*,*,#44469,.T.);
#58968=ORIENTED_EDGE('',*,*,#44474,.T.);
#58969=ORIENTED_EDGE('',*,*,#44475,.F.);
#58970=ORIENTED_EDGE('',*,*,#44476,.T.);
#58971=ORIENTED_EDGE('',*,*,#44472,.T.);
#58972=ORIENTED_EDGE('',*,*,#44477,.T.);
#58973=ORIENTED_EDGE('',*,*,#44478,.F.);
#58974=ORIENTED_EDGE('',*,*,#44479,.T.);
#58975=ORIENTED_EDGE('',*,*,#44475,.T.);
#58976=ORIENTED_EDGE('',*,*,#44480,.T.);
#58977=ORIENTED_EDGE('',*,*,#44481,.F.);
#58978=ORIENTED_EDGE('',*,*,#44482,.T.);
#58979=ORIENTED_EDGE('',*,*,#44478,.T.);
#58980=ORIENTED_EDGE('',*,*,#44483,.T.);
#58981=ORIENTED_EDGE('',*,*,#44484,.F.);
#58982=ORIENTED_EDGE('',*,*,#44485,.T.);
#58983=ORIENTED_EDGE('',*,*,#44481,.T.);
#58984=ORIENTED_EDGE('',*,*,#44486,.T.);
#58985=ORIENTED_EDGE('',*,*,#44487,.T.);
#58986=ORIENTED_EDGE('',*,*,#44488,.T.);
#58987=ORIENTED_EDGE('',*,*,#44489,.T.);
#58988=ORIENTED_EDGE('',*,*,#44490,.F.);
#58989=ORIENTED_EDGE('',*,*,#44489,.F.);
#58990=ORIENTED_EDGE('',*,*,#44491,.T.);
#58991=ORIENTED_EDGE('',*,*,#44492,.T.);
#58992=ORIENTED_EDGE('',*,*,#44493,.T.);
#58993=ORIENTED_EDGE('',*,*,#44494,.T.);
#58994=ORIENTED_EDGE('',*,*,#44495,.T.);
#58995=ORIENTED_EDGE('',*,*,#44496,.T.);
#58996=ORIENTED_EDGE('',*,*,#44497,.F.);
#58997=ORIENTED_EDGE('',*,*,#44496,.F.);
#58998=ORIENTED_EDGE('',*,*,#44498,.T.);
#58999=ORIENTED_EDGE('',*,*,#44499,.T.);
#59000=ORIENTED_EDGE('',*,*,#44500,.T.);
#59001=ORIENTED_EDGE('',*,*,#44501,.T.);
#59002=ORIENTED_EDGE('',*,*,#44502,.T.);
#59003=ORIENTED_EDGE('',*,*,#44503,.T.);
#59004=ORIENTED_EDGE('',*,*,#44504,.T.);
#59005=ORIENTED_EDGE('',*,*,#44501,.F.);
#59006=ORIENTED_EDGE('',*,*,#44505,.T.);
#59007=ORIENTED_EDGE('',*,*,#44506,.T.);
#59008=ORIENTED_EDGE('',*,*,#44507,.T.);
#59009=ORIENTED_EDGE('',*,*,#44508,.T.);
#59010=ORIENTED_EDGE('',*,*,#44509,.F.);
#59011=ORIENTED_EDGE('',*,*,#44510,.T.);
#59012=ORIENTED_EDGE('',*,*,#44511,.F.);
#59013=ORIENTED_EDGE('',*,*,#44512,.F.);
#59014=ORIENTED_EDGE('',*,*,#44513,.T.);
#59015=ORIENTED_EDGE('',*,*,#44514,.T.);
#59016=ORIENTED_EDGE('',*,*,#44515,.T.);
#59017=ORIENTED_EDGE('',*,*,#44516,.F.);
#59018=ORIENTED_EDGE('',*,*,#44517,.T.);
#59019=ORIENTED_EDGE('',*,*,#44512,.T.);
#59020=ORIENTED_EDGE('',*,*,#44518,.T.);
#59021=ORIENTED_EDGE('',*,*,#44519,.F.);
#59022=ORIENTED_EDGE('',*,*,#44520,.T.);
#59023=ORIENTED_EDGE('',*,*,#44516,.T.);
#59024=ORIENTED_EDGE('',*,*,#44521,.T.);
#59025=ORIENTED_EDGE('',*,*,#44519,.T.);
#59026=ORIENTED_EDGE('',*,*,#44522,.T.);
#59027=ORIENTED_EDGE('',*,*,#44523,.T.);
#59028=ORIENTED_EDGE('',*,*,#44524,.T.);
#59029=ORIENTED_EDGE('',*,*,#44523,.F.);
#59030=ORIENTED_EDGE('',*,*,#44525,.T.);
#59031=ORIENTED_EDGE('',*,*,#44526,.T.);
#59032=ORIENTED_EDGE('',*,*,#44527,.T.);
#59033=ORIENTED_EDGE('',*,*,#44528,.T.);
#59034=ORIENTED_EDGE('',*,*,#44529,.F.);
#59035=ORIENTED_EDGE('',*,*,#44530,.T.);
#59036=ORIENTED_EDGE('',*,*,#44531,.F.);
#59037=ORIENTED_EDGE('',*,*,#44532,.F.);
#59038=ORIENTED_EDGE('',*,*,#44533,.T.);
#59039=ORIENTED_EDGE('',*,*,#44534,.T.);
#59040=ORIENTED_EDGE('',*,*,#44535,.T.);
#59041=ORIENTED_EDGE('',*,*,#44536,.F.);
#59042=ORIENTED_EDGE('',*,*,#44537,.T.);
#59043=ORIENTED_EDGE('',*,*,#44532,.T.);
#59044=ORIENTED_EDGE('',*,*,#44538,.T.);
#59045=ORIENTED_EDGE('',*,*,#44539,.F.);
#59046=ORIENTED_EDGE('',*,*,#44540,.T.);
#59047=ORIENTED_EDGE('',*,*,#44536,.T.);
#59048=ORIENTED_EDGE('',*,*,#44541,.T.);
#59049=ORIENTED_EDGE('',*,*,#44539,.T.);
#59050=ORIENTED_EDGE('',*,*,#44542,.T.);
#59051=ORIENTED_EDGE('',*,*,#44543,.T.);
#59052=ORIENTED_EDGE('',*,*,#44544,.T.);
#59053=ORIENTED_EDGE('',*,*,#44543,.F.);
#59054=ORIENTED_EDGE('',*,*,#44545,.T.);
#59055=ORIENTED_EDGE('',*,*,#44546,.T.);
#59056=ORIENTED_EDGE('',*,*,#44547,.T.);
#59057=ORIENTED_EDGE('',*,*,#44548,.T.);
#59058=ORIENTED_EDGE('',*,*,#44549,.F.);
#59059=ORIENTED_EDGE('',*,*,#44550,.T.);
#59060=ORIENTED_EDGE('',*,*,#44551,.F.);
#59061=ORIENTED_EDGE('',*,*,#44552,.F.);
#59062=ORIENTED_EDGE('',*,*,#44553,.T.);
#59063=ORIENTED_EDGE('',*,*,#44554,.T.);
#59064=ORIENTED_EDGE('',*,*,#44555,.T.);
#59065=ORIENTED_EDGE('',*,*,#44556,.F.);
#59066=ORIENTED_EDGE('',*,*,#44557,.T.);
#59067=ORIENTED_EDGE('',*,*,#44552,.T.);
#59068=ORIENTED_EDGE('',*,*,#44558,.T.);
#59069=ORIENTED_EDGE('',*,*,#44559,.F.);
#59070=ORIENTED_EDGE('',*,*,#44560,.F.);
#59071=ORIENTED_EDGE('',*,*,#44561,.T.);
#59072=ORIENTED_EDGE('',*,*,#44485,.F.);
#59073=ORIENTED_EDGE('',*,*,#44562,.T.);
#59074=ORIENTED_EDGE('',*,*,#44563,.F.);
#59075=ORIENTED_EDGE('',*,*,#44564,.F.);
#59076=ORIENTED_EDGE('',*,*,#44565,.T.);
#59077=ORIENTED_EDGE('',*,*,#44566,.T.);
#59078=ORIENTED_EDGE('',*,*,#44567,.T.);
#59079=ORIENTED_EDGE('',*,*,#44503,.F.);
#59080=ORIENTED_EDGE('',*,*,#44568,.T.);
#59081=ORIENTED_EDGE('',*,*,#44564,.T.);
#59082=ORIENTED_EDGE('',*,*,#44569,.T.);
#59083=ORIENTED_EDGE('',*,*,#44570,.T.);
#59084=ORIENTED_EDGE('',*,*,#44571,.T.);
#59085=ORIENTED_EDGE('',*,*,#44572,.T.);
#59086=ORIENTED_EDGE('',*,*,#44557,.F.);
#59087=ORIENTED_EDGE('',*,*,#44571,.F.);
#59088=ORIENTED_EDGE('',*,*,#44573,.T.);
#59089=ORIENTED_EDGE('',*,*,#44574,.T.);
#59090=ORIENTED_EDGE('',*,*,#44575,.T.);
#59091=ORIENTED_EDGE('',*,*,#44576,.T.);
#59092=ORIENTED_EDGE('',*,*,#44574,.F.);
#59093=ORIENTED_EDGE('',*,*,#44577,.T.);
#59094=ORIENTED_EDGE('',*,*,#43835,.F.);
#59095=ORIENTED_EDGE('',*,*,#44578,.F.);
#59096=ORIENTED_EDGE('',*,*,#44579,.T.);
#59097=ORIENTED_EDGE('',*,*,#43838,.T.);
#59098=ORIENTED_EDGE('',*,*,#43842,.T.);
#59099=ORIENTED_EDGE('',*,*,#44572,.F.);
#59100=ORIENTED_EDGE('',*,*,#44575,.F.);
#59101=ORIENTED_EDGE('',*,*,#44576,.F.);
#59102=ORIENTED_EDGE('',*,*,#43839,.F.);
#59103=ORIENTED_EDGE('',*,*,#44579,.F.);
#59104=ORIENTED_EDGE('',*,*,#44580,.F.);
#59105=ORIENTED_EDGE('',*,*,#44581,.F.);
#59106=ORIENTED_EDGE('',*,*,#44582,.F.);
#59107=ORIENTED_EDGE('',*,*,#44583,.F.);
#59108=ORIENTED_EDGE('',*,*,#44584,.F.);
#59109=ORIENTED_EDGE('',*,*,#44585,.F.);
#59110=ORIENTED_EDGE('',*,*,#44553,.F.);
#59111=ORIENTED_EDGE('',*,*,#44586,.F.);
#59112=ORIENTED_EDGE('',*,*,#44587,.F.);
#59113=ORIENTED_EDGE('',*,*,#43841,.F.);
#59114=ORIENTED_EDGE('',*,*,#44588,.F.);
#59115=ORIENTED_EDGE('',*,*,#44589,.F.);
#59116=ORIENTED_EDGE('',*,*,#43844,.T.);
#59117=ORIENTED_EDGE('',*,*,#43848,.T.);
#59118=ORIENTED_EDGE('',*,*,#43847,.T.);
#59119=ORIENTED_EDGE('',*,*,#44590,.T.);
#59120=ORIENTED_EDGE('',*,*,#44591,.F.);
#59121=ORIENTED_EDGE('',*,*,#44592,.F.);
#59122=ORIENTED_EDGE('',*,*,#44593,.F.);
#59123=ORIENTED_EDGE('',*,*,#44547,.F.);
#59124=ORIENTED_EDGE('',*,*,#44594,.F.);
#59125=ORIENTED_EDGE('',*,*,#44595,.F.);
#59126=ORIENTED_EDGE('',*,*,#44596,.F.);
#59127=ORIENTED_EDGE('',*,*,#44597,.F.);
#59128=ORIENTED_EDGE('',*,*,#44598,.F.);
#59129=ORIENTED_EDGE('',*,*,#44599,.F.);
#59130=ORIENTED_EDGE('',*,*,#44590,.F.);
#59131=ORIENTED_EDGE('',*,*,#43846,.F.);
#59132=ORIENTED_EDGE('',*,*,#44600,.T.);
#59133=ORIENTED_EDGE('',*,*,#44601,.T.);
#59134=ORIENTED_EDGE('',*,*,#44591,.T.);
#59135=ORIENTED_EDGE('',*,*,#43853,.F.);
#59136=ORIENTED_EDGE('',*,*,#44602,.F.);
#59137=ORIENTED_EDGE('',*,*,#44603,.T.);
#59138=ORIENTED_EDGE('',*,*,#44600,.F.);
#59139=ORIENTED_EDGE('',*,*,#43856,.F.);
#59140=ORIENTED_EDGE('',*,*,#44604,.T.);
#59141=ORIENTED_EDGE('',*,*,#44605,.F.);
#59142=ORIENTED_EDGE('',*,*,#44602,.T.);
#59143=ORIENTED_EDGE('',*,*,#43859,.F.);
#59144=ORIENTED_EDGE('',*,*,#44606,.F.);
#59145=ORIENTED_EDGE('',*,*,#44607,.T.);
#59146=ORIENTED_EDGE('',*,*,#43860,.T.);
#59147=ORIENTED_EDGE('',*,*,#43864,.T.);
#59148=ORIENTED_EDGE('',*,*,#44608,.F.);
#59149=ORIENTED_EDGE('',*,*,#44609,.F.);
#59150=ORIENTED_EDGE('',*,*,#44604,.F.);
#59151=ORIENTED_EDGE('',*,*,#43861,.F.);
#59152=ORIENTED_EDGE('',*,*,#44607,.F.);
#59153=ORIENTED_EDGE('',*,*,#44610,.F.);
#59154=ORIENTED_EDGE('',*,*,#44611,.F.);
#59155=ORIENTED_EDGE('',*,*,#44612,.F.);
#59156=ORIENTED_EDGE('',*,*,#44613,.F.);
#59157=ORIENTED_EDGE('',*,*,#44614,.F.);
#59158=ORIENTED_EDGE('',*,*,#44615,.F.);
#59159=ORIENTED_EDGE('',*,*,#44533,.F.);
#59160=ORIENTED_EDGE('',*,*,#44616,.F.);
#59161=ORIENTED_EDGE('',*,*,#44617,.F.);
#59162=ORIENTED_EDGE('',*,*,#43863,.F.);
#59163=ORIENTED_EDGE('',*,*,#44618,.F.);
#59164=ORIENTED_EDGE('',*,*,#44619,.F.);
#59165=ORIENTED_EDGE('',*,*,#43866,.T.);
#59166=ORIENTED_EDGE('',*,*,#43870,.T.);
#59167=ORIENTED_EDGE('',*,*,#43869,.T.);
#59168=ORIENTED_EDGE('',*,*,#44620,.T.);
#59169=ORIENTED_EDGE('',*,*,#44621,.F.);
#59170=ORIENTED_EDGE('',*,*,#44622,.F.);
#59171=ORIENTED_EDGE('',*,*,#44623,.F.);
#59172=ORIENTED_EDGE('',*,*,#44624,.F.);
#59173=ORIENTED_EDGE('',*,*,#44625,.F.);
#59174=ORIENTED_EDGE('',*,*,#44527,.F.);
#59175=ORIENTED_EDGE('',*,*,#44626,.F.);
#59176=ORIENTED_EDGE('',*,*,#44627,.F.);
#59177=ORIENTED_EDGE('',*,*,#44628,.F.);
#59178=ORIENTED_EDGE('',*,*,#44629,.F.);
#59179=ORIENTED_EDGE('',*,*,#44630,.F.);
#59180=ORIENTED_EDGE('',*,*,#44631,.F.);
#59181=ORIENTED_EDGE('',*,*,#44620,.F.);
#59182=ORIENTED_EDGE('',*,*,#43868,.F.);
#59183=ORIENTED_EDGE('',*,*,#44632,.T.);
#59184=ORIENTED_EDGE('',*,*,#44633,.T.);
#59185=ORIENTED_EDGE('',*,*,#44621,.T.);
#59186=ORIENTED_EDGE('',*,*,#43874,.F.);
#59187=ORIENTED_EDGE('',*,*,#44634,.F.);
#59188=ORIENTED_EDGE('',*,*,#44635,.F.);
#59189=ORIENTED_EDGE('',*,*,#44632,.F.);
#59190=ORIENTED_EDGE('',*,*,#43877,.F.);
#59191=ORIENTED_EDGE('',*,*,#44636,.T.);
#59192=ORIENTED_EDGE('',*,*,#44637,.F.);
#59193=ORIENTED_EDGE('',*,*,#44634,.T.);
#59194=ORIENTED_EDGE('',*,*,#43880,.F.);
#59195=ORIENTED_EDGE('',*,*,#44638,.F.);
#59196=ORIENTED_EDGE('',*,*,#44639,.T.);
#59197=ORIENTED_EDGE('',*,*,#43881,.T.);
#59198=ORIENTED_EDGE('',*,*,#43885,.T.);
#59199=ORIENTED_EDGE('',*,*,#44640,.F.);
#59200=ORIENTED_EDGE('',*,*,#44641,.F.);
#59201=ORIENTED_EDGE('',*,*,#44642,.F.);
#59202=ORIENTED_EDGE('',*,*,#44643,.F.);
#59203=ORIENTED_EDGE('',*,*,#44636,.F.);
#59204=ORIENTED_EDGE('',*,*,#43882,.F.);
#59205=ORIENTED_EDGE('',*,*,#44639,.F.);
#59206=ORIENTED_EDGE('',*,*,#44644,.F.);
#59207=ORIENTED_EDGE('',*,*,#44645,.F.);
#59208=ORIENTED_EDGE('',*,*,#44646,.F.);
#59209=ORIENTED_EDGE('',*,*,#44647,.F.);
#59210=ORIENTED_EDGE('',*,*,#44648,.F.);
#59211=ORIENTED_EDGE('',*,*,#44649,.F.);
#59212=ORIENTED_EDGE('',*,*,#44513,.F.);
#59213=ORIENTED_EDGE('',*,*,#44650,.F.);
#59214=ORIENTED_EDGE('',*,*,#44651,.F.);
#59215=ORIENTED_EDGE('',*,*,#43884,.F.);
#59216=ORIENTED_EDGE('',*,*,#44652,.F.);
#59217=ORIENTED_EDGE('',*,*,#44653,.F.);
#59218=ORIENTED_EDGE('',*,*,#43887,.T.);
#59219=ORIENTED_EDGE('',*,*,#43890,.T.);
#59220=ORIENTED_EDGE('',*,*,#44654,.T.);
#59221=ORIENTED_EDGE('',*,*,#44655,.F.);
#59222=ORIENTED_EDGE('',*,*,#44656,.F.);
#59223=ORIENTED_EDGE('',*,*,#44657,.F.);
#59224=ORIENTED_EDGE('',*,*,#44658,.F.);
#59225=ORIENTED_EDGE('',*,*,#44659,.F.);
#59226=ORIENTED_EDGE('',*,*,#44507,.F.);
#59227=ORIENTED_EDGE('',*,*,#44660,.F.);
#59228=ORIENTED_EDGE('',*,*,#44661,.F.);
#59229=ORIENTED_EDGE('',*,*,#44662,.F.);
#59230=ORIENTED_EDGE('',*,*,#44663,.F.);
#59231=ORIENTED_EDGE('',*,*,#44664,.F.);
#59232=ORIENTED_EDGE('',*,*,#44665,.F.);
#59233=ORIENTED_EDGE('',*,*,#44654,.F.);
#59234=ORIENTED_EDGE('',*,*,#43889,.F.);
#59235=ORIENTED_EDGE('',*,*,#44302,.T.);
#59236=ORIENTED_EDGE('',*,*,#44666,.T.);
#59237=ORIENTED_EDGE('',*,*,#44655,.T.);
#59238=ORIENTED_EDGE('',*,*,#43894,.F.);
#59239=ORIENTED_EDGE('',*,*,#44667,.T.);
#59240=ORIENTED_EDGE('',*,*,#44668,.F.);
#59241=ORIENTED_EDGE('',*,*,#44198,.F.);
#59242=ORIENTED_EDGE('',*,*,#44183,.F.);
#59243=ORIENTED_EDGE('',*,*,#43901,.F.);
#59244=ORIENTED_EDGE('',*,*,#44669,.F.);
#59245=ORIENTED_EDGE('',*,*,#43907,.F.);
#59246=ORIENTED_EDGE('',*,*,#44670,.T.);
#59247=ORIENTED_EDGE('',*,*,#44671,.T.);
#59248=ORIENTED_EDGE('',*,*,#43904,.T.);
#59249=ORIENTED_EDGE('',*,*,#44672,.F.);
#59250=ORIENTED_EDGE('',*,*,#44673,.F.);
#59251=ORIENTED_EDGE('',*,*,#44674,.F.);
#59252=ORIENTED_EDGE('',*,*,#44393,.F.);
#59253=ORIENTED_EDGE('',*,*,#44675,.F.);
#59254=ORIENTED_EDGE('',*,*,#44676,.F.);
#59255=ORIENTED_EDGE('',*,*,#44677,.F.);
#59256=ORIENTED_EDGE('',*,*,#44678,.F.);
#59257=ORIENTED_EDGE('',*,*,#44679,.F.);
#59258=ORIENTED_EDGE('',*,*,#44670,.F.);
#59259=ORIENTED_EDGE('',*,*,#43906,.F.);
#59260=ORIENTED_EDGE('',*,*,#44680,.T.);
#59261=ORIENTED_EDGE('',*,*,#44681,.T.);
#59262=ORIENTED_EDGE('',*,*,#44672,.T.);
#59263=ORIENTED_EDGE('',*,*,#43910,.F.);
#59264=ORIENTED_EDGE('',*,*,#44682,.F.);
#59265=ORIENTED_EDGE('',*,*,#44683,.F.);
#59266=ORIENTED_EDGE('',*,*,#44680,.F.);
#59267=ORIENTED_EDGE('',*,*,#43913,.F.);
#59268=ORIENTED_EDGE('',*,*,#44684,.T.);
#59269=ORIENTED_EDGE('',*,*,#44685,.F.);
#59270=ORIENTED_EDGE('',*,*,#44682,.T.);
#59271=ORIENTED_EDGE('',*,*,#43916,.F.);
#59272=ORIENTED_EDGE('',*,*,#44686,.F.);
#59273=ORIENTED_EDGE('',*,*,#44687,.F.);
#59274=ORIENTED_EDGE('',*,*,#44688,.F.);
#59275=ORIENTED_EDGE('',*,*,#44689,.F.);
#59276=ORIENTED_EDGE('',*,*,#44690,.F.);
#59277=ORIENTED_EDGE('',*,*,#44381,.F.);
#59278=ORIENTED_EDGE('',*,*,#44691,.F.);
#59279=ORIENTED_EDGE('',*,*,#44692,.F.);
#59280=ORIENTED_EDGE('',*,*,#44684,.F.);
#59281=ORIENTED_EDGE('',*,*,#43920,.F.);
#59282=ORIENTED_EDGE('',*,*,#43919,.F.);
#59283=ORIENTED_EDGE('',*,*,#43922,.T.);
#59284=ORIENTED_EDGE('',*,*,#44693,.T.);
#59285=ORIENTED_EDGE('',*,*,#44686,.T.);
#59286=ORIENTED_EDGE('',*,*,#44694,.F.);
#59287=ORIENTED_EDGE('',*,*,#44695,.F.);
#59288=ORIENTED_EDGE('',*,*,#43921,.F.);
#59289=ORIENTED_EDGE('',*,*,#44696,.F.);
#59290=ORIENTED_EDGE('',*,*,#43927,.F.);
#59291=ORIENTED_EDGE('',*,*,#44697,.T.);
#59292=ORIENTED_EDGE('',*,*,#44698,.T.);
#59293=ORIENTED_EDGE('',*,*,#43924,.T.);
#59294=ORIENTED_EDGE('',*,*,#44699,.F.);
#59295=ORIENTED_EDGE('',*,*,#44700,.F.);
#59296=ORIENTED_EDGE('',*,*,#44367,.F.);
#59297=ORIENTED_EDGE('',*,*,#44701,.F.);
#59298=ORIENTED_EDGE('',*,*,#44702,.F.);
#59299=ORIENTED_EDGE('',*,*,#44703,.F.);
#59300=ORIENTED_EDGE('',*,*,#44704,.F.);
#59301=ORIENTED_EDGE('',*,*,#44697,.F.);
#59302=ORIENTED_EDGE('',*,*,#43926,.F.);
#59303=ORIENTED_EDGE('',*,*,#44705,.T.);
#59304=ORIENTED_EDGE('',*,*,#44706,.T.);
#59305=ORIENTED_EDGE('',*,*,#44699,.T.);
#59306=ORIENTED_EDGE('',*,*,#43930,.F.);
#59307=ORIENTED_EDGE('',*,*,#44707,.F.);
#59308=ORIENTED_EDGE('',*,*,#44708,.T.);
#59309=ORIENTED_EDGE('',*,*,#44705,.F.);
#59310=ORIENTED_EDGE('',*,*,#43933,.F.);
#59311=ORIENTED_EDGE('',*,*,#44709,.T.);
#59312=ORIENTED_EDGE('',*,*,#44710,.T.);
#59313=ORIENTED_EDGE('',*,*,#44707,.T.);
#59314=ORIENTED_EDGE('',*,*,#43936,.F.);
#59315=ORIENTED_EDGE('',*,*,#44711,.T.);
#59316=ORIENTED_EDGE('',*,*,#44712,.T.);
#59317=ORIENTED_EDGE('',*,*,#43938,.T.);
#59318=ORIENTED_EDGE('',*,*,#43942,.T.);
#59319=ORIENTED_EDGE('',*,*,#44712,.F.);
#59320=ORIENTED_EDGE('',*,*,#44713,.F.);
#59321=ORIENTED_EDGE('',*,*,#44714,.F.);
#59322=ORIENTED_EDGE('',*,*,#44355,.F.);
#59323=ORIENTED_EDGE('',*,*,#44715,.F.);
#59324=ORIENTED_EDGE('',*,*,#44709,.F.);
#59325=ORIENTED_EDGE('',*,*,#43939,.F.);
#59326=ORIENTED_EDGE('',*,*,#44347,.F.);
#59327=ORIENTED_EDGE('',*,*,#44716,.F.);
#59328=ORIENTED_EDGE('',*,*,#43941,.F.);
#59329=ORIENTED_EDGE('',*,*,#44717,.F.);
#59330=ORIENTED_EDGE('',*,*,#43947,.F.);
#59331=ORIENTED_EDGE('',*,*,#44718,.T.);
#59332=ORIENTED_EDGE('',*,*,#44719,.T.);
#59333=ORIENTED_EDGE('',*,*,#43944,.T.);
#59334=ORIENTED_EDGE('',*,*,#44720,.F.);
#59335=ORIENTED_EDGE('',*,*,#44721,.F.);
#59336=ORIENTED_EDGE('',*,*,#44345,.F.);
#59337=ORIENTED_EDGE('',*,*,#44722,.F.);
#59338=ORIENTED_EDGE('',*,*,#44723,.F.);
#59339=ORIENTED_EDGE('',*,*,#44718,.F.);
#59340=ORIENTED_EDGE('',*,*,#43946,.F.);
#59341=ORIENTED_EDGE('',*,*,#44724,.T.);
#59342=ORIENTED_EDGE('',*,*,#44725,.T.);
#59343=ORIENTED_EDGE('',*,*,#44720,.T.);
#59344=ORIENTED_EDGE('',*,*,#43950,.F.);
#59345=ORIENTED_EDGE('',*,*,#44726,.F.);
#59346=ORIENTED_EDGE('',*,*,#44727,.T.);
#59347=ORIENTED_EDGE('',*,*,#44724,.F.);
#59348=ORIENTED_EDGE('',*,*,#43953,.F.);
#59349=ORIENTED_EDGE('',*,*,#44728,.T.);
#59350=ORIENTED_EDGE('',*,*,#44729,.T.);
#59351=ORIENTED_EDGE('',*,*,#44726,.T.);
#59352=ORIENTED_EDGE('',*,*,#43956,.F.);
#59353=ORIENTED_EDGE('',*,*,#44306,.F.);
#59354=ORIENTED_EDGE('',*,*,#44310,.F.);
#59355=ORIENTED_EDGE('',*,*,#44314,.F.);
#59356=ORIENTED_EDGE('',*,*,#44333,.F.);
#59357=ORIENTED_EDGE('',*,*,#44730,.F.);
#59358=ORIENTED_EDGE('',*,*,#44728,.F.);
#59359=ORIENTED_EDGE('',*,*,#43959,.F.);
#59360=ORIENTED_EDGE('',*,*,#44011,.F.);
#59361=ORIENTED_EDGE('',*,*,#44731,.T.);
#59362=ORIENTED_EDGE('',*,*,#44732,.T.);
#59363=ORIENTED_EDGE('',*,*,#44733,.T.);
#59364=ORIENTED_EDGE('',*,*,#44144,.F.);
#59365=ORIENTED_EDGE('',*,*,#44734,.F.);
#59366=ORIENTED_EDGE('',*,*,#44735,.F.);
#59367=ORIENTED_EDGE('',*,*,#44731,.F.);
#59368=ORIENTED_EDGE('',*,*,#44014,.F.);
#59369=ORIENTED_EDGE('',*,*,#44736,.T.);
#59370=ORIENTED_EDGE('',*,*,#44737,.F.);
#59371=ORIENTED_EDGE('',*,*,#44734,.T.);
#59372=ORIENTED_EDGE('',*,*,#44016,.F.);
#59373=ORIENTED_EDGE('',*,*,#44231,.F.);
#59374=ORIENTED_EDGE('',*,*,#44738,.T.);
#59375=ORIENTED_EDGE('',*,*,#44739,.T.);
#59376=ORIENTED_EDGE('',*,*,#44740,.T.);
#59377=ORIENTED_EDGE('',*,*,#44257,.F.);
#59378=ORIENTED_EDGE('',*,*,#43963,.F.);
#59379=ORIENTED_EDGE('',*,*,#44741,.F.);
#59380=ORIENTED_EDGE('',*,*,#44742,.F.);
#59381=ORIENTED_EDGE('',*,*,#44738,.F.);
#59382=ORIENTED_EDGE('',*,*,#43965,.F.);
#59383=ORIENTED_EDGE('',*,*,#44743,.T.);
#59384=ORIENTED_EDGE('',*,*,#44744,.F.);
#59385=ORIENTED_EDGE('',*,*,#44741,.T.);
#59386=ORIENTED_EDGE('',*,*,#43967,.F.);
#59387=ORIENTED_EDGE('',*,*,#44065,.F.);
#59388=ORIENTED_EDGE('',*,*,#44745,.F.);
#59389=ORIENTED_EDGE('',*,*,#44746,.F.);
#59390=ORIENTED_EDGE('',*,*,#44747,.F.);
#59391=ORIENTED_EDGE('',*,*,#44748,.F.);
#59392=ORIENTED_EDGE('',*,*,#44743,.F.);
#59393=ORIENTED_EDGE('',*,*,#44067,.F.);
#59394=ORIENTED_EDGE('',*,*,#44749,.F.);
#59395=ORIENTED_EDGE('',*,*,#44750,.F.);
#59396=ORIENTED_EDGE('',*,*,#44751,.F.);
#59397=ORIENTED_EDGE('',*,*,#44752,.F.);
#59398=ORIENTED_EDGE('',*,*,#44753,.F.);
#59399=ORIENTED_EDGE('',*,*,#44754,.F.);
#59400=ORIENTED_EDGE('',*,*,#44755,.F.);
#59401=ORIENTED_EDGE('',*,*,#44756,.F.);
#59402=ORIENTED_EDGE('',*,*,#44066,.F.);
#59403=ORIENTED_EDGE('',*,*,#44069,.T.);
#59404=ORIENTED_EDGE('',*,*,#44757,.T.);
#59405=ORIENTED_EDGE('',*,*,#44749,.T.);
#59406=ORIENTED_EDGE('',*,*,#44758,.F.);
#59407=ORIENTED_EDGE('',*,*,#44759,.F.);
#59408=ORIENTED_EDGE('',*,*,#44068,.F.);
#59409=ORIENTED_EDGE('',*,*,#44760,.F.);
#59410=ORIENTED_EDGE('',*,*,#44073,.F.);
#59411=ORIENTED_EDGE('',*,*,#44761,.T.);
#59412=ORIENTED_EDGE('',*,*,#44762,.T.);
#59413=ORIENTED_EDGE('',*,*,#44070,.T.);
#59414=ORIENTED_EDGE('',*,*,#44763,.F.);
#59415=ORIENTED_EDGE('',*,*,#44764,.F.);
#59416=ORIENTED_EDGE('',*,*,#44765,.F.);
#59417=ORIENTED_EDGE('',*,*,#44766,.F.);
#59418=ORIENTED_EDGE('',*,*,#44767,.F.);
#59419=ORIENTED_EDGE('',*,*,#44768,.F.);
#59420=ORIENTED_EDGE('',*,*,#44769,.F.);
#59421=ORIENTED_EDGE('',*,*,#44770,.F.);
#59422=ORIENTED_EDGE('',*,*,#44771,.F.);
#59423=ORIENTED_EDGE('',*,*,#44772,.F.);
#59424=ORIENTED_EDGE('',*,*,#44773,.F.);
#59425=ORIENTED_EDGE('',*,*,#44774,.F.);
#59426=ORIENTED_EDGE('',*,*,#44761,.F.);
#59427=ORIENTED_EDGE('',*,*,#44072,.F.);
#59428=ORIENTED_EDGE('',*,*,#44775,.T.);
#59429=ORIENTED_EDGE('',*,*,#44776,.T.);
#59430=ORIENTED_EDGE('',*,*,#44763,.T.);
#59431=ORIENTED_EDGE('',*,*,#44075,.F.);
#59432=ORIENTED_EDGE('',*,*,#44777,.F.);
#59433=ORIENTED_EDGE('',*,*,#44778,.F.);
#59434=ORIENTED_EDGE('',*,*,#44775,.F.);
#59435=ORIENTED_EDGE('',*,*,#44077,.F.);
#59436=ORIENTED_EDGE('',*,*,#44779,.T.);
#59437=ORIENTED_EDGE('',*,*,#44780,.F.);
#59438=ORIENTED_EDGE('',*,*,#44777,.T.);
#59439=ORIENTED_EDGE('',*,*,#44079,.F.);
#59440=ORIENTED_EDGE('',*,*,#44781,.F.);
#59441=ORIENTED_EDGE('',*,*,#44782,.T.);
#59442=ORIENTED_EDGE('',*,*,#44080,.T.);
#59443=ORIENTED_EDGE('',*,*,#44083,.T.);
#59444=ORIENTED_EDGE('',*,*,#44782,.F.);
#59445=ORIENTED_EDGE('',*,*,#44783,.F.);
#59446=ORIENTED_EDGE('',*,*,#44784,.F.);
#59447=ORIENTED_EDGE('',*,*,#44785,.F.);
#59448=ORIENTED_EDGE('',*,*,#44786,.F.);
#59449=ORIENTED_EDGE('',*,*,#44787,.F.);
#59450=ORIENTED_EDGE('',*,*,#44788,.F.);
#59451=ORIENTED_EDGE('',*,*,#44789,.F.);
#59452=ORIENTED_EDGE('',*,*,#44790,.F.);
#59453=ORIENTED_EDGE('',*,*,#44791,.F.);
#59454=ORIENTED_EDGE('',*,*,#44792,.F.);
#59455=ORIENTED_EDGE('',*,*,#44779,.F.);
#59456=ORIENTED_EDGE('',*,*,#44081,.F.);
#59457=ORIENTED_EDGE('',*,*,#44793,.F.);
#59458=ORIENTED_EDGE('',*,*,#44794,.F.);
#59459=ORIENTED_EDGE('',*,*,#44082,.F.);
#59460=ORIENTED_EDGE('',*,*,#44795,.F.);
#59461=ORIENTED_EDGE('',*,*,#44796,.F.);
#59462=ORIENTED_EDGE('',*,*,#44084,.T.);
#59463=ORIENTED_EDGE('',*,*,#44085,.T.);
#59464=ORIENTED_EDGE('',*,*,#44797,.T.);
#59465=ORIENTED_EDGE('',*,*,#44798,.F.);
#59466=ORIENTED_EDGE('',*,*,#44799,.F.);
#59467=ORIENTED_EDGE('',*,*,#44800,.F.);
#59468=ORIENTED_EDGE('',*,*,#44801,.F.);
#59469=ORIENTED_EDGE('',*,*,#44802,.F.);
#59470=ORIENTED_EDGE('',*,*,#44803,.F.);
#59471=ORIENTED_EDGE('',*,*,#44804,.F.);
#59472=ORIENTED_EDGE('',*,*,#44805,.F.);
#59473=ORIENTED_EDGE('',*,*,#44806,.F.);
#59474=ORIENTED_EDGE('',*,*,#44807,.F.);
#59475=ORIENTED_EDGE('',*,*,#44797,.F.);
#59476=ORIENTED_EDGE('',*,*,#44087,.F.);
#59477=ORIENTED_EDGE('',*,*,#44808,.T.);
#59478=ORIENTED_EDGE('',*,*,#44809,.T.);
#59479=ORIENTED_EDGE('',*,*,#44798,.T.);
#59480=ORIENTED_EDGE('',*,*,#44089,.F.);
#59481=ORIENTED_EDGE('',*,*,#44810,.F.);
#59482=ORIENTED_EDGE('',*,*,#44811,.T.);
#59483=ORIENTED_EDGE('',*,*,#44808,.F.);
#59484=ORIENTED_EDGE('',*,*,#44091,.F.);
#59485=ORIENTED_EDGE('',*,*,#44812,.T.);
#59486=ORIENTED_EDGE('',*,*,#44813,.F.);
#59487=ORIENTED_EDGE('',*,*,#44810,.T.);
#59488=ORIENTED_EDGE('',*,*,#44093,.F.);
#59489=ORIENTED_EDGE('',*,*,#44814,.F.);
#59490=ORIENTED_EDGE('',*,*,#44815,.T.);
#59491=ORIENTED_EDGE('',*,*,#44094,.T.);
#59492=ORIENTED_EDGE('',*,*,#44097,.T.);
#59493=ORIENTED_EDGE('',*,*,#44816,.F.);
#59494=ORIENTED_EDGE('',*,*,#44817,.F.);
#59495=ORIENTED_EDGE('',*,*,#44812,.F.);
#59496=ORIENTED_EDGE('',*,*,#44095,.F.);
#59497=ORIENTED_EDGE('',*,*,#44815,.F.);
#59498=ORIENTED_EDGE('',*,*,#44818,.F.);
#59499=ORIENTED_EDGE('',*,*,#44819,.F.);
#59500=ORIENTED_EDGE('',*,*,#44820,.F.);
#59501=ORIENTED_EDGE('',*,*,#44821,.F.);
#59502=ORIENTED_EDGE('',*,*,#44822,.F.);
#59503=ORIENTED_EDGE('',*,*,#44823,.F.);
#59504=ORIENTED_EDGE('',*,*,#44824,.F.);
#59505=ORIENTED_EDGE('',*,*,#44825,.F.);
#59506=ORIENTED_EDGE('',*,*,#44826,.F.);
#59507=ORIENTED_EDGE('',*,*,#44096,.F.);
#59508=ORIENTED_EDGE('',*,*,#44827,.F.);
#59509=ORIENTED_EDGE('',*,*,#44828,.F.);
#59510=ORIENTED_EDGE('',*,*,#44098,.T.);
#59511=ORIENTED_EDGE('',*,*,#44099,.T.);
#59512=ORIENTED_EDGE('',*,*,#44829,.T.);
#59513=ORIENTED_EDGE('',*,*,#44830,.F.);
#59514=ORIENTED_EDGE('',*,*,#44831,.F.);
#59515=ORIENTED_EDGE('',*,*,#44832,.F.);
#59516=ORIENTED_EDGE('',*,*,#44833,.F.);
#59517=ORIENTED_EDGE('',*,*,#44834,.F.);
#59518=ORIENTED_EDGE('',*,*,#44835,.F.);
#59519=ORIENTED_EDGE('',*,*,#44836,.F.);
#59520=ORIENTED_EDGE('',*,*,#44837,.F.);
#59521=ORIENTED_EDGE('',*,*,#44838,.F.);
#59522=ORIENTED_EDGE('',*,*,#44839,.F.);
#59523=ORIENTED_EDGE('',*,*,#44829,.F.);
#59524=ORIENTED_EDGE('',*,*,#44101,.F.);
#59525=ORIENTED_EDGE('',*,*,#44840,.T.);
#59526=ORIENTED_EDGE('',*,*,#44841,.T.);
#59527=ORIENTED_EDGE('',*,*,#44830,.T.);
#59528=ORIENTED_EDGE('',*,*,#44103,.F.);
#59529=ORIENTED_EDGE('',*,*,#44842,.F.);
#59530=ORIENTED_EDGE('',*,*,#44843,.T.);
#59531=ORIENTED_EDGE('',*,*,#44840,.F.);
#59532=ORIENTED_EDGE('',*,*,#44105,.F.);
#59533=ORIENTED_EDGE('',*,*,#44844,.T.);
#59534=ORIENTED_EDGE('',*,*,#44845,.T.);
#59535=ORIENTED_EDGE('',*,*,#44842,.T.);
#59536=ORIENTED_EDGE('',*,*,#44107,.F.);
#59537=ORIENTED_EDGE('',*,*,#44846,.F.);
#59538=ORIENTED_EDGE('',*,*,#44847,.T.);
#59539=ORIENTED_EDGE('',*,*,#44108,.T.);
#59540=ORIENTED_EDGE('',*,*,#44111,.T.);
#59541=ORIENTED_EDGE('',*,*,#44847,.F.);
#59542=ORIENTED_EDGE('',*,*,#44848,.F.);
#59543=ORIENTED_EDGE('',*,*,#44849,.F.);
#59544=ORIENTED_EDGE('',*,*,#44850,.F.);
#59545=ORIENTED_EDGE('',*,*,#44851,.F.);
#59546=ORIENTED_EDGE('',*,*,#44852,.F.);
#59547=ORIENTED_EDGE('',*,*,#44853,.F.);
#59548=ORIENTED_EDGE('',*,*,#44854,.F.);
#59549=ORIENTED_EDGE('',*,*,#44855,.F.);
#59550=ORIENTED_EDGE('',*,*,#44856,.F.);
#59551=ORIENTED_EDGE('',*,*,#44844,.F.);
#59552=ORIENTED_EDGE('',*,*,#44109,.F.);
#59553=ORIENTED_EDGE('',*,*,#44857,.F.);
#59554=ORIENTED_EDGE('',*,*,#44858,.F.);
#59555=ORIENTED_EDGE('',*,*,#44110,.F.);
#59556=ORIENTED_EDGE('',*,*,#44859,.F.);
#59557=ORIENTED_EDGE('',*,*,#44860,.F.);
#59558=ORIENTED_EDGE('',*,*,#44112,.T.);
#59559=ORIENTED_EDGE('',*,*,#44113,.T.);
#59560=ORIENTED_EDGE('',*,*,#44861,.T.);
#59561=ORIENTED_EDGE('',*,*,#44862,.F.);
#59562=ORIENTED_EDGE('',*,*,#44863,.F.);
#59563=ORIENTED_EDGE('',*,*,#44864,.F.);
#59564=ORIENTED_EDGE('',*,*,#44865,.F.);
#59565=ORIENTED_EDGE('',*,*,#44866,.F.);
#59566=ORIENTED_EDGE('',*,*,#44867,.F.);
#59567=ORIENTED_EDGE('',*,*,#44868,.F.);
#59568=ORIENTED_EDGE('',*,*,#44869,.F.);
#59569=ORIENTED_EDGE('',*,*,#44870,.F.);
#59570=ORIENTED_EDGE('',*,*,#44871,.F.);
#59571=ORIENTED_EDGE('',*,*,#44861,.F.);
#59572=ORIENTED_EDGE('',*,*,#44115,.F.);
#59573=ORIENTED_EDGE('',*,*,#44872,.T.);
#59574=ORIENTED_EDGE('',*,*,#44873,.T.);
#59575=ORIENTED_EDGE('',*,*,#44862,.T.);
#59576=ORIENTED_EDGE('',*,*,#44117,.F.);
#59577=ORIENTED_EDGE('',*,*,#44874,.F.);
#59578=ORIENTED_EDGE('',*,*,#44875,.T.);
#59579=ORIENTED_EDGE('',*,*,#44872,.F.);
#59580=ORIENTED_EDGE('',*,*,#44119,.F.);
#59581=ORIENTED_EDGE('',*,*,#44876,.T.);
#59582=ORIENTED_EDGE('',*,*,#44877,.T.);
#59583=ORIENTED_EDGE('',*,*,#44874,.T.);
#59584=ORIENTED_EDGE('',*,*,#44121,.F.);
#59585=ORIENTED_EDGE('',*,*,#44878,.F.);
#59586=ORIENTED_EDGE('',*,*,#44879,.T.);
#59587=ORIENTED_EDGE('',*,*,#44122,.T.);
#59588=ORIENTED_EDGE('',*,*,#44125,.T.);
#59589=ORIENTED_EDGE('',*,*,#44879,.F.);
#59590=ORIENTED_EDGE('',*,*,#44880,.F.);
#59591=ORIENTED_EDGE('',*,*,#44881,.F.);
#59592=ORIENTED_EDGE('',*,*,#44882,.F.);
#59593=ORIENTED_EDGE('',*,*,#44883,.F.);
#59594=ORIENTED_EDGE('',*,*,#44884,.F.);
#59595=ORIENTED_EDGE('',*,*,#44885,.F.);
#59596=ORIENTED_EDGE('',*,*,#44886,.F.);
#59597=ORIENTED_EDGE('',*,*,#44887,.F.);
#59598=ORIENTED_EDGE('',*,*,#44888,.F.);
#59599=ORIENTED_EDGE('',*,*,#44876,.F.);
#59600=ORIENTED_EDGE('',*,*,#44123,.F.);
#59601=ORIENTED_EDGE('',*,*,#44889,.F.);
#59602=ORIENTED_EDGE('',*,*,#44890,.F.);
#59603=ORIENTED_EDGE('',*,*,#44124,.F.);
#59604=ORIENTED_EDGE('',*,*,#44891,.F.);
#59605=ORIENTED_EDGE('',*,*,#44129,.F.);
#59606=ORIENTED_EDGE('',*,*,#44892,.T.);
#59607=ORIENTED_EDGE('',*,*,#44893,.T.);
#59608=ORIENTED_EDGE('',*,*,#44126,.T.);
#59609=ORIENTED_EDGE('',*,*,#44894,.F.);
#59610=ORIENTED_EDGE('',*,*,#44895,.F.);
#59611=ORIENTED_EDGE('',*,*,#44896,.F.);
#59612=ORIENTED_EDGE('',*,*,#44897,.F.);
#59613=ORIENTED_EDGE('',*,*,#44898,.F.);
#59614=ORIENTED_EDGE('',*,*,#44899,.F.);
#59615=ORIENTED_EDGE('',*,*,#44900,.F.);
#59616=ORIENTED_EDGE('',*,*,#44901,.F.);
#59617=ORIENTED_EDGE('',*,*,#44902,.F.);
#59618=ORIENTED_EDGE('',*,*,#44903,.F.);
#59619=ORIENTED_EDGE('',*,*,#44904,.F.);
#59620=ORIENTED_EDGE('',*,*,#44892,.F.);
#59621=ORIENTED_EDGE('',*,*,#44128,.F.);
#59622=ORIENTED_EDGE('',*,*,#44905,.T.);
#59623=ORIENTED_EDGE('',*,*,#44906,.T.);
#59624=ORIENTED_EDGE('',*,*,#44894,.T.);
#59625=ORIENTED_EDGE('',*,*,#44131,.F.);
#59626=ORIENTED_EDGE('',*,*,#44907,.F.);
#59627=ORIENTED_EDGE('',*,*,#44908,.F.);
#59628=ORIENTED_EDGE('',*,*,#44905,.F.);
#59629=ORIENTED_EDGE('',*,*,#44133,.F.);
#59630=ORIENTED_EDGE('',*,*,#44909,.T.);
#59631=ORIENTED_EDGE('',*,*,#44910,.F.);
#59632=ORIENTED_EDGE('',*,*,#44907,.T.);
#59633=ORIENTED_EDGE('',*,*,#44135,.F.);
#59634=ORIENTED_EDGE('',*,*,#44911,.F.);
#59635=ORIENTED_EDGE('',*,*,#44912,.T.);
#59636=ORIENTED_EDGE('',*,*,#44136,.T.);
#59637=ORIENTED_EDGE('',*,*,#44139,.T.);
#59638=ORIENTED_EDGE('',*,*,#44912,.F.);
#59639=ORIENTED_EDGE('',*,*,#44913,.F.);
#59640=ORIENTED_EDGE('',*,*,#44914,.F.);
#59641=ORIENTED_EDGE('',*,*,#44915,.F.);
#59642=ORIENTED_EDGE('',*,*,#44916,.F.);
#59643=ORIENTED_EDGE('',*,*,#44917,.F.);
#59644=ORIENTED_EDGE('',*,*,#44918,.F.);
#59645=ORIENTED_EDGE('',*,*,#44919,.F.);
#59646=ORIENTED_EDGE('',*,*,#44920,.F.);
#59647=ORIENTED_EDGE('',*,*,#44921,.F.);
#59648=ORIENTED_EDGE('',*,*,#44922,.F.);
#59649=ORIENTED_EDGE('',*,*,#44923,.F.);
#59650=ORIENTED_EDGE('',*,*,#44909,.F.);
#59651=ORIENTED_EDGE('',*,*,#44137,.F.);
#59652=ORIENTED_EDGE('',*,*,#44924,.F.);
#59653=ORIENTED_EDGE('',*,*,#44925,.F.);
#59654=ORIENTED_EDGE('',*,*,#44138,.F.);
#59655=ORIENTED_EDGE('',*,*,#44926,.F.);
#59656=ORIENTED_EDGE('',*,*,#44143,.F.);
#59657=ORIENTED_EDGE('',*,*,#44927,.T.);
#59658=ORIENTED_EDGE('',*,*,#44928,.T.);
#59659=ORIENTED_EDGE('',*,*,#44140,.T.);
#59660=ORIENTED_EDGE('',*,*,#44929,.F.);
#59661=ORIENTED_EDGE('',*,*,#44930,.F.);
#59662=ORIENTED_EDGE('',*,*,#44931,.F.);
#59663=ORIENTED_EDGE('',*,*,#44932,.F.);
#59664=ORIENTED_EDGE('',*,*,#44933,.F.);
#59665=ORIENTED_EDGE('',*,*,#44934,.F.);
#59666=ORIENTED_EDGE('',*,*,#44927,.F.);
#59667=ORIENTED_EDGE('',*,*,#44142,.F.);
#59668=ORIENTED_EDGE('',*,*,#44733,.F.);
#59669=ORIENTED_EDGE('',*,*,#44935,.F.);
#59670=ORIENTED_EDGE('',*,*,#44936,.F.);
#59671=ORIENTED_EDGE('',*,*,#44937,.F.);
#59672=ORIENTED_EDGE('',*,*,#44938,.F.);
#59673=ORIENTED_EDGE('',*,*,#44939,.F.);
#59674=ORIENTED_EDGE('',*,*,#44940,.F.);
#59675=ORIENTED_EDGE('',*,*,#44941,.F.);
#59676=ORIENTED_EDGE('',*,*,#44942,.F.);
#59677=ORIENTED_EDGE('',*,*,#44145,.F.);
#59678=ORIENTED_EDGE('',*,*,#44943,.F.);
#59679=ORIENTED_EDGE('',*,*,#44944,.F.);
#59680=ORIENTED_EDGE('',*,*,#44147,.T.);
#59681=ORIENTED_EDGE('',*,*,#44148,.T.);
#59682=ORIENTED_EDGE('',*,*,#44945,.T.);
#59683=ORIENTED_EDGE('',*,*,#44946,.F.);
#59684=ORIENTED_EDGE('',*,*,#44947,.T.);
#59685=ORIENTED_EDGE('',*,*,#44179,.T.);
#59686=ORIENTED_EDGE('',*,*,#44146,.T.);
#59687=ORIENTED_EDGE('',*,*,#44948,.F.);
#59688=ORIENTED_EDGE('',*,*,#44949,.F.);
#59689=ORIENTED_EDGE('',*,*,#44950,.F.);
#59690=ORIENTED_EDGE('',*,*,#44951,.F.);
#59691=ORIENTED_EDGE('',*,*,#44952,.F.);
#59692=ORIENTED_EDGE('',*,*,#44953,.F.);
#59693=ORIENTED_EDGE('',*,*,#44954,.F.);
#59694=ORIENTED_EDGE('',*,*,#44955,.F.);
#59695=ORIENTED_EDGE('',*,*,#44956,.F.);
#59696=ORIENTED_EDGE('',*,*,#44945,.F.);
#59697=ORIENTED_EDGE('',*,*,#44150,.F.);
#59698=ORIENTED_EDGE('',*,*,#44957,.F.);
#59699=ORIENTED_EDGE('',*,*,#44958,.F.);
#59700=ORIENTED_EDGE('',*,*,#44959,.F.);
#59701=ORIENTED_EDGE('',*,*,#44960,.F.);
#59702=ORIENTED_EDGE('',*,*,#44961,.F.);
#59703=ORIENTED_EDGE('',*,*,#44962,.F.);
#59704=ORIENTED_EDGE('',*,*,#44963,.T.);
#59705=ORIENTED_EDGE('',*,*,#44964,.T.);
#59706=ORIENTED_EDGE('',*,*,#44957,.T.);
#59707=ORIENTED_EDGE('',*,*,#44152,.F.);
#59708=ORIENTED_EDGE('',*,*,#44965,.F.);
#59709=ORIENTED_EDGE('',*,*,#44966,.F.);
#59710=ORIENTED_EDGE('',*,*,#44963,.F.);
#59711=ORIENTED_EDGE('',*,*,#44154,.F.);
#59712=ORIENTED_EDGE('',*,*,#44967,.T.);
#59713=ORIENTED_EDGE('',*,*,#44968,.T.);
#59714=ORIENTED_EDGE('',*,*,#44965,.T.);
#59715=ORIENTED_EDGE('',*,*,#44156,.F.);
#59716=ORIENTED_EDGE('',*,*,#44969,.F.);
#59717=ORIENTED_EDGE('',*,*,#44970,.F.);
#59718=ORIENTED_EDGE('',*,*,#44971,.F.);
#59719=ORIENTED_EDGE('',*,*,#44972,.F.);
#59720=ORIENTED_EDGE('',*,*,#44973,.F.);
#59721=ORIENTED_EDGE('',*,*,#44974,.F.);
#59722=ORIENTED_EDGE('',*,*,#44975,.F.);
#59723=ORIENTED_EDGE('',*,*,#44976,.F.);
#59724=ORIENTED_EDGE('',*,*,#44967,.F.);
#59725=ORIENTED_EDGE('',*,*,#44158,.F.);
#59726=ORIENTED_EDGE('',*,*,#44977,.F.);
#59727=ORIENTED_EDGE('',*,*,#44978,.F.);
#59728=ORIENTED_EDGE('',*,*,#44979,.F.);
#59729=ORIENTED_EDGE('',*,*,#44980,.F.);
#59730=ORIENTED_EDGE('',*,*,#44981,.F.);
#59731=ORIENTED_EDGE('',*,*,#44982,.F.);
#59732=ORIENTED_EDGE('',*,*,#44157,.F.);
#59733=ORIENTED_EDGE('',*,*,#44160,.T.);
#59734=ORIENTED_EDGE('',*,*,#44983,.T.);
#59735=ORIENTED_EDGE('',*,*,#44977,.T.);
#59736=ORIENTED_EDGE('',*,*,#44984,.F.);
#59737=ORIENTED_EDGE('',*,*,#44985,.T.);
#59738=ORIENTED_EDGE('',*,*,#44163,.T.);
#59739=ORIENTED_EDGE('',*,*,#44167,.T.);
#59740=ORIENTED_EDGE('',*,*,#44986,.F.);
#59741=ORIENTED_EDGE('',*,*,#44987,.F.);
#59742=ORIENTED_EDGE('',*,*,#44988,.F.);
#59743=ORIENTED_EDGE('',*,*,#44989,.F.);
#59744=ORIENTED_EDGE('',*,*,#44303,.F.);
#59745=ORIENTED_EDGE('',*,*,#44164,.F.);
#59746=ORIENTED_EDGE('',*,*,#44985,.F.);
#59747=ORIENTED_EDGE('',*,*,#44990,.F.);
#59748=ORIENTED_EDGE('',*,*,#44991,.F.);
#59749=ORIENTED_EDGE('',*,*,#44992,.F.);
#59750=ORIENTED_EDGE('',*,*,#44993,.F.);
#59751=ORIENTED_EDGE('',*,*,#44994,.F.);
#59752=ORIENTED_EDGE('',*,*,#44995,.F.);
#59753=ORIENTED_EDGE('',*,*,#44996,.F.);
#59754=ORIENTED_EDGE('',*,*,#44997,.F.);
#59755=ORIENTED_EDGE('',*,*,#44998,.F.);
#59756=ORIENTED_EDGE('',*,*,#44999,.T.);
#59757=ORIENTED_EDGE('',*,*,#45000,.F.);
#59758=ORIENTED_EDGE('',*,*,#44166,.F.);
#59759=ORIENTED_EDGE('',*,*,#45001,.T.);
#59760=ORIENTED_EDGE('',*,*,#45002,.F.);
#59761=ORIENTED_EDGE('',*,*,#45001,.F.);
#59762=ORIENTED_EDGE('',*,*,#44168,.F.);
#59763=ORIENTED_EDGE('',*,*,#45003,.F.);
#59764=ORIENTED_EDGE('',*,*,#45004,.F.);
#59765=ORIENTED_EDGE('',*,*,#44169,.T.);
#59766=ORIENTED_EDGE('',*,*,#44170,.T.);
#59767=ORIENTED_EDGE('',*,*,#45005,.T.);
#59768=ORIENTED_EDGE('',*,*,#45006,.F.);
#59769=ORIENTED_EDGE('',*,*,#45007,.F.);
#59770=ORIENTED_EDGE('',*,*,#45008,.F.);
#59771=ORIENTED_EDGE('',*,*,#45009,.F.);
#59772=ORIENTED_EDGE('',*,*,#45010,.F.);
#59773=ORIENTED_EDGE('',*,*,#45011,.F.);
#59774=ORIENTED_EDGE('',*,*,#45012,.F.);
#59775=ORIENTED_EDGE('',*,*,#45013,.F.);
#59776=ORIENTED_EDGE('',*,*,#45014,.F.);
#59777=ORIENTED_EDGE('',*,*,#45015,.F.);
#59778=ORIENTED_EDGE('',*,*,#45016,.F.);
#59779=ORIENTED_EDGE('',*,*,#45017,.F.);
#59780=ORIENTED_EDGE('',*,*,#45018,.F.);
#59781=ORIENTED_EDGE('',*,*,#45019,.F.);
#59782=ORIENTED_EDGE('',*,*,#45020,.F.);
#59783=ORIENTED_EDGE('',*,*,#45021,.F.);
#59784=ORIENTED_EDGE('',*,*,#45005,.F.);
#59785=ORIENTED_EDGE('',*,*,#44172,.F.);
#59786=ORIENTED_EDGE('',*,*,#45022,.T.);
#59787=ORIENTED_EDGE('',*,*,#45023,.T.);
#59788=ORIENTED_EDGE('',*,*,#45006,.T.);
#59789=ORIENTED_EDGE('',*,*,#44174,.F.);
#59790=ORIENTED_EDGE('',*,*,#45024,.F.);
#59791=ORIENTED_EDGE('',*,*,#45025,.F.);
#59792=ORIENTED_EDGE('',*,*,#45022,.F.);
#59793=ORIENTED_EDGE('',*,*,#44176,.F.);
#59794=ORIENTED_EDGE('',*,*,#45026,.T.);
#59795=ORIENTED_EDGE('',*,*,#45027,.F.);
#59796=ORIENTED_EDGE('',*,*,#45024,.T.);
#59797=ORIENTED_EDGE('',*,*,#44178,.F.);
#59798=ORIENTED_EDGE('',*,*,#45028,.F.);
#59799=ORIENTED_EDGE('',*,*,#45029,.F.);
#59800=ORIENTED_EDGE('',*,*,#45030,.F.);
#59801=ORIENTED_EDGE('',*,*,#45031,.F.);
#59802=ORIENTED_EDGE('',*,*,#45026,.F.);
#59803=ORIENTED_EDGE('',*,*,#44180,.F.);
#59804=ORIENTED_EDGE('',*,*,#44947,.F.);
#59805=ORIENTED_EDGE('',*,*,#45032,.F.);
#59806=ORIENTED_EDGE('',*,*,#45033,.F.);
#59807=ORIENTED_EDGE('',*,*,#45034,.F.);
#59808=ORIENTED_EDGE('',*,*,#45035,.F.);
#59809=ORIENTED_EDGE('',*,*,#45036,.F.);
#59810=ORIENTED_EDGE('',*,*,#45037,.F.);
#59811=ORIENTED_EDGE('',*,*,#45038,.F.);
#59812=ORIENTED_EDGE('',*,*,#45039,.F.);
#59813=ORIENTED_EDGE('',*,*,#45040,.F.);
#59814=ORIENTED_EDGE('',*,*,#45041,.F.);
#59815=ORIENTED_EDGE('',*,*,#45042,.F.);
#59816=ORIENTED_EDGE('',*,*,#45043,.F.);
#59817=ORIENTED_EDGE('',*,*,#45044,.F.);
#59818=ORIENTED_EDGE('',*,*,#44184,.F.);
#59819=ORIENTED_EDGE('',*,*,#45045,.F.);
#59820=ORIENTED_EDGE('',*,*,#44189,.F.);
#59821=ORIENTED_EDGE('',*,*,#45046,.T.);
#59822=ORIENTED_EDGE('',*,*,#45047,.T.);
#59823=ORIENTED_EDGE('',*,*,#44186,.T.);
#59824=ORIENTED_EDGE('',*,*,#44211,.F.);
#59825=ORIENTED_EDGE('',*,*,#44185,.T.);
#59826=ORIENTED_EDGE('',*,*,#45048,.T.);
#59827=ORIENTED_EDGE('',*,*,#45049,.T.);
#59828=ORIENTED_EDGE('',*,*,#45050,.F.);
#59829=ORIENTED_EDGE('',*,*,#45051,.F.);
#59830=ORIENTED_EDGE('',*,*,#45052,.F.);
#59831=ORIENTED_EDGE('',*,*,#44413,.F.);
#59832=ORIENTED_EDGE('',*,*,#45053,.F.);
#59833=ORIENTED_EDGE('',*,*,#45054,.F.);
#59834=ORIENTED_EDGE('',*,*,#45055,.F.);
#59835=ORIENTED_EDGE('',*,*,#45056,.F.);
#59836=ORIENTED_EDGE('',*,*,#45057,.F.);
#59837=ORIENTED_EDGE('',*,*,#45058,.F.);
#59838=ORIENTED_EDGE('',*,*,#45046,.F.);
#59839=ORIENTED_EDGE('',*,*,#44188,.F.);
#59840=ORIENTED_EDGE('',*,*,#45059,.T.);
#59841=ORIENTED_EDGE('',*,*,#45060,.T.);
#59842=ORIENTED_EDGE('',*,*,#45050,.T.);
#59843=ORIENTED_EDGE('',*,*,#44191,.F.);
#59844=ORIENTED_EDGE('',*,*,#45061,.F.);
#59845=ORIENTED_EDGE('',*,*,#45062,.F.);
#59846=ORIENTED_EDGE('',*,*,#45059,.F.);
#59847=ORIENTED_EDGE('',*,*,#44193,.F.);
#59848=ORIENTED_EDGE('',*,*,#45063,.T.);
#59849=ORIENTED_EDGE('',*,*,#45064,.F.);
#59850=ORIENTED_EDGE('',*,*,#45061,.T.);
#59851=ORIENTED_EDGE('',*,*,#44195,.F.);
#59852=ORIENTED_EDGE('',*,*,#45065,.F.);
#59853=ORIENTED_EDGE('',*,*,#45066,.F.);
#59854=ORIENTED_EDGE('',*,*,#45067,.F.);
#59855=ORIENTED_EDGE('',*,*,#45068,.F.);
#59856=ORIENTED_EDGE('',*,*,#45069,.F.);
#59857=ORIENTED_EDGE('',*,*,#45070,.F.);
#59858=ORIENTED_EDGE('',*,*,#44401,.F.);
#59859=ORIENTED_EDGE('',*,*,#45071,.F.);
#59860=ORIENTED_EDGE('',*,*,#45072,.F.);
#59861=ORIENTED_EDGE('',*,*,#45063,.F.);
#59862=ORIENTED_EDGE('',*,*,#44197,.F.);
#59863=ORIENTED_EDGE('',*,*,#44196,.F.);
#59864=ORIENTED_EDGE('',*,*,#44199,.T.);
#59865=ORIENTED_EDGE('',*,*,#45073,.T.);
#59866=ORIENTED_EDGE('',*,*,#45065,.T.);
#59867=ORIENTED_EDGE('',*,*,#45074,.F.);
#59868=ORIENTED_EDGE('',*,*,#44201,.T.);
#59869=ORIENTED_EDGE('',*,*,#44202,.T.);
#59870=ORIENTED_EDGE('',*,*,#45075,.T.);
#59871=ORIENTED_EDGE('',*,*,#45076,.F.);
#59872=ORIENTED_EDGE('',*,*,#45077,.F.);
#59873=ORIENTED_EDGE('',*,*,#45075,.F.);
#59874=ORIENTED_EDGE('',*,*,#44204,.F.);
#59875=ORIENTED_EDGE('',*,*,#45078,.F.);
#59876=ORIENTED_EDGE('',*,*,#45079,.F.);
#59877=ORIENTED_EDGE('',*,*,#45080,.F.);
#59878=ORIENTED_EDGE('',*,*,#45081,.F.);
#59879=ORIENTED_EDGE('',*,*,#45082,.T.);
#59880=ORIENTED_EDGE('',*,*,#45083,.T.);
#59881=ORIENTED_EDGE('',*,*,#45078,.T.);
#59882=ORIENTED_EDGE('',*,*,#44206,.F.);
#59883=ORIENTED_EDGE('',*,*,#45084,.F.);
#59884=ORIENTED_EDGE('',*,*,#45085,.F.);
#59885=ORIENTED_EDGE('',*,*,#45082,.F.);
#59886=ORIENTED_EDGE('',*,*,#44208,.F.);
#59887=ORIENTED_EDGE('',*,*,#45086,.T.);
#59888=ORIENTED_EDGE('',*,*,#45087,.F.);
#59889=ORIENTED_EDGE('',*,*,#45084,.T.);
#59890=ORIENTED_EDGE('',*,*,#44210,.F.);
#59891=ORIENTED_EDGE('',*,*,#45088,.F.);
#59892=ORIENTED_EDGE('',*,*,#45089,.F.);
#59893=ORIENTED_EDGE('',*,*,#45086,.F.);
#59894=ORIENTED_EDGE('',*,*,#44212,.F.);
#59895=ORIENTED_EDGE('',*,*,#45049,.F.);
#59896=ORIENTED_EDGE('',*,*,#45090,.F.);
#59897=ORIENTED_EDGE('',*,*,#45091,.F.);
#59898=ORIENTED_EDGE('',*,*,#45092,.F.);
#59899=ORIENTED_EDGE('',*,*,#45093,.F.);
#59900=ORIENTED_EDGE('',*,*,#45094,.F.);
#59901=ORIENTED_EDGE('',*,*,#45095,.F.);
#59902=ORIENTED_EDGE('',*,*,#44420,.F.);
#59903=ORIENTED_EDGE('',*,*,#45096,.F.);
#59904=ORIENTED_EDGE('',*,*,#45097,.F.);
#59905=ORIENTED_EDGE('',*,*,#44214,.F.);
#59906=ORIENTED_EDGE('',*,*,#45098,.F.);
#59907=ORIENTED_EDGE('',*,*,#44219,.F.);
#59908=ORIENTED_EDGE('',*,*,#45099,.T.);
#59909=ORIENTED_EDGE('',*,*,#45100,.T.);
#59910=ORIENTED_EDGE('',*,*,#44216,.T.);
#59911=ORIENTED_EDGE('',*,*,#45101,.F.);
#59912=ORIENTED_EDGE('',*,*,#45102,.T.);
#59913=ORIENTED_EDGE('',*,*,#44249,.T.);
#59914=ORIENTED_EDGE('',*,*,#44215,.T.);
#59915=ORIENTED_EDGE('',*,*,#45103,.F.);
#59916=ORIENTED_EDGE('',*,*,#45104,.F.);
#59917=ORIENTED_EDGE('',*,*,#45105,.F.);
#59918=ORIENTED_EDGE('',*,*,#45106,.F.);
#59919=ORIENTED_EDGE('',*,*,#45107,.F.);
#59920=ORIENTED_EDGE('',*,*,#45108,.F.);
#59921=ORIENTED_EDGE('',*,*,#45109,.F.);
#59922=ORIENTED_EDGE('',*,*,#45110,.F.);
#59923=ORIENTED_EDGE('',*,*,#45111,.F.);
#59924=ORIENTED_EDGE('',*,*,#45112,.F.);
#59925=ORIENTED_EDGE('',*,*,#45099,.F.);
#59926=ORIENTED_EDGE('',*,*,#44218,.F.);
#59927=ORIENTED_EDGE('',*,*,#45113,.F.);
#59928=ORIENTED_EDGE('',*,*,#45114,.F.);
#59929=ORIENTED_EDGE('',*,*,#45115,.F.);
#59930=ORIENTED_EDGE('',*,*,#45116,.F.);
#59931=ORIENTED_EDGE('',*,*,#45117,.F.);
#59932=ORIENTED_EDGE('',*,*,#45118,.F.);
#59933=ORIENTED_EDGE('',*,*,#45119,.T.);
#59934=ORIENTED_EDGE('',*,*,#45120,.T.);
#59935=ORIENTED_EDGE('',*,*,#45113,.T.);
#59936=ORIENTED_EDGE('',*,*,#44221,.F.);
#59937=ORIENTED_EDGE('',*,*,#45121,.F.);
#59938=ORIENTED_EDGE('',*,*,#45122,.F.);
#59939=ORIENTED_EDGE('',*,*,#45119,.F.);
#59940=ORIENTED_EDGE('',*,*,#44223,.F.);
#59941=ORIENTED_EDGE('',*,*,#45123,.T.);
#59942=ORIENTED_EDGE('',*,*,#45124,.F.);
#59943=ORIENTED_EDGE('',*,*,#45121,.T.);
#59944=ORIENTED_EDGE('',*,*,#44225,.F.);
#59945=ORIENTED_EDGE('',*,*,#45125,.F.);
#59946=ORIENTED_EDGE('',*,*,#45126,.T.);
#59947=ORIENTED_EDGE('',*,*,#44226,.T.);
#59948=ORIENTED_EDGE('',*,*,#44229,.T.);
#59949=ORIENTED_EDGE('',*,*,#45127,.F.);
#59950=ORIENTED_EDGE('',*,*,#45128,.F.);
#59951=ORIENTED_EDGE('',*,*,#45129,.F.);
#59952=ORIENTED_EDGE('',*,*,#45130,.F.);
#59953=ORIENTED_EDGE('',*,*,#45131,.F.);
#59954=ORIENTED_EDGE('',*,*,#45132,.F.);
#59955=ORIENTED_EDGE('',*,*,#45133,.F.);
#59956=ORIENTED_EDGE('',*,*,#45134,.F.);
#59957=ORIENTED_EDGE('',*,*,#45135,.F.);
#59958=ORIENTED_EDGE('',*,*,#45136,.F.);
#59959=ORIENTED_EDGE('',*,*,#45123,.F.);
#59960=ORIENTED_EDGE('',*,*,#44227,.F.);
#59961=ORIENTED_EDGE('',*,*,#45126,.F.);
#59962=ORIENTED_EDGE('',*,*,#45137,.F.);
#59963=ORIENTED_EDGE('',*,*,#45138,.F.);
#59964=ORIENTED_EDGE('',*,*,#45139,.F.);
#59965=ORIENTED_EDGE('',*,*,#45140,.F.);
#59966=ORIENTED_EDGE('',*,*,#45141,.F.);
#59967=ORIENTED_EDGE('',*,*,#45142,.F.);
#59968=ORIENTED_EDGE('',*,*,#45143,.F.);
#59969=ORIENTED_EDGE('',*,*,#45144,.F.);
#59970=ORIENTED_EDGE('',*,*,#45145,.F.);
#59971=ORIENTED_EDGE('',*,*,#44736,.F.);
#59972=ORIENTED_EDGE('',*,*,#44233,.F.);
#59973=ORIENTED_EDGE('',*,*,#45146,.F.);
#59974=ORIENTED_EDGE('',*,*,#45147,.F.);
#59975=ORIENTED_EDGE('',*,*,#45148,.F.);
#59976=ORIENTED_EDGE('',*,*,#45149,.F.);
#59977=ORIENTED_EDGE('',*,*,#45150,.F.);
#59978=ORIENTED_EDGE('',*,*,#45151,.F.);
#59979=ORIENTED_EDGE('',*,*,#45152,.F.);
#59980=ORIENTED_EDGE('',*,*,#45153,.F.);
#59981=ORIENTED_EDGE('',*,*,#45154,.F.);
#59982=ORIENTED_EDGE('',*,*,#45155,.F.);
#59983=ORIENTED_EDGE('',*,*,#45156,.F.);
#59984=ORIENTED_EDGE('',*,*,#44232,.F.);
#59985=ORIENTED_EDGE('',*,*,#44237,.T.);
#59986=ORIENTED_EDGE('',*,*,#45157,.T.);
#59987=ORIENTED_EDGE('',*,*,#45146,.T.);
#59988=ORIENTED_EDGE('',*,*,#44236,.F.);
#59989=ORIENTED_EDGE('',*,*,#45158,.T.);
#59990=ORIENTED_EDGE('',*,*,#45159,.F.);
#59991=ORIENTED_EDGE('',*,*,#45160,.T.);
#59992=ORIENTED_EDGE('',*,*,#45161,.F.);
#59993=ORIENTED_EDGE('',*,*,#45158,.F.);
#59994=ORIENTED_EDGE('',*,*,#44235,.F.);
#59995=ORIENTED_EDGE('',*,*,#45162,.T.);
#59996=ORIENTED_EDGE('',*,*,#45163,.F.);
#59997=ORIENTED_EDGE('',*,*,#45162,.F.);
#59998=ORIENTED_EDGE('',*,*,#44238,.F.);
#59999=ORIENTED_EDGE('',*,*,#45164,.F.);
#60000=ORIENTED_EDGE('',*,*,#45165,.F.);
#60001=ORIENTED_EDGE('',*,*,#44239,.T.);
#60002=ORIENTED_EDGE('',*,*,#44240,.T.);
#60003=ORIENTED_EDGE('',*,*,#45166,.T.);
#60004=ORIENTED_EDGE('',*,*,#45167,.F.);
#60005=ORIENTED_EDGE('',*,*,#45168,.F.);
#60006=ORIENTED_EDGE('',*,*,#45169,.F.);
#60007=ORIENTED_EDGE('',*,*,#45170,.F.);
#60008=ORIENTED_EDGE('',*,*,#45171,.F.);
#60009=ORIENTED_EDGE('',*,*,#45172,.F.);
#60010=ORIENTED_EDGE('',*,*,#45173,.F.);
#60011=ORIENTED_EDGE('',*,*,#45174,.F.);
#60012=ORIENTED_EDGE('',*,*,#45175,.F.);
#60013=ORIENTED_EDGE('',*,*,#45176,.F.);
#60014=ORIENTED_EDGE('',*,*,#45177,.F.);
#60015=ORIENTED_EDGE('',*,*,#45178,.F.);
#60016=ORIENTED_EDGE('',*,*,#45179,.F.);
#60017=ORIENTED_EDGE('',*,*,#45180,.F.);
#60018=ORIENTED_EDGE('',*,*,#45181,.F.);
#60019=ORIENTED_EDGE('',*,*,#45182,.F.);
#60020=ORIENTED_EDGE('',*,*,#45166,.F.);
#60021=ORIENTED_EDGE('',*,*,#44242,.F.);
#60022=ORIENTED_EDGE('',*,*,#45183,.T.);
#60023=ORIENTED_EDGE('',*,*,#45184,.T.);
#60024=ORIENTED_EDGE('',*,*,#45167,.T.);
#60025=ORIENTED_EDGE('',*,*,#44244,.F.);
#60026=ORIENTED_EDGE('',*,*,#45185,.F.);
#60027=ORIENTED_EDGE('',*,*,#45186,.F.);
#60028=ORIENTED_EDGE('',*,*,#45183,.F.);
#60029=ORIENTED_EDGE('',*,*,#44246,.F.);
#60030=ORIENTED_EDGE('',*,*,#45187,.T.);
#60031=ORIENTED_EDGE('',*,*,#45188,.F.);
#60032=ORIENTED_EDGE('',*,*,#45185,.T.);
#60033=ORIENTED_EDGE('',*,*,#44248,.F.);
#60034=ORIENTED_EDGE('',*,*,#45189,.F.);
#60035=ORIENTED_EDGE('',*,*,#45190,.F.);
#60036=ORIENTED_EDGE('',*,*,#45191,.F.);
#60037=ORIENTED_EDGE('',*,*,#45192,.F.);
#60038=ORIENTED_EDGE('',*,*,#45187,.F.);
#60039=ORIENTED_EDGE('',*,*,#44250,.F.);
#60040=ORIENTED_EDGE('',*,*,#45102,.F.);
#60041=ORIENTED_EDGE('',*,*,#45193,.F.);
#60042=ORIENTED_EDGE('',*,*,#45194,.F.);
#60043=ORIENTED_EDGE('',*,*,#45195,.F.);
#60044=ORIENTED_EDGE('',*,*,#45196,.F.);
#60045=ORIENTED_EDGE('',*,*,#45197,.F.);
#60046=ORIENTED_EDGE('',*,*,#45198,.F.);
#60047=ORIENTED_EDGE('',*,*,#45199,.F.);
#60048=ORIENTED_EDGE('',*,*,#45200,.F.);
#60049=ORIENTED_EDGE('',*,*,#45201,.F.);
#60050=ORIENTED_EDGE('',*,*,#45202,.F.);
#60051=ORIENTED_EDGE('',*,*,#45203,.F.);
#60052=ORIENTED_EDGE('',*,*,#45204,.T.);
#60053=ORIENTED_EDGE('',*,*,#45205,.F.);
#60054=ORIENTED_EDGE('',*,*,#45206,.T.);
#60055=ORIENTED_EDGE('',*,*,#44251,.F.);
#60056=ORIENTED_EDGE('',*,*,#45207,.F.);
#60057=ORIENTED_EDGE('',*,*,#44256,.F.);
#60058=ORIENTED_EDGE('',*,*,#45208,.T.);
#60059=ORIENTED_EDGE('',*,*,#45209,.T.);
#60060=ORIENTED_EDGE('',*,*,#44253,.T.);
#60061=ORIENTED_EDGE('',*,*,#45210,.F.);
#60062=ORIENTED_EDGE('',*,*,#45211,.F.);
#60063=ORIENTED_EDGE('',*,*,#45212,.F.);
#60064=ORIENTED_EDGE('',*,*,#45213,.F.);
#60065=ORIENTED_EDGE('',*,*,#45214,.F.);
#60066=ORIENTED_EDGE('',*,*,#45215,.F.);
#60067=ORIENTED_EDGE('',*,*,#45216,.F.);
#60068=ORIENTED_EDGE('',*,*,#45217,.F.);
#60069=ORIENTED_EDGE('',*,*,#45208,.F.);
#60070=ORIENTED_EDGE('',*,*,#44255,.F.);
#60071=ORIENTED_EDGE('',*,*,#44740,.F.);
#60072=ORIENTED_EDGE('',*,*,#45218,.F.);
#60073=ORIENTED_EDGE('',*,*,#45219,.F.);
#60074=ORIENTED_EDGE('',*,*,#45220,.F.);
#60075=ORIENTED_EDGE('',*,*,#45221,.F.);
#60076=ORIENTED_EDGE('',*,*,#45222,.F.);
#60077=ORIENTED_EDGE('',*,*,#45223,.F.);
#60078=ORIENTED_EDGE('',*,*,#44259,.T.);
#60079=ORIENTED_EDGE('',*,*,#44260,.T.);
#60080=ORIENTED_EDGE('',*,*,#45224,.T.);
#60081=ORIENTED_EDGE('',*,*,#45225,.F.);
#60082=ORIENTED_EDGE('',*,*,#45226,.F.);
#60083=ORIENTED_EDGE('',*,*,#45227,.F.);
#60084=ORIENTED_EDGE('',*,*,#45228,.F.);
#60085=ORIENTED_EDGE('',*,*,#45229,.F.);
#60086=ORIENTED_EDGE('',*,*,#45230,.F.);
#60087=ORIENTED_EDGE('',*,*,#45231,.F.);
#60088=ORIENTED_EDGE('',*,*,#45232,.F.);
#60089=ORIENTED_EDGE('',*,*,#45224,.F.);
#60090=ORIENTED_EDGE('',*,*,#44262,.F.);
#60091=ORIENTED_EDGE('',*,*,#45233,.F.);
#60092=ORIENTED_EDGE('',*,*,#45234,.F.);
#60093=ORIENTED_EDGE('',*,*,#45235,.F.);
#60094=ORIENTED_EDGE('',*,*,#45236,.F.);
#60095=ORIENTED_EDGE('',*,*,#45237,.F.);
#60096=ORIENTED_EDGE('',*,*,#45238,.F.);
#60097=ORIENTED_EDGE('',*,*,#45239,.T.);
#60098=ORIENTED_EDGE('',*,*,#45240,.F.);
#60099=ORIENTED_EDGE('',*,*,#45233,.T.);
#60100=ORIENTED_EDGE('',*,*,#44264,.F.);
#60101=ORIENTED_EDGE('',*,*,#45241,.F.);
#60102=ORIENTED_EDGE('',*,*,#45242,.F.);
#60103=ORIENTED_EDGE('',*,*,#45239,.F.);
#60104=ORIENTED_EDGE('',*,*,#44266,.F.);
#60105=ORIENTED_EDGE('',*,*,#45243,.T.);
#60106=ORIENTED_EDGE('',*,*,#45244,.F.);
#60107=ORIENTED_EDGE('',*,*,#45241,.T.);
#60108=ORIENTED_EDGE('',*,*,#44268,.F.);
#60109=ORIENTED_EDGE('',*,*,#45245,.F.);
#60110=ORIENTED_EDGE('',*,*,#45246,.F.);
#60111=ORIENTED_EDGE('',*,*,#45247,.F.);
#60112=ORIENTED_EDGE('',*,*,#45248,.F.);
#60113=ORIENTED_EDGE('',*,*,#45243,.F.);
#60114=ORIENTED_EDGE('',*,*,#44270,.F.);
#60115=ORIENTED_EDGE('',*,*,#45249,.F.);
#60116=ORIENTED_EDGE('',*,*,#45250,.F.);
#60117=ORIENTED_EDGE('',*,*,#45251,.F.);
#60118=ORIENTED_EDGE('',*,*,#45252,.F.);
#60119=ORIENTED_EDGE('',*,*,#45253,.F.);
#60120=ORIENTED_EDGE('',*,*,#45254,.F.);
#60121=ORIENTED_EDGE('',*,*,#45255,.F.);
#60122=ORIENTED_EDGE('',*,*,#45256,.F.);
#60123=ORIENTED_EDGE('',*,*,#45257,.F.);
#60124=ORIENTED_EDGE('',*,*,#45258,.F.);
#60125=ORIENTED_EDGE('',*,*,#45259,.F.);
#60126=ORIENTED_EDGE('',*,*,#45260,.F.);
#60127=ORIENTED_EDGE('',*,*,#44269,.F.);
#60128=ORIENTED_EDGE('',*,*,#44272,.T.);
#60129=ORIENTED_EDGE('',*,*,#45261,.T.);
#60130=ORIENTED_EDGE('',*,*,#45249,.T.);
#60131=ORIENTED_EDGE('',*,*,#45262,.F.);
#60132=ORIENTED_EDGE('',*,*,#45263,.F.);
#60133=ORIENTED_EDGE('',*,*,#44271,.F.);
#60134=ORIENTED_EDGE('',*,*,#45264,.F.);
#60135=ORIENTED_EDGE('',*,*,#45265,.F.);
#60136=ORIENTED_EDGE('',*,*,#44273,.T.);
#60137=ORIENTED_EDGE('',*,*,#44274,.T.);
#60138=ORIENTED_EDGE('',*,*,#45266,.T.);
#60139=ORIENTED_EDGE('',*,*,#45267,.F.);
#60140=ORIENTED_EDGE('',*,*,#45268,.F.);
#60141=ORIENTED_EDGE('',*,*,#45269,.F.);
#60142=ORIENTED_EDGE('',*,*,#45270,.F.);
#60143=ORIENTED_EDGE('',*,*,#45271,.F.);
#60144=ORIENTED_EDGE('',*,*,#45272,.F.);
#60145=ORIENTED_EDGE('',*,*,#45273,.F.);
#60146=ORIENTED_EDGE('',*,*,#45274,.F.);
#60147=ORIENTED_EDGE('',*,*,#45275,.F.);
#60148=ORIENTED_EDGE('',*,*,#45276,.F.);
#60149=ORIENTED_EDGE('',*,*,#45277,.F.);
#60150=ORIENTED_EDGE('',*,*,#45278,.F.);
#60151=ORIENTED_EDGE('',*,*,#45279,.F.);
#60152=ORIENTED_EDGE('',*,*,#45280,.F.);
#60153=ORIENTED_EDGE('',*,*,#45281,.F.);
#60154=ORIENTED_EDGE('',*,*,#45282,.F.);
#60155=ORIENTED_EDGE('',*,*,#45266,.F.);
#60156=ORIENTED_EDGE('',*,*,#44276,.F.);
#60157=ORIENTED_EDGE('',*,*,#45283,.T.);
#60158=ORIENTED_EDGE('',*,*,#45284,.T.);
#60159=ORIENTED_EDGE('',*,*,#45267,.T.);
#60160=ORIENTED_EDGE('',*,*,#44278,.F.);
#60161=ORIENTED_EDGE('',*,*,#45285,.F.);
#60162=ORIENTED_EDGE('',*,*,#45286,.F.);
#60163=ORIENTED_EDGE('',*,*,#45283,.F.);
#60164=ORIENTED_EDGE('',*,*,#44280,.F.);
#60165=ORIENTED_EDGE('',*,*,#45287,.T.);
#60166=ORIENTED_EDGE('',*,*,#45288,.F.);
#60167=ORIENTED_EDGE('',*,*,#45285,.T.);
#60168=ORIENTED_EDGE('',*,*,#44283,.F.);
#60169=ORIENTED_EDGE('',*,*,#45289,.F.);
#60170=ORIENTED_EDGE('',*,*,#45290,.T.);
#60171=ORIENTED_EDGE('',*,*,#44285,.T.);
#60172=ORIENTED_EDGE('',*,*,#44284,.T.);
#60173=ORIENTED_EDGE('',*,*,#44288,.T.);
#60174=ORIENTED_EDGE('',*,*,#45291,.F.);
#60175=ORIENTED_EDGE('',*,*,#45292,.F.);
#60176=ORIENTED_EDGE('',*,*,#45293,.F.);
#60177=ORIENTED_EDGE('',*,*,#45294,.F.);
#60178=ORIENTED_EDGE('',*,*,#45287,.F.);
#60179=ORIENTED_EDGE('',*,*,#44286,.F.);
#60180=ORIENTED_EDGE('',*,*,#45290,.F.);
#60181=ORIENTED_EDGE('',*,*,#45295,.F.);
#60182=ORIENTED_EDGE('',*,*,#45296,.F.);
#60183=ORIENTED_EDGE('',*,*,#45297,.F.);
#60184=ORIENTED_EDGE('',*,*,#45298,.F.);
#60185=ORIENTED_EDGE('',*,*,#45299,.F.);
#60186=ORIENTED_EDGE('',*,*,#45300,.F.);
#60187=ORIENTED_EDGE('',*,*,#45301,.F.);
#60188=ORIENTED_EDGE('',*,*,#45302,.F.);
#60189=ORIENTED_EDGE('',*,*,#45303,.F.);
#60190=ORIENTED_EDGE('',*,*,#45304,.F.);
#60191=ORIENTED_EDGE('',*,*,#45305,.F.);
#60192=ORIENTED_EDGE('',*,*,#44287,.F.);
#60193=ORIENTED_EDGE('',*,*,#45206,.F.);
#60194=ORIENTED_EDGE('',*,*,#45306,.F.);
#60195=ORIENTED_EDGE('',*,*,#45307,.F.);
#60196=ORIENTED_EDGE('',*,*,#45137,.T.);
#60197=ORIENTED_EDGE('',*,*,#45125,.T.);
#60198=ORIENTED_EDGE('',*,*,#44295,.T.);
#60199=ORIENTED_EDGE('',*,*,#45308,.F.);
#60200=ORIENTED_EDGE('',*,*,#45309,.T.);
#60201=ORIENTED_EDGE('',*,*,#45310,.F.);
#60202=ORIENTED_EDGE('',*,*,#45309,.F.);
#60203=ORIENTED_EDGE('',*,*,#45311,.F.);
#60204=ORIENTED_EDGE('',*,*,#45310,.T.);
#60205=ORIENTED_EDGE('',*,*,#45311,.T.);
#60206=ORIENTED_EDGE('',*,*,#45312,.T.);
#60207=ORIENTED_EDGE('',*,*,#45313,.F.);
#60208=ORIENTED_EDGE('',*,*,#44294,.F.);
#60209=ORIENTED_EDGE('',*,*,#45314,.F.);
#60210=ORIENTED_EDGE('',*,*,#45312,.F.);
#60211=ORIENTED_EDGE('',*,*,#45315,.F.);
#60212=ORIENTED_EDGE('',*,*,#44293,.T.);
#60213=ORIENTED_EDGE('',*,*,#45316,.T.);
#60214=ORIENTED_EDGE('',*,*,#45139,.T.);
#60215=ORIENTED_EDGE('',*,*,#45316,.F.);
#60216=ORIENTED_EDGE('',*,*,#44292,.T.);
#60217=ORIENTED_EDGE('',*,*,#45317,.T.);
#60218=ORIENTED_EDGE('',*,*,#45318,.T.);
#60219=ORIENTED_EDGE('',*,*,#45317,.F.);
#60220=ORIENTED_EDGE('',*,*,#44291,.T.);
#60221=ORIENTED_EDGE('',*,*,#45319,.T.);
#60222=ORIENTED_EDGE('',*,*,#45320,.T.);
#60223=ORIENTED_EDGE('',*,*,#45319,.F.);
#60224=ORIENTED_EDGE('',*,*,#44290,.T.);
#60225=ORIENTED_EDGE('',*,*,#45321,.T.);
#60226=ORIENTED_EDGE('',*,*,#45322,.T.);
#60227=ORIENTED_EDGE('',*,*,#45321,.F.);
#60228=ORIENTED_EDGE('',*,*,#44289,.T.);
#60229=ORIENTED_EDGE('',*,*,#45074,.T.);
#60230=ORIENTED_EDGE('',*,*,#45077,.T.);
#60231=ORIENTED_EDGE('',*,*,#44983,.F.);
#60232=ORIENTED_EDGE('',*,*,#44299,.T.);
#60233=ORIENTED_EDGE('',*,*,#45323,.T.);
#60234=ORIENTED_EDGE('',*,*,#44978,.T.);
#60235=ORIENTED_EDGE('',*,*,#45324,.F.);
#60236=ORIENTED_EDGE('',*,*,#45325,.T.);
#60237=ORIENTED_EDGE('',*,*,#45326,.F.);
#60238=ORIENTED_EDGE('',*,*,#45325,.F.);
#60239=ORIENTED_EDGE('',*,*,#45327,.F.);
#60240=ORIENTED_EDGE('',*,*,#45326,.T.);
#60241=ORIENTED_EDGE('',*,*,#45327,.T.);
#60242=ORIENTED_EDGE('',*,*,#45328,.T.);
#60243=ORIENTED_EDGE('',*,*,#44297,.F.);
#60244=ORIENTED_EDGE('',*,*,#45329,.F.);
#60245=ORIENTED_EDGE('',*,*,#45330,.F.);
#60246=ORIENTED_EDGE('',*,*,#45331,.F.);
#60247=ORIENTED_EDGE('',*,*,#44298,.F.);
#60248=ORIENTED_EDGE('',*,*,#45328,.F.);
#60249=ORIENTED_EDGE('',*,*,#45332,.F.);
#60250=ORIENTED_EDGE('',*,*,#44296,.T.);
#60251=ORIENTED_EDGE('',*,*,#45223,.T.);
#60252=ORIENTED_EDGE('',*,*,#45232,.T.);
#60253=ORIENTED_EDGE('',*,*,#44301,.T.);
#60254=ORIENTED_EDGE('',*,*,#45333,.F.);
#60255=ORIENTED_EDGE('',*,*,#45334,.T.);
#60256=ORIENTED_EDGE('',*,*,#45335,.F.);
#60257=ORIENTED_EDGE('',*,*,#45336,.F.);
#60258=ORIENTED_EDGE('',*,*,#45333,.T.);
#60259=ORIENTED_EDGE('',*,*,#44304,.T.);
#60260=ORIENTED_EDGE('',*,*,#44989,.T.);
#60261=ORIENTED_EDGE('',*,*,#45337,.T.);
#60262=ORIENTED_EDGE('',*,*,#45338,.T.);
#60263=ORIENTED_EDGE('',*,*,#45088,.T.);
#60264=ORIENTED_EDGE('',*,*,#44318,.F.);
#60265=ORIENTED_EDGE('',*,*,#45339,.F.);
#60266=ORIENTED_EDGE('',*,*,#45340,.F.);
#60267=ORIENTED_EDGE('',*,*,#45337,.F.);
#60268=ORIENTED_EDGE('',*,*,#44321,.F.);
#60269=ORIENTED_EDGE('',*,*,#44320,.F.);
#60270=ORIENTED_EDGE('',*,*,#44326,.T.);
#60271=ORIENTED_EDGE('',*,*,#45341,.T.);
#60272=ORIENTED_EDGE('',*,*,#45342,.T.);
#60273=ORIENTED_EDGE('',*,*,#45343,.F.);
#60274=ORIENTED_EDGE('',*,*,#44322,.T.);
#60275=ORIENTED_EDGE('',*,*,#45344,.T.);
#60276=ORIENTED_EDGE('',*,*,#45345,.T.);
#60277=ORIENTED_EDGE('',*,*,#45344,.F.);
#60278=ORIENTED_EDGE('',*,*,#44330,.T.);
#60279=ORIENTED_EDGE('',*,*,#45346,.T.);
#60280=ORIENTED_EDGE('',*,*,#45141,.T.);
#60281=ORIENTED_EDGE('',*,*,#45341,.F.);
#60282=ORIENTED_EDGE('',*,*,#44325,.T.);
#60283=ORIENTED_EDGE('',*,*,#45347,.T.);
#60284=ORIENTED_EDGE('',*,*,#45081,.T.);
#60285=ORIENTED_EDGE('',*,*,#45347,.F.);
#60286=ORIENTED_EDGE('',*,*,#44324,.T.);
#60287=ORIENTED_EDGE('',*,*,#45348,.T.);
#60288=ORIENTED_EDGE('',*,*,#45349,.T.);
#60289=ORIENTED_EDGE('',*,*,#45348,.F.);
#60290=ORIENTED_EDGE('',*,*,#44323,.T.);
#60291=ORIENTED_EDGE('',*,*,#45343,.T.);
#60292=ORIENTED_EDGE('',*,*,#45350,.T.);
#60293=ORIENTED_EDGE('',*,*,#45351,.T.);
#60294=ORIENTED_EDGE('',*,*,#44729,.F.);
#60295=ORIENTED_EDGE('',*,*,#44730,.T.);
#60296=ORIENTED_EDGE('',*,*,#44336,.F.);
#60297=ORIENTED_EDGE('',*,*,#45352,.F.);
#60298=ORIENTED_EDGE('',*,*,#44727,.F.);
#60299=ORIENTED_EDGE('',*,*,#45351,.F.);
#60300=ORIENTED_EDGE('',*,*,#44339,.F.);
#60301=ORIENTED_EDGE('',*,*,#44721,.T.);
#60302=ORIENTED_EDGE('',*,*,#44725,.F.);
#60303=ORIENTED_EDGE('',*,*,#45352,.T.);
#60304=ORIENTED_EDGE('',*,*,#44342,.F.);
#60305=ORIENTED_EDGE('',*,*,#45353,.F.);
#60306=ORIENTED_EDGE('',*,*,#44722,.T.);
#60307=ORIENTED_EDGE('',*,*,#44344,.F.);
#60308=ORIENTED_EDGE('',*,*,#44349,.T.);
#60309=ORIENTED_EDGE('',*,*,#44348,.T.);
#60310=ORIENTED_EDGE('',*,*,#45354,.F.);
#60311=ORIENTED_EDGE('',*,*,#44346,.T.);
#60312=ORIENTED_EDGE('',*,*,#44351,.T.);
#60313=ORIENTED_EDGE('',*,*,#44352,.T.);
#60314=ORIENTED_EDGE('',*,*,#44714,.T.);
#60315=ORIENTED_EDGE('',*,*,#45355,.T.);
#60316=ORIENTED_EDGE('',*,*,#44710,.F.);
#60317=ORIENTED_EDGE('',*,*,#44715,.T.);
#60318=ORIENTED_EDGE('',*,*,#44358,.F.);
#60319=ORIENTED_EDGE('',*,*,#45356,.F.);
#60320=ORIENTED_EDGE('',*,*,#44708,.F.);
#60321=ORIENTED_EDGE('',*,*,#45355,.F.);
#60322=ORIENTED_EDGE('',*,*,#44361,.F.);
#60323=ORIENTED_EDGE('',*,*,#44700,.T.);
#60324=ORIENTED_EDGE('',*,*,#44706,.F.);
#60325=ORIENTED_EDGE('',*,*,#45356,.T.);
#60326=ORIENTED_EDGE('',*,*,#44364,.F.);
#60327=ORIENTED_EDGE('',*,*,#44366,.F.);
#60328=ORIENTED_EDGE('',*,*,#44370,.T.);
#60329=ORIENTED_EDGE('',*,*,#45357,.T.);
#60330=ORIENTED_EDGE('',*,*,#44701,.T.);
#60331=ORIENTED_EDGE('',*,*,#45358,.F.);
#60332=ORIENTED_EDGE('',*,*,#44702,.T.);
#60333=ORIENTED_EDGE('',*,*,#45357,.F.);
#60334=ORIENTED_EDGE('',*,*,#44374,.T.);
#60335=ORIENTED_EDGE('',*,*,#44373,.F.);
#60336=ORIENTED_EDGE('',*,*,#45359,.T.);
#60337=ORIENTED_EDGE('',*,*,#45360,.F.);
#60338=ORIENTED_EDGE('',*,*,#44694,.T.);
#60339=ORIENTED_EDGE('',*,*,#45361,.F.);
#60340=ORIENTED_EDGE('',*,*,#45359,.F.);
#60341=ORIENTED_EDGE('',*,*,#44375,.F.);
#60342=ORIENTED_EDGE('',*,*,#45362,.F.);
#60343=ORIENTED_EDGE('',*,*,#45363,.F.);
#60344=ORIENTED_EDGE('',*,*,#44377,.T.);
#60345=ORIENTED_EDGE('',*,*,#44378,.T.);
#60346=ORIENTED_EDGE('',*,*,#44690,.T.);
#60347=ORIENTED_EDGE('',*,*,#45364,.T.);
#60348=ORIENTED_EDGE('',*,*,#45365,.T.);
#60349=ORIENTED_EDGE('',*,*,#44691,.T.);
#60350=ORIENTED_EDGE('',*,*,#44384,.F.);
#60351=ORIENTED_EDGE('',*,*,#45366,.F.);
#60352=ORIENTED_EDGE('',*,*,#45367,.F.);
#60353=ORIENTED_EDGE('',*,*,#45364,.F.);
#60354=ORIENTED_EDGE('',*,*,#44387,.F.);
#60355=ORIENTED_EDGE('',*,*,#44674,.T.);
#60356=ORIENTED_EDGE('',*,*,#45368,.F.);
#60357=ORIENTED_EDGE('',*,*,#45366,.T.);
#60358=ORIENTED_EDGE('',*,*,#44390,.F.);
#60359=ORIENTED_EDGE('',*,*,#45369,.F.);
#60360=ORIENTED_EDGE('',*,*,#44675,.T.);
#60361=ORIENTED_EDGE('',*,*,#44392,.F.);
#60362=ORIENTED_EDGE('',*,*,#44397,.T.);
#60363=ORIENTED_EDGE('',*,*,#44396,.F.);
#60364=ORIENTED_EDGE('',*,*,#45370,.F.);
#60365=ORIENTED_EDGE('',*,*,#45371,.F.);
#60366=ORIENTED_EDGE('',*,*,#45372,.F.);
#60367=ORIENTED_EDGE('',*,*,#45373,.F.);
#60368=ORIENTED_EDGE('',*,*,#44395,.T.);
#60369=ORIENTED_EDGE('',*,*,#44398,.T.);
#60370=ORIENTED_EDGE('',*,*,#45070,.T.);
#60371=ORIENTED_EDGE('',*,*,#45374,.T.);
#60372=ORIENTED_EDGE('',*,*,#45375,.T.);
#60373=ORIENTED_EDGE('',*,*,#45071,.T.);
#60374=ORIENTED_EDGE('',*,*,#44404,.F.);
#60375=ORIENTED_EDGE('',*,*,#45376,.F.);
#60376=ORIENTED_EDGE('',*,*,#45377,.F.);
#60377=ORIENTED_EDGE('',*,*,#45374,.F.);
#60378=ORIENTED_EDGE('',*,*,#44407,.F.);
#60379=ORIENTED_EDGE('',*,*,#45052,.T.);
#60380=ORIENTED_EDGE('',*,*,#45378,.F.);
#60381=ORIENTED_EDGE('',*,*,#45376,.T.);
#60382=ORIENTED_EDGE('',*,*,#44410,.F.);
#60383=ORIENTED_EDGE('',*,*,#45379,.F.);
#60384=ORIENTED_EDGE('',*,*,#45053,.T.);
#60385=ORIENTED_EDGE('',*,*,#44412,.F.);
#60386=ORIENTED_EDGE('',*,*,#44417,.T.);
#60387=ORIENTED_EDGE('',*,*,#44416,.F.);
#60388=ORIENTED_EDGE('',*,*,#45380,.F.);
#60389=ORIENTED_EDGE('',*,*,#45381,.F.);
#60390=ORIENTED_EDGE('',*,*,#45382,.F.);
#60391=ORIENTED_EDGE('',*,*,#45383,.F.);
#60392=ORIENTED_EDGE('',*,*,#44415,.T.);
#60393=ORIENTED_EDGE('',*,*,#44418,.T.);
#60394=ORIENTED_EDGE('',*,*,#45095,.T.);
#60395=ORIENTED_EDGE('',*,*,#45127,.T.);
#60396=ORIENTED_EDGE('',*,*,#45346,.F.);
#60397=ORIENTED_EDGE('',*,*,#44421,.T.);
#60398=ORIENTED_EDGE('',*,*,#45384,.F.);
#60399=ORIENTED_EDGE('',*,*,#45385,.F.);
#60400=ORIENTED_EDGE('',*,*,#44428,.T.);
#60401=ORIENTED_EDGE('',*,*,#45386,.T.);
#60402=ORIENTED_EDGE('',*,*,#45387,.T.);
#60403=ORIENTED_EDGE('',*,*,#45386,.F.);
#60404=ORIENTED_EDGE('',*,*,#44427,.T.);
#60405=ORIENTED_EDGE('',*,*,#45388,.T.);
#60406=ORIENTED_EDGE('',*,*,#44500,.F.);
#60407=ORIENTED_EDGE('',*,*,#45388,.F.);
#60408=ORIENTED_EDGE('',*,*,#44426,.T.);
#60409=ORIENTED_EDGE('',*,*,#45389,.T.);
#60410=ORIENTED_EDGE('',*,*,#45390,.T.);
#60411=ORIENTED_EDGE('',*,*,#45389,.F.);
#60412=ORIENTED_EDGE('',*,*,#44425,.T.);
#60413=ORIENTED_EDGE('',*,*,#45391,.T.);
#60414=ORIENTED_EDGE('',*,*,#45392,.T.);
#60415=ORIENTED_EDGE('',*,*,#45391,.F.);
#60416=ORIENTED_EDGE('',*,*,#44424,.T.);
#60417=ORIENTED_EDGE('',*,*,#45393,.T.);
#60418=ORIENTED_EDGE('',*,*,#45394,.T.);
#60419=ORIENTED_EDGE('',*,*,#45393,.F.);
#60420=ORIENTED_EDGE('',*,*,#44431,.T.);
#60421=ORIENTED_EDGE('',*,*,#44436,.T.);
#60422=ORIENTED_EDGE('',*,*,#45395,.T.);
#60423=ORIENTED_EDGE('',*,*,#44441,.F.);
#60424=ORIENTED_EDGE('',*,*,#44446,.F.);
#60425=ORIENTED_EDGE('',*,*,#45396,.F.);
#60426=ORIENTED_EDGE('',*,*,#45397,.F.);
#60427=ORIENTED_EDGE('',*,*,#45394,.F.);
#60428=ORIENTED_EDGE('',*,*,#45395,.F.);
#60429=ORIENTED_EDGE('',*,*,#44438,.F.);
#60430=ORIENTED_EDGE('',*,*,#45398,.T.);
#60431=ORIENTED_EDGE('',*,*,#45399,.F.);
#60432=ORIENTED_EDGE('',*,*,#45396,.T.);
#60433=ORIENTED_EDGE('',*,*,#44449,.F.);
#60434=ORIENTED_EDGE('',*,*,#45400,.F.);
#60435=ORIENTED_EDGE('',*,*,#45401,.F.);
#60436=ORIENTED_EDGE('',*,*,#45398,.F.);
#60437=ORIENTED_EDGE('',*,*,#44452,.F.);
#60438=ORIENTED_EDGE('',*,*,#45402,.T.);
#60439=ORIENTED_EDGE('',*,*,#45403,.F.);
#60440=ORIENTED_EDGE('',*,*,#45400,.T.);
#60441=ORIENTED_EDGE('',*,*,#44455,.F.);
#60442=ORIENTED_EDGE('',*,*,#45404,.F.);
#60443=ORIENTED_EDGE('',*,*,#45402,.F.);
#60444=ORIENTED_EDGE('',*,*,#44458,.F.);
#60445=ORIENTED_EDGE('',*,*,#45405,.F.);
#60446=ORIENTED_EDGE('',*,*,#45406,.F.);
#60447=ORIENTED_EDGE('',*,*,#45407,.F.);
#60448=ORIENTED_EDGE('',*,*,#45408,.F.);
#60449=ORIENTED_EDGE('',*,*,#45409,.F.);
#60450=ORIENTED_EDGE('',*,*,#45410,.F.);
#60451=ORIENTED_EDGE('',*,*,#45411,.F.);
#60452=ORIENTED_EDGE('',*,*,#45412,.F.);
#60453=ORIENTED_EDGE('',*,*,#45413,.F.);
#60454=ORIENTED_EDGE('',*,*,#45414,.F.);
#60455=ORIENTED_EDGE('',*,*,#45415,.F.);
#60456=ORIENTED_EDGE('',*,*,#45416,.F.);
#60457=ORIENTED_EDGE('',*,*,#45417,.F.);
#60458=ORIENTED_EDGE('',*,*,#45418,.F.);
#60459=ORIENTED_EDGE('',*,*,#45419,.F.);
#60460=ORIENTED_EDGE('',*,*,#45420,.F.);
#60461=ORIENTED_EDGE('',*,*,#45405,.T.);
#60462=ORIENTED_EDGE('',*,*,#44461,.F.);
#60463=ORIENTED_EDGE('',*,*,#45421,.T.);
#60464=ORIENTED_EDGE('',*,*,#45422,.F.);
#60465=ORIENTED_EDGE('',*,*,#45421,.F.);
#60466=ORIENTED_EDGE('',*,*,#44464,.F.);
#60467=ORIENTED_EDGE('',*,*,#45423,.F.);
#60468=ORIENTED_EDGE('',*,*,#45424,.F.);
#60469=ORIENTED_EDGE('',*,*,#45425,.F.);
#60470=ORIENTED_EDGE('',*,*,#45426,.F.);
#60471=ORIENTED_EDGE('',*,*,#45427,.F.);
#60472=ORIENTED_EDGE('',*,*,#45428,.F.);
#60473=ORIENTED_EDGE('',*,*,#45429,.F.);
#60474=ORIENTED_EDGE('',*,*,#45430,.F.);
#60475=ORIENTED_EDGE('',*,*,#45431,.F.);
#60476=ORIENTED_EDGE('',*,*,#45432,.F.);
#60477=ORIENTED_EDGE('',*,*,#45433,.F.);
#60478=ORIENTED_EDGE('',*,*,#45434,.F.);
#60479=ORIENTED_EDGE('',*,*,#45435,.F.);
#60480=ORIENTED_EDGE('',*,*,#45436,.F.);
#60481=ORIENTED_EDGE('',*,*,#45437,.F.);
#60482=ORIENTED_EDGE('',*,*,#45438,.F.);
#60483=ORIENTED_EDGE('',*,*,#45439,.F.);
#60484=ORIENTED_EDGE('',*,*,#45440,.F.);
#60485=ORIENTED_EDGE('',*,*,#45441,.F.);
#60486=ORIENTED_EDGE('',*,*,#45442,.F.);
#60487=ORIENTED_EDGE('',*,*,#45443,.F.);
#60488=ORIENTED_EDGE('',*,*,#45444,.F.);
#60489=ORIENTED_EDGE('',*,*,#45445,.F.);
#60490=ORIENTED_EDGE('',*,*,#45446,.F.);
#60491=ORIENTED_EDGE('',*,*,#45447,.F.);
#60492=ORIENTED_EDGE('',*,*,#45448,.F.);
#60493=ORIENTED_EDGE('',*,*,#45449,.F.);
#60494=ORIENTED_EDGE('',*,*,#45450,.F.);
#60495=ORIENTED_EDGE('',*,*,#45451,.F.);
#60496=ORIENTED_EDGE('',*,*,#45452,.F.);
#60497=ORIENTED_EDGE('',*,*,#45453,.F.);
#60498=ORIENTED_EDGE('',*,*,#45454,.F.);
#60499=ORIENTED_EDGE('',*,*,#45455,.F.);
#60500=ORIENTED_EDGE('',*,*,#45456,.F.);
#60501=ORIENTED_EDGE('',*,*,#45457,.F.);
#60502=ORIENTED_EDGE('',*,*,#45458,.F.);
#60503=ORIENTED_EDGE('',*,*,#45459,.F.);
#60504=ORIENTED_EDGE('',*,*,#45460,.F.);
#60505=ORIENTED_EDGE('',*,*,#45461,.F.);
#60506=ORIENTED_EDGE('',*,*,#45462,.F.);
#60507=ORIENTED_EDGE('',*,*,#45463,.F.);
#60508=ORIENTED_EDGE('',*,*,#45464,.F.);
#60509=ORIENTED_EDGE('',*,*,#45423,.T.);
#60510=ORIENTED_EDGE('',*,*,#44467,.F.);
#60511=ORIENTED_EDGE('',*,*,#45465,.T.);
#60512=ORIENTED_EDGE('',*,*,#45466,.F.);
#60513=ORIENTED_EDGE('',*,*,#45467,.F.);
#60514=ORIENTED_EDGE('',*,*,#45468,.F.);
#60515=ORIENTED_EDGE('',*,*,#45469,.F.);
#60516=ORIENTED_EDGE('',*,*,#45470,.F.);
#60517=ORIENTED_EDGE('',*,*,#45471,.F.);
#60518=ORIENTED_EDGE('',*,*,#45472,.F.);
#60519=ORIENTED_EDGE('',*,*,#45473,.F.);
#60520=ORIENTED_EDGE('',*,*,#45474,.F.);
#60521=ORIENTED_EDGE('',*,*,#45475,.F.);
#60522=ORIENTED_EDGE('',*,*,#45476,.F.);
#60523=ORIENTED_EDGE('',*,*,#45465,.F.);
#60524=ORIENTED_EDGE('',*,*,#44470,.F.);
#60525=ORIENTED_EDGE('',*,*,#45477,.F.);
#60526=ORIENTED_EDGE('',*,*,#45478,.F.);
#60527=ORIENTED_EDGE('',*,*,#45479,.F.);
#60528=ORIENTED_EDGE('',*,*,#45480,.F.);
#60529=ORIENTED_EDGE('',*,*,#45481,.F.);
#60530=ORIENTED_EDGE('',*,*,#45482,.F.);
#60531=ORIENTED_EDGE('',*,*,#45483,.F.);
#60532=ORIENTED_EDGE('',*,*,#45484,.T.);
#60533=ORIENTED_EDGE('',*,*,#45485,.F.);
#60534=ORIENTED_EDGE('',*,*,#45477,.T.);
#60535=ORIENTED_EDGE('',*,*,#44473,.F.);
#60536=ORIENTED_EDGE('',*,*,#45486,.F.);
#60537=ORIENTED_EDGE('',*,*,#45487,.F.);
#60538=ORIENTED_EDGE('',*,*,#45484,.F.);
#60539=ORIENTED_EDGE('',*,*,#44476,.F.);
#60540=ORIENTED_EDGE('',*,*,#45488,.T.);
#60541=ORIENTED_EDGE('',*,*,#45489,.F.);
#60542=ORIENTED_EDGE('',*,*,#45486,.T.);
#60543=ORIENTED_EDGE('',*,*,#44479,.F.);
#60544=ORIENTED_EDGE('',*,*,#45490,.F.);
#60545=ORIENTED_EDGE('',*,*,#45488,.F.);
#60546=ORIENTED_EDGE('',*,*,#44482,.F.);
#60547=ORIENTED_EDGE('',*,*,#44561,.F.);
#60548=ORIENTED_EDGE('',*,*,#45491,.F.);
#60549=ORIENTED_EDGE('',*,*,#45492,.F.);
#60550=ORIENTED_EDGE('',*,*,#45493,.F.);
#60551=ORIENTED_EDGE('',*,*,#45494,.F.);
#60552=ORIENTED_EDGE('',*,*,#45495,.F.);
#60553=ORIENTED_EDGE('',*,*,#45496,.F.);
#60554=ORIENTED_EDGE('',*,*,#45497,.F.);
#60555=ORIENTED_EDGE('',*,*,#45498,.F.);
#60556=ORIENTED_EDGE('',*,*,#45499,.F.);
#60557=ORIENTED_EDGE('',*,*,#45500,.F.);
#60558=ORIENTED_EDGE('',*,*,#45501,.F.);
#60559=ORIENTED_EDGE('',*,*,#45502,.F.);
#60560=ORIENTED_EDGE('',*,*,#45503,.F.);
#60561=ORIENTED_EDGE('',*,*,#45504,.F.);
#60562=ORIENTED_EDGE('',*,*,#44969,.T.);
#60563=ORIENTED_EDGE('',*,*,#45505,.T.);
#60564=ORIENTED_EDGE('',*,*,#44492,.F.);
#60565=ORIENTED_EDGE('',*,*,#45506,.F.);
#60566=ORIENTED_EDGE('',*,*,#45507,.F.);
#60567=ORIENTED_EDGE('',*,*,#45508,.F.);
#60568=ORIENTED_EDGE('',*,*,#45509,.F.);
#60569=ORIENTED_EDGE('',*,*,#45510,.F.);
#60570=ORIENTED_EDGE('',*,*,#45511,.F.);
#60571=ORIENTED_EDGE('',*,*,#44491,.F.);
#60572=ORIENTED_EDGE('',*,*,#44488,.F.);
#60573=ORIENTED_EDGE('',*,*,#45512,.F.);
#60574=ORIENTED_EDGE('',*,*,#45513,.F.);
#60575=ORIENTED_EDGE('',*,*,#45227,.T.);
#60576=ORIENTED_EDGE('',*,*,#45514,.T.);
#60577=ORIENTED_EDGE('',*,*,#44487,.F.);
#60578=ORIENTED_EDGE('',*,*,#44493,.F.);
#60579=ORIENTED_EDGE('',*,*,#45515,.F.);
#60580=ORIENTED_EDGE('',*,*,#45516,.F.);
#60581=ORIENTED_EDGE('',*,*,#45517,.F.);
#60582=ORIENTED_EDGE('',*,*,#45518,.F.);
#60583=ORIENTED_EDGE('',*,*,#45129,.T.);
#60584=ORIENTED_EDGE('',*,*,#45519,.T.);
#60585=ORIENTED_EDGE('',*,*,#44498,.F.);
#60586=ORIENTED_EDGE('',*,*,#44495,.F.);
#60587=ORIENTED_EDGE('',*,*,#45520,.F.);
#60588=ORIENTED_EDGE('',*,*,#45521,.F.);
#60589=ORIENTED_EDGE('',*,*,#45522,.F.);
#60590=ORIENTED_EDGE('',*,*,#45523,.F.);
#60591=ORIENTED_EDGE('',*,*,#45524,.F.);
#60592=ORIENTED_EDGE('',*,*,#45525,.F.);
#60593=ORIENTED_EDGE('',*,*,#44494,.F.);
#60594=ORIENTED_EDGE('',*,*,#45390,.F.);
#60595=ORIENTED_EDGE('',*,*,#44499,.F.);
#60596=ORIENTED_EDGE('',*,*,#45526,.F.);
#60597=ORIENTED_EDGE('',*,*,#45387,.F.);
#60598=ORIENTED_EDGE('',*,*,#44659,.T.);
#60599=ORIENTED_EDGE('',*,*,#45527,.F.);
#60600=ORIENTED_EDGE('',*,*,#45528,.T.);
#60601=ORIENTED_EDGE('',*,*,#44502,.F.);
#60602=ORIENTED_EDGE('',*,*,#44506,.F.);
#60603=ORIENTED_EDGE('',*,*,#44511,.T.);
#60604=ORIENTED_EDGE('',*,*,#45529,.T.);
#60605=ORIENTED_EDGE('',*,*,#44660,.T.);
#60606=ORIENTED_EDGE('',*,*,#44510,.F.);
#60607=ORIENTED_EDGE('',*,*,#45530,.F.);
#60608=ORIENTED_EDGE('',*,*,#45531,.F.);
#60609=ORIENTED_EDGE('',*,*,#45532,.F.);
#60610=ORIENTED_EDGE('',*,*,#44514,.F.);
#60611=ORIENTED_EDGE('',*,*,#44649,.T.);
#60612=ORIENTED_EDGE('',*,*,#45533,.T.);
#60613=ORIENTED_EDGE('',*,*,#44509,.T.);
#60614=ORIENTED_EDGE('',*,*,#45534,.T.);
#60615=ORIENTED_EDGE('',*,*,#45535,.T.);
#60616=ORIENTED_EDGE('',*,*,#44640,.T.);
#60617=ORIENTED_EDGE('',*,*,#44517,.F.);
#60618=ORIENTED_EDGE('',*,*,#45536,.F.);
#60619=ORIENTED_EDGE('',*,*,#45537,.F.);
#60620=ORIENTED_EDGE('',*,*,#45534,.F.);
#60621=ORIENTED_EDGE('',*,*,#44520,.F.);
#60622=ORIENTED_EDGE('',*,*,#44625,.T.);
#60623=ORIENTED_EDGE('',*,*,#45538,.F.);
#60624=ORIENTED_EDGE('',*,*,#45536,.T.);
#60625=ORIENTED_EDGE('',*,*,#44524,.F.);
#60626=ORIENTED_EDGE('',*,*,#44526,.F.);
#60627=ORIENTED_EDGE('',*,*,#44531,.T.);
#60628=ORIENTED_EDGE('',*,*,#45539,.T.);
#60629=ORIENTED_EDGE('',*,*,#44626,.T.);
#60630=ORIENTED_EDGE('',*,*,#44530,.F.);
#60631=ORIENTED_EDGE('',*,*,#45540,.F.);
#60632=ORIENTED_EDGE('',*,*,#45541,.F.);
#60633=ORIENTED_EDGE('',*,*,#45542,.F.);
#60634=ORIENTED_EDGE('',*,*,#44534,.F.);
#60635=ORIENTED_EDGE('',*,*,#44615,.T.);
#60636=ORIENTED_EDGE('',*,*,#45543,.T.);
#60637=ORIENTED_EDGE('',*,*,#44529,.T.);
#60638=ORIENTED_EDGE('',*,*,#45544,.T.);
#60639=ORIENTED_EDGE('',*,*,#45545,.T.);
#60640=ORIENTED_EDGE('',*,*,#44608,.T.);
#60641=ORIENTED_EDGE('',*,*,#44537,.F.);
#60642=ORIENTED_EDGE('',*,*,#45546,.F.);
#60643=ORIENTED_EDGE('',*,*,#45547,.T.);
#60644=ORIENTED_EDGE('',*,*,#45544,.F.);
#60645=ORIENTED_EDGE('',*,*,#44540,.F.);
#60646=ORIENTED_EDGE('',*,*,#44593,.T.);
#60647=ORIENTED_EDGE('',*,*,#45548,.F.);
#60648=ORIENTED_EDGE('',*,*,#45546,.T.);
#60649=ORIENTED_EDGE('',*,*,#44544,.F.);
#60650=ORIENTED_EDGE('',*,*,#44546,.F.);
#60651=ORIENTED_EDGE('',*,*,#44551,.T.);
#60652=ORIENTED_EDGE('',*,*,#45549,.T.);
#60653=ORIENTED_EDGE('',*,*,#44594,.T.);
#60654=ORIENTED_EDGE('',*,*,#44550,.F.);
#60655=ORIENTED_EDGE('',*,*,#45550,.F.);
#60656=ORIENTED_EDGE('',*,*,#45551,.F.);
#60657=ORIENTED_EDGE('',*,*,#45552,.F.);
#60658=ORIENTED_EDGE('',*,*,#44554,.F.);
#60659=ORIENTED_EDGE('',*,*,#44585,.T.);
#60660=ORIENTED_EDGE('',*,*,#45553,.T.);
#60661=ORIENTED_EDGE('',*,*,#44549,.T.);
#60662=ORIENTED_EDGE('',*,*,#45554,.F.);
#60663=ORIENTED_EDGE('',*,*,#44998,.T.);
#60664=ORIENTED_EDGE('',*,*,#45555,.T.);
#60665=ORIENTED_EDGE('',*,*,#44559,.T.);
#60666=ORIENTED_EDGE('',*,*,#44566,.F.);
#60667=ORIENTED_EDGE('',*,*,#45556,.T.);
#60668=ORIENTED_EDGE('',*,*,#45554,.T.);
#60669=ORIENTED_EDGE('',*,*,#44563,.T.);
#60670=ORIENTED_EDGE('',*,*,#45557,.T.);
#60671=ORIENTED_EDGE('',*,*,#45558,.F.);
#60672=ORIENTED_EDGE('',*,*,#44560,.T.);
#60673=ORIENTED_EDGE('',*,*,#45559,.F.);
#60674=ORIENTED_EDGE('',*,*,#45560,.T.);
#60675=ORIENTED_EDGE('',*,*,#45561,.T.);
#60676=ORIENTED_EDGE('',*,*,#44986,.T.);
#60677=ORIENTED_EDGE('',*,*,#45556,.F.);
#60678=ORIENTED_EDGE('',*,*,#44565,.F.);
#60679=ORIENTED_EDGE('',*,*,#45528,.F.);
#60680=ORIENTED_EDGE('',*,*,#45562,.F.);
#60681=ORIENTED_EDGE('',*,*,#45560,.F.);
#60682=ORIENTED_EDGE('',*,*,#44568,.F.);
#60683=ORIENTED_EDGE('',*,*,#45563,.F.);
#60684=ORIENTED_EDGE('',*,*,#44580,.T.);
#60685=ORIENTED_EDGE('',*,*,#44578,.T.);
#60686=ORIENTED_EDGE('',*,*,#44587,.T.);
#60687=ORIENTED_EDGE('',*,*,#45553,.F.);
#60688=ORIENTED_EDGE('',*,*,#44584,.T.);
#60689=ORIENTED_EDGE('',*,*,#45564,.T.);
#60690=ORIENTED_EDGE('',*,*,#45550,.T.);
#60691=ORIENTED_EDGE('',*,*,#45564,.F.);
#60692=ORIENTED_EDGE('',*,*,#44583,.T.);
#60693=ORIENTED_EDGE('',*,*,#45565,.T.);
#60694=ORIENTED_EDGE('',*,*,#45566,.T.);
#60695=ORIENTED_EDGE('',*,*,#45565,.F.);
#60696=ORIENTED_EDGE('',*,*,#44582,.T.);
#60697=ORIENTED_EDGE('',*,*,#45567,.T.);
#60698=ORIENTED_EDGE('',*,*,#45568,.T.);
#60699=ORIENTED_EDGE('',*,*,#45567,.F.);
#60700=ORIENTED_EDGE('',*,*,#44581,.T.);
#60701=ORIENTED_EDGE('',*,*,#45563,.T.);
#60702=ORIENTED_EDGE('',*,*,#45569,.T.);
#60703=ORIENTED_EDGE('',*,*,#45570,.T.);
#60704=ORIENTED_EDGE('',*,*,#45569,.F.);
#60705=ORIENTED_EDGE('',*,*,#44586,.T.);
#60706=ORIENTED_EDGE('',*,*,#45571,.F.);
#60707=ORIENTED_EDGE('',*,*,#45572,.F.);
#60708=ORIENTED_EDGE('',*,*,#44588,.T.);
#60709=ORIENTED_EDGE('',*,*,#44589,.T.);
#60710=ORIENTED_EDGE('',*,*,#44599,.T.);
#60711=ORIENTED_EDGE('',*,*,#45573,.F.);
#60712=ORIENTED_EDGE('',*,*,#45571,.T.);
#60713=ORIENTED_EDGE('',*,*,#45572,.T.);
#60714=ORIENTED_EDGE('',*,*,#44598,.T.);
#60715=ORIENTED_EDGE('',*,*,#45574,.F.);
#60716=ORIENTED_EDGE('',*,*,#45575,.T.);
#60717=ORIENTED_EDGE('',*,*,#45573,.T.);
#60718=ORIENTED_EDGE('',*,*,#44597,.T.);
#60719=ORIENTED_EDGE('',*,*,#45576,.F.);
#60720=ORIENTED_EDGE('',*,*,#45577,.T.);
#60721=ORIENTED_EDGE('',*,*,#45574,.T.);
#60722=ORIENTED_EDGE('',*,*,#44596,.T.);
#60723=ORIENTED_EDGE('',*,*,#45549,.F.);
#60724=ORIENTED_EDGE('',*,*,#45552,.T.);
#60725=ORIENTED_EDGE('',*,*,#45576,.T.);
#60726=ORIENTED_EDGE('',*,*,#44595,.T.);
#60727=ORIENTED_EDGE('',*,*,#44601,.F.);
#60728=ORIENTED_EDGE('',*,*,#45578,.T.);
#60729=ORIENTED_EDGE('',*,*,#45548,.T.);
#60730=ORIENTED_EDGE('',*,*,#44592,.T.);
#60731=ORIENTED_EDGE('',*,*,#44603,.F.);
#60732=ORIENTED_EDGE('',*,*,#45579,.F.);
#60733=ORIENTED_EDGE('',*,*,#45547,.F.);
#60734=ORIENTED_EDGE('',*,*,#45578,.F.);
#60735=ORIENTED_EDGE('',*,*,#45545,.F.);
#60736=ORIENTED_EDGE('',*,*,#45579,.T.);
#60737=ORIENTED_EDGE('',*,*,#44605,.T.);
#60738=ORIENTED_EDGE('',*,*,#44609,.T.);
#60739=ORIENTED_EDGE('',*,*,#45580,.F.);
#60740=ORIENTED_EDGE('',*,*,#44610,.T.);
#60741=ORIENTED_EDGE('',*,*,#44606,.T.);
#60742=ORIENTED_EDGE('',*,*,#44617,.T.);
#60743=ORIENTED_EDGE('',*,*,#45543,.F.);
#60744=ORIENTED_EDGE('',*,*,#44614,.T.);
#60745=ORIENTED_EDGE('',*,*,#45581,.T.);
#60746=ORIENTED_EDGE('',*,*,#45540,.T.);
#60747=ORIENTED_EDGE('',*,*,#45581,.F.);
#60748=ORIENTED_EDGE('',*,*,#44613,.T.);
#60749=ORIENTED_EDGE('',*,*,#45582,.T.);
#60750=ORIENTED_EDGE('',*,*,#45583,.T.);
#60751=ORIENTED_EDGE('',*,*,#45582,.F.);
#60752=ORIENTED_EDGE('',*,*,#44612,.T.);
#60753=ORIENTED_EDGE('',*,*,#45584,.T.);
#60754=ORIENTED_EDGE('',*,*,#45585,.T.);
#60755=ORIENTED_EDGE('',*,*,#45584,.F.);
#60756=ORIENTED_EDGE('',*,*,#44611,.T.);
#60757=ORIENTED_EDGE('',*,*,#45580,.T.);
#60758=ORIENTED_EDGE('',*,*,#45586,.T.);
#60759=ORIENTED_EDGE('',*,*,#45587,.T.);
#60760=ORIENTED_EDGE('',*,*,#45586,.F.);
#60761=ORIENTED_EDGE('',*,*,#44616,.T.);
#60762=ORIENTED_EDGE('',*,*,#45588,.F.);
#60763=ORIENTED_EDGE('',*,*,#45589,.F.);
#60764=ORIENTED_EDGE('',*,*,#44618,.T.);
#60765=ORIENTED_EDGE('',*,*,#44619,.T.);
#60766=ORIENTED_EDGE('',*,*,#44631,.T.);
#60767=ORIENTED_EDGE('',*,*,#45590,.F.);
#60768=ORIENTED_EDGE('',*,*,#45588,.T.);
#60769=ORIENTED_EDGE('',*,*,#45589,.T.);
#60770=ORIENTED_EDGE('',*,*,#44630,.T.);
#60771=ORIENTED_EDGE('',*,*,#45591,.F.);
#60772=ORIENTED_EDGE('',*,*,#45592,.T.);
#60773=ORIENTED_EDGE('',*,*,#45590,.T.);
#60774=ORIENTED_EDGE('',*,*,#44629,.T.);
#60775=ORIENTED_EDGE('',*,*,#45593,.F.);
#60776=ORIENTED_EDGE('',*,*,#45594,.T.);
#60777=ORIENTED_EDGE('',*,*,#45591,.T.);
#60778=ORIENTED_EDGE('',*,*,#44628,.T.);
#60779=ORIENTED_EDGE('',*,*,#45539,.F.);
#60780=ORIENTED_EDGE('',*,*,#45542,.T.);
#60781=ORIENTED_EDGE('',*,*,#45593,.T.);
#60782=ORIENTED_EDGE('',*,*,#44627,.T.);
#60783=ORIENTED_EDGE('',*,*,#45595,.F.);
#60784=ORIENTED_EDGE('',*,*,#45596,.T.);
#60785=ORIENTED_EDGE('',*,*,#45538,.T.);
#60786=ORIENTED_EDGE('',*,*,#44624,.T.);
#60787=ORIENTED_EDGE('',*,*,#45597,.F.);
#60788=ORIENTED_EDGE('',*,*,#45598,.T.);
#60789=ORIENTED_EDGE('',*,*,#45595,.T.);
#60790=ORIENTED_EDGE('',*,*,#44623,.T.);
#60791=ORIENTED_EDGE('',*,*,#44633,.F.);
#60792=ORIENTED_EDGE('',*,*,#45599,.T.);
#60793=ORIENTED_EDGE('',*,*,#45597,.T.);
#60794=ORIENTED_EDGE('',*,*,#44622,.T.);
#60795=ORIENTED_EDGE('',*,*,#44635,.T.);
#60796=ORIENTED_EDGE('',*,*,#45600,.F.);
#60797=ORIENTED_EDGE('',*,*,#45601,.T.);
#60798=ORIENTED_EDGE('',*,*,#45599,.F.);
#60799=ORIENTED_EDGE('',*,*,#45602,.F.);
#60800=ORIENTED_EDGE('',*,*,#45600,.T.);
#60801=ORIENTED_EDGE('',*,*,#44637,.T.);
#60802=ORIENTED_EDGE('',*,*,#44643,.T.);
#60803=ORIENTED_EDGE('',*,*,#45603,.F.);
#60804=ORIENTED_EDGE('',*,*,#44644,.T.);
#60805=ORIENTED_EDGE('',*,*,#44638,.T.);
#60806=ORIENTED_EDGE('',*,*,#44651,.T.);
#60807=ORIENTED_EDGE('',*,*,#45533,.F.);
#60808=ORIENTED_EDGE('',*,*,#44648,.T.);
#60809=ORIENTED_EDGE('',*,*,#45604,.T.);
#60810=ORIENTED_EDGE('',*,*,#45530,.T.);
#60811=ORIENTED_EDGE('',*,*,#45604,.F.);
#60812=ORIENTED_EDGE('',*,*,#44647,.T.);
#60813=ORIENTED_EDGE('',*,*,#45605,.T.);
#60814=ORIENTED_EDGE('',*,*,#45606,.T.);
#60815=ORIENTED_EDGE('',*,*,#45605,.F.);
#60816=ORIENTED_EDGE('',*,*,#44646,.T.);
#60817=ORIENTED_EDGE('',*,*,#45607,.T.);
#60818=ORIENTED_EDGE('',*,*,#45608,.T.);
#60819=ORIENTED_EDGE('',*,*,#45607,.F.);
#60820=ORIENTED_EDGE('',*,*,#44645,.T.);
#60821=ORIENTED_EDGE('',*,*,#45603,.T.);
#60822=ORIENTED_EDGE('',*,*,#45609,.T.);
#60823=ORIENTED_EDGE('',*,*,#45610,.F.);
#60824=ORIENTED_EDGE('',*,*,#45611,.T.);
#60825=ORIENTED_EDGE('',*,*,#45602,.T.);
#60826=ORIENTED_EDGE('',*,*,#44642,.T.);
#60827=ORIENTED_EDGE('',*,*,#45535,.F.);
#60828=ORIENTED_EDGE('',*,*,#45612,.T.);
#60829=ORIENTED_EDGE('',*,*,#45610,.T.);
#60830=ORIENTED_EDGE('',*,*,#44641,.T.);
#60831=ORIENTED_EDGE('',*,*,#45613,.T.);
#60832=ORIENTED_EDGE('',*,*,#45609,.F.);
#60833=ORIENTED_EDGE('',*,*,#44650,.T.);
#60834=ORIENTED_EDGE('',*,*,#45614,.F.);
#60835=ORIENTED_EDGE('',*,*,#45615,.F.);
#60836=ORIENTED_EDGE('',*,*,#44652,.T.);
#60837=ORIENTED_EDGE('',*,*,#44653,.T.);
#60838=ORIENTED_EDGE('',*,*,#44665,.T.);
#60839=ORIENTED_EDGE('',*,*,#45616,.F.);
#60840=ORIENTED_EDGE('',*,*,#45614,.T.);
#60841=ORIENTED_EDGE('',*,*,#45615,.T.);
#60842=ORIENTED_EDGE('',*,*,#44664,.T.);
#60843=ORIENTED_EDGE('',*,*,#45617,.F.);
#60844=ORIENTED_EDGE('',*,*,#45618,.T.);
#60845=ORIENTED_EDGE('',*,*,#45616,.T.);
#60846=ORIENTED_EDGE('',*,*,#44663,.T.);
#60847=ORIENTED_EDGE('',*,*,#45619,.F.);
#60848=ORIENTED_EDGE('',*,*,#45620,.T.);
#60849=ORIENTED_EDGE('',*,*,#45617,.T.);
#60850=ORIENTED_EDGE('',*,*,#44662,.T.);
#60851=ORIENTED_EDGE('',*,*,#45529,.F.);
#60852=ORIENTED_EDGE('',*,*,#45532,.T.);
#60853=ORIENTED_EDGE('',*,*,#45619,.T.);
#60854=ORIENTED_EDGE('',*,*,#44661,.T.);
#60855=ORIENTED_EDGE('',*,*,#45621,.F.);
#60856=ORIENTED_EDGE('',*,*,#45622,.T.);
#60857=ORIENTED_EDGE('',*,*,#45527,.T.);
#60858=ORIENTED_EDGE('',*,*,#44658,.T.);
#60859=ORIENTED_EDGE('',*,*,#45623,.F.);
#60860=ORIENTED_EDGE('',*,*,#45624,.T.);
#60861=ORIENTED_EDGE('',*,*,#45621,.T.);
#60862=ORIENTED_EDGE('',*,*,#44657,.T.);
#60863=ORIENTED_EDGE('',*,*,#44666,.F.);
#60864=ORIENTED_EDGE('',*,*,#45335,.T.);
#60865=ORIENTED_EDGE('',*,*,#45623,.T.);
#60866=ORIENTED_EDGE('',*,*,#44656,.T.);
#60867=ORIENTED_EDGE('',*,*,#45625,.F.);
#60868=ORIENTED_EDGE('',*,*,#45626,.F.);
#60869=ORIENTED_EDGE('',*,*,#44667,.F.);
#60870=ORIENTED_EDGE('',*,*,#45627,.F.);
#60871=ORIENTED_EDGE('',*,*,#44671,.F.);
#60872=ORIENTED_EDGE('',*,*,#44679,.T.);
#60873=ORIENTED_EDGE('',*,*,#45628,.T.);
#60874=ORIENTED_EDGE('',*,*,#44669,.T.);
#60875=ORIENTED_EDGE('',*,*,#45073,.F.);
#60876=ORIENTED_EDGE('',*,*,#44668,.T.);
#60877=ORIENTED_EDGE('',*,*,#45629,.T.);
#60878=ORIENTED_EDGE('',*,*,#45066,.T.);
#60879=ORIENTED_EDGE('',*,*,#45628,.F.);
#60880=ORIENTED_EDGE('',*,*,#44678,.T.);
#60881=ORIENTED_EDGE('',*,*,#45630,.T.);
#60882=ORIENTED_EDGE('',*,*,#45627,.T.);
#60883=ORIENTED_EDGE('',*,*,#45630,.F.);
#60884=ORIENTED_EDGE('',*,*,#44677,.T.);
#60885=ORIENTED_EDGE('',*,*,#45631,.T.);
#60886=ORIENTED_EDGE('',*,*,#45632,.T.);
#60887=ORIENTED_EDGE('',*,*,#45631,.F.);
#60888=ORIENTED_EDGE('',*,*,#44676,.T.);
#60889=ORIENTED_EDGE('',*,*,#45369,.T.);
#60890=ORIENTED_EDGE('',*,*,#45372,.T.);
#60891=ORIENTED_EDGE('',*,*,#44681,.F.);
#60892=ORIENTED_EDGE('',*,*,#45633,.T.);
#60893=ORIENTED_EDGE('',*,*,#45368,.T.);
#60894=ORIENTED_EDGE('',*,*,#44673,.T.);
#60895=ORIENTED_EDGE('',*,*,#45367,.T.);
#60896=ORIENTED_EDGE('',*,*,#45633,.F.);
#60897=ORIENTED_EDGE('',*,*,#44683,.T.);
#60898=ORIENTED_EDGE('',*,*,#45634,.F.);
#60899=ORIENTED_EDGE('',*,*,#45365,.F.);
#60900=ORIENTED_EDGE('',*,*,#45634,.T.);
#60901=ORIENTED_EDGE('',*,*,#44685,.T.);
#60902=ORIENTED_EDGE('',*,*,#44692,.T.);
#60903=ORIENTED_EDGE('',*,*,#45635,.F.);
#60904=ORIENTED_EDGE('',*,*,#45362,.T.);
#60905=ORIENTED_EDGE('',*,*,#45363,.T.);
#60906=ORIENTED_EDGE('',*,*,#44689,.T.);
#60907=ORIENTED_EDGE('',*,*,#45636,.F.);
#60908=ORIENTED_EDGE('',*,*,#45360,.T.);
#60909=ORIENTED_EDGE('',*,*,#45635,.T.);
#60910=ORIENTED_EDGE('',*,*,#44688,.T.);
#60911=ORIENTED_EDGE('',*,*,#44693,.F.);
#60912=ORIENTED_EDGE('',*,*,#44695,.T.);
#60913=ORIENTED_EDGE('',*,*,#45636,.T.);
#60914=ORIENTED_EDGE('',*,*,#44687,.T.);
#60915=ORIENTED_EDGE('',*,*,#44698,.F.);
#60916=ORIENTED_EDGE('',*,*,#44704,.T.);
#60917=ORIENTED_EDGE('',*,*,#45637,.T.);
#60918=ORIENTED_EDGE('',*,*,#44696,.T.);
#60919=ORIENTED_EDGE('',*,*,#45637,.F.);
#60920=ORIENTED_EDGE('',*,*,#44703,.T.);
#60921=ORIENTED_EDGE('',*,*,#45358,.T.);
#60922=ORIENTED_EDGE('',*,*,#45361,.T.);
#60923=ORIENTED_EDGE('',*,*,#44711,.F.);
#60924=ORIENTED_EDGE('',*,*,#44716,.T.);
#60925=ORIENTED_EDGE('',*,*,#45354,.T.);
#60926=ORIENTED_EDGE('',*,*,#44713,.T.);
#60927=ORIENTED_EDGE('',*,*,#44719,.F.);
#60928=ORIENTED_EDGE('',*,*,#44723,.T.);
#60929=ORIENTED_EDGE('',*,*,#45353,.T.);
#60930=ORIENTED_EDGE('',*,*,#44717,.T.);
#60931=ORIENTED_EDGE('',*,*,#44732,.F.);
#60932=ORIENTED_EDGE('',*,*,#45638,.T.);
#60933=ORIENTED_EDGE('',*,*,#45639,.T.);
#60934=ORIENTED_EDGE('',*,*,#44935,.T.);
#60935=ORIENTED_EDGE('',*,*,#44735,.T.);
#60936=ORIENTED_EDGE('',*,*,#45640,.F.);
#60937=ORIENTED_EDGE('',*,*,#45641,.T.);
#60938=ORIENTED_EDGE('',*,*,#45638,.F.);
#60939=ORIENTED_EDGE('',*,*,#45642,.F.);
#60940=ORIENTED_EDGE('',*,*,#45640,.T.);
#60941=ORIENTED_EDGE('',*,*,#44737,.T.);
#60942=ORIENTED_EDGE('',*,*,#45145,.T.);
#60943=ORIENTED_EDGE('',*,*,#44739,.F.);
#60944=ORIENTED_EDGE('',*,*,#45643,.T.);
#60945=ORIENTED_EDGE('',*,*,#45644,.T.);
#60946=ORIENTED_EDGE('',*,*,#45218,.T.);
#60947=ORIENTED_EDGE('',*,*,#44742,.T.);
#60948=ORIENTED_EDGE('',*,*,#45645,.F.);
#60949=ORIENTED_EDGE('',*,*,#45646,.T.);
#60950=ORIENTED_EDGE('',*,*,#45643,.F.);
#60951=ORIENTED_EDGE('',*,*,#45647,.F.);
#60952=ORIENTED_EDGE('',*,*,#45645,.T.);
#60953=ORIENTED_EDGE('',*,*,#44744,.T.);
#60954=ORIENTED_EDGE('',*,*,#44748,.T.);
#60955=ORIENTED_EDGE('',*,*,#45648,.T.);
#60956=ORIENTED_EDGE('',*,*,#45649,.T.);
#60957=ORIENTED_EDGE('',*,*,#44745,.T.);
#60958=ORIENTED_EDGE('',*,*,#45650,.F.);
#60959=ORIENTED_EDGE('',*,*,#45651,.F.);
#60960=ORIENTED_EDGE('',*,*,#45427,.T.);
#60961=ORIENTED_EDGE('',*,*,#45652,.T.);
#60962=ORIENTED_EDGE('',*,*,#44756,.T.);
#60963=ORIENTED_EDGE('',*,*,#45653,.F.);
#60964=ORIENTED_EDGE('',*,*,#45654,.T.);
#60965=ORIENTED_EDGE('',*,*,#45651,.T.);
#60966=ORIENTED_EDGE('',*,*,#44755,.T.);
#60967=ORIENTED_EDGE('',*,*,#45655,.F.);
#60968=ORIENTED_EDGE('',*,*,#45656,.T.);
#60969=ORIENTED_EDGE('',*,*,#45653,.T.);
#60970=ORIENTED_EDGE('',*,*,#44754,.T.);
#60971=ORIENTED_EDGE('',*,*,#45657,.F.);
#60972=ORIENTED_EDGE('',*,*,#45658,.T.);
#60973=ORIENTED_EDGE('',*,*,#45655,.T.);
#60974=ORIENTED_EDGE('',*,*,#44753,.T.);
#60975=ORIENTED_EDGE('',*,*,#45659,.F.);
#60976=ORIENTED_EDGE('',*,*,#45660,.T.);
#60977=ORIENTED_EDGE('',*,*,#45657,.T.);
#60978=ORIENTED_EDGE('',*,*,#44752,.T.);
#60979=ORIENTED_EDGE('',*,*,#45661,.F.);
#60980=ORIENTED_EDGE('',*,*,#45662,.T.);
#60981=ORIENTED_EDGE('',*,*,#45659,.T.);
#60982=ORIENTED_EDGE('',*,*,#44751,.T.);
#60983=ORIENTED_EDGE('',*,*,#44757,.F.);
#60984=ORIENTED_EDGE('',*,*,#44759,.T.);
#60985=ORIENTED_EDGE('',*,*,#45661,.T.);
#60986=ORIENTED_EDGE('',*,*,#44750,.T.);
#60987=ORIENTED_EDGE('',*,*,#45663,.F.);
#60988=ORIENTED_EDGE('',*,*,#45664,.T.);
#60989=ORIENTED_EDGE('',*,*,#45647,.T.);
#60990=ORIENTED_EDGE('',*,*,#44747,.T.);
#60991=ORIENTED_EDGE('',*,*,#45649,.F.);
#60992=ORIENTED_EDGE('',*,*,#45665,.T.);
#60993=ORIENTED_EDGE('',*,*,#45663,.T.);
#60994=ORIENTED_EDGE('',*,*,#44746,.T.);
#60995=ORIENTED_EDGE('',*,*,#45666,.T.);
#60996=ORIENTED_EDGE('',*,*,#45662,.F.);
#60997=ORIENTED_EDGE('',*,*,#44758,.T.);
#60998=ORIENTED_EDGE('',*,*,#45667,.F.);
#60999=ORIENTED_EDGE('',*,*,#44762,.F.);
#61000=ORIENTED_EDGE('',*,*,#44774,.T.);
#61001=ORIENTED_EDGE('',*,*,#45668,.T.);
#61002=ORIENTED_EDGE('',*,*,#44760,.T.);
#61003=ORIENTED_EDGE('',*,*,#45668,.F.);
#61004=ORIENTED_EDGE('',*,*,#44773,.T.);
#61005=ORIENTED_EDGE('',*,*,#45669,.F.);
#61006=ORIENTED_EDGE('',*,*,#45667,.T.);
#61007=ORIENTED_EDGE('',*,*,#45670,.F.);
#61008=ORIENTED_EDGE('',*,*,#45671,.T.);
#61009=ORIENTED_EDGE('',*,*,#45669,.T.);
#61010=ORIENTED_EDGE('',*,*,#44772,.T.);
#61011=ORIENTED_EDGE('',*,*,#45672,.F.);
#61012=ORIENTED_EDGE('',*,*,#45673,.T.);
#61013=ORIENTED_EDGE('',*,*,#45670,.T.);
#61014=ORIENTED_EDGE('',*,*,#44771,.T.);
#61015=ORIENTED_EDGE('',*,*,#45674,.F.);
#61016=ORIENTED_EDGE('',*,*,#45675,.T.);
#61017=ORIENTED_EDGE('',*,*,#45672,.T.);
#61018=ORIENTED_EDGE('',*,*,#44770,.T.);
#61019=ORIENTED_EDGE('',*,*,#45676,.F.);
#61020=ORIENTED_EDGE('',*,*,#45677,.T.);
#61021=ORIENTED_EDGE('',*,*,#45674,.T.);
#61022=ORIENTED_EDGE('',*,*,#44769,.T.);
#61023=ORIENTED_EDGE('',*,*,#45678,.F.);
#61024=ORIENTED_EDGE('',*,*,#45429,.T.);
#61025=ORIENTED_EDGE('',*,*,#45676,.T.);
#61026=ORIENTED_EDGE('',*,*,#44768,.T.);
#61027=ORIENTED_EDGE('',*,*,#44767,.T.);
#61028=ORIENTED_EDGE('',*,*,#45679,.F.);
#61029=ORIENTED_EDGE('',*,*,#45680,.T.);
#61030=ORIENTED_EDGE('',*,*,#45681,.F.);
#61031=ORIENTED_EDGE('',*,*,#45682,.F.);
#61032=ORIENTED_EDGE('',*,*,#45683,.T.);
#61033=ORIENTED_EDGE('',*,*,#45679,.T.);
#61034=ORIENTED_EDGE('',*,*,#44766,.T.);
#61035=ORIENTED_EDGE('',*,*,#45684,.F.);
#61036=ORIENTED_EDGE('',*,*,#45685,.T.);
#61037=ORIENTED_EDGE('',*,*,#45682,.T.);
#61038=ORIENTED_EDGE('',*,*,#44765,.T.);
#61039=ORIENTED_EDGE('',*,*,#44776,.F.);
#61040=ORIENTED_EDGE('',*,*,#45686,.T.);
#61041=ORIENTED_EDGE('',*,*,#45684,.T.);
#61042=ORIENTED_EDGE('',*,*,#44764,.T.);
#61043=ORIENTED_EDGE('',*,*,#44778,.T.);
#61044=ORIENTED_EDGE('',*,*,#45687,.F.);
#61045=ORIENTED_EDGE('',*,*,#45688,.T.);
#61046=ORIENTED_EDGE('',*,*,#45686,.F.);
#61047=ORIENTED_EDGE('',*,*,#45689,.F.);
#61048=ORIENTED_EDGE('',*,*,#45687,.T.);
#61049=ORIENTED_EDGE('',*,*,#44780,.T.);
#61050=ORIENTED_EDGE('',*,*,#44792,.T.);
#61051=ORIENTED_EDGE('',*,*,#45690,.F.);
#61052=ORIENTED_EDGE('',*,*,#44783,.T.);
#61053=ORIENTED_EDGE('',*,*,#44781,.T.);
#61054=ORIENTED_EDGE('',*,*,#44794,.T.);
#61055=ORIENTED_EDGE('',*,*,#45691,.F.);
#61056=ORIENTED_EDGE('',*,*,#45692,.T.);
#61057=ORIENTED_EDGE('',*,*,#45689,.T.);
#61058=ORIENTED_EDGE('',*,*,#44791,.T.);
#61059=ORIENTED_EDGE('',*,*,#45693,.F.);
#61060=ORIENTED_EDGE('',*,*,#45694,.T.);
#61061=ORIENTED_EDGE('',*,*,#45691,.T.);
#61062=ORIENTED_EDGE('',*,*,#44790,.T.);
#61063=ORIENTED_EDGE('',*,*,#45695,.F.);
#61064=ORIENTED_EDGE('',*,*,#45696,.F.);
#61065=ORIENTED_EDGE('',*,*,#45434,.T.);
#61066=ORIENTED_EDGE('',*,*,#45697,.T.);
#61067=ORIENTED_EDGE('',*,*,#44789,.T.);
#61068=ORIENTED_EDGE('',*,*,#45698,.F.);
#61069=ORIENTED_EDGE('',*,*,#45699,.T.);
#61070=ORIENTED_EDGE('',*,*,#45696,.T.);
#61071=ORIENTED_EDGE('',*,*,#44788,.T.);
#61072=ORIENTED_EDGE('',*,*,#45700,.F.);
#61073=ORIENTED_EDGE('',*,*,#45701,.T.);
#61074=ORIENTED_EDGE('',*,*,#45698,.T.);
#61075=ORIENTED_EDGE('',*,*,#44787,.T.);
#61076=ORIENTED_EDGE('',*,*,#45702,.T.);
#61077=ORIENTED_EDGE('',*,*,#45703,.T.);
#61078=ORIENTED_EDGE('',*,*,#45700,.T.);
#61079=ORIENTED_EDGE('',*,*,#44786,.T.);
#61080=ORIENTED_EDGE('',*,*,#45702,.F.);
#61081=ORIENTED_EDGE('',*,*,#44785,.T.);
#61082=ORIENTED_EDGE('',*,*,#45704,.T.);
#61083=ORIENTED_EDGE('',*,*,#45705,.T.);
#61084=ORIENTED_EDGE('',*,*,#45704,.F.);
#61085=ORIENTED_EDGE('',*,*,#44784,.T.);
#61086=ORIENTED_EDGE('',*,*,#45690,.T.);
#61087=ORIENTED_EDGE('',*,*,#45706,.T.);
#61088=ORIENTED_EDGE('',*,*,#45707,.T.);
#61089=ORIENTED_EDGE('',*,*,#45706,.F.);
#61090=ORIENTED_EDGE('',*,*,#44793,.T.);
#61091=ORIENTED_EDGE('',*,*,#45708,.F.);
#61092=ORIENTED_EDGE('',*,*,#45709,.F.);
#61093=ORIENTED_EDGE('',*,*,#44795,.T.);
#61094=ORIENTED_EDGE('',*,*,#44796,.T.);
#61095=ORIENTED_EDGE('',*,*,#44807,.T.);
#61096=ORIENTED_EDGE('',*,*,#45710,.F.);
#61097=ORIENTED_EDGE('',*,*,#45708,.T.);
#61098=ORIENTED_EDGE('',*,*,#45709,.T.);
#61099=ORIENTED_EDGE('',*,*,#44806,.T.);
#61100=ORIENTED_EDGE('',*,*,#45711,.F.);
#61101=ORIENTED_EDGE('',*,*,#45712,.T.);
#61102=ORIENTED_EDGE('',*,*,#45710,.T.);
#61103=ORIENTED_EDGE('',*,*,#44805,.T.);
#61104=ORIENTED_EDGE('',*,*,#45713,.F.);
#61105=ORIENTED_EDGE('',*,*,#45714,.T.);
#61106=ORIENTED_EDGE('',*,*,#45711,.T.);
#61107=ORIENTED_EDGE('',*,*,#44804,.T.);
#61108=ORIENTED_EDGE('',*,*,#45715,.F.);
#61109=ORIENTED_EDGE('',*,*,#45716,.T.);
#61110=ORIENTED_EDGE('',*,*,#45713,.T.);
#61111=ORIENTED_EDGE('',*,*,#44803,.T.);
#61112=ORIENTED_EDGE('',*,*,#45717,.F.);
#61113=ORIENTED_EDGE('',*,*,#45718,.T.);
#61114=ORIENTED_EDGE('',*,*,#45715,.T.);
#61115=ORIENTED_EDGE('',*,*,#44802,.T.);
#61116=ORIENTED_EDGE('',*,*,#45719,.F.);
#61117=ORIENTED_EDGE('',*,*,#45436,.T.);
#61118=ORIENTED_EDGE('',*,*,#45717,.T.);
#61119=ORIENTED_EDGE('',*,*,#44801,.T.);
#61120=ORIENTED_EDGE('',*,*,#44800,.T.);
#61121=ORIENTED_EDGE('',*,*,#45720,.F.);
#61122=ORIENTED_EDGE('',*,*,#45721,.T.);
#61123=ORIENTED_EDGE('',*,*,#45722,.F.);
#61124=ORIENTED_EDGE('',*,*,#44809,.F.);
#61125=ORIENTED_EDGE('',*,*,#45723,.T.);
#61126=ORIENTED_EDGE('',*,*,#45720,.T.);
#61127=ORIENTED_EDGE('',*,*,#44799,.T.);
#61128=ORIENTED_EDGE('',*,*,#44811,.F.);
#61129=ORIENTED_EDGE('',*,*,#45724,.F.);
#61130=ORIENTED_EDGE('',*,*,#45725,.F.);
#61131=ORIENTED_EDGE('',*,*,#45723,.F.);
#61132=ORIENTED_EDGE('',*,*,#45726,.F.);
#61133=ORIENTED_EDGE('',*,*,#45724,.T.);
#61134=ORIENTED_EDGE('',*,*,#44813,.T.);
#61135=ORIENTED_EDGE('',*,*,#44817,.T.);
#61136=ORIENTED_EDGE('',*,*,#45727,.F.);
#61137=ORIENTED_EDGE('',*,*,#44818,.T.);
#61138=ORIENTED_EDGE('',*,*,#44814,.T.);
#61139=ORIENTED_EDGE('',*,*,#44826,.T.);
#61140=ORIENTED_EDGE('',*,*,#45728,.T.);
#61141=ORIENTED_EDGE('',*,*,#45726,.T.);
#61142=ORIENTED_EDGE('',*,*,#44816,.T.);
#61143=ORIENTED_EDGE('',*,*,#45729,.F.);
#61144=ORIENTED_EDGE('',*,*,#45730,.F.);
#61145=ORIENTED_EDGE('',*,*,#44824,.T.);
#61146=ORIENTED_EDGE('',*,*,#45731,.T.);
#61147=ORIENTED_EDGE('',*,*,#45440,.T.);
#61148=ORIENTED_EDGE('',*,*,#45731,.F.);
#61149=ORIENTED_EDGE('',*,*,#44823,.T.);
#61150=ORIENTED_EDGE('',*,*,#45732,.T.);
#61151=ORIENTED_EDGE('',*,*,#45733,.T.);
#61152=ORIENTED_EDGE('',*,*,#45732,.F.);
#61153=ORIENTED_EDGE('',*,*,#44822,.T.);
#61154=ORIENTED_EDGE('',*,*,#45734,.T.);
#61155=ORIENTED_EDGE('',*,*,#45735,.T.);
#61156=ORIENTED_EDGE('',*,*,#45734,.F.);
#61157=ORIENTED_EDGE('',*,*,#44821,.T.);
#61158=ORIENTED_EDGE('',*,*,#45736,.T.);
#61159=ORIENTED_EDGE('',*,*,#45737,.T.);
#61160=ORIENTED_EDGE('',*,*,#45736,.F.);
#61161=ORIENTED_EDGE('',*,*,#44820,.T.);
#61162=ORIENTED_EDGE('',*,*,#45738,.T.);
#61163=ORIENTED_EDGE('',*,*,#45739,.T.);
#61164=ORIENTED_EDGE('',*,*,#45738,.F.);
#61165=ORIENTED_EDGE('',*,*,#44819,.T.);
#61166=ORIENTED_EDGE('',*,*,#45727,.T.);
#61167=ORIENTED_EDGE('',*,*,#45740,.T.);
#61168=ORIENTED_EDGE('',*,*,#45741,.T.);
#61169=ORIENTED_EDGE('',*,*,#45740,.F.);
#61170=ORIENTED_EDGE('',*,*,#44825,.T.);
#61171=ORIENTED_EDGE('',*,*,#45742,.F.);
#61172=ORIENTED_EDGE('',*,*,#45743,.F.);
#61173=ORIENTED_EDGE('',*,*,#44827,.T.);
#61174=ORIENTED_EDGE('',*,*,#44828,.T.);
#61175=ORIENTED_EDGE('',*,*,#44839,.T.);
#61176=ORIENTED_EDGE('',*,*,#45744,.F.);
#61177=ORIENTED_EDGE('',*,*,#45742,.T.);
#61178=ORIENTED_EDGE('',*,*,#45743,.T.);
#61179=ORIENTED_EDGE('',*,*,#44838,.T.);
#61180=ORIENTED_EDGE('',*,*,#45745,.F.);
#61181=ORIENTED_EDGE('',*,*,#45746,.T.);
#61182=ORIENTED_EDGE('',*,*,#45744,.T.);
#61183=ORIENTED_EDGE('',*,*,#44837,.T.);
#61184=ORIENTED_EDGE('',*,*,#45747,.F.);
#61185=ORIENTED_EDGE('',*,*,#45748,.T.);
#61186=ORIENTED_EDGE('',*,*,#45745,.T.);
#61187=ORIENTED_EDGE('',*,*,#44836,.T.);
#61188=ORIENTED_EDGE('',*,*,#45749,.F.);
#61189=ORIENTED_EDGE('',*,*,#45750,.T.);
#61190=ORIENTED_EDGE('',*,*,#45747,.T.);
#61191=ORIENTED_EDGE('',*,*,#44835,.T.);
#61192=ORIENTED_EDGE('',*,*,#45751,.F.);
#61193=ORIENTED_EDGE('',*,*,#45752,.T.);
#61194=ORIENTED_EDGE('',*,*,#45749,.T.);
#61195=ORIENTED_EDGE('',*,*,#44834,.T.);
#61196=ORIENTED_EDGE('',*,*,#45753,.F.);
#61197=ORIENTED_EDGE('',*,*,#45442,.T.);
#61198=ORIENTED_EDGE('',*,*,#45751,.T.);
#61199=ORIENTED_EDGE('',*,*,#44833,.T.);
#61200=ORIENTED_EDGE('',*,*,#44832,.T.);
#61201=ORIENTED_EDGE('',*,*,#45754,.F.);
#61202=ORIENTED_EDGE('',*,*,#45755,.T.);
#61203=ORIENTED_EDGE('',*,*,#45756,.F.);
#61204=ORIENTED_EDGE('',*,*,#44841,.F.);
#61205=ORIENTED_EDGE('',*,*,#45757,.T.);
#61206=ORIENTED_EDGE('',*,*,#45754,.T.);
#61207=ORIENTED_EDGE('',*,*,#44831,.T.);
#61208=ORIENTED_EDGE('',*,*,#44843,.F.);
#61209=ORIENTED_EDGE('',*,*,#45758,.F.);
#61210=ORIENTED_EDGE('',*,*,#45759,.F.);
#61211=ORIENTED_EDGE('',*,*,#45757,.F.);
#61212=ORIENTED_EDGE('',*,*,#44845,.F.);
#61213=ORIENTED_EDGE('',*,*,#44856,.T.);
#61214=ORIENTED_EDGE('',*,*,#45760,.T.);
#61215=ORIENTED_EDGE('',*,*,#45758,.T.);
#61216=ORIENTED_EDGE('',*,*,#45761,.F.);
#61217=ORIENTED_EDGE('',*,*,#44848,.T.);
#61218=ORIENTED_EDGE('',*,*,#44846,.T.);
#61219=ORIENTED_EDGE('',*,*,#44858,.T.);
#61220=ORIENTED_EDGE('',*,*,#45762,.T.);
#61221=ORIENTED_EDGE('',*,*,#45760,.F.);
#61222=ORIENTED_EDGE('',*,*,#44855,.T.);
#61223=ORIENTED_EDGE('',*,*,#45763,.F.);
#61224=ORIENTED_EDGE('',*,*,#45764,.F.);
#61225=ORIENTED_EDGE('',*,*,#44854,.T.);
#61226=ORIENTED_EDGE('',*,*,#45765,.T.);
#61227=ORIENTED_EDGE('',*,*,#45446,.T.);
#61228=ORIENTED_EDGE('',*,*,#45765,.F.);
#61229=ORIENTED_EDGE('',*,*,#44853,.T.);
#61230=ORIENTED_EDGE('',*,*,#45766,.T.);
#61231=ORIENTED_EDGE('',*,*,#45767,.T.);
#61232=ORIENTED_EDGE('',*,*,#45766,.F.);
#61233=ORIENTED_EDGE('',*,*,#44852,.T.);
#61234=ORIENTED_EDGE('',*,*,#45768,.T.);
#61235=ORIENTED_EDGE('',*,*,#45769,.T.);
#61236=ORIENTED_EDGE('',*,*,#45768,.F.);
#61237=ORIENTED_EDGE('',*,*,#44851,.T.);
#61238=ORIENTED_EDGE('',*,*,#45770,.T.);
#61239=ORIENTED_EDGE('',*,*,#45771,.T.);
#61240=ORIENTED_EDGE('',*,*,#45770,.F.);
#61241=ORIENTED_EDGE('',*,*,#44850,.T.);
#61242=ORIENTED_EDGE('',*,*,#45772,.T.);
#61243=ORIENTED_EDGE('',*,*,#45773,.T.);
#61244=ORIENTED_EDGE('',*,*,#45772,.F.);
#61245=ORIENTED_EDGE('',*,*,#44849,.T.);
#61246=ORIENTED_EDGE('',*,*,#45761,.T.);
#61247=ORIENTED_EDGE('',*,*,#45774,.T.);
#61248=ORIENTED_EDGE('',*,*,#45775,.T.);
#61249=ORIENTED_EDGE('',*,*,#45774,.F.);
#61250=ORIENTED_EDGE('',*,*,#44857,.T.);
#61251=ORIENTED_EDGE('',*,*,#45776,.F.);
#61252=ORIENTED_EDGE('',*,*,#45777,.F.);
#61253=ORIENTED_EDGE('',*,*,#44859,.T.);
#61254=ORIENTED_EDGE('',*,*,#44860,.T.);
#61255=ORIENTED_EDGE('',*,*,#44871,.T.);
#61256=ORIENTED_EDGE('',*,*,#45778,.F.);
#61257=ORIENTED_EDGE('',*,*,#45776,.T.);
#61258=ORIENTED_EDGE('',*,*,#45777,.T.);
#61259=ORIENTED_EDGE('',*,*,#44870,.T.);
#61260=ORIENTED_EDGE('',*,*,#45779,.F.);
#61261=ORIENTED_EDGE('',*,*,#45780,.T.);
#61262=ORIENTED_EDGE('',*,*,#45778,.T.);
#61263=ORIENTED_EDGE('',*,*,#44869,.T.);
#61264=ORIENTED_EDGE('',*,*,#45781,.F.);
#61265=ORIENTED_EDGE('',*,*,#45782,.T.);
#61266=ORIENTED_EDGE('',*,*,#45779,.T.);
#61267=ORIENTED_EDGE('',*,*,#44868,.T.);
#61268=ORIENTED_EDGE('',*,*,#45783,.F.);
#61269=ORIENTED_EDGE('',*,*,#45784,.T.);
#61270=ORIENTED_EDGE('',*,*,#45781,.T.);
#61271=ORIENTED_EDGE('',*,*,#44867,.T.);
#61272=ORIENTED_EDGE('',*,*,#45785,.F.);
#61273=ORIENTED_EDGE('',*,*,#45786,.T.);
#61274=ORIENTED_EDGE('',*,*,#45783,.T.);
#61275=ORIENTED_EDGE('',*,*,#44866,.T.);
#61276=ORIENTED_EDGE('',*,*,#45787,.F.);
#61277=ORIENTED_EDGE('',*,*,#45448,.T.);
#61278=ORIENTED_EDGE('',*,*,#45785,.T.);
#61279=ORIENTED_EDGE('',*,*,#44865,.T.);
#61280=ORIENTED_EDGE('',*,*,#44864,.T.);
#61281=ORIENTED_EDGE('',*,*,#45788,.F.);
#61282=ORIENTED_EDGE('',*,*,#45789,.T.);
#61283=ORIENTED_EDGE('',*,*,#45790,.F.);
#61284=ORIENTED_EDGE('',*,*,#44873,.F.);
#61285=ORIENTED_EDGE('',*,*,#45791,.T.);
#61286=ORIENTED_EDGE('',*,*,#45788,.T.);
#61287=ORIENTED_EDGE('',*,*,#44863,.T.);
#61288=ORIENTED_EDGE('',*,*,#44875,.F.);
#61289=ORIENTED_EDGE('',*,*,#45792,.F.);
#61290=ORIENTED_EDGE('',*,*,#45793,.F.);
#61291=ORIENTED_EDGE('',*,*,#45791,.F.);
#61292=ORIENTED_EDGE('',*,*,#44877,.F.);
#61293=ORIENTED_EDGE('',*,*,#44888,.T.);
#61294=ORIENTED_EDGE('',*,*,#45794,.T.);
#61295=ORIENTED_EDGE('',*,*,#45792,.T.);
#61296=ORIENTED_EDGE('',*,*,#45795,.F.);
#61297=ORIENTED_EDGE('',*,*,#44880,.T.);
#61298=ORIENTED_EDGE('',*,*,#44878,.T.);
#61299=ORIENTED_EDGE('',*,*,#44890,.T.);
#61300=ORIENTED_EDGE('',*,*,#45796,.T.);
#61301=ORIENTED_EDGE('',*,*,#45794,.F.);
#61302=ORIENTED_EDGE('',*,*,#44887,.T.);
#61303=ORIENTED_EDGE('',*,*,#45797,.F.);
#61304=ORIENTED_EDGE('',*,*,#45798,.F.);
#61305=ORIENTED_EDGE('',*,*,#44886,.T.);
#61306=ORIENTED_EDGE('',*,*,#45799,.T.);
#61307=ORIENTED_EDGE('',*,*,#45452,.T.);
#61308=ORIENTED_EDGE('',*,*,#45799,.F.);
#61309=ORIENTED_EDGE('',*,*,#44885,.T.);
#61310=ORIENTED_EDGE('',*,*,#45800,.T.);
#61311=ORIENTED_EDGE('',*,*,#45801,.T.);
#61312=ORIENTED_EDGE('',*,*,#45800,.F.);
#61313=ORIENTED_EDGE('',*,*,#44884,.T.);
#61314=ORIENTED_EDGE('',*,*,#45802,.T.);
#61315=ORIENTED_EDGE('',*,*,#45803,.T.);
#61316=ORIENTED_EDGE('',*,*,#45802,.F.);
#61317=ORIENTED_EDGE('',*,*,#44883,.T.);
#61318=ORIENTED_EDGE('',*,*,#45804,.T.);
#61319=ORIENTED_EDGE('',*,*,#45805,.T.);
#61320=ORIENTED_EDGE('',*,*,#45804,.F.);
#61321=ORIENTED_EDGE('',*,*,#44882,.T.);
#61322=ORIENTED_EDGE('',*,*,#45806,.T.);
#61323=ORIENTED_EDGE('',*,*,#45807,.T.);
#61324=ORIENTED_EDGE('',*,*,#45806,.F.);
#61325=ORIENTED_EDGE('',*,*,#44881,.T.);
#61326=ORIENTED_EDGE('',*,*,#45795,.T.);
#61327=ORIENTED_EDGE('',*,*,#45808,.T.);
#61328=ORIENTED_EDGE('',*,*,#45809,.T.);
#61329=ORIENTED_EDGE('',*,*,#45808,.F.);
#61330=ORIENTED_EDGE('',*,*,#44889,.T.);
#61331=ORIENTED_EDGE('',*,*,#45810,.F.);
#61332=ORIENTED_EDGE('',*,*,#44893,.F.);
#61333=ORIENTED_EDGE('',*,*,#44904,.T.);
#61334=ORIENTED_EDGE('',*,*,#45811,.T.);
#61335=ORIENTED_EDGE('',*,*,#44891,.T.);
#61336=ORIENTED_EDGE('',*,*,#45811,.F.);
#61337=ORIENTED_EDGE('',*,*,#44903,.T.);
#61338=ORIENTED_EDGE('',*,*,#45812,.F.);
#61339=ORIENTED_EDGE('',*,*,#45810,.T.);
#61340=ORIENTED_EDGE('',*,*,#45813,.F.);
#61341=ORIENTED_EDGE('',*,*,#45814,.T.);
#61342=ORIENTED_EDGE('',*,*,#45812,.T.);
#61343=ORIENTED_EDGE('',*,*,#44902,.T.);
#61344=ORIENTED_EDGE('',*,*,#45815,.F.);
#61345=ORIENTED_EDGE('',*,*,#45816,.T.);
#61346=ORIENTED_EDGE('',*,*,#45813,.T.);
#61347=ORIENTED_EDGE('',*,*,#44901,.T.);
#61348=ORIENTED_EDGE('',*,*,#45817,.F.);
#61349=ORIENTED_EDGE('',*,*,#45818,.T.);
#61350=ORIENTED_EDGE('',*,*,#45815,.T.);
#61351=ORIENTED_EDGE('',*,*,#44900,.T.);
#61352=ORIENTED_EDGE('',*,*,#45819,.F.);
#61353=ORIENTED_EDGE('',*,*,#45820,.T.);
#61354=ORIENTED_EDGE('',*,*,#45817,.T.);
#61355=ORIENTED_EDGE('',*,*,#44899,.T.);
#61356=ORIENTED_EDGE('',*,*,#45821,.F.);
#61357=ORIENTED_EDGE('',*,*,#45454,.T.);
#61358=ORIENTED_EDGE('',*,*,#45819,.T.);
#61359=ORIENTED_EDGE('',*,*,#44898,.T.);
#61360=ORIENTED_EDGE('',*,*,#44897,.T.);
#61361=ORIENTED_EDGE('',*,*,#45822,.F.);
#61362=ORIENTED_EDGE('',*,*,#45823,.T.);
#61363=ORIENTED_EDGE('',*,*,#45824,.T.);
#61364=ORIENTED_EDGE('',*,*,#45825,.F.);
#61365=ORIENTED_EDGE('',*,*,#45826,.F.);
#61366=ORIENTED_EDGE('',*,*,#45827,.T.);
#61367=ORIENTED_EDGE('',*,*,#45822,.T.);
#61368=ORIENTED_EDGE('',*,*,#44896,.T.);
#61369=ORIENTED_EDGE('',*,*,#44906,.F.);
#61370=ORIENTED_EDGE('',*,*,#45828,.T.);
#61371=ORIENTED_EDGE('',*,*,#45826,.T.);
#61372=ORIENTED_EDGE('',*,*,#44895,.T.);
#61373=ORIENTED_EDGE('',*,*,#44908,.T.);
#61374=ORIENTED_EDGE('',*,*,#45829,.F.);
#61375=ORIENTED_EDGE('',*,*,#45830,.T.);
#61376=ORIENTED_EDGE('',*,*,#45828,.F.);
#61377=ORIENTED_EDGE('',*,*,#45831,.F.);
#61378=ORIENTED_EDGE('',*,*,#45829,.T.);
#61379=ORIENTED_EDGE('',*,*,#44910,.T.);
#61380=ORIENTED_EDGE('',*,*,#44923,.T.);
#61381=ORIENTED_EDGE('',*,*,#45832,.F.);
#61382=ORIENTED_EDGE('',*,*,#44913,.T.);
#61383=ORIENTED_EDGE('',*,*,#44911,.T.);
#61384=ORIENTED_EDGE('',*,*,#44925,.T.);
#61385=ORIENTED_EDGE('',*,*,#45833,.F.);
#61386=ORIENTED_EDGE('',*,*,#45834,.T.);
#61387=ORIENTED_EDGE('',*,*,#45831,.T.);
#61388=ORIENTED_EDGE('',*,*,#44922,.T.);
#61389=ORIENTED_EDGE('',*,*,#45835,.F.);
#61390=ORIENTED_EDGE('',*,*,#45836,.T.);
#61391=ORIENTED_EDGE('',*,*,#45833,.T.);
#61392=ORIENTED_EDGE('',*,*,#44921,.T.);
#61393=ORIENTED_EDGE('',*,*,#45837,.T.);
#61394=ORIENTED_EDGE('',*,*,#45835,.T.);
#61395=ORIENTED_EDGE('',*,*,#44920,.T.);
#61396=ORIENTED_EDGE('',*,*,#45838,.F.);
#61397=ORIENTED_EDGE('',*,*,#45839,.F.);
#61398=ORIENTED_EDGE('',*,*,#45459,.T.);
#61399=ORIENTED_EDGE('',*,*,#45840,.T.);
#61400=ORIENTED_EDGE('',*,*,#44919,.T.);
#61401=ORIENTED_EDGE('',*,*,#45841,.F.);
#61402=ORIENTED_EDGE('',*,*,#45842,.T.);
#61403=ORIENTED_EDGE('',*,*,#45839,.T.);
#61404=ORIENTED_EDGE('',*,*,#44918,.T.);
#61405=ORIENTED_EDGE('',*,*,#45843,.F.);
#61406=ORIENTED_EDGE('',*,*,#45844,.T.);
#61407=ORIENTED_EDGE('',*,*,#45841,.T.);
#61408=ORIENTED_EDGE('',*,*,#44917,.T.);
#61409=ORIENTED_EDGE('',*,*,#45845,.T.);
#61410=ORIENTED_EDGE('',*,*,#45846,.T.);
#61411=ORIENTED_EDGE('',*,*,#45843,.T.);
#61412=ORIENTED_EDGE('',*,*,#44916,.T.);
#61413=ORIENTED_EDGE('',*,*,#45845,.F.);
#61414=ORIENTED_EDGE('',*,*,#44915,.T.);
#61415=ORIENTED_EDGE('',*,*,#45847,.T.);
#61416=ORIENTED_EDGE('',*,*,#45848,.T.);
#61417=ORIENTED_EDGE('',*,*,#45847,.F.);
#61418=ORIENTED_EDGE('',*,*,#44914,.T.);
#61419=ORIENTED_EDGE('',*,*,#45832,.T.);
#61420=ORIENTED_EDGE('',*,*,#45849,.T.);
#61421=ORIENTED_EDGE('',*,*,#45850,.T.);
#61422=ORIENTED_EDGE('',*,*,#45849,.F.);
#61423=ORIENTED_EDGE('',*,*,#44924,.T.);
#61424=ORIENTED_EDGE('',*,*,#45851,.F.);
#61425=ORIENTED_EDGE('',*,*,#44928,.F.);
#61426=ORIENTED_EDGE('',*,*,#44934,.T.);
#61427=ORIENTED_EDGE('',*,*,#45852,.T.);
#61428=ORIENTED_EDGE('',*,*,#44926,.T.);
#61429=ORIENTED_EDGE('',*,*,#45853,.F.);
#61430=ORIENTED_EDGE('',*,*,#44929,.T.);
#61431=ORIENTED_EDGE('',*,*,#45854,.T.);
#61432=ORIENTED_EDGE('',*,*,#45855,.T.);
#61433=ORIENTED_EDGE('',*,*,#45854,.F.);
#61434=ORIENTED_EDGE('',*,*,#44939,.T.);
#61435=ORIENTED_EDGE('',*,*,#45856,.T.);
#61436=ORIENTED_EDGE('',*,*,#45461,.T.);
#61437=ORIENTED_EDGE('',*,*,#44938,.T.);
#61438=ORIENTED_EDGE('',*,*,#45857,.F.);
#61439=ORIENTED_EDGE('',*,*,#45858,.T.);
#61440=ORIENTED_EDGE('',*,*,#45859,.F.);
#61441=ORIENTED_EDGE('',*,*,#45860,.F.);
#61442=ORIENTED_EDGE('',*,*,#45861,.T.);
#61443=ORIENTED_EDGE('',*,*,#45857,.T.);
#61444=ORIENTED_EDGE('',*,*,#44937,.T.);
#61445=ORIENTED_EDGE('',*,*,#45639,.F.);
#61446=ORIENTED_EDGE('',*,*,#45862,.T.);
#61447=ORIENTED_EDGE('',*,*,#45860,.T.);
#61448=ORIENTED_EDGE('',*,*,#44936,.T.);
#61449=ORIENTED_EDGE('',*,*,#45852,.F.);
#61450=ORIENTED_EDGE('',*,*,#44933,.T.);
#61451=ORIENTED_EDGE('',*,*,#45863,.T.);
#61452=ORIENTED_EDGE('',*,*,#45851,.T.);
#61453=ORIENTED_EDGE('',*,*,#45863,.F.);
#61454=ORIENTED_EDGE('',*,*,#44932,.T.);
#61455=ORIENTED_EDGE('',*,*,#45864,.T.);
#61456=ORIENTED_EDGE('',*,*,#45865,.T.);
#61457=ORIENTED_EDGE('',*,*,#45864,.F.);
#61458=ORIENTED_EDGE('',*,*,#44931,.T.);
#61459=ORIENTED_EDGE('',*,*,#45866,.T.);
#61460=ORIENTED_EDGE('',*,*,#45867,.T.);
#61461=ORIENTED_EDGE('',*,*,#45866,.F.);
#61462=ORIENTED_EDGE('',*,*,#44930,.T.);
#61463=ORIENTED_EDGE('',*,*,#45853,.T.);
#61464=ORIENTED_EDGE('',*,*,#45868,.T.);
#61465=ORIENTED_EDGE('',*,*,#45869,.T.);
#61466=ORIENTED_EDGE('',*,*,#45870,.F.);
#61467=ORIENTED_EDGE('',*,*,#44940,.T.);
#61468=ORIENTED_EDGE('',*,*,#45871,.F.);
#61469=ORIENTED_EDGE('',*,*,#45872,.F.);
#61470=ORIENTED_EDGE('',*,*,#44943,.T.);
#61471=ORIENTED_EDGE('',*,*,#44944,.T.);
#61472=ORIENTED_EDGE('',*,*,#44956,.T.);
#61473=ORIENTED_EDGE('',*,*,#45873,.F.);
#61474=ORIENTED_EDGE('',*,*,#45032,.T.);
#61475=ORIENTED_EDGE('',*,*,#44946,.T.);
#61476=ORIENTED_EDGE('',*,*,#44942,.T.);
#61477=ORIENTED_EDGE('',*,*,#44941,.T.);
#61478=ORIENTED_EDGE('',*,*,#45870,.T.);
#61479=ORIENTED_EDGE('',*,*,#45874,.T.);
#61480=ORIENTED_EDGE('',*,*,#45875,.F.);
#61481=ORIENTED_EDGE('',*,*,#45876,.F.);
#61482=ORIENTED_EDGE('',*,*,#44948,.T.);
#61483=ORIENTED_EDGE('',*,*,#45877,.T.);
#61484=ORIENTED_EDGE('',*,*,#45878,.T.);
#61485=ORIENTED_EDGE('',*,*,#45879,.T.);
#61486=ORIENTED_EDGE('',*,*,#45877,.F.);
#61487=ORIENTED_EDGE('',*,*,#44962,.T.);
#61488=ORIENTED_EDGE('',*,*,#45880,.T.);
#61489=ORIENTED_EDGE('',*,*,#45499,.T.);
#61490=ORIENTED_EDGE('',*,*,#45878,.F.);
#61491=ORIENTED_EDGE('',*,*,#44961,.T.);
#61492=ORIENTED_EDGE('',*,*,#45881,.F.);
#61493=ORIENTED_EDGE('',*,*,#45882,.T.);
#61494=ORIENTED_EDGE('',*,*,#45883,.F.);
#61495=ORIENTED_EDGE('',*,*,#45884,.F.);
#61496=ORIENTED_EDGE('',*,*,#45885,.T.);
#61497=ORIENTED_EDGE('',*,*,#45881,.T.);
#61498=ORIENTED_EDGE('',*,*,#44960,.T.);
#61499=ORIENTED_EDGE('',*,*,#45886,.F.);
#61500=ORIENTED_EDGE('',*,*,#45887,.T.);
#61501=ORIENTED_EDGE('',*,*,#45884,.T.);
#61502=ORIENTED_EDGE('',*,*,#44959,.T.);
#61503=ORIENTED_EDGE('',*,*,#44964,.F.);
#61504=ORIENTED_EDGE('',*,*,#45888,.T.);
#61505=ORIENTED_EDGE('',*,*,#45886,.T.);
#61506=ORIENTED_EDGE('',*,*,#44958,.T.);
#61507=ORIENTED_EDGE('',*,*,#45889,.F.);
#61508=ORIENTED_EDGE('',*,*,#45871,.T.);
#61509=ORIENTED_EDGE('',*,*,#45872,.T.);
#61510=ORIENTED_EDGE('',*,*,#44955,.T.);
#61511=ORIENTED_EDGE('',*,*,#45890,.F.);
#61512=ORIENTED_EDGE('',*,*,#45891,.T.);
#61513=ORIENTED_EDGE('',*,*,#45889,.T.);
#61514=ORIENTED_EDGE('',*,*,#44954,.T.);
#61515=ORIENTED_EDGE('',*,*,#45892,.T.);
#61516=ORIENTED_EDGE('',*,*,#45893,.T.);
#61517=ORIENTED_EDGE('',*,*,#45890,.T.);
#61518=ORIENTED_EDGE('',*,*,#44953,.T.);
#61519=ORIENTED_EDGE('',*,*,#45892,.F.);
#61520=ORIENTED_EDGE('',*,*,#44952,.T.);
#61521=ORIENTED_EDGE('',*,*,#45894,.T.);
#61522=ORIENTED_EDGE('',*,*,#45895,.T.);
#61523=ORIENTED_EDGE('',*,*,#45894,.F.);
#61524=ORIENTED_EDGE('',*,*,#44951,.T.);
#61525=ORIENTED_EDGE('',*,*,#45896,.T.);
#61526=ORIENTED_EDGE('',*,*,#45897,.T.);
#61527=ORIENTED_EDGE('',*,*,#45896,.F.);
#61528=ORIENTED_EDGE('',*,*,#44950,.T.);
#61529=ORIENTED_EDGE('',*,*,#45898,.T.);
#61530=ORIENTED_EDGE('',*,*,#45899,.T.);
#61531=ORIENTED_EDGE('',*,*,#45898,.F.);
#61532=ORIENTED_EDGE('',*,*,#44949,.T.);
#61533=ORIENTED_EDGE('',*,*,#45876,.T.);
#61534=ORIENTED_EDGE('',*,*,#45900,.T.);
#61535=ORIENTED_EDGE('',*,*,#45901,.T.);
#61536=ORIENTED_EDGE('',*,*,#45888,.F.);
#61537=ORIENTED_EDGE('',*,*,#44966,.T.);
#61538=ORIENTED_EDGE('',*,*,#45902,.F.);
#61539=ORIENTED_EDGE('',*,*,#44968,.F.);
#61540=ORIENTED_EDGE('',*,*,#44976,.T.);
#61541=ORIENTED_EDGE('',*,*,#45903,.T.);
#61542=ORIENTED_EDGE('',*,*,#45902,.T.);
#61543=ORIENTED_EDGE('',*,*,#45505,.F.);
#61544=ORIENTED_EDGE('',*,*,#44982,.T.);
#61545=ORIENTED_EDGE('',*,*,#45904,.T.);
#61546=ORIENTED_EDGE('',*,*,#45515,.T.);
#61547=ORIENTED_EDGE('',*,*,#44981,.T.);
#61548=ORIENTED_EDGE('',*,*,#45905,.F.);
#61549=ORIENTED_EDGE('',*,*,#45229,.T.);
#61550=ORIENTED_EDGE('',*,*,#45906,.F.);
#61551=ORIENTED_EDGE('',*,*,#45907,.F.);
#61552=ORIENTED_EDGE('',*,*,#45908,.T.);
#61553=ORIENTED_EDGE('',*,*,#45909,.T.);
#61554=ORIENTED_EDGE('',*,*,#44980,.T.);
#61555=ORIENTED_EDGE('',*,*,#45323,.F.);
#61556=ORIENTED_EDGE('',*,*,#45331,.T.);
#61557=ORIENTED_EDGE('',*,*,#45907,.T.);
#61558=ORIENTED_EDGE('',*,*,#44979,.T.);
#61559=ORIENTED_EDGE('',*,*,#45903,.F.);
#61560=ORIENTED_EDGE('',*,*,#44975,.T.);
#61561=ORIENTED_EDGE('',*,*,#45910,.T.);
#61562=ORIENTED_EDGE('',*,*,#45911,.T.);
#61563=ORIENTED_EDGE('',*,*,#45910,.F.);
#61564=ORIENTED_EDGE('',*,*,#44974,.T.);
#61565=ORIENTED_EDGE('',*,*,#45912,.T.);
#61566=ORIENTED_EDGE('',*,*,#45913,.T.);
#61567=ORIENTED_EDGE('',*,*,#45914,.T.);
#61568=ORIENTED_EDGE('',*,*,#45912,.F.);
#61569=ORIENTED_EDGE('',*,*,#44973,.T.);
#61570=ORIENTED_EDGE('',*,*,#45915,.F.);
#61571=ORIENTED_EDGE('',*,*,#45916,.F.);
#61572=ORIENTED_EDGE('',*,*,#44972,.T.);
#61573=ORIENTED_EDGE('',*,*,#45917,.T.);
#61574=ORIENTED_EDGE('',*,*,#45503,.T.);
#61575=ORIENTED_EDGE('',*,*,#45917,.F.);
#61576=ORIENTED_EDGE('',*,*,#44971,.T.);
#61577=ORIENTED_EDGE('',*,*,#45918,.T.);
#61578=ORIENTED_EDGE('',*,*,#45919,.T.);
#61579=ORIENTED_EDGE('',*,*,#45918,.F.);
#61580=ORIENTED_EDGE('',*,*,#44970,.T.);
#61581=ORIENTED_EDGE('',*,*,#45504,.T.);
#61582=ORIENTED_EDGE('',*,*,#45511,.T.);
#61583=ORIENTED_EDGE('',*,*,#45920,.F.);
#61584=ORIENTED_EDGE('',*,*,#44990,.T.);
#61585=ORIENTED_EDGE('',*,*,#44984,.T.);
#61586=ORIENTED_EDGE('',*,*,#45000,.T.);
#61587=ORIENTED_EDGE('',*,*,#45555,.F.);
#61588=ORIENTED_EDGE('',*,*,#44997,.T.);
#61589=ORIENTED_EDGE('',*,*,#45921,.T.);
#61590=ORIENTED_EDGE('',*,*,#45559,.T.);
#61591=ORIENTED_EDGE('',*,*,#45921,.F.);
#61592=ORIENTED_EDGE('',*,*,#44996,.T.);
#61593=ORIENTED_EDGE('',*,*,#45922,.T.);
#61594=ORIENTED_EDGE('',*,*,#45923,.T.);
#61595=ORIENTED_EDGE('',*,*,#45922,.F.);
#61596=ORIENTED_EDGE('',*,*,#44995,.T.);
#61597=ORIENTED_EDGE('',*,*,#45924,.T.);
#61598=ORIENTED_EDGE('',*,*,#45925,.T.);
#61599=ORIENTED_EDGE('',*,*,#45924,.F.);
#61600=ORIENTED_EDGE('',*,*,#44994,.T.);
#61601=ORIENTED_EDGE('',*,*,#45926,.T.);
#61602=ORIENTED_EDGE('',*,*,#45927,.T.);
#61603=ORIENTED_EDGE('',*,*,#45926,.F.);
#61604=ORIENTED_EDGE('',*,*,#44993,.T.);
#61605=ORIENTED_EDGE('',*,*,#45928,.T.);
#61606=ORIENTED_EDGE('',*,*,#45929,.T.);
#61607=ORIENTED_EDGE('',*,*,#45928,.F.);
#61608=ORIENTED_EDGE('',*,*,#44992,.T.);
#61609=ORIENTED_EDGE('',*,*,#45930,.T.);
#61610=ORIENTED_EDGE('',*,*,#45931,.T.);
#61611=ORIENTED_EDGE('',*,*,#45930,.F.);
#61612=ORIENTED_EDGE('',*,*,#44991,.T.);
#61613=ORIENTED_EDGE('',*,*,#45920,.T.);
#61614=ORIENTED_EDGE('',*,*,#45932,.T.);
#61615=ORIENTED_EDGE('',*,*,#45933,.F.);
#61616=ORIENTED_EDGE('',*,*,#45934,.T.);
#61617=ORIENTED_EDGE('',*,*,#45336,.T.);
#61618=ORIENTED_EDGE('',*,*,#44988,.T.);
#61619=ORIENTED_EDGE('',*,*,#45561,.F.);
#61620=ORIENTED_EDGE('',*,*,#45935,.T.);
#61621=ORIENTED_EDGE('',*,*,#45933,.T.);
#61622=ORIENTED_EDGE('',*,*,#44987,.T.);
#61623=ORIENTED_EDGE('',*,*,#45936,.F.);
#61624=ORIENTED_EDGE('',*,*,#45932,.F.);
#61625=ORIENTED_EDGE('',*,*,#44999,.F.);
#61626=ORIENTED_EDGE('',*,*,#45937,.F.);
#61627=ORIENTED_EDGE('',*,*,#45938,.F.);
#61628=ORIENTED_EDGE('',*,*,#45002,.T.);
#61629=ORIENTED_EDGE('',*,*,#45939,.T.);
#61630=ORIENTED_EDGE('',*,*,#45020,.T.);
#61631=ORIENTED_EDGE('',*,*,#45939,.F.);
#61632=ORIENTED_EDGE('',*,*,#45003,.T.);
#61633=ORIENTED_EDGE('',*,*,#45004,.T.);
#61634=ORIENTED_EDGE('',*,*,#45021,.T.);
#61635=ORIENTED_EDGE('',*,*,#45940,.F.);
#61636=ORIENTED_EDGE('',*,*,#45937,.T.);
#61637=ORIENTED_EDGE('',*,*,#45938,.T.);
#61638=ORIENTED_EDGE('',*,*,#45019,.T.);
#61639=ORIENTED_EDGE('',*,*,#45941,.F.);
#61640=ORIENTED_EDGE('',*,*,#45942,.T.);
#61641=ORIENTED_EDGE('',*,*,#45940,.T.);
#61642=ORIENTED_EDGE('',*,*,#45018,.T.);
#61643=ORIENTED_EDGE('',*,*,#45943,.F.);
#61644=ORIENTED_EDGE('',*,*,#45944,.T.);
#61645=ORIENTED_EDGE('',*,*,#45941,.T.);
#61646=ORIENTED_EDGE('',*,*,#45017,.T.);
#61647=ORIENTED_EDGE('',*,*,#45945,.F.);
#61648=ORIENTED_EDGE('',*,*,#45946,.T.);
#61649=ORIENTED_EDGE('',*,*,#45943,.T.);
#61650=ORIENTED_EDGE('',*,*,#45016,.T.);
#61651=ORIENTED_EDGE('',*,*,#45947,.F.);
#61652=ORIENTED_EDGE('',*,*,#45948,.T.);
#61653=ORIENTED_EDGE('',*,*,#45945,.T.);
#61654=ORIENTED_EDGE('',*,*,#45015,.T.);
#61655=ORIENTED_EDGE('',*,*,#45949,.F.);
#61656=ORIENTED_EDGE('',*,*,#45950,.T.);
#61657=ORIENTED_EDGE('',*,*,#45947,.T.);
#61658=ORIENTED_EDGE('',*,*,#45014,.T.);
#61659=ORIENTED_EDGE('',*,*,#45951,.F.);
#61660=ORIENTED_EDGE('',*,*,#45952,.T.);
#61661=ORIENTED_EDGE('',*,*,#45949,.T.);
#61662=ORIENTED_EDGE('',*,*,#45013,.T.);
#61663=ORIENTED_EDGE('',*,*,#45953,.F.);
#61664=ORIENTED_EDGE('',*,*,#45954,.T.);
#61665=ORIENTED_EDGE('',*,*,#45951,.T.);
#61666=ORIENTED_EDGE('',*,*,#45012,.T.);
#61667=ORIENTED_EDGE('',*,*,#45955,.F.);
#61668=ORIENTED_EDGE('',*,*,#45493,.T.);
#61669=ORIENTED_EDGE('',*,*,#45953,.T.);
#61670=ORIENTED_EDGE('',*,*,#45011,.T.);
#61671=ORIENTED_EDGE('',*,*,#45010,.T.);
#61672=ORIENTED_EDGE('',*,*,#45956,.F.);
#61673=ORIENTED_EDGE('',*,*,#45957,.T.);
#61674=ORIENTED_EDGE('',*,*,#45958,.F.);
#61675=ORIENTED_EDGE('',*,*,#45959,.F.);
#61676=ORIENTED_EDGE('',*,*,#45960,.T.);
#61677=ORIENTED_EDGE('',*,*,#45956,.T.);
#61678=ORIENTED_EDGE('',*,*,#45009,.T.);
#61679=ORIENTED_EDGE('',*,*,#45961,.F.);
#61680=ORIENTED_EDGE('',*,*,#45962,.T.);
#61681=ORIENTED_EDGE('',*,*,#45959,.T.);
#61682=ORIENTED_EDGE('',*,*,#45008,.T.);
#61683=ORIENTED_EDGE('',*,*,#45023,.F.);
#61684=ORIENTED_EDGE('',*,*,#45963,.T.);
#61685=ORIENTED_EDGE('',*,*,#45961,.T.);
#61686=ORIENTED_EDGE('',*,*,#45007,.T.);
#61687=ORIENTED_EDGE('',*,*,#45025,.T.);
#61688=ORIENTED_EDGE('',*,*,#45964,.F.);
#61689=ORIENTED_EDGE('',*,*,#45965,.T.);
#61690=ORIENTED_EDGE('',*,*,#45963,.F.);
#61691=ORIENTED_EDGE('',*,*,#45966,.F.);
#61692=ORIENTED_EDGE('',*,*,#45964,.T.);
#61693=ORIENTED_EDGE('',*,*,#45027,.T.);
#61694=ORIENTED_EDGE('',*,*,#45031,.T.);
#61695=ORIENTED_EDGE('',*,*,#45967,.T.);
#61696=ORIENTED_EDGE('',*,*,#45968,.T.);
#61697=ORIENTED_EDGE('',*,*,#45028,.T.);
#61698=ORIENTED_EDGE('',*,*,#45969,.F.);
#61699=ORIENTED_EDGE('',*,*,#45970,.F.);
#61700=ORIENTED_EDGE('',*,*,#45042,.T.);
#61701=ORIENTED_EDGE('',*,*,#45971,.T.);
#61702=ORIENTED_EDGE('',*,*,#45497,.T.);
#61703=ORIENTED_EDGE('',*,*,#45971,.F.);
#61704=ORIENTED_EDGE('',*,*,#45041,.T.);
#61705=ORIENTED_EDGE('',*,*,#45972,.T.);
#61706=ORIENTED_EDGE('',*,*,#45973,.T.);
#61707=ORIENTED_EDGE('',*,*,#45972,.F.);
#61708=ORIENTED_EDGE('',*,*,#45040,.T.);
#61709=ORIENTED_EDGE('',*,*,#45974,.T.);
#61710=ORIENTED_EDGE('',*,*,#45975,.T.);
#61711=ORIENTED_EDGE('',*,*,#45974,.F.);
#61712=ORIENTED_EDGE('',*,*,#45039,.T.);
#61713=ORIENTED_EDGE('',*,*,#45976,.T.);
#61714=ORIENTED_EDGE('',*,*,#45977,.T.);
#61715=ORIENTED_EDGE('',*,*,#45976,.F.);
#61716=ORIENTED_EDGE('',*,*,#45038,.T.);
#61717=ORIENTED_EDGE('',*,*,#45978,.T.);
#61718=ORIENTED_EDGE('',*,*,#45979,.T.);
#61719=ORIENTED_EDGE('',*,*,#45978,.F.);
#61720=ORIENTED_EDGE('',*,*,#45037,.T.);
#61721=ORIENTED_EDGE('',*,*,#45980,.T.);
#61722=ORIENTED_EDGE('',*,*,#45981,.T.);
#61723=ORIENTED_EDGE('',*,*,#45980,.F.);
#61724=ORIENTED_EDGE('',*,*,#45036,.T.);
#61725=ORIENTED_EDGE('',*,*,#45982,.T.);
#61726=ORIENTED_EDGE('',*,*,#45983,.T.);
#61727=ORIENTED_EDGE('',*,*,#45982,.F.);
#61728=ORIENTED_EDGE('',*,*,#45035,.T.);
#61729=ORIENTED_EDGE('',*,*,#45984,.T.);
#61730=ORIENTED_EDGE('',*,*,#45985,.T.);
#61731=ORIENTED_EDGE('',*,*,#45984,.F.);
#61732=ORIENTED_EDGE('',*,*,#45034,.T.);
#61733=ORIENTED_EDGE('',*,*,#45986,.T.);
#61734=ORIENTED_EDGE('',*,*,#45987,.T.);
#61735=ORIENTED_EDGE('',*,*,#45986,.F.);
#61736=ORIENTED_EDGE('',*,*,#45033,.T.);
#61737=ORIENTED_EDGE('',*,*,#45873,.T.);
#61738=ORIENTED_EDGE('',*,*,#45875,.T.);
#61739=ORIENTED_EDGE('',*,*,#45988,.F.);
#61740=ORIENTED_EDGE('',*,*,#45989,.T.);
#61741=ORIENTED_EDGE('',*,*,#45966,.T.);
#61742=ORIENTED_EDGE('',*,*,#45030,.T.);
#61743=ORIENTED_EDGE('',*,*,#45968,.F.);
#61744=ORIENTED_EDGE('',*,*,#45990,.T.);
#61745=ORIENTED_EDGE('',*,*,#45988,.T.);
#61746=ORIENTED_EDGE('',*,*,#45029,.T.);
#61747=ORIENTED_EDGE('',*,*,#45991,.T.);
#61748=ORIENTED_EDGE('',*,*,#45992,.F.);
#61749=ORIENTED_EDGE('',*,*,#45043,.T.);
#61750=ORIENTED_EDGE('',*,*,#45993,.F.);
#61751=ORIENTED_EDGE('',*,*,#45047,.F.);
#61752=ORIENTED_EDGE('',*,*,#45058,.T.);
#61753=ORIENTED_EDGE('',*,*,#45994,.T.);
#61754=ORIENTED_EDGE('',*,*,#45045,.T.);
#61755=ORIENTED_EDGE('',*,*,#45048,.F.);
#61756=ORIENTED_EDGE('',*,*,#45044,.T.);
#61757=ORIENTED_EDGE('',*,*,#45995,.T.);
#61758=ORIENTED_EDGE('',*,*,#45090,.T.);
#61759=ORIENTED_EDGE('',*,*,#45994,.F.);
#61760=ORIENTED_EDGE('',*,*,#45057,.T.);
#61761=ORIENTED_EDGE('',*,*,#45996,.T.);
#61762=ORIENTED_EDGE('',*,*,#45993,.T.);
#61763=ORIENTED_EDGE('',*,*,#45996,.F.);
#61764=ORIENTED_EDGE('',*,*,#45056,.T.);
#61765=ORIENTED_EDGE('',*,*,#45997,.T.);
#61766=ORIENTED_EDGE('',*,*,#45998,.T.);
#61767=ORIENTED_EDGE('',*,*,#45997,.F.);
#61768=ORIENTED_EDGE('',*,*,#45055,.T.);
#61769=ORIENTED_EDGE('',*,*,#45999,.T.);
#61770=ORIENTED_EDGE('',*,*,#46000,.T.);
#61771=ORIENTED_EDGE('',*,*,#45999,.F.);
#61772=ORIENTED_EDGE('',*,*,#45054,.T.);
#61773=ORIENTED_EDGE('',*,*,#45379,.T.);
#61774=ORIENTED_EDGE('',*,*,#45382,.T.);
#61775=ORIENTED_EDGE('',*,*,#45060,.F.);
#61776=ORIENTED_EDGE('',*,*,#46001,.T.);
#61777=ORIENTED_EDGE('',*,*,#45378,.T.);
#61778=ORIENTED_EDGE('',*,*,#45051,.T.);
#61779=ORIENTED_EDGE('',*,*,#45377,.T.);
#61780=ORIENTED_EDGE('',*,*,#46001,.F.);
#61781=ORIENTED_EDGE('',*,*,#45062,.T.);
#61782=ORIENTED_EDGE('',*,*,#46002,.F.);
#61783=ORIENTED_EDGE('',*,*,#45375,.F.);
#61784=ORIENTED_EDGE('',*,*,#46002,.T.);
#61785=ORIENTED_EDGE('',*,*,#45064,.T.);
#61786=ORIENTED_EDGE('',*,*,#45072,.T.);
#61787=ORIENTED_EDGE('',*,*,#46003,.F.);
#61788=ORIENTED_EDGE('',*,*,#45370,.T.);
#61789=ORIENTED_EDGE('',*,*,#45373,.T.);
#61790=ORIENTED_EDGE('',*,*,#45069,.T.);
#61791=ORIENTED_EDGE('',*,*,#46004,.F.);
#61792=ORIENTED_EDGE('',*,*,#46005,.T.);
#61793=ORIENTED_EDGE('',*,*,#46003,.T.);
#61794=ORIENTED_EDGE('',*,*,#45068,.T.);
#61795=ORIENTED_EDGE('',*,*,#45629,.F.);
#61796=ORIENTED_EDGE('',*,*,#45626,.T.);
#61797=ORIENTED_EDGE('',*,*,#46004,.T.);
#61798=ORIENTED_EDGE('',*,*,#45067,.T.);
#61799=ORIENTED_EDGE('',*,*,#46006,.T.);
#61800=ORIENTED_EDGE('',*,*,#45322,.F.);
#61801=ORIENTED_EDGE('',*,*,#45076,.T.);
#61802=ORIENTED_EDGE('',*,*,#45349,.F.);
#61803=ORIENTED_EDGE('',*,*,#45080,.T.);
#61804=ORIENTED_EDGE('',*,*,#46007,.F.);
#61805=ORIENTED_EDGE('',*,*,#45339,.T.);
#61806=ORIENTED_EDGE('',*,*,#45342,.F.);
#61807=ORIENTED_EDGE('',*,*,#45083,.F.);
#61808=ORIENTED_EDGE('',*,*,#46008,.T.);
#61809=ORIENTED_EDGE('',*,*,#46007,.T.);
#61810=ORIENTED_EDGE('',*,*,#45079,.T.);
#61811=ORIENTED_EDGE('',*,*,#45085,.T.);
#61812=ORIENTED_EDGE('',*,*,#46009,.F.);
#61813=ORIENTED_EDGE('',*,*,#45340,.T.);
#61814=ORIENTED_EDGE('',*,*,#46008,.F.);
#61815=ORIENTED_EDGE('',*,*,#45338,.F.);
#61816=ORIENTED_EDGE('',*,*,#46009,.T.);
#61817=ORIENTED_EDGE('',*,*,#45087,.T.);
#61818=ORIENTED_EDGE('',*,*,#45089,.T.);
#61819=ORIENTED_EDGE('',*,*,#46010,.F.);
#61820=ORIENTED_EDGE('',*,*,#45380,.T.);
#61821=ORIENTED_EDGE('',*,*,#45383,.T.);
#61822=ORIENTED_EDGE('',*,*,#45094,.T.);
#61823=ORIENTED_EDGE('',*,*,#46011,.F.);
#61824=ORIENTED_EDGE('',*,*,#46012,.T.);
#61825=ORIENTED_EDGE('',*,*,#46010,.T.);
#61826=ORIENTED_EDGE('',*,*,#45093,.T.);
#61827=ORIENTED_EDGE('',*,*,#46013,.F.);
#61828=ORIENTED_EDGE('',*,*,#46014,.T.);
#61829=ORIENTED_EDGE('',*,*,#46011,.T.);
#61830=ORIENTED_EDGE('',*,*,#45092,.T.);
#61831=ORIENTED_EDGE('',*,*,#45995,.F.);
#61832=ORIENTED_EDGE('',*,*,#45992,.T.);
#61833=ORIENTED_EDGE('',*,*,#46013,.T.);
#61834=ORIENTED_EDGE('',*,*,#45091,.T.);
#61835=ORIENTED_EDGE('',*,*,#46015,.T.);
#61836=ORIENTED_EDGE('',*,*,#46016,.F.);
#61837=ORIENTED_EDGE('',*,*,#45096,.T.);
#61838=ORIENTED_EDGE('',*,*,#46017,.F.);
#61839=ORIENTED_EDGE('',*,*,#45100,.F.);
#61840=ORIENTED_EDGE('',*,*,#45112,.T.);
#61841=ORIENTED_EDGE('',*,*,#46018,.T.);
#61842=ORIENTED_EDGE('',*,*,#45098,.T.);
#61843=ORIENTED_EDGE('',*,*,#46019,.F.);
#61844=ORIENTED_EDGE('',*,*,#45193,.T.);
#61845=ORIENTED_EDGE('',*,*,#45101,.T.);
#61846=ORIENTED_EDGE('',*,*,#45097,.T.);
#61847=ORIENTED_EDGE('',*,*,#46020,.F.);
#61848=ORIENTED_EDGE('',*,*,#45103,.T.);
#61849=ORIENTED_EDGE('',*,*,#46021,.T.);
#61850=ORIENTED_EDGE('',*,*,#46022,.T.);
#61851=ORIENTED_EDGE('',*,*,#46023,.T.);
#61852=ORIENTED_EDGE('',*,*,#46021,.F.);
#61853=ORIENTED_EDGE('',*,*,#45118,.T.);
#61854=ORIENTED_EDGE('',*,*,#46024,.T.);
#61855=ORIENTED_EDGE('',*,*,#45414,.T.);
#61856=ORIENTED_EDGE('',*,*,#46022,.F.);
#61857=ORIENTED_EDGE('',*,*,#45117,.T.);
#61858=ORIENTED_EDGE('',*,*,#46025,.F.);
#61859=ORIENTED_EDGE('',*,*,#46026,.T.);
#61860=ORIENTED_EDGE('',*,*,#46027,.F.);
#61861=ORIENTED_EDGE('',*,*,#46028,.F.);
#61862=ORIENTED_EDGE('',*,*,#46029,.T.);
#61863=ORIENTED_EDGE('',*,*,#46025,.T.);
#61864=ORIENTED_EDGE('',*,*,#45116,.T.);
#61865=ORIENTED_EDGE('',*,*,#46030,.F.);
#61866=ORIENTED_EDGE('',*,*,#46031,.T.);
#61867=ORIENTED_EDGE('',*,*,#46028,.T.);
#61868=ORIENTED_EDGE('',*,*,#45115,.T.);
#61869=ORIENTED_EDGE('',*,*,#45120,.F.);
#61870=ORIENTED_EDGE('',*,*,#46032,.T.);
#61871=ORIENTED_EDGE('',*,*,#46030,.T.);
#61872=ORIENTED_EDGE('',*,*,#45114,.T.);
#61873=ORIENTED_EDGE('',*,*,#46018,.F.);
#61874=ORIENTED_EDGE('',*,*,#45111,.T.);
#61875=ORIENTED_EDGE('',*,*,#46033,.T.);
#61876=ORIENTED_EDGE('',*,*,#46017,.T.);
#61877=ORIENTED_EDGE('',*,*,#46033,.F.);
#61878=ORIENTED_EDGE('',*,*,#45110,.T.);
#61879=ORIENTED_EDGE('',*,*,#46034,.T.);
#61880=ORIENTED_EDGE('',*,*,#46035,.T.);
#61881=ORIENTED_EDGE('',*,*,#46034,.F.);
#61882=ORIENTED_EDGE('',*,*,#45109,.T.);
#61883=ORIENTED_EDGE('',*,*,#46036,.T.);
#61884=ORIENTED_EDGE('',*,*,#46037,.T.);
#61885=ORIENTED_EDGE('',*,*,#46036,.F.);
#61886=ORIENTED_EDGE('',*,*,#45108,.T.);
#61887=ORIENTED_EDGE('',*,*,#46038,.T.);
#61888=ORIENTED_EDGE('',*,*,#46039,.T.);
#61889=ORIENTED_EDGE('',*,*,#46038,.F.);
#61890=ORIENTED_EDGE('',*,*,#45107,.T.);
#61891=ORIENTED_EDGE('',*,*,#46040,.T.);
#61892=ORIENTED_EDGE('',*,*,#46041,.T.);
#61893=ORIENTED_EDGE('',*,*,#46040,.F.);
#61894=ORIENTED_EDGE('',*,*,#45106,.T.);
#61895=ORIENTED_EDGE('',*,*,#46042,.T.);
#61896=ORIENTED_EDGE('',*,*,#46043,.T.);
#61897=ORIENTED_EDGE('',*,*,#46042,.F.);
#61898=ORIENTED_EDGE('',*,*,#45105,.T.);
#61899=ORIENTED_EDGE('',*,*,#46044,.T.);
#61900=ORIENTED_EDGE('',*,*,#46045,.T.);
#61901=ORIENTED_EDGE('',*,*,#46044,.F.);
#61902=ORIENTED_EDGE('',*,*,#45104,.T.);
#61903=ORIENTED_EDGE('',*,*,#46020,.T.);
#61904=ORIENTED_EDGE('',*,*,#46046,.T.);
#61905=ORIENTED_EDGE('',*,*,#46047,.T.);
#61906=ORIENTED_EDGE('',*,*,#46032,.F.);
#61907=ORIENTED_EDGE('',*,*,#45122,.T.);
#61908=ORIENTED_EDGE('',*,*,#46048,.F.);
#61909=ORIENTED_EDGE('',*,*,#46049,.F.);
#61910=ORIENTED_EDGE('',*,*,#46048,.T.);
#61911=ORIENTED_EDGE('',*,*,#45124,.T.);
#61912=ORIENTED_EDGE('',*,*,#45136,.T.);
#61913=ORIENTED_EDGE('',*,*,#45140,.T.);
#61914=ORIENTED_EDGE('',*,*,#45318,.F.);
#61915=ORIENTED_EDGE('',*,*,#46050,.T.);
#61916=ORIENTED_EDGE('',*,*,#45345,.F.);
#61917=ORIENTED_EDGE('',*,*,#45307,.T.);
#61918=ORIENTED_EDGE('',*,*,#45313,.T.);
#61919=ORIENTED_EDGE('',*,*,#45314,.T.);
#61920=ORIENTED_EDGE('',*,*,#45315,.T.);
#61921=ORIENTED_EDGE('',*,*,#45138,.T.);
#61922=ORIENTED_EDGE('',*,*,#46051,.F.);
#61923=ORIENTED_EDGE('',*,*,#46052,.T.);
#61924=ORIENTED_EDGE('',*,*,#46049,.T.);
#61925=ORIENTED_EDGE('',*,*,#45135,.T.);
#61926=ORIENTED_EDGE('',*,*,#46053,.F.);
#61927=ORIENTED_EDGE('',*,*,#46054,.T.);
#61928=ORIENTED_EDGE('',*,*,#46051,.T.);
#61929=ORIENTED_EDGE('',*,*,#45134,.T.);
#61930=ORIENTED_EDGE('',*,*,#46055,.T.);
#61931=ORIENTED_EDGE('',*,*,#46053,.T.);
#61932=ORIENTED_EDGE('',*,*,#45133,.T.);
#61933=ORIENTED_EDGE('',*,*,#46056,.F.);
#61934=ORIENTED_EDGE('',*,*,#46057,.F.);
#61935=ORIENTED_EDGE('',*,*,#45132,.T.);
#61936=ORIENTED_EDGE('',*,*,#46058,.T.);
#61937=ORIENTED_EDGE('',*,*,#45418,.T.);
#61938=ORIENTED_EDGE('',*,*,#46058,.F.);
#61939=ORIENTED_EDGE('',*,*,#45131,.T.);
#61940=ORIENTED_EDGE('',*,*,#46059,.T.);
#61941=ORIENTED_EDGE('',*,*,#46060,.T.);
#61942=ORIENTED_EDGE('',*,*,#46059,.F.);
#61943=ORIENTED_EDGE('',*,*,#45130,.T.);
#61944=ORIENTED_EDGE('',*,*,#45518,.T.);
#61945=ORIENTED_EDGE('',*,*,#45525,.T.);
#61946=ORIENTED_EDGE('',*,*,#45526,.T.);
#61947=ORIENTED_EDGE('',*,*,#45519,.F.);
#61948=ORIENTED_EDGE('',*,*,#45128,.T.);
#61949=ORIENTED_EDGE('',*,*,#46061,.F.);
#61950=ORIENTED_EDGE('',*,*,#46062,.F.);
#61951=ORIENTED_EDGE('',*,*,#46063,.T.);
#61952=ORIENTED_EDGE('',*,*,#46064,.T.);
#61953=ORIENTED_EDGE('',*,*,#45142,.T.);
#61954=ORIENTED_EDGE('',*,*,#46065,.F.);
#61955=ORIENTED_EDGE('',*,*,#46066,.F.);
#61956=ORIENTED_EDGE('',*,*,#45419,.T.);
#61957=ORIENTED_EDGE('',*,*,#46067,.T.);
#61958=ORIENTED_EDGE('',*,*,#45156,.T.);
#61959=ORIENTED_EDGE('',*,*,#46068,.F.);
#61960=ORIENTED_EDGE('',*,*,#46069,.T.);
#61961=ORIENTED_EDGE('',*,*,#46066,.T.);
#61962=ORIENTED_EDGE('',*,*,#45155,.T.);
#61963=ORIENTED_EDGE('',*,*,#46070,.F.);
#61964=ORIENTED_EDGE('',*,*,#46071,.T.);
#61965=ORIENTED_EDGE('',*,*,#46068,.T.);
#61966=ORIENTED_EDGE('',*,*,#45154,.T.);
#61967=ORIENTED_EDGE('',*,*,#46072,.F.);
#61968=ORIENTED_EDGE('',*,*,#46073,.T.);
#61969=ORIENTED_EDGE('',*,*,#46070,.T.);
#61970=ORIENTED_EDGE('',*,*,#45153,.T.);
#61971=ORIENTED_EDGE('',*,*,#46074,.F.);
#61972=ORIENTED_EDGE('',*,*,#46075,.T.);
#61973=ORIENTED_EDGE('',*,*,#46072,.T.);
#61974=ORIENTED_EDGE('',*,*,#45152,.T.);
#61975=ORIENTED_EDGE('',*,*,#46076,.F.);
#61976=ORIENTED_EDGE('',*,*,#46077,.T.);
#61977=ORIENTED_EDGE('',*,*,#46074,.T.);
#61978=ORIENTED_EDGE('',*,*,#45151,.T.);
#61979=ORIENTED_EDGE('',*,*,#46078,.F.);
#61980=ORIENTED_EDGE('',*,*,#46079,.T.);
#61981=ORIENTED_EDGE('',*,*,#46076,.T.);
#61982=ORIENTED_EDGE('',*,*,#45150,.T.);
#61983=ORIENTED_EDGE('',*,*,#46080,.F.);
#61984=ORIENTED_EDGE('',*,*,#46081,.T.);
#61985=ORIENTED_EDGE('',*,*,#46078,.T.);
#61986=ORIENTED_EDGE('',*,*,#45149,.T.);
#61987=ORIENTED_EDGE('',*,*,#46082,.F.);
#61988=ORIENTED_EDGE('',*,*,#45161,.T.);
#61989=ORIENTED_EDGE('',*,*,#46080,.T.);
#61990=ORIENTED_EDGE('',*,*,#45148,.T.);
#61991=ORIENTED_EDGE('',*,*,#45157,.F.);
#61992=ORIENTED_EDGE('',*,*,#45159,.T.);
#61993=ORIENTED_EDGE('',*,*,#46082,.T.);
#61994=ORIENTED_EDGE('',*,*,#45147,.T.);
#61995=ORIENTED_EDGE('',*,*,#46083,.F.);
#61996=ORIENTED_EDGE('',*,*,#46084,.T.);
#61997=ORIENTED_EDGE('',*,*,#45642,.T.);
#61998=ORIENTED_EDGE('',*,*,#45144,.T.);
#61999=ORIENTED_EDGE('',*,*,#46064,.F.);
#62000=ORIENTED_EDGE('',*,*,#46085,.T.);
#62001=ORIENTED_EDGE('',*,*,#46083,.T.);
#62002=ORIENTED_EDGE('',*,*,#45143,.T.);
#62003=ORIENTED_EDGE('',*,*,#46086,.F.);
#62004=ORIENTED_EDGE('',*,*,#46081,.F.);
#62005=ORIENTED_EDGE('',*,*,#45160,.F.);
#62006=ORIENTED_EDGE('',*,*,#46087,.F.);
#62007=ORIENTED_EDGE('',*,*,#46088,.F.);
#62008=ORIENTED_EDGE('',*,*,#45163,.T.);
#62009=ORIENTED_EDGE('',*,*,#46089,.T.);
#62010=ORIENTED_EDGE('',*,*,#45181,.T.);
#62011=ORIENTED_EDGE('',*,*,#46089,.F.);
#62012=ORIENTED_EDGE('',*,*,#45164,.T.);
#62013=ORIENTED_EDGE('',*,*,#45165,.T.);
#62014=ORIENTED_EDGE('',*,*,#45182,.T.);
#62015=ORIENTED_EDGE('',*,*,#46090,.F.);
#62016=ORIENTED_EDGE('',*,*,#46087,.T.);
#62017=ORIENTED_EDGE('',*,*,#46088,.T.);
#62018=ORIENTED_EDGE('',*,*,#45180,.T.);
#62019=ORIENTED_EDGE('',*,*,#46091,.F.);
#62020=ORIENTED_EDGE('',*,*,#46092,.T.);
#62021=ORIENTED_EDGE('',*,*,#46090,.T.);
#62022=ORIENTED_EDGE('',*,*,#45179,.T.);
#62023=ORIENTED_EDGE('',*,*,#46093,.F.);
#62024=ORIENTED_EDGE('',*,*,#46094,.T.);
#62025=ORIENTED_EDGE('',*,*,#46091,.T.);
#62026=ORIENTED_EDGE('',*,*,#45178,.T.);
#62027=ORIENTED_EDGE('',*,*,#46095,.F.);
#62028=ORIENTED_EDGE('',*,*,#46096,.T.);
#62029=ORIENTED_EDGE('',*,*,#46093,.T.);
#62030=ORIENTED_EDGE('',*,*,#45177,.T.);
#62031=ORIENTED_EDGE('',*,*,#46097,.F.);
#62032=ORIENTED_EDGE('',*,*,#46098,.T.);
#62033=ORIENTED_EDGE('',*,*,#46095,.T.);
#62034=ORIENTED_EDGE('',*,*,#45176,.T.);
#62035=ORIENTED_EDGE('',*,*,#46099,.F.);
#62036=ORIENTED_EDGE('',*,*,#46100,.T.);
#62037=ORIENTED_EDGE('',*,*,#46097,.T.);
#62038=ORIENTED_EDGE('',*,*,#45175,.T.);
#62039=ORIENTED_EDGE('',*,*,#46101,.F.);
#62040=ORIENTED_EDGE('',*,*,#46102,.T.);
#62041=ORIENTED_EDGE('',*,*,#46099,.T.);
#62042=ORIENTED_EDGE('',*,*,#45174,.T.);
#62043=ORIENTED_EDGE('',*,*,#46103,.F.);
#62044=ORIENTED_EDGE('',*,*,#46104,.T.);
#62045=ORIENTED_EDGE('',*,*,#46101,.T.);
#62046=ORIENTED_EDGE('',*,*,#45173,.T.);
#62047=ORIENTED_EDGE('',*,*,#46105,.F.);
#62048=ORIENTED_EDGE('',*,*,#45408,.T.);
#62049=ORIENTED_EDGE('',*,*,#46103,.T.);
#62050=ORIENTED_EDGE('',*,*,#45172,.T.);
#62051=ORIENTED_EDGE('',*,*,#45171,.T.);
#62052=ORIENTED_EDGE('',*,*,#46106,.F.);
#62053=ORIENTED_EDGE('',*,*,#46107,.T.);
#62054=ORIENTED_EDGE('',*,*,#46108,.F.);
#62055=ORIENTED_EDGE('',*,*,#46109,.F.);
#62056=ORIENTED_EDGE('',*,*,#46110,.T.);
#62057=ORIENTED_EDGE('',*,*,#46106,.T.);
#62058=ORIENTED_EDGE('',*,*,#45170,.T.);
#62059=ORIENTED_EDGE('',*,*,#46111,.F.);
#62060=ORIENTED_EDGE('',*,*,#46112,.T.);
#62061=ORIENTED_EDGE('',*,*,#46109,.T.);
#62062=ORIENTED_EDGE('',*,*,#45169,.T.);
#62063=ORIENTED_EDGE('',*,*,#45184,.F.);
#62064=ORIENTED_EDGE('',*,*,#46113,.T.);
#62065=ORIENTED_EDGE('',*,*,#46111,.T.);
#62066=ORIENTED_EDGE('',*,*,#45168,.T.);
#62067=ORIENTED_EDGE('',*,*,#45186,.T.);
#62068=ORIENTED_EDGE('',*,*,#46114,.F.);
#62069=ORIENTED_EDGE('',*,*,#46115,.T.);
#62070=ORIENTED_EDGE('',*,*,#46113,.F.);
#62071=ORIENTED_EDGE('',*,*,#46116,.F.);
#62072=ORIENTED_EDGE('',*,*,#46114,.T.);
#62073=ORIENTED_EDGE('',*,*,#45188,.T.);
#62074=ORIENTED_EDGE('',*,*,#45192,.T.);
#62075=ORIENTED_EDGE('',*,*,#46117,.T.);
#62076=ORIENTED_EDGE('',*,*,#46118,.T.);
#62077=ORIENTED_EDGE('',*,*,#45189,.T.);
#62078=ORIENTED_EDGE('',*,*,#46119,.F.);
#62079=ORIENTED_EDGE('',*,*,#46120,.F.);
#62080=ORIENTED_EDGE('',*,*,#45203,.T.);
#62081=ORIENTED_EDGE('',*,*,#46121,.T.);
#62082=ORIENTED_EDGE('',*,*,#45412,.T.);
#62083=ORIENTED_EDGE('',*,*,#46121,.F.);
#62084=ORIENTED_EDGE('',*,*,#45202,.T.);
#62085=ORIENTED_EDGE('',*,*,#46122,.T.);
#62086=ORIENTED_EDGE('',*,*,#46123,.T.);
#62087=ORIENTED_EDGE('',*,*,#46122,.F.);
#62088=ORIENTED_EDGE('',*,*,#45201,.T.);
#62089=ORIENTED_EDGE('',*,*,#46124,.T.);
#62090=ORIENTED_EDGE('',*,*,#46125,.T.);
#62091=ORIENTED_EDGE('',*,*,#46124,.F.);
#62092=ORIENTED_EDGE('',*,*,#45200,.T.);
#62093=ORIENTED_EDGE('',*,*,#46126,.T.);
#62094=ORIENTED_EDGE('',*,*,#46127,.T.);
#62095=ORIENTED_EDGE('',*,*,#46126,.F.);
#62096=ORIENTED_EDGE('',*,*,#45199,.T.);
#62097=ORIENTED_EDGE('',*,*,#46128,.T.);
#62098=ORIENTED_EDGE('',*,*,#46129,.T.);
#62099=ORIENTED_EDGE('',*,*,#46128,.F.);
#62100=ORIENTED_EDGE('',*,*,#45198,.T.);
#62101=ORIENTED_EDGE('',*,*,#46130,.T.);
#62102=ORIENTED_EDGE('',*,*,#46131,.T.);
#62103=ORIENTED_EDGE('',*,*,#46130,.F.);
#62104=ORIENTED_EDGE('',*,*,#45197,.T.);
#62105=ORIENTED_EDGE('',*,*,#46132,.T.);
#62106=ORIENTED_EDGE('',*,*,#46133,.T.);
#62107=ORIENTED_EDGE('',*,*,#46132,.F.);
#62108=ORIENTED_EDGE('',*,*,#45196,.T.);
#62109=ORIENTED_EDGE('',*,*,#46134,.T.);
#62110=ORIENTED_EDGE('',*,*,#46135,.T.);
#62111=ORIENTED_EDGE('',*,*,#46134,.F.);
#62112=ORIENTED_EDGE('',*,*,#45195,.T.);
#62113=ORIENTED_EDGE('',*,*,#46136,.T.);
#62114=ORIENTED_EDGE('',*,*,#46137,.T.);
#62115=ORIENTED_EDGE('',*,*,#46136,.F.);
#62116=ORIENTED_EDGE('',*,*,#45194,.T.);
#62117=ORIENTED_EDGE('',*,*,#46019,.T.);
#62118=ORIENTED_EDGE('',*,*,#46016,.T.);
#62119=ORIENTED_EDGE('',*,*,#46138,.F.);
#62120=ORIENTED_EDGE('',*,*,#46139,.T.);
#62121=ORIENTED_EDGE('',*,*,#46116,.T.);
#62122=ORIENTED_EDGE('',*,*,#45191,.T.);
#62123=ORIENTED_EDGE('',*,*,#46118,.F.);
#62124=ORIENTED_EDGE('',*,*,#46140,.T.);
#62125=ORIENTED_EDGE('',*,*,#46138,.T.);
#62126=ORIENTED_EDGE('',*,*,#45190,.T.);
#62127=ORIENTED_EDGE('',*,*,#46141,.F.);
#62128=ORIENTED_EDGE('',*,*,#46142,.F.);
#62129=ORIENTED_EDGE('',*,*,#45204,.F.);
#62130=ORIENTED_EDGE('',*,*,#46143,.F.);
#62131=ORIENTED_EDGE('',*,*,#45209,.F.);
#62132=ORIENTED_EDGE('',*,*,#45217,.T.);
#62133=ORIENTED_EDGE('',*,*,#46144,.T.);
#62134=ORIENTED_EDGE('',*,*,#45207,.T.);
#62135=ORIENTED_EDGE('',*,*,#46145,.F.);
#62136=ORIENTED_EDGE('',*,*,#45296,.T.);
#62137=ORIENTED_EDGE('',*,*,#46146,.T.);
#62138=ORIENTED_EDGE('',*,*,#45205,.T.);
#62139=ORIENTED_EDGE('',*,*,#46147,.F.);
#62140=ORIENTED_EDGE('',*,*,#45210,.T.);
#62141=ORIENTED_EDGE('',*,*,#46148,.T.);
#62142=ORIENTED_EDGE('',*,*,#46149,.T.);
#62143=ORIENTED_EDGE('',*,*,#46148,.F.);
#62144=ORIENTED_EDGE('',*,*,#45222,.T.);
#62145=ORIENTED_EDGE('',*,*,#46150,.T.);
#62146=ORIENTED_EDGE('',*,*,#45467,.T.);
#62147=ORIENTED_EDGE('',*,*,#46151,.F.);
#62148=ORIENTED_EDGE('',*,*,#45221,.T.);
#62149=ORIENTED_EDGE('',*,*,#46152,.F.);
#62150=ORIENTED_EDGE('',*,*,#46153,.T.);
#62151=ORIENTED_EDGE('',*,*,#46154,.F.);
#62152=ORIENTED_EDGE('',*,*,#46155,.F.);
#62153=ORIENTED_EDGE('',*,*,#46156,.T.);
#62154=ORIENTED_EDGE('',*,*,#46152,.T.);
#62155=ORIENTED_EDGE('',*,*,#45220,.T.);
#62156=ORIENTED_EDGE('',*,*,#45644,.F.);
#62157=ORIENTED_EDGE('',*,*,#46157,.T.);
#62158=ORIENTED_EDGE('',*,*,#46155,.T.);
#62159=ORIENTED_EDGE('',*,*,#45219,.T.);
#62160=ORIENTED_EDGE('',*,*,#46144,.F.);
#62161=ORIENTED_EDGE('',*,*,#45216,.T.);
#62162=ORIENTED_EDGE('',*,*,#46158,.T.);
#62163=ORIENTED_EDGE('',*,*,#46143,.T.);
#62164=ORIENTED_EDGE('',*,*,#46158,.F.);
#62165=ORIENTED_EDGE('',*,*,#45215,.T.);
#62166=ORIENTED_EDGE('',*,*,#46159,.T.);
#62167=ORIENTED_EDGE('',*,*,#46160,.T.);
#62168=ORIENTED_EDGE('',*,*,#46159,.F.);
#62169=ORIENTED_EDGE('',*,*,#45214,.T.);
#62170=ORIENTED_EDGE('',*,*,#46161,.T.);
#62171=ORIENTED_EDGE('',*,*,#46162,.T.);
#62172=ORIENTED_EDGE('',*,*,#46161,.F.);
#62173=ORIENTED_EDGE('',*,*,#45213,.T.);
#62174=ORIENTED_EDGE('',*,*,#46163,.T.);
#62175=ORIENTED_EDGE('',*,*,#46164,.T.);
#62176=ORIENTED_EDGE('',*,*,#46163,.F.);
#62177=ORIENTED_EDGE('',*,*,#45212,.T.);
#62178=ORIENTED_EDGE('',*,*,#46165,.T.);
#62179=ORIENTED_EDGE('',*,*,#46166,.T.);
#62180=ORIENTED_EDGE('',*,*,#46165,.F.);
#62181=ORIENTED_EDGE('',*,*,#45211,.T.);
#62182=ORIENTED_EDGE('',*,*,#46147,.T.);
#62183=ORIENTED_EDGE('',*,*,#46167,.T.);
#62184=ORIENTED_EDGE('',*,*,#46168,.F.);
#62185=ORIENTED_EDGE('',*,*,#45225,.T.);
#62186=ORIENTED_EDGE('',*,*,#46169,.T.);
#62187=ORIENTED_EDGE('',*,*,#46170,.T.);
#62188=ORIENTED_EDGE('',*,*,#46169,.F.);
#62189=ORIENTED_EDGE('',*,*,#45238,.T.);
#62190=ORIENTED_EDGE('',*,*,#46171,.T.);
#62191=ORIENTED_EDGE('',*,*,#45479,.T.);
#62192=ORIENTED_EDGE('',*,*,#45237,.T.);
#62193=ORIENTED_EDGE('',*,*,#46172,.T.);
#62194=ORIENTED_EDGE('',*,*,#46173,.T.);
#62195=ORIENTED_EDGE('',*,*,#46174,.F.);
#62196=ORIENTED_EDGE('',*,*,#46172,.F.);
#62197=ORIENTED_EDGE('',*,*,#45236,.T.);
#62198=ORIENTED_EDGE('',*,*,#46175,.T.);
#62199=ORIENTED_EDGE('',*,*,#46176,.T.);
#62200=ORIENTED_EDGE('',*,*,#46175,.F.);
#62201=ORIENTED_EDGE('',*,*,#45235,.T.);
#62202=ORIENTED_EDGE('',*,*,#46177,.T.);
#62203=ORIENTED_EDGE('',*,*,#46178,.T.);
#62204=ORIENTED_EDGE('',*,*,#46177,.F.);
#62205=ORIENTED_EDGE('',*,*,#45234,.T.);
#62206=ORIENTED_EDGE('',*,*,#45240,.T.);
#62207=ORIENTED_EDGE('',*,*,#46179,.T.);
#62208=ORIENTED_EDGE('',*,*,#46180,.F.);
#62209=ORIENTED_EDGE('',*,*,#45329,.T.);
#62210=ORIENTED_EDGE('',*,*,#45332,.T.);
#62211=ORIENTED_EDGE('',*,*,#45231,.T.);
#62212=ORIENTED_EDGE('',*,*,#46181,.F.);
#62213=ORIENTED_EDGE('',*,*,#46182,.T.);
#62214=ORIENTED_EDGE('',*,*,#46180,.T.);
#62215=ORIENTED_EDGE('',*,*,#45230,.T.);
#62216=ORIENTED_EDGE('',*,*,#46183,.F.);
#62217=ORIENTED_EDGE('',*,*,#45228,.T.);
#62218=ORIENTED_EDGE('',*,*,#45513,.T.);
#62219=ORIENTED_EDGE('',*,*,#45517,.T.);
#62220=ORIENTED_EDGE('',*,*,#45514,.F.);
#62221=ORIENTED_EDGE('',*,*,#45226,.T.);
#62222=ORIENTED_EDGE('',*,*,#46168,.T.);
#62223=ORIENTED_EDGE('',*,*,#45512,.T.);
#62224=ORIENTED_EDGE('',*,*,#45242,.T.);
#62225=ORIENTED_EDGE('',*,*,#46184,.F.);
#62226=ORIENTED_EDGE('',*,*,#46185,.T.);
#62227=ORIENTED_EDGE('',*,*,#46179,.F.);
#62228=ORIENTED_EDGE('',*,*,#46186,.F.);
#62229=ORIENTED_EDGE('',*,*,#46184,.T.);
#62230=ORIENTED_EDGE('',*,*,#45244,.T.);
#62231=ORIENTED_EDGE('',*,*,#45248,.T.);
#62232=ORIENTED_EDGE('',*,*,#46187,.T.);
#62233=ORIENTED_EDGE('',*,*,#46188,.T.);
#62234=ORIENTED_EDGE('',*,*,#45245,.T.);
#62235=ORIENTED_EDGE('',*,*,#46189,.F.);
#62236=ORIENTED_EDGE('',*,*,#46190,.T.);
#62237=ORIENTED_EDGE('',*,*,#45483,.T.);
#62238=ORIENTED_EDGE('',*,*,#46191,.F.);
#62239=ORIENTED_EDGE('',*,*,#45260,.T.);
#62240=ORIENTED_EDGE('',*,*,#46192,.T.);
#62241=ORIENTED_EDGE('',*,*,#46192,.F.);
#62242=ORIENTED_EDGE('',*,*,#45259,.T.);
#62243=ORIENTED_EDGE('',*,*,#46193,.T.);
#62244=ORIENTED_EDGE('',*,*,#46194,.T.);
#62245=ORIENTED_EDGE('',*,*,#46190,.F.);
#62246=ORIENTED_EDGE('',*,*,#46193,.F.);
#62247=ORIENTED_EDGE('',*,*,#45258,.T.);
#62248=ORIENTED_EDGE('',*,*,#46195,.T.);
#62249=ORIENTED_EDGE('',*,*,#46196,.T.);
#62250=ORIENTED_EDGE('',*,*,#46195,.F.);
#62251=ORIENTED_EDGE('',*,*,#45257,.T.);
#62252=ORIENTED_EDGE('',*,*,#46197,.T.);
#62253=ORIENTED_EDGE('',*,*,#46198,.T.);
#62254=ORIENTED_EDGE('',*,*,#46197,.F.);
#62255=ORIENTED_EDGE('',*,*,#45256,.T.);
#62256=ORIENTED_EDGE('',*,*,#46199,.T.);
#62257=ORIENTED_EDGE('',*,*,#46200,.T.);
#62258=ORIENTED_EDGE('',*,*,#46199,.F.);
#62259=ORIENTED_EDGE('',*,*,#45255,.T.);
#62260=ORIENTED_EDGE('',*,*,#46201,.F.);
#62261=ORIENTED_EDGE('',*,*,#46202,.T.);
#62262=ORIENTED_EDGE('',*,*,#46203,.F.);
#62263=ORIENTED_EDGE('',*,*,#46204,.T.);
#62264=ORIENTED_EDGE('',*,*,#46201,.T.);
#62265=ORIENTED_EDGE('',*,*,#45254,.T.);
#62266=ORIENTED_EDGE('',*,*,#46205,.F.);
#62267=ORIENTED_EDGE('',*,*,#46206,.T.);
#62268=ORIENTED_EDGE('',*,*,#46203,.T.);
#62269=ORIENTED_EDGE('',*,*,#45253,.T.);
#62270=ORIENTED_EDGE('',*,*,#46207,.F.);
#62271=ORIENTED_EDGE('',*,*,#46208,.T.);
#62272=ORIENTED_EDGE('',*,*,#46205,.T.);
#62273=ORIENTED_EDGE('',*,*,#45252,.T.);
#62274=ORIENTED_EDGE('',*,*,#46209,.F.);
#62275=ORIENTED_EDGE('',*,*,#46210,.T.);
#62276=ORIENTED_EDGE('',*,*,#46207,.T.);
#62277=ORIENTED_EDGE('',*,*,#45251,.T.);
#62278=ORIENTED_EDGE('',*,*,#45261,.F.);
#62279=ORIENTED_EDGE('',*,*,#45263,.T.);
#62280=ORIENTED_EDGE('',*,*,#46209,.T.);
#62281=ORIENTED_EDGE('',*,*,#45250,.T.);
#62282=ORIENTED_EDGE('',*,*,#46211,.F.);
#62283=ORIENTED_EDGE('',*,*,#46212,.T.);
#62284=ORIENTED_EDGE('',*,*,#46186,.T.);
#62285=ORIENTED_EDGE('',*,*,#45247,.T.);
#62286=ORIENTED_EDGE('',*,*,#46188,.F.);
#62287=ORIENTED_EDGE('',*,*,#46213,.T.);
#62288=ORIENTED_EDGE('',*,*,#46211,.T.);
#62289=ORIENTED_EDGE('',*,*,#45246,.T.);
#62290=ORIENTED_EDGE('',*,*,#46214,.T.);
#62291=ORIENTED_EDGE('',*,*,#46210,.F.);
#62292=ORIENTED_EDGE('',*,*,#45262,.T.);
#62293=ORIENTED_EDGE('',*,*,#46215,.F.);
#62294=ORIENTED_EDGE('',*,*,#46216,.F.);
#62295=ORIENTED_EDGE('',*,*,#45264,.T.);
#62296=ORIENTED_EDGE('',*,*,#45265,.T.);
#62297=ORIENTED_EDGE('',*,*,#45282,.T.);
#62298=ORIENTED_EDGE('',*,*,#46217,.F.);
#62299=ORIENTED_EDGE('',*,*,#46215,.T.);
#62300=ORIENTED_EDGE('',*,*,#46216,.T.);
#62301=ORIENTED_EDGE('',*,*,#45281,.T.);
#62302=ORIENTED_EDGE('',*,*,#46218,.F.);
#62303=ORIENTED_EDGE('',*,*,#46219,.T.);
#62304=ORIENTED_EDGE('',*,*,#46217,.T.);
#62305=ORIENTED_EDGE('',*,*,#45280,.T.);
#62306=ORIENTED_EDGE('',*,*,#46220,.F.);
#62307=ORIENTED_EDGE('',*,*,#46221,.T.);
#62308=ORIENTED_EDGE('',*,*,#46218,.T.);
#62309=ORIENTED_EDGE('',*,*,#45279,.T.);
#62310=ORIENTED_EDGE('',*,*,#46222,.F.);
#62311=ORIENTED_EDGE('',*,*,#46223,.T.);
#62312=ORIENTED_EDGE('',*,*,#46220,.T.);
#62313=ORIENTED_EDGE('',*,*,#45278,.T.);
#62314=ORIENTED_EDGE('',*,*,#46224,.F.);
#62315=ORIENTED_EDGE('',*,*,#46225,.T.);
#62316=ORIENTED_EDGE('',*,*,#46222,.T.);
#62317=ORIENTED_EDGE('',*,*,#45277,.T.);
#62318=ORIENTED_EDGE('',*,*,#46226,.F.);
#62319=ORIENTED_EDGE('',*,*,#46227,.T.);
#62320=ORIENTED_EDGE('',*,*,#46224,.T.);
#62321=ORIENTED_EDGE('',*,*,#45276,.T.);
#62322=ORIENTED_EDGE('',*,*,#46228,.F.);
#62323=ORIENTED_EDGE('',*,*,#46229,.T.);
#62324=ORIENTED_EDGE('',*,*,#46226,.T.);
#62325=ORIENTED_EDGE('',*,*,#45275,.T.);
#62326=ORIENTED_EDGE('',*,*,#46230,.F.);
#62327=ORIENTED_EDGE('',*,*,#46231,.T.);
#62328=ORIENTED_EDGE('',*,*,#46228,.T.);
#62329=ORIENTED_EDGE('',*,*,#45274,.T.);
#62330=ORIENTED_EDGE('',*,*,#46232,.F.);
#62331=ORIENTED_EDGE('',*,*,#46233,.T.);
#62332=ORIENTED_EDGE('',*,*,#46230,.T.);
#62333=ORIENTED_EDGE('',*,*,#45273,.T.);
#62334=ORIENTED_EDGE('',*,*,#46234,.F.);
#62335=ORIENTED_EDGE('',*,*,#45470,.T.);
#62336=ORIENTED_EDGE('',*,*,#46232,.T.);
#62337=ORIENTED_EDGE('',*,*,#45272,.T.);
#62338=ORIENTED_EDGE('',*,*,#45271,.T.);
#62339=ORIENTED_EDGE('',*,*,#46235,.F.);
#62340=ORIENTED_EDGE('',*,*,#46236,.T.);
#62341=ORIENTED_EDGE('',*,*,#46237,.F.);
#62342=ORIENTED_EDGE('',*,*,#46238,.F.);
#62343=ORIENTED_EDGE('',*,*,#46239,.T.);
#62344=ORIENTED_EDGE('',*,*,#46235,.T.);
#62345=ORIENTED_EDGE('',*,*,#45270,.T.);
#62346=ORIENTED_EDGE('',*,*,#46240,.F.);
#62347=ORIENTED_EDGE('',*,*,#46241,.T.);
#62348=ORIENTED_EDGE('',*,*,#46238,.T.);
#62349=ORIENTED_EDGE('',*,*,#45269,.T.);
#62350=ORIENTED_EDGE('',*,*,#45284,.F.);
#62351=ORIENTED_EDGE('',*,*,#46242,.T.);
#62352=ORIENTED_EDGE('',*,*,#46240,.T.);
#62353=ORIENTED_EDGE('',*,*,#45268,.T.);
#62354=ORIENTED_EDGE('',*,*,#45286,.T.);
#62355=ORIENTED_EDGE('',*,*,#46243,.F.);
#62356=ORIENTED_EDGE('',*,*,#46244,.T.);
#62357=ORIENTED_EDGE('',*,*,#46242,.F.);
#62358=ORIENTED_EDGE('',*,*,#46245,.F.);
#62359=ORIENTED_EDGE('',*,*,#46243,.T.);
#62360=ORIENTED_EDGE('',*,*,#45288,.T.);
#62361=ORIENTED_EDGE('',*,*,#45294,.T.);
#62362=ORIENTED_EDGE('',*,*,#46146,.F.);
#62363=ORIENTED_EDGE('',*,*,#45295,.T.);
#62364=ORIENTED_EDGE('',*,*,#45289,.T.);
#62365=ORIENTED_EDGE('',*,*,#45306,.T.);
#62366=ORIENTED_EDGE('',*,*,#46246,.T.);
#62367=ORIENTED_EDGE('',*,*,#46247,.T.);
#62368=ORIENTED_EDGE('',*,*,#45291,.T.);
#62369=ORIENTED_EDGE('',*,*,#46248,.F.);
#62370=ORIENTED_EDGE('',*,*,#46249,.T.);
#62371=ORIENTED_EDGE('',*,*,#45474,.T.);
#62372=ORIENTED_EDGE('',*,*,#46250,.F.);
#62373=ORIENTED_EDGE('',*,*,#45305,.T.);
#62374=ORIENTED_EDGE('',*,*,#46251,.T.);
#62375=ORIENTED_EDGE('',*,*,#46251,.F.);
#62376=ORIENTED_EDGE('',*,*,#45304,.T.);
#62377=ORIENTED_EDGE('',*,*,#46252,.T.);
#62378=ORIENTED_EDGE('',*,*,#46253,.T.);
#62379=ORIENTED_EDGE('',*,*,#46249,.F.);
#62380=ORIENTED_EDGE('',*,*,#46252,.F.);
#62381=ORIENTED_EDGE('',*,*,#45303,.T.);
#62382=ORIENTED_EDGE('',*,*,#46254,.T.);
#62383=ORIENTED_EDGE('',*,*,#46255,.T.);
#62384=ORIENTED_EDGE('',*,*,#46254,.F.);
#62385=ORIENTED_EDGE('',*,*,#45302,.T.);
#62386=ORIENTED_EDGE('',*,*,#46256,.T.);
#62387=ORIENTED_EDGE('',*,*,#46257,.T.);
#62388=ORIENTED_EDGE('',*,*,#46256,.F.);
#62389=ORIENTED_EDGE('',*,*,#45301,.T.);
#62390=ORIENTED_EDGE('',*,*,#46258,.T.);
#62391=ORIENTED_EDGE('',*,*,#46259,.T.);
#62392=ORIENTED_EDGE('',*,*,#46258,.F.);
#62393=ORIENTED_EDGE('',*,*,#45300,.T.);
#62394=ORIENTED_EDGE('',*,*,#46260,.T.);
#62395=ORIENTED_EDGE('',*,*,#46261,.T.);
#62396=ORIENTED_EDGE('',*,*,#46260,.F.);
#62397=ORIENTED_EDGE('',*,*,#45299,.T.);
#62398=ORIENTED_EDGE('',*,*,#46262,.T.);
#62399=ORIENTED_EDGE('',*,*,#46263,.T.);
#62400=ORIENTED_EDGE('',*,*,#46262,.F.);
#62401=ORIENTED_EDGE('',*,*,#45298,.T.);
#62402=ORIENTED_EDGE('',*,*,#46264,.T.);
#62403=ORIENTED_EDGE('',*,*,#46265,.T.);
#62404=ORIENTED_EDGE('',*,*,#46264,.F.);
#62405=ORIENTED_EDGE('',*,*,#45297,.T.);
#62406=ORIENTED_EDGE('',*,*,#46145,.T.);
#62407=ORIENTED_EDGE('',*,*,#46142,.T.);
#62408=ORIENTED_EDGE('',*,*,#46266,.F.);
#62409=ORIENTED_EDGE('',*,*,#46267,.T.);
#62410=ORIENTED_EDGE('',*,*,#46245,.T.);
#62411=ORIENTED_EDGE('',*,*,#45293,.T.);
#62412=ORIENTED_EDGE('',*,*,#46247,.F.);
#62413=ORIENTED_EDGE('',*,*,#46268,.T.);
#62414=ORIENTED_EDGE('',*,*,#46266,.T.);
#62415=ORIENTED_EDGE('',*,*,#45292,.T.);
#62416=ORIENTED_EDGE('',*,*,#45330,.T.);
#62417=ORIENTED_EDGE('',*,*,#46182,.F.);
#62418=ORIENTED_EDGE('',*,*,#46269,.F.);
#62419=ORIENTED_EDGE('',*,*,#45908,.F.);
#62420=ORIENTED_EDGE('',*,*,#46050,.F.);
#62421=ORIENTED_EDGE('',*,*,#45320,.F.);
#62422=ORIENTED_EDGE('',*,*,#46006,.F.);
#62423=ORIENTED_EDGE('',*,*,#45350,.F.);
#62424=ORIENTED_EDGE('',*,*,#45334,.F.);
#62425=ORIENTED_EDGE('',*,*,#45934,.F.);
#62426=ORIENTED_EDGE('',*,*,#46270,.F.);
#62427=ORIENTED_EDGE('',*,*,#45624,.F.);
#62428=ORIENTED_EDGE('',*,*,#45371,.T.);
#62429=ORIENTED_EDGE('',*,*,#46005,.F.);
#62430=ORIENTED_EDGE('',*,*,#45625,.T.);
#62431=ORIENTED_EDGE('',*,*,#45632,.F.);
#62432=ORIENTED_EDGE('',*,*,#45381,.T.);
#62433=ORIENTED_EDGE('',*,*,#46012,.F.);
#62434=ORIENTED_EDGE('',*,*,#46271,.T.);
#62435=ORIENTED_EDGE('',*,*,#46000,.F.);
#62436=ORIENTED_EDGE('',*,*,#45384,.T.);
#62437=ORIENTED_EDGE('',*,*,#45385,.T.);
#62438=ORIENTED_EDGE('',*,*,#46061,.T.);
#62439=ORIENTED_EDGE('',*,*,#45397,.T.);
#62440=ORIENTED_EDGE('',*,*,#46272,.F.);
#62441=ORIENTED_EDGE('',*,*,#45520,.T.);
#62442=ORIENTED_EDGE('',*,*,#45392,.F.);
#62443=ORIENTED_EDGE('',*,*,#46273,.F.);
#62444=ORIENTED_EDGE('',*,*,#45521,.T.);
#62445=ORIENTED_EDGE('',*,*,#46272,.T.);
#62446=ORIENTED_EDGE('',*,*,#45399,.T.);
#62447=ORIENTED_EDGE('',*,*,#46274,.F.);
#62448=ORIENTED_EDGE('',*,*,#45522,.T.);
#62449=ORIENTED_EDGE('',*,*,#46273,.T.);
#62450=ORIENTED_EDGE('',*,*,#45401,.T.);
#62451=ORIENTED_EDGE('',*,*,#46275,.F.);
#62452=ORIENTED_EDGE('',*,*,#45523,.T.);
#62453=ORIENTED_EDGE('',*,*,#46274,.T.);
#62454=ORIENTED_EDGE('',*,*,#45403,.T.);
#62455=ORIENTED_EDGE('',*,*,#45524,.T.);
#62456=ORIENTED_EDGE('',*,*,#46275,.T.);
#62457=ORIENTED_EDGE('',*,*,#45404,.T.);
#62458=ORIENTED_EDGE('',*,*,#46060,.F.);
#62459=ORIENTED_EDGE('',*,*,#46276,.F.);
#62460=ORIENTED_EDGE('',*,*,#46056,.T.);
#62461=ORIENTED_EDGE('',*,*,#46057,.T.);
#62462=ORIENTED_EDGE('',*,*,#45417,.T.);
#62463=ORIENTED_EDGE('',*,*,#46277,.F.);
#62464=ORIENTED_EDGE('',*,*,#46278,.T.);
#62465=ORIENTED_EDGE('',*,*,#46276,.T.);
#62466=ORIENTED_EDGE('',*,*,#45416,.T.);
#62467=ORIENTED_EDGE('',*,*,#46024,.F.);
#62468=ORIENTED_EDGE('',*,*,#46027,.T.);
#62469=ORIENTED_EDGE('',*,*,#46277,.T.);
#62470=ORIENTED_EDGE('',*,*,#45415,.T.);
#62471=ORIENTED_EDGE('',*,*,#45413,.T.);
#62472=ORIENTED_EDGE('',*,*,#46123,.F.);
#62473=ORIENTED_EDGE('',*,*,#46279,.T.);
#62474=ORIENTED_EDGE('',*,*,#46023,.F.);
#62475=ORIENTED_EDGE('',*,*,#46280,.F.);
#62476=ORIENTED_EDGE('',*,*,#46119,.T.);
#62477=ORIENTED_EDGE('',*,*,#46120,.T.);
#62478=ORIENTED_EDGE('',*,*,#45411,.T.);
#62479=ORIENTED_EDGE('',*,*,#46281,.F.);
#62480=ORIENTED_EDGE('',*,*,#46282,.T.);
#62481=ORIENTED_EDGE('',*,*,#46280,.T.);
#62482=ORIENTED_EDGE('',*,*,#45410,.T.);
#62483=ORIENTED_EDGE('',*,*,#46281,.T.);
#62484=ORIENTED_EDGE('',*,*,#45409,.T.);
#62485=ORIENTED_EDGE('',*,*,#46105,.T.);
#62486=ORIENTED_EDGE('',*,*,#46108,.T.);
#62487=ORIENTED_EDGE('',*,*,#45407,.T.);
#62488=ORIENTED_EDGE('',*,*,#46283,.T.);
#62489=ORIENTED_EDGE('',*,*,#46284,.T.);
#62490=ORIENTED_EDGE('',*,*,#46104,.F.);
#62491=ORIENTED_EDGE('',*,*,#46283,.F.);
#62492=ORIENTED_EDGE('',*,*,#45406,.T.);
#62493=ORIENTED_EDGE('',*,*,#46285,.T.);
#62494=ORIENTED_EDGE('',*,*,#46286,.T.);
#62495=ORIENTED_EDGE('',*,*,#46067,.F.);
#62496=ORIENTED_EDGE('',*,*,#45422,.T.);
#62497=ORIENTED_EDGE('',*,*,#46287,.F.);
#62498=ORIENTED_EDGE('',*,*,#46065,.T.);
#62499=ORIENTED_EDGE('',*,*,#46288,.T.);
#62500=ORIENTED_EDGE('',*,*,#46285,.F.);
#62501=ORIENTED_EDGE('',*,*,#45420,.T.);
#62502=ORIENTED_EDGE('',*,*,#46069,.F.);
#62503=ORIENTED_EDGE('',*,*,#46289,.F.);
#62504=ORIENTED_EDGE('',*,*,#46062,.T.);
#62505=ORIENTED_EDGE('',*,*,#46287,.T.);
#62506=ORIENTED_EDGE('',*,*,#45464,.T.);
#62507=ORIENTED_EDGE('',*,*,#46290,.F.);
#62508=ORIENTED_EDGE('',*,*,#46291,.T.);
#62509=ORIENTED_EDGE('',*,*,#46289,.T.);
#62510=ORIENTED_EDGE('',*,*,#45463,.T.);
#62511=ORIENTED_EDGE('',*,*,#45856,.F.);
#62512=ORIENTED_EDGE('',*,*,#45859,.T.);
#62513=ORIENTED_EDGE('',*,*,#46290,.T.);
#62514=ORIENTED_EDGE('',*,*,#45462,.T.);
#62515=ORIENTED_EDGE('',*,*,#45460,.T.);
#62516=ORIENTED_EDGE('',*,*,#45842,.F.);
#62517=ORIENTED_EDGE('',*,*,#46292,.T.);
#62518=ORIENTED_EDGE('',*,*,#45855,.F.);
#62519=ORIENTED_EDGE('',*,*,#45840,.F.);
#62520=ORIENTED_EDGE('',*,*,#45458,.T.);
#62521=ORIENTED_EDGE('',*,*,#46293,.T.);
#62522=ORIENTED_EDGE('',*,*,#45838,.T.);
#62523=ORIENTED_EDGE('',*,*,#46293,.F.);
#62524=ORIENTED_EDGE('',*,*,#45457,.T.);
#62525=ORIENTED_EDGE('',*,*,#46294,.T.);
#62526=ORIENTED_EDGE('',*,*,#46295,.T.);
#62527=ORIENTED_EDGE('',*,*,#46294,.F.);
#62528=ORIENTED_EDGE('',*,*,#45456,.T.);
#62529=ORIENTED_EDGE('',*,*,#46296,.T.);
#62530=ORIENTED_EDGE('',*,*,#46297,.T.);
#62531=ORIENTED_EDGE('',*,*,#46296,.F.);
#62532=ORIENTED_EDGE('',*,*,#45455,.T.);
#62533=ORIENTED_EDGE('',*,*,#45821,.T.);
#62534=ORIENTED_EDGE('',*,*,#45825,.T.);
#62535=ORIENTED_EDGE('',*,*,#45453,.T.);
#62536=ORIENTED_EDGE('',*,*,#45801,.F.);
#62537=ORIENTED_EDGE('',*,*,#46298,.T.);
#62538=ORIENTED_EDGE('',*,*,#45820,.F.);
#62539=ORIENTED_EDGE('',*,*,#46299,.F.);
#62540=ORIENTED_EDGE('',*,*,#45797,.T.);
#62541=ORIENTED_EDGE('',*,*,#45798,.T.);
#62542=ORIENTED_EDGE('',*,*,#45451,.T.);
#62543=ORIENTED_EDGE('',*,*,#46300,.F.);
#62544=ORIENTED_EDGE('',*,*,#46301,.T.);
#62545=ORIENTED_EDGE('',*,*,#46299,.T.);
#62546=ORIENTED_EDGE('',*,*,#45450,.T.);
#62547=ORIENTED_EDGE('',*,*,#46300,.T.);
#62548=ORIENTED_EDGE('',*,*,#45449,.T.);
#62549=ORIENTED_EDGE('',*,*,#45787,.T.);
#62550=ORIENTED_EDGE('',*,*,#45790,.T.);
#62551=ORIENTED_EDGE('',*,*,#45447,.T.);
#62552=ORIENTED_EDGE('',*,*,#45767,.F.);
#62553=ORIENTED_EDGE('',*,*,#46302,.T.);
#62554=ORIENTED_EDGE('',*,*,#45786,.F.);
#62555=ORIENTED_EDGE('',*,*,#46303,.F.);
#62556=ORIENTED_EDGE('',*,*,#45763,.T.);
#62557=ORIENTED_EDGE('',*,*,#45764,.T.);
#62558=ORIENTED_EDGE('',*,*,#45445,.T.);
#62559=ORIENTED_EDGE('',*,*,#46304,.F.);
#62560=ORIENTED_EDGE('',*,*,#46305,.T.);
#62561=ORIENTED_EDGE('',*,*,#46303,.T.);
#62562=ORIENTED_EDGE('',*,*,#45444,.T.);
#62563=ORIENTED_EDGE('',*,*,#46304,.T.);
#62564=ORIENTED_EDGE('',*,*,#45443,.T.);
#62565=ORIENTED_EDGE('',*,*,#45753,.T.);
#62566=ORIENTED_EDGE('',*,*,#45756,.T.);
#62567=ORIENTED_EDGE('',*,*,#45441,.T.);
#62568=ORIENTED_EDGE('',*,*,#45733,.F.);
#62569=ORIENTED_EDGE('',*,*,#46306,.T.);
#62570=ORIENTED_EDGE('',*,*,#45752,.F.);
#62571=ORIENTED_EDGE('',*,*,#46307,.F.);
#62572=ORIENTED_EDGE('',*,*,#45729,.T.);
#62573=ORIENTED_EDGE('',*,*,#45730,.T.);
#62574=ORIENTED_EDGE('',*,*,#45439,.T.);
#62575=ORIENTED_EDGE('',*,*,#46308,.F.);
#62576=ORIENTED_EDGE('',*,*,#46309,.T.);
#62577=ORIENTED_EDGE('',*,*,#46307,.T.);
#62578=ORIENTED_EDGE('',*,*,#45438,.T.);
#62579=ORIENTED_EDGE('',*,*,#46308,.T.);
#62580=ORIENTED_EDGE('',*,*,#45437,.T.);
#62581=ORIENTED_EDGE('',*,*,#45719,.T.);
#62582=ORIENTED_EDGE('',*,*,#45722,.T.);
#62583=ORIENTED_EDGE('',*,*,#45435,.T.);
#62584=ORIENTED_EDGE('',*,*,#45699,.F.);
#62585=ORIENTED_EDGE('',*,*,#46310,.T.);
#62586=ORIENTED_EDGE('',*,*,#45718,.F.);
#62587=ORIENTED_EDGE('',*,*,#45697,.F.);
#62588=ORIENTED_EDGE('',*,*,#45433,.T.);
#62589=ORIENTED_EDGE('',*,*,#46311,.T.);
#62590=ORIENTED_EDGE('',*,*,#45695,.T.);
#62591=ORIENTED_EDGE('',*,*,#46311,.F.);
#62592=ORIENTED_EDGE('',*,*,#45432,.T.);
#62593=ORIENTED_EDGE('',*,*,#46312,.T.);
#62594=ORIENTED_EDGE('',*,*,#46313,.T.);
#62595=ORIENTED_EDGE('',*,*,#46312,.F.);
#62596=ORIENTED_EDGE('',*,*,#45431,.T.);
#62597=ORIENTED_EDGE('',*,*,#46314,.T.);
#62598=ORIENTED_EDGE('',*,*,#46315,.T.);
#62599=ORIENTED_EDGE('',*,*,#46314,.F.);
#62600=ORIENTED_EDGE('',*,*,#45430,.T.);
#62601=ORIENTED_EDGE('',*,*,#45678,.T.);
#62602=ORIENTED_EDGE('',*,*,#45681,.T.);
#62603=ORIENTED_EDGE('',*,*,#45428,.T.);
#62604=ORIENTED_EDGE('',*,*,#45654,.F.);
#62605=ORIENTED_EDGE('',*,*,#46316,.T.);
#62606=ORIENTED_EDGE('',*,*,#45677,.F.);
#62607=ORIENTED_EDGE('',*,*,#45652,.F.);
#62608=ORIENTED_EDGE('',*,*,#45426,.T.);
#62609=ORIENTED_EDGE('',*,*,#46317,.F.);
#62610=ORIENTED_EDGE('',*,*,#45650,.T.);
#62611=ORIENTED_EDGE('',*,*,#46318,.F.);
#62612=ORIENTED_EDGE('',*,*,#46319,.T.);
#62613=ORIENTED_EDGE('',*,*,#46317,.T.);
#62614=ORIENTED_EDGE('',*,*,#45425,.T.);
#62615=ORIENTED_EDGE('',*,*,#46320,.F.);
#62616=ORIENTED_EDGE('',*,*,#46154,.T.);
#62617=ORIENTED_EDGE('',*,*,#46318,.T.);
#62618=ORIENTED_EDGE('',*,*,#45424,.T.);
#62619=ORIENTED_EDGE('',*,*,#46150,.F.);
#62620=ORIENTED_EDGE('',*,*,#46151,.T.);
#62621=ORIENTED_EDGE('',*,*,#46320,.T.);
#62622=ORIENTED_EDGE('',*,*,#45468,.T.);
#62623=ORIENTED_EDGE('',*,*,#45466,.T.);
#62624=ORIENTED_EDGE('',*,*,#46321,.F.);
#62625=ORIENTED_EDGE('',*,*,#46322,.T.);
#62626=ORIENTED_EDGE('',*,*,#46149,.F.);
#62627=ORIENTED_EDGE('',*,*,#45469,.T.);
#62628=ORIENTED_EDGE('',*,*,#46194,.F.);
#62629=ORIENTED_EDGE('',*,*,#46323,.T.);
#62630=ORIENTED_EDGE('',*,*,#46233,.F.);
#62631=ORIENTED_EDGE('',*,*,#46324,.F.);
#62632=ORIENTED_EDGE('',*,*,#46189,.T.);
#62633=ORIENTED_EDGE('',*,*,#46191,.T.);
#62634=ORIENTED_EDGE('',*,*,#45482,.T.);
#62635=ORIENTED_EDGE('',*,*,#46325,.F.);
#62636=ORIENTED_EDGE('',*,*,#46326,.T.);
#62637=ORIENTED_EDGE('',*,*,#46324,.T.);
#62638=ORIENTED_EDGE('',*,*,#45481,.T.);
#62639=ORIENTED_EDGE('',*,*,#46171,.F.);
#62640=ORIENTED_EDGE('',*,*,#46174,.T.);
#62641=ORIENTED_EDGE('',*,*,#46325,.T.);
#62642=ORIENTED_EDGE('',*,*,#45480,.T.);
#62643=ORIENTED_EDGE('',*,*,#45478,.T.);
#62644=ORIENTED_EDGE('',*,*,#46327,.F.);
#62645=ORIENTED_EDGE('',*,*,#45506,.T.);
#62646=ORIENTED_EDGE('',*,*,#46170,.F.);
#62647=ORIENTED_EDGE('',*,*,#46328,.F.);
#62648=ORIENTED_EDGE('',*,*,#46329,.T.);
#62649=ORIENTED_EDGE('',*,*,#46321,.T.);
#62650=ORIENTED_EDGE('',*,*,#45476,.T.);
#62651=ORIENTED_EDGE('',*,*,#46330,.T.);
#62652=ORIENTED_EDGE('',*,*,#46328,.T.);
#62653=ORIENTED_EDGE('',*,*,#45475,.T.);
#62654=ORIENTED_EDGE('',*,*,#46253,.F.);
#62655=ORIENTED_EDGE('',*,*,#46331,.F.);
#62656=ORIENTED_EDGE('',*,*,#46248,.T.);
#62657=ORIENTED_EDGE('',*,*,#46250,.T.);
#62658=ORIENTED_EDGE('',*,*,#45473,.T.);
#62659=ORIENTED_EDGE('',*,*,#46332,.F.);
#62660=ORIENTED_EDGE('',*,*,#46333,.T.);
#62661=ORIENTED_EDGE('',*,*,#46331,.T.);
#62662=ORIENTED_EDGE('',*,*,#45472,.T.);
#62663=ORIENTED_EDGE('',*,*,#46332,.T.);
#62664=ORIENTED_EDGE('',*,*,#45471,.T.);
#62665=ORIENTED_EDGE('',*,*,#46234,.T.);
#62666=ORIENTED_EDGE('',*,*,#46237,.T.);
#62667=ORIENTED_EDGE('',*,*,#46334,.F.);
#62668=ORIENTED_EDGE('',*,*,#45507,.T.);
#62669=ORIENTED_EDGE('',*,*,#46327,.T.);
#62670=ORIENTED_EDGE('',*,*,#45485,.T.);
#62671=ORIENTED_EDGE('',*,*,#46335,.F.);
#62672=ORIENTED_EDGE('',*,*,#45508,.T.);
#62673=ORIENTED_EDGE('',*,*,#46334,.T.);
#62674=ORIENTED_EDGE('',*,*,#45487,.T.);
#62675=ORIENTED_EDGE('',*,*,#46336,.F.);
#62676=ORIENTED_EDGE('',*,*,#45509,.T.);
#62677=ORIENTED_EDGE('',*,*,#46335,.T.);
#62678=ORIENTED_EDGE('',*,*,#45489,.T.);
#62679=ORIENTED_EDGE('',*,*,#45510,.T.);
#62680=ORIENTED_EDGE('',*,*,#46336,.T.);
#62681=ORIENTED_EDGE('',*,*,#45490,.T.);
#62682=ORIENTED_EDGE('',*,*,#45919,.F.);
#62683=ORIENTED_EDGE('',*,*,#46337,.F.);
#62684=ORIENTED_EDGE('',*,*,#45915,.T.);
#62685=ORIENTED_EDGE('',*,*,#45916,.T.);
#62686=ORIENTED_EDGE('',*,*,#45502,.T.);
#62687=ORIENTED_EDGE('',*,*,#46338,.F.);
#62688=ORIENTED_EDGE('',*,*,#46339,.T.);
#62689=ORIENTED_EDGE('',*,*,#46337,.T.);
#62690=ORIENTED_EDGE('',*,*,#45501,.T.);
#62691=ORIENTED_EDGE('',*,*,#45880,.F.);
#62692=ORIENTED_EDGE('',*,*,#45883,.T.);
#62693=ORIENTED_EDGE('',*,*,#46338,.T.);
#62694=ORIENTED_EDGE('',*,*,#45500,.T.);
#62695=ORIENTED_EDGE('',*,*,#45498,.T.);
#62696=ORIENTED_EDGE('',*,*,#45973,.F.);
#62697=ORIENTED_EDGE('',*,*,#46340,.T.);
#62698=ORIENTED_EDGE('',*,*,#45879,.F.);
#62699=ORIENTED_EDGE('',*,*,#46341,.F.);
#62700=ORIENTED_EDGE('',*,*,#45969,.T.);
#62701=ORIENTED_EDGE('',*,*,#45970,.T.);
#62702=ORIENTED_EDGE('',*,*,#45496,.T.);
#62703=ORIENTED_EDGE('',*,*,#46342,.F.);
#62704=ORIENTED_EDGE('',*,*,#46343,.T.);
#62705=ORIENTED_EDGE('',*,*,#46341,.T.);
#62706=ORIENTED_EDGE('',*,*,#45495,.T.);
#62707=ORIENTED_EDGE('',*,*,#46342,.T.);
#62708=ORIENTED_EDGE('',*,*,#45494,.T.);
#62709=ORIENTED_EDGE('',*,*,#45955,.T.);
#62710=ORIENTED_EDGE('',*,*,#45958,.T.);
#62711=ORIENTED_EDGE('',*,*,#45492,.T.);
#62712=ORIENTED_EDGE('',*,*,#46344,.T.);
#62713=ORIENTED_EDGE('',*,*,#46345,.T.);
#62714=ORIENTED_EDGE('',*,*,#45954,.F.);
#62715=ORIENTED_EDGE('',*,*,#46344,.F.);
#62716=ORIENTED_EDGE('',*,*,#45491,.T.);
#62717=ORIENTED_EDGE('',*,*,#45558,.T.);
#62718=ORIENTED_EDGE('',*,*,#46346,.T.);
#62719=ORIENTED_EDGE('',*,*,#45904,.F.);
#62720=ORIENTED_EDGE('',*,*,#45906,.T.);
#62721=ORIENTED_EDGE('',*,*,#46183,.T.);
#62722=ORIENTED_EDGE('',*,*,#45516,.T.);
#62723=ORIENTED_EDGE('',*,*,#45531,.T.);
#62724=ORIENTED_EDGE('',*,*,#45606,.F.);
#62725=ORIENTED_EDGE('',*,*,#46347,.T.);
#62726=ORIENTED_EDGE('',*,*,#45620,.F.);
#62727=ORIENTED_EDGE('',*,*,#46348,.T.);
#62728=ORIENTED_EDGE('',*,*,#45612,.F.);
#62729=ORIENTED_EDGE('',*,*,#45537,.T.);
#62730=ORIENTED_EDGE('',*,*,#45596,.F.);
#62731=ORIENTED_EDGE('',*,*,#45541,.T.);
#62732=ORIENTED_EDGE('',*,*,#45583,.F.);
#62733=ORIENTED_EDGE('',*,*,#46349,.T.);
#62734=ORIENTED_EDGE('',*,*,#45594,.F.);
#62735=ORIENTED_EDGE('',*,*,#45551,.T.);
#62736=ORIENTED_EDGE('',*,*,#45566,.F.);
#62737=ORIENTED_EDGE('',*,*,#46350,.T.);
#62738=ORIENTED_EDGE('',*,*,#45577,.F.);
#62739=ORIENTED_EDGE('',*,*,#46351,.T.);
#62740=ORIENTED_EDGE('',*,*,#46346,.F.);
#62741=ORIENTED_EDGE('',*,*,#45557,.F.);
#62742=ORIENTED_EDGE('',*,*,#45923,.F.);
#62743=ORIENTED_EDGE('',*,*,#46352,.T.);
#62744=ORIENTED_EDGE('',*,*,#45950,.F.);
#62745=ORIENTED_EDGE('',*,*,#46270,.T.);
#62746=ORIENTED_EDGE('',*,*,#45935,.F.);
#62747=ORIENTED_EDGE('',*,*,#45562,.T.);
#62748=ORIENTED_EDGE('',*,*,#45622,.F.);
#62749=ORIENTED_EDGE('',*,*,#46350,.F.);
#62750=ORIENTED_EDGE('',*,*,#45568,.F.);
#62751=ORIENTED_EDGE('',*,*,#45570,.F.);
#62752=ORIENTED_EDGE('',*,*,#45575,.F.);
#62753=ORIENTED_EDGE('',*,*,#46349,.F.);
#62754=ORIENTED_EDGE('',*,*,#45585,.F.);
#62755=ORIENTED_EDGE('',*,*,#45587,.F.);
#62756=ORIENTED_EDGE('',*,*,#45592,.F.);
#62757=ORIENTED_EDGE('',*,*,#45601,.F.);
#62758=ORIENTED_EDGE('',*,*,#45611,.F.);
#62759=ORIENTED_EDGE('',*,*,#46348,.F.);
#62760=ORIENTED_EDGE('',*,*,#45598,.F.);
#62761=ORIENTED_EDGE('',*,*,#46347,.F.);
#62762=ORIENTED_EDGE('',*,*,#45608,.F.);
#62763=ORIENTED_EDGE('',*,*,#45613,.F.);
#62764=ORIENTED_EDGE('',*,*,#45618,.F.);
#62765=ORIENTED_EDGE('',*,*,#45641,.F.);
#62766=ORIENTED_EDGE('',*,*,#46084,.F.);
#62767=ORIENTED_EDGE('',*,*,#46353,.F.);
#62768=ORIENTED_EDGE('',*,*,#45862,.F.);
#62769=ORIENTED_EDGE('',*,*,#45646,.F.);
#62770=ORIENTED_EDGE('',*,*,#45664,.F.);
#62771=ORIENTED_EDGE('',*,*,#46354,.F.);
#62772=ORIENTED_EDGE('',*,*,#46157,.F.);
#62773=ORIENTED_EDGE('',*,*,#46153,.F.);
#62774=ORIENTED_EDGE('',*,*,#46355,.F.);
#62775=ORIENTED_EDGE('',*,*,#45648,.F.);
#62776=ORIENTED_EDGE('',*,*,#46319,.F.);
#62777=ORIENTED_EDGE('',*,*,#46316,.F.);
#62778=ORIENTED_EDGE('',*,*,#45656,.F.);
#62779=ORIENTED_EDGE('',*,*,#46356,.F.);
#62780=ORIENTED_EDGE('',*,*,#45675,.F.);
#62781=ORIENTED_EDGE('',*,*,#46356,.T.);
#62782=ORIENTED_EDGE('',*,*,#45658,.F.);
#62783=ORIENTED_EDGE('',*,*,#46357,.T.);
#62784=ORIENTED_EDGE('',*,*,#45673,.F.);
#62785=ORIENTED_EDGE('',*,*,#45666,.F.);
#62786=ORIENTED_EDGE('',*,*,#45671,.F.);
#62787=ORIENTED_EDGE('',*,*,#46357,.F.);
#62788=ORIENTED_EDGE('',*,*,#45660,.F.);
#62789=ORIENTED_EDGE('',*,*,#46354,.T.);
#62790=ORIENTED_EDGE('',*,*,#45665,.F.);
#62791=ORIENTED_EDGE('',*,*,#46355,.T.);
#62792=ORIENTED_EDGE('',*,*,#46156,.F.);
#62793=ORIENTED_EDGE('',*,*,#45680,.F.);
#62794=ORIENTED_EDGE('',*,*,#46358,.F.);
#62795=ORIENTED_EDGE('',*,*,#46359,.F.);
#62796=ORIENTED_EDGE('',*,*,#46315,.F.);
#62797=ORIENTED_EDGE('',*,*,#46360,.T.);
#62798=ORIENTED_EDGE('',*,*,#45694,.F.);
#62799=ORIENTED_EDGE('',*,*,#46358,.T.);
#62800=ORIENTED_EDGE('',*,*,#45683,.F.);
#62801=ORIENTED_EDGE('',*,*,#45688,.F.);
#62802=ORIENTED_EDGE('',*,*,#45692,.F.);
#62803=ORIENTED_EDGE('',*,*,#46360,.F.);
#62804=ORIENTED_EDGE('',*,*,#45685,.F.);
#62805=ORIENTED_EDGE('',*,*,#46359,.T.);
#62806=ORIENTED_EDGE('',*,*,#45693,.T.);
#62807=ORIENTED_EDGE('',*,*,#46313,.F.);
#62808=ORIENTED_EDGE('',*,*,#46310,.F.);
#62809=ORIENTED_EDGE('',*,*,#45701,.F.);
#62810=ORIENTED_EDGE('',*,*,#46361,.F.);
#62811=ORIENTED_EDGE('',*,*,#45716,.F.);
#62812=ORIENTED_EDGE('',*,*,#46361,.T.);
#62813=ORIENTED_EDGE('',*,*,#45703,.F.);
#62814=ORIENTED_EDGE('',*,*,#46362,.T.);
#62815=ORIENTED_EDGE('',*,*,#45714,.F.);
#62816=ORIENTED_EDGE('',*,*,#46362,.F.);
#62817=ORIENTED_EDGE('',*,*,#45705,.F.);
#62818=ORIENTED_EDGE('',*,*,#45707,.F.);
#62819=ORIENTED_EDGE('',*,*,#45712,.F.);
#62820=ORIENTED_EDGE('',*,*,#45721,.F.);
#62821=ORIENTED_EDGE('',*,*,#45725,.T.);
#62822=ORIENTED_EDGE('',*,*,#45728,.F.);
#62823=ORIENTED_EDGE('',*,*,#46309,.F.);
#62824=ORIENTED_EDGE('',*,*,#46306,.F.);
#62825=ORIENTED_EDGE('',*,*,#45735,.F.);
#62826=ORIENTED_EDGE('',*,*,#46363,.F.);
#62827=ORIENTED_EDGE('',*,*,#45750,.F.);
#62828=ORIENTED_EDGE('',*,*,#46363,.T.);
#62829=ORIENTED_EDGE('',*,*,#45737,.F.);
#62830=ORIENTED_EDGE('',*,*,#46364,.T.);
#62831=ORIENTED_EDGE('',*,*,#45748,.F.);
#62832=ORIENTED_EDGE('',*,*,#46364,.F.);
#62833=ORIENTED_EDGE('',*,*,#45739,.F.);
#62834=ORIENTED_EDGE('',*,*,#45741,.F.);
#62835=ORIENTED_EDGE('',*,*,#45746,.F.);
#62836=ORIENTED_EDGE('',*,*,#45755,.F.);
#62837=ORIENTED_EDGE('',*,*,#45759,.T.);
#62838=ORIENTED_EDGE('',*,*,#45762,.F.);
#62839=ORIENTED_EDGE('',*,*,#46305,.F.);
#62840=ORIENTED_EDGE('',*,*,#46302,.F.);
#62841=ORIENTED_EDGE('',*,*,#45769,.F.);
#62842=ORIENTED_EDGE('',*,*,#46365,.F.);
#62843=ORIENTED_EDGE('',*,*,#45784,.F.);
#62844=ORIENTED_EDGE('',*,*,#46365,.T.);
#62845=ORIENTED_EDGE('',*,*,#45771,.F.);
#62846=ORIENTED_EDGE('',*,*,#46366,.T.);
#62847=ORIENTED_EDGE('',*,*,#45782,.F.);
#62848=ORIENTED_EDGE('',*,*,#46366,.F.);
#62849=ORIENTED_EDGE('',*,*,#45773,.F.);
#62850=ORIENTED_EDGE('',*,*,#45775,.F.);
#62851=ORIENTED_EDGE('',*,*,#45780,.F.);
#62852=ORIENTED_EDGE('',*,*,#45789,.F.);
#62853=ORIENTED_EDGE('',*,*,#45793,.T.);
#62854=ORIENTED_EDGE('',*,*,#45796,.F.);
#62855=ORIENTED_EDGE('',*,*,#46301,.F.);
#62856=ORIENTED_EDGE('',*,*,#46298,.F.);
#62857=ORIENTED_EDGE('',*,*,#45803,.F.);
#62858=ORIENTED_EDGE('',*,*,#46367,.F.);
#62859=ORIENTED_EDGE('',*,*,#45818,.F.);
#62860=ORIENTED_EDGE('',*,*,#46367,.T.);
#62861=ORIENTED_EDGE('',*,*,#45805,.F.);
#62862=ORIENTED_EDGE('',*,*,#46368,.T.);
#62863=ORIENTED_EDGE('',*,*,#45816,.F.);
#62864=ORIENTED_EDGE('',*,*,#45809,.F.);
#62865=ORIENTED_EDGE('',*,*,#45814,.F.);
#62866=ORIENTED_EDGE('',*,*,#46368,.F.);
#62867=ORIENTED_EDGE('',*,*,#45807,.F.);
#62868=ORIENTED_EDGE('',*,*,#45824,.F.);
#62869=ORIENTED_EDGE('',*,*,#46369,.T.);
#62870=ORIENTED_EDGE('',*,*,#46297,.F.);
#62871=ORIENTED_EDGE('',*,*,#46370,.T.);
#62872=ORIENTED_EDGE('',*,*,#45836,.F.);
#62873=ORIENTED_EDGE('',*,*,#46371,.T.);
#62874=ORIENTED_EDGE('',*,*,#45823,.F.);
#62875=ORIENTED_EDGE('',*,*,#45830,.F.);
#62876=ORIENTED_EDGE('',*,*,#45834,.F.);
#62877=ORIENTED_EDGE('',*,*,#46370,.F.);
#62878=ORIENTED_EDGE('',*,*,#45827,.F.);
#62879=ORIENTED_EDGE('',*,*,#46369,.F.);
#62880=ORIENTED_EDGE('',*,*,#46371,.F.);
#62881=ORIENTED_EDGE('',*,*,#45837,.F.);
#62882=ORIENTED_EDGE('',*,*,#46295,.F.);
#62883=ORIENTED_EDGE('',*,*,#46292,.F.);
#62884=ORIENTED_EDGE('',*,*,#45844,.F.);
#62885=ORIENTED_EDGE('',*,*,#46372,.F.);
#62886=ORIENTED_EDGE('',*,*,#45868,.F.);
#62887=ORIENTED_EDGE('',*,*,#46372,.T.);
#62888=ORIENTED_EDGE('',*,*,#45846,.F.);
#62889=ORIENTED_EDGE('',*,*,#46373,.T.);
#62890=ORIENTED_EDGE('',*,*,#45867,.F.);
#62891=ORIENTED_EDGE('',*,*,#46373,.F.);
#62892=ORIENTED_EDGE('',*,*,#45848,.F.);
#62893=ORIENTED_EDGE('',*,*,#45850,.F.);
#62894=ORIENTED_EDGE('',*,*,#45865,.F.);
#62895=ORIENTED_EDGE('',*,*,#45858,.F.);
#62896=ORIENTED_EDGE('',*,*,#46374,.F.);
#62897=ORIENTED_EDGE('',*,*,#46063,.F.);
#62898=ORIENTED_EDGE('',*,*,#46291,.F.);
#62899=ORIENTED_EDGE('',*,*,#46353,.T.);
#62900=ORIENTED_EDGE('',*,*,#46085,.F.);
#62901=ORIENTED_EDGE('',*,*,#46374,.T.);
#62902=ORIENTED_EDGE('',*,*,#45861,.F.);
#62903=ORIENTED_EDGE('',*,*,#46375,.T.);
#62904=ORIENTED_EDGE('',*,*,#45985,.F.);
#62905=ORIENTED_EDGE('',*,*,#46376,.T.);
#62906=ORIENTED_EDGE('',*,*,#45869,.F.);
#62907=ORIENTED_EDGE('',*,*,#45891,.F.);
#62908=ORIENTED_EDGE('',*,*,#45874,.F.);
#62909=ORIENTED_EDGE('',*,*,#46376,.F.);
#62910=ORIENTED_EDGE('',*,*,#45987,.F.);
#62911=ORIENTED_EDGE('',*,*,#45882,.F.);
#62912=ORIENTED_EDGE('',*,*,#46377,.F.);
#62913=ORIENTED_EDGE('',*,*,#45914,.F.);
#62914=ORIENTED_EDGE('',*,*,#46339,.F.);
#62915=ORIENTED_EDGE('',*,*,#46377,.T.);
#62916=ORIENTED_EDGE('',*,*,#45885,.F.);
#62917=ORIENTED_EDGE('',*,*,#46378,.T.);
#62918=ORIENTED_EDGE('',*,*,#45913,.F.);
#62919=ORIENTED_EDGE('',*,*,#46378,.F.);
#62920=ORIENTED_EDGE('',*,*,#45887,.F.);
#62921=ORIENTED_EDGE('',*,*,#45901,.F.);
#62922=ORIENTED_EDGE('',*,*,#45911,.F.);
#62923=ORIENTED_EDGE('',*,*,#46379,.F.);
#62924=ORIENTED_EDGE('',*,*,#45983,.F.);
#62925=ORIENTED_EDGE('',*,*,#46375,.F.);
#62926=ORIENTED_EDGE('',*,*,#45893,.F.);
#62927=ORIENTED_EDGE('',*,*,#46380,.F.);
#62928=ORIENTED_EDGE('',*,*,#46381,.T.);
#62929=ORIENTED_EDGE('',*,*,#45981,.F.);
#62930=ORIENTED_EDGE('',*,*,#46379,.T.);
#62931=ORIENTED_EDGE('',*,*,#45895,.F.);
#62932=ORIENTED_EDGE('',*,*,#46382,.F.);
#62933=ORIENTED_EDGE('',*,*,#46380,.T.);
#62934=ORIENTED_EDGE('',*,*,#45897,.F.);
#62935=ORIENTED_EDGE('',*,*,#46383,.T.);
#62936=ORIENTED_EDGE('',*,*,#45977,.F.);
#62937=ORIENTED_EDGE('',*,*,#46384,.T.);
#62938=ORIENTED_EDGE('',*,*,#46382,.T.);
#62939=ORIENTED_EDGE('',*,*,#45899,.F.);
#62940=ORIENTED_EDGE('',*,*,#46340,.F.);
#62941=ORIENTED_EDGE('',*,*,#45975,.F.);
#62942=ORIENTED_EDGE('',*,*,#46383,.F.);
#62943=ORIENTED_EDGE('',*,*,#45900,.F.);
#62944=ORIENTED_EDGE('',*,*,#45909,.F.);
#62945=ORIENTED_EDGE('',*,*,#46269,.T.);
#62946=ORIENTED_EDGE('',*,*,#46181,.T.);
#62947=ORIENTED_EDGE('',*,*,#45905,.T.);
#62948=ORIENTED_EDGE('',*,*,#46352,.F.);
#62949=ORIENTED_EDGE('',*,*,#45925,.F.);
#62950=ORIENTED_EDGE('',*,*,#46385,.F.);
#62951=ORIENTED_EDGE('',*,*,#45948,.F.);
#62952=ORIENTED_EDGE('',*,*,#46385,.T.);
#62953=ORIENTED_EDGE('',*,*,#45927,.F.);
#62954=ORIENTED_EDGE('',*,*,#46386,.T.);
#62955=ORIENTED_EDGE('',*,*,#45946,.F.);
#62956=ORIENTED_EDGE('',*,*,#46386,.F.);
#62957=ORIENTED_EDGE('',*,*,#45929,.F.);
#62958=ORIENTED_EDGE('',*,*,#46387,.F.);
#62959=ORIENTED_EDGE('',*,*,#45944,.F.);
#62960=ORIENTED_EDGE('',*,*,#46387,.T.);
#62961=ORIENTED_EDGE('',*,*,#45931,.F.);
#62962=ORIENTED_EDGE('',*,*,#45936,.T.);
#62963=ORIENTED_EDGE('',*,*,#45942,.F.);
#62964=ORIENTED_EDGE('',*,*,#46345,.F.);
#62965=ORIENTED_EDGE('',*,*,#46351,.F.);
#62966=ORIENTED_EDGE('',*,*,#45952,.F.);
#62967=ORIENTED_EDGE('',*,*,#45957,.F.);
#62968=ORIENTED_EDGE('',*,*,#46388,.F.);
#62969=ORIENTED_EDGE('',*,*,#45967,.F.);
#62970=ORIENTED_EDGE('',*,*,#46343,.F.);
#62971=ORIENTED_EDGE('',*,*,#46389,.T.);
#62972=ORIENTED_EDGE('',*,*,#45990,.F.);
#62973=ORIENTED_EDGE('',*,*,#46388,.T.);
#62974=ORIENTED_EDGE('',*,*,#45960,.F.);
#62975=ORIENTED_EDGE('',*,*,#45965,.F.);
#62976=ORIENTED_EDGE('',*,*,#45989,.F.);
#62977=ORIENTED_EDGE('',*,*,#46389,.F.);
#62978=ORIENTED_EDGE('',*,*,#45962,.F.);
#62979=ORIENTED_EDGE('',*,*,#46381,.F.);
#62980=ORIENTED_EDGE('',*,*,#46384,.F.);
#62981=ORIENTED_EDGE('',*,*,#45979,.F.);
#62982=ORIENTED_EDGE('',*,*,#46271,.F.);
#62983=ORIENTED_EDGE('',*,*,#46014,.F.);
#62984=ORIENTED_EDGE('',*,*,#45991,.F.);
#62985=ORIENTED_EDGE('',*,*,#45998,.F.);
#62986=ORIENTED_EDGE('',*,*,#46390,.F.);
#62987=ORIENTED_EDGE('',*,*,#46137,.F.);
#62988=ORIENTED_EDGE('',*,*,#46015,.F.);
#62989=ORIENTED_EDGE('',*,*,#46035,.F.);
#62990=ORIENTED_EDGE('',*,*,#46026,.F.);
#62991=ORIENTED_EDGE('',*,*,#46391,.F.);
#62992=ORIENTED_EDGE('',*,*,#46055,.F.);
#62993=ORIENTED_EDGE('',*,*,#46278,.F.);
#62994=ORIENTED_EDGE('',*,*,#46391,.T.);
#62995=ORIENTED_EDGE('',*,*,#46029,.F.);
#62996=ORIENTED_EDGE('',*,*,#46392,.T.);
#62997=ORIENTED_EDGE('',*,*,#46054,.F.);
#62998=ORIENTED_EDGE('',*,*,#46392,.F.);
#62999=ORIENTED_EDGE('',*,*,#46031,.F.);
#63000=ORIENTED_EDGE('',*,*,#46047,.F.);
#63001=ORIENTED_EDGE('',*,*,#46052,.F.);
#63002=ORIENTED_EDGE('',*,*,#46393,.T.);
#63003=ORIENTED_EDGE('',*,*,#46135,.F.);
#63004=ORIENTED_EDGE('',*,*,#46390,.T.);
#63005=ORIENTED_EDGE('',*,*,#46037,.F.);
#63006=ORIENTED_EDGE('',*,*,#46394,.F.);
#63007=ORIENTED_EDGE('',*,*,#46133,.F.);
#63008=ORIENTED_EDGE('',*,*,#46393,.F.);
#63009=ORIENTED_EDGE('',*,*,#46039,.F.);
#63010=ORIENTED_EDGE('',*,*,#46395,.T.);
#63011=ORIENTED_EDGE('',*,*,#46131,.F.);
#63012=ORIENTED_EDGE('',*,*,#46394,.T.);
#63013=ORIENTED_EDGE('',*,*,#46041,.F.);
#63014=ORIENTED_EDGE('',*,*,#46396,.F.);
#63015=ORIENTED_EDGE('',*,*,#46129,.F.);
#63016=ORIENTED_EDGE('',*,*,#46395,.F.);
#63017=ORIENTED_EDGE('',*,*,#46043,.F.);
#63018=ORIENTED_EDGE('',*,*,#46397,.T.);
#63019=ORIENTED_EDGE('',*,*,#46127,.F.);
#63020=ORIENTED_EDGE('',*,*,#46396,.T.);
#63021=ORIENTED_EDGE('',*,*,#46045,.F.);
#63022=ORIENTED_EDGE('',*,*,#46279,.F.);
#63023=ORIENTED_EDGE('',*,*,#46125,.F.);
#63024=ORIENTED_EDGE('',*,*,#46397,.F.);
#63025=ORIENTED_EDGE('',*,*,#46046,.F.);
#63026=ORIENTED_EDGE('',*,*,#46398,.T.);
#63027=ORIENTED_EDGE('',*,*,#46286,.F.);
#63028=ORIENTED_EDGE('',*,*,#46288,.F.);
#63029=ORIENTED_EDGE('',*,*,#46071,.F.);
#63030=ORIENTED_EDGE('',*,*,#46399,.T.);
#63031=ORIENTED_EDGE('',*,*,#46100,.F.);
#63032=ORIENTED_EDGE('',*,*,#46399,.F.);
#63033=ORIENTED_EDGE('',*,*,#46073,.F.);
#63034=ORIENTED_EDGE('',*,*,#46400,.F.);
#63035=ORIENTED_EDGE('',*,*,#46098,.F.);
#63036=ORIENTED_EDGE('',*,*,#46400,.T.);
#63037=ORIENTED_EDGE('',*,*,#46075,.F.);
#63038=ORIENTED_EDGE('',*,*,#46401,.T.);
#63039=ORIENTED_EDGE('',*,*,#46096,.F.);
#63040=ORIENTED_EDGE('',*,*,#46401,.F.);
#63041=ORIENTED_EDGE('',*,*,#46077,.F.);
#63042=ORIENTED_EDGE('',*,*,#46402,.F.);
#63043=ORIENTED_EDGE('',*,*,#46094,.F.);
#63044=ORIENTED_EDGE('',*,*,#46402,.T.);
#63045=ORIENTED_EDGE('',*,*,#46079,.F.);
#63046=ORIENTED_EDGE('',*,*,#46086,.T.);
#63047=ORIENTED_EDGE('',*,*,#46092,.F.);
#63048=ORIENTED_EDGE('',*,*,#46284,.F.);
#63049=ORIENTED_EDGE('',*,*,#46398,.F.);
#63050=ORIENTED_EDGE('',*,*,#46102,.F.);
#63051=ORIENTED_EDGE('',*,*,#46107,.F.);
#63052=ORIENTED_EDGE('',*,*,#46403,.F.);
#63053=ORIENTED_EDGE('',*,*,#46117,.F.);
#63054=ORIENTED_EDGE('',*,*,#46282,.F.);
#63055=ORIENTED_EDGE('',*,*,#46404,.T.);
#63056=ORIENTED_EDGE('',*,*,#46140,.F.);
#63057=ORIENTED_EDGE('',*,*,#46403,.T.);
#63058=ORIENTED_EDGE('',*,*,#46110,.F.);
#63059=ORIENTED_EDGE('',*,*,#46115,.F.);
#63060=ORIENTED_EDGE('',*,*,#46139,.F.);
#63061=ORIENTED_EDGE('',*,*,#46404,.F.);
#63062=ORIENTED_EDGE('',*,*,#46112,.F.);
#63063=ORIENTED_EDGE('',*,*,#46405,.T.);
#63064=ORIENTED_EDGE('',*,*,#46265,.F.);
#63065=ORIENTED_EDGE('',*,*,#46141,.T.);
#63066=ORIENTED_EDGE('',*,*,#46160,.F.);
#63067=ORIENTED_EDGE('',*,*,#46406,.F.);
#63068=ORIENTED_EDGE('',*,*,#46263,.F.);
#63069=ORIENTED_EDGE('',*,*,#46405,.F.);
#63070=ORIENTED_EDGE('',*,*,#46162,.F.);
#63071=ORIENTED_EDGE('',*,*,#46407,.T.);
#63072=ORIENTED_EDGE('',*,*,#46261,.F.);
#63073=ORIENTED_EDGE('',*,*,#46406,.T.);
#63074=ORIENTED_EDGE('',*,*,#46164,.F.);
#63075=ORIENTED_EDGE('',*,*,#46408,.F.);
#63076=ORIENTED_EDGE('',*,*,#46259,.F.);
#63077=ORIENTED_EDGE('',*,*,#46407,.F.);
#63078=ORIENTED_EDGE('',*,*,#46166,.F.);
#63079=ORIENTED_EDGE('',*,*,#46322,.F.);
#63080=ORIENTED_EDGE('',*,*,#46329,.F.);
#63081=ORIENTED_EDGE('',*,*,#46409,.T.);
#63082=ORIENTED_EDGE('',*,*,#46257,.F.);
#63083=ORIENTED_EDGE('',*,*,#46408,.T.);
#63084=ORIENTED_EDGE('',*,*,#46167,.F.);
#63085=ORIENTED_EDGE('',*,*,#46173,.F.);
#63086=ORIENTED_EDGE('',*,*,#46410,.F.);
#63087=ORIENTED_EDGE('',*,*,#46187,.F.);
#63088=ORIENTED_EDGE('',*,*,#46326,.F.);
#63089=ORIENTED_EDGE('',*,*,#46411,.T.);
#63090=ORIENTED_EDGE('',*,*,#46213,.F.);
#63091=ORIENTED_EDGE('',*,*,#46410,.T.);
#63092=ORIENTED_EDGE('',*,*,#46176,.F.);
#63093=ORIENTED_EDGE('',*,*,#46185,.F.);
#63094=ORIENTED_EDGE('',*,*,#46212,.F.);
#63095=ORIENTED_EDGE('',*,*,#46411,.F.);
#63096=ORIENTED_EDGE('',*,*,#46178,.F.);
#63097=ORIENTED_EDGE('',*,*,#46323,.F.);
#63098=ORIENTED_EDGE('',*,*,#46196,.F.);
#63099=ORIENTED_EDGE('',*,*,#46412,.F.);
#63100=ORIENTED_EDGE('',*,*,#46231,.F.);
#63101=ORIENTED_EDGE('',*,*,#46412,.T.);
#63102=ORIENTED_EDGE('',*,*,#46198,.F.);
#63103=ORIENTED_EDGE('',*,*,#46413,.T.);
#63104=ORIENTED_EDGE('',*,*,#46229,.F.);
#63105=ORIENTED_EDGE('',*,*,#46413,.F.);
#63106=ORIENTED_EDGE('',*,*,#46200,.F.);
#63107=ORIENTED_EDGE('',*,*,#46414,.F.);
#63108=ORIENTED_EDGE('',*,*,#46227,.F.);
#63109=ORIENTED_EDGE('',*,*,#46414,.T.);
#63110=ORIENTED_EDGE('',*,*,#46202,.F.);
#63111=ORIENTED_EDGE('',*,*,#46415,.T.);
#63112=ORIENTED_EDGE('',*,*,#46225,.F.);
#63113=ORIENTED_EDGE('',*,*,#46415,.F.);
#63114=ORIENTED_EDGE('',*,*,#46204,.F.);
#63115=ORIENTED_EDGE('',*,*,#46416,.F.);
#63116=ORIENTED_EDGE('',*,*,#46223,.F.);
#63117=ORIENTED_EDGE('',*,*,#46416,.T.);
#63118=ORIENTED_EDGE('',*,*,#46206,.F.);
#63119=ORIENTED_EDGE('',*,*,#46417,.T.);
#63120=ORIENTED_EDGE('',*,*,#46221,.F.);
#63121=ORIENTED_EDGE('',*,*,#46417,.F.);
#63122=ORIENTED_EDGE('',*,*,#46208,.F.);
#63123=ORIENTED_EDGE('',*,*,#46214,.F.);
#63124=ORIENTED_EDGE('',*,*,#46219,.F.);
#63125=ORIENTED_EDGE('',*,*,#46236,.F.);
#63126=ORIENTED_EDGE('',*,*,#46418,.F.);
#63127=ORIENTED_EDGE('',*,*,#46246,.F.);
#63128=ORIENTED_EDGE('',*,*,#46333,.F.);
#63129=ORIENTED_EDGE('',*,*,#46419,.T.);
#63130=ORIENTED_EDGE('',*,*,#46268,.F.);
#63131=ORIENTED_EDGE('',*,*,#46418,.T.);
#63132=ORIENTED_EDGE('',*,*,#46239,.F.);
#63133=ORIENTED_EDGE('',*,*,#46244,.F.);
#63134=ORIENTED_EDGE('',*,*,#46267,.F.);
#63135=ORIENTED_EDGE('',*,*,#46419,.F.);
#63136=ORIENTED_EDGE('',*,*,#46241,.F.);
#63137=ORIENTED_EDGE('',*,*,#46409,.F.);
#63138=ORIENTED_EDGE('',*,*,#46330,.F.);
#63139=ORIENTED_EDGE('',*,*,#46255,.F.);
#63140=ORIENTED_EDGE('',*,*,#46420,.T.);
#63141=ORIENTED_EDGE('',*,*,#46421,.T.);
#63142=ORIENTED_EDGE('',*,*,#46422,.T.);
#63143=ORIENTED_EDGE('',*,*,#46423,.T.);
#63144=ORIENTED_EDGE('',*,*,#46424,.T.);
#63145=ORIENTED_EDGE('',*,*,#46425,.T.);
#63146=ORIENTED_EDGE('',*,*,#46426,.T.);
#63147=ORIENTED_EDGE('',*,*,#46425,.F.);
#63148=ORIENTED_EDGE('',*,*,#46427,.T.);
#63149=ORIENTED_EDGE('',*,*,#46428,.F.);
#63150=ORIENTED_EDGE('',*,*,#46429,.T.);
#63151=ORIENTED_EDGE('',*,*,#46430,.T.);
#63152=ORIENTED_EDGE('',*,*,#46431,.T.);
#63153=ORIENTED_EDGE('',*,*,#46432,.T.);
#63154=ORIENTED_EDGE('',*,*,#46428,.T.);
#63155=ORIENTED_EDGE('',*,*,#46433,.T.);
#63156=ORIENTED_EDGE('',*,*,#46434,.T.);
#63157=ORIENTED_EDGE('',*,*,#46435,.T.);
#63158=ORIENTED_EDGE('',*,*,#46436,.T.);
#63159=ORIENTED_EDGE('',*,*,#46437,.F.);
#63160=ORIENTED_EDGE('',*,*,#46438,.T.);
#63161=ORIENTED_EDGE('',*,*,#46433,.F.);
#63162=ORIENTED_EDGE('',*,*,#46439,.T.);
#63163=ORIENTED_EDGE('',*,*,#46440,.T.);
#63164=ORIENTED_EDGE('',*,*,#46441,.T.);
#63165=ORIENTED_EDGE('',*,*,#46437,.T.);
#63166=ORIENTED_EDGE('',*,*,#46442,.T.);
#63167=ORIENTED_EDGE('',*,*,#46443,.F.);
#63168=ORIENTED_EDGE('',*,*,#46444,.T.);
#63169=ORIENTED_EDGE('',*,*,#46440,.F.);
#63170=ORIENTED_EDGE('',*,*,#46445,.T.);
#63171=ORIENTED_EDGE('',*,*,#46446,.T.);
#63172=ORIENTED_EDGE('',*,*,#46447,.T.);
#63173=ORIENTED_EDGE('',*,*,#46443,.T.);
#63174=ORIENTED_EDGE('',*,*,#46448,.T.);
#63175=ORIENTED_EDGE('',*,*,#46449,.F.);
#63176=ORIENTED_EDGE('',*,*,#46450,.T.);
#63177=ORIENTED_EDGE('',*,*,#46446,.F.);
#63178=ORIENTED_EDGE('',*,*,#46451,.T.);
#63179=ORIENTED_EDGE('',*,*,#46452,.T.);
#63180=ORIENTED_EDGE('',*,*,#46453,.T.);
#63181=ORIENTED_EDGE('',*,*,#46449,.T.);
#63182=ORIENTED_EDGE('',*,*,#46454,.T.);
#63183=ORIENTED_EDGE('',*,*,#46455,.T.);
#63184=ORIENTED_EDGE('',*,*,#46456,.T.);
#63185=ORIENTED_EDGE('',*,*,#46457,.T.);
#63186=ORIENTED_EDGE('',*,*,#46458,.T.);
#63187=ORIENTED_EDGE('',*,*,#46457,.F.);
#63188=ORIENTED_EDGE('',*,*,#46459,.T.);
#63189=ORIENTED_EDGE('',*,*,#46460,.F.);
#63190=ORIENTED_EDGE('',*,*,#46461,.T.);
#63191=ORIENTED_EDGE('',*,*,#46462,.T.);
#63192=ORIENTED_EDGE('',*,*,#46463,.T.);
#63193=ORIENTED_EDGE('',*,*,#46464,.T.);
#63194=ORIENTED_EDGE('',*,*,#46460,.T.);
#63195=ORIENTED_EDGE('',*,*,#46465,.T.);
#63196=ORIENTED_EDGE('',*,*,#46466,.T.);
#63197=ORIENTED_EDGE('',*,*,#46467,.F.);
#63198=ORIENTED_EDGE('',*,*,#46468,.T.);
#63199=ORIENTED_EDGE('',*,*,#46420,.F.);
#63200=ORIENTED_EDGE('',*,*,#46469,.T.);
#63201=ORIENTED_EDGE('',*,*,#46467,.T.);
#63202=ORIENTED_EDGE('',*,*,#46470,.T.);
#63203=ORIENTED_EDGE('',*,*,#46471,.T.);
#63204=ORIENTED_EDGE('',*,*,#46472,.T.);
#63205=ORIENTED_EDGE('',*,*,#46471,.F.);
#63206=ORIENTED_EDGE('',*,*,#46473,.T.);
#63207=ORIENTED_EDGE('',*,*,#46474,.F.);
#63208=ORIENTED_EDGE('',*,*,#46475,.T.);
#63209=ORIENTED_EDGE('',*,*,#46474,.T.);
#63210=ORIENTED_EDGE('',*,*,#46476,.T.);
#63211=ORIENTED_EDGE('',*,*,#46477,.T.);
#63212=ORIENTED_EDGE('',*,*,#46478,.T.);
#63213=ORIENTED_EDGE('',*,*,#46477,.F.);
#63214=ORIENTED_EDGE('',*,*,#46479,.T.);
#63215=ORIENTED_EDGE('',*,*,#46480,.F.);
#63216=ORIENTED_EDGE('',*,*,#46481,.T.);
#63217=ORIENTED_EDGE('',*,*,#46482,.T.);
#63218=ORIENTED_EDGE('',*,*,#46483,.T.);
#63219=ORIENTED_EDGE('',*,*,#46484,.T.);
#63220=ORIENTED_EDGE('',*,*,#46485,.T.);
#63221=ORIENTED_EDGE('',*,*,#46484,.F.);
#63222=ORIENTED_EDGE('',*,*,#46486,.T.);
#63223=ORIENTED_EDGE('',*,*,#46487,.F.);
#63224=ORIENTED_EDGE('',*,*,#46488,.T.);
#63225=ORIENTED_EDGE('',*,*,#46489,.T.);
#63226=ORIENTED_EDGE('',*,*,#46490,.T.);
#63227=ORIENTED_EDGE('',*,*,#46491,.T.);
#63228=ORIENTED_EDGE('',*,*,#46487,.T.);
#63229=ORIENTED_EDGE('',*,*,#46492,.T.);
#63230=ORIENTED_EDGE('',*,*,#46493,.T.);
#63231=ORIENTED_EDGE('',*,*,#46494,.T.);
#63232=ORIENTED_EDGE('',*,*,#46495,.F.);
#63233=ORIENTED_EDGE('',*,*,#46496,.T.);
#63234=ORIENTED_EDGE('',*,*,#46497,.F.);
#63235=ORIENTED_EDGE('',*,*,#46498,.T.);
#63236=ORIENTED_EDGE('',*,*,#46499,.T.);
#63237=ORIENTED_EDGE('',*,*,#46500,.T.);
#63238=ORIENTED_EDGE('',*,*,#46495,.T.);
#63239=ORIENTED_EDGE('',*,*,#46501,.T.);
#63240=ORIENTED_EDGE('',*,*,#46502,.F.);
#63241=ORIENTED_EDGE('',*,*,#46503,.T.);
#63242=ORIENTED_EDGE('',*,*,#46499,.F.);
#63243=ORIENTED_EDGE('',*,*,#46504,.T.);
#63244=ORIENTED_EDGE('',*,*,#46505,.T.);
#63245=ORIENTED_EDGE('',*,*,#46506,.T.);
#63246=ORIENTED_EDGE('',*,*,#46502,.T.);
#63247=ORIENTED_EDGE('',*,*,#46507,.T.);
#63248=ORIENTED_EDGE('',*,*,#46494,.F.);
#63249=ORIENTED_EDGE('',*,*,#46508,.T.);
#63250=ORIENTED_EDGE('',*,*,#46505,.F.);
#63251=ORIENTED_EDGE('',*,*,#46509,.T.);
#63252=ORIENTED_EDGE('',*,*,#46510,.T.);
#63253=ORIENTED_EDGE('',*,*,#46511,.T.);
#63254=ORIENTED_EDGE('',*,*,#46512,.T.);
#63255=ORIENTED_EDGE('',*,*,#46513,.T.);
#63256=ORIENTED_EDGE('',*,*,#46514,.T.);
#63257=ORIENTED_EDGE('',*,*,#46515,.T.);
#63258=ORIENTED_EDGE('',*,*,#46514,.F.);
#63259=ORIENTED_EDGE('',*,*,#46516,.T.);
#63260=ORIENTED_EDGE('',*,*,#46517,.F.);
#63261=ORIENTED_EDGE('',*,*,#46518,.T.);
#63262=ORIENTED_EDGE('',*,*,#46517,.T.);
#63263=ORIENTED_EDGE('',*,*,#46519,.T.);
#63264=ORIENTED_EDGE('',*,*,#46520,.T.);
#63265=ORIENTED_EDGE('',*,*,#46521,.T.);
#63266=ORIENTED_EDGE('',*,*,#46520,.F.);
#63267=ORIENTED_EDGE('',*,*,#46522,.T.);
#63268=ORIENTED_EDGE('',*,*,#46523,.F.);
#63269=ORIENTED_EDGE('',*,*,#46524,.T.);
#63270=ORIENTED_EDGE('',*,*,#46523,.T.);
#63271=ORIENTED_EDGE('',*,*,#46525,.T.);
#63272=ORIENTED_EDGE('',*,*,#46526,.T.);
#63273=ORIENTED_EDGE('',*,*,#46527,.T.);
#63274=ORIENTED_EDGE('',*,*,#46526,.F.);
#63275=ORIENTED_EDGE('',*,*,#46528,.T.);
#63276=ORIENTED_EDGE('',*,*,#46529,.F.);
#63277=ORIENTED_EDGE('',*,*,#46530,.T.);
#63278=ORIENTED_EDGE('',*,*,#46531,.T.);
#63279=ORIENTED_EDGE('',*,*,#46532,.T.);
#63280=ORIENTED_EDGE('',*,*,#46533,.T.);
#63281=ORIENTED_EDGE('',*,*,#46534,.T.);
#63282=ORIENTED_EDGE('',*,*,#46535,.F.);
#63283=ORIENTED_EDGE('',*,*,#46536,.T.);
#63284=ORIENTED_EDGE('',*,*,#46531,.F.);
#63285=ORIENTED_EDGE('',*,*,#46537,.T.);
#63286=ORIENTED_EDGE('',*,*,#46538,.T.);
#63287=ORIENTED_EDGE('',*,*,#46539,.T.);
#63288=ORIENTED_EDGE('',*,*,#46540,.T.);
#63289=ORIENTED_EDGE('',*,*,#46535,.T.);
#63290=ORIENTED_EDGE('',*,*,#46529,.T.);
#63291=ORIENTED_EDGE('',*,*,#46541,.T.);
#63292=ORIENTED_EDGE('',*,*,#46542,.T.);
#63293=ORIENTED_EDGE('',*,*,#46543,.T.);
#63294=ORIENTED_EDGE('',*,*,#46544,.T.);
#63295=ORIENTED_EDGE('',*,*,#46545,.T.);
#63296=ORIENTED_EDGE('',*,*,#46546,.T.);
#63297=ORIENTED_EDGE('',*,*,#46547,.T.);
#63298=ORIENTED_EDGE('',*,*,#46548,.T.);
#63299=ORIENTED_EDGE('',*,*,#46549,.T.);
#63300=ORIENTED_EDGE('',*,*,#46550,.T.);
#63301=ORIENTED_EDGE('',*,*,#46551,.T.);
#63302=ORIENTED_EDGE('',*,*,#46552,.T.);
#63303=ORIENTED_EDGE('',*,*,#46553,.T.);
#63304=ORIENTED_EDGE('',*,*,#46554,.T.);
#63305=ORIENTED_EDGE('',*,*,#46553,.F.);
#63306=ORIENTED_EDGE('',*,*,#46555,.T.);
#63307=ORIENTED_EDGE('',*,*,#46556,.F.);
#63308=ORIENTED_EDGE('',*,*,#46557,.T.);
#63309=ORIENTED_EDGE('',*,*,#46558,.T.);
#63310=ORIENTED_EDGE('',*,*,#46559,.T.);
#63311=ORIENTED_EDGE('',*,*,#46560,.T.);
#63312=ORIENTED_EDGE('',*,*,#46556,.T.);
#63313=ORIENTED_EDGE('',*,*,#46561,.T.);
#63314=ORIENTED_EDGE('',*,*,#46562,.T.);
#63315=ORIENTED_EDGE('',*,*,#46563,.T.);
#63316=ORIENTED_EDGE('',*,*,#46564,.F.);
#63317=ORIENTED_EDGE('',*,*,#46565,.T.);
#63318=ORIENTED_EDGE('',*,*,#46566,.F.);
#63319=ORIENTED_EDGE('',*,*,#46567,.T.);
#63320=ORIENTED_EDGE('',*,*,#46568,.T.);
#63321=ORIENTED_EDGE('',*,*,#46569,.T.);
#63322=ORIENTED_EDGE('',*,*,#46564,.T.);
#63323=ORIENTED_EDGE('',*,*,#46570,.T.);
#63324=ORIENTED_EDGE('',*,*,#46571,.F.);
#63325=ORIENTED_EDGE('',*,*,#46572,.T.);
#63326=ORIENTED_EDGE('',*,*,#46568,.F.);
#63327=ORIENTED_EDGE('',*,*,#46573,.T.);
#63328=ORIENTED_EDGE('',*,*,#46574,.T.);
#63329=ORIENTED_EDGE('',*,*,#46575,.T.);
#63330=ORIENTED_EDGE('',*,*,#46571,.T.);
#63331=ORIENTED_EDGE('',*,*,#46576,.T.);
#63332=ORIENTED_EDGE('',*,*,#46577,.T.);
#63333=ORIENTED_EDGE('',*,*,#46578,.F.);
#63334=ORIENTED_EDGE('',*,*,#46579,.F.);
#63335=ORIENTED_EDGE('',*,*,#46580,.F.);
#63336=ORIENTED_EDGE('',*,*,#46581,.T.);
#63337=ORIENTED_EDGE('',*,*,#46582,.T.);
#63338=ORIENTED_EDGE('',*,*,#46583,.T.);
#63339=ORIENTED_EDGE('',*,*,#46584,.T.);
#63340=ORIENTED_EDGE('',*,*,#46583,.F.);
#63341=ORIENTED_EDGE('',*,*,#46585,.T.);
#63342=ORIENTED_EDGE('',*,*,#46586,.F.);
#63343=ORIENTED_EDGE('',*,*,#46550,.F.);
#63344=ORIENTED_EDGE('',*,*,#46587,.T.);
#63345=ORIENTED_EDGE('',*,*,#46586,.T.);
#63346=ORIENTED_EDGE('',*,*,#46588,.T.);
#63347=ORIENTED_EDGE('',*,*,#46589,.F.);
#63348=ORIENTED_EDGE('',*,*,#46589,.T.);
#63349=ORIENTED_EDGE('',*,*,#46590,.T.);
#63350=ORIENTED_EDGE('',*,*,#46591,.F.);
#63351=ORIENTED_EDGE('',*,*,#46592,.T.);
#63352=ORIENTED_EDGE('',*,*,#46548,.F.);
#63353=ORIENTED_EDGE('',*,*,#46591,.T.);
#63354=ORIENTED_EDGE('',*,*,#46593,.T.);
#63355=ORIENTED_EDGE('',*,*,#46594,.T.);
#63356=ORIENTED_EDGE('',*,*,#46595,.T.);
#63357=ORIENTED_EDGE('',*,*,#46596,.T.);
#63358=ORIENTED_EDGE('',*,*,#46597,.T.);
#63359=ORIENTED_EDGE('',*,*,#46598,.T.);
#63360=ORIENTED_EDGE('',*,*,#46599,.T.);
#63361=ORIENTED_EDGE('',*,*,#46600,.F.);
#63362=ORIENTED_EDGE('',*,*,#46601,.T.);
#63363=ORIENTED_EDGE('',*,*,#46596,.F.);
#63364=ORIENTED_EDGE('',*,*,#46602,.T.);
#63365=ORIENTED_EDGE('',*,*,#46603,.T.);
#63366=ORIENTED_EDGE('',*,*,#46604,.T.);
#63367=ORIENTED_EDGE('',*,*,#46605,.T.);
#63368=ORIENTED_EDGE('',*,*,#46600,.T.);
#63369=ORIENTED_EDGE('',*,*,#46606,.T.);
#63370=ORIENTED_EDGE('',*,*,#46607,.T.);
#63371=ORIENTED_EDGE('',*,*,#46608,.T.);
#63372=ORIENTED_EDGE('',*,*,#46594,.F.);
#63373=ORIENTED_EDGE('',*,*,#46609,.T.);
#63374=ORIENTED_EDGE('',*,*,#46610,.T.);
#63375=ORIENTED_EDGE('',*,*,#46608,.F.);
#63376=ORIENTED_EDGE('',*,*,#46611,.T.);
#63377=ORIENTED_EDGE('',*,*,#46612,.F.);
#63378=ORIENTED_EDGE('',*,*,#46613,.T.);
#63379=ORIENTED_EDGE('',*,*,#46614,.F.);
#63380=ORIENTED_EDGE('',*,*,#46615,.T.);
#63381=ORIENTED_EDGE('',*,*,#46616,.T.);
#63382=ORIENTED_EDGE('',*,*,#46617,.T.);
#63383=ORIENTED_EDGE('',*,*,#46618,.T.);
#63384=ORIENTED_EDGE('',*,*,#46614,.T.);
#63385=ORIENTED_EDGE('',*,*,#46619,.T.);
#63386=ORIENTED_EDGE('',*,*,#46620,.T.);
#63387=ORIENTED_EDGE('',*,*,#46621,.T.);
#63388=ORIENTED_EDGE('',*,*,#46622,.T.);
#63389=ORIENTED_EDGE('',*,*,#46623,.F.);
#63390=ORIENTED_EDGE('',*,*,#46624,.T.);
#63391=ORIENTED_EDGE('',*,*,#46619,.F.);
#63392=ORIENTED_EDGE('',*,*,#46625,.T.);
#63393=ORIENTED_EDGE('',*,*,#46626,.T.);
#63394=ORIENTED_EDGE('',*,*,#46627,.T.);
#63395=ORIENTED_EDGE('',*,*,#46623,.T.);
#63396=ORIENTED_EDGE('',*,*,#46628,.T.);
#63397=ORIENTED_EDGE('',*,*,#46629,.T.);
#63398=ORIENTED_EDGE('',*,*,#46630,.T.);
#63399=ORIENTED_EDGE('',*,*,#46631,.T.);
#63400=ORIENTED_EDGE('',*,*,#46632,.T.);
#63401=ORIENTED_EDGE('',*,*,#46633,.T.);
#63402=ORIENTED_EDGE('',*,*,#46634,.T.);
#63403=ORIENTED_EDGE('',*,*,#46635,.T.);
#63404=ORIENTED_EDGE('',*,*,#46636,.T.);
#63405=ORIENTED_EDGE('',*,*,#46635,.F.);
#63406=ORIENTED_EDGE('',*,*,#46637,.T.);
#63407=ORIENTED_EDGE('',*,*,#46632,.F.);
#63408=ORIENTED_EDGE('',*,*,#46638,.T.);
#63409=ORIENTED_EDGE('',*,*,#46639,.T.);
#63410=ORIENTED_EDGE('',*,*,#46640,.T.);
#63411=ORIENTED_EDGE('',*,*,#46629,.F.);
#63412=ORIENTED_EDGE('',*,*,#46641,.T.);
#63413=ORIENTED_EDGE('',*,*,#46642,.T.);
#63414=ORIENTED_EDGE('',*,*,#46643,.T.);
#63415=ORIENTED_EDGE('',*,*,#46644,.T.);
#63416=ORIENTED_EDGE('',*,*,#46645,.F.);
#63417=ORIENTED_EDGE('',*,*,#46646,.T.);
#63418=ORIENTED_EDGE('',*,*,#46643,.F.);
#63419=ORIENTED_EDGE('',*,*,#46647,.T.);
#63420=ORIENTED_EDGE('',*,*,#46648,.T.);
#63421=ORIENTED_EDGE('',*,*,#46649,.T.);
#63422=ORIENTED_EDGE('',*,*,#46645,.T.);
#63423=ORIENTED_EDGE('',*,*,#46650,.T.);
#63424=ORIENTED_EDGE('',*,*,#46651,.T.);
#63425=ORIENTED_EDGE('',*,*,#46652,.T.);
#63426=ORIENTED_EDGE('',*,*,#46653,.T.);
#63427=ORIENTED_EDGE('',*,*,#46654,.F.);
#63428=ORIENTED_EDGE('',*,*,#46655,.T.);
#63429=ORIENTED_EDGE('',*,*,#46656,.T.);
#63430=ORIENTED_EDGE('',*,*,#46657,.T.);
#63431=ORIENTED_EDGE('',*,*,#46658,.T.);
#63432=ORIENTED_EDGE('',*,*,#46659,.F.);
#63433=ORIENTED_EDGE('',*,*,#46660,.T.);
#63434=ORIENTED_EDGE('',*,*,#46655,.F.);
#63435=ORIENTED_EDGE('',*,*,#46661,.T.);
#63436=ORIENTED_EDGE('',*,*,#46662,.T.);
#63437=ORIENTED_EDGE('',*,*,#46663,.T.);
#63438=ORIENTED_EDGE('',*,*,#46659,.T.);
#63439=ORIENTED_EDGE('',*,*,#46664,.T.);
#63440=ORIENTED_EDGE('',*,*,#46665,.T.);
#63441=ORIENTED_EDGE('',*,*,#46666,.T.);
#63442=ORIENTED_EDGE('',*,*,#46667,.T.);
#63443=ORIENTED_EDGE('',*,*,#46668,.F.);
#63444=ORIENTED_EDGE('',*,*,#46669,.T.);
#63445=ORIENTED_EDGE('',*,*,#46670,.T.);
#63446=ORIENTED_EDGE('',*,*,#46671,.T.);
#63447=ORIENTED_EDGE('',*,*,#46672,.T.);
#63448=ORIENTED_EDGE('',*,*,#46673,.F.);
#63449=ORIENTED_EDGE('',*,*,#46674,.T.);
#63450=ORIENTED_EDGE('',*,*,#46669,.F.);
#63451=ORIENTED_EDGE('',*,*,#46675,.T.);
#63452=ORIENTED_EDGE('',*,*,#46676,.T.);
#63453=ORIENTED_EDGE('',*,*,#46677,.T.);
#63454=ORIENTED_EDGE('',*,*,#46673,.T.);
#63455=ORIENTED_EDGE('',*,*,#46678,.T.);
#63456=ORIENTED_EDGE('',*,*,#46679,.T.);
#63457=ORIENTED_EDGE('',*,*,#46680,.T.);
#63458=ORIENTED_EDGE('',*,*,#46681,.T.);
#63459=ORIENTED_EDGE('',*,*,#46682,.F.);
#63460=ORIENTED_EDGE('',*,*,#46683,.T.);
#63461=ORIENTED_EDGE('',*,*,#46684,.T.);
#63462=ORIENTED_EDGE('',*,*,#46685,.T.);
#63463=ORIENTED_EDGE('',*,*,#46686,.T.);
#63464=ORIENTED_EDGE('',*,*,#46687,.F.);
#63465=ORIENTED_EDGE('',*,*,#46688,.T.);
#63466=ORIENTED_EDGE('',*,*,#46683,.F.);
#63467=ORIENTED_EDGE('',*,*,#46689,.T.);
#63468=ORIENTED_EDGE('',*,*,#46690,.T.);
#63469=ORIENTED_EDGE('',*,*,#46691,.T.);
#63470=ORIENTED_EDGE('',*,*,#46687,.T.);
#63471=ORIENTED_EDGE('',*,*,#46692,.T.);
#63472=ORIENTED_EDGE('',*,*,#46693,.F.);
#63473=ORIENTED_EDGE('',*,*,#46694,.T.);
#63474=ORIENTED_EDGE('',*,*,#46695,.F.);
#63475=ORIENTED_EDGE('',*,*,#46696,.T.);
#63476=ORIENTED_EDGE('',*,*,#46697,.T.);
#63477=ORIENTED_EDGE('',*,*,#46698,.T.);
#63478=ORIENTED_EDGE('',*,*,#46699,.T.);
#63479=ORIENTED_EDGE('',*,*,#46698,.F.);
#63480=ORIENTED_EDGE('',*,*,#46700,.T.);
#63481=ORIENTED_EDGE('',*,*,#46701,.F.);
#63482=ORIENTED_EDGE('',*,*,#46702,.T.);
#63483=ORIENTED_EDGE('',*,*,#46703,.T.);
#63484=ORIENTED_EDGE('',*,*,#46704,.T.);
#63485=ORIENTED_EDGE('',*,*,#46693,.T.);
#63486=ORIENTED_EDGE('',*,*,#46701,.T.);
#63487=ORIENTED_EDGE('',*,*,#46705,.F.);
#63488=ORIENTED_EDGE('',*,*,#46706,.T.);
#63489=ORIENTED_EDGE('',*,*,#46707,.F.);
#63490=ORIENTED_EDGE('',*,*,#46708,.T.);
#63491=ORIENTED_EDGE('',*,*,#46709,.T.);
#63492=ORIENTED_EDGE('',*,*,#46710,.T.);
#63493=ORIENTED_EDGE('',*,*,#46711,.T.);
#63494=ORIENTED_EDGE('',*,*,#46712,.T.);
#63495=ORIENTED_EDGE('',*,*,#46713,.F.);
#63496=ORIENTED_EDGE('',*,*,#46714,.T.);
#63497=ORIENTED_EDGE('',*,*,#46711,.F.);
#63498=ORIENTED_EDGE('',*,*,#46715,.T.);
#63499=ORIENTED_EDGE('',*,*,#46716,.T.);
#63500=ORIENTED_EDGE('',*,*,#46717,.T.);
#63501=ORIENTED_EDGE('',*,*,#46713,.T.);
#63502=ORIENTED_EDGE('',*,*,#46718,.T.);
#63503=ORIENTED_EDGE('',*,*,#46719,.T.);
#63504=ORIENTED_EDGE('',*,*,#46720,.T.);
#63505=ORIENTED_EDGE('',*,*,#46721,.T.);
#63506=ORIENTED_EDGE('',*,*,#46707,.T.);
#63507=ORIENTED_EDGE('',*,*,#46722,.T.);
#63508=ORIENTED_EDGE('',*,*,#46723,.T.);
#63509=ORIENTED_EDGE('',*,*,#46705,.T.);
#63510=ORIENTED_EDGE('',*,*,#46724,.T.);
#63511=ORIENTED_EDGE('',*,*,#46725,.T.);
#63512=ORIENTED_EDGE('',*,*,#46726,.T.);
#63513=ORIENTED_EDGE('',*,*,#46612,.T.);
#63514=ORIENTED_EDGE('',*,*,#46727,.T.);
#63515=ORIENTED_EDGE('',*,*,#46728,.T.);
#63516=ORIENTED_EDGE('',*,*,#46729,.T.);
#63517=ORIENTED_EDGE('',*,*,#46730,.T.);
#63518=ORIENTED_EDGE('',*,*,#46731,.T.);
#63519=ORIENTED_EDGE('',*,*,#46732,.T.);
#63520=ORIENTED_EDGE('',*,*,#46733,.T.);
#63521=ORIENTED_EDGE('',*,*,#46734,.T.);
#63522=ORIENTED_EDGE('',*,*,#46735,.T.);
#63523=ORIENTED_EDGE('',*,*,#46736,.T.);
#63524=ORIENTED_EDGE('',*,*,#46737,.T.);
#63525=ORIENTED_EDGE('',*,*,#46738,.T.);
#63526=ORIENTED_EDGE('',*,*,#46739,.T.);
#63527=ORIENTED_EDGE('',*,*,#46740,.T.);
#63528=ORIENTED_EDGE('',*,*,#46741,.T.);
#63529=ORIENTED_EDGE('',*,*,#46742,.T.);
#63530=ORIENTED_EDGE('',*,*,#46743,.T.);
#63531=ORIENTED_EDGE('',*,*,#46744,.F.);
#63532=ORIENTED_EDGE('',*,*,#46745,.T.);
#63533=ORIENTED_EDGE('',*,*,#46746,.F.);
#63534=ORIENTED_EDGE('',*,*,#46747,.T.);
#63535=ORIENTED_EDGE('',*,*,#46563,.F.);
#63536=ORIENTED_EDGE('',*,*,#46748,.T.);
#63537=ORIENTED_EDGE('',*,*,#46574,.F.);
#63538=ORIENTED_EDGE('',*,*,#46749,.T.);
#63539=ORIENTED_EDGE('',*,*,#46750,.T.);
#63540=ORIENTED_EDGE('',*,*,#46751,.T.);
#63541=ORIENTED_EDGE('',*,*,#46752,.F.);
#63542=ORIENTED_EDGE('',*,*,#46753,.T.);
#63543=ORIENTED_EDGE('',*,*,#46740,.F.);
#63544=ORIENTED_EDGE('',*,*,#46754,.T.);
#63545=ORIENTED_EDGE('',*,*,#46755,.F.);
#63546=ORIENTED_EDGE('',*,*,#46756,.T.);
#63547=ORIENTED_EDGE('',*,*,#46736,.F.);
#63548=ORIENTED_EDGE('',*,*,#46757,.T.);
#63549=ORIENTED_EDGE('',*,*,#46734,.F.);
#63550=ORIENTED_EDGE('',*,*,#46758,.T.);
#63551=ORIENTED_EDGE('',*,*,#46759,.F.);
#63552=ORIENTED_EDGE('',*,*,#46760,.T.);
#63553=ORIENTED_EDGE('',*,*,#46761,.F.);
#63554=ORIENTED_EDGE('',*,*,#46762,.T.);
#63555=ORIENTED_EDGE('',*,*,#46728,.F.);
#63556=ORIENTED_EDGE('',*,*,#46763,.T.);
#63557=ORIENTED_EDGE('',*,*,#46764,.T.);
#63558=ORIENTED_EDGE('',*,*,#46765,.F.);
#63559=ORIENTED_EDGE('',*,*,#46766,.F.);
#63560=ORIENTED_EDGE('',*,*,#46767,.F.);
#63561=ORIENTED_EDGE('',*,*,#46768,.T.);
#63562=ORIENTED_EDGE('',*,*,#46751,.F.);
#63563=ORIENTED_EDGE('',*,*,#46769,.F.);
#63564=ORIENTED_EDGE('',*,*,#46770,.F.);
#63565=ORIENTED_EDGE('',*,*,#46771,.F.);
#63566=ORIENTED_EDGE('',*,*,#46772,.T.);
#63567=ORIENTED_EDGE('',*,*,#46561,.F.);
#63568=ORIENTED_EDGE('',*,*,#46768,.F.);
#63569=ORIENTED_EDGE('',*,*,#46773,.F.);
#63570=ORIENTED_EDGE('',*,*,#46774,.F.);
#63571=ORIENTED_EDGE('',*,*,#46775,.F.);
#63572=ORIENTED_EDGE('',*,*,#46776,.F.);
#63573=ORIENTED_EDGE('',*,*,#46773,.T.);
#63574=ORIENTED_EDGE('',*,*,#46777,.F.);
#63575=ORIENTED_EDGE('',*,*,#46778,.F.);
#63576=ORIENTED_EDGE('',*,*,#46559,.F.);
#63577=ORIENTED_EDGE('',*,*,#46778,.T.);
#63578=ORIENTED_EDGE('',*,*,#46779,.F.);
#63579=ORIENTED_EDGE('',*,*,#46780,.F.);
#63580=ORIENTED_EDGE('',*,*,#46781,.F.);
#63581=ORIENTED_EDGE('',*,*,#46782,.F.);
#63582=ORIENTED_EDGE('',*,*,#46783,.T.);
#63583=ORIENTED_EDGE('',*,*,#46581,.F.);
#63584=ORIENTED_EDGE('',*,*,#46784,.T.);
#63585=ORIENTED_EDGE('',*,*,#46785,.T.);
#63586=ORIENTED_EDGE('',*,*,#46786,.F.);
#63587=ORIENTED_EDGE('',*,*,#46787,.F.);
#63588=ORIENTED_EDGE('',*,*,#46788,.F.);
#63589=ORIENTED_EDGE('',*,*,#46787,.T.);
#63590=ORIENTED_EDGE('',*,*,#46789,.F.);
#63591=ORIENTED_EDGE('',*,*,#46790,.F.);
#63592=ORIENTED_EDGE('',*,*,#46604,.F.);
#63593=ORIENTED_EDGE('',*,*,#46790,.T.);
#63594=ORIENTED_EDGE('',*,*,#46791,.F.);
#63595=ORIENTED_EDGE('',*,*,#46792,.F.);
#63596=ORIENTED_EDGE('',*,*,#46793,.F.);
#63597=ORIENTED_EDGE('',*,*,#46794,.F.);
#63598=ORIENTED_EDGE('',*,*,#46795,.T.);
#63599=ORIENTED_EDGE('',*,*,#46796,.F.);
#63600=ORIENTED_EDGE('',*,*,#46797,.F.);
#63601=ORIENTED_EDGE('',*,*,#46797,.T.);
#63602=ORIENTED_EDGE('',*,*,#46798,.F.);
#63603=ORIENTED_EDGE('',*,*,#46799,.F.);
#63604=ORIENTED_EDGE('',*,*,#46800,.F.);
#63605=ORIENTED_EDGE('',*,*,#46799,.T.);
#63606=ORIENTED_EDGE('',*,*,#46801,.F.);
#63607=ORIENTED_EDGE('',*,*,#46802,.F.);
#63608=ORIENTED_EDGE('',*,*,#46803,.F.);
#63609=ORIENTED_EDGE('',*,*,#46802,.T.);
#63610=ORIENTED_EDGE('',*,*,#46804,.F.);
#63611=ORIENTED_EDGE('',*,*,#46805,.F.);
#63612=ORIENTED_EDGE('',*,*,#46806,.F.);
#63613=ORIENTED_EDGE('',*,*,#46807,.F.);
#63614=ORIENTED_EDGE('',*,*,#46808,.F.);
#63615=ORIENTED_EDGE('',*,*,#46809,.F.);
#63616=ORIENTED_EDGE('',*,*,#46810,.F.);
#63617=ORIENTED_EDGE('',*,*,#46807,.T.);
#63618=ORIENTED_EDGE('',*,*,#46811,.F.);
#63619=ORIENTED_EDGE('',*,*,#46812,.F.);
#63620=ORIENTED_EDGE('',*,*,#46431,.F.);
#63621=ORIENTED_EDGE('',*,*,#46812,.T.);
#63622=ORIENTED_EDGE('',*,*,#46813,.F.);
#63623=ORIENTED_EDGE('',*,*,#46814,.F.);
#63624=ORIENTED_EDGE('',*,*,#46815,.F.);
#63625=ORIENTED_EDGE('',*,*,#46422,.F.);
#63626=ORIENTED_EDGE('',*,*,#46816,.T.);
#63627=ORIENTED_EDGE('',*,*,#46817,.F.);
#63628=ORIENTED_EDGE('',*,*,#46818,.F.);
#63629=ORIENTED_EDGE('',*,*,#46818,.T.);
#63630=ORIENTED_EDGE('',*,*,#46819,.F.);
#63631=ORIENTED_EDGE('',*,*,#46820,.F.);
#63632=ORIENTED_EDGE('',*,*,#46469,.F.);
#63633=ORIENTED_EDGE('',*,*,#46821,.F.);
#63634=ORIENTED_EDGE('',*,*,#46822,.T.);
#63635=ORIENTED_EDGE('',*,*,#46823,.F.);
#63636=ORIENTED_EDGE('',*,*,#46805,.T.);
#63637=ORIENTED_EDGE('',*,*,#46824,.T.);
#63638=ORIENTED_EDGE('',*,*,#46825,.F.);
#63639=ORIENTED_EDGE('',*,*,#46826,.F.);
#63640=ORIENTED_EDGE('',*,*,#46827,.F.);
#63641=ORIENTED_EDGE('',*,*,#46826,.T.);
#63642=ORIENTED_EDGE('',*,*,#46828,.F.);
#63643=ORIENTED_EDGE('',*,*,#46829,.F.);
#63644=ORIENTED_EDGE('',*,*,#46463,.F.);
#63645=ORIENTED_EDGE('',*,*,#46829,.T.);
#63646=ORIENTED_EDGE('',*,*,#46830,.F.);
#63647=ORIENTED_EDGE('',*,*,#46831,.F.);
#63648=ORIENTED_EDGE('',*,*,#46832,.F.);
#63649=ORIENTED_EDGE('',*,*,#46833,.F.);
#63650=ORIENTED_EDGE('',*,*,#46834,.T.);
#63651=ORIENTED_EDGE('',*,*,#46452,.F.);
#63652=ORIENTED_EDGE('',*,*,#46835,.T.);
#63653=ORIENTED_EDGE('',*,*,#46836,.F.);
#63654=ORIENTED_EDGE('',*,*,#46837,.T.);
#63655=ORIENTED_EDGE('',*,*,#46465,.F.);
#63656=ORIENTED_EDGE('',*,*,#46820,.T.);
#63657=ORIENTED_EDGE('',*,*,#46838,.T.);
#63658=ORIENTED_EDGE('',*,*,#46839,.F.);
#63659=ORIENTED_EDGE('',*,*,#46840,.F.);
#63660=ORIENTED_EDGE('',*,*,#46841,.F.);
#63661=ORIENTED_EDGE('',*,*,#46840,.T.);
#63662=ORIENTED_EDGE('',*,*,#46842,.F.);
#63663=ORIENTED_EDGE('',*,*,#46843,.F.);
#63664=ORIENTED_EDGE('',*,*,#46844,.F.);
#63665=ORIENTED_EDGE('',*,*,#46843,.T.);
#63666=ORIENTED_EDGE('',*,*,#46845,.F.);
#63667=ORIENTED_EDGE('',*,*,#46846,.F.);
#63668=ORIENTED_EDGE('',*,*,#46720,.F.);
#63669=ORIENTED_EDGE('',*,*,#46847,.T.);
#63670=ORIENTED_EDGE('',*,*,#46848,.F.);
#63671=ORIENTED_EDGE('',*,*,#46846,.T.);
#63672=ORIENTED_EDGE('',*,*,#46849,.F.);
#63673=ORIENTED_EDGE('',*,*,#46850,.F.);
#63674=ORIENTED_EDGE('',*,*,#46851,.T.);
#63675=ORIENTED_EDGE('',*,*,#46716,.F.);
#63676=ORIENTED_EDGE('',*,*,#46852,.T.);
#63677=ORIENTED_EDGE('',*,*,#46853,.T.);
#63678=ORIENTED_EDGE('',*,*,#46854,.F.);
#63679=ORIENTED_EDGE('',*,*,#46855,.F.);
#63680=ORIENTED_EDGE('',*,*,#46856,.F.);
#63681=ORIENTED_EDGE('',*,*,#46857,.T.);
#63682=ORIENTED_EDGE('',*,*,#46704,.F.);
#63683=ORIENTED_EDGE('',*,*,#46853,.F.);
#63684=ORIENTED_EDGE('',*,*,#46858,.F.);
#63685=ORIENTED_EDGE('',*,*,#46859,.T.);
#63686=ORIENTED_EDGE('',*,*,#46694,.F.);
#63687=ORIENTED_EDGE('',*,*,#46857,.F.);
#63688=ORIENTED_EDGE('',*,*,#46860,.F.);
#63689=ORIENTED_EDGE('',*,*,#46861,.T.);
#63690=ORIENTED_EDGE('',*,*,#46862,.F.);
#63691=ORIENTED_EDGE('',*,*,#46859,.F.);
#63692=ORIENTED_EDGE('',*,*,#46863,.F.);
#63693=ORIENTED_EDGE('',*,*,#46864,.F.);
#63694=ORIENTED_EDGE('',*,*,#46865,.T.);
#63695=ORIENTED_EDGE('',*,*,#46690,.F.);
#63696=ORIENTED_EDGE('',*,*,#46866,.T.);
#63697=ORIENTED_EDGE('',*,*,#46867,.F.);
#63698=ORIENTED_EDGE('',*,*,#46868,.F.);
#63699=ORIENTED_EDGE('',*,*,#46869,.F.);
#63700=ORIENTED_EDGE('',*,*,#46870,.F.);
#63701=ORIENTED_EDGE('',*,*,#46867,.T.);
#63702=ORIENTED_EDGE('',*,*,#46871,.F.);
#63703=ORIENTED_EDGE('',*,*,#46872,.F.);
#63704=ORIENTED_EDGE('',*,*,#46680,.F.);
#63705=ORIENTED_EDGE('',*,*,#46872,.T.);
#63706=ORIENTED_EDGE('',*,*,#46873,.F.);
#63707=ORIENTED_EDGE('',*,*,#46874,.F.);
#63708=ORIENTED_EDGE('',*,*,#46875,.F.);
#63709=ORIENTED_EDGE('',*,*,#46876,.F.);
#63710=ORIENTED_EDGE('',*,*,#46877,.T.);
#63711=ORIENTED_EDGE('',*,*,#46676,.F.);
#63712=ORIENTED_EDGE('',*,*,#46878,.T.);
#63713=ORIENTED_EDGE('',*,*,#46879,.F.);
#63714=ORIENTED_EDGE('',*,*,#46880,.F.);
#63715=ORIENTED_EDGE('',*,*,#46881,.F.);
#63716=ORIENTED_EDGE('',*,*,#46882,.F.);
#63717=ORIENTED_EDGE('',*,*,#46879,.T.);
#63718=ORIENTED_EDGE('',*,*,#46883,.F.);
#63719=ORIENTED_EDGE('',*,*,#46884,.F.);
#63720=ORIENTED_EDGE('',*,*,#46666,.F.);
#63721=ORIENTED_EDGE('',*,*,#46884,.T.);
#63722=ORIENTED_EDGE('',*,*,#46885,.F.);
#63723=ORIENTED_EDGE('',*,*,#46886,.F.);
#63724=ORIENTED_EDGE('',*,*,#46887,.F.);
#63725=ORIENTED_EDGE('',*,*,#46888,.F.);
#63726=ORIENTED_EDGE('',*,*,#46889,.T.);
#63727=ORIENTED_EDGE('',*,*,#46662,.F.);
#63728=ORIENTED_EDGE('',*,*,#46890,.T.);
#63729=ORIENTED_EDGE('',*,*,#46891,.F.);
#63730=ORIENTED_EDGE('',*,*,#46892,.F.);
#63731=ORIENTED_EDGE('',*,*,#46893,.F.);
#63732=ORIENTED_EDGE('',*,*,#46894,.F.);
#63733=ORIENTED_EDGE('',*,*,#46891,.T.);
#63734=ORIENTED_EDGE('',*,*,#46895,.F.);
#63735=ORIENTED_EDGE('',*,*,#46896,.F.);
#63736=ORIENTED_EDGE('',*,*,#46652,.F.);
#63737=ORIENTED_EDGE('',*,*,#46896,.T.);
#63738=ORIENTED_EDGE('',*,*,#46897,.F.);
#63739=ORIENTED_EDGE('',*,*,#46898,.F.);
#63740=ORIENTED_EDGE('',*,*,#46899,.F.);
#63741=ORIENTED_EDGE('',*,*,#46900,.F.);
#63742=ORIENTED_EDGE('',*,*,#46901,.T.);
#63743=ORIENTED_EDGE('',*,*,#46648,.F.);
#63744=ORIENTED_EDGE('',*,*,#46902,.T.);
#63745=ORIENTED_EDGE('',*,*,#46903,.T.);
#63746=ORIENTED_EDGE('',*,*,#46904,.F.);
#63747=ORIENTED_EDGE('',*,*,#46905,.F.);
#63748=ORIENTED_EDGE('',*,*,#46906,.F.);
#63749=ORIENTED_EDGE('',*,*,#46907,.T.);
#63750=ORIENTED_EDGE('',*,*,#46640,.F.);
#63751=ORIENTED_EDGE('',*,*,#46903,.F.);
#63752=ORIENTED_EDGE('',*,*,#46908,.F.);
#63753=ORIENTED_EDGE('',*,*,#46909,.T.);
#63754=ORIENTED_EDGE('',*,*,#46630,.F.);
#63755=ORIENTED_EDGE('',*,*,#46907,.F.);
#63756=ORIENTED_EDGE('',*,*,#46910,.F.);
#63757=ORIENTED_EDGE('',*,*,#46911,.T.);
#63758=ORIENTED_EDGE('',*,*,#46912,.F.);
#63759=ORIENTED_EDGE('',*,*,#46909,.F.);
#63760=ORIENTED_EDGE('',*,*,#46913,.F.);
#63761=ORIENTED_EDGE('',*,*,#46914,.F.);
#63762=ORIENTED_EDGE('',*,*,#46915,.T.);
#63763=ORIENTED_EDGE('',*,*,#46626,.F.);
#63764=ORIENTED_EDGE('',*,*,#46916,.T.);
#63765=ORIENTED_EDGE('',*,*,#46917,.T.);
#63766=ORIENTED_EDGE('',*,*,#46918,.F.);
#63767=ORIENTED_EDGE('',*,*,#46919,.F.);
#63768=ORIENTED_EDGE('',*,*,#46920,.F.);
#63769=ORIENTED_EDGE('',*,*,#46919,.T.);
#63770=ORIENTED_EDGE('',*,*,#46921,.F.);
#63771=ORIENTED_EDGE('',*,*,#46922,.F.);
#63772=ORIENTED_EDGE('',*,*,#46617,.F.);
#63773=ORIENTED_EDGE('',*,*,#46922,.T.);
#63774=ORIENTED_EDGE('',*,*,#46923,.F.);
#63775=ORIENTED_EDGE('',*,*,#46924,.F.);
#63776=ORIENTED_EDGE('',*,*,#46925,.F.);
#63777=ORIENTED_EDGE('',*,*,#46510,.F.);
#63778=ORIENTED_EDGE('',*,*,#46926,.T.);
#63779=ORIENTED_EDGE('',*,*,#46927,.F.);
#63780=ORIENTED_EDGE('',*,*,#46928,.T.);
#63781=ORIENTED_EDGE('',*,*,#46929,.T.);
#63782=ORIENTED_EDGE('',*,*,#46930,.F.);
#63783=ORIENTED_EDGE('',*,*,#46924,.T.);
#63784=ORIENTED_EDGE('',*,*,#46931,.F.);
#63785=ORIENTED_EDGE('',*,*,#46932,.T.);
#63786=ORIENTED_EDGE('',*,*,#46511,.F.);
#63787=ORIENTED_EDGE('',*,*,#46928,.F.);
#63788=ORIENTED_EDGE('',*,*,#46933,.F.);
#63789=ORIENTED_EDGE('',*,*,#46934,.F.);
#63790=ORIENTED_EDGE('',*,*,#46935,.T.);
#63791=ORIENTED_EDGE('',*,*,#46492,.F.);
#63792=ORIENTED_EDGE('',*,*,#46932,.F.);
#63793=ORIENTED_EDGE('',*,*,#46936,.F.);
#63794=ORIENTED_EDGE('',*,*,#46937,.F.);
#63795=ORIENTED_EDGE('',*,*,#46938,.F.);
#63796=ORIENTED_EDGE('',*,*,#46939,.F.);
#63797=ORIENTED_EDGE('',*,*,#46936,.T.);
#63798=ORIENTED_EDGE('',*,*,#46940,.F.);
#63799=ORIENTED_EDGE('',*,*,#46941,.F.);
#63800=ORIENTED_EDGE('',*,*,#46490,.F.);
#63801=ORIENTED_EDGE('',*,*,#46941,.T.);
#63802=ORIENTED_EDGE('',*,*,#46942,.F.);
#63803=ORIENTED_EDGE('',*,*,#46943,.F.);
#63804=ORIENTED_EDGE('',*,*,#46944,.F.);
#63805=ORIENTED_EDGE('',*,*,#46945,.F.);
#63806=ORIENTED_EDGE('',*,*,#46946,.T.);
#63807=ORIENTED_EDGE('',*,*,#46512,.F.);
#63808=ORIENTED_EDGE('',*,*,#46947,.T.);
#63809=ORIENTED_EDGE('',*,*,#46948,.T.);
#63810=ORIENTED_EDGE('',*,*,#46949,.F.);
#63811=ORIENTED_EDGE('',*,*,#46950,.F.);
#63812=ORIENTED_EDGE('',*,*,#46951,.F.);
#63813=ORIENTED_EDGE('',*,*,#46950,.T.);
#63814=ORIENTED_EDGE('',*,*,#46952,.F.);
#63815=ORIENTED_EDGE('',*,*,#46953,.F.);
#63816=ORIENTED_EDGE('',*,*,#46539,.F.);
#63817=ORIENTED_EDGE('',*,*,#46953,.T.);
#63818=ORIENTED_EDGE('',*,*,#46954,.F.);
#63819=ORIENTED_EDGE('',*,*,#46955,.F.);
#63820=ORIENTED_EDGE('',*,*,#46956,.F.);
#63821=ORIENTED_EDGE('',*,*,#46957,.F.);
#63822=ORIENTED_EDGE('',*,*,#46958,.T.);
#63823=ORIENTED_EDGE('',*,*,#46959,.F.);
#63824=ORIENTED_EDGE('',*,*,#46960,.F.);
#63825=ORIENTED_EDGE('',*,*,#46960,.T.);
#63826=ORIENTED_EDGE('',*,*,#46961,.F.);
#63827=ORIENTED_EDGE('',*,*,#46962,.F.);
#63828=ORIENTED_EDGE('',*,*,#46963,.F.);
#63829=ORIENTED_EDGE('',*,*,#46962,.T.);
#63830=ORIENTED_EDGE('',*,*,#46964,.F.);
#63831=ORIENTED_EDGE('',*,*,#46965,.F.);
#63832=ORIENTED_EDGE('',*,*,#46966,.F.);
#63833=ORIENTED_EDGE('',*,*,#46965,.T.);
#63834=ORIENTED_EDGE('',*,*,#46967,.F.);
#63835=ORIENTED_EDGE('',*,*,#46968,.F.);
#63836=ORIENTED_EDGE('',*,*,#46969,.F.);
#63837=ORIENTED_EDGE('',*,*,#46970,.F.);
#63838=ORIENTED_EDGE('',*,*,#46971,.T.);
#63839=ORIENTED_EDGE('',*,*,#46972,.F.);
#63840=ORIENTED_EDGE('',*,*,#46968,.T.);
#63841=ORIENTED_EDGE('',*,*,#46973,.F.);
#63842=ORIENTED_EDGE('',*,*,#46974,.F.);
#63843=ORIENTED_EDGE('',*,*,#46975,.F.);
#63844=ORIENTED_EDGE('',*,*,#46976,.F.);
#63845=ORIENTED_EDGE('',*,*,#46977,.T.);
#63846=ORIENTED_EDGE('',*,*,#46544,.F.);
#63847=ORIENTED_EDGE('',*,*,#46978,.T.);
#63848=ORIENTED_EDGE('',*,*,#46979,.F.);
#63849=ORIENTED_EDGE('',*,*,#46980,.T.);
#63850=ORIENTED_EDGE('',*,*,#46981,.F.);
#63851=ORIENTED_EDGE('',*,*,#46982,.T.);
#63852=ORIENTED_EDGE('',*,*,#46983,.T.);
#63853=ORIENTED_EDGE('',*,*,#46984,.T.);
#63854=ORIENTED_EDGE('',*,*,#46744,.T.);
#63855=ORIENTED_EDGE('',*,*,#46985,.T.);
#63856=ORIENTED_EDGE('',*,*,#46986,.T.);
#63857=ORIENTED_EDGE('',*,*,#46987,.T.);
#63858=ORIENTED_EDGE('',*,*,#46988,.T.);
#63859=ORIENTED_EDGE('',*,*,#46989,.T.);
#63860=ORIENTED_EDGE('',*,*,#46990,.F.);
#63861=ORIENTED_EDGE('',*,*,#46991,.T.);
#63862=ORIENTED_EDGE('',*,*,#46580,.T.);
#63863=ORIENTED_EDGE('',*,*,#46992,.T.);
#63864=ORIENTED_EDGE('',*,*,#46993,.T.);
#63865=ORIENTED_EDGE('',*,*,#46994,.F.);
#63866=ORIENTED_EDGE('',*,*,#46995,.F.);
#63867=ORIENTED_EDGE('',*,*,#46429,.F.);
#63868=ORIENTED_EDGE('',*,*,#46995,.T.);
#63869=ORIENTED_EDGE('',*,*,#46996,.F.);
#63870=ORIENTED_EDGE('',*,*,#46997,.F.);
#63871=ORIENTED_EDGE('',*,*,#46426,.F.);
#63872=ORIENTED_EDGE('',*,*,#46998,.T.);
#63873=ORIENTED_EDGE('',*,*,#46999,.F.);
#63874=ORIENTED_EDGE('',*,*,#47000,.F.);
#63875=ORIENTED_EDGE('',*,*,#47001,.F.);
#63876=ORIENTED_EDGE('',*,*,#47002,.T.);
#63877=ORIENTED_EDGE('',*,*,#46481,.F.);
#63878=ORIENTED_EDGE('',*,*,#46998,.F.);
#63879=ORIENTED_EDGE('',*,*,#47003,.F.);
#63880=ORIENTED_EDGE('',*,*,#47004,.T.);
#63881=ORIENTED_EDGE('',*,*,#46478,.F.);
#63882=ORIENTED_EDGE('',*,*,#47002,.F.);
#63883=ORIENTED_EDGE('',*,*,#47005,.F.);
#63884=ORIENTED_EDGE('',*,*,#47006,.T.);
#63885=ORIENTED_EDGE('',*,*,#46475,.F.);
#63886=ORIENTED_EDGE('',*,*,#47004,.F.);
#63887=ORIENTED_EDGE('',*,*,#47007,.F.);
#63888=ORIENTED_EDGE('',*,*,#47008,.T.);
#63889=ORIENTED_EDGE('',*,*,#46472,.F.);
#63890=ORIENTED_EDGE('',*,*,#47006,.F.);
#63891=ORIENTED_EDGE('',*,*,#47009,.F.);
#63892=ORIENTED_EDGE('',*,*,#47010,.T.);
#63893=ORIENTED_EDGE('',*,*,#46468,.F.);
#63894=ORIENTED_EDGE('',*,*,#47008,.F.);
#63895=ORIENTED_EDGE('',*,*,#47011,.F.);
#63896=ORIENTED_EDGE('',*,*,#47012,.T.);
#63897=ORIENTED_EDGE('',*,*,#46421,.F.);
#63898=ORIENTED_EDGE('',*,*,#47010,.F.);
#63899=ORIENTED_EDGE('',*,*,#47013,.F.);
#63900=ORIENTED_EDGE('',*,*,#47014,.T.);
#63901=ORIENTED_EDGE('',*,*,#47015,.T.);
#63902=ORIENTED_EDGE('',*,*,#46816,.F.);
#63903=ORIENTED_EDGE('',*,*,#47012,.F.);
#63904=ORIENTED_EDGE('',*,*,#47016,.F.);
#63905=ORIENTED_EDGE('',*,*,#47014,.F.);
#63906=ORIENTED_EDGE('',*,*,#47017,.F.);
#63907=ORIENTED_EDGE('',*,*,#46814,.T.);
#63908=ORIENTED_EDGE('',*,*,#47018,.F.);
#63909=ORIENTED_EDGE('',*,*,#47015,.F.);
#63910=ORIENTED_EDGE('',*,*,#46432,.F.);
#63911=ORIENTED_EDGE('',*,*,#46815,.T.);
#63912=ORIENTED_EDGE('',*,*,#47019,.F.);
#63913=ORIENTED_EDGE('',*,*,#46993,.F.);
#63914=ORIENTED_EDGE('',*,*,#47020,.T.);
#63915=ORIENTED_EDGE('',*,*,#47021,.F.);
#63916=ORIENTED_EDGE('',*,*,#47022,.F.);
#63917=ORIENTED_EDGE('',*,*,#47023,.F.);
#63918=ORIENTED_EDGE('',*,*,#46997,.T.);
#63919=ORIENTED_EDGE('',*,*,#47024,.F.);
#63920=ORIENTED_EDGE('',*,*,#47025,.F.);
#63921=ORIENTED_EDGE('',*,*,#47026,.F.);
#63922=ORIENTED_EDGE('',*,*,#47027,.F.);
#63923=ORIENTED_EDGE('',*,*,#47028,.T.);
#63924=ORIENTED_EDGE('',*,*,#46423,.F.);
#63925=ORIENTED_EDGE('',*,*,#47026,.T.);
#63926=ORIENTED_EDGE('',*,*,#47029,.T.);
#63927=ORIENTED_EDGE('',*,*,#47030,.F.);
#63928=ORIENTED_EDGE('',*,*,#47031,.F.);
#63929=ORIENTED_EDGE('',*,*,#47028,.F.);
#63930=ORIENTED_EDGE('',*,*,#47031,.T.);
#63931=ORIENTED_EDGE('',*,*,#47032,.F.);
#63932=ORIENTED_EDGE('',*,*,#47033,.F.);
#63933=ORIENTED_EDGE('',*,*,#46424,.F.);
#63934=ORIENTED_EDGE('',*,*,#47033,.T.);
#63935=ORIENTED_EDGE('',*,*,#47034,.F.);
#63936=ORIENTED_EDGE('',*,*,#47035,.F.);
#63937=ORIENTED_EDGE('',*,*,#46427,.F.);
#63938=ORIENTED_EDGE('',*,*,#47036,.F.);
#63939=ORIENTED_EDGE('',*,*,#46808,.T.);
#63940=ORIENTED_EDGE('',*,*,#46430,.F.);
#63941=ORIENTED_EDGE('',*,*,#47035,.T.);
#63942=ORIENTED_EDGE('',*,*,#46809,.T.);
#63943=ORIENTED_EDGE('',*,*,#47037,.F.);
#63944=ORIENTED_EDGE('',*,*,#47038,.F.);
#63945=ORIENTED_EDGE('',*,*,#47039,.F.);
#63946=ORIENTED_EDGE('',*,*,#47038,.T.);
#63947=ORIENTED_EDGE('',*,*,#47040,.F.);
#63948=ORIENTED_EDGE('',*,*,#47041,.F.);
#63949=ORIENTED_EDGE('',*,*,#46834,.F.);
#63950=ORIENTED_EDGE('',*,*,#47041,.T.);
#63951=ORIENTED_EDGE('',*,*,#47042,.F.);
#63952=ORIENTED_EDGE('',*,*,#47043,.F.);
#63953=ORIENTED_EDGE('',*,*,#46453,.F.);
#63954=ORIENTED_EDGE('',*,*,#47043,.T.);
#63955=ORIENTED_EDGE('',*,*,#47044,.F.);
#63956=ORIENTED_EDGE('',*,*,#47045,.F.);
#63957=ORIENTED_EDGE('',*,*,#46450,.F.);
#63958=ORIENTED_EDGE('',*,*,#47045,.T.);
#63959=ORIENTED_EDGE('',*,*,#47046,.F.);
#63960=ORIENTED_EDGE('',*,*,#47047,.F.);
#63961=ORIENTED_EDGE('',*,*,#46447,.F.);
#63962=ORIENTED_EDGE('',*,*,#47047,.T.);
#63963=ORIENTED_EDGE('',*,*,#47048,.F.);
#63964=ORIENTED_EDGE('',*,*,#47049,.F.);
#63965=ORIENTED_EDGE('',*,*,#46444,.F.);
#63966=ORIENTED_EDGE('',*,*,#47049,.T.);
#63967=ORIENTED_EDGE('',*,*,#47050,.F.);
#63968=ORIENTED_EDGE('',*,*,#47051,.F.);
#63969=ORIENTED_EDGE('',*,*,#46441,.F.);
#63970=ORIENTED_EDGE('',*,*,#47051,.T.);
#63971=ORIENTED_EDGE('',*,*,#47052,.F.);
#63972=ORIENTED_EDGE('',*,*,#47053,.F.);
#63973=ORIENTED_EDGE('',*,*,#46438,.F.);
#63974=ORIENTED_EDGE('',*,*,#47053,.T.);
#63975=ORIENTED_EDGE('',*,*,#47054,.F.);
#63976=ORIENTED_EDGE('',*,*,#47055,.F.);
#63977=ORIENTED_EDGE('',*,*,#46434,.F.);
#63978=ORIENTED_EDGE('',*,*,#47055,.T.);
#63979=ORIENTED_EDGE('',*,*,#47056,.F.);
#63980=ORIENTED_EDGE('',*,*,#47057,.F.);
#63981=ORIENTED_EDGE('',*,*,#47058,.F.);
#63982=ORIENTED_EDGE('',*,*,#47057,.T.);
#63983=ORIENTED_EDGE('',*,*,#47059,.F.);
#63984=ORIENTED_EDGE('',*,*,#47060,.F.);
#63985=ORIENTED_EDGE('',*,*,#47061,.F.);
#63986=ORIENTED_EDGE('',*,*,#46435,.F.);
#63987=ORIENTED_EDGE('',*,*,#47058,.T.);
#63988=ORIENTED_EDGE('',*,*,#47062,.F.);
#63989=ORIENTED_EDGE('',*,*,#47063,.T.);
#63990=ORIENTED_EDGE('',*,*,#47064,.T.);
#63991=ORIENTED_EDGE('',*,*,#47065,.F.);
#63992=ORIENTED_EDGE('',*,*,#47066,.F.);
#63993=ORIENTED_EDGE('',*,*,#46461,.F.);
#63994=ORIENTED_EDGE('',*,*,#47066,.T.);
#63995=ORIENTED_EDGE('',*,*,#47067,.F.);
#63996=ORIENTED_EDGE('',*,*,#47068,.F.);
#63997=ORIENTED_EDGE('',*,*,#46458,.F.);
#63998=ORIENTED_EDGE('',*,*,#47069,.T.);
#63999=ORIENTED_EDGE('',*,*,#47070,.F.);
#64000=ORIENTED_EDGE('',*,*,#47071,.F.);
#64001=ORIENTED_EDGE('',*,*,#47072,.F.);
#64002=ORIENTED_EDGE('',*,*,#47071,.T.);
#64003=ORIENTED_EDGE('',*,*,#47073,.F.);
#64004=ORIENTED_EDGE('',*,*,#47074,.F.);
#64005=ORIENTED_EDGE('',*,*,#47063,.F.);
#64006=ORIENTED_EDGE('',*,*,#47074,.T.);
#64007=ORIENTED_EDGE('',*,*,#47075,.F.);
#64008=ORIENTED_EDGE('',*,*,#47076,.F.);
#64009=ORIENTED_EDGE('',*,*,#46436,.F.);
#64010=ORIENTED_EDGE('',*,*,#47076,.T.);
#64011=ORIENTED_EDGE('',*,*,#47077,.F.);
#64012=ORIENTED_EDGE('',*,*,#47078,.F.);
#64013=ORIENTED_EDGE('',*,*,#46439,.F.);
#64014=ORIENTED_EDGE('',*,*,#47078,.T.);
#64015=ORIENTED_EDGE('',*,*,#47079,.F.);
#64016=ORIENTED_EDGE('',*,*,#47080,.F.);
#64017=ORIENTED_EDGE('',*,*,#46442,.F.);
#64018=ORIENTED_EDGE('',*,*,#47081,.T.);
#64019=ORIENTED_EDGE('',*,*,#46445,.F.);
#64020=ORIENTED_EDGE('',*,*,#47080,.T.);
#64021=ORIENTED_EDGE('',*,*,#47082,.F.);
#64022=ORIENTED_EDGE('',*,*,#47083,.T.);
#64023=ORIENTED_EDGE('',*,*,#46448,.F.);
#64024=ORIENTED_EDGE('',*,*,#47081,.F.);
#64025=ORIENTED_EDGE('',*,*,#47084,.F.);
#64026=ORIENTED_EDGE('',*,*,#47085,.T.);
#64027=ORIENTED_EDGE('',*,*,#46451,.F.);
#64028=ORIENTED_EDGE('',*,*,#47083,.F.);
#64029=ORIENTED_EDGE('',*,*,#47086,.F.);
#64030=ORIENTED_EDGE('',*,*,#47087,.T.);
#64031=ORIENTED_EDGE('',*,*,#46454,.F.);
#64032=ORIENTED_EDGE('',*,*,#47085,.F.);
#64033=ORIENTED_EDGE('',*,*,#47088,.F.);
#64034=ORIENTED_EDGE('',*,*,#47089,.T.);
#64035=ORIENTED_EDGE('',*,*,#47090,.T.);
#64036=ORIENTED_EDGE('',*,*,#46835,.F.);
#64037=ORIENTED_EDGE('',*,*,#47087,.F.);
#64038=ORIENTED_EDGE('',*,*,#47091,.F.);
#64039=ORIENTED_EDGE('',*,*,#47089,.F.);
#64040=ORIENTED_EDGE('',*,*,#47092,.F.);
#64041=ORIENTED_EDGE('',*,*,#46831,.T.);
#64042=ORIENTED_EDGE('',*,*,#47093,.F.);
#64043=ORIENTED_EDGE('',*,*,#47090,.F.);
#64044=ORIENTED_EDGE('',*,*,#46464,.F.);
#64045=ORIENTED_EDGE('',*,*,#46832,.T.);
#64046=ORIENTED_EDGE('',*,*,#47094,.F.);
#64047=ORIENTED_EDGE('',*,*,#47064,.F.);
#64048=ORIENTED_EDGE('',*,*,#47068,.T.);
#64049=ORIENTED_EDGE('',*,*,#47095,.F.);
#64050=ORIENTED_EDGE('',*,*,#47096,.F.);
#64051=ORIENTED_EDGE('',*,*,#47097,.F.);
#64052=ORIENTED_EDGE('',*,*,#47098,.F.);
#64053=ORIENTED_EDGE('',*,*,#47099,.T.);
#64054=ORIENTED_EDGE('',*,*,#46455,.F.);
#64055=ORIENTED_EDGE('',*,*,#47097,.T.);
#64056=ORIENTED_EDGE('',*,*,#47100,.T.);
#64057=ORIENTED_EDGE('',*,*,#47101,.F.);
#64058=ORIENTED_EDGE('',*,*,#47102,.F.);
#64059=ORIENTED_EDGE('',*,*,#47103,.F.);
#64060=ORIENTED_EDGE('',*,*,#46766,.T.);
#64061=ORIENTED_EDGE('',*,*,#47104,.F.);
#64062=ORIENTED_EDGE('',*,*,#47105,.F.);
#64063=ORIENTED_EDGE('',*,*,#47106,.F.);
#64064=ORIENTED_EDGE('',*,*,#46579,.T.);
#64065=ORIENTED_EDGE('',*,*,#47107,.F.);
#64066=ORIENTED_EDGE('',*,*,#47108,.F.);
#64067=ORIENTED_EDGE('',*,*,#46992,.F.);
#64068=ORIENTED_EDGE('',*,*,#47108,.T.);
#64069=ORIENTED_EDGE('',*,*,#47109,.F.);
#64070=ORIENTED_EDGE('',*,*,#47110,.F.);
#64071=ORIENTED_EDGE('',*,*,#47111,.F.);
#64072=ORIENTED_EDGE('',*,*,#47112,.T.);
#64073=ORIENTED_EDGE('',*,*,#47099,.F.);
#64074=ORIENTED_EDGE('',*,*,#47113,.F.);
#64075=ORIENTED_EDGE('',*,*,#47114,.F.);
#64076=ORIENTED_EDGE('',*,*,#47115,.T.);
#64077=ORIENTED_EDGE('',*,*,#46456,.F.);
#64078=ORIENTED_EDGE('',*,*,#47112,.F.);
#64079=ORIENTED_EDGE('',*,*,#47116,.F.);
#64080=ORIENTED_EDGE('',*,*,#47117,.T.);
#64081=ORIENTED_EDGE('',*,*,#46459,.F.);
#64082=ORIENTED_EDGE('',*,*,#47115,.F.);
#64083=ORIENTED_EDGE('',*,*,#47118,.F.);
#64084=ORIENTED_EDGE('',*,*,#47119,.F.);
#64085=ORIENTED_EDGE('',*,*,#46827,.T.);
#64086=ORIENTED_EDGE('',*,*,#46462,.F.);
#64087=ORIENTED_EDGE('',*,*,#47117,.F.);
#64088=ORIENTED_EDGE('',*,*,#47120,.T.);
#64089=ORIENTED_EDGE('',*,*,#47121,.F.);
#64090=ORIENTED_EDGE('',*,*,#46824,.F.);
#64091=ORIENTED_EDGE('',*,*,#47122,.F.);
#64092=ORIENTED_EDGE('',*,*,#47102,.T.);
#64093=ORIENTED_EDGE('',*,*,#46822,.F.);
#64094=ORIENTED_EDGE('',*,*,#47120,.F.);
#64095=ORIENTED_EDGE('',*,*,#47123,.F.);
#64096=ORIENTED_EDGE('',*,*,#47124,.T.);
#64097=ORIENTED_EDGE('',*,*,#46466,.F.);
#64098=ORIENTED_EDGE('',*,*,#47125,.F.);
#64099=ORIENTED_EDGE('',*,*,#47126,.F.);
#64100=ORIENTED_EDGE('',*,*,#47127,.T.);
#64101=ORIENTED_EDGE('',*,*,#46470,.F.);
#64102=ORIENTED_EDGE('',*,*,#47124,.F.);
#64103=ORIENTED_EDGE('',*,*,#47128,.F.);
#64104=ORIENTED_EDGE('',*,*,#47129,.T.);
#64105=ORIENTED_EDGE('',*,*,#46473,.F.);
#64106=ORIENTED_EDGE('',*,*,#47127,.F.);
#64107=ORIENTED_EDGE('',*,*,#47130,.F.);
#64108=ORIENTED_EDGE('',*,*,#47131,.T.);
#64109=ORIENTED_EDGE('',*,*,#46476,.F.);
#64110=ORIENTED_EDGE('',*,*,#47129,.F.);
#64111=ORIENTED_EDGE('',*,*,#47132,.F.);
#64112=ORIENTED_EDGE('',*,*,#47133,.T.);
#64113=ORIENTED_EDGE('',*,*,#46479,.F.);
#64114=ORIENTED_EDGE('',*,*,#47131,.F.);
#64115=ORIENTED_EDGE('',*,*,#47134,.F.);
#64116=ORIENTED_EDGE('',*,*,#47135,.T.);
#64117=ORIENTED_EDGE('',*,*,#47136,.F.);
#64118=ORIENTED_EDGE('',*,*,#47133,.F.);
#64119=ORIENTED_EDGE('',*,*,#47137,.F.);
#64120=ORIENTED_EDGE('',*,*,#47138,.T.);
#64121=ORIENTED_EDGE('',*,*,#47139,.F.);
#64122=ORIENTED_EDGE('',*,*,#47140,.F.);
#64123=ORIENTED_EDGE('',*,*,#46723,.F.);
#64124=ORIENTED_EDGE('',*,*,#47140,.T.);
#64125=ORIENTED_EDGE('',*,*,#47141,.F.);
#64126=ORIENTED_EDGE('',*,*,#47142,.F.);
#64127=ORIENTED_EDGE('',*,*,#46706,.F.);
#64128=ORIENTED_EDGE('',*,*,#46841,.T.);
#64129=ORIENTED_EDGE('',*,*,#46844,.T.);
#64130=ORIENTED_EDGE('',*,*,#46719,.F.);
#64131=ORIENTED_EDGE('',*,*,#47142,.T.);
#64132=ORIENTED_EDGE('',*,*,#47143,.F.);
#64133=ORIENTED_EDGE('',*,*,#47144,.T.);
#64134=ORIENTED_EDGE('',*,*,#47145,.F.);
#64135=ORIENTED_EDGE('',*,*,#46838,.F.);
#64136=ORIENTED_EDGE('',*,*,#47146,.F.);
#64137=ORIENTED_EDGE('',*,*,#47125,.T.);
#64138=ORIENTED_EDGE('',*,*,#46837,.F.);
#64139=ORIENTED_EDGE('',*,*,#47144,.F.);
#64140=ORIENTED_EDGE('',*,*,#47147,.F.);
#64141=ORIENTED_EDGE('',*,*,#47000,.T.);
#64142=ORIENTED_EDGE('',*,*,#47148,.F.);
#64143=ORIENTED_EDGE('',*,*,#47020,.F.);
#64144=ORIENTED_EDGE('',*,*,#47149,.F.);
#64145=ORIENTED_EDGE('',*,*,#47150,.T.);
#64146=ORIENTED_EDGE('',*,*,#47151,.F.);
#64147=ORIENTED_EDGE('',*,*,#47135,.F.);
#64148=ORIENTED_EDGE('',*,*,#47152,.F.);
#64149=ORIENTED_EDGE('',*,*,#46480,.T.);
#64150=ORIENTED_EDGE('',*,*,#47136,.T.);
#64151=ORIENTED_EDGE('',*,*,#47153,.T.);
#64152=ORIENTED_EDGE('',*,*,#46999,.T.);
#64153=ORIENTED_EDGE('',*,*,#47154,.T.);
#64154=ORIENTED_EDGE('',*,*,#47155,.F.);
#64155=ORIENTED_EDGE('',*,*,#47156,.F.);
#64156=ORIENTED_EDGE('',*,*,#46488,.F.);
#64157=ORIENTED_EDGE('',*,*,#47156,.T.);
#64158=ORIENTED_EDGE('',*,*,#47157,.F.);
#64159=ORIENTED_EDGE('',*,*,#47158,.F.);
#64160=ORIENTED_EDGE('',*,*,#46485,.F.);
#64161=ORIENTED_EDGE('',*,*,#47159,.T.);
#64162=ORIENTED_EDGE('',*,*,#47160,.F.);
#64163=ORIENTED_EDGE('',*,*,#47161,.F.);
#64164=ORIENTED_EDGE('',*,*,#47162,.F.);
#64165=ORIENTED_EDGE('',*,*,#47163,.T.);
#64166=ORIENTED_EDGE('',*,*,#46543,.F.);
#64167=ORIENTED_EDGE('',*,*,#47159,.F.);
#64168=ORIENTED_EDGE('',*,*,#47164,.F.);
#64169=ORIENTED_EDGE('',*,*,#47165,.T.);
#64170=ORIENTED_EDGE('',*,*,#46530,.F.);
#64171=ORIENTED_EDGE('',*,*,#47163,.F.);
#64172=ORIENTED_EDGE('',*,*,#47166,.F.);
#64173=ORIENTED_EDGE('',*,*,#47167,.T.);
#64174=ORIENTED_EDGE('',*,*,#46527,.F.);
#64175=ORIENTED_EDGE('',*,*,#47165,.F.);
#64176=ORIENTED_EDGE('',*,*,#47168,.F.);
#64177=ORIENTED_EDGE('',*,*,#47169,.T.);
#64178=ORIENTED_EDGE('',*,*,#46524,.F.);
#64179=ORIENTED_EDGE('',*,*,#47167,.F.);
#64180=ORIENTED_EDGE('',*,*,#47170,.F.);
#64181=ORIENTED_EDGE('',*,*,#47171,.T.);
#64182=ORIENTED_EDGE('',*,*,#46521,.F.);
#64183=ORIENTED_EDGE('',*,*,#47169,.F.);
#64184=ORIENTED_EDGE('',*,*,#47172,.F.);
#64185=ORIENTED_EDGE('',*,*,#47173,.T.);
#64186=ORIENTED_EDGE('',*,*,#46518,.F.);
#64187=ORIENTED_EDGE('',*,*,#47171,.F.);
#64188=ORIENTED_EDGE('',*,*,#47174,.F.);
#64189=ORIENTED_EDGE('',*,*,#47175,.T.);
#64190=ORIENTED_EDGE('',*,*,#46515,.F.);
#64191=ORIENTED_EDGE('',*,*,#47173,.F.);
#64192=ORIENTED_EDGE('',*,*,#47176,.F.);
#64193=ORIENTED_EDGE('',*,*,#47177,.T.);
#64194=ORIENTED_EDGE('',*,*,#46947,.F.);
#64195=ORIENTED_EDGE('',*,*,#47175,.F.);
#64196=ORIENTED_EDGE('',*,*,#47178,.F.);
#64197=ORIENTED_EDGE('',*,*,#46943,.T.);
#64198=ORIENTED_EDGE('',*,*,#47179,.F.);
#64199=ORIENTED_EDGE('',*,*,#47177,.F.);
#64200=ORIENTED_EDGE('',*,*,#47180,.F.);
#64201=ORIENTED_EDGE('',*,*,#46491,.F.);
#64202=ORIENTED_EDGE('',*,*,#46944,.T.);
#64203=ORIENTED_EDGE('',*,*,#47181,.F.);
#64204=ORIENTED_EDGE('',*,*,#47154,.F.);
#64205=ORIENTED_EDGE('',*,*,#47158,.T.);
#64206=ORIENTED_EDGE('',*,*,#47182,.F.);
#64207=ORIENTED_EDGE('',*,*,#47183,.F.);
#64208=ORIENTED_EDGE('',*,*,#47184,.F.);
#64209=ORIENTED_EDGE('',*,*,#47185,.F.);
#64210=ORIENTED_EDGE('',*,*,#47186,.T.);
#64211=ORIENTED_EDGE('',*,*,#46482,.F.);
#64212=ORIENTED_EDGE('',*,*,#47184,.T.);
#64213=ORIENTED_EDGE('',*,*,#47187,.T.);
#64214=ORIENTED_EDGE('',*,*,#47188,.F.);
#64215=ORIENTED_EDGE('',*,*,#47189,.F.);
#64216=ORIENTED_EDGE('',*,*,#47186,.F.);
#64217=ORIENTED_EDGE('',*,*,#47189,.T.);
#64218=ORIENTED_EDGE('',*,*,#47190,.F.);
#64219=ORIENTED_EDGE('',*,*,#47191,.F.);
#64220=ORIENTED_EDGE('',*,*,#46483,.F.);
#64221=ORIENTED_EDGE('',*,*,#47191,.T.);
#64222=ORIENTED_EDGE('',*,*,#47192,.F.);
#64223=ORIENTED_EDGE('',*,*,#47193,.F.);
#64224=ORIENTED_EDGE('',*,*,#46486,.F.);
#64225=ORIENTED_EDGE('',*,*,#47194,.F.);
#64226=ORIENTED_EDGE('',*,*,#46937,.T.);
#64227=ORIENTED_EDGE('',*,*,#46489,.F.);
#64228=ORIENTED_EDGE('',*,*,#47193,.T.);
#64229=ORIENTED_EDGE('',*,*,#46938,.T.);
#64230=ORIENTED_EDGE('',*,*,#47195,.F.);
#64231=ORIENTED_EDGE('',*,*,#47196,.F.);
#64232=ORIENTED_EDGE('',*,*,#47197,.F.);
#64233=ORIENTED_EDGE('',*,*,#47196,.T.);
#64234=ORIENTED_EDGE('',*,*,#47198,.F.);
#64235=ORIENTED_EDGE('',*,*,#47199,.F.);
#64236=ORIENTED_EDGE('',*,*,#46935,.F.);
#64237=ORIENTED_EDGE('',*,*,#47199,.T.);
#64238=ORIENTED_EDGE('',*,*,#47200,.F.);
#64239=ORIENTED_EDGE('',*,*,#47201,.F.);
#64240=ORIENTED_EDGE('',*,*,#46493,.F.);
#64241=ORIENTED_EDGE('',*,*,#47201,.T.);
#64242=ORIENTED_EDGE('',*,*,#47202,.F.);
#64243=ORIENTED_EDGE('',*,*,#47203,.F.);
#64244=ORIENTED_EDGE('',*,*,#46508,.F.);
#64245=ORIENTED_EDGE('',*,*,#47203,.T.);
#64246=ORIENTED_EDGE('',*,*,#47204,.F.);
#64247=ORIENTED_EDGE('',*,*,#47205,.F.);
#64248=ORIENTED_EDGE('',*,*,#46506,.F.);
#64249=ORIENTED_EDGE('',*,*,#47205,.T.);
#64250=ORIENTED_EDGE('',*,*,#47206,.F.);
#64251=ORIENTED_EDGE('',*,*,#47207,.F.);
#64252=ORIENTED_EDGE('',*,*,#46503,.F.);
#64253=ORIENTED_EDGE('',*,*,#47207,.T.);
#64254=ORIENTED_EDGE('',*,*,#47208,.F.);
#64255=ORIENTED_EDGE('',*,*,#47209,.F.);
#64256=ORIENTED_EDGE('',*,*,#46500,.F.);
#64257=ORIENTED_EDGE('',*,*,#47209,.T.);
#64258=ORIENTED_EDGE('',*,*,#47210,.F.);
#64259=ORIENTED_EDGE('',*,*,#47211,.F.);
#64260=ORIENTED_EDGE('',*,*,#46496,.F.);
#64261=ORIENTED_EDGE('',*,*,#47211,.T.);
#64262=ORIENTED_EDGE('',*,*,#47212,.F.);
#64263=ORIENTED_EDGE('',*,*,#47213,.F.);
#64264=ORIENTED_EDGE('',*,*,#47214,.F.);
#64265=ORIENTED_EDGE('',*,*,#47215,.T.);
#64266=ORIENTED_EDGE('',*,*,#47216,.F.);
#64267=ORIENTED_EDGE('',*,*,#47217,.F.);
#64268=ORIENTED_EDGE('',*,*,#47218,.F.);
#64269=ORIENTED_EDGE('',*,*,#47213,.T.);
#64270=ORIENTED_EDGE('',*,*,#47219,.F.);
#64271=ORIENTED_EDGE('',*,*,#47215,.F.);
#64272=ORIENTED_EDGE('',*,*,#47220,.F.);
#64273=ORIENTED_EDGE('',*,*,#46497,.T.);
#64274=ORIENTED_EDGE('',*,*,#47214,.T.);
#64275=ORIENTED_EDGE('',*,*,#47221,.T.);
#64276=ORIENTED_EDGE('',*,*,#47222,.T.);
#64277=ORIENTED_EDGE('',*,*,#47223,.T.);
#64278=ORIENTED_EDGE('',*,*,#47224,.F.);
#64279=ORIENTED_EDGE('',*,*,#47225,.F.);
#64280=ORIENTED_EDGE('',*,*,#46615,.F.);
#64281=ORIENTED_EDGE('',*,*,#47225,.T.);
#64282=ORIENTED_EDGE('',*,*,#47226,.F.);
#64283=ORIENTED_EDGE('',*,*,#47227,.F.);
#64284=ORIENTED_EDGE('',*,*,#46727,.F.);
#64285=ORIENTED_EDGE('',*,*,#47228,.T.);
#64286=ORIENTED_EDGE('',*,*,#47229,.F.);
#64287=ORIENTED_EDGE('',*,*,#47230,.F.);
#64288=ORIENTED_EDGE('',*,*,#47231,.F.);
#64289=ORIENTED_EDGE('',*,*,#47230,.T.);
#64290=ORIENTED_EDGE('',*,*,#47232,.F.);
#64291=ORIENTED_EDGE('',*,*,#47233,.F.);
#64292=ORIENTED_EDGE('',*,*,#47234,.F.);
#64293=ORIENTED_EDGE('',*,*,#47233,.T.);
#64294=ORIENTED_EDGE('',*,*,#47235,.F.);
#64295=ORIENTED_EDGE('',*,*,#47236,.F.);
#64296=ORIENTED_EDGE('',*,*,#47222,.F.);
#64297=ORIENTED_EDGE('',*,*,#47236,.T.);
#64298=ORIENTED_EDGE('',*,*,#47237,.F.);
#64299=ORIENTED_EDGE('',*,*,#47238,.F.);
#64300=ORIENTED_EDGE('',*,*,#46498,.F.);
#64301=ORIENTED_EDGE('',*,*,#47238,.T.);
#64302=ORIENTED_EDGE('',*,*,#47239,.F.);
#64303=ORIENTED_EDGE('',*,*,#47240,.F.);
#64304=ORIENTED_EDGE('',*,*,#46501,.F.);
#64305=ORIENTED_EDGE('',*,*,#47240,.T.);
#64306=ORIENTED_EDGE('',*,*,#47241,.F.);
#64307=ORIENTED_EDGE('',*,*,#47242,.F.);
#64308=ORIENTED_EDGE('',*,*,#46504,.F.);
#64309=ORIENTED_EDGE('',*,*,#47242,.T.);
#64310=ORIENTED_EDGE('',*,*,#47243,.F.);
#64311=ORIENTED_EDGE('',*,*,#47244,.F.);
#64312=ORIENTED_EDGE('',*,*,#46507,.F.);
#64313=ORIENTED_EDGE('',*,*,#47244,.T.);
#64314=ORIENTED_EDGE('',*,*,#47245,.F.);
#64315=ORIENTED_EDGE('',*,*,#47246,.F.);
#64316=ORIENTED_EDGE('',*,*,#46509,.F.);
#64317=ORIENTED_EDGE('',*,*,#47246,.T.);
#64318=ORIENTED_EDGE('',*,*,#47247,.F.);
#64319=ORIENTED_EDGE('',*,*,#47248,.F.);
#64320=ORIENTED_EDGE('',*,*,#46926,.F.);
#64321=ORIENTED_EDGE('',*,*,#47248,.T.);
#64322=ORIENTED_EDGE('',*,*,#47249,.F.);
#64323=ORIENTED_EDGE('',*,*,#46929,.F.);
#64324=ORIENTED_EDGE('',*,*,#47250,.F.);
#64325=ORIENTED_EDGE('',*,*,#46925,.T.);
#64326=ORIENTED_EDGE('',*,*,#46930,.T.);
#64327=ORIENTED_EDGE('',*,*,#47251,.F.);
#64328=ORIENTED_EDGE('',*,*,#47223,.F.);
#64329=ORIENTED_EDGE('',*,*,#46618,.F.);
#64330=ORIENTED_EDGE('',*,*,#47252,.F.);
#64331=ORIENTED_EDGE('',*,*,#46974,.T.);
#64332=ORIENTED_EDGE('',*,*,#47253,.F.);
#64333=ORIENTED_EDGE('',*,*,#47254,.T.);
#64334=ORIENTED_EDGE('',*,*,#47255,.T.);
#64335=ORIENTED_EDGE('',*,*,#47256,.F.);
#64336=ORIENTED_EDGE('',*,*,#47257,.F.);
#64337=ORIENTED_EDGE('',*,*,#47258,.F.);
#64338=ORIENTED_EDGE('',*,*,#47259,.T.);
#64339=ORIENTED_EDGE('',*,*,#46958,.F.);
#64340=ORIENTED_EDGE('',*,*,#47255,.F.);
#64341=ORIENTED_EDGE('',*,*,#47260,.F.);
#64342=ORIENTED_EDGE('',*,*,#46955,.T.);
#64343=ORIENTED_EDGE('',*,*,#47261,.F.);
#64344=ORIENTED_EDGE('',*,*,#47259,.F.);
#64345=ORIENTED_EDGE('',*,*,#47262,.F.);
#64346=ORIENTED_EDGE('',*,*,#46540,.F.);
#64347=ORIENTED_EDGE('',*,*,#46956,.T.);
#64348=ORIENTED_EDGE('',*,*,#47263,.F.);
#64349=ORIENTED_EDGE('',*,*,#47264,.F.);
#64350=ORIENTED_EDGE('',*,*,#47264,.T.);
#64351=ORIENTED_EDGE('',*,*,#47265,.F.);
#64352=ORIENTED_EDGE('',*,*,#47266,.F.);
#64353=ORIENTED_EDGE('',*,*,#46536,.F.);
#64354=ORIENTED_EDGE('',*,*,#47266,.T.);
#64355=ORIENTED_EDGE('',*,*,#47267,.F.);
#64356=ORIENTED_EDGE('',*,*,#47268,.F.);
#64357=ORIENTED_EDGE('',*,*,#46532,.F.);
#64358=ORIENTED_EDGE('',*,*,#47269,.F.);
#64359=ORIENTED_EDGE('',*,*,#47270,.F.);
#64360=ORIENTED_EDGE('',*,*,#47271,.F.);
#64361=ORIENTED_EDGE('',*,*,#47272,.F.);
#64362=ORIENTED_EDGE('',*,*,#47273,.F.);
#64363=ORIENTED_EDGE('',*,*,#47274,.F.);
#64364=ORIENTED_EDGE('',*,*,#47275,.T.);
#64365=ORIENTED_EDGE('',*,*,#46986,.F.);
#64366=ORIENTED_EDGE('',*,*,#47276,.T.);
#64367=ORIENTED_EDGE('',*,*,#47268,.T.);
#64368=ORIENTED_EDGE('',*,*,#47277,.F.);
#64369=ORIENTED_EDGE('',*,*,#47278,.F.);
#64370=ORIENTED_EDGE('',*,*,#47279,.F.);
#64371=ORIENTED_EDGE('',*,*,#46533,.F.);
#64372=ORIENTED_EDGE('',*,*,#47279,.T.);
#64373=ORIENTED_EDGE('',*,*,#47280,.F.);
#64374=ORIENTED_EDGE('',*,*,#47281,.T.);
#64375=ORIENTED_EDGE('',*,*,#47282,.T.);
#64376=ORIENTED_EDGE('',*,*,#46513,.F.);
#64377=ORIENTED_EDGE('',*,*,#47283,.F.);
#64378=ORIENTED_EDGE('',*,*,#47284,.F.);
#64379=ORIENTED_EDGE('',*,*,#47285,.T.);
#64380=ORIENTED_EDGE('',*,*,#46516,.F.);
#64381=ORIENTED_EDGE('',*,*,#47282,.F.);
#64382=ORIENTED_EDGE('',*,*,#47286,.F.);
#64383=ORIENTED_EDGE('',*,*,#47287,.T.);
#64384=ORIENTED_EDGE('',*,*,#46519,.F.);
#64385=ORIENTED_EDGE('',*,*,#47285,.F.);
#64386=ORIENTED_EDGE('',*,*,#47288,.F.);
#64387=ORIENTED_EDGE('',*,*,#47289,.T.);
#64388=ORIENTED_EDGE('',*,*,#46522,.F.);
#64389=ORIENTED_EDGE('',*,*,#47287,.F.);
#64390=ORIENTED_EDGE('',*,*,#47290,.F.);
#64391=ORIENTED_EDGE('',*,*,#47291,.T.);
#64392=ORIENTED_EDGE('',*,*,#46525,.F.);
#64393=ORIENTED_EDGE('',*,*,#47289,.F.);
#64394=ORIENTED_EDGE('',*,*,#47292,.F.);
#64395=ORIENTED_EDGE('',*,*,#47293,.T.);
#64396=ORIENTED_EDGE('',*,*,#46528,.F.);
#64397=ORIENTED_EDGE('',*,*,#47291,.F.);
#64398=ORIENTED_EDGE('',*,*,#47294,.F.);
#64399=ORIENTED_EDGE('',*,*,#47295,.T.);
#64400=ORIENTED_EDGE('',*,*,#46541,.F.);
#64401=ORIENTED_EDGE('',*,*,#47293,.F.);
#64402=ORIENTED_EDGE('',*,*,#47296,.F.);
#64403=ORIENTED_EDGE('',*,*,#47297,.T.);
#64404=ORIENTED_EDGE('',*,*,#47298,.F.);
#64405=ORIENTED_EDGE('',*,*,#47295,.F.);
#64406=ORIENTED_EDGE('',*,*,#47299,.F.);
#64407=ORIENTED_EDGE('',*,*,#47300,.T.);
#64408=ORIENTED_EDGE('',*,*,#47301,.F.);
#64409=ORIENTED_EDGE('',*,*,#47302,.F.);
#64410=ORIENTED_EDGE('',*,*,#47281,.F.);
#64411=ORIENTED_EDGE('',*,*,#47302,.T.);
#64412=ORIENTED_EDGE('',*,*,#47303,.F.);
#64413=ORIENTED_EDGE('',*,*,#47304,.F.);
#64414=ORIENTED_EDGE('',*,*,#46534,.F.);
#64415=ORIENTED_EDGE('',*,*,#47304,.T.);
#64416=ORIENTED_EDGE('',*,*,#47305,.F.);
#64417=ORIENTED_EDGE('',*,*,#47306,.F.);
#64418=ORIENTED_EDGE('',*,*,#46537,.F.);
#64419=ORIENTED_EDGE('',*,*,#47307,.F.);
#64420=ORIENTED_EDGE('',*,*,#46951,.T.);
#64421=ORIENTED_EDGE('',*,*,#46538,.F.);
#64422=ORIENTED_EDGE('',*,*,#47306,.T.);
#64423=ORIENTED_EDGE('',*,*,#47308,.T.);
#64424=ORIENTED_EDGE('',*,*,#47309,.F.);
#64425=ORIENTED_EDGE('',*,*,#46948,.F.);
#64426=ORIENTED_EDGE('',*,*,#47310,.F.);
#64427=ORIENTED_EDGE('',*,*,#47311,.T.);
#64428=ORIENTED_EDGE('',*,*,#47283,.T.);
#64429=ORIENTED_EDGE('',*,*,#46946,.F.);
#64430=ORIENTED_EDGE('',*,*,#47308,.F.);
#64431=ORIENTED_EDGE('',*,*,#47311,.F.);
#64432=ORIENTED_EDGE('',*,*,#47312,.F.);
#64433=ORIENTED_EDGE('',*,*,#47161,.T.);
#64434=ORIENTED_EDGE('',*,*,#47313,.F.);
#64435=ORIENTED_EDGE('',*,*,#47314,.F.);
#64436=ORIENTED_EDGE('',*,*,#47315,.F.);
#64437=ORIENTED_EDGE('',*,*,#47316,.T.);
#64438=ORIENTED_EDGE('',*,*,#47317,.F.);
#64439=ORIENTED_EDGE('',*,*,#47297,.F.);
#64440=ORIENTED_EDGE('',*,*,#47318,.F.);
#64441=ORIENTED_EDGE('',*,*,#46542,.F.);
#64442=ORIENTED_EDGE('',*,*,#47298,.T.);
#64443=ORIENTED_EDGE('',*,*,#47319,.F.);
#64444=ORIENTED_EDGE('',*,*,#47160,.T.);
#64445=ORIENTED_EDGE('',*,*,#47320,.T.);
#64446=ORIENTED_EDGE('',*,*,#47321,.F.);
#64447=ORIENTED_EDGE('',*,*,#47322,.F.);
#64448=ORIENTED_EDGE('',*,*,#47323,.F.);
#64449=ORIENTED_EDGE('',*,*,#47322,.T.);
#64450=ORIENTED_EDGE('',*,*,#47324,.F.);
#64451=ORIENTED_EDGE('',*,*,#47325,.F.);
#64452=ORIENTED_EDGE('',*,*,#46547,.F.);
#64453=ORIENTED_EDGE('',*,*,#47325,.T.);
#64454=ORIENTED_EDGE('',*,*,#47326,.F.);
#64455=ORIENTED_EDGE('',*,*,#47327,.F.);
#64456=ORIENTED_EDGE('',*,*,#46978,.F.);
#64457=ORIENTED_EDGE('',*,*,#47327,.T.);
#64458=ORIENTED_EDGE('',*,*,#47328,.F.);
#64459=ORIENTED_EDGE('',*,*,#47329,.F.);
#64460=ORIENTED_EDGE('',*,*,#47330,.F.);
#64461=ORIENTED_EDGE('',*,*,#47331,.T.);
#64462=ORIENTED_EDGE('',*,*,#47332,.F.);
#64463=ORIENTED_EDGE('',*,*,#47333,.F.);
#64464=ORIENTED_EDGE('',*,*,#47334,.F.);
#64465=ORIENTED_EDGE('',*,*,#47335,.F.);
#64466=ORIENTED_EDGE('',*,*,#47336,.T.);
#64467=ORIENTED_EDGE('',*,*,#47337,.F.);
#64468=ORIENTED_EDGE('',*,*,#47334,.T.);
#64469=ORIENTED_EDGE('',*,*,#47338,.T.);
#64470=ORIENTED_EDGE('',*,*,#47339,.F.);
#64471=ORIENTED_EDGE('',*,*,#47340,.F.);
#64472=ORIENTED_EDGE('',*,*,#47336,.F.);
#64473=ORIENTED_EDGE('',*,*,#47341,.F.);
#64474=ORIENTED_EDGE('',*,*,#47342,.T.);
#64475=ORIENTED_EDGE('',*,*,#47343,.F.);
#64476=ORIENTED_EDGE('',*,*,#47340,.T.);
#64477=ORIENTED_EDGE('',*,*,#46988,.F.);
#64478=ORIENTED_EDGE('',*,*,#47344,.T.);
#64479=ORIENTED_EDGE('',*,*,#47345,.F.);
#64480=ORIENTED_EDGE('',*,*,#47346,.T.);
#64481=ORIENTED_EDGE('',*,*,#47347,.T.);
#64482=ORIENTED_EDGE('',*,*,#47348,.F.);
#64483=ORIENTED_EDGE('',*,*,#47349,.F.);
#64484=ORIENTED_EDGE('',*,*,#47350,.F.);
#64485=ORIENTED_EDGE('',*,*,#47349,.T.);
#64486=ORIENTED_EDGE('',*,*,#47351,.F.);
#64487=ORIENTED_EDGE('',*,*,#47352,.F.);
#64488=ORIENTED_EDGE('',*,*,#46982,.F.);
#64489=ORIENTED_EDGE('',*,*,#47352,.T.);
#64490=ORIENTED_EDGE('',*,*,#47353,.F.);
#64491=ORIENTED_EDGE('',*,*,#47354,.F.);
#64492=ORIENTED_EDGE('',*,*,#47355,.F.);
#64493=ORIENTED_EDGE('',*,*,#47356,.T.);
#64494=ORIENTED_EDGE('',*,*,#47357,.F.);
#64495=ORIENTED_EDGE('',*,*,#47358,.F.);
#64496=ORIENTED_EDGE('',*,*,#47359,.F.);
#64497=ORIENTED_EDGE('',*,*,#47360,.F.);
#64498=ORIENTED_EDGE('',*,*,#47359,.T.);
#64499=ORIENTED_EDGE('',*,*,#47361,.F.);
#64500=ORIENTED_EDGE('',*,*,#47362,.T.);
#64501=ORIENTED_EDGE('',*,*,#47363,.T.);
#64502=ORIENTED_EDGE('',*,*,#47364,.F.);
#64503=ORIENTED_EDGE('',*,*,#47365,.F.);
#64504=ORIENTED_EDGE('',*,*,#47362,.F.);
#64505=ORIENTED_EDGE('',*,*,#47366,.T.);
#64506=ORIENTED_EDGE('',*,*,#47367,.F.);
#64507=ORIENTED_EDGE('',*,*,#47368,.F.);
#64508=ORIENTED_EDGE('',*,*,#47369,.F.);
#64509=ORIENTED_EDGE('',*,*,#47370,.T.);
#64510=ORIENTED_EDGE('',*,*,#46977,.F.);
#64511=ORIENTED_EDGE('',*,*,#47366,.F.);
#64512=ORIENTED_EDGE('',*,*,#47371,.F.);
#64513=ORIENTED_EDGE('',*,*,#47372,.T.);
#64514=ORIENTED_EDGE('',*,*,#46545,.F.);
#64515=ORIENTED_EDGE('',*,*,#47370,.F.);
#64516=ORIENTED_EDGE('',*,*,#47373,.F.);
#64517=ORIENTED_EDGE('',*,*,#47374,.T.);
#64518=ORIENTED_EDGE('',*,*,#47375,.F.);
#64519=ORIENTED_EDGE('',*,*,#47372,.F.);
#64520=ORIENTED_EDGE('',*,*,#47376,.F.);
#64521=ORIENTED_EDGE('',*,*,#47377,.T.);
#64522=ORIENTED_EDGE('',*,*,#47378,.F.);
#64523=ORIENTED_EDGE('',*,*,#47320,.F.);
#64524=ORIENTED_EDGE('',*,*,#47379,.F.);
#64525=ORIENTED_EDGE('',*,*,#47380,.T.);
#64526=ORIENTED_EDGE('',*,*,#47381,.F.);
#64527=ORIENTED_EDGE('',*,*,#47374,.F.);
#64528=ORIENTED_EDGE('',*,*,#47382,.F.);
#64529=ORIENTED_EDGE('',*,*,#46546,.F.);
#64530=ORIENTED_EDGE('',*,*,#47375,.T.);
#64531=ORIENTED_EDGE('',*,*,#47383,.F.);
#64532=ORIENTED_EDGE('',*,*,#47323,.T.);
#64533=ORIENTED_EDGE('',*,*,#47384,.T.);
#64534=ORIENTED_EDGE('',*,*,#47385,.F.);
#64535=ORIENTED_EDGE('',*,*,#47386,.F.);
#64536=ORIENTED_EDGE('',*,*,#46557,.F.);
#64537=ORIENTED_EDGE('',*,*,#47386,.T.);
#64538=ORIENTED_EDGE('',*,*,#47387,.F.);
#64539=ORIENTED_EDGE('',*,*,#47388,.F.);
#64540=ORIENTED_EDGE('',*,*,#46554,.F.);
#64541=ORIENTED_EDGE('',*,*,#47389,.T.);
#64542=ORIENTED_EDGE('',*,*,#47390,.F.);
#64543=ORIENTED_EDGE('',*,*,#47391,.F.);
#64544=ORIENTED_EDGE('',*,*,#47392,.F.);
#64545=ORIENTED_EDGE('',*,*,#47393,.T.);
#64546=ORIENTED_EDGE('',*,*,#46607,.F.);
#64547=ORIENTED_EDGE('',*,*,#47389,.F.);
#64548=ORIENTED_EDGE('',*,*,#47394,.F.);
#64549=ORIENTED_EDGE('',*,*,#47395,.T.);
#64550=ORIENTED_EDGE('',*,*,#46611,.F.);
#64551=ORIENTED_EDGE('',*,*,#47393,.F.);
#64552=ORIENTED_EDGE('',*,*,#47396,.F.);
#64553=ORIENTED_EDGE('',*,*,#47397,.T.);
#64554=ORIENTED_EDGE('',*,*,#46595,.F.);
#64555=ORIENTED_EDGE('',*,*,#47395,.F.);
#64556=ORIENTED_EDGE('',*,*,#47398,.F.);
#64557=ORIENTED_EDGE('',*,*,#47399,.T.);
#64558=ORIENTED_EDGE('',*,*,#46592,.F.);
#64559=ORIENTED_EDGE('',*,*,#47397,.F.);
#64560=ORIENTED_EDGE('',*,*,#47400,.F.);
#64561=ORIENTED_EDGE('',*,*,#47401,.T.);
#64562=ORIENTED_EDGE('',*,*,#46549,.F.);
#64563=ORIENTED_EDGE('',*,*,#47399,.F.);
#64564=ORIENTED_EDGE('',*,*,#47402,.F.);
#64565=ORIENTED_EDGE('',*,*,#47403,.T.);
#64566=ORIENTED_EDGE('',*,*,#46587,.F.);
#64567=ORIENTED_EDGE('',*,*,#47401,.F.);
#64568=ORIENTED_EDGE('',*,*,#47404,.F.);
#64569=ORIENTED_EDGE('',*,*,#47405,.T.);
#64570=ORIENTED_EDGE('',*,*,#46584,.F.);
#64571=ORIENTED_EDGE('',*,*,#47403,.F.);
#64572=ORIENTED_EDGE('',*,*,#47406,.F.);
#64573=ORIENTED_EDGE('',*,*,#47407,.T.);
#64574=ORIENTED_EDGE('',*,*,#46784,.F.);
#64575=ORIENTED_EDGE('',*,*,#47405,.F.);
#64576=ORIENTED_EDGE('',*,*,#47408,.F.);
#64577=ORIENTED_EDGE('',*,*,#46780,.T.);
#64578=ORIENTED_EDGE('',*,*,#47409,.F.);
#64579=ORIENTED_EDGE('',*,*,#47407,.F.);
#64580=ORIENTED_EDGE('',*,*,#47410,.F.);
#64581=ORIENTED_EDGE('',*,*,#46560,.F.);
#64582=ORIENTED_EDGE('',*,*,#46781,.T.);
#64583=ORIENTED_EDGE('',*,*,#47411,.F.);
#64584=ORIENTED_EDGE('',*,*,#47384,.F.);
#64585=ORIENTED_EDGE('',*,*,#47388,.T.);
#64586=ORIENTED_EDGE('',*,*,#47412,.F.);
#64587=ORIENTED_EDGE('',*,*,#47413,.F.);
#64588=ORIENTED_EDGE('',*,*,#47414,.F.);
#64589=ORIENTED_EDGE('',*,*,#47415,.F.);
#64590=ORIENTED_EDGE('',*,*,#47416,.T.);
#64591=ORIENTED_EDGE('',*,*,#46551,.F.);
#64592=ORIENTED_EDGE('',*,*,#47414,.T.);
#64593=ORIENTED_EDGE('',*,*,#47417,.T.);
#64594=ORIENTED_EDGE('',*,*,#47418,.F.);
#64595=ORIENTED_EDGE('',*,*,#47419,.F.);
#64596=ORIENTED_EDGE('',*,*,#47416,.F.);
#64597=ORIENTED_EDGE('',*,*,#47419,.T.);
#64598=ORIENTED_EDGE('',*,*,#47420,.F.);
#64599=ORIENTED_EDGE('',*,*,#47421,.F.);
#64600=ORIENTED_EDGE('',*,*,#46552,.F.);
#64601=ORIENTED_EDGE('',*,*,#47421,.T.);
#64602=ORIENTED_EDGE('',*,*,#47422,.F.);
#64603=ORIENTED_EDGE('',*,*,#47423,.F.);
#64604=ORIENTED_EDGE('',*,*,#46555,.F.);
#64605=ORIENTED_EDGE('',*,*,#47424,.F.);
#64606=ORIENTED_EDGE('',*,*,#46774,.T.);
#64607=ORIENTED_EDGE('',*,*,#46558,.F.);
#64608=ORIENTED_EDGE('',*,*,#47423,.T.);
#64609=ORIENTED_EDGE('',*,*,#46775,.T.);
#64610=ORIENTED_EDGE('',*,*,#47425,.F.);
#64611=ORIENTED_EDGE('',*,*,#47426,.F.);
#64612=ORIENTED_EDGE('',*,*,#47427,.F.);
#64613=ORIENTED_EDGE('',*,*,#47426,.T.);
#64614=ORIENTED_EDGE('',*,*,#47428,.F.);
#64615=ORIENTED_EDGE('',*,*,#47429,.F.);
#64616=ORIENTED_EDGE('',*,*,#46772,.F.);
#64617=ORIENTED_EDGE('',*,*,#47429,.T.);
#64618=ORIENTED_EDGE('',*,*,#47430,.F.);
#64619=ORIENTED_EDGE('',*,*,#47431,.F.);
#64620=ORIENTED_EDGE('',*,*,#46562,.F.);
#64621=ORIENTED_EDGE('',*,*,#47431,.T.);
#64622=ORIENTED_EDGE('',*,*,#47432,.F.);
#64623=ORIENTED_EDGE('',*,*,#47433,.F.);
#64624=ORIENTED_EDGE('',*,*,#46748,.F.);
#64625=ORIENTED_EDGE('',*,*,#47433,.T.);
#64626=ORIENTED_EDGE('',*,*,#47434,.F.);
#64627=ORIENTED_EDGE('',*,*,#47435,.F.);
#64628=ORIENTED_EDGE('',*,*,#46575,.F.);
#64629=ORIENTED_EDGE('',*,*,#47435,.T.);
#64630=ORIENTED_EDGE('',*,*,#47436,.F.);
#64631=ORIENTED_EDGE('',*,*,#47437,.F.);
#64632=ORIENTED_EDGE('',*,*,#46572,.F.);
#64633=ORIENTED_EDGE('',*,*,#47437,.T.);
#64634=ORIENTED_EDGE('',*,*,#47438,.F.);
#64635=ORIENTED_EDGE('',*,*,#47439,.F.);
#64636=ORIENTED_EDGE('',*,*,#46569,.F.);
#64637=ORIENTED_EDGE('',*,*,#47439,.T.);
#64638=ORIENTED_EDGE('',*,*,#47440,.F.);
#64639=ORIENTED_EDGE('',*,*,#47441,.F.);
#64640=ORIENTED_EDGE('',*,*,#46565,.F.);
#64641=ORIENTED_EDGE('',*,*,#47441,.T.);
#64642=ORIENTED_EDGE('',*,*,#47442,.F.);
#64643=ORIENTED_EDGE('',*,*,#47443,.F.);
#64644=ORIENTED_EDGE('',*,*,#47444,.F.);
#64645=ORIENTED_EDGE('',*,*,#47445,.T.);
#64646=ORIENTED_EDGE('',*,*,#47446,.F.);
#64647=ORIENTED_EDGE('',*,*,#47447,.F.);
#64648=ORIENTED_EDGE('',*,*,#47448,.F.);
#64649=ORIENTED_EDGE('',*,*,#47443,.T.);
#64650=ORIENTED_EDGE('',*,*,#47449,.F.);
#64651=ORIENTED_EDGE('',*,*,#47445,.F.);
#64652=ORIENTED_EDGE('',*,*,#47450,.F.);
#64653=ORIENTED_EDGE('',*,*,#46566,.T.);
#64654=ORIENTED_EDGE('',*,*,#47444,.T.);
#64655=ORIENTED_EDGE('',*,*,#47451,.T.);
#64656=ORIENTED_EDGE('',*,*,#47452,.T.);
#64657=ORIENTED_EDGE('',*,*,#47453,.T.);
#64658=ORIENTED_EDGE('',*,*,#47454,.F.);
#64659=ORIENTED_EDGE('',*,*,#47455,.F.);
#64660=ORIENTED_EDGE('',*,*,#46747,.F.);
#64661=ORIENTED_EDGE('',*,*,#47455,.T.);
#64662=ORIENTED_EDGE('',*,*,#47456,.F.);
#64663=ORIENTED_EDGE('',*,*,#47457,.F.);
#64664=ORIENTED_EDGE('',*,*,#46985,.F.);
#64665=ORIENTED_EDGE('',*,*,#47458,.T.);
#64666=ORIENTED_EDGE('',*,*,#47452,.F.);
#64667=ORIENTED_EDGE('',*,*,#47459,.F.);
#64668=ORIENTED_EDGE('',*,*,#47460,.F.);
#64669=ORIENTED_EDGE('',*,*,#47461,.T.);
#64670=ORIENTED_EDGE('',*,*,#46567,.F.);
#64671=ORIENTED_EDGE('',*,*,#47458,.F.);
#64672=ORIENTED_EDGE('',*,*,#47462,.F.);
#64673=ORIENTED_EDGE('',*,*,#47463,.T.);
#64674=ORIENTED_EDGE('',*,*,#46570,.F.);
#64675=ORIENTED_EDGE('',*,*,#47461,.F.);
#64676=ORIENTED_EDGE('',*,*,#47464,.F.);
#64677=ORIENTED_EDGE('',*,*,#47465,.T.);
#64678=ORIENTED_EDGE('',*,*,#46573,.F.);
#64679=ORIENTED_EDGE('',*,*,#47463,.F.);
#64680=ORIENTED_EDGE('',*,*,#47466,.F.);
#64681=ORIENTED_EDGE('',*,*,#47467,.T.);
#64682=ORIENTED_EDGE('',*,*,#46576,.F.);
#64683=ORIENTED_EDGE('',*,*,#47465,.F.);
#64684=ORIENTED_EDGE('',*,*,#47468,.F.);
#64685=ORIENTED_EDGE('',*,*,#47469,.T.);
#64686=ORIENTED_EDGE('',*,*,#46749,.F.);
#64687=ORIENTED_EDGE('',*,*,#47467,.F.);
#64688=ORIENTED_EDGE('',*,*,#47470,.F.);
#64689=ORIENTED_EDGE('',*,*,#47471,.T.);
#64690=ORIENTED_EDGE('',*,*,#47472,.F.);
#64691=ORIENTED_EDGE('',*,*,#47469,.F.);
#64692=ORIENTED_EDGE('',*,*,#47473,.F.);
#64693=ORIENTED_EDGE('',*,*,#47459,.T.);
#64694=ORIENTED_EDGE('',*,*,#47474,.F.);
#64695=ORIENTED_EDGE('',*,*,#47475,.F.);
#64696=ORIENTED_EDGE('',*,*,#47476,.F.);
#64697=ORIENTED_EDGE('',*,*,#47477,.T.);
#64698=ORIENTED_EDGE('',*,*,#47478,.F.);
#64699=ORIENTED_EDGE('',*,*,#47479,.F.);
#64700=ORIENTED_EDGE('',*,*,#47480,.F.);
#64701=ORIENTED_EDGE('',*,*,#47481,.T.);
#64702=ORIENTED_EDGE('',*,*,#46795,.F.);
#64703=ORIENTED_EDGE('',*,*,#47477,.F.);
#64704=ORIENTED_EDGE('',*,*,#47482,.F.);
#64705=ORIENTED_EDGE('',*,*,#46792,.T.);
#64706=ORIENTED_EDGE('',*,*,#47483,.F.);
#64707=ORIENTED_EDGE('',*,*,#47481,.F.);
#64708=ORIENTED_EDGE('',*,*,#47484,.F.);
#64709=ORIENTED_EDGE('',*,*,#46605,.F.);
#64710=ORIENTED_EDGE('',*,*,#46793,.T.);
#64711=ORIENTED_EDGE('',*,*,#47485,.F.);
#64712=ORIENTED_EDGE('',*,*,#47486,.T.);
#64713=ORIENTED_EDGE('',*,*,#47487,.T.);
#64714=ORIENTED_EDGE('',*,*,#46601,.F.);
#64715=ORIENTED_EDGE('',*,*,#47486,.F.);
#64716=ORIENTED_EDGE('',*,*,#47488,.F.);
#64717=ORIENTED_EDGE('',*,*,#47489,.T.);
#64718=ORIENTED_EDGE('',*,*,#46597,.F.);
#64719=ORIENTED_EDGE('',*,*,#47487,.F.);
#64720=ORIENTED_EDGE('',*,*,#47490,.F.);
#64721=ORIENTED_EDGE('',*,*,#47491,.T.);
#64722=ORIENTED_EDGE('',*,*,#47492,.F.);
#64723=ORIENTED_EDGE('',*,*,#47493,.F.);
#64724=ORIENTED_EDGE('',*,*,#47494,.F.);
#64725=ORIENTED_EDGE('',*,*,#47493,.T.);
#64726=ORIENTED_EDGE('',*,*,#47495,.F.);
#64727=ORIENTED_EDGE('',*,*,#46577,.F.);
#64728=ORIENTED_EDGE('',*,*,#46991,.F.);
#64729=ORIENTED_EDGE('',*,*,#47496,.F.);
#64730=ORIENTED_EDGE('',*,*,#46767,.T.);
#64731=ORIENTED_EDGE('',*,*,#47497,.F.);
#64732=ORIENTED_EDGE('',*,*,#46578,.T.);
#64733=ORIENTED_EDGE('',*,*,#47498,.T.);
#64734=ORIENTED_EDGE('',*,*,#47499,.F.);
#64735=ORIENTED_EDGE('',*,*,#46764,.F.);
#64736=ORIENTED_EDGE('',*,*,#47500,.F.);
#64737=ORIENTED_EDGE('',*,*,#47501,.T.);
#64738=ORIENTED_EDGE('',*,*,#47502,.F.);
#64739=ORIENTED_EDGE('',*,*,#47489,.F.);
#64740=ORIENTED_EDGE('',*,*,#47503,.F.);
#64741=ORIENTED_EDGE('',*,*,#46598,.F.);
#64742=ORIENTED_EDGE('',*,*,#47502,.T.);
#64743=ORIENTED_EDGE('',*,*,#47504,.F.);
#64744=ORIENTED_EDGE('',*,*,#47505,.T.);
#64745=ORIENTED_EDGE('',*,*,#47506,.T.);
#64746=ORIENTED_EDGE('',*,*,#46582,.F.);
#64747=ORIENTED_EDGE('',*,*,#47507,.F.);
#64748=ORIENTED_EDGE('',*,*,#47508,.F.);
#64749=ORIENTED_EDGE('',*,*,#47509,.T.);
#64750=ORIENTED_EDGE('',*,*,#46585,.F.);
#64751=ORIENTED_EDGE('',*,*,#47506,.F.);
#64752=ORIENTED_EDGE('',*,*,#47510,.F.);
#64753=ORIENTED_EDGE('',*,*,#47511,.T.);
#64754=ORIENTED_EDGE('',*,*,#46588,.F.);
#64755=ORIENTED_EDGE('',*,*,#47509,.F.);
#64756=ORIENTED_EDGE('',*,*,#47512,.F.);
#64757=ORIENTED_EDGE('',*,*,#47513,.T.);
#64758=ORIENTED_EDGE('',*,*,#46590,.F.);
#64759=ORIENTED_EDGE('',*,*,#47511,.F.);
#64760=ORIENTED_EDGE('',*,*,#47514,.F.);
#64761=ORIENTED_EDGE('',*,*,#47513,.F.);
#64762=ORIENTED_EDGE('',*,*,#47515,.F.);
#64763=ORIENTED_EDGE('',*,*,#47516,.F.);
#64764=ORIENTED_EDGE('',*,*,#46593,.F.);
#64765=ORIENTED_EDGE('',*,*,#47516,.T.);
#64766=ORIENTED_EDGE('',*,*,#47517,.F.);
#64767=ORIENTED_EDGE('',*,*,#47518,.F.);
#64768=ORIENTED_EDGE('',*,*,#46609,.F.);
#64769=ORIENTED_EDGE('',*,*,#47518,.T.);
#64770=ORIENTED_EDGE('',*,*,#47519,.F.);
#64771=ORIENTED_EDGE('',*,*,#47520,.F.);
#64772=ORIENTED_EDGE('',*,*,#47521,.F.);
#64773=ORIENTED_EDGE('',*,*,#47522,.T.);
#64774=ORIENTED_EDGE('',*,*,#47523,.F.);
#64775=ORIENTED_EDGE('',*,*,#47524,.F.);
#64776=ORIENTED_EDGE('',*,*,#47505,.F.);
#64777=ORIENTED_EDGE('',*,*,#47524,.T.);
#64778=ORIENTED_EDGE('',*,*,#47525,.F.);
#64779=ORIENTED_EDGE('',*,*,#47526,.F.);
#64780=ORIENTED_EDGE('',*,*,#46599,.F.);
#64781=ORIENTED_EDGE('',*,*,#47526,.T.);
#64782=ORIENTED_EDGE('',*,*,#47527,.F.);
#64783=ORIENTED_EDGE('',*,*,#47528,.F.);
#64784=ORIENTED_EDGE('',*,*,#46602,.F.);
#64785=ORIENTED_EDGE('',*,*,#47529,.F.);
#64786=ORIENTED_EDGE('',*,*,#46788,.T.);
#64787=ORIENTED_EDGE('',*,*,#46603,.F.);
#64788=ORIENTED_EDGE('',*,*,#47528,.T.);
#64789=ORIENTED_EDGE('',*,*,#47530,.T.);
#64790=ORIENTED_EDGE('',*,*,#47531,.F.);
#64791=ORIENTED_EDGE('',*,*,#46785,.F.);
#64792=ORIENTED_EDGE('',*,*,#47532,.F.);
#64793=ORIENTED_EDGE('',*,*,#47533,.T.);
#64794=ORIENTED_EDGE('',*,*,#47507,.T.);
#64795=ORIENTED_EDGE('',*,*,#46783,.F.);
#64796=ORIENTED_EDGE('',*,*,#47530,.F.);
#64797=ORIENTED_EDGE('',*,*,#47533,.F.);
#64798=ORIENTED_EDGE('',*,*,#47534,.F.);
#64799=ORIENTED_EDGE('',*,*,#47535,.F.);
#64800=ORIENTED_EDGE('',*,*,#47390,.T.);
#64801=ORIENTED_EDGE('',*,*,#46606,.F.);
#64802=ORIENTED_EDGE('',*,*,#47536,.F.);
#64803=ORIENTED_EDGE('',*,*,#47391,.T.);
#64804=ORIENTED_EDGE('',*,*,#47537,.F.);
#64805=ORIENTED_EDGE('',*,*,#47538,.F.);
#64806=ORIENTED_EDGE('',*,*,#47539,.F.);
#64807=ORIENTED_EDGE('',*,*,#47520,.T.);
#64808=ORIENTED_EDGE('',*,*,#47540,.F.);
#64809=ORIENTED_EDGE('',*,*,#47541,.F.);
#64810=ORIENTED_EDGE('',*,*,#47542,.F.);
#64811=ORIENTED_EDGE('',*,*,#46610,.F.);
#64812=ORIENTED_EDGE('',*,*,#47521,.T.);
#64813=ORIENTED_EDGE('',*,*,#47543,.F.);
#64814=ORIENTED_EDGE('',*,*,#47536,.T.);
#64815=ORIENTED_EDGE('',*,*,#47544,.T.);
#64816=ORIENTED_EDGE('',*,*,#46627,.F.);
#64817=ORIENTED_EDGE('',*,*,#47545,.F.);
#64818=ORIENTED_EDGE('',*,*,#47546,.F.);
#64819=ORIENTED_EDGE('',*,*,#47547,.T.);
#64820=ORIENTED_EDGE('',*,*,#46624,.F.);
#64821=ORIENTED_EDGE('',*,*,#47544,.F.);
#64822=ORIENTED_EDGE('',*,*,#47548,.F.);
#64823=ORIENTED_EDGE('',*,*,#47549,.T.);
#64824=ORIENTED_EDGE('',*,*,#46620,.F.);
#64825=ORIENTED_EDGE('',*,*,#47547,.F.);
#64826=ORIENTED_EDGE('',*,*,#47550,.F.);
#64827=ORIENTED_EDGE('',*,*,#47551,.T.);
#64828=ORIENTED_EDGE('',*,*,#47552,.F.);
#64829=ORIENTED_EDGE('',*,*,#47549,.F.);
#64830=ORIENTED_EDGE('',*,*,#47553,.F.);
#64831=ORIENTED_EDGE('',*,*,#47554,.T.);
#64832=ORIENTED_EDGE('',*,*,#47555,.F.);
#64833=ORIENTED_EDGE('',*,*,#47556,.F.);
#64834=ORIENTED_EDGE('',*,*,#46726,.F.);
#64835=ORIENTED_EDGE('',*,*,#47556,.T.);
#64836=ORIENTED_EDGE('',*,*,#47557,.F.);
#64837=ORIENTED_EDGE('',*,*,#47558,.F.);
#64838=ORIENTED_EDGE('',*,*,#46613,.F.);
#64839=ORIENTED_EDGE('',*,*,#47559,.F.);
#64840=ORIENTED_EDGE('',*,*,#46920,.T.);
#64841=ORIENTED_EDGE('',*,*,#46616,.F.);
#64842=ORIENTED_EDGE('',*,*,#47558,.T.);
#64843=ORIENTED_EDGE('',*,*,#47560,.T.);
#64844=ORIENTED_EDGE('',*,*,#47561,.F.);
#64845=ORIENTED_EDGE('',*,*,#46917,.F.);
#64846=ORIENTED_EDGE('',*,*,#47562,.F.);
#64847=ORIENTED_EDGE('',*,*,#47545,.T.);
#64848=ORIENTED_EDGE('',*,*,#46915,.F.);
#64849=ORIENTED_EDGE('',*,*,#47560,.F.);
#64850=ORIENTED_EDGE('',*,*,#47563,.F.);
#64851=ORIENTED_EDGE('',*,*,#47564,.T.);
#64852=ORIENTED_EDGE('',*,*,#47565,.F.);
#64853=ORIENTED_EDGE('',*,*,#47551,.F.);
#64854=ORIENTED_EDGE('',*,*,#47566,.F.);
#64855=ORIENTED_EDGE('',*,*,#46621,.F.);
#64856=ORIENTED_EDGE('',*,*,#47552,.T.);
#64857=ORIENTED_EDGE('',*,*,#47567,.F.);
#64858=ORIENTED_EDGE('',*,*,#47568,.T.);
#64859=ORIENTED_EDGE('',*,*,#47569,.T.);
#64860=ORIENTED_EDGE('',*,*,#47568,.F.);
#64861=ORIENTED_EDGE('',*,*,#47570,.F.);
#64862=ORIENTED_EDGE('',*,*,#47571,.F.);
#64863=ORIENTED_EDGE('',*,*,#47572,.T.);
#64864=ORIENTED_EDGE('',*,*,#46622,.F.);
#64865=ORIENTED_EDGE('',*,*,#47569,.F.);
#64866=ORIENTED_EDGE('',*,*,#47573,.F.);
#64867=ORIENTED_EDGE('',*,*,#47572,.F.);
#64868=ORIENTED_EDGE('',*,*,#47574,.F.);
#64869=ORIENTED_EDGE('',*,*,#47575,.F.);
#64870=ORIENTED_EDGE('',*,*,#46625,.F.);
#64871=ORIENTED_EDGE('',*,*,#47575,.T.);
#64872=ORIENTED_EDGE('',*,*,#47576,.F.);
#64873=ORIENTED_EDGE('',*,*,#47577,.F.);
#64874=ORIENTED_EDGE('',*,*,#46628,.F.);
#64875=ORIENTED_EDGE('',*,*,#47577,.T.);
#64876=ORIENTED_EDGE('',*,*,#47578,.F.);
#64877=ORIENTED_EDGE('',*,*,#47579,.F.);
#64878=ORIENTED_EDGE('',*,*,#46916,.F.);
#64879=ORIENTED_EDGE('',*,*,#47579,.T.);
#64880=ORIENTED_EDGE('',*,*,#47580,.F.);
#64881=ORIENTED_EDGE('',*,*,#46911,.F.);
#64882=ORIENTED_EDGE('',*,*,#47581,.F.);
#64883=ORIENTED_EDGE('',*,*,#46631,.F.);
#64884=ORIENTED_EDGE('',*,*,#46912,.T.);
#64885=ORIENTED_EDGE('',*,*,#47582,.F.);
#64886=ORIENTED_EDGE('',*,*,#47583,.F.);
#64887=ORIENTED_EDGE('',*,*,#47583,.T.);
#64888=ORIENTED_EDGE('',*,*,#47584,.F.);
#64889=ORIENTED_EDGE('',*,*,#47585,.F.);
#64890=ORIENTED_EDGE('',*,*,#46638,.F.);
#64891=ORIENTED_EDGE('',*,*,#47585,.T.);
#64892=ORIENTED_EDGE('',*,*,#47586,.F.);
#64893=ORIENTED_EDGE('',*,*,#47587,.F.);
#64894=ORIENTED_EDGE('',*,*,#46636,.F.);
#64895=ORIENTED_EDGE('',*,*,#47570,.T.);
#64896=ORIENTED_EDGE('',*,*,#47588,.F.);
#64897=ORIENTED_EDGE('',*,*,#47589,.F.);
#64898=ORIENTED_EDGE('',*,*,#47590,.F.);
#64899=ORIENTED_EDGE('',*,*,#47587,.T.);
#64900=ORIENTED_EDGE('',*,*,#47591,.F.);
#64901=ORIENTED_EDGE('',*,*,#47592,.F.);
#64902=ORIENTED_EDGE('',*,*,#47593,.F.);
#64903=ORIENTED_EDGE('',*,*,#47594,.F.);
#64904=ORIENTED_EDGE('',*,*,#47595,.T.);
#64905=ORIENTED_EDGE('',*,*,#46633,.F.);
#64906=ORIENTED_EDGE('',*,*,#47593,.T.);
#64907=ORIENTED_EDGE('',*,*,#47596,.T.);
#64908=ORIENTED_EDGE('',*,*,#47597,.F.);
#64909=ORIENTED_EDGE('',*,*,#47598,.F.);
#64910=ORIENTED_EDGE('',*,*,#47595,.F.);
#64911=ORIENTED_EDGE('',*,*,#47598,.T.);
#64912=ORIENTED_EDGE('',*,*,#47599,.F.);
#64913=ORIENTED_EDGE('',*,*,#47600,.F.);
#64914=ORIENTED_EDGE('',*,*,#46634,.F.);
#64915=ORIENTED_EDGE('',*,*,#47601,.F.);
#64916=ORIENTED_EDGE('',*,*,#46904,.T.);
#64917=ORIENTED_EDGE('',*,*,#46639,.F.);
#64918=ORIENTED_EDGE('',*,*,#46637,.F.);
#64919=ORIENTED_EDGE('',*,*,#47600,.T.);
#64920=ORIENTED_EDGE('',*,*,#46905,.T.);
#64921=ORIENTED_EDGE('',*,*,#47602,.F.);
#64922=ORIENTED_EDGE('',*,*,#47603,.F.);
#64923=ORIENTED_EDGE('',*,*,#47604,.F.);
#64924=ORIENTED_EDGE('',*,*,#47603,.T.);
#64925=ORIENTED_EDGE('',*,*,#47605,.F.);
#64926=ORIENTED_EDGE('',*,*,#47606,.F.);
#64927=ORIENTED_EDGE('',*,*,#46901,.F.);
#64928=ORIENTED_EDGE('',*,*,#47606,.T.);
#64929=ORIENTED_EDGE('',*,*,#47607,.F.);
#64930=ORIENTED_EDGE('',*,*,#47608,.F.);
#64931=ORIENTED_EDGE('',*,*,#46649,.F.);
#64932=ORIENTED_EDGE('',*,*,#47608,.T.);
#64933=ORIENTED_EDGE('',*,*,#47609,.F.);
#64934=ORIENTED_EDGE('',*,*,#47610,.F.);
#64935=ORIENTED_EDGE('',*,*,#46646,.F.);
#64936=ORIENTED_EDGE('',*,*,#47610,.T.);
#64937=ORIENTED_EDGE('',*,*,#47611,.F.);
#64938=ORIENTED_EDGE('',*,*,#47612,.F.);
#64939=ORIENTED_EDGE('',*,*,#46644,.F.);
#64940=ORIENTED_EDGE('',*,*,#47613,.T.);
#64941=ORIENTED_EDGE('',*,*,#47614,.F.);
#64942=ORIENTED_EDGE('',*,*,#47612,.T.);
#64943=ORIENTED_EDGE('',*,*,#47615,.F.);
#64944=ORIENTED_EDGE('',*,*,#47616,.T.);
#64945=ORIENTED_EDGE('',*,*,#47617,.F.);
#64946=ORIENTED_EDGE('',*,*,#47613,.F.);
#64947=ORIENTED_EDGE('',*,*,#47618,.F.);
#64948=ORIENTED_EDGE('',*,*,#46641,.F.);
#64949=ORIENTED_EDGE('',*,*,#47614,.T.);
#64950=ORIENTED_EDGE('',*,*,#47619,.F.);
#64951=ORIENTED_EDGE('',*,*,#47620,.T.);
#64952=ORIENTED_EDGE('',*,*,#47621,.T.);
#64953=ORIENTED_EDGE('',*,*,#47620,.F.);
#64954=ORIENTED_EDGE('',*,*,#47622,.F.);
#64955=ORIENTED_EDGE('',*,*,#47623,.F.);
#64956=ORIENTED_EDGE('',*,*,#47624,.T.);
#64957=ORIENTED_EDGE('',*,*,#46642,.F.);
#64958=ORIENTED_EDGE('',*,*,#47621,.F.);
#64959=ORIENTED_EDGE('',*,*,#47625,.F.);
#64960=ORIENTED_EDGE('',*,*,#47626,.T.);
#64961=ORIENTED_EDGE('',*,*,#46647,.F.);
#64962=ORIENTED_EDGE('',*,*,#47624,.F.);
#64963=ORIENTED_EDGE('',*,*,#47627,.F.);
#64964=ORIENTED_EDGE('',*,*,#47628,.T.);
#64965=ORIENTED_EDGE('',*,*,#46650,.F.);
#64966=ORIENTED_EDGE('',*,*,#47626,.F.);
#64967=ORIENTED_EDGE('',*,*,#47629,.F.);
#64968=ORIENTED_EDGE('',*,*,#47630,.T.);
#64969=ORIENTED_EDGE('',*,*,#46902,.F.);
#64970=ORIENTED_EDGE('',*,*,#47628,.F.);
#64971=ORIENTED_EDGE('',*,*,#47631,.F.);
#64972=ORIENTED_EDGE('',*,*,#46898,.T.);
#64973=ORIENTED_EDGE('',*,*,#47632,.F.);
#64974=ORIENTED_EDGE('',*,*,#47630,.F.);
#64975=ORIENTED_EDGE('',*,*,#47633,.F.);
#64976=ORIENTED_EDGE('',*,*,#46653,.F.);
#64977=ORIENTED_EDGE('',*,*,#46899,.T.);
#64978=ORIENTED_EDGE('',*,*,#47634,.F.);
#64979=ORIENTED_EDGE('',*,*,#47635,.T.);
#64980=ORIENTED_EDGE('',*,*,#47622,.T.);
#64981=ORIENTED_EDGE('',*,*,#47636,.F.);
#64982=ORIENTED_EDGE('',*,*,#47637,.F.);
#64983=ORIENTED_EDGE('',*,*,#47638,.F.);
#64984=ORIENTED_EDGE('',*,*,#47639,.T.);
#64985=ORIENTED_EDGE('',*,*,#47640,.F.);
#64986=ORIENTED_EDGE('',*,*,#47635,.F.);
#64987=ORIENTED_EDGE('',*,*,#47641,.F.);
#64988=ORIENTED_EDGE('',*,*,#47642,.T.);
#64989=ORIENTED_EDGE('',*,*,#47643,.T.);
#64990=ORIENTED_EDGE('',*,*,#46654,.T.);
#64991=ORIENTED_EDGE('',*,*,#47640,.T.);
#64992=ORIENTED_EDGE('',*,*,#47644,.T.);
#64993=ORIENTED_EDGE('',*,*,#47645,.F.);
#64994=ORIENTED_EDGE('',*,*,#47646,.F.);
#64995=ORIENTED_EDGE('',*,*,#47643,.F.);
#64996=ORIENTED_EDGE('',*,*,#47647,.F.);
#64997=ORIENTED_EDGE('',*,*,#46892,.T.);
#64998=ORIENTED_EDGE('',*,*,#46651,.F.);
#64999=ORIENTED_EDGE('',*,*,#47646,.T.);
#65000=ORIENTED_EDGE('',*,*,#46893,.T.);
#65001=ORIENTED_EDGE('',*,*,#47648,.F.);
#65002=ORIENTED_EDGE('',*,*,#47649,.F.);
#65003=ORIENTED_EDGE('',*,*,#47650,.F.);
#65004=ORIENTED_EDGE('',*,*,#47649,.T.);
#65005=ORIENTED_EDGE('',*,*,#47651,.F.);
#65006=ORIENTED_EDGE('',*,*,#47652,.F.);
#65007=ORIENTED_EDGE('',*,*,#46889,.F.);
#65008=ORIENTED_EDGE('',*,*,#47652,.T.);
#65009=ORIENTED_EDGE('',*,*,#47653,.F.);
#65010=ORIENTED_EDGE('',*,*,#47654,.F.);
#65011=ORIENTED_EDGE('',*,*,#46663,.F.);
#65012=ORIENTED_EDGE('',*,*,#47654,.T.);
#65013=ORIENTED_EDGE('',*,*,#47655,.F.);
#65014=ORIENTED_EDGE('',*,*,#47656,.F.);
#65015=ORIENTED_EDGE('',*,*,#46660,.F.);
#65016=ORIENTED_EDGE('',*,*,#47656,.T.);
#65017=ORIENTED_EDGE('',*,*,#47657,.F.);
#65018=ORIENTED_EDGE('',*,*,#47658,.F.);
#65019=ORIENTED_EDGE('',*,*,#46656,.F.);
#65020=ORIENTED_EDGE('',*,*,#47658,.T.);
#65021=ORIENTED_EDGE('',*,*,#47659,.F.);
#65022=ORIENTED_EDGE('',*,*,#47660,.F.);
#65023=ORIENTED_EDGE('',*,*,#47661,.F.);
#65024=ORIENTED_EDGE('',*,*,#47660,.T.);
#65025=ORIENTED_EDGE('',*,*,#47662,.F.);
#65026=ORIENTED_EDGE('',*,*,#47663,.F.);
#65027=ORIENTED_EDGE('',*,*,#47664,.F.);
#65028=ORIENTED_EDGE('',*,*,#46657,.F.);
#65029=ORIENTED_EDGE('',*,*,#47661,.T.);
#65030=ORIENTED_EDGE('',*,*,#47665,.F.);
#65031=ORIENTED_EDGE('',*,*,#47666,.T.);
#65032=ORIENTED_EDGE('',*,*,#47667,.T.);
#65033=ORIENTED_EDGE('',*,*,#47666,.F.);
#65034=ORIENTED_EDGE('',*,*,#47668,.F.);
#65035=ORIENTED_EDGE('',*,*,#47669,.F.);
#65036=ORIENTED_EDGE('',*,*,#47670,.T.);
#65037=ORIENTED_EDGE('',*,*,#46658,.F.);
#65038=ORIENTED_EDGE('',*,*,#47667,.F.);
#65039=ORIENTED_EDGE('',*,*,#47671,.F.);
#65040=ORIENTED_EDGE('',*,*,#47672,.T.);
#65041=ORIENTED_EDGE('',*,*,#46661,.F.);
#65042=ORIENTED_EDGE('',*,*,#47670,.F.);
#65043=ORIENTED_EDGE('',*,*,#47673,.F.);
#65044=ORIENTED_EDGE('',*,*,#47674,.T.);
#65045=ORIENTED_EDGE('',*,*,#46664,.F.);
#65046=ORIENTED_EDGE('',*,*,#47672,.F.);
#65047=ORIENTED_EDGE('',*,*,#47675,.F.);
#65048=ORIENTED_EDGE('',*,*,#47676,.T.);
#65049=ORIENTED_EDGE('',*,*,#46890,.F.);
#65050=ORIENTED_EDGE('',*,*,#47674,.F.);
#65051=ORIENTED_EDGE('',*,*,#47677,.F.);
#65052=ORIENTED_EDGE('',*,*,#46886,.T.);
#65053=ORIENTED_EDGE('',*,*,#47678,.F.);
#65054=ORIENTED_EDGE('',*,*,#47676,.F.);
#65055=ORIENTED_EDGE('',*,*,#47679,.F.);
#65056=ORIENTED_EDGE('',*,*,#46667,.F.);
#65057=ORIENTED_EDGE('',*,*,#46887,.T.);
#65058=ORIENTED_EDGE('',*,*,#47680,.F.);
#65059=ORIENTED_EDGE('',*,*,#47681,.T.);
#65060=ORIENTED_EDGE('',*,*,#47668,.T.);
#65061=ORIENTED_EDGE('',*,*,#47682,.F.);
#65062=ORIENTED_EDGE('',*,*,#47683,.F.);
#65063=ORIENTED_EDGE('',*,*,#47684,.F.);
#65064=ORIENTED_EDGE('',*,*,#47685,.T.);
#65065=ORIENTED_EDGE('',*,*,#47686,.F.);
#65066=ORIENTED_EDGE('',*,*,#47681,.F.);
#65067=ORIENTED_EDGE('',*,*,#47687,.F.);
#65068=ORIENTED_EDGE('',*,*,#47688,.T.);
#65069=ORIENTED_EDGE('',*,*,#47689,.T.);
#65070=ORIENTED_EDGE('',*,*,#46668,.T.);
#65071=ORIENTED_EDGE('',*,*,#47686,.T.);
#65072=ORIENTED_EDGE('',*,*,#47690,.T.);
#65073=ORIENTED_EDGE('',*,*,#47691,.F.);
#65074=ORIENTED_EDGE('',*,*,#47692,.F.);
#65075=ORIENTED_EDGE('',*,*,#47689,.F.);
#65076=ORIENTED_EDGE('',*,*,#47693,.F.);
#65077=ORIENTED_EDGE('',*,*,#46880,.T.);
#65078=ORIENTED_EDGE('',*,*,#46665,.F.);
#65079=ORIENTED_EDGE('',*,*,#47692,.T.);
#65080=ORIENTED_EDGE('',*,*,#46881,.T.);
#65081=ORIENTED_EDGE('',*,*,#47694,.F.);
#65082=ORIENTED_EDGE('',*,*,#47695,.F.);
#65083=ORIENTED_EDGE('',*,*,#47696,.F.);
#65084=ORIENTED_EDGE('',*,*,#47695,.T.);
#65085=ORIENTED_EDGE('',*,*,#47697,.F.);
#65086=ORIENTED_EDGE('',*,*,#47698,.F.);
#65087=ORIENTED_EDGE('',*,*,#46877,.F.);
#65088=ORIENTED_EDGE('',*,*,#47698,.T.);
#65089=ORIENTED_EDGE('',*,*,#47699,.F.);
#65090=ORIENTED_EDGE('',*,*,#47700,.F.);
#65091=ORIENTED_EDGE('',*,*,#46677,.F.);
#65092=ORIENTED_EDGE('',*,*,#47700,.T.);
#65093=ORIENTED_EDGE('',*,*,#47701,.F.);
#65094=ORIENTED_EDGE('',*,*,#47702,.F.);
#65095=ORIENTED_EDGE('',*,*,#46674,.F.);
#65096=ORIENTED_EDGE('',*,*,#47702,.T.);
#65097=ORIENTED_EDGE('',*,*,#47703,.F.);
#65098=ORIENTED_EDGE('',*,*,#47704,.F.);
#65099=ORIENTED_EDGE('',*,*,#46670,.F.);
#65100=ORIENTED_EDGE('',*,*,#47704,.T.);
#65101=ORIENTED_EDGE('',*,*,#47705,.F.);
#65102=ORIENTED_EDGE('',*,*,#47706,.F.);
#65103=ORIENTED_EDGE('',*,*,#47707,.F.);
#65104=ORIENTED_EDGE('',*,*,#47706,.T.);
#65105=ORIENTED_EDGE('',*,*,#47708,.F.);
#65106=ORIENTED_EDGE('',*,*,#47709,.F.);
#65107=ORIENTED_EDGE('',*,*,#47710,.F.);
#65108=ORIENTED_EDGE('',*,*,#46671,.F.);
#65109=ORIENTED_EDGE('',*,*,#47707,.T.);
#65110=ORIENTED_EDGE('',*,*,#47711,.F.);
#65111=ORIENTED_EDGE('',*,*,#47712,.T.);
#65112=ORIENTED_EDGE('',*,*,#47713,.T.);
#65113=ORIENTED_EDGE('',*,*,#47712,.F.);
#65114=ORIENTED_EDGE('',*,*,#47714,.F.);
#65115=ORIENTED_EDGE('',*,*,#47715,.F.);
#65116=ORIENTED_EDGE('',*,*,#47716,.T.);
#65117=ORIENTED_EDGE('',*,*,#46672,.F.);
#65118=ORIENTED_EDGE('',*,*,#47713,.F.);
#65119=ORIENTED_EDGE('',*,*,#47717,.F.);
#65120=ORIENTED_EDGE('',*,*,#47718,.T.);
#65121=ORIENTED_EDGE('',*,*,#46675,.F.);
#65122=ORIENTED_EDGE('',*,*,#47716,.F.);
#65123=ORIENTED_EDGE('',*,*,#47719,.F.);
#65124=ORIENTED_EDGE('',*,*,#47720,.T.);
#65125=ORIENTED_EDGE('',*,*,#46678,.F.);
#65126=ORIENTED_EDGE('',*,*,#47718,.F.);
#65127=ORIENTED_EDGE('',*,*,#47721,.F.);
#65128=ORIENTED_EDGE('',*,*,#47722,.T.);
#65129=ORIENTED_EDGE('',*,*,#46878,.F.);
#65130=ORIENTED_EDGE('',*,*,#47720,.F.);
#65131=ORIENTED_EDGE('',*,*,#47723,.F.);
#65132=ORIENTED_EDGE('',*,*,#46874,.T.);
#65133=ORIENTED_EDGE('',*,*,#47724,.F.);
#65134=ORIENTED_EDGE('',*,*,#47722,.F.);
#65135=ORIENTED_EDGE('',*,*,#47725,.F.);
#65136=ORIENTED_EDGE('',*,*,#46681,.F.);
#65137=ORIENTED_EDGE('',*,*,#46875,.T.);
#65138=ORIENTED_EDGE('',*,*,#47726,.F.);
#65139=ORIENTED_EDGE('',*,*,#47727,.F.);
#65140=ORIENTED_EDGE('',*,*,#47714,.T.);
#65141=ORIENTED_EDGE('',*,*,#47728,.F.);
#65142=ORIENTED_EDGE('',*,*,#47729,.F.);
#65143=ORIENTED_EDGE('',*,*,#47730,.F.);
#65144=ORIENTED_EDGE('',*,*,#47727,.T.);
#65145=ORIENTED_EDGE('',*,*,#47731,.F.);
#65146=ORIENTED_EDGE('',*,*,#47732,.F.);
#65147=ORIENTED_EDGE('',*,*,#47733,.F.);
#65148=ORIENTED_EDGE('',*,*,#47734,.T.);
#65149=ORIENTED_EDGE('',*,*,#47735,.T.);
#65150=ORIENTED_EDGE('',*,*,#46682,.T.);
#65151=ORIENTED_EDGE('',*,*,#47733,.T.);
#65152=ORIENTED_EDGE('',*,*,#47736,.T.);
#65153=ORIENTED_EDGE('',*,*,#47737,.F.);
#65154=ORIENTED_EDGE('',*,*,#47738,.F.);
#65155=ORIENTED_EDGE('',*,*,#47735,.F.);
#65156=ORIENTED_EDGE('',*,*,#47739,.F.);
#65157=ORIENTED_EDGE('',*,*,#46868,.T.);
#65158=ORIENTED_EDGE('',*,*,#46679,.F.);
#65159=ORIENTED_EDGE('',*,*,#47738,.T.);
#65160=ORIENTED_EDGE('',*,*,#46869,.T.);
#65161=ORIENTED_EDGE('',*,*,#47740,.F.);
#65162=ORIENTED_EDGE('',*,*,#47741,.F.);
#65163=ORIENTED_EDGE('',*,*,#47742,.F.);
#65164=ORIENTED_EDGE('',*,*,#47741,.T.);
#65165=ORIENTED_EDGE('',*,*,#47743,.F.);
#65166=ORIENTED_EDGE('',*,*,#47744,.F.);
#65167=ORIENTED_EDGE('',*,*,#46865,.F.);
#65168=ORIENTED_EDGE('',*,*,#47744,.T.);
#65169=ORIENTED_EDGE('',*,*,#47745,.F.);
#65170=ORIENTED_EDGE('',*,*,#47746,.F.);
#65171=ORIENTED_EDGE('',*,*,#46691,.F.);
#65172=ORIENTED_EDGE('',*,*,#47746,.T.);
#65173=ORIENTED_EDGE('',*,*,#47747,.F.);
#65174=ORIENTED_EDGE('',*,*,#47748,.F.);
#65175=ORIENTED_EDGE('',*,*,#46688,.F.);
#65176=ORIENTED_EDGE('',*,*,#47748,.T.);
#65177=ORIENTED_EDGE('',*,*,#47749,.F.);
#65178=ORIENTED_EDGE('',*,*,#47750,.F.);
#65179=ORIENTED_EDGE('',*,*,#46684,.F.);
#65180=ORIENTED_EDGE('',*,*,#47750,.T.);
#65181=ORIENTED_EDGE('',*,*,#47751,.F.);
#65182=ORIENTED_EDGE('',*,*,#47752,.F.);
#65183=ORIENTED_EDGE('',*,*,#47753,.F.);
#65184=ORIENTED_EDGE('',*,*,#47752,.T.);
#65185=ORIENTED_EDGE('',*,*,#47754,.F.);
#65186=ORIENTED_EDGE('',*,*,#47755,.F.);
#65187=ORIENTED_EDGE('',*,*,#47756,.F.);
#65188=ORIENTED_EDGE('',*,*,#46685,.F.);
#65189=ORIENTED_EDGE('',*,*,#47753,.T.);
#65190=ORIENTED_EDGE('',*,*,#47757,.F.);
#65191=ORIENTED_EDGE('',*,*,#47758,.T.);
#65192=ORIENTED_EDGE('',*,*,#47759,.T.);
#65193=ORIENTED_EDGE('',*,*,#47758,.F.);
#65194=ORIENTED_EDGE('',*,*,#47760,.F.);
#65195=ORIENTED_EDGE('',*,*,#47761,.F.);
#65196=ORIENTED_EDGE('',*,*,#47762,.T.);
#65197=ORIENTED_EDGE('',*,*,#46686,.F.);
#65198=ORIENTED_EDGE('',*,*,#47759,.F.);
#65199=ORIENTED_EDGE('',*,*,#47763,.F.);
#65200=ORIENTED_EDGE('',*,*,#47762,.F.);
#65201=ORIENTED_EDGE('',*,*,#47764,.F.);
#65202=ORIENTED_EDGE('',*,*,#47765,.F.);
#65203=ORIENTED_EDGE('',*,*,#46689,.F.);
#65204=ORIENTED_EDGE('',*,*,#47765,.T.);
#65205=ORIENTED_EDGE('',*,*,#47766,.F.);
#65206=ORIENTED_EDGE('',*,*,#47767,.F.);
#65207=ORIENTED_EDGE('',*,*,#46692,.F.);
#65208=ORIENTED_EDGE('',*,*,#47767,.T.);
#65209=ORIENTED_EDGE('',*,*,#47768,.F.);
#65210=ORIENTED_EDGE('',*,*,#47769,.F.);
#65211=ORIENTED_EDGE('',*,*,#46866,.F.);
#65212=ORIENTED_EDGE('',*,*,#47769,.T.);
#65213=ORIENTED_EDGE('',*,*,#47770,.F.);
#65214=ORIENTED_EDGE('',*,*,#46861,.F.);
#65215=ORIENTED_EDGE('',*,*,#47771,.F.);
#65216=ORIENTED_EDGE('',*,*,#46695,.T.);
#65217=ORIENTED_EDGE('',*,*,#46862,.T.);
#65218=ORIENTED_EDGE('',*,*,#47772,.F.);
#65219=ORIENTED_EDGE('',*,*,#47773,.F.);
#65220=ORIENTED_EDGE('',*,*,#46702,.F.);
#65221=ORIENTED_EDGE('',*,*,#47773,.T.);
#65222=ORIENTED_EDGE('',*,*,#47774,.F.);
#65223=ORIENTED_EDGE('',*,*,#47775,.F.);
#65224=ORIENTED_EDGE('',*,*,#46699,.F.);
#65225=ORIENTED_EDGE('',*,*,#47760,.T.);
#65226=ORIENTED_EDGE('',*,*,#47776,.F.);
#65227=ORIENTED_EDGE('',*,*,#47777,.F.);
#65228=ORIENTED_EDGE('',*,*,#47778,.F.);
#65229=ORIENTED_EDGE('',*,*,#47775,.T.);
#65230=ORIENTED_EDGE('',*,*,#47779,.F.);
#65231=ORIENTED_EDGE('',*,*,#47780,.F.);
#65232=ORIENTED_EDGE('',*,*,#47781,.F.);
#65233=ORIENTED_EDGE('',*,*,#47782,.F.);
#65234=ORIENTED_EDGE('',*,*,#47783,.T.);
#65235=ORIENTED_EDGE('',*,*,#46696,.F.);
#65236=ORIENTED_EDGE('',*,*,#47781,.T.);
#65237=ORIENTED_EDGE('',*,*,#47784,.T.);
#65238=ORIENTED_EDGE('',*,*,#47785,.F.);
#65239=ORIENTED_EDGE('',*,*,#47786,.F.);
#65240=ORIENTED_EDGE('',*,*,#47783,.F.);
#65241=ORIENTED_EDGE('',*,*,#47786,.T.);
#65242=ORIENTED_EDGE('',*,*,#47787,.F.);
#65243=ORIENTED_EDGE('',*,*,#47788,.F.);
#65244=ORIENTED_EDGE('',*,*,#46697,.F.);
#65245=ORIENTED_EDGE('',*,*,#47788,.T.);
#65246=ORIENTED_EDGE('',*,*,#47789,.F.);
#65247=ORIENTED_EDGE('',*,*,#47790,.F.);
#65248=ORIENTED_EDGE('',*,*,#46700,.F.);
#65249=ORIENTED_EDGE('',*,*,#47791,.F.);
#65250=ORIENTED_EDGE('',*,*,#46854,.T.);
#65251=ORIENTED_EDGE('',*,*,#46703,.F.);
#65252=ORIENTED_EDGE('',*,*,#47790,.T.);
#65253=ORIENTED_EDGE('',*,*,#46855,.T.);
#65254=ORIENTED_EDGE('',*,*,#47792,.F.);
#65255=ORIENTED_EDGE('',*,*,#47793,.F.);
#65256=ORIENTED_EDGE('',*,*,#47794,.F.);
#65257=ORIENTED_EDGE('',*,*,#47793,.T.);
#65258=ORIENTED_EDGE('',*,*,#47795,.F.);
#65259=ORIENTED_EDGE('',*,*,#47796,.F.);
#65260=ORIENTED_EDGE('',*,*,#46851,.F.);
#65261=ORIENTED_EDGE('',*,*,#47796,.T.);
#65262=ORIENTED_EDGE('',*,*,#47797,.F.);
#65263=ORIENTED_EDGE('',*,*,#47798,.F.);
#65264=ORIENTED_EDGE('',*,*,#46717,.F.);
#65265=ORIENTED_EDGE('',*,*,#47798,.T.);
#65266=ORIENTED_EDGE('',*,*,#47799,.F.);
#65267=ORIENTED_EDGE('',*,*,#47800,.F.);
#65268=ORIENTED_EDGE('',*,*,#46714,.F.);
#65269=ORIENTED_EDGE('',*,*,#47800,.T.);
#65270=ORIENTED_EDGE('',*,*,#47801,.F.);
#65271=ORIENTED_EDGE('',*,*,#47802,.F.);
#65272=ORIENTED_EDGE('',*,*,#46712,.F.);
#65273=ORIENTED_EDGE('',*,*,#47803,.T.);
#65274=ORIENTED_EDGE('',*,*,#47804,.F.);
#65275=ORIENTED_EDGE('',*,*,#47802,.T.);
#65276=ORIENTED_EDGE('',*,*,#47805,.F.);
#65277=ORIENTED_EDGE('',*,*,#47806,.T.);
#65278=ORIENTED_EDGE('',*,*,#47807,.F.);
#65279=ORIENTED_EDGE('',*,*,#47803,.F.);
#65280=ORIENTED_EDGE('',*,*,#47808,.F.);
#65281=ORIENTED_EDGE('',*,*,#46709,.F.);
#65282=ORIENTED_EDGE('',*,*,#47804,.T.);
#65283=ORIENTED_EDGE('',*,*,#47809,.F.);
#65284=ORIENTED_EDGE('',*,*,#47810,.T.);
#65285=ORIENTED_EDGE('',*,*,#47811,.T.);
#65286=ORIENTED_EDGE('',*,*,#47812,.F.);
#65287=ORIENTED_EDGE('',*,*,#47813,.F.);
#65288=ORIENTED_EDGE('',*,*,#46708,.F.);
#65289=ORIENTED_EDGE('',*,*,#47813,.T.);
#65290=ORIENTED_EDGE('',*,*,#47814,.F.);
#65291=ORIENTED_EDGE('',*,*,#47815,.F.);
#65292=ORIENTED_EDGE('',*,*,#46724,.F.);
#65293=ORIENTED_EDGE('',*,*,#47816,.T.);
#65294=ORIENTED_EDGE('',*,*,#47817,.F.);
#65295=ORIENTED_EDGE('',*,*,#47818,.F.);
#65296=ORIENTED_EDGE('',*,*,#47819,.F.);
#65297=ORIENTED_EDGE('',*,*,#47818,.T.);
#65298=ORIENTED_EDGE('',*,*,#47820,.F.);
#65299=ORIENTED_EDGE('',*,*,#47821,.F.);
#65300=ORIENTED_EDGE('',*,*,#47810,.F.);
#65301=ORIENTED_EDGE('',*,*,#47821,.T.);
#65302=ORIENTED_EDGE('',*,*,#47822,.F.);
#65303=ORIENTED_EDGE('',*,*,#47823,.F.);
#65304=ORIENTED_EDGE('',*,*,#46710,.F.);
#65305=ORIENTED_EDGE('',*,*,#47823,.T.);
#65306=ORIENTED_EDGE('',*,*,#47824,.F.);
#65307=ORIENTED_EDGE('',*,*,#47825,.F.);
#65308=ORIENTED_EDGE('',*,*,#46715,.F.);
#65309=ORIENTED_EDGE('',*,*,#47825,.T.);
#65310=ORIENTED_EDGE('',*,*,#47826,.F.);
#65311=ORIENTED_EDGE('',*,*,#47827,.F.);
#65312=ORIENTED_EDGE('',*,*,#46718,.F.);
#65313=ORIENTED_EDGE('',*,*,#47827,.T.);
#65314=ORIENTED_EDGE('',*,*,#47828,.F.);
#65315=ORIENTED_EDGE('',*,*,#47829,.F.);
#65316=ORIENTED_EDGE('',*,*,#46852,.F.);
#65317=ORIENTED_EDGE('',*,*,#47829,.T.);
#65318=ORIENTED_EDGE('',*,*,#47830,.F.);
#65319=ORIENTED_EDGE('',*,*,#46847,.F.);
#65320=ORIENTED_EDGE('',*,*,#47831,.F.);
#65321=ORIENTED_EDGE('',*,*,#46721,.F.);
#65322=ORIENTED_EDGE('',*,*,#46848,.T.);
#65323=ORIENTED_EDGE('',*,*,#47832,.F.);
#65324=ORIENTED_EDGE('',*,*,#47811,.F.);
#65325=ORIENTED_EDGE('',*,*,#47815,.T.);
#65326=ORIENTED_EDGE('',*,*,#47833,.F.);
#65327=ORIENTED_EDGE('',*,*,#47834,.F.);
#65328=ORIENTED_EDGE('',*,*,#47835,.F.);
#65329=ORIENTED_EDGE('',*,*,#47836,.F.);
#65330=ORIENTED_EDGE('',*,*,#47837,.T.);
#65331=ORIENTED_EDGE('',*,*,#46722,.F.);
#65332=ORIENTED_EDGE('',*,*,#47835,.T.);
#65333=ORIENTED_EDGE('',*,*,#47838,.T.);
#65334=ORIENTED_EDGE('',*,*,#47839,.F.);
#65335=ORIENTED_EDGE('',*,*,#47138,.F.);
#65336=ORIENTED_EDGE('',*,*,#47837,.F.);
#65337=ORIENTED_EDGE('',*,*,#47227,.T.);
#65338=ORIENTED_EDGE('',*,*,#47840,.F.);
#65339=ORIENTED_EDGE('',*,*,#47841,.F.);
#65340=ORIENTED_EDGE('',*,*,#47842,.F.);
#65341=ORIENTED_EDGE('',*,*,#47843,.F.);
#65342=ORIENTED_EDGE('',*,*,#47844,.T.);
#65343=ORIENTED_EDGE('',*,*,#46725,.F.);
#65344=ORIENTED_EDGE('',*,*,#47842,.T.);
#65345=ORIENTED_EDGE('',*,*,#47845,.T.);
#65346=ORIENTED_EDGE('',*,*,#47846,.F.);
#65347=ORIENTED_EDGE('',*,*,#47554,.F.);
#65348=ORIENTED_EDGE('',*,*,#47844,.F.);
#65349=ORIENTED_EDGE('',*,*,#47847,.T.);
#65350=ORIENTED_EDGE('',*,*,#47848,.F.);
#65351=ORIENTED_EDGE('',*,*,#47849,.F.);
#65352=ORIENTED_EDGE('',*,*,#47850,.F.);
#65353=ORIENTED_EDGE('',*,*,#47851,.T.);
#65354=ORIENTED_EDGE('',*,*,#47852,.F.);
#65355=ORIENTED_EDGE('',*,*,#47853,.F.);
#65356=ORIENTED_EDGE('',*,*,#47854,.F.);
#65357=ORIENTED_EDGE('',*,*,#47855,.T.);
#65358=ORIENTED_EDGE('',*,*,#47856,.F.);
#65359=ORIENTED_EDGE('',*,*,#47857,.F.);
#65360=ORIENTED_EDGE('',*,*,#47858,.F.);
#65361=ORIENTED_EDGE('',*,*,#47859,.T.);
#65362=ORIENTED_EDGE('',*,*,#47860,.F.);
#65363=ORIENTED_EDGE('',*,*,#47855,.F.);
#65364=ORIENTED_EDGE('',*,*,#47861,.F.);
#65365=ORIENTED_EDGE('',*,*,#47862,.T.);
#65366=ORIENTED_EDGE('',*,*,#47863,.F.);
#65367=ORIENTED_EDGE('',*,*,#47864,.F.);
#65368=ORIENTED_EDGE('',*,*,#47865,.F.);
#65369=ORIENTED_EDGE('',*,*,#47864,.T.);
#65370=ORIENTED_EDGE('',*,*,#47866,.F.);
#65371=ORIENTED_EDGE('',*,*,#47867,.F.);
#65372=ORIENTED_EDGE('',*,*,#47868,.F.);
#65373=ORIENTED_EDGE('',*,*,#47867,.T.);
#65374=ORIENTED_EDGE('',*,*,#47869,.F.);
#65375=ORIENTED_EDGE('',*,*,#47870,.F.);
#65376=ORIENTED_EDGE('',*,*,#47871,.F.);
#65377=ORIENTED_EDGE('',*,*,#47872,.T.);
#65378=ORIENTED_EDGE('',*,*,#47873,.F.);
#65379=ORIENTED_EDGE('',*,*,#47874,.F.);
#65380=ORIENTED_EDGE('',*,*,#47875,.F.);
#65381=ORIENTED_EDGE('',*,*,#47876,.F.);
#65382=ORIENTED_EDGE('',*,*,#47875,.T.);
#65383=ORIENTED_EDGE('',*,*,#47877,.F.);
#65384=ORIENTED_EDGE('',*,*,#47878,.T.);
#65385=ORIENTED_EDGE('',*,*,#47879,.T.);
#65386=ORIENTED_EDGE('',*,*,#47880,.F.);
#65387=ORIENTED_EDGE('',*,*,#47881,.F.);
#65388=ORIENTED_EDGE('',*,*,#47878,.F.);
#65389=ORIENTED_EDGE('',*,*,#47882,.T.);
#65390=ORIENTED_EDGE('',*,*,#47883,.F.);
#65391=ORIENTED_EDGE('',*,*,#47884,.F.);
#65392=ORIENTED_EDGE('',*,*,#47885,.F.);
#65393=ORIENTED_EDGE('',*,*,#47886,.T.);
#65394=ORIENTED_EDGE('',*,*,#46980,.F.);
#65395=ORIENTED_EDGE('',*,*,#47882,.F.);
#65396=ORIENTED_EDGE('',*,*,#47887,.F.);
#65397=ORIENTED_EDGE('',*,*,#47888,.T.);
#65398=ORIENTED_EDGE('',*,*,#47889,.F.);
#65399=ORIENTED_EDGE('',*,*,#47886,.F.);
#65400=ORIENTED_EDGE('',*,*,#47890,.F.);
#65401=ORIENTED_EDGE('',*,*,#47891,.T.);
#65402=ORIENTED_EDGE('',*,*,#47892,.F.);
#65403=ORIENTED_EDGE('',*,*,#47347,.F.);
#65404=ORIENTED_EDGE('',*,*,#47893,.F.);
#65405=ORIENTED_EDGE('',*,*,#47894,.T.);
#65406=ORIENTED_EDGE('',*,*,#47895,.F.);
#65407=ORIENTED_EDGE('',*,*,#47888,.F.);
#65408=ORIENTED_EDGE('',*,*,#47896,.F.);
#65409=ORIENTED_EDGE('',*,*,#46981,.T.);
#65410=ORIENTED_EDGE('',*,*,#47889,.T.);
#65411=ORIENTED_EDGE('',*,*,#47897,.T.);
#65412=ORIENTED_EDGE('',*,*,#47350,.T.);
#65413=ORIENTED_EDGE('',*,*,#47898,.T.);
#65414=ORIENTED_EDGE('',*,*,#47899,.F.);
#65415=ORIENTED_EDGE('',*,*,#47900,.F.);
#65416=ORIENTED_EDGE('',*,*,#47901,.F.);
#65417=ORIENTED_EDGE('',*,*,#47900,.T.);
#65418=ORIENTED_EDGE('',*,*,#47902,.F.);
#65419=ORIENTED_EDGE('',*,*,#47903,.F.);
#65420=ORIENTED_EDGE('',*,*,#46984,.F.);
#65421=ORIENTED_EDGE('',*,*,#47903,.T.);
#65422=ORIENTED_EDGE('',*,*,#47904,.F.);
#65423=ORIENTED_EDGE('',*,*,#47905,.F.);
#65424=ORIENTED_EDGE('',*,*,#46745,.F.);
#65425=ORIENTED_EDGE('',*,*,#47906,.T.);
#65426=ORIENTED_EDGE('',*,*,#47907,.F.);
#65427=ORIENTED_EDGE('',*,*,#47908,.F.);
#65428=ORIENTED_EDGE('',*,*,#47909,.F.);
#65429=ORIENTED_EDGE('',*,*,#47908,.T.);
#65430=ORIENTED_EDGE('',*,*,#47910,.F.);
#65431=ORIENTED_EDGE('',*,*,#47911,.F.);
#65432=ORIENTED_EDGE('',*,*,#46762,.F.);
#65433=ORIENTED_EDGE('',*,*,#47911,.T.);
#65434=ORIENTED_EDGE('',*,*,#47912,.F.);
#65435=ORIENTED_EDGE('',*,*,#47913,.F.);
#65436=ORIENTED_EDGE('',*,*,#46729,.F.);
#65437=ORIENTED_EDGE('',*,*,#47913,.T.);
#65438=ORIENTED_EDGE('',*,*,#47914,.F.);
#65439=ORIENTED_EDGE('',*,*,#47915,.F.);
#65440=ORIENTED_EDGE('',*,*,#47916,.F.);
#65441=ORIENTED_EDGE('',*,*,#47915,.T.);
#65442=ORIENTED_EDGE('',*,*,#47917,.F.);
#65443=ORIENTED_EDGE('',*,*,#47918,.F.);
#65444=ORIENTED_EDGE('',*,*,#47919,.F.);
#65445=ORIENTED_EDGE('',*,*,#46730,.F.);
#65446=ORIENTED_EDGE('',*,*,#47916,.T.);
#65447=ORIENTED_EDGE('',*,*,#47920,.F.);
#65448=ORIENTED_EDGE('',*,*,#47921,.T.);
#65449=ORIENTED_EDGE('',*,*,#47922,.T.);
#65450=ORIENTED_EDGE('',*,*,#47923,.F.);
#65451=ORIENTED_EDGE('',*,*,#47924,.F.);
#65452=ORIENTED_EDGE('',*,*,#46760,.F.);
#65453=ORIENTED_EDGE('',*,*,#47924,.T.);
#65454=ORIENTED_EDGE('',*,*,#47925,.F.);
#65455=ORIENTED_EDGE('',*,*,#47926,.F.);
#65456=ORIENTED_EDGE('',*,*,#46735,.F.);
#65457=ORIENTED_EDGE('',*,*,#47927,.T.);
#65458=ORIENTED_EDGE('',*,*,#47921,.F.);
#65459=ORIENTED_EDGE('',*,*,#47928,.F.);
#65460=ORIENTED_EDGE('',*,*,#47929,.F.);
#65461=ORIENTED_EDGE('',*,*,#47930,.T.);
#65462=ORIENTED_EDGE('',*,*,#46731,.F.);
#65463=ORIENTED_EDGE('',*,*,#47927,.F.);
#65464=ORIENTED_EDGE('',*,*,#47931,.F.);
#65465=ORIENTED_EDGE('',*,*,#47932,.T.);
#65466=ORIENTED_EDGE('',*,*,#46763,.F.);
#65467=ORIENTED_EDGE('',*,*,#47930,.F.);
#65468=ORIENTED_EDGE('',*,*,#47933,.F.);
#65469=ORIENTED_EDGE('',*,*,#47934,.T.);
#65470=ORIENTED_EDGE('',*,*,#47935,.F.);
#65471=ORIENTED_EDGE('',*,*,#47932,.F.);
#65472=ORIENTED_EDGE('',*,*,#47936,.F.);
#65473=ORIENTED_EDGE('',*,*,#47928,.T.);
#65474=ORIENTED_EDGE('',*,*,#47937,.F.);
#65475=ORIENTED_EDGE('',*,*,#47938,.F.);
#65476=ORIENTED_EDGE('',*,*,#47939,.F.);
#65477=ORIENTED_EDGE('',*,*,#47926,.T.);
#65478=ORIENTED_EDGE('',*,*,#47940,.F.);
#65479=ORIENTED_EDGE('',*,*,#47941,.F.);
#65480=ORIENTED_EDGE('',*,*,#47942,.F.);
#65481=ORIENTED_EDGE('',*,*,#47943,.F.);
#65482=ORIENTED_EDGE('',*,*,#47944,.T.);
#65483=ORIENTED_EDGE('',*,*,#46732,.F.);
#65484=ORIENTED_EDGE('',*,*,#47942,.T.);
#65485=ORIENTED_EDGE('',*,*,#47945,.T.);
#65486=ORIENTED_EDGE('',*,*,#47946,.F.);
#65487=ORIENTED_EDGE('',*,*,#47947,.F.);
#65488=ORIENTED_EDGE('',*,*,#47944,.F.);
#65489=ORIENTED_EDGE('',*,*,#47947,.T.);
#65490=ORIENTED_EDGE('',*,*,#47948,.F.);
#65491=ORIENTED_EDGE('',*,*,#47949,.F.);
#65492=ORIENTED_EDGE('',*,*,#46733,.F.);
#65493=ORIENTED_EDGE('',*,*,#47949,.T.);
#65494=ORIENTED_EDGE('',*,*,#47950,.F.);
#65495=ORIENTED_EDGE('',*,*,#47951,.F.);
#65496=ORIENTED_EDGE('',*,*,#46758,.F.);
#65497=ORIENTED_EDGE('',*,*,#47952,.T.);
#65498=ORIENTED_EDGE('',*,*,#47953,.F.);
#65499=ORIENTED_EDGE('',*,*,#47954,.F.);
#65500=ORIENTED_EDGE('',*,*,#47955,.F.);
#65501=ORIENTED_EDGE('',*,*,#47954,.T.);
#65502=ORIENTED_EDGE('',*,*,#47956,.F.);
#65503=ORIENTED_EDGE('',*,*,#47957,.F.);
#65504=ORIENTED_EDGE('',*,*,#46756,.F.);
#65505=ORIENTED_EDGE('',*,*,#47957,.T.);
#65506=ORIENTED_EDGE('',*,*,#47958,.F.);
#65507=ORIENTED_EDGE('',*,*,#47959,.F.);
#65508=ORIENTED_EDGE('',*,*,#46737,.F.);
#65509=ORIENTED_EDGE('',*,*,#47959,.T.);
#65510=ORIENTED_EDGE('',*,*,#47960,.F.);
#65511=ORIENTED_EDGE('',*,*,#47961,.F.);
#65512=ORIENTED_EDGE('',*,*,#47962,.F.);
#65513=ORIENTED_EDGE('',*,*,#47961,.T.);
#65514=ORIENTED_EDGE('',*,*,#47963,.F.);
#65515=ORIENTED_EDGE('',*,*,#47964,.F.);
#65516=ORIENTED_EDGE('',*,*,#47965,.F.);
#65517=ORIENTED_EDGE('',*,*,#46738,.F.);
#65518=ORIENTED_EDGE('',*,*,#47962,.T.);
#65519=ORIENTED_EDGE('',*,*,#47966,.F.);
#65520=ORIENTED_EDGE('',*,*,#47967,.T.);
#65521=ORIENTED_EDGE('',*,*,#47968,.T.);
#65522=ORIENTED_EDGE('',*,*,#47967,.F.);
#65523=ORIENTED_EDGE('',*,*,#47969,.F.);
#65524=ORIENTED_EDGE('',*,*,#47970,.F.);
#65525=ORIENTED_EDGE('',*,*,#47971,.T.);
#65526=ORIENTED_EDGE('',*,*,#46739,.F.);
#65527=ORIENTED_EDGE('',*,*,#47968,.F.);
#65528=ORIENTED_EDGE('',*,*,#47972,.F.);
#65529=ORIENTED_EDGE('',*,*,#47973,.T.);
#65530=ORIENTED_EDGE('',*,*,#46757,.F.);
#65531=ORIENTED_EDGE('',*,*,#47971,.F.);
#65532=ORIENTED_EDGE('',*,*,#47974,.F.);
#65533=ORIENTED_EDGE('',*,*,#47975,.T.);
#65534=ORIENTED_EDGE('',*,*,#47976,.F.);
#65535=ORIENTED_EDGE('',*,*,#47973,.F.);
#65536=ORIENTED_EDGE('',*,*,#47977,.F.);
#65537=ORIENTED_EDGE('',*,*,#47969,.T.);
#65538=ORIENTED_EDGE('',*,*,#47978,.F.);
#65539=ORIENTED_EDGE('',*,*,#47979,.F.);
#65540=ORIENTED_EDGE('',*,*,#47980,.F.);
#65541=ORIENTED_EDGE('',*,*,#47981,.T.);
#65542=ORIENTED_EDGE('',*,*,#47982,.F.);
#65543=ORIENTED_EDGE('',*,*,#47983,.F.);
#65544=ORIENTED_EDGE('',*,*,#47984,.F.);
#65545=ORIENTED_EDGE('',*,*,#47985,.T.);
#65546=ORIENTED_EDGE('',*,*,#47986,.T.);
#65547=ORIENTED_EDGE('',*,*,#47987,.T.);
#65548=ORIENTED_EDGE('',*,*,#47984,.T.);
#65549=ORIENTED_EDGE('',*,*,#47988,.T.);
#65550=ORIENTED_EDGE('',*,*,#47989,.F.);
#65551=ORIENTED_EDGE('',*,*,#47990,.F.);
#65552=ORIENTED_EDGE('',*,*,#47986,.F.);
#65553=ORIENTED_EDGE('',*,*,#47991,.T.);
#65554=ORIENTED_EDGE('',*,*,#47992,.F.);
#65555=ORIENTED_EDGE('',*,*,#47993,.F.);
#65556=ORIENTED_EDGE('',*,*,#47994,.F.);
#65557=ORIENTED_EDGE('',*,*,#47993,.T.);
#65558=ORIENTED_EDGE('',*,*,#47995,.F.);
#65559=ORIENTED_EDGE('',*,*,#47996,.F.);
#65560=ORIENTED_EDGE('',*,*,#46753,.F.);
#65561=ORIENTED_EDGE('',*,*,#47996,.T.);
#65562=ORIENTED_EDGE('',*,*,#47997,.F.);
#65563=ORIENTED_EDGE('',*,*,#47998,.F.);
#65564=ORIENTED_EDGE('',*,*,#46741,.F.);
#65565=ORIENTED_EDGE('',*,*,#47998,.T.);
#65566=ORIENTED_EDGE('',*,*,#47999,.F.);
#65567=ORIENTED_EDGE('',*,*,#48000,.F.);
#65568=ORIENTED_EDGE('',*,*,#48001,.F.);
#65569=ORIENTED_EDGE('',*,*,#48000,.T.);
#65570=ORIENTED_EDGE('',*,*,#48002,.F.);
#65571=ORIENTED_EDGE('',*,*,#48003,.F.);
#65572=ORIENTED_EDGE('',*,*,#48004,.F.);
#65573=ORIENTED_EDGE('',*,*,#46742,.F.);
#65574=ORIENTED_EDGE('',*,*,#48001,.T.);
#65575=ORIENTED_EDGE('',*,*,#48005,.F.);
#65576=ORIENTED_EDGE('',*,*,#48006,.T.);
#65577=ORIENTED_EDGE('',*,*,#48007,.T.);
#65578=ORIENTED_EDGE('',*,*,#48006,.F.);
#65579=ORIENTED_EDGE('',*,*,#48008,.F.);
#65580=ORIENTED_EDGE('',*,*,#48009,.F.);
#65581=ORIENTED_EDGE('',*,*,#48010,.T.);
#65582=ORIENTED_EDGE('',*,*,#46743,.F.);
#65583=ORIENTED_EDGE('',*,*,#48007,.F.);
#65584=ORIENTED_EDGE('',*,*,#48011,.F.);
#65585=ORIENTED_EDGE('',*,*,#48012,.T.);
#65586=ORIENTED_EDGE('',*,*,#46754,.F.);
#65587=ORIENTED_EDGE('',*,*,#48010,.F.);
#65588=ORIENTED_EDGE('',*,*,#48013,.F.);
#65589=ORIENTED_EDGE('',*,*,#48014,.T.);
#65590=ORIENTED_EDGE('',*,*,#48015,.F.);
#65591=ORIENTED_EDGE('',*,*,#48012,.F.);
#65592=ORIENTED_EDGE('',*,*,#48016,.F.);
#65593=ORIENTED_EDGE('',*,*,#48008,.T.);
#65594=ORIENTED_EDGE('',*,*,#48017,.F.);
#65595=ORIENTED_EDGE('',*,*,#48018,.F.);
#65596=ORIENTED_EDGE('',*,*,#48019,.F.);
#65597=ORIENTED_EDGE('',*,*,#48020,.T.);
#65598=ORIENTED_EDGE('',*,*,#48021,.T.);
#65599=ORIENTED_EDGE('',*,*,#48022,.T.);
#65600=ORIENTED_EDGE('',*,*,#46746,.T.);
#65601=ORIENTED_EDGE('',*,*,#48022,.F.);
#65602=ORIENTED_EDGE('',*,*,#48023,.T.);
#65603=ORIENTED_EDGE('',*,*,#48024,.T.);
#65604=ORIENTED_EDGE('',*,*,#48025,.F.);
#65605=ORIENTED_EDGE('',*,*,#47453,.F.);
#65606=ORIENTED_EDGE('',*,*,#46750,.F.);
#65607=ORIENTED_EDGE('',*,*,#47472,.T.);
#65608=ORIENTED_EDGE('',*,*,#48026,.F.);
#65609=ORIENTED_EDGE('',*,*,#46769,.T.);
#65610=ORIENTED_EDGE('',*,*,#48027,.T.);
#65611=ORIENTED_EDGE('',*,*,#48028,.F.);
#65612=ORIENTED_EDGE('',*,*,#48029,.F.);
#65613=ORIENTED_EDGE('',*,*,#48024,.F.);
#65614=ORIENTED_EDGE('',*,*,#48029,.T.);
#65615=ORIENTED_EDGE('',*,*,#48030,.F.);
#65616=ORIENTED_EDGE('',*,*,#47471,.F.);
#65617=ORIENTED_EDGE('',*,*,#48031,.F.);
#65618=ORIENTED_EDGE('',*,*,#48032,.T.);
#65619=ORIENTED_EDGE('',*,*,#48033,.F.);
#65620=ORIENTED_EDGE('',*,*,#48014,.F.);
#65621=ORIENTED_EDGE('',*,*,#48034,.F.);
#65622=ORIENTED_EDGE('',*,*,#48035,.T.);
#65623=ORIENTED_EDGE('',*,*,#47994,.T.);
#65624=ORIENTED_EDGE('',*,*,#46752,.T.);
#65625=ORIENTED_EDGE('',*,*,#48015,.T.);
#65626=ORIENTED_EDGE('',*,*,#48036,.T.);
#65627=ORIENTED_EDGE('',*,*,#48037,.F.);
#65628=ORIENTED_EDGE('',*,*,#47991,.F.);
#65629=ORIENTED_EDGE('',*,*,#48038,.F.);
#65630=ORIENTED_EDGE('',*,*,#48039,.F.);
#65631=ORIENTED_EDGE('',*,*,#48040,.T.);
#65632=ORIENTED_EDGE('',*,*,#48041,.F.);
#65633=ORIENTED_EDGE('',*,*,#47990,.T.);
#65634=ORIENTED_EDGE('',*,*,#48041,.T.);
#65635=ORIENTED_EDGE('',*,*,#48042,.T.);
#65636=ORIENTED_EDGE('',*,*,#48043,.T.);
#65637=ORIENTED_EDGE('',*,*,#47987,.F.);
#65638=ORIENTED_EDGE('',*,*,#48043,.F.);
#65639=ORIENTED_EDGE('',*,*,#48044,.T.);
#65640=ORIENTED_EDGE('',*,*,#48045,.F.);
#65641=ORIENTED_EDGE('',*,*,#47981,.F.);
#65642=ORIENTED_EDGE('',*,*,#48046,.T.);
#65643=ORIENTED_EDGE('',*,*,#48047,.F.);
#65644=ORIENTED_EDGE('',*,*,#47975,.F.);
#65645=ORIENTED_EDGE('',*,*,#48048,.F.);
#65646=ORIENTED_EDGE('',*,*,#48049,.T.);
#65647=ORIENTED_EDGE('',*,*,#47955,.T.);
#65648=ORIENTED_EDGE('',*,*,#46755,.T.);
#65649=ORIENTED_EDGE('',*,*,#47976,.T.);
#65650=ORIENTED_EDGE('',*,*,#48050,.T.);
#65651=ORIENTED_EDGE('',*,*,#48051,.F.);
#65652=ORIENTED_EDGE('',*,*,#47952,.F.);
#65653=ORIENTED_EDGE('',*,*,#48052,.F.);
#65654=ORIENTED_EDGE('',*,*,#48053,.F.);
#65655=ORIENTED_EDGE('',*,*,#48054,.T.);
#65656=ORIENTED_EDGE('',*,*,#48055,.F.);
#65657=ORIENTED_EDGE('',*,*,#47951,.T.);
#65658=ORIENTED_EDGE('',*,*,#48055,.T.);
#65659=ORIENTED_EDGE('',*,*,#48056,.T.);
#65660=ORIENTED_EDGE('',*,*,#48057,.T.);
#65661=ORIENTED_EDGE('',*,*,#46759,.T.);
#65662=ORIENTED_EDGE('',*,*,#48057,.F.);
#65663=ORIENTED_EDGE('',*,*,#48058,.T.);
#65664=ORIENTED_EDGE('',*,*,#48059,.F.);
#65665=ORIENTED_EDGE('',*,*,#47922,.F.);
#65666=ORIENTED_EDGE('',*,*,#48060,.T.);
#65667=ORIENTED_EDGE('',*,*,#48061,.F.);
#65668=ORIENTED_EDGE('',*,*,#47934,.F.);
#65669=ORIENTED_EDGE('',*,*,#48062,.F.);
#65670=ORIENTED_EDGE('',*,*,#48063,.T.);
#65671=ORIENTED_EDGE('',*,*,#47909,.T.);
#65672=ORIENTED_EDGE('',*,*,#46761,.T.);
#65673=ORIENTED_EDGE('',*,*,#47935,.T.);
#65674=ORIENTED_EDGE('',*,*,#48064,.T.);
#65675=ORIENTED_EDGE('',*,*,#48065,.F.);
#65676=ORIENTED_EDGE('',*,*,#47906,.F.);
#65677=ORIENTED_EDGE('',*,*,#48066,.F.);
#65678=ORIENTED_EDGE('',*,*,#48067,.F.);
#65679=ORIENTED_EDGE('',*,*,#48068,.T.);
#65680=ORIENTED_EDGE('',*,*,#48020,.F.);
#65681=ORIENTED_EDGE('',*,*,#47905,.T.);
#65682=ORIENTED_EDGE('',*,*,#48069,.T.);
#65683=ORIENTED_EDGE('',*,*,#48070,.T.);
#65684=ORIENTED_EDGE('',*,*,#47252,.T.);
#65685=ORIENTED_EDGE('',*,*,#46972,.T.);
#65686=ORIENTED_EDGE('',*,*,#48071,.T.);
#65687=ORIENTED_EDGE('',*,*,#48072,.T.);
#65688=ORIENTED_EDGE('',*,*,#47256,.T.);
#65689=ORIENTED_EDGE('',*,*,#46957,.T.);
#65690=ORIENTED_EDGE('',*,*,#46963,.T.);
#65691=ORIENTED_EDGE('',*,*,#46966,.T.);
#65692=ORIENTED_EDGE('',*,*,#46969,.T.);
#65693=ORIENTED_EDGE('',*,*,#47257,.T.);
#65694=ORIENTED_EDGE('',*,*,#48073,.T.);
#65695=ORIENTED_EDGE('',*,*,#48074,.T.);
#65696=ORIENTED_EDGE('',*,*,#47254,.F.);
#65697=ORIENTED_EDGE('',*,*,#48075,.F.);
#65698=ORIENTED_EDGE('',*,*,#48076,.T.);
#65699=ORIENTED_EDGE('',*,*,#47104,.T.);
#65700=ORIENTED_EDGE('',*,*,#46765,.T.);
#65701=ORIENTED_EDGE('',*,*,#47499,.T.);
#65702=ORIENTED_EDGE('',*,*,#47105,.T.);
#65703=ORIENTED_EDGE('',*,*,#48077,.T.);
#65704=ORIENTED_EDGE('',*,*,#47100,.F.);
#65705=ORIENTED_EDGE('',*,*,#48078,.F.);
#65706=ORIENTED_EDGE('',*,*,#46823,.T.);
#65707=ORIENTED_EDGE('',*,*,#47101,.T.);
#65708=ORIENTED_EDGE('',*,*,#48079,.T.);
#65709=ORIENTED_EDGE('',*,*,#48080,.T.);
#65710=ORIENTED_EDGE('',*,*,#47478,.T.);
#65711=ORIENTED_EDGE('',*,*,#46794,.T.);
#65712=ORIENTED_EDGE('',*,*,#46800,.T.);
#65713=ORIENTED_EDGE('',*,*,#46803,.T.);
#65714=ORIENTED_EDGE('',*,*,#46806,.T.);
#65715=ORIENTED_EDGE('',*,*,#47479,.T.);
#65716=ORIENTED_EDGE('',*,*,#48081,.T.);
#65717=ORIENTED_EDGE('',*,*,#47498,.F.);
#65718=ORIENTED_EDGE('',*,*,#48082,.F.);
#65719=ORIENTED_EDGE('',*,*,#46796,.T.);
#65720=ORIENTED_EDGE('',*,*,#47483,.T.);
#65721=ORIENTED_EDGE('',*,*,#46791,.T.);
#65722=ORIENTED_EDGE('',*,*,#46789,.T.);
#65723=ORIENTED_EDGE('',*,*,#46786,.T.);
#65724=ORIENTED_EDGE('',*,*,#47531,.T.);
#65725=ORIENTED_EDGE('',*,*,#46782,.T.);
#65726=ORIENTED_EDGE('',*,*,#47409,.T.);
#65727=ORIENTED_EDGE('',*,*,#46779,.T.);
#65728=ORIENTED_EDGE('',*,*,#46777,.T.);
#65729=ORIENTED_EDGE('',*,*,#46776,.T.);
#65730=ORIENTED_EDGE('',*,*,#47427,.T.);
#65731=ORIENTED_EDGE('',*,*,#46771,.T.);
#65732=ORIENTED_EDGE('',*,*,#46770,.T.);
#65733=ORIENTED_EDGE('',*,*,#48083,.T.);
#65734=ORIENTED_EDGE('',*,*,#48084,.T.);
#65735=ORIENTED_EDGE('',*,*,#48085,.T.);
#65736=ORIENTED_EDGE('',*,*,#48085,.F.);
#65737=ORIENTED_EDGE('',*,*,#48086,.T.);
#65738=ORIENTED_EDGE('',*,*,#48087,.F.);
#65739=ORIENTED_EDGE('',*,*,#46798,.T.);
#65740=ORIENTED_EDGE('',*,*,#48087,.T.);
#65741=ORIENTED_EDGE('',*,*,#48088,.T.);
#65742=ORIENTED_EDGE('',*,*,#48089,.T.);
#65743=ORIENTED_EDGE('',*,*,#46801,.T.);
#65744=ORIENTED_EDGE('',*,*,#48089,.F.);
#65745=ORIENTED_EDGE('',*,*,#48090,.T.);
#65746=ORIENTED_EDGE('',*,*,#48091,.F.);
#65747=ORIENTED_EDGE('',*,*,#46804,.T.);
#65748=ORIENTED_EDGE('',*,*,#46833,.T.);
#65749=ORIENTED_EDGE('',*,*,#47093,.T.);
#65750=ORIENTED_EDGE('',*,*,#46830,.T.);
#65751=ORIENTED_EDGE('',*,*,#46828,.T.);
#65752=ORIENTED_EDGE('',*,*,#46825,.T.);
#65753=ORIENTED_EDGE('',*,*,#47121,.T.);
#65754=ORIENTED_EDGE('',*,*,#46821,.T.);
#65755=ORIENTED_EDGE('',*,*,#48091,.T.);
#65756=ORIENTED_EDGE('',*,*,#48092,.T.);
#65757=ORIENTED_EDGE('',*,*,#48093,.T.);
#65758=ORIENTED_EDGE('',*,*,#46819,.T.);
#65759=ORIENTED_EDGE('',*,*,#46817,.T.);
#65760=ORIENTED_EDGE('',*,*,#47018,.T.);
#65761=ORIENTED_EDGE('',*,*,#46813,.T.);
#65762=ORIENTED_EDGE('',*,*,#46811,.T.);
#65763=ORIENTED_EDGE('',*,*,#46810,.T.);
#65764=ORIENTED_EDGE('',*,*,#47039,.T.);
#65765=ORIENTED_EDGE('',*,*,#48094,.F.);
#65766=ORIENTED_EDGE('',*,*,#46839,.T.);
#65767=ORIENTED_EDGE('',*,*,#47145,.T.);
#65768=ORIENTED_EDGE('',*,*,#46836,.T.);
#65769=ORIENTED_EDGE('',*,*,#48093,.F.);
#65770=ORIENTED_EDGE('',*,*,#48095,.T.);
#65771=ORIENTED_EDGE('',*,*,#48096,.T.);
#65772=ORIENTED_EDGE('',*,*,#46923,.T.);
#65773=ORIENTED_EDGE('',*,*,#46921,.T.);
#65774=ORIENTED_EDGE('',*,*,#46918,.T.);
#65775=ORIENTED_EDGE('',*,*,#47561,.T.);
#65776=ORIENTED_EDGE('',*,*,#46914,.T.);
#65777=ORIENTED_EDGE('',*,*,#47581,.T.);
#65778=ORIENTED_EDGE('',*,*,#46913,.T.);
#65779=ORIENTED_EDGE('',*,*,#46910,.T.);
#65780=ORIENTED_EDGE('',*,*,#46908,.T.);
#65781=ORIENTED_EDGE('',*,*,#46906,.T.);
#65782=ORIENTED_EDGE('',*,*,#47604,.T.);
#65783=ORIENTED_EDGE('',*,*,#46900,.T.);
#65784=ORIENTED_EDGE('',*,*,#47632,.T.);
#65785=ORIENTED_EDGE('',*,*,#46897,.T.);
#65786=ORIENTED_EDGE('',*,*,#46895,.T.);
#65787=ORIENTED_EDGE('',*,*,#46894,.T.);
#65788=ORIENTED_EDGE('',*,*,#47650,.T.);
#65789=ORIENTED_EDGE('',*,*,#46888,.T.);
#65790=ORIENTED_EDGE('',*,*,#47678,.T.);
#65791=ORIENTED_EDGE('',*,*,#46885,.T.);
#65792=ORIENTED_EDGE('',*,*,#46883,.T.);
#65793=ORIENTED_EDGE('',*,*,#46882,.T.);
#65794=ORIENTED_EDGE('',*,*,#47696,.T.);
#65795=ORIENTED_EDGE('',*,*,#46876,.T.);
#65796=ORIENTED_EDGE('',*,*,#47724,.T.);
#65797=ORIENTED_EDGE('',*,*,#46873,.T.);
#65798=ORIENTED_EDGE('',*,*,#46871,.T.);
#65799=ORIENTED_EDGE('',*,*,#46870,.T.);
#65800=ORIENTED_EDGE('',*,*,#47742,.T.);
#65801=ORIENTED_EDGE('',*,*,#46864,.T.);
#65802=ORIENTED_EDGE('',*,*,#47771,.T.);
#65803=ORIENTED_EDGE('',*,*,#46863,.T.);
#65804=ORIENTED_EDGE('',*,*,#46860,.T.);
#65805=ORIENTED_EDGE('',*,*,#46858,.T.);
#65806=ORIENTED_EDGE('',*,*,#46856,.T.);
#65807=ORIENTED_EDGE('',*,*,#47794,.T.);
#65808=ORIENTED_EDGE('',*,*,#46850,.T.);
#65809=ORIENTED_EDGE('',*,*,#47831,.T.);
#65810=ORIENTED_EDGE('',*,*,#46849,.T.);
#65811=ORIENTED_EDGE('',*,*,#46845,.T.);
#65812=ORIENTED_EDGE('',*,*,#46842,.T.);
#65813=ORIENTED_EDGE('',*,*,#48094,.T.);
#65814=ORIENTED_EDGE('',*,*,#48097,.T.);
#65815=ORIENTED_EDGE('',*,*,#47250,.T.);
#65816=ORIENTED_EDGE('',*,*,#46931,.T.);
#65817=ORIENTED_EDGE('',*,*,#48096,.F.);
#65818=ORIENTED_EDGE('',*,*,#48098,.T.);
#65819=ORIENTED_EDGE('',*,*,#48099,.F.);
#65820=ORIENTED_EDGE('',*,*,#46927,.T.);
#65821=ORIENTED_EDGE('',*,*,#46959,.T.);
#65822=ORIENTED_EDGE('',*,*,#47261,.T.);
#65823=ORIENTED_EDGE('',*,*,#46954,.T.);
#65824=ORIENTED_EDGE('',*,*,#46952,.T.);
#65825=ORIENTED_EDGE('',*,*,#46949,.T.);
#65826=ORIENTED_EDGE('',*,*,#47309,.T.);
#65827=ORIENTED_EDGE('',*,*,#46945,.T.);
#65828=ORIENTED_EDGE('',*,*,#47179,.T.);
#65829=ORIENTED_EDGE('',*,*,#46942,.T.);
#65830=ORIENTED_EDGE('',*,*,#46940,.T.);
#65831=ORIENTED_EDGE('',*,*,#46939,.T.);
#65832=ORIENTED_EDGE('',*,*,#47197,.T.);
#65833=ORIENTED_EDGE('',*,*,#46934,.T.);
#65834=ORIENTED_EDGE('',*,*,#46933,.T.);
#65835=ORIENTED_EDGE('',*,*,#48099,.T.);
#65836=ORIENTED_EDGE('',*,*,#48100,.T.);
#65837=ORIENTED_EDGE('',*,*,#48101,.T.);
#65838=ORIENTED_EDGE('',*,*,#48101,.F.);
#65839=ORIENTED_EDGE('',*,*,#48102,.T.);
#65840=ORIENTED_EDGE('',*,*,#48103,.F.);
#65841=ORIENTED_EDGE('',*,*,#46961,.T.);
#65842=ORIENTED_EDGE('',*,*,#48103,.T.);
#65843=ORIENTED_EDGE('',*,*,#48104,.T.);
#65844=ORIENTED_EDGE('',*,*,#48105,.T.);
#65845=ORIENTED_EDGE('',*,*,#46964,.T.);
#65846=ORIENTED_EDGE('',*,*,#48105,.F.);
#65847=ORIENTED_EDGE('',*,*,#48106,.T.);
#65848=ORIENTED_EDGE('',*,*,#48107,.F.);
#65849=ORIENTED_EDGE('',*,*,#46967,.T.);
#65850=ORIENTED_EDGE('',*,*,#48108,.T.);
#65851=ORIENTED_EDGE('',*,*,#48109,.T.);
#65852=ORIENTED_EDGE('',*,*,#48110,.T.);
#65853=ORIENTED_EDGE('',*,*,#48111,.T.);
#65854=ORIENTED_EDGE('',*,*,#46970,.T.);
#65855=ORIENTED_EDGE('',*,*,#48107,.T.);
#65856=ORIENTED_EDGE('',*,*,#48112,.T.);
#65857=ORIENTED_EDGE('',*,*,#48113,.T.);
#65858=ORIENTED_EDGE('',*,*,#48110,.F.);
#65859=ORIENTED_EDGE('',*,*,#48114,.F.);
#65860=ORIENTED_EDGE('',*,*,#48115,.F.);
#65861=ORIENTED_EDGE('',*,*,#48116,.T.);
#65862=ORIENTED_EDGE('',*,*,#48111,.F.);
#65863=ORIENTED_EDGE('',*,*,#48113,.F.);
#65864=ORIENTED_EDGE('',*,*,#48117,.F.);
#65865=ORIENTED_EDGE('',*,*,#48118,.T.);
#65866=ORIENTED_EDGE('',*,*,#46971,.F.);
#65867=ORIENTED_EDGE('',*,*,#48116,.F.);
#65868=ORIENTED_EDGE('',*,*,#48119,.F.);
#65869=ORIENTED_EDGE('',*,*,#48120,.T.);
#65870=ORIENTED_EDGE('',*,*,#48071,.F.);
#65871=ORIENTED_EDGE('',*,*,#48118,.F.);
#65872=ORIENTED_EDGE('',*,*,#48121,.F.);
#65873=ORIENTED_EDGE('',*,*,#48122,.T.);
#65874=ORIENTED_EDGE('',*,*,#48123,.T.);
#65875=ORIENTED_EDGE('',*,*,#48120,.F.);
#65876=ORIENTED_EDGE('',*,*,#48124,.F.);
#65877=ORIENTED_EDGE('',*,*,#46975,.T.);
#65878=ORIENTED_EDGE('',*,*,#48070,.F.);
#65879=ORIENTED_EDGE('',*,*,#48122,.F.);
#65880=ORIENTED_EDGE('',*,*,#48125,.F.);
#65881=ORIENTED_EDGE('',*,*,#48126,.F.);
#65882=ORIENTED_EDGE('',*,*,#46973,.T.);
#65883=ORIENTED_EDGE('',*,*,#48127,.F.);
#65884=ORIENTED_EDGE('',*,*,#48128,.T.);
#65885=ORIENTED_EDGE('',*,*,#47329,.T.);
#65886=ORIENTED_EDGE('',*,*,#48129,.F.);
#65887=ORIENTED_EDGE('',*,*,#48130,.F.);
#65888=ORIENTED_EDGE('',*,*,#48131,.F.);
#65889=ORIENTED_EDGE('',*,*,#48132,.T.);
#65890=ORIENTED_EDGE('',*,*,#47367,.T.);
#65891=ORIENTED_EDGE('',*,*,#46976,.T.);
#65892=ORIENTED_EDGE('',*,*,#47330,.T.);
#65893=ORIENTED_EDGE('',*,*,#47368,.T.);
#65894=ORIENTED_EDGE('',*,*,#48133,.F.);
#65895=ORIENTED_EDGE('',*,*,#48134,.T.);
#65896=ORIENTED_EDGE('',*,*,#48135,.F.);
#65897=ORIENTED_EDGE('',*,*,#48136,.F.);
#65898=ORIENTED_EDGE('',*,*,#48137,.T.);
#65899=ORIENTED_EDGE('',*,*,#48138,.F.);
#65900=ORIENTED_EDGE('',*,*,#47365,.T.);
#65901=ORIENTED_EDGE('',*,*,#48138,.T.);
#65902=ORIENTED_EDGE('',*,*,#48139,.T.);
#65903=ORIENTED_EDGE('',*,*,#48140,.T.);
#65904=ORIENTED_EDGE('',*,*,#47360,.T.);
#65905=ORIENTED_EDGE('',*,*,#48140,.F.);
#65906=ORIENTED_EDGE('',*,*,#48141,.T.);
#65907=ORIENTED_EDGE('',*,*,#48142,.F.);
#65908=ORIENTED_EDGE('',*,*,#47356,.F.);
#65909=ORIENTED_EDGE('',*,*,#47354,.T.);
#65910=ORIENTED_EDGE('',*,*,#48143,.F.);
#65911=ORIENTED_EDGE('',*,*,#48144,.F.);
#65912=ORIENTED_EDGE('',*,*,#48145,.F.);
#65913=ORIENTED_EDGE('',*,*,#48146,.T.);
#65914=ORIENTED_EDGE('',*,*,#47883,.T.);
#65915=ORIENTED_EDGE('',*,*,#46979,.T.);
#65916=ORIENTED_EDGE('',*,*,#47355,.T.);
#65917=ORIENTED_EDGE('',*,*,#47884,.T.);
#65918=ORIENTED_EDGE('',*,*,#48147,.F.);
#65919=ORIENTED_EDGE('',*,*,#48148,.T.);
#65920=ORIENTED_EDGE('',*,*,#48149,.F.);
#65921=ORIENTED_EDGE('',*,*,#48150,.F.);
#65922=ORIENTED_EDGE('',*,*,#48151,.T.);
#65923=ORIENTED_EDGE('',*,*,#48152,.F.);
#65924=ORIENTED_EDGE('',*,*,#47881,.T.);
#65925=ORIENTED_EDGE('',*,*,#48152,.T.);
#65926=ORIENTED_EDGE('',*,*,#48153,.T.);
#65927=ORIENTED_EDGE('',*,*,#48154,.T.);
#65928=ORIENTED_EDGE('',*,*,#47876,.T.);
#65929=ORIENTED_EDGE('',*,*,#48154,.F.);
#65930=ORIENTED_EDGE('',*,*,#48155,.T.);
#65931=ORIENTED_EDGE('',*,*,#48156,.F.);
#65932=ORIENTED_EDGE('',*,*,#47872,.F.);
#65933=ORIENTED_EDGE('',*,*,#47870,.T.);
#65934=ORIENTED_EDGE('',*,*,#48157,.F.);
#65935=ORIENTED_EDGE('',*,*,#48158,.F.);
#65936=ORIENTED_EDGE('',*,*,#48159,.F.);
#65937=ORIENTED_EDGE('',*,*,#48160,.T.);
#65938=ORIENTED_EDGE('',*,*,#47871,.T.);
#65939=ORIENTED_EDGE('',*,*,#48161,.T.);
#65940=ORIENTED_EDGE('',*,*,#48162,.T.);
#65941=ORIENTED_EDGE('',*,*,#47856,.T.);
#65942=ORIENTED_EDGE('',*,*,#48163,.F.);
#65943=ORIENTED_EDGE('',*,*,#47868,.T.);
#65944=ORIENTED_EDGE('',*,*,#48160,.F.);
#65945=ORIENTED_EDGE('',*,*,#47857,.T.);
#65946=ORIENTED_EDGE('',*,*,#48164,.F.);
#65947=ORIENTED_EDGE('',*,*,#48165,.T.);
#65948=ORIENTED_EDGE('',*,*,#48166,.F.);
#65949=ORIENTED_EDGE('',*,*,#48167,.T.);
#65950=ORIENTED_EDGE('',*,*,#48168,.F.);
#65951=ORIENTED_EDGE('',*,*,#48165,.F.);
#65952=ORIENTED_EDGE('',*,*,#48169,.F.);
#65953=ORIENTED_EDGE('',*,*,#48170,.F.);
#65954=ORIENTED_EDGE('',*,*,#48171,.T.);
#65955=ORIENTED_EDGE('',*,*,#48172,.F.);
#65956=ORIENTED_EDGE('',*,*,#48173,.T.);
#65957=ORIENTED_EDGE('',*,*,#48172,.T.);
#65958=ORIENTED_EDGE('',*,*,#48174,.T.);
#65959=ORIENTED_EDGE('',*,*,#48175,.T.);
#65960=ORIENTED_EDGE('',*,*,#48176,.T.);
#65961=ORIENTED_EDGE('',*,*,#48175,.F.);
#65962=ORIENTED_EDGE('',*,*,#48177,.T.);
#65963=ORIENTED_EDGE('',*,*,#48178,.F.);
#65964=ORIENTED_EDGE('',*,*,#48179,.T.);
#65965=ORIENTED_EDGE('',*,*,#47853,.T.);
#65966=ORIENTED_EDGE('',*,*,#48180,.F.);
#65967=ORIENTED_EDGE('',*,*,#48181,.F.);
#65968=ORIENTED_EDGE('',*,*,#48182,.F.);
#65969=ORIENTED_EDGE('',*,*,#48183,.F.);
#65970=ORIENTED_EDGE('',*,*,#47849,.T.);
#65971=ORIENTED_EDGE('',*,*,#48184,.F.);
#65972=ORIENTED_EDGE('',*,*,#48185,.F.);
#65973=ORIENTED_EDGE('',*,*,#48186,.T.);
#65974=ORIENTED_EDGE('',*,*,#48187,.F.);
#65975=ORIENTED_EDGE('',*,*,#48188,.F.);
#65976=ORIENTED_EDGE('',*,*,#48189,.T.);
#65977=ORIENTED_EDGE('',*,*,#48190,.F.);
#65978=ORIENTED_EDGE('',*,*,#48191,.T.);
#65979=ORIENTED_EDGE('',*,*,#48190,.T.);
#65980=ORIENTED_EDGE('',*,*,#48192,.T.);
#65981=ORIENTED_EDGE('',*,*,#48193,.T.);
#65982=ORIENTED_EDGE('',*,*,#48194,.T.);
#65983=ORIENTED_EDGE('',*,*,#48193,.F.);
#65984=ORIENTED_EDGE('',*,*,#48195,.T.);
#65985=ORIENTED_EDGE('',*,*,#48196,.F.);
#65986=ORIENTED_EDGE('',*,*,#48197,.T.);
#65987=ORIENTED_EDGE('',*,*,#48198,.T.);
#65988=ORIENTED_EDGE('',*,*,#46987,.F.);
#65989=ORIENTED_EDGE('',*,*,#48199,.F.);
#65990=ORIENTED_EDGE('',*,*,#48200,.F.);
#65991=ORIENTED_EDGE('',*,*,#48201,.T.);
#65992=ORIENTED_EDGE('',*,*,#47344,.F.);
#65993=ORIENTED_EDGE('',*,*,#48198,.F.);
#65994=ORIENTED_EDGE('',*,*,#48202,.F.);
#65995=ORIENTED_EDGE('',*,*,#48203,.T.);
#65996=ORIENTED_EDGE('',*,*,#48204,.F.);
#65997=ORIENTED_EDGE('',*,*,#48201,.F.);
#65998=ORIENTED_EDGE('',*,*,#48205,.F.);
#65999=ORIENTED_EDGE('',*,*,#48206,.T.);
#66000=ORIENTED_EDGE('',*,*,#48207,.F.);
#66001=ORIENTED_EDGE('',*,*,#48128,.F.);
#66002=ORIENTED_EDGE('',*,*,#48208,.F.);
#66003=ORIENTED_EDGE('',*,*,#48199,.T.);
#66004=ORIENTED_EDGE('',*,*,#47275,.F.);
#66005=ORIENTED_EDGE('',*,*,#48206,.F.);
#66006=ORIENTED_EDGE('',*,*,#48209,.F.);
#66007=ORIENTED_EDGE('',*,*,#48210,.T.);
#66008=ORIENTED_EDGE('',*,*,#47342,.F.);
#66009=ORIENTED_EDGE('',*,*,#48203,.F.);
#66010=ORIENTED_EDGE('',*,*,#48211,.F.);
#66011=ORIENTED_EDGE('',*,*,#47343,.T.);
#66012=ORIENTED_EDGE('',*,*,#48212,.T.);
#66013=ORIENTED_EDGE('',*,*,#48213,.T.);
#66014=ORIENTED_EDGE('',*,*,#47337,.T.);
#66015=ORIENTED_EDGE('',*,*,#48213,.F.);
#66016=ORIENTED_EDGE('',*,*,#48214,.T.);
#66017=ORIENTED_EDGE('',*,*,#48215,.F.);
#66018=ORIENTED_EDGE('',*,*,#47331,.F.);
#66019=ORIENTED_EDGE('',*,*,#47457,.T.);
#66020=ORIENTED_EDGE('',*,*,#48216,.F.);
#66021=ORIENTED_EDGE('',*,*,#48217,.F.);
#66022=ORIENTED_EDGE('',*,*,#48218,.F.);
#66023=ORIENTED_EDGE('',*,*,#48219,.F.);
#66024=ORIENTED_EDGE('',*,*,#47901,.T.);
#66025=ORIENTED_EDGE('',*,*,#46983,.F.);
#66026=ORIENTED_EDGE('',*,*,#48218,.T.);
#66027=ORIENTED_EDGE('',*,*,#47110,.T.);
#66028=ORIENTED_EDGE('',*,*,#48220,.F.);
#66029=ORIENTED_EDGE('',*,*,#48221,.F.);
#66030=ORIENTED_EDGE('',*,*,#48222,.F.);
#66031=ORIENTED_EDGE('',*,*,#48223,.F.);
#66032=ORIENTED_EDGE('',*,*,#48224,.T.);
#66033=ORIENTED_EDGE('',*,*,#48225,.T.);
#66034=ORIENTED_EDGE('',*,*,#47494,.T.);
#66035=ORIENTED_EDGE('',*,*,#46990,.T.);
#66036=ORIENTED_EDGE('',*,*,#47111,.T.);
#66037=ORIENTED_EDGE('',*,*,#48226,.T.);
#66038=ORIENTED_EDGE('',*,*,#48224,.F.);
#66039=ORIENTED_EDGE('',*,*,#48223,.T.);
#66040=ORIENTED_EDGE('',*,*,#48227,.F.);
#66041=ORIENTED_EDGE('',*,*,#48228,.T.);
#66042=ORIENTED_EDGE('',*,*,#48229,.T.);
#66043=ORIENTED_EDGE('',*,*,#48227,.T.);
#66044=ORIENTED_EDGE('',*,*,#48229,.F.);
#66045=ORIENTED_EDGE('',*,*,#48230,.T.);
#66046=ORIENTED_EDGE('',*,*,#48231,.F.);
#66047=ORIENTED_EDGE('',*,*,#47491,.F.);
#66048=ORIENTED_EDGE('',*,*,#48232,.F.);
#66049=ORIENTED_EDGE('',*,*,#48233,.T.);
#66050=ORIENTED_EDGE('',*,*,#48234,.F.);
#66051=ORIENTED_EDGE('',*,*,#48235,.F.);
#66052=ORIENTED_EDGE('',*,*,#48236,.F.);
#66053=ORIENTED_EDGE('',*,*,#48237,.T.);
#66054=ORIENTED_EDGE('',*,*,#47346,.F.);
#66055=ORIENTED_EDGE('',*,*,#48233,.F.);
#66056=ORIENTED_EDGE('',*,*,#48238,.F.);
#66057=ORIENTED_EDGE('',*,*,#48239,.T.);
#66058=ORIENTED_EDGE('',*,*,#46989,.F.);
#66059=ORIENTED_EDGE('',*,*,#48237,.F.);
#66060=ORIENTED_EDGE('',*,*,#48240,.F.);
#66061=ORIENTED_EDGE('',*,*,#48241,.T.);
#66062=ORIENTED_EDGE('',*,*,#47276,.F.);
#66063=ORIENTED_EDGE('',*,*,#48239,.F.);
#66064=ORIENTED_EDGE('',*,*,#48242,.F.);
#66065=ORIENTED_EDGE('',*,*,#47271,.T.);
#66066=ORIENTED_EDGE('',*,*,#48243,.F.);
#66067=ORIENTED_EDGE('',*,*,#48241,.F.);
#66068=ORIENTED_EDGE('',*,*,#48244,.F.);
#66069=ORIENTED_EDGE('',*,*,#48245,.F.);
#66070=ORIENTED_EDGE('',*,*,#48246,.T.);
#66071=ORIENTED_EDGE('',*,*,#47272,.T.);
#66072=ORIENTED_EDGE('',*,*,#48247,.T.);
#66073=ORIENTED_EDGE('',*,*,#47273,.T.);
#66074=ORIENTED_EDGE('',*,*,#48246,.F.);
#66075=ORIENTED_EDGE('',*,*,#48245,.T.);
#66076=ORIENTED_EDGE('',*,*,#48248,.F.);
#66077=ORIENTED_EDGE('',*,*,#48249,.T.);
#66078=ORIENTED_EDGE('',*,*,#48250,.T.);
#66079=ORIENTED_EDGE('',*,*,#48248,.T.);
#66080=ORIENTED_EDGE('',*,*,#48250,.F.);
#66081=ORIENTED_EDGE('',*,*,#47269,.T.);
#66082=ORIENTED_EDGE('',*,*,#48251,.F.);
#66083=ORIENTED_EDGE('',*,*,#48252,.F.);
#66084=ORIENTED_EDGE('',*,*,#48253,.F.);
#66085=ORIENTED_EDGE('',*,*,#48254,.T.);
#66086=ORIENTED_EDGE('',*,*,#47021,.T.);
#66087=ORIENTED_EDGE('',*,*,#48255,.T.);
#66088=ORIENTED_EDGE('',*,*,#47019,.T.);
#66089=ORIENTED_EDGE('',*,*,#47017,.T.);
#66090=ORIENTED_EDGE('',*,*,#47016,.T.);
#66091=ORIENTED_EDGE('',*,*,#47013,.T.);
#66092=ORIENTED_EDGE('',*,*,#47011,.T.);
#66093=ORIENTED_EDGE('',*,*,#47009,.T.);
#66094=ORIENTED_EDGE('',*,*,#47007,.T.);
#66095=ORIENTED_EDGE('',*,*,#47005,.T.);
#66096=ORIENTED_EDGE('',*,*,#47003,.T.);
#66097=ORIENTED_EDGE('',*,*,#47001,.T.);
#66098=ORIENTED_EDGE('',*,*,#47149,.T.);
#66099=ORIENTED_EDGE('',*,*,#47023,.T.);
#66100=ORIENTED_EDGE('',*,*,#48256,.T.);
#66101=ORIENTED_EDGE('',*,*,#48257,.T.);
#66102=ORIENTED_EDGE('',*,*,#48258,.T.);
#66103=ORIENTED_EDGE('',*,*,#47024,.T.);
#66104=ORIENTED_EDGE('',*,*,#46996,.T.);
#66105=ORIENTED_EDGE('',*,*,#46994,.T.);
#66106=ORIENTED_EDGE('',*,*,#47022,.T.);
#66107=ORIENTED_EDGE('',*,*,#48259,.F.);
#66108=ORIENTED_EDGE('',*,*,#48260,.F.);
#66109=ORIENTED_EDGE('',*,*,#48261,.F.);
#66110=ORIENTED_EDGE('',*,*,#48256,.F.);
#66111=ORIENTED_EDGE('',*,*,#48258,.F.);
#66112=ORIENTED_EDGE('',*,*,#48262,.T.);
#66113=ORIENTED_EDGE('',*,*,#48263,.F.);
#66114=ORIENTED_EDGE('',*,*,#47025,.T.);
#66115=ORIENTED_EDGE('',*,*,#48263,.T.);
#66116=ORIENTED_EDGE('',*,*,#48264,.T.);
#66117=ORIENTED_EDGE('',*,*,#48265,.T.);
#66118=ORIENTED_EDGE('',*,*,#47027,.T.);
#66119=ORIENTED_EDGE('',*,*,#48265,.F.);
#66120=ORIENTED_EDGE('',*,*,#48266,.T.);
#66121=ORIENTED_EDGE('',*,*,#48267,.F.);
#66122=ORIENTED_EDGE('',*,*,#47029,.F.);
#66123=ORIENTED_EDGE('',*,*,#48267,.T.);
#66124=ORIENTED_EDGE('',*,*,#48268,.T.);
#66125=ORIENTED_EDGE('',*,*,#48269,.T.);
#66126=ORIENTED_EDGE('',*,*,#47059,.T.);
#66127=ORIENTED_EDGE('',*,*,#47056,.T.);
#66128=ORIENTED_EDGE('',*,*,#47054,.T.);
#66129=ORIENTED_EDGE('',*,*,#47052,.T.);
#66130=ORIENTED_EDGE('',*,*,#47050,.T.);
#66131=ORIENTED_EDGE('',*,*,#47048,.T.);
#66132=ORIENTED_EDGE('',*,*,#47046,.T.);
#66133=ORIENTED_EDGE('',*,*,#47044,.T.);
#66134=ORIENTED_EDGE('',*,*,#47042,.T.);
#66135=ORIENTED_EDGE('',*,*,#47040,.T.);
#66136=ORIENTED_EDGE('',*,*,#47037,.T.);
#66137=ORIENTED_EDGE('',*,*,#47036,.T.);
#66138=ORIENTED_EDGE('',*,*,#47034,.T.);
#66139=ORIENTED_EDGE('',*,*,#47032,.T.);
#66140=ORIENTED_EDGE('',*,*,#47030,.T.);
#66141=ORIENTED_EDGE('',*,*,#47060,.T.);
#66142=ORIENTED_EDGE('',*,*,#48269,.F.);
#66143=ORIENTED_EDGE('',*,*,#48270,.F.);
#66144=ORIENTED_EDGE('',*,*,#48271,.F.);
#66145=ORIENTED_EDGE('',*,*,#47062,.T.);
#66146=ORIENTED_EDGE('',*,*,#47061,.T.);
#66147=ORIENTED_EDGE('',*,*,#48272,.T.);
#66148=ORIENTED_EDGE('',*,*,#47072,.T.);
#66149=ORIENTED_EDGE('',*,*,#48273,.T.);
#66150=ORIENTED_EDGE('',*,*,#48274,.F.);
#66151=ORIENTED_EDGE('',*,*,#47069,.F.);
#66152=ORIENTED_EDGE('',*,*,#48275,.F.);
#66153=ORIENTED_EDGE('',*,*,#47094,.T.);
#66154=ORIENTED_EDGE('',*,*,#47092,.T.);
#66155=ORIENTED_EDGE('',*,*,#47091,.T.);
#66156=ORIENTED_EDGE('',*,*,#47088,.T.);
#66157=ORIENTED_EDGE('',*,*,#47086,.T.);
#66158=ORIENTED_EDGE('',*,*,#47084,.T.);
#66159=ORIENTED_EDGE('',*,*,#47082,.T.);
#66160=ORIENTED_EDGE('',*,*,#47079,.T.);
#66161=ORIENTED_EDGE('',*,*,#47077,.T.);
#66162=ORIENTED_EDGE('',*,*,#47075,.T.);
#66163=ORIENTED_EDGE('',*,*,#47073,.T.);
#66164=ORIENTED_EDGE('',*,*,#47070,.T.);
#66165=ORIENTED_EDGE('',*,*,#48274,.T.);
#66166=ORIENTED_EDGE('',*,*,#48276,.T.);
#66167=ORIENTED_EDGE('',*,*,#48277,.T.);
#66168=ORIENTED_EDGE('',*,*,#47095,.T.);
#66169=ORIENTED_EDGE('',*,*,#47067,.T.);
#66170=ORIENTED_EDGE('',*,*,#47065,.T.);
#66171=ORIENTED_EDGE('',*,*,#48277,.F.);
#66172=ORIENTED_EDGE('',*,*,#48278,.T.);
#66173=ORIENTED_EDGE('',*,*,#48279,.F.);
#66174=ORIENTED_EDGE('',*,*,#47096,.T.);
#66175=ORIENTED_EDGE('',*,*,#48279,.T.);
#66176=ORIENTED_EDGE('',*,*,#48280,.T.);
#66177=ORIENTED_EDGE('',*,*,#48281,.T.);
#66178=ORIENTED_EDGE('',*,*,#47098,.T.);
#66179=ORIENTED_EDGE('',*,*,#48281,.F.);
#66180=ORIENTED_EDGE('',*,*,#48282,.T.);
#66181=ORIENTED_EDGE('',*,*,#48283,.F.);
#66182=ORIENTED_EDGE('',*,*,#47113,.T.);
#66183=ORIENTED_EDGE('',*,*,#47123,.T.);
#66184=ORIENTED_EDGE('',*,*,#47122,.T.);
#66185=ORIENTED_EDGE('',*,*,#47119,.T.);
#66186=ORIENTED_EDGE('',*,*,#47118,.T.);
#66187=ORIENTED_EDGE('',*,*,#47116,.T.);
#66188=ORIENTED_EDGE('',*,*,#47114,.T.);
#66189=ORIENTED_EDGE('',*,*,#48283,.T.);
#66190=ORIENTED_EDGE('',*,*,#48284,.T.);
#66191=ORIENTED_EDGE('',*,*,#48285,.T.);
#66192=ORIENTED_EDGE('',*,*,#48220,.T.);
#66193=ORIENTED_EDGE('',*,*,#47109,.T.);
#66194=ORIENTED_EDGE('',*,*,#47107,.T.);
#66195=ORIENTED_EDGE('',*,*,#47497,.T.);
#66196=ORIENTED_EDGE('',*,*,#47106,.T.);
#66197=ORIENTED_EDGE('',*,*,#48078,.T.);
#66198=ORIENTED_EDGE('',*,*,#47103,.T.);
#66199=ORIENTED_EDGE('',*,*,#48221,.T.);
#66200=ORIENTED_EDGE('',*,*,#48285,.F.);
#66201=ORIENTED_EDGE('',*,*,#48286,.F.);
#66202=ORIENTED_EDGE('',*,*,#48287,.F.);
#66203=ORIENTED_EDGE('',*,*,#47147,.T.);
#66204=ORIENTED_EDGE('',*,*,#47146,.T.);
#66205=ORIENTED_EDGE('',*,*,#47143,.T.);
#66206=ORIENTED_EDGE('',*,*,#47141,.T.);
#66207=ORIENTED_EDGE('',*,*,#47139,.T.);
#66208=ORIENTED_EDGE('',*,*,#47839,.T.);
#66209=ORIENTED_EDGE('',*,*,#48288,.T.);
#66210=ORIENTED_EDGE('',*,*,#48289,.T.);
#66211=ORIENTED_EDGE('',*,*,#48290,.T.);
#66212=ORIENTED_EDGE('',*,*,#47152,.T.);
#66213=ORIENTED_EDGE('',*,*,#47137,.T.);
#66214=ORIENTED_EDGE('',*,*,#47134,.T.);
#66215=ORIENTED_EDGE('',*,*,#47132,.T.);
#66216=ORIENTED_EDGE('',*,*,#47130,.T.);
#66217=ORIENTED_EDGE('',*,*,#47128,.T.);
#66218=ORIENTED_EDGE('',*,*,#47126,.T.);
#66219=ORIENTED_EDGE('',*,*,#48291,.T.);
#66220=ORIENTED_EDGE('',*,*,#48292,.F.);
#66221=ORIENTED_EDGE('',*,*,#47150,.F.);
#66222=ORIENTED_EDGE('',*,*,#48290,.F.);
#66223=ORIENTED_EDGE('',*,*,#47153,.F.);
#66224=ORIENTED_EDGE('',*,*,#47151,.T.);
#66225=ORIENTED_EDGE('',*,*,#48293,.T.);
#66226=ORIENTED_EDGE('',*,*,#48255,.F.);
#66227=ORIENTED_EDGE('',*,*,#47148,.T.);
#66228=ORIENTED_EDGE('',*,*,#47181,.T.);
#66229=ORIENTED_EDGE('',*,*,#47180,.T.);
#66230=ORIENTED_EDGE('',*,*,#47178,.T.);
#66231=ORIENTED_EDGE('',*,*,#47176,.T.);
#66232=ORIENTED_EDGE('',*,*,#47174,.T.);
#66233=ORIENTED_EDGE('',*,*,#47172,.T.);
#66234=ORIENTED_EDGE('',*,*,#47170,.T.);
#66235=ORIENTED_EDGE('',*,*,#47168,.T.);
#66236=ORIENTED_EDGE('',*,*,#47166,.T.);
#66237=ORIENTED_EDGE('',*,*,#47164,.T.);
#66238=ORIENTED_EDGE('',*,*,#47162,.T.);
#66239=ORIENTED_EDGE('',*,*,#47315,.T.);
#66240=ORIENTED_EDGE('',*,*,#48294,.T.);
#66241=ORIENTED_EDGE('',*,*,#48295,.T.);
#66242=ORIENTED_EDGE('',*,*,#48296,.T.);
#66243=ORIENTED_EDGE('',*,*,#47182,.T.);
#66244=ORIENTED_EDGE('',*,*,#47157,.T.);
#66245=ORIENTED_EDGE('',*,*,#47155,.T.);
#66246=ORIENTED_EDGE('',*,*,#48296,.F.);
#66247=ORIENTED_EDGE('',*,*,#48297,.T.);
#66248=ORIENTED_EDGE('',*,*,#48298,.F.);
#66249=ORIENTED_EDGE('',*,*,#47183,.T.);
#66250=ORIENTED_EDGE('',*,*,#48298,.T.);
#66251=ORIENTED_EDGE('',*,*,#48299,.T.);
#66252=ORIENTED_EDGE('',*,*,#48300,.T.);
#66253=ORIENTED_EDGE('',*,*,#47185,.T.);
#66254=ORIENTED_EDGE('',*,*,#48300,.F.);
#66255=ORIENTED_EDGE('',*,*,#48301,.T.);
#66256=ORIENTED_EDGE('',*,*,#48302,.F.);
#66257=ORIENTED_EDGE('',*,*,#47187,.F.);
#66258=ORIENTED_EDGE('',*,*,#48302,.T.);
#66259=ORIENTED_EDGE('',*,*,#48303,.T.);
#66260=ORIENTED_EDGE('',*,*,#48304,.T.);
#66261=ORIENTED_EDGE('',*,*,#47216,.T.);
#66262=ORIENTED_EDGE('',*,*,#47219,.T.);
#66263=ORIENTED_EDGE('',*,*,#47212,.T.);
#66264=ORIENTED_EDGE('',*,*,#47210,.T.);
#66265=ORIENTED_EDGE('',*,*,#47208,.T.);
#66266=ORIENTED_EDGE('',*,*,#47206,.T.);
#66267=ORIENTED_EDGE('',*,*,#47204,.T.);
#66268=ORIENTED_EDGE('',*,*,#47202,.T.);
#66269=ORIENTED_EDGE('',*,*,#47200,.T.);
#66270=ORIENTED_EDGE('',*,*,#47198,.T.);
#66271=ORIENTED_EDGE('',*,*,#47195,.T.);
#66272=ORIENTED_EDGE('',*,*,#47194,.T.);
#66273=ORIENTED_EDGE('',*,*,#47192,.T.);
#66274=ORIENTED_EDGE('',*,*,#47190,.T.);
#66275=ORIENTED_EDGE('',*,*,#47188,.T.);
#66276=ORIENTED_EDGE('',*,*,#47217,.T.);
#66277=ORIENTED_EDGE('',*,*,#48304,.F.);
#66278=ORIENTED_EDGE('',*,*,#48305,.F.);
#66279=ORIENTED_EDGE('',*,*,#48306,.F.);
#66280=ORIENTED_EDGE('',*,*,#48307,.T.);
#66281=ORIENTED_EDGE('',*,*,#47218,.T.);
#66282=ORIENTED_EDGE('',*,*,#48308,.T.);
#66283=ORIENTED_EDGE('',*,*,#47221,.F.);
#66284=ORIENTED_EDGE('',*,*,#47220,.T.);
#66285=ORIENTED_EDGE('',*,*,#48307,.F.);
#66286=ORIENTED_EDGE('',*,*,#48309,.T.);
#66287=ORIENTED_EDGE('',*,*,#48310,.T.);
#66288=ORIENTED_EDGE('',*,*,#47234,.T.);
#66289=ORIENTED_EDGE('',*,*,#48311,.T.);
#66290=ORIENTED_EDGE('',*,*,#47231,.T.);
#66291=ORIENTED_EDGE('',*,*,#48310,.F.);
#66292=ORIENTED_EDGE('',*,*,#48312,.T.);
#66293=ORIENTED_EDGE('',*,*,#48313,.F.);
#66294=ORIENTED_EDGE('',*,*,#47228,.F.);
#66295=ORIENTED_EDGE('',*,*,#48314,.F.);
#66296=ORIENTED_EDGE('',*,*,#47251,.T.);
#66297=ORIENTED_EDGE('',*,*,#47249,.T.);
#66298=ORIENTED_EDGE('',*,*,#47247,.T.);
#66299=ORIENTED_EDGE('',*,*,#47245,.T.);
#66300=ORIENTED_EDGE('',*,*,#47243,.T.);
#66301=ORIENTED_EDGE('',*,*,#47241,.T.);
#66302=ORIENTED_EDGE('',*,*,#47239,.T.);
#66303=ORIENTED_EDGE('',*,*,#47237,.T.);
#66304=ORIENTED_EDGE('',*,*,#47235,.T.);
#66305=ORIENTED_EDGE('',*,*,#47232,.T.);
#66306=ORIENTED_EDGE('',*,*,#47229,.T.);
#66307=ORIENTED_EDGE('',*,*,#48313,.T.);
#66308=ORIENTED_EDGE('',*,*,#48315,.T.);
#66309=ORIENTED_EDGE('',*,*,#48316,.T.);
#66310=ORIENTED_EDGE('',*,*,#47840,.T.);
#66311=ORIENTED_EDGE('',*,*,#47226,.T.);
#66312=ORIENTED_EDGE('',*,*,#47224,.T.);
#66313=ORIENTED_EDGE('',*,*,#48126,.T.);
#66314=ORIENTED_EDGE('',*,*,#48207,.T.);
#66315=ORIENTED_EDGE('',*,*,#47274,.T.);
#66316=ORIENTED_EDGE('',*,*,#48243,.T.);
#66317=ORIENTED_EDGE('',*,*,#47270,.T.);
#66318=ORIENTED_EDGE('',*,*,#48253,.T.);
#66319=ORIENTED_EDGE('',*,*,#48317,.T.);
#66320=ORIENTED_EDGE('',*,*,#48318,.T.);
#66321=ORIENTED_EDGE('',*,*,#48319,.T.);
#66322=ORIENTED_EDGE('',*,*,#47277,.T.);
#66323=ORIENTED_EDGE('',*,*,#47267,.T.);
#66324=ORIENTED_EDGE('',*,*,#47265,.T.);
#66325=ORIENTED_EDGE('',*,*,#47263,.T.);
#66326=ORIENTED_EDGE('',*,*,#47262,.T.);
#66327=ORIENTED_EDGE('',*,*,#47260,.T.);
#66328=ORIENTED_EDGE('',*,*,#47258,.T.);
#66329=ORIENTED_EDGE('',*,*,#48075,.T.);
#66330=ORIENTED_EDGE('',*,*,#47253,.T.);
#66331=ORIENTED_EDGE('',*,*,#48252,.T.);
#66332=ORIENTED_EDGE('',*,*,#48320,.F.);
#66333=ORIENTED_EDGE('',*,*,#48321,.F.);
#66334=ORIENTED_EDGE('',*,*,#48317,.F.);
#66335=ORIENTED_EDGE('',*,*,#48319,.F.);
#66336=ORIENTED_EDGE('',*,*,#48322,.T.);
#66337=ORIENTED_EDGE('',*,*,#48323,.F.);
#66338=ORIENTED_EDGE('',*,*,#47278,.T.);
#66339=ORIENTED_EDGE('',*,*,#48323,.T.);
#66340=ORIENTED_EDGE('',*,*,#48324,.T.);
#66341=ORIENTED_EDGE('',*,*,#48325,.T.);
#66342=ORIENTED_EDGE('',*,*,#47280,.T.);
#66343=ORIENTED_EDGE('',*,*,#48325,.F.);
#66344=ORIENTED_EDGE('',*,*,#48326,.T.);
#66345=ORIENTED_EDGE('',*,*,#48327,.F.);
#66346=ORIENTED_EDGE('',*,*,#47300,.F.);
#66347=ORIENTED_EDGE('',*,*,#47312,.T.);
#66348=ORIENTED_EDGE('',*,*,#47310,.T.);
#66349=ORIENTED_EDGE('',*,*,#47307,.T.);
#66350=ORIENTED_EDGE('',*,*,#47305,.T.);
#66351=ORIENTED_EDGE('',*,*,#47303,.T.);
#66352=ORIENTED_EDGE('',*,*,#47301,.T.);
#66353=ORIENTED_EDGE('',*,*,#48327,.T.);
#66354=ORIENTED_EDGE('',*,*,#48328,.T.);
#66355=ORIENTED_EDGE('',*,*,#48329,.T.);
#66356=ORIENTED_EDGE('',*,*,#47318,.T.);
#66357=ORIENTED_EDGE('',*,*,#47299,.T.);
#66358=ORIENTED_EDGE('',*,*,#47296,.T.);
#66359=ORIENTED_EDGE('',*,*,#47294,.T.);
#66360=ORIENTED_EDGE('',*,*,#47292,.T.);
#66361=ORIENTED_EDGE('',*,*,#47290,.T.);
#66362=ORIENTED_EDGE('',*,*,#47288,.T.);
#66363=ORIENTED_EDGE('',*,*,#47286,.T.);
#66364=ORIENTED_EDGE('',*,*,#47284,.T.);
#66365=ORIENTED_EDGE('',*,*,#47314,.T.);
#66366=ORIENTED_EDGE('',*,*,#48330,.F.);
#66367=ORIENTED_EDGE('',*,*,#48331,.F.);
#66368=ORIENTED_EDGE('',*,*,#48294,.F.);
#66369=ORIENTED_EDGE('',*,*,#48332,.T.);
#66370=ORIENTED_EDGE('',*,*,#48333,.F.);
#66371=ORIENTED_EDGE('',*,*,#47316,.F.);
#66372=ORIENTED_EDGE('',*,*,#48329,.F.);
#66373=ORIENTED_EDGE('',*,*,#47319,.T.);
#66374=ORIENTED_EDGE('',*,*,#47317,.T.);
#66375=ORIENTED_EDGE('',*,*,#48334,.T.);
#66376=ORIENTED_EDGE('',*,*,#47313,.T.);
#66377=ORIENTED_EDGE('',*,*,#48215,.T.);
#66378=ORIENTED_EDGE('',*,*,#48335,.T.);
#66379=ORIENTED_EDGE('',*,*,#48129,.T.);
#66380=ORIENTED_EDGE('',*,*,#47328,.T.);
#66381=ORIENTED_EDGE('',*,*,#47326,.T.);
#66382=ORIENTED_EDGE('',*,*,#47324,.T.);
#66383=ORIENTED_EDGE('',*,*,#47321,.T.);
#66384=ORIENTED_EDGE('',*,*,#47378,.T.);
#66385=ORIENTED_EDGE('',*,*,#48336,.T.);
#66386=ORIENTED_EDGE('',*,*,#48337,.T.);
#66387=ORIENTED_EDGE('',*,*,#48338,.T.);
#66388=ORIENTED_EDGE('',*,*,#47332,.T.);
#66389=ORIENTED_EDGE('',*,*,#48338,.F.);
#66390=ORIENTED_EDGE('',*,*,#48339,.T.);
#66391=ORIENTED_EDGE('',*,*,#48340,.F.);
#66392=ORIENTED_EDGE('',*,*,#47333,.T.);
#66393=ORIENTED_EDGE('',*,*,#48340,.T.);
#66394=ORIENTED_EDGE('',*,*,#48341,.T.);
#66395=ORIENTED_EDGE('',*,*,#48342,.T.);
#66396=ORIENTED_EDGE('',*,*,#47335,.T.);
#66397=ORIENTED_EDGE('',*,*,#48342,.F.);
#66398=ORIENTED_EDGE('',*,*,#48343,.T.);
#66399=ORIENTED_EDGE('',*,*,#48344,.F.);
#66400=ORIENTED_EDGE('',*,*,#47338,.F.);
#66401=ORIENTED_EDGE('',*,*,#47345,.T.);
#66402=ORIENTED_EDGE('',*,*,#48204,.T.);
#66403=ORIENTED_EDGE('',*,*,#47341,.T.);
#66404=ORIENTED_EDGE('',*,*,#47339,.T.);
#66405=ORIENTED_EDGE('',*,*,#48344,.T.);
#66406=ORIENTED_EDGE('',*,*,#48345,.T.);
#66407=ORIENTED_EDGE('',*,*,#48346,.T.);
#66408=ORIENTED_EDGE('',*,*,#48234,.T.);
#66409=ORIENTED_EDGE('',*,*,#48235,.T.);
#66410=ORIENTED_EDGE('',*,*,#48346,.F.);
#66411=ORIENTED_EDGE('',*,*,#48347,.F.);
#66412=ORIENTED_EDGE('',*,*,#48348,.F.);
#66413=ORIENTED_EDGE('',*,*,#48349,.T.);
#66414=ORIENTED_EDGE('',*,*,#48350,.F.);
#66415=ORIENTED_EDGE('',*,*,#47891,.F.);
#66416=ORIENTED_EDGE('',*,*,#48351,.F.);
#66417=ORIENTED_EDGE('',*,*,#48350,.T.);
#66418=ORIENTED_EDGE('',*,*,#48352,.T.);
#66419=ORIENTED_EDGE('',*,*,#48353,.T.);
#66420=ORIENTED_EDGE('',*,*,#47357,.T.);
#66421=ORIENTED_EDGE('',*,*,#48142,.T.);
#66422=ORIENTED_EDGE('',*,*,#48354,.T.);
#66423=ORIENTED_EDGE('',*,*,#48143,.T.);
#66424=ORIENTED_EDGE('',*,*,#47353,.T.);
#66425=ORIENTED_EDGE('',*,*,#47351,.T.);
#66426=ORIENTED_EDGE('',*,*,#47348,.T.);
#66427=ORIENTED_EDGE('',*,*,#47892,.T.);
#66428=ORIENTED_EDGE('',*,*,#48353,.F.);
#66429=ORIENTED_EDGE('',*,*,#48355,.T.);
#66430=ORIENTED_EDGE('',*,*,#48356,.F.);
#66431=ORIENTED_EDGE('',*,*,#47358,.T.);
#66432=ORIENTED_EDGE('',*,*,#48356,.T.);
#66433=ORIENTED_EDGE('',*,*,#48357,.T.);
#66434=ORIENTED_EDGE('',*,*,#48358,.T.);
#66435=ORIENTED_EDGE('',*,*,#47361,.T.);
#66436=ORIENTED_EDGE('',*,*,#48358,.F.);
#66437=ORIENTED_EDGE('',*,*,#48359,.T.);
#66438=ORIENTED_EDGE('',*,*,#48360,.F.);
#66439=ORIENTED_EDGE('',*,*,#47363,.F.);
#66440=ORIENTED_EDGE('',*,*,#48360,.T.);
#66441=ORIENTED_EDGE('',*,*,#48361,.T.);
#66442=ORIENTED_EDGE('',*,*,#48362,.T.);
#66443=ORIENTED_EDGE('',*,*,#47382,.T.);
#66444=ORIENTED_EDGE('',*,*,#47376,.T.);
#66445=ORIENTED_EDGE('',*,*,#47373,.T.);
#66446=ORIENTED_EDGE('',*,*,#47371,.T.);
#66447=ORIENTED_EDGE('',*,*,#47369,.T.);
#66448=ORIENTED_EDGE('',*,*,#48135,.T.);
#66449=ORIENTED_EDGE('',*,*,#48363,.T.);
#66450=ORIENTED_EDGE('',*,*,#48136,.T.);
#66451=ORIENTED_EDGE('',*,*,#47364,.T.);
#66452=ORIENTED_EDGE('',*,*,#48364,.T.);
#66453=ORIENTED_EDGE('',*,*,#48336,.F.);
#66454=ORIENTED_EDGE('',*,*,#47377,.F.);
#66455=ORIENTED_EDGE('',*,*,#48365,.F.);
#66456=ORIENTED_EDGE('',*,*,#48366,.T.);
#66457=ORIENTED_EDGE('',*,*,#48367,.F.);
#66458=ORIENTED_EDGE('',*,*,#47380,.F.);
#66459=ORIENTED_EDGE('',*,*,#48362,.F.);
#66460=ORIENTED_EDGE('',*,*,#47383,.T.);
#66461=ORIENTED_EDGE('',*,*,#47381,.T.);
#66462=ORIENTED_EDGE('',*,*,#48368,.T.);
#66463=ORIENTED_EDGE('',*,*,#47379,.T.);
#66464=ORIENTED_EDGE('',*,*,#47411,.T.);
#66465=ORIENTED_EDGE('',*,*,#47410,.T.);
#66466=ORIENTED_EDGE('',*,*,#47408,.T.);
#66467=ORIENTED_EDGE('',*,*,#47406,.T.);
#66468=ORIENTED_EDGE('',*,*,#47404,.T.);
#66469=ORIENTED_EDGE('',*,*,#47402,.T.);
#66470=ORIENTED_EDGE('',*,*,#47400,.T.);
#66471=ORIENTED_EDGE('',*,*,#47398,.T.);
#66472=ORIENTED_EDGE('',*,*,#47396,.T.);
#66473=ORIENTED_EDGE('',*,*,#47394,.T.);
#66474=ORIENTED_EDGE('',*,*,#47392,.T.);
#66475=ORIENTED_EDGE('',*,*,#47539,.T.);
#66476=ORIENTED_EDGE('',*,*,#48369,.T.);
#66477=ORIENTED_EDGE('',*,*,#48370,.T.);
#66478=ORIENTED_EDGE('',*,*,#48371,.T.);
#66479=ORIENTED_EDGE('',*,*,#47412,.T.);
#66480=ORIENTED_EDGE('',*,*,#47387,.T.);
#66481=ORIENTED_EDGE('',*,*,#47385,.T.);
#66482=ORIENTED_EDGE('',*,*,#48371,.F.);
#66483=ORIENTED_EDGE('',*,*,#48372,.T.);
#66484=ORIENTED_EDGE('',*,*,#48373,.F.);
#66485=ORIENTED_EDGE('',*,*,#47413,.T.);
#66486=ORIENTED_EDGE('',*,*,#48373,.T.);
#66487=ORIENTED_EDGE('',*,*,#48374,.T.);
#66488=ORIENTED_EDGE('',*,*,#48375,.T.);
#66489=ORIENTED_EDGE('',*,*,#47415,.T.);
#66490=ORIENTED_EDGE('',*,*,#48375,.F.);
#66491=ORIENTED_EDGE('',*,*,#48376,.T.);
#66492=ORIENTED_EDGE('',*,*,#48377,.F.);
#66493=ORIENTED_EDGE('',*,*,#47417,.F.);
#66494=ORIENTED_EDGE('',*,*,#48377,.T.);
#66495=ORIENTED_EDGE('',*,*,#48378,.T.);
#66496=ORIENTED_EDGE('',*,*,#48379,.T.);
#66497=ORIENTED_EDGE('',*,*,#47446,.T.);
#66498=ORIENTED_EDGE('',*,*,#47449,.T.);
#66499=ORIENTED_EDGE('',*,*,#47442,.T.);
#66500=ORIENTED_EDGE('',*,*,#47440,.T.);
#66501=ORIENTED_EDGE('',*,*,#47438,.T.);
#66502=ORIENTED_EDGE('',*,*,#47436,.T.);
#66503=ORIENTED_EDGE('',*,*,#47434,.T.);
#66504=ORIENTED_EDGE('',*,*,#47432,.T.);
#66505=ORIENTED_EDGE('',*,*,#47430,.T.);
#66506=ORIENTED_EDGE('',*,*,#47428,.T.);
#66507=ORIENTED_EDGE('',*,*,#47425,.T.);
#66508=ORIENTED_EDGE('',*,*,#47424,.T.);
#66509=ORIENTED_EDGE('',*,*,#47422,.T.);
#66510=ORIENTED_EDGE('',*,*,#47420,.T.);
#66511=ORIENTED_EDGE('',*,*,#47418,.T.);
#66512=ORIENTED_EDGE('',*,*,#47447,.T.);
#66513=ORIENTED_EDGE('',*,*,#48379,.F.);
#66514=ORIENTED_EDGE('',*,*,#48380,.F.);
#66515=ORIENTED_EDGE('',*,*,#48381,.F.);
#66516=ORIENTED_EDGE('',*,*,#48382,.T.);
#66517=ORIENTED_EDGE('',*,*,#47448,.T.);
#66518=ORIENTED_EDGE('',*,*,#48383,.T.);
#66519=ORIENTED_EDGE('',*,*,#47451,.F.);
#66520=ORIENTED_EDGE('',*,*,#47450,.T.);
#66521=ORIENTED_EDGE('',*,*,#48382,.F.);
#66522=ORIENTED_EDGE('',*,*,#48384,.T.);
#66523=ORIENTED_EDGE('',*,*,#47474,.T.);
#66524=ORIENTED_EDGE('',*,*,#48025,.T.);
#66525=ORIENTED_EDGE('',*,*,#48031,.T.);
#66526=ORIENTED_EDGE('',*,*,#47473,.T.);
#66527=ORIENTED_EDGE('',*,*,#47470,.T.);
#66528=ORIENTED_EDGE('',*,*,#47468,.T.);
#66529=ORIENTED_EDGE('',*,*,#47466,.T.);
#66530=ORIENTED_EDGE('',*,*,#47464,.T.);
#66531=ORIENTED_EDGE('',*,*,#47462,.T.);
#66532=ORIENTED_EDGE('',*,*,#47460,.T.);
#66533=ORIENTED_EDGE('',*,*,#47476,.T.);
#66534=ORIENTED_EDGE('',*,*,#48385,.T.);
#66535=ORIENTED_EDGE('',*,*,#48386,.T.);
#66536=ORIENTED_EDGE('',*,*,#48387,.T.);
#66537=ORIENTED_EDGE('',*,*,#48216,.T.);
#66538=ORIENTED_EDGE('',*,*,#47456,.T.);
#66539=ORIENTED_EDGE('',*,*,#47454,.T.);
#66540=ORIENTED_EDGE('',*,*,#47475,.T.);
#66541=ORIENTED_EDGE('',*,*,#48388,.F.);
#66542=ORIENTED_EDGE('',*,*,#48389,.F.);
#66543=ORIENTED_EDGE('',*,*,#48385,.F.);
#66544=ORIENTED_EDGE('',*,*,#48390,.T.);
#66545=ORIENTED_EDGE('',*,*,#48391,.F.);
#66546=ORIENTED_EDGE('',*,*,#48230,.F.);
#66547=ORIENTED_EDGE('',*,*,#48392,.F.);
#66548=ORIENTED_EDGE('',*,*,#48082,.T.);
#66549=ORIENTED_EDGE('',*,*,#47500,.T.);
#66550=ORIENTED_EDGE('',*,*,#47496,.T.);
#66551=ORIENTED_EDGE('',*,*,#47495,.T.);
#66552=ORIENTED_EDGE('',*,*,#47492,.T.);
#66553=ORIENTED_EDGE('',*,*,#48231,.T.);
#66554=ORIENTED_EDGE('',*,*,#48391,.T.);
#66555=ORIENTED_EDGE('',*,*,#48393,.T.);
#66556=ORIENTED_EDGE('',*,*,#48394,.T.);
#66557=ORIENTED_EDGE('',*,*,#47503,.T.);
#66558=ORIENTED_EDGE('',*,*,#47490,.T.);
#66559=ORIENTED_EDGE('',*,*,#47488,.T.);
#66560=ORIENTED_EDGE('',*,*,#47485,.T.);
#66561=ORIENTED_EDGE('',*,*,#47484,.T.);
#66562=ORIENTED_EDGE('',*,*,#47482,.T.);
#66563=ORIENTED_EDGE('',*,*,#47480,.T.);
#66564=ORIENTED_EDGE('',*,*,#48394,.F.);
#66565=ORIENTED_EDGE('',*,*,#48395,.T.);
#66566=ORIENTED_EDGE('',*,*,#48396,.F.);
#66567=ORIENTED_EDGE('',*,*,#47501,.F.);
#66568=ORIENTED_EDGE('',*,*,#48396,.T.);
#66569=ORIENTED_EDGE('',*,*,#48397,.T.);
#66570=ORIENTED_EDGE('',*,*,#48398,.T.);
#66571=ORIENTED_EDGE('',*,*,#47504,.T.);
#66572=ORIENTED_EDGE('',*,*,#48398,.F.);
#66573=ORIENTED_EDGE('',*,*,#48399,.T.);
#66574=ORIENTED_EDGE('',*,*,#48400,.F.);
#66575=ORIENTED_EDGE('',*,*,#47522,.F.);
#66576=ORIENTED_EDGE('',*,*,#47534,.T.);
#66577=ORIENTED_EDGE('',*,*,#47532,.T.);
#66578=ORIENTED_EDGE('',*,*,#47529,.T.);
#66579=ORIENTED_EDGE('',*,*,#47527,.T.);
#66580=ORIENTED_EDGE('',*,*,#47525,.T.);
#66581=ORIENTED_EDGE('',*,*,#47523,.T.);
#66582=ORIENTED_EDGE('',*,*,#48400,.T.);
#66583=ORIENTED_EDGE('',*,*,#48401,.T.);
#66584=ORIENTED_EDGE('',*,*,#48402,.T.);
#66585=ORIENTED_EDGE('',*,*,#47540,.T.);
#66586=ORIENTED_EDGE('',*,*,#47519,.T.);
#66587=ORIENTED_EDGE('',*,*,#47517,.T.);
#66588=ORIENTED_EDGE('',*,*,#47515,.T.);
#66589=ORIENTED_EDGE('',*,*,#47514,.T.);
#66590=ORIENTED_EDGE('',*,*,#47512,.T.);
#66591=ORIENTED_EDGE('',*,*,#47510,.T.);
#66592=ORIENTED_EDGE('',*,*,#47508,.T.);
#66593=ORIENTED_EDGE('',*,*,#47538,.T.);
#66594=ORIENTED_EDGE('',*,*,#48403,.F.);
#66595=ORIENTED_EDGE('',*,*,#48404,.F.);
#66596=ORIENTED_EDGE('',*,*,#48369,.F.);
#66597=ORIENTED_EDGE('',*,*,#47541,.T.);
#66598=ORIENTED_EDGE('',*,*,#48402,.F.);
#66599=ORIENTED_EDGE('',*,*,#48405,.F.);
#66600=ORIENTED_EDGE('',*,*,#48406,.F.);
#66601=ORIENTED_EDGE('',*,*,#47543,.T.);
#66602=ORIENTED_EDGE('',*,*,#47542,.T.);
#66603=ORIENTED_EDGE('',*,*,#48407,.T.);
#66604=ORIENTED_EDGE('',*,*,#47537,.T.);
#66605=ORIENTED_EDGE('',*,*,#47535,.T.);
#66606=ORIENTED_EDGE('',*,*,#47563,.T.);
#66607=ORIENTED_EDGE('',*,*,#47562,.T.);
#66608=ORIENTED_EDGE('',*,*,#47559,.T.);
#66609=ORIENTED_EDGE('',*,*,#47557,.T.);
#66610=ORIENTED_EDGE('',*,*,#47555,.T.);
#66611=ORIENTED_EDGE('',*,*,#47846,.T.);
#66612=ORIENTED_EDGE('',*,*,#48408,.T.);
#66613=ORIENTED_EDGE('',*,*,#48409,.T.);
#66614=ORIENTED_EDGE('',*,*,#48410,.T.);
#66615=ORIENTED_EDGE('',*,*,#47566,.T.);
#66616=ORIENTED_EDGE('',*,*,#47553,.T.);
#66617=ORIENTED_EDGE('',*,*,#47550,.T.);
#66618=ORIENTED_EDGE('',*,*,#47548,.T.);
#66619=ORIENTED_EDGE('',*,*,#47546,.T.);
#66620=ORIENTED_EDGE('',*,*,#48411,.T.);
#66621=ORIENTED_EDGE('',*,*,#48412,.F.);
#66622=ORIENTED_EDGE('',*,*,#47564,.F.);
#66623=ORIENTED_EDGE('',*,*,#48410,.F.);
#66624=ORIENTED_EDGE('',*,*,#47567,.T.);
#66625=ORIENTED_EDGE('',*,*,#47565,.T.);
#66626=ORIENTED_EDGE('',*,*,#48413,.T.);
#66627=ORIENTED_EDGE('',*,*,#47588,.T.);
#66628=ORIENTED_EDGE('',*,*,#48414,.T.);
#66629=ORIENTED_EDGE('',*,*,#48415,.T.);
#66630=ORIENTED_EDGE('',*,*,#48416,.T.);
#66631=ORIENTED_EDGE('',*,*,#47591,.T.);
#66632=ORIENTED_EDGE('',*,*,#47586,.T.);
#66633=ORIENTED_EDGE('',*,*,#47584,.T.);
#66634=ORIENTED_EDGE('',*,*,#47582,.T.);
#66635=ORIENTED_EDGE('',*,*,#47580,.T.);
#66636=ORIENTED_EDGE('',*,*,#47578,.T.);
#66637=ORIENTED_EDGE('',*,*,#47576,.T.);
#66638=ORIENTED_EDGE('',*,*,#47574,.T.);
#66639=ORIENTED_EDGE('',*,*,#47573,.T.);
#66640=ORIENTED_EDGE('',*,*,#47571,.T.);
#66641=ORIENTED_EDGE('',*,*,#47590,.T.);
#66642=ORIENTED_EDGE('',*,*,#47589,.T.);
#66643=ORIENTED_EDGE('',*,*,#48417,.F.);
#66644=ORIENTED_EDGE('',*,*,#48418,.F.);
#66645=ORIENTED_EDGE('',*,*,#48414,.F.);
#66646=ORIENTED_EDGE('',*,*,#48416,.F.);
#66647=ORIENTED_EDGE('',*,*,#48419,.T.);
#66648=ORIENTED_EDGE('',*,*,#48420,.F.);
#66649=ORIENTED_EDGE('',*,*,#47592,.T.);
#66650=ORIENTED_EDGE('',*,*,#48420,.T.);
#66651=ORIENTED_EDGE('',*,*,#48421,.T.);
#66652=ORIENTED_EDGE('',*,*,#48422,.T.);
#66653=ORIENTED_EDGE('',*,*,#47594,.T.);
#66654=ORIENTED_EDGE('',*,*,#48422,.F.);
#66655=ORIENTED_EDGE('',*,*,#48423,.T.);
#66656=ORIENTED_EDGE('',*,*,#48424,.F.);
#66657=ORIENTED_EDGE('',*,*,#47596,.F.);
#66658=ORIENTED_EDGE('',*,*,#48424,.T.);
#66659=ORIENTED_EDGE('',*,*,#48425,.T.);
#66660=ORIENTED_EDGE('',*,*,#48426,.T.);
#66661=ORIENTED_EDGE('',*,*,#47618,.T.);
#66662=ORIENTED_EDGE('',*,*,#47615,.T.);
#66663=ORIENTED_EDGE('',*,*,#47611,.T.);
#66664=ORIENTED_EDGE('',*,*,#47609,.T.);
#66665=ORIENTED_EDGE('',*,*,#47607,.T.);
#66666=ORIENTED_EDGE('',*,*,#47605,.T.);
#66667=ORIENTED_EDGE('',*,*,#47602,.T.);
#66668=ORIENTED_EDGE('',*,*,#47601,.T.);
#66669=ORIENTED_EDGE('',*,*,#47599,.T.);
#66670=ORIENTED_EDGE('',*,*,#47597,.T.);
#66671=ORIENTED_EDGE('',*,*,#48427,.T.);
#66672=ORIENTED_EDGE('',*,*,#48428,.F.);
#66673=ORIENTED_EDGE('',*,*,#47616,.F.);
#66674=ORIENTED_EDGE('',*,*,#48426,.F.);
#66675=ORIENTED_EDGE('',*,*,#47619,.T.);
#66676=ORIENTED_EDGE('',*,*,#47617,.T.);
#66677=ORIENTED_EDGE('',*,*,#48429,.T.);
#66678=ORIENTED_EDGE('',*,*,#47636,.T.);
#66679=ORIENTED_EDGE('',*,*,#48430,.T.);
#66680=ORIENTED_EDGE('',*,*,#48431,.T.);
#66681=ORIENTED_EDGE('',*,*,#48432,.T.);
#66682=ORIENTED_EDGE('',*,*,#47641,.T.);
#66683=ORIENTED_EDGE('',*,*,#47634,.T.);
#66684=ORIENTED_EDGE('',*,*,#47633,.T.);
#66685=ORIENTED_EDGE('',*,*,#47631,.T.);
#66686=ORIENTED_EDGE('',*,*,#47629,.T.);
#66687=ORIENTED_EDGE('',*,*,#47627,.T.);
#66688=ORIENTED_EDGE('',*,*,#47625,.T.);
#66689=ORIENTED_EDGE('',*,*,#47623,.T.);
#66690=ORIENTED_EDGE('',*,*,#47638,.T.);
#66691=ORIENTED_EDGE('',*,*,#47637,.T.);
#66692=ORIENTED_EDGE('',*,*,#48433,.F.);
#66693=ORIENTED_EDGE('',*,*,#48434,.F.);
#66694=ORIENTED_EDGE('',*,*,#48430,.F.);
#66695=ORIENTED_EDGE('',*,*,#48432,.F.);
#66696=ORIENTED_EDGE('',*,*,#48435,.T.);
#66697=ORIENTED_EDGE('',*,*,#48436,.F.);
#66698=ORIENTED_EDGE('',*,*,#47639,.F.);
#66699=ORIENTED_EDGE('',*,*,#48436,.T.);
#66700=ORIENTED_EDGE('',*,*,#48437,.T.);
#66701=ORIENTED_EDGE('',*,*,#48438,.T.);
#66702=ORIENTED_EDGE('',*,*,#47642,.F.);
#66703=ORIENTED_EDGE('',*,*,#48438,.F.);
#66704=ORIENTED_EDGE('',*,*,#48439,.T.);
#66705=ORIENTED_EDGE('',*,*,#48440,.F.);
#66706=ORIENTED_EDGE('',*,*,#47644,.F.);
#66707=ORIENTED_EDGE('',*,*,#48440,.T.);
#66708=ORIENTED_EDGE('',*,*,#48441,.T.);
#66709=ORIENTED_EDGE('',*,*,#48442,.T.);
#66710=ORIENTED_EDGE('',*,*,#47662,.T.);
#66711=ORIENTED_EDGE('',*,*,#47659,.T.);
#66712=ORIENTED_EDGE('',*,*,#47657,.T.);
#66713=ORIENTED_EDGE('',*,*,#47655,.T.);
#66714=ORIENTED_EDGE('',*,*,#47653,.T.);
#66715=ORIENTED_EDGE('',*,*,#47651,.T.);
#66716=ORIENTED_EDGE('',*,*,#47648,.T.);
#66717=ORIENTED_EDGE('',*,*,#47647,.T.);
#66718=ORIENTED_EDGE('',*,*,#47645,.T.);
#66719=ORIENTED_EDGE('',*,*,#47663,.T.);
#66720=ORIENTED_EDGE('',*,*,#48442,.F.);
#66721=ORIENTED_EDGE('',*,*,#48443,.F.);
#66722=ORIENTED_EDGE('',*,*,#48444,.F.);
#66723=ORIENTED_EDGE('',*,*,#47665,.T.);
#66724=ORIENTED_EDGE('',*,*,#47664,.T.);
#66725=ORIENTED_EDGE('',*,*,#48445,.T.);
#66726=ORIENTED_EDGE('',*,*,#47682,.T.);
#66727=ORIENTED_EDGE('',*,*,#48446,.T.);
#66728=ORIENTED_EDGE('',*,*,#48447,.T.);
#66729=ORIENTED_EDGE('',*,*,#48448,.T.);
#66730=ORIENTED_EDGE('',*,*,#47687,.T.);
#66731=ORIENTED_EDGE('',*,*,#47680,.T.);
#66732=ORIENTED_EDGE('',*,*,#47679,.T.);
#66733=ORIENTED_EDGE('',*,*,#47677,.T.);
#66734=ORIENTED_EDGE('',*,*,#47675,.T.);
#66735=ORIENTED_EDGE('',*,*,#47673,.T.);
#66736=ORIENTED_EDGE('',*,*,#47671,.T.);
#66737=ORIENTED_EDGE('',*,*,#47669,.T.);
#66738=ORIENTED_EDGE('',*,*,#47684,.T.);
#66739=ORIENTED_EDGE('',*,*,#47683,.T.);
#66740=ORIENTED_EDGE('',*,*,#48449,.F.);
#66741=ORIENTED_EDGE('',*,*,#48450,.F.);
#66742=ORIENTED_EDGE('',*,*,#48446,.F.);
#66743=ORIENTED_EDGE('',*,*,#48448,.F.);
#66744=ORIENTED_EDGE('',*,*,#48451,.T.);
#66745=ORIENTED_EDGE('',*,*,#48452,.F.);
#66746=ORIENTED_EDGE('',*,*,#47685,.F.);
#66747=ORIENTED_EDGE('',*,*,#48452,.T.);
#66748=ORIENTED_EDGE('',*,*,#48453,.T.);
#66749=ORIENTED_EDGE('',*,*,#48454,.T.);
#66750=ORIENTED_EDGE('',*,*,#47688,.F.);
#66751=ORIENTED_EDGE('',*,*,#48454,.F.);
#66752=ORIENTED_EDGE('',*,*,#48455,.T.);
#66753=ORIENTED_EDGE('',*,*,#48456,.F.);
#66754=ORIENTED_EDGE('',*,*,#47690,.F.);
#66755=ORIENTED_EDGE('',*,*,#48456,.T.);
#66756=ORIENTED_EDGE('',*,*,#48457,.T.);
#66757=ORIENTED_EDGE('',*,*,#48458,.T.);
#66758=ORIENTED_EDGE('',*,*,#47708,.T.);
#66759=ORIENTED_EDGE('',*,*,#47705,.T.);
#66760=ORIENTED_EDGE('',*,*,#47703,.T.);
#66761=ORIENTED_EDGE('',*,*,#47701,.T.);
#66762=ORIENTED_EDGE('',*,*,#47699,.T.);
#66763=ORIENTED_EDGE('',*,*,#47697,.T.);
#66764=ORIENTED_EDGE('',*,*,#47694,.T.);
#66765=ORIENTED_EDGE('',*,*,#47693,.T.);
#66766=ORIENTED_EDGE('',*,*,#47691,.T.);
#66767=ORIENTED_EDGE('',*,*,#47709,.T.);
#66768=ORIENTED_EDGE('',*,*,#48458,.F.);
#66769=ORIENTED_EDGE('',*,*,#48459,.F.);
#66770=ORIENTED_EDGE('',*,*,#48460,.F.);
#66771=ORIENTED_EDGE('',*,*,#47711,.T.);
#66772=ORIENTED_EDGE('',*,*,#47710,.T.);
#66773=ORIENTED_EDGE('',*,*,#48461,.T.);
#66774=ORIENTED_EDGE('',*,*,#47728,.T.);
#66775=ORIENTED_EDGE('',*,*,#47726,.T.);
#66776=ORIENTED_EDGE('',*,*,#47725,.T.);
#66777=ORIENTED_EDGE('',*,*,#47723,.T.);
#66778=ORIENTED_EDGE('',*,*,#47721,.T.);
#66779=ORIENTED_EDGE('',*,*,#47719,.T.);
#66780=ORIENTED_EDGE('',*,*,#47717,.T.);
#66781=ORIENTED_EDGE('',*,*,#47715,.T.);
#66782=ORIENTED_EDGE('',*,*,#47730,.T.);
#66783=ORIENTED_EDGE('',*,*,#48462,.T.);
#66784=ORIENTED_EDGE('',*,*,#48463,.T.);
#66785=ORIENTED_EDGE('',*,*,#48464,.T.);
#66786=ORIENTED_EDGE('',*,*,#47731,.T.);
#66787=ORIENTED_EDGE('',*,*,#47729,.T.);
#66788=ORIENTED_EDGE('',*,*,#48465,.F.);
#66789=ORIENTED_EDGE('',*,*,#48466,.F.);
#66790=ORIENTED_EDGE('',*,*,#48462,.F.);
#66791=ORIENTED_EDGE('',*,*,#48464,.F.);
#66792=ORIENTED_EDGE('',*,*,#48467,.T.);
#66793=ORIENTED_EDGE('',*,*,#48468,.F.);
#66794=ORIENTED_EDGE('',*,*,#47732,.T.);
#66795=ORIENTED_EDGE('',*,*,#48468,.T.);
#66796=ORIENTED_EDGE('',*,*,#48469,.T.);
#66797=ORIENTED_EDGE('',*,*,#48470,.T.);
#66798=ORIENTED_EDGE('',*,*,#47734,.F.);
#66799=ORIENTED_EDGE('',*,*,#48470,.F.);
#66800=ORIENTED_EDGE('',*,*,#48471,.T.);
#66801=ORIENTED_EDGE('',*,*,#48472,.F.);
#66802=ORIENTED_EDGE('',*,*,#47736,.F.);
#66803=ORIENTED_EDGE('',*,*,#48472,.T.);
#66804=ORIENTED_EDGE('',*,*,#48473,.T.);
#66805=ORIENTED_EDGE('',*,*,#48474,.T.);
#66806=ORIENTED_EDGE('',*,*,#47754,.T.);
#66807=ORIENTED_EDGE('',*,*,#47751,.T.);
#66808=ORIENTED_EDGE('',*,*,#47749,.T.);
#66809=ORIENTED_EDGE('',*,*,#47747,.T.);
#66810=ORIENTED_EDGE('',*,*,#47745,.T.);
#66811=ORIENTED_EDGE('',*,*,#47743,.T.);
#66812=ORIENTED_EDGE('',*,*,#47740,.T.);
#66813=ORIENTED_EDGE('',*,*,#47739,.T.);
#66814=ORIENTED_EDGE('',*,*,#47737,.T.);
#66815=ORIENTED_EDGE('',*,*,#47755,.T.);
#66816=ORIENTED_EDGE('',*,*,#48474,.F.);
#66817=ORIENTED_EDGE('',*,*,#48475,.F.);
#66818=ORIENTED_EDGE('',*,*,#48476,.F.);
#66819=ORIENTED_EDGE('',*,*,#47757,.T.);
#66820=ORIENTED_EDGE('',*,*,#47756,.T.);
#66821=ORIENTED_EDGE('',*,*,#48477,.T.);
#66822=ORIENTED_EDGE('',*,*,#47776,.T.);
#66823=ORIENTED_EDGE('',*,*,#48478,.T.);
#66824=ORIENTED_EDGE('',*,*,#48479,.T.);
#66825=ORIENTED_EDGE('',*,*,#48480,.T.);
#66826=ORIENTED_EDGE('',*,*,#47779,.T.);
#66827=ORIENTED_EDGE('',*,*,#47774,.T.);
#66828=ORIENTED_EDGE('',*,*,#47772,.T.);
#66829=ORIENTED_EDGE('',*,*,#47770,.T.);
#66830=ORIENTED_EDGE('',*,*,#47768,.T.);
#66831=ORIENTED_EDGE('',*,*,#47766,.T.);
#66832=ORIENTED_EDGE('',*,*,#47764,.T.);
#66833=ORIENTED_EDGE('',*,*,#47763,.T.);
#66834=ORIENTED_EDGE('',*,*,#47761,.T.);
#66835=ORIENTED_EDGE('',*,*,#47778,.T.);
#66836=ORIENTED_EDGE('',*,*,#47777,.T.);
#66837=ORIENTED_EDGE('',*,*,#48481,.F.);
#66838=ORIENTED_EDGE('',*,*,#48482,.F.);
#66839=ORIENTED_EDGE('',*,*,#48478,.F.);
#66840=ORIENTED_EDGE('',*,*,#48480,.F.);
#66841=ORIENTED_EDGE('',*,*,#48483,.T.);
#66842=ORIENTED_EDGE('',*,*,#48484,.F.);
#66843=ORIENTED_EDGE('',*,*,#47780,.T.);
#66844=ORIENTED_EDGE('',*,*,#48484,.T.);
#66845=ORIENTED_EDGE('',*,*,#48485,.T.);
#66846=ORIENTED_EDGE('',*,*,#48486,.T.);
#66847=ORIENTED_EDGE('',*,*,#47782,.T.);
#66848=ORIENTED_EDGE('',*,*,#48486,.F.);
#66849=ORIENTED_EDGE('',*,*,#48487,.T.);
#66850=ORIENTED_EDGE('',*,*,#48488,.F.);
#66851=ORIENTED_EDGE('',*,*,#47784,.F.);
#66852=ORIENTED_EDGE('',*,*,#48488,.T.);
#66853=ORIENTED_EDGE('',*,*,#48489,.T.);
#66854=ORIENTED_EDGE('',*,*,#48490,.T.);
#66855=ORIENTED_EDGE('',*,*,#47808,.T.);
#66856=ORIENTED_EDGE('',*,*,#47805,.T.);
#66857=ORIENTED_EDGE('',*,*,#47801,.T.);
#66858=ORIENTED_EDGE('',*,*,#47799,.T.);
#66859=ORIENTED_EDGE('',*,*,#47797,.T.);
#66860=ORIENTED_EDGE('',*,*,#47795,.T.);
#66861=ORIENTED_EDGE('',*,*,#47792,.T.);
#66862=ORIENTED_EDGE('',*,*,#47791,.T.);
#66863=ORIENTED_EDGE('',*,*,#47789,.T.);
#66864=ORIENTED_EDGE('',*,*,#47787,.T.);
#66865=ORIENTED_EDGE('',*,*,#47785,.T.);
#66866=ORIENTED_EDGE('',*,*,#48491,.T.);
#66867=ORIENTED_EDGE('',*,*,#48492,.F.);
#66868=ORIENTED_EDGE('',*,*,#47806,.F.);
#66869=ORIENTED_EDGE('',*,*,#48490,.F.);
#66870=ORIENTED_EDGE('',*,*,#47809,.T.);
#66871=ORIENTED_EDGE('',*,*,#47807,.T.);
#66872=ORIENTED_EDGE('',*,*,#48493,.T.);
#66873=ORIENTED_EDGE('',*,*,#47819,.T.);
#66874=ORIENTED_EDGE('',*,*,#48494,.T.);
#66875=ORIENTED_EDGE('',*,*,#48495,.F.);
#66876=ORIENTED_EDGE('',*,*,#47816,.F.);
#66877=ORIENTED_EDGE('',*,*,#48496,.F.);
#66878=ORIENTED_EDGE('',*,*,#47832,.T.);
#66879=ORIENTED_EDGE('',*,*,#47830,.T.);
#66880=ORIENTED_EDGE('',*,*,#47828,.T.);
#66881=ORIENTED_EDGE('',*,*,#47826,.T.);
#66882=ORIENTED_EDGE('',*,*,#47824,.T.);
#66883=ORIENTED_EDGE('',*,*,#47822,.T.);
#66884=ORIENTED_EDGE('',*,*,#47820,.T.);
#66885=ORIENTED_EDGE('',*,*,#47817,.T.);
#66886=ORIENTED_EDGE('',*,*,#48495,.T.);
#66887=ORIENTED_EDGE('',*,*,#48497,.T.);
#66888=ORIENTED_EDGE('',*,*,#48498,.T.);
#66889=ORIENTED_EDGE('',*,*,#47833,.T.);
#66890=ORIENTED_EDGE('',*,*,#47814,.T.);
#66891=ORIENTED_EDGE('',*,*,#47812,.T.);
#66892=ORIENTED_EDGE('',*,*,#48498,.F.);
#66893=ORIENTED_EDGE('',*,*,#48499,.T.);
#66894=ORIENTED_EDGE('',*,*,#48500,.T.);
#66895=ORIENTED_EDGE('',*,*,#48501,.F.);
#66896=ORIENTED_EDGE('',*,*,#47834,.T.);
#66897=ORIENTED_EDGE('',*,*,#48501,.T.);
#66898=ORIENTED_EDGE('',*,*,#48502,.T.);
#66899=ORIENTED_EDGE('',*,*,#48503,.T.);
#66900=ORIENTED_EDGE('',*,*,#47836,.T.);
#66901=ORIENTED_EDGE('',*,*,#48503,.F.);
#66902=ORIENTED_EDGE('',*,*,#48504,.T.);
#66903=ORIENTED_EDGE('',*,*,#48505,.T.);
#66904=ORIENTED_EDGE('',*,*,#48288,.F.);
#66905=ORIENTED_EDGE('',*,*,#47838,.F.);
#66906=ORIENTED_EDGE('',*,*,#48316,.F.);
#66907=ORIENTED_EDGE('',*,*,#48506,.T.);
#66908=ORIENTED_EDGE('',*,*,#48507,.T.);
#66909=ORIENTED_EDGE('',*,*,#48508,.F.);
#66910=ORIENTED_EDGE('',*,*,#47841,.T.);
#66911=ORIENTED_EDGE('',*,*,#48508,.T.);
#66912=ORIENTED_EDGE('',*,*,#48509,.T.);
#66913=ORIENTED_EDGE('',*,*,#48510,.T.);
#66914=ORIENTED_EDGE('',*,*,#47843,.T.);
#66915=ORIENTED_EDGE('',*,*,#48511,.T.);
#66916=ORIENTED_EDGE('',*,*,#48512,.T.);
#66917=ORIENTED_EDGE('',*,*,#48408,.F.);
#66918=ORIENTED_EDGE('',*,*,#47845,.F.);
#66919=ORIENTED_EDGE('',*,*,#48510,.F.);
#66920=ORIENTED_EDGE('',*,*,#48513,.T.);
#66921=ORIENTED_EDGE('',*,*,#48514,.T.);
#66922=ORIENTED_EDGE('',*,*,#48515,.T.);
#66923=ORIENTED_EDGE('',*,*,#48196,.T.);
#66924=ORIENTED_EDGE('',*,*,#48516,.T.);
#66925=ORIENTED_EDGE('',*,*,#48517,.T.);
#66926=ORIENTED_EDGE('',*,*,#48518,.T.);
#66927=ORIENTED_EDGE('',*,*,#48515,.F.);
#66928=ORIENTED_EDGE('',*,*,#48519,.T.);
#66929=ORIENTED_EDGE('',*,*,#48520,.F.);
#66930=ORIENTED_EDGE('',*,*,#48197,.F.);
#66931=ORIENTED_EDGE('',*,*,#48520,.T.);
#66932=ORIENTED_EDGE('',*,*,#48521,.T.);
#66933=ORIENTED_EDGE('',*,*,#48522,.T.);
#66934=ORIENTED_EDGE('',*,*,#48194,.F.);
#66935=ORIENTED_EDGE('',*,*,#48522,.F.);
#66936=ORIENTED_EDGE('',*,*,#48523,.T.);
#66937=ORIENTED_EDGE('',*,*,#48524,.F.);
#66938=ORIENTED_EDGE('',*,*,#48191,.F.);
#66939=ORIENTED_EDGE('',*,*,#48524,.T.);
#66940=ORIENTED_EDGE('',*,*,#48525,.T.);
#66941=ORIENTED_EDGE('',*,*,#48526,.T.);
#66942=ORIENTED_EDGE('',*,*,#47850,.T.);
#66943=ORIENTED_EDGE('',*,*,#48187,.T.);
#66944=ORIENTED_EDGE('',*,*,#48527,.T.);
#66945=ORIENTED_EDGE('',*,*,#48188,.T.);
#66946=ORIENTED_EDGE('',*,*,#48528,.T.);
#66947=ORIENTED_EDGE('',*,*,#48529,.F.);
#66948=ORIENTED_EDGE('',*,*,#47847,.F.);
#66949=ORIENTED_EDGE('',*,*,#48526,.F.);
#66950=ORIENTED_EDGE('',*,*,#48530,.T.);
#66951=ORIENTED_EDGE('',*,*,#47848,.T.);
#66952=ORIENTED_EDGE('',*,*,#48531,.T.);
#66953=ORIENTED_EDGE('',*,*,#47854,.T.);
#66954=ORIENTED_EDGE('',*,*,#48532,.T.);
#66955=ORIENTED_EDGE('',*,*,#48533,.T.);
#66956=ORIENTED_EDGE('',*,*,#48534,.T.);
#66957=ORIENTED_EDGE('',*,*,#48178,.T.);
#66958=ORIENTED_EDGE('',*,*,#48535,.T.);
#66959=ORIENTED_EDGE('',*,*,#48180,.T.);
#66960=ORIENTED_EDGE('',*,*,#47852,.T.);
#66961=ORIENTED_EDGE('',*,*,#47851,.F.);
#66962=ORIENTED_EDGE('',*,*,#48536,.F.);
#66963=ORIENTED_EDGE('',*,*,#48537,.F.);
#66964=ORIENTED_EDGE('',*,*,#48532,.F.);
#66965=ORIENTED_EDGE('',*,*,#48534,.F.);
#66966=ORIENTED_EDGE('',*,*,#48538,.T.);
#66967=ORIENTED_EDGE('',*,*,#48539,.F.);
#66968=ORIENTED_EDGE('',*,*,#48179,.F.);
#66969=ORIENTED_EDGE('',*,*,#48539,.T.);
#66970=ORIENTED_EDGE('',*,*,#48540,.T.);
#66971=ORIENTED_EDGE('',*,*,#48541,.T.);
#66972=ORIENTED_EDGE('',*,*,#48176,.F.);
#66973=ORIENTED_EDGE('',*,*,#48541,.F.);
#66974=ORIENTED_EDGE('',*,*,#48542,.T.);
#66975=ORIENTED_EDGE('',*,*,#48543,.F.);
#66976=ORIENTED_EDGE('',*,*,#48173,.F.);
#66977=ORIENTED_EDGE('',*,*,#48543,.T.);
#66978=ORIENTED_EDGE('',*,*,#48544,.T.);
#66979=ORIENTED_EDGE('',*,*,#48545,.T.);
#66980=ORIENTED_EDGE('',*,*,#47861,.T.);
#66981=ORIENTED_EDGE('',*,*,#47858,.T.);
#66982=ORIENTED_EDGE('',*,*,#48166,.T.);
#66983=ORIENTED_EDGE('',*,*,#48168,.T.);
#66984=ORIENTED_EDGE('',*,*,#48546,.T.);
#66985=ORIENTED_EDGE('',*,*,#48170,.T.);
#66986=ORIENTED_EDGE('',*,*,#48547,.T.);
#66987=ORIENTED_EDGE('',*,*,#48548,.F.);
#66988=ORIENTED_EDGE('',*,*,#47859,.F.);
#66989=ORIENTED_EDGE('',*,*,#48545,.F.);
#66990=ORIENTED_EDGE('',*,*,#48163,.T.);
#66991=ORIENTED_EDGE('',*,*,#47860,.T.);
#66992=ORIENTED_EDGE('',*,*,#48549,.T.);
#66993=ORIENTED_EDGE('',*,*,#47865,.T.);
#66994=ORIENTED_EDGE('',*,*,#48550,.T.);
#66995=ORIENTED_EDGE('',*,*,#48551,.F.);
#66996=ORIENTED_EDGE('',*,*,#47862,.F.);
#66997=ORIENTED_EDGE('',*,*,#48552,.F.);
#66998=ORIENTED_EDGE('',*,*,#48551,.T.);
#66999=ORIENTED_EDGE('',*,*,#48553,.T.);
#67000=ORIENTED_EDGE('',*,*,#48554,.T.);
#67001=ORIENTED_EDGE('',*,*,#47873,.T.);
#67002=ORIENTED_EDGE('',*,*,#48156,.T.);
#67003=ORIENTED_EDGE('',*,*,#48555,.T.);
#67004=ORIENTED_EDGE('',*,*,#48157,.T.);
#67005=ORIENTED_EDGE('',*,*,#47869,.T.);
#67006=ORIENTED_EDGE('',*,*,#47866,.T.);
#67007=ORIENTED_EDGE('',*,*,#47863,.T.);
#67008=ORIENTED_EDGE('',*,*,#48554,.F.);
#67009=ORIENTED_EDGE('',*,*,#48556,.T.);
#67010=ORIENTED_EDGE('',*,*,#48557,.F.);
#67011=ORIENTED_EDGE('',*,*,#47874,.T.);
#67012=ORIENTED_EDGE('',*,*,#48557,.T.);
#67013=ORIENTED_EDGE('',*,*,#48558,.T.);
#67014=ORIENTED_EDGE('',*,*,#48559,.T.);
#67015=ORIENTED_EDGE('',*,*,#47877,.T.);
#67016=ORIENTED_EDGE('',*,*,#48559,.F.);
#67017=ORIENTED_EDGE('',*,*,#48560,.T.);
#67018=ORIENTED_EDGE('',*,*,#48561,.F.);
#67019=ORIENTED_EDGE('',*,*,#47879,.F.);
#67020=ORIENTED_EDGE('',*,*,#48561,.T.);
#67021=ORIENTED_EDGE('',*,*,#48562,.T.);
#67022=ORIENTED_EDGE('',*,*,#48563,.T.);
#67023=ORIENTED_EDGE('',*,*,#47896,.T.);
#67024=ORIENTED_EDGE('',*,*,#47890,.T.);
#67025=ORIENTED_EDGE('',*,*,#47887,.T.);
#67026=ORIENTED_EDGE('',*,*,#47885,.T.);
#67027=ORIENTED_EDGE('',*,*,#48149,.T.);
#67028=ORIENTED_EDGE('',*,*,#48564,.T.);
#67029=ORIENTED_EDGE('',*,*,#48150,.T.);
#67030=ORIENTED_EDGE('',*,*,#47880,.T.);
#67031=ORIENTED_EDGE('',*,*,#48565,.T.);
#67032=ORIENTED_EDGE('',*,*,#48566,.F.);
#67033=ORIENTED_EDGE('',*,*,#47894,.F.);
#67034=ORIENTED_EDGE('',*,*,#48563,.F.);
#67035=ORIENTED_EDGE('',*,*,#47897,.F.);
#67036=ORIENTED_EDGE('',*,*,#47895,.T.);
#67037=ORIENTED_EDGE('',*,*,#48567,.T.);
#67038=ORIENTED_EDGE('',*,*,#48568,.T.);
#67039=ORIENTED_EDGE('',*,*,#48569,.T.);
#67040=ORIENTED_EDGE('',*,*,#47893,.T.);
#67041=ORIENTED_EDGE('',*,*,#48570,.F.);
#67042=ORIENTED_EDGE('',*,*,#48571,.T.);
#67043=ORIENTED_EDGE('',*,*,#48572,.F.);
#67044=ORIENTED_EDGE('',*,*,#47898,.F.);
#67045=ORIENTED_EDGE('',*,*,#48572,.T.);
#67046=ORIENTED_EDGE('',*,*,#48573,.T.);
#67047=ORIENTED_EDGE('',*,*,#48574,.T.);
#67048=ORIENTED_EDGE('',*,*,#47917,.T.);
#67049=ORIENTED_EDGE('',*,*,#47914,.T.);
#67050=ORIENTED_EDGE('',*,*,#47912,.T.);
#67051=ORIENTED_EDGE('',*,*,#47910,.T.);
#67052=ORIENTED_EDGE('',*,*,#47907,.T.);
#67053=ORIENTED_EDGE('',*,*,#48065,.T.);
#67054=ORIENTED_EDGE('',*,*,#48575,.T.);
#67055=ORIENTED_EDGE('',*,*,#48067,.T.);
#67056=ORIENTED_EDGE('',*,*,#47904,.T.);
#67057=ORIENTED_EDGE('',*,*,#47902,.T.);
#67058=ORIENTED_EDGE('',*,*,#47899,.T.);
#67059=ORIENTED_EDGE('',*,*,#47918,.T.);
#67060=ORIENTED_EDGE('',*,*,#48574,.F.);
#67061=ORIENTED_EDGE('',*,*,#48576,.F.);
#67062=ORIENTED_EDGE('',*,*,#48577,.F.);
#67063=ORIENTED_EDGE('',*,*,#47920,.T.);
#67064=ORIENTED_EDGE('',*,*,#47919,.T.);
#67065=ORIENTED_EDGE('',*,*,#48578,.T.);
#67066=ORIENTED_EDGE('',*,*,#47937,.T.);
#67067=ORIENTED_EDGE('',*,*,#48059,.T.);
#67068=ORIENTED_EDGE('',*,*,#48579,.T.);
#67069=ORIENTED_EDGE('',*,*,#48062,.T.);
#67070=ORIENTED_EDGE('',*,*,#47936,.T.);
#67071=ORIENTED_EDGE('',*,*,#47933,.T.);
#67072=ORIENTED_EDGE('',*,*,#47931,.T.);
#67073=ORIENTED_EDGE('',*,*,#47929,.T.);
#67074=ORIENTED_EDGE('',*,*,#47939,.T.);
#67075=ORIENTED_EDGE('',*,*,#48580,.T.);
#67076=ORIENTED_EDGE('',*,*,#48581,.T.);
#67077=ORIENTED_EDGE('',*,*,#48582,.T.);
#67078=ORIENTED_EDGE('',*,*,#47940,.T.);
#67079=ORIENTED_EDGE('',*,*,#47925,.T.);
#67080=ORIENTED_EDGE('',*,*,#47923,.T.);
#67081=ORIENTED_EDGE('',*,*,#47938,.T.);
#67082=ORIENTED_EDGE('',*,*,#48583,.F.);
#67083=ORIENTED_EDGE('',*,*,#48584,.F.);
#67084=ORIENTED_EDGE('',*,*,#48580,.F.);
#67085=ORIENTED_EDGE('',*,*,#48582,.F.);
#67086=ORIENTED_EDGE('',*,*,#48585,.T.);
#67087=ORIENTED_EDGE('',*,*,#48586,.F.);
#67088=ORIENTED_EDGE('',*,*,#47941,.T.);
#67089=ORIENTED_EDGE('',*,*,#48586,.T.);
#67090=ORIENTED_EDGE('',*,*,#48587,.T.);
#67091=ORIENTED_EDGE('',*,*,#48588,.T.);
#67092=ORIENTED_EDGE('',*,*,#47943,.T.);
#67093=ORIENTED_EDGE('',*,*,#48588,.F.);
#67094=ORIENTED_EDGE('',*,*,#48589,.T.);
#67095=ORIENTED_EDGE('',*,*,#48590,.F.);
#67096=ORIENTED_EDGE('',*,*,#47945,.F.);
#67097=ORIENTED_EDGE('',*,*,#48590,.T.);
#67098=ORIENTED_EDGE('',*,*,#48591,.T.);
#67099=ORIENTED_EDGE('',*,*,#48592,.T.);
#67100=ORIENTED_EDGE('',*,*,#47963,.T.);
#67101=ORIENTED_EDGE('',*,*,#47960,.T.);
#67102=ORIENTED_EDGE('',*,*,#47958,.T.);
#67103=ORIENTED_EDGE('',*,*,#47956,.T.);
#67104=ORIENTED_EDGE('',*,*,#47953,.T.);
#67105=ORIENTED_EDGE('',*,*,#48051,.T.);
#67106=ORIENTED_EDGE('',*,*,#48593,.T.);
#67107=ORIENTED_EDGE('',*,*,#48053,.T.);
#67108=ORIENTED_EDGE('',*,*,#47950,.T.);
#67109=ORIENTED_EDGE('',*,*,#47948,.T.);
#67110=ORIENTED_EDGE('',*,*,#47946,.T.);
#67111=ORIENTED_EDGE('',*,*,#47964,.T.);
#67112=ORIENTED_EDGE('',*,*,#48592,.F.);
#67113=ORIENTED_EDGE('',*,*,#48594,.F.);
#67114=ORIENTED_EDGE('',*,*,#48595,.F.);
#67115=ORIENTED_EDGE('',*,*,#48596,.F.);
#67116=ORIENTED_EDGE('',*,*,#47966,.T.);
#67117=ORIENTED_EDGE('',*,*,#47965,.T.);
#67118=ORIENTED_EDGE('',*,*,#48597,.T.);
#67119=ORIENTED_EDGE('',*,*,#47978,.T.);
#67120=ORIENTED_EDGE('',*,*,#48045,.T.);
#67121=ORIENTED_EDGE('',*,*,#48598,.T.);
#67122=ORIENTED_EDGE('',*,*,#48048,.T.);
#67123=ORIENTED_EDGE('',*,*,#47977,.T.);
#67124=ORIENTED_EDGE('',*,*,#47974,.T.);
#67125=ORIENTED_EDGE('',*,*,#47972,.T.);
#67126=ORIENTED_EDGE('',*,*,#47970,.T.);
#67127=ORIENTED_EDGE('',*,*,#47980,.T.);
#67128=ORIENTED_EDGE('',*,*,#48599,.T.);
#67129=ORIENTED_EDGE('',*,*,#48600,.T.);
#67130=ORIENTED_EDGE('',*,*,#48601,.T.);
#67131=ORIENTED_EDGE('',*,*,#47982,.T.);
#67132=ORIENTED_EDGE('',*,*,#47979,.T.);
#67133=ORIENTED_EDGE('',*,*,#48602,.F.);
#67134=ORIENTED_EDGE('',*,*,#48603,.F.);
#67135=ORIENTED_EDGE('',*,*,#48599,.F.);
#67136=ORIENTED_EDGE('',*,*,#48601,.F.);
#67137=ORIENTED_EDGE('',*,*,#48604,.T.);
#67138=ORIENTED_EDGE('',*,*,#48605,.F.);
#67139=ORIENTED_EDGE('',*,*,#47983,.T.);
#67140=ORIENTED_EDGE('',*,*,#48605,.T.);
#67141=ORIENTED_EDGE('',*,*,#48606,.T.);
#67142=ORIENTED_EDGE('',*,*,#48607,.T.);
#67143=ORIENTED_EDGE('',*,*,#47985,.F.);
#67144=ORIENTED_EDGE('',*,*,#48607,.F.);
#67145=ORIENTED_EDGE('',*,*,#48608,.T.);
#67146=ORIENTED_EDGE('',*,*,#48609,.F.);
#67147=ORIENTED_EDGE('',*,*,#47988,.F.);
#67148=ORIENTED_EDGE('',*,*,#48609,.T.);
#67149=ORIENTED_EDGE('',*,*,#48610,.T.);
#67150=ORIENTED_EDGE('',*,*,#48611,.T.);
#67151=ORIENTED_EDGE('',*,*,#48002,.T.);
#67152=ORIENTED_EDGE('',*,*,#47999,.T.);
#67153=ORIENTED_EDGE('',*,*,#47997,.T.);
#67154=ORIENTED_EDGE('',*,*,#47995,.T.);
#67155=ORIENTED_EDGE('',*,*,#47992,.T.);
#67156=ORIENTED_EDGE('',*,*,#48037,.T.);
#67157=ORIENTED_EDGE('',*,*,#48612,.T.);
#67158=ORIENTED_EDGE('',*,*,#48039,.T.);
#67159=ORIENTED_EDGE('',*,*,#47989,.T.);
#67160=ORIENTED_EDGE('',*,*,#48003,.T.);
#67161=ORIENTED_EDGE('',*,*,#48611,.F.);
#67162=ORIENTED_EDGE('',*,*,#48613,.F.);
#67163=ORIENTED_EDGE('',*,*,#48614,.F.);
#67164=ORIENTED_EDGE('',*,*,#48615,.F.);
#67165=ORIENTED_EDGE('',*,*,#48005,.T.);
#67166=ORIENTED_EDGE('',*,*,#48004,.T.);
#67167=ORIENTED_EDGE('',*,*,#48616,.T.);
#67168=ORIENTED_EDGE('',*,*,#48017,.T.);
#67169=ORIENTED_EDGE('',*,*,#48617,.T.);
#67170=ORIENTED_EDGE('',*,*,#48618,.T.);
#67171=ORIENTED_EDGE('',*,*,#48034,.T.);
#67172=ORIENTED_EDGE('',*,*,#48016,.T.);
#67173=ORIENTED_EDGE('',*,*,#48013,.T.);
#67174=ORIENTED_EDGE('',*,*,#48011,.T.);
#67175=ORIENTED_EDGE('',*,*,#48009,.T.);
#67176=ORIENTED_EDGE('',*,*,#48019,.T.);
#67177=ORIENTED_EDGE('',*,*,#48619,.T.);
#67178=ORIENTED_EDGE('',*,*,#48620,.T.);
#67179=ORIENTED_EDGE('',*,*,#48621,.T.);
#67180=ORIENTED_EDGE('',*,*,#48622,.T.);
#67181=ORIENTED_EDGE('',*,*,#48018,.T.);
#67182=ORIENTED_EDGE('',*,*,#48623,.F.);
#67183=ORIENTED_EDGE('',*,*,#48624,.F.);
#67184=ORIENTED_EDGE('',*,*,#48619,.F.);
#67185=ORIENTED_EDGE('',*,*,#48621,.F.);
#67186=ORIENTED_EDGE('',*,*,#48625,.T.);
#67187=ORIENTED_EDGE('',*,*,#48626,.F.);
#67188=ORIENTED_EDGE('',*,*,#48627,.T.);
#67189=ORIENTED_EDGE('',*,*,#48628,.T.);
#67190=ORIENTED_EDGE('',*,*,#48622,.F.);
#67191=ORIENTED_EDGE('',*,*,#48627,.F.);
#67192=ORIENTED_EDGE('',*,*,#48629,.F.);
#67193=ORIENTED_EDGE('',*,*,#48630,.F.);
#67194=ORIENTED_EDGE('',*,*,#48631,.T.);
#67195=ORIENTED_EDGE('',*,*,#48617,.F.);
#67196=ORIENTED_EDGE('',*,*,#48628,.F.);
#67197=ORIENTED_EDGE('',*,*,#48632,.T.);
#67198=ORIENTED_EDGE('',*,*,#48633,.F.);
#67199=ORIENTED_EDGE('',*,*,#48634,.F.);
#67200=ORIENTED_EDGE('',*,*,#48021,.F.);
#67201=ORIENTED_EDGE('',*,*,#48634,.T.);
#67202=ORIENTED_EDGE('',*,*,#48635,.F.);
#67203=ORIENTED_EDGE('',*,*,#48027,.F.);
#67204=ORIENTED_EDGE('',*,*,#48023,.F.);
#67205=ORIENTED_EDGE('',*,*,#48030,.T.);
#67206=ORIENTED_EDGE('',*,*,#48028,.T.);
#67207=ORIENTED_EDGE('',*,*,#48636,.F.);
#67208=ORIENTED_EDGE('',*,*,#48637,.T.);
#67209=ORIENTED_EDGE('',*,*,#48083,.F.);
#67210=ORIENTED_EDGE('',*,*,#48026,.T.);
#67211=ORIENTED_EDGE('',*,*,#48638,.T.);
#67212=ORIENTED_EDGE('',*,*,#48639,.F.);
#67213=ORIENTED_EDGE('',*,*,#48640,.F.);
#67214=ORIENTED_EDGE('',*,*,#48631,.F.);
#67215=ORIENTED_EDGE('',*,*,#48640,.T.);
#67216=ORIENTED_EDGE('',*,*,#48641,.F.);
#67217=ORIENTED_EDGE('',*,*,#48032,.F.);
#67218=ORIENTED_EDGE('',*,*,#48618,.F.);
#67219=ORIENTED_EDGE('',*,*,#48642,.F.);
#67220=ORIENTED_EDGE('',*,*,#48038,.T.);
#67221=ORIENTED_EDGE('',*,*,#48035,.F.);
#67222=ORIENTED_EDGE('',*,*,#48033,.T.);
#67223=ORIENTED_EDGE('',*,*,#48643,.T.);
#67224=ORIENTED_EDGE('',*,*,#48612,.F.);
#67225=ORIENTED_EDGE('',*,*,#48036,.F.);
#67226=ORIENTED_EDGE('',*,*,#48644,.F.);
#67227=ORIENTED_EDGE('',*,*,#48645,.F.);
#67228=ORIENTED_EDGE('',*,*,#48040,.F.);
#67229=ORIENTED_EDGE('',*,*,#48643,.F.);
#67230=ORIENTED_EDGE('',*,*,#48646,.F.);
#67231=ORIENTED_EDGE('',*,*,#48645,.T.);
#67232=ORIENTED_EDGE('',*,*,#48647,.F.);
#67233=ORIENTED_EDGE('',*,*,#48648,.F.);
#67234=ORIENTED_EDGE('',*,*,#48042,.F.);
#67235=ORIENTED_EDGE('',*,*,#48648,.T.);
#67236=ORIENTED_EDGE('',*,*,#48649,.F.);
#67237=ORIENTED_EDGE('',*,*,#48650,.F.);
#67238=ORIENTED_EDGE('',*,*,#48044,.F.);
#67239=ORIENTED_EDGE('',*,*,#48650,.T.);
#67240=ORIENTED_EDGE('',*,*,#48651,.F.);
#67241=ORIENTED_EDGE('',*,*,#48046,.F.);
#67242=ORIENTED_EDGE('',*,*,#48598,.F.);
#67243=ORIENTED_EDGE('',*,*,#48652,.F.);
#67244=ORIENTED_EDGE('',*,*,#48052,.T.);
#67245=ORIENTED_EDGE('',*,*,#48049,.F.);
#67246=ORIENTED_EDGE('',*,*,#48047,.T.);
#67247=ORIENTED_EDGE('',*,*,#48653,.T.);
#67248=ORIENTED_EDGE('',*,*,#48593,.F.);
#67249=ORIENTED_EDGE('',*,*,#48050,.F.);
#67250=ORIENTED_EDGE('',*,*,#48654,.F.);
#67251=ORIENTED_EDGE('',*,*,#48655,.F.);
#67252=ORIENTED_EDGE('',*,*,#48054,.F.);
#67253=ORIENTED_EDGE('',*,*,#48653,.F.);
#67254=ORIENTED_EDGE('',*,*,#48656,.F.);
#67255=ORIENTED_EDGE('',*,*,#48655,.T.);
#67256=ORIENTED_EDGE('',*,*,#48657,.F.);
#67257=ORIENTED_EDGE('',*,*,#48658,.F.);
#67258=ORIENTED_EDGE('',*,*,#48056,.F.);
#67259=ORIENTED_EDGE('',*,*,#48658,.T.);
#67260=ORIENTED_EDGE('',*,*,#48659,.F.);
#67261=ORIENTED_EDGE('',*,*,#48660,.F.);
#67262=ORIENTED_EDGE('',*,*,#48058,.F.);
#67263=ORIENTED_EDGE('',*,*,#48660,.T.);
#67264=ORIENTED_EDGE('',*,*,#48661,.F.);
#67265=ORIENTED_EDGE('',*,*,#48060,.F.);
#67266=ORIENTED_EDGE('',*,*,#48579,.F.);
#67267=ORIENTED_EDGE('',*,*,#48662,.F.);
#67268=ORIENTED_EDGE('',*,*,#48066,.T.);
#67269=ORIENTED_EDGE('',*,*,#48063,.F.);
#67270=ORIENTED_EDGE('',*,*,#48061,.T.);
#67271=ORIENTED_EDGE('',*,*,#48663,.T.);
#67272=ORIENTED_EDGE('',*,*,#48575,.F.);
#67273=ORIENTED_EDGE('',*,*,#48064,.F.);
#67274=ORIENTED_EDGE('',*,*,#48664,.F.);
#67275=ORIENTED_EDGE('',*,*,#48663,.F.);
#67276=ORIENTED_EDGE('',*,*,#48665,.F.);
#67277=ORIENTED_EDGE('',*,*,#48632,.F.);
#67278=ORIENTED_EDGE('',*,*,#48068,.F.);
#67279=ORIENTED_EDGE('',*,*,#48072,.F.);
#67280=ORIENTED_EDGE('',*,*,#48123,.F.);
#67281=ORIENTED_EDGE('',*,*,#48069,.F.);
#67282=ORIENTED_EDGE('',*,*,#48074,.F.);
#67283=ORIENTED_EDGE('',*,*,#48666,.T.);
#67284=ORIENTED_EDGE('',*,*,#48667,.T.);
#67285=ORIENTED_EDGE('',*,*,#48666,.F.);
#67286=ORIENTED_EDGE('',*,*,#48073,.F.);
#67287=ORIENTED_EDGE('',*,*,#48077,.F.);
#67288=ORIENTED_EDGE('',*,*,#48076,.F.);
#67289=ORIENTED_EDGE('',*,*,#48081,.F.);
#67290=ORIENTED_EDGE('',*,*,#48080,.F.);
#67291=ORIENTED_EDGE('',*,*,#48668,.T.);
#67292=ORIENTED_EDGE('',*,*,#48669,.T.);
#67293=ORIENTED_EDGE('',*,*,#48668,.F.);
#67294=ORIENTED_EDGE('',*,*,#48079,.F.);
#67295=ORIENTED_EDGE('',*,*,#48670,.T.);
#67296=ORIENTED_EDGE('',*,*,#48671,.F.);
#67297=ORIENTED_EDGE('',*,*,#48672,.F.);
#67298=ORIENTED_EDGE('',*,*,#48637,.F.);
#67299=ORIENTED_EDGE('',*,*,#48672,.T.);
#67300=ORIENTED_EDGE('',*,*,#48673,.F.);
#67301=ORIENTED_EDGE('',*,*,#48674,.F.);
#67302=ORIENTED_EDGE('',*,*,#48084,.F.);
#67303=ORIENTED_EDGE('',*,*,#48674,.T.);
#67304=ORIENTED_EDGE('',*,*,#48675,.F.);
#67305=ORIENTED_EDGE('',*,*,#48676,.F.);
#67306=ORIENTED_EDGE('',*,*,#48086,.F.);
#67307=ORIENTED_EDGE('',*,*,#48676,.T.);
#67308=ORIENTED_EDGE('',*,*,#48677,.F.);
#67309=ORIENTED_EDGE('',*,*,#48678,.F.);
#67310=ORIENTED_EDGE('',*,*,#48088,.F.);
#67311=ORIENTED_EDGE('',*,*,#48678,.T.);
#67312=ORIENTED_EDGE('',*,*,#48679,.F.);
#67313=ORIENTED_EDGE('',*,*,#48680,.F.);
#67314=ORIENTED_EDGE('',*,*,#48090,.F.);
#67315=ORIENTED_EDGE('',*,*,#48680,.T.);
#67316=ORIENTED_EDGE('',*,*,#48681,.F.);
#67317=ORIENTED_EDGE('',*,*,#48682,.F.);
#67318=ORIENTED_EDGE('',*,*,#48092,.F.);
#67319=ORIENTED_EDGE('',*,*,#48682,.T.);
#67320=ORIENTED_EDGE('',*,*,#48683,.F.);
#67321=ORIENTED_EDGE('',*,*,#48684,.F.);
#67322=ORIENTED_EDGE('',*,*,#48095,.F.);
#67323=ORIENTED_EDGE('',*,*,#48684,.T.);
#67324=ORIENTED_EDGE('',*,*,#48685,.F.);
#67325=ORIENTED_EDGE('',*,*,#48686,.F.);
#67326=ORIENTED_EDGE('',*,*,#48097,.F.);
#67327=ORIENTED_EDGE('',*,*,#48686,.T.);
#67328=ORIENTED_EDGE('',*,*,#48687,.F.);
#67329=ORIENTED_EDGE('',*,*,#48688,.F.);
#67330=ORIENTED_EDGE('',*,*,#48098,.F.);
#67331=ORIENTED_EDGE('',*,*,#48688,.T.);
#67332=ORIENTED_EDGE('',*,*,#48689,.F.);
#67333=ORIENTED_EDGE('',*,*,#48690,.F.);
#67334=ORIENTED_EDGE('',*,*,#48100,.F.);
#67335=ORIENTED_EDGE('',*,*,#48690,.T.);
#67336=ORIENTED_EDGE('',*,*,#48691,.F.);
#67337=ORIENTED_EDGE('',*,*,#48692,.F.);
#67338=ORIENTED_EDGE('',*,*,#48102,.F.);
#67339=ORIENTED_EDGE('',*,*,#48692,.T.);
#67340=ORIENTED_EDGE('',*,*,#48693,.F.);
#67341=ORIENTED_EDGE('',*,*,#48694,.F.);
#67342=ORIENTED_EDGE('',*,*,#48104,.F.);
#67343=ORIENTED_EDGE('',*,*,#48694,.T.);
#67344=ORIENTED_EDGE('',*,*,#48695,.F.);
#67345=ORIENTED_EDGE('',*,*,#48696,.F.);
#67346=ORIENTED_EDGE('',*,*,#48106,.F.);
#67347=ORIENTED_EDGE('',*,*,#48696,.T.);
#67348=ORIENTED_EDGE('',*,*,#48697,.F.);
#67349=ORIENTED_EDGE('',*,*,#48698,.F.);
#67350=ORIENTED_EDGE('',*,*,#48112,.F.);
#67351=ORIENTED_EDGE('',*,*,#48698,.T.);
#67352=ORIENTED_EDGE('',*,*,#48699,.F.);
#67353=ORIENTED_EDGE('',*,*,#48700,.F.);
#67354=ORIENTED_EDGE('',*,*,#48701,.F.);
#67355=ORIENTED_EDGE('',*,*,#48702,.F.);
#67356=ORIENTED_EDGE('',*,*,#48703,.T.);
#67357=ORIENTED_EDGE('',*,*,#48108,.F.);
#67358=ORIENTED_EDGE('',*,*,#48701,.T.);
#67359=ORIENTED_EDGE('',*,*,#48114,.T.);
#67360=ORIENTED_EDGE('',*,*,#48109,.F.);
#67361=ORIENTED_EDGE('',*,*,#48704,.F.);
#67362=ORIENTED_EDGE('',*,*,#48705,.F.);
#67363=ORIENTED_EDGE('',*,*,#48704,.T.);
#67364=ORIENTED_EDGE('',*,*,#48703,.F.);
#67365=ORIENTED_EDGE('',*,*,#48706,.F.);
#67366=ORIENTED_EDGE('',*,*,#48707,.F.);
#67367=ORIENTED_EDGE('',*,*,#48708,.F.);
#67368=ORIENTED_EDGE('',*,*,#48115,.T.);
#67369=ORIENTED_EDGE('',*,*,#48709,.F.);
#67370=ORIENTED_EDGE('',*,*,#48710,.F.);
#67371=ORIENTED_EDGE('',*,*,#48127,.T.);
#67372=ORIENTED_EDGE('',*,*,#48125,.T.);
#67373=ORIENTED_EDGE('',*,*,#48124,.T.);
#67374=ORIENTED_EDGE('',*,*,#48121,.T.);
#67375=ORIENTED_EDGE('',*,*,#48119,.T.);
#67376=ORIENTED_EDGE('',*,*,#48117,.T.);
#67377=ORIENTED_EDGE('',*,*,#48708,.T.);
#67378=ORIENTED_EDGE('',*,*,#48711,.F.);
#67379=ORIENTED_EDGE('',*,*,#48712,.T.);
#67380=ORIENTED_EDGE('',*,*,#48130,.T.);
#67381=ORIENTED_EDGE('',*,*,#48335,.F.);
#67382=ORIENTED_EDGE('',*,*,#48713,.F.);
#67383=ORIENTED_EDGE('',*,*,#48714,.F.);
#67384=ORIENTED_EDGE('',*,*,#48715,.F.);
#67385=ORIENTED_EDGE('',*,*,#48133,.T.);
#67386=ORIENTED_EDGE('',*,*,#48132,.F.);
#67387=ORIENTED_EDGE('',*,*,#48131,.T.);
#67388=ORIENTED_EDGE('',*,*,#48716,.T.);
#67389=ORIENTED_EDGE('',*,*,#48363,.F.);
#67390=ORIENTED_EDGE('',*,*,#48134,.F.);
#67391=ORIENTED_EDGE('',*,*,#48717,.F.);
#67392=ORIENTED_EDGE('',*,*,#48718,.T.);
#67393=ORIENTED_EDGE('',*,*,#48137,.F.);
#67394=ORIENTED_EDGE('',*,*,#48716,.F.);
#67395=ORIENTED_EDGE('',*,*,#48719,.F.);
#67396=ORIENTED_EDGE('',*,*,#48720,.T.);
#67397=ORIENTED_EDGE('',*,*,#48139,.F.);
#67398=ORIENTED_EDGE('',*,*,#48718,.F.);
#67399=ORIENTED_EDGE('',*,*,#48721,.F.);
#67400=ORIENTED_EDGE('',*,*,#48722,.T.);
#67401=ORIENTED_EDGE('',*,*,#48141,.F.);
#67402=ORIENTED_EDGE('',*,*,#48720,.F.);
#67403=ORIENTED_EDGE('',*,*,#48723,.F.);
#67404=ORIENTED_EDGE('',*,*,#48144,.T.);
#67405=ORIENTED_EDGE('',*,*,#48354,.F.);
#67406=ORIENTED_EDGE('',*,*,#48722,.F.);
#67407=ORIENTED_EDGE('',*,*,#48724,.F.);
#67408=ORIENTED_EDGE('',*,*,#48725,.F.);
#67409=ORIENTED_EDGE('',*,*,#48147,.T.);
#67410=ORIENTED_EDGE('',*,*,#48146,.F.);
#67411=ORIENTED_EDGE('',*,*,#48145,.T.);
#67412=ORIENTED_EDGE('',*,*,#48726,.T.);
#67413=ORIENTED_EDGE('',*,*,#48564,.F.);
#67414=ORIENTED_EDGE('',*,*,#48148,.F.);
#67415=ORIENTED_EDGE('',*,*,#48727,.F.);
#67416=ORIENTED_EDGE('',*,*,#48728,.T.);
#67417=ORIENTED_EDGE('',*,*,#48151,.F.);
#67418=ORIENTED_EDGE('',*,*,#48726,.F.);
#67419=ORIENTED_EDGE('',*,*,#48729,.F.);
#67420=ORIENTED_EDGE('',*,*,#48730,.T.);
#67421=ORIENTED_EDGE('',*,*,#48153,.F.);
#67422=ORIENTED_EDGE('',*,*,#48728,.F.);
#67423=ORIENTED_EDGE('',*,*,#48731,.F.);
#67424=ORIENTED_EDGE('',*,*,#48732,.T.);
#67425=ORIENTED_EDGE('',*,*,#48155,.F.);
#67426=ORIENTED_EDGE('',*,*,#48730,.F.);
#67427=ORIENTED_EDGE('',*,*,#48733,.F.);
#67428=ORIENTED_EDGE('',*,*,#48158,.T.);
#67429=ORIENTED_EDGE('',*,*,#48555,.F.);
#67430=ORIENTED_EDGE('',*,*,#48732,.F.);
#67431=ORIENTED_EDGE('',*,*,#48734,.F.);
#67432=ORIENTED_EDGE('',*,*,#48161,.F.);
#67433=ORIENTED_EDGE('',*,*,#48159,.T.);
#67434=ORIENTED_EDGE('',*,*,#48735,.F.);
#67435=ORIENTED_EDGE('',*,*,#48736,.F.);
#67436=ORIENTED_EDGE('',*,*,#48737,.F.);
#67437=ORIENTED_EDGE('',*,*,#48164,.T.);
#67438=ORIENTED_EDGE('',*,*,#48162,.F.);
#67439=ORIENTED_EDGE('',*,*,#48736,.T.);
#67440=ORIENTED_EDGE('',*,*,#48738,.F.);
#67441=ORIENTED_EDGE('',*,*,#48739,.F.);
#67442=ORIENTED_EDGE('',*,*,#48169,.T.);
#67443=ORIENTED_EDGE('',*,*,#48737,.T.);
#67444=ORIENTED_EDGE('',*,*,#48740,.T.);
#67445=ORIENTED_EDGE('',*,*,#48546,.F.);
#67446=ORIENTED_EDGE('',*,*,#48167,.F.);
#67447=ORIENTED_EDGE('',*,*,#48741,.F.);
#67448=ORIENTED_EDGE('',*,*,#48742,.T.);
#67449=ORIENTED_EDGE('',*,*,#48171,.F.);
#67450=ORIENTED_EDGE('',*,*,#48740,.F.);
#67451=ORIENTED_EDGE('',*,*,#48743,.F.);
#67452=ORIENTED_EDGE('',*,*,#48744,.T.);
#67453=ORIENTED_EDGE('',*,*,#48174,.F.);
#67454=ORIENTED_EDGE('',*,*,#48742,.F.);
#67455=ORIENTED_EDGE('',*,*,#48745,.F.);
#67456=ORIENTED_EDGE('',*,*,#48746,.T.);
#67457=ORIENTED_EDGE('',*,*,#48177,.F.);
#67458=ORIENTED_EDGE('',*,*,#48744,.F.);
#67459=ORIENTED_EDGE('',*,*,#48747,.F.);
#67460=ORIENTED_EDGE('',*,*,#48181,.T.);
#67461=ORIENTED_EDGE('',*,*,#48535,.F.);
#67462=ORIENTED_EDGE('',*,*,#48746,.F.);
#67463=ORIENTED_EDGE('',*,*,#48748,.F.);
#67464=ORIENTED_EDGE('',*,*,#48184,.T.);
#67465=ORIENTED_EDGE('',*,*,#48530,.F.);
#67466=ORIENTED_EDGE('',*,*,#48183,.T.);
#67467=ORIENTED_EDGE('',*,*,#48182,.T.);
#67468=ORIENTED_EDGE('',*,*,#48749,.F.);
#67469=ORIENTED_EDGE('',*,*,#48185,.T.);
#67470=ORIENTED_EDGE('',*,*,#48750,.T.);
#67471=ORIENTED_EDGE('',*,*,#48527,.F.);
#67472=ORIENTED_EDGE('',*,*,#48186,.F.);
#67473=ORIENTED_EDGE('',*,*,#48751,.F.);
#67474=ORIENTED_EDGE('',*,*,#48752,.T.);
#67475=ORIENTED_EDGE('',*,*,#48189,.F.);
#67476=ORIENTED_EDGE('',*,*,#48750,.F.);
#67477=ORIENTED_EDGE('',*,*,#48753,.F.);
#67478=ORIENTED_EDGE('',*,*,#48754,.T.);
#67479=ORIENTED_EDGE('',*,*,#48192,.F.);
#67480=ORIENTED_EDGE('',*,*,#48752,.F.);
#67481=ORIENTED_EDGE('',*,*,#48755,.F.);
#67482=ORIENTED_EDGE('',*,*,#48756,.T.);
#67483=ORIENTED_EDGE('',*,*,#48195,.F.);
#67484=ORIENTED_EDGE('',*,*,#48754,.F.);
#67485=ORIENTED_EDGE('',*,*,#48757,.F.);
#67486=ORIENTED_EDGE('',*,*,#48758,.T.);
#67487=ORIENTED_EDGE('',*,*,#48516,.F.);
#67488=ORIENTED_EDGE('',*,*,#48756,.F.);
#67489=ORIENTED_EDGE('',*,*,#48759,.F.);
#67490=ORIENTED_EDGE('',*,*,#48209,.T.);
#67491=ORIENTED_EDGE('',*,*,#48208,.T.);
#67492=ORIENTED_EDGE('',*,*,#48712,.F.);
#67493=ORIENTED_EDGE('',*,*,#48760,.F.);
#67494=ORIENTED_EDGE('',*,*,#48761,.F.);
#67495=ORIENTED_EDGE('',*,*,#48211,.T.);
#67496=ORIENTED_EDGE('',*,*,#48205,.T.);
#67497=ORIENTED_EDGE('',*,*,#48202,.T.);
#67498=ORIENTED_EDGE('',*,*,#48200,.T.);
#67499=ORIENTED_EDGE('',*,*,#48762,.T.);
#67500=ORIENTED_EDGE('',*,*,#48212,.F.);
#67501=ORIENTED_EDGE('',*,*,#48210,.F.);
#67502=ORIENTED_EDGE('',*,*,#48763,.F.);
#67503=ORIENTED_EDGE('',*,*,#48713,.T.);
#67504=ORIENTED_EDGE('',*,*,#48214,.F.);
#67505=ORIENTED_EDGE('',*,*,#48762,.F.);
#67506=ORIENTED_EDGE('',*,*,#48764,.F.);
#67507=ORIENTED_EDGE('',*,*,#48765,.T.);
#67508=ORIENTED_EDGE('',*,*,#48517,.F.);
#67509=ORIENTED_EDGE('',*,*,#48758,.F.);
#67510=ORIENTED_EDGE('',*,*,#48766,.F.);
#67511=ORIENTED_EDGE('',*,*,#48767,.F.);
#67512=ORIENTED_EDGE('',*,*,#48768,.T.);
#67513=ORIENTED_EDGE('',*,*,#48518,.F.);
#67514=ORIENTED_EDGE('',*,*,#48765,.F.);
#67515=ORIENTED_EDGE('',*,*,#48769,.F.);
#67516=ORIENTED_EDGE('',*,*,#48768,.F.);
#67517=ORIENTED_EDGE('',*,*,#48770,.F.);
#67518=ORIENTED_EDGE('',*,*,#48771,.F.);
#67519=ORIENTED_EDGE('',*,*,#48513,.F.);
#67520=ORIENTED_EDGE('',*,*,#48387,.F.);
#67521=ORIENTED_EDGE('',*,*,#48772,.T.);
#67522=ORIENTED_EDGE('',*,*,#48773,.T.);
#67523=ORIENTED_EDGE('',*,*,#48774,.F.);
#67524=ORIENTED_EDGE('',*,*,#48217,.T.);
#67525=ORIENTED_EDGE('',*,*,#48774,.T.);
#67526=ORIENTED_EDGE('',*,*,#48775,.T.);
#67527=ORIENTED_EDGE('',*,*,#48776,.T.);
#67528=ORIENTED_EDGE('',*,*,#48570,.T.);
#67529=ORIENTED_EDGE('',*,*,#48219,.T.);
#67530=ORIENTED_EDGE('',*,*,#48777,.T.);
#67531=ORIENTED_EDGE('',*,*,#48232,.T.);
#67532=ORIENTED_EDGE('',*,*,#48225,.F.);
#67533=ORIENTED_EDGE('',*,*,#48226,.F.);
#67534=ORIENTED_EDGE('',*,*,#48222,.T.);
#67535=ORIENTED_EDGE('',*,*,#48778,.T.);
#67536=ORIENTED_EDGE('',*,*,#48779,.T.);
#67537=ORIENTED_EDGE('',*,*,#48780,.T.);
#67538=ORIENTED_EDGE('',*,*,#48781,.T.);
#67539=ORIENTED_EDGE('',*,*,#48782,.T.);
#67540=ORIENTED_EDGE('',*,*,#48251,.T.);
#67541=ORIENTED_EDGE('',*,*,#48247,.F.);
#67542=ORIENTED_EDGE('',*,*,#48244,.T.);
#67543=ORIENTED_EDGE('',*,*,#48242,.T.);
#67544=ORIENTED_EDGE('',*,*,#48240,.T.);
#67545=ORIENTED_EDGE('',*,*,#48238,.T.);
#67546=ORIENTED_EDGE('',*,*,#48236,.T.);
#67547=ORIENTED_EDGE('',*,*,#48783,.T.);
#67548=ORIENTED_EDGE('',*,*,#48784,.T.);
#67549=ORIENTED_EDGE('',*,*,#48785,.T.);
#67550=ORIENTED_EDGE('',*,*,#48786,.T.);
#67551=ORIENTED_EDGE('',*,*,#48787,.F.);
#67552=ORIENTED_EDGE('',*,*,#48259,.T.);
#67553=ORIENTED_EDGE('',*,*,#48254,.F.);
#67554=ORIENTED_EDGE('',*,*,#48788,.F.);
#67555=ORIENTED_EDGE('',*,*,#48789,.F.);
#67556=ORIENTED_EDGE('',*,*,#48257,.F.);
#67557=ORIENTED_EDGE('',*,*,#48261,.T.);
#67558=ORIENTED_EDGE('',*,*,#48260,.T.);
#67559=ORIENTED_EDGE('',*,*,#48790,.F.);
#67560=ORIENTED_EDGE('',*,*,#48791,.F.);
#67561=ORIENTED_EDGE('',*,*,#48792,.T.);
#67562=ORIENTED_EDGE('',*,*,#48262,.F.);
#67563=ORIENTED_EDGE('',*,*,#48789,.T.);
#67564=ORIENTED_EDGE('',*,*,#48791,.T.);
#67565=ORIENTED_EDGE('',*,*,#48793,.F.);
#67566=ORIENTED_EDGE('',*,*,#48794,.T.);
#67567=ORIENTED_EDGE('',*,*,#48264,.F.);
#67568=ORIENTED_EDGE('',*,*,#48792,.F.);
#67569=ORIENTED_EDGE('',*,*,#48795,.F.);
#67570=ORIENTED_EDGE('',*,*,#48796,.T.);
#67571=ORIENTED_EDGE('',*,*,#48266,.F.);
#67572=ORIENTED_EDGE('',*,*,#48794,.F.);
#67573=ORIENTED_EDGE('',*,*,#48797,.F.);
#67574=ORIENTED_EDGE('',*,*,#48270,.T.);
#67575=ORIENTED_EDGE('',*,*,#48268,.F.);
#67576=ORIENTED_EDGE('',*,*,#48796,.F.);
#67577=ORIENTED_EDGE('',*,*,#48798,.F.);
#67578=ORIENTED_EDGE('',*,*,#48272,.F.);
#67579=ORIENTED_EDGE('',*,*,#48271,.T.);
#67580=ORIENTED_EDGE('',*,*,#48799,.F.);
#67581=ORIENTED_EDGE('',*,*,#48275,.T.);
#67582=ORIENTED_EDGE('',*,*,#48800,.T.);
#67583=ORIENTED_EDGE('',*,*,#48276,.F.);
#67584=ORIENTED_EDGE('',*,*,#48273,.F.);
#67585=ORIENTED_EDGE('',*,*,#48801,.F.);
#67586=ORIENTED_EDGE('',*,*,#48802,.T.);
#67587=ORIENTED_EDGE('',*,*,#48278,.F.);
#67588=ORIENTED_EDGE('',*,*,#48800,.F.);
#67589=ORIENTED_EDGE('',*,*,#48803,.F.);
#67590=ORIENTED_EDGE('',*,*,#48804,.T.);
#67591=ORIENTED_EDGE('',*,*,#48280,.F.);
#67592=ORIENTED_EDGE('',*,*,#48802,.F.);
#67593=ORIENTED_EDGE('',*,*,#48805,.F.);
#67594=ORIENTED_EDGE('',*,*,#48806,.T.);
#67595=ORIENTED_EDGE('',*,*,#48282,.F.);
#67596=ORIENTED_EDGE('',*,*,#48804,.F.);
#67597=ORIENTED_EDGE('',*,*,#48807,.F.);
#67598=ORIENTED_EDGE('',*,*,#48286,.T.);
#67599=ORIENTED_EDGE('',*,*,#48284,.F.);
#67600=ORIENTED_EDGE('',*,*,#48806,.F.);
#67601=ORIENTED_EDGE('',*,*,#48808,.F.);
#67602=ORIENTED_EDGE('',*,*,#48778,.F.);
#67603=ORIENTED_EDGE('',*,*,#48287,.T.);
#67604=ORIENTED_EDGE('',*,*,#48809,.F.);
#67605=ORIENTED_EDGE('',*,*,#48810,.T.);
#67606=ORIENTED_EDGE('',*,*,#48811,.F.);
#67607=ORIENTED_EDGE('',*,*,#48812,.F.);
#67608=ORIENTED_EDGE('',*,*,#48813,.F.);
#67609=ORIENTED_EDGE('',*,*,#48505,.F.);
#67610=ORIENTED_EDGE('',*,*,#48813,.T.);
#67611=ORIENTED_EDGE('',*,*,#48814,.F.);
#67612=ORIENTED_EDGE('',*,*,#48291,.F.);
#67613=ORIENTED_EDGE('',*,*,#48289,.F.);
#67614=ORIENTED_EDGE('',*,*,#48293,.F.);
#67615=ORIENTED_EDGE('',*,*,#48292,.T.);
#67616=ORIENTED_EDGE('',*,*,#48815,.F.);
#67617=ORIENTED_EDGE('',*,*,#48788,.T.);
#67618=ORIENTED_EDGE('',*,*,#48331,.T.);
#67619=ORIENTED_EDGE('',*,*,#48816,.F.);
#67620=ORIENTED_EDGE('',*,*,#48817,.F.);
#67621=ORIENTED_EDGE('',*,*,#48295,.F.);
#67622=ORIENTED_EDGE('',*,*,#48818,.T.);
#67623=ORIENTED_EDGE('',*,*,#48297,.F.);
#67624=ORIENTED_EDGE('',*,*,#48817,.T.);
#67625=ORIENTED_EDGE('',*,*,#48819,.F.);
#67626=ORIENTED_EDGE('',*,*,#48820,.T.);
#67627=ORIENTED_EDGE('',*,*,#48299,.F.);
#67628=ORIENTED_EDGE('',*,*,#48818,.F.);
#67629=ORIENTED_EDGE('',*,*,#48821,.F.);
#67630=ORIENTED_EDGE('',*,*,#48822,.T.);
#67631=ORIENTED_EDGE('',*,*,#48301,.F.);
#67632=ORIENTED_EDGE('',*,*,#48820,.F.);
#67633=ORIENTED_EDGE('',*,*,#48823,.F.);
#67634=ORIENTED_EDGE('',*,*,#48305,.T.);
#67635=ORIENTED_EDGE('',*,*,#48303,.F.);
#67636=ORIENTED_EDGE('',*,*,#48822,.F.);
#67637=ORIENTED_EDGE('',*,*,#48824,.F.);
#67638=ORIENTED_EDGE('',*,*,#48308,.F.);
#67639=ORIENTED_EDGE('',*,*,#48306,.T.);
#67640=ORIENTED_EDGE('',*,*,#48825,.F.);
#67641=ORIENTED_EDGE('',*,*,#48826,.F.);
#67642=ORIENTED_EDGE('',*,*,#48827,.F.);
#67643=ORIENTED_EDGE('',*,*,#48314,.T.);
#67644=ORIENTED_EDGE('',*,*,#48311,.F.);
#67645=ORIENTED_EDGE('',*,*,#48309,.F.);
#67646=ORIENTED_EDGE('',*,*,#48826,.T.);
#67647=ORIENTED_EDGE('',*,*,#48828,.T.);
#67648=ORIENTED_EDGE('',*,*,#48315,.F.);
#67649=ORIENTED_EDGE('',*,*,#48312,.F.);
#67650=ORIENTED_EDGE('',*,*,#48829,.F.);
#67651=ORIENTED_EDGE('',*,*,#48830,.T.);
#67652=ORIENTED_EDGE('',*,*,#48506,.F.);
#67653=ORIENTED_EDGE('',*,*,#48828,.F.);
#67654=ORIENTED_EDGE('',*,*,#48831,.F.);
#67655=ORIENTED_EDGE('',*,*,#48832,.F.);
#67656=ORIENTED_EDGE('',*,*,#48320,.T.);
#67657=ORIENTED_EDGE('',*,*,#48782,.F.);
#67658=ORIENTED_EDGE('',*,*,#48833,.F.);
#67659=ORIENTED_EDGE('',*,*,#48321,.T.);
#67660=ORIENTED_EDGE('',*,*,#48834,.F.);
#67661=ORIENTED_EDGE('',*,*,#48835,.F.);
#67662=ORIENTED_EDGE('',*,*,#48318,.F.);
#67663=ORIENTED_EDGE('',*,*,#48835,.T.);
#67664=ORIENTED_EDGE('',*,*,#48836,.F.);
#67665=ORIENTED_EDGE('',*,*,#48837,.F.);
#67666=ORIENTED_EDGE('',*,*,#48322,.F.);
#67667=ORIENTED_EDGE('',*,*,#48837,.T.);
#67668=ORIENTED_EDGE('',*,*,#48838,.F.);
#67669=ORIENTED_EDGE('',*,*,#48839,.F.);
#67670=ORIENTED_EDGE('',*,*,#48324,.F.);
#67671=ORIENTED_EDGE('',*,*,#48839,.T.);
#67672=ORIENTED_EDGE('',*,*,#48840,.F.);
#67673=ORIENTED_EDGE('',*,*,#48841,.F.);
#67674=ORIENTED_EDGE('',*,*,#48326,.F.);
#67675=ORIENTED_EDGE('',*,*,#48841,.T.);
#67676=ORIENTED_EDGE('',*,*,#48842,.F.);
#67677=ORIENTED_EDGE('',*,*,#48332,.F.);
#67678=ORIENTED_EDGE('',*,*,#48328,.F.);
#67679=ORIENTED_EDGE('',*,*,#48334,.F.);
#67680=ORIENTED_EDGE('',*,*,#48333,.T.);
#67681=ORIENTED_EDGE('',*,*,#48843,.F.);
#67682=ORIENTED_EDGE('',*,*,#48330,.T.);
#67683=ORIENTED_EDGE('',*,*,#48844,.T.);
#67684=ORIENTED_EDGE('',*,*,#48785,.F.);
#67685=ORIENTED_EDGE('',*,*,#48845,.F.);
#67686=ORIENTED_EDGE('',*,*,#48846,.F.);
#67687=ORIENTED_EDGE('',*,*,#48847,.T.);
#67688=ORIENTED_EDGE('',*,*,#48337,.F.);
#67689=ORIENTED_EDGE('',*,*,#48364,.F.);
#67690=ORIENTED_EDGE('',*,*,#48848,.F.);
#67691=ORIENTED_EDGE('',*,*,#48849,.T.);
#67692=ORIENTED_EDGE('',*,*,#48339,.F.);
#67693=ORIENTED_EDGE('',*,*,#48847,.F.);
#67694=ORIENTED_EDGE('',*,*,#48850,.F.);
#67695=ORIENTED_EDGE('',*,*,#48851,.T.);
#67696=ORIENTED_EDGE('',*,*,#48341,.F.);
#67697=ORIENTED_EDGE('',*,*,#48849,.F.);
#67698=ORIENTED_EDGE('',*,*,#48852,.F.);
#67699=ORIENTED_EDGE('',*,*,#48853,.T.);
#67700=ORIENTED_EDGE('',*,*,#48343,.F.);
#67701=ORIENTED_EDGE('',*,*,#48851,.F.);
#67702=ORIENTED_EDGE('',*,*,#48854,.F.);
#67703=ORIENTED_EDGE('',*,*,#48347,.T.);
#67704=ORIENTED_EDGE('',*,*,#48345,.F.);
#67705=ORIENTED_EDGE('',*,*,#48853,.F.);
#67706=ORIENTED_EDGE('',*,*,#48855,.F.);
#67707=ORIENTED_EDGE('',*,*,#48783,.F.);
#67708=ORIENTED_EDGE('',*,*,#48348,.T.);
#67709=ORIENTED_EDGE('',*,*,#48856,.F.);
#67710=ORIENTED_EDGE('',*,*,#48857,.T.);
#67711=ORIENTED_EDGE('',*,*,#48858,.F.);
#67712=ORIENTED_EDGE('',*,*,#48351,.T.);
#67713=ORIENTED_EDGE('',*,*,#48569,.F.);
#67714=ORIENTED_EDGE('',*,*,#48859,.F.);
#67715=ORIENTED_EDGE('',*,*,#48860,.F.);
#67716=ORIENTED_EDGE('',*,*,#48352,.F.);
#67717=ORIENTED_EDGE('',*,*,#48349,.F.);
#67718=ORIENTED_EDGE('',*,*,#48861,.F.);
#67719=ORIENTED_EDGE('',*,*,#48860,.T.);
#67720=ORIENTED_EDGE('',*,*,#48862,.F.);
#67721=ORIENTED_EDGE('',*,*,#48863,.F.);
#67722=ORIENTED_EDGE('',*,*,#48355,.F.);
#67723=ORIENTED_EDGE('',*,*,#48863,.T.);
#67724=ORIENTED_EDGE('',*,*,#48864,.F.);
#67725=ORIENTED_EDGE('',*,*,#48865,.F.);
#67726=ORIENTED_EDGE('',*,*,#48357,.F.);
#67727=ORIENTED_EDGE('',*,*,#48865,.T.);
#67728=ORIENTED_EDGE('',*,*,#48866,.F.);
#67729=ORIENTED_EDGE('',*,*,#48867,.F.);
#67730=ORIENTED_EDGE('',*,*,#48359,.F.);
#67731=ORIENTED_EDGE('',*,*,#48867,.T.);
#67732=ORIENTED_EDGE('',*,*,#48868,.F.);
#67733=ORIENTED_EDGE('',*,*,#48366,.F.);
#67734=ORIENTED_EDGE('',*,*,#48361,.F.);
#67735=ORIENTED_EDGE('',*,*,#48368,.F.);
#67736=ORIENTED_EDGE('',*,*,#48367,.T.);
#67737=ORIENTED_EDGE('',*,*,#48869,.F.);
#67738=ORIENTED_EDGE('',*,*,#48365,.T.);
#67739=ORIENTED_EDGE('',*,*,#48859,.T.);
#67740=ORIENTED_EDGE('',*,*,#48568,.F.);
#67741=ORIENTED_EDGE('',*,*,#48870,.F.);
#67742=ORIENTED_EDGE('',*,*,#48871,.F.);
#67743=ORIENTED_EDGE('',*,*,#48872,.T.);
#67744=ORIENTED_EDGE('',*,*,#48780,.F.);
#67745=ORIENTED_EDGE('',*,*,#48873,.F.);
#67746=ORIENTED_EDGE('',*,*,#48874,.F.);
#67747=ORIENTED_EDGE('',*,*,#48404,.T.);
#67748=ORIENTED_EDGE('',*,*,#48875,.F.);
#67749=ORIENTED_EDGE('',*,*,#48876,.F.);
#67750=ORIENTED_EDGE('',*,*,#48370,.F.);
#67751=ORIENTED_EDGE('',*,*,#48877,.T.);
#67752=ORIENTED_EDGE('',*,*,#48372,.F.);
#67753=ORIENTED_EDGE('',*,*,#48876,.T.);
#67754=ORIENTED_EDGE('',*,*,#48878,.F.);
#67755=ORIENTED_EDGE('',*,*,#48879,.T.);
#67756=ORIENTED_EDGE('',*,*,#48374,.F.);
#67757=ORIENTED_EDGE('',*,*,#48877,.F.);
#67758=ORIENTED_EDGE('',*,*,#48880,.F.);
#67759=ORIENTED_EDGE('',*,*,#48881,.T.);
#67760=ORIENTED_EDGE('',*,*,#48376,.F.);
#67761=ORIENTED_EDGE('',*,*,#48879,.F.);
#67762=ORIENTED_EDGE('',*,*,#48882,.F.);
#67763=ORIENTED_EDGE('',*,*,#48380,.T.);
#67764=ORIENTED_EDGE('',*,*,#48378,.F.);
#67765=ORIENTED_EDGE('',*,*,#48881,.F.);
#67766=ORIENTED_EDGE('',*,*,#48883,.F.);
#67767=ORIENTED_EDGE('',*,*,#48383,.F.);
#67768=ORIENTED_EDGE('',*,*,#48381,.T.);
#67769=ORIENTED_EDGE('',*,*,#48884,.F.);
#67770=ORIENTED_EDGE('',*,*,#48885,.F.);
#67771=ORIENTED_EDGE('',*,*,#48886,.F.);
#67772=ORIENTED_EDGE('',*,*,#48388,.T.);
#67773=ORIENTED_EDGE('',*,*,#48384,.F.);
#67774=ORIENTED_EDGE('',*,*,#48885,.T.);
#67775=ORIENTED_EDGE('',*,*,#48389,.T.);
#67776=ORIENTED_EDGE('',*,*,#48887,.F.);
#67777=ORIENTED_EDGE('',*,*,#48888,.F.);
#67778=ORIENTED_EDGE('',*,*,#48386,.F.);
#67779=ORIENTED_EDGE('',*,*,#48889,.T.);
#67780=ORIENTED_EDGE('',*,*,#48772,.F.);
#67781=ORIENTED_EDGE('',*,*,#48888,.T.);
#67782=ORIENTED_EDGE('',*,*,#48890,.F.);
#67783=ORIENTED_EDGE('',*,*,#48891,.F.);
#67784=ORIENTED_EDGE('',*,*,#48392,.T.);
#67785=ORIENTED_EDGE('',*,*,#48777,.F.);
#67786=ORIENTED_EDGE('',*,*,#48892,.F.);
#67787=ORIENTED_EDGE('',*,*,#48893,.T.);
#67788=ORIENTED_EDGE('',*,*,#48393,.F.);
#67789=ORIENTED_EDGE('',*,*,#48390,.F.);
#67790=ORIENTED_EDGE('',*,*,#48894,.F.);
#67791=ORIENTED_EDGE('',*,*,#48895,.T.);
#67792=ORIENTED_EDGE('',*,*,#48395,.F.);
#67793=ORIENTED_EDGE('',*,*,#48893,.F.);
#67794=ORIENTED_EDGE('',*,*,#48896,.F.);
#67795=ORIENTED_EDGE('',*,*,#48897,.T.);
#67796=ORIENTED_EDGE('',*,*,#48397,.F.);
#67797=ORIENTED_EDGE('',*,*,#48895,.F.);
#67798=ORIENTED_EDGE('',*,*,#48898,.F.);
#67799=ORIENTED_EDGE('',*,*,#48899,.T.);
#67800=ORIENTED_EDGE('',*,*,#48399,.F.);
#67801=ORIENTED_EDGE('',*,*,#48897,.F.);
#67802=ORIENTED_EDGE('',*,*,#48900,.F.);
#67803=ORIENTED_EDGE('',*,*,#48405,.T.);
#67804=ORIENTED_EDGE('',*,*,#48401,.F.);
#67805=ORIENTED_EDGE('',*,*,#48899,.F.);
#67806=ORIENTED_EDGE('',*,*,#48901,.F.);
#67807=ORIENTED_EDGE('',*,*,#48407,.F.);
#67808=ORIENTED_EDGE('',*,*,#48406,.T.);
#67809=ORIENTED_EDGE('',*,*,#48902,.F.);
#67810=ORIENTED_EDGE('',*,*,#48403,.T.);
#67811=ORIENTED_EDGE('',*,*,#48903,.T.);
#67812=ORIENTED_EDGE('',*,*,#48904,.F.);
#67813=ORIENTED_EDGE('',*,*,#48905,.F.);
#67814=ORIENTED_EDGE('',*,*,#48512,.F.);
#67815=ORIENTED_EDGE('',*,*,#48905,.T.);
#67816=ORIENTED_EDGE('',*,*,#48906,.F.);
#67817=ORIENTED_EDGE('',*,*,#48411,.F.);
#67818=ORIENTED_EDGE('',*,*,#48409,.F.);
#67819=ORIENTED_EDGE('',*,*,#48413,.F.);
#67820=ORIENTED_EDGE('',*,*,#48412,.T.);
#67821=ORIENTED_EDGE('',*,*,#48907,.F.);
#67822=ORIENTED_EDGE('',*,*,#48417,.T.);
#67823=ORIENTED_EDGE('',*,*,#48418,.T.);
#67824=ORIENTED_EDGE('',*,*,#48908,.F.);
#67825=ORIENTED_EDGE('',*,*,#48909,.F.);
#67826=ORIENTED_EDGE('',*,*,#48415,.F.);
#67827=ORIENTED_EDGE('',*,*,#48909,.T.);
#67828=ORIENTED_EDGE('',*,*,#48910,.F.);
#67829=ORIENTED_EDGE('',*,*,#48911,.F.);
#67830=ORIENTED_EDGE('',*,*,#48419,.F.);
#67831=ORIENTED_EDGE('',*,*,#48911,.T.);
#67832=ORIENTED_EDGE('',*,*,#48912,.F.);
#67833=ORIENTED_EDGE('',*,*,#48913,.F.);
#67834=ORIENTED_EDGE('',*,*,#48421,.F.);
#67835=ORIENTED_EDGE('',*,*,#48913,.T.);
#67836=ORIENTED_EDGE('',*,*,#48914,.F.);
#67837=ORIENTED_EDGE('',*,*,#48915,.F.);
#67838=ORIENTED_EDGE('',*,*,#48423,.F.);
#67839=ORIENTED_EDGE('',*,*,#48915,.T.);
#67840=ORIENTED_EDGE('',*,*,#48916,.F.);
#67841=ORIENTED_EDGE('',*,*,#48427,.F.);
#67842=ORIENTED_EDGE('',*,*,#48425,.F.);
#67843=ORIENTED_EDGE('',*,*,#48429,.F.);
#67844=ORIENTED_EDGE('',*,*,#48428,.T.);
#67845=ORIENTED_EDGE('',*,*,#48917,.F.);
#67846=ORIENTED_EDGE('',*,*,#48433,.T.);
#67847=ORIENTED_EDGE('',*,*,#48434,.T.);
#67848=ORIENTED_EDGE('',*,*,#48918,.F.);
#67849=ORIENTED_EDGE('',*,*,#48919,.F.);
#67850=ORIENTED_EDGE('',*,*,#48431,.F.);
#67851=ORIENTED_EDGE('',*,*,#48920,.T.);
#67852=ORIENTED_EDGE('',*,*,#48435,.F.);
#67853=ORIENTED_EDGE('',*,*,#48919,.T.);
#67854=ORIENTED_EDGE('',*,*,#48921,.F.);
#67855=ORIENTED_EDGE('',*,*,#48922,.T.);
#67856=ORIENTED_EDGE('',*,*,#48437,.F.);
#67857=ORIENTED_EDGE('',*,*,#48920,.F.);
#67858=ORIENTED_EDGE('',*,*,#48923,.F.);
#67859=ORIENTED_EDGE('',*,*,#48924,.T.);
#67860=ORIENTED_EDGE('',*,*,#48439,.F.);
#67861=ORIENTED_EDGE('',*,*,#48922,.F.);
#67862=ORIENTED_EDGE('',*,*,#48925,.F.);
#67863=ORIENTED_EDGE('',*,*,#48443,.T.);
#67864=ORIENTED_EDGE('',*,*,#48441,.F.);
#67865=ORIENTED_EDGE('',*,*,#48924,.F.);
#67866=ORIENTED_EDGE('',*,*,#48926,.F.);
#67867=ORIENTED_EDGE('',*,*,#48445,.F.);
#67868=ORIENTED_EDGE('',*,*,#48444,.T.);
#67869=ORIENTED_EDGE('',*,*,#48927,.F.);
#67870=ORIENTED_EDGE('',*,*,#48449,.T.);
#67871=ORIENTED_EDGE('',*,*,#48450,.T.);
#67872=ORIENTED_EDGE('',*,*,#48928,.F.);
#67873=ORIENTED_EDGE('',*,*,#48929,.F.);
#67874=ORIENTED_EDGE('',*,*,#48447,.F.);
#67875=ORIENTED_EDGE('',*,*,#48930,.T.);
#67876=ORIENTED_EDGE('',*,*,#48451,.F.);
#67877=ORIENTED_EDGE('',*,*,#48929,.T.);
#67878=ORIENTED_EDGE('',*,*,#48931,.F.);
#67879=ORIENTED_EDGE('',*,*,#48932,.T.);
#67880=ORIENTED_EDGE('',*,*,#48453,.F.);
#67881=ORIENTED_EDGE('',*,*,#48930,.F.);
#67882=ORIENTED_EDGE('',*,*,#48933,.F.);
#67883=ORIENTED_EDGE('',*,*,#48934,.T.);
#67884=ORIENTED_EDGE('',*,*,#48455,.F.);
#67885=ORIENTED_EDGE('',*,*,#48932,.F.);
#67886=ORIENTED_EDGE('',*,*,#48935,.F.);
#67887=ORIENTED_EDGE('',*,*,#48459,.T.);
#67888=ORIENTED_EDGE('',*,*,#48457,.F.);
#67889=ORIENTED_EDGE('',*,*,#48934,.F.);
#67890=ORIENTED_EDGE('',*,*,#48936,.F.);
#67891=ORIENTED_EDGE('',*,*,#48461,.F.);
#67892=ORIENTED_EDGE('',*,*,#48460,.T.);
#67893=ORIENTED_EDGE('',*,*,#48937,.F.);
#67894=ORIENTED_EDGE('',*,*,#48465,.T.);
#67895=ORIENTED_EDGE('',*,*,#48466,.T.);
#67896=ORIENTED_EDGE('',*,*,#48938,.F.);
#67897=ORIENTED_EDGE('',*,*,#48939,.F.);
#67898=ORIENTED_EDGE('',*,*,#48463,.F.);
#67899=ORIENTED_EDGE('',*,*,#48940,.T.);
#67900=ORIENTED_EDGE('',*,*,#48467,.F.);
#67901=ORIENTED_EDGE('',*,*,#48939,.T.);
#67902=ORIENTED_EDGE('',*,*,#48941,.F.);
#67903=ORIENTED_EDGE('',*,*,#48942,.T.);
#67904=ORIENTED_EDGE('',*,*,#48469,.F.);
#67905=ORIENTED_EDGE('',*,*,#48940,.F.);
#67906=ORIENTED_EDGE('',*,*,#48943,.F.);
#67907=ORIENTED_EDGE('',*,*,#48944,.T.);
#67908=ORIENTED_EDGE('',*,*,#48471,.F.);
#67909=ORIENTED_EDGE('',*,*,#48942,.F.);
#67910=ORIENTED_EDGE('',*,*,#48945,.F.);
#67911=ORIENTED_EDGE('',*,*,#48475,.T.);
#67912=ORIENTED_EDGE('',*,*,#48473,.F.);
#67913=ORIENTED_EDGE('',*,*,#48944,.F.);
#67914=ORIENTED_EDGE('',*,*,#48946,.F.);
#67915=ORIENTED_EDGE('',*,*,#48477,.F.);
#67916=ORIENTED_EDGE('',*,*,#48476,.T.);
#67917=ORIENTED_EDGE('',*,*,#48947,.F.);
#67918=ORIENTED_EDGE('',*,*,#48481,.T.);
#67919=ORIENTED_EDGE('',*,*,#48482,.T.);
#67920=ORIENTED_EDGE('',*,*,#48948,.F.);
#67921=ORIENTED_EDGE('',*,*,#48949,.F.);
#67922=ORIENTED_EDGE('',*,*,#48479,.F.);
#67923=ORIENTED_EDGE('',*,*,#48949,.T.);
#67924=ORIENTED_EDGE('',*,*,#48950,.F.);
#67925=ORIENTED_EDGE('',*,*,#48951,.F.);
#67926=ORIENTED_EDGE('',*,*,#48483,.F.);
#67927=ORIENTED_EDGE('',*,*,#48951,.T.);
#67928=ORIENTED_EDGE('',*,*,#48952,.F.);
#67929=ORIENTED_EDGE('',*,*,#48953,.F.);
#67930=ORIENTED_EDGE('',*,*,#48485,.F.);
#67931=ORIENTED_EDGE('',*,*,#48953,.T.);
#67932=ORIENTED_EDGE('',*,*,#48954,.F.);
#67933=ORIENTED_EDGE('',*,*,#48955,.F.);
#67934=ORIENTED_EDGE('',*,*,#48487,.F.);
#67935=ORIENTED_EDGE('',*,*,#48955,.T.);
#67936=ORIENTED_EDGE('',*,*,#48956,.F.);
#67937=ORIENTED_EDGE('',*,*,#48491,.F.);
#67938=ORIENTED_EDGE('',*,*,#48489,.F.);
#67939=ORIENTED_EDGE('',*,*,#48493,.F.);
#67940=ORIENTED_EDGE('',*,*,#48492,.T.);
#67941=ORIENTED_EDGE('',*,*,#48957,.F.);
#67942=ORIENTED_EDGE('',*,*,#48496,.T.);
#67943=ORIENTED_EDGE('',*,*,#48958,.T.);
#67944=ORIENTED_EDGE('',*,*,#48497,.F.);
#67945=ORIENTED_EDGE('',*,*,#48494,.F.);
#67946=ORIENTED_EDGE('',*,*,#48959,.F.);
#67947=ORIENTED_EDGE('',*,*,#48960,.T.);
#67948=ORIENTED_EDGE('',*,*,#48499,.F.);
#67949=ORIENTED_EDGE('',*,*,#48958,.F.);
#67950=ORIENTED_EDGE('',*,*,#48961,.F.);
#67951=ORIENTED_EDGE('',*,*,#48869,.T.);
#67952=ORIENTED_EDGE('',*,*,#48868,.T.);
#67953=ORIENTED_EDGE('',*,*,#48866,.T.);
#67954=ORIENTED_EDGE('',*,*,#48864,.T.);
#67955=ORIENTED_EDGE('',*,*,#48862,.T.);
#67956=ORIENTED_EDGE('',*,*,#48861,.T.);
#67957=ORIENTED_EDGE('',*,*,#48858,.T.);
#67958=ORIENTED_EDGE('',*,*,#48962,.T.);
#67959=ORIENTED_EDGE('',*,*,#48963,.T.);
#67960=ORIENTED_EDGE('',*,*,#48964,.T.);
#67961=ORIENTED_EDGE('',*,*,#48856,.T.);
#67962=ORIENTED_EDGE('',*,*,#48855,.T.);
#67963=ORIENTED_EDGE('',*,*,#48854,.T.);
#67964=ORIENTED_EDGE('',*,*,#48852,.T.);
#67965=ORIENTED_EDGE('',*,*,#48850,.T.);
#67966=ORIENTED_EDGE('',*,*,#48848,.T.);
#67967=ORIENTED_EDGE('',*,*,#48845,.T.);
#67968=ORIENTED_EDGE('',*,*,#48784,.F.);
#67969=ORIENTED_EDGE('',*,*,#48857,.F.);
#67970=ORIENTED_EDGE('',*,*,#48965,.F.);
#67971=ORIENTED_EDGE('',*,*,#48966,.T.);
#67972=ORIENTED_EDGE('',*,*,#48846,.T.);
#67973=ORIENTED_EDGE('',*,*,#48967,.T.);
#67974=ORIENTED_EDGE('',*,*,#48968,.T.);
#67975=ORIENTED_EDGE('',*,*,#48967,.F.);
#67976=ORIENTED_EDGE('',*,*,#48965,.T.);
#67977=ORIENTED_EDGE('',*,*,#48964,.F.);
#67978=ORIENTED_EDGE('',*,*,#48969,.F.);
#67979=ORIENTED_EDGE('',*,*,#48833,.T.);
#67980=ORIENTED_EDGE('',*,*,#48786,.F.);
#67981=ORIENTED_EDGE('',*,*,#48844,.F.);
#67982=ORIENTED_EDGE('',*,*,#48970,.F.);
#67983=ORIENTED_EDGE('',*,*,#48843,.T.);
#67984=ORIENTED_EDGE('',*,*,#48842,.T.);
#67985=ORIENTED_EDGE('',*,*,#48840,.T.);
#67986=ORIENTED_EDGE('',*,*,#48838,.T.);
#67987=ORIENTED_EDGE('',*,*,#48836,.T.);
#67988=ORIENTED_EDGE('',*,*,#48834,.T.);
#67989=ORIENTED_EDGE('',*,*,#48832,.T.);
#67990=ORIENTED_EDGE('',*,*,#48971,.T.);
#67991=ORIENTED_EDGE('',*,*,#48972,.T.);
#67992=ORIENTED_EDGE('',*,*,#48973,.T.);
#67993=ORIENTED_EDGE('',*,*,#48831,.T.);
#67994=ORIENTED_EDGE('',*,*,#48829,.T.);
#67995=ORIENTED_EDGE('',*,*,#48827,.T.);
#67996=ORIENTED_EDGE('',*,*,#48825,.T.);
#67997=ORIENTED_EDGE('',*,*,#48824,.T.);
#67998=ORIENTED_EDGE('',*,*,#48823,.T.);
#67999=ORIENTED_EDGE('',*,*,#48821,.T.);
#68000=ORIENTED_EDGE('',*,*,#48819,.T.);
#68001=ORIENTED_EDGE('',*,*,#48816,.T.);
#68002=ORIENTED_EDGE('',*,*,#48971,.F.);
#68003=ORIENTED_EDGE('',*,*,#48970,.T.);
#68004=ORIENTED_EDGE('',*,*,#48966,.F.);
#68005=ORIENTED_EDGE('',*,*,#48974,.F.);
#68006=ORIENTED_EDGE('',*,*,#48975,.T.);
#68007=ORIENTED_EDGE('',*,*,#48507,.F.);
#68008=ORIENTED_EDGE('',*,*,#48830,.F.);
#68009=ORIENTED_EDGE('',*,*,#48976,.F.);
#68010=ORIENTED_EDGE('',*,*,#48977,.F.);
#68011=ORIENTED_EDGE('',*,*,#48509,.F.);
#68012=ORIENTED_EDGE('',*,*,#48975,.F.);
#68013=ORIENTED_EDGE('',*,*,#48978,.F.);
#68014=ORIENTED_EDGE('',*,*,#48977,.T.);
#68015=ORIENTED_EDGE('',*,*,#48979,.F.);
#68016=ORIENTED_EDGE('',*,*,#48903,.F.);
#68017=ORIENTED_EDGE('',*,*,#48511,.F.);
#68018=ORIENTED_EDGE('',*,*,#48980,.F.);
#68019=ORIENTED_EDGE('',*,*,#48981,.T.);
#68020=ORIENTED_EDGE('',*,*,#48961,.T.);
#68021=ORIENTED_EDGE('',*,*,#48959,.T.);
#68022=ORIENTED_EDGE('',*,*,#48957,.T.);
#68023=ORIENTED_EDGE('',*,*,#48956,.T.);
#68024=ORIENTED_EDGE('',*,*,#48954,.T.);
#68025=ORIENTED_EDGE('',*,*,#48952,.T.);
#68026=ORIENTED_EDGE('',*,*,#48950,.T.);
#68027=ORIENTED_EDGE('',*,*,#48948,.T.);
#68028=ORIENTED_EDGE('',*,*,#48947,.T.);
#68029=ORIENTED_EDGE('',*,*,#48946,.T.);
#68030=ORIENTED_EDGE('',*,*,#48945,.T.);
#68031=ORIENTED_EDGE('',*,*,#48943,.T.);
#68032=ORIENTED_EDGE('',*,*,#48941,.T.);
#68033=ORIENTED_EDGE('',*,*,#48938,.T.);
#68034=ORIENTED_EDGE('',*,*,#48937,.T.);
#68035=ORIENTED_EDGE('',*,*,#48936,.T.);
#68036=ORIENTED_EDGE('',*,*,#48935,.T.);
#68037=ORIENTED_EDGE('',*,*,#48933,.T.);
#68038=ORIENTED_EDGE('',*,*,#48931,.T.);
#68039=ORIENTED_EDGE('',*,*,#48928,.T.);
#68040=ORIENTED_EDGE('',*,*,#48927,.T.);
#68041=ORIENTED_EDGE('',*,*,#48926,.T.);
#68042=ORIENTED_EDGE('',*,*,#48925,.T.);
#68043=ORIENTED_EDGE('',*,*,#48923,.T.);
#68044=ORIENTED_EDGE('',*,*,#48921,.T.);
#68045=ORIENTED_EDGE('',*,*,#48918,.T.);
#68046=ORIENTED_EDGE('',*,*,#48917,.T.);
#68047=ORIENTED_EDGE('',*,*,#48916,.T.);
#68048=ORIENTED_EDGE('',*,*,#48914,.T.);
#68049=ORIENTED_EDGE('',*,*,#48912,.T.);
#68050=ORIENTED_EDGE('',*,*,#48910,.T.);
#68051=ORIENTED_EDGE('',*,*,#48908,.T.);
#68052=ORIENTED_EDGE('',*,*,#48907,.T.);
#68053=ORIENTED_EDGE('',*,*,#48906,.T.);
#68054=ORIENTED_EDGE('',*,*,#48904,.T.);
#68055=ORIENTED_EDGE('',*,*,#48982,.T.);
#68056=ORIENTED_EDGE('',*,*,#48982,.F.);
#68057=ORIENTED_EDGE('',*,*,#48979,.T.);
#68058=ORIENTED_EDGE('',*,*,#48978,.T.);
#68059=ORIENTED_EDGE('',*,*,#48976,.T.);
#68060=ORIENTED_EDGE('',*,*,#48973,.F.);
#68061=ORIENTED_EDGE('',*,*,#48983,.F.);
#68062=ORIENTED_EDGE('',*,*,#48984,.T.);
#68063=ORIENTED_EDGE('',*,*,#48500,.F.);
#68064=ORIENTED_EDGE('',*,*,#48960,.F.);
#68065=ORIENTED_EDGE('',*,*,#48985,.F.);
#68066=ORIENTED_EDGE('',*,*,#48986,.T.);
#68067=ORIENTED_EDGE('',*,*,#48502,.F.);
#68068=ORIENTED_EDGE('',*,*,#48984,.F.);
#68069=ORIENTED_EDGE('',*,*,#48987,.F.);
#68070=ORIENTED_EDGE('',*,*,#48811,.T.);
#68071=ORIENTED_EDGE('',*,*,#48504,.F.);
#68072=ORIENTED_EDGE('',*,*,#48986,.F.);
#68073=ORIENTED_EDGE('',*,*,#48988,.F.);
#68074=ORIENTED_EDGE('',*,*,#48771,.T.);
#68075=ORIENTED_EDGE('',*,*,#48989,.F.);
#68076=ORIENTED_EDGE('',*,*,#48990,.F.);
#68077=ORIENTED_EDGE('',*,*,#48514,.F.);
#68078=ORIENTED_EDGE('',*,*,#48990,.T.);
#68079=ORIENTED_EDGE('',*,*,#48991,.F.);
#68080=ORIENTED_EDGE('',*,*,#48992,.F.);
#68081=ORIENTED_EDGE('',*,*,#48519,.F.);
#68082=ORIENTED_EDGE('',*,*,#48992,.T.);
#68083=ORIENTED_EDGE('',*,*,#48993,.F.);
#68084=ORIENTED_EDGE('',*,*,#48994,.F.);
#68085=ORIENTED_EDGE('',*,*,#48521,.F.);
#68086=ORIENTED_EDGE('',*,*,#48994,.T.);
#68087=ORIENTED_EDGE('',*,*,#48995,.F.);
#68088=ORIENTED_EDGE('',*,*,#48996,.F.);
#68089=ORIENTED_EDGE('',*,*,#48523,.F.);
#68090=ORIENTED_EDGE('',*,*,#48996,.T.);
#68091=ORIENTED_EDGE('',*,*,#48997,.F.);
#68092=ORIENTED_EDGE('',*,*,#48528,.F.);
#68093=ORIENTED_EDGE('',*,*,#48525,.F.);
#68094=ORIENTED_EDGE('',*,*,#48531,.F.);
#68095=ORIENTED_EDGE('',*,*,#48529,.T.);
#68096=ORIENTED_EDGE('',*,*,#48998,.F.);
#68097=ORIENTED_EDGE('',*,*,#48536,.T.);
#68098=ORIENTED_EDGE('',*,*,#48537,.T.);
#68099=ORIENTED_EDGE('',*,*,#48999,.F.);
#68100=ORIENTED_EDGE('',*,*,#49000,.F.);
#68101=ORIENTED_EDGE('',*,*,#48533,.F.);
#68102=ORIENTED_EDGE('',*,*,#49000,.T.);
#68103=ORIENTED_EDGE('',*,*,#49001,.F.);
#68104=ORIENTED_EDGE('',*,*,#49002,.F.);
#68105=ORIENTED_EDGE('',*,*,#48538,.F.);
#68106=ORIENTED_EDGE('',*,*,#49002,.T.);
#68107=ORIENTED_EDGE('',*,*,#49003,.F.);
#68108=ORIENTED_EDGE('',*,*,#49004,.F.);
#68109=ORIENTED_EDGE('',*,*,#48540,.F.);
#68110=ORIENTED_EDGE('',*,*,#49004,.T.);
#68111=ORIENTED_EDGE('',*,*,#49005,.F.);
#68112=ORIENTED_EDGE('',*,*,#49006,.F.);
#68113=ORIENTED_EDGE('',*,*,#48542,.F.);
#68114=ORIENTED_EDGE('',*,*,#49006,.T.);
#68115=ORIENTED_EDGE('',*,*,#49007,.F.);
#68116=ORIENTED_EDGE('',*,*,#48547,.F.);
#68117=ORIENTED_EDGE('',*,*,#48544,.F.);
#68118=ORIENTED_EDGE('',*,*,#48549,.F.);
#68119=ORIENTED_EDGE('',*,*,#48548,.T.);
#68120=ORIENTED_EDGE('',*,*,#49008,.F.);
#68121=ORIENTED_EDGE('',*,*,#48552,.T.);
#68122=ORIENTED_EDGE('',*,*,#49009,.F.);
#68123=ORIENTED_EDGE('',*,*,#48553,.F.);
#68124=ORIENTED_EDGE('',*,*,#48550,.F.);
#68125=ORIENTED_EDGE('',*,*,#49010,.F.);
#68126=ORIENTED_EDGE('',*,*,#49009,.T.);
#68127=ORIENTED_EDGE('',*,*,#49011,.F.);
#68128=ORIENTED_EDGE('',*,*,#49012,.F.);
#68129=ORIENTED_EDGE('',*,*,#48556,.F.);
#68130=ORIENTED_EDGE('',*,*,#49012,.T.);
#68131=ORIENTED_EDGE('',*,*,#49013,.F.);
#68132=ORIENTED_EDGE('',*,*,#49014,.F.);
#68133=ORIENTED_EDGE('',*,*,#48558,.F.);
#68134=ORIENTED_EDGE('',*,*,#49014,.T.);
#68135=ORIENTED_EDGE('',*,*,#49015,.F.);
#68136=ORIENTED_EDGE('',*,*,#49016,.F.);
#68137=ORIENTED_EDGE('',*,*,#48560,.F.);
#68138=ORIENTED_EDGE('',*,*,#49016,.T.);
#68139=ORIENTED_EDGE('',*,*,#49017,.F.);
#68140=ORIENTED_EDGE('',*,*,#48565,.F.);
#68141=ORIENTED_EDGE('',*,*,#48562,.F.);
#68142=ORIENTED_EDGE('',*,*,#48567,.F.);
#68143=ORIENTED_EDGE('',*,*,#48566,.T.);
#68144=ORIENTED_EDGE('',*,*,#49018,.F.);
#68145=ORIENTED_EDGE('',*,*,#48870,.T.);
#68146=ORIENTED_EDGE('',*,*,#48962,.F.);
#68147=ORIENTED_EDGE('',*,*,#48871,.T.);
#68148=ORIENTED_EDGE('',*,*,#49019,.F.);
#68149=ORIENTED_EDGE('',*,*,#49020,.F.);
#68150=ORIENTED_EDGE('',*,*,#49021,.T.);
#68151=ORIENTED_EDGE('',*,*,#48776,.F.);
#68152=ORIENTED_EDGE('',*,*,#49022,.F.);
#68153=ORIENTED_EDGE('',*,*,#49023,.F.);
#68154=ORIENTED_EDGE('',*,*,#49024,.T.);
#68155=ORIENTED_EDGE('',*,*,#48571,.F.);
#68156=ORIENTED_EDGE('',*,*,#49021,.F.);
#68157=ORIENTED_EDGE('',*,*,#49025,.F.);
#68158=ORIENTED_EDGE('',*,*,#49024,.F.);
#68159=ORIENTED_EDGE('',*,*,#49026,.F.);
#68160=ORIENTED_EDGE('',*,*,#48576,.T.);
#68161=ORIENTED_EDGE('',*,*,#48573,.F.);
#68162=ORIENTED_EDGE('',*,*,#48578,.F.);
#68163=ORIENTED_EDGE('',*,*,#48577,.T.);
#68164=ORIENTED_EDGE('',*,*,#49027,.F.);
#68165=ORIENTED_EDGE('',*,*,#48583,.T.);
#68166=ORIENTED_EDGE('',*,*,#48584,.T.);
#68167=ORIENTED_EDGE('',*,*,#49028,.F.);
#68168=ORIENTED_EDGE('',*,*,#49029,.F.);
#68169=ORIENTED_EDGE('',*,*,#48581,.F.);
#68170=ORIENTED_EDGE('',*,*,#49030,.T.);
#68171=ORIENTED_EDGE('',*,*,#48585,.F.);
#68172=ORIENTED_EDGE('',*,*,#49029,.T.);
#68173=ORIENTED_EDGE('',*,*,#49031,.F.);
#68174=ORIENTED_EDGE('',*,*,#49032,.T.);
#68175=ORIENTED_EDGE('',*,*,#48587,.F.);
#68176=ORIENTED_EDGE('',*,*,#49030,.F.);
#68177=ORIENTED_EDGE('',*,*,#49033,.F.);
#68178=ORIENTED_EDGE('',*,*,#49034,.T.);
#68179=ORIENTED_EDGE('',*,*,#48589,.F.);
#68180=ORIENTED_EDGE('',*,*,#49032,.F.);
#68181=ORIENTED_EDGE('',*,*,#49035,.F.);
#68182=ORIENTED_EDGE('',*,*,#49034,.F.);
#68183=ORIENTED_EDGE('',*,*,#49036,.F.);
#68184=ORIENTED_EDGE('',*,*,#48595,.T.);
#68185=ORIENTED_EDGE('',*,*,#48594,.T.);
#68186=ORIENTED_EDGE('',*,*,#48591,.F.);
#68187=ORIENTED_EDGE('',*,*,#48597,.F.);
#68188=ORIENTED_EDGE('',*,*,#48596,.T.);
#68189=ORIENTED_EDGE('',*,*,#49037,.F.);
#68190=ORIENTED_EDGE('',*,*,#48602,.T.);
#68191=ORIENTED_EDGE('',*,*,#48603,.T.);
#68192=ORIENTED_EDGE('',*,*,#49038,.F.);
#68193=ORIENTED_EDGE('',*,*,#49039,.F.);
#68194=ORIENTED_EDGE('',*,*,#48600,.F.);
#68195=ORIENTED_EDGE('',*,*,#49040,.T.);
#68196=ORIENTED_EDGE('',*,*,#48604,.F.);
#68197=ORIENTED_EDGE('',*,*,#49039,.T.);
#68198=ORIENTED_EDGE('',*,*,#49041,.F.);
#68199=ORIENTED_EDGE('',*,*,#49042,.T.);
#68200=ORIENTED_EDGE('',*,*,#48606,.F.);
#68201=ORIENTED_EDGE('',*,*,#49040,.F.);
#68202=ORIENTED_EDGE('',*,*,#49043,.F.);
#68203=ORIENTED_EDGE('',*,*,#49044,.T.);
#68204=ORIENTED_EDGE('',*,*,#49045,.T.);
#68205=ORIENTED_EDGE('',*,*,#48608,.F.);
#68206=ORIENTED_EDGE('',*,*,#49042,.F.);
#68207=ORIENTED_EDGE('',*,*,#49046,.F.);
#68208=ORIENTED_EDGE('',*,*,#49044,.F.);
#68209=ORIENTED_EDGE('',*,*,#49047,.F.);
#68210=ORIENTED_EDGE('',*,*,#48614,.T.);
#68211=ORIENTED_EDGE('',*,*,#48613,.T.);
#68212=ORIENTED_EDGE('',*,*,#48610,.F.);
#68213=ORIENTED_EDGE('',*,*,#49045,.F.);
#68214=ORIENTED_EDGE('',*,*,#48616,.F.);
#68215=ORIENTED_EDGE('',*,*,#48615,.T.);
#68216=ORIENTED_EDGE('',*,*,#49048,.F.);
#68217=ORIENTED_EDGE('',*,*,#48623,.T.);
#68218=ORIENTED_EDGE('',*,*,#48624,.T.);
#68219=ORIENTED_EDGE('',*,*,#49049,.F.);
#68220=ORIENTED_EDGE('',*,*,#49050,.F.);
#68221=ORIENTED_EDGE('',*,*,#48620,.F.);
#68222=ORIENTED_EDGE('',*,*,#49050,.T.);
#68223=ORIENTED_EDGE('',*,*,#49051,.F.);
#68224=ORIENTED_EDGE('',*,*,#49052,.F.);
#68225=ORIENTED_EDGE('',*,*,#48625,.F.);
#68226=ORIENTED_EDGE('',*,*,#49053,.F.);
#68227=ORIENTED_EDGE('',*,*,#43775,.F.);
#68228=ORIENTED_EDGE('',*,*,#43895,.F.);
#68229=ORIENTED_EDGE('',*,*,#43892,.F.);
#68230=ORIENTED_EDGE('',*,*,#43891,.F.);
#68231=ORIENTED_EDGE('',*,*,#43886,.F.);
#68232=ORIENTED_EDGE('',*,*,#43883,.F.);
#68233=ORIENTED_EDGE('',*,*,#43878,.F.);
#68234=ORIENTED_EDGE('',*,*,#43875,.F.);
#68235=ORIENTED_EDGE('',*,*,#43872,.F.);
#68236=ORIENTED_EDGE('',*,*,#43871,.F.);
#68237=ORIENTED_EDGE('',*,*,#43865,.F.);
#68238=ORIENTED_EDGE('',*,*,#43862,.F.);
#68239=ORIENTED_EDGE('',*,*,#43857,.F.);
#68240=ORIENTED_EDGE('',*,*,#43854,.F.);
#68241=ORIENTED_EDGE('',*,*,#43851,.F.);
#68242=ORIENTED_EDGE('',*,*,#43849,.F.);
#68243=ORIENTED_EDGE('',*,*,#43843,.F.);
#68244=ORIENTED_EDGE('',*,*,#43840,.F.);
#68245=ORIENTED_EDGE('',*,*,#43837,.F.);
#68246=ORIENTED_EDGE('',*,*,#49054,.T.);
#68247=ORIENTED_EDGE('',*,*,#49051,.T.);
#68248=ORIENTED_EDGE('',*,*,#49049,.T.);
#68249=ORIENTED_EDGE('',*,*,#49048,.T.);
#68250=ORIENTED_EDGE('',*,*,#49047,.T.);
#68251=ORIENTED_EDGE('',*,*,#49046,.T.);
#68252=ORIENTED_EDGE('',*,*,#49043,.T.);
#68253=ORIENTED_EDGE('',*,*,#49041,.T.);
#68254=ORIENTED_EDGE('',*,*,#49038,.T.);
#68255=ORIENTED_EDGE('',*,*,#49037,.T.);
#68256=ORIENTED_EDGE('',*,*,#49036,.T.);
#68257=ORIENTED_EDGE('',*,*,#49035,.T.);
#68258=ORIENTED_EDGE('',*,*,#49033,.T.);
#68259=ORIENTED_EDGE('',*,*,#49031,.T.);
#68260=ORIENTED_EDGE('',*,*,#49028,.T.);
#68261=ORIENTED_EDGE('',*,*,#49027,.T.);
#68262=ORIENTED_EDGE('',*,*,#49026,.T.);
#68263=ORIENTED_EDGE('',*,*,#49025,.T.);
#68264=ORIENTED_EDGE('',*,*,#49023,.T.);
#68265=ORIENTED_EDGE('',*,*,#49055,.T.);
#68266=ORIENTED_EDGE('',*,*,#48815,.T.);
#68267=ORIENTED_EDGE('',*,*,#48814,.T.);
#68268=ORIENTED_EDGE('',*,*,#48812,.T.);
#68269=ORIENTED_EDGE('',*,*,#49056,.T.);
#68270=ORIENTED_EDGE('',*,*,#49057,.T.);
#68271=ORIENTED_EDGE('',*,*,#49058,.T.);
#68272=ORIENTED_EDGE('',*,*,#48809,.T.);
#68273=ORIENTED_EDGE('',*,*,#48808,.T.);
#68274=ORIENTED_EDGE('',*,*,#48807,.T.);
#68275=ORIENTED_EDGE('',*,*,#48805,.T.);
#68276=ORIENTED_EDGE('',*,*,#48803,.T.);
#68277=ORIENTED_EDGE('',*,*,#48801,.T.);
#68278=ORIENTED_EDGE('',*,*,#48799,.T.);
#68279=ORIENTED_EDGE('',*,*,#48798,.T.);
#68280=ORIENTED_EDGE('',*,*,#48797,.T.);
#68281=ORIENTED_EDGE('',*,*,#48795,.T.);
#68282=ORIENTED_EDGE('',*,*,#48793,.T.);
#68283=ORIENTED_EDGE('',*,*,#48790,.T.);
#68284=ORIENTED_EDGE('',*,*,#48787,.T.);
#68285=ORIENTED_EDGE('',*,*,#48873,.T.);
#68286=ORIENTED_EDGE('',*,*,#48779,.F.);
#68287=ORIENTED_EDGE('',*,*,#48810,.F.);
#68288=ORIENTED_EDGE('',*,*,#49059,.F.);
#68289=ORIENTED_EDGE('',*,*,#49060,.T.);
#68290=ORIENTED_EDGE('',*,*,#48874,.T.);
#68291=ORIENTED_EDGE('',*,*,#49061,.T.);
#68292=ORIENTED_EDGE('',*,*,#49062,.T.);
#68293=ORIENTED_EDGE('',*,*,#49061,.F.);
#68294=ORIENTED_EDGE('',*,*,#49059,.T.);
#68295=ORIENTED_EDGE('',*,*,#49058,.F.);
#68296=ORIENTED_EDGE('',*,*,#49063,.F.);
#68297=ORIENTED_EDGE('',*,*,#48892,.T.);
#68298=ORIENTED_EDGE('',*,*,#48781,.F.);
#68299=ORIENTED_EDGE('',*,*,#48872,.F.);
#68300=ORIENTED_EDGE('',*,*,#49064,.F.);
#68301=ORIENTED_EDGE('',*,*,#48902,.T.);
#68302=ORIENTED_EDGE('',*,*,#48901,.T.);
#68303=ORIENTED_EDGE('',*,*,#48900,.T.);
#68304=ORIENTED_EDGE('',*,*,#48898,.T.);
#68305=ORIENTED_EDGE('',*,*,#48896,.T.);
#68306=ORIENTED_EDGE('',*,*,#48894,.T.);
#68307=ORIENTED_EDGE('',*,*,#48891,.T.);
#68308=ORIENTED_EDGE('',*,*,#49065,.T.);
#68309=ORIENTED_EDGE('',*,*,#49066,.T.);
#68310=ORIENTED_EDGE('',*,*,#49067,.T.);
#68311=ORIENTED_EDGE('',*,*,#48890,.T.);
#68312=ORIENTED_EDGE('',*,*,#48887,.T.);
#68313=ORIENTED_EDGE('',*,*,#48886,.T.);
#68314=ORIENTED_EDGE('',*,*,#48884,.T.);
#68315=ORIENTED_EDGE('',*,*,#48883,.T.);
#68316=ORIENTED_EDGE('',*,*,#48882,.T.);
#68317=ORIENTED_EDGE('',*,*,#48880,.T.);
#68318=ORIENTED_EDGE('',*,*,#48878,.T.);
#68319=ORIENTED_EDGE('',*,*,#48875,.T.);
#68320=ORIENTED_EDGE('',*,*,#49065,.F.);
#68321=ORIENTED_EDGE('',*,*,#49064,.T.);
#68322=ORIENTED_EDGE('',*,*,#49060,.F.);
#68323=ORIENTED_EDGE('',*,*,#49068,.F.);
#68324=ORIENTED_EDGE('',*,*,#49069,.T.);
#68325=ORIENTED_EDGE('',*,*,#48773,.F.);
#68326=ORIENTED_EDGE('',*,*,#48889,.F.);
#68327=ORIENTED_EDGE('',*,*,#49070,.F.);
#68328=ORIENTED_EDGE('',*,*,#49022,.T.);
#68329=ORIENTED_EDGE('',*,*,#48775,.F.);
#68330=ORIENTED_EDGE('',*,*,#49069,.F.);
#68331=ORIENTED_EDGE('',*,*,#49071,.F.);
#68332=ORIENTED_EDGE('',*,*,#49071,.T.);
#68333=ORIENTED_EDGE('',*,*,#49070,.T.);
#68334=ORIENTED_EDGE('',*,*,#49067,.F.);
#68335=ORIENTED_EDGE('',*,*,#49072,.F.);
#68336=ORIENTED_EDGE('',*,*,#49055,.F.);
#68337=ORIENTED_EDGE('',*,*,#49054,.F.);
#68338=ORIENTED_EDGE('',*,*,#43836,.F.);
#68339=ORIENTED_EDGE('',*,*,#49073,.F.);
#68340=ORIENTED_EDGE('',*,*,#49052,.T.);
#68341=ORIENTED_EDGE('',*,*,#48626,.T.);
#68342=ORIENTED_EDGE('',*,*,#49073,.T.);
#68343=ORIENTED_EDGE('',*,*,#44577,.F.);
#68344=ORIENTED_EDGE('',*,*,#49074,.F.);
#68345=ORIENTED_EDGE('',*,*,#49075,.T.);
#68346=ORIENTED_EDGE('',*,*,#48629,.T.);
#68347=ORIENTED_EDGE('',*,*,#49074,.T.);
#68348=ORIENTED_EDGE('',*,*,#44573,.F.);
#68349=ORIENTED_EDGE('',*,*,#49075,.F.);
#68350=ORIENTED_EDGE('',*,*,#44570,.F.);
#68351=ORIENTED_EDGE('',*,*,#49076,.T.);
#68352=ORIENTED_EDGE('',*,*,#48630,.T.);
#68353=ORIENTED_EDGE('',*,*,#49076,.F.);
#68354=ORIENTED_EDGE('',*,*,#44556,.T.);
#68355=ORIENTED_EDGE('',*,*,#49077,.F.);
#68356=ORIENTED_EDGE('',*,*,#48638,.F.);
#68357=ORIENTED_EDGE('',*,*,#49078,.T.);
#68358=ORIENTED_EDGE('',*,*,#48636,.T.);
#68359=ORIENTED_EDGE('',*,*,#48635,.T.);
#68360=ORIENTED_EDGE('',*,*,#48633,.T.);
#68361=ORIENTED_EDGE('',*,*,#48665,.T.);
#68362=ORIENTED_EDGE('',*,*,#48664,.T.);
#68363=ORIENTED_EDGE('',*,*,#48662,.T.);
#68364=ORIENTED_EDGE('',*,*,#48661,.T.);
#68365=ORIENTED_EDGE('',*,*,#48659,.T.);
#68366=ORIENTED_EDGE('',*,*,#48657,.T.);
#68367=ORIENTED_EDGE('',*,*,#48656,.T.);
#68368=ORIENTED_EDGE('',*,*,#48654,.T.);
#68369=ORIENTED_EDGE('',*,*,#48652,.T.);
#68370=ORIENTED_EDGE('',*,*,#48651,.T.);
#68371=ORIENTED_EDGE('',*,*,#48649,.T.);
#68372=ORIENTED_EDGE('',*,*,#48647,.T.);
#68373=ORIENTED_EDGE('',*,*,#48646,.T.);
#68374=ORIENTED_EDGE('',*,*,#48644,.T.);
#68375=ORIENTED_EDGE('',*,*,#48642,.T.);
#68376=ORIENTED_EDGE('',*,*,#48641,.T.);
#68377=ORIENTED_EDGE('',*,*,#48639,.T.);
#68378=ORIENTED_EDGE('',*,*,#49077,.T.);
#68379=ORIENTED_EDGE('',*,*,#44558,.F.);
#68380=ORIENTED_EDGE('',*,*,#44555,.F.);
#68381=ORIENTED_EDGE('',*,*,#44548,.F.);
#68382=ORIENTED_EDGE('',*,*,#44545,.F.);
#68383=ORIENTED_EDGE('',*,*,#44542,.F.);
#68384=ORIENTED_EDGE('',*,*,#44541,.F.);
#68385=ORIENTED_EDGE('',*,*,#44538,.F.);
#68386=ORIENTED_EDGE('',*,*,#44535,.F.);
#68387=ORIENTED_EDGE('',*,*,#44528,.F.);
#68388=ORIENTED_EDGE('',*,*,#44525,.F.);
#68389=ORIENTED_EDGE('',*,*,#44522,.F.);
#68390=ORIENTED_EDGE('',*,*,#44521,.F.);
#68391=ORIENTED_EDGE('',*,*,#44518,.F.);
#68392=ORIENTED_EDGE('',*,*,#44515,.F.);
#68393=ORIENTED_EDGE('',*,*,#44508,.F.);
#68394=ORIENTED_EDGE('',*,*,#44505,.F.);
#68395=ORIENTED_EDGE('',*,*,#44504,.F.);
#68396=ORIENTED_EDGE('',*,*,#44569,.F.);
#68397=ORIENTED_EDGE('',*,*,#44567,.F.);
#68398=ORIENTED_EDGE('',*,*,#44562,.F.);
#68399=ORIENTED_EDGE('',*,*,#49079,.F.);
#68400=ORIENTED_EDGE('',*,*,#48670,.F.);
#68401=ORIENTED_EDGE('',*,*,#49078,.F.);
#68402=ORIENTED_EDGE('',*,*,#44484,.T.);
#68403=ORIENTED_EDGE('',*,*,#49079,.T.);
#68404=ORIENTED_EDGE('',*,*,#44486,.F.);
#68405=ORIENTED_EDGE('',*,*,#44483,.F.);
#68406=ORIENTED_EDGE('',*,*,#44480,.F.);
#68407=ORIENTED_EDGE('',*,*,#44477,.F.);
#68408=ORIENTED_EDGE('',*,*,#44474,.F.);
#68409=ORIENTED_EDGE('',*,*,#44471,.F.);
#68410=ORIENTED_EDGE('',*,*,#44468,.F.);
#68411=ORIENTED_EDGE('',*,*,#44465,.F.);
#68412=ORIENTED_EDGE('',*,*,#44462,.F.);
#68413=ORIENTED_EDGE('',*,*,#44459,.F.);
#68414=ORIENTED_EDGE('',*,*,#44456,.F.);
#68415=ORIENTED_EDGE('',*,*,#44453,.F.);
#68416=ORIENTED_EDGE('',*,*,#44450,.F.);
#68417=ORIENTED_EDGE('',*,*,#44447,.F.);
#68418=ORIENTED_EDGE('',*,*,#44444,.F.);
#68419=ORIENTED_EDGE('',*,*,#49080,.T.);
#68420=ORIENTED_EDGE('',*,*,#48699,.T.);
#68421=ORIENTED_EDGE('',*,*,#48697,.T.);
#68422=ORIENTED_EDGE('',*,*,#48695,.T.);
#68423=ORIENTED_EDGE('',*,*,#48693,.T.);
#68424=ORIENTED_EDGE('',*,*,#48691,.T.);
#68425=ORIENTED_EDGE('',*,*,#48689,.T.);
#68426=ORIENTED_EDGE('',*,*,#48687,.T.);
#68427=ORIENTED_EDGE('',*,*,#48685,.T.);
#68428=ORIENTED_EDGE('',*,*,#48683,.T.);
#68429=ORIENTED_EDGE('',*,*,#48681,.T.);
#68430=ORIENTED_EDGE('',*,*,#48679,.T.);
#68431=ORIENTED_EDGE('',*,*,#48677,.T.);
#68432=ORIENTED_EDGE('',*,*,#48675,.T.);
#68433=ORIENTED_EDGE('',*,*,#48673,.T.);
#68434=ORIENTED_EDGE('',*,*,#48671,.T.);
#68435=ORIENTED_EDGE('',*,*,#44497,.T.);
#68436=ORIENTED_EDGE('',*,*,#44490,.T.);
#68437=ORIENTED_EDGE('',*,*,#48667,.F.);
#68438=ORIENTED_EDGE('',*,*,#48669,.F.);
#68439=ORIENTED_EDGE('',*,*,#49080,.F.);
#68440=ORIENTED_EDGE('',*,*,#44443,.F.);
#68441=ORIENTED_EDGE('',*,*,#49081,.F.);
#68442=ORIENTED_EDGE('',*,*,#48700,.T.);
#68443=ORIENTED_EDGE('',*,*,#49081,.T.);
#68444=ORIENTED_EDGE('',*,*,#44439,.F.);
#68445=ORIENTED_EDGE('',*,*,#49082,.T.);
#68446=ORIENTED_EDGE('',*,*,#48702,.T.);
#68447=ORIENTED_EDGE('',*,*,#48706,.T.);
#68448=ORIENTED_EDGE('',*,*,#49082,.F.);
#68449=ORIENTED_EDGE('',*,*,#44434,.F.);
#68450=ORIENTED_EDGE('',*,*,#49083,.F.);
#68451=ORIENTED_EDGE('',*,*,#48707,.T.);
#68452=ORIENTED_EDGE('',*,*,#49083,.T.);
#68453=ORIENTED_EDGE('',*,*,#44433,.F.);
#68454=ORIENTED_EDGE('',*,*,#44437,.F.);
#68455=ORIENTED_EDGE('',*,*,#44430,.F.);
#68456=ORIENTED_EDGE('',*,*,#49084,.F.);
#68457=ORIENTED_EDGE('',*,*,#48709,.T.);
#68458=ORIENTED_EDGE('',*,*,#48705,.T.);
#68459=ORIENTED_EDGE('',*,*,#49084,.T.);
#68460=ORIENTED_EDGE('',*,*,#44429,.F.);
#68461=ORIENTED_EDGE('',*,*,#44422,.F.);
#68462=ORIENTED_EDGE('',*,*,#44328,.F.);
#68463=ORIENTED_EDGE('',*,*,#49085,.T.);
#68464=ORIENTED_EDGE('',*,*,#48760,.T.);
#68465=ORIENTED_EDGE('',*,*,#48711,.T.);
#68466=ORIENTED_EDGE('',*,*,#48710,.T.);
#68467=ORIENTED_EDGE('',*,*,#48764,.T.);
#68468=ORIENTED_EDGE('',*,*,#48763,.T.);
#68469=ORIENTED_EDGE('',*,*,#48761,.T.);
#68470=ORIENTED_EDGE('',*,*,#49085,.F.);
#68471=ORIENTED_EDGE('',*,*,#44327,.F.);
#68472=ORIENTED_EDGE('',*,*,#44319,.F.);
#68473=ORIENTED_EDGE('',*,*,#44316,.F.);
#68474=ORIENTED_EDGE('',*,*,#44419,.F.);
#68475=ORIENTED_EDGE('',*,*,#44414,.F.);
#68476=ORIENTED_EDGE('',*,*,#44411,.F.);
#68477=ORIENTED_EDGE('',*,*,#44408,.F.);
#68478=ORIENTED_EDGE('',*,*,#44405,.F.);
#68479=ORIENTED_EDGE('',*,*,#44402,.F.);
#68480=ORIENTED_EDGE('',*,*,#44399,.F.);
#68481=ORIENTED_EDGE('',*,*,#44394,.F.);
#68482=ORIENTED_EDGE('',*,*,#44391,.F.);
#68483=ORIENTED_EDGE('',*,*,#44388,.F.);
#68484=ORIENTED_EDGE('',*,*,#44385,.F.);
#68485=ORIENTED_EDGE('',*,*,#44382,.F.);
#68486=ORIENTED_EDGE('',*,*,#44379,.F.);
#68487=ORIENTED_EDGE('',*,*,#44376,.F.);
#68488=ORIENTED_EDGE('',*,*,#44371,.F.);
#68489=ORIENTED_EDGE('',*,*,#44368,.F.);
#68490=ORIENTED_EDGE('',*,*,#44365,.F.);
#68491=ORIENTED_EDGE('',*,*,#44362,.F.);
#68492=ORIENTED_EDGE('',*,*,#44359,.F.);
#68493=ORIENTED_EDGE('',*,*,#44356,.F.);
#68494=ORIENTED_EDGE('',*,*,#44353,.F.);
#68495=ORIENTED_EDGE('',*,*,#44350,.F.);
#68496=ORIENTED_EDGE('',*,*,#44343,.F.);
#68497=ORIENTED_EDGE('',*,*,#44340,.F.);
#68498=ORIENTED_EDGE('',*,*,#44337,.F.);
#68499=ORIENTED_EDGE('',*,*,#44334,.F.);
#68500=ORIENTED_EDGE('',*,*,#44331,.F.);
#68501=ORIENTED_EDGE('',*,*,#49086,.T.);
#68502=ORIENTED_EDGE('',*,*,#48759,.T.);
#68503=ORIENTED_EDGE('',*,*,#48757,.T.);
#68504=ORIENTED_EDGE('',*,*,#48755,.T.);
#68505=ORIENTED_EDGE('',*,*,#48753,.T.);
#68506=ORIENTED_EDGE('',*,*,#48751,.T.);
#68507=ORIENTED_EDGE('',*,*,#48749,.T.);
#68508=ORIENTED_EDGE('',*,*,#48748,.T.);
#68509=ORIENTED_EDGE('',*,*,#48747,.T.);
#68510=ORIENTED_EDGE('',*,*,#48745,.T.);
#68511=ORIENTED_EDGE('',*,*,#48743,.T.);
#68512=ORIENTED_EDGE('',*,*,#48741,.T.);
#68513=ORIENTED_EDGE('',*,*,#48739,.T.);
#68514=ORIENTED_EDGE('',*,*,#48738,.T.);
#68515=ORIENTED_EDGE('',*,*,#48735,.T.);
#68516=ORIENTED_EDGE('',*,*,#48734,.T.);
#68517=ORIENTED_EDGE('',*,*,#48733,.T.);
#68518=ORIENTED_EDGE('',*,*,#48731,.T.);
#68519=ORIENTED_EDGE('',*,*,#48729,.T.);
#68520=ORIENTED_EDGE('',*,*,#48727,.T.);
#68521=ORIENTED_EDGE('',*,*,#48725,.T.);
#68522=ORIENTED_EDGE('',*,*,#48724,.T.);
#68523=ORIENTED_EDGE('',*,*,#48723,.T.);
#68524=ORIENTED_EDGE('',*,*,#48721,.T.);
#68525=ORIENTED_EDGE('',*,*,#48719,.T.);
#68526=ORIENTED_EDGE('',*,*,#48717,.T.);
#68527=ORIENTED_EDGE('',*,*,#48715,.T.);
#68528=ORIENTED_EDGE('',*,*,#48714,.T.);
#68529=ORIENTED_EDGE('',*,*,#44311,.F.);
#68530=ORIENTED_EDGE('',*,*,#49087,.F.);
#68531=ORIENTED_EDGE('',*,*,#48767,.T.);
#68532=ORIENTED_EDGE('',*,*,#48766,.T.);
#68533=ORIENTED_EDGE('',*,*,#49086,.F.);
#68534=ORIENTED_EDGE('',*,*,#44312,.F.);
#68535=ORIENTED_EDGE('',*,*,#49087,.T.);
#68536=ORIENTED_EDGE('',*,*,#44308,.F.);
#68537=ORIENTED_EDGE('',*,*,#49088,.T.);
#68538=ORIENTED_EDGE('',*,*,#48769,.T.);
#68539=ORIENTED_EDGE('',*,*,#49089,.F.);
#68540=ORIENTED_EDGE('',*,*,#48770,.T.);
#68541=ORIENTED_EDGE('',*,*,#49088,.F.);
#68542=ORIENTED_EDGE('',*,*,#44307,.F.);
#68543=ORIENTED_EDGE('',*,*,#49090,.F.);
#68544=ORIENTED_EDGE('',*,*,#49019,.T.);
#68545=ORIENTED_EDGE('',*,*,#49018,.T.);
#68546=ORIENTED_EDGE('',*,*,#49017,.T.);
#68547=ORIENTED_EDGE('',*,*,#49015,.T.);
#68548=ORIENTED_EDGE('',*,*,#49013,.T.);
#68549=ORIENTED_EDGE('',*,*,#49011,.T.);
#68550=ORIENTED_EDGE('',*,*,#49010,.T.);
#68551=ORIENTED_EDGE('',*,*,#49008,.T.);
#68552=ORIENTED_EDGE('',*,*,#49007,.T.);
#68553=ORIENTED_EDGE('',*,*,#49005,.T.);
#68554=ORIENTED_EDGE('',*,*,#49003,.T.);
#68555=ORIENTED_EDGE('',*,*,#49001,.T.);
#68556=ORIENTED_EDGE('',*,*,#48999,.T.);
#68557=ORIENTED_EDGE('',*,*,#48998,.T.);
#68558=ORIENTED_EDGE('',*,*,#48997,.T.);
#68559=ORIENTED_EDGE('',*,*,#48995,.T.);
#68560=ORIENTED_EDGE('',*,*,#48993,.T.);
#68561=ORIENTED_EDGE('',*,*,#48991,.T.);
#68562=ORIENTED_EDGE('',*,*,#48989,.T.);
#68563=ORIENTED_EDGE('',*,*,#49089,.T.);
#68564=ORIENTED_EDGE('',*,*,#43960,.F.);
#68565=ORIENTED_EDGE('',*,*,#43957,.F.);
#68566=ORIENTED_EDGE('',*,*,#43954,.F.);
#68567=ORIENTED_EDGE('',*,*,#43951,.F.);
#68568=ORIENTED_EDGE('',*,*,#43948,.F.);
#68569=ORIENTED_EDGE('',*,*,#43943,.F.);
#68570=ORIENTED_EDGE('',*,*,#43940,.F.);
#68571=ORIENTED_EDGE('',*,*,#43937,.F.);
#68572=ORIENTED_EDGE('',*,*,#43934,.F.);
#68573=ORIENTED_EDGE('',*,*,#43931,.F.);
#68574=ORIENTED_EDGE('',*,*,#43928,.F.);
#68575=ORIENTED_EDGE('',*,*,#43923,.F.);
#68576=ORIENTED_EDGE('',*,*,#43918,.F.);
#68577=ORIENTED_EDGE('',*,*,#43917,.F.);
#68578=ORIENTED_EDGE('',*,*,#43914,.F.);
#68579=ORIENTED_EDGE('',*,*,#43911,.F.);
#68580=ORIENTED_EDGE('',*,*,#43908,.F.);
#68581=ORIENTED_EDGE('',*,*,#43903,.F.);
#68582=ORIENTED_EDGE('',*,*,#43899,.F.);
#68583=ORIENTED_EDGE('',*,*,#49056,.F.);
#68584=ORIENTED_EDGE('',*,*,#48988,.T.);
#68585=ORIENTED_EDGE('',*,*,#48987,.T.);
#68586=ORIENTED_EDGE('',*,*,#48985,.T.);
#68587=ORIENTED_EDGE('',*,*,#48981,.F.);
#68588=ORIENTED_EDGE('',*,*,#49091,.F.);
#68589=ORIENTED_EDGE('',*,*,#49020,.T.);
#68590=ORIENTED_EDGE('',*,*,#49090,.T.);
#68591=ORIENTED_EDGE('',*,*,#43898,.F.);
#68592=ORIENTED_EDGE('',*,*,#44057,.T.);
#68593=ORIENTED_EDGE('',*,*,#44042,.F.);
#68594=ORIENTED_EDGE('',*,*,#44045,.T.);
#68595=ORIENTED_EDGE('',*,*,#44018,.F.);
#68596=ORIENTED_EDGE('',*,*,#44031,.T.);
#68597=ORIENTED_EDGE('',*,*,#43969,.F.);
#68598=ORIENTED_EDGE('',*,*,#43974,.F.);
#68599=ORIENTED_EDGE('',*,*,#43769,.F.);
#68600=ORIENTED_EDGE('',*,*,#43831,.T.);
#68601=ORIENTED_EDGE('',*,*,#43809,.F.);
#68602=ORIENTED_EDGE('',*,*,#43812,.T.);
#68603=ORIENTED_EDGE('',*,*,#43785,.F.);
#68604=ORIENTED_EDGE('',*,*,#43798,.T.);
#68605=ORIENTED_EDGE('',*,*,#43776,.F.);
#68606=ORIENTED_EDGE('',*,*,#49053,.T.);
#68607=ORIENTED_EDGE('',*,*,#49072,.T.);
#68608=ORIENTED_EDGE('',*,*,#49066,.F.);
#68609=ORIENTED_EDGE('',*,*,#49068,.T.);
#68610=ORIENTED_EDGE('',*,*,#49062,.F.);
#68611=ORIENTED_EDGE('',*,*,#49063,.T.);
#68612=ORIENTED_EDGE('',*,*,#49057,.F.);
#68613=ORIENTED_EDGE('',*,*,#49091,.T.);
#68614=ORIENTED_EDGE('',*,*,#48980,.T.);
#68615=ORIENTED_EDGE('',*,*,#48983,.T.);
#68616=ORIENTED_EDGE('',*,*,#48972,.F.);
#68617=ORIENTED_EDGE('',*,*,#48974,.T.);
#68618=ORIENTED_EDGE('',*,*,#48968,.F.);
#68619=ORIENTED_EDGE('',*,*,#48969,.T.);
#68620=ORIENTED_EDGE('',*,*,#48963,.F.);
#68621=ORIENTED_EDGE('',*,*,#45308,.T.);
#68622=ORIENTED_EDGE('',*,*,#45324,.T.);
#68623=ORIENTED_EDGE('',*,*,#48249,.F.);
#68624=ORIENTED_EDGE('',*,*,#48228,.F.);
#68625=ORIENTED_EDGE('',*,*,#49092,.T.);
#68626=ORIENTED_EDGE('',*,*,#49093,.T.);
#68627=ORIENTED_EDGE('',*,*,#49094,.F.);
#68628=ORIENTED_EDGE('',*,*,#49095,.T.);
#68629=ORIENTED_EDGE('',*,*,#49096,.T.);
#68630=ORIENTED_EDGE('',*,*,#49097,.T.);
#68631=ORIENTED_EDGE('',*,*,#49092,.F.);
#68632=ORIENTED_EDGE('',*,*,#49098,.T.);
#68633=ORIENTED_EDGE('',*,*,#49099,.T.);
#68634=ORIENTED_EDGE('',*,*,#49100,.T.);
#68635=ORIENTED_EDGE('',*,*,#49096,.F.);
#68636=ORIENTED_EDGE('',*,*,#49101,.T.);
#68637=ORIENTED_EDGE('',*,*,#49102,.T.);
#68638=ORIENTED_EDGE('',*,*,#49103,.T.);
#68639=ORIENTED_EDGE('',*,*,#49099,.F.);
#68640=ORIENTED_EDGE('',*,*,#49104,.T.);
#68641=ORIENTED_EDGE('',*,*,#49105,.T.);
#68642=ORIENTED_EDGE('',*,*,#49106,.T.);
#68643=ORIENTED_EDGE('',*,*,#49102,.F.);
#68644=ORIENTED_EDGE('',*,*,#49107,.T.);
#68645=ORIENTED_EDGE('',*,*,#49094,.T.);
#68646=ORIENTED_EDGE('',*,*,#49108,.T.);
#68647=ORIENTED_EDGE('',*,*,#49105,.F.);
#68648=ORIENTED_EDGE('',*,*,#49109,.T.);
#68649=ORIENTED_EDGE('',*,*,#49110,.T.);
#68650=ORIENTED_EDGE('',*,*,#49101,.F.);
#68651=ORIENTED_EDGE('',*,*,#49098,.F.);
#68652=ORIENTED_EDGE('',*,*,#49095,.F.);
#68653=ORIENTED_EDGE('',*,*,#49109,.F.);
#68654=ORIENTED_EDGE('',*,*,#49107,.F.);
#68655=ORIENTED_EDGE('',*,*,#49104,.F.);
#68656=ORIENTED_EDGE('',*,*,#49110,.F.);
#68657=ORIENTED_EDGE('',*,*,#49111,.T.);
#68658=ORIENTED_EDGE('',*,*,#49093,.F.);
#68659=ORIENTED_EDGE('',*,*,#49112,.T.);
#68660=ORIENTED_EDGE('',*,*,#49097,.F.);
#68661=ORIENTED_EDGE('',*,*,#49113,.T.);
#68662=ORIENTED_EDGE('',*,*,#49100,.F.);
#68663=ORIENTED_EDGE('',*,*,#49114,.T.);
#68664=ORIENTED_EDGE('',*,*,#49103,.F.);
#68665=ORIENTED_EDGE('',*,*,#49115,.T.);
#68666=ORIENTED_EDGE('',*,*,#49106,.F.);
#68667=ORIENTED_EDGE('',*,*,#49116,.T.);
#68668=ORIENTED_EDGE('',*,*,#49108,.F.);
#68669=ORIENTED_EDGE('',*,*,#49117,.F.);
#68670=ORIENTED_EDGE('',*,*,#49118,.T.);
#68671=ORIENTED_EDGE('',*,*,#49119,.F.);
#68672=ORIENTED_EDGE('',*,*,#49120,.F.);
#68673=ORIENTED_EDGE('',*,*,#49118,.F.);
#68674=ORIENTED_EDGE('',*,*,#49121,.F.);
#68675=ORIENTED_EDGE('',*,*,#49117,.T.);
#68676=ORIENTED_EDGE('',*,*,#49116,.F.);
#68677=ORIENTED_EDGE('',*,*,#49111,.F.);
#68678=ORIENTED_EDGE('',*,*,#49112,.F.);
#68679=ORIENTED_EDGE('',*,*,#49113,.F.);
#68680=ORIENTED_EDGE('',*,*,#49114,.F.);
#68681=ORIENTED_EDGE('',*,*,#49115,.F.);
#68682=ORIENTED_EDGE('',*,*,#49121,.T.);
#68683=ORIENTED_EDGE('',*,*,#49122,.T.);
#68684=ORIENTED_EDGE('',*,*,#49119,.T.);
#68685=ORIENTED_EDGE('',*,*,#49120,.T.);
#68686=ORIENTED_EDGE('',*,*,#49122,.F.);
#68687=ORIENTED_EDGE('',*,*,#49123,.F.);
#68688=ORIENTED_EDGE('',*,*,#49124,.T.);
#68689=ORIENTED_EDGE('',*,*,#49125,.F.);
#68690=ORIENTED_EDGE('',*,*,#49124,.F.);
#68691=ORIENTED_EDGE('',*,*,#49125,.T.);
#68692=ORIENTED_EDGE('',*,*,#49126,.T.);
#68693=ORIENTED_EDGE('',*,*,#49127,.T.);
#68694=ORIENTED_EDGE('',*,*,#49123,.T.);
#68695=ORIENTED_EDGE('',*,*,#49127,.F.);
#68696=ORIENTED_EDGE('',*,*,#49128,.F.);
#68697=ORIENTED_EDGE('',*,*,#49126,.F.);
#68698=ORIENTED_EDGE('',*,*,#49129,.T.);
#68699=ORIENTED_EDGE('',*,*,#49130,.T.);
#68700=ORIENTED_EDGE('',*,*,#49128,.T.);
#68701=ORIENTED_EDGE('',*,*,#49130,.F.);
#68702=ORIENTED_EDGE('',*,*,#49129,.F.);
#68703=ORIENTED_EDGE('',*,*,#49131,.F.);
#68704=ORIENTED_EDGE('',*,*,#49132,.T.);
#68705=ORIENTED_EDGE('',*,*,#49133,.F.);
#68706=ORIENTED_EDGE('',*,*,#49134,.T.);
#68707=ORIENTED_EDGE('',*,*,#49135,.T.);
#68708=ORIENTED_EDGE('',*,*,#49136,.T.);
#68709=ORIENTED_EDGE('',*,*,#49137,.T.);
#68710=ORIENTED_EDGE('',*,*,#49138,.T.);
#68711=ORIENTED_EDGE('',*,*,#49136,.F.);
#68712=ORIENTED_EDGE('',*,*,#49139,.F.);
#68713=ORIENTED_EDGE('',*,*,#49140,.T.);
#68714=ORIENTED_EDGE('',*,*,#49141,.F.);
#68715=ORIENTED_EDGE('',*,*,#49142,.T.);
#68716=ORIENTED_EDGE('',*,*,#49143,.F.);
#68717=ORIENTED_EDGE('',*,*,#49144,.T.);
#68718=ORIENTED_EDGE('',*,*,#49141,.T.);
#68719=ORIENTED_EDGE('',*,*,#49145,.T.);
#68720=ORIENTED_EDGE('',*,*,#49146,.T.);
#68721=ORIENTED_EDGE('',*,*,#49139,.T.);
#68722=ORIENTED_EDGE('',*,*,#49147,.F.);
#68723=ORIENTED_EDGE('',*,*,#49148,.F.);
#68724=ORIENTED_EDGE('',*,*,#49149,.T.);
#68725=ORIENTED_EDGE('',*,*,#49143,.T.);
#68726=ORIENTED_EDGE('',*,*,#49150,.T.);
#68727=ORIENTED_EDGE('',*,*,#49151,.F.);
#68728=ORIENTED_EDGE('',*,*,#49152,.T.);
#68729=ORIENTED_EDGE('',*,*,#49147,.T.);
#68730=ORIENTED_EDGE('',*,*,#49153,.T.);
#68731=ORIENTED_EDGE('',*,*,#49154,.F.);
#68732=ORIENTED_EDGE('',*,*,#49155,.T.);
#68733=ORIENTED_EDGE('',*,*,#49148,.T.);
#68734=ORIENTED_EDGE('',*,*,#49156,.T.);
#68735=ORIENTED_EDGE('',*,*,#49157,.F.);
#68736=ORIENTED_EDGE('',*,*,#49158,.T.);
#68737=ORIENTED_EDGE('',*,*,#49151,.T.);
#68738=ORIENTED_EDGE('',*,*,#49159,.T.);
#68739=ORIENTED_EDGE('',*,*,#49160,.F.);
#68740=ORIENTED_EDGE('',*,*,#49161,.T.);
#68741=ORIENTED_EDGE('',*,*,#49154,.T.);
#68742=ORIENTED_EDGE('',*,*,#49162,.T.);
#68743=ORIENTED_EDGE('',*,*,#49163,.F.);
#68744=ORIENTED_EDGE('',*,*,#49164,.T.);
#68745=ORIENTED_EDGE('',*,*,#49157,.T.);
#68746=ORIENTED_EDGE('',*,*,#49165,.T.);
#68747=ORIENTED_EDGE('',*,*,#49166,.F.);
#68748=ORIENTED_EDGE('',*,*,#49167,.T.);
#68749=ORIENTED_EDGE('',*,*,#49160,.T.);
#68750=ORIENTED_EDGE('',*,*,#49168,.T.);
#68751=ORIENTED_EDGE('',*,*,#49169,.F.);
#68752=ORIENTED_EDGE('',*,*,#49170,.T.);
#68753=ORIENTED_EDGE('',*,*,#49163,.T.);
#68754=ORIENTED_EDGE('',*,*,#49171,.T.);
#68755=ORIENTED_EDGE('',*,*,#49172,.F.);
#68756=ORIENTED_EDGE('',*,*,#49173,.T.);
#68757=ORIENTED_EDGE('',*,*,#49174,.T.);
#68758=ORIENTED_EDGE('',*,*,#49166,.T.);
#68759=ORIENTED_EDGE('',*,*,#49175,.T.);
#68760=ORIENTED_EDGE('',*,*,#49169,.T.);
#68761=ORIENTED_EDGE('',*,*,#49172,.T.);
#68762=ORIENTED_EDGE('',*,*,#49176,.T.);
#68763=ORIENTED_EDGE('',*,*,#49177,.F.);
#68764=ORIENTED_EDGE('',*,*,#49178,.T.);
#68765=ORIENTED_EDGE('',*,*,#49179,.F.);
#68766=ORIENTED_EDGE('',*,*,#49180,.T.);
#68767=ORIENTED_EDGE('',*,*,#49181,.F.);
#68768=ORIENTED_EDGE('',*,*,#49182,.T.);
#68769=ORIENTED_EDGE('',*,*,#49179,.T.);
#68770=ORIENTED_EDGE('',*,*,#49183,.T.);
#68771=ORIENTED_EDGE('',*,*,#49184,.F.);
#68772=ORIENTED_EDGE('',*,*,#49185,.T.);
#68773=ORIENTED_EDGE('',*,*,#49177,.T.);
#68774=ORIENTED_EDGE('',*,*,#49186,.T.);
#68775=ORIENTED_EDGE('',*,*,#49187,.F.);
#68776=ORIENTED_EDGE('',*,*,#49188,.T.);
#68777=ORIENTED_EDGE('',*,*,#49181,.T.);
#68778=ORIENTED_EDGE('',*,*,#49189,.T.);
#68779=ORIENTED_EDGE('',*,*,#49190,.F.);
#68780=ORIENTED_EDGE('',*,*,#49191,.T.);
#68781=ORIENTED_EDGE('',*,*,#49184,.T.);
#68782=ORIENTED_EDGE('',*,*,#49192,.T.);
#68783=ORIENTED_EDGE('',*,*,#49193,.F.);
#68784=ORIENTED_EDGE('',*,*,#49187,.T.);
#68785=ORIENTED_EDGE('',*,*,#49194,.T.);
#68786=ORIENTED_EDGE('',*,*,#49195,.F.);
#68787=ORIENTED_EDGE('',*,*,#49196,.T.);
#68788=ORIENTED_EDGE('',*,*,#49190,.T.);
#68789=ORIENTED_EDGE('',*,*,#49197,.T.);
#68790=ORIENTED_EDGE('',*,*,#49198,.F.);
#68791=ORIENTED_EDGE('',*,*,#49199,.T.);
#68792=ORIENTED_EDGE('',*,*,#49193,.T.);
#68793=ORIENTED_EDGE('',*,*,#49200,.T.);
#68794=ORIENTED_EDGE('',*,*,#49201,.F.);
#68795=ORIENTED_EDGE('',*,*,#49202,.T.);
#68796=ORIENTED_EDGE('',*,*,#49195,.T.);
#68797=ORIENTED_EDGE('',*,*,#49203,.T.);
#68798=ORIENTED_EDGE('',*,*,#49204,.F.);
#68799=ORIENTED_EDGE('',*,*,#49205,.T.);
#68800=ORIENTED_EDGE('',*,*,#49198,.T.);
#68801=ORIENTED_EDGE('',*,*,#49206,.T.);
#68802=ORIENTED_EDGE('',*,*,#49207,.T.);
#68803=ORIENTED_EDGE('',*,*,#49201,.T.);
#68804=ORIENTED_EDGE('',*,*,#49208,.F.);
#68805=ORIENTED_EDGE('',*,*,#49209,.F.);
#68806=ORIENTED_EDGE('',*,*,#49210,.T.);
#68807=ORIENTED_EDGE('',*,*,#49204,.T.);
#68808=ORIENTED_EDGE('',*,*,#49211,.T.);
#68809=ORIENTED_EDGE('',*,*,#49212,.F.);
#68810=ORIENTED_EDGE('',*,*,#49213,.T.);
#68811=ORIENTED_EDGE('',*,*,#49208,.T.);
#68812=ORIENTED_EDGE('',*,*,#49214,.T.);
#68813=ORIENTED_EDGE('',*,*,#49209,.T.);
#68814=ORIENTED_EDGE('',*,*,#49215,.T.);
#68815=ORIENTED_EDGE('',*,*,#49212,.T.);
#68816=ORIENTED_EDGE('',*,*,#49216,.T.);
#68817=ORIENTED_EDGE('',*,*,#49217,.F.);
#68818=ORIENTED_EDGE('',*,*,#49218,.T.);
#68819=ORIENTED_EDGE('',*,*,#49219,.T.);
#68820=ORIENTED_EDGE('',*,*,#49220,.T.);
#68821=ORIENTED_EDGE('',*,*,#49221,.F.);
#68822=ORIENTED_EDGE('',*,*,#49222,.T.);
#68823=ORIENTED_EDGE('',*,*,#49217,.T.);
#68824=ORIENTED_EDGE('',*,*,#49223,.T.);
#68825=ORIENTED_EDGE('',*,*,#49224,.F.);
#68826=ORIENTED_EDGE('',*,*,#49225,.T.);
#68827=ORIENTED_EDGE('',*,*,#49221,.T.);
#68828=ORIENTED_EDGE('',*,*,#49226,.T.);
#68829=ORIENTED_EDGE('',*,*,#49227,.F.);
#68830=ORIENTED_EDGE('',*,*,#49228,.T.);
#68831=ORIENTED_EDGE('',*,*,#49224,.T.);
#68832=ORIENTED_EDGE('',*,*,#49229,.T.);
#68833=ORIENTED_EDGE('',*,*,#49230,.F.);
#68834=ORIENTED_EDGE('',*,*,#49231,.T.);
#68835=ORIENTED_EDGE('',*,*,#49227,.T.);
#68836=ORIENTED_EDGE('',*,*,#49232,.T.);
#68837=ORIENTED_EDGE('',*,*,#49233,.F.);
#68838=ORIENTED_EDGE('',*,*,#49234,.T.);
#68839=ORIENTED_EDGE('',*,*,#49230,.T.);
#68840=ORIENTED_EDGE('',*,*,#49235,.T.);
#68841=ORIENTED_EDGE('',*,*,#49236,.F.);
#68842=ORIENTED_EDGE('',*,*,#49237,.T.);
#68843=ORIENTED_EDGE('',*,*,#49233,.T.);
#68844=ORIENTED_EDGE('',*,*,#49238,.T.);
#68845=ORIENTED_EDGE('',*,*,#49239,.T.);
#68846=ORIENTED_EDGE('',*,*,#49240,.F.);
#68847=ORIENTED_EDGE('',*,*,#49241,.T.);
#68848=ORIENTED_EDGE('',*,*,#49146,.F.);
#68849=ORIENTED_EDGE('',*,*,#49242,.F.);
#68850=ORIENTED_EDGE('',*,*,#49243,.T.);
#68851=ORIENTED_EDGE('',*,*,#49240,.T.);
#68852=ORIENTED_EDGE('',*,*,#49244,.T.);
#68853=ORIENTED_EDGE('',*,*,#49245,.T.);
#68854=ORIENTED_EDGE('',*,*,#49246,.F.);
#68855=ORIENTED_EDGE('',*,*,#49247,.T.);
#68856=ORIENTED_EDGE('',*,*,#49176,.F.);
#68857=ORIENTED_EDGE('',*,*,#49248,.F.);
#68858=ORIENTED_EDGE('',*,*,#49249,.T.);
#68859=ORIENTED_EDGE('',*,*,#49242,.T.);
#68860=ORIENTED_EDGE('',*,*,#49250,.T.);
#68861=ORIENTED_EDGE('',*,*,#49251,.F.);
#68862=ORIENTED_EDGE('',*,*,#49252,.T.);
#68863=ORIENTED_EDGE('',*,*,#49246,.T.);
#68864=ORIENTED_EDGE('',*,*,#49253,.T.);
#68865=ORIENTED_EDGE('',*,*,#49254,.F.);
#68866=ORIENTED_EDGE('',*,*,#49255,.T.);
#68867=ORIENTED_EDGE('',*,*,#49248,.T.);
#68868=ORIENTED_EDGE('',*,*,#49256,.T.);
#68869=ORIENTED_EDGE('',*,*,#49257,.F.);
#68870=ORIENTED_EDGE('',*,*,#49258,.T.);
#68871=ORIENTED_EDGE('',*,*,#49251,.T.);
#68872=ORIENTED_EDGE('',*,*,#49259,.T.);
#68873=ORIENTED_EDGE('',*,*,#49260,.F.);
#68874=ORIENTED_EDGE('',*,*,#49261,.T.);
#68875=ORIENTED_EDGE('',*,*,#49254,.T.);
#68876=ORIENTED_EDGE('',*,*,#49262,.T.);
#68877=ORIENTED_EDGE('',*,*,#49263,.F.);
#68878=ORIENTED_EDGE('',*,*,#49264,.T.);
#68879=ORIENTED_EDGE('',*,*,#49257,.T.);
#68880=ORIENTED_EDGE('',*,*,#49265,.T.);
#68881=ORIENTED_EDGE('',*,*,#49266,.F.);
#68882=ORIENTED_EDGE('',*,*,#49267,.T.);
#68883=ORIENTED_EDGE('',*,*,#49260,.T.);
#68884=ORIENTED_EDGE('',*,*,#49268,.T.);
#68885=ORIENTED_EDGE('',*,*,#49269,.F.);
#68886=ORIENTED_EDGE('',*,*,#49270,.T.);
#68887=ORIENTED_EDGE('',*,*,#49263,.T.);
#68888=ORIENTED_EDGE('',*,*,#49271,.T.);
#68889=ORIENTED_EDGE('',*,*,#49272,.F.);
#68890=ORIENTED_EDGE('',*,*,#49273,.T.);
#68891=ORIENTED_EDGE('',*,*,#49266,.T.);
#68892=ORIENTED_EDGE('',*,*,#49274,.T.);
#68893=ORIENTED_EDGE('',*,*,#49269,.T.);
#68894=ORIENTED_EDGE('',*,*,#49275,.T.);
#68895=ORIENTED_EDGE('',*,*,#49272,.T.);
#68896=ORIENTED_EDGE('',*,*,#49276,.T.);
#68897=ORIENTED_EDGE('',*,*,#49277,.F.);
#68898=ORIENTED_EDGE('',*,*,#49278,.T.);
#68899=ORIENTED_EDGE('',*,*,#49279,.F.);
#68900=ORIENTED_EDGE('',*,*,#49280,.T.);
#68901=ORIENTED_EDGE('',*,*,#49281,.F.);
#68902=ORIENTED_EDGE('',*,*,#49282,.T.);
#68903=ORIENTED_EDGE('',*,*,#49279,.T.);
#68904=ORIENTED_EDGE('',*,*,#49283,.T.);
#68905=ORIENTED_EDGE('',*,*,#49284,.F.);
#68906=ORIENTED_EDGE('',*,*,#49285,.T.);
#68907=ORIENTED_EDGE('',*,*,#49277,.T.);
#68908=ORIENTED_EDGE('',*,*,#49286,.T.);
#68909=ORIENTED_EDGE('',*,*,#49287,.F.);
#68910=ORIENTED_EDGE('',*,*,#49288,.T.);
#68911=ORIENTED_EDGE('',*,*,#49281,.T.);
#68912=ORIENTED_EDGE('',*,*,#49289,.T.);
#68913=ORIENTED_EDGE('',*,*,#49290,.F.);
#68914=ORIENTED_EDGE('',*,*,#49291,.T.);
#68915=ORIENTED_EDGE('',*,*,#49284,.T.);
#68916=ORIENTED_EDGE('',*,*,#49292,.T.);
#68917=ORIENTED_EDGE('',*,*,#49293,.F.);
#68918=ORIENTED_EDGE('',*,*,#49294,.T.);
#68919=ORIENTED_EDGE('',*,*,#49295,.T.);
#68920=ORIENTED_EDGE('',*,*,#49287,.T.);
#68921=ORIENTED_EDGE('',*,*,#49296,.T.);
#68922=ORIENTED_EDGE('',*,*,#49297,.F.);
#68923=ORIENTED_EDGE('',*,*,#49298,.T.);
#68924=ORIENTED_EDGE('',*,*,#49290,.T.);
#68925=ORIENTED_EDGE('',*,*,#49299,.T.);
#68926=ORIENTED_EDGE('',*,*,#49300,.F.);
#68927=ORIENTED_EDGE('',*,*,#49301,.T.);
#68928=ORIENTED_EDGE('',*,*,#49293,.T.);
#68929=ORIENTED_EDGE('',*,*,#49302,.T.);
#68930=ORIENTED_EDGE('',*,*,#49303,.T.);
#68931=ORIENTED_EDGE('',*,*,#49297,.T.);
#68932=ORIENTED_EDGE('',*,*,#49304,.T.);
#68933=ORIENTED_EDGE('',*,*,#49194,.F.);
#68934=ORIENTED_EDGE('',*,*,#49305,.F.);
#68935=ORIENTED_EDGE('',*,*,#49306,.T.);
#68936=ORIENTED_EDGE('',*,*,#49300,.T.);
#68937=ORIENTED_EDGE('',*,*,#49307,.T.);
#68938=ORIENTED_EDGE('',*,*,#49308,.T.);
#68939=ORIENTED_EDGE('',*,*,#49305,.T.);
#68940=ORIENTED_EDGE('',*,*,#49309,.T.);
#68941=ORIENTED_EDGE('',*,*,#49207,.F.);
#68942=ORIENTED_EDGE('',*,*,#49310,.T.);
#68943=ORIENTED_EDGE('',*,*,#49311,.F.);
#68944=ORIENTED_EDGE('',*,*,#49312,.T.);
#68945=ORIENTED_EDGE('',*,*,#49192,.F.);
#68946=ORIENTED_EDGE('',*,*,#49313,.T.);
#68947=ORIENTED_EDGE('',*,*,#49311,.T.);
#68948=ORIENTED_EDGE('',*,*,#49314,.T.);
#68949=ORIENTED_EDGE('',*,*,#49315,.F.);
#68950=ORIENTED_EDGE('',*,*,#49316,.T.);
#68951=ORIENTED_EDGE('',*,*,#49317,.F.);
#68952=ORIENTED_EDGE('',*,*,#49318,.T.);
#68953=ORIENTED_EDGE('',*,*,#49315,.T.);
#68954=ORIENTED_EDGE('',*,*,#49319,.T.);
#68955=ORIENTED_EDGE('',*,*,#49132,.F.);
#68956=ORIENTED_EDGE('',*,*,#49320,.F.);
#68957=ORIENTED_EDGE('',*,*,#49321,.T.);
#68958=ORIENTED_EDGE('',*,*,#49317,.T.);
#68959=ORIENTED_EDGE('',*,*,#49322,.T.);
#68960=ORIENTED_EDGE('',*,*,#49323,.T.);
#68961=ORIENTED_EDGE('',*,*,#49320,.T.);
#68962=ORIENTED_EDGE('',*,*,#49324,.T.);
#68963=ORIENTED_EDGE('',*,*,#49180,.F.);
#68964=ORIENTED_EDGE('',*,*,#49325,.T.);
#68965=ORIENTED_EDGE('',*,*,#49326,.F.);
#68966=ORIENTED_EDGE('',*,*,#49327,.T.);
#68967=ORIENTED_EDGE('',*,*,#49308,.F.);
#68968=ORIENTED_EDGE('',*,*,#49213,.F.);
#68969=ORIENTED_EDGE('',*,*,#49328,.T.);
#68970=ORIENTED_EDGE('',*,*,#49326,.T.);
#68971=ORIENTED_EDGE('',*,*,#49329,.T.);
#68972=ORIENTED_EDGE('',*,*,#49330,.F.);
#68973=ORIENTED_EDGE('',*,*,#49331,.F.);
#68974=ORIENTED_EDGE('',*,*,#49332,.T.);
#68975=ORIENTED_EDGE('',*,*,#49330,.T.);
#68976=ORIENTED_EDGE('',*,*,#49333,.T.);
#68977=ORIENTED_EDGE('',*,*,#49334,.F.);
#68978=ORIENTED_EDGE('',*,*,#49335,.T.);
#68979=ORIENTED_EDGE('',*,*,#49331,.T.);
#68980=ORIENTED_EDGE('',*,*,#49336,.T.);
#68981=ORIENTED_EDGE('',*,*,#49304,.F.);
#68982=ORIENTED_EDGE('',*,*,#49337,.T.);
#68983=ORIENTED_EDGE('',*,*,#49334,.T.);
#68984=ORIENTED_EDGE('',*,*,#49338,.T.);
#68985=ORIENTED_EDGE('',*,*,#49200,.F.);
#68986=ORIENTED_EDGE('',*,*,#49339,.T.);
#68987=ORIENTED_EDGE('',*,*,#49340,.F.);
#68988=ORIENTED_EDGE('',*,*,#49341,.T.);
#68989=ORIENTED_EDGE('',*,*,#49250,.F.);
#68990=ORIENTED_EDGE('',*,*,#49342,.F.);
#68991=ORIENTED_EDGE('',*,*,#49343,.T.);
#68992=ORIENTED_EDGE('',*,*,#49340,.T.);
#68993=ORIENTED_EDGE('',*,*,#49344,.T.);
#68994=ORIENTED_EDGE('',*,*,#49345,.F.);
#68995=ORIENTED_EDGE('',*,*,#49346,.T.);
#68996=ORIENTED_EDGE('',*,*,#49342,.T.);
#68997=ORIENTED_EDGE('',*,*,#49347,.T.);
#68998=ORIENTED_EDGE('',*,*,#49348,.T.);
#68999=ORIENTED_EDGE('',*,*,#49349,.F.);
#69000=ORIENTED_EDGE('',*,*,#49350,.T.);
#69001=ORIENTED_EDGE('',*,*,#49345,.T.);
#69002=ORIENTED_EDGE('',*,*,#49247,.F.);
#69003=ORIENTED_EDGE('',*,*,#49351,.T.);
#69004=ORIENTED_EDGE('',*,*,#49349,.T.);
#69005=ORIENTED_EDGE('',*,*,#49352,.T.);
#69006=ORIENTED_EDGE('',*,*,#49170,.F.);
#69007=ORIENTED_EDGE('',*,*,#49353,.T.);
#69008=ORIENTED_EDGE('',*,*,#49354,.F.);
#69009=ORIENTED_EDGE('',*,*,#49355,.T.);
#69010=ORIENTED_EDGE('',*,*,#49149,.F.);
#69011=ORIENTED_EDGE('',*,*,#49356,.F.);
#69012=ORIENTED_EDGE('',*,*,#49357,.T.);
#69013=ORIENTED_EDGE('',*,*,#49354,.T.);
#69014=ORIENTED_EDGE('',*,*,#49358,.T.);
#69015=ORIENTED_EDGE('',*,*,#49359,.F.);
#69016=ORIENTED_EDGE('',*,*,#49360,.T.);
#69017=ORIENTED_EDGE('',*,*,#49356,.T.);
#69018=ORIENTED_EDGE('',*,*,#49361,.T.);
#69019=ORIENTED_EDGE('',*,*,#49362,.T.);
#69020=ORIENTED_EDGE('',*,*,#49363,.F.);
#69021=ORIENTED_EDGE('',*,*,#49364,.T.);
#69022=ORIENTED_EDGE('',*,*,#49359,.T.);
#69023=ORIENTED_EDGE('',*,*,#49365,.T.);
#69024=ORIENTED_EDGE('',*,*,#49363,.T.);
#69025=ORIENTED_EDGE('',*,*,#49366,.T.);
#69026=ORIENTED_EDGE('',*,*,#49161,.F.);
#69027=ORIENTED_EDGE('',*,*,#49367,.T.);
#69028=ORIENTED_EDGE('',*,*,#49335,.F.);
#69029=ORIENTED_EDGE('',*,*,#49368,.T.);
#69030=ORIENTED_EDGE('',*,*,#49286,.F.);
#69031=ORIENTED_EDGE('',*,*,#49280,.F.);
#69032=ORIENTED_EDGE('',*,*,#49294,.F.);
#69033=ORIENTED_EDGE('',*,*,#49369,.T.);
#69034=ORIENTED_EDGE('',*,*,#49328,.F.);
#69035=ORIENTED_EDGE('',*,*,#49370,.T.);
#69036=ORIENTED_EDGE('',*,*,#49288,.F.);
#69037=ORIENTED_EDGE('',*,*,#49295,.F.);
#69038=ORIENTED_EDGE('',*,*,#49371,.T.);
#69039=ORIENTED_EDGE('',*,*,#49321,.F.);
#69040=ORIENTED_EDGE('',*,*,#49372,.T.);
#69041=ORIENTED_EDGE('',*,*,#49188,.F.);
#69042=ORIENTED_EDGE('',*,*,#49199,.F.);
#69043=ORIENTED_EDGE('',*,*,#49205,.F.);
#69044=ORIENTED_EDGE('',*,*,#49373,.T.);
#69045=ORIENTED_EDGE('',*,*,#49313,.F.);
#69046=ORIENTED_EDGE('',*,*,#49374,.T.);
#69047=ORIENTED_EDGE('',*,*,#49216,.F.);
#69048=ORIENTED_EDGE('',*,*,#49214,.F.);
#69049=ORIENTED_EDGE('',*,*,#49203,.F.);
#69050=ORIENTED_EDGE('',*,*,#49375,.T.);
#69051=ORIENTED_EDGE('',*,*,#49357,.F.);
#69052=ORIENTED_EDGE('',*,*,#49376,.T.);
#69053=ORIENTED_EDGE('',*,*,#49153,.F.);
#69054=ORIENTED_EDGE('',*,*,#49142,.F.);
#69055=ORIENTED_EDGE('',*,*,#49364,.F.);
#69056=ORIENTED_EDGE('',*,*,#49377,.T.);
#69057=ORIENTED_EDGE('',*,*,#49174,.F.);
#69058=ORIENTED_EDGE('',*,*,#49173,.F.);
#69059=ORIENTED_EDGE('',*,*,#49171,.F.);
#69060=ORIENTED_EDGE('',*,*,#49165,.F.);
#69061=ORIENTED_EDGE('',*,*,#49378,.T.);
#69062=ORIENTED_EDGE('',*,*,#49270,.F.);
#69063=ORIENTED_EDGE('',*,*,#49379,.T.);
#69064=ORIENTED_EDGE('',*,*,#49350,.F.);
#69065=ORIENTED_EDGE('',*,*,#49380,.T.);
#69066=ORIENTED_EDGE('',*,*,#49264,.F.);
#69067=ORIENTED_EDGE('',*,*,#49268,.F.);
#69068=ORIENTED_EDGE('',*,*,#49381,.T.);
#69069=ORIENTED_EDGE('',*,*,#49343,.F.);
#69070=ORIENTED_EDGE('',*,*,#49382,.T.);
#69071=ORIENTED_EDGE('',*,*,#49274,.F.);
#69072=ORIENTED_EDGE('',*,*,#49383,.T.);
#69073=ORIENTED_EDGE('',*,*,#49384,.F.);
#69074=ORIENTED_EDGE('',*,*,#49385,.T.);
#69075=ORIENTED_EDGE('',*,*,#49386,.F.);
#69076=ORIENTED_EDGE('',*,*,#49387,.F.);
#69077=ORIENTED_EDGE('',*,*,#49388,.T.);
#69078=ORIENTED_EDGE('',*,*,#49384,.T.);
#69079=ORIENTED_EDGE('',*,*,#49389,.T.);
#69080=ORIENTED_EDGE('',*,*,#49390,.F.);
#69081=ORIENTED_EDGE('',*,*,#49391,.T.);
#69082=ORIENTED_EDGE('',*,*,#49386,.T.);
#69083=ORIENTED_EDGE('',*,*,#49392,.T.);
#69084=ORIENTED_EDGE('',*,*,#49393,.F.);
#69085=ORIENTED_EDGE('',*,*,#49394,.T.);
#69086=ORIENTED_EDGE('',*,*,#49387,.T.);
#69087=ORIENTED_EDGE('',*,*,#49395,.T.);
#69088=ORIENTED_EDGE('',*,*,#49396,.F.);
#69089=ORIENTED_EDGE('',*,*,#49397,.T.);
#69090=ORIENTED_EDGE('',*,*,#49390,.T.);
#69091=ORIENTED_EDGE('',*,*,#49398,.T.);
#69092=ORIENTED_EDGE('',*,*,#49399,.F.);
#69093=ORIENTED_EDGE('',*,*,#49400,.T.);
#69094=ORIENTED_EDGE('',*,*,#49393,.T.);
#69095=ORIENTED_EDGE('',*,*,#49401,.T.);
#69096=ORIENTED_EDGE('',*,*,#49402,.F.);
#69097=ORIENTED_EDGE('',*,*,#49403,.T.);
#69098=ORIENTED_EDGE('',*,*,#49396,.T.);
#69099=ORIENTED_EDGE('',*,*,#49404,.T.);
#69100=ORIENTED_EDGE('',*,*,#49405,.F.);
#69101=ORIENTED_EDGE('',*,*,#49406,.T.);
#69102=ORIENTED_EDGE('',*,*,#49399,.T.);
#69103=ORIENTED_EDGE('',*,*,#49407,.T.);
#69104=ORIENTED_EDGE('',*,*,#49408,.F.);
#69105=ORIENTED_EDGE('',*,*,#49409,.T.);
#69106=ORIENTED_EDGE('',*,*,#49402,.T.);
#69107=ORIENTED_EDGE('',*,*,#49410,.T.);
#69108=ORIENTED_EDGE('',*,*,#49405,.T.);
#69109=ORIENTED_EDGE('',*,*,#49411,.T.);
#69110=ORIENTED_EDGE('',*,*,#49408,.T.);
#69111=ORIENTED_EDGE('',*,*,#49412,.T.);
#69112=ORIENTED_EDGE('',*,*,#49413,.T.);
#69113=ORIENTED_EDGE('',*,*,#49414,.F.);
#69114=ORIENTED_EDGE('',*,*,#49415,.T.);
#69115=ORIENTED_EDGE('',*,*,#49416,.F.);
#69116=ORIENTED_EDGE('',*,*,#49417,.F.);
#69117=ORIENTED_EDGE('',*,*,#49418,.T.);
#69118=ORIENTED_EDGE('',*,*,#49414,.T.);
#69119=ORIENTED_EDGE('',*,*,#49419,.T.);
#69120=ORIENTED_EDGE('',*,*,#49420,.F.);
#69121=ORIENTED_EDGE('',*,*,#49421,.T.);
#69122=ORIENTED_EDGE('',*,*,#49416,.T.);
#69123=ORIENTED_EDGE('',*,*,#49422,.T.);
#69124=ORIENTED_EDGE('',*,*,#49423,.F.);
#69125=ORIENTED_EDGE('',*,*,#49424,.T.);
#69126=ORIENTED_EDGE('',*,*,#49417,.T.);
#69127=ORIENTED_EDGE('',*,*,#49425,.T.);
#69128=ORIENTED_EDGE('',*,*,#49426,.F.);
#69129=ORIENTED_EDGE('',*,*,#49427,.T.);
#69130=ORIENTED_EDGE('',*,*,#49420,.T.);
#69131=ORIENTED_EDGE('',*,*,#49428,.T.);
#69132=ORIENTED_EDGE('',*,*,#49429,.F.);
#69133=ORIENTED_EDGE('',*,*,#49430,.T.);
#69134=ORIENTED_EDGE('',*,*,#49423,.T.);
#69135=ORIENTED_EDGE('',*,*,#49431,.T.);
#69136=ORIENTED_EDGE('',*,*,#49432,.F.);
#69137=ORIENTED_EDGE('',*,*,#49433,.T.);
#69138=ORIENTED_EDGE('',*,*,#49426,.T.);
#69139=ORIENTED_EDGE('',*,*,#49434,.T.);
#69140=ORIENTED_EDGE('',*,*,#49429,.T.);
#69141=ORIENTED_EDGE('',*,*,#49435,.T.);
#69142=ORIENTED_EDGE('',*,*,#49432,.T.);
#69143=ORIENTED_EDGE('',*,*,#49436,.T.);
#69144=ORIENTED_EDGE('',*,*,#49437,.T.);
#69145=ORIENTED_EDGE('',*,*,#49438,.F.);
#69146=ORIENTED_EDGE('',*,*,#49439,.T.);
#69147=ORIENTED_EDGE('',*,*,#49440,.F.);
#69148=ORIENTED_EDGE('',*,*,#49441,.F.);
#69149=ORIENTED_EDGE('',*,*,#49442,.T.);
#69150=ORIENTED_EDGE('',*,*,#49438,.T.);
#69151=ORIENTED_EDGE('',*,*,#49443,.T.);
#69152=ORIENTED_EDGE('',*,*,#49444,.F.);
#69153=ORIENTED_EDGE('',*,*,#49445,.T.);
#69154=ORIENTED_EDGE('',*,*,#49440,.T.);
#69155=ORIENTED_EDGE('',*,*,#49446,.T.);
#69156=ORIENTED_EDGE('',*,*,#49447,.F.);
#69157=ORIENTED_EDGE('',*,*,#49448,.T.);
#69158=ORIENTED_EDGE('',*,*,#49441,.T.);
#69159=ORIENTED_EDGE('',*,*,#49449,.T.);
#69160=ORIENTED_EDGE('',*,*,#49450,.F.);
#69161=ORIENTED_EDGE('',*,*,#49451,.T.);
#69162=ORIENTED_EDGE('',*,*,#49444,.T.);
#69163=ORIENTED_EDGE('',*,*,#49452,.T.);
#69164=ORIENTED_EDGE('',*,*,#49453,.F.);
#69165=ORIENTED_EDGE('',*,*,#49454,.T.);
#69166=ORIENTED_EDGE('',*,*,#49447,.T.);
#69167=ORIENTED_EDGE('',*,*,#49455,.T.);
#69168=ORIENTED_EDGE('',*,*,#49456,.F.);
#69169=ORIENTED_EDGE('',*,*,#49457,.T.);
#69170=ORIENTED_EDGE('',*,*,#49450,.T.);
#69171=ORIENTED_EDGE('',*,*,#49458,.T.);
#69172=ORIENTED_EDGE('',*,*,#49453,.T.);
#69173=ORIENTED_EDGE('',*,*,#49459,.T.);
#69174=ORIENTED_EDGE('',*,*,#49456,.T.);
#69175=ORIENTED_EDGE('',*,*,#49460,.T.);
#69176=ORIENTED_EDGE('',*,*,#49461,.F.);
#69177=ORIENTED_EDGE('',*,*,#49462,.T.);
#69178=ORIENTED_EDGE('',*,*,#49463,.F.);
#69179=ORIENTED_EDGE('',*,*,#49464,.T.);
#69180=ORIENTED_EDGE('',*,*,#49465,.F.);
#69181=ORIENTED_EDGE('',*,*,#49466,.T.);
#69182=ORIENTED_EDGE('',*,*,#49463,.T.);
#69183=ORIENTED_EDGE('',*,*,#49467,.T.);
#69184=ORIENTED_EDGE('',*,*,#49468,.F.);
#69185=ORIENTED_EDGE('',*,*,#49469,.T.);
#69186=ORIENTED_EDGE('',*,*,#49461,.T.);
#69187=ORIENTED_EDGE('',*,*,#49470,.T.);
#69188=ORIENTED_EDGE('',*,*,#49471,.F.);
#69189=ORIENTED_EDGE('',*,*,#49472,.T.);
#69190=ORIENTED_EDGE('',*,*,#49465,.T.);
#69191=ORIENTED_EDGE('',*,*,#49473,.T.);
#69192=ORIENTED_EDGE('',*,*,#49474,.F.);
#69193=ORIENTED_EDGE('',*,*,#49475,.T.);
#69194=ORIENTED_EDGE('',*,*,#49468,.T.);
#69195=ORIENTED_EDGE('',*,*,#49476,.T.);
#69196=ORIENTED_EDGE('',*,*,#49477,.F.);
#69197=ORIENTED_EDGE('',*,*,#49478,.T.);
#69198=ORIENTED_EDGE('',*,*,#49471,.T.);
#69199=ORIENTED_EDGE('',*,*,#49479,.T.);
#69200=ORIENTED_EDGE('',*,*,#49480,.F.);
#69201=ORIENTED_EDGE('',*,*,#49481,.T.);
#69202=ORIENTED_EDGE('',*,*,#49474,.T.);
#69203=ORIENTED_EDGE('',*,*,#49482,.T.);
#69204=ORIENTED_EDGE('',*,*,#49477,.T.);
#69205=ORIENTED_EDGE('',*,*,#49483,.T.);
#69206=ORIENTED_EDGE('',*,*,#49480,.T.);
#69207=ORIENTED_EDGE('',*,*,#49484,.T.);
#69208=ORIENTED_EDGE('',*,*,#49485,.F.);
#69209=ORIENTED_EDGE('',*,*,#49486,.T.);
#69210=ORIENTED_EDGE('',*,*,#49487,.F.);
#69211=ORIENTED_EDGE('',*,*,#49488,.T.);
#69212=ORIENTED_EDGE('',*,*,#49489,.F.);
#69213=ORIENTED_EDGE('',*,*,#49490,.T.);
#69214=ORIENTED_EDGE('',*,*,#49487,.T.);
#69215=ORIENTED_EDGE('',*,*,#49491,.T.);
#69216=ORIENTED_EDGE('',*,*,#49492,.F.);
#69217=ORIENTED_EDGE('',*,*,#49493,.T.);
#69218=ORIENTED_EDGE('',*,*,#49485,.T.);
#69219=ORIENTED_EDGE('',*,*,#49494,.T.);
#69220=ORIENTED_EDGE('',*,*,#49495,.F.);
#69221=ORIENTED_EDGE('',*,*,#49496,.T.);
#69222=ORIENTED_EDGE('',*,*,#49489,.T.);
#69223=ORIENTED_EDGE('',*,*,#49497,.T.);
#69224=ORIENTED_EDGE('',*,*,#49498,.F.);
#69225=ORIENTED_EDGE('',*,*,#49499,.T.);
#69226=ORIENTED_EDGE('',*,*,#49492,.T.);
#69227=ORIENTED_EDGE('',*,*,#49500,.T.);
#69228=ORIENTED_EDGE('',*,*,#49501,.F.);
#69229=ORIENTED_EDGE('',*,*,#49502,.T.);
#69230=ORIENTED_EDGE('',*,*,#49495,.T.);
#69231=ORIENTED_EDGE('',*,*,#49503,.T.);
#69232=ORIENTED_EDGE('',*,*,#49504,.F.);
#69233=ORIENTED_EDGE('',*,*,#49505,.T.);
#69234=ORIENTED_EDGE('',*,*,#49498,.T.);
#69235=ORIENTED_EDGE('',*,*,#49506,.T.);
#69236=ORIENTED_EDGE('',*,*,#49507,.F.);
#69237=ORIENTED_EDGE('',*,*,#49508,.T.);
#69238=ORIENTED_EDGE('',*,*,#49501,.T.);
#69239=ORIENTED_EDGE('',*,*,#49509,.T.);
#69240=ORIENTED_EDGE('',*,*,#49504,.T.);
#69241=ORIENTED_EDGE('',*,*,#49510,.T.);
#69242=ORIENTED_EDGE('',*,*,#49507,.T.);
#69243=ORIENTED_EDGE('',*,*,#49511,.T.);
#69244=ORIENTED_EDGE('',*,*,#49512,.F.);
#69245=ORIENTED_EDGE('',*,*,#49513,.T.);
#69246=ORIENTED_EDGE('',*,*,#49514,.F.);
#69247=ORIENTED_EDGE('',*,*,#49515,.T.);
#69248=ORIENTED_EDGE('',*,*,#49516,.F.);
#69249=ORIENTED_EDGE('',*,*,#49517,.T.);
#69250=ORIENTED_EDGE('',*,*,#49514,.T.);
#69251=ORIENTED_EDGE('',*,*,#49518,.T.);
#69252=ORIENTED_EDGE('',*,*,#49519,.F.);
#69253=ORIENTED_EDGE('',*,*,#49520,.T.);
#69254=ORIENTED_EDGE('',*,*,#49512,.T.);
#69255=ORIENTED_EDGE('',*,*,#49521,.T.);
#69256=ORIENTED_EDGE('',*,*,#49522,.F.);
#69257=ORIENTED_EDGE('',*,*,#49523,.T.);
#69258=ORIENTED_EDGE('',*,*,#49516,.T.);
#69259=ORIENTED_EDGE('',*,*,#49524,.T.);
#69260=ORIENTED_EDGE('',*,*,#49525,.F.);
#69261=ORIENTED_EDGE('',*,*,#49526,.T.);
#69262=ORIENTED_EDGE('',*,*,#49519,.T.);
#69263=ORIENTED_EDGE('',*,*,#49527,.T.);
#69264=ORIENTED_EDGE('',*,*,#49528,.F.);
#69265=ORIENTED_EDGE('',*,*,#49529,.T.);
#69266=ORIENTED_EDGE('',*,*,#49522,.T.);
#69267=ORIENTED_EDGE('',*,*,#49530,.T.);
#69268=ORIENTED_EDGE('',*,*,#49531,.F.);
#69269=ORIENTED_EDGE('',*,*,#49532,.T.);
#69270=ORIENTED_EDGE('',*,*,#49525,.T.);
#69271=ORIENTED_EDGE('',*,*,#49533,.T.);
#69272=ORIENTED_EDGE('',*,*,#49528,.T.);
#69273=ORIENTED_EDGE('',*,*,#49534,.T.);
#69274=ORIENTED_EDGE('',*,*,#49531,.T.);
#69275=ORIENTED_EDGE('',*,*,#49535,.T.);
#69276=ORIENTED_EDGE('',*,*,#49536,.F.);
#69277=ORIENTED_EDGE('',*,*,#49537,.T.);
#69278=ORIENTED_EDGE('',*,*,#49538,.F.);
#69279=ORIENTED_EDGE('',*,*,#49539,.T.);
#69280=ORIENTED_EDGE('',*,*,#49540,.F.);
#69281=ORIENTED_EDGE('',*,*,#49541,.T.);
#69282=ORIENTED_EDGE('',*,*,#49538,.T.);
#69283=ORIENTED_EDGE('',*,*,#49542,.T.);
#69284=ORIENTED_EDGE('',*,*,#49543,.F.);
#69285=ORIENTED_EDGE('',*,*,#49544,.T.);
#69286=ORIENTED_EDGE('',*,*,#49536,.T.);
#69287=ORIENTED_EDGE('',*,*,#49545,.T.);
#69288=ORIENTED_EDGE('',*,*,#49546,.F.);
#69289=ORIENTED_EDGE('',*,*,#49547,.T.);
#69290=ORIENTED_EDGE('',*,*,#49540,.T.);
#69291=ORIENTED_EDGE('',*,*,#49548,.T.);
#69292=ORIENTED_EDGE('',*,*,#49549,.F.);
#69293=ORIENTED_EDGE('',*,*,#49550,.T.);
#69294=ORIENTED_EDGE('',*,*,#49543,.T.);
#69295=ORIENTED_EDGE('',*,*,#49551,.T.);
#69296=ORIENTED_EDGE('',*,*,#49552,.F.);
#69297=ORIENTED_EDGE('',*,*,#49553,.T.);
#69298=ORIENTED_EDGE('',*,*,#49546,.T.);
#69299=ORIENTED_EDGE('',*,*,#49554,.T.);
#69300=ORIENTED_EDGE('',*,*,#49555,.F.);
#69301=ORIENTED_EDGE('',*,*,#49556,.T.);
#69302=ORIENTED_EDGE('',*,*,#49549,.T.);
#69303=ORIENTED_EDGE('',*,*,#49557,.T.);
#69304=ORIENTED_EDGE('',*,*,#49552,.T.);
#69305=ORIENTED_EDGE('',*,*,#49558,.T.);
#69306=ORIENTED_EDGE('',*,*,#49555,.T.);
#69307=ORIENTED_EDGE('',*,*,#49559,.T.);
#69308=ORIENTED_EDGE('',*,*,#49560,.F.);
#69309=ORIENTED_EDGE('',*,*,#49561,.T.);
#69310=ORIENTED_EDGE('',*,*,#49562,.F.);
#69311=ORIENTED_EDGE('',*,*,#49563,.T.);
#69312=ORIENTED_EDGE('',*,*,#49564,.F.);
#69313=ORIENTED_EDGE('',*,*,#49565,.T.);
#69314=ORIENTED_EDGE('',*,*,#49562,.T.);
#69315=ORIENTED_EDGE('',*,*,#49566,.T.);
#69316=ORIENTED_EDGE('',*,*,#49567,.F.);
#69317=ORIENTED_EDGE('',*,*,#49568,.T.);
#69318=ORIENTED_EDGE('',*,*,#49560,.T.);
#69319=ORIENTED_EDGE('',*,*,#49569,.T.);
#69320=ORIENTED_EDGE('',*,*,#49570,.F.);
#69321=ORIENTED_EDGE('',*,*,#49571,.T.);
#69322=ORIENTED_EDGE('',*,*,#49564,.T.);
#69323=ORIENTED_EDGE('',*,*,#49572,.T.);
#69324=ORIENTED_EDGE('',*,*,#49573,.F.);
#69325=ORIENTED_EDGE('',*,*,#49574,.T.);
#69326=ORIENTED_EDGE('',*,*,#49567,.T.);
#69327=ORIENTED_EDGE('',*,*,#49575,.T.);
#69328=ORIENTED_EDGE('',*,*,#49576,.F.);
#69329=ORIENTED_EDGE('',*,*,#49577,.T.);
#69330=ORIENTED_EDGE('',*,*,#49570,.T.);
#69331=ORIENTED_EDGE('',*,*,#49578,.T.);
#69332=ORIENTED_EDGE('',*,*,#49579,.F.);
#69333=ORIENTED_EDGE('',*,*,#49580,.T.);
#69334=ORIENTED_EDGE('',*,*,#49573,.T.);
#69335=ORIENTED_EDGE('',*,*,#49581,.T.);
#69336=ORIENTED_EDGE('',*,*,#49576,.T.);
#69337=ORIENTED_EDGE('',*,*,#49582,.T.);
#69338=ORIENTED_EDGE('',*,*,#49579,.T.);
#69339=ORIENTED_EDGE('',*,*,#49583,.T.);
#69340=ORIENTED_EDGE('',*,*,#49584,.F.);
#69341=ORIENTED_EDGE('',*,*,#49585,.T.);
#69342=ORIENTED_EDGE('',*,*,#49586,.F.);
#69343=ORIENTED_EDGE('',*,*,#49587,.T.);
#69344=ORIENTED_EDGE('',*,*,#49588,.F.);
#69345=ORIENTED_EDGE('',*,*,#49589,.T.);
#69346=ORIENTED_EDGE('',*,*,#49586,.T.);
#69347=ORIENTED_EDGE('',*,*,#49590,.T.);
#69348=ORIENTED_EDGE('',*,*,#49591,.F.);
#69349=ORIENTED_EDGE('',*,*,#49592,.T.);
#69350=ORIENTED_EDGE('',*,*,#49584,.T.);
#69351=ORIENTED_EDGE('',*,*,#49593,.T.);
#69352=ORIENTED_EDGE('',*,*,#49594,.F.);
#69353=ORIENTED_EDGE('',*,*,#49595,.T.);
#69354=ORIENTED_EDGE('',*,*,#49588,.T.);
#69355=ORIENTED_EDGE('',*,*,#49596,.T.);
#69356=ORIENTED_EDGE('',*,*,#49597,.F.);
#69357=ORIENTED_EDGE('',*,*,#49598,.T.);
#69358=ORIENTED_EDGE('',*,*,#49591,.T.);
#69359=ORIENTED_EDGE('',*,*,#49599,.T.);
#69360=ORIENTED_EDGE('',*,*,#49600,.F.);
#69361=ORIENTED_EDGE('',*,*,#49601,.T.);
#69362=ORIENTED_EDGE('',*,*,#49594,.T.);
#69363=ORIENTED_EDGE('',*,*,#49602,.T.);
#69364=ORIENTED_EDGE('',*,*,#49603,.F.);
#69365=ORIENTED_EDGE('',*,*,#49604,.T.);
#69366=ORIENTED_EDGE('',*,*,#49597,.T.);
#69367=ORIENTED_EDGE('',*,*,#49605,.T.);
#69368=ORIENTED_EDGE('',*,*,#49600,.T.);
#69369=ORIENTED_EDGE('',*,*,#49606,.T.);
#69370=ORIENTED_EDGE('',*,*,#49603,.T.);
#69371=ORIENTED_EDGE('',*,*,#49607,.T.);
#69372=ORIENTED_EDGE('',*,*,#49608,.F.);
#69373=ORIENTED_EDGE('',*,*,#49609,.T.);
#69374=ORIENTED_EDGE('',*,*,#49610,.F.);
#69375=ORIENTED_EDGE('',*,*,#49611,.T.);
#69376=ORIENTED_EDGE('',*,*,#49612,.F.);
#69377=ORIENTED_EDGE('',*,*,#49613,.T.);
#69378=ORIENTED_EDGE('',*,*,#49610,.T.);
#69379=ORIENTED_EDGE('',*,*,#49614,.T.);
#69380=ORIENTED_EDGE('',*,*,#49615,.F.);
#69381=ORIENTED_EDGE('',*,*,#49616,.T.);
#69382=ORIENTED_EDGE('',*,*,#49608,.T.);
#69383=ORIENTED_EDGE('',*,*,#49617,.T.);
#69384=ORIENTED_EDGE('',*,*,#49618,.F.);
#69385=ORIENTED_EDGE('',*,*,#49619,.T.);
#69386=ORIENTED_EDGE('',*,*,#49612,.T.);
#69387=ORIENTED_EDGE('',*,*,#49620,.T.);
#69388=ORIENTED_EDGE('',*,*,#49621,.F.);
#69389=ORIENTED_EDGE('',*,*,#49622,.T.);
#69390=ORIENTED_EDGE('',*,*,#49615,.T.);
#69391=ORIENTED_EDGE('',*,*,#49623,.T.);
#69392=ORIENTED_EDGE('',*,*,#49624,.F.);
#69393=ORIENTED_EDGE('',*,*,#49625,.T.);
#69394=ORIENTED_EDGE('',*,*,#49618,.T.);
#69395=ORIENTED_EDGE('',*,*,#49626,.T.);
#69396=ORIENTED_EDGE('',*,*,#49627,.F.);
#69397=ORIENTED_EDGE('',*,*,#49628,.T.);
#69398=ORIENTED_EDGE('',*,*,#49621,.T.);
#69399=ORIENTED_EDGE('',*,*,#49629,.T.);
#69400=ORIENTED_EDGE('',*,*,#49624,.T.);
#69401=ORIENTED_EDGE('',*,*,#49630,.T.);
#69402=ORIENTED_EDGE('',*,*,#49627,.T.);
#69403=ORIENTED_EDGE('',*,*,#49631,.T.);
#69404=ORIENTED_EDGE('',*,*,#49632,.F.);
#69405=ORIENTED_EDGE('',*,*,#49633,.T.);
#69406=ORIENTED_EDGE('',*,*,#49634,.F.);
#69407=ORIENTED_EDGE('',*,*,#49635,.T.);
#69408=ORIENTED_EDGE('',*,*,#49636,.F.);
#69409=ORIENTED_EDGE('',*,*,#49637,.T.);
#69410=ORIENTED_EDGE('',*,*,#49634,.T.);
#69411=ORIENTED_EDGE('',*,*,#49638,.T.);
#69412=ORIENTED_EDGE('',*,*,#49639,.F.);
#69413=ORIENTED_EDGE('',*,*,#49640,.T.);
#69414=ORIENTED_EDGE('',*,*,#49632,.T.);
#69415=ORIENTED_EDGE('',*,*,#49641,.T.);
#69416=ORIENTED_EDGE('',*,*,#49642,.F.);
#69417=ORIENTED_EDGE('',*,*,#49643,.T.);
#69418=ORIENTED_EDGE('',*,*,#49636,.T.);
#69419=ORIENTED_EDGE('',*,*,#49644,.T.);
#69420=ORIENTED_EDGE('',*,*,#49645,.F.);
#69421=ORIENTED_EDGE('',*,*,#49646,.T.);
#69422=ORIENTED_EDGE('',*,*,#49639,.T.);
#69423=ORIENTED_EDGE('',*,*,#49647,.T.);
#69424=ORIENTED_EDGE('',*,*,#49648,.F.);
#69425=ORIENTED_EDGE('',*,*,#49649,.T.);
#69426=ORIENTED_EDGE('',*,*,#49642,.T.);
#69427=ORIENTED_EDGE('',*,*,#49650,.T.);
#69428=ORIENTED_EDGE('',*,*,#49651,.F.);
#69429=ORIENTED_EDGE('',*,*,#49652,.T.);
#69430=ORIENTED_EDGE('',*,*,#49645,.T.);
#69431=ORIENTED_EDGE('',*,*,#49653,.T.);
#69432=ORIENTED_EDGE('',*,*,#49654,.F.);
#69433=ORIENTED_EDGE('',*,*,#49655,.T.);
#69434=ORIENTED_EDGE('',*,*,#49648,.T.);
#69435=ORIENTED_EDGE('',*,*,#49656,.T.);
#69436=ORIENTED_EDGE('',*,*,#49657,.F.);
#69437=ORIENTED_EDGE('',*,*,#49658,.T.);
#69438=ORIENTED_EDGE('',*,*,#49651,.T.);
#69439=ORIENTED_EDGE('',*,*,#49659,.T.);
#69440=ORIENTED_EDGE('',*,*,#49654,.T.);
#69441=ORIENTED_EDGE('',*,*,#49660,.T.);
#69442=ORIENTED_EDGE('',*,*,#49657,.T.);
#69443=ORIENTED_EDGE('',*,*,#49661,.T.);
#69444=ORIENTED_EDGE('',*,*,#49662,.F.);
#69445=ORIENTED_EDGE('',*,*,#49663,.T.);
#69446=ORIENTED_EDGE('',*,*,#49664,.F.);
#69447=ORIENTED_EDGE('',*,*,#49665,.T.);
#69448=ORIENTED_EDGE('',*,*,#49666,.F.);
#69449=ORIENTED_EDGE('',*,*,#49667,.T.);
#69450=ORIENTED_EDGE('',*,*,#49664,.T.);
#69451=ORIENTED_EDGE('',*,*,#49668,.T.);
#69452=ORIENTED_EDGE('',*,*,#49669,.F.);
#69453=ORIENTED_EDGE('',*,*,#49670,.T.);
#69454=ORIENTED_EDGE('',*,*,#49662,.T.);
#69455=ORIENTED_EDGE('',*,*,#49671,.T.);
#69456=ORIENTED_EDGE('',*,*,#49672,.F.);
#69457=ORIENTED_EDGE('',*,*,#49673,.T.);
#69458=ORIENTED_EDGE('',*,*,#49666,.T.);
#69459=ORIENTED_EDGE('',*,*,#49674,.T.);
#69460=ORIENTED_EDGE('',*,*,#49675,.F.);
#69461=ORIENTED_EDGE('',*,*,#49676,.T.);
#69462=ORIENTED_EDGE('',*,*,#49669,.T.);
#69463=ORIENTED_EDGE('',*,*,#49677,.T.);
#69464=ORIENTED_EDGE('',*,*,#49678,.F.);
#69465=ORIENTED_EDGE('',*,*,#49679,.T.);
#69466=ORIENTED_EDGE('',*,*,#49672,.T.);
#69467=ORIENTED_EDGE('',*,*,#49680,.T.);
#69468=ORIENTED_EDGE('',*,*,#49681,.F.);
#69469=ORIENTED_EDGE('',*,*,#49682,.T.);
#69470=ORIENTED_EDGE('',*,*,#49675,.T.);
#69471=ORIENTED_EDGE('',*,*,#49683,.T.);
#69472=ORIENTED_EDGE('',*,*,#49678,.T.);
#69473=ORIENTED_EDGE('',*,*,#49684,.T.);
#69474=ORIENTED_EDGE('',*,*,#49681,.T.);
#69475=ORIENTED_EDGE('',*,*,#49685,.T.);
#69476=ORIENTED_EDGE('',*,*,#49686,.F.);
#69477=ORIENTED_EDGE('',*,*,#49687,.T.);
#69478=ORIENTED_EDGE('',*,*,#49688,.F.);
#69479=ORIENTED_EDGE('',*,*,#49689,.T.);
#69480=ORIENTED_EDGE('',*,*,#49690,.F.);
#69481=ORIENTED_EDGE('',*,*,#49691,.T.);
#69482=ORIENTED_EDGE('',*,*,#49688,.T.);
#69483=ORIENTED_EDGE('',*,*,#49692,.T.);
#69484=ORIENTED_EDGE('',*,*,#49693,.F.);
#69485=ORIENTED_EDGE('',*,*,#49694,.T.);
#69486=ORIENTED_EDGE('',*,*,#49686,.T.);
#69487=ORIENTED_EDGE('',*,*,#49695,.T.);
#69488=ORIENTED_EDGE('',*,*,#49696,.F.);
#69489=ORIENTED_EDGE('',*,*,#49697,.T.);
#69490=ORIENTED_EDGE('',*,*,#49690,.T.);
#69491=ORIENTED_EDGE('',*,*,#49698,.T.);
#69492=ORIENTED_EDGE('',*,*,#49699,.F.);
#69493=ORIENTED_EDGE('',*,*,#49700,.T.);
#69494=ORIENTED_EDGE('',*,*,#49693,.T.);
#69495=ORIENTED_EDGE('',*,*,#49701,.T.);
#69496=ORIENTED_EDGE('',*,*,#49702,.F.);
#69497=ORIENTED_EDGE('',*,*,#49703,.T.);
#69498=ORIENTED_EDGE('',*,*,#49696,.T.);
#69499=ORIENTED_EDGE('',*,*,#49704,.T.);
#69500=ORIENTED_EDGE('',*,*,#49705,.F.);
#69501=ORIENTED_EDGE('',*,*,#49706,.T.);
#69502=ORIENTED_EDGE('',*,*,#49699,.T.);
#69503=ORIENTED_EDGE('',*,*,#49707,.T.);
#69504=ORIENTED_EDGE('',*,*,#49702,.T.);
#69505=ORIENTED_EDGE('',*,*,#49708,.T.);
#69506=ORIENTED_EDGE('',*,*,#49705,.T.);
#69507=ORIENTED_EDGE('',*,*,#49709,.T.);
#69508=ORIENTED_EDGE('',*,*,#49710,.F.);
#69509=ORIENTED_EDGE('',*,*,#49711,.T.);
#69510=ORIENTED_EDGE('',*,*,#49712,.F.);
#69511=ORIENTED_EDGE('',*,*,#49713,.T.);
#69512=ORIENTED_EDGE('',*,*,#49714,.F.);
#69513=ORIENTED_EDGE('',*,*,#49715,.T.);
#69514=ORIENTED_EDGE('',*,*,#49712,.T.);
#69515=ORIENTED_EDGE('',*,*,#49716,.T.);
#69516=ORIENTED_EDGE('',*,*,#49717,.F.);
#69517=ORIENTED_EDGE('',*,*,#49718,.T.);
#69518=ORIENTED_EDGE('',*,*,#49710,.T.);
#69519=ORIENTED_EDGE('',*,*,#49719,.T.);
#69520=ORIENTED_EDGE('',*,*,#49720,.F.);
#69521=ORIENTED_EDGE('',*,*,#49721,.T.);
#69522=ORIENTED_EDGE('',*,*,#49714,.T.);
#69523=ORIENTED_EDGE('',*,*,#49722,.T.);
#69524=ORIENTED_EDGE('',*,*,#49723,.F.);
#69525=ORIENTED_EDGE('',*,*,#49724,.T.);
#69526=ORIENTED_EDGE('',*,*,#49717,.T.);
#69527=ORIENTED_EDGE('',*,*,#49725,.T.);
#69528=ORIENTED_EDGE('',*,*,#49726,.F.);
#69529=ORIENTED_EDGE('',*,*,#49727,.T.);
#69530=ORIENTED_EDGE('',*,*,#49720,.T.);
#69531=ORIENTED_EDGE('',*,*,#49728,.T.);
#69532=ORIENTED_EDGE('',*,*,#49729,.F.);
#69533=ORIENTED_EDGE('',*,*,#49730,.T.);
#69534=ORIENTED_EDGE('',*,*,#49723,.T.);
#69535=ORIENTED_EDGE('',*,*,#49731,.T.);
#69536=ORIENTED_EDGE('',*,*,#49732,.F.);
#69537=ORIENTED_EDGE('',*,*,#49733,.T.);
#69538=ORIENTED_EDGE('',*,*,#49726,.T.);
#69539=ORIENTED_EDGE('',*,*,#49734,.T.);
#69540=ORIENTED_EDGE('',*,*,#49735,.F.);
#69541=ORIENTED_EDGE('',*,*,#49736,.T.);
#69542=ORIENTED_EDGE('',*,*,#49729,.T.);
#69543=ORIENTED_EDGE('',*,*,#49737,.T.);
#69544=ORIENTED_EDGE('',*,*,#49732,.T.);
#69545=ORIENTED_EDGE('',*,*,#49738,.T.);
#69546=ORIENTED_EDGE('',*,*,#49735,.T.);
#69547=ORIENTED_EDGE('',*,*,#49739,.T.);
#69548=ORIENTED_EDGE('',*,*,#49740,.F.);
#69549=ORIENTED_EDGE('',*,*,#49741,.T.);
#69550=ORIENTED_EDGE('',*,*,#49742,.F.);
#69551=ORIENTED_EDGE('',*,*,#49743,.T.);
#69552=ORIENTED_EDGE('',*,*,#49744,.F.);
#69553=ORIENTED_EDGE('',*,*,#49745,.T.);
#69554=ORIENTED_EDGE('',*,*,#49742,.T.);
#69555=ORIENTED_EDGE('',*,*,#49746,.T.);
#69556=ORIENTED_EDGE('',*,*,#49747,.F.);
#69557=ORIENTED_EDGE('',*,*,#49748,.T.);
#69558=ORIENTED_EDGE('',*,*,#49740,.T.);
#69559=ORIENTED_EDGE('',*,*,#49749,.T.);
#69560=ORIENTED_EDGE('',*,*,#49750,.F.);
#69561=ORIENTED_EDGE('',*,*,#49751,.T.);
#69562=ORIENTED_EDGE('',*,*,#49744,.T.);
#69563=ORIENTED_EDGE('',*,*,#49752,.T.);
#69564=ORIENTED_EDGE('',*,*,#49753,.F.);
#69565=ORIENTED_EDGE('',*,*,#49754,.T.);
#69566=ORIENTED_EDGE('',*,*,#49747,.T.);
#69567=ORIENTED_EDGE('',*,*,#49755,.T.);
#69568=ORIENTED_EDGE('',*,*,#49756,.F.);
#69569=ORIENTED_EDGE('',*,*,#49757,.T.);
#69570=ORIENTED_EDGE('',*,*,#49750,.T.);
#69571=ORIENTED_EDGE('',*,*,#49758,.T.);
#69572=ORIENTED_EDGE('',*,*,#49759,.F.);
#69573=ORIENTED_EDGE('',*,*,#49760,.T.);
#69574=ORIENTED_EDGE('',*,*,#49753,.T.);
#69575=ORIENTED_EDGE('',*,*,#49761,.T.);
#69576=ORIENTED_EDGE('',*,*,#49762,.F.);
#69577=ORIENTED_EDGE('',*,*,#49763,.T.);
#69578=ORIENTED_EDGE('',*,*,#49756,.T.);
#69579=ORIENTED_EDGE('',*,*,#49764,.T.);
#69580=ORIENTED_EDGE('',*,*,#49765,.F.);
#69581=ORIENTED_EDGE('',*,*,#49766,.T.);
#69582=ORIENTED_EDGE('',*,*,#49759,.T.);
#69583=ORIENTED_EDGE('',*,*,#49767,.T.);
#69584=ORIENTED_EDGE('',*,*,#49762,.T.);
#69585=ORIENTED_EDGE('',*,*,#49768,.T.);
#69586=ORIENTED_EDGE('',*,*,#49765,.T.);
#69587=ORIENTED_EDGE('',*,*,#49769,.T.);
#69588=ORIENTED_EDGE('',*,*,#49770,.F.);
#69589=ORIENTED_EDGE('',*,*,#49771,.T.);
#69590=ORIENTED_EDGE('',*,*,#49772,.F.);
#69591=ORIENTED_EDGE('',*,*,#49773,.T.);
#69592=ORIENTED_EDGE('',*,*,#49774,.F.);
#69593=ORIENTED_EDGE('',*,*,#49775,.T.);
#69594=ORIENTED_EDGE('',*,*,#49772,.T.);
#69595=ORIENTED_EDGE('',*,*,#49776,.T.);
#69596=ORIENTED_EDGE('',*,*,#49777,.F.);
#69597=ORIENTED_EDGE('',*,*,#49778,.T.);
#69598=ORIENTED_EDGE('',*,*,#49770,.T.);
#69599=ORIENTED_EDGE('',*,*,#49779,.T.);
#69600=ORIENTED_EDGE('',*,*,#49780,.F.);
#69601=ORIENTED_EDGE('',*,*,#49781,.T.);
#69602=ORIENTED_EDGE('',*,*,#49774,.T.);
#69603=ORIENTED_EDGE('',*,*,#49782,.T.);
#69604=ORIENTED_EDGE('',*,*,#49783,.F.);
#69605=ORIENTED_EDGE('',*,*,#49784,.T.);
#69606=ORIENTED_EDGE('',*,*,#49777,.T.);
#69607=ORIENTED_EDGE('',*,*,#49785,.T.);
#69608=ORIENTED_EDGE('',*,*,#49786,.F.);
#69609=ORIENTED_EDGE('',*,*,#49787,.T.);
#69610=ORIENTED_EDGE('',*,*,#49780,.T.);
#69611=ORIENTED_EDGE('',*,*,#49788,.T.);
#69612=ORIENTED_EDGE('',*,*,#49789,.F.);
#69613=ORIENTED_EDGE('',*,*,#49790,.T.);
#69614=ORIENTED_EDGE('',*,*,#49783,.T.);
#69615=ORIENTED_EDGE('',*,*,#49791,.T.);
#69616=ORIENTED_EDGE('',*,*,#49786,.T.);
#69617=ORIENTED_EDGE('',*,*,#49792,.T.);
#69618=ORIENTED_EDGE('',*,*,#49789,.T.);
#69619=ORIENTED_EDGE('',*,*,#49793,.T.);
#69620=ORIENTED_EDGE('',*,*,#49794,.F.);
#69621=ORIENTED_EDGE('',*,*,#49795,.T.);
#69622=ORIENTED_EDGE('',*,*,#49796,.F.);
#69623=ORIENTED_EDGE('',*,*,#49797,.T.);
#69624=ORIENTED_EDGE('',*,*,#49798,.F.);
#69625=ORIENTED_EDGE('',*,*,#49799,.T.);
#69626=ORIENTED_EDGE('',*,*,#49796,.T.);
#69627=ORIENTED_EDGE('',*,*,#49800,.T.);
#69628=ORIENTED_EDGE('',*,*,#49801,.F.);
#69629=ORIENTED_EDGE('',*,*,#49802,.T.);
#69630=ORIENTED_EDGE('',*,*,#49794,.T.);
#69631=ORIENTED_EDGE('',*,*,#49803,.T.);
#69632=ORIENTED_EDGE('',*,*,#49804,.F.);
#69633=ORIENTED_EDGE('',*,*,#49805,.T.);
#69634=ORIENTED_EDGE('',*,*,#49798,.T.);
#69635=ORIENTED_EDGE('',*,*,#49806,.T.);
#69636=ORIENTED_EDGE('',*,*,#49807,.F.);
#69637=ORIENTED_EDGE('',*,*,#49808,.T.);
#69638=ORIENTED_EDGE('',*,*,#49801,.T.);
#69639=ORIENTED_EDGE('',*,*,#49809,.T.);
#69640=ORIENTED_EDGE('',*,*,#49810,.F.);
#69641=ORIENTED_EDGE('',*,*,#49811,.T.);
#69642=ORIENTED_EDGE('',*,*,#49804,.T.);
#69643=ORIENTED_EDGE('',*,*,#49812,.T.);
#69644=ORIENTED_EDGE('',*,*,#49813,.F.);
#69645=ORIENTED_EDGE('',*,*,#49814,.T.);
#69646=ORIENTED_EDGE('',*,*,#49807,.T.);
#69647=ORIENTED_EDGE('',*,*,#49815,.T.);
#69648=ORIENTED_EDGE('',*,*,#49810,.T.);
#69649=ORIENTED_EDGE('',*,*,#49816,.T.);
#69650=ORIENTED_EDGE('',*,*,#49813,.T.);
#69651=ORIENTED_EDGE('',*,*,#49817,.T.);
#69652=ORIENTED_EDGE('',*,*,#49818,.F.);
#69653=ORIENTED_EDGE('',*,*,#49819,.T.);
#69654=ORIENTED_EDGE('',*,*,#49820,.F.);
#69655=ORIENTED_EDGE('',*,*,#49821,.T.);
#69656=ORIENTED_EDGE('',*,*,#49822,.F.);
#69657=ORIENTED_EDGE('',*,*,#49823,.T.);
#69658=ORIENTED_EDGE('',*,*,#49820,.T.);
#69659=ORIENTED_EDGE('',*,*,#49824,.T.);
#69660=ORIENTED_EDGE('',*,*,#49825,.F.);
#69661=ORIENTED_EDGE('',*,*,#49826,.T.);
#69662=ORIENTED_EDGE('',*,*,#49818,.T.);
#69663=ORIENTED_EDGE('',*,*,#49827,.T.);
#69664=ORIENTED_EDGE('',*,*,#49828,.F.);
#69665=ORIENTED_EDGE('',*,*,#49829,.T.);
#69666=ORIENTED_EDGE('',*,*,#49822,.T.);
#69667=ORIENTED_EDGE('',*,*,#49830,.T.);
#69668=ORIENTED_EDGE('',*,*,#49831,.F.);
#69669=ORIENTED_EDGE('',*,*,#49832,.T.);
#69670=ORIENTED_EDGE('',*,*,#49825,.T.);
#69671=ORIENTED_EDGE('',*,*,#49833,.T.);
#69672=ORIENTED_EDGE('',*,*,#49834,.F.);
#69673=ORIENTED_EDGE('',*,*,#49835,.T.);
#69674=ORIENTED_EDGE('',*,*,#49828,.T.);
#69675=ORIENTED_EDGE('',*,*,#49836,.T.);
#69676=ORIENTED_EDGE('',*,*,#49837,.F.);
#69677=ORIENTED_EDGE('',*,*,#49838,.T.);
#69678=ORIENTED_EDGE('',*,*,#49831,.T.);
#69679=ORIENTED_EDGE('',*,*,#49839,.T.);
#69680=ORIENTED_EDGE('',*,*,#49834,.T.);
#69681=ORIENTED_EDGE('',*,*,#49840,.T.);
#69682=ORIENTED_EDGE('',*,*,#49837,.T.);
#69683=ORIENTED_EDGE('',*,*,#49841,.T.);
#69684=ORIENTED_EDGE('',*,*,#49842,.F.);
#69685=ORIENTED_EDGE('',*,*,#49843,.T.);
#69686=ORIENTED_EDGE('',*,*,#49844,.F.);
#69687=ORIENTED_EDGE('',*,*,#49845,.T.);
#69688=ORIENTED_EDGE('',*,*,#49846,.F.);
#69689=ORIENTED_EDGE('',*,*,#49847,.T.);
#69690=ORIENTED_EDGE('',*,*,#49844,.T.);
#69691=ORIENTED_EDGE('',*,*,#49848,.T.);
#69692=ORIENTED_EDGE('',*,*,#49849,.F.);
#69693=ORIENTED_EDGE('',*,*,#49850,.T.);
#69694=ORIENTED_EDGE('',*,*,#49842,.T.);
#69695=ORIENTED_EDGE('',*,*,#49851,.T.);
#69696=ORIENTED_EDGE('',*,*,#49852,.F.);
#69697=ORIENTED_EDGE('',*,*,#49853,.T.);
#69698=ORIENTED_EDGE('',*,*,#49846,.T.);
#69699=ORIENTED_EDGE('',*,*,#49854,.T.);
#69700=ORIENTED_EDGE('',*,*,#49855,.F.);
#69701=ORIENTED_EDGE('',*,*,#49856,.T.);
#69702=ORIENTED_EDGE('',*,*,#49849,.T.);
#69703=ORIENTED_EDGE('',*,*,#49857,.T.);
#69704=ORIENTED_EDGE('',*,*,#49858,.F.);
#69705=ORIENTED_EDGE('',*,*,#49859,.T.);
#69706=ORIENTED_EDGE('',*,*,#49852,.T.);
#69707=ORIENTED_EDGE('',*,*,#49860,.T.);
#69708=ORIENTED_EDGE('',*,*,#49861,.F.);
#69709=ORIENTED_EDGE('',*,*,#49862,.T.);
#69710=ORIENTED_EDGE('',*,*,#49855,.T.);
#69711=ORIENTED_EDGE('',*,*,#49863,.T.);
#69712=ORIENTED_EDGE('',*,*,#49858,.T.);
#69713=ORIENTED_EDGE('',*,*,#49864,.T.);
#69714=ORIENTED_EDGE('',*,*,#49861,.T.);
#69715=ORIENTED_EDGE('',*,*,#49865,.T.);
#69716=ORIENTED_EDGE('',*,*,#49866,.F.);
#69717=ORIENTED_EDGE('',*,*,#49867,.T.);
#69718=ORIENTED_EDGE('',*,*,#49868,.F.);
#69719=ORIENTED_EDGE('',*,*,#49869,.T.);
#69720=ORIENTED_EDGE('',*,*,#49870,.F.);
#69721=ORIENTED_EDGE('',*,*,#49871,.T.);
#69722=ORIENTED_EDGE('',*,*,#49868,.T.);
#69723=ORIENTED_EDGE('',*,*,#49872,.T.);
#69724=ORIENTED_EDGE('',*,*,#49873,.F.);
#69725=ORIENTED_EDGE('',*,*,#49874,.T.);
#69726=ORIENTED_EDGE('',*,*,#49866,.T.);
#69727=ORIENTED_EDGE('',*,*,#49875,.T.);
#69728=ORIENTED_EDGE('',*,*,#49876,.F.);
#69729=ORIENTED_EDGE('',*,*,#49877,.T.);
#69730=ORIENTED_EDGE('',*,*,#49870,.T.);
#69731=ORIENTED_EDGE('',*,*,#49878,.T.);
#69732=ORIENTED_EDGE('',*,*,#49879,.F.);
#69733=ORIENTED_EDGE('',*,*,#49880,.T.);
#69734=ORIENTED_EDGE('',*,*,#49873,.T.);
#69735=ORIENTED_EDGE('',*,*,#49881,.T.);
#69736=ORIENTED_EDGE('',*,*,#49882,.F.);
#69737=ORIENTED_EDGE('',*,*,#49883,.T.);
#69738=ORIENTED_EDGE('',*,*,#49876,.T.);
#69739=ORIENTED_EDGE('',*,*,#49884,.T.);
#69740=ORIENTED_EDGE('',*,*,#49885,.F.);
#69741=ORIENTED_EDGE('',*,*,#49886,.T.);
#69742=ORIENTED_EDGE('',*,*,#49879,.T.);
#69743=ORIENTED_EDGE('',*,*,#49887,.T.);
#69744=ORIENTED_EDGE('',*,*,#49888,.T.);
#69745=ORIENTED_EDGE('',*,*,#49889,.F.);
#69746=ORIENTED_EDGE('',*,*,#49890,.T.);
#69747=ORIENTED_EDGE('',*,*,#49882,.T.);
#69748=ORIENTED_EDGE('',*,*,#49885,.T.);
#69749=ORIENTED_EDGE('',*,*,#49891,.T.);
#69750=ORIENTED_EDGE('',*,*,#49889,.T.);
#69751=ORIENTED_EDGE('',*,*,#49892,.T.);
#69752=ORIENTED_EDGE('',*,*,#49893,.F.);
#69753=ORIENTED_EDGE('',*,*,#49894,.T.);
#69754=ORIENTED_EDGE('',*,*,#49895,.F.);
#69755=ORIENTED_EDGE('',*,*,#49896,.T.);
#69756=ORIENTED_EDGE('',*,*,#49897,.F.);
#69757=ORIENTED_EDGE('',*,*,#49898,.T.);
#69758=ORIENTED_EDGE('',*,*,#49895,.T.);
#69759=ORIENTED_EDGE('',*,*,#49899,.T.);
#69760=ORIENTED_EDGE('',*,*,#49900,.F.);
#69761=ORIENTED_EDGE('',*,*,#49901,.T.);
#69762=ORIENTED_EDGE('',*,*,#49893,.T.);
#69763=ORIENTED_EDGE('',*,*,#49902,.T.);
#69764=ORIENTED_EDGE('',*,*,#49903,.F.);
#69765=ORIENTED_EDGE('',*,*,#49904,.T.);
#69766=ORIENTED_EDGE('',*,*,#49897,.T.);
#69767=ORIENTED_EDGE('',*,*,#49905,.T.);
#69768=ORIENTED_EDGE('',*,*,#49906,.F.);
#69769=ORIENTED_EDGE('',*,*,#49907,.T.);
#69770=ORIENTED_EDGE('',*,*,#49900,.T.);
#69771=ORIENTED_EDGE('',*,*,#49908,.T.);
#69772=ORIENTED_EDGE('',*,*,#49909,.F.);
#69773=ORIENTED_EDGE('',*,*,#49910,.T.);
#69774=ORIENTED_EDGE('',*,*,#49903,.T.);
#69775=ORIENTED_EDGE('',*,*,#49911,.T.);
#69776=ORIENTED_EDGE('',*,*,#49912,.F.);
#69777=ORIENTED_EDGE('',*,*,#49913,.T.);
#69778=ORIENTED_EDGE('',*,*,#49906,.T.);
#69779=ORIENTED_EDGE('',*,*,#49914,.T.);
#69780=ORIENTED_EDGE('',*,*,#49909,.T.);
#69781=ORIENTED_EDGE('',*,*,#49915,.T.);
#69782=ORIENTED_EDGE('',*,*,#49912,.T.);
#69783=ORIENTED_EDGE('',*,*,#49916,.T.);
#69784=ORIENTED_EDGE('',*,*,#49917,.F.);
#69785=ORIENTED_EDGE('',*,*,#49918,.T.);
#69786=ORIENTED_EDGE('',*,*,#49919,.F.);
#69787=ORIENTED_EDGE('',*,*,#49920,.T.);
#69788=ORIENTED_EDGE('',*,*,#49921,.F.);
#69789=ORIENTED_EDGE('',*,*,#49922,.T.);
#69790=ORIENTED_EDGE('',*,*,#49919,.T.);
#69791=ORIENTED_EDGE('',*,*,#49923,.T.);
#69792=ORIENTED_EDGE('',*,*,#49924,.F.);
#69793=ORIENTED_EDGE('',*,*,#49925,.T.);
#69794=ORIENTED_EDGE('',*,*,#49917,.T.);
#69795=ORIENTED_EDGE('',*,*,#49926,.T.);
#69796=ORIENTED_EDGE('',*,*,#49927,.F.);
#69797=ORIENTED_EDGE('',*,*,#49928,.T.);
#69798=ORIENTED_EDGE('',*,*,#49921,.T.);
#69799=ORIENTED_EDGE('',*,*,#49929,.T.);
#69800=ORIENTED_EDGE('',*,*,#49930,.F.);
#69801=ORIENTED_EDGE('',*,*,#49931,.T.);
#69802=ORIENTED_EDGE('',*,*,#49924,.T.);
#69803=ORIENTED_EDGE('',*,*,#49932,.T.);
#69804=ORIENTED_EDGE('',*,*,#49933,.F.);
#69805=ORIENTED_EDGE('',*,*,#49934,.T.);
#69806=ORIENTED_EDGE('',*,*,#49927,.T.);
#69807=ORIENTED_EDGE('',*,*,#49935,.T.);
#69808=ORIENTED_EDGE('',*,*,#49936,.F.);
#69809=ORIENTED_EDGE('',*,*,#49937,.T.);
#69810=ORIENTED_EDGE('',*,*,#49930,.T.);
#69811=ORIENTED_EDGE('',*,*,#49938,.T.);
#69812=ORIENTED_EDGE('',*,*,#49939,.F.);
#69813=ORIENTED_EDGE('',*,*,#49940,.T.);
#69814=ORIENTED_EDGE('',*,*,#49933,.T.);
#69815=ORIENTED_EDGE('',*,*,#49941,.T.);
#69816=ORIENTED_EDGE('',*,*,#49942,.F.);
#69817=ORIENTED_EDGE('',*,*,#49943,.T.);
#69818=ORIENTED_EDGE('',*,*,#49936,.T.);
#69819=ORIENTED_EDGE('',*,*,#49944,.T.);
#69820=ORIENTED_EDGE('',*,*,#49939,.T.);
#69821=ORIENTED_EDGE('',*,*,#49945,.T.);
#69822=ORIENTED_EDGE('',*,*,#49942,.T.);
#69823=ORIENTED_EDGE('',*,*,#49946,.T.);
#69824=ORIENTED_EDGE('',*,*,#49947,.F.);
#69825=ORIENTED_EDGE('',*,*,#49948,.T.);
#69826=ORIENTED_EDGE('',*,*,#49949,.F.);
#69827=ORIENTED_EDGE('',*,*,#49950,.T.);
#69828=ORIENTED_EDGE('',*,*,#49951,.F.);
#69829=ORIENTED_EDGE('',*,*,#49952,.T.);
#69830=ORIENTED_EDGE('',*,*,#49949,.T.);
#69831=ORIENTED_EDGE('',*,*,#49953,.T.);
#69832=ORIENTED_EDGE('',*,*,#49954,.F.);
#69833=ORIENTED_EDGE('',*,*,#49955,.T.);
#69834=ORIENTED_EDGE('',*,*,#49947,.T.);
#69835=ORIENTED_EDGE('',*,*,#49956,.T.);
#69836=ORIENTED_EDGE('',*,*,#49957,.F.);
#69837=ORIENTED_EDGE('',*,*,#49958,.T.);
#69838=ORIENTED_EDGE('',*,*,#49951,.T.);
#69839=ORIENTED_EDGE('',*,*,#49959,.T.);
#69840=ORIENTED_EDGE('',*,*,#49960,.F.);
#69841=ORIENTED_EDGE('',*,*,#49961,.T.);
#69842=ORIENTED_EDGE('',*,*,#49954,.T.);
#69843=ORIENTED_EDGE('',*,*,#49962,.T.);
#69844=ORIENTED_EDGE('',*,*,#49963,.F.);
#69845=ORIENTED_EDGE('',*,*,#49964,.T.);
#69846=ORIENTED_EDGE('',*,*,#49957,.T.);
#69847=ORIENTED_EDGE('',*,*,#49965,.T.);
#69848=ORIENTED_EDGE('',*,*,#49966,.F.);
#69849=ORIENTED_EDGE('',*,*,#49967,.T.);
#69850=ORIENTED_EDGE('',*,*,#49960,.T.);
#69851=ORIENTED_EDGE('',*,*,#49968,.T.);
#69852=ORIENTED_EDGE('',*,*,#49963,.T.);
#69853=ORIENTED_EDGE('',*,*,#49969,.T.);
#69854=ORIENTED_EDGE('',*,*,#49966,.T.);
#69855=ORIENTED_EDGE('',*,*,#49970,.T.);
#69856=ORIENTED_EDGE('',*,*,#49971,.F.);
#69857=ORIENTED_EDGE('',*,*,#49972,.T.);
#69858=ORIENTED_EDGE('',*,*,#49973,.F.);
#69859=ORIENTED_EDGE('',*,*,#49974,.T.);
#69860=ORIENTED_EDGE('',*,*,#49975,.F.);
#69861=ORIENTED_EDGE('',*,*,#49976,.T.);
#69862=ORIENTED_EDGE('',*,*,#49973,.T.);
#69863=ORIENTED_EDGE('',*,*,#49977,.T.);
#69864=ORIENTED_EDGE('',*,*,#49978,.F.);
#69865=ORIENTED_EDGE('',*,*,#49979,.T.);
#69866=ORIENTED_EDGE('',*,*,#49971,.T.);
#69867=ORIENTED_EDGE('',*,*,#49980,.T.);
#69868=ORIENTED_EDGE('',*,*,#49981,.F.);
#69869=ORIENTED_EDGE('',*,*,#49982,.T.);
#69870=ORIENTED_EDGE('',*,*,#49975,.T.);
#69871=ORIENTED_EDGE('',*,*,#49983,.T.);
#69872=ORIENTED_EDGE('',*,*,#49984,.F.);
#69873=ORIENTED_EDGE('',*,*,#49985,.T.);
#69874=ORIENTED_EDGE('',*,*,#49978,.T.);
#69875=ORIENTED_EDGE('',*,*,#49986,.T.);
#69876=ORIENTED_EDGE('',*,*,#49987,.F.);
#69877=ORIENTED_EDGE('',*,*,#49988,.T.);
#69878=ORIENTED_EDGE('',*,*,#49981,.T.);
#69879=ORIENTED_EDGE('',*,*,#49989,.T.);
#69880=ORIENTED_EDGE('',*,*,#49990,.F.);
#69881=ORIENTED_EDGE('',*,*,#49991,.T.);
#69882=ORIENTED_EDGE('',*,*,#49984,.T.);
#69883=ORIENTED_EDGE('',*,*,#49992,.T.);
#69884=ORIENTED_EDGE('',*,*,#49993,.F.);
#69885=ORIENTED_EDGE('',*,*,#49994,.T.);
#69886=ORIENTED_EDGE('',*,*,#49987,.T.);
#69887=ORIENTED_EDGE('',*,*,#49995,.T.);
#69888=ORIENTED_EDGE('',*,*,#49996,.F.);
#69889=ORIENTED_EDGE('',*,*,#49997,.T.);
#69890=ORIENTED_EDGE('',*,*,#49990,.T.);
#69891=ORIENTED_EDGE('',*,*,#49998,.T.);
#69892=ORIENTED_EDGE('',*,*,#49993,.T.);
#69893=ORIENTED_EDGE('',*,*,#49999,.T.);
#69894=ORIENTED_EDGE('',*,*,#49996,.T.);
#69895=ORIENTED_EDGE('',*,*,#50000,.T.);
#69896=ORIENTED_EDGE('',*,*,#50001,.F.);
#69897=ORIENTED_EDGE('',*,*,#50002,.T.);
#69898=ORIENTED_EDGE('',*,*,#50003,.F.);
#69899=ORIENTED_EDGE('',*,*,#50004,.T.);
#69900=ORIENTED_EDGE('',*,*,#50005,.F.);
#69901=ORIENTED_EDGE('',*,*,#50006,.T.);
#69902=ORIENTED_EDGE('',*,*,#50003,.T.);
#69903=ORIENTED_EDGE('',*,*,#50007,.T.);
#69904=ORIENTED_EDGE('',*,*,#50008,.F.);
#69905=ORIENTED_EDGE('',*,*,#50009,.T.);
#69906=ORIENTED_EDGE('',*,*,#50001,.T.);
#69907=ORIENTED_EDGE('',*,*,#50010,.T.);
#69908=ORIENTED_EDGE('',*,*,#50011,.F.);
#69909=ORIENTED_EDGE('',*,*,#50012,.T.);
#69910=ORIENTED_EDGE('',*,*,#50005,.T.);
#69911=ORIENTED_EDGE('',*,*,#50013,.T.);
#69912=ORIENTED_EDGE('',*,*,#50014,.F.);
#69913=ORIENTED_EDGE('',*,*,#50015,.T.);
#69914=ORIENTED_EDGE('',*,*,#50008,.T.);
#69915=ORIENTED_EDGE('',*,*,#50016,.T.);
#69916=ORIENTED_EDGE('',*,*,#50017,.F.);
#69917=ORIENTED_EDGE('',*,*,#50018,.T.);
#69918=ORIENTED_EDGE('',*,*,#50011,.T.);
#69919=ORIENTED_EDGE('',*,*,#50019,.T.);
#69920=ORIENTED_EDGE('',*,*,#50020,.F.);
#69921=ORIENTED_EDGE('',*,*,#50021,.T.);
#69922=ORIENTED_EDGE('',*,*,#50014,.T.);
#69923=ORIENTED_EDGE('',*,*,#50022,.T.);
#69924=ORIENTED_EDGE('',*,*,#50017,.T.);
#69925=ORIENTED_EDGE('',*,*,#50023,.T.);
#69926=ORIENTED_EDGE('',*,*,#50020,.T.);
#69927=ORIENTED_EDGE('',*,*,#50024,.T.);
#69928=ORIENTED_EDGE('',*,*,#50025,.F.);
#69929=ORIENTED_EDGE('',*,*,#50026,.T.);
#69930=ORIENTED_EDGE('',*,*,#50027,.F.);
#69931=ORIENTED_EDGE('',*,*,#50028,.T.);
#69932=ORIENTED_EDGE('',*,*,#50029,.F.);
#69933=ORIENTED_EDGE('',*,*,#50030,.T.);
#69934=ORIENTED_EDGE('',*,*,#50027,.T.);
#69935=ORIENTED_EDGE('',*,*,#50031,.T.);
#69936=ORIENTED_EDGE('',*,*,#50032,.F.);
#69937=ORIENTED_EDGE('',*,*,#50033,.T.);
#69938=ORIENTED_EDGE('',*,*,#50025,.T.);
#69939=ORIENTED_EDGE('',*,*,#50034,.T.);
#69940=ORIENTED_EDGE('',*,*,#50035,.F.);
#69941=ORIENTED_EDGE('',*,*,#50036,.T.);
#69942=ORIENTED_EDGE('',*,*,#50029,.T.);
#69943=ORIENTED_EDGE('',*,*,#50037,.T.);
#69944=ORIENTED_EDGE('',*,*,#50038,.F.);
#69945=ORIENTED_EDGE('',*,*,#50039,.T.);
#69946=ORIENTED_EDGE('',*,*,#50032,.T.);
#69947=ORIENTED_EDGE('',*,*,#50040,.T.);
#69948=ORIENTED_EDGE('',*,*,#50041,.F.);
#69949=ORIENTED_EDGE('',*,*,#50042,.T.);
#69950=ORIENTED_EDGE('',*,*,#50035,.T.);
#69951=ORIENTED_EDGE('',*,*,#50043,.T.);
#69952=ORIENTED_EDGE('',*,*,#50044,.F.);
#69953=ORIENTED_EDGE('',*,*,#50045,.T.);
#69954=ORIENTED_EDGE('',*,*,#50038,.T.);
#69955=ORIENTED_EDGE('',*,*,#50046,.T.);
#69956=ORIENTED_EDGE('',*,*,#50041,.T.);
#69957=ORIENTED_EDGE('',*,*,#50047,.T.);
#69958=ORIENTED_EDGE('',*,*,#50044,.T.);
#69959=ORIENTED_EDGE('',*,*,#50048,.T.);
#69960=ORIENTED_EDGE('',*,*,#50049,.F.);
#69961=ORIENTED_EDGE('',*,*,#50050,.T.);
#69962=ORIENTED_EDGE('',*,*,#50051,.F.);
#69963=ORIENTED_EDGE('',*,*,#50052,.T.);
#69964=ORIENTED_EDGE('',*,*,#50053,.F.);
#69965=ORIENTED_EDGE('',*,*,#50054,.T.);
#69966=ORIENTED_EDGE('',*,*,#50051,.T.);
#69967=ORIENTED_EDGE('',*,*,#50055,.T.);
#69968=ORIENTED_EDGE('',*,*,#50056,.F.);
#69969=ORIENTED_EDGE('',*,*,#50057,.T.);
#69970=ORIENTED_EDGE('',*,*,#50049,.T.);
#69971=ORIENTED_EDGE('',*,*,#50058,.T.);
#69972=ORIENTED_EDGE('',*,*,#50059,.F.);
#69973=ORIENTED_EDGE('',*,*,#50060,.T.);
#69974=ORIENTED_EDGE('',*,*,#50053,.T.);
#69975=ORIENTED_EDGE('',*,*,#50061,.T.);
#69976=ORIENTED_EDGE('',*,*,#50062,.F.);
#69977=ORIENTED_EDGE('',*,*,#50063,.T.);
#69978=ORIENTED_EDGE('',*,*,#50056,.T.);
#69979=ORIENTED_EDGE('',*,*,#50064,.T.);
#69980=ORIENTED_EDGE('',*,*,#50065,.F.);
#69981=ORIENTED_EDGE('',*,*,#50066,.T.);
#69982=ORIENTED_EDGE('',*,*,#50059,.T.);
#69983=ORIENTED_EDGE('',*,*,#50067,.T.);
#69984=ORIENTED_EDGE('',*,*,#50068,.F.);
#69985=ORIENTED_EDGE('',*,*,#50069,.T.);
#69986=ORIENTED_EDGE('',*,*,#50062,.T.);
#69987=ORIENTED_EDGE('',*,*,#50070,.T.);
#69988=ORIENTED_EDGE('',*,*,#50065,.T.);
#69989=ORIENTED_EDGE('',*,*,#50071,.T.);
#69990=ORIENTED_EDGE('',*,*,#50068,.T.);
#69991=ORIENTED_EDGE('',*,*,#50072,.T.);
#69992=ORIENTED_EDGE('',*,*,#50073,.F.);
#69993=ORIENTED_EDGE('',*,*,#50074,.T.);
#69994=ORIENTED_EDGE('',*,*,#50075,.F.);
#69995=ORIENTED_EDGE('',*,*,#50076,.T.);
#69996=ORIENTED_EDGE('',*,*,#50077,.F.);
#69997=ORIENTED_EDGE('',*,*,#50078,.T.);
#69998=ORIENTED_EDGE('',*,*,#50075,.T.);
#69999=ORIENTED_EDGE('',*,*,#50079,.T.);
#70000=ORIENTED_EDGE('',*,*,#50080,.F.);
#70001=ORIENTED_EDGE('',*,*,#50081,.T.);
#70002=ORIENTED_EDGE('',*,*,#50073,.T.);
#70003=ORIENTED_EDGE('',*,*,#50082,.T.);
#70004=ORIENTED_EDGE('',*,*,#50083,.F.);
#70005=ORIENTED_EDGE('',*,*,#50084,.T.);
#70006=ORIENTED_EDGE('',*,*,#50077,.T.);
#70007=ORIENTED_EDGE('',*,*,#50085,.T.);
#70008=ORIENTED_EDGE('',*,*,#50086,.F.);
#70009=ORIENTED_EDGE('',*,*,#50087,.T.);
#70010=ORIENTED_EDGE('',*,*,#50080,.T.);
#70011=ORIENTED_EDGE('',*,*,#50088,.T.);
#70012=ORIENTED_EDGE('',*,*,#50089,.F.);
#70013=ORIENTED_EDGE('',*,*,#50090,.T.);
#70014=ORIENTED_EDGE('',*,*,#50083,.T.);
#70015=ORIENTED_EDGE('',*,*,#50091,.T.);
#70016=ORIENTED_EDGE('',*,*,#50092,.F.);
#70017=ORIENTED_EDGE('',*,*,#50093,.T.);
#70018=ORIENTED_EDGE('',*,*,#50086,.T.);
#70019=ORIENTED_EDGE('',*,*,#50094,.T.);
#70020=ORIENTED_EDGE('',*,*,#50089,.T.);
#70021=ORIENTED_EDGE('',*,*,#50095,.T.);
#70022=ORIENTED_EDGE('',*,*,#50092,.T.);
#70023=ORIENTED_EDGE('',*,*,#50096,.T.);
#70024=ORIENTED_EDGE('',*,*,#50097,.F.);
#70025=ORIENTED_EDGE('',*,*,#50098,.T.);
#70026=ORIENTED_EDGE('',*,*,#50099,.F.);
#70027=ORIENTED_EDGE('',*,*,#50100,.T.);
#70028=ORIENTED_EDGE('',*,*,#50101,.F.);
#70029=ORIENTED_EDGE('',*,*,#50102,.T.);
#70030=ORIENTED_EDGE('',*,*,#50099,.T.);
#70031=ORIENTED_EDGE('',*,*,#50103,.T.);
#70032=ORIENTED_EDGE('',*,*,#50104,.F.);
#70033=ORIENTED_EDGE('',*,*,#50105,.T.);
#70034=ORIENTED_EDGE('',*,*,#50097,.T.);
#70035=ORIENTED_EDGE('',*,*,#50106,.T.);
#70036=ORIENTED_EDGE('',*,*,#50107,.F.);
#70037=ORIENTED_EDGE('',*,*,#50108,.T.);
#70038=ORIENTED_EDGE('',*,*,#50101,.T.);
#70039=ORIENTED_EDGE('',*,*,#50109,.T.);
#70040=ORIENTED_EDGE('',*,*,#50110,.F.);
#70041=ORIENTED_EDGE('',*,*,#50111,.T.);
#70042=ORIENTED_EDGE('',*,*,#50104,.T.);
#70043=ORIENTED_EDGE('',*,*,#50112,.T.);
#70044=ORIENTED_EDGE('',*,*,#50107,.T.);
#70045=ORIENTED_EDGE('',*,*,#50113,.T.);
#70046=ORIENTED_EDGE('',*,*,#50110,.T.);
#70047=ORIENTED_EDGE('',*,*,#50114,.T.);
#70048=ORIENTED_EDGE('',*,*,#50115,.T.);
#70049=ORIENTED_EDGE('',*,*,#50116,.F.);
#70050=ORIENTED_EDGE('',*,*,#50117,.T.);
#70051=ORIENTED_EDGE('',*,*,#50118,.F.);
#70052=ORIENTED_EDGE('',*,*,#50119,.F.);
#70053=ORIENTED_EDGE('',*,*,#50120,.T.);
#70054=ORIENTED_EDGE('',*,*,#50116,.T.);
#70055=ORIENTED_EDGE('',*,*,#50121,.T.);
#70056=ORIENTED_EDGE('',*,*,#50122,.F.);
#70057=ORIENTED_EDGE('',*,*,#50123,.T.);
#70058=ORIENTED_EDGE('',*,*,#50118,.T.);
#70059=ORIENTED_EDGE('',*,*,#50124,.T.);
#70060=ORIENTED_EDGE('',*,*,#50125,.F.);
#70061=ORIENTED_EDGE('',*,*,#50126,.T.);
#70062=ORIENTED_EDGE('',*,*,#50119,.T.);
#70063=ORIENTED_EDGE('',*,*,#50127,.T.);
#70064=ORIENTED_EDGE('',*,*,#50128,.F.);
#70065=ORIENTED_EDGE('',*,*,#50129,.T.);
#70066=ORIENTED_EDGE('',*,*,#50122,.T.);
#70067=ORIENTED_EDGE('',*,*,#50130,.T.);
#70068=ORIENTED_EDGE('',*,*,#50125,.T.);
#70069=ORIENTED_EDGE('',*,*,#50131,.T.);
#70070=ORIENTED_EDGE('',*,*,#50128,.T.);
#70071=ORIENTED_EDGE('',*,*,#50132,.T.);
#70072=ORIENTED_EDGE('',*,*,#50133,.F.);
#70073=ORIENTED_EDGE('',*,*,#50134,.T.);
#70074=ORIENTED_EDGE('',*,*,#50135,.T.);
#70075=ORIENTED_EDGE('',*,*,#50136,.T.);
#70076=ORIENTED_EDGE('',*,*,#50137,.F.);
#70077=ORIENTED_EDGE('',*,*,#50138,.T.);
#70078=ORIENTED_EDGE('',*,*,#50133,.T.);
#70079=ORIENTED_EDGE('',*,*,#50139,.T.);
#70080=ORIENTED_EDGE('',*,*,#50140,.F.);
#70081=ORIENTED_EDGE('',*,*,#50141,.T.);
#70082=ORIENTED_EDGE('',*,*,#50137,.T.);
#70083=ORIENTED_EDGE('',*,*,#50142,.T.);
#70084=ORIENTED_EDGE('',*,*,#50143,.F.);
#70085=ORIENTED_EDGE('',*,*,#50144,.T.);
#70086=ORIENTED_EDGE('',*,*,#50140,.T.);
#70087=ORIENTED_EDGE('',*,*,#50145,.T.);
#70088=ORIENTED_EDGE('',*,*,#50146,.F.);
#70089=ORIENTED_EDGE('',*,*,#50147,.T.);
#70090=ORIENTED_EDGE('',*,*,#50143,.T.);
#70091=ORIENTED_EDGE('',*,*,#50148,.T.);
#70092=ORIENTED_EDGE('',*,*,#50149,.F.);
#70093=ORIENTED_EDGE('',*,*,#50150,.T.);
#70094=ORIENTED_EDGE('',*,*,#50146,.T.);
#70095=ORIENTED_EDGE('',*,*,#50151,.T.);
#70096=ORIENTED_EDGE('',*,*,#50152,.F.);
#70097=ORIENTED_EDGE('',*,*,#50153,.T.);
#70098=ORIENTED_EDGE('',*,*,#50149,.T.);
#70099=ORIENTED_EDGE('',*,*,#50154,.T.);
#70100=ORIENTED_EDGE('',*,*,#50155,.F.);
#70101=ORIENTED_EDGE('',*,*,#50156,.T.);
#70102=ORIENTED_EDGE('',*,*,#50157,.T.);
#70103=ORIENTED_EDGE('',*,*,#50158,.T.);
#70104=ORIENTED_EDGE('',*,*,#50159,.F.);
#70105=ORIENTED_EDGE('',*,*,#50160,.T.);
#70106=ORIENTED_EDGE('',*,*,#50155,.T.);
#70107=ORIENTED_EDGE('',*,*,#50161,.T.);
#70108=ORIENTED_EDGE('',*,*,#50162,.F.);
#70109=ORIENTED_EDGE('',*,*,#50163,.T.);
#70110=ORIENTED_EDGE('',*,*,#50159,.T.);
#70111=ORIENTED_EDGE('',*,*,#50164,.T.);
#70112=ORIENTED_EDGE('',*,*,#50165,.F.);
#70113=ORIENTED_EDGE('',*,*,#50166,.T.);
#70114=ORIENTED_EDGE('',*,*,#50162,.T.);
#70115=ORIENTED_EDGE('',*,*,#50167,.T.);
#70116=ORIENTED_EDGE('',*,*,#50168,.F.);
#70117=ORIENTED_EDGE('',*,*,#50169,.T.);
#70118=ORIENTED_EDGE('',*,*,#50165,.T.);
#70119=ORIENTED_EDGE('',*,*,#50170,.T.);
#70120=ORIENTED_EDGE('',*,*,#50171,.F.);
#70121=ORIENTED_EDGE('',*,*,#50172,.T.);
#70122=ORIENTED_EDGE('',*,*,#50168,.T.);
#70123=ORIENTED_EDGE('',*,*,#50173,.T.);
#70124=ORIENTED_EDGE('',*,*,#50174,.F.);
#70125=ORIENTED_EDGE('',*,*,#50175,.T.);
#70126=ORIENTED_EDGE('',*,*,#50171,.T.);
#70127=ORIENTED_EDGE('',*,*,#50176,.T.);
#70128=ORIENTED_EDGE('',*,*,#50177,.F.);
#70129=ORIENTED_EDGE('',*,*,#50178,.T.);
#70130=ORIENTED_EDGE('',*,*,#50179,.T.);
#70131=ORIENTED_EDGE('',*,*,#50180,.T.);
#70132=ORIENTED_EDGE('',*,*,#50181,.F.);
#70133=ORIENTED_EDGE('',*,*,#50182,.T.);
#70134=ORIENTED_EDGE('',*,*,#50177,.T.);
#70135=ORIENTED_EDGE('',*,*,#50183,.T.);
#70136=ORIENTED_EDGE('',*,*,#50184,.T.);
#70137=ORIENTED_EDGE('',*,*,#50181,.T.);
#70138=ORIENTED_EDGE('',*,*,#50185,.T.);
#70139=ORIENTED_EDGE('',*,*,#50186,.F.);
#70140=ORIENTED_EDGE('',*,*,#50187,.F.);
#70141=ORIENTED_EDGE('',*,*,#50188,.T.);
#70142=ORIENTED_EDGE('',*,*,#50186,.T.);
#70143=ORIENTED_EDGE('',*,*,#50189,.T.);
#70144=ORIENTED_EDGE('',*,*,#50190,.F.);
#70145=ORIENTED_EDGE('',*,*,#50191,.T.);
#70146=ORIENTED_EDGE('',*,*,#50187,.T.);
#70147=ORIENTED_EDGE('',*,*,#50192,.T.);
#70148=ORIENTED_EDGE('',*,*,#50193,.F.);
#70149=ORIENTED_EDGE('',*,*,#50194,.T.);
#70150=ORIENTED_EDGE('',*,*,#50190,.T.);
#70151=ORIENTED_EDGE('',*,*,#50195,.T.);
#70152=ORIENTED_EDGE('',*,*,#50196,.T.);
#70153=ORIENTED_EDGE('',*,*,#50197,.T.);
#70154=ORIENTED_EDGE('',*,*,#50193,.T.);
#70155=ORIENTED_EDGE('',*,*,#50198,.T.);
#70156=ORIENTED_EDGE('',*,*,#50199,.F.);
#70157=ORIENTED_EDGE('',*,*,#50200,.T.);
#70158=ORIENTED_EDGE('',*,*,#50201,.T.);
#70159=ORIENTED_EDGE('',*,*,#50202,.T.);
#70160=ORIENTED_EDGE('',*,*,#50203,.F.);
#70161=ORIENTED_EDGE('',*,*,#50204,.T.);
#70162=ORIENTED_EDGE('',*,*,#50199,.T.);
#70163=ORIENTED_EDGE('',*,*,#50205,.T.);
#70164=ORIENTED_EDGE('',*,*,#50206,.F.);
#70165=ORIENTED_EDGE('',*,*,#50207,.T.);
#70166=ORIENTED_EDGE('',*,*,#50203,.T.);
#70167=ORIENTED_EDGE('',*,*,#50208,.T.);
#70168=ORIENTED_EDGE('',*,*,#50209,.F.);
#70169=ORIENTED_EDGE('',*,*,#50210,.T.);
#70170=ORIENTED_EDGE('',*,*,#50206,.T.);
#70171=ORIENTED_EDGE('',*,*,#50211,.T.);
#70172=ORIENTED_EDGE('',*,*,#50212,.F.);
#70173=ORIENTED_EDGE('',*,*,#50213,.T.);
#70174=ORIENTED_EDGE('',*,*,#50209,.T.);
#70175=ORIENTED_EDGE('',*,*,#50214,.T.);
#70176=ORIENTED_EDGE('',*,*,#50215,.F.);
#70177=ORIENTED_EDGE('',*,*,#50216,.T.);
#70178=ORIENTED_EDGE('',*,*,#50212,.T.);
#70179=ORIENTED_EDGE('',*,*,#50217,.T.);
#70180=ORIENTED_EDGE('',*,*,#50218,.T.);
#70181=ORIENTED_EDGE('',*,*,#50219,.T.);
#70182=ORIENTED_EDGE('',*,*,#50215,.T.);
#70183=ORIENTED_EDGE('',*,*,#50220,.T.);
#70184=ORIENTED_EDGE('',*,*,#50221,.F.);
#70185=ORIENTED_EDGE('',*,*,#50222,.T.);
#70186=ORIENTED_EDGE('',*,*,#50223,.T.);
#70187=ORIENTED_EDGE('',*,*,#50224,.T.);
#70188=ORIENTED_EDGE('',*,*,#50225,.F.);
#70189=ORIENTED_EDGE('',*,*,#50226,.T.);
#70190=ORIENTED_EDGE('',*,*,#50221,.T.);
#70191=ORIENTED_EDGE('',*,*,#50227,.T.);
#70192=ORIENTED_EDGE('',*,*,#50228,.T.);
#70193=ORIENTED_EDGE('',*,*,#50225,.T.);
#70194=ORIENTED_EDGE('',*,*,#50229,.T.);
#70195=ORIENTED_EDGE('',*,*,#50230,.F.);
#70196=ORIENTED_EDGE('',*,*,#50231,.F.);
#70197=ORIENTED_EDGE('',*,*,#50232,.T.);
#70198=ORIENTED_EDGE('',*,*,#50230,.T.);
#70199=ORIENTED_EDGE('',*,*,#50233,.T.);
#70200=ORIENTED_EDGE('',*,*,#50234,.F.);
#70201=ORIENTED_EDGE('',*,*,#50235,.T.);
#70202=ORIENTED_EDGE('',*,*,#50231,.T.);
#70203=ORIENTED_EDGE('',*,*,#50236,.T.);
#70204=ORIENTED_EDGE('',*,*,#50237,.F.);
#70205=ORIENTED_EDGE('',*,*,#50238,.T.);
#70206=ORIENTED_EDGE('',*,*,#50234,.T.);
#70207=ORIENTED_EDGE('',*,*,#50239,.T.);
#70208=ORIENTED_EDGE('',*,*,#50240,.T.);
#70209=ORIENTED_EDGE('',*,*,#50241,.T.);
#70210=ORIENTED_EDGE('',*,*,#50237,.T.);
#70211=ORIENTED_EDGE('',*,*,#50242,.T.);
#70212=ORIENTED_EDGE('',*,*,#50243,.T.);
#70213=ORIENTED_EDGE('',*,*,#50244,.T.);
#70214=ORIENTED_EDGE('',*,*,#50245,.F.);
#70215=ORIENTED_EDGE('',*,*,#50246,.T.);
#70216=ORIENTED_EDGE('',*,*,#50247,.F.);
#70217=ORIENTED_EDGE('',*,*,#50248,.T.);
#70218=ORIENTED_EDGE('',*,*,#50245,.T.);
#70219=ORIENTED_EDGE('',*,*,#50249,.T.);
#70220=ORIENTED_EDGE('',*,*,#50250,.F.);
#70221=ORIENTED_EDGE('',*,*,#50251,.T.);
#70222=ORIENTED_EDGE('',*,*,#50247,.T.);
#70223=ORIENTED_EDGE('',*,*,#50252,.T.);
#70224=ORIENTED_EDGE('',*,*,#50253,.F.);
#70225=ORIENTED_EDGE('',*,*,#50254,.T.);
#70226=ORIENTED_EDGE('',*,*,#50250,.T.);
#70227=ORIENTED_EDGE('',*,*,#50255,.T.);
#70228=ORIENTED_EDGE('',*,*,#50256,.F.);
#70229=ORIENTED_EDGE('',*,*,#50257,.T.);
#70230=ORIENTED_EDGE('',*,*,#50253,.T.);
#70231=ORIENTED_EDGE('',*,*,#50258,.T.);
#70232=ORIENTED_EDGE('',*,*,#50259,.F.);
#70233=ORIENTED_EDGE('',*,*,#50260,.T.);
#70234=ORIENTED_EDGE('',*,*,#50256,.T.);
#70235=ORIENTED_EDGE('',*,*,#50261,.T.);
#70236=ORIENTED_EDGE('',*,*,#50262,.T.);
#70237=ORIENTED_EDGE('',*,*,#50263,.T.);
#70238=ORIENTED_EDGE('',*,*,#50259,.T.);
#70239=ORIENTED_EDGE('',*,*,#50264,.T.);
#70240=ORIENTED_EDGE('',*,*,#50265,.F.);
#70241=ORIENTED_EDGE('',*,*,#50266,.T.);
#70242=ORIENTED_EDGE('',*,*,#50267,.T.);
#70243=ORIENTED_EDGE('',*,*,#50268,.T.);
#70244=ORIENTED_EDGE('',*,*,#50269,.F.);
#70245=ORIENTED_EDGE('',*,*,#50270,.T.);
#70246=ORIENTED_EDGE('',*,*,#50265,.T.);
#70247=ORIENTED_EDGE('',*,*,#50271,.T.);
#70248=ORIENTED_EDGE('',*,*,#50272,.F.);
#70249=ORIENTED_EDGE('',*,*,#50273,.T.);
#70250=ORIENTED_EDGE('',*,*,#50269,.T.);
#70251=ORIENTED_EDGE('',*,*,#50274,.T.);
#70252=ORIENTED_EDGE('',*,*,#50275,.F.);
#70253=ORIENTED_EDGE('',*,*,#50276,.T.);
#70254=ORIENTED_EDGE('',*,*,#50272,.T.);
#70255=ORIENTED_EDGE('',*,*,#50277,.T.);
#70256=ORIENTED_EDGE('',*,*,#50278,.F.);
#70257=ORIENTED_EDGE('',*,*,#50279,.T.);
#70258=ORIENTED_EDGE('',*,*,#50275,.T.);
#70259=ORIENTED_EDGE('',*,*,#50280,.T.);
#70260=ORIENTED_EDGE('',*,*,#50281,.F.);
#70261=ORIENTED_EDGE('',*,*,#50282,.T.);
#70262=ORIENTED_EDGE('',*,*,#50278,.T.);
#70263=ORIENTED_EDGE('',*,*,#50283,.T.);
#70264=ORIENTED_EDGE('',*,*,#50284,.F.);
#70265=ORIENTED_EDGE('',*,*,#50285,.T.);
#70266=ORIENTED_EDGE('',*,*,#50281,.T.);
#70267=ORIENTED_EDGE('',*,*,#50286,.T.);
#70268=ORIENTED_EDGE('',*,*,#50287,.T.);
#70269=ORIENTED_EDGE('',*,*,#50288,.T.);
#70270=ORIENTED_EDGE('',*,*,#50289,.T.);
#70271=ORIENTED_EDGE('',*,*,#50290,.T.);
#70272=ORIENTED_EDGE('',*,*,#50291,.F.);
#70273=ORIENTED_EDGE('',*,*,#50292,.T.);
#70274=ORIENTED_EDGE('',*,*,#50293,.F.);
#70275=ORIENTED_EDGE('',*,*,#50294,.T.);
#70276=ORIENTED_EDGE('',*,*,#50291,.T.);
#70277=ORIENTED_EDGE('',*,*,#50295,.T.);
#70278=ORIENTED_EDGE('',*,*,#50296,.F.);
#70279=ORIENTED_EDGE('',*,*,#50297,.T.);
#70280=ORIENTED_EDGE('',*,*,#50293,.T.);
#70281=ORIENTED_EDGE('',*,*,#50298,.T.);
#70282=ORIENTED_EDGE('',*,*,#50299,.F.);
#70283=ORIENTED_EDGE('',*,*,#50300,.T.);
#70284=ORIENTED_EDGE('',*,*,#50296,.T.);
#70285=ORIENTED_EDGE('',*,*,#50301,.T.);
#70286=ORIENTED_EDGE('',*,*,#50302,.F.);
#70287=ORIENTED_EDGE('',*,*,#50303,.T.);
#70288=ORIENTED_EDGE('',*,*,#50299,.T.);
#70289=ORIENTED_EDGE('',*,*,#50304,.T.);
#70290=ORIENTED_EDGE('',*,*,#50305,.F.);
#70291=ORIENTED_EDGE('',*,*,#50306,.T.);
#70292=ORIENTED_EDGE('',*,*,#50302,.T.);
#70293=ORIENTED_EDGE('',*,*,#50307,.T.);
#70294=ORIENTED_EDGE('',*,*,#50308,.F.);
#70295=ORIENTED_EDGE('',*,*,#50309,.T.);
#70296=ORIENTED_EDGE('',*,*,#50305,.T.);
#70297=ORIENTED_EDGE('',*,*,#50310,.T.);
#70298=ORIENTED_EDGE('',*,*,#50311,.F.);
#70299=ORIENTED_EDGE('',*,*,#50312,.T.);
#70300=ORIENTED_EDGE('',*,*,#50308,.T.);
#70301=ORIENTED_EDGE('',*,*,#50313,.T.);
#70302=ORIENTED_EDGE('',*,*,#50314,.F.);
#70303=ORIENTED_EDGE('',*,*,#50315,.T.);
#70304=ORIENTED_EDGE('',*,*,#50316,.T.);
#70305=ORIENTED_EDGE('',*,*,#50317,.T.);
#70306=ORIENTED_EDGE('',*,*,#50318,.T.);
#70307=ORIENTED_EDGE('',*,*,#50319,.T.);
#70308=ORIENTED_EDGE('',*,*,#50320,.T.);
#70309=ORIENTED_EDGE('',*,*,#50311,.T.);
#70310=ORIENTED_EDGE('',*,*,#50321,.T.);
#70311=ORIENTED_EDGE('',*,*,#50322,.F.);
#70312=ORIENTED_EDGE('',*,*,#50323,.T.);
#70313=ORIENTED_EDGE('',*,*,#50314,.T.);
#70314=ORIENTED_EDGE('',*,*,#50324,.T.);
#70315=ORIENTED_EDGE('',*,*,#50325,.F.);
#70316=ORIENTED_EDGE('',*,*,#50326,.T.);
#70317=ORIENTED_EDGE('',*,*,#50322,.T.);
#70318=ORIENTED_EDGE('',*,*,#50327,.T.);
#70319=ORIENTED_EDGE('',*,*,#50328,.F.);
#70320=ORIENTED_EDGE('',*,*,#50329,.T.);
#70321=ORIENTED_EDGE('',*,*,#50325,.T.);
#70322=ORIENTED_EDGE('',*,*,#50330,.T.);
#70323=ORIENTED_EDGE('',*,*,#50331,.F.);
#70324=ORIENTED_EDGE('',*,*,#50332,.T.);
#70325=ORIENTED_EDGE('',*,*,#50328,.T.);
#70326=ORIENTED_EDGE('',*,*,#50333,.T.);
#70327=ORIENTED_EDGE('',*,*,#50334,.F.);
#70328=ORIENTED_EDGE('',*,*,#50335,.T.);
#70329=ORIENTED_EDGE('',*,*,#50331,.T.);
#70330=ORIENTED_EDGE('',*,*,#50336,.T.);
#70331=ORIENTED_EDGE('',*,*,#50337,.F.);
#70332=ORIENTED_EDGE('',*,*,#50338,.T.);
#70333=ORIENTED_EDGE('',*,*,#50334,.T.);
#70334=ORIENTED_EDGE('',*,*,#50339,.T.);
#70335=ORIENTED_EDGE('',*,*,#50340,.F.);
#70336=ORIENTED_EDGE('',*,*,#50341,.T.);
#70337=ORIENTED_EDGE('',*,*,#50337,.T.);
#70338=ORIENTED_EDGE('',*,*,#50342,.T.);
#70339=ORIENTED_EDGE('',*,*,#50343,.T.);
#70340=ORIENTED_EDGE('',*,*,#50344,.F.);
#70341=ORIENTED_EDGE('',*,*,#50345,.T.);
#70342=ORIENTED_EDGE('',*,*,#49261,.F.);
#70343=ORIENTED_EDGE('',*,*,#49267,.F.);
#70344=ORIENTED_EDGE('',*,*,#50346,.F.);
#70345=ORIENTED_EDGE('',*,*,#50347,.T.);
#70346=ORIENTED_EDGE('',*,*,#50344,.T.);
#70347=ORIENTED_EDGE('',*,*,#50348,.T.);
#70348=ORIENTED_EDGE('',*,*,#50349,.F.);
#70349=ORIENTED_EDGE('',*,*,#50350,.T.);
#70350=ORIENTED_EDGE('',*,*,#50346,.T.);
#70351=ORIENTED_EDGE('',*,*,#50351,.T.);
#70352=ORIENTED_EDGE('',*,*,#50352,.F.);
#70353=ORIENTED_EDGE('',*,*,#50353,.T.);
#70354=ORIENTED_EDGE('',*,*,#50349,.T.);
#70355=ORIENTED_EDGE('',*,*,#50354,.T.);
#70356=ORIENTED_EDGE('',*,*,#50355,.F.);
#70357=ORIENTED_EDGE('',*,*,#50356,.F.);
#70358=ORIENTED_EDGE('',*,*,#50357,.T.);
#70359=ORIENTED_EDGE('',*,*,#50352,.T.);
#70360=ORIENTED_EDGE('',*,*,#50358,.T.);
#70361=ORIENTED_EDGE('',*,*,#50359,.T.);
#70362=ORIENTED_EDGE('',*,*,#50360,.T.);
#70363=ORIENTED_EDGE('',*,*,#50356,.T.);
#70364=ORIENTED_EDGE('',*,*,#50361,.F.);
#70365=ORIENTED_EDGE('',*,*,#50361,.T.);
#70366=ORIENTED_EDGE('',*,*,#50355,.T.);
#70367=ORIENTED_EDGE('',*,*,#50362,.F.);
#70368=ORIENTED_EDGE('',*,*,#50363,.F.);
#70369=ORIENTED_EDGE('',*,*,#50364,.T.);
#70370=ORIENTED_EDGE('',*,*,#50365,.T.);
#70371=ORIENTED_EDGE('',*,*,#50366,.T.);
#70372=ORIENTED_EDGE('',*,*,#50367,.T.);
#70373=ORIENTED_EDGE('',*,*,#50368,.T.);
#70374=ORIENTED_EDGE('',*,*,#50369,.T.);
#70375=ORIENTED_EDGE('',*,*,#50370,.T.);
#70376=ORIENTED_EDGE('',*,*,#50362,.T.);
#70377=ORIENTED_EDGE('',*,*,#50371,.T.);
#70378=ORIENTED_EDGE('',*,*,#50372,.F.);
#70379=ORIENTED_EDGE('',*,*,#50363,.T.);
#70380=ORIENTED_EDGE('',*,*,#50373,.F.);
#70381=ORIENTED_EDGE('',*,*,#50374,.T.);
#70382=ORIENTED_EDGE('',*,*,#50375,.T.);
#70383=ORIENTED_EDGE('',*,*,#50372,.T.);
#70384=ORIENTED_EDGE('',*,*,#50376,.F.);
#70385=ORIENTED_EDGE('',*,*,#50376,.T.);
#70386=ORIENTED_EDGE('',*,*,#50373,.T.);
#70387=ORIENTED_EDGE('',*,*,#50377,.T.);
#70388=ORIENTED_EDGE('',*,*,#50378,.F.);
#70389=ORIENTED_EDGE('',*,*,#50379,.T.);
#70390=ORIENTED_EDGE('',*,*,#50380,.F.);
#70391=ORIENTED_EDGE('',*,*,#50381,.T.);
#70392=ORIENTED_EDGE('',*,*,#50378,.T.);
#70393=ORIENTED_EDGE('',*,*,#50382,.T.);
#70394=ORIENTED_EDGE('',*,*,#50383,.F.);
#70395=ORIENTED_EDGE('',*,*,#50384,.T.);
#70396=ORIENTED_EDGE('',*,*,#50380,.T.);
#70397=ORIENTED_EDGE('',*,*,#50385,.T.);
#70398=ORIENTED_EDGE('',*,*,#50386,.F.);
#70399=ORIENTED_EDGE('',*,*,#50387,.T.);
#70400=ORIENTED_EDGE('',*,*,#50383,.T.);
#70401=ORIENTED_EDGE('',*,*,#50388,.T.);
#70402=ORIENTED_EDGE('',*,*,#49291,.F.);
#70403=ORIENTED_EDGE('',*,*,#50389,.T.);
#70404=ORIENTED_EDGE('',*,*,#50386,.T.);
#70405=ORIENTED_EDGE('',*,*,#50390,.T.);
#70406=ORIENTED_EDGE('',*,*,#49285,.F.);
#70407=ORIENTED_EDGE('',*,*,#50391,.F.);
#70408=ORIENTED_EDGE('',*,*,#50392,.T.);
#70409=ORIENTED_EDGE('',*,*,#50393,.F.);
#70410=ORIENTED_EDGE('',*,*,#50394,.T.);
#70411=ORIENTED_EDGE('',*,*,#50395,.T.);
#70412=ORIENTED_EDGE('',*,*,#50391,.T.);
#70413=ORIENTED_EDGE('',*,*,#50396,.F.);
#70414=ORIENTED_EDGE('',*,*,#50396,.T.);
#70415=ORIENTED_EDGE('',*,*,#50393,.T.);
#70416=ORIENTED_EDGE('',*,*,#50397,.T.);
#70417=ORIENTED_EDGE('',*,*,#50398,.F.);
#70418=ORIENTED_EDGE('',*,*,#50399,.T.);
#70419=ORIENTED_EDGE('',*,*,#50400,.F.);
#70420=ORIENTED_EDGE('',*,*,#50401,.T.);
#70421=ORIENTED_EDGE('',*,*,#50398,.T.);
#70422=ORIENTED_EDGE('',*,*,#50402,.T.);
#70423=ORIENTED_EDGE('',*,*,#50403,.F.);
#70424=ORIENTED_EDGE('',*,*,#50404,.T.);
#70425=ORIENTED_EDGE('',*,*,#50400,.T.);
#70426=ORIENTED_EDGE('',*,*,#50405,.T.);
#70427=ORIENTED_EDGE('',*,*,#50406,.F.);
#70428=ORIENTED_EDGE('',*,*,#50407,.T.);
#70429=ORIENTED_EDGE('',*,*,#50403,.T.);
#70430=ORIENTED_EDGE('',*,*,#50408,.T.);
#70431=ORIENTED_EDGE('',*,*,#50409,.T.);
#70432=ORIENTED_EDGE('',*,*,#50406,.T.);
#70433=ORIENTED_EDGE('',*,*,#50410,.T.);
#70434=ORIENTED_EDGE('',*,*,#49265,.F.);
#70435=ORIENTED_EDGE('',*,*,#49259,.F.);
#70436=ORIENTED_EDGE('',*,*,#50411,.T.);
#70437=ORIENTED_EDGE('',*,*,#50412,.T.);
#70438=ORIENTED_EDGE('',*,*,#50413,.F.);
#70439=ORIENTED_EDGE('',*,*,#50414,.T.);
#70440=ORIENTED_EDGE('',*,*,#50415,.T.);
#70441=ORIENTED_EDGE('',*,*,#50416,.T.);
#70442=ORIENTED_EDGE('',*,*,#50417,.T.);
#70443=ORIENTED_EDGE('',*,*,#50418,.F.);
#70444=ORIENTED_EDGE('',*,*,#50419,.T.);
#70445=ORIENTED_EDGE('',*,*,#50413,.T.);
#70446=ORIENTED_EDGE('',*,*,#50420,.T.);
#70447=ORIENTED_EDGE('',*,*,#50421,.F.);
#70448=ORIENTED_EDGE('',*,*,#50418,.T.);
#70449=ORIENTED_EDGE('',*,*,#50422,.F.);
#70450=ORIENTED_EDGE('',*,*,#50423,.T.);
#70451=ORIENTED_EDGE('',*,*,#50424,.F.);
#70452=ORIENTED_EDGE('',*,*,#50425,.T.);
#70453=ORIENTED_EDGE('',*,*,#50421,.T.);
#70454=ORIENTED_EDGE('',*,*,#50426,.F.);
#70455=ORIENTED_EDGE('',*,*,#50426,.T.);
#70456=ORIENTED_EDGE('',*,*,#50422,.T.);
#70457=ORIENTED_EDGE('',*,*,#50427,.T.);
#70458=ORIENTED_EDGE('',*,*,#50428,.T.);
#70459=ORIENTED_EDGE('',*,*,#50429,.F.);
#70460=ORIENTED_EDGE('',*,*,#50430,.T.);
#70461=ORIENTED_EDGE('',*,*,#50424,.T.);
#70462=ORIENTED_EDGE('',*,*,#50431,.T.);
#70463=ORIENTED_EDGE('',*,*,#50432,.F.);
#70464=ORIENTED_EDGE('',*,*,#50433,.T.);
#70465=ORIENTED_EDGE('',*,*,#50429,.T.);
#70466=ORIENTED_EDGE('',*,*,#50434,.T.);
#70467=ORIENTED_EDGE('',*,*,#50435,.F.);
#70468=ORIENTED_EDGE('',*,*,#50436,.T.);
#70469=ORIENTED_EDGE('',*,*,#50432,.T.);
#70470=ORIENTED_EDGE('',*,*,#50437,.T.);
#70471=ORIENTED_EDGE('',*,*,#49296,.F.);
#70472=ORIENTED_EDGE('',*,*,#50438,.T.);
#70473=ORIENTED_EDGE('',*,*,#50435,.T.);
#70474=ORIENTED_EDGE('',*,*,#50439,.T.);
#70475=ORIENTED_EDGE('',*,*,#49302,.F.);
#70476=ORIENTED_EDGE('',*,*,#50440,.T.);
#70477=ORIENTED_EDGE('',*,*,#50394,.F.);
#70478=ORIENTED_EDGE('',*,*,#50441,.T.);
#70479=ORIENTED_EDGE('',*,*,#50341,.F.);
#70480=ORIENTED_EDGE('',*,*,#50442,.T.);
#70481=ORIENTED_EDGE('',*,*,#50360,.F.);
#70482=ORIENTED_EDGE('',*,*,#50443,.T.);
#70483=ORIENTED_EDGE('',*,*,#50323,.F.);
#70484=ORIENTED_EDGE('',*,*,#50444,.T.);
#70485=ORIENTED_EDGE('',*,*,#50374,.F.);
#70486=ORIENTED_EDGE('',*,*,#50445,.T.);
#70487=ORIENTED_EDGE('',*,*,#50312,.F.);
#70488=ORIENTED_EDGE('',*,*,#50446,.T.);
#70489=ORIENTED_EDGE('',*,*,#50428,.F.);
#70490=ORIENTED_EDGE('',*,*,#50447,.T.);
#70491=ORIENTED_EDGE('',*,*,#50294,.F.);
#70492=ORIENTED_EDGE('',*,*,#50448,.T.);
#70493=ORIENTED_EDGE('',*,*,#50449,.T.);
#70494=ORIENTED_EDGE('',*,*,#50185,.F.);
#70495=ORIENTED_EDGE('',*,*,#50450,.T.);
#70496=ORIENTED_EDGE('',*,*,#50451,.T.);
#70497=ORIENTED_EDGE('',*,*,#50452,.T.);
#70498=ORIENTED_EDGE('',*,*,#50453,.T.);
#70499=ORIENTED_EDGE('',*,*,#50264,.F.);
#70500=ORIENTED_EDGE('',*,*,#50454,.T.);
#70501=ORIENTED_EDGE('',*,*,#50455,.T.);
#70502=ORIENTED_EDGE('',*,*,#50456,.T.);
#70503=ORIENTED_EDGE('',*,*,#50208,.F.);
#70504=ORIENTED_EDGE('',*,*,#50457,.T.);
#70505=ORIENTED_EDGE('',*,*,#50458,.T.);
#70506=ORIENTED_EDGE('',*,*,#50459,.T.);
#70507=ORIENTED_EDGE('',*,*,#50202,.F.);
#70508=ORIENTED_EDGE('',*,*,#50460,.T.);
#70509=ORIENTED_EDGE('',*,*,#50461,.T.);
#70510=ORIENTED_EDGE('',*,*,#50462,.T.);
#70511=ORIENTED_EDGE('',*,*,#50198,.F.);
#70512=ORIENTED_EDGE('',*,*,#50463,.T.);
#70513=ORIENTED_EDGE('',*,*,#50464,.T.);
#70514=ORIENTED_EDGE('',*,*,#50465,.T.);
#70515=ORIENTED_EDGE('',*,*,#50192,.F.);
#70516=ORIENTED_EDGE('',*,*,#50466,.T.);
#70517=ORIENTED_EDGE('',*,*,#50467,.T.);
#70518=ORIENTED_EDGE('',*,*,#50468,.T.);
#70519=ORIENTED_EDGE('',*,*,#50180,.F.);
#70520=ORIENTED_EDGE('',*,*,#50469,.T.);
#70521=ORIENTED_EDGE('',*,*,#50470,.T.);
#70522=ORIENTED_EDGE('',*,*,#50471,.T.);
#70523=ORIENTED_EDGE('',*,*,#50242,.F.);
#70524=ORIENTED_EDGE('',*,*,#50472,.T.);
#70525=ORIENTED_EDGE('',*,*,#50473,.T.);
#70526=ORIENTED_EDGE('',*,*,#50474,.T.);
#70527=ORIENTED_EDGE('',*,*,#50224,.F.);
#70528=ORIENTED_EDGE('',*,*,#50475,.T.);
#70529=ORIENTED_EDGE('',*,*,#50476,.T.);
#70530=ORIENTED_EDGE('',*,*,#49890,.F.);
#70531=ORIENTED_EDGE('',*,*,#50477,.T.);
#70532=ORIENTED_EDGE('',*,*,#50478,.T.);
#70533=ORIENTED_EDGE('',*,*,#50479,.T.);
#70534=ORIENTED_EDGE('',*,*,#50480,.T.);
#70535=ORIENTED_EDGE('',*,*,#49767,.F.);
#70536=ORIENTED_EDGE('',*,*,#50481,.T.);
#70537=ORIENTED_EDGE('',*,*,#50482,.T.);
#70538=ORIENTED_EDGE('',*,*,#50483,.T.);
#70539=ORIENTED_EDGE('',*,*,#49743,.F.);
#70540=ORIENTED_EDGE('',*,*,#50484,.T.);
#70541=ORIENTED_EDGE('',*,*,#50485,.T.);
#70542=ORIENTED_EDGE('',*,*,#50486,.T.);
#70543=ORIENTED_EDGE('',*,*,#49751,.F.);
#70544=ORIENTED_EDGE('',*,*,#50487,.T.);
#70545=ORIENTED_EDGE('',*,*,#50488,.T.);
#70546=ORIENTED_EDGE('',*,*,#50489,.T.);
#70547=ORIENTED_EDGE('',*,*,#49763,.F.);
#70548=ORIENTED_EDGE('',*,*,#50490,.T.);
#70549=ORIENTED_EDGE('',*,*,#50491,.T.);
#70550=ORIENTED_EDGE('',*,*,#50492,.T.);
#70551=ORIENTED_EDGE('',*,*,#49713,.F.);
#70552=ORIENTED_EDGE('',*,*,#50493,.T.);
#70553=ORIENTED_EDGE('',*,*,#50494,.T.);
#70554=ORIENTED_EDGE('',*,*,#50495,.T.);
#70555=ORIENTED_EDGE('',*,*,#49721,.F.);
#70556=ORIENTED_EDGE('',*,*,#50496,.T.);
#70557=ORIENTED_EDGE('',*,*,#50497,.T.);
#70558=ORIENTED_EDGE('',*,*,#50498,.T.);
#70559=ORIENTED_EDGE('',*,*,#49733,.F.);
#70560=ORIENTED_EDGE('',*,*,#50499,.T.);
#70561=ORIENTED_EDGE('',*,*,#50500,.T.);
#70562=ORIENTED_EDGE('',*,*,#50501,.T.);
#70563=ORIENTED_EDGE('',*,*,#49737,.F.);
#70564=ORIENTED_EDGE('',*,*,#50502,.T.);
#70565=ORIENTED_EDGE('',*,*,#50503,.T.);
#70566=ORIENTED_EDGE('',*,*,#50504,.T.);
#70567=ORIENTED_EDGE('',*,*,#49510,.F.);
#70568=ORIENTED_EDGE('',*,*,#50505,.T.);
#70569=ORIENTED_EDGE('',*,*,#50506,.T.);
#70570=ORIENTED_EDGE('',*,*,#50507,.T.);
#70571=ORIENTED_EDGE('',*,*,#49500,.F.);
#70572=ORIENTED_EDGE('',*,*,#50508,.T.);
#70573=ORIENTED_EDGE('',*,*,#50509,.T.);
#70574=ORIENTED_EDGE('',*,*,#50510,.T.);
#70575=ORIENTED_EDGE('',*,*,#49488,.F.);
#70576=ORIENTED_EDGE('',*,*,#50511,.T.);
#70577=ORIENTED_EDGE('',*,*,#50512,.T.);
#70578=ORIENTED_EDGE('',*,*,#50513,.T.);
#70579=ORIENTED_EDGE('',*,*,#49496,.F.);
#70580=ORIENTED_EDGE('',*,*,#50514,.T.);
#70581=ORIENTED_EDGE('',*,*,#50515,.T.);
#70582=ORIENTED_EDGE('',*,*,#50516,.T.);
#70583=ORIENTED_EDGE('',*,*,#49881,.F.);
#70584=ORIENTED_EDGE('',*,*,#50517,.T.);
#70585=ORIENTED_EDGE('',*,*,#50518,.T.);
#70586=ORIENTED_EDGE('',*,*,#50519,.T.);
#70587=ORIENTED_EDGE('',*,*,#49869,.F.);
#70588=ORIENTED_EDGE('',*,*,#50520,.T.);
#70589=ORIENTED_EDGE('',*,*,#50521,.T.);
#70590=ORIENTED_EDGE('',*,*,#50522,.T.);
#70591=ORIENTED_EDGE('',*,*,#49877,.F.);
#70592=ORIENTED_EDGE('',*,*,#50523,.T.);
#70593=ORIENTED_EDGE('',*,*,#50524,.T.);
#70594=ORIENTED_EDGE('',*,*,#50525,.T.);
#70595=ORIENTED_EDGE('',*,*,#50126,.F.);
#70596=ORIENTED_EDGE('',*,*,#50526,.T.);
#70597=ORIENTED_EDGE('',*,*,#50527,.T.);
#70598=ORIENTED_EDGE('',*,*,#50528,.T.);
#70599=ORIENTED_EDGE('',*,*,#50130,.F.);
#70600=ORIENTED_EDGE('',*,*,#50529,.T.);
#70601=ORIENTED_EDGE('',*,*,#50530,.T.);
#70602=ORIENTED_EDGE('',*,*,#50117,.F.);
#70603=ORIENTED_EDGE('',*,*,#50531,.T.);
#70604=ORIENTED_EDGE('',*,*,#50532,.T.);
#70605=ORIENTED_EDGE('',*,*,#50533,.T.);
#70606=ORIENTED_EDGE('',*,*,#50534,.T.);
#70607=ORIENTED_EDGE('',*,*,#49575,.F.);
#70608=ORIENTED_EDGE('',*,*,#50535,.T.);
#70609=ORIENTED_EDGE('',*,*,#50536,.T.);
#70610=ORIENTED_EDGE('',*,*,#50537,.T.);
#70611=ORIENTED_EDGE('',*,*,#49563,.F.);
#70612=ORIENTED_EDGE('',*,*,#50538,.T.);
#70613=ORIENTED_EDGE('',*,*,#50539,.T.);
#70614=ORIENTED_EDGE('',*,*,#50540,.T.);
#70615=ORIENTED_EDGE('',*,*,#49571,.F.);
#70616=ORIENTED_EDGE('',*,*,#50541,.T.);
#70617=ORIENTED_EDGE('',*,*,#50542,.T.);
#70618=ORIENTED_EDGE('',*,*,#50543,.T.);
#70619=ORIENTED_EDGE('',*,*,#49583,.F.);
#70620=ORIENTED_EDGE('',*,*,#50544,.T.);
#70621=ORIENTED_EDGE('',*,*,#50545,.T.);
#70622=ORIENTED_EDGE('',*,*,#50546,.T.);
#70623=ORIENTED_EDGE('',*,*,#49599,.F.);
#70624=ORIENTED_EDGE('',*,*,#50547,.T.);
#70625=ORIENTED_EDGE('',*,*,#50548,.T.);
#70626=ORIENTED_EDGE('',*,*,#50549,.T.);
#70627=ORIENTED_EDGE('',*,*,#49587,.F.);
#70628=ORIENTED_EDGE('',*,*,#50550,.T.);
#70629=ORIENTED_EDGE('',*,*,#50551,.T.);
#70630=ORIENTED_EDGE('',*,*,#50552,.T.);
#70631=ORIENTED_EDGE('',*,*,#49595,.F.);
#70632=ORIENTED_EDGE('',*,*,#50553,.T.);
#70633=ORIENTED_EDGE('',*,*,#50554,.T.);
#70634=ORIENTED_EDGE('',*,*,#50555,.T.);
#70635=ORIENTED_EDGE('',*,*,#49607,.F.);
#70636=ORIENTED_EDGE('',*,*,#50556,.T.);
#70637=ORIENTED_EDGE('',*,*,#50557,.T.);
#70638=ORIENTED_EDGE('',*,*,#50558,.T.);
#70639=ORIENTED_EDGE('',*,*,#49974,.F.);
#70640=ORIENTED_EDGE('',*,*,#50559,.T.);
#70641=ORIENTED_EDGE('',*,*,#50560,.T.);
#70642=ORIENTED_EDGE('',*,*,#50561,.T.);
#70643=ORIENTED_EDGE('',*,*,#49982,.F.);
#70644=ORIENTED_EDGE('',*,*,#50562,.T.);
#70645=ORIENTED_EDGE('',*,*,#50563,.T.);
#70646=ORIENTED_EDGE('',*,*,#50564,.T.);
#70647=ORIENTED_EDGE('',*,*,#49994,.F.);
#70648=ORIENTED_EDGE('',*,*,#50565,.T.);
#70649=ORIENTED_EDGE('',*,*,#50566,.T.);
#70650=ORIENTED_EDGE('',*,*,#50567,.T.);
#70651=ORIENTED_EDGE('',*,*,#49986,.F.);
#70652=ORIENTED_EDGE('',*,*,#50568,.T.);
#70653=ORIENTED_EDGE('',*,*,#50569,.T.);
#70654=ORIENTED_EDGE('',*,*,#50570,.T.);
#70655=ORIENTED_EDGE('',*,*,#49920,.F.);
#70656=ORIENTED_EDGE('',*,*,#50571,.T.);
#70657=ORIENTED_EDGE('',*,*,#50572,.T.);
#70658=ORIENTED_EDGE('',*,*,#50573,.T.);
#70659=ORIENTED_EDGE('',*,*,#49928,.F.);
#70660=ORIENTED_EDGE('',*,*,#50574,.T.);
#70661=ORIENTED_EDGE('',*,*,#50575,.T.);
#70662=ORIENTED_EDGE('',*,*,#50576,.T.);
#70663=ORIENTED_EDGE('',*,*,#49944,.F.);
#70664=ORIENTED_EDGE('',*,*,#50577,.T.);
#70665=ORIENTED_EDGE('',*,*,#50578,.T.);
#70666=ORIENTED_EDGE('',*,*,#50579,.T.);
#70667=ORIENTED_EDGE('',*,*,#49932,.F.);
#70668=ORIENTED_EDGE('',*,*,#50580,.T.);
#70669=ORIENTED_EDGE('',*,*,#50581,.T.);
#70670=ORIENTED_EDGE('',*,*,#50582,.T.);
#70671=ORIENTED_EDGE('',*,*,#49701,.F.);
#70672=ORIENTED_EDGE('',*,*,#50583,.T.);
#70673=ORIENTED_EDGE('',*,*,#50584,.T.);
#70674=ORIENTED_EDGE('',*,*,#50585,.T.);
#70675=ORIENTED_EDGE('',*,*,#49689,.F.);
#70676=ORIENTED_EDGE('',*,*,#50586,.T.);
#70677=ORIENTED_EDGE('',*,*,#50587,.T.);
#70678=ORIENTED_EDGE('',*,*,#50588,.T.);
#70679=ORIENTED_EDGE('',*,*,#49697,.F.);
#70680=ORIENTED_EDGE('',*,*,#50589,.T.);
#70681=ORIENTED_EDGE('',*,*,#50590,.T.);
#70682=ORIENTED_EDGE('',*,*,#50591,.T.);
#70683=ORIENTED_EDGE('',*,*,#49709,.F.);
#70684=ORIENTED_EDGE('',*,*,#50592,.T.);
#70685=ORIENTED_EDGE('',*,*,#50593,.T.);
#70686=ORIENTED_EDGE('',*,*,#50594,.T.);
#70687=ORIENTED_EDGE('',*,*,#49793,.F.);
#70688=ORIENTED_EDGE('',*,*,#50595,.T.);
#70689=ORIENTED_EDGE('',*,*,#50596,.T.);
#70690=ORIENTED_EDGE('',*,*,#50597,.T.);
#70691=ORIENTED_EDGE('',*,*,#49785,.F.);
#70692=ORIENTED_EDGE('',*,*,#50598,.T.);
#70693=ORIENTED_EDGE('',*,*,#50599,.T.);
#70694=ORIENTED_EDGE('',*,*,#50600,.T.);
#70695=ORIENTED_EDGE('',*,*,#49773,.F.);
#70696=ORIENTED_EDGE('',*,*,#50601,.T.);
#70697=ORIENTED_EDGE('',*,*,#50602,.T.);
#70698=ORIENTED_EDGE('',*,*,#50603,.T.);
#70699=ORIENTED_EDGE('',*,*,#49781,.F.);
#70700=ORIENTED_EDGE('',*,*,#50604,.T.);
#70701=ORIENTED_EDGE('',*,*,#50605,.T.);
#70702=ORIENTED_EDGE('',*,*,#50606,.T.);
#70703=ORIENTED_EDGE('',*,*,#49821,.F.);
#70704=ORIENTED_EDGE('',*,*,#50607,.T.);
#70705=ORIENTED_EDGE('',*,*,#50608,.T.);
#70706=ORIENTED_EDGE('',*,*,#50609,.T.);
#70707=ORIENTED_EDGE('',*,*,#49829,.F.);
#70708=ORIENTED_EDGE('',*,*,#50610,.T.);
#70709=ORIENTED_EDGE('',*,*,#50611,.T.);
#70710=ORIENTED_EDGE('',*,*,#50612,.T.);
#70711=ORIENTED_EDGE('',*,*,#49841,.F.);
#70712=ORIENTED_EDGE('',*,*,#50613,.T.);
#70713=ORIENTED_EDGE('',*,*,#50614,.T.);
#70714=ORIENTED_EDGE('',*,*,#50615,.T.);
#70715=ORIENTED_EDGE('',*,*,#49833,.F.);
#70716=ORIENTED_EDGE('',*,*,#50616,.T.);
#70717=ORIENTED_EDGE('',*,*,#50617,.T.);
#70718=ORIENTED_EDGE('',*,*,#50618,.T.);
#70719=ORIENTED_EDGE('',*,*,#50108,.F.);
#70720=ORIENTED_EDGE('',*,*,#50619,.T.);
#70721=ORIENTED_EDGE('',*,*,#50620,.T.);
#70722=ORIENTED_EDGE('',*,*,#50621,.T.);
#70723=ORIENTED_EDGE('',*,*,#50112,.F.);
#70724=ORIENTED_EDGE('',*,*,#50622,.T.);
#70725=ORIENTED_EDGE('',*,*,#50623,.T.);
#70726=ORIENTED_EDGE('',*,*,#50624,.T.);
#70727=ORIENTED_EDGE('',*,*,#50100,.F.);
#70728=ORIENTED_EDGE('',*,*,#50625,.T.);
#70729=ORIENTED_EDGE('',*,*,#50626,.T.);
#70730=ORIENTED_EDGE('',*,*,#50627,.T.);
#70731=ORIENTED_EDGE('',*,*,#49958,.F.);
#70732=ORIENTED_EDGE('',*,*,#50628,.T.);
#70733=ORIENTED_EDGE('',*,*,#50629,.T.);
#70734=ORIENTED_EDGE('',*,*,#50630,.T.);
#70735=ORIENTED_EDGE('',*,*,#49970,.F.);
#70736=ORIENTED_EDGE('',*,*,#50631,.T.);
#70737=ORIENTED_EDGE('',*,*,#50632,.T.);
#70738=ORIENTED_EDGE('',*,*,#50633,.T.);
#70739=ORIENTED_EDGE('',*,*,#49962,.F.);
#70740=ORIENTED_EDGE('',*,*,#50634,.T.);
#70741=ORIENTED_EDGE('',*,*,#50635,.T.);
#70742=ORIENTED_EDGE('',*,*,#50636,.T.);
#70743=ORIENTED_EDGE('',*,*,#49950,.F.);
#70744=ORIENTED_EDGE('',*,*,#50637,.T.);
#70745=ORIENTED_EDGE('',*,*,#50638,.T.);
#70746=ORIENTED_EDGE('',*,*,#50639,.T.);
#70747=ORIENTED_EDGE('',*,*,#49908,.F.);
#70748=ORIENTED_EDGE('',*,*,#50640,.T.);
#70749=ORIENTED_EDGE('',*,*,#50641,.T.);
#70750=ORIENTED_EDGE('',*,*,#50642,.T.);
#70751=ORIENTED_EDGE('',*,*,#49896,.F.);
#70752=ORIENTED_EDGE('',*,*,#50643,.T.);
#70753=ORIENTED_EDGE('',*,*,#50644,.T.);
#70754=ORIENTED_EDGE('',*,*,#50645,.T.);
#70755=ORIENTED_EDGE('',*,*,#49904,.F.);
#70756=ORIENTED_EDGE('',*,*,#50646,.T.);
#70757=ORIENTED_EDGE('',*,*,#50647,.T.);
#70758=ORIENTED_EDGE('',*,*,#50648,.T.);
#70759=ORIENTED_EDGE('',*,*,#49916,.F.);
#70760=ORIENTED_EDGE('',*,*,#50649,.T.);
#70761=ORIENTED_EDGE('',*,*,#50650,.T.);
#70762=ORIENTED_EDGE('',*,*,#50651,.T.);
#70763=ORIENTED_EDGE('',*,*,#49809,.F.);
#70764=ORIENTED_EDGE('',*,*,#50652,.T.);
#70765=ORIENTED_EDGE('',*,*,#50653,.T.);
#70766=ORIENTED_EDGE('',*,*,#50654,.T.);
#70767=ORIENTED_EDGE('',*,*,#49797,.F.);
#70768=ORIENTED_EDGE('',*,*,#50655,.T.);
#70769=ORIENTED_EDGE('',*,*,#50656,.T.);
#70770=ORIENTED_EDGE('',*,*,#50657,.T.);
#70771=ORIENTED_EDGE('',*,*,#49805,.F.);
#70772=ORIENTED_EDGE('',*,*,#50658,.T.);
#70773=ORIENTED_EDGE('',*,*,#50659,.T.);
#70774=ORIENTED_EDGE('',*,*,#50660,.T.);
#70775=ORIENTED_EDGE('',*,*,#49817,.F.);
#70776=ORIENTED_EDGE('',*,*,#50661,.T.);
#70777=ORIENTED_EDGE('',*,*,#50662,.T.);
#70778=ORIENTED_EDGE('',*,*,#50663,.T.);
#70779=ORIENTED_EDGE('',*,*,#49665,.F.);
#70780=ORIENTED_EDGE('',*,*,#50664,.T.);
#70781=ORIENTED_EDGE('',*,*,#50665,.T.);
#70782=ORIENTED_EDGE('',*,*,#50666,.T.);
#70783=ORIENTED_EDGE('',*,*,#49673,.F.);
#70784=ORIENTED_EDGE('',*,*,#50667,.T.);
#70785=ORIENTED_EDGE('',*,*,#50668,.T.);
#70786=ORIENTED_EDGE('',*,*,#50669,.T.);
#70787=ORIENTED_EDGE('',*,*,#49685,.F.);
#70788=ORIENTED_EDGE('',*,*,#50670,.T.);
#70789=ORIENTED_EDGE('',*,*,#50671,.T.);
#70790=ORIENTED_EDGE('',*,*,#50672,.T.);
#70791=ORIENTED_EDGE('',*,*,#49677,.F.);
#70792=ORIENTED_EDGE('',*,*,#50673,.T.);
#70793=ORIENTED_EDGE('',*,*,#50674,.T.);
#70794=ORIENTED_EDGE('',*,*,#50675,.T.);
#70795=ORIENTED_EDGE('',*,*,#49611,.F.);
#70796=ORIENTED_EDGE('',*,*,#50676,.T.);
#70797=ORIENTED_EDGE('',*,*,#50677,.T.);
#70798=ORIENTED_EDGE('',*,*,#50678,.T.);
#70799=ORIENTED_EDGE('',*,*,#49619,.F.);
#70800=ORIENTED_EDGE('',*,*,#50679,.T.);
#70801=ORIENTED_EDGE('',*,*,#50680,.T.);
#70802=ORIENTED_EDGE('',*,*,#50681,.T.);
#70803=ORIENTED_EDGE('',*,*,#49631,.F.);
#70804=ORIENTED_EDGE('',*,*,#50682,.T.);
#70805=ORIENTED_EDGE('',*,*,#50683,.T.);
#70806=ORIENTED_EDGE('',*,*,#50684,.T.);
#70807=ORIENTED_EDGE('',*,*,#49623,.F.);
#70808=ORIENTED_EDGE('',*,*,#50685,.T.);
#70809=ORIENTED_EDGE('',*,*,#50686,.T.);
#70810=ORIENTED_EDGE('',*,*,#50687,.T.);
#70811=ORIENTED_EDGE('',*,*,#49635,.F.);
#70812=ORIENTED_EDGE('',*,*,#50688,.T.);
#70813=ORIENTED_EDGE('',*,*,#50689,.T.);
#70814=ORIENTED_EDGE('',*,*,#50690,.T.);
#70815=ORIENTED_EDGE('',*,*,#49643,.F.);
#70816=ORIENTED_EDGE('',*,*,#50691,.T.);
#70817=ORIENTED_EDGE('',*,*,#50692,.T.);
#70818=ORIENTED_EDGE('',*,*,#50693,.T.);
#70819=ORIENTED_EDGE('',*,*,#49655,.F.);
#70820=ORIENTED_EDGE('',*,*,#50694,.T.);
#70821=ORIENTED_EDGE('',*,*,#50695,.T.);
#70822=ORIENTED_EDGE('',*,*,#50696,.T.);
#70823=ORIENTED_EDGE('',*,*,#49647,.F.);
#70824=ORIENTED_EDGE('',*,*,#50697,.T.);
#70825=ORIENTED_EDGE('',*,*,#50698,.T.);
#70826=ORIENTED_EDGE('',*,*,#50699,.T.);
#70827=ORIENTED_EDGE('',*,*,#49406,.F.);
#70828=ORIENTED_EDGE('',*,*,#50700,.T.);
#70829=ORIENTED_EDGE('',*,*,#50701,.T.);
#70830=ORIENTED_EDGE('',*,*,#50702,.T.);
#70831=ORIENTED_EDGE('',*,*,#49410,.F.);
#70832=ORIENTED_EDGE('',*,*,#50703,.T.);
#70833=ORIENTED_EDGE('',*,*,#50704,.T.);
#70834=ORIENTED_EDGE('',*,*,#49385,.F.);
#70835=ORIENTED_EDGE('',*,*,#50705,.T.);
#70836=ORIENTED_EDGE('',*,*,#50706,.T.);
#70837=ORIENTED_EDGE('',*,*,#50707,.T.);
#70838=ORIENTED_EDGE('',*,*,#50708,.T.);
#70839=ORIENTED_EDGE('',*,*,#49394,.F.);
#70840=ORIENTED_EDGE('',*,*,#50709,.T.);
#70841=ORIENTED_EDGE('',*,*,#50710,.T.);
#70842=ORIENTED_EDGE('',*,*,#50711,.T.);
#70843=ORIENTED_EDGE('',*,*,#50016,.F.);
#70844=ORIENTED_EDGE('',*,*,#50712,.T.);
#70845=ORIENTED_EDGE('',*,*,#50713,.T.);
#70846=ORIENTED_EDGE('',*,*,#50714,.T.);
#70847=ORIENTED_EDGE('',*,*,#50004,.F.);
#70848=ORIENTED_EDGE('',*,*,#50715,.T.);
#70849=ORIENTED_EDGE('',*,*,#50716,.T.);
#70850=ORIENTED_EDGE('',*,*,#50717,.T.);
#70851=ORIENTED_EDGE('',*,*,#50012,.F.);
#70852=ORIENTED_EDGE('',*,*,#50718,.T.);
#70853=ORIENTED_EDGE('',*,*,#50719,.T.);
#70854=ORIENTED_EDGE('',*,*,#50720,.T.);
#70855=ORIENTED_EDGE('',*,*,#50024,.F.);
#70856=ORIENTED_EDGE('',*,*,#50721,.T.);
#70857=ORIENTED_EDGE('',*,*,#50722,.T.);
#70858=ORIENTED_EDGE('',*,*,#50723,.T.);
#70859=ORIENTED_EDGE('',*,*,#49551,.F.);
#70860=ORIENTED_EDGE('',*,*,#50724,.T.);
#70861=ORIENTED_EDGE('',*,*,#50725,.T.);
#70862=ORIENTED_EDGE('',*,*,#50726,.T.);
#70863=ORIENTED_EDGE('',*,*,#49539,.F.);
#70864=ORIENTED_EDGE('',*,*,#50727,.T.);
#70865=ORIENTED_EDGE('',*,*,#50728,.T.);
#70866=ORIENTED_EDGE('',*,*,#50729,.T.);
#70867=ORIENTED_EDGE('',*,*,#49547,.F.);
#70868=ORIENTED_EDGE('',*,*,#50730,.T.);
#70869=ORIENTED_EDGE('',*,*,#50731,.T.);
#70870=ORIENTED_EDGE('',*,*,#50732,.T.);
#70871=ORIENTED_EDGE('',*,*,#49559,.F.);
#70872=ORIENTED_EDGE('',*,*,#50733,.T.);
#70873=ORIENTED_EDGE('',*,*,#50734,.T.);
#70874=ORIENTED_EDGE('',*,*,#50735,.T.);
#70875=ORIENTED_EDGE('',*,*,#49527,.F.);
#70876=ORIENTED_EDGE('',*,*,#50736,.T.);
#70877=ORIENTED_EDGE('',*,*,#50737,.T.);
#70878=ORIENTED_EDGE('',*,*,#50738,.T.);
#70879=ORIENTED_EDGE('',*,*,#49515,.F.);
#70880=ORIENTED_EDGE('',*,*,#50739,.T.);
#70881=ORIENTED_EDGE('',*,*,#50740,.T.);
#70882=ORIENTED_EDGE('',*,*,#50741,.T.);
#70883=ORIENTED_EDGE('',*,*,#49523,.F.);
#70884=ORIENTED_EDGE('',*,*,#50742,.T.);
#70885=ORIENTED_EDGE('',*,*,#50743,.T.);
#70886=ORIENTED_EDGE('',*,*,#50744,.T.);
#70887=ORIENTED_EDGE('',*,*,#49535,.F.);
#70888=ORIENTED_EDGE('',*,*,#50745,.T.);
#70889=ORIENTED_EDGE('',*,*,#50746,.T.);
#70890=ORIENTED_EDGE('',*,*,#50747,.T.);
#70891=ORIENTED_EDGE('',*,*,#49845,.F.);
#70892=ORIENTED_EDGE('',*,*,#50748,.T.);
#70893=ORIENTED_EDGE('',*,*,#50749,.T.);
#70894=ORIENTED_EDGE('',*,*,#50750,.T.);
#70895=ORIENTED_EDGE('',*,*,#49853,.F.);
#70896=ORIENTED_EDGE('',*,*,#50751,.T.);
#70897=ORIENTED_EDGE('',*,*,#50752,.T.);
#70898=ORIENTED_EDGE('',*,*,#50753,.T.);
#70899=ORIENTED_EDGE('',*,*,#49865,.F.);
#70900=ORIENTED_EDGE('',*,*,#50754,.T.);
#70901=ORIENTED_EDGE('',*,*,#50755,.T.);
#70902=ORIENTED_EDGE('',*,*,#50756,.T.);
#70903=ORIENTED_EDGE('',*,*,#49857,.F.);
#70904=ORIENTED_EDGE('',*,*,#50757,.T.);
#70905=ORIENTED_EDGE('',*,*,#50758,.T.);
#70906=ORIENTED_EDGE('',*,*,#50759,.T.);
#70907=ORIENTED_EDGE('',*,*,#50036,.F.);
#70908=ORIENTED_EDGE('',*,*,#50760,.T.);
#70909=ORIENTED_EDGE('',*,*,#50761,.T.);
#70910=ORIENTED_EDGE('',*,*,#50762,.T.);
#70911=ORIENTED_EDGE('',*,*,#50048,.F.);
#70912=ORIENTED_EDGE('',*,*,#50763,.T.);
#70913=ORIENTED_EDGE('',*,*,#50764,.T.);
#70914=ORIENTED_EDGE('',*,*,#50765,.T.);
#70915=ORIENTED_EDGE('',*,*,#50040,.F.);
#70916=ORIENTED_EDGE('',*,*,#50766,.T.);
#70917=ORIENTED_EDGE('',*,*,#50767,.T.);
#70918=ORIENTED_EDGE('',*,*,#50768,.T.);
#70919=ORIENTED_EDGE('',*,*,#50028,.F.);
#70920=ORIENTED_EDGE('',*,*,#50769,.T.);
#70921=ORIENTED_EDGE('',*,*,#50770,.T.);
#70922=ORIENTED_EDGE('',*,*,#50771,.T.);
#70923=ORIENTED_EDGE('',*,*,#49436,.F.);
#70924=ORIENTED_EDGE('',*,*,#50772,.T.);
#70925=ORIENTED_EDGE('',*,*,#50773,.T.);
#70926=ORIENTED_EDGE('',*,*,#50774,.T.);
#70927=ORIENTED_EDGE('',*,*,#49428,.F.);
#70928=ORIENTED_EDGE('',*,*,#50775,.T.);
#70929=ORIENTED_EDGE('',*,*,#50776,.T.);
#70930=ORIENTED_EDGE('',*,*,#49415,.F.);
#70931=ORIENTED_EDGE('',*,*,#50777,.T.);
#70932=ORIENTED_EDGE('',*,*,#50778,.T.);
#70933=ORIENTED_EDGE('',*,*,#50779,.T.);
#70934=ORIENTED_EDGE('',*,*,#50780,.T.);
#70935=ORIENTED_EDGE('',*,*,#49424,.F.);
#70936=ORIENTED_EDGE('',*,*,#50781,.T.);
#70937=ORIENTED_EDGE('',*,*,#50782,.T.);
#70938=ORIENTED_EDGE('',*,*,#50783,.T.);
#70939=ORIENTED_EDGE('',*,*,#50064,.F.);
#70940=ORIENTED_EDGE('',*,*,#50784,.T.);
#70941=ORIENTED_EDGE('',*,*,#50785,.T.);
#70942=ORIENTED_EDGE('',*,*,#50786,.T.);
#70943=ORIENTED_EDGE('',*,*,#50052,.F.);
#70944=ORIENTED_EDGE('',*,*,#50787,.T.);
#70945=ORIENTED_EDGE('',*,*,#50788,.T.);
#70946=ORIENTED_EDGE('',*,*,#50789,.T.);
#70947=ORIENTED_EDGE('',*,*,#50060,.F.);
#70948=ORIENTED_EDGE('',*,*,#50790,.T.);
#70949=ORIENTED_EDGE('',*,*,#50791,.T.);
#70950=ORIENTED_EDGE('',*,*,#50792,.T.);
#70951=ORIENTED_EDGE('',*,*,#50072,.F.);
#70952=ORIENTED_EDGE('',*,*,#50793,.T.);
#70953=ORIENTED_EDGE('',*,*,#50794,.T.);
#70954=ORIENTED_EDGE('',*,*,#50795,.T.);
#70955=ORIENTED_EDGE('',*,*,#49476,.F.);
#70956=ORIENTED_EDGE('',*,*,#50796,.T.);
#70957=ORIENTED_EDGE('',*,*,#50797,.T.);
#70958=ORIENTED_EDGE('',*,*,#50798,.T.);
#70959=ORIENTED_EDGE('',*,*,#49464,.F.);
#70960=ORIENTED_EDGE('',*,*,#50799,.T.);
#70961=ORIENTED_EDGE('',*,*,#50800,.T.);
#70962=ORIENTED_EDGE('',*,*,#50801,.T.);
#70963=ORIENTED_EDGE('',*,*,#49472,.F.);
#70964=ORIENTED_EDGE('',*,*,#50802,.T.);
#70965=ORIENTED_EDGE('',*,*,#50803,.T.);
#70966=ORIENTED_EDGE('',*,*,#50804,.T.);
#70967=ORIENTED_EDGE('',*,*,#49484,.F.);
#70968=ORIENTED_EDGE('',*,*,#50805,.T.);
#70969=ORIENTED_EDGE('',*,*,#50806,.T.);
#70970=ORIENTED_EDGE('',*,*,#50807,.T.);
#70971=ORIENTED_EDGE('',*,*,#50084,.F.);
#70972=ORIENTED_EDGE('',*,*,#50808,.T.);
#70973=ORIENTED_EDGE('',*,*,#50809,.T.);
#70974=ORIENTED_EDGE('',*,*,#50810,.T.);
#70975=ORIENTED_EDGE('',*,*,#50096,.F.);
#70976=ORIENTED_EDGE('',*,*,#50811,.T.);
#70977=ORIENTED_EDGE('',*,*,#50812,.T.);
#70978=ORIENTED_EDGE('',*,*,#50813,.T.);
#70979=ORIENTED_EDGE('',*,*,#50088,.F.);
#70980=ORIENTED_EDGE('',*,*,#50814,.T.);
#70981=ORIENTED_EDGE('',*,*,#50815,.T.);
#70982=ORIENTED_EDGE('',*,*,#50816,.T.);
#70983=ORIENTED_EDGE('',*,*,#50076,.F.);
#70984=ORIENTED_EDGE('',*,*,#50817,.T.);
#70985=ORIENTED_EDGE('',*,*,#50818,.T.);
#70986=ORIENTED_EDGE('',*,*,#50819,.T.);
#70987=ORIENTED_EDGE('',*,*,#49460,.F.);
#70988=ORIENTED_EDGE('',*,*,#50820,.T.);
#70989=ORIENTED_EDGE('',*,*,#50821,.T.);
#70990=ORIENTED_EDGE('',*,*,#50822,.T.);
#70991=ORIENTED_EDGE('',*,*,#49452,.F.);
#70992=ORIENTED_EDGE('',*,*,#50823,.T.);
#70993=ORIENTED_EDGE('',*,*,#50824,.T.);
#70994=ORIENTED_EDGE('',*,*,#49439,.F.);
#70995=ORIENTED_EDGE('',*,*,#50825,.T.);
#70996=ORIENTED_EDGE('',*,*,#50826,.T.);
#70997=ORIENTED_EDGE('',*,*,#50827,.T.);
#70998=ORIENTED_EDGE('',*,*,#50828,.T.);
#70999=ORIENTED_EDGE('',*,*,#49448,.F.);
#71000=ORIENTED_EDGE('',*,*,#50829,.T.);
#71001=ORIENTED_EDGE('',*,*,#50830,.T.);
#71002=ORIENTED_EDGE('',*,*,#50831,.T.);
#71003=ORIENTED_EDGE('',*,*,#50214,.F.);
#71004=ORIENTED_EDGE('',*,*,#50832,.T.);
#71005=ORIENTED_EDGE('',*,*,#50833,.T.);
#71006=ORIENTED_EDGE('',*,*,#50834,.T.);
#71007=ORIENTED_EDGE('',*,*,#50252,.F.);
#71008=ORIENTED_EDGE('',*,*,#50835,.T.);
#71009=ORIENTED_EDGE('',*,*,#50836,.T.);
#71010=ORIENTED_EDGE('',*,*,#50837,.T.);
#71011=ORIENTED_EDGE('',*,*,#50236,.F.);
#71012=ORIENTED_EDGE('',*,*,#50838,.T.);
#71013=ORIENTED_EDGE('',*,*,#50839,.T.);
#71014=ORIENTED_EDGE('',*,*,#50229,.F.);
#71015=ORIENTED_EDGE('',*,*,#50840,.T.);
#71016=ORIENTED_EDGE('',*,*,#50841,.T.);
#71017=ORIENTED_EDGE('',*,*,#50842,.T.);
#71018=ORIENTED_EDGE('',*,*,#50843,.T.);
#71019=ORIENTED_EDGE('',*,*,#50258,.F.);
#71020=ORIENTED_EDGE('',*,*,#50844,.T.);
#71021=ORIENTED_EDGE('',*,*,#50845,.T.);
#71022=ORIENTED_EDGE('',*,*,#50244,.F.);
#71023=ORIENTED_EDGE('',*,*,#50846,.T.);
#71024=ORIENTED_EDGE('',*,*,#50847,.T.);
#71025=ORIENTED_EDGE('',*,*,#50848,.T.);
#71026=ORIENTED_EDGE('',*,*,#50849,.T.);
#71027=ORIENTED_EDGE('',*,*,#50220,.F.);
#71028=ORIENTED_EDGE('',*,*,#50850,.T.);
#71029=ORIENTED_EDGE('',*,*,#50851,.T.);
#71030=ORIENTED_EDGE('',*,*,#50852,.T.);
#71031=ORIENTED_EDGE('',*,*,#49725,.F.);
#71032=ORIENTED_EDGE('',*,*,#50853,.T.);
#71033=ORIENTED_EDGE('',*,*,#50854,.T.);
#71034=ORIENTED_EDGE('',*,*,#50855,.T.);
#71035=ORIENTED_EDGE('',*,*,#49755,.F.);
#71036=ORIENTED_EDGE('',*,*,#50856,.T.);
#71037=ORIENTED_EDGE('',*,*,#50857,.T.);
#71038=ORIENTED_EDGE('',*,*,#50477,.F.);
#71039=ORIENTED_EDGE('',*,*,#49891,.F.);
#71040=ORIENTED_EDGE('',*,*,#50504,.F.);
#71041=ORIENTED_EDGE('',*,*,#50858,.T.);
#71042=ORIENTED_EDGE('',*,*,#50859,.T.);
#71043=ORIENTED_EDGE('',*,*,#49508,.F.);
#71044=ORIENTED_EDGE('',*,*,#50516,.F.);
#71045=ORIENTED_EDGE('',*,*,#50860,.T.);
#71046=ORIENTED_EDGE('',*,*,#50856,.F.);
#71047=ORIENTED_EDGE('',*,*,#49887,.F.);
#71048=ORIENTED_EDGE('',*,*,#50859,.F.);
#71049=ORIENTED_EDGE('',*,*,#50861,.T.);
#71050=ORIENTED_EDGE('',*,*,#50511,.F.);
#71051=ORIENTED_EDGE('',*,*,#49502,.F.);
#71052=ORIENTED_EDGE('',*,*,#50834,.F.);
#71053=ORIENTED_EDGE('',*,*,#50862,.F.);
#71054=ORIENTED_EDGE('',*,*,#50841,.F.);
#71055=ORIENTED_EDGE('',*,*,#50255,.F.);
#71056=ORIENTED_EDGE('',*,*,#50845,.F.);
#71057=ORIENTED_EDGE('',*,*,#50863,.F.);
#71058=ORIENTED_EDGE('',*,*,#50832,.F.);
#71059=ORIENTED_EDGE('',*,*,#50249,.F.);
#71060=ORIENTED_EDGE('',*,*,#50831,.F.);
#71061=ORIENTED_EDGE('',*,*,#50864,.F.);
#71062=ORIENTED_EDGE('',*,*,#50847,.F.);
#71063=ORIENTED_EDGE('',*,*,#50217,.F.);
#71064=ORIENTED_EDGE('',*,*,#50456,.F.);
#71065=ORIENTED_EDGE('',*,*,#50865,.F.);
#71066=ORIENTED_EDGE('',*,*,#50829,.F.);
#71067=ORIENTED_EDGE('',*,*,#50211,.F.);
#71068=ORIENTED_EDGE('',*,*,#50855,.F.);
#71069=ORIENTED_EDGE('',*,*,#50866,.T.);
#71070=ORIENTED_EDGE('',*,*,#50478,.F.);
#71071=ORIENTED_EDGE('',*,*,#49761,.F.);
#71072=ORIENTED_EDGE('',*,*,#50839,.F.);
#71073=ORIENTED_EDGE('',*,*,#50867,.F.);
#71074=ORIENTED_EDGE('',*,*,#50835,.F.);
#71075=ORIENTED_EDGE('',*,*,#50233,.F.);
#71076=ORIENTED_EDGE('',*,*,#50837,.F.);
#71077=ORIENTED_EDGE('',*,*,#50868,.T.);
#71078=ORIENTED_EDGE('',*,*,#50469,.F.);
#71079=ORIENTED_EDGE('',*,*,#50239,.F.);
#71080=ORIENTED_EDGE('',*,*,#50468,.F.);
#71081=ORIENTED_EDGE('',*,*,#50869,.T.);
#71082=ORIENTED_EDGE('',*,*,#50450,.F.);
#71083=ORIENTED_EDGE('',*,*,#50183,.F.);
#71084=ORIENTED_EDGE('',*,*,#50449,.F.);
#71085=ORIENTED_EDGE('',*,*,#50870,.F.);
#71086=ORIENTED_EDGE('',*,*,#50463,.F.);
#71087=ORIENTED_EDGE('',*,*,#50189,.F.);
#71088=ORIENTED_EDGE('',*,*,#50492,.F.);
#71089=ORIENTED_EDGE('',*,*,#50871,.T.);
#71090=ORIENTED_EDGE('',*,*,#50850,.F.);
#71091=ORIENTED_EDGE('',*,*,#49719,.F.);
#71092=ORIENTED_EDGE('',*,*,#50534,.F.);
#71093=ORIENTED_EDGE('',*,*,#50872,.F.);
#71094=ORIENTED_EDGE('',*,*,#50541,.F.);
#71095=ORIENTED_EDGE('',*,*,#49581,.F.);
#71096=ORIENTED_EDGE('',*,*,#50690,.F.);
#71097=ORIENTED_EDGE('',*,*,#50873,.F.);
#71098=ORIENTED_EDGE('',*,*,#50685,.F.);
#71099=ORIENTED_EDGE('',*,*,#49637,.F.);
#71100=ORIENTED_EDGE('',*,*,#50678,.F.);
#71101=ORIENTED_EDGE('',*,*,#50874,.F.);
#71102=ORIENTED_EDGE('',*,*,#50673,.F.);
#71103=ORIENTED_EDGE('',*,*,#49613,.F.);
#71104=ORIENTED_EDGE('',*,*,#50546,.F.);
#71105=ORIENTED_EDGE('',*,*,#50875,.F.);
#71106=ORIENTED_EDGE('',*,*,#50553,.F.);
#71107=ORIENTED_EDGE('',*,*,#49605,.F.);
#71108=ORIENTED_EDGE('',*,*,#50666,.F.);
#71109=ORIENTED_EDGE('',*,*,#50876,.F.);
#71110=ORIENTED_EDGE('',*,*,#50661,.F.);
#71111=ORIENTED_EDGE('',*,*,#49667,.F.);
#71112=ORIENTED_EDGE('',*,*,#50582,.F.);
#71113=ORIENTED_EDGE('',*,*,#50877,.F.);
#71114=ORIENTED_EDGE('',*,*,#50589,.F.);
#71115=ORIENTED_EDGE('',*,*,#49707,.F.);
#71116=ORIENTED_EDGE('',*,*,#50654,.F.);
#71117=ORIENTED_EDGE('',*,*,#50878,.F.);
#71118=ORIENTED_EDGE('',*,*,#50649,.F.);
#71119=ORIENTED_EDGE('',*,*,#49803,.F.);
#71120=ORIENTED_EDGE('',*,*,#50594,.F.);
#71121=ORIENTED_EDGE('',*,*,#50879,.F.);
#71122=ORIENTED_EDGE('',*,*,#50601,.F.);
#71123=ORIENTED_EDGE('',*,*,#49787,.F.);
#71124=ORIENTED_EDGE('',*,*,#50570,.F.);
#71125=ORIENTED_EDGE('',*,*,#50880,.F.);
#71126=ORIENTED_EDGE('',*,*,#50577,.F.);
#71127=ORIENTED_EDGE('',*,*,#49926,.F.);
#71128=ORIENTED_EDGE('',*,*,#50630,.F.);
#71129=ORIENTED_EDGE('',*,*,#50881,.F.);
#71130=ORIENTED_EDGE('',*,*,#50625,.F.);
#71131=ORIENTED_EDGE('',*,*,#49964,.F.);
#71132=ORIENTED_EDGE('',*,*,#50642,.F.);
#71133=ORIENTED_EDGE('',*,*,#50882,.F.);
#71134=ORIENTED_EDGE('',*,*,#50637,.F.);
#71135=ORIENTED_EDGE('',*,*,#49902,.F.);
#71136=ORIENTED_EDGE('',*,*,#50606,.F.);
#71137=ORIENTED_EDGE('',*,*,#50883,.F.);
#71138=ORIENTED_EDGE('',*,*,#50613,.F.);
#71139=ORIENTED_EDGE('',*,*,#49827,.F.);
#71140=ORIENTED_EDGE('',*,*,#50621,.F.);
#71141=ORIENTED_EDGE('',*,*,#50884,.F.);
#71142=ORIENTED_EDGE('',*,*,#50616,.F.);
#71143=ORIENTED_EDGE('',*,*,#50114,.F.);
#71144=ORIENTED_EDGE('',*,*,#50558,.F.);
#71145=ORIENTED_EDGE('',*,*,#50885,.F.);
#71146=ORIENTED_EDGE('',*,*,#50565,.F.);
#71147=ORIENTED_EDGE('',*,*,#49980,.F.);
#71148=ORIENTED_EDGE('',*,*,#50525,.F.);
#71149=ORIENTED_EDGE('',*,*,#50886,.F.);
#71150=ORIENTED_EDGE('',*,*,#50531,.F.);
#71151=ORIENTED_EDGE('',*,*,#50120,.F.);
#71152=ORIENTED_EDGE('',*,*,#50702,.F.);
#71153=ORIENTED_EDGE('',*,*,#50887,.F.);
#71154=ORIENTED_EDGE('',*,*,#50697,.F.);
#71155=ORIENTED_EDGE('',*,*,#49412,.F.);
#71156=ORIENTED_EDGE('',*,*,#50774,.F.);
#71157=ORIENTED_EDGE('',*,*,#50888,.F.);
#71158=ORIENTED_EDGE('',*,*,#50769,.F.);
#71159=ORIENTED_EDGE('',*,*,#49434,.F.);
#71160=ORIENTED_EDGE('',*,*,#50708,.F.);
#71161=ORIENTED_EDGE('',*,*,#50889,.F.);
#71162=ORIENTED_EDGE('',*,*,#50705,.F.);
#71163=ORIENTED_EDGE('',*,*,#49388,.F.);
#71164=ORIENTED_EDGE('',*,*,#50540,.F.);
#71165=ORIENTED_EDGE('',*,*,#50890,.F.);
#71166=ORIENTED_EDGE('',*,*,#50535,.F.);
#71167=ORIENTED_EDGE('',*,*,#49565,.F.);
#71168=ORIENTED_EDGE('',*,*,#50723,.F.);
#71169=ORIENTED_EDGE('',*,*,#50891,.F.);
#71170=ORIENTED_EDGE('',*,*,#50730,.F.);
#71171=ORIENTED_EDGE('',*,*,#49557,.F.);
#71172=ORIENTED_EDGE('',*,*,#50564,.F.);
#71173=ORIENTED_EDGE('',*,*,#50892,.F.);
#71174=ORIENTED_EDGE('',*,*,#50559,.F.);
#71175=ORIENTED_EDGE('',*,*,#49988,.F.);
#71176=ORIENTED_EDGE('',*,*,#50714,.F.);
#71177=ORIENTED_EDGE('',*,*,#50893,.F.);
#71178=ORIENTED_EDGE('',*,*,#50709,.F.);
#71179=ORIENTED_EDGE('',*,*,#50010,.F.);
#71180=ORIENTED_EDGE('',*,*,#50552,.F.);
#71181=ORIENTED_EDGE('',*,*,#50894,.F.);
#71182=ORIENTED_EDGE('',*,*,#50547,.F.);
#71183=ORIENTED_EDGE('',*,*,#49589,.F.);
#71184=ORIENTED_EDGE('',*,*,#50735,.F.);
#71185=ORIENTED_EDGE('',*,*,#50895,.F.);
#71186=ORIENTED_EDGE('',*,*,#50742,.F.);
#71187=ORIENTED_EDGE('',*,*,#49533,.F.);
#71188=ORIENTED_EDGE('',*,*,#50588,.F.);
#71189=ORIENTED_EDGE('',*,*,#50896,.F.);
#71190=ORIENTED_EDGE('',*,*,#50583,.F.);
#71191=ORIENTED_EDGE('',*,*,#49691,.F.);
#71192=ORIENTED_EDGE('',*,*,#50498,.F.);
#71193=ORIENTED_EDGE('',*,*,#50897,.F.);
#71194=ORIENTED_EDGE('',*,*,#50493,.F.);
#71195=ORIENTED_EDGE('',*,*,#49727,.F.);
#71196=ORIENTED_EDGE('',*,*,#50600,.F.);
#71197=ORIENTED_EDGE('',*,*,#50898,.F.);
#71198=ORIENTED_EDGE('',*,*,#50595,.F.);
#71199=ORIENTED_EDGE('',*,*,#49779,.F.);
#71200=ORIENTED_EDGE('',*,*,#50489,.F.);
#71201=ORIENTED_EDGE('',*,*,#50899,.F.);
#71202=ORIENTED_EDGE('',*,*,#50484,.F.);
#71203=ORIENTED_EDGE('',*,*,#49757,.F.);
#71204=ORIENTED_EDGE('',*,*,#50636,.F.);
#71205=ORIENTED_EDGE('',*,*,#50900,.F.);
#71206=ORIENTED_EDGE('',*,*,#50631,.F.);
#71207=ORIENTED_EDGE('',*,*,#49956,.F.);
#71208=ORIENTED_EDGE('',*,*,#50762,.F.);
#71209=ORIENTED_EDGE('',*,*,#50901,.F.);
#71210=ORIENTED_EDGE('',*,*,#50757,.F.);
#71211=ORIENTED_EDGE('',*,*,#50042,.F.);
#71212=ORIENTED_EDGE('',*,*,#50612,.F.);
#71213=ORIENTED_EDGE('',*,*,#50902,.F.);
#71214=ORIENTED_EDGE('',*,*,#50607,.F.);
#71215=ORIENTED_EDGE('',*,*,#49835,.F.);
#71216=ORIENTED_EDGE('',*,*,#50747,.F.);
#71217=ORIENTED_EDGE('',*,*,#50903,.F.);
#71218=ORIENTED_EDGE('',*,*,#50754,.F.);
#71219=ORIENTED_EDGE('',*,*,#49851,.F.);
#71220=ORIENTED_EDGE('',*,*,#50904,.T.);
#71221=ORIENTED_EDGE('',*,*,#50905,.F.);
#71222=ORIENTED_EDGE('',*,*,#50906,.F.);
#71223=ORIENTED_EDGE('',*,*,#50907,.F.);
#71224=ORIENTED_EDGE('',*,*,#50908,.T.);
#71225=ORIENTED_EDGE('',*,*,#50909,.F.);
#71226=ORIENTED_EDGE('',*,*,#50904,.F.);
#71227=ORIENTED_EDGE('',*,*,#50910,.F.);
#71228=ORIENTED_EDGE('',*,*,#50906,.T.);
#71229=ORIENTED_EDGE('',*,*,#50911,.F.);
#71230=ORIENTED_EDGE('',*,*,#50912,.T.);
#71231=ORIENTED_EDGE('',*,*,#50913,.F.);
#71232=ORIENTED_EDGE('',*,*,#50822,.F.);
#71233=ORIENTED_EDGE('',*,*,#50914,.F.);
#71234=ORIENTED_EDGE('',*,*,#50817,.F.);
#71235=ORIENTED_EDGE('',*,*,#49458,.F.);
#71236=ORIENTED_EDGE('',*,*,#50780,.F.);
#71237=ORIENTED_EDGE('',*,*,#50915,.F.);
#71238=ORIENTED_EDGE('',*,*,#50777,.F.);
#71239=ORIENTED_EDGE('',*,*,#49418,.F.);
#71240=ORIENTED_EDGE('',*,*,#50729,.F.);
#71241=ORIENTED_EDGE('',*,*,#50916,.F.);
#71242=ORIENTED_EDGE('',*,*,#50724,.F.);
#71243=ORIENTED_EDGE('',*,*,#49541,.F.);
#71244=ORIENTED_EDGE('',*,*,#50795,.F.);
#71245=ORIENTED_EDGE('',*,*,#50917,.F.);
#71246=ORIENTED_EDGE('',*,*,#50802,.F.);
#71247=ORIENTED_EDGE('',*,*,#49482,.F.);
#71248=ORIENTED_EDGE('',*,*,#50720,.F.);
#71249=ORIENTED_EDGE('',*,*,#50918,.F.);
#71250=ORIENTED_EDGE('',*,*,#50715,.F.);
#71251=ORIENTED_EDGE('',*,*,#50018,.F.);
#71252=ORIENTED_EDGE('',*,*,#50786,.F.);
#71253=ORIENTED_EDGE('',*,*,#50919,.F.);
#71254=ORIENTED_EDGE('',*,*,#50781,.F.);
#71255=ORIENTED_EDGE('',*,*,#50058,.F.);
#71256=ORIENTED_EDGE('',*,*,#50741,.F.);
#71257=ORIENTED_EDGE('',*,*,#50920,.F.);
#71258=ORIENTED_EDGE('',*,*,#50736,.F.);
#71259=ORIENTED_EDGE('',*,*,#49517,.F.);
#71260=ORIENTED_EDGE('',*,*,#50507,.F.);
#71261=ORIENTED_EDGE('',*,*,#50921,.F.);
#71262=ORIENTED_EDGE('',*,*,#50502,.F.);
#71263=ORIENTED_EDGE('',*,*,#49506,.F.);
#71264=ORIENTED_EDGE('',*,*,#50852,.F.);
#71265=ORIENTED_EDGE('',*,*,#50922,.F.);
#71266=ORIENTED_EDGE('',*,*,#50499,.F.);
#71267=ORIENTED_EDGE('',*,*,#49731,.F.);
#71268=ORIENTED_EDGE('',*,*,#50483,.F.);
#71269=ORIENTED_EDGE('',*,*,#50923,.F.);
#71270=ORIENTED_EDGE('',*,*,#50853,.F.);
#71271=ORIENTED_EDGE('',*,*,#49749,.F.);
#71272=ORIENTED_EDGE('',*,*,#50768,.F.);
#71273=ORIENTED_EDGE('',*,*,#50924,.F.);
#71274=ORIENTED_EDGE('',*,*,#50763,.F.);
#71275=ORIENTED_EDGE('',*,*,#50034,.F.);
#71276=ORIENTED_EDGE('',*,*,#50810,.F.);
#71277=ORIENTED_EDGE('',*,*,#50925,.F.);
#71278=ORIENTED_EDGE('',*,*,#50805,.F.);
#71279=ORIENTED_EDGE('',*,*,#50090,.F.);
#71280=ORIENTED_EDGE('',*,*,#50753,.F.);
#71281=ORIENTED_EDGE('',*,*,#50926,.F.);
#71282=ORIENTED_EDGE('',*,*,#50748,.F.);
#71283=ORIENTED_EDGE('',*,*,#49859,.F.);
#71284=ORIENTED_EDGE('',*,*,#50476,.F.);
#71285=ORIENTED_EDGE('',*,*,#50927,.F.);
#71286=ORIENTED_EDGE('',*,*,#50520,.F.);
#71287=ORIENTED_EDGE('',*,*,#49883,.F.);
#71288=ORIENTED_EDGE('',*,*,#50513,.F.);
#71289=ORIENTED_EDGE('',*,*,#50928,.F.);
#71290=ORIENTED_EDGE('',*,*,#50508,.F.);
#71291=ORIENTED_EDGE('',*,*,#49490,.F.);
#71292=ORIENTED_EDGE('',*,*,#50816,.F.);
#71293=ORIENTED_EDGE('',*,*,#50929,.F.);
#71294=ORIENTED_EDGE('',*,*,#50811,.F.);
#71295=ORIENTED_EDGE('',*,*,#50082,.F.);
#71296=ORIENTED_EDGE('',*,*,#50519,.F.);
#71297=ORIENTED_EDGE('',*,*,#50930,.F.);
#71298=ORIENTED_EDGE('',*,*,#50514,.F.);
#71299=ORIENTED_EDGE('',*,*,#49875,.F.);
#71300=ORIENTED_EDGE('',*,*,#50843,.F.);
#71301=ORIENTED_EDGE('',*,*,#50931,.F.);
#71302=ORIENTED_EDGE('',*,*,#50451,.F.);
#71303=ORIENTED_EDGE('',*,*,#50261,.F.);
#71304=ORIENTED_EDGE('',*,*,#50474,.F.);
#71305=ORIENTED_EDGE('',*,*,#50932,.F.);
#71306=ORIENTED_EDGE('',*,*,#50840,.F.);
#71307=ORIENTED_EDGE('',*,*,#50227,.F.);
#71308=ORIENTED_EDGE('',*,*,#50801,.F.);
#71309=ORIENTED_EDGE('',*,*,#50933,.F.);
#71310=ORIENTED_EDGE('',*,*,#50796,.F.);
#71311=ORIENTED_EDGE('',*,*,#49466,.F.);
#71312=ORIENTED_EDGE('',*,*,#50828,.F.);
#71313=ORIENTED_EDGE('',*,*,#50934,.F.);
#71314=ORIENTED_EDGE('',*,*,#50825,.F.);
#71315=ORIENTED_EDGE('',*,*,#49442,.F.);
#71316=ORIENTED_EDGE('',*,*,#50792,.F.);
#71317=ORIENTED_EDGE('',*,*,#50935,.F.);
#71318=ORIENTED_EDGE('',*,*,#50787,.F.);
#71319=ORIENTED_EDGE('',*,*,#50066,.F.);
#71320=ORIENTED_EDGE('',*,*,#50936,.T.);
#71321=ORIENTED_EDGE('',*,*,#50937,.T.);
#71322=ORIENTED_EDGE('',*,*,#50938,.F.);
#71323=ORIENTED_EDGE('',*,*,#50939,.F.);
#71324=ORIENTED_EDGE('',*,*,#50940,.F.);
#71325=ORIENTED_EDGE('',*,*,#50941,.F.);
#71326=ORIENTED_EDGE('',*,*,#50942,.F.);
#71327=ORIENTED_EDGE('',*,*,#50938,.T.);
#71328=ORIENTED_EDGE('',*,*,#50941,.T.);
#71329=ORIENTED_EDGE('',*,*,#50943,.T.);
#71330=ORIENTED_EDGE('',*,*,#50944,.F.);
#71331=ORIENTED_EDGE('',*,*,#50945,.F.);
#71332=ORIENTED_EDGE('',*,*,#50944,.T.);
#71333=ORIENTED_EDGE('',*,*,#50946,.T.);
#71334=ORIENTED_EDGE('',*,*,#50947,.F.);
#71335=ORIENTED_EDGE('',*,*,#50948,.F.);
#71336=ORIENTED_EDGE('',*,*,#50947,.T.);
#71337=ORIENTED_EDGE('',*,*,#50949,.T.);
#71338=ORIENTED_EDGE('',*,*,#50950,.F.);
#71339=ORIENTED_EDGE('',*,*,#50951,.F.);
#71340=ORIENTED_EDGE('',*,*,#50952,.F.);
#71341=ORIENTED_EDGE('',*,*,#50953,.F.);
#71342=ORIENTED_EDGE('',*,*,#50954,.F.);
#71343=ORIENTED_EDGE('',*,*,#50950,.T.);
#71344=ORIENTED_EDGE('',*,*,#50953,.T.);
#71345=ORIENTED_EDGE('',*,*,#50955,.T.);
#71346=ORIENTED_EDGE('',*,*,#50956,.F.);
#71347=ORIENTED_EDGE('',*,*,#50957,.F.);
#71348=ORIENTED_EDGE('',*,*,#50958,.T.);
#71349=ORIENTED_EDGE('',*,*,#50959,.F.);
#71350=ORIENTED_EDGE('',*,*,#50960,.T.);
#71351=ORIENTED_EDGE('',*,*,#50961,.F.);
#71352=ORIENTED_EDGE('',*,*,#50962,.F.);
#71353=ORIENTED_EDGE('',*,*,#50963,.T.);
#71354=ORIENTED_EDGE('',*,*,#50958,.F.);
#71355=ORIENTED_EDGE('',*,*,#50964,.T.);
#71356=ORIENTED_EDGE('',*,*,#50965,.T.);
#71357=ORIENTED_EDGE('',*,*,#50966,.T.);
#71358=ORIENTED_EDGE('',*,*,#50967,.F.);
#71359=ORIENTED_EDGE('',*,*,#50968,.T.);
#71360=ORIENTED_EDGE('',*,*,#50966,.F.);
#71361=ORIENTED_EDGE('',*,*,#50969,.F.);
#71362=ORIENTED_EDGE('',*,*,#50970,.T.);
#71363=ORIENTED_EDGE('',*,*,#50971,.F.);
#71364=ORIENTED_EDGE('',*,*,#50972,.T.);
#71365=ORIENTED_EDGE('',*,*,#50973,.F.);
#71366=ORIENTED_EDGE('',*,*,#50974,.T.);
#71367=ORIENTED_EDGE('',*,*,#50975,.F.);
#71368=ORIENTED_EDGE('',*,*,#50976,.F.);
#71369=ORIENTED_EDGE('',*,*,#50977,.F.);
#71370=ORIENTED_EDGE('',*,*,#50976,.T.);
#71371=ORIENTED_EDGE('',*,*,#50978,.F.);
#71372=ORIENTED_EDGE('',*,*,#50970,.F.);
#71373=ORIENTED_EDGE('',*,*,#50979,.F.);
#71374=ORIENTED_EDGE('',*,*,#50980,.T.);
#71375=ORIENTED_EDGE('',*,*,#50981,.F.);
#71376=ORIENTED_EDGE('',*,*,#50982,.F.);
#71377=ORIENTED_EDGE('',*,*,#50983,.F.);
#71378=ORIENTED_EDGE('',*,*,#50984,.T.);
#71379=ORIENTED_EDGE('',*,*,#50985,.F.);
#71380=ORIENTED_EDGE('',*,*,#50986,.T.);
#71381=ORIENTED_EDGE('',*,*,#50987,.F.);
#71382=ORIENTED_EDGE('',*,*,#50982,.T.);
#71383=ORIENTED_EDGE('',*,*,#50988,.F.);
#71384=ORIENTED_EDGE('',*,*,#50984,.F.);
#71385=ORIENTED_EDGE('',*,*,#50989,.T.);
#71386=ORIENTED_EDGE('',*,*,#50990,.F.);
#71387=ORIENTED_EDGE('',*,*,#50991,.F.);
#71388=ORIENTED_EDGE('',*,*,#50992,.T.);
#71389=ORIENTED_EDGE('',*,*,#50993,.T.);
#71390=ORIENTED_EDGE('',*,*,#50994,.F.);
#71391=ORIENTED_EDGE('',*,*,#50995,.F.);
#71392=ORIENTED_EDGE('',*,*,#50996,.T.);
#71393=ORIENTED_EDGE('',*,*,#50997,.T.);
#71394=ORIENTED_EDGE('',*,*,#50998,.F.);
#71395=ORIENTED_EDGE('',*,*,#50999,.F.);
#71396=ORIENTED_EDGE('',*,*,#50994,.T.);
#71397=ORIENTED_EDGE('',*,*,#51000,.T.);
#71398=ORIENTED_EDGE('',*,*,#51001,.F.);
#71399=ORIENTED_EDGE('',*,*,#51002,.F.);
#71400=ORIENTED_EDGE('',*,*,#50998,.T.);
#71401=ORIENTED_EDGE('',*,*,#51003,.F.);
#71402=ORIENTED_EDGE('',*,*,#51004,.F.);
#71403=ORIENTED_EDGE('',*,*,#51001,.T.);
#71404=ORIENTED_EDGE('',*,*,#51005,.T.);
#71405=ORIENTED_EDGE('',*,*,#51006,.T.);
#71406=ORIENTED_EDGE('',*,*,#51007,.F.);
#71407=ORIENTED_EDGE('',*,*,#51008,.F.);
#71408=ORIENTED_EDGE('',*,*,#51009,.T.);
#71409=ORIENTED_EDGE('',*,*,#51010,.T.);
#71410=ORIENTED_EDGE('',*,*,#50992,.F.);
#71411=ORIENTED_EDGE('',*,*,#51011,.F.);
#71412=ORIENTED_EDGE('',*,*,#51007,.T.);
#71413=ORIENTED_EDGE('',*,*,#51012,.F.);
#71414=ORIENTED_EDGE('',*,*,#51013,.T.);
#71415=ORIENTED_EDGE('',*,*,#51014,.F.);
#71416=ORIENTED_EDGE('',*,*,#51015,.T.);
#71417=ORIENTED_EDGE('',*,*,#51016,.F.);
#71418=ORIENTED_EDGE('',*,*,#51017,.F.);
#71419=ORIENTED_EDGE('',*,*,#51018,.T.);
#71420=ORIENTED_EDGE('',*,*,#51019,.T.);
#71421=ORIENTED_EDGE('',*,*,#51020,.T.);
#71422=ORIENTED_EDGE('',*,*,#51021,.F.);
#71423=ORIENTED_EDGE('',*,*,#51022,.F.);
#71424=ORIENTED_EDGE('',*,*,#51023,.T.);
#71425=ORIENTED_EDGE('',*,*,#51024,.F.);
#71426=ORIENTED_EDGE('',*,*,#51025,.T.);
#71427=ORIENTED_EDGE('',*,*,#51026,.F.);
#71428=ORIENTED_EDGE('',*,*,#51027,.F.);
#71429=ORIENTED_EDGE('',*,*,#51028,.T.);
#71430=ORIENTED_EDGE('',*,*,#51029,.T.);
#71431=ORIENTED_EDGE('',*,*,#51030,.T.);
#71432=ORIENTED_EDGE('',*,*,#51031,.T.);
#71433=ORIENTED_EDGE('',*,*,#51032,.T.);
#71434=ORIENTED_EDGE('',*,*,#51033,.F.);
#71435=ORIENTED_EDGE('',*,*,#51019,.F.);
#71436=ORIENTED_EDGE('',*,*,#51034,.F.);
#71437=ORIENTED_EDGE('',*,*,#51035,.T.);
#71438=ORIENTED_EDGE('',*,*,#51036,.F.);
#71439=ORIENTED_EDGE('',*,*,#50973,.T.);
#71440=ORIENTED_EDGE('',*,*,#50977,.T.);
#71441=ORIENTED_EDGE('',*,*,#50969,.T.);
#71442=ORIENTED_EDGE('',*,*,#51037,.F.);
#71443=ORIENTED_EDGE('',*,*,#51038,.T.);
#71444=ORIENTED_EDGE('',*,*,#51039,.T.);
#71445=ORIENTED_EDGE('',*,*,#51035,.F.);
#71446=ORIENTED_EDGE('',*,*,#51040,.T.);
#71447=ORIENTED_EDGE('',*,*,#51038,.F.);
#71448=ORIENTED_EDGE('',*,*,#51041,.T.);
#71449=ORIENTED_EDGE('',*,*,#51015,.F.);
#71450=ORIENTED_EDGE('',*,*,#51042,.T.);
#71451=ORIENTED_EDGE('',*,*,#51043,.T.);
#71452=ORIENTED_EDGE('',*,*,#51044,.F.);
#71453=ORIENTED_EDGE('',*,*,#51029,.F.);
#71454=ORIENTED_EDGE('',*,*,#51045,.F.);
#71455=ORIENTED_EDGE('',*,*,#51046,.T.);
#71456=ORIENTED_EDGE('',*,*,#50987,.T.);
#71457=ORIENTED_EDGE('',*,*,#50983,.T.);
#71458=ORIENTED_EDGE('',*,*,#51047,.F.);
#71459=ORIENTED_EDGE('',*,*,#51048,.T.);
#71460=ORIENTED_EDGE('',*,*,#51049,.T.);
#71461=ORIENTED_EDGE('',*,*,#51046,.F.);
#71462=ORIENTED_EDGE('',*,*,#51050,.F.);
#71463=ORIENTED_EDGE('',*,*,#50979,.T.);
#71464=ORIENTED_EDGE('',*,*,#51051,.T.);
#71465=ORIENTED_EDGE('',*,*,#51048,.F.);
#71466=ORIENTED_EDGE('',*,*,#51052,.T.);
#71467=ORIENTED_EDGE('',*,*,#51025,.F.);
#71468=ORIENTED_EDGE('',*,*,#51053,.T.);
#71469=ORIENTED_EDGE('',*,*,#51054,.T.);
#71470=ORIENTED_EDGE('',*,*,#51055,.F.);
#71471=ORIENTED_EDGE('',*,*,#51056,.F.);
#71472=ORIENTED_EDGE('',*,*,#51057,.T.);
#71473=ORIENTED_EDGE('',*,*,#51058,.T.);
#71474=ORIENTED_EDGE('',*,*,#51057,.F.);
#71475=ORIENTED_EDGE('',*,*,#51059,.F.);
#71476=ORIENTED_EDGE('',*,*,#51060,.T.);
#71477=ORIENTED_EDGE('',*,*,#51061,.T.);
#71478=ORIENTED_EDGE('',*,*,#51060,.F.);
#71479=ORIENTED_EDGE('',*,*,#51062,.F.);
#71480=ORIENTED_EDGE('',*,*,#51063,.T.);
#71481=ORIENTED_EDGE('',*,*,#51064,.T.);
#71482=ORIENTED_EDGE('',*,*,#51063,.F.);
#71483=ORIENTED_EDGE('',*,*,#51065,.F.);
#71484=ORIENTED_EDGE('',*,*,#51066,.T.);
#71485=ORIENTED_EDGE('',*,*,#51067,.T.);
#71486=ORIENTED_EDGE('',*,*,#51068,.F.);
#71487=ORIENTED_EDGE('',*,*,#51069,.F.);
#71488=ORIENTED_EDGE('',*,*,#51070,.T.);
#71489=ORIENTED_EDGE('',*,*,#51071,.T.);
#71490=ORIENTED_EDGE('',*,*,#51070,.F.);
#71491=ORIENTED_EDGE('',*,*,#51072,.F.);
#71492=ORIENTED_EDGE('',*,*,#51073,.T.);
#71493=ORIENTED_EDGE('',*,*,#51074,.T.);
#71494=ORIENTED_EDGE('',*,*,#51073,.F.);
#71495=ORIENTED_EDGE('',*,*,#51075,.F.);
#71496=ORIENTED_EDGE('',*,*,#51055,.T.);
#71497=ORIENTED_EDGE('',*,*,#51076,.F.);
#71498=ORIENTED_EDGE('',*,*,#51077,.T.);
#71499=ORIENTED_EDGE('',*,*,#51078,.T.);
#71500=ORIENTED_EDGE('',*,*,#51013,.F.);
#71501=ORIENTED_EDGE('',*,*,#51079,.T.);
#71502=ORIENTED_EDGE('',*,*,#51080,.T.);
#71503=ORIENTED_EDGE('',*,*,#51081,.F.);
#71504=ORIENTED_EDGE('',*,*,#51031,.F.);
#71505=ORIENTED_EDGE('',*,*,#51082,.F.);
#71506=ORIENTED_EDGE('',*,*,#51079,.F.);
#71507=ORIENTED_EDGE('',*,*,#51030,.F.);
#71508=ORIENTED_EDGE('',*,*,#51044,.T.);
#71509=ORIENTED_EDGE('',*,*,#51083,.T.);
#71510=ORIENTED_EDGE('',*,*,#51042,.F.);
#71511=ORIENTED_EDGE('',*,*,#51014,.T.);
#71512=ORIENTED_EDGE('',*,*,#51078,.F.);
#71513=ORIENTED_EDGE('',*,*,#51084,.F.);
#71514=ORIENTED_EDGE('',*,*,#51085,.T.);
#71515=ORIENTED_EDGE('',*,*,#51086,.T.);
#71516=ORIENTED_EDGE('',*,*,#51023,.F.);
#71517=ORIENTED_EDGE('',*,*,#51087,.F.);
#71518=ORIENTED_EDGE('',*,*,#51088,.T.);
#71519=ORIENTED_EDGE('',*,*,#51076,.T.);
#71520=ORIENTED_EDGE('',*,*,#51012,.T.);
#71521=ORIENTED_EDGE('',*,*,#51089,.T.);
#71522=ORIENTED_EDGE('',*,*,#51017,.T.);
#71523=ORIENTED_EDGE('',*,*,#51090,.T.);
#71524=ORIENTED_EDGE('',*,*,#51091,.F.);
#71525=ORIENTED_EDGE('',*,*,#51092,.F.);
#71526=ORIENTED_EDGE('',*,*,#50989,.F.);
#71527=ORIENTED_EDGE('',*,*,#51010,.F.);
#71528=ORIENTED_EDGE('',*,*,#51006,.F.);
#71529=ORIENTED_EDGE('',*,*,#51093,.F.);
#71530=ORIENTED_EDGE('',*,*,#51090,.F.);
#71531=ORIENTED_EDGE('',*,*,#51021,.T.);
#71532=ORIENTED_EDGE('',*,*,#51094,.T.);
#71533=ORIENTED_EDGE('',*,*,#51095,.F.);
#71534=ORIENTED_EDGE('',*,*,#50985,.T.);
#71535=ORIENTED_EDGE('',*,*,#50988,.T.);
#71536=ORIENTED_EDGE('',*,*,#50981,.T.);
#71537=ORIENTED_EDGE('',*,*,#51096,.F.);
#71538=ORIENTED_EDGE('',*,*,#51097,.T.);
#71539=ORIENTED_EDGE('',*,*,#51098,.F.);
#71540=ORIENTED_EDGE('',*,*,#51096,.T.);
#71541=ORIENTED_EDGE('',*,*,#50980,.F.);
#71542=ORIENTED_EDGE('',*,*,#51050,.T.);
#71543=ORIENTED_EDGE('',*,*,#51045,.T.);
#71544=ORIENTED_EDGE('',*,*,#51028,.F.);
#71545=ORIENTED_EDGE('',*,*,#51099,.F.);
#71546=ORIENTED_EDGE('',*,*,#51026,.T.);
#71547=ORIENTED_EDGE('',*,*,#51052,.F.);
#71548=ORIENTED_EDGE('',*,*,#51047,.T.);
#71549=ORIENTED_EDGE('',*,*,#50986,.F.);
#71550=ORIENTED_EDGE('',*,*,#51095,.T.);
#71551=ORIENTED_EDGE('',*,*,#51100,.T.);
#71552=ORIENTED_EDGE('',*,*,#50967,.T.);
#71553=ORIENTED_EDGE('',*,*,#50965,.F.);
#71554=ORIENTED_EDGE('',*,*,#51101,.F.);
#71555=ORIENTED_EDGE('',*,*,#51102,.F.);
#71556=ORIENTED_EDGE('',*,*,#51103,.T.);
#71557=ORIENTED_EDGE('',*,*,#50975,.T.);
#71558=ORIENTED_EDGE('',*,*,#51104,.F.);
#71559=ORIENTED_EDGE('',*,*,#51105,.T.);
#71560=ORIENTED_EDGE('',*,*,#51106,.F.);
#71561=ORIENTED_EDGE('',*,*,#50971,.T.);
#71562=ORIENTED_EDGE('',*,*,#50978,.T.);
#71563=ORIENTED_EDGE('',*,*,#51107,.F.);
#71564=ORIENTED_EDGE('',*,*,#51104,.T.);
#71565=ORIENTED_EDGE('',*,*,#50974,.F.);
#71566=ORIENTED_EDGE('',*,*,#51036,.T.);
#71567=ORIENTED_EDGE('',*,*,#51034,.T.);
#71568=ORIENTED_EDGE('',*,*,#51018,.F.);
#71569=ORIENTED_EDGE('',*,*,#51089,.F.);
#71570=ORIENTED_EDGE('',*,*,#51016,.T.);
#71571=ORIENTED_EDGE('',*,*,#51041,.F.);
#71572=ORIENTED_EDGE('',*,*,#51037,.T.);
#71573=ORIENTED_EDGE('',*,*,#50972,.F.);
#71574=ORIENTED_EDGE('',*,*,#51106,.T.);
#71575=ORIENTED_EDGE('',*,*,#51108,.F.);
#71576=ORIENTED_EDGE('',*,*,#50962,.T.);
#71577=ORIENTED_EDGE('',*,*,#50961,.T.);
#71578=ORIENTED_EDGE('',*,*,#51109,.T.);
#71579=ORIENTED_EDGE('',*,*,#51110,.F.);
#71580=ORIENTED_EDGE('',*,*,#51111,.T.);
#71581=ORIENTED_EDGE('',*,*,#51112,.T.);
#71582=ORIENTED_EDGE('',*,*,#51005,.F.);
#71583=ORIENTED_EDGE('',*,*,#51000,.F.);
#71584=ORIENTED_EDGE('',*,*,#50997,.F.);
#71585=ORIENTED_EDGE('',*,*,#50993,.F.);
#71586=ORIENTED_EDGE('',*,*,#51113,.F.);
#71587=ORIENTED_EDGE('',*,*,#51114,.T.);
#71588=ORIENTED_EDGE('',*,*,#51084,.T.);
#71589=ORIENTED_EDGE('',*,*,#51022,.T.);
#71590=ORIENTED_EDGE('',*,*,#51099,.T.);
#71591=ORIENTED_EDGE('',*,*,#51027,.T.);
#71592=ORIENTED_EDGE('',*,*,#51081,.T.);
#71593=ORIENTED_EDGE('',*,*,#51115,.F.);
#71594=ORIENTED_EDGE('',*,*,#51116,.T.);
#71595=ORIENTED_EDGE('',*,*,#51117,.F.);
#71596=ORIENTED_EDGE('',*,*,#51118,.T.);
#71597=ORIENTED_EDGE('',*,*,#51119,.F.);
#71598=ORIENTED_EDGE('',*,*,#51120,.T.);
#71599=ORIENTED_EDGE('',*,*,#51121,.F.);
#71600=ORIENTED_EDGE('',*,*,#51122,.F.);
#71601=ORIENTED_EDGE('',*,*,#51102,.T.);
#71602=ORIENTED_EDGE('',*,*,#51123,.T.);
#71603=ORIENTED_EDGE('',*,*,#51124,.T.);
#71604=ORIENTED_EDGE('',*,*,#51125,.F.);
#71605=ORIENTED_EDGE('',*,*,#51126,.F.);
#71606=ORIENTED_EDGE('',*,*,#51127,.T.);
#71607=ORIENTED_EDGE('',*,*,#51117,.T.);
#71608=ORIENTED_EDGE('',*,*,#51128,.F.);
#71609=ORIENTED_EDGE('',*,*,#51129,.T.);
#71610=ORIENTED_EDGE('',*,*,#51115,.T.);
#71611=ORIENTED_EDGE('',*,*,#51130,.T.);
#71612=ORIENTED_EDGE('',*,*,#51131,.F.);
#71613=ORIENTED_EDGE('',*,*,#51132,.T.);
#71614=ORIENTED_EDGE('',*,*,#51087,.T.);
#71615=ORIENTED_EDGE('',*,*,#51009,.F.);
#71616=ORIENTED_EDGE('',*,*,#51133,.F.);
#71617=ORIENTED_EDGE('',*,*,#51134,.T.);
#71618=ORIENTED_EDGE('',*,*,#51119,.T.);
#71619=ORIENTED_EDGE('',*,*,#51135,.T.);
#71620=ORIENTED_EDGE('',*,*,#51136,.F.);
#71621=ORIENTED_EDGE('',*,*,#51122,.T.);
#71622=ORIENTED_EDGE('',*,*,#51137,.T.);
#71623=ORIENTED_EDGE('',*,*,#51138,.F.);
#71624=ORIENTED_EDGE('',*,*,#50990,.T.);
#71625=ORIENTED_EDGE('',*,*,#51092,.T.);
#71626=ORIENTED_EDGE('',*,*,#50960,.F.);
#71627=ORIENTED_EDGE('',*,*,#51139,.T.);
#71628=ORIENTED_EDGE('',*,*,#51109,.F.);
#71629=ORIENTED_EDGE('',*,*,#51140,.F.);
#71630=ORIENTED_EDGE('',*,*,#51123,.F.);
#71631=ORIENTED_EDGE('',*,*,#51101,.T.);
#71632=ORIENTED_EDGE('',*,*,#50964,.F.);
#71633=ORIENTED_EDGE('',*,*,#50968,.F.);
#71634=ORIENTED_EDGE('',*,*,#51100,.F.);
#71635=ORIENTED_EDGE('',*,*,#51097,.F.);
#71636=ORIENTED_EDGE('',*,*,#51098,.T.);
#71637=ORIENTED_EDGE('',*,*,#51124,.F.);
#71638=ORIENTED_EDGE('',*,*,#51140,.T.);
#71639=ORIENTED_EDGE('',*,*,#51103,.F.);
#71640=ORIENTED_EDGE('',*,*,#51141,.F.);
#71641=ORIENTED_EDGE('',*,*,#51142,.T.);
#71642=ORIENTED_EDGE('',*,*,#51003,.T.);
#71643=ORIENTED_EDGE('',*,*,#51112,.F.);
#71644=ORIENTED_EDGE('',*,*,#51080,.F.);
#71645=ORIENTED_EDGE('',*,*,#51082,.T.);
#71646=ORIENTED_EDGE('',*,*,#51077,.F.);
#71647=ORIENTED_EDGE('',*,*,#51088,.F.);
#71648=ORIENTED_EDGE('',*,*,#51132,.F.);
#71649=ORIENTED_EDGE('',*,*,#51143,.F.);
#71650=ORIENTED_EDGE('',*,*,#51144,.F.);
#71651=ORIENTED_EDGE('',*,*,#51135,.F.);
#71652=ORIENTED_EDGE('',*,*,#51120,.F.);
#71653=ORIENTED_EDGE('',*,*,#51134,.F.);
#71654=ORIENTED_EDGE('',*,*,#51145,.F.);
#71655=ORIENTED_EDGE('',*,*,#51125,.T.);
#71656=ORIENTED_EDGE('',*,*,#51118,.F.);
#71657=ORIENTED_EDGE('',*,*,#51127,.F.);
#71658=ORIENTED_EDGE('',*,*,#51146,.F.);
#71659=ORIENTED_EDGE('',*,*,#51130,.F.);
#71660=ORIENTED_EDGE('',*,*,#51116,.F.);
#71661=ORIENTED_EDGE('',*,*,#51129,.F.);
#71662=ORIENTED_EDGE('',*,*,#51105,.F.);
#71663=ORIENTED_EDGE('',*,*,#51107,.T.);
#71664=ORIENTED_EDGE('',*,*,#51139,.F.);
#71665=ORIENTED_EDGE('',*,*,#50959,.T.);
#71666=ORIENTED_EDGE('',*,*,#50963,.F.);
#71667=ORIENTED_EDGE('',*,*,#51108,.T.);
#71668=ORIENTED_EDGE('',*,*,#51147,.F.);
#71669=ORIENTED_EDGE('',*,*,#51148,.T.);
#71670=ORIENTED_EDGE('',*,*,#51149,.T.);
#71671=ORIENTED_EDGE('',*,*,#49398,.F.);
#71672=ORIENTED_EDGE('',*,*,#50696,.F.);
#71673=ORIENTED_EDGE('',*,*,#51150,.T.);
#71674=ORIENTED_EDGE('',*,*,#51151,.T.);
#71675=ORIENTED_EDGE('',*,*,#49653,.F.);
#71676=ORIENTED_EDGE('',*,*,#51151,.F.);
#71677=ORIENTED_EDGE('',*,*,#51152,.T.);
#71678=ORIENTED_EDGE('',*,*,#51153,.T.);
#71679=ORIENTED_EDGE('',*,*,#49659,.F.);
#71680=ORIENTED_EDGE('',*,*,#50684,.F.);
#71681=ORIENTED_EDGE('',*,*,#51154,.T.);
#71682=ORIENTED_EDGE('',*,*,#50679,.F.);
#71683=ORIENTED_EDGE('',*,*,#49629,.F.);
#71684=ORIENTED_EDGE('',*,*,#51155,.F.);
#71685=ORIENTED_EDGE('',*,*,#51156,.T.);
#71686=ORIENTED_EDGE('',*,*,#51157,.T.);
#71687=ORIENTED_EDGE('',*,*,#49940,.F.);
#71688=ORIENTED_EDGE('',*,*,#51157,.F.);
#71689=ORIENTED_EDGE('',*,*,#51158,.T.);
#71690=ORIENTED_EDGE('',*,*,#50571,.F.);
#71691=ORIENTED_EDGE('',*,*,#49934,.F.);
#71692=ORIENTED_EDGE('',*,*,#51159,.F.);
#71693=ORIENTED_EDGE('',*,*,#51160,.T.);
#71694=ORIENTED_EDGE('',*,*,#51161,.T.);
#71695=ORIENTED_EDGE('',*,*,#49998,.F.);
#71696=ORIENTED_EDGE('',*,*,#51162,.F.);
#71697=ORIENTED_EDGE('',*,*,#51162,.T.);
#71698=ORIENTED_EDGE('',*,*,#51163,.T.);
#71699=ORIENTED_EDGE('',*,*,#51164,.F.);
#71700=ORIENTED_EDGE('',*,*,#49134,.F.);
#71701=ORIENTED_EDGE('',*,*,#51165,.F.);
#71702=ORIENTED_EDGE('',*,*,#51163,.F.);
#71703=ORIENTED_EDGE('',*,*,#51166,.F.);
#71704=ORIENTED_EDGE('',*,*,#51166,.T.);
#71705=ORIENTED_EDGE('',*,*,#51167,.T.);
#71706=ORIENTED_EDGE('',*,*,#49137,.F.);
#71707=ORIENTED_EDGE('',*,*,#49138,.F.);
#71708=ORIENTED_EDGE('',*,*,#51167,.F.);
#71709=ORIENTED_EDGE('',*,*,#49366,.F.);
#71710=ORIENTED_EDGE('',*,*,#49362,.F.);
#71711=ORIENTED_EDGE('',*,*,#49361,.F.);
#71712=ORIENTED_EDGE('',*,*,#49358,.F.);
#71713=ORIENTED_EDGE('',*,*,#49353,.F.);
#71714=ORIENTED_EDGE('',*,*,#49155,.F.);
#71715=ORIENTED_EDGE('',*,*,#49135,.F.);
#71716=ORIENTED_EDGE('',*,*,#49355,.F.);
#71717=ORIENTED_EDGE('',*,*,#49375,.F.);
#71718=ORIENTED_EDGE('',*,*,#49144,.F.);
#71719=ORIENTED_EDGE('',*,*,#49377,.F.);
#71720=ORIENTED_EDGE('',*,*,#49365,.F.);
#71721=ORIENTED_EDGE('',*,*,#49167,.F.);
#71722=ORIENTED_EDGE('',*,*,#49376,.F.);
#71723=ORIENTED_EDGE('',*,*,#49360,.F.);
#71724=ORIENTED_EDGE('',*,*,#49378,.F.);
#71725=ORIENTED_EDGE('',*,*,#49159,.F.);
#71726=ORIENTED_EDGE('',*,*,#49324,.F.);
#71727=ORIENTED_EDGE('',*,*,#49322,.F.);
#71728=ORIENTED_EDGE('',*,*,#49316,.F.);
#71729=ORIENTED_EDGE('',*,*,#51168,.F.);
#71730=ORIENTED_EDGE('',*,*,#49319,.F.);
#71731=ORIENTED_EDGE('',*,*,#49314,.F.);
#71732=ORIENTED_EDGE('',*,*,#49310,.F.);
#71733=ORIENTED_EDGE('',*,*,#49186,.F.);
#71734=ORIENTED_EDGE('',*,*,#49312,.F.);
#71735=ORIENTED_EDGE('',*,*,#49373,.F.);
#71736=ORIENTED_EDGE('',*,*,#49197,.F.);
#71737=ORIENTED_EDGE('',*,*,#49372,.F.);
#71738=ORIENTED_EDGE('',*,*,#49323,.F.);
#71739=ORIENTED_EDGE('',*,*,#49182,.F.);
#71740=ORIENTED_EDGE('',*,*,#49374,.F.);
#71741=ORIENTED_EDGE('',*,*,#49318,.F.);
#71742=ORIENTED_EDGE('',*,*,#49371,.F.);
#71743=ORIENTED_EDGE('',*,*,#49210,.F.);
#71744=ORIENTED_EDGE('',*,*,#49341,.F.);
#71745=ORIENTED_EDGE('',*,*,#49381,.F.);
#71746=ORIENTED_EDGE('',*,*,#49262,.F.);
#71747=ORIENTED_EDGE('',*,*,#49256,.F.);
#71748=ORIENTED_EDGE('',*,*,#49258,.F.);
#71749=ORIENTED_EDGE('',*,*,#49380,.F.);
#71750=ORIENTED_EDGE('',*,*,#49351,.F.);
#71751=ORIENTED_EDGE('',*,*,#49252,.F.);
#71752=ORIENTED_EDGE('',*,*,#49382,.F.);
#71753=ORIENTED_EDGE('',*,*,#49346,.F.);
#71754=ORIENTED_EDGE('',*,*,#49379,.F.);
#71755=ORIENTED_EDGE('',*,*,#49276,.F.);
#71756=ORIENTED_EDGE('',*,*,#49368,.F.);
#71757=ORIENTED_EDGE('',*,*,#49337,.F.);
#71758=ORIENTED_EDGE('',*,*,#49299,.F.);
#71759=ORIENTED_EDGE('',*,*,#49292,.F.);
#71760=ORIENTED_EDGE('',*,*,#49327,.F.);
#71761=ORIENTED_EDGE('',*,*,#49369,.F.);
#71762=ORIENTED_EDGE('',*,*,#49301,.F.);
#71763=ORIENTED_EDGE('',*,*,#49306,.F.);
#71764=ORIENTED_EDGE('',*,*,#49370,.F.);
#71765=ORIENTED_EDGE('',*,*,#49332,.F.);
#71766=ORIENTED_EDGE('',*,*,#49367,.F.);
#71767=ORIENTED_EDGE('',*,*,#49282,.F.);
#71768=ORIENTED_EDGE('',*,*,#50443,.F.);
#71769=ORIENTED_EDGE('',*,*,#50359,.F.);
#71770=ORIENTED_EDGE('',*,*,#50370,.F.);
#71771=ORIENTED_EDGE('',*,*,#50369,.F.);
#71772=ORIENTED_EDGE('',*,*,#50368,.F.);
#71773=ORIENTED_EDGE('',*,*,#50367,.F.);
#71774=ORIENTED_EDGE('',*,*,#50366,.F.);
#71775=ORIENTED_EDGE('',*,*,#50365,.F.);
#71776=ORIENTED_EDGE('',*,*,#50364,.F.);
#71777=ORIENTED_EDGE('',*,*,#50375,.F.);
#71778=ORIENTED_EDGE('',*,*,#50444,.F.);
#71779=ORIENTED_EDGE('',*,*,#50320,.F.);
#71780=ORIENTED_EDGE('',*,*,#50319,.F.);
#71781=ORIENTED_EDGE('',*,*,#50318,.F.);
#71782=ORIENTED_EDGE('',*,*,#50317,.F.);
#71783=ORIENTED_EDGE('',*,*,#50316,.F.);
#71784=ORIENTED_EDGE('',*,*,#50315,.F.);
#71785=ORIENTED_EDGE('',*,*,#51169,.F.);
#71786=ORIENTED_EDGE('',*,*,#51170,.F.);
#71787=ORIENTED_EDGE('',*,*,#51171,.T.);
#71788=ORIENTED_EDGE('',*,*,#50173,.F.);
#71789=ORIENTED_EDGE('',*,*,#51172,.F.);
#71790=ORIENTED_EDGE('',*,*,#51173,.F.);
#71791=ORIENTED_EDGE('',*,*,#51169,.T.);
#71792=ORIENTED_EDGE('',*,*,#50170,.F.);
#71793=ORIENTED_EDGE('',*,*,#51174,.F.);
#71794=ORIENTED_EDGE('',*,*,#51175,.F.);
#71795=ORIENTED_EDGE('',*,*,#51172,.T.);
#71796=ORIENTED_EDGE('',*,*,#50167,.F.);
#71797=ORIENTED_EDGE('',*,*,#51176,.F.);
#71798=ORIENTED_EDGE('',*,*,#51177,.F.);
#71799=ORIENTED_EDGE('',*,*,#51174,.T.);
#71800=ORIENTED_EDGE('',*,*,#50164,.F.);
#71801=ORIENTED_EDGE('',*,*,#51178,.F.);
#71802=ORIENTED_EDGE('',*,*,#51179,.F.);
#71803=ORIENTED_EDGE('',*,*,#51176,.T.);
#71804=ORIENTED_EDGE('',*,*,#50161,.F.);
#71805=ORIENTED_EDGE('',*,*,#51180,.F.);
#71806=ORIENTED_EDGE('',*,*,#51181,.F.);
#71807=ORIENTED_EDGE('',*,*,#51178,.T.);
#71808=ORIENTED_EDGE('',*,*,#50158,.F.);
#71809=ORIENTED_EDGE('',*,*,#51171,.F.);
#71810=ORIENTED_EDGE('',*,*,#51182,.F.);
#71811=ORIENTED_EDGE('',*,*,#51183,.T.);
#71812=ORIENTED_EDGE('',*,*,#50176,.F.);
#71813=ORIENTED_EDGE('',*,*,#51184,.F.);
#71814=ORIENTED_EDGE('',*,*,#51185,.T.);
#71815=ORIENTED_EDGE('',*,*,#51186,.T.);
#71816=ORIENTED_EDGE('',*,*,#50134,.F.);
#71817=ORIENTED_EDGE('',*,*,#51187,.F.);
#71818=ORIENTED_EDGE('',*,*,#51188,.T.);
#71819=ORIENTED_EDGE('',*,*,#51189,.T.);
#71820=ORIENTED_EDGE('',*,*,#50153,.F.);
#71821=ORIENTED_EDGE('',*,*,#51189,.F.);
#71822=ORIENTED_EDGE('',*,*,#51190,.T.);
#71823=ORIENTED_EDGE('',*,*,#51191,.T.);
#71824=ORIENTED_EDGE('',*,*,#50150,.F.);
#71825=ORIENTED_EDGE('',*,*,#51191,.F.);
#71826=ORIENTED_EDGE('',*,*,#51192,.T.);
#71827=ORIENTED_EDGE('',*,*,#51193,.T.);
#71828=ORIENTED_EDGE('',*,*,#50147,.F.);
#71829=ORIENTED_EDGE('',*,*,#51193,.F.);
#71830=ORIENTED_EDGE('',*,*,#51194,.T.);
#71831=ORIENTED_EDGE('',*,*,#51195,.T.);
#71832=ORIENTED_EDGE('',*,*,#50144,.F.);
#71833=ORIENTED_EDGE('',*,*,#51195,.F.);
#71834=ORIENTED_EDGE('',*,*,#51196,.T.);
#71835=ORIENTED_EDGE('',*,*,#51197,.T.);
#71836=ORIENTED_EDGE('',*,*,#50141,.F.);
#71837=ORIENTED_EDGE('',*,*,#51197,.F.);
#71838=ORIENTED_EDGE('',*,*,#51198,.T.);
#71839=ORIENTED_EDGE('',*,*,#51184,.T.);
#71840=ORIENTED_EDGE('',*,*,#50138,.F.);
#71841=ORIENTED_EDGE('',*,*,#51199,.T.);
#71842=ORIENTED_EDGE('',*,*,#50350,.F.);
#71843=ORIENTED_EDGE('',*,*,#50353,.F.);
#71844=ORIENTED_EDGE('',*,*,#51200,.F.);
#71845=ORIENTED_EDGE('',*,*,#50329,.F.);
#71846=ORIENTED_EDGE('',*,*,#51201,.T.);
#71847=ORIENTED_EDGE('',*,*,#50401,.F.);
#71848=ORIENTED_EDGE('',*,*,#50404,.F.);
#71849=ORIENTED_EDGE('',*,*,#51202,.F.);
#71850=ORIENTED_EDGE('',*,*,#50335,.F.);
#71851=ORIENTED_EDGE('',*,*,#51203,.T.);
#71852=ORIENTED_EDGE('',*,*,#50434,.F.);
#71853=ORIENTED_EDGE('',*,*,#50431,.F.);
#71854=ORIENTED_EDGE('',*,*,#51204,.F.);
#71855=ORIENTED_EDGE('',*,*,#50300,.F.);
#71856=ORIENTED_EDGE('',*,*,#51205,.F.);
#71857=ORIENTED_EDGE('',*,*,#50381,.F.);
#71858=ORIENTED_EDGE('',*,*,#50384,.F.);
#71859=ORIENTED_EDGE('',*,*,#51206,.F.);
#71860=ORIENTED_EDGE('',*,*,#50306,.F.);
#71861=ORIENTED_EDGE('',*,*,#51207,.F.);
#71862=ORIENTED_EDGE('',*,*,#50408,.F.);
#71863=ORIENTED_EDGE('',*,*,#50405,.F.);
#71864=ORIENTED_EDGE('',*,*,#51208,.T.);
#71865=ORIENTED_EDGE('',*,*,#49238,.F.);
#71866=ORIENTED_EDGE('',*,*,#51209,.F.);
#71867=ORIENTED_EDGE('',*,*,#50343,.F.);
#71868=ORIENTED_EDGE('',*,*,#49273,.F.);
#71869=ORIENTED_EDGE('',*,*,#49275,.F.);
#71870=ORIENTED_EDGE('',*,*,#49271,.F.);
#71871=ORIENTED_EDGE('',*,*,#50410,.F.);
#71872=ORIENTED_EDGE('',*,*,#51207,.T.);
#71873=ORIENTED_EDGE('',*,*,#49235,.F.);
#71874=ORIENTED_EDGE('',*,*,#51210,.F.);
#71875=ORIENTED_EDGE('',*,*,#50351,.F.);
#71876=ORIENTED_EDGE('',*,*,#50348,.F.);
#71877=ORIENTED_EDGE('',*,*,#51209,.T.);
#71878=ORIENTED_EDGE('',*,*,#49232,.F.);
#71879=ORIENTED_EDGE('',*,*,#51211,.F.);
#71880=ORIENTED_EDGE('',*,*,#50388,.F.);
#71881=ORIENTED_EDGE('',*,*,#50385,.F.);
#71882=ORIENTED_EDGE('',*,*,#51212,.T.);
#71883=ORIENTED_EDGE('',*,*,#49226,.F.);
#71884=ORIENTED_EDGE('',*,*,#51213,.F.);
#71885=ORIENTED_EDGE('',*,*,#50438,.F.);
#71886=ORIENTED_EDGE('',*,*,#49289,.F.);
#71887=ORIENTED_EDGE('',*,*,#49283,.F.);
#71888=ORIENTED_EDGE('',*,*,#49278,.F.);
#71889=ORIENTED_EDGE('',*,*,#50390,.F.);
#71890=ORIENTED_EDGE('',*,*,#51211,.T.);
#71891=ORIENTED_EDGE('',*,*,#49223,.F.);
#71892=ORIENTED_EDGE('',*,*,#51214,.F.);
#71893=ORIENTED_EDGE('',*,*,#50433,.F.);
#71894=ORIENTED_EDGE('',*,*,#50436,.F.);
#71895=ORIENTED_EDGE('',*,*,#51213,.T.);
#71896=ORIENTED_EDGE('',*,*,#49220,.F.);
#71897=ORIENTED_EDGE('',*,*,#51215,.T.);
#71898=ORIENTED_EDGE('',*,*,#51216,.F.);
#71899=ORIENTED_EDGE('',*,*,#51217,.F.);
#71900=ORIENTED_EDGE('',*,*,#50276,.F.);
#71901=ORIENTED_EDGE('',*,*,#51217,.T.);
#71902=ORIENTED_EDGE('',*,*,#51218,.F.);
#71903=ORIENTED_EDGE('',*,*,#51219,.F.);
#71904=ORIENTED_EDGE('',*,*,#50273,.F.);
#71905=ORIENTED_EDGE('',*,*,#51219,.T.);
#71906=ORIENTED_EDGE('',*,*,#51220,.F.);
#71907=ORIENTED_EDGE('',*,*,#51221,.F.);
#71908=ORIENTED_EDGE('',*,*,#50270,.F.);
#71909=ORIENTED_EDGE('',*,*,#51221,.T.);
#71910=ORIENTED_EDGE('',*,*,#51222,.F.);
#71911=ORIENTED_EDGE('',*,*,#51223,.F.);
#71912=ORIENTED_EDGE('',*,*,#50266,.F.);
#71913=ORIENTED_EDGE('',*,*,#51224,.T.);
#71914=ORIENTED_EDGE('',*,*,#51225,.F.);
#71915=ORIENTED_EDGE('',*,*,#51226,.F.);
#71916=ORIENTED_EDGE('',*,*,#50285,.F.);
#71917=ORIENTED_EDGE('',*,*,#51226,.T.);
#71918=ORIENTED_EDGE('',*,*,#51227,.F.);
#71919=ORIENTED_EDGE('',*,*,#51228,.F.);
#71920=ORIENTED_EDGE('',*,*,#50282,.F.);
#71921=ORIENTED_EDGE('',*,*,#51228,.T.);
#71922=ORIENTED_EDGE('',*,*,#51229,.F.);
#71923=ORIENTED_EDGE('',*,*,#51215,.F.);
#71924=ORIENTED_EDGE('',*,*,#50279,.F.);
#71925=ORIENTED_EDGE('',*,*,#51200,.T.);
#71926=ORIENTED_EDGE('',*,*,#50357,.F.);
#71927=ORIENTED_EDGE('',*,*,#50442,.F.);
#71928=ORIENTED_EDGE('',*,*,#50326,.F.);
#71929=ORIENTED_EDGE('',*,*,#50445,.F.);
#71930=ORIENTED_EDGE('',*,*,#50379,.F.);
#71931=ORIENTED_EDGE('',*,*,#51205,.T.);
#71932=ORIENTED_EDGE('',*,*,#50309,.F.);
#71933=ORIENTED_EDGE('',*,*,#51212,.F.);
#71934=ORIENTED_EDGE('',*,*,#50382,.F.);
#71935=ORIENTED_EDGE('',*,*,#50377,.F.);
#71936=ORIENTED_EDGE('',*,*,#50371,.F.);
#71937=ORIENTED_EDGE('',*,*,#50358,.F.);
#71938=ORIENTED_EDGE('',*,*,#50354,.F.);
#71939=ORIENTED_EDGE('',*,*,#51210,.T.);
#71940=ORIENTED_EDGE('',*,*,#49229,.F.);
#71941=ORIENTED_EDGE('',*,*,#51204,.T.);
#71942=ORIENTED_EDGE('',*,*,#50423,.F.);
#71943=ORIENTED_EDGE('',*,*,#50446,.F.);
#71944=ORIENTED_EDGE('',*,*,#50297,.F.);
#71945=ORIENTED_EDGE('',*,*,#50441,.F.);
#71946=ORIENTED_EDGE('',*,*,#50399,.F.);
#71947=ORIENTED_EDGE('',*,*,#51201,.F.);
#71948=ORIENTED_EDGE('',*,*,#50338,.F.);
#71949=ORIENTED_EDGE('',*,*,#49338,.F.);
#71950=ORIENTED_EDGE('',*,*,#49336,.F.);
#71951=ORIENTED_EDGE('',*,*,#49333,.F.);
#71952=ORIENTED_EDGE('',*,*,#49329,.F.);
#71953=ORIENTED_EDGE('',*,*,#49325,.F.);
#71954=ORIENTED_EDGE('',*,*,#49215,.F.);
#71955=ORIENTED_EDGE('',*,*,#49211,.F.);
#71956=ORIENTED_EDGE('',*,*,#49206,.F.);
#71957=ORIENTED_EDGE('',*,*,#49309,.F.);
#71958=ORIENTED_EDGE('',*,*,#49307,.F.);
#71959=ORIENTED_EDGE('',*,*,#50439,.F.);
#71960=ORIENTED_EDGE('',*,*,#50437,.F.);
#71961=ORIENTED_EDGE('',*,*,#51203,.F.);
#71962=ORIENTED_EDGE('',*,*,#50303,.F.);
#71963=ORIENTED_EDGE('',*,*,#51206,.T.);
#71964=ORIENTED_EDGE('',*,*,#50387,.F.);
#71965=ORIENTED_EDGE('',*,*,#50389,.F.);
#71966=ORIENTED_EDGE('',*,*,#49298,.F.);
#71967=ORIENTED_EDGE('',*,*,#49303,.F.);
#71968=ORIENTED_EDGE('',*,*,#49189,.F.);
#71969=ORIENTED_EDGE('',*,*,#49183,.F.);
#71970=ORIENTED_EDGE('',*,*,#49178,.F.);
#71971=ORIENTED_EDGE('',*,*,#49185,.F.);
#71972=ORIENTED_EDGE('',*,*,#49191,.F.);
#71973=ORIENTED_EDGE('',*,*,#49196,.F.);
#71974=ORIENTED_EDGE('',*,*,#49202,.F.);
#71975=ORIENTED_EDGE('',*,*,#49158,.F.);
#71976=ORIENTED_EDGE('',*,*,#49164,.F.);
#71977=ORIENTED_EDGE('',*,*,#49352,.F.);
#71978=ORIENTED_EDGE('',*,*,#49348,.F.);
#71979=ORIENTED_EDGE('',*,*,#49347,.F.);
#71980=ORIENTED_EDGE('',*,*,#49344,.F.);
#71981=ORIENTED_EDGE('',*,*,#49339,.F.);
#71982=ORIENTED_EDGE('',*,*,#49244,.F.);
#71983=ORIENTED_EDGE('',*,*,#49239,.F.);
#71984=ORIENTED_EDGE('',*,*,#49152,.F.);
#71985=ORIENTED_EDGE('',*,*,#49241,.F.);
#71986=ORIENTED_EDGE('',*,*,#49243,.F.);
#71987=ORIENTED_EDGE('',*,*,#49249,.F.);
#71988=ORIENTED_EDGE('',*,*,#49255,.F.);
#71989=ORIENTED_EDGE('',*,*,#50345,.F.);
#71990=ORIENTED_EDGE('',*,*,#50347,.F.);
#71991=ORIENTED_EDGE('',*,*,#51199,.F.);
#71992=ORIENTED_EDGE('',*,*,#50332,.F.);
#71993=ORIENTED_EDGE('',*,*,#51202,.T.);
#71994=ORIENTED_EDGE('',*,*,#50407,.F.);
#71995=ORIENTED_EDGE('',*,*,#50409,.F.);
#71996=ORIENTED_EDGE('',*,*,#49253,.F.);
#71997=ORIENTED_EDGE('',*,*,#49245,.F.);
#71998=ORIENTED_EDGE('',*,*,#49175,.F.);
#71999=ORIENTED_EDGE('',*,*,#49168,.F.);
#72000=ORIENTED_EDGE('',*,*,#49162,.F.);
#72001=ORIENTED_EDGE('',*,*,#49156,.F.);
#72002=ORIENTED_EDGE('',*,*,#49150,.F.);
#72003=ORIENTED_EDGE('',*,*,#49145,.F.);
#72004=ORIENTED_EDGE('',*,*,#49140,.F.);
#72005=ORIENTED_EDGE('',*,*,#51153,.F.);
#72006=ORIENTED_EDGE('',*,*,#51230,.T.);
#72007=ORIENTED_EDGE('',*,*,#50691,.F.);
#72008=ORIENTED_EDGE('',*,*,#49661,.F.);
#72009=ORIENTED_EDGE('',*,*,#50672,.F.);
#72010=ORIENTED_EDGE('',*,*,#51231,.T.);
#72011=ORIENTED_EDGE('',*,*,#50667,.F.);
#72012=ORIENTED_EDGE('',*,*,#49683,.F.);
#72013=ORIENTED_EDGE('',*,*,#50660,.F.);
#72014=ORIENTED_EDGE('',*,*,#51232,.T.);
#72015=ORIENTED_EDGE('',*,*,#50655,.F.);
#72016=ORIENTED_EDGE('',*,*,#49811,.F.);
#72017=ORIENTED_EDGE('',*,*,#50648,.F.);
#72018=ORIENTED_EDGE('',*,*,#51233,.T.);
#72019=ORIENTED_EDGE('',*,*,#50643,.F.);
#72020=ORIENTED_EDGE('',*,*,#49910,.F.);
#72021=ORIENTED_EDGE('',*,*,#50576,.F.);
#72022=ORIENTED_EDGE('',*,*,#51234,.T.);
#72023=ORIENTED_EDGE('',*,*,#51155,.T.);
#72024=ORIENTED_EDGE('',*,*,#49946,.F.);
#72025=ORIENTED_EDGE('',*,*,#50522,.F.);
#72026=ORIENTED_EDGE('',*,*,#51235,.F.);
#72027=ORIENTED_EDGE('',*,*,#50517,.F.);
#72028=ORIENTED_EDGE('',*,*,#49871,.F.);
#72029=ORIENTED_EDGE('',*,*,#50813,.F.);
#72030=ORIENTED_EDGE('',*,*,#51236,.F.);
#72031=ORIENTED_EDGE('',*,*,#50808,.F.);
#72032=ORIENTED_EDGE('',*,*,#50094,.F.);
#72033=ORIENTED_EDGE('',*,*,#50465,.F.);
#72034=ORIENTED_EDGE('',*,*,#51237,.F.);
#72035=ORIENTED_EDGE('',*,*,#50460,.F.);
#72036=ORIENTED_EDGE('',*,*,#50195,.F.);
#72037=ORIENTED_EDGE('',*,*,#50459,.F.);
#72038=ORIENTED_EDGE('',*,*,#51238,.F.);
#72039=ORIENTED_EDGE('',*,*,#50454,.F.);
#72040=ORIENTED_EDGE('',*,*,#50205,.F.);
#72041=ORIENTED_EDGE('',*,*,#50807,.F.);
#72042=ORIENTED_EDGE('',*,*,#51239,.F.);
#72043=ORIENTED_EDGE('',*,*,#50814,.F.);
#72044=ORIENTED_EDGE('',*,*,#50078,.F.);
#72045=ORIENTED_EDGE('',*,*,#50789,.F.);
#72046=ORIENTED_EDGE('',*,*,#51240,.F.);
#72047=ORIENTED_EDGE('',*,*,#50784,.F.);
#72048=ORIENTED_EDGE('',*,*,#50054,.F.);
#72049=ORIENTED_EDGE('',*,*,#50510,.F.);
#72050=ORIENTED_EDGE('',*,*,#51241,.F.);
#72051=ORIENTED_EDGE('',*,*,#50505,.F.);
#72052=ORIENTED_EDGE('',*,*,#49494,.F.);
#72053=ORIENTED_EDGE('',*,*,#50804,.F.);
#72054=ORIENTED_EDGE('',*,*,#51242,.F.);
#72055=ORIENTED_EDGE('',*,*,#50799,.F.);
#72056=ORIENTED_EDGE('',*,*,#49478,.F.);
#72057=ORIENTED_EDGE('',*,*,#50798,.F.);
#72058=ORIENTED_EDGE('',*,*,#51243,.F.);
#72059=ORIENTED_EDGE('',*,*,#50793,.F.);
#72060=ORIENTED_EDGE('',*,*,#49470,.F.);
#72061=ORIENTED_EDGE('',*,*,#50819,.F.);
#72062=ORIENTED_EDGE('',*,*,#51244,.F.);
#72063=ORIENTED_EDGE('',*,*,#50826,.F.);
#72064=ORIENTED_EDGE('',*,*,#49454,.F.);
#72065=ORIENTED_EDGE('',*,*,#50824,.F.);
#72066=ORIENTED_EDGE('',*,*,#51245,.T.);
#72067=ORIENTED_EDGE('',*,*,#50820,.F.);
#72068=ORIENTED_EDGE('',*,*,#49446,.F.);
#72069=ORIENTED_EDGE('',*,*,#50783,.F.);
#72070=ORIENTED_EDGE('',*,*,#51246,.T.);
#72071=ORIENTED_EDGE('',*,*,#50790,.F.);
#72072=ORIENTED_EDGE('',*,*,#50070,.F.);
#72073=ORIENTED_EDGE('',*,*,#51247,.F.);
#72074=ORIENTED_EDGE('',*,*,#50936,.F.);
#72075=ORIENTED_EDGE('',*,*,#51248,.F.);
#72076=ORIENTED_EDGE('',*,*,#50908,.F.);
#72077=ORIENTED_EDGE('',*,*,#50756,.F.);
#72078=ORIENTED_EDGE('',*,*,#51249,.F.);
#72079=ORIENTED_EDGE('',*,*,#50751,.F.);
#72080=ORIENTED_EDGE('',*,*,#49863,.F.);
#72081=ORIENTED_EDGE('',*,*,#50765,.F.);
#72082=ORIENTED_EDGE('',*,*,#51250,.F.);
#72083=ORIENTED_EDGE('',*,*,#50760,.F.);
#72084=ORIENTED_EDGE('',*,*,#50046,.F.);
#72085=ORIENTED_EDGE('',*,*,#50486,.F.);
#72086=ORIENTED_EDGE('',*,*,#51251,.F.);
#72087=ORIENTED_EDGE('',*,*,#50481,.F.);
#72088=ORIENTED_EDGE('',*,*,#49745,.F.);
#72089=ORIENTED_EDGE('',*,*,#50750,.F.);
#72090=ORIENTED_EDGE('',*,*,#51252,.F.);
#72091=ORIENTED_EDGE('',*,*,#50745,.F.);
#72092=ORIENTED_EDGE('',*,*,#49847,.F.);
#72093=ORIENTED_EDGE('',*,*,#50495,.F.);
#72094=ORIENTED_EDGE('',*,*,#51253,.F.);
#72095=ORIENTED_EDGE('',*,*,#50490,.F.);
#72096=ORIENTED_EDGE('',*,*,#49715,.F.);
#72097=ORIENTED_EDGE('',*,*,#50480,.F.);
#72098=ORIENTED_EDGE('',*,*,#51254,.F.);
#72099=ORIENTED_EDGE('',*,*,#50487,.F.);
#72100=ORIENTED_EDGE('',*,*,#49769,.F.);
#72101=ORIENTED_EDGE('',*,*,#50744,.F.);
#72102=ORIENTED_EDGE('',*,*,#51255,.F.);
#72103=ORIENTED_EDGE('',*,*,#50739,.F.);
#72104=ORIENTED_EDGE('',*,*,#49529,.F.);
#72105=ORIENTED_EDGE('',*,*,#50501,.F.);
#72106=ORIENTED_EDGE('',*,*,#51256,.F.);
#72107=ORIENTED_EDGE('',*,*,#50496,.F.);
#72108=ORIENTED_EDGE('',*,*,#49739,.F.);
#72109=ORIENTED_EDGE('',*,*,#50759,.F.);
#72110=ORIENTED_EDGE('',*,*,#51257,.F.);
#72111=ORIENTED_EDGE('',*,*,#50766,.F.);
#72112=ORIENTED_EDGE('',*,*,#50030,.F.);
#72113=ORIENTED_EDGE('',*,*,#50717,.F.);
#72114=ORIENTED_EDGE('',*,*,#51258,.F.);
#72115=ORIENTED_EDGE('',*,*,#50712,.F.);
#72116=ORIENTED_EDGE('',*,*,#50006,.F.);
#72117=ORIENTED_EDGE('',*,*,#50738,.F.);
#72118=ORIENTED_EDGE('',*,*,#51259,.F.);
#72119=ORIENTED_EDGE('',*,*,#50733,.F.);
#72120=ORIENTED_EDGE('',*,*,#49521,.F.);
#72121=ORIENTED_EDGE('',*,*,#50732,.F.);
#72122=ORIENTED_EDGE('',*,*,#51260,.F.);
#72123=ORIENTED_EDGE('',*,*,#50727,.F.);
#72124=ORIENTED_EDGE('',*,*,#49553,.F.);
#72125=ORIENTED_EDGE('',*,*,#50726,.F.);
#72126=ORIENTED_EDGE('',*,*,#51261,.F.);
#72127=ORIENTED_EDGE('',*,*,#50721,.F.);
#72128=ORIENTED_EDGE('',*,*,#49545,.F.);
#72129=ORIENTED_EDGE('',*,*,#50771,.F.);
#72130=ORIENTED_EDGE('',*,*,#51262,.F.);
#72131=ORIENTED_EDGE('',*,*,#50778,.F.);
#72132=ORIENTED_EDGE('',*,*,#49430,.F.);
#72133=ORIENTED_EDGE('',*,*,#50776,.F.);
#72134=ORIENTED_EDGE('',*,*,#51263,.T.);
#72135=ORIENTED_EDGE('',*,*,#50772,.F.);
#72136=ORIENTED_EDGE('',*,*,#49422,.F.);
#72137=ORIENTED_EDGE('',*,*,#50704,.F.);
#72138=ORIENTED_EDGE('',*,*,#51264,.T.);
#72139=ORIENTED_EDGE('',*,*,#51147,.T.);
#72140=ORIENTED_EDGE('',*,*,#49392,.F.);
#72141=ORIENTED_EDGE('',*,*,#50711,.F.);
#72142=ORIENTED_EDGE('',*,*,#51265,.T.);
#72143=ORIENTED_EDGE('',*,*,#50718,.F.);
#72144=ORIENTED_EDGE('',*,*,#50022,.F.);
#72145=ORIENTED_EDGE('',*,*,#51161,.F.);
#72146=ORIENTED_EDGE('',*,*,#51266,.T.);
#72147=ORIENTED_EDGE('',*,*,#50562,.F.);
#72148=ORIENTED_EDGE('',*,*,#50000,.F.);
#72149=ORIENTED_EDGE('',*,*,#51149,.F.);
#72150=ORIENTED_EDGE('',*,*,#51267,.T.);
#72151=ORIENTED_EDGE('',*,*,#50700,.F.);
#72152=ORIENTED_EDGE('',*,*,#49404,.F.);
#72153=ORIENTED_EDGE('',*,*,#50530,.F.);
#72154=ORIENTED_EDGE('',*,*,#51268,.T.);
#72155=ORIENTED_EDGE('',*,*,#50526,.F.);
#72156=ORIENTED_EDGE('',*,*,#50124,.F.);
#72157=ORIENTED_EDGE('',*,*,#50567,.F.);
#72158=ORIENTED_EDGE('',*,*,#51269,.T.);
#72159=ORIENTED_EDGE('',*,*,#51159,.T.);
#72160=ORIENTED_EDGE('',*,*,#49992,.F.);
#72161=ORIENTED_EDGE('',*,*,#50624,.F.);
#72162=ORIENTED_EDGE('',*,*,#51270,.T.);
#72163=ORIENTED_EDGE('',*,*,#50619,.F.);
#72164=ORIENTED_EDGE('',*,*,#50106,.F.);
#72165=ORIENTED_EDGE('',*,*,#50615,.F.);
#72166=ORIENTED_EDGE('',*,*,#51271,.F.);
#72167=ORIENTED_EDGE('',*,*,#50610,.F.);
#72168=ORIENTED_EDGE('',*,*,#49839,.F.);
#72169=ORIENTED_EDGE('',*,*,#50645,.F.);
#72170=ORIENTED_EDGE('',*,*,#51272,.F.);
#72171=ORIENTED_EDGE('',*,*,#50640,.F.);
#72172=ORIENTED_EDGE('',*,*,#49898,.F.);
#72173=ORIENTED_EDGE('',*,*,#50633,.F.);
#72174=ORIENTED_EDGE('',*,*,#51273,.F.);
#72175=ORIENTED_EDGE('',*,*,#50628,.F.);
#72176=ORIENTED_EDGE('',*,*,#49968,.F.);
#72177=ORIENTED_EDGE('',*,*,#50579,.F.);
#72178=ORIENTED_EDGE('',*,*,#51274,.F.);
#72179=ORIENTED_EDGE('',*,*,#50574,.F.);
#72180=ORIENTED_EDGE('',*,*,#49938,.F.);
#72181=ORIENTED_EDGE('',*,*,#50603,.F.);
#72182=ORIENTED_EDGE('',*,*,#51275,.F.);
#72183=ORIENTED_EDGE('',*,*,#50598,.F.);
#72184=ORIENTED_EDGE('',*,*,#49775,.F.);
#72185=ORIENTED_EDGE('',*,*,#50657,.F.);
#72186=ORIENTED_EDGE('',*,*,#51276,.F.);
#72187=ORIENTED_EDGE('',*,*,#50652,.F.);
#72188=ORIENTED_EDGE('',*,*,#49799,.F.);
#72189=ORIENTED_EDGE('',*,*,#50609,.F.);
#72190=ORIENTED_EDGE('',*,*,#51277,.F.);
#72191=ORIENTED_EDGE('',*,*,#50604,.F.);
#72192=ORIENTED_EDGE('',*,*,#49823,.F.);
#72193=ORIENTED_EDGE('',*,*,#50639,.F.);
#72194=ORIENTED_EDGE('',*,*,#51278,.F.);
#72195=ORIENTED_EDGE('',*,*,#50646,.F.);
#72196=ORIENTED_EDGE('',*,*,#49914,.F.);
#72197=ORIENTED_EDGE('',*,*,#50591,.F.);
#72198=ORIENTED_EDGE('',*,*,#51279,.F.);
#72199=ORIENTED_EDGE('',*,*,#50586,.F.);
#72200=ORIENTED_EDGE('',*,*,#49703,.F.);
#72201=ORIENTED_EDGE('',*,*,#50669,.F.);
#72202=ORIENTED_EDGE('',*,*,#51280,.F.);
#72203=ORIENTED_EDGE('',*,*,#50664,.F.);
#72204=ORIENTED_EDGE('',*,*,#49679,.F.);
#72205=ORIENTED_EDGE('',*,*,#50597,.F.);
#72206=ORIENTED_EDGE('',*,*,#51281,.F.);
#72207=ORIENTED_EDGE('',*,*,#50592,.F.);
#72208=ORIENTED_EDGE('',*,*,#49791,.F.);
#72209=ORIENTED_EDGE('',*,*,#50651,.F.);
#72210=ORIENTED_EDGE('',*,*,#51282,.F.);
#72211=ORIENTED_EDGE('',*,*,#50658,.F.);
#72212=ORIENTED_EDGE('',*,*,#49815,.F.);
#72213=ORIENTED_EDGE('',*,*,#50555,.F.);
#72214=ORIENTED_EDGE('',*,*,#51283,.F.);
#72215=ORIENTED_EDGE('',*,*,#50550,.F.);
#72216=ORIENTED_EDGE('',*,*,#49601,.F.);
#72217=ORIENTED_EDGE('',*,*,#50681,.F.);
#72218=ORIENTED_EDGE('',*,*,#51284,.F.);
#72219=ORIENTED_EDGE('',*,*,#50676,.F.);
#72220=ORIENTED_EDGE('',*,*,#49625,.F.);
#72221=ORIENTED_EDGE('',*,*,#50585,.F.);
#72222=ORIENTED_EDGE('',*,*,#51285,.F.);
#72223=ORIENTED_EDGE('',*,*,#50580,.F.);
#72224=ORIENTED_EDGE('',*,*,#49695,.F.);
#72225=ORIENTED_EDGE('',*,*,#50663,.F.);
#72226=ORIENTED_EDGE('',*,*,#51286,.F.);
#72227=ORIENTED_EDGE('',*,*,#50670,.F.);
#72228=ORIENTED_EDGE('',*,*,#49671,.F.);
#72229=ORIENTED_EDGE('',*,*,#50627,.F.);
#72230=ORIENTED_EDGE('',*,*,#51287,.F.);
#72231=ORIENTED_EDGE('',*,*,#50634,.F.);
#72232=ORIENTED_EDGE('',*,*,#49952,.F.);
#72233=ORIENTED_EDGE('',*,*,#50573,.F.);
#72234=ORIENTED_EDGE('',*,*,#51288,.F.);
#72235=ORIENTED_EDGE('',*,*,#50568,.F.);
#72236=ORIENTED_EDGE('',*,*,#49922,.F.);
#72237=ORIENTED_EDGE('',*,*,#50561,.F.);
#72238=ORIENTED_EDGE('',*,*,#51289,.F.);
#72239=ORIENTED_EDGE('',*,*,#50556,.F.);
#72240=ORIENTED_EDGE('',*,*,#49976,.F.);
#72241=ORIENTED_EDGE('',*,*,#50618,.F.);
#72242=ORIENTED_EDGE('',*,*,#51290,.F.);
#72243=ORIENTED_EDGE('',*,*,#50622,.F.);
#72244=ORIENTED_EDGE('',*,*,#50102,.F.);
#72245=ORIENTED_EDGE('',*,*,#50549,.F.);
#72246=ORIENTED_EDGE('',*,*,#51291,.F.);
#72247=ORIENTED_EDGE('',*,*,#50544,.F.);
#72248=ORIENTED_EDGE('',*,*,#49593,.F.);
#72249=ORIENTED_EDGE('',*,*,#50675,.F.);
#72250=ORIENTED_EDGE('',*,*,#51292,.F.);
#72251=ORIENTED_EDGE('',*,*,#50682,.F.);
#72252=ORIENTED_EDGE('',*,*,#49617,.F.);
#72253=ORIENTED_EDGE('',*,*,#50543,.F.);
#72254=ORIENTED_EDGE('',*,*,#51293,.F.);
#72255=ORIENTED_EDGE('',*,*,#50538,.F.);
#72256=ORIENTED_EDGE('',*,*,#49577,.F.);
#72257=ORIENTED_EDGE('',*,*,#50693,.F.);
#72258=ORIENTED_EDGE('',*,*,#51294,.F.);
#72259=ORIENTED_EDGE('',*,*,#50688,.F.);
#72260=ORIENTED_EDGE('',*,*,#49649,.F.);
#72261=ORIENTED_EDGE('',*,*,#50537,.F.);
#72262=ORIENTED_EDGE('',*,*,#51295,.F.);
#72263=ORIENTED_EDGE('',*,*,#50532,.F.);
#72264=ORIENTED_EDGE('',*,*,#49569,.F.);
#72265=ORIENTED_EDGE('',*,*,#50687,.F.);
#72266=ORIENTED_EDGE('',*,*,#51296,.F.);
#72267=ORIENTED_EDGE('',*,*,#50694,.F.);
#72268=ORIENTED_EDGE('',*,*,#49641,.F.);
#72269=ORIENTED_EDGE('',*,*,#50699,.F.);
#72270=ORIENTED_EDGE('',*,*,#51297,.F.);
#72271=ORIENTED_EDGE('',*,*,#50706,.F.);
#72272=ORIENTED_EDGE('',*,*,#49400,.F.);
#72273=ORIENTED_EDGE('',*,*,#50528,.F.);
#72274=ORIENTED_EDGE('',*,*,#51298,.F.);
#72275=ORIENTED_EDGE('',*,*,#50523,.F.);
#72276=ORIENTED_EDGE('',*,*,#50132,.F.);
#72277=ORIENTED_EDGE('',*,*,#51299,.T.);
#72278=ORIENTED_EDGE('',*,*,#51300,.F.);
#72279=ORIENTED_EDGE('',*,*,#51301,.T.);
#72280=ORIENTED_EDGE('',*,*,#51302,.F.);
#72281=ORIENTED_EDGE('',*,*,#51303,.F.);
#72282=ORIENTED_EDGE('',*,*,#51301,.F.);
#72283=ORIENTED_EDGE('',*,*,#51304,.F.);
#72284=ORIENTED_EDGE('',*,*,#51305,.F.);
#72285=ORIENTED_EDGE('',*,*,#51299,.F.);
#72286=ORIENTED_EDGE('',*,*,#51306,.F.);
#72287=ORIENTED_EDGE('',*,*,#51307,.T.);
#72288=ORIENTED_EDGE('',*,*,#51308,.F.);
#72289=ORIENTED_EDGE('',*,*,#51309,.F.);
#72290=ORIENTED_EDGE('',*,*,#51307,.F.);
#72291=ORIENTED_EDGE('',*,*,#51310,.T.);
#72292=ORIENTED_EDGE('',*,*,#51311,.F.);
#72293=ORIENTED_EDGE('',*,*,#51312,.T.);
#72294=ORIENTED_EDGE('',*,*,#51313,.F.);
#72295=ORIENTED_EDGE('',*,*,#51314,.T.);
#72296=ORIENTED_EDGE('',*,*,#51315,.F.);
#72297=ORIENTED_EDGE('',*,*,#51312,.F.);
#72298=ORIENTED_EDGE('',*,*,#51316,.F.);
#72299=ORIENTED_EDGE('',*,*,#51317,.F.);
#72300=ORIENTED_EDGE('',*,*,#51318,.T.);
#72301=ORIENTED_EDGE('',*,*,#51310,.F.);
#72302=ORIENTED_EDGE('',*,*,#51319,.T.);
#72303=ORIENTED_EDGE('',*,*,#51320,.F.);
#72304=ORIENTED_EDGE('',*,*,#51314,.F.);
#72305=ORIENTED_EDGE('',*,*,#51321,.F.);
#72306=ORIENTED_EDGE('',*,*,#51322,.T.);
#72307=ORIENTED_EDGE('',*,*,#51323,.F.);
#72308=ORIENTED_EDGE('',*,*,#51318,.F.);
#72309=ORIENTED_EDGE('',*,*,#51324,.F.);
#72310=ORIENTED_EDGE('',*,*,#51325,.T.);
#72311=ORIENTED_EDGE('',*,*,#51326,.F.);
#72312=ORIENTED_EDGE('',*,*,#51319,.F.);
#72313=ORIENTED_EDGE('',*,*,#51327,.F.);
#72314=ORIENTED_EDGE('',*,*,#51328,.T.);
#72315=ORIENTED_EDGE('',*,*,#51329,.F.);
#72316=ORIENTED_EDGE('',*,*,#51322,.F.);
#72317=ORIENTED_EDGE('',*,*,#51330,.F.);
#72318=ORIENTED_EDGE('',*,*,#51331,.T.);
#72319=ORIENTED_EDGE('',*,*,#51332,.F.);
#72320=ORIENTED_EDGE('',*,*,#51325,.F.);
#72321=ORIENTED_EDGE('',*,*,#51333,.F.);
#72322=ORIENTED_EDGE('',*,*,#51334,.T.);
#72323=ORIENTED_EDGE('',*,*,#51335,.F.);
#72324=ORIENTED_EDGE('',*,*,#51328,.F.);
#72325=ORIENTED_EDGE('',*,*,#51336,.F.);
#72326=ORIENTED_EDGE('',*,*,#51337,.T.);
#72327=ORIENTED_EDGE('',*,*,#51338,.F.);
#72328=ORIENTED_EDGE('',*,*,#51331,.F.);
#72329=ORIENTED_EDGE('',*,*,#51339,.F.);
#72330=ORIENTED_EDGE('',*,*,#51340,.T.);
#72331=ORIENTED_EDGE('',*,*,#51341,.F.);
#72332=ORIENTED_EDGE('',*,*,#51334,.F.);
#72333=ORIENTED_EDGE('',*,*,#51342,.F.);
#72334=ORIENTED_EDGE('',*,*,#51343,.T.);
#72335=ORIENTED_EDGE('',*,*,#51344,.F.);
#72336=ORIENTED_EDGE('',*,*,#51337,.F.);
#72337=ORIENTED_EDGE('',*,*,#51345,.F.);
#72338=ORIENTED_EDGE('',*,*,#51346,.F.);
#72339=ORIENTED_EDGE('',*,*,#51340,.F.);
#72340=ORIENTED_EDGE('',*,*,#51347,.F.);
#72341=ORIENTED_EDGE('',*,*,#51343,.F.);
#72342=ORIENTED_EDGE('',*,*,#51348,.T.);
#72343=ORIENTED_EDGE('',*,*,#51349,.F.);
#72344=ORIENTED_EDGE('',*,*,#51350,.T.);
#72345=ORIENTED_EDGE('',*,*,#51351,.F.);
#72346=ORIENTED_EDGE('',*,*,#51352,.T.);
#72347=ORIENTED_EDGE('',*,*,#51353,.F.);
#72348=ORIENTED_EDGE('',*,*,#51350,.F.);
#72349=ORIENTED_EDGE('',*,*,#51354,.F.);
#72350=ORIENTED_EDGE('',*,*,#51355,.T.);
#72351=ORIENTED_EDGE('',*,*,#51356,.F.);
#72352=ORIENTED_EDGE('',*,*,#51348,.F.);
#72353=ORIENTED_EDGE('',*,*,#51357,.F.);
#72354=ORIENTED_EDGE('',*,*,#51358,.T.);
#72355=ORIENTED_EDGE('',*,*,#51359,.F.);
#72356=ORIENTED_EDGE('',*,*,#51352,.F.);
#72357=ORIENTED_EDGE('',*,*,#51360,.F.);
#72358=ORIENTED_EDGE('',*,*,#51361,.T.);
#72359=ORIENTED_EDGE('',*,*,#51362,.F.);
#72360=ORIENTED_EDGE('',*,*,#51355,.F.);
#72361=ORIENTED_EDGE('',*,*,#51363,.F.);
#72362=ORIENTED_EDGE('',*,*,#51364,.T.);
#72363=ORIENTED_EDGE('',*,*,#51365,.F.);
#72364=ORIENTED_EDGE('',*,*,#51358,.F.);
#72365=ORIENTED_EDGE('',*,*,#51366,.T.);
#72366=ORIENTED_EDGE('',*,*,#51367,.F.);
#72367=ORIENTED_EDGE('',*,*,#51361,.F.);
#72368=ORIENTED_EDGE('',*,*,#51368,.F.);
#72369=ORIENTED_EDGE('',*,*,#51369,.T.);
#72370=ORIENTED_EDGE('',*,*,#51370,.F.);
#72371=ORIENTED_EDGE('',*,*,#51364,.F.);
#72372=ORIENTED_EDGE('',*,*,#51371,.F.);
#72373=ORIENTED_EDGE('',*,*,#51372,.T.);
#72374=ORIENTED_EDGE('',*,*,#51373,.F.);
#72375=ORIENTED_EDGE('',*,*,#51366,.F.);
#72376=ORIENTED_EDGE('',*,*,#51374,.F.);
#72377=ORIENTED_EDGE('',*,*,#51375,.T.);
#72378=ORIENTED_EDGE('',*,*,#51376,.F.);
#72379=ORIENTED_EDGE('',*,*,#51369,.F.);
#72380=ORIENTED_EDGE('',*,*,#51377,.F.);
#72381=ORIENTED_EDGE('',*,*,#51378,.F.);
#72382=ORIENTED_EDGE('',*,*,#51379,.T.);
#72383=ORIENTED_EDGE('',*,*,#51372,.F.);
#72384=ORIENTED_EDGE('',*,*,#51380,.T.);
#72385=ORIENTED_EDGE('',*,*,#51381,.F.);
#72386=ORIENTED_EDGE('',*,*,#51375,.F.);
#72387=ORIENTED_EDGE('',*,*,#51382,.F.);
#72388=ORIENTED_EDGE('',*,*,#51383,.T.);
#72389=ORIENTED_EDGE('',*,*,#51384,.F.);
#72390=ORIENTED_EDGE('',*,*,#51379,.F.);
#72391=ORIENTED_EDGE('',*,*,#51385,.F.);
#72392=ORIENTED_EDGE('',*,*,#51380,.F.);
#72393=ORIENTED_EDGE('',*,*,#51386,.F.);
#72394=ORIENTED_EDGE('',*,*,#51383,.F.);
#72395=ORIENTED_EDGE('',*,*,#51387,.F.);
#72396=ORIENTED_EDGE('',*,*,#51388,.F.);
#72397=ORIENTED_EDGE('',*,*,#49219,.F.);
#72398=ORIENTED_EDGE('',*,*,#51389,.F.);
#72399=ORIENTED_EDGE('',*,*,#51390,.T.);
#72400=ORIENTED_EDGE('',*,*,#51391,.T.);
#72401=ORIENTED_EDGE('',*,*,#51392,.F.);
#72402=ORIENTED_EDGE('',*,*,#51390,.F.);
#72403=ORIENTED_EDGE('',*,*,#51393,.F.);
#72404=ORIENTED_EDGE('',*,*,#51394,.T.);
#72405=ORIENTED_EDGE('',*,*,#51395,.F.);
#72406=ORIENTED_EDGE('',*,*,#51391,.F.);
#72407=ORIENTED_EDGE('',*,*,#51396,.F.);
#72408=ORIENTED_EDGE('',*,*,#51397,.T.);
#72409=ORIENTED_EDGE('',*,*,#51398,.F.);
#72410=ORIENTED_EDGE('',*,*,#51394,.F.);
#72411=ORIENTED_EDGE('',*,*,#51399,.F.);
#72412=ORIENTED_EDGE('',*,*,#51400,.T.);
#72413=ORIENTED_EDGE('',*,*,#51401,.F.);
#72414=ORIENTED_EDGE('',*,*,#51397,.F.);
#72415=ORIENTED_EDGE('',*,*,#51402,.F.);
#72416=ORIENTED_EDGE('',*,*,#51403,.T.);
#72417=ORIENTED_EDGE('',*,*,#51404,.F.);
#72418=ORIENTED_EDGE('',*,*,#51400,.F.);
#72419=ORIENTED_EDGE('',*,*,#51405,.F.);
#72420=ORIENTED_EDGE('',*,*,#51406,.T.);
#72421=ORIENTED_EDGE('',*,*,#51407,.F.);
#72422=ORIENTED_EDGE('',*,*,#51403,.F.);
#72423=ORIENTED_EDGE('',*,*,#51408,.F.);
#72424=ORIENTED_EDGE('',*,*,#51409,.T.);
#72425=ORIENTED_EDGE('',*,*,#51410,.F.);
#72426=ORIENTED_EDGE('',*,*,#51406,.F.);
#72427=ORIENTED_EDGE('',*,*,#51411,.F.);
#72428=ORIENTED_EDGE('',*,*,#51412,.F.);
#72429=ORIENTED_EDGE('',*,*,#49236,.T.);
#72430=ORIENTED_EDGE('',*,*,#51413,.F.);
#72431=ORIENTED_EDGE('',*,*,#51409,.F.);
#72432=ORIENTED_EDGE('',*,*,#51414,.F.);
#72433=ORIENTED_EDGE('',*,*,#51317,.T.);
#72434=ORIENTED_EDGE('',*,*,#51415,.F.);
#72435=ORIENTED_EDGE('',*,*,#51416,.T.);
#72436=ORIENTED_EDGE('',*,*,#51417,.T.);
#72437=ORIENTED_EDGE('',*,*,#51418,.F.);
#72438=ORIENTED_EDGE('',*,*,#51416,.F.);
#72439=ORIENTED_EDGE('',*,*,#51419,.F.);
#72440=ORIENTED_EDGE('',*,*,#51420,.F.);
#72441=ORIENTED_EDGE('',*,*,#51347,.T.);
#72442=ORIENTED_EDGE('',*,*,#51421,.F.);
#72443=ORIENTED_EDGE('',*,*,#51422,.T.);
#72444=ORIENTED_EDGE('',*,*,#51423,.T.);
#72445=ORIENTED_EDGE('',*,*,#51424,.F.);
#72446=ORIENTED_EDGE('',*,*,#51417,.F.);
#72447=ORIENTED_EDGE('',*,*,#51425,.F.);
#72448=ORIENTED_EDGE('',*,*,#51426,.T.);
#72449=ORIENTED_EDGE('',*,*,#51427,.F.);
#72450=ORIENTED_EDGE('',*,*,#51422,.F.);
#72451=ORIENTED_EDGE('',*,*,#51428,.F.);
#72452=ORIENTED_EDGE('',*,*,#51429,.T.);
#72453=ORIENTED_EDGE('',*,*,#51430,.F.);
#72454=ORIENTED_EDGE('',*,*,#51423,.F.);
#72455=ORIENTED_EDGE('',*,*,#51431,.F.);
#72456=ORIENTED_EDGE('',*,*,#51432,.T.);
#72457=ORIENTED_EDGE('',*,*,#51433,.F.);
#72458=ORIENTED_EDGE('',*,*,#51426,.F.);
#72459=ORIENTED_EDGE('',*,*,#51434,.F.);
#72460=ORIENTED_EDGE('',*,*,#51435,.T.);
#72461=ORIENTED_EDGE('',*,*,#51436,.F.);
#72462=ORIENTED_EDGE('',*,*,#51429,.F.);
#72463=ORIENTED_EDGE('',*,*,#51437,.F.);
#72464=ORIENTED_EDGE('',*,*,#51438,.T.);
#72465=ORIENTED_EDGE('',*,*,#51439,.F.);
#72466=ORIENTED_EDGE('',*,*,#51432,.F.);
#72467=ORIENTED_EDGE('',*,*,#51440,.F.);
#72468=ORIENTED_EDGE('',*,*,#51441,.T.);
#72469=ORIENTED_EDGE('',*,*,#51442,.F.);
#72470=ORIENTED_EDGE('',*,*,#51435,.F.);
#72471=ORIENTED_EDGE('',*,*,#51443,.F.);
#72472=ORIENTED_EDGE('',*,*,#51444,.T.);
#72473=ORIENTED_EDGE('',*,*,#51445,.F.);
#72474=ORIENTED_EDGE('',*,*,#51438,.F.);
#72475=ORIENTED_EDGE('',*,*,#51446,.F.);
#72476=ORIENTED_EDGE('',*,*,#51447,.T.);
#72477=ORIENTED_EDGE('',*,*,#51448,.F.);
#72478=ORIENTED_EDGE('',*,*,#51441,.F.);
#72479=ORIENTED_EDGE('',*,*,#51449,.F.);
#72480=ORIENTED_EDGE('',*,*,#51444,.F.);
#72481=ORIENTED_EDGE('',*,*,#51450,.F.);
#72482=ORIENTED_EDGE('',*,*,#51447,.F.);
#72483=ORIENTED_EDGE('',*,*,#51451,.F.);
#72484=ORIENTED_EDGE('',*,*,#51452,.T.);
#72485=ORIENTED_EDGE('',*,*,#51453,.F.);
#72486=ORIENTED_EDGE('',*,*,#51454,.T.);
#72487=ORIENTED_EDGE('',*,*,#51455,.F.);
#72488=ORIENTED_EDGE('',*,*,#51456,.T.);
#72489=ORIENTED_EDGE('',*,*,#51457,.F.);
#72490=ORIENTED_EDGE('',*,*,#51454,.F.);
#72491=ORIENTED_EDGE('',*,*,#51458,.F.);
#72492=ORIENTED_EDGE('',*,*,#51459,.T.);
#72493=ORIENTED_EDGE('',*,*,#51460,.F.);
#72494=ORIENTED_EDGE('',*,*,#51452,.F.);
#72495=ORIENTED_EDGE('',*,*,#51461,.F.);
#72496=ORIENTED_EDGE('',*,*,#51462,.T.);
#72497=ORIENTED_EDGE('',*,*,#51463,.F.);
#72498=ORIENTED_EDGE('',*,*,#51456,.F.);
#72499=ORIENTED_EDGE('',*,*,#51464,.F.);
#72500=ORIENTED_EDGE('',*,*,#51465,.T.);
#72501=ORIENTED_EDGE('',*,*,#51466,.F.);
#72502=ORIENTED_EDGE('',*,*,#51459,.F.);
#72503=ORIENTED_EDGE('',*,*,#51467,.F.);
#72504=ORIENTED_EDGE('',*,*,#51468,.T.);
#72505=ORIENTED_EDGE('',*,*,#51469,.F.);
#72506=ORIENTED_EDGE('',*,*,#51462,.F.);
#72507=ORIENTED_EDGE('',*,*,#51470,.F.);
#72508=ORIENTED_EDGE('',*,*,#51471,.F.);
#72509=ORIENTED_EDGE('',*,*,#51472,.T.);
#72510=ORIENTED_EDGE('',*,*,#51473,.F.);
#72511=ORIENTED_EDGE('',*,*,#51465,.F.);
#72512=ORIENTED_EDGE('',*,*,#51474,.F.);
#72513=ORIENTED_EDGE('',*,*,#51475,.T.);
#72514=ORIENTED_EDGE('',*,*,#51476,.F.);
#72515=ORIENTED_EDGE('',*,*,#51468,.F.);
#72516=ORIENTED_EDGE('',*,*,#51477,.F.);
#72517=ORIENTED_EDGE('',*,*,#51478,.F.);
#72518=ORIENTED_EDGE('',*,*,#51365,.T.);
#72519=ORIENTED_EDGE('',*,*,#51479,.F.);
#72520=ORIENTED_EDGE('',*,*,#51472,.F.);
#72521=ORIENTED_EDGE('',*,*,#51480,.T.);
#72522=ORIENTED_EDGE('',*,*,#51481,.F.);
#72523=ORIENTED_EDGE('',*,*,#51475,.F.);
#72524=ORIENTED_EDGE('',*,*,#51482,.F.);
#72525=ORIENTED_EDGE('',*,*,#51483,.F.);
#72526=ORIENTED_EDGE('',*,*,#51378,.T.);
#72527=ORIENTED_EDGE('',*,*,#51484,.F.);
#72528=ORIENTED_EDGE('',*,*,#51480,.F.);
#72529=ORIENTED_EDGE('',*,*,#51485,.F.);
#72530=ORIENTED_EDGE('',*,*,#51362,.T.);
#72531=ORIENTED_EDGE('',*,*,#51486,.F.);
#72532=ORIENTED_EDGE('',*,*,#51487,.T.);
#72533=ORIENTED_EDGE('',*,*,#51488,.F.);
#72534=ORIENTED_EDGE('',*,*,#51489,.T.);
#72535=ORIENTED_EDGE('',*,*,#51490,.F.);
#72536=ORIENTED_EDGE('',*,*,#51487,.F.);
#72537=ORIENTED_EDGE('',*,*,#51491,.F.);
#72538=ORIENTED_EDGE('',*,*,#51302,.T.);
#72539=ORIENTED_EDGE('',*,*,#51492,.F.);
#72540=ORIENTED_EDGE('',*,*,#51489,.F.);
#72541=ORIENTED_EDGE('',*,*,#51493,.F.);
#72542=ORIENTED_EDGE('',*,*,#51494,.T.);
#72543=ORIENTED_EDGE('',*,*,#51495,.T.);
#72544=ORIENTED_EDGE('',*,*,#51496,.F.);
#72545=ORIENTED_EDGE('',*,*,#51494,.F.);
#72546=ORIENTED_EDGE('',*,*,#51497,.F.);
#72547=ORIENTED_EDGE('',*,*,#51498,.F.);
#72548=ORIENTED_EDGE('',*,*,#51349,.T.);
#72549=ORIENTED_EDGE('',*,*,#51499,.F.);
#72550=ORIENTED_EDGE('',*,*,#51495,.F.);
#72551=ORIENTED_EDGE('',*,*,#51500,.F.);
#72552=ORIENTED_EDGE('',*,*,#51385,.T.);
#72553=ORIENTED_EDGE('',*,*,#51483,.T.);
#72554=ORIENTED_EDGE('',*,*,#51501,.F.);
#72555=ORIENTED_EDGE('',*,*,#51502,.T.);
#72556=ORIENTED_EDGE('',*,*,#51503,.F.);
#72557=ORIENTED_EDGE('',*,*,#51504,.T.);
#72558=ORIENTED_EDGE('',*,*,#51505,.F.);
#72559=ORIENTED_EDGE('',*,*,#51502,.F.);
#72560=ORIENTED_EDGE('',*,*,#51506,.T.);
#72561=ORIENTED_EDGE('',*,*,#51507,.F.);
#72562=ORIENTED_EDGE('',*,*,#51504,.F.);
#72563=ORIENTED_EDGE('',*,*,#51508,.F.);
#72564=ORIENTED_EDGE('',*,*,#51509,.T.);
#72565=ORIENTED_EDGE('',*,*,#51510,.F.);
#72566=ORIENTED_EDGE('',*,*,#51506,.F.);
#72567=ORIENTED_EDGE('',*,*,#51511,.F.);
#72568=ORIENTED_EDGE('',*,*,#51479,.T.);
#72569=ORIENTED_EDGE('',*,*,#51370,.T.);
#72570=ORIENTED_EDGE('',*,*,#51512,.F.);
#72571=ORIENTED_EDGE('',*,*,#51509,.F.);
#72572=ORIENTED_EDGE('',*,*,#51513,.F.);
#72573=ORIENTED_EDGE('',*,*,#51514,.F.);
#72574=ORIENTED_EDGE('',*,*,#51424,.T.);
#72575=ORIENTED_EDGE('',*,*,#51515,.F.);
#72576=ORIENTED_EDGE('',*,*,#51516,.T.);
#72577=ORIENTED_EDGE('',*,*,#51517,.T.);
#72578=ORIENTED_EDGE('',*,*,#51518,.F.);
#72579=ORIENTED_EDGE('',*,*,#51516,.F.);
#72580=ORIENTED_EDGE('',*,*,#51519,.F.);
#72581=ORIENTED_EDGE('',*,*,#51520,.T.);
#72582=ORIENTED_EDGE('',*,*,#51521,.F.);
#72583=ORIENTED_EDGE('',*,*,#51517,.F.);
#72584=ORIENTED_EDGE('',*,*,#51522,.F.);
#72585=ORIENTED_EDGE('',*,*,#51523,.F.);
#72586=ORIENTED_EDGE('',*,*,#51520,.F.);
#72587=ORIENTED_EDGE('',*,*,#51524,.F.);
#72588=ORIENTED_EDGE('',*,*,#51525,.T.);
#72589=ORIENTED_EDGE('',*,*,#51421,.T.);
#72590=ORIENTED_EDGE('',*,*,#51342,.T.);
#72591=ORIENTED_EDGE('',*,*,#51526,.F.);
#72592=ORIENTED_EDGE('',*,*,#51525,.F.);
#72593=ORIENTED_EDGE('',*,*,#51527,.F.);
#72594=ORIENTED_EDGE('',*,*,#51528,.F.);
#72595=ORIENTED_EDGE('',*,*,#51321,.T.);
#72596=ORIENTED_EDGE('',*,*,#51529,.F.);
#72597=ORIENTED_EDGE('',*,*,#51530,.T.);
#72598=ORIENTED_EDGE('',*,*,#51531,.T.);
#72599=ORIENTED_EDGE('',*,*,#51532,.F.);
#72600=ORIENTED_EDGE('',*,*,#51530,.F.);
#72601=ORIENTED_EDGE('',*,*,#51533,.F.);
#72602=ORIENTED_EDGE('',*,*,#51534,.T.);
#72603=ORIENTED_EDGE('',*,*,#51535,.F.);
#72604=ORIENTED_EDGE('',*,*,#51531,.F.);
#72605=ORIENTED_EDGE('',*,*,#51536,.F.);
#72606=ORIENTED_EDGE('',*,*,#51537,.F.);
#72607=ORIENTED_EDGE('',*,*,#51534,.F.);
#72608=ORIENTED_EDGE('',*,*,#51538,.F.);
#72609=ORIENTED_EDGE('',*,*,#51539,.T.);
#72610=ORIENTED_EDGE('',*,*,#51540,.F.);
#72611=ORIENTED_EDGE('',*,*,#51333,.T.);
#72612=ORIENTED_EDGE('',*,*,#51541,.F.);
#72613=ORIENTED_EDGE('',*,*,#51539,.F.);
#72614=ORIENTED_EDGE('',*,*,#51542,.F.);
#72615=ORIENTED_EDGE('',*,*,#51453,.T.);
#72616=ORIENTED_EDGE('',*,*,#51460,.T.);
#72617=ORIENTED_EDGE('',*,*,#51543,.F.);
#72618=ORIENTED_EDGE('',*,*,#51511,.T.);
#72619=ORIENTED_EDGE('',*,*,#51470,.T.);
#72620=ORIENTED_EDGE('',*,*,#51464,.T.);
#72621=ORIENTED_EDGE('',*,*,#51544,.F.);
#72622=ORIENTED_EDGE('',*,*,#51503,.T.);
#72623=ORIENTED_EDGE('',*,*,#51545,.F.);
#72624=ORIENTED_EDGE('',*,*,#51471,.T.);
#72625=ORIENTED_EDGE('',*,*,#51546,.F.);
#72626=ORIENTED_EDGE('',*,*,#51377,.T.);
#72627=ORIENTED_EDGE('',*,*,#51371,.T.);
#72628=ORIENTED_EDGE('',*,*,#51360,.T.);
#72629=ORIENTED_EDGE('',*,*,#51547,.F.);
#72630=ORIENTED_EDGE('',*,*,#51497,.T.);
#72631=ORIENTED_EDGE('',*,*,#51548,.F.);
#72632=ORIENTED_EDGE('',*,*,#51373,.T.);
#72633=ORIENTED_EDGE('',*,*,#51384,.T.);
#72634=ORIENTED_EDGE('',*,*,#51386,.T.);
#72635=ORIENTED_EDGE('',*,*,#51549,.F.);
#72636=ORIENTED_EDGE('',*,*,#51488,.T.);
#72637=ORIENTED_EDGE('',*,*,#51550,.F.);
#72638=ORIENTED_EDGE('',*,*,#51311,.T.);
#72639=ORIENTED_EDGE('',*,*,#51323,.T.);
#72640=ORIENTED_EDGE('',*,*,#51551,.F.);
#72641=ORIENTED_EDGE('',*,*,#51533,.T.);
#72642=ORIENTED_EDGE('',*,*,#51538,.T.);
#72643=ORIENTED_EDGE('',*,*,#51552,.F.);
#72644=ORIENTED_EDGE('',*,*,#51335,.T.);
#72645=ORIENTED_EDGE('',*,*,#51341,.T.);
#72646=ORIENTED_EDGE('',*,*,#51346,.T.);
#72647=ORIENTED_EDGE('',*,*,#51345,.T.);
#72648=ORIENTED_EDGE('',*,*,#51553,.F.);
#72649=ORIENTED_EDGE('',*,*,#51446,.T.);
#72650=ORIENTED_EDGE('',*,*,#51440,.T.);
#72651=ORIENTED_EDGE('',*,*,#51554,.F.);
#72652=ORIENTED_EDGE('',*,*,#51524,.T.);
#72653=ORIENTED_EDGE('',*,*,#51555,.F.);
#72654=ORIENTED_EDGE('',*,*,#51442,.T.);
#72655=ORIENTED_EDGE('',*,*,#51448,.T.);
#72656=ORIENTED_EDGE('',*,*,#51556,.F.);
#72657=ORIENTED_EDGE('',*,*,#51519,.T.);
#72658=ORIENTED_EDGE('',*,*,#51557,.F.);
#72659=ORIENTED_EDGE('',*,*,#51558,.F.);
#72660=ORIENTED_EDGE('',*,*,#51559,.T.);
#72661=ORIENTED_EDGE('',*,*,#51560,.F.);
#72662=ORIENTED_EDGE('',*,*,#51561,.T.);
#72663=ORIENTED_EDGE('',*,*,#51562,.T.);
#72664=ORIENTED_EDGE('',*,*,#51563,.F.);
#72665=ORIENTED_EDGE('',*,*,#51561,.F.);
#72666=ORIENTED_EDGE('',*,*,#51564,.F.);
#72667=ORIENTED_EDGE('',*,*,#51565,.T.);
#72668=ORIENTED_EDGE('',*,*,#51566,.F.);
#72669=ORIENTED_EDGE('',*,*,#51559,.F.);
#72670=ORIENTED_EDGE('',*,*,#51567,.F.);
#72671=ORIENTED_EDGE('',*,*,#51568,.T.);
#72672=ORIENTED_EDGE('',*,*,#51569,.F.);
#72673=ORIENTED_EDGE('',*,*,#51562,.F.);
#72674=ORIENTED_EDGE('',*,*,#51570,.F.);
#72675=ORIENTED_EDGE('',*,*,#51571,.T.);
#72676=ORIENTED_EDGE('',*,*,#51572,.F.);
#72677=ORIENTED_EDGE('',*,*,#51565,.F.);
#72678=ORIENTED_EDGE('',*,*,#51573,.F.);
#72679=ORIENTED_EDGE('',*,*,#51574,.T.);
#72680=ORIENTED_EDGE('',*,*,#51575,.F.);
#72681=ORIENTED_EDGE('',*,*,#51568,.F.);
#72682=ORIENTED_EDGE('',*,*,#51576,.F.);
#72683=ORIENTED_EDGE('',*,*,#51577,.T.);
#72684=ORIENTED_EDGE('',*,*,#51578,.F.);
#72685=ORIENTED_EDGE('',*,*,#51571,.F.);
#72686=ORIENTED_EDGE('',*,*,#51579,.F.);
#72687=ORIENTED_EDGE('',*,*,#51580,.T.);
#72688=ORIENTED_EDGE('',*,*,#51581,.F.);
#72689=ORIENTED_EDGE('',*,*,#51574,.F.);
#72690=ORIENTED_EDGE('',*,*,#51582,.F.);
#72691=ORIENTED_EDGE('',*,*,#51583,.T.);
#72692=ORIENTED_EDGE('',*,*,#51584,.F.);
#72693=ORIENTED_EDGE('',*,*,#51577,.F.);
#72694=ORIENTED_EDGE('',*,*,#51585,.F.);
#72695=ORIENTED_EDGE('',*,*,#51580,.F.);
#72696=ORIENTED_EDGE('',*,*,#51586,.F.);
#72697=ORIENTED_EDGE('',*,*,#51583,.F.);
#72698=ORIENTED_EDGE('',*,*,#51587,.F.);
#72699=ORIENTED_EDGE('',*,*,#51588,.F.);
#72700=ORIENTED_EDGE('',*,*,#51589,.T.);
#72701=ORIENTED_EDGE('',*,*,#51590,.F.);
#72702=ORIENTED_EDGE('',*,*,#51591,.T.);
#72703=ORIENTED_EDGE('',*,*,#51592,.T.);
#72704=ORIENTED_EDGE('',*,*,#51593,.F.);
#72705=ORIENTED_EDGE('',*,*,#51591,.F.);
#72706=ORIENTED_EDGE('',*,*,#51594,.F.);
#72707=ORIENTED_EDGE('',*,*,#51595,.T.);
#72708=ORIENTED_EDGE('',*,*,#51596,.F.);
#72709=ORIENTED_EDGE('',*,*,#51589,.F.);
#72710=ORIENTED_EDGE('',*,*,#51597,.F.);
#72711=ORIENTED_EDGE('',*,*,#51598,.T.);
#72712=ORIENTED_EDGE('',*,*,#51599,.F.);
#72713=ORIENTED_EDGE('',*,*,#51592,.F.);
#72714=ORIENTED_EDGE('',*,*,#51600,.F.);
#72715=ORIENTED_EDGE('',*,*,#51601,.T.);
#72716=ORIENTED_EDGE('',*,*,#51602,.F.);
#72717=ORIENTED_EDGE('',*,*,#51595,.F.);
#72718=ORIENTED_EDGE('',*,*,#51603,.F.);
#72719=ORIENTED_EDGE('',*,*,#51604,.T.);
#72720=ORIENTED_EDGE('',*,*,#51605,.F.);
#72721=ORIENTED_EDGE('',*,*,#51598,.F.);
#72722=ORIENTED_EDGE('',*,*,#51606,.F.);
#72723=ORIENTED_EDGE('',*,*,#51607,.T.);
#72724=ORIENTED_EDGE('',*,*,#51608,.F.);
#72725=ORIENTED_EDGE('',*,*,#51601,.F.);
#72726=ORIENTED_EDGE('',*,*,#51609,.F.);
#72727=ORIENTED_EDGE('',*,*,#51604,.F.);
#72728=ORIENTED_EDGE('',*,*,#51610,.F.);
#72729=ORIENTED_EDGE('',*,*,#51607,.F.);
#72730=ORIENTED_EDGE('',*,*,#51611,.F.);
#72731=ORIENTED_EDGE('',*,*,#51612,.F.);
#72732=ORIENTED_EDGE('',*,*,#51613,.T.);
#72733=ORIENTED_EDGE('',*,*,#51614,.F.);
#72734=ORIENTED_EDGE('',*,*,#51615,.T.);
#72735=ORIENTED_EDGE('',*,*,#51616,.T.);
#72736=ORIENTED_EDGE('',*,*,#51617,.F.);
#72737=ORIENTED_EDGE('',*,*,#51615,.F.);
#72738=ORIENTED_EDGE('',*,*,#51618,.F.);
#72739=ORIENTED_EDGE('',*,*,#51619,.T.);
#72740=ORIENTED_EDGE('',*,*,#51620,.F.);
#72741=ORIENTED_EDGE('',*,*,#51613,.F.);
#72742=ORIENTED_EDGE('',*,*,#51621,.F.);
#72743=ORIENTED_EDGE('',*,*,#51622,.T.);
#72744=ORIENTED_EDGE('',*,*,#51623,.F.);
#72745=ORIENTED_EDGE('',*,*,#51616,.F.);
#72746=ORIENTED_EDGE('',*,*,#51624,.F.);
#72747=ORIENTED_EDGE('',*,*,#51625,.T.);
#72748=ORIENTED_EDGE('',*,*,#51626,.F.);
#72749=ORIENTED_EDGE('',*,*,#51619,.F.);
#72750=ORIENTED_EDGE('',*,*,#51627,.F.);
#72751=ORIENTED_EDGE('',*,*,#51628,.T.);
#72752=ORIENTED_EDGE('',*,*,#51629,.F.);
#72753=ORIENTED_EDGE('',*,*,#51622,.F.);
#72754=ORIENTED_EDGE('',*,*,#51630,.F.);
#72755=ORIENTED_EDGE('',*,*,#51631,.T.);
#72756=ORIENTED_EDGE('',*,*,#51632,.F.);
#72757=ORIENTED_EDGE('',*,*,#51625,.F.);
#72758=ORIENTED_EDGE('',*,*,#51633,.F.);
#72759=ORIENTED_EDGE('',*,*,#51628,.F.);
#72760=ORIENTED_EDGE('',*,*,#51634,.F.);
#72761=ORIENTED_EDGE('',*,*,#51631,.F.);
#72762=ORIENTED_EDGE('',*,*,#51635,.F.);
#72763=ORIENTED_EDGE('',*,*,#51636,.T.);
#72764=ORIENTED_EDGE('',*,*,#51637,.F.);
#72765=ORIENTED_EDGE('',*,*,#51638,.T.);
#72766=ORIENTED_EDGE('',*,*,#51639,.F.);
#72767=ORIENTED_EDGE('',*,*,#51640,.T.);
#72768=ORIENTED_EDGE('',*,*,#51641,.F.);
#72769=ORIENTED_EDGE('',*,*,#51638,.F.);
#72770=ORIENTED_EDGE('',*,*,#51642,.F.);
#72771=ORIENTED_EDGE('',*,*,#51643,.T.);
#72772=ORIENTED_EDGE('',*,*,#51644,.F.);
#72773=ORIENTED_EDGE('',*,*,#51636,.F.);
#72774=ORIENTED_EDGE('',*,*,#51645,.F.);
#72775=ORIENTED_EDGE('',*,*,#51646,.T.);
#72776=ORIENTED_EDGE('',*,*,#51647,.F.);
#72777=ORIENTED_EDGE('',*,*,#51640,.F.);
#72778=ORIENTED_EDGE('',*,*,#51648,.F.);
#72779=ORIENTED_EDGE('',*,*,#51649,.T.);
#72780=ORIENTED_EDGE('',*,*,#51650,.F.);
#72781=ORIENTED_EDGE('',*,*,#51643,.F.);
#72782=ORIENTED_EDGE('',*,*,#51651,.F.);
#72783=ORIENTED_EDGE('',*,*,#51652,.T.);
#72784=ORIENTED_EDGE('',*,*,#51653,.F.);
#72785=ORIENTED_EDGE('',*,*,#51646,.F.);
#72786=ORIENTED_EDGE('',*,*,#51654,.F.);
#72787=ORIENTED_EDGE('',*,*,#51655,.T.);
#72788=ORIENTED_EDGE('',*,*,#51656,.F.);
#72789=ORIENTED_EDGE('',*,*,#51649,.F.);
#72790=ORIENTED_EDGE('',*,*,#51657,.F.);
#72791=ORIENTED_EDGE('',*,*,#51652,.F.);
#72792=ORIENTED_EDGE('',*,*,#51658,.F.);
#72793=ORIENTED_EDGE('',*,*,#51655,.F.);
#72794=ORIENTED_EDGE('',*,*,#51659,.F.);
#72795=ORIENTED_EDGE('',*,*,#51660,.T.);
#72796=ORIENTED_EDGE('',*,*,#51661,.F.);
#72797=ORIENTED_EDGE('',*,*,#51662,.T.);
#72798=ORIENTED_EDGE('',*,*,#51663,.F.);
#72799=ORIENTED_EDGE('',*,*,#51664,.T.);
#72800=ORIENTED_EDGE('',*,*,#51665,.F.);
#72801=ORIENTED_EDGE('',*,*,#51662,.F.);
#72802=ORIENTED_EDGE('',*,*,#51666,.F.);
#72803=ORIENTED_EDGE('',*,*,#51667,.T.);
#72804=ORIENTED_EDGE('',*,*,#51668,.F.);
#72805=ORIENTED_EDGE('',*,*,#51660,.F.);
#72806=ORIENTED_EDGE('',*,*,#51669,.F.);
#72807=ORIENTED_EDGE('',*,*,#51670,.T.);
#72808=ORIENTED_EDGE('',*,*,#51671,.F.);
#72809=ORIENTED_EDGE('',*,*,#51664,.F.);
#72810=ORIENTED_EDGE('',*,*,#51672,.F.);
#72811=ORIENTED_EDGE('',*,*,#51673,.T.);
#72812=ORIENTED_EDGE('',*,*,#51674,.F.);
#72813=ORIENTED_EDGE('',*,*,#51667,.F.);
#72814=ORIENTED_EDGE('',*,*,#51675,.F.);
#72815=ORIENTED_EDGE('',*,*,#51676,.T.);
#72816=ORIENTED_EDGE('',*,*,#51677,.F.);
#72817=ORIENTED_EDGE('',*,*,#51670,.F.);
#72818=ORIENTED_EDGE('',*,*,#51678,.F.);
#72819=ORIENTED_EDGE('',*,*,#51679,.T.);
#72820=ORIENTED_EDGE('',*,*,#51680,.F.);
#72821=ORIENTED_EDGE('',*,*,#51673,.F.);
#72822=ORIENTED_EDGE('',*,*,#51681,.F.);
#72823=ORIENTED_EDGE('',*,*,#51682,.T.);
#72824=ORIENTED_EDGE('',*,*,#51683,.F.);
#72825=ORIENTED_EDGE('',*,*,#51676,.F.);
#72826=ORIENTED_EDGE('',*,*,#51684,.F.);
#72827=ORIENTED_EDGE('',*,*,#51679,.F.);
#72828=ORIENTED_EDGE('',*,*,#51685,.F.);
#72829=ORIENTED_EDGE('',*,*,#51682,.F.);
#72830=ORIENTED_EDGE('',*,*,#51686,.F.);
#72831=ORIENTED_EDGE('',*,*,#51687,.T.);
#72832=ORIENTED_EDGE('',*,*,#51688,.F.);
#72833=ORIENTED_EDGE('',*,*,#51689,.T.);
#72834=ORIENTED_EDGE('',*,*,#51690,.F.);
#72835=ORIENTED_EDGE('',*,*,#51691,.T.);
#72836=ORIENTED_EDGE('',*,*,#51692,.F.);
#72837=ORIENTED_EDGE('',*,*,#51689,.F.);
#72838=ORIENTED_EDGE('',*,*,#51693,.F.);
#72839=ORIENTED_EDGE('',*,*,#51694,.T.);
#72840=ORIENTED_EDGE('',*,*,#51695,.F.);
#72841=ORIENTED_EDGE('',*,*,#51687,.F.);
#72842=ORIENTED_EDGE('',*,*,#51696,.F.);
#72843=ORIENTED_EDGE('',*,*,#51697,.T.);
#72844=ORIENTED_EDGE('',*,*,#51698,.F.);
#72845=ORIENTED_EDGE('',*,*,#51691,.F.);
#72846=ORIENTED_EDGE('',*,*,#51699,.F.);
#72847=ORIENTED_EDGE('',*,*,#51700,.T.);
#72848=ORIENTED_EDGE('',*,*,#51701,.F.);
#72849=ORIENTED_EDGE('',*,*,#51694,.F.);
#72850=ORIENTED_EDGE('',*,*,#51702,.F.);
#72851=ORIENTED_EDGE('',*,*,#51703,.T.);
#72852=ORIENTED_EDGE('',*,*,#51704,.F.);
#72853=ORIENTED_EDGE('',*,*,#51697,.F.);
#72854=ORIENTED_EDGE('',*,*,#51705,.F.);
#72855=ORIENTED_EDGE('',*,*,#51706,.T.);
#72856=ORIENTED_EDGE('',*,*,#51707,.F.);
#72857=ORIENTED_EDGE('',*,*,#51700,.F.);
#72858=ORIENTED_EDGE('',*,*,#51708,.F.);
#72859=ORIENTED_EDGE('',*,*,#51703,.F.);
#72860=ORIENTED_EDGE('',*,*,#51709,.F.);
#72861=ORIENTED_EDGE('',*,*,#51706,.F.);
#72862=ORIENTED_EDGE('',*,*,#51710,.F.);
#72863=ORIENTED_EDGE('',*,*,#51711,.T.);
#72864=ORIENTED_EDGE('',*,*,#51712,.F.);
#72865=ORIENTED_EDGE('',*,*,#51713,.T.);
#72866=ORIENTED_EDGE('',*,*,#51714,.F.);
#72867=ORIENTED_EDGE('',*,*,#51715,.T.);
#72868=ORIENTED_EDGE('',*,*,#51716,.F.);
#72869=ORIENTED_EDGE('',*,*,#51713,.F.);
#72870=ORIENTED_EDGE('',*,*,#51717,.F.);
#72871=ORIENTED_EDGE('',*,*,#51718,.T.);
#72872=ORIENTED_EDGE('',*,*,#51719,.F.);
#72873=ORIENTED_EDGE('',*,*,#51711,.F.);
#72874=ORIENTED_EDGE('',*,*,#51720,.F.);
#72875=ORIENTED_EDGE('',*,*,#51721,.T.);
#72876=ORIENTED_EDGE('',*,*,#51722,.F.);
#72877=ORIENTED_EDGE('',*,*,#51715,.F.);
#72878=ORIENTED_EDGE('',*,*,#51723,.F.);
#72879=ORIENTED_EDGE('',*,*,#51724,.T.);
#72880=ORIENTED_EDGE('',*,*,#51725,.F.);
#72881=ORIENTED_EDGE('',*,*,#51718,.F.);
#72882=ORIENTED_EDGE('',*,*,#51726,.F.);
#72883=ORIENTED_EDGE('',*,*,#51727,.T.);
#72884=ORIENTED_EDGE('',*,*,#51728,.F.);
#72885=ORIENTED_EDGE('',*,*,#51721,.F.);
#72886=ORIENTED_EDGE('',*,*,#51729,.F.);
#72887=ORIENTED_EDGE('',*,*,#51730,.T.);
#72888=ORIENTED_EDGE('',*,*,#51731,.F.);
#72889=ORIENTED_EDGE('',*,*,#51724,.F.);
#72890=ORIENTED_EDGE('',*,*,#51732,.F.);
#72891=ORIENTED_EDGE('',*,*,#51727,.F.);
#72892=ORIENTED_EDGE('',*,*,#51733,.F.);
#72893=ORIENTED_EDGE('',*,*,#51730,.F.);
#72894=ORIENTED_EDGE('',*,*,#51734,.F.);
#72895=ORIENTED_EDGE('',*,*,#51735,.T.);
#72896=ORIENTED_EDGE('',*,*,#51736,.F.);
#72897=ORIENTED_EDGE('',*,*,#51737,.T.);
#72898=ORIENTED_EDGE('',*,*,#51738,.F.);
#72899=ORIENTED_EDGE('',*,*,#51739,.T.);
#72900=ORIENTED_EDGE('',*,*,#51740,.F.);
#72901=ORIENTED_EDGE('',*,*,#51737,.F.);
#72902=ORIENTED_EDGE('',*,*,#51741,.F.);
#72903=ORIENTED_EDGE('',*,*,#51742,.T.);
#72904=ORIENTED_EDGE('',*,*,#51743,.F.);
#72905=ORIENTED_EDGE('',*,*,#51735,.F.);
#72906=ORIENTED_EDGE('',*,*,#51744,.F.);
#72907=ORIENTED_EDGE('',*,*,#51745,.T.);
#72908=ORIENTED_EDGE('',*,*,#51746,.F.);
#72909=ORIENTED_EDGE('',*,*,#51739,.F.);
#72910=ORIENTED_EDGE('',*,*,#51747,.F.);
#72911=ORIENTED_EDGE('',*,*,#51748,.T.);
#72912=ORIENTED_EDGE('',*,*,#51749,.F.);
#72913=ORIENTED_EDGE('',*,*,#51742,.F.);
#72914=ORIENTED_EDGE('',*,*,#51750,.F.);
#72915=ORIENTED_EDGE('',*,*,#51751,.T.);
#72916=ORIENTED_EDGE('',*,*,#51752,.F.);
#72917=ORIENTED_EDGE('',*,*,#51745,.F.);
#72918=ORIENTED_EDGE('',*,*,#51753,.F.);
#72919=ORIENTED_EDGE('',*,*,#51754,.T.);
#72920=ORIENTED_EDGE('',*,*,#51755,.F.);
#72921=ORIENTED_EDGE('',*,*,#51748,.F.);
#72922=ORIENTED_EDGE('',*,*,#51756,.F.);
#72923=ORIENTED_EDGE('',*,*,#51751,.F.);
#72924=ORIENTED_EDGE('',*,*,#51757,.F.);
#72925=ORIENTED_EDGE('',*,*,#51754,.F.);
#72926=ORIENTED_EDGE('',*,*,#51758,.F.);
#72927=ORIENTED_EDGE('',*,*,#51759,.T.);
#72928=ORIENTED_EDGE('',*,*,#51760,.F.);
#72929=ORIENTED_EDGE('',*,*,#51761,.T.);
#72930=ORIENTED_EDGE('',*,*,#51762,.F.);
#72931=ORIENTED_EDGE('',*,*,#51763,.T.);
#72932=ORIENTED_EDGE('',*,*,#51764,.F.);
#72933=ORIENTED_EDGE('',*,*,#51761,.F.);
#72934=ORIENTED_EDGE('',*,*,#51765,.F.);
#72935=ORIENTED_EDGE('',*,*,#51766,.T.);
#72936=ORIENTED_EDGE('',*,*,#51767,.F.);
#72937=ORIENTED_EDGE('',*,*,#51759,.F.);
#72938=ORIENTED_EDGE('',*,*,#51768,.F.);
#72939=ORIENTED_EDGE('',*,*,#51769,.T.);
#72940=ORIENTED_EDGE('',*,*,#51770,.F.);
#72941=ORIENTED_EDGE('',*,*,#51763,.F.);
#72942=ORIENTED_EDGE('',*,*,#51771,.F.);
#72943=ORIENTED_EDGE('',*,*,#51772,.T.);
#72944=ORIENTED_EDGE('',*,*,#51773,.F.);
#72945=ORIENTED_EDGE('',*,*,#51766,.F.);
#72946=ORIENTED_EDGE('',*,*,#51774,.F.);
#72947=ORIENTED_EDGE('',*,*,#51775,.T.);
#72948=ORIENTED_EDGE('',*,*,#51776,.F.);
#72949=ORIENTED_EDGE('',*,*,#51769,.F.);
#72950=ORIENTED_EDGE('',*,*,#51777,.F.);
#72951=ORIENTED_EDGE('',*,*,#51778,.T.);
#72952=ORIENTED_EDGE('',*,*,#51779,.F.);
#72953=ORIENTED_EDGE('',*,*,#51772,.F.);
#72954=ORIENTED_EDGE('',*,*,#51780,.F.);
#72955=ORIENTED_EDGE('',*,*,#51775,.F.);
#72956=ORIENTED_EDGE('',*,*,#51781,.F.);
#72957=ORIENTED_EDGE('',*,*,#51778,.F.);
#72958=ORIENTED_EDGE('',*,*,#51782,.F.);
#72959=ORIENTED_EDGE('',*,*,#51783,.T.);
#72960=ORIENTED_EDGE('',*,*,#51784,.F.);
#72961=ORIENTED_EDGE('',*,*,#51785,.T.);
#72962=ORIENTED_EDGE('',*,*,#51786,.F.);
#72963=ORIENTED_EDGE('',*,*,#51787,.T.);
#72964=ORIENTED_EDGE('',*,*,#51788,.F.);
#72965=ORIENTED_EDGE('',*,*,#51785,.F.);
#72966=ORIENTED_EDGE('',*,*,#51789,.F.);
#72967=ORIENTED_EDGE('',*,*,#51790,.T.);
#72968=ORIENTED_EDGE('',*,*,#51791,.F.);
#72969=ORIENTED_EDGE('',*,*,#51783,.F.);
#72970=ORIENTED_EDGE('',*,*,#51792,.F.);
#72971=ORIENTED_EDGE('',*,*,#51793,.T.);
#72972=ORIENTED_EDGE('',*,*,#51794,.F.);
#72973=ORIENTED_EDGE('',*,*,#51787,.F.);
#72974=ORIENTED_EDGE('',*,*,#51795,.F.);
#72975=ORIENTED_EDGE('',*,*,#51796,.T.);
#72976=ORIENTED_EDGE('',*,*,#51797,.F.);
#72977=ORIENTED_EDGE('',*,*,#51790,.F.);
#72978=ORIENTED_EDGE('',*,*,#51798,.F.);
#72979=ORIENTED_EDGE('',*,*,#51799,.T.);
#72980=ORIENTED_EDGE('',*,*,#51800,.F.);
#72981=ORIENTED_EDGE('',*,*,#51793,.F.);
#72982=ORIENTED_EDGE('',*,*,#51801,.F.);
#72983=ORIENTED_EDGE('',*,*,#51802,.T.);
#72984=ORIENTED_EDGE('',*,*,#51803,.F.);
#72985=ORIENTED_EDGE('',*,*,#51796,.F.);
#72986=ORIENTED_EDGE('',*,*,#51804,.F.);
#72987=ORIENTED_EDGE('',*,*,#51799,.F.);
#72988=ORIENTED_EDGE('',*,*,#51805,.F.);
#72989=ORIENTED_EDGE('',*,*,#51802,.F.);
#72990=ORIENTED_EDGE('',*,*,#51806,.F.);
#72991=ORIENTED_EDGE('',*,*,#51807,.T.);
#72992=ORIENTED_EDGE('',*,*,#51808,.F.);
#72993=ORIENTED_EDGE('',*,*,#51809,.T.);
#72994=ORIENTED_EDGE('',*,*,#51810,.F.);
#72995=ORIENTED_EDGE('',*,*,#51811,.T.);
#72996=ORIENTED_EDGE('',*,*,#51812,.F.);
#72997=ORIENTED_EDGE('',*,*,#51809,.F.);
#72998=ORIENTED_EDGE('',*,*,#51813,.F.);
#72999=ORIENTED_EDGE('',*,*,#51814,.T.);
#73000=ORIENTED_EDGE('',*,*,#51815,.F.);
#73001=ORIENTED_EDGE('',*,*,#51807,.F.);
#73002=ORIENTED_EDGE('',*,*,#51816,.F.);
#73003=ORIENTED_EDGE('',*,*,#51817,.T.);
#73004=ORIENTED_EDGE('',*,*,#51818,.F.);
#73005=ORIENTED_EDGE('',*,*,#51811,.F.);
#73006=ORIENTED_EDGE('',*,*,#51819,.F.);
#73007=ORIENTED_EDGE('',*,*,#51820,.T.);
#73008=ORIENTED_EDGE('',*,*,#51821,.F.);
#73009=ORIENTED_EDGE('',*,*,#51814,.F.);
#73010=ORIENTED_EDGE('',*,*,#51822,.F.);
#73011=ORIENTED_EDGE('',*,*,#51823,.T.);
#73012=ORIENTED_EDGE('',*,*,#51824,.F.);
#73013=ORIENTED_EDGE('',*,*,#51817,.F.);
#73014=ORIENTED_EDGE('',*,*,#51825,.F.);
#73015=ORIENTED_EDGE('',*,*,#51826,.T.);
#73016=ORIENTED_EDGE('',*,*,#51827,.F.);
#73017=ORIENTED_EDGE('',*,*,#51820,.F.);
#73018=ORIENTED_EDGE('',*,*,#51828,.F.);
#73019=ORIENTED_EDGE('',*,*,#51829,.T.);
#73020=ORIENTED_EDGE('',*,*,#51830,.F.);
#73021=ORIENTED_EDGE('',*,*,#51823,.F.);
#73022=ORIENTED_EDGE('',*,*,#51831,.F.);
#73023=ORIENTED_EDGE('',*,*,#51832,.T.);
#73024=ORIENTED_EDGE('',*,*,#51833,.F.);
#73025=ORIENTED_EDGE('',*,*,#51826,.F.);
#73026=ORIENTED_EDGE('',*,*,#51834,.F.);
#73027=ORIENTED_EDGE('',*,*,#51829,.F.);
#73028=ORIENTED_EDGE('',*,*,#51835,.F.);
#73029=ORIENTED_EDGE('',*,*,#51832,.F.);
#73030=ORIENTED_EDGE('',*,*,#51836,.F.);
#73031=ORIENTED_EDGE('',*,*,#51837,.T.);
#73032=ORIENTED_EDGE('',*,*,#51838,.F.);
#73033=ORIENTED_EDGE('',*,*,#51839,.T.);
#73034=ORIENTED_EDGE('',*,*,#51840,.F.);
#73035=ORIENTED_EDGE('',*,*,#51841,.T.);
#73036=ORIENTED_EDGE('',*,*,#51842,.F.);
#73037=ORIENTED_EDGE('',*,*,#51839,.F.);
#73038=ORIENTED_EDGE('',*,*,#51843,.F.);
#73039=ORIENTED_EDGE('',*,*,#51844,.T.);
#73040=ORIENTED_EDGE('',*,*,#51845,.F.);
#73041=ORIENTED_EDGE('',*,*,#51837,.F.);
#73042=ORIENTED_EDGE('',*,*,#51846,.F.);
#73043=ORIENTED_EDGE('',*,*,#51847,.T.);
#73044=ORIENTED_EDGE('',*,*,#51848,.F.);
#73045=ORIENTED_EDGE('',*,*,#51841,.F.);
#73046=ORIENTED_EDGE('',*,*,#51849,.F.);
#73047=ORIENTED_EDGE('',*,*,#51850,.T.);
#73048=ORIENTED_EDGE('',*,*,#51851,.F.);
#73049=ORIENTED_EDGE('',*,*,#51844,.F.);
#73050=ORIENTED_EDGE('',*,*,#51852,.F.);
#73051=ORIENTED_EDGE('',*,*,#51853,.T.);
#73052=ORIENTED_EDGE('',*,*,#51854,.F.);
#73053=ORIENTED_EDGE('',*,*,#51847,.F.);
#73054=ORIENTED_EDGE('',*,*,#51855,.F.);
#73055=ORIENTED_EDGE('',*,*,#51856,.T.);
#73056=ORIENTED_EDGE('',*,*,#51857,.F.);
#73057=ORIENTED_EDGE('',*,*,#51850,.F.);
#73058=ORIENTED_EDGE('',*,*,#51858,.F.);
#73059=ORIENTED_EDGE('',*,*,#51853,.F.);
#73060=ORIENTED_EDGE('',*,*,#51859,.F.);
#73061=ORIENTED_EDGE('',*,*,#51856,.F.);
#73062=ORIENTED_EDGE('',*,*,#51860,.F.);
#73063=ORIENTED_EDGE('',*,*,#51861,.T.);
#73064=ORIENTED_EDGE('',*,*,#51862,.F.);
#73065=ORIENTED_EDGE('',*,*,#51863,.T.);
#73066=ORIENTED_EDGE('',*,*,#51864,.F.);
#73067=ORIENTED_EDGE('',*,*,#51865,.T.);
#73068=ORIENTED_EDGE('',*,*,#51866,.F.);
#73069=ORIENTED_EDGE('',*,*,#51863,.F.);
#73070=ORIENTED_EDGE('',*,*,#51867,.F.);
#73071=ORIENTED_EDGE('',*,*,#51868,.T.);
#73072=ORIENTED_EDGE('',*,*,#51869,.F.);
#73073=ORIENTED_EDGE('',*,*,#51861,.F.);
#73074=ORIENTED_EDGE('',*,*,#51870,.F.);
#73075=ORIENTED_EDGE('',*,*,#51871,.T.);
#73076=ORIENTED_EDGE('',*,*,#51872,.F.);
#73077=ORIENTED_EDGE('',*,*,#51865,.F.);
#73078=ORIENTED_EDGE('',*,*,#51873,.F.);
#73079=ORIENTED_EDGE('',*,*,#51874,.T.);
#73080=ORIENTED_EDGE('',*,*,#51875,.F.);
#73081=ORIENTED_EDGE('',*,*,#51868,.F.);
#73082=ORIENTED_EDGE('',*,*,#51876,.F.);
#73083=ORIENTED_EDGE('',*,*,#51877,.T.);
#73084=ORIENTED_EDGE('',*,*,#51878,.F.);
#73085=ORIENTED_EDGE('',*,*,#51871,.F.);
#73086=ORIENTED_EDGE('',*,*,#51879,.F.);
#73087=ORIENTED_EDGE('',*,*,#51880,.T.);
#73088=ORIENTED_EDGE('',*,*,#51881,.F.);
#73089=ORIENTED_EDGE('',*,*,#51874,.F.);
#73090=ORIENTED_EDGE('',*,*,#51882,.F.);
#73091=ORIENTED_EDGE('',*,*,#51877,.F.);
#73092=ORIENTED_EDGE('',*,*,#51883,.F.);
#73093=ORIENTED_EDGE('',*,*,#51880,.F.);
#73094=ORIENTED_EDGE('',*,*,#51884,.F.);
#73095=ORIENTED_EDGE('',*,*,#51885,.T.);
#73096=ORIENTED_EDGE('',*,*,#51886,.F.);
#73097=ORIENTED_EDGE('',*,*,#51887,.T.);
#73098=ORIENTED_EDGE('',*,*,#51888,.F.);
#73099=ORIENTED_EDGE('',*,*,#51889,.T.);
#73100=ORIENTED_EDGE('',*,*,#51890,.F.);
#73101=ORIENTED_EDGE('',*,*,#51887,.F.);
#73102=ORIENTED_EDGE('',*,*,#51891,.F.);
#73103=ORIENTED_EDGE('',*,*,#51892,.T.);
#73104=ORIENTED_EDGE('',*,*,#51893,.F.);
#73105=ORIENTED_EDGE('',*,*,#51885,.F.);
#73106=ORIENTED_EDGE('',*,*,#51894,.F.);
#73107=ORIENTED_EDGE('',*,*,#51895,.T.);
#73108=ORIENTED_EDGE('',*,*,#51896,.F.);
#73109=ORIENTED_EDGE('',*,*,#51889,.F.);
#73110=ORIENTED_EDGE('',*,*,#51897,.F.);
#73111=ORIENTED_EDGE('',*,*,#51898,.T.);
#73112=ORIENTED_EDGE('',*,*,#51899,.F.);
#73113=ORIENTED_EDGE('',*,*,#51892,.F.);
#73114=ORIENTED_EDGE('',*,*,#51900,.F.);
#73115=ORIENTED_EDGE('',*,*,#51901,.T.);
#73116=ORIENTED_EDGE('',*,*,#51902,.F.);
#73117=ORIENTED_EDGE('',*,*,#51895,.F.);
#73118=ORIENTED_EDGE('',*,*,#51903,.F.);
#73119=ORIENTED_EDGE('',*,*,#51904,.T.);
#73120=ORIENTED_EDGE('',*,*,#51905,.F.);
#73121=ORIENTED_EDGE('',*,*,#51898,.F.);
#73122=ORIENTED_EDGE('',*,*,#51906,.F.);
#73123=ORIENTED_EDGE('',*,*,#51907,.T.);
#73124=ORIENTED_EDGE('',*,*,#51908,.F.);
#73125=ORIENTED_EDGE('',*,*,#51901,.F.);
#73126=ORIENTED_EDGE('',*,*,#51909,.F.);
#73127=ORIENTED_EDGE('',*,*,#51910,.T.);
#73128=ORIENTED_EDGE('',*,*,#51911,.F.);
#73129=ORIENTED_EDGE('',*,*,#51904,.F.);
#73130=ORIENTED_EDGE('',*,*,#51912,.F.);
#73131=ORIENTED_EDGE('',*,*,#51907,.F.);
#73132=ORIENTED_EDGE('',*,*,#51913,.F.);
#73133=ORIENTED_EDGE('',*,*,#51910,.F.);
#73134=ORIENTED_EDGE('',*,*,#51914,.F.);
#73135=ORIENTED_EDGE('',*,*,#51915,.T.);
#73136=ORIENTED_EDGE('',*,*,#51916,.F.);
#73137=ORIENTED_EDGE('',*,*,#51917,.T.);
#73138=ORIENTED_EDGE('',*,*,#51918,.F.);
#73139=ORIENTED_EDGE('',*,*,#51919,.T.);
#73140=ORIENTED_EDGE('',*,*,#51920,.F.);
#73141=ORIENTED_EDGE('',*,*,#51917,.F.);
#73142=ORIENTED_EDGE('',*,*,#51921,.F.);
#73143=ORIENTED_EDGE('',*,*,#51922,.T.);
#73144=ORIENTED_EDGE('',*,*,#51923,.F.);
#73145=ORIENTED_EDGE('',*,*,#51915,.F.);
#73146=ORIENTED_EDGE('',*,*,#51924,.F.);
#73147=ORIENTED_EDGE('',*,*,#51925,.T.);
#73148=ORIENTED_EDGE('',*,*,#51926,.F.);
#73149=ORIENTED_EDGE('',*,*,#51919,.F.);
#73150=ORIENTED_EDGE('',*,*,#51927,.F.);
#73151=ORIENTED_EDGE('',*,*,#51928,.T.);
#73152=ORIENTED_EDGE('',*,*,#51929,.F.);
#73153=ORIENTED_EDGE('',*,*,#51922,.F.);
#73154=ORIENTED_EDGE('',*,*,#51930,.F.);
#73155=ORIENTED_EDGE('',*,*,#51931,.T.);
#73156=ORIENTED_EDGE('',*,*,#51932,.F.);
#73157=ORIENTED_EDGE('',*,*,#51925,.F.);
#73158=ORIENTED_EDGE('',*,*,#51933,.F.);
#73159=ORIENTED_EDGE('',*,*,#51934,.T.);
#73160=ORIENTED_EDGE('',*,*,#51935,.F.);
#73161=ORIENTED_EDGE('',*,*,#51928,.F.);
#73162=ORIENTED_EDGE('',*,*,#51936,.F.);
#73163=ORIENTED_EDGE('',*,*,#51937,.T.);
#73164=ORIENTED_EDGE('',*,*,#51938,.F.);
#73165=ORIENTED_EDGE('',*,*,#51931,.F.);
#73166=ORIENTED_EDGE('',*,*,#51939,.F.);
#73167=ORIENTED_EDGE('',*,*,#51940,.T.);
#73168=ORIENTED_EDGE('',*,*,#51941,.F.);
#73169=ORIENTED_EDGE('',*,*,#51934,.F.);
#73170=ORIENTED_EDGE('',*,*,#51942,.F.);
#73171=ORIENTED_EDGE('',*,*,#51937,.F.);
#73172=ORIENTED_EDGE('',*,*,#51943,.F.);
#73173=ORIENTED_EDGE('',*,*,#51940,.F.);
#73174=ORIENTED_EDGE('',*,*,#51944,.F.);
#73175=ORIENTED_EDGE('',*,*,#51945,.T.);
#73176=ORIENTED_EDGE('',*,*,#51946,.F.);
#73177=ORIENTED_EDGE('',*,*,#51947,.T.);
#73178=ORIENTED_EDGE('',*,*,#51948,.F.);
#73179=ORIENTED_EDGE('',*,*,#51949,.T.);
#73180=ORIENTED_EDGE('',*,*,#51950,.F.);
#73181=ORIENTED_EDGE('',*,*,#51947,.F.);
#73182=ORIENTED_EDGE('',*,*,#51951,.F.);
#73183=ORIENTED_EDGE('',*,*,#51952,.T.);
#73184=ORIENTED_EDGE('',*,*,#51953,.F.);
#73185=ORIENTED_EDGE('',*,*,#51945,.F.);
#73186=ORIENTED_EDGE('',*,*,#51954,.F.);
#73187=ORIENTED_EDGE('',*,*,#51955,.T.);
#73188=ORIENTED_EDGE('',*,*,#51956,.F.);
#73189=ORIENTED_EDGE('',*,*,#51949,.F.);
#73190=ORIENTED_EDGE('',*,*,#51957,.F.);
#73191=ORIENTED_EDGE('',*,*,#51958,.T.);
#73192=ORIENTED_EDGE('',*,*,#51959,.F.);
#73193=ORIENTED_EDGE('',*,*,#51952,.F.);
#73194=ORIENTED_EDGE('',*,*,#51960,.F.);
#73195=ORIENTED_EDGE('',*,*,#51961,.T.);
#73196=ORIENTED_EDGE('',*,*,#51962,.F.);
#73197=ORIENTED_EDGE('',*,*,#51955,.F.);
#73198=ORIENTED_EDGE('',*,*,#51963,.F.);
#73199=ORIENTED_EDGE('',*,*,#51964,.T.);
#73200=ORIENTED_EDGE('',*,*,#51965,.F.);
#73201=ORIENTED_EDGE('',*,*,#51958,.F.);
#73202=ORIENTED_EDGE('',*,*,#51966,.F.);
#73203=ORIENTED_EDGE('',*,*,#51961,.F.);
#73204=ORIENTED_EDGE('',*,*,#51967,.F.);
#73205=ORIENTED_EDGE('',*,*,#51964,.F.);
#73206=ORIENTED_EDGE('',*,*,#51968,.F.);
#73207=ORIENTED_EDGE('',*,*,#51969,.T.);
#73208=ORIENTED_EDGE('',*,*,#51970,.F.);
#73209=ORIENTED_EDGE('',*,*,#51971,.T.);
#73210=ORIENTED_EDGE('',*,*,#51972,.F.);
#73211=ORIENTED_EDGE('',*,*,#51973,.T.);
#73212=ORIENTED_EDGE('',*,*,#51974,.F.);
#73213=ORIENTED_EDGE('',*,*,#51971,.F.);
#73214=ORIENTED_EDGE('',*,*,#51975,.F.);
#73215=ORIENTED_EDGE('',*,*,#51976,.T.);
#73216=ORIENTED_EDGE('',*,*,#51977,.F.);
#73217=ORIENTED_EDGE('',*,*,#51969,.F.);
#73218=ORIENTED_EDGE('',*,*,#51978,.F.);
#73219=ORIENTED_EDGE('',*,*,#51979,.T.);
#73220=ORIENTED_EDGE('',*,*,#51980,.F.);
#73221=ORIENTED_EDGE('',*,*,#51973,.F.);
#73222=ORIENTED_EDGE('',*,*,#51981,.F.);
#73223=ORIENTED_EDGE('',*,*,#51982,.T.);
#73224=ORIENTED_EDGE('',*,*,#51983,.F.);
#73225=ORIENTED_EDGE('',*,*,#51976,.F.);
#73226=ORIENTED_EDGE('',*,*,#51984,.F.);
#73227=ORIENTED_EDGE('',*,*,#51985,.T.);
#73228=ORIENTED_EDGE('',*,*,#51986,.F.);
#73229=ORIENTED_EDGE('',*,*,#51979,.F.);
#73230=ORIENTED_EDGE('',*,*,#51987,.F.);
#73231=ORIENTED_EDGE('',*,*,#51988,.T.);
#73232=ORIENTED_EDGE('',*,*,#51989,.F.);
#73233=ORIENTED_EDGE('',*,*,#51982,.F.);
#73234=ORIENTED_EDGE('',*,*,#51990,.F.);
#73235=ORIENTED_EDGE('',*,*,#51985,.F.);
#73236=ORIENTED_EDGE('',*,*,#51991,.F.);
#73237=ORIENTED_EDGE('',*,*,#51988,.F.);
#73238=ORIENTED_EDGE('',*,*,#51992,.F.);
#73239=ORIENTED_EDGE('',*,*,#51993,.T.);
#73240=ORIENTED_EDGE('',*,*,#51994,.F.);
#73241=ORIENTED_EDGE('',*,*,#51995,.T.);
#73242=ORIENTED_EDGE('',*,*,#51996,.F.);
#73243=ORIENTED_EDGE('',*,*,#51997,.T.);
#73244=ORIENTED_EDGE('',*,*,#51998,.F.);
#73245=ORIENTED_EDGE('',*,*,#51995,.F.);
#73246=ORIENTED_EDGE('',*,*,#51999,.F.);
#73247=ORIENTED_EDGE('',*,*,#52000,.T.);
#73248=ORIENTED_EDGE('',*,*,#52001,.F.);
#73249=ORIENTED_EDGE('',*,*,#51993,.F.);
#73250=ORIENTED_EDGE('',*,*,#52002,.F.);
#73251=ORIENTED_EDGE('',*,*,#52003,.T.);
#73252=ORIENTED_EDGE('',*,*,#52004,.F.);
#73253=ORIENTED_EDGE('',*,*,#51997,.F.);
#73254=ORIENTED_EDGE('',*,*,#52005,.F.);
#73255=ORIENTED_EDGE('',*,*,#52006,.T.);
#73256=ORIENTED_EDGE('',*,*,#52007,.F.);
#73257=ORIENTED_EDGE('',*,*,#52000,.F.);
#73258=ORIENTED_EDGE('',*,*,#52008,.F.);
#73259=ORIENTED_EDGE('',*,*,#52009,.T.);
#73260=ORIENTED_EDGE('',*,*,#52010,.F.);
#73261=ORIENTED_EDGE('',*,*,#52003,.F.);
#73262=ORIENTED_EDGE('',*,*,#52011,.F.);
#73263=ORIENTED_EDGE('',*,*,#52012,.T.);
#73264=ORIENTED_EDGE('',*,*,#52013,.F.);
#73265=ORIENTED_EDGE('',*,*,#52006,.F.);
#73266=ORIENTED_EDGE('',*,*,#52014,.F.);
#73267=ORIENTED_EDGE('',*,*,#52009,.F.);
#73268=ORIENTED_EDGE('',*,*,#52015,.F.);
#73269=ORIENTED_EDGE('',*,*,#52012,.F.);
#73270=ORIENTED_EDGE('',*,*,#52016,.F.);
#73271=ORIENTED_EDGE('',*,*,#52017,.T.);
#73272=ORIENTED_EDGE('',*,*,#52018,.F.);
#73273=ORIENTED_EDGE('',*,*,#52019,.T.);
#73274=ORIENTED_EDGE('',*,*,#52020,.F.);
#73275=ORIENTED_EDGE('',*,*,#52021,.T.);
#73276=ORIENTED_EDGE('',*,*,#52022,.F.);
#73277=ORIENTED_EDGE('',*,*,#52019,.F.);
#73278=ORIENTED_EDGE('',*,*,#52023,.F.);
#73279=ORIENTED_EDGE('',*,*,#52024,.T.);
#73280=ORIENTED_EDGE('',*,*,#52025,.F.);
#73281=ORIENTED_EDGE('',*,*,#52017,.F.);
#73282=ORIENTED_EDGE('',*,*,#52026,.F.);
#73283=ORIENTED_EDGE('',*,*,#52027,.T.);
#73284=ORIENTED_EDGE('',*,*,#52028,.F.);
#73285=ORIENTED_EDGE('',*,*,#52021,.F.);
#73286=ORIENTED_EDGE('',*,*,#52029,.F.);
#73287=ORIENTED_EDGE('',*,*,#52030,.T.);
#73288=ORIENTED_EDGE('',*,*,#52031,.F.);
#73289=ORIENTED_EDGE('',*,*,#52024,.F.);
#73290=ORIENTED_EDGE('',*,*,#52032,.F.);
#73291=ORIENTED_EDGE('',*,*,#52033,.T.);
#73292=ORIENTED_EDGE('',*,*,#52034,.F.);
#73293=ORIENTED_EDGE('',*,*,#52027,.F.);
#73294=ORIENTED_EDGE('',*,*,#52035,.F.);
#73295=ORIENTED_EDGE('',*,*,#52036,.T.);
#73296=ORIENTED_EDGE('',*,*,#52037,.F.);
#73297=ORIENTED_EDGE('',*,*,#52030,.F.);
#73298=ORIENTED_EDGE('',*,*,#52038,.F.);
#73299=ORIENTED_EDGE('',*,*,#52033,.F.);
#73300=ORIENTED_EDGE('',*,*,#52039,.F.);
#73301=ORIENTED_EDGE('',*,*,#52036,.F.);
#73302=ORIENTED_EDGE('',*,*,#52040,.F.);
#73303=ORIENTED_EDGE('',*,*,#52041,.T.);
#73304=ORIENTED_EDGE('',*,*,#52042,.F.);
#73305=ORIENTED_EDGE('',*,*,#52043,.T.);
#73306=ORIENTED_EDGE('',*,*,#52044,.F.);
#73307=ORIENTED_EDGE('',*,*,#52045,.T.);
#73308=ORIENTED_EDGE('',*,*,#52046,.F.);
#73309=ORIENTED_EDGE('',*,*,#52043,.F.);
#73310=ORIENTED_EDGE('',*,*,#52047,.F.);
#73311=ORIENTED_EDGE('',*,*,#52048,.T.);
#73312=ORIENTED_EDGE('',*,*,#52049,.F.);
#73313=ORIENTED_EDGE('',*,*,#52041,.F.);
#73314=ORIENTED_EDGE('',*,*,#52050,.F.);
#73315=ORIENTED_EDGE('',*,*,#52051,.T.);
#73316=ORIENTED_EDGE('',*,*,#52052,.F.);
#73317=ORIENTED_EDGE('',*,*,#52045,.F.);
#73318=ORIENTED_EDGE('',*,*,#52053,.F.);
#73319=ORIENTED_EDGE('',*,*,#52054,.T.);
#73320=ORIENTED_EDGE('',*,*,#52055,.F.);
#73321=ORIENTED_EDGE('',*,*,#52048,.F.);
#73322=ORIENTED_EDGE('',*,*,#52056,.F.);
#73323=ORIENTED_EDGE('',*,*,#52057,.T.);
#73324=ORIENTED_EDGE('',*,*,#52058,.F.);
#73325=ORIENTED_EDGE('',*,*,#52051,.F.);
#73326=ORIENTED_EDGE('',*,*,#52059,.F.);
#73327=ORIENTED_EDGE('',*,*,#52060,.T.);
#73328=ORIENTED_EDGE('',*,*,#52061,.F.);
#73329=ORIENTED_EDGE('',*,*,#52054,.F.);
#73330=ORIENTED_EDGE('',*,*,#52062,.F.);
#73331=ORIENTED_EDGE('',*,*,#52063,.F.);
#73332=ORIENTED_EDGE('',*,*,#52057,.F.);
#73333=ORIENTED_EDGE('',*,*,#52064,.F.);
#73334=ORIENTED_EDGE('',*,*,#52065,.T.);
#73335=ORIENTED_EDGE('',*,*,#52060,.F.);
#73336=ORIENTED_EDGE('',*,*,#52066,.F.);
#73337=ORIENTED_EDGE('',*,*,#52065,.F.);
#73338=ORIENTED_EDGE('',*,*,#52067,.F.);
#73339=ORIENTED_EDGE('',*,*,#52068,.T.);
#73340=ORIENTED_EDGE('',*,*,#52069,.F.);
#73341=ORIENTED_EDGE('',*,*,#52070,.T.);
#73342=ORIENTED_EDGE('',*,*,#52071,.F.);
#73343=ORIENTED_EDGE('',*,*,#52072,.T.);
#73344=ORIENTED_EDGE('',*,*,#52073,.F.);
#73345=ORIENTED_EDGE('',*,*,#52070,.F.);
#73346=ORIENTED_EDGE('',*,*,#52074,.F.);
#73347=ORIENTED_EDGE('',*,*,#52075,.T.);
#73348=ORIENTED_EDGE('',*,*,#52076,.F.);
#73349=ORIENTED_EDGE('',*,*,#52068,.F.);
#73350=ORIENTED_EDGE('',*,*,#52077,.F.);
#73351=ORIENTED_EDGE('',*,*,#52078,.T.);
#73352=ORIENTED_EDGE('',*,*,#52079,.F.);
#73353=ORIENTED_EDGE('',*,*,#52072,.F.);
#73354=ORIENTED_EDGE('',*,*,#52080,.F.);
#73355=ORIENTED_EDGE('',*,*,#52081,.T.);
#73356=ORIENTED_EDGE('',*,*,#52082,.F.);
#73357=ORIENTED_EDGE('',*,*,#52075,.F.);
#73358=ORIENTED_EDGE('',*,*,#52083,.F.);
#73359=ORIENTED_EDGE('',*,*,#52084,.T.);
#73360=ORIENTED_EDGE('',*,*,#52085,.F.);
#73361=ORIENTED_EDGE('',*,*,#52078,.F.);
#73362=ORIENTED_EDGE('',*,*,#52086,.F.);
#73363=ORIENTED_EDGE('',*,*,#52087,.T.);
#73364=ORIENTED_EDGE('',*,*,#52088,.F.);
#73365=ORIENTED_EDGE('',*,*,#52081,.F.);
#73366=ORIENTED_EDGE('',*,*,#52089,.F.);
#73367=ORIENTED_EDGE('',*,*,#52084,.F.);
#73368=ORIENTED_EDGE('',*,*,#52090,.F.);
#73369=ORIENTED_EDGE('',*,*,#52087,.F.);
#73370=ORIENTED_EDGE('',*,*,#52091,.F.);
#73371=ORIENTED_EDGE('',*,*,#52092,.T.);
#73372=ORIENTED_EDGE('',*,*,#52093,.F.);
#73373=ORIENTED_EDGE('',*,*,#52094,.T.);
#73374=ORIENTED_EDGE('',*,*,#52095,.F.);
#73375=ORIENTED_EDGE('',*,*,#52096,.T.);
#73376=ORIENTED_EDGE('',*,*,#52097,.F.);
#73377=ORIENTED_EDGE('',*,*,#52094,.F.);
#73378=ORIENTED_EDGE('',*,*,#52098,.F.);
#73379=ORIENTED_EDGE('',*,*,#52099,.T.);
#73380=ORIENTED_EDGE('',*,*,#52100,.F.);
#73381=ORIENTED_EDGE('',*,*,#52092,.F.);
#73382=ORIENTED_EDGE('',*,*,#52101,.F.);
#73383=ORIENTED_EDGE('',*,*,#52102,.T.);
#73384=ORIENTED_EDGE('',*,*,#52103,.F.);
#73385=ORIENTED_EDGE('',*,*,#52096,.F.);
#73386=ORIENTED_EDGE('',*,*,#52104,.F.);
#73387=ORIENTED_EDGE('',*,*,#52105,.T.);
#73388=ORIENTED_EDGE('',*,*,#52106,.F.);
#73389=ORIENTED_EDGE('',*,*,#52099,.F.);
#73390=ORIENTED_EDGE('',*,*,#52107,.F.);
#73391=ORIENTED_EDGE('',*,*,#52108,.T.);
#73392=ORIENTED_EDGE('',*,*,#52109,.F.);
#73393=ORIENTED_EDGE('',*,*,#52102,.F.);
#73394=ORIENTED_EDGE('',*,*,#52110,.F.);
#73395=ORIENTED_EDGE('',*,*,#52111,.T.);
#73396=ORIENTED_EDGE('',*,*,#52112,.F.);
#73397=ORIENTED_EDGE('',*,*,#52105,.F.);
#73398=ORIENTED_EDGE('',*,*,#52113,.F.);
#73399=ORIENTED_EDGE('',*,*,#52114,.T.);
#73400=ORIENTED_EDGE('',*,*,#52115,.F.);
#73401=ORIENTED_EDGE('',*,*,#52108,.F.);
#73402=ORIENTED_EDGE('',*,*,#52116,.F.);
#73403=ORIENTED_EDGE('',*,*,#52117,.T.);
#73404=ORIENTED_EDGE('',*,*,#52118,.F.);
#73405=ORIENTED_EDGE('',*,*,#52111,.F.);
#73406=ORIENTED_EDGE('',*,*,#52119,.F.);
#73407=ORIENTED_EDGE('',*,*,#52114,.F.);
#73408=ORIENTED_EDGE('',*,*,#52120,.F.);
#73409=ORIENTED_EDGE('',*,*,#52117,.F.);
#73410=ORIENTED_EDGE('',*,*,#52121,.F.);
#73411=ORIENTED_EDGE('',*,*,#52122,.T.);
#73412=ORIENTED_EDGE('',*,*,#52123,.F.);
#73413=ORIENTED_EDGE('',*,*,#52124,.T.);
#73414=ORIENTED_EDGE('',*,*,#52125,.F.);
#73415=ORIENTED_EDGE('',*,*,#52126,.T.);
#73416=ORIENTED_EDGE('',*,*,#52127,.F.);
#73417=ORIENTED_EDGE('',*,*,#52124,.F.);
#73418=ORIENTED_EDGE('',*,*,#52128,.F.);
#73419=ORIENTED_EDGE('',*,*,#52129,.T.);
#73420=ORIENTED_EDGE('',*,*,#52130,.F.);
#73421=ORIENTED_EDGE('',*,*,#52122,.F.);
#73422=ORIENTED_EDGE('',*,*,#52131,.F.);
#73423=ORIENTED_EDGE('',*,*,#52132,.T.);
#73424=ORIENTED_EDGE('',*,*,#52133,.F.);
#73425=ORIENTED_EDGE('',*,*,#52126,.F.);
#73426=ORIENTED_EDGE('',*,*,#52134,.F.);
#73427=ORIENTED_EDGE('',*,*,#52135,.T.);
#73428=ORIENTED_EDGE('',*,*,#52136,.F.);
#73429=ORIENTED_EDGE('',*,*,#52129,.F.);
#73430=ORIENTED_EDGE('',*,*,#52137,.F.);
#73431=ORIENTED_EDGE('',*,*,#52138,.T.);
#73432=ORIENTED_EDGE('',*,*,#52139,.F.);
#73433=ORIENTED_EDGE('',*,*,#52132,.F.);
#73434=ORIENTED_EDGE('',*,*,#52140,.F.);
#73435=ORIENTED_EDGE('',*,*,#52141,.T.);
#73436=ORIENTED_EDGE('',*,*,#52142,.F.);
#73437=ORIENTED_EDGE('',*,*,#52135,.F.);
#73438=ORIENTED_EDGE('',*,*,#52143,.F.);
#73439=ORIENTED_EDGE('',*,*,#52138,.F.);
#73440=ORIENTED_EDGE('',*,*,#52144,.F.);
#73441=ORIENTED_EDGE('',*,*,#52141,.F.);
#73442=ORIENTED_EDGE('',*,*,#52145,.F.);
#73443=ORIENTED_EDGE('',*,*,#52146,.T.);
#73444=ORIENTED_EDGE('',*,*,#52147,.F.);
#73445=ORIENTED_EDGE('',*,*,#52148,.T.);
#73446=ORIENTED_EDGE('',*,*,#52149,.F.);
#73447=ORIENTED_EDGE('',*,*,#52150,.T.);
#73448=ORIENTED_EDGE('',*,*,#52151,.F.);
#73449=ORIENTED_EDGE('',*,*,#52148,.F.);
#73450=ORIENTED_EDGE('',*,*,#52152,.F.);
#73451=ORIENTED_EDGE('',*,*,#52153,.T.);
#73452=ORIENTED_EDGE('',*,*,#52154,.F.);
#73453=ORIENTED_EDGE('',*,*,#52146,.F.);
#73454=ORIENTED_EDGE('',*,*,#52155,.F.);
#73455=ORIENTED_EDGE('',*,*,#52156,.T.);
#73456=ORIENTED_EDGE('',*,*,#52157,.F.);
#73457=ORIENTED_EDGE('',*,*,#52150,.F.);
#73458=ORIENTED_EDGE('',*,*,#52158,.F.);
#73459=ORIENTED_EDGE('',*,*,#52159,.T.);
#73460=ORIENTED_EDGE('',*,*,#52160,.F.);
#73461=ORIENTED_EDGE('',*,*,#52153,.F.);
#73462=ORIENTED_EDGE('',*,*,#52161,.F.);
#73463=ORIENTED_EDGE('',*,*,#52162,.T.);
#73464=ORIENTED_EDGE('',*,*,#52163,.F.);
#73465=ORIENTED_EDGE('',*,*,#52156,.F.);
#73466=ORIENTED_EDGE('',*,*,#52164,.F.);
#73467=ORIENTED_EDGE('',*,*,#52165,.T.);
#73468=ORIENTED_EDGE('',*,*,#52166,.F.);
#73469=ORIENTED_EDGE('',*,*,#52159,.F.);
#73470=ORIENTED_EDGE('',*,*,#52167,.F.);
#73471=ORIENTED_EDGE('',*,*,#52168,.T.);
#73472=ORIENTED_EDGE('',*,*,#52169,.F.);
#73473=ORIENTED_EDGE('',*,*,#52162,.F.);
#73474=ORIENTED_EDGE('',*,*,#52170,.F.);
#73475=ORIENTED_EDGE('',*,*,#52171,.T.);
#73476=ORIENTED_EDGE('',*,*,#52172,.F.);
#73477=ORIENTED_EDGE('',*,*,#52165,.F.);
#73478=ORIENTED_EDGE('',*,*,#52173,.F.);
#73479=ORIENTED_EDGE('',*,*,#52168,.F.);
#73480=ORIENTED_EDGE('',*,*,#52174,.F.);
#73481=ORIENTED_EDGE('',*,*,#52171,.F.);
#73482=ORIENTED_EDGE('',*,*,#52175,.F.);
#73483=ORIENTED_EDGE('',*,*,#52176,.T.);
#73484=ORIENTED_EDGE('',*,*,#52177,.F.);
#73485=ORIENTED_EDGE('',*,*,#52178,.T.);
#73486=ORIENTED_EDGE('',*,*,#52179,.F.);
#73487=ORIENTED_EDGE('',*,*,#52180,.T.);
#73488=ORIENTED_EDGE('',*,*,#52181,.F.);
#73489=ORIENTED_EDGE('',*,*,#52178,.F.);
#73490=ORIENTED_EDGE('',*,*,#52182,.F.);
#73491=ORIENTED_EDGE('',*,*,#52183,.T.);
#73492=ORIENTED_EDGE('',*,*,#52184,.F.);
#73493=ORIENTED_EDGE('',*,*,#52176,.F.);
#73494=ORIENTED_EDGE('',*,*,#52185,.F.);
#73495=ORIENTED_EDGE('',*,*,#52186,.T.);
#73496=ORIENTED_EDGE('',*,*,#52187,.F.);
#73497=ORIENTED_EDGE('',*,*,#52180,.F.);
#73498=ORIENTED_EDGE('',*,*,#52188,.F.);
#73499=ORIENTED_EDGE('',*,*,#52189,.T.);
#73500=ORIENTED_EDGE('',*,*,#52190,.F.);
#73501=ORIENTED_EDGE('',*,*,#52183,.F.);
#73502=ORIENTED_EDGE('',*,*,#52191,.F.);
#73503=ORIENTED_EDGE('',*,*,#52192,.T.);
#73504=ORIENTED_EDGE('',*,*,#52193,.F.);
#73505=ORIENTED_EDGE('',*,*,#52186,.F.);
#73506=ORIENTED_EDGE('',*,*,#52194,.F.);
#73507=ORIENTED_EDGE('',*,*,#52195,.T.);
#73508=ORIENTED_EDGE('',*,*,#52196,.F.);
#73509=ORIENTED_EDGE('',*,*,#52189,.F.);
#73510=ORIENTED_EDGE('',*,*,#52197,.F.);
#73511=ORIENTED_EDGE('',*,*,#52192,.F.);
#73512=ORIENTED_EDGE('',*,*,#52198,.F.);
#73513=ORIENTED_EDGE('',*,*,#52195,.F.);
#73514=ORIENTED_EDGE('',*,*,#52199,.F.);
#73515=ORIENTED_EDGE('',*,*,#52200,.T.);
#73516=ORIENTED_EDGE('',*,*,#52201,.F.);
#73517=ORIENTED_EDGE('',*,*,#52202,.T.);
#73518=ORIENTED_EDGE('',*,*,#52203,.F.);
#73519=ORIENTED_EDGE('',*,*,#52204,.T.);
#73520=ORIENTED_EDGE('',*,*,#52205,.F.);
#73521=ORIENTED_EDGE('',*,*,#52202,.F.);
#73522=ORIENTED_EDGE('',*,*,#52206,.F.);
#73523=ORIENTED_EDGE('',*,*,#52207,.T.);
#73524=ORIENTED_EDGE('',*,*,#52208,.F.);
#73525=ORIENTED_EDGE('',*,*,#52200,.F.);
#73526=ORIENTED_EDGE('',*,*,#52209,.F.);
#73527=ORIENTED_EDGE('',*,*,#52210,.T.);
#73528=ORIENTED_EDGE('',*,*,#52211,.F.);
#73529=ORIENTED_EDGE('',*,*,#52204,.F.);
#73530=ORIENTED_EDGE('',*,*,#52212,.F.);
#73531=ORIENTED_EDGE('',*,*,#52213,.T.);
#73532=ORIENTED_EDGE('',*,*,#52214,.F.);
#73533=ORIENTED_EDGE('',*,*,#52207,.F.);
#73534=ORIENTED_EDGE('',*,*,#52215,.F.);
#73535=ORIENTED_EDGE('',*,*,#52216,.T.);
#73536=ORIENTED_EDGE('',*,*,#52217,.F.);
#73537=ORIENTED_EDGE('',*,*,#52210,.F.);
#73538=ORIENTED_EDGE('',*,*,#52218,.F.);
#73539=ORIENTED_EDGE('',*,*,#52219,.T.);
#73540=ORIENTED_EDGE('',*,*,#52220,.F.);
#73541=ORIENTED_EDGE('',*,*,#52213,.F.);
#73542=ORIENTED_EDGE('',*,*,#52221,.F.);
#73543=ORIENTED_EDGE('',*,*,#52216,.F.);
#73544=ORIENTED_EDGE('',*,*,#52222,.F.);
#73545=ORIENTED_EDGE('',*,*,#52219,.F.);
#73546=ORIENTED_EDGE('',*,*,#52223,.F.);
#73547=ORIENTED_EDGE('',*,*,#52224,.T.);
#73548=ORIENTED_EDGE('',*,*,#52225,.F.);
#73549=ORIENTED_EDGE('',*,*,#52226,.T.);
#73550=ORIENTED_EDGE('',*,*,#52227,.F.);
#73551=ORIENTED_EDGE('',*,*,#52228,.T.);
#73552=ORIENTED_EDGE('',*,*,#52229,.F.);
#73553=ORIENTED_EDGE('',*,*,#52226,.F.);
#73554=ORIENTED_EDGE('',*,*,#52230,.F.);
#73555=ORIENTED_EDGE('',*,*,#52231,.T.);
#73556=ORIENTED_EDGE('',*,*,#52232,.F.);
#73557=ORIENTED_EDGE('',*,*,#52224,.F.);
#73558=ORIENTED_EDGE('',*,*,#52233,.F.);
#73559=ORIENTED_EDGE('',*,*,#52234,.T.);
#73560=ORIENTED_EDGE('',*,*,#52235,.F.);
#73561=ORIENTED_EDGE('',*,*,#52228,.F.);
#73562=ORIENTED_EDGE('',*,*,#52236,.F.);
#73563=ORIENTED_EDGE('',*,*,#52237,.T.);
#73564=ORIENTED_EDGE('',*,*,#52238,.F.);
#73565=ORIENTED_EDGE('',*,*,#52231,.F.);
#73566=ORIENTED_EDGE('',*,*,#52239,.F.);
#73567=ORIENTED_EDGE('',*,*,#52240,.T.);
#73568=ORIENTED_EDGE('',*,*,#52241,.F.);
#73569=ORIENTED_EDGE('',*,*,#52234,.F.);
#73570=ORIENTED_EDGE('',*,*,#52242,.F.);
#73571=ORIENTED_EDGE('',*,*,#52243,.T.);
#73572=ORIENTED_EDGE('',*,*,#52244,.F.);
#73573=ORIENTED_EDGE('',*,*,#52237,.F.);
#73574=ORIENTED_EDGE('',*,*,#52245,.F.);
#73575=ORIENTED_EDGE('',*,*,#52240,.F.);
#73576=ORIENTED_EDGE('',*,*,#52246,.F.);
#73577=ORIENTED_EDGE('',*,*,#52243,.F.);
#73578=ORIENTED_EDGE('',*,*,#52247,.F.);
#73579=ORIENTED_EDGE('',*,*,#52248,.T.);
#73580=ORIENTED_EDGE('',*,*,#52249,.F.);
#73581=ORIENTED_EDGE('',*,*,#52250,.T.);
#73582=ORIENTED_EDGE('',*,*,#52251,.F.);
#73583=ORIENTED_EDGE('',*,*,#52252,.T.);
#73584=ORIENTED_EDGE('',*,*,#52253,.F.);
#73585=ORIENTED_EDGE('',*,*,#52250,.F.);
#73586=ORIENTED_EDGE('',*,*,#52254,.F.);
#73587=ORIENTED_EDGE('',*,*,#52255,.T.);
#73588=ORIENTED_EDGE('',*,*,#52256,.F.);
#73589=ORIENTED_EDGE('',*,*,#52248,.F.);
#73590=ORIENTED_EDGE('',*,*,#52257,.F.);
#73591=ORIENTED_EDGE('',*,*,#52258,.T.);
#73592=ORIENTED_EDGE('',*,*,#52259,.F.);
#73593=ORIENTED_EDGE('',*,*,#52252,.F.);
#73594=ORIENTED_EDGE('',*,*,#52260,.F.);
#73595=ORIENTED_EDGE('',*,*,#52261,.T.);
#73596=ORIENTED_EDGE('',*,*,#52262,.F.);
#73597=ORIENTED_EDGE('',*,*,#52255,.F.);
#73598=ORIENTED_EDGE('',*,*,#52263,.F.);
#73599=ORIENTED_EDGE('',*,*,#52264,.T.);
#73600=ORIENTED_EDGE('',*,*,#52265,.F.);
#73601=ORIENTED_EDGE('',*,*,#52258,.F.);
#73602=ORIENTED_EDGE('',*,*,#52266,.F.);
#73603=ORIENTED_EDGE('',*,*,#52267,.T.);
#73604=ORIENTED_EDGE('',*,*,#52268,.F.);
#73605=ORIENTED_EDGE('',*,*,#52261,.F.);
#73606=ORIENTED_EDGE('',*,*,#52269,.F.);
#73607=ORIENTED_EDGE('',*,*,#52264,.F.);
#73608=ORIENTED_EDGE('',*,*,#52270,.F.);
#73609=ORIENTED_EDGE('',*,*,#52267,.F.);
#73610=ORIENTED_EDGE('',*,*,#52271,.F.);
#73611=ORIENTED_EDGE('',*,*,#52272,.T.);
#73612=ORIENTED_EDGE('',*,*,#52273,.F.);
#73613=ORIENTED_EDGE('',*,*,#52274,.T.);
#73614=ORIENTED_EDGE('',*,*,#52275,.F.);
#73615=ORIENTED_EDGE('',*,*,#52276,.T.);
#73616=ORIENTED_EDGE('',*,*,#52277,.F.);
#73617=ORIENTED_EDGE('',*,*,#52274,.F.);
#73618=ORIENTED_EDGE('',*,*,#52278,.F.);
#73619=ORIENTED_EDGE('',*,*,#52279,.T.);
#73620=ORIENTED_EDGE('',*,*,#52280,.F.);
#73621=ORIENTED_EDGE('',*,*,#52272,.F.);
#73622=ORIENTED_EDGE('',*,*,#52281,.F.);
#73623=ORIENTED_EDGE('',*,*,#52282,.T.);
#73624=ORIENTED_EDGE('',*,*,#52283,.F.);
#73625=ORIENTED_EDGE('',*,*,#52276,.F.);
#73626=ORIENTED_EDGE('',*,*,#52284,.F.);
#73627=ORIENTED_EDGE('',*,*,#52285,.T.);
#73628=ORIENTED_EDGE('',*,*,#52286,.F.);
#73629=ORIENTED_EDGE('',*,*,#52279,.F.);
#73630=ORIENTED_EDGE('',*,*,#52287,.F.);
#73631=ORIENTED_EDGE('',*,*,#52282,.F.);
#73632=ORIENTED_EDGE('',*,*,#52288,.F.);
#73633=ORIENTED_EDGE('',*,*,#52285,.F.);
#73634=ORIENTED_EDGE('',*,*,#52289,.F.);
#73635=ORIENTED_EDGE('',*,*,#52290,.F.);
#73636=ORIENTED_EDGE('',*,*,#52291,.T.);
#73637=ORIENTED_EDGE('',*,*,#52292,.F.);
#73638=ORIENTED_EDGE('',*,*,#52293,.T.);
#73639=ORIENTED_EDGE('',*,*,#52294,.T.);
#73640=ORIENTED_EDGE('',*,*,#52295,.F.);
#73641=ORIENTED_EDGE('',*,*,#52293,.F.);
#73642=ORIENTED_EDGE('',*,*,#52296,.F.);
#73643=ORIENTED_EDGE('',*,*,#52297,.T.);
#73644=ORIENTED_EDGE('',*,*,#52298,.F.);
#73645=ORIENTED_EDGE('',*,*,#52291,.F.);
#73646=ORIENTED_EDGE('',*,*,#52299,.F.);
#73647=ORIENTED_EDGE('',*,*,#52300,.T.);
#73648=ORIENTED_EDGE('',*,*,#52301,.F.);
#73649=ORIENTED_EDGE('',*,*,#52294,.F.);
#73650=ORIENTED_EDGE('',*,*,#52302,.F.);
#73651=ORIENTED_EDGE('',*,*,#52303,.T.);
#73652=ORIENTED_EDGE('',*,*,#52304,.F.);
#73653=ORIENTED_EDGE('',*,*,#52297,.F.);
#73654=ORIENTED_EDGE('',*,*,#52305,.F.);
#73655=ORIENTED_EDGE('',*,*,#52300,.F.);
#73656=ORIENTED_EDGE('',*,*,#52306,.F.);
#73657=ORIENTED_EDGE('',*,*,#52303,.F.);
#73658=ORIENTED_EDGE('',*,*,#52307,.F.);
#73659=ORIENTED_EDGE('',*,*,#52308,.F.);
#73660=ORIENTED_EDGE('',*,*,#52309,.T.);
#73661=ORIENTED_EDGE('',*,*,#52310,.F.);
#73662=ORIENTED_EDGE('',*,*,#52309,.F.);
#73663=ORIENTED_EDGE('',*,*,#52311,.F.);
#73664=ORIENTED_EDGE('',*,*,#52312,.T.);
#73665=ORIENTED_EDGE('',*,*,#52313,.F.);
#73666=ORIENTED_EDGE('',*,*,#52312,.F.);
#73667=ORIENTED_EDGE('',*,*,#52314,.T.);
#73668=ORIENTED_EDGE('',*,*,#52315,.F.);
#73669=ORIENTED_EDGE('',*,*,#50135,.F.);
#73670=ORIENTED_EDGE('',*,*,#52316,.F.);
#73671=ORIENTED_EDGE('',*,*,#52317,.T.);
#73672=ORIENTED_EDGE('',*,*,#52318,.F.);
#73673=ORIENTED_EDGE('',*,*,#52314,.F.);
#73674=ORIENTED_EDGE('',*,*,#52319,.F.);
#73675=ORIENTED_EDGE('',*,*,#52320,.T.);
#73676=ORIENTED_EDGE('',*,*,#52321,.F.);
#73677=ORIENTED_EDGE('',*,*,#52317,.F.);
#73678=ORIENTED_EDGE('',*,*,#52322,.F.);
#73679=ORIENTED_EDGE('',*,*,#52323,.T.);
#73680=ORIENTED_EDGE('',*,*,#52324,.F.);
#73681=ORIENTED_EDGE('',*,*,#52320,.F.);
#73682=ORIENTED_EDGE('',*,*,#52325,.F.);
#73683=ORIENTED_EDGE('',*,*,#52326,.T.);
#73684=ORIENTED_EDGE('',*,*,#52327,.F.);
#73685=ORIENTED_EDGE('',*,*,#52323,.F.);
#73686=ORIENTED_EDGE('',*,*,#52328,.F.);
#73687=ORIENTED_EDGE('',*,*,#52329,.T.);
#73688=ORIENTED_EDGE('',*,*,#52330,.F.);
#73689=ORIENTED_EDGE('',*,*,#52326,.F.);
#73690=ORIENTED_EDGE('',*,*,#52331,.F.);
#73691=ORIENTED_EDGE('',*,*,#52332,.T.);
#73692=ORIENTED_EDGE('',*,*,#52333,.F.);
#73693=ORIENTED_EDGE('',*,*,#52329,.F.);
#73694=ORIENTED_EDGE('',*,*,#52334,.F.);
#73695=ORIENTED_EDGE('',*,*,#52335,.T.);
#73696=ORIENTED_EDGE('',*,*,#52336,.F.);
#73697=ORIENTED_EDGE('',*,*,#52332,.F.);
#73698=ORIENTED_EDGE('',*,*,#52337,.F.);
#73699=ORIENTED_EDGE('',*,*,#52338,.F.);
#73700=ORIENTED_EDGE('',*,*,#52335,.F.);
#73701=ORIENTED_EDGE('',*,*,#52339,.F.);
#73702=ORIENTED_EDGE('',*,*,#50152,.T.);
#73703=ORIENTED_EDGE('',*,*,#52340,.T.);
#73704=ORIENTED_EDGE('',*,*,#52341,.F.);
#73705=ORIENTED_EDGE('',*,*,#50157,.F.);
#73706=ORIENTED_EDGE('',*,*,#52342,.F.);
#73707=ORIENTED_EDGE('',*,*,#52343,.T.);
#73708=ORIENTED_EDGE('',*,*,#52344,.F.);
#73709=ORIENTED_EDGE('',*,*,#52340,.F.);
#73710=ORIENTED_EDGE('',*,*,#52345,.F.);
#73711=ORIENTED_EDGE('',*,*,#52346,.T.);
#73712=ORIENTED_EDGE('',*,*,#52347,.F.);
#73713=ORIENTED_EDGE('',*,*,#52343,.F.);
#73714=ORIENTED_EDGE('',*,*,#52348,.F.);
#73715=ORIENTED_EDGE('',*,*,#52349,.T.);
#73716=ORIENTED_EDGE('',*,*,#52350,.F.);
#73717=ORIENTED_EDGE('',*,*,#52346,.F.);
#73718=ORIENTED_EDGE('',*,*,#52351,.F.);
#73719=ORIENTED_EDGE('',*,*,#52352,.T.);
#73720=ORIENTED_EDGE('',*,*,#52353,.F.);
#73721=ORIENTED_EDGE('',*,*,#52349,.F.);
#73722=ORIENTED_EDGE('',*,*,#52354,.F.);
#73723=ORIENTED_EDGE('',*,*,#52355,.T.);
#73724=ORIENTED_EDGE('',*,*,#52356,.F.);
#73725=ORIENTED_EDGE('',*,*,#52352,.F.);
#73726=ORIENTED_EDGE('',*,*,#52357,.F.);
#73727=ORIENTED_EDGE('',*,*,#52358,.T.);
#73728=ORIENTED_EDGE('',*,*,#52359,.F.);
#73729=ORIENTED_EDGE('',*,*,#52355,.F.);
#73730=ORIENTED_EDGE('',*,*,#52360,.F.);
#73731=ORIENTED_EDGE('',*,*,#52361,.T.);
#73732=ORIENTED_EDGE('',*,*,#52362,.F.);
#73733=ORIENTED_EDGE('',*,*,#52358,.F.);
#73734=ORIENTED_EDGE('',*,*,#52363,.F.);
#73735=ORIENTED_EDGE('',*,*,#52364,.F.);
#73736=ORIENTED_EDGE('',*,*,#52361,.F.);
#73737=ORIENTED_EDGE('',*,*,#52365,.F.);
#73738=ORIENTED_EDGE('',*,*,#50174,.T.);
#73739=ORIENTED_EDGE('',*,*,#52366,.T.);
#73740=ORIENTED_EDGE('',*,*,#52367,.F.);
#73741=ORIENTED_EDGE('',*,*,#52368,.F.);
#73742=ORIENTED_EDGE('',*,*,#52369,.F.);
#73743=ORIENTED_EDGE('',*,*,#52370,.T.);
#73744=ORIENTED_EDGE('',*,*,#52371,.F.);
#73745=ORIENTED_EDGE('',*,*,#52366,.F.);
#73746=ORIENTED_EDGE('',*,*,#52372,.F.);
#73747=ORIENTED_EDGE('',*,*,#52373,.F.);
#73748=ORIENTED_EDGE('',*,*,#52374,.T.);
#73749=ORIENTED_EDGE('',*,*,#52375,.F.);
#73750=ORIENTED_EDGE('',*,*,#52370,.F.);
#73751=ORIENTED_EDGE('',*,*,#52376,.T.);
#73752=ORIENTED_EDGE('',*,*,#52377,.F.);
#73753=ORIENTED_EDGE('',*,*,#52374,.F.);
#73754=ORIENTED_EDGE('',*,*,#52378,.F.);
#73755=ORIENTED_EDGE('',*,*,#52379,.T.);
#73756=ORIENTED_EDGE('',*,*,#52380,.F.);
#73757=ORIENTED_EDGE('',*,*,#52376,.F.);
#73758=ORIENTED_EDGE('',*,*,#52381,.F.);
#73759=ORIENTED_EDGE('',*,*,#52382,.T.);
#73760=ORIENTED_EDGE('',*,*,#52383,.F.);
#73761=ORIENTED_EDGE('',*,*,#52379,.F.);
#73762=ORIENTED_EDGE('',*,*,#52384,.F.);
#73763=ORIENTED_EDGE('',*,*,#52385,.F.);
#73764=ORIENTED_EDGE('',*,*,#52386,.F.);
#73765=ORIENTED_EDGE('',*,*,#52382,.F.);
#73766=ORIENTED_EDGE('',*,*,#52387,.F.);
#73767=ORIENTED_EDGE('',*,*,#52388,.T.);
#73768=ORIENTED_EDGE('',*,*,#52389,.F.);
#73769=ORIENTED_EDGE('',*,*,#52390,.F.);
#73770=ORIENTED_EDGE('',*,*,#52391,.F.);
#73771=ORIENTED_EDGE('',*,*,#52392,.T.);
#73772=ORIENTED_EDGE('',*,*,#52393,.F.);
#73773=ORIENTED_EDGE('',*,*,#52388,.F.);
#73774=ORIENTED_EDGE('',*,*,#52394,.F.);
#73775=ORIENTED_EDGE('',*,*,#52395,.T.);
#73776=ORIENTED_EDGE('',*,*,#52396,.F.);
#73777=ORIENTED_EDGE('',*,*,#52392,.F.);
#73778=ORIENTED_EDGE('',*,*,#52397,.F.);
#73779=ORIENTED_EDGE('',*,*,#52398,.T.);
#73780=ORIENTED_EDGE('',*,*,#52399,.F.);
#73781=ORIENTED_EDGE('',*,*,#52395,.F.);
#73782=ORIENTED_EDGE('',*,*,#52400,.F.);
#73783=ORIENTED_EDGE('',*,*,#52401,.T.);
#73784=ORIENTED_EDGE('',*,*,#52402,.F.);
#73785=ORIENTED_EDGE('',*,*,#52398,.F.);
#73786=ORIENTED_EDGE('',*,*,#52403,.F.);
#73787=ORIENTED_EDGE('',*,*,#52404,.T.);
#73788=ORIENTED_EDGE('',*,*,#52405,.F.);
#73789=ORIENTED_EDGE('',*,*,#52401,.F.);
#73790=ORIENTED_EDGE('',*,*,#52406,.F.);
#73791=ORIENTED_EDGE('',*,*,#52407,.F.);
#73792=ORIENTED_EDGE('',*,*,#52408,.F.);
#73793=ORIENTED_EDGE('',*,*,#52404,.F.);
#73794=ORIENTED_EDGE('',*,*,#52409,.F.);
#73795=ORIENTED_EDGE('',*,*,#52410,.T.);
#73796=ORIENTED_EDGE('',*,*,#52411,.F.);
#73797=ORIENTED_EDGE('',*,*,#52412,.F.);
#73798=ORIENTED_EDGE('',*,*,#52413,.F.);
#73799=ORIENTED_EDGE('',*,*,#52414,.T.);
#73800=ORIENTED_EDGE('',*,*,#52415,.F.);
#73801=ORIENTED_EDGE('',*,*,#52410,.F.);
#73802=ORIENTED_EDGE('',*,*,#52416,.F.);
#73803=ORIENTED_EDGE('',*,*,#52417,.F.);
#73804=ORIENTED_EDGE('',*,*,#52418,.T.);
#73805=ORIENTED_EDGE('',*,*,#52419,.F.);
#73806=ORIENTED_EDGE('',*,*,#52414,.F.);
#73807=ORIENTED_EDGE('',*,*,#52420,.T.);
#73808=ORIENTED_EDGE('',*,*,#52421,.F.);
#73809=ORIENTED_EDGE('',*,*,#52418,.F.);
#73810=ORIENTED_EDGE('',*,*,#52422,.F.);
#73811=ORIENTED_EDGE('',*,*,#52423,.T.);
#73812=ORIENTED_EDGE('',*,*,#52424,.F.);
#73813=ORIENTED_EDGE('',*,*,#52420,.F.);
#73814=ORIENTED_EDGE('',*,*,#52425,.F.);
#73815=ORIENTED_EDGE('',*,*,#52426,.T.);
#73816=ORIENTED_EDGE('',*,*,#52427,.F.);
#73817=ORIENTED_EDGE('',*,*,#52423,.F.);
#73818=ORIENTED_EDGE('',*,*,#52428,.F.);
#73819=ORIENTED_EDGE('',*,*,#52429,.F.);
#73820=ORIENTED_EDGE('',*,*,#52430,.F.);
#73821=ORIENTED_EDGE('',*,*,#52426,.F.);
#73822=ORIENTED_EDGE('',*,*,#52431,.F.);
#73823=ORIENTED_EDGE('',*,*,#52432,.F.);
#73824=ORIENTED_EDGE('',*,*,#52433,.F.);
#73825=ORIENTED_EDGE('',*,*,#52434,.T.);
#73826=ORIENTED_EDGE('',*,*,#52435,.F.);
#73827=ORIENTED_EDGE('',*,*,#52436,.T.);
#73828=ORIENTED_EDGE('',*,*,#52437,.F.);
#73829=ORIENTED_EDGE('',*,*,#52434,.F.);
#73830=ORIENTED_EDGE('',*,*,#52438,.F.);
#73831=ORIENTED_EDGE('',*,*,#52439,.T.);
#73832=ORIENTED_EDGE('',*,*,#52440,.F.);
#73833=ORIENTED_EDGE('',*,*,#52436,.F.);
#73834=ORIENTED_EDGE('',*,*,#52441,.F.);
#73835=ORIENTED_EDGE('',*,*,#52442,.T.);
#73836=ORIENTED_EDGE('',*,*,#52443,.F.);
#73837=ORIENTED_EDGE('',*,*,#52439,.F.);
#73838=ORIENTED_EDGE('',*,*,#52444,.F.);
#73839=ORIENTED_EDGE('',*,*,#52445,.T.);
#73840=ORIENTED_EDGE('',*,*,#52446,.F.);
#73841=ORIENTED_EDGE('',*,*,#52442,.F.);
#73842=ORIENTED_EDGE('',*,*,#52447,.F.);
#73843=ORIENTED_EDGE('',*,*,#52448,.T.);
#73844=ORIENTED_EDGE('',*,*,#52449,.F.);
#73845=ORIENTED_EDGE('',*,*,#52445,.F.);
#73846=ORIENTED_EDGE('',*,*,#52450,.F.);
#73847=ORIENTED_EDGE('',*,*,#52451,.F.);
#73848=ORIENTED_EDGE('',*,*,#52452,.F.);
#73849=ORIENTED_EDGE('',*,*,#52448,.F.);
#73850=ORIENTED_EDGE('',*,*,#52453,.F.);
#73851=ORIENTED_EDGE('',*,*,#52454,.F.);
#73852=ORIENTED_EDGE('',*,*,#50267,.F.);
#73853=ORIENTED_EDGE('',*,*,#52455,.F.);
#73854=ORIENTED_EDGE('',*,*,#52456,.T.);
#73855=ORIENTED_EDGE('',*,*,#52457,.T.);
#73856=ORIENTED_EDGE('',*,*,#52458,.F.);
#73857=ORIENTED_EDGE('',*,*,#52456,.F.);
#73858=ORIENTED_EDGE('',*,*,#52459,.F.);
#73859=ORIENTED_EDGE('',*,*,#52460,.T.);
#73860=ORIENTED_EDGE('',*,*,#52461,.F.);
#73861=ORIENTED_EDGE('',*,*,#52457,.F.);
#73862=ORIENTED_EDGE('',*,*,#52462,.F.);
#73863=ORIENTED_EDGE('',*,*,#52463,.T.);
#73864=ORIENTED_EDGE('',*,*,#52464,.F.);
#73865=ORIENTED_EDGE('',*,*,#52460,.F.);
#73866=ORIENTED_EDGE('',*,*,#52465,.F.);
#73867=ORIENTED_EDGE('',*,*,#52466,.T.);
#73868=ORIENTED_EDGE('',*,*,#52467,.F.);
#73869=ORIENTED_EDGE('',*,*,#52463,.F.);
#73870=ORIENTED_EDGE('',*,*,#52468,.F.);
#73871=ORIENTED_EDGE('',*,*,#52469,.T.);
#73872=ORIENTED_EDGE('',*,*,#52470,.F.);
#73873=ORIENTED_EDGE('',*,*,#52466,.F.);
#73874=ORIENTED_EDGE('',*,*,#52471,.F.);
#73875=ORIENTED_EDGE('',*,*,#52472,.T.);
#73876=ORIENTED_EDGE('',*,*,#52473,.F.);
#73877=ORIENTED_EDGE('',*,*,#52469,.F.);
#73878=ORIENTED_EDGE('',*,*,#52474,.F.);
#73879=ORIENTED_EDGE('',*,*,#52475,.T.);
#73880=ORIENTED_EDGE('',*,*,#52476,.F.);
#73881=ORIENTED_EDGE('',*,*,#52472,.F.);
#73882=ORIENTED_EDGE('',*,*,#52477,.F.);
#73883=ORIENTED_EDGE('',*,*,#52478,.F.);
#73884=ORIENTED_EDGE('',*,*,#52475,.F.);
#73885=ORIENTED_EDGE('',*,*,#52479,.F.);
#73886=ORIENTED_EDGE('',*,*,#50284,.T.);
#73887=ORIENTED_EDGE('',*,*,#52480,.F.);
#73888=ORIENTED_EDGE('',*,*,#52481,.F.);
#73889=ORIENTED_EDGE('',*,*,#52482,.T.);
#73890=ORIENTED_EDGE('',*,*,#52483,.F.);
#73891=ORIENTED_EDGE('',*,*,#50289,.F.);
#73892=ORIENTED_EDGE('',*,*,#52484,.F.);
#73893=ORIENTED_EDGE('',*,*,#52485,.T.);
#73894=ORIENTED_EDGE('',*,*,#52486,.F.);
#73895=ORIENTED_EDGE('',*,*,#52482,.F.);
#73896=ORIENTED_EDGE('',*,*,#52487,.F.);
#73897=ORIENTED_EDGE('',*,*,#52488,.T.);
#73898=ORIENTED_EDGE('',*,*,#52489,.F.);
#73899=ORIENTED_EDGE('',*,*,#52485,.F.);
#73900=ORIENTED_EDGE('',*,*,#52490,.F.);
#73901=ORIENTED_EDGE('',*,*,#52491,.T.);
#73902=ORIENTED_EDGE('',*,*,#52492,.F.);
#73903=ORIENTED_EDGE('',*,*,#52488,.F.);
#73904=ORIENTED_EDGE('',*,*,#52493,.F.);
#73905=ORIENTED_EDGE('',*,*,#52494,.T.);
#73906=ORIENTED_EDGE('',*,*,#52495,.F.);
#73907=ORIENTED_EDGE('',*,*,#52491,.F.);
#73908=ORIENTED_EDGE('',*,*,#52496,.F.);
#73909=ORIENTED_EDGE('',*,*,#52497,.T.);
#73910=ORIENTED_EDGE('',*,*,#52498,.F.);
#73911=ORIENTED_EDGE('',*,*,#52494,.F.);
#73912=ORIENTED_EDGE('',*,*,#52499,.F.);
#73913=ORIENTED_EDGE('',*,*,#52500,.T.);
#73914=ORIENTED_EDGE('',*,*,#52501,.F.);
#73915=ORIENTED_EDGE('',*,*,#52497,.F.);
#73916=ORIENTED_EDGE('',*,*,#52502,.F.);
#73917=ORIENTED_EDGE('',*,*,#52503,.T.);
#73918=ORIENTED_EDGE('',*,*,#52504,.F.);
#73919=ORIENTED_EDGE('',*,*,#52500,.F.);
#73920=ORIENTED_EDGE('',*,*,#52505,.F.);
#73921=ORIENTED_EDGE('',*,*,#52506,.T.);
#73922=ORIENTED_EDGE('',*,*,#52507,.F.);
#73923=ORIENTED_EDGE('',*,*,#52503,.F.);
#73924=ORIENTED_EDGE('',*,*,#52508,.F.);
#73925=ORIENTED_EDGE('',*,*,#52509,.F.);
#73926=ORIENTED_EDGE('',*,*,#52510,.F.);
#73927=ORIENTED_EDGE('',*,*,#52511,.F.);
#73928=ORIENTED_EDGE('',*,*,#52512,.F.);
#73929=ORIENTED_EDGE('',*,*,#52513,.F.);
#73930=ORIENTED_EDGE('',*,*,#52514,.T.);
#73931=ORIENTED_EDGE('',*,*,#52515,.F.);
#73932=ORIENTED_EDGE('',*,*,#52506,.F.);
#73933=ORIENTED_EDGE('',*,*,#52516,.F.);
#73934=ORIENTED_EDGE('',*,*,#52517,.T.);
#73935=ORIENTED_EDGE('',*,*,#52518,.F.);
#73936=ORIENTED_EDGE('',*,*,#52514,.F.);
#73937=ORIENTED_EDGE('',*,*,#52519,.F.);
#73938=ORIENTED_EDGE('',*,*,#52520,.T.);
#73939=ORIENTED_EDGE('',*,*,#52521,.F.);
#73940=ORIENTED_EDGE('',*,*,#52517,.F.);
#73941=ORIENTED_EDGE('',*,*,#52522,.F.);
#73942=ORIENTED_EDGE('',*,*,#52523,.T.);
#73943=ORIENTED_EDGE('',*,*,#52524,.F.);
#73944=ORIENTED_EDGE('',*,*,#52520,.F.);
#73945=ORIENTED_EDGE('',*,*,#52525,.F.);
#73946=ORIENTED_EDGE('',*,*,#52526,.T.);
#73947=ORIENTED_EDGE('',*,*,#52527,.F.);
#73948=ORIENTED_EDGE('',*,*,#52523,.F.);
#73949=ORIENTED_EDGE('',*,*,#52528,.F.);
#73950=ORIENTED_EDGE('',*,*,#52529,.T.);
#73951=ORIENTED_EDGE('',*,*,#52530,.F.);
#73952=ORIENTED_EDGE('',*,*,#52526,.F.);
#73953=ORIENTED_EDGE('',*,*,#52531,.F.);
#73954=ORIENTED_EDGE('',*,*,#52532,.T.);
#73955=ORIENTED_EDGE('',*,*,#52533,.F.);
#73956=ORIENTED_EDGE('',*,*,#52529,.F.);
#73957=ORIENTED_EDGE('',*,*,#52534,.F.);
#73958=ORIENTED_EDGE('',*,*,#52535,.F.);
#73959=ORIENTED_EDGE('',*,*,#52536,.T.);
#73960=ORIENTED_EDGE('',*,*,#52537,.T.);
#73961=ORIENTED_EDGE('',*,*,#52538,.T.);
#73962=ORIENTED_EDGE('',*,*,#50340,.T.);
#73963=ORIENTED_EDGE('',*,*,#52539,.F.);
#73964=ORIENTED_EDGE('',*,*,#52532,.F.);
#73965=ORIENTED_EDGE('',*,*,#52540,.F.);
#73966=ORIENTED_EDGE('',*,*,#52541,.F.);
#73967=ORIENTED_EDGE('',*,*,#52542,.F.);
#73968=ORIENTED_EDGE('',*,*,#51443,.T.);
#73969=ORIENTED_EDGE('',*,*,#51437,.T.);
#73970=ORIENTED_EDGE('',*,*,#52543,.F.);
#73971=ORIENTED_EDGE('',*,*,#52544,.T.);
#73972=ORIENTED_EDGE('',*,*,#52545,.T.);
#73973=ORIENTED_EDGE('',*,*,#52546,.F.);
#73974=ORIENTED_EDGE('',*,*,#52544,.F.);
#73975=ORIENTED_EDGE('',*,*,#52547,.F.);
#73976=ORIENTED_EDGE('',*,*,#52548,.T.);
#73977=ORIENTED_EDGE('',*,*,#52549,.F.);
#73978=ORIENTED_EDGE('',*,*,#52545,.F.);
#73979=ORIENTED_EDGE('',*,*,#52550,.F.);
#73980=ORIENTED_EDGE('',*,*,#52551,.T.);
#73981=ORIENTED_EDGE('',*,*,#52552,.F.);
#73982=ORIENTED_EDGE('',*,*,#52548,.F.);
#73983=ORIENTED_EDGE('',*,*,#52553,.F.);
#73984=ORIENTED_EDGE('',*,*,#52554,.T.);
#73985=ORIENTED_EDGE('',*,*,#52555,.F.);
#73986=ORIENTED_EDGE('',*,*,#52551,.F.);
#73987=ORIENTED_EDGE('',*,*,#52556,.F.);
#73988=ORIENTED_EDGE('',*,*,#52557,.T.);
#73989=ORIENTED_EDGE('',*,*,#52558,.F.);
#73990=ORIENTED_EDGE('',*,*,#52559,.T.);
#73991=ORIENTED_EDGE('',*,*,#52557,.F.);
#73992=ORIENTED_EDGE('',*,*,#52560,.F.);
#73993=ORIENTED_EDGE('',*,*,#52559,.F.);
#73994=ORIENTED_EDGE('',*,*,#52561,.T.);
#73995=ORIENTED_EDGE('',*,*,#52554,.F.);
#73996=ORIENTED_EDGE('',*,*,#52562,.T.);
#73997=ORIENTED_EDGE('',*,*,#52563,.F.);
#73998=ORIENTED_EDGE('',*,*,#52561,.F.);
#73999=ORIENTED_EDGE('',*,*,#52564,.F.);
#74000=ORIENTED_EDGE('',*,*,#52565,.F.);
#74001=ORIENTED_EDGE('',*,*,#52566,.F.);
#74002=ORIENTED_EDGE('',*,*,#52567,.F.);
#74003=ORIENTED_EDGE('',*,*,#52568,.F.);
#74004=ORIENTED_EDGE('',*,*,#52569,.F.);
#74005=ORIENTED_EDGE('',*,*,#52570,.F.);
#74006=ORIENTED_EDGE('',*,*,#52571,.T.);
#74007=ORIENTED_EDGE('',*,*,#52572,.T.);
#74008=ORIENTED_EDGE('',*,*,#52562,.F.);
#74009=ORIENTED_EDGE('',*,*,#52573,.F.);
#74010=ORIENTED_EDGE('',*,*,#52574,.T.);
#74011=ORIENTED_EDGE('',*,*,#52571,.F.);
#74012=ORIENTED_EDGE('',*,*,#52575,.F.);
#74013=ORIENTED_EDGE('',*,*,#52574,.F.);
#74014=ORIENTED_EDGE('',*,*,#52576,.F.);
#74015=ORIENTED_EDGE('',*,*,#52577,.T.);
#74016=ORIENTED_EDGE('',*,*,#52578,.F.);
#74017=ORIENTED_EDGE('',*,*,#52572,.F.);
#74018=ORIENTED_EDGE('',*,*,#52579,.T.);
#74019=ORIENTED_EDGE('',*,*,#52580,.F.);
#74020=ORIENTED_EDGE('',*,*,#52577,.F.);
#74021=ORIENTED_EDGE('',*,*,#52581,.F.);
#74022=ORIENTED_EDGE('',*,*,#52582,.T.);
#74023=ORIENTED_EDGE('',*,*,#52583,.F.);
#74024=ORIENTED_EDGE('',*,*,#52579,.F.);
#74025=ORIENTED_EDGE('',*,*,#52584,.F.);
#74026=ORIENTED_EDGE('',*,*,#52585,.T.);
#74027=ORIENTED_EDGE('',*,*,#52586,.F.);
#74028=ORIENTED_EDGE('',*,*,#52582,.F.);
#74029=ORIENTED_EDGE('',*,*,#52587,.F.);
#74030=ORIENTED_EDGE('',*,*,#51467,.T.);
#74031=ORIENTED_EDGE('',*,*,#51461,.T.);
#74032=ORIENTED_EDGE('',*,*,#52588,.F.);
#74033=ORIENTED_EDGE('',*,*,#52585,.F.);
#74034=ORIENTED_EDGE('',*,*,#52589,.F.);
#74035=ORIENTED_EDGE('',*,*,#52590,.F.);
#74036=ORIENTED_EDGE('',*,*,#52591,.F.);
#74037=ORIENTED_EDGE('',*,*,#52592,.T.);
#74038=ORIENTED_EDGE('',*,*,#52593,.F.);
#74039=ORIENTED_EDGE('',*,*,#50392,.F.);
#74040=ORIENTED_EDGE('',*,*,#52594,.T.);
#74041=ORIENTED_EDGE('',*,*,#52595,.T.);
#74042=ORIENTED_EDGE('',*,*,#52596,.T.);
#74043=ORIENTED_EDGE('',*,*,#52597,.T.);
#74044=ORIENTED_EDGE('',*,*,#52598,.F.);
#74045=ORIENTED_EDGE('',*,*,#52599,.F.);
#74046=ORIENTED_EDGE('',*,*,#52600,.T.);
#74047=ORIENTED_EDGE('',*,*,#52601,.T.);
#74048=ORIENTED_EDGE('',*,*,#52592,.F.);
#74049=ORIENTED_EDGE('',*,*,#52602,.F.);
#74050=ORIENTED_EDGE('',*,*,#52603,.T.);
#74051=ORIENTED_EDGE('',*,*,#52600,.F.);
#74052=ORIENTED_EDGE('',*,*,#52604,.F.);
#74053=ORIENTED_EDGE('',*,*,#52603,.F.);
#74054=ORIENTED_EDGE('',*,*,#52605,.F.);
#74055=ORIENTED_EDGE('',*,*,#52606,.T.);
#74056=ORIENTED_EDGE('',*,*,#52607,.F.);
#74057=ORIENTED_EDGE('',*,*,#52601,.F.);
#74058=ORIENTED_EDGE('',*,*,#52608,.T.);
#74059=ORIENTED_EDGE('',*,*,#52609,.F.);
#74060=ORIENTED_EDGE('',*,*,#52606,.F.);
#74061=ORIENTED_EDGE('',*,*,#52610,.F.);
#74062=ORIENTED_EDGE('',*,*,#52611,.T.);
#74063=ORIENTED_EDGE('',*,*,#52612,.F.);
#74064=ORIENTED_EDGE('',*,*,#52608,.F.);
#74065=ORIENTED_EDGE('',*,*,#52613,.F.);
#74066=ORIENTED_EDGE('',*,*,#52614,.T.);
#74067=ORIENTED_EDGE('',*,*,#52615,.F.);
#74068=ORIENTED_EDGE('',*,*,#52611,.F.);
#74069=ORIENTED_EDGE('',*,*,#52616,.F.);
#74070=ORIENTED_EDGE('',*,*,#52617,.F.);
#74071=ORIENTED_EDGE('',*,*,#51433,.T.);
#74072=ORIENTED_EDGE('',*,*,#51439,.T.);
#74073=ORIENTED_EDGE('',*,*,#52618,.F.);
#74074=ORIENTED_EDGE('',*,*,#52614,.F.);
#74075=ORIENTED_EDGE('',*,*,#50411,.F.);
#74076=ORIENTED_EDGE('',*,*,#52619,.F.);
#74077=ORIENTED_EDGE('',*,*,#52620,.T.);
#74078=ORIENTED_EDGE('',*,*,#52621,.F.);
#74079=ORIENTED_EDGE('',*,*,#52622,.F.);
#74080=ORIENTED_EDGE('',*,*,#52623,.F.);
#74081=ORIENTED_EDGE('',*,*,#52620,.F.);
#74082=ORIENTED_EDGE('',*,*,#52624,.F.);
#74083=ORIENTED_EDGE('',*,*,#52625,.T.);
#74084=ORIENTED_EDGE('',*,*,#52626,.F.);
#74085=ORIENTED_EDGE('',*,*,#52627,.F.);
#74086=ORIENTED_EDGE('',*,*,#52628,.T.);
#74087=ORIENTED_EDGE('',*,*,#52629,.T.);
#74088=ORIENTED_EDGE('',*,*,#52625,.F.);
#74089=ORIENTED_EDGE('',*,*,#52630,.F.);
#74090=ORIENTED_EDGE('',*,*,#52631,.T.);
#74091=ORIENTED_EDGE('',*,*,#52628,.F.);
#74092=ORIENTED_EDGE('',*,*,#52632,.F.);
#74093=ORIENTED_EDGE('',*,*,#52633,.T.);
#74094=ORIENTED_EDGE('',*,*,#52631,.F.);
#74095=ORIENTED_EDGE('',*,*,#52634,.F.);
#74096=ORIENTED_EDGE('',*,*,#52635,.F.);
#74097=ORIENTED_EDGE('',*,*,#52629,.F.);
#74098=ORIENTED_EDGE('',*,*,#52636,.T.);
#74099=ORIENTED_EDGE('',*,*,#52637,.F.);
#74100=ORIENTED_EDGE('',*,*,#52633,.F.);
#74101=ORIENTED_EDGE('',*,*,#52638,.F.);
#74102=ORIENTED_EDGE('',*,*,#52639,.T.);
#74103=ORIENTED_EDGE('',*,*,#52640,.F.);
#74104=ORIENTED_EDGE('',*,*,#52636,.F.);
#74105=ORIENTED_EDGE('',*,*,#52641,.F.);
#74106=ORIENTED_EDGE('',*,*,#52642,.T.);
#74107=ORIENTED_EDGE('',*,*,#52643,.F.);
#74108=ORIENTED_EDGE('',*,*,#52639,.F.);
#74109=ORIENTED_EDGE('',*,*,#52644,.F.);
#74110=ORIENTED_EDGE('',*,*,#51469,.T.);
#74111=ORIENTED_EDGE('',*,*,#51476,.T.);
#74112=ORIENTED_EDGE('',*,*,#52645,.F.);
#74113=ORIENTED_EDGE('',*,*,#52642,.F.);
#74114=ORIENTED_EDGE('',*,*,#52646,.F.);
#74115=ORIENTED_EDGE('',*,*,#52647,.F.);
#74116=ORIENTED_EDGE('',*,*,#52534,.T.);
#74117=ORIENTED_EDGE('',*,*,#52648,.F.);
#74118=ORIENTED_EDGE('',*,*,#52602,.T.);
#74119=ORIENTED_EDGE('',*,*,#52649,.F.);
#74120=ORIENTED_EDGE('',*,*,#52516,.T.);
#74121=ORIENTED_EDGE('',*,*,#52650,.F.);
#74122=ORIENTED_EDGE('',*,*,#52560,.T.);
#74123=ORIENTED_EDGE('',*,*,#52651,.F.);
#74124=ORIENTED_EDGE('',*,*,#52505,.T.);
#74125=ORIENTED_EDGE('',*,*,#52652,.F.);
#74126=ORIENTED_EDGE('',*,*,#52573,.T.);
#74127=ORIENTED_EDGE('',*,*,#52653,.F.);
#74128=ORIENTED_EDGE('',*,*,#52487,.T.);
#74129=ORIENTED_EDGE('',*,*,#52654,.F.);
#74130=ORIENTED_EDGE('',*,*,#52634,.T.);
#74131=ORIENTED_EDGE('',*,*,#52655,.F.);
#74132=ORIENTED_EDGE('',*,*,#52656,.F.);
#74133=ORIENTED_EDGE('',*,*,#52375,.T.);
#74134=ORIENTED_EDGE('',*,*,#52657,.F.);
#74135=ORIENTED_EDGE('',*,*,#52658,.F.);
#74136=ORIENTED_EDGE('',*,*,#52452,.T.);
#74137=ORIENTED_EDGE('',*,*,#52659,.F.);
#74138=ORIENTED_EDGE('',*,*,#52660,.F.);
#74139=ORIENTED_EDGE('',*,*,#52661,.F.);
#74140=ORIENTED_EDGE('',*,*,#52396,.T.);
#74141=ORIENTED_EDGE('',*,*,#52662,.F.);
#74142=ORIENTED_EDGE('',*,*,#52663,.F.);
#74143=ORIENTED_EDGE('',*,*,#52664,.F.);
#74144=ORIENTED_EDGE('',*,*,#52389,.T.);
#74145=ORIENTED_EDGE('',*,*,#52665,.F.);
#74146=ORIENTED_EDGE('',*,*,#52666,.F.);
#74147=ORIENTED_EDGE('',*,*,#52667,.F.);
#74148=ORIENTED_EDGE('',*,*,#52386,.T.);
#74149=ORIENTED_EDGE('',*,*,#52668,.F.);
#74150=ORIENTED_EDGE('',*,*,#52669,.F.);
#74151=ORIENTED_EDGE('',*,*,#52670,.F.);
#74152=ORIENTED_EDGE('',*,*,#52380,.T.);
#74153=ORIENTED_EDGE('',*,*,#52671,.F.);
#74154=ORIENTED_EDGE('',*,*,#52672,.F.);
#74155=ORIENTED_EDGE('',*,*,#52673,.F.);
#74156=ORIENTED_EDGE('',*,*,#52367,.T.);
#74157=ORIENTED_EDGE('',*,*,#52674,.F.);
#74158=ORIENTED_EDGE('',*,*,#52675,.F.);
#74159=ORIENTED_EDGE('',*,*,#52676,.F.);
#74160=ORIENTED_EDGE('',*,*,#52430,.T.);
#74161=ORIENTED_EDGE('',*,*,#52677,.F.);
#74162=ORIENTED_EDGE('',*,*,#52678,.F.);
#74163=ORIENTED_EDGE('',*,*,#52679,.F.);
#74164=ORIENTED_EDGE('',*,*,#52411,.T.);
#74165=ORIENTED_EDGE('',*,*,#52680,.F.);
#74166=ORIENTED_EDGE('',*,*,#52681,.F.);
#74167=ORIENTED_EDGE('',*,*,#52682,.F.);
#74168=ORIENTED_EDGE('',*,*,#52683,.F.);
#74169=ORIENTED_EDGE('',*,*,#52064,.T.);
#74170=ORIENTED_EDGE('',*,*,#52684,.F.);
#74171=ORIENTED_EDGE('',*,*,#52685,.F.);
#74172=ORIENTED_EDGE('',*,*,#51941,.T.);
#74173=ORIENTED_EDGE('',*,*,#52686,.F.);
#74174=ORIENTED_EDGE('',*,*,#52687,.F.);
#74175=ORIENTED_EDGE('',*,*,#52688,.F.);
#74176=ORIENTED_EDGE('',*,*,#51916,.T.);
#74177=ORIENTED_EDGE('',*,*,#52689,.F.);
#74178=ORIENTED_EDGE('',*,*,#52690,.F.);
#74179=ORIENTED_EDGE('',*,*,#52691,.F.);
#74180=ORIENTED_EDGE('',*,*,#51927,.T.);
#74181=ORIENTED_EDGE('',*,*,#52692,.F.);
#74182=ORIENTED_EDGE('',*,*,#52693,.F.);
#74183=ORIENTED_EDGE('',*,*,#52694,.F.);
#74184=ORIENTED_EDGE('',*,*,#51939,.T.);
#74185=ORIENTED_EDGE('',*,*,#52695,.F.);
#74186=ORIENTED_EDGE('',*,*,#52696,.F.);
#74187=ORIENTED_EDGE('',*,*,#52697,.F.);
#74188=ORIENTED_EDGE('',*,*,#51886,.T.);
#74189=ORIENTED_EDGE('',*,*,#52698,.F.);
#74190=ORIENTED_EDGE('',*,*,#52699,.F.);
#74191=ORIENTED_EDGE('',*,*,#52700,.F.);
#74192=ORIENTED_EDGE('',*,*,#51897,.T.);
#74193=ORIENTED_EDGE('',*,*,#52701,.F.);
#74194=ORIENTED_EDGE('',*,*,#52702,.F.);
#74195=ORIENTED_EDGE('',*,*,#52703,.F.);
#74196=ORIENTED_EDGE('',*,*,#51909,.T.);
#74197=ORIENTED_EDGE('',*,*,#52704,.F.);
#74198=ORIENTED_EDGE('',*,*,#52705,.F.);
#74199=ORIENTED_EDGE('',*,*,#52706,.F.);
#74200=ORIENTED_EDGE('',*,*,#51911,.T.);
#74201=ORIENTED_EDGE('',*,*,#52707,.F.);
#74202=ORIENTED_EDGE('',*,*,#52708,.F.);
#74203=ORIENTED_EDGE('',*,*,#52709,.F.);
#74204=ORIENTED_EDGE('',*,*,#51686,.T.);
#74205=ORIENTED_EDGE('',*,*,#52710,.F.);
#74206=ORIENTED_EDGE('',*,*,#52711,.F.);
#74207=ORIENTED_EDGE('',*,*,#52712,.F.);
#74208=ORIENTED_EDGE('',*,*,#51674,.T.);
#74209=ORIENTED_EDGE('',*,*,#52713,.F.);
#74210=ORIENTED_EDGE('',*,*,#52714,.F.);
#74211=ORIENTED_EDGE('',*,*,#52715,.F.);
#74212=ORIENTED_EDGE('',*,*,#51661,.T.);
#74213=ORIENTED_EDGE('',*,*,#52716,.F.);
#74214=ORIENTED_EDGE('',*,*,#52717,.F.);
#74215=ORIENTED_EDGE('',*,*,#52718,.F.);
#74216=ORIENTED_EDGE('',*,*,#51672,.T.);
#74217=ORIENTED_EDGE('',*,*,#52719,.F.);
#74218=ORIENTED_EDGE('',*,*,#52720,.F.);
#74219=ORIENTED_EDGE('',*,*,#52721,.F.);
#74220=ORIENTED_EDGE('',*,*,#52055,.T.);
#74221=ORIENTED_EDGE('',*,*,#52722,.F.);
#74222=ORIENTED_EDGE('',*,*,#52723,.F.);
#74223=ORIENTED_EDGE('',*,*,#52724,.F.);
#74224=ORIENTED_EDGE('',*,*,#52042,.T.);
#74225=ORIENTED_EDGE('',*,*,#52725,.F.);
#74226=ORIENTED_EDGE('',*,*,#52726,.F.);
#74227=ORIENTED_EDGE('',*,*,#52727,.F.);
#74228=ORIENTED_EDGE('',*,*,#52053,.T.);
#74229=ORIENTED_EDGE('',*,*,#52728,.F.);
#74230=ORIENTED_EDGE('',*,*,#52729,.F.);
#74231=ORIENTED_EDGE('',*,*,#52730,.F.);
#74232=ORIENTED_EDGE('',*,*,#52302,.T.);
#74233=ORIENTED_EDGE('',*,*,#52731,.F.);
#74234=ORIENTED_EDGE('',*,*,#52732,.F.);
#74235=ORIENTED_EDGE('',*,*,#52733,.F.);
#74236=ORIENTED_EDGE('',*,*,#52304,.T.);
#74237=ORIENTED_EDGE('',*,*,#52734,.F.);
#74238=ORIENTED_EDGE('',*,*,#52735,.F.);
#74239=ORIENTED_EDGE('',*,*,#52736,.F.);
#74240=ORIENTED_EDGE('',*,*,#52737,.F.);
#74241=ORIENTED_EDGE('',*,*,#52292,.T.);
#74242=ORIENTED_EDGE('',*,*,#52738,.F.);
#74243=ORIENTED_EDGE('',*,*,#52739,.F.);
#74244=ORIENTED_EDGE('',*,*,#51749,.T.);
#74245=ORIENTED_EDGE('',*,*,#52740,.F.);
#74246=ORIENTED_EDGE('',*,*,#52741,.F.);
#74247=ORIENTED_EDGE('',*,*,#52742,.F.);
#74248=ORIENTED_EDGE('',*,*,#51736,.T.);
#74249=ORIENTED_EDGE('',*,*,#52743,.F.);
#74250=ORIENTED_EDGE('',*,*,#52744,.F.);
#74251=ORIENTED_EDGE('',*,*,#52745,.F.);
#74252=ORIENTED_EDGE('',*,*,#51747,.T.);
#74253=ORIENTED_EDGE('',*,*,#52746,.F.);
#74254=ORIENTED_EDGE('',*,*,#52747,.F.);
#74255=ORIENTED_EDGE('',*,*,#52748,.F.);
#74256=ORIENTED_EDGE('',*,*,#51757,.T.);
#74257=ORIENTED_EDGE('',*,*,#52749,.F.);
#74258=ORIENTED_EDGE('',*,*,#52750,.F.);
#74259=ORIENTED_EDGE('',*,*,#52751,.F.);
#74260=ORIENTED_EDGE('',*,*,#51773,.T.);
#74261=ORIENTED_EDGE('',*,*,#52752,.F.);
#74262=ORIENTED_EDGE('',*,*,#52753,.F.);
#74263=ORIENTED_EDGE('',*,*,#52754,.F.);
#74264=ORIENTED_EDGE('',*,*,#51760,.T.);
#74265=ORIENTED_EDGE('',*,*,#52755,.F.);
#74266=ORIENTED_EDGE('',*,*,#52756,.F.);
#74267=ORIENTED_EDGE('',*,*,#52757,.F.);
#74268=ORIENTED_EDGE('',*,*,#51771,.T.);
#74269=ORIENTED_EDGE('',*,*,#52758,.F.);
#74270=ORIENTED_EDGE('',*,*,#52759,.F.);
#74271=ORIENTED_EDGE('',*,*,#52760,.F.);
#74272=ORIENTED_EDGE('',*,*,#51781,.T.);
#74273=ORIENTED_EDGE('',*,*,#52761,.F.);
#74274=ORIENTED_EDGE('',*,*,#52762,.F.);
#74275=ORIENTED_EDGE('',*,*,#52763,.F.);
#74276=ORIENTED_EDGE('',*,*,#52147,.T.);
#74277=ORIENTED_EDGE('',*,*,#52764,.F.);
#74278=ORIENTED_EDGE('',*,*,#52765,.F.);
#74279=ORIENTED_EDGE('',*,*,#52766,.F.);
#74280=ORIENTED_EDGE('',*,*,#52158,.T.);
#74281=ORIENTED_EDGE('',*,*,#52767,.F.);
#74282=ORIENTED_EDGE('',*,*,#52768,.F.);
#74283=ORIENTED_EDGE('',*,*,#52769,.F.);
#74284=ORIENTED_EDGE('',*,*,#52170,.T.);
#74285=ORIENTED_EDGE('',*,*,#52770,.F.);
#74286=ORIENTED_EDGE('',*,*,#52771,.F.);
#74287=ORIENTED_EDGE('',*,*,#52772,.F.);
#74288=ORIENTED_EDGE('',*,*,#52160,.T.);
#74289=ORIENTED_EDGE('',*,*,#52773,.F.);
#74290=ORIENTED_EDGE('',*,*,#52774,.F.);
#74291=ORIENTED_EDGE('',*,*,#52775,.F.);
#74292=ORIENTED_EDGE('',*,*,#52093,.T.);
#74293=ORIENTED_EDGE('',*,*,#52776,.F.);
#74294=ORIENTED_EDGE('',*,*,#52777,.F.);
#74295=ORIENTED_EDGE('',*,*,#52778,.F.);
#74296=ORIENTED_EDGE('',*,*,#52104,.T.);
#74297=ORIENTED_EDGE('',*,*,#52779,.F.);
#74298=ORIENTED_EDGE('',*,*,#52780,.F.);
#74299=ORIENTED_EDGE('',*,*,#52781,.F.);
#74300=ORIENTED_EDGE('',*,*,#52118,.T.);
#74301=ORIENTED_EDGE('',*,*,#52782,.F.);
#74302=ORIENTED_EDGE('',*,*,#52783,.F.);
#74303=ORIENTED_EDGE('',*,*,#52784,.F.);
#74304=ORIENTED_EDGE('',*,*,#52106,.T.);
#74305=ORIENTED_EDGE('',*,*,#52785,.F.);
#74306=ORIENTED_EDGE('',*,*,#52786,.F.);
#74307=ORIENTED_EDGE('',*,*,#52787,.F.);
#74308=ORIENTED_EDGE('',*,*,#51875,.T.);
#74309=ORIENTED_EDGE('',*,*,#52788,.F.);
#74310=ORIENTED_EDGE('',*,*,#52789,.F.);
#74311=ORIENTED_EDGE('',*,*,#52790,.F.);
#74312=ORIENTED_EDGE('',*,*,#51862,.T.);
#74313=ORIENTED_EDGE('',*,*,#52791,.F.);
#74314=ORIENTED_EDGE('',*,*,#52792,.F.);
#74315=ORIENTED_EDGE('',*,*,#52793,.F.);
#74316=ORIENTED_EDGE('',*,*,#51873,.T.);
#74317=ORIENTED_EDGE('',*,*,#52794,.F.);
#74318=ORIENTED_EDGE('',*,*,#52795,.F.);
#74319=ORIENTED_EDGE('',*,*,#52796,.F.);
#74320=ORIENTED_EDGE('',*,*,#51883,.T.);
#74321=ORIENTED_EDGE('',*,*,#52797,.F.);
#74322=ORIENTED_EDGE('',*,*,#52798,.F.);
#74323=ORIENTED_EDGE('',*,*,#52799,.F.);
#74324=ORIENTED_EDGE('',*,*,#51967,.T.);
#74325=ORIENTED_EDGE('',*,*,#52800,.F.);
#74326=ORIENTED_EDGE('',*,*,#52801,.F.);
#74327=ORIENTED_EDGE('',*,*,#52802,.F.);
#74328=ORIENTED_EDGE('',*,*,#51959,.T.);
#74329=ORIENTED_EDGE('',*,*,#52803,.F.);
#74330=ORIENTED_EDGE('',*,*,#52804,.F.);
#74331=ORIENTED_EDGE('',*,*,#52805,.F.);
#74332=ORIENTED_EDGE('',*,*,#51946,.T.);
#74333=ORIENTED_EDGE('',*,*,#52806,.F.);
#74334=ORIENTED_EDGE('',*,*,#52807,.F.);
#74335=ORIENTED_EDGE('',*,*,#52808,.F.);
#74336=ORIENTED_EDGE('',*,*,#51957,.T.);
#74337=ORIENTED_EDGE('',*,*,#52809,.F.);
#74338=ORIENTED_EDGE('',*,*,#52810,.F.);
#74339=ORIENTED_EDGE('',*,*,#52811,.F.);
#74340=ORIENTED_EDGE('',*,*,#51994,.T.);
#74341=ORIENTED_EDGE('',*,*,#52812,.F.);
#74342=ORIENTED_EDGE('',*,*,#52813,.F.);
#74343=ORIENTED_EDGE('',*,*,#52814,.F.);
#74344=ORIENTED_EDGE('',*,*,#52005,.T.);
#74345=ORIENTED_EDGE('',*,*,#52815,.F.);
#74346=ORIENTED_EDGE('',*,*,#52816,.F.);
#74347=ORIENTED_EDGE('',*,*,#52817,.F.);
#74348=ORIENTED_EDGE('',*,*,#52015,.T.);
#74349=ORIENTED_EDGE('',*,*,#52818,.F.);
#74350=ORIENTED_EDGE('',*,*,#52819,.F.);
#74351=ORIENTED_EDGE('',*,*,#52820,.F.);
#74352=ORIENTED_EDGE('',*,*,#52007,.T.);
#74353=ORIENTED_EDGE('',*,*,#52821,.F.);
#74354=ORIENTED_EDGE('',*,*,#52822,.F.);
#74355=ORIENTED_EDGE('',*,*,#52823,.F.);
#74356=ORIENTED_EDGE('',*,*,#52284,.T.);
#74357=ORIENTED_EDGE('',*,*,#52824,.F.);
#74358=ORIENTED_EDGE('',*,*,#52825,.F.);
#74359=ORIENTED_EDGE('',*,*,#52826,.F.);
#74360=ORIENTED_EDGE('',*,*,#52286,.T.);
#74361=ORIENTED_EDGE('',*,*,#52827,.F.);
#74362=ORIENTED_EDGE('',*,*,#52828,.F.);
#74363=ORIENTED_EDGE('',*,*,#52829,.F.);
#74364=ORIENTED_EDGE('',*,*,#52273,.T.);
#74365=ORIENTED_EDGE('',*,*,#52830,.F.);
#74366=ORIENTED_EDGE('',*,*,#52831,.F.);
#74367=ORIENTED_EDGE('',*,*,#52832,.F.);
#74368=ORIENTED_EDGE('',*,*,#52134,.T.);
#74369=ORIENTED_EDGE('',*,*,#52833,.F.);
#74370=ORIENTED_EDGE('',*,*,#52834,.F.);
#74371=ORIENTED_EDGE('',*,*,#52835,.F.);
#74372=ORIENTED_EDGE('',*,*,#52144,.T.);
#74373=ORIENTED_EDGE('',*,*,#52836,.F.);
#74374=ORIENTED_EDGE('',*,*,#52837,.F.);
#74375=ORIENTED_EDGE('',*,*,#52838,.F.);
#74376=ORIENTED_EDGE('',*,*,#52136,.T.);
#74377=ORIENTED_EDGE('',*,*,#52839,.F.);
#74378=ORIENTED_EDGE('',*,*,#52840,.F.);
#74379=ORIENTED_EDGE('',*,*,#52841,.F.);
#74380=ORIENTED_EDGE('',*,*,#52123,.T.);
#74381=ORIENTED_EDGE('',*,*,#52842,.F.);
#74382=ORIENTED_EDGE('',*,*,#52843,.F.);
#74383=ORIENTED_EDGE('',*,*,#52844,.F.);
#74384=ORIENTED_EDGE('',*,*,#52082,.T.);
#74385=ORIENTED_EDGE('',*,*,#52845,.F.);
#74386=ORIENTED_EDGE('',*,*,#52846,.F.);
#74387=ORIENTED_EDGE('',*,*,#52847,.F.);
#74388=ORIENTED_EDGE('',*,*,#52069,.T.);
#74389=ORIENTED_EDGE('',*,*,#52848,.F.);
#74390=ORIENTED_EDGE('',*,*,#52849,.F.);
#74391=ORIENTED_EDGE('',*,*,#52850,.F.);
#74392=ORIENTED_EDGE('',*,*,#52080,.T.);
#74393=ORIENTED_EDGE('',*,*,#52851,.F.);
#74394=ORIENTED_EDGE('',*,*,#52852,.F.);
#74395=ORIENTED_EDGE('',*,*,#52853,.F.);
#74396=ORIENTED_EDGE('',*,*,#52090,.T.);
#74397=ORIENTED_EDGE('',*,*,#52854,.F.);
#74398=ORIENTED_EDGE('',*,*,#52855,.F.);
#74399=ORIENTED_EDGE('',*,*,#52856,.F.);
#74400=ORIENTED_EDGE('',*,*,#51983,.T.);
#74401=ORIENTED_EDGE('',*,*,#52857,.F.);
#74402=ORIENTED_EDGE('',*,*,#52858,.F.);
#74403=ORIENTED_EDGE('',*,*,#52859,.F.);
#74404=ORIENTED_EDGE('',*,*,#51970,.T.);
#74405=ORIENTED_EDGE('',*,*,#52860,.F.);
#74406=ORIENTED_EDGE('',*,*,#52861,.F.);
#74407=ORIENTED_EDGE('',*,*,#52862,.F.);
#74408=ORIENTED_EDGE('',*,*,#51981,.T.);
#74409=ORIENTED_EDGE('',*,*,#52863,.F.);
#74410=ORIENTED_EDGE('',*,*,#52864,.F.);
#74411=ORIENTED_EDGE('',*,*,#52865,.F.);
#74412=ORIENTED_EDGE('',*,*,#51991,.T.);
#74413=ORIENTED_EDGE('',*,*,#52866,.F.);
#74414=ORIENTED_EDGE('',*,*,#52867,.F.);
#74415=ORIENTED_EDGE('',*,*,#52868,.F.);
#74416=ORIENTED_EDGE('',*,*,#51838,.T.);
#74417=ORIENTED_EDGE('',*,*,#52869,.F.);
#74418=ORIENTED_EDGE('',*,*,#52870,.F.);
#74419=ORIENTED_EDGE('',*,*,#52871,.F.);
#74420=ORIENTED_EDGE('',*,*,#51849,.T.);
#74421=ORIENTED_EDGE('',*,*,#52872,.F.);
#74422=ORIENTED_EDGE('',*,*,#52873,.F.);
#74423=ORIENTED_EDGE('',*,*,#52874,.F.);
#74424=ORIENTED_EDGE('',*,*,#51859,.T.);
#74425=ORIENTED_EDGE('',*,*,#52875,.F.);
#74426=ORIENTED_EDGE('',*,*,#52876,.F.);
#74427=ORIENTED_EDGE('',*,*,#52877,.F.);
#74428=ORIENTED_EDGE('',*,*,#51851,.T.);
#74429=ORIENTED_EDGE('',*,*,#52878,.F.);
#74430=ORIENTED_EDGE('',*,*,#52879,.F.);
#74431=ORIENTED_EDGE('',*,*,#52880,.F.);
#74432=ORIENTED_EDGE('',*,*,#51784,.T.);
#74433=ORIENTED_EDGE('',*,*,#52881,.F.);
#74434=ORIENTED_EDGE('',*,*,#52882,.F.);
#74435=ORIENTED_EDGE('',*,*,#52883,.F.);
#74436=ORIENTED_EDGE('',*,*,#51795,.T.);
#74437=ORIENTED_EDGE('',*,*,#52884,.F.);
#74438=ORIENTED_EDGE('',*,*,#52885,.F.);
#74439=ORIENTED_EDGE('',*,*,#52886,.F.);
#74440=ORIENTED_EDGE('',*,*,#51805,.T.);
#74441=ORIENTED_EDGE('',*,*,#52887,.F.);
#74442=ORIENTED_EDGE('',*,*,#52888,.F.);
#74443=ORIENTED_EDGE('',*,*,#52889,.F.);
#74444=ORIENTED_EDGE('',*,*,#51797,.T.);
#74445=ORIENTED_EDGE('',*,*,#52890,.F.);
#74446=ORIENTED_EDGE('',*,*,#52891,.F.);
#74447=ORIENTED_EDGE('',*,*,#52892,.F.);
#74448=ORIENTED_EDGE('',*,*,#51808,.T.);
#74449=ORIENTED_EDGE('',*,*,#52893,.F.);
#74450=ORIENTED_EDGE('',*,*,#52894,.F.);
#74451=ORIENTED_EDGE('',*,*,#52895,.F.);
#74452=ORIENTED_EDGE('',*,*,#51819,.T.);
#74453=ORIENTED_EDGE('',*,*,#52896,.F.);
#74454=ORIENTED_EDGE('',*,*,#52897,.F.);
#74455=ORIENTED_EDGE('',*,*,#52898,.F.);
#74456=ORIENTED_EDGE('',*,*,#51831,.T.);
#74457=ORIENTED_EDGE('',*,*,#52899,.F.);
#74458=ORIENTED_EDGE('',*,*,#52900,.F.);
#74459=ORIENTED_EDGE('',*,*,#52901,.F.);
#74460=ORIENTED_EDGE('',*,*,#51821,.T.);
#74461=ORIENTED_EDGE('',*,*,#52902,.F.);
#74462=ORIENTED_EDGE('',*,*,#52903,.F.);
#74463=ORIENTED_EDGE('',*,*,#52904,.F.);
#74464=ORIENTED_EDGE('',*,*,#51582,.T.);
#74465=ORIENTED_EDGE('',*,*,#52905,.F.);
#74466=ORIENTED_EDGE('',*,*,#52906,.F.);
#74467=ORIENTED_EDGE('',*,*,#52907,.F.);
#74468=ORIENTED_EDGE('',*,*,#51584,.T.);
#74469=ORIENTED_EDGE('',*,*,#52908,.F.);
#74470=ORIENTED_EDGE('',*,*,#52909,.F.);
#74471=ORIENTED_EDGE('',*,*,#52910,.F.);
#74472=ORIENTED_EDGE('',*,*,#52911,.F.);
#74473=ORIENTED_EDGE('',*,*,#51560,.T.);
#74474=ORIENTED_EDGE('',*,*,#52912,.F.);
#74475=ORIENTED_EDGE('',*,*,#52913,.F.);
#74476=ORIENTED_EDGE('',*,*,#51570,.T.);
#74477=ORIENTED_EDGE('',*,*,#52914,.F.);
#74478=ORIENTED_EDGE('',*,*,#52915,.F.);
#74479=ORIENTED_EDGE('',*,*,#52916,.F.);
#74480=ORIENTED_EDGE('',*,*,#52190,.T.);
#74481=ORIENTED_EDGE('',*,*,#52917,.F.);
#74482=ORIENTED_EDGE('',*,*,#52918,.F.);
#74483=ORIENTED_EDGE('',*,*,#52919,.F.);
#74484=ORIENTED_EDGE('',*,*,#52177,.T.);
#74485=ORIENTED_EDGE('',*,*,#52920,.F.);
#74486=ORIENTED_EDGE('',*,*,#52921,.F.);
#74487=ORIENTED_EDGE('',*,*,#52922,.F.);
#74488=ORIENTED_EDGE('',*,*,#52188,.T.);
#74489=ORIENTED_EDGE('',*,*,#52923,.F.);
#74490=ORIENTED_EDGE('',*,*,#52924,.F.);
#74491=ORIENTED_EDGE('',*,*,#52925,.F.);
#74492=ORIENTED_EDGE('',*,*,#52198,.T.);
#74493=ORIENTED_EDGE('',*,*,#52926,.F.);
#74494=ORIENTED_EDGE('',*,*,#52927,.F.);
#74495=ORIENTED_EDGE('',*,*,#52928,.F.);
#74496=ORIENTED_EDGE('',*,*,#51725,.T.);
#74497=ORIENTED_EDGE('',*,*,#52929,.F.);
#74498=ORIENTED_EDGE('',*,*,#52930,.F.);
#74499=ORIENTED_EDGE('',*,*,#52931,.F.);
#74500=ORIENTED_EDGE('',*,*,#51712,.T.);
#74501=ORIENTED_EDGE('',*,*,#52932,.F.);
#74502=ORIENTED_EDGE('',*,*,#52933,.F.);
#74503=ORIENTED_EDGE('',*,*,#52934,.F.);
#74504=ORIENTED_EDGE('',*,*,#51723,.T.);
#74505=ORIENTED_EDGE('',*,*,#52935,.F.);
#74506=ORIENTED_EDGE('',*,*,#52936,.F.);
#74507=ORIENTED_EDGE('',*,*,#52937,.F.);
#74508=ORIENTED_EDGE('',*,*,#51733,.T.);
#74509=ORIENTED_EDGE('',*,*,#52938,.F.);
#74510=ORIENTED_EDGE('',*,*,#52939,.F.);
#74511=ORIENTED_EDGE('',*,*,#52940,.F.);
#74512=ORIENTED_EDGE('',*,*,#51701,.T.);
#74513=ORIENTED_EDGE('',*,*,#52941,.F.);
#74514=ORIENTED_EDGE('',*,*,#52942,.F.);
#74515=ORIENTED_EDGE('',*,*,#52943,.F.);
#74516=ORIENTED_EDGE('',*,*,#51688,.T.);
#74517=ORIENTED_EDGE('',*,*,#52944,.F.);
#74518=ORIENTED_EDGE('',*,*,#52945,.F.);
#74519=ORIENTED_EDGE('',*,*,#52946,.F.);
#74520=ORIENTED_EDGE('',*,*,#51699,.T.);
#74521=ORIENTED_EDGE('',*,*,#52947,.F.);
#74522=ORIENTED_EDGE('',*,*,#52948,.F.);
#74523=ORIENTED_EDGE('',*,*,#52949,.F.);
#74524=ORIENTED_EDGE('',*,*,#51709,.T.);
#74525=ORIENTED_EDGE('',*,*,#52950,.F.);
#74526=ORIENTED_EDGE('',*,*,#52951,.F.);
#74527=ORIENTED_EDGE('',*,*,#52952,.F.);
#74528=ORIENTED_EDGE('',*,*,#52018,.T.);
#74529=ORIENTED_EDGE('',*,*,#52953,.F.);
#74530=ORIENTED_EDGE('',*,*,#52954,.F.);
#74531=ORIENTED_EDGE('',*,*,#52955,.F.);
#74532=ORIENTED_EDGE('',*,*,#52029,.T.);
#74533=ORIENTED_EDGE('',*,*,#52956,.F.);
#74534=ORIENTED_EDGE('',*,*,#52957,.F.);
#74535=ORIENTED_EDGE('',*,*,#52958,.F.);
#74536=ORIENTED_EDGE('',*,*,#52039,.T.);
#74537=ORIENTED_EDGE('',*,*,#52959,.F.);
#74538=ORIENTED_EDGE('',*,*,#52960,.F.);
#74539=ORIENTED_EDGE('',*,*,#52961,.F.);
#74540=ORIENTED_EDGE('',*,*,#52031,.T.);
#74541=ORIENTED_EDGE('',*,*,#52962,.F.);
#74542=ORIENTED_EDGE('',*,*,#52963,.F.);
#74543=ORIENTED_EDGE('',*,*,#52964,.F.);
#74544=ORIENTED_EDGE('',*,*,#52212,.T.);
#74545=ORIENTED_EDGE('',*,*,#52965,.F.);
#74546=ORIENTED_EDGE('',*,*,#52966,.F.);
#74547=ORIENTED_EDGE('',*,*,#52967,.F.);
#74548=ORIENTED_EDGE('',*,*,#52222,.T.);
#74549=ORIENTED_EDGE('',*,*,#52968,.F.);
#74550=ORIENTED_EDGE('',*,*,#52969,.F.);
#74551=ORIENTED_EDGE('',*,*,#52970,.F.);
#74552=ORIENTED_EDGE('',*,*,#52214,.T.);
#74553=ORIENTED_EDGE('',*,*,#52971,.F.);
#74554=ORIENTED_EDGE('',*,*,#52972,.F.);
#74555=ORIENTED_EDGE('',*,*,#52973,.F.);
#74556=ORIENTED_EDGE('',*,*,#52201,.T.);
#74557=ORIENTED_EDGE('',*,*,#52974,.F.);
#74558=ORIENTED_EDGE('',*,*,#52975,.F.);
#74559=ORIENTED_EDGE('',*,*,#52976,.F.);
#74560=ORIENTED_EDGE('',*,*,#51610,.T.);
#74561=ORIENTED_EDGE('',*,*,#52977,.F.);
#74562=ORIENTED_EDGE('',*,*,#52978,.F.);
#74563=ORIENTED_EDGE('',*,*,#52979,.F.);
#74564=ORIENTED_EDGE('',*,*,#51602,.T.);
#74565=ORIENTED_EDGE('',*,*,#52980,.F.);
#74566=ORIENTED_EDGE('',*,*,#52981,.F.);
#74567=ORIENTED_EDGE('',*,*,#52982,.F.);
#74568=ORIENTED_EDGE('',*,*,#52983,.F.);
#74569=ORIENTED_EDGE('',*,*,#51590,.T.);
#74570=ORIENTED_EDGE('',*,*,#52984,.F.);
#74571=ORIENTED_EDGE('',*,*,#52985,.F.);
#74572=ORIENTED_EDGE('',*,*,#51600,.T.);
#74573=ORIENTED_EDGE('',*,*,#52986,.F.);
#74574=ORIENTED_EDGE('',*,*,#52987,.F.);
#74575=ORIENTED_EDGE('',*,*,#52988,.F.);
#74576=ORIENTED_EDGE('',*,*,#52238,.T.);
#74577=ORIENTED_EDGE('',*,*,#52989,.F.);
#74578=ORIENTED_EDGE('',*,*,#52990,.F.);
#74579=ORIENTED_EDGE('',*,*,#52991,.F.);
#74580=ORIENTED_EDGE('',*,*,#52225,.T.);
#74581=ORIENTED_EDGE('',*,*,#52992,.F.);
#74582=ORIENTED_EDGE('',*,*,#52993,.F.);
#74583=ORIENTED_EDGE('',*,*,#52994,.F.);
#74584=ORIENTED_EDGE('',*,*,#52236,.T.);
#74585=ORIENTED_EDGE('',*,*,#52995,.F.);
#74586=ORIENTED_EDGE('',*,*,#52996,.F.);
#74587=ORIENTED_EDGE('',*,*,#52997,.F.);
#74588=ORIENTED_EDGE('',*,*,#52246,.T.);
#74589=ORIENTED_EDGE('',*,*,#52998,.F.);
#74590=ORIENTED_EDGE('',*,*,#52999,.F.);
#74591=ORIENTED_EDGE('',*,*,#53000,.F.);
#74592=ORIENTED_EDGE('',*,*,#51650,.T.);
#74593=ORIENTED_EDGE('',*,*,#53001,.F.);
#74594=ORIENTED_EDGE('',*,*,#53002,.F.);
#74595=ORIENTED_EDGE('',*,*,#53003,.F.);
#74596=ORIENTED_EDGE('',*,*,#51637,.T.);
#74597=ORIENTED_EDGE('',*,*,#53004,.F.);
#74598=ORIENTED_EDGE('',*,*,#53005,.F.);
#74599=ORIENTED_EDGE('',*,*,#53006,.F.);
#74600=ORIENTED_EDGE('',*,*,#51648,.T.);
#74601=ORIENTED_EDGE('',*,*,#53007,.F.);
#74602=ORIENTED_EDGE('',*,*,#53008,.F.);
#74603=ORIENTED_EDGE('',*,*,#53009,.F.);
#74604=ORIENTED_EDGE('',*,*,#51658,.T.);
#74605=ORIENTED_EDGE('',*,*,#53010,.F.);
#74606=ORIENTED_EDGE('',*,*,#53011,.F.);
#74607=ORIENTED_EDGE('',*,*,#53012,.F.);
#74608=ORIENTED_EDGE('',*,*,#52260,.T.);
#74609=ORIENTED_EDGE('',*,*,#53013,.F.);
#74610=ORIENTED_EDGE('',*,*,#53014,.F.);
#74611=ORIENTED_EDGE('',*,*,#53015,.F.);
#74612=ORIENTED_EDGE('',*,*,#52270,.T.);
#74613=ORIENTED_EDGE('',*,*,#53016,.F.);
#74614=ORIENTED_EDGE('',*,*,#53017,.F.);
#74615=ORIENTED_EDGE('',*,*,#53018,.F.);
#74616=ORIENTED_EDGE('',*,*,#52262,.T.);
#74617=ORIENTED_EDGE('',*,*,#53019,.F.);
#74618=ORIENTED_EDGE('',*,*,#53020,.F.);
#74619=ORIENTED_EDGE('',*,*,#53021,.F.);
#74620=ORIENTED_EDGE('',*,*,#52249,.T.);
#74621=ORIENTED_EDGE('',*,*,#53022,.F.);
#74622=ORIENTED_EDGE('',*,*,#53023,.F.);
#74623=ORIENTED_EDGE('',*,*,#53024,.F.);
#74624=ORIENTED_EDGE('',*,*,#51634,.T.);
#74625=ORIENTED_EDGE('',*,*,#53025,.F.);
#74626=ORIENTED_EDGE('',*,*,#53026,.F.);
#74627=ORIENTED_EDGE('',*,*,#53027,.F.);
#74628=ORIENTED_EDGE('',*,*,#51626,.T.);
#74629=ORIENTED_EDGE('',*,*,#53028,.F.);
#74630=ORIENTED_EDGE('',*,*,#53029,.F.);
#74631=ORIENTED_EDGE('',*,*,#53030,.F.);
#74632=ORIENTED_EDGE('',*,*,#53031,.F.);
#74633=ORIENTED_EDGE('',*,*,#51614,.T.);
#74634=ORIENTED_EDGE('',*,*,#53032,.F.);
#74635=ORIENTED_EDGE('',*,*,#53033,.F.);
#74636=ORIENTED_EDGE('',*,*,#51624,.T.);
#74637=ORIENTED_EDGE('',*,*,#53034,.F.);
#74638=ORIENTED_EDGE('',*,*,#53035,.F.);
#74639=ORIENTED_EDGE('',*,*,#53036,.F.);
#74640=ORIENTED_EDGE('',*,*,#52402,.T.);
#74641=ORIENTED_EDGE('',*,*,#53037,.F.);
#74642=ORIENTED_EDGE('',*,*,#53038,.F.);
#74643=ORIENTED_EDGE('',*,*,#53039,.F.);
#74644=ORIENTED_EDGE('',*,*,#52440,.T.);
#74645=ORIENTED_EDGE('',*,*,#53040,.F.);
#74646=ORIENTED_EDGE('',*,*,#53041,.F.);
#74647=ORIENTED_EDGE('',*,*,#53042,.F.);
#74648=ORIENTED_EDGE('',*,*,#52424,.T.);
#74649=ORIENTED_EDGE('',*,*,#53043,.F.);
#74650=ORIENTED_EDGE('',*,*,#53044,.F.);
#74651=ORIENTED_EDGE('',*,*,#53045,.F.);
#74652=ORIENTED_EDGE('',*,*,#53046,.F.);
#74653=ORIENTED_EDGE('',*,*,#52419,.T.);
#74654=ORIENTED_EDGE('',*,*,#53047,.F.);
#74655=ORIENTED_EDGE('',*,*,#53048,.F.);
#74656=ORIENTED_EDGE('',*,*,#52446,.T.);
#74657=ORIENTED_EDGE('',*,*,#53049,.F.);
#74658=ORIENTED_EDGE('',*,*,#53050,.F.);
#74659=ORIENTED_EDGE('',*,*,#53051,.F.);
#74660=ORIENTED_EDGE('',*,*,#53052,.F.);
#74661=ORIENTED_EDGE('',*,*,#52435,.T.);
#74662=ORIENTED_EDGE('',*,*,#53053,.F.);
#74663=ORIENTED_EDGE('',*,*,#53054,.F.);
#74664=ORIENTED_EDGE('',*,*,#52408,.T.);
#74665=ORIENTED_EDGE('',*,*,#53055,.F.);
#74666=ORIENTED_EDGE('',*,*,#53056,.F.);
#74667=ORIENTED_EDGE('',*,*,#53057,.F.);
#74668=ORIENTED_EDGE('',*,*,#51899,.T.);
#74669=ORIENTED_EDGE('',*,*,#53058,.F.);
#74670=ORIENTED_EDGE('',*,*,#53059,.F.);
#74671=ORIENTED_EDGE('',*,*,#53060,.F.);
#74672=ORIENTED_EDGE('',*,*,#51929,.T.);
#74673=ORIENTED_EDGE('',*,*,#53061,.F.);
#74674=ORIENTED_EDGE('',*,*,#53062,.F.);
#74675=ORIENTED_EDGE('',*,*,#53063,.F.);
#74676=ORIENTED_EDGE('',*,*,#52067,.T.);
#74677=ORIENTED_EDGE('',*,*,#52683,.T.);
#74678=ORIENTED_EDGE('',*,*,#53064,.F.);
#74679=ORIENTED_EDGE('',*,*,#52710,.T.);
#74680=ORIENTED_EDGE('',*,*,#51684,.T.);
#74681=ORIENTED_EDGE('',*,*,#53065,.F.);
#74682=ORIENTED_EDGE('',*,*,#53066,.F.);
#74683=ORIENTED_EDGE('',*,*,#53067,.T.);
#74684=ORIENTED_EDGE('',*,*,#53067,.F.);
#74685=ORIENTED_EDGE('',*,*,#53068,.T.);
#74686=ORIENTED_EDGE('',*,*,#52311,.T.);
#74687=ORIENTED_EDGE('',*,*,#53068,.F.);
#74688=ORIENTED_EDGE('',*,*,#52308,.T.);
#74689=ORIENTED_EDGE('',*,*,#52313,.T.);
#74690=ORIENTED_EDGE('',*,*,#52722,.T.);
#74691=ORIENTED_EDGE('',*,*,#52061,.T.);
#74692=ORIENTED_EDGE('',*,*,#53063,.T.);
#74693=ORIENTED_EDGE('',*,*,#53069,.F.);
#74694=ORIENTED_EDGE('',*,*,#53065,.T.);
#74695=ORIENTED_EDGE('',*,*,#51678,.T.);
#74696=ORIENTED_EDGE('',*,*,#52718,.T.);
#74697=ORIENTED_EDGE('',*,*,#53070,.F.);
#74698=ORIENTED_EDGE('',*,*,#52310,.T.);
#74699=ORIENTED_EDGE('',*,*,#53071,.T.);
#74700=ORIENTED_EDGE('',*,*,#53072,.T.);
#74701=ORIENTED_EDGE('',*,*,#50262,.F.);
#74702=ORIENTED_EDGE('',*,*,#50453,.F.);
#74703=ORIENTED_EDGE('',*,*,#53073,.T.);
#74704=ORIENTED_EDGE('',*,*,#50846,.F.);
#74705=ORIENTED_EDGE('',*,*,#50243,.F.);
#74706=ORIENTED_EDGE('',*,*,#53074,.F.);
#74707=ORIENTED_EDGE('',*,*,#50218,.F.);
#74708=ORIENTED_EDGE('',*,*,#50849,.F.);
#74709=ORIENTED_EDGE('',*,*,#53075,.T.);
#74710=ORIENTED_EDGE('',*,*,#50457,.F.);
#74711=ORIENTED_EDGE('',*,*,#50201,.F.);
#74712=ORIENTED_EDGE('',*,*,#53076,.F.);
#74713=ORIENTED_EDGE('',*,*,#50196,.F.);
#74714=ORIENTED_EDGE('',*,*,#50462,.F.);
#74715=ORIENTED_EDGE('',*,*,#53077,.T.);
#74716=ORIENTED_EDGE('',*,*,#50466,.F.);
#74717=ORIENTED_EDGE('',*,*,#50179,.F.);
#74718=ORIENTED_EDGE('',*,*,#53078,.F.);
#74719=ORIENTED_EDGE('',*,*,#50240,.F.);
#74720=ORIENTED_EDGE('',*,*,#50471,.F.);
#74721=ORIENTED_EDGE('',*,*,#53079,.T.);
#74722=ORIENTED_EDGE('',*,*,#50472,.F.);
#74723=ORIENTED_EDGE('',*,*,#50223,.F.);
#74724=ORIENTED_EDGE('',*,*,#53080,.T.);
#74725=ORIENTED_EDGE('',*,*,#52412,.T.);
#74726=ORIENTED_EDGE('',*,*,#52679,.T.);
#74727=ORIENTED_EDGE('',*,*,#53081,.F.);
#74728=ORIENTED_EDGE('',*,*,#52677,.T.);
#74729=ORIENTED_EDGE('',*,*,#52429,.T.);
#74730=ORIENTED_EDGE('',*,*,#53082,.T.);
#74731=ORIENTED_EDGE('',*,*,#52368,.T.);
#74732=ORIENTED_EDGE('',*,*,#52673,.T.);
#74733=ORIENTED_EDGE('',*,*,#53083,.F.);
#74734=ORIENTED_EDGE('',*,*,#52668,.T.);
#74735=ORIENTED_EDGE('',*,*,#52385,.T.);
#74736=ORIENTED_EDGE('',*,*,#53084,.T.);
#74737=ORIENTED_EDGE('',*,*,#52390,.T.);
#74738=ORIENTED_EDGE('',*,*,#52664,.T.);
#74739=ORIENTED_EDGE('',*,*,#53085,.F.);
#74740=ORIENTED_EDGE('',*,*,#53055,.T.);
#74741=ORIENTED_EDGE('',*,*,#52407,.T.);
#74742=ORIENTED_EDGE('',*,*,#53086,.T.);
#74743=ORIENTED_EDGE('',*,*,#52432,.T.);
#74744=ORIENTED_EDGE('',*,*,#53052,.T.);
#74745=ORIENTED_EDGE('',*,*,#53087,.F.);
#74746=ORIENTED_EDGE('',*,*,#52659,.T.);
#74747=ORIENTED_EDGE('',*,*,#52451,.T.);
#74748=ORIENTED_EDGE('',*,*,#53088,.T.);
#74749=ORIENTED_EDGE('',*,*,#53071,.F.);
#74750=ORIENTED_EDGE('',*,*,#53040,.T.);
#74751=ORIENTED_EDGE('',*,*,#52443,.T.);
#74752=ORIENTED_EDGE('',*,*,#53048,.T.);
#74753=ORIENTED_EDGE('',*,*,#53089,.T.);
#74754=ORIENTED_EDGE('',*,*,#53053,.T.);
#74755=ORIENTED_EDGE('',*,*,#52437,.T.);
#74756=ORIENTED_EDGE('',*,*,#53039,.T.);
#74757=ORIENTED_EDGE('',*,*,#53090,.T.);
#74758=ORIENTED_EDGE('',*,*,#53037,.T.);
#74759=ORIENTED_EDGE('',*,*,#52405,.T.);
#74760=ORIENTED_EDGE('',*,*,#53054,.T.);
#74761=ORIENTED_EDGE('',*,*,#53091,.T.);
#74762=ORIENTED_EDGE('',*,*,#52662,.T.);
#74763=ORIENTED_EDGE('',*,*,#52399,.T.);
#74764=ORIENTED_EDGE('',*,*,#53036,.T.);
#74765=ORIENTED_EDGE('',*,*,#53092,.T.);
#74766=ORIENTED_EDGE('',*,*,#53061,.T.);
#74767=ORIENTED_EDGE('',*,*,#51935,.T.);
#74768=ORIENTED_EDGE('',*,*,#52685,.T.);
#74769=ORIENTED_EDGE('',*,*,#53093,.F.);
#74770=ORIENTED_EDGE('',*,*,#53047,.T.);
#74771=ORIENTED_EDGE('',*,*,#52421,.T.);
#74772=ORIENTED_EDGE('',*,*,#53042,.T.);
#74773=ORIENTED_EDGE('',*,*,#53094,.T.);
#74774=ORIENTED_EDGE('',*,*,#53043,.T.);
#74775=ORIENTED_EDGE('',*,*,#52427,.T.);
#74776=ORIENTED_EDGE('',*,*,#52676,.T.);
#74777=ORIENTED_EDGE('',*,*,#53095,.F.);
#74778=ORIENTED_EDGE('',*,*,#52674,.T.);
#74779=ORIENTED_EDGE('',*,*,#52371,.T.);
#74780=ORIENTED_EDGE('',*,*,#52656,.T.);
#74781=ORIENTED_EDGE('',*,*,#53096,.F.);
#74782=ORIENTED_EDGE('',*,*,#52657,.T.);
#74783=ORIENTED_EDGE('',*,*,#52377,.T.);
#74784=ORIENTED_EDGE('',*,*,#52670,.T.);
#74785=ORIENTED_EDGE('',*,*,#53097,.T.);
#74786=ORIENTED_EDGE('',*,*,#52698,.T.);
#74787=ORIENTED_EDGE('',*,*,#51893,.T.);
#74788=ORIENTED_EDGE('',*,*,#53057,.T.);
#74789=ORIENTED_EDGE('',*,*,#53098,.F.);
#74790=ORIENTED_EDGE('',*,*,#52740,.T.);
#74791=ORIENTED_EDGE('',*,*,#51755,.T.);
#74792=ORIENTED_EDGE('',*,*,#52748,.T.);
#74793=ORIENTED_EDGE('',*,*,#53099,.T.);
#74794=ORIENTED_EDGE('',*,*,#52896,.T.);
#74795=ORIENTED_EDGE('',*,*,#51813,.T.);
#74796=ORIENTED_EDGE('',*,*,#52892,.T.);
#74797=ORIENTED_EDGE('',*,*,#53100,.T.);
#74798=ORIENTED_EDGE('',*,*,#52884,.T.);
#74799=ORIENTED_EDGE('',*,*,#51789,.T.);
#74800=ORIENTED_EDGE('',*,*,#52880,.T.);
#74801=ORIENTED_EDGE('',*,*,#53101,.T.);
#74802=ORIENTED_EDGE('',*,*,#52752,.T.);
#74803=ORIENTED_EDGE('',*,*,#51779,.T.);
#74804=ORIENTED_EDGE('',*,*,#52760,.T.);
#74805=ORIENTED_EDGE('',*,*,#53102,.T.);
#74806=ORIENTED_EDGE('',*,*,#52872,.T.);
#74807=ORIENTED_EDGE('',*,*,#51843,.T.);
#74808=ORIENTED_EDGE('',*,*,#52868,.T.);
#74809=ORIENTED_EDGE('',*,*,#53103,.T.);
#74810=ORIENTED_EDGE('',*,*,#52788,.T.);
#74811=ORIENTED_EDGE('',*,*,#51881,.T.);
#74812=ORIENTED_EDGE('',*,*,#52796,.T.);
#74813=ORIENTED_EDGE('',*,*,#53104,.T.);
#74814=ORIENTED_EDGE('',*,*,#52860,.T.);
#74815=ORIENTED_EDGE('',*,*,#51977,.T.);
#74816=ORIENTED_EDGE('',*,*,#52856,.T.);
#74817=ORIENTED_EDGE('',*,*,#53105,.T.);
#74818=ORIENTED_EDGE('',*,*,#52800,.T.);
#74819=ORIENTED_EDGE('',*,*,#51963,.T.);
#74820=ORIENTED_EDGE('',*,*,#52808,.T.);
#74821=ORIENTED_EDGE('',*,*,#53106,.T.);
#74822=ORIENTED_EDGE('',*,*,#52776,.T.);
#74823=ORIENTED_EDGE('',*,*,#52100,.T.);
#74824=ORIENTED_EDGE('',*,*,#52784,.T.);
#74825=ORIENTED_EDGE('',*,*,#53107,.T.);
#74826=ORIENTED_EDGE('',*,*,#52836,.T.);
#74827=ORIENTED_EDGE('',*,*,#52140,.T.);
#74828=ORIENTED_EDGE('',*,*,#52832,.T.);
#74829=ORIENTED_EDGE('',*,*,#53108,.T.);
#74830=ORIENTED_EDGE('',*,*,#52848,.T.);
#74831=ORIENTED_EDGE('',*,*,#52076,.T.);
#74832=ORIENTED_EDGE('',*,*,#52844,.T.);
#74833=ORIENTED_EDGE('',*,*,#53109,.T.);
#74834=ORIENTED_EDGE('',*,*,#52812,.T.);
#74835=ORIENTED_EDGE('',*,*,#52001,.T.);
#74836=ORIENTED_EDGE('',*,*,#52820,.T.);
#74837=ORIENTED_EDGE('',*,*,#53110,.T.);
#74838=ORIENTED_EDGE('',*,*,#52827,.T.);
#74839=ORIENTED_EDGE('',*,*,#52288,.T.);
#74840=ORIENTED_EDGE('',*,*,#52823,.T.);
#74841=ORIENTED_EDGE('',*,*,#53111,.T.);
#74842=ORIENTED_EDGE('',*,*,#52764,.T.);
#74843=ORIENTED_EDGE('',*,*,#52154,.T.);
#74844=ORIENTED_EDGE('',*,*,#52772,.T.);
#74845=ORIENTED_EDGE('',*,*,#53112,.T.);
#74846=ORIENTED_EDGE('',*,*,#52731,.T.);
#74847=ORIENTED_EDGE('',*,*,#52296,.T.);
#74848=ORIENTED_EDGE('',*,*,#52737,.T.);
#74849=ORIENTED_EDGE('',*,*,#53113,.T.);
#74850=ORIENTED_EDGE('',*,*,#52908,.T.);
#74851=ORIENTED_EDGE('',*,*,#51586,.T.);
#74852=ORIENTED_EDGE('',*,*,#52904,.T.);
#74853=ORIENTED_EDGE('',*,*,#53114,.T.);
#74854=ORIENTED_EDGE('',*,*,#52980,.T.);
#74855=ORIENTED_EDGE('',*,*,#51608,.T.);
#74856=ORIENTED_EDGE('',*,*,#52976,.T.);
#74857=ORIENTED_EDGE('',*,*,#53115,.T.);
#74858=ORIENTED_EDGE('',*,*,#52914,.T.);
#74859=ORIENTED_EDGE('',*,*,#51564,.T.);
#74860=ORIENTED_EDGE('',*,*,#52911,.T.);
#74861=ORIENTED_EDGE('',*,*,#53116,.T.);
#74862=ORIENTED_EDGE('',*,*,#52746,.T.);
#74863=ORIENTED_EDGE('',*,*,#51741,.T.);
#74864=ORIENTED_EDGE('',*,*,#52742,.T.);
#74865=ORIENTED_EDGE('',*,*,#53117,.T.);
#74866=ORIENTED_EDGE('',*,*,#52929,.T.);
#74867=ORIENTED_EDGE('',*,*,#51731,.T.);
#74868=ORIENTED_EDGE('',*,*,#52937,.T.);
#74869=ORIENTED_EDGE('',*,*,#53118,.T.);
#74870=ORIENTED_EDGE('',*,*,#52770,.T.);
#74871=ORIENTED_EDGE('',*,*,#52164,.T.);
#74872=ORIENTED_EDGE('',*,*,#52766,.T.);
#74873=ORIENTED_EDGE('',*,*,#53119,.T.);
#74874=ORIENTED_EDGE('',*,*,#52920,.T.);
#74875=ORIENTED_EDGE('',*,*,#52184,.T.);
#74876=ORIENTED_EDGE('',*,*,#52916,.T.);
#74877=ORIENTED_EDGE('',*,*,#53120,.T.);
#74878=ORIENTED_EDGE('',*,*,#52758,.T.);
#74879=ORIENTED_EDGE('',*,*,#51765,.T.);
#74880=ORIENTED_EDGE('',*,*,#52754,.T.);
#74881=ORIENTED_EDGE('',*,*,#53121,.T.);
#74882=ORIENTED_EDGE('',*,*,#52941,.T.);
#74883=ORIENTED_EDGE('',*,*,#51707,.T.);
#74884=ORIENTED_EDGE('',*,*,#52949,.T.);
#74885=ORIENTED_EDGE('',*,*,#53122,.T.);
#74886=ORIENTED_EDGE('',*,*,#52794,.T.);
#74887=ORIENTED_EDGE('',*,*,#51867,.T.);
#74888=ORIENTED_EDGE('',*,*,#52790,.T.);
#74889=ORIENTED_EDGE('',*,*,#53123,.T.);
#74890=ORIENTED_EDGE('',*,*,#52704,.T.);
#74891=ORIENTED_EDGE('',*,*,#51903,.T.);
#74892=ORIENTED_EDGE('',*,*,#52700,.T.);
#74893=ORIENTED_EDGE('',*,*,#53124,.T.);
#74894=ORIENTED_EDGE('',*,*,#52806,.T.);
#74895=ORIENTED_EDGE('',*,*,#51953,.T.);
#74896=ORIENTED_EDGE('',*,*,#52802,.T.);
#74897=ORIENTED_EDGE('',*,*,#53125,.T.);
#74898=ORIENTED_EDGE('',*,*,#52695,.T.);
#74899=ORIENTED_EDGE('',*,*,#51933,.T.);
#74900=ORIENTED_EDGE('',*,*,#52691,.T.);
#74901=ORIENTED_EDGE('',*,*,#53126,.T.);
#74902=ORIENTED_EDGE('',*,*,#52842,.T.);
#74903=ORIENTED_EDGE('',*,*,#52130,.T.);
#74904=ORIENTED_EDGE('',*,*,#52838,.T.);
#74905=ORIENTED_EDGE('',*,*,#53127,.T.);
#74906=ORIENTED_EDGE('',*,*,#52968,.T.);
#74907=ORIENTED_EDGE('',*,*,#52218,.T.);
#74908=ORIENTED_EDGE('',*,*,#52964,.T.);
#74909=ORIENTED_EDGE('',*,*,#53128,.T.);
#74910=ORIENTED_EDGE('',*,*,#52818,.T.);
#74911=ORIENTED_EDGE('',*,*,#52011,.T.);
#74912=ORIENTED_EDGE('',*,*,#52814,.T.);
#74913=ORIENTED_EDGE('',*,*,#53129,.T.);
#74914=ORIENTED_EDGE('',*,*,#52953,.T.);
#74915=ORIENTED_EDGE('',*,*,#52025,.T.);
#74916=ORIENTED_EDGE('',*,*,#52961,.T.);
#74917=ORIENTED_EDGE('',*,*,#53130,.T.);
#74918=ORIENTED_EDGE('',*,*,#53131,.F.);
#74919=ORIENTED_EDGE('',*,*,#53132,.T.);
#74920=ORIENTED_EDGE('',*,*,#53133,.T.);
#74921=ORIENTED_EDGE('',*,*,#53134,.T.);
#74922=ORIENTED_EDGE('',*,*,#53135,.F.);
#74923=ORIENTED_EDGE('',*,*,#53136,.T.);
#74924=ORIENTED_EDGE('',*,*,#53131,.T.);
#74925=ORIENTED_EDGE('',*,*,#53137,.T.);
#74926=ORIENTED_EDGE('',*,*,#53133,.F.);
#74927=ORIENTED_EDGE('',*,*,#53138,.T.);
#74928=ORIENTED_EDGE('',*,*,#53139,.F.);
#74929=ORIENTED_EDGE('',*,*,#53140,.T.);
#74930=ORIENTED_EDGE('',*,*,#53028,.T.);
#74931=ORIENTED_EDGE('',*,*,#51632,.T.);
#74932=ORIENTED_EDGE('',*,*,#53024,.T.);
#74933=ORIENTED_EDGE('',*,*,#53141,.T.);
#74934=ORIENTED_EDGE('',*,*,#52986,.T.);
#74935=ORIENTED_EDGE('',*,*,#51594,.T.);
#74936=ORIENTED_EDGE('',*,*,#52983,.T.);
#74937=ORIENTED_EDGE('',*,*,#53142,.T.);
#74938=ORIENTED_EDGE('',*,*,#52935,.T.);
#74939=ORIENTED_EDGE('',*,*,#51717,.T.);
#74940=ORIENTED_EDGE('',*,*,#52931,.T.);
#74941=ORIENTED_EDGE('',*,*,#53143,.T.);
#74942=ORIENTED_EDGE('',*,*,#53001,.T.);
#74943=ORIENTED_EDGE('',*,*,#51656,.T.);
#74944=ORIENTED_EDGE('',*,*,#53009,.T.);
#74945=ORIENTED_EDGE('',*,*,#53144,.T.);
#74946=ORIENTED_EDGE('',*,*,#52926,.T.);
#74947=ORIENTED_EDGE('',*,*,#52194,.T.);
#74948=ORIENTED_EDGE('',*,*,#52922,.T.);
#74949=ORIENTED_EDGE('',*,*,#53145,.T.);
#74950=ORIENTED_EDGE('',*,*,#52992,.T.);
#74951=ORIENTED_EDGE('',*,*,#52232,.T.);
#74952=ORIENTED_EDGE('',*,*,#52988,.T.);
#74953=ORIENTED_EDGE('',*,*,#53146,.T.);
#74954=ORIENTED_EDGE('',*,*,#52947,.T.);
#74955=ORIENTED_EDGE('',*,*,#51693,.T.);
#74956=ORIENTED_EDGE('',*,*,#52943,.T.);
#74957=ORIENTED_EDGE('',*,*,#53147,.T.);
#74958=ORIENTED_EDGE('',*,*,#52713,.T.);
#74959=ORIENTED_EDGE('',*,*,#51680,.T.);
#74960=ORIENTED_EDGE('',*,*,#52709,.T.);
#74961=ORIENTED_EDGE('',*,*,#53148,.T.);
#74962=ORIENTED_EDGE('',*,*,#53058,.T.);
#74963=ORIENTED_EDGE('',*,*,#51905,.T.);
#74964=ORIENTED_EDGE('',*,*,#52706,.T.);
#74965=ORIENTED_EDGE('',*,*,#53149,.T.);
#74966=ORIENTED_EDGE('',*,*,#52689,.T.);
#74967=ORIENTED_EDGE('',*,*,#51923,.T.);
#74968=ORIENTED_EDGE('',*,*,#53060,.T.);
#74969=ORIENTED_EDGE('',*,*,#53150,.T.);
#74970=ORIENTED_EDGE('',*,*,#52974,.T.);
#74971=ORIENTED_EDGE('',*,*,#52208,.T.);
#74972=ORIENTED_EDGE('',*,*,#52970,.T.);
#74973=ORIENTED_EDGE('',*,*,#53151,.T.);
#74974=ORIENTED_EDGE('',*,*,#53016,.T.);
#74975=ORIENTED_EDGE('',*,*,#52266,.T.);
#74976=ORIENTED_EDGE('',*,*,#53012,.T.);
#74977=ORIENTED_EDGE('',*,*,#53152,.T.);
#74978=ORIENTED_EDGE('',*,*,#52959,.T.);
#74979=ORIENTED_EDGE('',*,*,#52035,.T.);
#74980=ORIENTED_EDGE('',*,*,#52955,.T.);
#74981=ORIENTED_EDGE('',*,*,#53153,.T.);
#74982=ORIENTED_EDGE('',*,*,#52684,.T.);
#74983=ORIENTED_EDGE('',*,*,#52059,.T.);
#74984=ORIENTED_EDGE('',*,*,#52727,.T.);
#74985=ORIENTED_EDGE('',*,*,#53154,.T.);
#74986=ORIENTED_EDGE('',*,*,#52719,.T.);
#74987=ORIENTED_EDGE('',*,*,#51666,.T.);
#74988=ORIENTED_EDGE('',*,*,#52715,.T.);
#74989=ORIENTED_EDGE('',*,*,#53155,.T.);
#74990=ORIENTED_EDGE('',*,*,#53022,.T.);
#74991=ORIENTED_EDGE('',*,*,#52256,.T.);
#74992=ORIENTED_EDGE('',*,*,#53018,.T.);
#74993=ORIENTED_EDGE('',*,*,#53156,.T.);
#74994=ORIENTED_EDGE('',*,*,#52725,.T.);
#74995=ORIENTED_EDGE('',*,*,#52049,.T.);
#74996=ORIENTED_EDGE('',*,*,#52721,.T.);
#74997=ORIENTED_EDGE('',*,*,#53157,.T.);
#74998=ORIENTED_EDGE('',*,*,#53049,.T.);
#74999=ORIENTED_EDGE('',*,*,#52449,.T.);
#75000=ORIENTED_EDGE('',*,*,#52658,.T.);
#75001=ORIENTED_EDGE('',*,*,#53158,.T.);
#75002=ORIENTED_EDGE('',*,*,#52680,.T.);
#75003=ORIENTED_EDGE('',*,*,#52415,.T.);
#75004=ORIENTED_EDGE('',*,*,#53046,.T.);
#75005=ORIENTED_EDGE('',*,*,#53159,.T.);
#75006=ORIENTED_EDGE('',*,*,#53007,.T.);
#75007=ORIENTED_EDGE('',*,*,#51642,.T.);
#75008=ORIENTED_EDGE('',*,*,#53003,.T.);
#75009=ORIENTED_EDGE('',*,*,#53160,.T.);
#75010=ORIENTED_EDGE('',*,*,#53034,.T.);
#75011=ORIENTED_EDGE('',*,*,#51618,.T.);
#75012=ORIENTED_EDGE('',*,*,#53031,.T.);
#75013=ORIENTED_EDGE('',*,*,#53161,.T.);
#75014=ORIENTED_EDGE('',*,*,#52998,.T.);
#75015=ORIENTED_EDGE('',*,*,#52242,.T.);
#75016=ORIENTED_EDGE('',*,*,#52994,.T.);
#75017=ORIENTED_EDGE('',*,*,#53162,.T.);
#75018=ORIENTED_EDGE('',*,*,#53163,.F.);
#75019=ORIENTED_EDGE('',*,*,#50911,.T.);
#75020=ORIENTED_EDGE('',*,*,#50905,.T.);
#75021=ORIENTED_EDGE('',*,*,#50909,.T.);
#75022=ORIENTED_EDGE('',*,*,#51248,.T.);
#75023=ORIENTED_EDGE('',*,*,#50939,.T.);
#75024=ORIENTED_EDGE('',*,*,#50942,.T.);
#75025=ORIENTED_EDGE('',*,*,#50945,.T.);
#75026=ORIENTED_EDGE('',*,*,#50948,.T.);
#75027=ORIENTED_EDGE('',*,*,#50951,.T.);
#75028=ORIENTED_EDGE('',*,*,#50954,.T.);
#75029=ORIENTED_EDGE('',*,*,#50957,.T.);
#75030=ORIENTED_EDGE('',*,*,#53164,.F.);
#75031=ORIENTED_EDGE('',*,*,#53165,.F.);
#75032=ORIENTED_EDGE('',*,*,#53166,.F.);
#75033=ORIENTED_EDGE('',*,*,#53167,.F.);
#75034=ORIENTED_EDGE('',*,*,#53168,.F.);
#75035=ORIENTED_EDGE('',*,*,#53169,.F.);
#75036=ORIENTED_EDGE('',*,*,#53170,.F.);
#75037=ORIENTED_EDGE('',*,*,#53171,.F.);
#75038=ORIENTED_EDGE('',*,*,#53172,.F.);
#75039=ORIENTED_EDGE('',*,*,#53137,.F.);
#75040=ORIENTED_EDGE('',*,*,#53134,.F.);
#75041=ORIENTED_EDGE('',*,*,#53140,.F.);
#75042=ORIENTED_EDGE('',*,*,#50893,.T.);
#75043=ORIENTED_EDGE('',*,*,#50713,.F.);
#75044=ORIENTED_EDGE('',*,*,#51258,.T.);
#75045=ORIENTED_EDGE('',*,*,#50716,.F.);
#75046=ORIENTED_EDGE('',*,*,#50918,.T.);
#75047=ORIENTED_EDGE('',*,*,#50719,.F.);
#75048=ORIENTED_EDGE('',*,*,#51265,.F.);
#75049=ORIENTED_EDGE('',*,*,#50710,.F.);
#75050=ORIENTED_EDGE('',*,*,#51261,.T.);
#75051=ORIENTED_EDGE('',*,*,#50725,.F.);
#75052=ORIENTED_EDGE('',*,*,#50916,.T.);
#75053=ORIENTED_EDGE('',*,*,#50728,.F.);
#75054=ORIENTED_EDGE('',*,*,#51260,.T.);
#75055=ORIENTED_EDGE('',*,*,#50731,.F.);
#75056=ORIENTED_EDGE('',*,*,#50891,.T.);
#75057=ORIENTED_EDGE('',*,*,#50722,.F.);
#75058=ORIENTED_EDGE('',*,*,#51259,.T.);
#75059=ORIENTED_EDGE('',*,*,#50737,.F.);
#75060=ORIENTED_EDGE('',*,*,#50920,.T.);
#75061=ORIENTED_EDGE('',*,*,#50740,.F.);
#75062=ORIENTED_EDGE('',*,*,#51255,.T.);
#75063=ORIENTED_EDGE('',*,*,#50743,.F.);
#75064=ORIENTED_EDGE('',*,*,#50895,.T.);
#75065=ORIENTED_EDGE('',*,*,#50734,.F.);
#75066=ORIENTED_EDGE('',*,*,#51252,.T.);
#75067=ORIENTED_EDGE('',*,*,#50749,.F.);
#75068=ORIENTED_EDGE('',*,*,#50926,.T.);
#75069=ORIENTED_EDGE('',*,*,#50752,.F.);
#75070=ORIENTED_EDGE('',*,*,#51249,.T.);
#75071=ORIENTED_EDGE('',*,*,#50755,.F.);
#75072=ORIENTED_EDGE('',*,*,#50903,.T.);
#75073=ORIENTED_EDGE('',*,*,#50746,.F.);
#75074=ORIENTED_EDGE('',*,*,#50901,.T.);
#75075=ORIENTED_EDGE('',*,*,#50761,.F.);
#75076=ORIENTED_EDGE('',*,*,#51250,.T.);
#75077=ORIENTED_EDGE('',*,*,#50764,.F.);
#75078=ORIENTED_EDGE('',*,*,#50924,.T.);
#75079=ORIENTED_EDGE('',*,*,#50767,.F.);
#75080=ORIENTED_EDGE('',*,*,#51257,.T.);
#75081=ORIENTED_EDGE('',*,*,#50758,.F.);
#75082=ORIENTED_EDGE('',*,*,#50915,.T.);
#75083=ORIENTED_EDGE('',*,*,#50779,.F.);
#75084=ORIENTED_EDGE('',*,*,#51262,.T.);
#75085=ORIENTED_EDGE('',*,*,#50770,.F.);
#75086=ORIENTED_EDGE('',*,*,#50888,.T.);
#75087=ORIENTED_EDGE('',*,*,#50773,.F.);
#75088=ORIENTED_EDGE('',*,*,#51263,.F.);
#75089=ORIENTED_EDGE('',*,*,#50775,.F.);
#75090=ORIENTED_EDGE('',*,*,#50934,.T.);
#75091=ORIENTED_EDGE('',*,*,#50827,.F.);
#75092=ORIENTED_EDGE('',*,*,#51244,.T.);
#75093=ORIENTED_EDGE('',*,*,#50818,.F.);
#75094=ORIENTED_EDGE('',*,*,#50914,.T.);
#75095=ORIENTED_EDGE('',*,*,#50821,.F.);
#75096=ORIENTED_EDGE('',*,*,#51245,.F.);
#75097=ORIENTED_EDGE('',*,*,#50823,.F.);
#75098=ORIENTED_EDGE('',*,*,#50925,.T.);
#75099=ORIENTED_EDGE('',*,*,#50809,.F.);
#75100=ORIENTED_EDGE('',*,*,#51236,.T.);
#75101=ORIENTED_EDGE('',*,*,#50812,.F.);
#75102=ORIENTED_EDGE('',*,*,#50929,.T.);
#75103=ORIENTED_EDGE('',*,*,#50815,.F.);
#75104=ORIENTED_EDGE('',*,*,#51239,.T.);
#75105=ORIENTED_EDGE('',*,*,#50806,.F.);
#75106=ORIENTED_EDGE('',*,*,#51243,.T.);
#75107=ORIENTED_EDGE('',*,*,#50797,.F.);
#75108=ORIENTED_EDGE('',*,*,#50933,.T.);
#75109=ORIENTED_EDGE('',*,*,#50800,.F.);
#75110=ORIENTED_EDGE('',*,*,#51242,.T.);
#75111=ORIENTED_EDGE('',*,*,#50803,.F.);
#75112=ORIENTED_EDGE('',*,*,#50917,.T.);
#75113=ORIENTED_EDGE('',*,*,#50794,.F.);
#75114=ORIENTED_EDGE('',*,*,#50919,.T.);
#75115=ORIENTED_EDGE('',*,*,#50785,.F.);
#75116=ORIENTED_EDGE('',*,*,#51240,.T.);
#75117=ORIENTED_EDGE('',*,*,#50788,.F.);
#75118=ORIENTED_EDGE('',*,*,#50935,.T.);
#75119=ORIENTED_EDGE('',*,*,#50791,.F.);
#75120=ORIENTED_EDGE('',*,*,#51246,.F.);
#75121=ORIENTED_EDGE('',*,*,#50782,.F.);
#75122=ORIENTED_EDGE('',*,*,#50887,.T.);
#75123=ORIENTED_EDGE('',*,*,#50701,.F.);
#75124=ORIENTED_EDGE('',*,*,#51267,.F.);
#75125=ORIENTED_EDGE('',*,*,#51148,.F.);
#75126=ORIENTED_EDGE('',*,*,#51264,.F.);
#75127=ORIENTED_EDGE('',*,*,#50703,.F.);
#75128=ORIENTED_EDGE('',*,*,#50889,.T.);
#75129=ORIENTED_EDGE('',*,*,#50707,.F.);
#75130=ORIENTED_EDGE('',*,*,#51297,.T.);
#75131=ORIENTED_EDGE('',*,*,#50698,.F.);
#75132=ORIENTED_EDGE('',*,*,#51294,.T.);
#75133=ORIENTED_EDGE('',*,*,#50692,.F.);
#75134=ORIENTED_EDGE('',*,*,#51230,.F.);
#75135=ORIENTED_EDGE('',*,*,#51152,.F.);
#75136=ORIENTED_EDGE('',*,*,#51150,.F.);
#75137=ORIENTED_EDGE('',*,*,#50695,.F.);
#75138=ORIENTED_EDGE('',*,*,#51296,.T.);
#75139=ORIENTED_EDGE('',*,*,#50686,.F.);
#75140=ORIENTED_EDGE('',*,*,#50873,.T.);
#75141=ORIENTED_EDGE('',*,*,#50689,.F.);
#75142=ORIENTED_EDGE('',*,*,#51284,.T.);
#75143=ORIENTED_EDGE('',*,*,#50680,.F.);
#75144=ORIENTED_EDGE('',*,*,#51154,.F.);
#75145=ORIENTED_EDGE('',*,*,#50683,.F.);
#75146=ORIENTED_EDGE('',*,*,#51292,.T.);
#75147=ORIENTED_EDGE('',*,*,#50674,.F.);
#75148=ORIENTED_EDGE('',*,*,#50874,.T.);
#75149=ORIENTED_EDGE('',*,*,#50677,.F.);
#75150=ORIENTED_EDGE('',*,*,#51280,.T.);
#75151=ORIENTED_EDGE('',*,*,#50668,.F.);
#75152=ORIENTED_EDGE('',*,*,#51231,.F.);
#75153=ORIENTED_EDGE('',*,*,#50671,.F.);
#75154=ORIENTED_EDGE('',*,*,#51286,.T.);
#75155=ORIENTED_EDGE('',*,*,#50662,.F.);
#75156=ORIENTED_EDGE('',*,*,#50876,.T.);
#75157=ORIENTED_EDGE('',*,*,#50665,.F.);
#75158=ORIENTED_EDGE('',*,*,#51276,.T.);
#75159=ORIENTED_EDGE('',*,*,#50656,.F.);
#75160=ORIENTED_EDGE('',*,*,#51232,.F.);
#75161=ORIENTED_EDGE('',*,*,#50659,.F.);
#75162=ORIENTED_EDGE('',*,*,#51282,.T.);
#75163=ORIENTED_EDGE('',*,*,#50650,.F.);
#75164=ORIENTED_EDGE('',*,*,#50878,.T.);
#75165=ORIENTED_EDGE('',*,*,#50653,.F.);
#75166=ORIENTED_EDGE('',*,*,#51272,.T.);
#75167=ORIENTED_EDGE('',*,*,#50644,.F.);
#75168=ORIENTED_EDGE('',*,*,#51233,.F.);
#75169=ORIENTED_EDGE('',*,*,#50647,.F.);
#75170=ORIENTED_EDGE('',*,*,#51278,.T.);
#75171=ORIENTED_EDGE('',*,*,#50638,.F.);
#75172=ORIENTED_EDGE('',*,*,#50882,.T.);
#75173=ORIENTED_EDGE('',*,*,#50641,.F.);
#75174=ORIENTED_EDGE('',*,*,#50881,.T.);
#75175=ORIENTED_EDGE('',*,*,#50629,.F.);
#75176=ORIENTED_EDGE('',*,*,#51273,.T.);
#75177=ORIENTED_EDGE('',*,*,#50632,.F.);
#75178=ORIENTED_EDGE('',*,*,#50900,.T.);
#75179=ORIENTED_EDGE('',*,*,#50635,.F.);
#75180=ORIENTED_EDGE('',*,*,#51287,.T.);
#75181=ORIENTED_EDGE('',*,*,#50626,.F.);
#75182=ORIENTED_EDGE('',*,*,#51290,.T.);
#75183=ORIENTED_EDGE('',*,*,#50617,.F.);
#75184=ORIENTED_EDGE('',*,*,#50884,.T.);
#75185=ORIENTED_EDGE('',*,*,#50620,.F.);
#75186=ORIENTED_EDGE('',*,*,#51270,.F.);
#75187=ORIENTED_EDGE('',*,*,#50623,.F.);
#75188=ORIENTED_EDGE('',*,*,#51277,.T.);
#75189=ORIENTED_EDGE('',*,*,#50608,.F.);
#75190=ORIENTED_EDGE('',*,*,#50902,.T.);
#75191=ORIENTED_EDGE('',*,*,#50611,.F.);
#75192=ORIENTED_EDGE('',*,*,#51271,.T.);
#75193=ORIENTED_EDGE('',*,*,#50614,.F.);
#75194=ORIENTED_EDGE('',*,*,#50883,.T.);
#75195=ORIENTED_EDGE('',*,*,#50605,.F.);
#75196=ORIENTED_EDGE('',*,*,#51281,.T.);
#75197=ORIENTED_EDGE('',*,*,#50596,.F.);
#75198=ORIENTED_EDGE('',*,*,#50898,.T.);
#75199=ORIENTED_EDGE('',*,*,#50599,.F.);
#75200=ORIENTED_EDGE('',*,*,#51275,.T.);
#75201=ORIENTED_EDGE('',*,*,#50602,.F.);
#75202=ORIENTED_EDGE('',*,*,#50879,.T.);
#75203=ORIENTED_EDGE('',*,*,#50593,.F.);
#75204=ORIENTED_EDGE('',*,*,#51285,.T.);
#75205=ORIENTED_EDGE('',*,*,#50584,.F.);
#75206=ORIENTED_EDGE('',*,*,#50896,.T.);
#75207=ORIENTED_EDGE('',*,*,#50587,.F.);
#75208=ORIENTED_EDGE('',*,*,#51279,.T.);
#75209=ORIENTED_EDGE('',*,*,#50590,.F.);
#75210=ORIENTED_EDGE('',*,*,#50877,.T.);
#75211=ORIENTED_EDGE('',*,*,#50581,.F.);
#75212=ORIENTED_EDGE('',*,*,#51288,.T.);
#75213=ORIENTED_EDGE('',*,*,#50572,.F.);
#75214=ORIENTED_EDGE('',*,*,#51158,.F.);
#75215=ORIENTED_EDGE('',*,*,#51156,.F.);
#75216=ORIENTED_EDGE('',*,*,#51234,.F.);
#75217=ORIENTED_EDGE('',*,*,#50575,.F.);
#75218=ORIENTED_EDGE('',*,*,#51274,.T.);
#75219=ORIENTED_EDGE('',*,*,#50578,.F.);
#75220=ORIENTED_EDGE('',*,*,#50880,.T.);
#75221=ORIENTED_EDGE('',*,*,#50569,.F.);
#75222=ORIENTED_EDGE('',*,*,#51289,.T.);
#75223=ORIENTED_EDGE('',*,*,#50560,.F.);
#75224=ORIENTED_EDGE('',*,*,#50892,.T.);
#75225=ORIENTED_EDGE('',*,*,#50563,.F.);
#75226=ORIENTED_EDGE('',*,*,#51266,.F.);
#75227=ORIENTED_EDGE('',*,*,#51160,.F.);
#75228=ORIENTED_EDGE('',*,*,#51269,.F.);
#75229=ORIENTED_EDGE('',*,*,#50566,.F.);
#75230=ORIENTED_EDGE('',*,*,#50885,.T.);
#75231=ORIENTED_EDGE('',*,*,#50557,.F.);
#75232=ORIENTED_EDGE('',*,*,#51291,.T.);
#75233=ORIENTED_EDGE('',*,*,#50548,.F.);
#75234=ORIENTED_EDGE('',*,*,#50894,.T.);
#75235=ORIENTED_EDGE('',*,*,#50551,.F.);
#75236=ORIENTED_EDGE('',*,*,#51283,.T.);
#75237=ORIENTED_EDGE('',*,*,#50554,.F.);
#75238=ORIENTED_EDGE('',*,*,#50875,.T.);
#75239=ORIENTED_EDGE('',*,*,#50545,.F.);
#75240=ORIENTED_EDGE('',*,*,#51295,.T.);
#75241=ORIENTED_EDGE('',*,*,#50536,.F.);
#75242=ORIENTED_EDGE('',*,*,#50890,.T.);
#75243=ORIENTED_EDGE('',*,*,#50539,.F.);
#75244=ORIENTED_EDGE('',*,*,#51293,.T.);
#75245=ORIENTED_EDGE('',*,*,#50542,.F.);
#75246=ORIENTED_EDGE('',*,*,#50872,.T.);
#75247=ORIENTED_EDGE('',*,*,#50533,.F.);
#75248=ORIENTED_EDGE('',*,*,#51298,.T.);
#75249=ORIENTED_EDGE('',*,*,#50527,.F.);
#75250=ORIENTED_EDGE('',*,*,#51268,.F.);
#75251=ORIENTED_EDGE('',*,*,#50529,.F.);
#75252=ORIENTED_EDGE('',*,*,#50886,.T.);
#75253=ORIENTED_EDGE('',*,*,#50524,.F.);
#75254=ORIENTED_EDGE('',*,*,#51253,.T.);
#75255=ORIENTED_EDGE('',*,*,#50494,.F.);
#75256=ORIENTED_EDGE('',*,*,#50897,.T.);
#75257=ORIENTED_EDGE('',*,*,#50497,.F.);
#75258=ORIENTED_EDGE('',*,*,#51256,.T.);
#75259=ORIENTED_EDGE('',*,*,#50500,.F.);
#75260=ORIENTED_EDGE('',*,*,#50922,.T.);
#75261=ORIENTED_EDGE('',*,*,#50851,.F.);
#75262=ORIENTED_EDGE('',*,*,#50871,.F.);
#75263=ORIENTED_EDGE('',*,*,#50491,.F.);
#75264=ORIENTED_EDGE('',*,*,#50932,.T.);
#75265=ORIENTED_EDGE('',*,*,#50473,.F.);
#75266=ORIENTED_EDGE('',*,*,#53079,.F.);
#75267=ORIENTED_EDGE('',*,*,#50470,.F.);
#75268=ORIENTED_EDGE('',*,*,#50868,.F.);
#75269=ORIENTED_EDGE('',*,*,#50836,.F.);
#75270=ORIENTED_EDGE('',*,*,#50867,.T.);
#75271=ORIENTED_EDGE('',*,*,#50838,.F.);
#75272=ORIENTED_EDGE('',*,*,#50862,.T.);
#75273=ORIENTED_EDGE('',*,*,#50833,.F.);
#75274=ORIENTED_EDGE('',*,*,#50863,.T.);
#75275=ORIENTED_EDGE('',*,*,#50844,.F.);
#75276=ORIENTED_EDGE('',*,*,#53073,.F.);
#75277=ORIENTED_EDGE('',*,*,#50452,.F.);
#75278=ORIENTED_EDGE('',*,*,#50931,.T.);
#75279=ORIENTED_EDGE('',*,*,#50842,.F.);
#75280=ORIENTED_EDGE('',*,*,#50930,.T.);
#75281=ORIENTED_EDGE('',*,*,#50518,.F.);
#75282=ORIENTED_EDGE('',*,*,#51235,.T.);
#75283=ORIENTED_EDGE('',*,*,#50521,.F.);
#75284=ORIENTED_EDGE('',*,*,#50927,.T.);
#75285=ORIENTED_EDGE('',*,*,#50475,.F.);
#75286=ORIENTED_EDGE('',*,*,#50857,.F.);
#75287=ORIENTED_EDGE('',*,*,#50860,.F.);
#75288=ORIENTED_EDGE('',*,*,#50515,.F.);
#75289=ORIENTED_EDGE('',*,*,#50864,.T.);
#75290=ORIENTED_EDGE('',*,*,#50830,.F.);
#75291=ORIENTED_EDGE('',*,*,#50865,.T.);
#75292=ORIENTED_EDGE('',*,*,#50455,.F.);
#75293=ORIENTED_EDGE('',*,*,#51238,.T.);
#75294=ORIENTED_EDGE('',*,*,#50458,.F.);
#75295=ORIENTED_EDGE('',*,*,#53075,.F.);
#75296=ORIENTED_EDGE('',*,*,#50848,.F.);
#75297=ORIENTED_EDGE('',*,*,#50921,.T.);
#75298=ORIENTED_EDGE('',*,*,#50506,.F.);
#75299=ORIENTED_EDGE('',*,*,#51241,.T.);
#75300=ORIENTED_EDGE('',*,*,#50509,.F.);
#75301=ORIENTED_EDGE('',*,*,#50928,.T.);
#75302=ORIENTED_EDGE('',*,*,#50512,.F.);
#75303=ORIENTED_EDGE('',*,*,#50861,.F.);
#75304=ORIENTED_EDGE('',*,*,#50858,.F.);
#75305=ORIENTED_EDGE('',*,*,#50503,.F.);
#75306=ORIENTED_EDGE('',*,*,#50870,.T.);
#75307=ORIENTED_EDGE('',*,*,#50448,.F.);
#75308=ORIENTED_EDGE('',*,*,#50869,.F.);
#75309=ORIENTED_EDGE('',*,*,#50467,.F.);
#75310=ORIENTED_EDGE('',*,*,#53077,.F.);
#75311=ORIENTED_EDGE('',*,*,#50461,.F.);
#75312=ORIENTED_EDGE('',*,*,#51237,.T.);
#75313=ORIENTED_EDGE('',*,*,#50464,.F.);
#75314=ORIENTED_EDGE('',*,*,#50923,.T.);
#75315=ORIENTED_EDGE('',*,*,#50482,.F.);
#75316=ORIENTED_EDGE('',*,*,#51251,.T.);
#75317=ORIENTED_EDGE('',*,*,#50485,.F.);
#75318=ORIENTED_EDGE('',*,*,#50899,.T.);
#75319=ORIENTED_EDGE('',*,*,#50488,.F.);
#75320=ORIENTED_EDGE('',*,*,#51254,.T.);
#75321=ORIENTED_EDGE('',*,*,#50479,.F.);
#75322=ORIENTED_EDGE('',*,*,#50866,.F.);
#75323=ORIENTED_EDGE('',*,*,#50854,.F.);
#75324=ORIENTED_EDGE('',*,*,#53120,.F.);
#75325=ORIENTED_EDGE('',*,*,#52918,.T.);
#75326=ORIENTED_EDGE('',*,*,#53173,.T.);
#75327=ORIENTED_EDGE('',*,*,#52927,.T.);
#75328=ORIENTED_EDGE('',*,*,#53145,.F.);
#75329=ORIENTED_EDGE('',*,*,#52924,.T.);
#75330=ORIENTED_EDGE('',*,*,#53174,.F.);
#75331=ORIENTED_EDGE('',*,*,#52921,.T.);
#75332=ORIENTED_EDGE('',*,*,#53175,.F.);
#75333=ORIENTED_EDGE('',*,*,#52930,.T.);
#75334=ORIENTED_EDGE('',*,*,#53118,.F.);
#75335=ORIENTED_EDGE('',*,*,#52939,.T.);
#75336=ORIENTED_EDGE('',*,*,#53176,.F.);
#75337=ORIENTED_EDGE('',*,*,#52936,.T.);
#75338=ORIENTED_EDGE('',*,*,#53143,.F.);
#75339=ORIENTED_EDGE('',*,*,#52933,.T.);
#75340=ORIENTED_EDGE('',*,*,#53177,.F.);
#75341=ORIENTED_EDGE('',*,*,#52942,.T.);
#75342=ORIENTED_EDGE('',*,*,#53122,.F.);
#75343=ORIENTED_EDGE('',*,*,#52951,.T.);
#75344=ORIENTED_EDGE('',*,*,#53178,.F.);
#75345=ORIENTED_EDGE('',*,*,#52948,.T.);
#75346=ORIENTED_EDGE('',*,*,#53147,.F.);
#75347=ORIENTED_EDGE('',*,*,#52945,.T.);
#75348=ORIENTED_EDGE('',*,*,#53179,.F.);
#75349=ORIENTED_EDGE('',*,*,#52954,.T.);
#75350=ORIENTED_EDGE('',*,*,#53130,.F.);
#75351=ORIENTED_EDGE('',*,*,#52963,.T.);
#75352=ORIENTED_EDGE('',*,*,#53180,.F.);
#75353=ORIENTED_EDGE('',*,*,#52960,.T.);
#75354=ORIENTED_EDGE('',*,*,#53153,.F.);
#75355=ORIENTED_EDGE('',*,*,#52957,.T.);
#75356=ORIENTED_EDGE('',*,*,#53128,.F.);
#75357=ORIENTED_EDGE('',*,*,#52966,.T.);
#75358=ORIENTED_EDGE('',*,*,#53181,.F.);
#75359=ORIENTED_EDGE('',*,*,#52975,.T.);
#75360=ORIENTED_EDGE('',*,*,#53151,.F.);
#75361=ORIENTED_EDGE('',*,*,#52972,.T.);
#75362=ORIENTED_EDGE('',*,*,#53182,.F.);
#75363=ORIENTED_EDGE('',*,*,#52969,.T.);
#75364=ORIENTED_EDGE('',*,*,#53142,.F.);
#75365=ORIENTED_EDGE('',*,*,#52982,.T.);
#75366=ORIENTED_EDGE('',*,*,#53183,.T.);
#75367=ORIENTED_EDGE('',*,*,#52981,.T.);
#75368=ORIENTED_EDGE('',*,*,#53115,.F.);
#75369=ORIENTED_EDGE('',*,*,#52978,.T.);
#75370=ORIENTED_EDGE('',*,*,#53184,.F.);
#75371=ORIENTED_EDGE('',*,*,#52987,.T.);
#75372=ORIENTED_EDGE('',*,*,#53161,.F.);
#75373=ORIENTED_EDGE('',*,*,#53030,.T.);
#75374=ORIENTED_EDGE('',*,*,#53185,.T.);
#75375=ORIENTED_EDGE('',*,*,#53029,.T.);
#75376=ORIENTED_EDGE('',*,*,#53141,.F.);
#75377=ORIENTED_EDGE('',*,*,#53026,.T.);
#75378=ORIENTED_EDGE('',*,*,#53186,.F.);
#75379=ORIENTED_EDGE('',*,*,#53035,.T.);
#75380=ORIENTED_EDGE('',*,*,#53152,.F.);
#75381=ORIENTED_EDGE('',*,*,#53014,.T.);
#75382=ORIENTED_EDGE('',*,*,#53187,.F.);
#75383=ORIENTED_EDGE('',*,*,#53023,.T.);
#75384=ORIENTED_EDGE('',*,*,#53156,.F.);
#75385=ORIENTED_EDGE('',*,*,#53020,.T.);
#75386=ORIENTED_EDGE('',*,*,#53188,.F.);
#75387=ORIENTED_EDGE('',*,*,#53017,.T.);
#75388=ORIENTED_EDGE('',*,*,#53189,.F.);
#75389=ORIENTED_EDGE('',*,*,#53002,.T.);
#75390=ORIENTED_EDGE('',*,*,#53144,.F.);
#75391=ORIENTED_EDGE('',*,*,#53011,.T.);
#75392=ORIENTED_EDGE('',*,*,#53190,.F.);
#75393=ORIENTED_EDGE('',*,*,#53008,.T.);
#75394=ORIENTED_EDGE('',*,*,#53160,.F.);
#75395=ORIENTED_EDGE('',*,*,#53005,.T.);
#75396=ORIENTED_EDGE('',*,*,#53146,.F.);
#75397=ORIENTED_EDGE('',*,*,#52990,.T.);
#75398=ORIENTED_EDGE('',*,*,#53191,.T.);
#75399=ORIENTED_EDGE('',*,*,#52999,.T.);
#75400=ORIENTED_EDGE('',*,*,#53162,.F.);
#75401=ORIENTED_EDGE('',*,*,#52996,.T.);
#75402=ORIENTED_EDGE('',*,*,#53192,.F.);
#75403=ORIENTED_EDGE('',*,*,#52993,.T.);
#75404=ORIENTED_EDGE('',*,*,#53114,.F.);
#75405=ORIENTED_EDGE('',*,*,#52906,.T.);
#75406=ORIENTED_EDGE('',*,*,#53193,.F.);
#75407=ORIENTED_EDGE('',*,*,#52915,.T.);
#75408=ORIENTED_EDGE('',*,*,#53116,.F.);
#75409=ORIENTED_EDGE('',*,*,#52910,.T.);
#75410=ORIENTED_EDGE('',*,*,#53194,.T.);
#75411=ORIENTED_EDGE('',*,*,#53195,.T.);
#75412=ORIENTED_EDGE('',*,*,#53196,.T.);
#75413=ORIENTED_EDGE('',*,*,#52909,.T.);
#75414=ORIENTED_EDGE('',*,*,#53197,.F.);
#75415=ORIENTED_EDGE('',*,*,#52897,.T.);
#75416=ORIENTED_EDGE('',*,*,#53100,.F.);
#75417=ORIENTED_EDGE('',*,*,#52894,.T.);
#75418=ORIENTED_EDGE('',*,*,#53198,.F.);
#75419=ORIENTED_EDGE('',*,*,#52903,.T.);
#75420=ORIENTED_EDGE('',*,*,#53199,.T.);
#75421=ORIENTED_EDGE('',*,*,#53200,.T.);
#75422=ORIENTED_EDGE('',*,*,#53201,.T.);
#75423=ORIENTED_EDGE('',*,*,#52900,.T.);
#75424=ORIENTED_EDGE('',*,*,#53202,.F.);
#75425=ORIENTED_EDGE('',*,*,#52885,.T.);
#75426=ORIENTED_EDGE('',*,*,#53101,.F.);
#75427=ORIENTED_EDGE('',*,*,#52882,.T.);
#75428=ORIENTED_EDGE('',*,*,#53203,.F.);
#75429=ORIENTED_EDGE('',*,*,#52891,.T.);
#75430=ORIENTED_EDGE('',*,*,#53204,.T.);
#75431=ORIENTED_EDGE('',*,*,#52888,.T.);
#75432=ORIENTED_EDGE('',*,*,#53205,.F.);
#75433=ORIENTED_EDGE('',*,*,#52873,.T.);
#75434=ORIENTED_EDGE('',*,*,#53103,.F.);
#75435=ORIENTED_EDGE('',*,*,#52870,.T.);
#75436=ORIENTED_EDGE('',*,*,#53206,.F.);
#75437=ORIENTED_EDGE('',*,*,#52879,.T.);
#75438=ORIENTED_EDGE('',*,*,#53207,.T.);
#75439=ORIENTED_EDGE('',*,*,#52876,.T.);
#75440=ORIENTED_EDGE('',*,*,#53208,.F.);
#75441=ORIENTED_EDGE('',*,*,#52861,.T.);
#75442=ORIENTED_EDGE('',*,*,#53105,.F.);
#75443=ORIENTED_EDGE('',*,*,#52858,.T.);
#75444=ORIENTED_EDGE('',*,*,#53209,.F.);
#75445=ORIENTED_EDGE('',*,*,#52867,.T.);
#75446=ORIENTED_EDGE('',*,*,#53210,.T.);
#75447=ORIENTED_EDGE('',*,*,#52864,.T.);
#75448=ORIENTED_EDGE('',*,*,#53211,.F.);
#75449=ORIENTED_EDGE('',*,*,#52849,.T.);
#75450=ORIENTED_EDGE('',*,*,#53109,.F.);
#75451=ORIENTED_EDGE('',*,*,#52846,.T.);
#75452=ORIENTED_EDGE('',*,*,#53212,.F.);
#75453=ORIENTED_EDGE('',*,*,#52855,.T.);
#75454=ORIENTED_EDGE('',*,*,#53213,.T.);
#75455=ORIENTED_EDGE('',*,*,#52852,.T.);
#75456=ORIENTED_EDGE('',*,*,#53108,.F.);
#75457=ORIENTED_EDGE('',*,*,#52834,.T.);
#75458=ORIENTED_EDGE('',*,*,#53214,.F.);
#75459=ORIENTED_EDGE('',*,*,#52843,.T.);
#75460=ORIENTED_EDGE('',*,*,#53127,.F.);
#75461=ORIENTED_EDGE('',*,*,#52840,.T.);
#75462=ORIENTED_EDGE('',*,*,#53215,.F.);
#75463=ORIENTED_EDGE('',*,*,#52837,.T.);
#75464=ORIENTED_EDGE('',*,*,#53216,.F.);
#75465=ORIENTED_EDGE('',*,*,#52831,.T.);
#75466=ORIENTED_EDGE('',*,*,#53217,.T.);
#75467=ORIENTED_EDGE('',*,*,#52828,.T.);
#75468=ORIENTED_EDGE('',*,*,#53111,.F.);
#75469=ORIENTED_EDGE('',*,*,#52825,.T.);
#75470=ORIENTED_EDGE('',*,*,#53218,.F.);
#75471=ORIENTED_EDGE('',*,*,#52813,.T.);
#75472=ORIENTED_EDGE('',*,*,#53110,.F.);
#75473=ORIENTED_EDGE('',*,*,#52822,.T.);
#75474=ORIENTED_EDGE('',*,*,#53219,.F.);
#75475=ORIENTED_EDGE('',*,*,#52819,.T.);
#75476=ORIENTED_EDGE('',*,*,#53129,.F.);
#75477=ORIENTED_EDGE('',*,*,#52816,.T.);
#75478=ORIENTED_EDGE('',*,*,#53220,.F.);
#75479=ORIENTED_EDGE('',*,*,#52801,.T.);
#75480=ORIENTED_EDGE('',*,*,#53106,.F.);
#75481=ORIENTED_EDGE('',*,*,#52810,.T.);
#75482=ORIENTED_EDGE('',*,*,#53221,.F.);
#75483=ORIENTED_EDGE('',*,*,#52807,.T.);
#75484=ORIENTED_EDGE('',*,*,#53125,.F.);
#75485=ORIENTED_EDGE('',*,*,#52804,.T.);
#75486=ORIENTED_EDGE('',*,*,#53222,.F.);
#75487=ORIENTED_EDGE('',*,*,#52789,.T.);
#75488=ORIENTED_EDGE('',*,*,#53104,.F.);
#75489=ORIENTED_EDGE('',*,*,#52798,.T.);
#75490=ORIENTED_EDGE('',*,*,#53223,.F.);
#75491=ORIENTED_EDGE('',*,*,#52795,.T.);
#75492=ORIENTED_EDGE('',*,*,#53123,.F.);
#75493=ORIENTED_EDGE('',*,*,#52792,.T.);
#75494=ORIENTED_EDGE('',*,*,#53224,.F.);
#75495=ORIENTED_EDGE('',*,*,#52777,.T.);
#75496=ORIENTED_EDGE('',*,*,#53107,.F.);
#75497=ORIENTED_EDGE('',*,*,#52786,.T.);
#75498=ORIENTED_EDGE('',*,*,#53225,.F.);
#75499=ORIENTED_EDGE('',*,*,#52783,.T.);
#75500=ORIENTED_EDGE('',*,*,#53226,.T.);
#75501=ORIENTED_EDGE('',*,*,#53227,.T.);
#75502=ORIENTED_EDGE('',*,*,#53228,.T.);
#75503=ORIENTED_EDGE('',*,*,#52780,.T.);
#75504=ORIENTED_EDGE('',*,*,#53229,.F.);
#75505=ORIENTED_EDGE('',*,*,#52765,.T.);
#75506=ORIENTED_EDGE('',*,*,#53112,.F.);
#75507=ORIENTED_EDGE('',*,*,#52774,.T.);
#75508=ORIENTED_EDGE('',*,*,#53230,.T.);
#75509=ORIENTED_EDGE('',*,*,#53231,.T.);
#75510=ORIENTED_EDGE('',*,*,#53232,.T.);
#75511=ORIENTED_EDGE('',*,*,#52771,.T.);
#75512=ORIENTED_EDGE('',*,*,#53119,.F.);
#75513=ORIENTED_EDGE('',*,*,#52768,.T.);
#75514=ORIENTED_EDGE('',*,*,#53233,.F.);
#75515=ORIENTED_EDGE('',*,*,#52753,.T.);
#75516=ORIENTED_EDGE('',*,*,#53102,.F.);
#75517=ORIENTED_EDGE('',*,*,#52762,.T.);
#75518=ORIENTED_EDGE('',*,*,#53234,.F.);
#75519=ORIENTED_EDGE('',*,*,#52759,.T.);
#75520=ORIENTED_EDGE('',*,*,#53121,.F.);
#75521=ORIENTED_EDGE('',*,*,#52756,.T.);
#75522=ORIENTED_EDGE('',*,*,#53235,.F.);
#75523=ORIENTED_EDGE('',*,*,#52741,.T.);
#75524=ORIENTED_EDGE('',*,*,#53099,.F.);
#75525=ORIENTED_EDGE('',*,*,#52750,.T.);
#75526=ORIENTED_EDGE('',*,*,#53236,.F.);
#75527=ORIENTED_EDGE('',*,*,#52747,.T.);
#75528=ORIENTED_EDGE('',*,*,#53117,.F.);
#75529=ORIENTED_EDGE('',*,*,#52744,.T.);
#75530=ORIENTED_EDGE('',*,*,#53237,.F.);
#75531=ORIENTED_EDGE('',*,*,#52732,.T.);
#75532=ORIENTED_EDGE('',*,*,#53113,.F.);
#75533=ORIENTED_EDGE('',*,*,#52736,.T.);
#75534=ORIENTED_EDGE('',*,*,#53238,.T.);
#75535=ORIENTED_EDGE('',*,*,#52735,.T.);
#75536=ORIENTED_EDGE('',*,*,#53239,.F.);
#75537=ORIENTED_EDGE('',*,*,#52699,.T.);
#75538=ORIENTED_EDGE('',*,*,#53098,.T.);
#75539=ORIENTED_EDGE('',*,*,#53059,.T.);
#75540=ORIENTED_EDGE('',*,*,#53149,.F.);
#75541=ORIENTED_EDGE('',*,*,#52708,.T.);
#75542=ORIENTED_EDGE('',*,*,#53240,.F.);
#75543=ORIENTED_EDGE('',*,*,#52705,.T.);
#75544=ORIENTED_EDGE('',*,*,#53124,.F.);
#75545=ORIENTED_EDGE('',*,*,#52702,.T.);
#75546=ORIENTED_EDGE('',*,*,#53159,.F.);
#75547=ORIENTED_EDGE('',*,*,#53045,.T.);
#75548=ORIENTED_EDGE('',*,*,#53094,.F.);
#75549=ORIENTED_EDGE('',*,*,#53044,.T.);
#75550=ORIENTED_EDGE('',*,*,#53095,.T.);
#75551=ORIENTED_EDGE('',*,*,#52678,.T.);
#75552=ORIENTED_EDGE('',*,*,#53081,.T.);
#75553=ORIENTED_EDGE('',*,*,#52681,.T.);
#75554=ORIENTED_EDGE('',*,*,#53089,.F.);
#75555=ORIENTED_EDGE('',*,*,#53050,.T.);
#75556=ORIENTED_EDGE('',*,*,#53158,.F.);
#75557=ORIENTED_EDGE('',*,*,#52660,.T.);
#75558=ORIENTED_EDGE('',*,*,#53087,.T.);
#75559=ORIENTED_EDGE('',*,*,#53051,.T.);
#75560=ORIENTED_EDGE('',*,*,#53090,.F.);
#75561=ORIENTED_EDGE('',*,*,#53041,.T.);
#75562=ORIENTED_EDGE('',*,*,#53157,.F.);
#75563=ORIENTED_EDGE('',*,*,#52723,.T.);
#75564=ORIENTED_EDGE('',*,*,#53069,.T.);
#75565=ORIENTED_EDGE('',*,*,#53064,.T.);
#75566=ORIENTED_EDGE('',*,*,#52682,.T.);
#75567=ORIENTED_EDGE('',*,*,#53154,.F.);
#75568=ORIENTED_EDGE('',*,*,#52729,.T.);
#75569=ORIENTED_EDGE('',*,*,#53241,.F.);
#75570=ORIENTED_EDGE('',*,*,#52726,.T.);
#75571=ORIENTED_EDGE('',*,*,#53091,.F.);
#75572=ORIENTED_EDGE('',*,*,#53056,.T.);
#75573=ORIENTED_EDGE('',*,*,#53085,.T.);
#75574=ORIENTED_EDGE('',*,*,#52666,.T.);
#75575=ORIENTED_EDGE('',*,*,#53242,.F.);
#75576=ORIENTED_EDGE('',*,*,#52663,.T.);
#75577=ORIENTED_EDGE('',*,*,#53092,.F.);
#75578=ORIENTED_EDGE('',*,*,#53038,.T.);
#75579=ORIENTED_EDGE('',*,*,#53148,.F.);
#75580=ORIENTED_EDGE('',*,*,#52711,.T.);
#75581=ORIENTED_EDGE('',*,*,#53066,.T.);
#75582=ORIENTED_EDGE('',*,*,#53070,.T.);
#75583=ORIENTED_EDGE('',*,*,#52720,.T.);
#75584=ORIENTED_EDGE('',*,*,#53155,.F.);
#75585=ORIENTED_EDGE('',*,*,#52717,.T.);
#75586=ORIENTED_EDGE('',*,*,#53243,.F.);
#75587=ORIENTED_EDGE('',*,*,#52714,.T.);
#75588=ORIENTED_EDGE('',*,*,#53097,.F.);
#75589=ORIENTED_EDGE('',*,*,#52672,.T.);
#75590=ORIENTED_EDGE('',*,*,#53244,.F.);
#75591=ORIENTED_EDGE('',*,*,#52669,.T.);
#75592=ORIENTED_EDGE('',*,*,#53083,.T.);
#75593=ORIENTED_EDGE('',*,*,#52675,.T.);
#75594=ORIENTED_EDGE('',*,*,#53096,.T.);
#75595=ORIENTED_EDGE('',*,*,#52655,.T.);
#75596=ORIENTED_EDGE('',*,*,#53150,.F.);
#75597=ORIENTED_EDGE('',*,*,#53062,.T.);
#75598=ORIENTED_EDGE('',*,*,#53093,.T.);
#75599=ORIENTED_EDGE('',*,*,#52687,.T.);
#75600=ORIENTED_EDGE('',*,*,#53245,.F.);
#75601=ORIENTED_EDGE('',*,*,#52696,.T.);
#75602=ORIENTED_EDGE('',*,*,#53126,.F.);
#75603=ORIENTED_EDGE('',*,*,#52693,.T.);
#75604=ORIENTED_EDGE('',*,*,#53246,.F.);
#75605=ORIENTED_EDGE('',*,*,#52690,.T.);
#75606=ORIENTED_EDGE('',*,*,#53247,.F.);
#75607=ORIENTED_EDGE('',*,*,#53171,.T.);
#75608=ORIENTED_EDGE('',*,*,#53248,.T.);
#75609=ORIENTED_EDGE('',*,*,#53249,.F.);
#75610=ORIENTED_EDGE('',*,*,#53250,.T.);
#75611=ORIENTED_EDGE('',*,*,#53248,.F.);
#75612=ORIENTED_EDGE('',*,*,#53170,.T.);
#75613=ORIENTED_EDGE('',*,*,#53251,.T.);
#75614=ORIENTED_EDGE('',*,*,#53251,.F.);
#75615=ORIENTED_EDGE('',*,*,#53169,.T.);
#75616=ORIENTED_EDGE('',*,*,#53252,.T.);
#75617=ORIENTED_EDGE('',*,*,#53253,.F.);
#75618=ORIENTED_EDGE('',*,*,#53252,.F.);
#75619=ORIENTED_EDGE('',*,*,#53168,.T.);
#75620=ORIENTED_EDGE('',*,*,#53254,.T.);
#75621=ORIENTED_EDGE('',*,*,#53255,.F.);
#75622=ORIENTED_EDGE('',*,*,#53254,.F.);
#75623=ORIENTED_EDGE('',*,*,#53167,.T.);
#75624=ORIENTED_EDGE('',*,*,#53256,.T.);
#75625=ORIENTED_EDGE('',*,*,#53257,.F.);
#75626=ORIENTED_EDGE('',*,*,#53258,.T.);
#75627=ORIENTED_EDGE('',*,*,#53256,.F.);
#75628=ORIENTED_EDGE('',*,*,#53166,.T.);
#75629=ORIENTED_EDGE('',*,*,#53259,.T.);
#75630=ORIENTED_EDGE('',*,*,#53259,.F.);
#75631=ORIENTED_EDGE('',*,*,#53165,.T.);
#75632=ORIENTED_EDGE('',*,*,#53260,.T.);
#75633=ORIENTED_EDGE('',*,*,#53261,.F.);
#75634=ORIENTED_EDGE('',*,*,#53260,.F.);
#75635=ORIENTED_EDGE('',*,*,#53164,.T.);
#75636=ORIENTED_EDGE('',*,*,#50956,.T.);
#75637=ORIENTED_EDGE('',*,*,#53262,.F.);
#75638=ORIENTED_EDGE('',*,*,#53263,.F.);
#75639=ORIENTED_EDGE('',*,*,#53264,.T.);
#75640=ORIENTED_EDGE('',*,*,#53265,.F.);
#75641=ORIENTED_EDGE('',*,*,#53266,.T.);
#75642=ORIENTED_EDGE('',*,*,#53267,.T.);
#75643=ORIENTED_EDGE('',*,*,#53263,.T.);
#75644=ORIENTED_EDGE('',*,*,#53268,.F.);
#75645=ORIENTED_EDGE('',*,*,#53269,.F.);
#75646=ORIENTED_EDGE('',*,*,#53270,.F.);
#75647=ORIENTED_EDGE('',*,*,#53271,.F.);
#75648=ORIENTED_EDGE('',*,*,#53272,.T.);
#75649=ORIENTED_EDGE('',*,*,#53270,.T.);
#75650=ORIENTED_EDGE('',*,*,#53273,.F.);
#75651=ORIENTED_EDGE('',*,*,#53274,.T.);
#75652=ORIENTED_EDGE('',*,*,#53275,.F.);
#75653=ORIENTED_EDGE('',*,*,#53276,.T.);
#75654=ORIENTED_EDGE('',*,*,#53277,.F.);
#75655=ORIENTED_EDGE('',*,*,#53278,.T.);
#75656=ORIENTED_EDGE('',*,*,#53279,.T.);
#75657=ORIENTED_EDGE('',*,*,#53280,.T.);
#75658=ORIENTED_EDGE('',*,*,#53281,.F.);
#75659=ORIENTED_EDGE('',*,*,#53282,.T.);
#75660=ORIENTED_EDGE('',*,*,#53277,.T.);
#75661=ORIENTED_EDGE('',*,*,#53283,.T.);
#75662=ORIENTED_EDGE('',*,*,#53279,.F.);
#75663=ORIENTED_EDGE('',*,*,#53284,.T.);
#75664=ORIENTED_EDGE('',*,*,#53285,.T.);
#75665=ORIENTED_EDGE('',*,*,#53286,.T.);
#75666=ORIENTED_EDGE('',*,*,#53287,.F.);
#75667=ORIENTED_EDGE('',*,*,#53288,.T.);
#75668=ORIENTED_EDGE('',*,*,#53289,.F.);
#75669=ORIENTED_EDGE('',*,*,#53290,.T.);
#75670=ORIENTED_EDGE('',*,*,#53291,.F.);
#75671=ORIENTED_EDGE('',*,*,#53292,.T.);
#75672=ORIENTED_EDGE('',*,*,#53291,.T.);
#75673=ORIENTED_EDGE('',*,*,#53293,.T.);
#75674=ORIENTED_EDGE('',*,*,#53285,.F.);
#75675=ORIENTED_EDGE('',*,*,#53294,.F.);
#75676=ORIENTED_EDGE('',*,*,#53295,.F.);
#75677=ORIENTED_EDGE('',*,*,#53296,.T.);
#75678=ORIENTED_EDGE('',*,*,#53297,.T.);
#75679=ORIENTED_EDGE('',*,*,#51137,.F.);
#75680=ORIENTED_EDGE('',*,*,#51121,.T.);
#75681=ORIENTED_EDGE('',*,*,#51136,.T.);
#75682=ORIENTED_EDGE('',*,*,#51091,.T.);
#75683=ORIENTED_EDGE('',*,*,#51093,.T.);
#75684=ORIENTED_EDGE('',*,*,#53298,.T.);
#75685=ORIENTED_EDGE('',*,*,#53299,.F.);
#75686=ORIENTED_EDGE('',*,*,#53300,.F.);
#75687=ORIENTED_EDGE('',*,*,#53301,.F.);
#75688=ORIENTED_EDGE('',*,*,#53302,.F.);
#75689=ORIENTED_EDGE('',*,*,#53303,.T.);
#75690=ORIENTED_EDGE('',*,*,#53304,.F.);
#75691=ORIENTED_EDGE('',*,*,#53305,.T.);
#75692=ORIENTED_EDGE('',*,*,#53306,.T.);
#75693=ORIENTED_EDGE('',*,*,#53307,.F.);
#75694=ORIENTED_EDGE('',*,*,#51085,.F.);
#75695=ORIENTED_EDGE('',*,*,#51114,.F.);
#75696=ORIENTED_EDGE('',*,*,#53308,.T.);
#75697=ORIENTED_EDGE('',*,*,#51111,.F.);
#75698=ORIENTED_EDGE('',*,*,#53309,.T.);
#75699=ORIENTED_EDGE('',*,*,#53310,.F.);
#75700=ORIENTED_EDGE('',*,*,#53311,.F.);
#75701=ORIENTED_EDGE('',*,*,#53312,.T.);
#75702=ORIENTED_EDGE('',*,*,#53313,.F.);
#75703=ORIENTED_EDGE('',*,*,#53314,.F.);
#75704=ORIENTED_EDGE('',*,*,#53315,.F.);
#75705=ORIENTED_EDGE('',*,*,#53316,.T.);
#75706=ORIENTED_EDGE('',*,*,#53317,.T.);
#75707=ORIENTED_EDGE('',*,*,#53294,.T.);
#75708=ORIENTED_EDGE('',*,*,#53318,.T.);
#75709=ORIENTED_EDGE('',*,*,#53296,.F.);
#75710=ORIENTED_EDGE('',*,*,#53319,.F.);
#75711=ORIENTED_EDGE('',*,*,#53320,.T.);
#75712=ORIENTED_EDGE('',*,*,#53321,.T.);
#75713=ORIENTED_EDGE('',*,*,#53322,.F.);
#75714=ORIENTED_EDGE('',*,*,#53313,.T.);
#75715=ORIENTED_EDGE('',*,*,#53323,.F.);
#75716=ORIENTED_EDGE('',*,*,#53311,.T.);
#75717=ORIENTED_EDGE('',*,*,#53324,.F.);
#75718=ORIENTED_EDGE('',*,*,#53309,.F.);
#75719=ORIENTED_EDGE('',*,*,#51110,.T.);
#75720=ORIENTED_EDGE('',*,*,#53308,.F.);
#75721=ORIENTED_EDGE('',*,*,#51113,.T.);
#75722=ORIENTED_EDGE('',*,*,#50996,.F.);
#75723=ORIENTED_EDGE('',*,*,#53325,.F.);
#75724=ORIENTED_EDGE('',*,*,#53321,.F.);
#75725=ORIENTED_EDGE('',*,*,#53326,.T.);
#75726=ORIENTED_EDGE('',*,*,#53327,.T.);
#75727=ORIENTED_EDGE('',*,*,#53328,.F.);
#75728=ORIENTED_EDGE('',*,*,#53327,.F.);
#75729=ORIENTED_EDGE('',*,*,#53329,.T.);
#75730=ORIENTED_EDGE('',*,*,#53330,.T.);
#75731=ORIENTED_EDGE('',*,*,#53331,.F.);
#75732=ORIENTED_EDGE('',*,*,#53330,.F.);
#75733=ORIENTED_EDGE('',*,*,#53332,.T.);
#75734=ORIENTED_EDGE('',*,*,#53333,.T.);
#75735=ORIENTED_EDGE('',*,*,#53334,.T.);
#75736=ORIENTED_EDGE('',*,*,#53335,.T.);
#75737=ORIENTED_EDGE('',*,*,#53336,.F.);
#75738=ORIENTED_EDGE('',*,*,#53333,.F.);
#75739=ORIENTED_EDGE('',*,*,#53337,.F.);
#75740=ORIENTED_EDGE('',*,*,#53338,.F.);
#75741=ORIENTED_EDGE('',*,*,#53339,.T.);
#75742=ORIENTED_EDGE('',*,*,#53340,.T.);
#75743=ORIENTED_EDGE('',*,*,#53341,.F.);
#75744=ORIENTED_EDGE('',*,*,#53340,.F.);
#75745=ORIENTED_EDGE('',*,*,#53342,.T.);
#75746=ORIENTED_EDGE('',*,*,#53315,.T.);
#75747=ORIENTED_EDGE('',*,*,#53343,.T.);
#75748=ORIENTED_EDGE('',*,*,#53344,.T.);
#75749=ORIENTED_EDGE('',*,*,#53345,.F.);
#75750=ORIENTED_EDGE('',*,*,#53346,.T.);
#75751=ORIENTED_EDGE('',*,*,#53347,.F.);
#75752=ORIENTED_EDGE('',*,*,#53348,.T.);
#75753=ORIENTED_EDGE('',*,*,#53349,.T.);
#75754=ORIENTED_EDGE('',*,*,#53350,.F.);
#75755=ORIENTED_EDGE('',*,*,#53351,.F.);
#75756=ORIENTED_EDGE('',*,*,#53352,.F.);
#75757=ORIENTED_EDGE('',*,*,#53353,.T.);
#75758=ORIENTED_EDGE('',*,*,#53354,.T.);
#75759=ORIENTED_EDGE('',*,*,#53355,.F.);
#75760=ORIENTED_EDGE('',*,*,#53356,.T.);
#75761=ORIENTED_EDGE('',*,*,#53357,.F.);
#75762=ORIENTED_EDGE('',*,*,#53358,.T.);
#75763=ORIENTED_EDGE('',*,*,#53359,.F.);
#75764=ORIENTED_EDGE('',*,*,#53360,.F.);
#75765=ORIENTED_EDGE('',*,*,#53361,.F.);
#75766=ORIENTED_EDGE('',*,*,#53362,.F.);
#75767=ORIENTED_EDGE('',*,*,#53363,.F.);
#75768=ORIENTED_EDGE('',*,*,#53364,.F.);
#75769=ORIENTED_EDGE('',*,*,#53365,.T.);
#75770=ORIENTED_EDGE('',*,*,#53351,.T.);
#75771=ORIENTED_EDGE('',*,*,#53366,.T.);
#75772=ORIENTED_EDGE('',*,*,#53367,.T.);
#75773=ORIENTED_EDGE('',*,*,#53364,.T.);
#75774=ORIENTED_EDGE('',*,*,#53368,.F.);
#75775=ORIENTED_EDGE('',*,*,#53369,.F.);
#75776=ORIENTED_EDGE('',*,*,#53370,.T.);
#75777=ORIENTED_EDGE('',*,*,#53274,.F.);
#75778=ORIENTED_EDGE('',*,*,#53282,.F.);
#75779=ORIENTED_EDGE('',*,*,#53278,.F.);
#75780=ORIENTED_EDGE('',*,*,#53371,.F.);
#75781=ORIENTED_EDGE('',*,*,#53372,.F.);
#75782=ORIENTED_EDGE('',*,*,#53345,.T.);
#75783=ORIENTED_EDGE('',*,*,#53373,.F.);
#75784=ORIENTED_EDGE('',*,*,#53369,.T.);
#75785=ORIENTED_EDGE('',*,*,#53374,.F.);
#75786=ORIENTED_EDGE('',*,*,#53375,.F.);
#75787=ORIENTED_EDGE('',*,*,#53376,.T.);
#75788=ORIENTED_EDGE('',*,*,#53361,.T.);
#75789=ORIENTED_EDGE('',*,*,#53377,.T.);
#75790=ORIENTED_EDGE('',*,*,#53292,.F.);
#75791=ORIENTED_EDGE('',*,*,#53284,.F.);
#75792=ORIENTED_EDGE('',*,*,#53378,.T.);
#75793=ORIENTED_EDGE('',*,*,#53375,.T.);
#75794=ORIENTED_EDGE('',*,*,#53379,.F.);
#75795=ORIENTED_EDGE('',*,*,#53380,.F.);
#75796=ORIENTED_EDGE('',*,*,#53381,.T.);
#75797=ORIENTED_EDGE('',*,*,#53288,.F.);
#75798=ORIENTED_EDGE('',*,*,#53382,.F.);
#75799=ORIENTED_EDGE('',*,*,#53383,.F.);
#75800=ORIENTED_EDGE('',*,*,#53355,.T.);
#75801=ORIENTED_EDGE('',*,*,#53384,.F.);
#75802=ORIENTED_EDGE('',*,*,#53380,.T.);
#75803=ORIENTED_EDGE('',*,*,#53385,.F.);
#75804=ORIENTED_EDGE('',*,*,#53366,.F.);
#75805=ORIENTED_EDGE('',*,*,#53350,.T.);
#75806=ORIENTED_EDGE('',*,*,#53386,.T.);
#75807=ORIENTED_EDGE('',*,*,#53298,.F.);
#75808=ORIENTED_EDGE('',*,*,#51094,.F.);
#75809=ORIENTED_EDGE('',*,*,#51020,.F.);
#75810=ORIENTED_EDGE('',*,*,#51033,.T.);
#75811=ORIENTED_EDGE('',*,*,#53387,.F.);
#75812=ORIENTED_EDGE('',*,*,#51065,.T.);
#75813=ORIENTED_EDGE('',*,*,#51062,.T.);
#75814=ORIENTED_EDGE('',*,*,#51059,.T.);
#75815=ORIENTED_EDGE('',*,*,#51056,.T.);
#75816=ORIENTED_EDGE('',*,*,#51075,.T.);
#75817=ORIENTED_EDGE('',*,*,#51072,.T.);
#75818=ORIENTED_EDGE('',*,*,#51069,.T.);
#75819=ORIENTED_EDGE('',*,*,#53388,.F.);
#75820=ORIENTED_EDGE('',*,*,#53389,.F.);
#75821=ORIENTED_EDGE('',*,*,#53390,.F.);
#75822=ORIENTED_EDGE('',*,*,#53391,.F.);
#75823=ORIENTED_EDGE('',*,*,#53392,.F.);
#75824=ORIENTED_EDGE('',*,*,#53393,.F.);
#75825=ORIENTED_EDGE('',*,*,#53394,.F.);
#75826=ORIENTED_EDGE('',*,*,#53395,.F.);
#75827=ORIENTED_EDGE('',*,*,#51051,.F.);
#75828=ORIENTED_EDGE('',*,*,#53396,.T.);
#75829=ORIENTED_EDGE('',*,*,#53382,.T.);
#75830=ORIENTED_EDGE('',*,*,#53379,.T.);
#75831=ORIENTED_EDGE('',*,*,#53374,.T.);
#75832=ORIENTED_EDGE('',*,*,#53397,.T.);
#75833=ORIENTED_EDGE('',*,*,#53371,.T.);
#75834=ORIENTED_EDGE('',*,*,#53368,.T.);
#75835=ORIENTED_EDGE('',*,*,#53363,.T.);
#75836=ORIENTED_EDGE('',*,*,#53385,.T.);
#75837=ORIENTED_EDGE('',*,*,#51032,.F.);
#75838=ORIENTED_EDGE('',*,*,#51039,.F.);
#75839=ORIENTED_EDGE('',*,*,#51040,.F.);
#75840=ORIENTED_EDGE('',*,*,#51083,.F.);
#75841=ORIENTED_EDGE('',*,*,#51043,.F.);
#75842=ORIENTED_EDGE('',*,*,#51049,.F.);
#75843=ORIENTED_EDGE('',*,*,#53398,.F.);
#75844=ORIENTED_EDGE('',*,*,#53399,.F.);
#75845=ORIENTED_EDGE('',*,*,#53392,.T.);
#75846=ORIENTED_EDGE('',*,*,#53400,.T.);
#75847=ORIENTED_EDGE('',*,*,#53401,.F.);
#75848=ORIENTED_EDGE('',*,*,#53402,.F.);
#75849=ORIENTED_EDGE('',*,*,#53393,.T.);
#75850=ORIENTED_EDGE('',*,*,#53399,.T.);
#75851=ORIENTED_EDGE('',*,*,#53403,.F.);
#75852=ORIENTED_EDGE('',*,*,#53404,.F.);
#75853=ORIENTED_EDGE('',*,*,#53394,.T.);
#75854=ORIENTED_EDGE('',*,*,#53402,.T.);
#75855=ORIENTED_EDGE('',*,*,#53405,.F.);
#75856=ORIENTED_EDGE('',*,*,#53406,.F.);
#75857=ORIENTED_EDGE('',*,*,#53395,.T.);
#75858=ORIENTED_EDGE('',*,*,#53404,.T.);
#75859=ORIENTED_EDGE('',*,*,#53387,.T.);
#75860=ORIENTED_EDGE('',*,*,#53406,.T.);
#75861=ORIENTED_EDGE('',*,*,#53407,.F.);
#75862=ORIENTED_EDGE('',*,*,#51066,.F.);
#75863=ORIENTED_EDGE('',*,*,#53408,.F.);
#75864=ORIENTED_EDGE('',*,*,#53409,.F.);
#75865=ORIENTED_EDGE('',*,*,#53388,.T.);
#75866=ORIENTED_EDGE('',*,*,#51068,.T.);
#75867=ORIENTED_EDGE('',*,*,#53410,.F.);
#75868=ORIENTED_EDGE('',*,*,#53411,.F.);
#75869=ORIENTED_EDGE('',*,*,#53389,.T.);
#75870=ORIENTED_EDGE('',*,*,#53409,.T.);
#75871=ORIENTED_EDGE('',*,*,#53412,.F.);
#75872=ORIENTED_EDGE('',*,*,#53413,.F.);
#75873=ORIENTED_EDGE('',*,*,#53390,.T.);
#75874=ORIENTED_EDGE('',*,*,#53411,.T.);
#75875=ORIENTED_EDGE('',*,*,#53414,.F.);
#75876=ORIENTED_EDGE('',*,*,#53400,.F.);
#75877=ORIENTED_EDGE('',*,*,#53391,.T.);
#75878=ORIENTED_EDGE('',*,*,#53413,.T.);
#75879=ORIENTED_EDGE('',*,*,#53415,.T.);
#75880=ORIENTED_EDGE('',*,*,#53347,.T.);
#75881=ORIENTED_EDGE('',*,*,#53416,.F.);
#75882=ORIENTED_EDGE('',*,*,#53417,.F.);
#75883=ORIENTED_EDGE('',*,*,#53418,.F.);
#75884=ORIENTED_EDGE('',*,*,#53359,.T.);
#75885=ORIENTED_EDGE('',*,*,#53419,.T.);
#75886=ORIENTED_EDGE('',*,*,#53420,.F.);
#75887=ORIENTED_EDGE('',*,*,#53421,.T.);
#75888=ORIENTED_EDGE('',*,*,#53416,.T.);
#75889=ORIENTED_EDGE('',*,*,#53346,.F.);
#75890=ORIENTED_EDGE('',*,*,#53372,.T.);
#75891=ORIENTED_EDGE('',*,*,#53397,.F.);
#75892=ORIENTED_EDGE('',*,*,#53377,.F.);
#75893=ORIENTED_EDGE('',*,*,#53360,.T.);
#75894=ORIENTED_EDGE('',*,*,#53418,.T.);
#75895=ORIENTED_EDGE('',*,*,#53422,.T.);
#75896=ORIENTED_EDGE('',*,*,#53357,.T.);
#75897=ORIENTED_EDGE('',*,*,#53423,.F.);
#75898=ORIENTED_EDGE('',*,*,#53306,.F.);
#75899=ORIENTED_EDGE('',*,*,#53307,.T.);
#75900=ORIENTED_EDGE('',*,*,#53423,.T.);
#75901=ORIENTED_EDGE('',*,*,#53356,.F.);
#75902=ORIENTED_EDGE('',*,*,#53383,.T.);
#75903=ORIENTED_EDGE('',*,*,#53396,.F.);
#75904=ORIENTED_EDGE('',*,*,#51053,.F.);
#75905=ORIENTED_EDGE('',*,*,#51024,.T.);
#75906=ORIENTED_EDGE('',*,*,#51086,.F.);
#75907=ORIENTED_EDGE('',*,*,#53424,.T.);
#75908=ORIENTED_EDGE('',*,*,#53337,.T.);
#75909=ORIENTED_EDGE('',*,*,#53341,.T.);
#75910=ORIENTED_EDGE('',*,*,#53314,.T.);
#75911=ORIENTED_EDGE('',*,*,#53425,.T.);
#75912=ORIENTED_EDGE('',*,*,#53300,.T.);
#75913=ORIENTED_EDGE('',*,*,#53426,.F.);
#75914=ORIENTED_EDGE('',*,*,#53348,.F.);
#75915=ORIENTED_EDGE('',*,*,#53427,.F.);
#75916=ORIENTED_EDGE('',*,*,#53343,.F.);
#75917=ORIENTED_EDGE('',*,*,#53415,.F.);
#75918=ORIENTED_EDGE('',*,*,#53428,.F.);
#75919=ORIENTED_EDGE('',*,*,#53299,.T.);
#75920=ORIENTED_EDGE('',*,*,#53386,.F.);
#75921=ORIENTED_EDGE('',*,*,#53349,.F.);
#75922=ORIENTED_EDGE('',*,*,#53426,.T.);
#75923=ORIENTED_EDGE('',*,*,#53429,.T.);
#75924=ORIENTED_EDGE('',*,*,#53430,.F.);
#75925=ORIENTED_EDGE('',*,*,#53431,.T.);
#75926=ORIENTED_EDGE('',*,*,#53286,.F.);
#75927=ORIENTED_EDGE('',*,*,#53293,.F.);
#75928=ORIENTED_EDGE('',*,*,#53290,.F.);
#75929=ORIENTED_EDGE('',*,*,#53432,.T.);
#75930=ORIENTED_EDGE('',*,*,#53433,.F.);
#75931=ORIENTED_EDGE('',*,*,#53434,.T.);
#75932=ORIENTED_EDGE('',*,*,#53435,.T.);
#75933=ORIENTED_EDGE('',*,*,#53271,.T.);
#75934=ORIENTED_EDGE('',*,*,#53272,.F.);
#75935=ORIENTED_EDGE('',*,*,#53436,.F.);
#75936=ORIENTED_EDGE('',*,*,#53429,.F.);
#75937=ORIENTED_EDGE('',*,*,#53289,.T.);
#75938=ORIENTED_EDGE('',*,*,#53381,.F.);
#75939=ORIENTED_EDGE('',*,*,#53384,.T.);
#75940=ORIENTED_EDGE('',*,*,#53354,.F.);
#75941=ORIENTED_EDGE('',*,*,#53437,.T.);
#75942=ORIENTED_EDGE('',*,*,#53362,.T.);
#75943=ORIENTED_EDGE('',*,*,#53376,.F.);
#75944=ORIENTED_EDGE('',*,*,#53378,.F.);
#75945=ORIENTED_EDGE('',*,*,#53287,.T.);
#75946=ORIENTED_EDGE('',*,*,#53431,.F.);
#75947=ORIENTED_EDGE('',*,*,#53280,.F.);
#75948=ORIENTED_EDGE('',*,*,#53283,.F.);
#75949=ORIENTED_EDGE('',*,*,#53276,.F.);
#75950=ORIENTED_EDGE('',*,*,#53438,.T.);
#75951=ORIENTED_EDGE('',*,*,#53439,.F.);
#75952=ORIENTED_EDGE('',*,*,#53440,.T.);
#75953=ORIENTED_EDGE('',*,*,#53441,.T.);
#75954=ORIENTED_EDGE('',*,*,#53442,.F.);
#75955=ORIENTED_EDGE('',*,*,#53264,.F.);
#75956=ORIENTED_EDGE('',*,*,#53267,.F.);
#75957=ORIENTED_EDGE('',*,*,#53443,.T.);
#75958=ORIENTED_EDGE('',*,*,#53438,.F.);
#75959=ORIENTED_EDGE('',*,*,#53275,.T.);
#75960=ORIENTED_EDGE('',*,*,#53370,.F.);
#75961=ORIENTED_EDGE('',*,*,#53373,.T.);
#75962=ORIENTED_EDGE('',*,*,#53344,.F.);
#75963=ORIENTED_EDGE('',*,*,#53427,.T.);
#75964=ORIENTED_EDGE('',*,*,#53352,.T.);
#75965=ORIENTED_EDGE('',*,*,#53365,.F.);
#75966=ORIENTED_EDGE('',*,*,#53367,.F.);
#75967=ORIENTED_EDGE('',*,*,#53281,.T.);
#75968=ORIENTED_EDGE('',*,*,#53440,.F.);
#75969=ORIENTED_EDGE('',*,*,#53310,.T.);
#75970=ORIENTED_EDGE('',*,*,#53324,.T.);
#75971=ORIENTED_EDGE('',*,*,#53323,.T.);
#75972=ORIENTED_EDGE('',*,*,#53312,.F.);
#75973=ORIENTED_EDGE('',*,*,#53444,.F.);
#75974=ORIENTED_EDGE('',*,*,#53419,.F.);
#75975=ORIENTED_EDGE('',*,*,#53358,.F.);
#75976=ORIENTED_EDGE('',*,*,#53437,.F.);
#75977=ORIENTED_EDGE('',*,*,#53353,.F.);
#75978=ORIENTED_EDGE('',*,*,#53422,.F.);
#75979=ORIENTED_EDGE('',*,*,#53305,.F.);
#75980=ORIENTED_EDGE('',*,*,#53322,.T.);
#75981=ORIENTED_EDGE('',*,*,#53325,.T.);
#75982=ORIENTED_EDGE('',*,*,#53328,.T.);
#75983=ORIENTED_EDGE('',*,*,#53331,.T.);
#75984=ORIENTED_EDGE('',*,*,#53336,.T.);
#75985=ORIENTED_EDGE('',*,*,#53445,.T.);
#75986=ORIENTED_EDGE('',*,*,#53446,.F.);
#75987=ORIENTED_EDGE('',*,*,#53447,.T.);
#75988=ORIENTED_EDGE('',*,*,#53448,.F.);
#75989=ORIENTED_EDGE('',*,*,#53449,.T.);
#75990=ORIENTED_EDGE('',*,*,#53450,.F.);
#75991=ORIENTED_EDGE('',*,*,#53319,.T.);
#75992=ORIENTED_EDGE('',*,*,#53295,.T.);
#75993=ORIENTED_EDGE('',*,*,#53302,.T.);
#75994=ORIENTED_EDGE('',*,*,#53451,.T.);
#75995=ORIENTED_EDGE('',*,*,#53434,.F.);
#75996=ORIENTED_EDGE('',*,*,#53452,.F.);
#75997=ORIENTED_EDGE('',*,*,#53453,.F.);
#75998=ORIENTED_EDGE('',*,*,#53454,.T.);
#75999=ORIENTED_EDGE('',*,*,#53447,.F.);
#76000=ORIENTED_EDGE('',*,*,#53455,.F.);
#76001=ORIENTED_EDGE('',*,*,#53456,.T.);
#76002=ORIENTED_EDGE('',*,*,#53457,.T.);
#76003=ORIENTED_EDGE('',*,*,#53458,.F.);
#76004=ORIENTED_EDGE('',*,*,#53445,.F.);
#76005=ORIENTED_EDGE('',*,*,#53459,.F.);
#76006=ORIENTED_EDGE('',*,*,#53460,.F.);
#76007=ORIENTED_EDGE('',*,*,#53461,.T.);
#76008=ORIENTED_EDGE('',*,*,#53338,.T.);
#76009=ORIENTED_EDGE('',*,*,#53424,.F.);
#76010=ORIENTED_EDGE('',*,*,#53462,.T.);
#76011=ORIENTED_EDGE('',*,*,#53463,.F.);
#76012=ORIENTED_EDGE('',*,*,#53449,.F.);
#76013=ORIENTED_EDGE('',*,*,#53464,.F.);
#76014=ORIENTED_EDGE('',*,*,#53301,.T.);
#76015=ORIENTED_EDGE('',*,*,#53425,.F.);
#76016=ORIENTED_EDGE('',*,*,#53317,.F.);
#76017=ORIENTED_EDGE('',*,*,#53465,.T.);
#76018=ORIENTED_EDGE('',*,*,#53303,.F.);
#76019=ORIENTED_EDGE('',*,*,#53451,.F.);
#76020=ORIENTED_EDGE('',*,*,#53265,.T.);
#76021=ORIENTED_EDGE('',*,*,#53442,.T.);
#76022=ORIENTED_EDGE('',*,*,#53466,.F.);
#76023=ORIENTED_EDGE('',*,*,#53467,.T.);
#76024=ORIENTED_EDGE('',*,*,#53432,.F.);
#76025=ORIENTED_EDGE('',*,*,#53430,.T.);
#76026=ORIENTED_EDGE('',*,*,#53436,.T.);
#76027=ORIENTED_EDGE('',*,*,#53273,.T.);
#76028=ORIENTED_EDGE('',*,*,#53269,.T.);
#76029=ORIENTED_EDGE('',*,*,#53435,.F.);
#76030=ORIENTED_EDGE('',*,*,#53453,.T.);
#76031=ORIENTED_EDGE('',*,*,#53452,.T.);
#76032=ORIENTED_EDGE('',*,*,#53433,.T.);
#76033=ORIENTED_EDGE('',*,*,#53467,.F.);
#76034=ORIENTED_EDGE('',*,*,#53468,.T.);
#76035=ORIENTED_EDGE('',*,*,#53459,.T.);
#76036=ORIENTED_EDGE('',*,*,#53446,.T.);
#76037=ORIENTED_EDGE('',*,*,#53458,.T.);
#76038=ORIENTED_EDGE('',*,*,#53469,.T.);
#76039=ORIENTED_EDGE('',*,*,#53455,.T.);
#76040=ORIENTED_EDGE('',*,*,#53448,.T.);
#76041=ORIENTED_EDGE('',*,*,#53454,.F.);
#76042=ORIENTED_EDGE('',*,*,#53470,.T.);
#76043=ORIENTED_EDGE('',*,*,#53464,.T.);
#76044=ORIENTED_EDGE('',*,*,#53450,.T.);
#76045=ORIENTED_EDGE('',*,*,#53463,.T.);
#76046=ORIENTED_EDGE('',*,*,#53471,.T.);
#76047=ORIENTED_EDGE('',*,*,#53472,.T.);
#76048=ORIENTED_EDGE('',*,*,#53460,.T.);
#76049=ORIENTED_EDGE('',*,*,#53428,.T.);
#76050=ORIENTED_EDGE('',*,*,#53417,.T.);
#76051=ORIENTED_EDGE('',*,*,#53421,.F.);
#76052=ORIENTED_EDGE('',*,*,#53420,.T.);
#76053=ORIENTED_EDGE('',*,*,#53444,.T.);
#76054=ORIENTED_EDGE('',*,*,#53335,.F.);
#76055=ORIENTED_EDGE('',*,*,#53473,.T.);
#76056=ORIENTED_EDGE('',*,*,#53439,.T.);
#76057=ORIENTED_EDGE('',*,*,#53443,.F.);
#76058=ORIENTED_EDGE('',*,*,#53268,.T.);
#76059=ORIENTED_EDGE('',*,*,#53266,.F.);
#76060=ORIENTED_EDGE('',*,*,#53466,.T.);
#76061=ORIENTED_EDGE('',*,*,#53441,.F.);
#76062=ORIENTED_EDGE('',*,*,#53474,.T.);
#76063=ORIENTED_EDGE('',*,*,#51572,.T.);
#76064=ORIENTED_EDGE('',*,*,#53475,.F.);
#76065=ORIENTED_EDGE('',*,*,#53195,.F.);
#76066=ORIENTED_EDGE('',*,*,#52902,.T.);
#76067=ORIENTED_EDGE('',*,*,#51827,.T.);
#76068=ORIENTED_EDGE('',*,*,#53476,.F.);
#76069=ORIENTED_EDGE('',*,*,#53199,.F.);
#76070=ORIENTED_EDGE('',*,*,#53476,.T.);
#76071=ORIENTED_EDGE('',*,*,#51833,.T.);
#76072=ORIENTED_EDGE('',*,*,#53477,.F.);
#76073=ORIENTED_EDGE('',*,*,#53200,.F.);
#76074=ORIENTED_EDGE('',*,*,#52890,.T.);
#76075=ORIENTED_EDGE('',*,*,#51803,.T.);
#76076=ORIENTED_EDGE('',*,*,#52886,.T.);
#76077=ORIENTED_EDGE('',*,*,#53204,.F.);
#76078=ORIENTED_EDGE('',*,*,#53478,.T.);
#76079=ORIENTED_EDGE('',*,*,#52116,.T.);
#76080=ORIENTED_EDGE('',*,*,#53479,.F.);
#76081=ORIENTED_EDGE('',*,*,#53227,.F.);
#76082=ORIENTED_EDGE('',*,*,#53479,.T.);
#76083=ORIENTED_EDGE('',*,*,#52110,.T.);
#76084=ORIENTED_EDGE('',*,*,#52778,.T.);
#76085=ORIENTED_EDGE('',*,*,#53228,.F.);
#76086=ORIENTED_EDGE('',*,*,#53480,.T.);
#76087=ORIENTED_EDGE('',*,*,#52172,.T.);
#76088=ORIENTED_EDGE('',*,*,#53481,.F.);
#76089=ORIENTED_EDGE('',*,*,#53231,.F.);
#76090=ORIENTED_EDGE('',*,*,#53482,.T.);
#76091=ORIENTED_EDGE('',*,*,#53482,.F.);
#76092=ORIENTED_EDGE('',*,*,#53483,.T.);
#76093=ORIENTED_EDGE('',*,*,#51304,.T.);
#76094=ORIENTED_EDGE('',*,*,#51300,.T.);
#76095=ORIENTED_EDGE('',*,*,#51305,.T.);
#76096=ORIENTED_EDGE('',*,*,#53483,.F.);
#76097=ORIENTED_EDGE('',*,*,#53484,.T.);
#76098=ORIENTED_EDGE('',*,*,#53484,.F.);
#76099=ORIENTED_EDGE('',*,*,#53485,.T.);
#76100=ORIENTED_EDGE('',*,*,#51308,.T.);
#76101=ORIENTED_EDGE('',*,*,#51309,.T.);
#76102=ORIENTED_EDGE('',*,*,#53485,.F.);
#76103=ORIENTED_EDGE('',*,*,#51541,.T.);
#76104=ORIENTED_EDGE('',*,*,#51327,.T.);
#76105=ORIENTED_EDGE('',*,*,#51528,.T.);
#76106=ORIENTED_EDGE('',*,*,#51532,.T.);
#76107=ORIENTED_EDGE('',*,*,#51535,.T.);
#76108=ORIENTED_EDGE('',*,*,#51537,.T.);
#76109=ORIENTED_EDGE('',*,*,#51306,.T.);
#76110=ORIENTED_EDGE('',*,*,#51529,.T.);
#76111=ORIENTED_EDGE('',*,*,#51316,.T.);
#76112=ORIENTED_EDGE('',*,*,#51550,.T.);
#76113=ORIENTED_EDGE('',*,*,#51553,.T.);
#76114=ORIENTED_EDGE('',*,*,#51339,.T.);
#76115=ORIENTED_EDGE('',*,*,#51540,.T.);
#76116=ORIENTED_EDGE('',*,*,#51551,.T.);
#76117=ORIENTED_EDGE('',*,*,#51329,.T.);
#76118=ORIENTED_EDGE('',*,*,#51552,.T.);
#76119=ORIENTED_EDGE('',*,*,#51536,.T.);
#76120=ORIENTED_EDGE('',*,*,#51499,.T.);
#76121=ORIENTED_EDGE('',*,*,#51356,.T.);
#76122=ORIENTED_EDGE('',*,*,#51485,.T.);
#76123=ORIENTED_EDGE('',*,*,#51490,.T.);
#76124=ORIENTED_EDGE('',*,*,#51492,.T.);
#76125=ORIENTED_EDGE('',*,*,#51303,.T.);
#76126=ORIENTED_EDGE('',*,*,#51491,.T.);
#76127=ORIENTED_EDGE('',*,*,#51496,.T.);
#76128=ORIENTED_EDGE('',*,*,#51486,.T.);
#76129=ORIENTED_EDGE('',*,*,#51367,.T.);
#76130=ORIENTED_EDGE('',*,*,#51548,.T.);
#76131=ORIENTED_EDGE('',*,*,#51547,.T.);
#76132=ORIENTED_EDGE('',*,*,#51354,.T.);
#76133=ORIENTED_EDGE('',*,*,#51498,.T.);
#76134=ORIENTED_EDGE('',*,*,#51549,.T.);
#76135=ORIENTED_EDGE('',*,*,#51382,.T.);
#76136=ORIENTED_EDGE('',*,*,#51546,.T.);
#76137=ORIENTED_EDGE('',*,*,#51493,.T.);
#76138=ORIENTED_EDGE('',*,*,#51515,.T.);
#76139=ORIENTED_EDGE('',*,*,#51430,.T.);
#76140=ORIENTED_EDGE('',*,*,#51436,.T.);
#76141=ORIENTED_EDGE('',*,*,#51557,.T.);
#76142=ORIENTED_EDGE('',*,*,#51434,.T.);
#76143=ORIENTED_EDGE('',*,*,#51428,.T.);
#76144=ORIENTED_EDGE('',*,*,#51527,.T.);
#76145=ORIENTED_EDGE('',*,*,#51554,.T.);
#76146=ORIENTED_EDGE('',*,*,#51556,.T.);
#76147=ORIENTED_EDGE('',*,*,#51450,.T.);
#76148=ORIENTED_EDGE('',*,*,#51555,.T.);
#76149=ORIENTED_EDGE('',*,*,#51522,.T.);
#76150=ORIENTED_EDGE('',*,*,#51543,.T.);
#76151=ORIENTED_EDGE('',*,*,#51466,.T.);
#76152=ORIENTED_EDGE('',*,*,#51473,.T.);
#76153=ORIENTED_EDGE('',*,*,#51513,.T.);
#76154=ORIENTED_EDGE('',*,*,#51501,.T.);
#76155=ORIENTED_EDGE('',*,*,#51482,.T.);
#76156=ORIENTED_EDGE('',*,*,#51477,.T.);
#76157=ORIENTED_EDGE('',*,*,#51545,.T.);
#76158=ORIENTED_EDGE('',*,*,#51544,.T.);
#76159=ORIENTED_EDGE('',*,*,#51458,.T.);
#76160=ORIENTED_EDGE('',*,*,#51542,.T.);
#76161=ORIENTED_EDGE('',*,*,#51508,.T.);
#76162=ORIENTED_EDGE('',*,*,#52598,.T.);
#76163=ORIENTED_EDGE('',*,*,#52597,.F.);
#76164=ORIENTED_EDGE('',*,*,#52596,.F.);
#76165=ORIENTED_EDGE('',*,*,#52595,.F.);
#76166=ORIENTED_EDGE('',*,*,#52594,.F.);
#76167=ORIENTED_EDGE('',*,*,#50395,.F.);
#76168=ORIENTED_EDGE('',*,*,#50440,.F.);
#76169=ORIENTED_EDGE('',*,*,#52538,.F.);
#76170=ORIENTED_EDGE('',*,*,#52537,.F.);
#76171=ORIENTED_EDGE('',*,*,#52536,.F.);
#76172=ORIENTED_EDGE('',*,*,#52535,.T.);
#76173=ORIENTED_EDGE('',*,*,#52541,.T.);
#76174=ORIENTED_EDGE('',*,*,#52540,.T.);
#76175=ORIENTED_EDGE('',*,*,#52647,.T.);
#76176=ORIENTED_EDGE('',*,*,#52604,.T.);
#76177=ORIENTED_EDGE('',*,*,#52591,.T.);
#76178=ORIENTED_EDGE('',*,*,#52590,.T.);
#76179=ORIENTED_EDGE('',*,*,#52599,.T.);
#76180=ORIENTED_EDGE('',*,*,#52654,.T.);
#76181=ORIENTED_EDGE('',*,*,#52481,.T.);
#76182=ORIENTED_EDGE('',*,*,#52480,.T.);
#76183=ORIENTED_EDGE('',*,*,#52484,.T.);
#76184=ORIENTED_EDGE('',*,*,#50288,.F.);
#76185=ORIENTED_EDGE('',*,*,#50287,.F.);
#76186=ORIENTED_EDGE('',*,*,#50292,.F.);
#76187=ORIENTED_EDGE('',*,*,#50447,.F.);
#76188=ORIENTED_EDGE('',*,*,#50427,.F.);
#76189=ORIENTED_EDGE('',*,*,#50417,.F.);
#76190=ORIENTED_EDGE('',*,*,#50416,.F.);
#76191=ORIENTED_EDGE('',*,*,#50415,.F.);
#76192=ORIENTED_EDGE('',*,*,#50420,.F.);
#76193=ORIENTED_EDGE('',*,*,#50412,.F.);
#76194=ORIENTED_EDGE('',*,*,#52621,.T.);
#76195=ORIENTED_EDGE('',*,*,#52623,.T.);
#76196=ORIENTED_EDGE('',*,*,#52622,.T.);
#76197=ORIENTED_EDGE('',*,*,#52627,.T.);
#76198=ORIENTED_EDGE('',*,*,#52626,.T.);
#76199=ORIENTED_EDGE('',*,*,#52635,.T.);
#76200=ORIENTED_EDGE('',*,*,#52650,.T.);
#76201=ORIENTED_EDGE('',*,*,#52513,.T.);
#76202=ORIENTED_EDGE('',*,*,#52512,.T.);
#76203=ORIENTED_EDGE('',*,*,#52511,.T.);
#76204=ORIENTED_EDGE('',*,*,#52510,.T.);
#76205=ORIENTED_EDGE('',*,*,#52509,.T.);
#76206=ORIENTED_EDGE('',*,*,#52508,.T.);
#76207=ORIENTED_EDGE('',*,*,#52651,.T.);
#76208=ORIENTED_EDGE('',*,*,#52575,.T.);
#76209=ORIENTED_EDGE('',*,*,#52570,.T.);
#76210=ORIENTED_EDGE('',*,*,#52569,.T.);
#76211=ORIENTED_EDGE('',*,*,#52568,.T.);
#76212=ORIENTED_EDGE('',*,*,#52567,.T.);
#76213=ORIENTED_EDGE('',*,*,#52566,.T.);
#76214=ORIENTED_EDGE('',*,*,#52565,.T.);
#76215=ORIENTED_EDGE('',*,*,#52564,.T.);
#76216=ORIENTED_EDGE('',*,*,#52558,.T.);
#76217=ORIENTED_EDGE('',*,*,#52342,.T.);
#76218=ORIENTED_EDGE('',*,*,#50156,.F.);
#76219=ORIENTED_EDGE('',*,*,#50160,.F.);
#76220=ORIENTED_EDGE('',*,*,#50163,.F.);
#76221=ORIENTED_EDGE('',*,*,#50166,.F.);
#76222=ORIENTED_EDGE('',*,*,#50169,.F.);
#76223=ORIENTED_EDGE('',*,*,#50172,.F.);
#76224=ORIENTED_EDGE('',*,*,#50175,.F.);
#76225=ORIENTED_EDGE('',*,*,#52365,.T.);
#76226=ORIENTED_EDGE('',*,*,#52363,.T.);
#76227=ORIENTED_EDGE('',*,*,#52360,.T.);
#76228=ORIENTED_EDGE('',*,*,#52357,.T.);
#76229=ORIENTED_EDGE('',*,*,#52354,.T.);
#76230=ORIENTED_EDGE('',*,*,#52351,.T.);
#76231=ORIENTED_EDGE('',*,*,#52348,.T.);
#76232=ORIENTED_EDGE('',*,*,#52345,.T.);
#76233=ORIENTED_EDGE('',*,*,#49391,.F.);
#76234=ORIENTED_EDGE('',*,*,#49397,.F.);
#76235=ORIENTED_EDGE('',*,*,#49403,.F.);
#76236=ORIENTED_EDGE('',*,*,#49409,.F.);
#76237=ORIENTED_EDGE('',*,*,#49411,.F.);
#76238=ORIENTED_EDGE('',*,*,#49407,.F.);
#76239=ORIENTED_EDGE('',*,*,#49401,.F.);
#76240=ORIENTED_EDGE('',*,*,#49395,.F.);
#76241=ORIENTED_EDGE('',*,*,#49389,.F.);
#76242=ORIENTED_EDGE('',*,*,#49383,.F.);
#76243=ORIENTED_EDGE('',*,*,#49421,.F.);
#76244=ORIENTED_EDGE('',*,*,#49427,.F.);
#76245=ORIENTED_EDGE('',*,*,#49433,.F.);
#76246=ORIENTED_EDGE('',*,*,#49435,.F.);
#76247=ORIENTED_EDGE('',*,*,#49431,.F.);
#76248=ORIENTED_EDGE('',*,*,#49425,.F.);
#76249=ORIENTED_EDGE('',*,*,#49419,.F.);
#76250=ORIENTED_EDGE('',*,*,#49413,.F.);
#76251=ORIENTED_EDGE('',*,*,#49445,.F.);
#76252=ORIENTED_EDGE('',*,*,#49451,.F.);
#76253=ORIENTED_EDGE('',*,*,#49457,.F.);
#76254=ORIENTED_EDGE('',*,*,#49459,.F.);
#76255=ORIENTED_EDGE('',*,*,#49455,.F.);
#76256=ORIENTED_EDGE('',*,*,#49449,.F.);
#76257=ORIENTED_EDGE('',*,*,#49443,.F.);
#76258=ORIENTED_EDGE('',*,*,#49437,.F.);
#76259=ORIENTED_EDGE('',*,*,#49469,.F.);
#76260=ORIENTED_EDGE('',*,*,#49475,.F.);
#76261=ORIENTED_EDGE('',*,*,#49481,.F.);
#76262=ORIENTED_EDGE('',*,*,#49483,.F.);
#76263=ORIENTED_EDGE('',*,*,#49479,.F.);
#76264=ORIENTED_EDGE('',*,*,#49473,.F.);
#76265=ORIENTED_EDGE('',*,*,#49467,.F.);
#76266=ORIENTED_EDGE('',*,*,#49462,.F.);
#76267=ORIENTED_EDGE('',*,*,#49493,.F.);
#76268=ORIENTED_EDGE('',*,*,#49499,.F.);
#76269=ORIENTED_EDGE('',*,*,#49505,.F.);
#76270=ORIENTED_EDGE('',*,*,#49511,.F.);
#76271=ORIENTED_EDGE('',*,*,#49509,.F.);
#76272=ORIENTED_EDGE('',*,*,#49503,.F.);
#76273=ORIENTED_EDGE('',*,*,#49497,.F.);
#76274=ORIENTED_EDGE('',*,*,#49491,.F.);
#76275=ORIENTED_EDGE('',*,*,#49486,.F.);
#76276=ORIENTED_EDGE('',*,*,#49520,.F.);
#76277=ORIENTED_EDGE('',*,*,#49526,.F.);
#76278=ORIENTED_EDGE('',*,*,#49532,.F.);
#76279=ORIENTED_EDGE('',*,*,#49534,.F.);
#76280=ORIENTED_EDGE('',*,*,#49530,.F.);
#76281=ORIENTED_EDGE('',*,*,#49524,.F.);
#76282=ORIENTED_EDGE('',*,*,#49518,.F.);
#76283=ORIENTED_EDGE('',*,*,#49513,.F.);
#76284=ORIENTED_EDGE('',*,*,#49544,.F.);
#76285=ORIENTED_EDGE('',*,*,#49550,.F.);
#76286=ORIENTED_EDGE('',*,*,#49556,.F.);
#76287=ORIENTED_EDGE('',*,*,#49558,.F.);
#76288=ORIENTED_EDGE('',*,*,#49554,.F.);
#76289=ORIENTED_EDGE('',*,*,#49548,.F.);
#76290=ORIENTED_EDGE('',*,*,#49542,.F.);
#76291=ORIENTED_EDGE('',*,*,#49537,.F.);
#76292=ORIENTED_EDGE('',*,*,#49568,.F.);
#76293=ORIENTED_EDGE('',*,*,#49574,.F.);
#76294=ORIENTED_EDGE('',*,*,#49580,.F.);
#76295=ORIENTED_EDGE('',*,*,#49582,.F.);
#76296=ORIENTED_EDGE('',*,*,#49578,.F.);
#76297=ORIENTED_EDGE('',*,*,#49572,.F.);
#76298=ORIENTED_EDGE('',*,*,#49566,.F.);
#76299=ORIENTED_EDGE('',*,*,#49561,.F.);
#76300=ORIENTED_EDGE('',*,*,#49592,.F.);
#76301=ORIENTED_EDGE('',*,*,#49598,.F.);
#76302=ORIENTED_EDGE('',*,*,#49604,.F.);
#76303=ORIENTED_EDGE('',*,*,#49606,.F.);
#76304=ORIENTED_EDGE('',*,*,#49602,.F.);
#76305=ORIENTED_EDGE('',*,*,#49596,.F.);
#76306=ORIENTED_EDGE('',*,*,#49590,.F.);
#76307=ORIENTED_EDGE('',*,*,#49585,.F.);
#76308=ORIENTED_EDGE('',*,*,#49616,.F.);
#76309=ORIENTED_EDGE('',*,*,#49622,.F.);
#76310=ORIENTED_EDGE('',*,*,#49628,.F.);
#76311=ORIENTED_EDGE('',*,*,#49630,.F.);
#76312=ORIENTED_EDGE('',*,*,#49626,.F.);
#76313=ORIENTED_EDGE('',*,*,#49620,.F.);
#76314=ORIENTED_EDGE('',*,*,#49614,.F.);
#76315=ORIENTED_EDGE('',*,*,#49609,.F.);
#76316=ORIENTED_EDGE('',*,*,#49640,.F.);
#76317=ORIENTED_EDGE('',*,*,#49646,.F.);
#76318=ORIENTED_EDGE('',*,*,#49652,.F.);
#76319=ORIENTED_EDGE('',*,*,#49658,.F.);
#76320=ORIENTED_EDGE('',*,*,#49660,.F.);
#76321=ORIENTED_EDGE('',*,*,#49656,.F.);
#76322=ORIENTED_EDGE('',*,*,#49650,.F.);
#76323=ORIENTED_EDGE('',*,*,#49644,.F.);
#76324=ORIENTED_EDGE('',*,*,#49638,.F.);
#76325=ORIENTED_EDGE('',*,*,#49633,.F.);
#76326=ORIENTED_EDGE('',*,*,#49670,.F.);
#76327=ORIENTED_EDGE('',*,*,#49676,.F.);
#76328=ORIENTED_EDGE('',*,*,#49682,.F.);
#76329=ORIENTED_EDGE('',*,*,#49684,.F.);
#76330=ORIENTED_EDGE('',*,*,#49680,.F.);
#76331=ORIENTED_EDGE('',*,*,#49674,.F.);
#76332=ORIENTED_EDGE('',*,*,#49668,.F.);
#76333=ORIENTED_EDGE('',*,*,#49663,.F.);
#76334=ORIENTED_EDGE('',*,*,#49694,.F.);
#76335=ORIENTED_EDGE('',*,*,#49700,.F.);
#76336=ORIENTED_EDGE('',*,*,#49706,.F.);
#76337=ORIENTED_EDGE('',*,*,#49708,.F.);
#76338=ORIENTED_EDGE('',*,*,#49704,.F.);
#76339=ORIENTED_EDGE('',*,*,#49698,.F.);
#76340=ORIENTED_EDGE('',*,*,#49692,.F.);
#76341=ORIENTED_EDGE('',*,*,#49687,.F.);
#76342=ORIENTED_EDGE('',*,*,#49718,.F.);
#76343=ORIENTED_EDGE('',*,*,#49724,.F.);
#76344=ORIENTED_EDGE('',*,*,#49730,.F.);
#76345=ORIENTED_EDGE('',*,*,#49736,.F.);
#76346=ORIENTED_EDGE('',*,*,#49738,.F.);
#76347=ORIENTED_EDGE('',*,*,#49734,.F.);
#76348=ORIENTED_EDGE('',*,*,#49728,.F.);
#76349=ORIENTED_EDGE('',*,*,#49722,.F.);
#76350=ORIENTED_EDGE('',*,*,#49716,.F.);
#76351=ORIENTED_EDGE('',*,*,#49711,.F.);
#76352=ORIENTED_EDGE('',*,*,#49748,.F.);
#76353=ORIENTED_EDGE('',*,*,#49754,.F.);
#76354=ORIENTED_EDGE('',*,*,#49760,.F.);
#76355=ORIENTED_EDGE('',*,*,#49766,.F.);
#76356=ORIENTED_EDGE('',*,*,#49768,.F.);
#76357=ORIENTED_EDGE('',*,*,#49764,.F.);
#76358=ORIENTED_EDGE('',*,*,#49758,.F.);
#76359=ORIENTED_EDGE('',*,*,#49752,.F.);
#76360=ORIENTED_EDGE('',*,*,#49746,.F.);
#76361=ORIENTED_EDGE('',*,*,#49741,.F.);
#76362=ORIENTED_EDGE('',*,*,#49778,.F.);
#76363=ORIENTED_EDGE('',*,*,#49784,.F.);
#76364=ORIENTED_EDGE('',*,*,#49790,.F.);
#76365=ORIENTED_EDGE('',*,*,#49792,.F.);
#76366=ORIENTED_EDGE('',*,*,#49788,.F.);
#76367=ORIENTED_EDGE('',*,*,#49782,.F.);
#76368=ORIENTED_EDGE('',*,*,#49776,.F.);
#76369=ORIENTED_EDGE('',*,*,#49771,.F.);
#76370=ORIENTED_EDGE('',*,*,#49802,.F.);
#76371=ORIENTED_EDGE('',*,*,#49808,.F.);
#76372=ORIENTED_EDGE('',*,*,#49814,.F.);
#76373=ORIENTED_EDGE('',*,*,#49816,.F.);
#76374=ORIENTED_EDGE('',*,*,#49812,.F.);
#76375=ORIENTED_EDGE('',*,*,#49806,.F.);
#76376=ORIENTED_EDGE('',*,*,#49800,.F.);
#76377=ORIENTED_EDGE('',*,*,#49795,.F.);
#76378=ORIENTED_EDGE('',*,*,#49826,.F.);
#76379=ORIENTED_EDGE('',*,*,#49832,.F.);
#76380=ORIENTED_EDGE('',*,*,#49838,.F.);
#76381=ORIENTED_EDGE('',*,*,#49840,.F.);
#76382=ORIENTED_EDGE('',*,*,#49836,.F.);
#76383=ORIENTED_EDGE('',*,*,#49830,.F.);
#76384=ORIENTED_EDGE('',*,*,#49824,.F.);
#76385=ORIENTED_EDGE('',*,*,#49819,.F.);
#76386=ORIENTED_EDGE('',*,*,#49850,.F.);
#76387=ORIENTED_EDGE('',*,*,#49856,.F.);
#76388=ORIENTED_EDGE('',*,*,#49862,.F.);
#76389=ORIENTED_EDGE('',*,*,#49864,.F.);
#76390=ORIENTED_EDGE('',*,*,#49860,.F.);
#76391=ORIENTED_EDGE('',*,*,#49854,.F.);
#76392=ORIENTED_EDGE('',*,*,#49848,.F.);
#76393=ORIENTED_EDGE('',*,*,#49843,.F.);
#76394=ORIENTED_EDGE('',*,*,#49874,.F.);
#76395=ORIENTED_EDGE('',*,*,#49880,.F.);
#76396=ORIENTED_EDGE('',*,*,#49886,.F.);
#76397=ORIENTED_EDGE('',*,*,#49892,.F.);
#76398=ORIENTED_EDGE('',*,*,#49888,.F.);
#76399=ORIENTED_EDGE('',*,*,#49884,.F.);
#76400=ORIENTED_EDGE('',*,*,#49878,.F.);
#76401=ORIENTED_EDGE('',*,*,#49872,.F.);
#76402=ORIENTED_EDGE('',*,*,#49867,.F.);
#76403=ORIENTED_EDGE('',*,*,#49901,.F.);
#76404=ORIENTED_EDGE('',*,*,#49907,.F.);
#76405=ORIENTED_EDGE('',*,*,#49913,.F.);
#76406=ORIENTED_EDGE('',*,*,#49915,.F.);
#76407=ORIENTED_EDGE('',*,*,#49911,.F.);
#76408=ORIENTED_EDGE('',*,*,#49905,.F.);
#76409=ORIENTED_EDGE('',*,*,#49899,.F.);
#76410=ORIENTED_EDGE('',*,*,#49894,.F.);
#76411=ORIENTED_EDGE('',*,*,#49925,.F.);
#76412=ORIENTED_EDGE('',*,*,#49931,.F.);
#76413=ORIENTED_EDGE('',*,*,#49937,.F.);
#76414=ORIENTED_EDGE('',*,*,#49943,.F.);
#76415=ORIENTED_EDGE('',*,*,#49945,.F.);
#76416=ORIENTED_EDGE('',*,*,#49941,.F.);
#76417=ORIENTED_EDGE('',*,*,#49935,.F.);
#76418=ORIENTED_EDGE('',*,*,#49929,.F.);
#76419=ORIENTED_EDGE('',*,*,#49923,.F.);
#76420=ORIENTED_EDGE('',*,*,#49918,.F.);
#76421=ORIENTED_EDGE('',*,*,#49955,.F.);
#76422=ORIENTED_EDGE('',*,*,#49961,.F.);
#76423=ORIENTED_EDGE('',*,*,#49967,.F.);
#76424=ORIENTED_EDGE('',*,*,#49969,.F.);
#76425=ORIENTED_EDGE('',*,*,#49965,.F.);
#76426=ORIENTED_EDGE('',*,*,#49959,.F.);
#76427=ORIENTED_EDGE('',*,*,#49953,.F.);
#76428=ORIENTED_EDGE('',*,*,#49948,.F.);
#76429=ORIENTED_EDGE('',*,*,#49979,.F.);
#76430=ORIENTED_EDGE('',*,*,#49985,.F.);
#76431=ORIENTED_EDGE('',*,*,#49991,.F.);
#76432=ORIENTED_EDGE('',*,*,#49997,.F.);
#76433=ORIENTED_EDGE('',*,*,#49999,.F.);
#76434=ORIENTED_EDGE('',*,*,#49995,.F.);
#76435=ORIENTED_EDGE('',*,*,#49989,.F.);
#76436=ORIENTED_EDGE('',*,*,#49983,.F.);
#76437=ORIENTED_EDGE('',*,*,#49977,.F.);
#76438=ORIENTED_EDGE('',*,*,#49972,.F.);
#76439=ORIENTED_EDGE('',*,*,#50009,.F.);
#76440=ORIENTED_EDGE('',*,*,#50015,.F.);
#76441=ORIENTED_EDGE('',*,*,#50021,.F.);
#76442=ORIENTED_EDGE('',*,*,#50023,.F.);
#76443=ORIENTED_EDGE('',*,*,#50019,.F.);
#76444=ORIENTED_EDGE('',*,*,#50013,.F.);
#76445=ORIENTED_EDGE('',*,*,#50007,.F.);
#76446=ORIENTED_EDGE('',*,*,#50002,.F.);
#76447=ORIENTED_EDGE('',*,*,#50033,.F.);
#76448=ORIENTED_EDGE('',*,*,#50039,.F.);
#76449=ORIENTED_EDGE('',*,*,#50045,.F.);
#76450=ORIENTED_EDGE('',*,*,#50047,.F.);
#76451=ORIENTED_EDGE('',*,*,#50043,.F.);
#76452=ORIENTED_EDGE('',*,*,#50037,.F.);
#76453=ORIENTED_EDGE('',*,*,#50031,.F.);
#76454=ORIENTED_EDGE('',*,*,#50026,.F.);
#76455=ORIENTED_EDGE('',*,*,#50057,.F.);
#76456=ORIENTED_EDGE('',*,*,#50063,.F.);
#76457=ORIENTED_EDGE('',*,*,#50069,.F.);
#76458=ORIENTED_EDGE('',*,*,#50071,.F.);
#76459=ORIENTED_EDGE('',*,*,#50067,.F.);
#76460=ORIENTED_EDGE('',*,*,#50061,.F.);
#76461=ORIENTED_EDGE('',*,*,#50055,.F.);
#76462=ORIENTED_EDGE('',*,*,#50050,.F.);
#76463=ORIENTED_EDGE('',*,*,#50081,.F.);
#76464=ORIENTED_EDGE('',*,*,#50087,.F.);
#76465=ORIENTED_EDGE('',*,*,#50093,.F.);
#76466=ORIENTED_EDGE('',*,*,#50095,.F.);
#76467=ORIENTED_EDGE('',*,*,#50091,.F.);
#76468=ORIENTED_EDGE('',*,*,#50085,.F.);
#76469=ORIENTED_EDGE('',*,*,#50079,.F.);
#76470=ORIENTED_EDGE('',*,*,#50074,.F.);
#76471=ORIENTED_EDGE('',*,*,#50105,.F.);
#76472=ORIENTED_EDGE('',*,*,#50111,.F.);
#76473=ORIENTED_EDGE('',*,*,#50113,.F.);
#76474=ORIENTED_EDGE('',*,*,#50109,.F.);
#76475=ORIENTED_EDGE('',*,*,#50103,.F.);
#76476=ORIENTED_EDGE('',*,*,#50098,.F.);
#76477=ORIENTED_EDGE('',*,*,#50123,.F.);
#76478=ORIENTED_EDGE('',*,*,#50129,.F.);
#76479=ORIENTED_EDGE('',*,*,#50131,.F.);
#76480=ORIENTED_EDGE('',*,*,#50127,.F.);
#76481=ORIENTED_EDGE('',*,*,#50121,.F.);
#76482=ORIENTED_EDGE('',*,*,#50115,.F.);
#76483=ORIENTED_EDGE('',*,*,#52438,.T.);
#76484=ORIENTED_EDGE('',*,*,#52433,.T.);
#76485=ORIENTED_EDGE('',*,*,#53086,.F.);
#76486=ORIENTED_EDGE('',*,*,#52409,.T.);
#76487=ORIENTED_EDGE('',*,*,#52406,.T.);
#76488=ORIENTED_EDGE('',*,*,#52403,.T.);
#76489=ORIENTED_EDGE('',*,*,#52400,.T.);
#76490=ORIENTED_EDGE('',*,*,#52397,.T.);
#76491=ORIENTED_EDGE('',*,*,#52394,.T.);
#76492=ORIENTED_EDGE('',*,*,#52391,.T.);
#76493=ORIENTED_EDGE('',*,*,#53084,.F.);
#76494=ORIENTED_EDGE('',*,*,#52387,.T.);
#76495=ORIENTED_EDGE('',*,*,#52384,.T.);
#76496=ORIENTED_EDGE('',*,*,#52381,.T.);
#76497=ORIENTED_EDGE('',*,*,#52378,.T.);
#76498=ORIENTED_EDGE('',*,*,#52373,.T.);
#76499=ORIENTED_EDGE('',*,*,#52372,.T.);
#76500=ORIENTED_EDGE('',*,*,#52369,.T.);
#76501=ORIENTED_EDGE('',*,*,#53082,.F.);
#76502=ORIENTED_EDGE('',*,*,#52431,.T.);
#76503=ORIENTED_EDGE('',*,*,#52428,.T.);
#76504=ORIENTED_EDGE('',*,*,#52425,.T.);
#76505=ORIENTED_EDGE('',*,*,#52422,.T.);
#76506=ORIENTED_EDGE('',*,*,#52417,.T.);
#76507=ORIENTED_EDGE('',*,*,#52416,.T.);
#76508=ORIENTED_EDGE('',*,*,#52413,.T.);
#76509=ORIENTED_EDGE('',*,*,#53080,.F.);
#76510=ORIENTED_EDGE('',*,*,#50222,.F.);
#76511=ORIENTED_EDGE('',*,*,#50226,.F.);
#76512=ORIENTED_EDGE('',*,*,#50228,.F.);
#76513=ORIENTED_EDGE('',*,*,#50232,.F.);
#76514=ORIENTED_EDGE('',*,*,#50235,.F.);
#76515=ORIENTED_EDGE('',*,*,#50238,.F.);
#76516=ORIENTED_EDGE('',*,*,#50241,.F.);
#76517=ORIENTED_EDGE('',*,*,#53078,.T.);
#76518=ORIENTED_EDGE('',*,*,#50178,.F.);
#76519=ORIENTED_EDGE('',*,*,#50182,.F.);
#76520=ORIENTED_EDGE('',*,*,#50184,.F.);
#76521=ORIENTED_EDGE('',*,*,#50188,.F.);
#76522=ORIENTED_EDGE('',*,*,#50191,.F.);
#76523=ORIENTED_EDGE('',*,*,#50194,.F.);
#76524=ORIENTED_EDGE('',*,*,#50197,.F.);
#76525=ORIENTED_EDGE('',*,*,#53076,.T.);
#76526=ORIENTED_EDGE('',*,*,#50200,.F.);
#76527=ORIENTED_EDGE('',*,*,#50204,.F.);
#76528=ORIENTED_EDGE('',*,*,#50207,.F.);
#76529=ORIENTED_EDGE('',*,*,#50210,.F.);
#76530=ORIENTED_EDGE('',*,*,#50213,.F.);
#76531=ORIENTED_EDGE('',*,*,#50216,.F.);
#76532=ORIENTED_EDGE('',*,*,#50219,.F.);
#76533=ORIENTED_EDGE('',*,*,#53074,.T.);
#76534=ORIENTED_EDGE('',*,*,#50246,.F.);
#76535=ORIENTED_EDGE('',*,*,#50248,.F.);
#76536=ORIENTED_EDGE('',*,*,#50251,.F.);
#76537=ORIENTED_EDGE('',*,*,#50254,.F.);
#76538=ORIENTED_EDGE('',*,*,#50257,.F.);
#76539=ORIENTED_EDGE('',*,*,#50260,.F.);
#76540=ORIENTED_EDGE('',*,*,#50263,.F.);
#76541=ORIENTED_EDGE('',*,*,#53072,.F.);
#76542=ORIENTED_EDGE('',*,*,#53088,.F.);
#76543=ORIENTED_EDGE('',*,*,#52453,.T.);
#76544=ORIENTED_EDGE('',*,*,#52450,.T.);
#76545=ORIENTED_EDGE('',*,*,#52447,.T.);
#76546=ORIENTED_EDGE('',*,*,#52444,.T.);
#76547=ORIENTED_EDGE('',*,*,#52441,.T.);
#76548=ORIENTED_EDGE('',*,*,#51567,.T.);
#76549=ORIENTED_EDGE('',*,*,#51558,.T.);
#76550=ORIENTED_EDGE('',*,*,#51563,.T.);
#76551=ORIENTED_EDGE('',*,*,#51569,.T.);
#76552=ORIENTED_EDGE('',*,*,#51575,.T.);
#76553=ORIENTED_EDGE('',*,*,#51581,.T.);
#76554=ORIENTED_EDGE('',*,*,#51587,.T.);
#76555=ORIENTED_EDGE('',*,*,#51585,.T.);
#76556=ORIENTED_EDGE('',*,*,#51579,.T.);
#76557=ORIENTED_EDGE('',*,*,#51573,.T.);
#76558=ORIENTED_EDGE('',*,*,#51597,.T.);
#76559=ORIENTED_EDGE('',*,*,#51588,.T.);
#76560=ORIENTED_EDGE('',*,*,#51593,.T.);
#76561=ORIENTED_EDGE('',*,*,#51599,.T.);
#76562=ORIENTED_EDGE('',*,*,#51605,.T.);
#76563=ORIENTED_EDGE('',*,*,#51611,.T.);
#76564=ORIENTED_EDGE('',*,*,#51609,.T.);
#76565=ORIENTED_EDGE('',*,*,#51603,.T.);
#76566=ORIENTED_EDGE('',*,*,#51621,.T.);
#76567=ORIENTED_EDGE('',*,*,#51612,.T.);
#76568=ORIENTED_EDGE('',*,*,#51617,.T.);
#76569=ORIENTED_EDGE('',*,*,#51623,.T.);
#76570=ORIENTED_EDGE('',*,*,#51629,.T.);
#76571=ORIENTED_EDGE('',*,*,#51635,.T.);
#76572=ORIENTED_EDGE('',*,*,#51633,.T.);
#76573=ORIENTED_EDGE('',*,*,#51627,.T.);
#76574=ORIENTED_EDGE('',*,*,#51645,.T.);
#76575=ORIENTED_EDGE('',*,*,#51639,.T.);
#76576=ORIENTED_EDGE('',*,*,#51641,.T.);
#76577=ORIENTED_EDGE('',*,*,#51647,.T.);
#76578=ORIENTED_EDGE('',*,*,#51653,.T.);
#76579=ORIENTED_EDGE('',*,*,#51659,.T.);
#76580=ORIENTED_EDGE('',*,*,#51657,.T.);
#76581=ORIENTED_EDGE('',*,*,#51651,.T.);
#76582=ORIENTED_EDGE('',*,*,#51669,.T.);
#76583=ORIENTED_EDGE('',*,*,#51663,.T.);
#76584=ORIENTED_EDGE('',*,*,#51665,.T.);
#76585=ORIENTED_EDGE('',*,*,#51671,.T.);
#76586=ORIENTED_EDGE('',*,*,#51677,.T.);
#76587=ORIENTED_EDGE('',*,*,#51683,.T.);
#76588=ORIENTED_EDGE('',*,*,#51685,.T.);
#76589=ORIENTED_EDGE('',*,*,#51681,.T.);
#76590=ORIENTED_EDGE('',*,*,#51675,.T.);
#76591=ORIENTED_EDGE('',*,*,#51696,.T.);
#76592=ORIENTED_EDGE('',*,*,#51690,.T.);
#76593=ORIENTED_EDGE('',*,*,#51692,.T.);
#76594=ORIENTED_EDGE('',*,*,#51698,.T.);
#76595=ORIENTED_EDGE('',*,*,#51704,.T.);
#76596=ORIENTED_EDGE('',*,*,#51710,.T.);
#76597=ORIENTED_EDGE('',*,*,#51708,.T.);
#76598=ORIENTED_EDGE('',*,*,#51702,.T.);
#76599=ORIENTED_EDGE('',*,*,#51720,.T.);
#76600=ORIENTED_EDGE('',*,*,#51714,.T.);
#76601=ORIENTED_EDGE('',*,*,#51716,.T.);
#76602=ORIENTED_EDGE('',*,*,#51722,.T.);
#76603=ORIENTED_EDGE('',*,*,#51728,.T.);
#76604=ORIENTED_EDGE('',*,*,#51734,.T.);
#76605=ORIENTED_EDGE('',*,*,#51732,.T.);
#76606=ORIENTED_EDGE('',*,*,#51726,.T.);
#76607=ORIENTED_EDGE('',*,*,#51744,.T.);
#76608=ORIENTED_EDGE('',*,*,#51738,.T.);
#76609=ORIENTED_EDGE('',*,*,#51740,.T.);
#76610=ORIENTED_EDGE('',*,*,#51746,.T.);
#76611=ORIENTED_EDGE('',*,*,#51752,.T.);
#76612=ORIENTED_EDGE('',*,*,#51758,.T.);
#76613=ORIENTED_EDGE('',*,*,#51756,.T.);
#76614=ORIENTED_EDGE('',*,*,#51750,.T.);
#76615=ORIENTED_EDGE('',*,*,#51768,.T.);
#76616=ORIENTED_EDGE('',*,*,#51762,.T.);
#76617=ORIENTED_EDGE('',*,*,#51764,.T.);
#76618=ORIENTED_EDGE('',*,*,#51770,.T.);
#76619=ORIENTED_EDGE('',*,*,#51776,.T.);
#76620=ORIENTED_EDGE('',*,*,#51782,.T.);
#76621=ORIENTED_EDGE('',*,*,#51780,.T.);
#76622=ORIENTED_EDGE('',*,*,#51774,.T.);
#76623=ORIENTED_EDGE('',*,*,#51792,.T.);
#76624=ORIENTED_EDGE('',*,*,#51786,.T.);
#76625=ORIENTED_EDGE('',*,*,#51788,.T.);
#76626=ORIENTED_EDGE('',*,*,#51794,.T.);
#76627=ORIENTED_EDGE('',*,*,#51800,.T.);
#76628=ORIENTED_EDGE('',*,*,#51806,.T.);
#76629=ORIENTED_EDGE('',*,*,#51804,.T.);
#76630=ORIENTED_EDGE('',*,*,#51798,.T.);
#76631=ORIENTED_EDGE('',*,*,#51816,.T.);
#76632=ORIENTED_EDGE('',*,*,#51810,.T.);
#76633=ORIENTED_EDGE('',*,*,#51812,.T.);
#76634=ORIENTED_EDGE('',*,*,#51818,.T.);
#76635=ORIENTED_EDGE('',*,*,#51824,.T.);
#76636=ORIENTED_EDGE('',*,*,#51830,.T.);
#76637=ORIENTED_EDGE('',*,*,#51836,.T.);
#76638=ORIENTED_EDGE('',*,*,#51834,.T.);
#76639=ORIENTED_EDGE('',*,*,#51828,.T.);
#76640=ORIENTED_EDGE('',*,*,#51822,.T.);
#76641=ORIENTED_EDGE('',*,*,#51846,.T.);
#76642=ORIENTED_EDGE('',*,*,#51840,.T.);
#76643=ORIENTED_EDGE('',*,*,#51842,.T.);
#76644=ORIENTED_EDGE('',*,*,#51848,.T.);
#76645=ORIENTED_EDGE('',*,*,#51854,.T.);
#76646=ORIENTED_EDGE('',*,*,#51860,.T.);
#76647=ORIENTED_EDGE('',*,*,#51858,.T.);
#76648=ORIENTED_EDGE('',*,*,#51852,.T.);
#76649=ORIENTED_EDGE('',*,*,#51870,.T.);
#76650=ORIENTED_EDGE('',*,*,#51864,.T.);
#76651=ORIENTED_EDGE('',*,*,#51866,.T.);
#76652=ORIENTED_EDGE('',*,*,#51872,.T.);
#76653=ORIENTED_EDGE('',*,*,#51878,.T.);
#76654=ORIENTED_EDGE('',*,*,#51884,.T.);
#76655=ORIENTED_EDGE('',*,*,#51882,.T.);
#76656=ORIENTED_EDGE('',*,*,#51876,.T.);
#76657=ORIENTED_EDGE('',*,*,#51894,.T.);
#76658=ORIENTED_EDGE('',*,*,#51888,.T.);
#76659=ORIENTED_EDGE('',*,*,#51890,.T.);
#76660=ORIENTED_EDGE('',*,*,#51896,.T.);
#76661=ORIENTED_EDGE('',*,*,#51902,.T.);
#76662=ORIENTED_EDGE('',*,*,#51908,.T.);
#76663=ORIENTED_EDGE('',*,*,#51914,.T.);
#76664=ORIENTED_EDGE('',*,*,#51912,.T.);
#76665=ORIENTED_EDGE('',*,*,#51906,.T.);
#76666=ORIENTED_EDGE('',*,*,#51900,.T.);
#76667=ORIENTED_EDGE('',*,*,#51924,.T.);
#76668=ORIENTED_EDGE('',*,*,#51918,.T.);
#76669=ORIENTED_EDGE('',*,*,#51920,.T.);
#76670=ORIENTED_EDGE('',*,*,#51926,.T.);
#76671=ORIENTED_EDGE('',*,*,#51932,.T.);
#76672=ORIENTED_EDGE('',*,*,#51938,.T.);
#76673=ORIENTED_EDGE('',*,*,#51944,.T.);
#76674=ORIENTED_EDGE('',*,*,#51942,.T.);
#76675=ORIENTED_EDGE('',*,*,#51936,.T.);
#76676=ORIENTED_EDGE('',*,*,#51930,.T.);
#76677=ORIENTED_EDGE('',*,*,#51954,.T.);
#76678=ORIENTED_EDGE('',*,*,#51948,.T.);
#76679=ORIENTED_EDGE('',*,*,#51950,.T.);
#76680=ORIENTED_EDGE('',*,*,#51956,.T.);
#76681=ORIENTED_EDGE('',*,*,#51962,.T.);
#76682=ORIENTED_EDGE('',*,*,#51968,.T.);
#76683=ORIENTED_EDGE('',*,*,#51966,.T.);
#76684=ORIENTED_EDGE('',*,*,#51960,.T.);
#76685=ORIENTED_EDGE('',*,*,#51978,.T.);
#76686=ORIENTED_EDGE('',*,*,#51972,.T.);
#76687=ORIENTED_EDGE('',*,*,#51974,.T.);
#76688=ORIENTED_EDGE('',*,*,#51980,.T.);
#76689=ORIENTED_EDGE('',*,*,#51986,.T.);
#76690=ORIENTED_EDGE('',*,*,#51992,.T.);
#76691=ORIENTED_EDGE('',*,*,#51990,.T.);
#76692=ORIENTED_EDGE('',*,*,#51984,.T.);
#76693=ORIENTED_EDGE('',*,*,#52002,.T.);
#76694=ORIENTED_EDGE('',*,*,#51996,.T.);
#76695=ORIENTED_EDGE('',*,*,#51998,.T.);
#76696=ORIENTED_EDGE('',*,*,#52004,.T.);
#76697=ORIENTED_EDGE('',*,*,#52010,.T.);
#76698=ORIENTED_EDGE('',*,*,#52016,.T.);
#76699=ORIENTED_EDGE('',*,*,#52014,.T.);
#76700=ORIENTED_EDGE('',*,*,#52008,.T.);
#76701=ORIENTED_EDGE('',*,*,#52026,.T.);
#76702=ORIENTED_EDGE('',*,*,#52020,.T.);
#76703=ORIENTED_EDGE('',*,*,#52022,.T.);
#76704=ORIENTED_EDGE('',*,*,#52028,.T.);
#76705=ORIENTED_EDGE('',*,*,#52034,.T.);
#76706=ORIENTED_EDGE('',*,*,#52040,.T.);
#76707=ORIENTED_EDGE('',*,*,#52038,.T.);
#76708=ORIENTED_EDGE('',*,*,#52032,.T.);
#76709=ORIENTED_EDGE('',*,*,#52050,.T.);
#76710=ORIENTED_EDGE('',*,*,#52044,.T.);
#76711=ORIENTED_EDGE('',*,*,#52046,.T.);
#76712=ORIENTED_EDGE('',*,*,#52052,.T.);
#76713=ORIENTED_EDGE('',*,*,#52058,.T.);
#76714=ORIENTED_EDGE('',*,*,#52063,.T.);
#76715=ORIENTED_EDGE('',*,*,#52066,.T.);
#76716=ORIENTED_EDGE('',*,*,#52062,.T.);
#76717=ORIENTED_EDGE('',*,*,#52056,.T.);
#76718=ORIENTED_EDGE('',*,*,#52077,.T.);
#76719=ORIENTED_EDGE('',*,*,#52071,.T.);
#76720=ORIENTED_EDGE('',*,*,#52073,.T.);
#76721=ORIENTED_EDGE('',*,*,#52079,.T.);
#76722=ORIENTED_EDGE('',*,*,#52085,.T.);
#76723=ORIENTED_EDGE('',*,*,#52091,.T.);
#76724=ORIENTED_EDGE('',*,*,#52089,.T.);
#76725=ORIENTED_EDGE('',*,*,#52083,.T.);
#76726=ORIENTED_EDGE('',*,*,#52101,.T.);
#76727=ORIENTED_EDGE('',*,*,#52095,.T.);
#76728=ORIENTED_EDGE('',*,*,#52097,.T.);
#76729=ORIENTED_EDGE('',*,*,#52103,.T.);
#76730=ORIENTED_EDGE('',*,*,#52109,.T.);
#76731=ORIENTED_EDGE('',*,*,#52115,.T.);
#76732=ORIENTED_EDGE('',*,*,#52121,.T.);
#76733=ORIENTED_EDGE('',*,*,#52119,.T.);
#76734=ORIENTED_EDGE('',*,*,#52113,.T.);
#76735=ORIENTED_EDGE('',*,*,#52107,.T.);
#76736=ORIENTED_EDGE('',*,*,#52131,.T.);
#76737=ORIENTED_EDGE('',*,*,#52125,.T.);
#76738=ORIENTED_EDGE('',*,*,#52127,.T.);
#76739=ORIENTED_EDGE('',*,*,#52133,.T.);
#76740=ORIENTED_EDGE('',*,*,#52139,.T.);
#76741=ORIENTED_EDGE('',*,*,#52145,.T.);
#76742=ORIENTED_EDGE('',*,*,#52143,.T.);
#76743=ORIENTED_EDGE('',*,*,#52137,.T.);
#76744=ORIENTED_EDGE('',*,*,#52155,.T.);
#76745=ORIENTED_EDGE('',*,*,#52149,.T.);
#76746=ORIENTED_EDGE('',*,*,#52151,.T.);
#76747=ORIENTED_EDGE('',*,*,#52157,.T.);
#76748=ORIENTED_EDGE('',*,*,#52163,.T.);
#76749=ORIENTED_EDGE('',*,*,#52169,.T.);
#76750=ORIENTED_EDGE('',*,*,#52175,.T.);
#76751=ORIENTED_EDGE('',*,*,#52173,.T.);
#76752=ORIENTED_EDGE('',*,*,#52167,.T.);
#76753=ORIENTED_EDGE('',*,*,#52161,.T.);
#76754=ORIENTED_EDGE('',*,*,#52185,.T.);
#76755=ORIENTED_EDGE('',*,*,#52179,.T.);
#76756=ORIENTED_EDGE('',*,*,#52181,.T.);
#76757=ORIENTED_EDGE('',*,*,#52187,.T.);
#76758=ORIENTED_EDGE('',*,*,#52193,.T.);
#76759=ORIENTED_EDGE('',*,*,#52199,.T.);
#76760=ORIENTED_EDGE('',*,*,#52197,.T.);
#76761=ORIENTED_EDGE('',*,*,#52191,.T.);
#76762=ORIENTED_EDGE('',*,*,#52209,.T.);
#76763=ORIENTED_EDGE('',*,*,#52203,.T.);
#76764=ORIENTED_EDGE('',*,*,#52205,.T.);
#76765=ORIENTED_EDGE('',*,*,#52211,.T.);
#76766=ORIENTED_EDGE('',*,*,#52217,.T.);
#76767=ORIENTED_EDGE('',*,*,#52223,.T.);
#76768=ORIENTED_EDGE('',*,*,#52221,.T.);
#76769=ORIENTED_EDGE('',*,*,#52215,.T.);
#76770=ORIENTED_EDGE('',*,*,#52233,.T.);
#76771=ORIENTED_EDGE('',*,*,#52227,.T.);
#76772=ORIENTED_EDGE('',*,*,#52229,.T.);
#76773=ORIENTED_EDGE('',*,*,#52235,.T.);
#76774=ORIENTED_EDGE('',*,*,#52241,.T.);
#76775=ORIENTED_EDGE('',*,*,#52247,.T.);
#76776=ORIENTED_EDGE('',*,*,#52245,.T.);
#76777=ORIENTED_EDGE('',*,*,#52239,.T.);
#76778=ORIENTED_EDGE('',*,*,#52257,.T.);
#76779=ORIENTED_EDGE('',*,*,#52251,.T.);
#76780=ORIENTED_EDGE('',*,*,#52253,.T.);
#76781=ORIENTED_EDGE('',*,*,#52259,.T.);
#76782=ORIENTED_EDGE('',*,*,#52265,.T.);
#76783=ORIENTED_EDGE('',*,*,#52271,.T.);
#76784=ORIENTED_EDGE('',*,*,#52269,.T.);
#76785=ORIENTED_EDGE('',*,*,#52263,.T.);
#76786=ORIENTED_EDGE('',*,*,#52281,.T.);
#76787=ORIENTED_EDGE('',*,*,#52275,.T.);
#76788=ORIENTED_EDGE('',*,*,#52277,.T.);
#76789=ORIENTED_EDGE('',*,*,#52283,.T.);
#76790=ORIENTED_EDGE('',*,*,#52289,.T.);
#76791=ORIENTED_EDGE('',*,*,#52287,.T.);
#76792=ORIENTED_EDGE('',*,*,#52299,.T.);
#76793=ORIENTED_EDGE('',*,*,#52290,.T.);
#76794=ORIENTED_EDGE('',*,*,#52295,.T.);
#76795=ORIENTED_EDGE('',*,*,#52301,.T.);
#76796=ORIENTED_EDGE('',*,*,#52307,.T.);
#76797=ORIENTED_EDGE('',*,*,#52305,.T.);
#76798=ORIENTED_EDGE('',*,*,#53486,.T.);
#76799=ORIENTED_EDGE('',*,*,#52359,.T.);
#76800=ORIENTED_EDGE('',*,*,#53487,.F.);
#76801=ORIENTED_EDGE('',*,*,#53488,.T.);
#76802=ORIENTED_EDGE('',*,*,#53489,.T.);
#76803=ORIENTED_EDGE('',*,*,#52356,.T.);
#76804=ORIENTED_EDGE('',*,*,#53486,.F.);
#76805=ORIENTED_EDGE('',*,*,#53490,.T.);
#76806=ORIENTED_EDGE('',*,*,#53491,.T.);
#76807=ORIENTED_EDGE('',*,*,#52353,.T.);
#76808=ORIENTED_EDGE('',*,*,#53489,.F.);
#76809=ORIENTED_EDGE('',*,*,#53492,.T.);
#76810=ORIENTED_EDGE('',*,*,#53493,.T.);
#76811=ORIENTED_EDGE('',*,*,#52350,.T.);
#76812=ORIENTED_EDGE('',*,*,#53491,.F.);
#76813=ORIENTED_EDGE('',*,*,#53494,.T.);
#76814=ORIENTED_EDGE('',*,*,#53495,.T.);
#76815=ORIENTED_EDGE('',*,*,#52347,.T.);
#76816=ORIENTED_EDGE('',*,*,#53493,.F.);
#76817=ORIENTED_EDGE('',*,*,#53496,.T.);
#76818=ORIENTED_EDGE('',*,*,#53497,.T.);
#76819=ORIENTED_EDGE('',*,*,#52344,.T.);
#76820=ORIENTED_EDGE('',*,*,#53495,.F.);
#76821=ORIENTED_EDGE('',*,*,#53498,.T.);
#76822=ORIENTED_EDGE('',*,*,#53499,.T.);
#76823=ORIENTED_EDGE('',*,*,#51180,.T.);
#76824=ORIENTED_EDGE('',*,*,#52341,.T.);
#76825=ORIENTED_EDGE('',*,*,#53497,.F.);
#76826=ORIENTED_EDGE('',*,*,#53500,.T.);
#76827=ORIENTED_EDGE('',*,*,#53501,.T.);
#76828=ORIENTED_EDGE('',*,*,#52364,.T.);
#76829=ORIENTED_EDGE('',*,*,#51183,.F.);
#76830=ORIENTED_EDGE('',*,*,#53487,.T.);
#76831=ORIENTED_EDGE('',*,*,#52362,.T.);
#76832=ORIENTED_EDGE('',*,*,#53501,.F.);
#76833=ORIENTED_EDGE('',*,*,#53502,.T.);
#76834=ORIENTED_EDGE('',*,*,#53503,.T.);
#76835=ORIENTED_EDGE('',*,*,#51185,.F.);
#76836=ORIENTED_EDGE('',*,*,#51198,.F.);
#76837=ORIENTED_EDGE('',*,*,#51196,.F.);
#76838=ORIENTED_EDGE('',*,*,#51194,.F.);
#76839=ORIENTED_EDGE('',*,*,#51192,.F.);
#76840=ORIENTED_EDGE('',*,*,#51190,.F.);
#76841=ORIENTED_EDGE('',*,*,#51188,.F.);
#76842=ORIENTED_EDGE('',*,*,#53504,.T.);
#76843=ORIENTED_EDGE('',*,*,#53505,.T.);
#76844=ORIENTED_EDGE('',*,*,#53506,.T.);
#76845=ORIENTED_EDGE('',*,*,#53507,.T.);
#76846=ORIENTED_EDGE('',*,*,#53508,.T.);
#76847=ORIENTED_EDGE('',*,*,#53509,.T.);
#76848=ORIENTED_EDGE('',*,*,#53510,.T.);
#76849=ORIENTED_EDGE('',*,*,#53511,.T.);
#76850=ORIENTED_EDGE('',*,*,#53500,.F.);
#76851=ORIENTED_EDGE('',*,*,#51182,.T.);
#76852=ORIENTED_EDGE('',*,*,#51170,.T.);
#76853=ORIENTED_EDGE('',*,*,#51173,.T.);
#76854=ORIENTED_EDGE('',*,*,#51175,.T.);
#76855=ORIENTED_EDGE('',*,*,#51177,.T.);
#76856=ORIENTED_EDGE('',*,*,#51179,.T.);
#76857=ORIENTED_EDGE('',*,*,#51181,.T.);
#76858=ORIENTED_EDGE('',*,*,#53499,.F.);
#76859=ORIENTED_EDGE('',*,*,#53498,.F.);
#76860=ORIENTED_EDGE('',*,*,#53496,.F.);
#76861=ORIENTED_EDGE('',*,*,#53494,.F.);
#76862=ORIENTED_EDGE('',*,*,#53492,.F.);
#76863=ORIENTED_EDGE('',*,*,#53490,.F.);
#76864=ORIENTED_EDGE('',*,*,#53488,.F.);
#76865=ORIENTED_EDGE('',*,*,#53502,.F.);
#76866=ORIENTED_EDGE('',*,*,#53512,.T.);
#76867=ORIENTED_EDGE('',*,*,#52319,.T.);
#76868=ORIENTED_EDGE('',*,*,#53513,.F.);
#76869=ORIENTED_EDGE('',*,*,#53511,.F.);
#76870=ORIENTED_EDGE('',*,*,#53513,.T.);
#76871=ORIENTED_EDGE('',*,*,#52316,.T.);
#76872=ORIENTED_EDGE('',*,*,#51186,.F.);
#76873=ORIENTED_EDGE('',*,*,#53503,.F.);
#76874=ORIENTED_EDGE('',*,*,#53504,.F.);
#76875=ORIENTED_EDGE('',*,*,#51187,.T.);
#76876=ORIENTED_EDGE('',*,*,#52339,.T.);
#76877=ORIENTED_EDGE('',*,*,#53514,.F.);
#76878=ORIENTED_EDGE('',*,*,#53514,.T.);
#76879=ORIENTED_EDGE('',*,*,#52337,.T.);
#76880=ORIENTED_EDGE('',*,*,#53515,.F.);
#76881=ORIENTED_EDGE('',*,*,#53505,.F.);
#76882=ORIENTED_EDGE('',*,*,#53515,.T.);
#76883=ORIENTED_EDGE('',*,*,#52334,.T.);
#76884=ORIENTED_EDGE('',*,*,#53516,.F.);
#76885=ORIENTED_EDGE('',*,*,#53506,.F.);
#76886=ORIENTED_EDGE('',*,*,#53516,.T.);
#76887=ORIENTED_EDGE('',*,*,#52331,.T.);
#76888=ORIENTED_EDGE('',*,*,#53517,.F.);
#76889=ORIENTED_EDGE('',*,*,#53507,.F.);
#76890=ORIENTED_EDGE('',*,*,#53517,.T.);
#76891=ORIENTED_EDGE('',*,*,#52328,.T.);
#76892=ORIENTED_EDGE('',*,*,#53518,.F.);
#76893=ORIENTED_EDGE('',*,*,#53508,.F.);
#76894=ORIENTED_EDGE('',*,*,#53518,.T.);
#76895=ORIENTED_EDGE('',*,*,#52325,.T.);
#76896=ORIENTED_EDGE('',*,*,#53519,.F.);
#76897=ORIENTED_EDGE('',*,*,#53509,.F.);
#76898=ORIENTED_EDGE('',*,*,#53519,.T.);
#76899=ORIENTED_EDGE('',*,*,#52322,.T.);
#76900=ORIENTED_EDGE('',*,*,#53512,.F.);
#76901=ORIENTED_EDGE('',*,*,#53510,.F.);
#76902=ORIENTED_EDGE('',*,*,#53520,.F.);
#76903=ORIENTED_EDGE('',*,*,#52522,.T.);
#76904=ORIENTED_EDGE('',*,*,#53521,.T.);
#76905=ORIENTED_EDGE('',*,*,#52553,.T.);
#76906=ORIENTED_EDGE('',*,*,#52550,.T.);
#76907=ORIENTED_EDGE('',*,*,#53522,.F.);
#76908=ORIENTED_EDGE('',*,*,#52528,.T.);
#76909=ORIENTED_EDGE('',*,*,#53523,.T.);
#76910=ORIENTED_EDGE('',*,*,#52613,.T.);
#76911=ORIENTED_EDGE('',*,*,#52610,.T.);
#76912=ORIENTED_EDGE('',*,*,#53524,.F.);
#76913=ORIENTED_EDGE('',*,*,#52493,.T.);
#76914=ORIENTED_EDGE('',*,*,#53525,.T.);
#76915=ORIENTED_EDGE('',*,*,#52637,.T.);
#76916=ORIENTED_EDGE('',*,*,#52640,.T.);
#76917=ORIENTED_EDGE('',*,*,#53526,.T.);
#76918=ORIENTED_EDGE('',*,*,#52499,.T.);
#76919=ORIENTED_EDGE('',*,*,#53527,.T.);
#76920=ORIENTED_EDGE('',*,*,#52584,.T.);
#76921=ORIENTED_EDGE('',*,*,#52581,.T.);
#76922=ORIENTED_EDGE('',*,*,#53528,.T.);
#76923=ORIENTED_EDGE('',*,*,#51410,.T.);
#76924=ORIENTED_EDGE('',*,*,#53529,.F.);
#76925=ORIENTED_EDGE('',*,*,#52612,.T.);
#76926=ORIENTED_EDGE('',*,*,#52615,.T.);
#76927=ORIENTED_EDGE('',*,*,#53530,.T.);
#76928=ORIENTED_EDGE('',*,*,#51407,.T.);
#76929=ORIENTED_EDGE('',*,*,#53528,.F.);
#76930=ORIENTED_EDGE('',*,*,#52618,.T.);
#76931=ORIENTED_EDGE('',*,*,#51445,.T.);
#76932=ORIENTED_EDGE('',*,*,#51451,.T.);
#76933=ORIENTED_EDGE('',*,*,#51449,.T.);
#76934=ORIENTED_EDGE('',*,*,#52542,.T.);
#76935=ORIENTED_EDGE('',*,*,#53531,.T.);
#76936=ORIENTED_EDGE('',*,*,#51404,.T.);
#76937=ORIENTED_EDGE('',*,*,#53530,.F.);
#76938=ORIENTED_EDGE('',*,*,#52546,.T.);
#76939=ORIENTED_EDGE('',*,*,#52549,.T.);
#76940=ORIENTED_EDGE('',*,*,#53532,.T.);
#76941=ORIENTED_EDGE('',*,*,#51398,.T.);
#76942=ORIENTED_EDGE('',*,*,#53533,.F.);
#76943=ORIENTED_EDGE('',*,*,#52583,.T.);
#76944=ORIENTED_EDGE('',*,*,#52586,.T.);
#76945=ORIENTED_EDGE('',*,*,#53534,.T.);
#76946=ORIENTED_EDGE('',*,*,#51395,.T.);
#76947=ORIENTED_EDGE('',*,*,#53532,.F.);
#76948=ORIENTED_EDGE('',*,*,#52588,.T.);
#76949=ORIENTED_EDGE('',*,*,#51455,.T.);
#76950=ORIENTED_EDGE('',*,*,#51457,.T.);
#76951=ORIENTED_EDGE('',*,*,#51463,.T.);
#76952=ORIENTED_EDGE('',*,*,#52646,.T.);
#76953=ORIENTED_EDGE('',*,*,#53535,.T.);
#76954=ORIENTED_EDGE('',*,*,#51392,.T.);
#76955=ORIENTED_EDGE('',*,*,#53534,.F.);
#76956=ORIENTED_EDGE('',*,*,#52644,.T.);
#76957=ORIENTED_EDGE('',*,*,#52641,.T.);
#76958=ORIENTED_EDGE('',*,*,#53529,.T.);
#76959=ORIENTED_EDGE('',*,*,#51413,.T.);
#76960=ORIENTED_EDGE('',*,*,#51208,.F.);
#76961=ORIENTED_EDGE('',*,*,#50402,.F.);
#76962=ORIENTED_EDGE('',*,*,#50397,.F.);
#76963=ORIENTED_EDGE('',*,*,#52593,.T.);
#76964=ORIENTED_EDGE('',*,*,#52607,.T.);
#76965=ORIENTED_EDGE('',*,*,#52609,.T.);
#76966=ORIENTED_EDGE('',*,*,#53536,.F.);
#76967=ORIENTED_EDGE('',*,*,#51222,.T.);
#76968=ORIENTED_EDGE('',*,*,#51220,.T.);
#76969=ORIENTED_EDGE('',*,*,#51218,.T.);
#76970=ORIENTED_EDGE('',*,*,#51216,.T.);
#76971=ORIENTED_EDGE('',*,*,#51229,.T.);
#76972=ORIENTED_EDGE('',*,*,#51227,.T.);
#76973=ORIENTED_EDGE('',*,*,#51225,.T.);
#76974=ORIENTED_EDGE('',*,*,#53537,.F.);
#76975=ORIENTED_EDGE('',*,*,#53538,.F.);
#76976=ORIENTED_EDGE('',*,*,#53539,.F.);
#76977=ORIENTED_EDGE('',*,*,#53540,.F.);
#76978=ORIENTED_EDGE('',*,*,#53541,.F.);
#76979=ORIENTED_EDGE('',*,*,#53542,.F.);
#76980=ORIENTED_EDGE('',*,*,#53543,.F.);
#76981=ORIENTED_EDGE('',*,*,#53544,.F.);
#76982=ORIENTED_EDGE('',*,*,#53410,.T.);
#76983=ORIENTED_EDGE('',*,*,#53408,.T.);
#76984=ORIENTED_EDGE('',*,*,#51067,.F.);
#76985=ORIENTED_EDGE('',*,*,#51071,.F.);
#76986=ORIENTED_EDGE('',*,*,#51074,.F.);
#76987=ORIENTED_EDGE('',*,*,#51054,.F.);
#76988=ORIENTED_EDGE('',*,*,#51058,.F.);
#76989=ORIENTED_EDGE('',*,*,#51061,.F.);
#76990=ORIENTED_EDGE('',*,*,#51064,.F.);
#76991=ORIENTED_EDGE('',*,*,#53407,.T.);
#76992=ORIENTED_EDGE('',*,*,#53405,.T.);
#76993=ORIENTED_EDGE('',*,*,#53403,.T.);
#76994=ORIENTED_EDGE('',*,*,#53401,.T.);
#76995=ORIENTED_EDGE('',*,*,#53398,.T.);
#76996=ORIENTED_EDGE('',*,*,#53414,.T.);
#76997=ORIENTED_EDGE('',*,*,#53412,.T.);
#76998=ORIENTED_EDGE('',*,*,#50268,.F.);
#76999=ORIENTED_EDGE('',*,*,#52454,.T.);
#77000=ORIENTED_EDGE('',*,*,#52458,.T.);
#77001=ORIENTED_EDGE('',*,*,#52461,.T.);
#77002=ORIENTED_EDGE('',*,*,#52464,.T.);
#77003=ORIENTED_EDGE('',*,*,#52467,.T.);
#77004=ORIENTED_EDGE('',*,*,#52470,.T.);
#77005=ORIENTED_EDGE('',*,*,#52473,.T.);
#77006=ORIENTED_EDGE('',*,*,#52476,.T.);
#77007=ORIENTED_EDGE('',*,*,#52478,.T.);
#77008=ORIENTED_EDGE('',*,*,#50286,.F.);
#77009=ORIENTED_EDGE('',*,*,#50283,.F.);
#77010=ORIENTED_EDGE('',*,*,#50280,.F.);
#77011=ORIENTED_EDGE('',*,*,#50277,.F.);
#77012=ORIENTED_EDGE('',*,*,#50274,.F.);
#77013=ORIENTED_EDGE('',*,*,#50271,.F.);
#77014=ORIENTED_EDGE('',*,*,#51393,.T.);
#77015=ORIENTED_EDGE('',*,*,#51389,.T.);
#77016=ORIENTED_EDGE('',*,*,#49218,.F.);
#77017=ORIENTED_EDGE('',*,*,#49222,.F.);
#77018=ORIENTED_EDGE('',*,*,#49225,.F.);
#77019=ORIENTED_EDGE('',*,*,#49228,.F.);
#77020=ORIENTED_EDGE('',*,*,#49231,.F.);
#77021=ORIENTED_EDGE('',*,*,#49234,.F.);
#77022=ORIENTED_EDGE('',*,*,#49237,.F.);
#77023=ORIENTED_EDGE('',*,*,#51412,.T.);
#77024=ORIENTED_EDGE('',*,*,#51411,.T.);
#77025=ORIENTED_EDGE('',*,*,#51408,.T.);
#77026=ORIENTED_EDGE('',*,*,#51405,.T.);
#77027=ORIENTED_EDGE('',*,*,#51402,.T.);
#77028=ORIENTED_EDGE('',*,*,#51399,.T.);
#77029=ORIENTED_EDGE('',*,*,#51396,.T.);
#77030=ORIENTED_EDGE('',*,*,#53545,.F.);
#77031=ORIENTED_EDGE('',*,*,#52468,.T.);
#77032=ORIENTED_EDGE('',*,*,#53546,.T.);
#77033=ORIENTED_EDGE('',*,*,#53541,.T.);
#77034=ORIENTED_EDGE('',*,*,#53546,.F.);
#77035=ORIENTED_EDGE('',*,*,#52465,.T.);
#77036=ORIENTED_EDGE('',*,*,#53547,.T.);
#77037=ORIENTED_EDGE('',*,*,#53542,.T.);
#77038=ORIENTED_EDGE('',*,*,#53547,.F.);
#77039=ORIENTED_EDGE('',*,*,#52462,.T.);
#77040=ORIENTED_EDGE('',*,*,#53548,.T.);
#77041=ORIENTED_EDGE('',*,*,#53543,.T.);
#77042=ORIENTED_EDGE('',*,*,#53548,.F.);
#77043=ORIENTED_EDGE('',*,*,#52459,.T.);
#77044=ORIENTED_EDGE('',*,*,#53549,.T.);
#77045=ORIENTED_EDGE('',*,*,#53544,.T.);
#77046=ORIENTED_EDGE('',*,*,#52455,.T.);
#77047=ORIENTED_EDGE('',*,*,#51223,.T.);
#77048=ORIENTED_EDGE('',*,*,#53536,.T.);
#77049=ORIENTED_EDGE('',*,*,#53549,.F.);
#77050=ORIENTED_EDGE('',*,*,#53537,.T.);
#77051=ORIENTED_EDGE('',*,*,#51224,.F.);
#77052=ORIENTED_EDGE('',*,*,#52479,.T.);
#77053=ORIENTED_EDGE('',*,*,#53550,.T.);
#77054=ORIENTED_EDGE('',*,*,#53550,.F.);
#77055=ORIENTED_EDGE('',*,*,#52477,.T.);
#77056=ORIENTED_EDGE('',*,*,#53551,.T.);
#77057=ORIENTED_EDGE('',*,*,#53538,.T.);
#77058=ORIENTED_EDGE('',*,*,#53551,.F.);
#77059=ORIENTED_EDGE('',*,*,#52474,.T.);
#77060=ORIENTED_EDGE('',*,*,#53552,.T.);
#77061=ORIENTED_EDGE('',*,*,#53539,.T.);
#77062=ORIENTED_EDGE('',*,*,#53552,.F.);
#77063=ORIENTED_EDGE('',*,*,#52471,.T.);
#77064=ORIENTED_EDGE('',*,*,#53545,.T.);
#77065=ORIENTED_EDGE('',*,*,#53540,.T.);
#77066=ORIENTED_EDGE('',*,*,#53521,.F.);
#77067=ORIENTED_EDGE('',*,*,#52519,.T.);
#77068=ORIENTED_EDGE('',*,*,#52649,.T.);
#77069=ORIENTED_EDGE('',*,*,#52556,.T.);
#77070=ORIENTED_EDGE('',*,*,#52652,.T.);
#77071=ORIENTED_EDGE('',*,*,#52502,.T.);
#77072=ORIENTED_EDGE('',*,*,#53526,.F.);
#77073=ORIENTED_EDGE('',*,*,#52576,.T.);
#77074=ORIENTED_EDGE('',*,*,#53533,.T.);
#77075=ORIENTED_EDGE('',*,*,#51401,.T.);
#77076=ORIENTED_EDGE('',*,*,#53531,.F.);
#77077=ORIENTED_EDGE('',*,*,#52552,.T.);
#77078=ORIENTED_EDGE('',*,*,#52555,.T.);
#77079=ORIENTED_EDGE('',*,*,#52563,.T.);
#77080=ORIENTED_EDGE('',*,*,#52578,.T.);
#77081=ORIENTED_EDGE('',*,*,#52580,.T.);
#77082=ORIENTED_EDGE('',*,*,#53525,.F.);
#77083=ORIENTED_EDGE('',*,*,#52490,.T.);
#77084=ORIENTED_EDGE('',*,*,#52653,.T.);
#77085=ORIENTED_EDGE('',*,*,#52630,.T.);
#77086=ORIENTED_EDGE('',*,*,#50414,.F.);
#77087=ORIENTED_EDGE('',*,*,#50419,.F.);
#77088=ORIENTED_EDGE('',*,*,#50425,.F.);
#77089=ORIENTED_EDGE('',*,*,#50430,.F.);
#77090=ORIENTED_EDGE('',*,*,#51214,.T.);
#77091=ORIENTED_EDGE('',*,*,#51388,.T.);
#77092=ORIENTED_EDGE('',*,*,#53535,.F.);
#77093=ORIENTED_EDGE('',*,*,#52638,.T.);
#77094=ORIENTED_EDGE('',*,*,#52632,.T.);
#77095=ORIENTED_EDGE('',*,*,#52624,.T.);
#77096=ORIENTED_EDGE('',*,*,#52619,.T.);
#77097=ORIENTED_EDGE('',*,*,#52539,.T.);
#77098=ORIENTED_EDGE('',*,*,#50342,.F.);
#77099=ORIENTED_EDGE('',*,*,#50339,.F.);
#77100=ORIENTED_EDGE('',*,*,#50336,.F.);
#77101=ORIENTED_EDGE('',*,*,#50333,.F.);
#77102=ORIENTED_EDGE('',*,*,#50330,.F.);
#77103=ORIENTED_EDGE('',*,*,#50327,.F.);
#77104=ORIENTED_EDGE('',*,*,#50324,.F.);
#77105=ORIENTED_EDGE('',*,*,#50321,.F.);
#77106=ORIENTED_EDGE('',*,*,#50313,.F.);
#77107=ORIENTED_EDGE('',*,*,#50310,.F.);
#77108=ORIENTED_EDGE('',*,*,#50307,.F.);
#77109=ORIENTED_EDGE('',*,*,#50304,.F.);
#77110=ORIENTED_EDGE('',*,*,#50301,.F.);
#77111=ORIENTED_EDGE('',*,*,#50298,.F.);
#77112=ORIENTED_EDGE('',*,*,#50295,.F.);
#77113=ORIENTED_EDGE('',*,*,#50290,.F.);
#77114=ORIENTED_EDGE('',*,*,#52483,.T.);
#77115=ORIENTED_EDGE('',*,*,#52486,.T.);
#77116=ORIENTED_EDGE('',*,*,#52489,.T.);
#77117=ORIENTED_EDGE('',*,*,#52492,.T.);
#77118=ORIENTED_EDGE('',*,*,#52495,.T.);
#77119=ORIENTED_EDGE('',*,*,#52498,.T.);
#77120=ORIENTED_EDGE('',*,*,#52501,.T.);
#77121=ORIENTED_EDGE('',*,*,#52504,.T.);
#77122=ORIENTED_EDGE('',*,*,#52507,.T.);
#77123=ORIENTED_EDGE('',*,*,#52515,.T.);
#77124=ORIENTED_EDGE('',*,*,#52518,.T.);
#77125=ORIENTED_EDGE('',*,*,#52521,.T.);
#77126=ORIENTED_EDGE('',*,*,#52524,.T.);
#77127=ORIENTED_EDGE('',*,*,#52527,.T.);
#77128=ORIENTED_EDGE('',*,*,#52530,.T.);
#77129=ORIENTED_EDGE('',*,*,#52533,.T.);
#77130=ORIENTED_EDGE('',*,*,#50136,.F.);
#77131=ORIENTED_EDGE('',*,*,#52315,.T.);
#77132=ORIENTED_EDGE('',*,*,#52318,.T.);
#77133=ORIENTED_EDGE('',*,*,#52321,.T.);
#77134=ORIENTED_EDGE('',*,*,#52324,.T.);
#77135=ORIENTED_EDGE('',*,*,#52327,.T.);
#77136=ORIENTED_EDGE('',*,*,#52330,.T.);
#77137=ORIENTED_EDGE('',*,*,#52333,.T.);
#77138=ORIENTED_EDGE('',*,*,#52336,.T.);
#77139=ORIENTED_EDGE('',*,*,#52338,.T.);
#77140=ORIENTED_EDGE('',*,*,#50154,.F.);
#77141=ORIENTED_EDGE('',*,*,#50151,.F.);
#77142=ORIENTED_EDGE('',*,*,#50148,.F.);
#77143=ORIENTED_EDGE('',*,*,#50145,.F.);
#77144=ORIENTED_EDGE('',*,*,#50142,.F.);
#77145=ORIENTED_EDGE('',*,*,#50139,.F.);
#77146=ORIENTED_EDGE('',*,*,#52648,.T.);
#77147=ORIENTED_EDGE('',*,*,#52531,.T.);
#77148=ORIENTED_EDGE('',*,*,#53522,.T.);
#77149=ORIENTED_EDGE('',*,*,#52605,.T.);
#77150=ORIENTED_EDGE('',*,*,#51512,.T.);
#77151=ORIENTED_EDGE('',*,*,#51376,.T.);
#77152=ORIENTED_EDGE('',*,*,#51381,.T.);
#77153=ORIENTED_EDGE('',*,*,#51387,.T.);
#77154=ORIENTED_EDGE('',*,*,#51500,.T.);
#77155=ORIENTED_EDGE('',*,*,#51505,.T.);
#77156=ORIENTED_EDGE('',*,*,#51507,.T.);
#77157=ORIENTED_EDGE('',*,*,#51510,.T.);
#77158=ORIENTED_EDGE('',*,*,#51484,.T.);
#77159=ORIENTED_EDGE('',*,*,#51374,.T.);
#77160=ORIENTED_EDGE('',*,*,#51368,.T.);
#77161=ORIENTED_EDGE('',*,*,#51363,.T.);
#77162=ORIENTED_EDGE('',*,*,#51357,.T.);
#77163=ORIENTED_EDGE('',*,*,#51351,.T.);
#77164=ORIENTED_EDGE('',*,*,#51353,.T.);
#77165=ORIENTED_EDGE('',*,*,#51359,.T.);
#77166=ORIENTED_EDGE('',*,*,#51478,.T.);
#77167=ORIENTED_EDGE('',*,*,#51474,.T.);
#77168=ORIENTED_EDGE('',*,*,#52589,.T.);
#77169=ORIENTED_EDGE('',*,*,#52587,.T.);
#77170=ORIENTED_EDGE('',*,*,#53527,.F.);
#77171=ORIENTED_EDGE('',*,*,#52496,.T.);
#77172=ORIENTED_EDGE('',*,*,#53524,.T.);
#77173=ORIENTED_EDGE('',*,*,#52643,.T.);
#77174=ORIENTED_EDGE('',*,*,#52645,.T.);
#77175=ORIENTED_EDGE('',*,*,#51481,.T.);
#77176=ORIENTED_EDGE('',*,*,#51330,.T.);
#77177=ORIENTED_EDGE('',*,*,#51324,.T.);
#77178=ORIENTED_EDGE('',*,*,#51414,.T.);
#77179=ORIENTED_EDGE('',*,*,#51418,.T.);
#77180=ORIENTED_EDGE('',*,*,#51514,.T.);
#77181=ORIENTED_EDGE('',*,*,#51518,.T.);
#77182=ORIENTED_EDGE('',*,*,#51521,.T.);
#77183=ORIENTED_EDGE('',*,*,#51523,.T.);
#77184=ORIENTED_EDGE('',*,*,#51526,.T.);
#77185=ORIENTED_EDGE('',*,*,#51336,.T.);
#77186=ORIENTED_EDGE('',*,*,#51415,.T.);
#77187=ORIENTED_EDGE('',*,*,#51313,.T.);
#77188=ORIENTED_EDGE('',*,*,#51315,.T.);
#77189=ORIENTED_EDGE('',*,*,#51320,.T.);
#77190=ORIENTED_EDGE('',*,*,#51326,.T.);
#77191=ORIENTED_EDGE('',*,*,#51332,.T.);
#77192=ORIENTED_EDGE('',*,*,#51338,.T.);
#77193=ORIENTED_EDGE('',*,*,#51344,.T.);
#77194=ORIENTED_EDGE('',*,*,#51420,.T.);
#77195=ORIENTED_EDGE('',*,*,#51427,.T.);
#77196=ORIENTED_EDGE('',*,*,#52617,.T.);
#77197=ORIENTED_EDGE('',*,*,#52616,.T.);
#77198=ORIENTED_EDGE('',*,*,#53523,.F.);
#77199=ORIENTED_EDGE('',*,*,#52525,.T.);
#77200=ORIENTED_EDGE('',*,*,#53520,.T.);
#77201=ORIENTED_EDGE('',*,*,#52547,.T.);
#77202=ORIENTED_EDGE('',*,*,#52543,.T.);
#77203=ORIENTED_EDGE('',*,*,#51431,.T.);
#77204=ORIENTED_EDGE('',*,*,#51425,.T.);
#77205=ORIENTED_EDGE('',*,*,#51419,.T.);
#77206=ORIENTED_EDGE('',*,*,#53477,.T.);
#77207=ORIENTED_EDGE('',*,*,#51835,.T.);
#77208=ORIENTED_EDGE('',*,*,#52898,.T.);
#77209=ORIENTED_EDGE('',*,*,#53201,.F.);
#77210=ORIENTED_EDGE('',*,*,#52878,.T.);
#77211=ORIENTED_EDGE('',*,*,#51857,.T.);
#77212=ORIENTED_EDGE('',*,*,#52874,.T.);
#77213=ORIENTED_EDGE('',*,*,#53207,.F.);
#77214=ORIENTED_EDGE('',*,*,#52866,.T.);
#77215=ORIENTED_EDGE('',*,*,#51987,.T.);
#77216=ORIENTED_EDGE('',*,*,#52862,.T.);
#77217=ORIENTED_EDGE('',*,*,#53210,.F.);
#77218=ORIENTED_EDGE('',*,*,#52854,.T.);
#77219=ORIENTED_EDGE('',*,*,#52086,.T.);
#77220=ORIENTED_EDGE('',*,*,#52850,.T.);
#77221=ORIENTED_EDGE('',*,*,#53213,.F.);
#77222=ORIENTED_EDGE('',*,*,#52782,.T.);
#77223=ORIENTED_EDGE('',*,*,#52120,.T.);
#77224=ORIENTED_EDGE('',*,*,#53478,.F.);
#77225=ORIENTED_EDGE('',*,*,#53226,.F.);
#77226=ORIENTED_EDGE('',*,*,#52728,.T.);
#77227=ORIENTED_EDGE('',*,*,#52047,.T.);
#77228=ORIENTED_EDGE('',*,*,#52724,.T.);
#77229=ORIENTED_EDGE('',*,*,#53241,.T.);
#77230=ORIENTED_EDGE('',*,*,#53019,.T.);
#77231=ORIENTED_EDGE('',*,*,#52268,.T.);
#77232=ORIENTED_EDGE('',*,*,#53015,.T.);
#77233=ORIENTED_EDGE('',*,*,#53188,.T.);
#77234=ORIENTED_EDGE('',*,*,#52671,.T.);
#77235=ORIENTED_EDGE('',*,*,#52383,.T.);
#77236=ORIENTED_EDGE('',*,*,#52667,.T.);
#77237=ORIENTED_EDGE('',*,*,#53244,.T.);
#77238=ORIENTED_EDGE('',*,*,#52665,.T.);
#77239=ORIENTED_EDGE('',*,*,#52393,.T.);
#77240=ORIENTED_EDGE('',*,*,#52661,.T.);
#77241=ORIENTED_EDGE('',*,*,#53242,.T.);
#77242=ORIENTED_EDGE('',*,*,#53013,.T.);
#77243=ORIENTED_EDGE('',*,*,#52254,.T.);
#77244=ORIENTED_EDGE('',*,*,#53021,.T.);
#77245=ORIENTED_EDGE('',*,*,#53187,.T.);
#77246=ORIENTED_EDGE('',*,*,#52995,.T.);
#77247=ORIENTED_EDGE('',*,*,#52230,.T.);
#77248=ORIENTED_EDGE('',*,*,#52991,.T.);
#77249=ORIENTED_EDGE('',*,*,#53192,.T.);
#77250=ORIENTED_EDGE('',*,*,#52716,.T.);
#77251=ORIENTED_EDGE('',*,*,#51668,.T.);
#77252=ORIENTED_EDGE('',*,*,#52712,.T.);
#77253=ORIENTED_EDGE('',*,*,#53243,.T.);
#77254=ORIENTED_EDGE('',*,*,#53010,.T.);
#77255=ORIENTED_EDGE('',*,*,#51654,.T.);
#77256=ORIENTED_EDGE('',*,*,#53006,.T.);
#77257=ORIENTED_EDGE('',*,*,#53190,.T.);
#77258=ORIENTED_EDGE('',*,*,#53004,.T.);
#77259=ORIENTED_EDGE('',*,*,#51644,.T.);
#77260=ORIENTED_EDGE('',*,*,#53000,.T.);
#77261=ORIENTED_EDGE('',*,*,#53189,.T.);
#77262=ORIENTED_EDGE('',*,*,#53025,.T.);
#77263=ORIENTED_EDGE('',*,*,#51630,.T.);
#77264=ORIENTED_EDGE('',*,*,#53033,.T.);
#77265=ORIENTED_EDGE('',*,*,#53186,.T.);
#77266=ORIENTED_EDGE('',*,*,#53032,.T.);
#77267=ORIENTED_EDGE('',*,*,#51620,.T.);
#77268=ORIENTED_EDGE('',*,*,#53027,.T.);
#77269=ORIENTED_EDGE('',*,*,#53185,.F.);
#77270=ORIENTED_EDGE('',*,*,#52989,.T.);
#77271=ORIENTED_EDGE('',*,*,#52244,.T.);
#77272=ORIENTED_EDGE('',*,*,#52997,.T.);
#77273=ORIENTED_EDGE('',*,*,#53191,.F.);
#77274=ORIENTED_EDGE('',*,*,#53163,.T.);
#77275=ORIENTED_EDGE('',*,*,#53139,.T.);
#77276=ORIENTED_EDGE('',*,*,#53553,.T.);
#77277=ORIENTED_EDGE('',*,*,#50912,.F.);
#77278=ORIENTED_EDGE('',*,*,#53554,.T.);
#77279=ORIENTED_EDGE('',*,*,#53135,.T.);
#77280=ORIENTED_EDGE('',*,*,#53172,.T.);
#77281=ORIENTED_EDGE('',*,*,#53247,.T.);
#77282=ORIENTED_EDGE('',*,*,#53297,.F.);
#77283=ORIENTED_EDGE('',*,*,#53318,.F.);
#77284=ORIENTED_EDGE('',*,*,#53304,.T.);
#77285=ORIENTED_EDGE('',*,*,#53465,.F.);
#77286=ORIENTED_EDGE('',*,*,#53316,.F.);
#77287=ORIENTED_EDGE('',*,*,#53342,.F.);
#77288=ORIENTED_EDGE('',*,*,#53339,.F.);
#77289=ORIENTED_EDGE('',*,*,#53461,.F.);
#77290=ORIENTED_EDGE('',*,*,#53472,.F.);
#77291=ORIENTED_EDGE('',*,*,#53471,.F.);
#77292=ORIENTED_EDGE('',*,*,#53462,.F.);
#77293=ORIENTED_EDGE('',*,*,#53470,.F.);
#77294=ORIENTED_EDGE('',*,*,#53456,.F.);
#77295=ORIENTED_EDGE('',*,*,#53469,.F.);
#77296=ORIENTED_EDGE('',*,*,#53457,.F.);
#77297=ORIENTED_EDGE('',*,*,#53468,.F.);
#77298=ORIENTED_EDGE('',*,*,#53473,.F.);
#77299=ORIENTED_EDGE('',*,*,#53334,.F.);
#77300=ORIENTED_EDGE('',*,*,#53332,.F.);
#77301=ORIENTED_EDGE('',*,*,#53329,.F.);
#77302=ORIENTED_EDGE('',*,*,#53326,.F.);
#77303=ORIENTED_EDGE('',*,*,#53320,.F.);
#77304=ORIENTED_EDGE('',*,*,#50995,.T.);
#77305=ORIENTED_EDGE('',*,*,#50999,.T.);
#77306=ORIENTED_EDGE('',*,*,#51002,.T.);
#77307=ORIENTED_EDGE('',*,*,#51004,.T.);
#77308=ORIENTED_EDGE('',*,*,#51142,.F.);
#77309=ORIENTED_EDGE('',*,*,#51141,.T.);
#77310=ORIENTED_EDGE('',*,*,#51128,.T.);
#77311=ORIENTED_EDGE('',*,*,#51146,.T.);
#77312=ORIENTED_EDGE('',*,*,#51126,.T.);
#77313=ORIENTED_EDGE('',*,*,#51145,.T.);
#77314=ORIENTED_EDGE('',*,*,#51133,.T.);
#77315=ORIENTED_EDGE('',*,*,#51144,.T.);
#77316=ORIENTED_EDGE('',*,*,#51143,.T.);
#77317=ORIENTED_EDGE('',*,*,#51131,.T.);
#77318=ORIENTED_EDGE('',*,*,#51008,.T.);
#77319=ORIENTED_EDGE('',*,*,#51011,.T.);
#77320=ORIENTED_EDGE('',*,*,#50991,.T.);
#77321=ORIENTED_EDGE('',*,*,#51138,.T.);
#77322=ORIENTED_EDGE('',*,*,#53136,.F.);
#77323=ORIENTED_EDGE('',*,*,#53554,.F.);
#77324=ORIENTED_EDGE('',*,*,#53249,.T.);
#77325=ORIENTED_EDGE('',*,*,#53250,.F.);
#77326=ORIENTED_EDGE('',*,*,#53253,.T.);
#77327=ORIENTED_EDGE('',*,*,#53255,.T.);
#77328=ORIENTED_EDGE('',*,*,#53257,.T.);
#77329=ORIENTED_EDGE('',*,*,#53258,.F.);
#77330=ORIENTED_EDGE('',*,*,#53261,.T.);
#77331=ORIENTED_EDGE('',*,*,#53262,.T.);
#77332=ORIENTED_EDGE('',*,*,#50955,.F.);
#77333=ORIENTED_EDGE('',*,*,#50952,.T.);
#77334=ORIENTED_EDGE('',*,*,#50949,.F.);
#77335=ORIENTED_EDGE('',*,*,#50946,.F.);
#77336=ORIENTED_EDGE('',*,*,#50943,.F.);
#77337=ORIENTED_EDGE('',*,*,#50940,.T.);
#77338=ORIENTED_EDGE('',*,*,#50937,.F.);
#77339=ORIENTED_EDGE('',*,*,#51247,.T.);
#77340=ORIENTED_EDGE('',*,*,#50910,.T.);
#77341=ORIENTED_EDGE('',*,*,#50907,.T.);
#77342=ORIENTED_EDGE('',*,*,#50913,.T.);
#77343=ORIENTED_EDGE('',*,*,#53553,.F.);
#77344=ORIENTED_EDGE('',*,*,#53138,.F.);
#77345=ORIENTED_EDGE('',*,*,#53132,.F.);
#77346=ORIENTED_EDGE('',*,*,#52962,.T.);
#77347=ORIENTED_EDGE('',*,*,#52037,.T.);
#77348=ORIENTED_EDGE('',*,*,#52958,.T.);
#77349=ORIENTED_EDGE('',*,*,#53180,.T.);
#77350=ORIENTED_EDGE('',*,*,#52971,.T.);
#77351=ORIENTED_EDGE('',*,*,#52220,.T.);
#77352=ORIENTED_EDGE('',*,*,#52967,.T.);
#77353=ORIENTED_EDGE('',*,*,#53182,.T.);
#77354=ORIENTED_EDGE('',*,*,#52692,.T.);
#77355=ORIENTED_EDGE('',*,*,#51921,.T.);
#77356=ORIENTED_EDGE('',*,*,#52688,.T.);
#77357=ORIENTED_EDGE('',*,*,#53246,.T.);
#77358=ORIENTED_EDGE('',*,*,#52956,.T.);
#77359=ORIENTED_EDGE('',*,*,#52023,.T.);
#77360=ORIENTED_EDGE('',*,*,#52952,.T.);
#77361=ORIENTED_EDGE('',*,*,#53179,.T.);
#77362=ORIENTED_EDGE('',*,*,#52701,.T.);
#77363=ORIENTED_EDGE('',*,*,#51891,.T.);
#77364=ORIENTED_EDGE('',*,*,#52697,.T.);
#77365=ORIENTED_EDGE('',*,*,#53239,.T.);
#77366=ORIENTED_EDGE('',*,*,#52686,.T.);
#77367=ORIENTED_EDGE('',*,*,#51943,.T.);
#77368=ORIENTED_EDGE('',*,*,#52694,.T.);
#77369=ORIENTED_EDGE('',*,*,#53245,.T.);
#77370=ORIENTED_EDGE('',*,*,#52950,.T.);
#77371=ORIENTED_EDGE('',*,*,#51705,.T.);
#77372=ORIENTED_EDGE('',*,*,#52946,.T.);
#77373=ORIENTED_EDGE('',*,*,#53178,.T.);
#77374=ORIENTED_EDGE('',*,*,#52707,.T.);
#77375=ORIENTED_EDGE('',*,*,#51913,.T.);
#77376=ORIENTED_EDGE('',*,*,#52703,.T.);
#77377=ORIENTED_EDGE('',*,*,#53240,.T.);
#77378=ORIENTED_EDGE('',*,*,#52965,.T.);
#77379=ORIENTED_EDGE('',*,*,#52206,.T.);
#77380=ORIENTED_EDGE('',*,*,#52973,.T.);
#77381=ORIENTED_EDGE('',*,*,#53181,.T.);
#77382=ORIENTED_EDGE('',*,*,#52923,.T.);
#77383=ORIENTED_EDGE('',*,*,#52182,.T.);
#77384=ORIENTED_EDGE('',*,*,#52919,.T.);
#77385=ORIENTED_EDGE('',*,*,#53174,.T.);
#77386=ORIENTED_EDGE('',*,*,#52944,.T.);
#77387=ORIENTED_EDGE('',*,*,#51695,.T.);
#77388=ORIENTED_EDGE('',*,*,#52940,.T.);
#77389=ORIENTED_EDGE('',*,*,#53177,.T.);
#77390=ORIENTED_EDGE('',*,*,#52938,.T.);
#77391=ORIENTED_EDGE('',*,*,#51729,.T.);
#77392=ORIENTED_EDGE('',*,*,#52934,.T.);
#77393=ORIENTED_EDGE('',*,*,#53176,.T.);
#77394=ORIENTED_EDGE('',*,*,#52932,.T.);
#77395=ORIENTED_EDGE('',*,*,#51719,.T.);
#77396=ORIENTED_EDGE('',*,*,#52928,.T.);
#77397=ORIENTED_EDGE('',*,*,#53175,.T.);
#77398=ORIENTED_EDGE('',*,*,#52977,.T.);
#77399=ORIENTED_EDGE('',*,*,#51606,.T.);
#77400=ORIENTED_EDGE('',*,*,#52985,.T.);
#77401=ORIENTED_EDGE('',*,*,#53184,.T.);
#77402=ORIENTED_EDGE('',*,*,#52984,.T.);
#77403=ORIENTED_EDGE('',*,*,#51596,.T.);
#77404=ORIENTED_EDGE('',*,*,#52979,.T.);
#77405=ORIENTED_EDGE('',*,*,#53183,.F.);
#77406=ORIENTED_EDGE('',*,*,#52912,.T.);
#77407=ORIENTED_EDGE('',*,*,#51566,.T.);
#77408=ORIENTED_EDGE('',*,*,#53474,.F.);
#77409=ORIENTED_EDGE('',*,*,#53194,.F.);
#77410=ORIENTED_EDGE('',*,*,#52917,.T.);
#77411=ORIENTED_EDGE('',*,*,#52196,.T.);
#77412=ORIENTED_EDGE('',*,*,#52925,.T.);
#77413=ORIENTED_EDGE('',*,*,#53173,.F.);
#77414=ORIENTED_EDGE('',*,*,#53481,.T.);
#77415=ORIENTED_EDGE('',*,*,#52174,.T.);
#77416=ORIENTED_EDGE('',*,*,#52769,.T.);
#77417=ORIENTED_EDGE('',*,*,#53232,.F.);
#77418=ORIENTED_EDGE('',*,*,#53475,.T.);
#77419=ORIENTED_EDGE('',*,*,#51578,.T.);
#77420=ORIENTED_EDGE('',*,*,#52907,.T.);
#77421=ORIENTED_EDGE('',*,*,#53196,.F.);
#77422=ORIENTED_EDGE('',*,*,#52738,.T.);
#77423=ORIENTED_EDGE('',*,*,#52298,.T.);
#77424=ORIENTED_EDGE('',*,*,#52733,.T.);
#77425=ORIENTED_EDGE('',*,*,#53238,.F.);
#77426=ORIENTED_EDGE('',*,*,#52773,.T.);
#77427=ORIENTED_EDGE('',*,*,#52166,.T.);
#77428=ORIENTED_EDGE('',*,*,#53480,.F.);
#77429=ORIENTED_EDGE('',*,*,#53230,.F.);
#77430=ORIENTED_EDGE('',*,*,#52830,.T.);
#77431=ORIENTED_EDGE('',*,*,#52280,.T.);
#77432=ORIENTED_EDGE('',*,*,#52826,.T.);
#77433=ORIENTED_EDGE('',*,*,#53217,.F.);
#77434=ORIENTED_EDGE('',*,*,#52821,.T.);
#77435=ORIENTED_EDGE('',*,*,#52013,.T.);
#77436=ORIENTED_EDGE('',*,*,#52817,.T.);
#77437=ORIENTED_EDGE('',*,*,#53219,.T.);
#77438=ORIENTED_EDGE('',*,*,#52851,.T.);
#77439=ORIENTED_EDGE('',*,*,#52074,.T.);
#77440=ORIENTED_EDGE('',*,*,#52847,.T.);
#77441=ORIENTED_EDGE('',*,*,#53211,.T.);
#77442=ORIENTED_EDGE('',*,*,#52839,.T.);
#77443=ORIENTED_EDGE('',*,*,#52142,.T.);
#77444=ORIENTED_EDGE('',*,*,#52835,.T.);
#77445=ORIENTED_EDGE('',*,*,#53215,.T.);
#77446=ORIENTED_EDGE('',*,*,#52785,.T.);
#77447=ORIENTED_EDGE('',*,*,#52112,.T.);
#77448=ORIENTED_EDGE('',*,*,#52781,.T.);
#77449=ORIENTED_EDGE('',*,*,#53225,.T.);
#77450=ORIENTED_EDGE('',*,*,#52809,.T.);
#77451=ORIENTED_EDGE('',*,*,#51951,.T.);
#77452=ORIENTED_EDGE('',*,*,#52805,.T.);
#77453=ORIENTED_EDGE('',*,*,#53221,.T.);
#77454=ORIENTED_EDGE('',*,*,#52863,.T.);
#77455=ORIENTED_EDGE('',*,*,#51975,.T.);
#77456=ORIENTED_EDGE('',*,*,#52859,.T.);
#77457=ORIENTED_EDGE('',*,*,#53208,.T.);
#77458=ORIENTED_EDGE('',*,*,#52815,.T.);
#77459=ORIENTED_EDGE('',*,*,#51999,.T.);
#77460=ORIENTED_EDGE('',*,*,#52811,.T.);
#77461=ORIENTED_EDGE('',*,*,#53218,.T.);
#77462=ORIENTED_EDGE('',*,*,#52845,.T.);
#77463=ORIENTED_EDGE('',*,*,#52088,.T.);
#77464=ORIENTED_EDGE('',*,*,#52853,.T.);
#77465=ORIENTED_EDGE('',*,*,#53212,.T.);
#77466=ORIENTED_EDGE('',*,*,#52797,.T.);
#77467=ORIENTED_EDGE('',*,*,#51879,.T.);
#77468=ORIENTED_EDGE('',*,*,#52793,.T.);
#77469=ORIENTED_EDGE('',*,*,#53223,.T.);
#77470=ORIENTED_EDGE('',*,*,#52875,.T.);
#77471=ORIENTED_EDGE('',*,*,#51855,.T.);
#77472=ORIENTED_EDGE('',*,*,#52871,.T.);
#77473=ORIENTED_EDGE('',*,*,#53205,.T.);
#77474=ORIENTED_EDGE('',*,*,#52803,.T.);
#77475=ORIENTED_EDGE('',*,*,#51965,.T.);
#77476=ORIENTED_EDGE('',*,*,#52799,.T.);
#77477=ORIENTED_EDGE('',*,*,#53220,.T.);
#77478=ORIENTED_EDGE('',*,*,#52857,.T.);
#77479=ORIENTED_EDGE('',*,*,#51989,.T.);
#77480=ORIENTED_EDGE('',*,*,#52865,.T.);
#77481=ORIENTED_EDGE('',*,*,#53209,.T.);
#77482=ORIENTED_EDGE('',*,*,#52761,.T.);
#77483=ORIENTED_EDGE('',*,*,#51777,.T.);
#77484=ORIENTED_EDGE('',*,*,#52757,.T.);
#77485=ORIENTED_EDGE('',*,*,#53234,.T.);
#77486=ORIENTED_EDGE('',*,*,#52887,.T.);
#77487=ORIENTED_EDGE('',*,*,#51801,.T.);
#77488=ORIENTED_EDGE('',*,*,#52883,.T.);
#77489=ORIENTED_EDGE('',*,*,#53202,.T.);
#77490=ORIENTED_EDGE('',*,*,#52791,.T.);
#77491=ORIENTED_EDGE('',*,*,#51869,.T.);
#77492=ORIENTED_EDGE('',*,*,#52787,.T.);
#77493=ORIENTED_EDGE('',*,*,#53222,.T.);
#77494=ORIENTED_EDGE('',*,*,#52869,.T.);
#77495=ORIENTED_EDGE('',*,*,#51845,.T.);
#77496=ORIENTED_EDGE('',*,*,#52877,.T.);
#77497=ORIENTED_EDGE('',*,*,#53206,.T.);
#77498=ORIENTED_EDGE('',*,*,#52833,.T.);
#77499=ORIENTED_EDGE('',*,*,#52128,.T.);
#77500=ORIENTED_EDGE('',*,*,#52841,.T.);
#77501=ORIENTED_EDGE('',*,*,#53214,.T.);
#77502=ORIENTED_EDGE('',*,*,#52779,.T.);
#77503=ORIENTED_EDGE('',*,*,#52098,.T.);
#77504=ORIENTED_EDGE('',*,*,#52775,.T.);
#77505=ORIENTED_EDGE('',*,*,#53224,.T.);
#77506=ORIENTED_EDGE('',*,*,#52767,.T.);
#77507=ORIENTED_EDGE('',*,*,#52152,.T.);
#77508=ORIENTED_EDGE('',*,*,#52763,.T.);
#77509=ORIENTED_EDGE('',*,*,#53229,.T.);
#77510=ORIENTED_EDGE('',*,*,#52824,.T.);
#77511=ORIENTED_EDGE('',*,*,#52278,.T.);
#77512=ORIENTED_EDGE('',*,*,#52829,.T.);
#77513=ORIENTED_EDGE('',*,*,#53216,.T.);
#77514=ORIENTED_EDGE('',*,*,#52755,.T.);
#77515=ORIENTED_EDGE('',*,*,#51767,.T.);
#77516=ORIENTED_EDGE('',*,*,#52751,.T.);
#77517=ORIENTED_EDGE('',*,*,#53233,.T.);
#77518=ORIENTED_EDGE('',*,*,#52881,.T.);
#77519=ORIENTED_EDGE('',*,*,#51791,.T.);
#77520=ORIENTED_EDGE('',*,*,#52889,.T.);
#77521=ORIENTED_EDGE('',*,*,#53203,.T.);
#77522=ORIENTED_EDGE('',*,*,#52749,.T.);
#77523=ORIENTED_EDGE('',*,*,#51753,.T.);
#77524=ORIENTED_EDGE('',*,*,#52745,.T.);
#77525=ORIENTED_EDGE('',*,*,#53236,.T.);
#77526=ORIENTED_EDGE('',*,*,#52899,.T.);
#77527=ORIENTED_EDGE('',*,*,#51825,.T.);
#77528=ORIENTED_EDGE('',*,*,#52895,.T.);
#77529=ORIENTED_EDGE('',*,*,#53197,.T.);
#77530=ORIENTED_EDGE('',*,*,#52743,.T.);
#77531=ORIENTED_EDGE('',*,*,#51743,.T.);
#77532=ORIENTED_EDGE('',*,*,#52739,.T.);
#77533=ORIENTED_EDGE('',*,*,#53235,.T.);
#77534=ORIENTED_EDGE('',*,*,#52893,.T.);
#77535=ORIENTED_EDGE('',*,*,#51815,.T.);
#77536=ORIENTED_EDGE('',*,*,#52901,.T.);
#77537=ORIENTED_EDGE('',*,*,#53198,.T.);
#77538=ORIENTED_EDGE('',*,*,#52905,.T.);
#77539=ORIENTED_EDGE('',*,*,#51576,.T.);
#77540=ORIENTED_EDGE('',*,*,#52913,.T.);
#77541=ORIENTED_EDGE('',*,*,#53193,.T.);
#77542=ORIENTED_EDGE('',*,*,#52734,.T.);
#77543=ORIENTED_EDGE('',*,*,#52306,.T.);
#77544=ORIENTED_EDGE('',*,*,#52730,.T.);
#77545=ORIENTED_EDGE('',*,*,#53237,.T.);
#77546=ORIENTED_EDGE('',*,*,#51168,.T.);
#77547=ORIENTED_EDGE('',*,*,#49131,.T.);
#77548=ORIENTED_EDGE('',*,*,#51164,.T.);
#77549=ORIENTED_EDGE('',*,*,#51165,.T.);
#77550=ORIENTED_EDGE('',*,*,#49133,.T.);
#77551=ORIENTED_EDGE('',*,*,#53555,.F.);
#77552=ORIENTED_EDGE('',*,*,#53556,.F.);
#77553=ORIENTED_EDGE('',*,*,#53557,.T.);
#77554=ORIENTED_EDGE('',*,*,#53558,.F.);
#77555=ORIENTED_EDGE('',*,*,#53559,.F.);
#77556=ORIENTED_EDGE('',*,*,#53560,.F.);
#77557=ORIENTED_EDGE('',*,*,#53555,.T.);
#77558=ORIENTED_EDGE('',*,*,#53561,.F.);
#77559=ORIENTED_EDGE('',*,*,#53562,.F.);
#77560=ORIENTED_EDGE('',*,*,#53563,.F.);
#77561=ORIENTED_EDGE('',*,*,#53559,.T.);
#77562=ORIENTED_EDGE('',*,*,#53564,.F.);
#77563=ORIENTED_EDGE('',*,*,#53565,.F.);
#77564=ORIENTED_EDGE('',*,*,#53566,.F.);
#77565=ORIENTED_EDGE('',*,*,#53562,.T.);
#77566=ORIENTED_EDGE('',*,*,#53567,.F.);
#77567=ORIENTED_EDGE('',*,*,#53568,.F.);
#77568=ORIENTED_EDGE('',*,*,#53569,.F.);
#77569=ORIENTED_EDGE('',*,*,#53565,.T.);
#77570=ORIENTED_EDGE('',*,*,#53570,.F.);
#77571=ORIENTED_EDGE('',*,*,#53557,.F.);
#77572=ORIENTED_EDGE('',*,*,#53571,.F.);
#77573=ORIENTED_EDGE('',*,*,#53568,.T.);
#77574=ORIENTED_EDGE('',*,*,#53572,.F.);
#77575=ORIENTED_EDGE('',*,*,#53573,.T.);
#77576=ORIENTED_EDGE('',*,*,#53566,.T.);
#77577=ORIENTED_EDGE('',*,*,#53569,.T.);
#77578=ORIENTED_EDGE('',*,*,#53571,.T.);
#77579=ORIENTED_EDGE('',*,*,#53556,.T.);
#77580=ORIENTED_EDGE('',*,*,#53560,.T.);
#77581=ORIENTED_EDGE('',*,*,#53563,.T.);
#77582=ORIENTED_EDGE('',*,*,#53573,.F.);
#77583=ORIENTED_EDGE('',*,*,#53574,.F.);
#77584=ORIENTED_EDGE('',*,*,#53558,.T.);
#77585=ORIENTED_EDGE('',*,*,#53575,.F.);
#77586=ORIENTED_EDGE('',*,*,#53561,.T.);
#77587=ORIENTED_EDGE('',*,*,#53576,.F.);
#77588=ORIENTED_EDGE('',*,*,#53564,.T.);
#77589=ORIENTED_EDGE('',*,*,#53577,.F.);
#77590=ORIENTED_EDGE('',*,*,#53567,.T.);
#77591=ORIENTED_EDGE('',*,*,#53578,.F.);
#77592=ORIENTED_EDGE('',*,*,#53570,.T.);
#77593=ORIENTED_EDGE('',*,*,#53579,.F.);
#77594=ORIENTED_EDGE('',*,*,#53572,.T.);
#77595=ORIENTED_EDGE('',*,*,#53580,.T.);
#77596=ORIENTED_EDGE('',*,*,#53581,.T.);
#77597=ORIENTED_EDGE('',*,*,#53582,.T.);
#77598=ORIENTED_EDGE('',*,*,#53583,.T.);
#77599=ORIENTED_EDGE('',*,*,#53581,.F.);
#77600=ORIENTED_EDGE('',*,*,#53584,.T.);
#77601=ORIENTED_EDGE('',*,*,#53580,.F.);
#77602=ORIENTED_EDGE('',*,*,#53579,.T.);
#77603=ORIENTED_EDGE('',*,*,#53578,.T.);
#77604=ORIENTED_EDGE('',*,*,#53577,.T.);
#77605=ORIENTED_EDGE('',*,*,#53576,.T.);
#77606=ORIENTED_EDGE('',*,*,#53575,.T.);
#77607=ORIENTED_EDGE('',*,*,#53574,.T.);
#77608=ORIENTED_EDGE('',*,*,#53584,.F.);
#77609=ORIENTED_EDGE('',*,*,#53585,.T.);
#77610=ORIENTED_EDGE('',*,*,#53582,.F.);
#77611=ORIENTED_EDGE('',*,*,#53583,.F.);
#77612=ORIENTED_EDGE('',*,*,#53585,.F.);
#77613=ORIENTED_EDGE('',*,*,#53586,.T.);
#77614=ORIENTED_EDGE('',*,*,#53587,.T.);
#77615=ORIENTED_EDGE('',*,*,#53588,.T.);
#77616=ORIENTED_EDGE('',*,*,#53589,.T.);
#77617=ORIENTED_EDGE('',*,*,#53590,.T.);
#77618=ORIENTED_EDGE('',*,*,#53591,.T.);
#77619=ORIENTED_EDGE('',*,*,#53592,.T.);
#77620=ORIENTED_EDGE('',*,*,#53587,.F.);
#77621=ORIENTED_EDGE('',*,*,#53593,.T.);
#77622=ORIENTED_EDGE('',*,*,#53594,.T.);
#77623=ORIENTED_EDGE('',*,*,#53595,.T.);
#77624=ORIENTED_EDGE('',*,*,#53588,.F.);
#77625=ORIENTED_EDGE('',*,*,#53596,.T.);
#77626=ORIENTED_EDGE('',*,*,#53597,.T.);
#77627=ORIENTED_EDGE('',*,*,#53589,.F.);
#77628=ORIENTED_EDGE('',*,*,#53598,.T.);
#77629=ORIENTED_EDGE('',*,*,#53599,.T.);
#77630=ORIENTED_EDGE('',*,*,#53590,.F.);
#77631=ORIENTED_EDGE('',*,*,#53600,.T.);
#77632=ORIENTED_EDGE('',*,*,#53601,.T.);
#77633=ORIENTED_EDGE('',*,*,#53591,.F.);
#77634=ORIENTED_EDGE('',*,*,#53602,.T.);
#77635=ORIENTED_EDGE('',*,*,#53603,.T.);
#77636=ORIENTED_EDGE('',*,*,#53586,.F.);
#77637=ORIENTED_EDGE('',*,*,#53604,.F.);
#77638=ORIENTED_EDGE('',*,*,#53605,.T.);
#77639=ORIENTED_EDGE('',*,*,#53606,.T.);
#77640=ORIENTED_EDGE('',*,*,#53607,.T.);
#77641=ORIENTED_EDGE('',*,*,#53608,.T.);
#77642=ORIENTED_EDGE('',*,*,#53609,.T.);
#77643=ORIENTED_EDGE('',*,*,#53605,.F.);
#77644=ORIENTED_EDGE('',*,*,#53610,.F.);
#77645=ORIENTED_EDGE('',*,*,#53611,.F.);
#77646=ORIENTED_EDGE('',*,*,#53606,.F.);
#77647=ORIENTED_EDGE('',*,*,#53612,.F.);
#77648=ORIENTED_EDGE('',*,*,#53613,.F.);
#77649=ORIENTED_EDGE('',*,*,#53607,.F.);
#77650=ORIENTED_EDGE('',*,*,#53614,.F.);
#77651=ORIENTED_EDGE('',*,*,#53615,.F.);
#77652=ORIENTED_EDGE('',*,*,#53608,.F.);
#77653=ORIENTED_EDGE('',*,*,#53616,.F.);
#77654=ORIENTED_EDGE('',*,*,#53617,.F.);
#77655=ORIENTED_EDGE('',*,*,#53609,.F.);
#77656=ORIENTED_EDGE('',*,*,#53618,.F.);
#77657=ORIENTED_EDGE('',*,*,#53619,.F.);
#77658=ORIENTED_EDGE('',*,*,#53620,.F.);
#77659=ORIENTED_EDGE('',*,*,#53604,.T.);
#77660=ORIENTED_EDGE('',*,*,#53621,.F.);
#77661=ORIENTED_EDGE('',*,*,#53603,.F.);
#77662=ORIENTED_EDGE('',*,*,#53622,.T.);
#77663=ORIENTED_EDGE('',*,*,#53610,.T.);
#77664=ORIENTED_EDGE('',*,*,#53620,.T.);
#77665=ORIENTED_EDGE('',*,*,#53623,.F.);
#77666=ORIENTED_EDGE('',*,*,#53593,.F.);
#77667=ORIENTED_EDGE('',*,*,#53601,.F.);
#77668=ORIENTED_EDGE('',*,*,#53624,.T.);
#77669=ORIENTED_EDGE('',*,*,#53612,.T.);
#77670=ORIENTED_EDGE('',*,*,#53611,.T.);
#77671=ORIENTED_EDGE('',*,*,#53622,.F.);
#77672=ORIENTED_EDGE('',*,*,#53602,.F.);
#77673=ORIENTED_EDGE('',*,*,#53599,.F.);
#77674=ORIENTED_EDGE('',*,*,#53625,.T.);
#77675=ORIENTED_EDGE('',*,*,#53614,.T.);
#77676=ORIENTED_EDGE('',*,*,#53613,.T.);
#77677=ORIENTED_EDGE('',*,*,#53624,.F.);
#77678=ORIENTED_EDGE('',*,*,#53600,.F.);
#77679=ORIENTED_EDGE('',*,*,#53597,.F.);
#77680=ORIENTED_EDGE('',*,*,#53626,.T.);
#77681=ORIENTED_EDGE('',*,*,#53616,.T.);
#77682=ORIENTED_EDGE('',*,*,#53615,.T.);
#77683=ORIENTED_EDGE('',*,*,#53625,.F.);
#77684=ORIENTED_EDGE('',*,*,#53598,.F.);
#77685=ORIENTED_EDGE('',*,*,#53595,.F.);
#77686=ORIENTED_EDGE('',*,*,#53627,.T.);
#77687=ORIENTED_EDGE('',*,*,#53618,.T.);
#77688=ORIENTED_EDGE('',*,*,#53617,.T.);
#77689=ORIENTED_EDGE('',*,*,#53626,.F.);
#77690=ORIENTED_EDGE('',*,*,#53596,.F.);
#77691=ORIENTED_EDGE('',*,*,#53592,.F.);
#77692=ORIENTED_EDGE('',*,*,#53623,.T.);
#77693=ORIENTED_EDGE('',*,*,#53621,.T.);
#77694=ORIENTED_EDGE('',*,*,#53619,.T.);
#77695=ORIENTED_EDGE('',*,*,#53627,.F.);
#77696=ORIENTED_EDGE('',*,*,#53594,.F.);
#77697=ORIENTED_EDGE('',*,*,#53628,.T.);
#77698=ORIENTED_EDGE('',*,*,#53629,.T.);
#77699=ORIENTED_EDGE('',*,*,#53630,.T.);
#77700=ORIENTED_EDGE('',*,*,#53631,.T.);
#77701=ORIENTED_EDGE('',*,*,#53632,.T.);
#77702=ORIENTED_EDGE('',*,*,#53633,.T.);
#77703=ORIENTED_EDGE('',*,*,#53634,.T.);
#77704=ORIENTED_EDGE('',*,*,#53629,.F.);
#77705=ORIENTED_EDGE('',*,*,#53635,.T.);
#77706=ORIENTED_EDGE('',*,*,#53636,.T.);
#77707=ORIENTED_EDGE('',*,*,#53637,.T.);
#77708=ORIENTED_EDGE('',*,*,#53630,.F.);
#77709=ORIENTED_EDGE('',*,*,#53638,.T.);
#77710=ORIENTED_EDGE('',*,*,#53639,.T.);
#77711=ORIENTED_EDGE('',*,*,#53631,.F.);
#77712=ORIENTED_EDGE('',*,*,#53640,.T.);
#77713=ORIENTED_EDGE('',*,*,#53641,.T.);
#77714=ORIENTED_EDGE('',*,*,#53632,.F.);
#77715=ORIENTED_EDGE('',*,*,#53642,.T.);
#77716=ORIENTED_EDGE('',*,*,#53643,.T.);
#77717=ORIENTED_EDGE('',*,*,#53633,.F.);
#77718=ORIENTED_EDGE('',*,*,#53644,.T.);
#77719=ORIENTED_EDGE('',*,*,#53645,.T.);
#77720=ORIENTED_EDGE('',*,*,#53628,.F.);
#77721=ORIENTED_EDGE('',*,*,#53646,.F.);
#77722=ORIENTED_EDGE('',*,*,#53647,.T.);
#77723=ORIENTED_EDGE('',*,*,#53648,.T.);
#77724=ORIENTED_EDGE('',*,*,#53649,.T.);
#77725=ORIENTED_EDGE('',*,*,#53650,.T.);
#77726=ORIENTED_EDGE('',*,*,#53651,.T.);
#77727=ORIENTED_EDGE('',*,*,#53647,.F.);
#77728=ORIENTED_EDGE('',*,*,#53652,.F.);
#77729=ORIENTED_EDGE('',*,*,#53653,.F.);
#77730=ORIENTED_EDGE('',*,*,#53648,.F.);
#77731=ORIENTED_EDGE('',*,*,#53654,.F.);
#77732=ORIENTED_EDGE('',*,*,#53655,.F.);
#77733=ORIENTED_EDGE('',*,*,#53649,.F.);
#77734=ORIENTED_EDGE('',*,*,#53656,.F.);
#77735=ORIENTED_EDGE('',*,*,#53657,.F.);
#77736=ORIENTED_EDGE('',*,*,#53650,.F.);
#77737=ORIENTED_EDGE('',*,*,#53658,.F.);
#77738=ORIENTED_EDGE('',*,*,#53659,.F.);
#77739=ORIENTED_EDGE('',*,*,#53651,.F.);
#77740=ORIENTED_EDGE('',*,*,#53660,.F.);
#77741=ORIENTED_EDGE('',*,*,#53661,.F.);
#77742=ORIENTED_EDGE('',*,*,#53662,.F.);
#77743=ORIENTED_EDGE('',*,*,#53646,.T.);
#77744=ORIENTED_EDGE('',*,*,#53663,.F.);
#77745=ORIENTED_EDGE('',*,*,#53645,.F.);
#77746=ORIENTED_EDGE('',*,*,#53664,.T.);
#77747=ORIENTED_EDGE('',*,*,#53652,.T.);
#77748=ORIENTED_EDGE('',*,*,#53662,.T.);
#77749=ORIENTED_EDGE('',*,*,#53665,.F.);
#77750=ORIENTED_EDGE('',*,*,#53635,.F.);
#77751=ORIENTED_EDGE('',*,*,#53643,.F.);
#77752=ORIENTED_EDGE('',*,*,#53666,.T.);
#77753=ORIENTED_EDGE('',*,*,#53654,.T.);
#77754=ORIENTED_EDGE('',*,*,#53653,.T.);
#77755=ORIENTED_EDGE('',*,*,#53664,.F.);
#77756=ORIENTED_EDGE('',*,*,#53644,.F.);
#77757=ORIENTED_EDGE('',*,*,#53641,.F.);
#77758=ORIENTED_EDGE('',*,*,#53667,.T.);
#77759=ORIENTED_EDGE('',*,*,#53656,.T.);
#77760=ORIENTED_EDGE('',*,*,#53655,.T.);
#77761=ORIENTED_EDGE('',*,*,#53666,.F.);
#77762=ORIENTED_EDGE('',*,*,#53642,.F.);
#77763=ORIENTED_EDGE('',*,*,#53639,.F.);
#77764=ORIENTED_EDGE('',*,*,#53668,.T.);
#77765=ORIENTED_EDGE('',*,*,#53658,.T.);
#77766=ORIENTED_EDGE('',*,*,#53657,.T.);
#77767=ORIENTED_EDGE('',*,*,#53667,.F.);
#77768=ORIENTED_EDGE('',*,*,#53640,.F.);
#77769=ORIENTED_EDGE('',*,*,#53637,.F.);
#77770=ORIENTED_EDGE('',*,*,#53669,.T.);
#77771=ORIENTED_EDGE('',*,*,#53660,.T.);
#77772=ORIENTED_EDGE('',*,*,#53659,.T.);
#77773=ORIENTED_EDGE('',*,*,#53668,.F.);
#77774=ORIENTED_EDGE('',*,*,#53638,.F.);
#77775=ORIENTED_EDGE('',*,*,#53634,.F.);
#77776=ORIENTED_EDGE('',*,*,#53665,.T.);
#77777=ORIENTED_EDGE('',*,*,#53663,.T.);
#77778=ORIENTED_EDGE('',*,*,#53661,.T.);
#77779=ORIENTED_EDGE('',*,*,#53669,.F.);
#77780=ORIENTED_EDGE('',*,*,#53636,.F.);
#77781=ORIENTED_EDGE('',*,*,#53670,.T.);
#77782=ORIENTED_EDGE('',*,*,#53671,.T.);
#77783=ORIENTED_EDGE('',*,*,#53672,.F.);
#77784=ORIENTED_EDGE('',*,*,#53673,.T.);
#77785=ORIENTED_EDGE('',*,*,#53674,.T.);
#77786=ORIENTED_EDGE('',*,*,#53675,.T.);
#77787=ORIENTED_EDGE('',*,*,#53670,.F.);
#77788=ORIENTED_EDGE('',*,*,#53676,.T.);
#77789=ORIENTED_EDGE('',*,*,#53677,.T.);
#77790=ORIENTED_EDGE('',*,*,#53678,.T.);
#77791=ORIENTED_EDGE('',*,*,#53674,.F.);
#77792=ORIENTED_EDGE('',*,*,#53679,.T.);
#77793=ORIENTED_EDGE('',*,*,#53680,.T.);
#77794=ORIENTED_EDGE('',*,*,#53681,.T.);
#77795=ORIENTED_EDGE('',*,*,#53677,.F.);
#77796=ORIENTED_EDGE('',*,*,#53682,.T.);
#77797=ORIENTED_EDGE('',*,*,#53683,.T.);
#77798=ORIENTED_EDGE('',*,*,#53684,.T.);
#77799=ORIENTED_EDGE('',*,*,#53680,.F.);
#77800=ORIENTED_EDGE('',*,*,#53685,.T.);
#77801=ORIENTED_EDGE('',*,*,#53672,.T.);
#77802=ORIENTED_EDGE('',*,*,#53686,.T.);
#77803=ORIENTED_EDGE('',*,*,#53683,.F.);
#77804=ORIENTED_EDGE('',*,*,#53687,.T.);
#77805=ORIENTED_EDGE('',*,*,#53688,.T.);
#77806=ORIENTED_EDGE('',*,*,#53679,.F.);
#77807=ORIENTED_EDGE('',*,*,#53676,.F.);
#77808=ORIENTED_EDGE('',*,*,#53673,.F.);
#77809=ORIENTED_EDGE('',*,*,#53687,.F.);
#77810=ORIENTED_EDGE('',*,*,#53685,.F.);
#77811=ORIENTED_EDGE('',*,*,#53682,.F.);
#77812=ORIENTED_EDGE('',*,*,#53688,.F.);
#77813=ORIENTED_EDGE('',*,*,#53689,.T.);
#77814=ORIENTED_EDGE('',*,*,#53671,.F.);
#77815=ORIENTED_EDGE('',*,*,#53690,.T.);
#77816=ORIENTED_EDGE('',*,*,#53675,.F.);
#77817=ORIENTED_EDGE('',*,*,#53691,.T.);
#77818=ORIENTED_EDGE('',*,*,#53678,.F.);
#77819=ORIENTED_EDGE('',*,*,#53692,.T.);
#77820=ORIENTED_EDGE('',*,*,#53681,.F.);
#77821=ORIENTED_EDGE('',*,*,#53693,.T.);
#77822=ORIENTED_EDGE('',*,*,#53684,.F.);
#77823=ORIENTED_EDGE('',*,*,#53694,.T.);
#77824=ORIENTED_EDGE('',*,*,#53686,.F.);
#77825=ORIENTED_EDGE('',*,*,#53695,.F.);
#77826=ORIENTED_EDGE('',*,*,#53696,.T.);
#77827=ORIENTED_EDGE('',*,*,#53697,.F.);
#77828=ORIENTED_EDGE('',*,*,#53698,.F.);
#77829=ORIENTED_EDGE('',*,*,#53696,.F.);
#77830=ORIENTED_EDGE('',*,*,#53699,.F.);
#77831=ORIENTED_EDGE('',*,*,#53695,.T.);
#77832=ORIENTED_EDGE('',*,*,#53694,.F.);
#77833=ORIENTED_EDGE('',*,*,#53689,.F.);
#77834=ORIENTED_EDGE('',*,*,#53690,.F.);
#77835=ORIENTED_EDGE('',*,*,#53691,.F.);
#77836=ORIENTED_EDGE('',*,*,#53692,.F.);
#77837=ORIENTED_EDGE('',*,*,#53693,.F.);
#77838=ORIENTED_EDGE('',*,*,#53699,.T.);
#77839=ORIENTED_EDGE('',*,*,#53700,.T.);
#77840=ORIENTED_EDGE('',*,*,#53697,.T.);
#77841=ORIENTED_EDGE('',*,*,#53698,.T.);
#77842=ORIENTED_EDGE('',*,*,#53700,.F.);
#77843=ORIENTED_EDGE('',*,*,#53701,.T.);
#77844=ORIENTED_EDGE('',*,*,#53702,.F.);
#77845=ORIENTED_EDGE('',*,*,#53703,.F.);
#77846=ORIENTED_EDGE('',*,*,#53704,.F.);
#77847=ORIENTED_EDGE('',*,*,#53705,.F.);
#77848=ORIENTED_EDGE('',*,*,#53706,.F.);
#77849=ORIENTED_EDGE('',*,*,#53707,.F.);
#77850=ORIENTED_EDGE('',*,*,#53708,.T.);
#77851=ORIENTED_EDGE('',*,*,#53701,.F.);
#77852=ORIENTED_EDGE('',*,*,#53708,.F.);
#77853=ORIENTED_EDGE('',*,*,#53709,.F.);
#77854=ORIENTED_EDGE('',*,*,#53710,.T.);
#77855=ORIENTED_EDGE('',*,*,#53711,.F.);
#77856=ORIENTED_EDGE('',*,*,#53712,.F.);
#77857=ORIENTED_EDGE('',*,*,#53710,.F.);
#77858=ORIENTED_EDGE('',*,*,#53713,.F.);
#77859=ORIENTED_EDGE('',*,*,#53714,.F.);
#77860=ORIENTED_EDGE('',*,*,#53715,.F.);
#77861=ORIENTED_EDGE('',*,*,#53716,.F.);
#77862=ORIENTED_EDGE('',*,*,#53702,.T.);
#77863=ORIENTED_EDGE('',*,*,#53717,.T.);
#77864=ORIENTED_EDGE('',*,*,#53716,.T.);
#77865=ORIENTED_EDGE('',*,*,#53718,.F.);
#77866=ORIENTED_EDGE('',*,*,#53703,.T.);
#77867=ORIENTED_EDGE('',*,*,#53718,.T.);
#77868=ORIENTED_EDGE('',*,*,#53715,.T.);
#77869=ORIENTED_EDGE('',*,*,#53719,.F.);
#77870=ORIENTED_EDGE('',*,*,#53704,.T.);
#77871=ORIENTED_EDGE('',*,*,#53719,.T.);
#77872=ORIENTED_EDGE('',*,*,#53714,.T.);
#77873=ORIENTED_EDGE('',*,*,#53720,.F.);
#77874=ORIENTED_EDGE('',*,*,#53705,.T.);
#77875=ORIENTED_EDGE('',*,*,#53720,.T.);
#77876=ORIENTED_EDGE('',*,*,#53713,.T.);
#77877=ORIENTED_EDGE('',*,*,#53717,.F.);
#77878=ORIENTED_EDGE('',*,*,#53721,.T.);
#77879=ORIENTED_EDGE('',*,*,#53722,.T.);
#77880=ORIENTED_EDGE('',*,*,#53723,.T.);
#77881=ORIENTED_EDGE('',*,*,#53721,.F.);
#77882=ORIENTED_EDGE('',*,*,#53723,.F.);
#77883=ORIENTED_EDGE('',*,*,#53706,.T.);
#77884=ORIENTED_EDGE('',*,*,#53707,.T.);
#77885=ORIENTED_EDGE('',*,*,#53724,.T.);
#77886=ORIENTED_EDGE('',*,*,#53711,.T.);
#77887=ORIENTED_EDGE('',*,*,#53712,.T.);
#77888=ORIENTED_EDGE('',*,*,#53724,.F.);
#77889=ORIENTED_EDGE('',*,*,#53709,.T.);
#77890=ORIENTED_EDGE('',*,*,#53722,.F.);
#77891=ORIENTED_EDGE('',*,*,#53725,.T.);
#77892=ORIENTED_EDGE('',*,*,#53726,.T.);
#77893=ORIENTED_EDGE('',*,*,#53727,.T.);
#77894=ORIENTED_EDGE('',*,*,#53726,.F.);
#77895=ORIENTED_EDGE('',*,*,#53727,.F.);
#77896=ORIENTED_EDGE('',*,*,#53728,.F.);
#77897=ORIENTED_EDGE('',*,*,#53729,.T.);
#77898=ORIENTED_EDGE('',*,*,#53725,.F.);
#77899=ORIENTED_EDGE('',*,*,#53729,.F.);
#77900=ORIENTED_EDGE('',*,*,#53730,.T.);
#77901=ORIENTED_EDGE('',*,*,#53728,.T.);
#77902=ORIENTED_EDGE('',*,*,#53731,.F.);
#77903=ORIENTED_EDGE('',*,*,#53732,.T.);
#77904=ORIENTED_EDGE('',*,*,#53730,.F.);
#77905=ORIENTED_EDGE('',*,*,#53732,.F.);
#77906=ORIENTED_EDGE('',*,*,#53731,.T.);
#77907=ORIENTED_EDGE('',*,*,#53733,.T.);
#77908=ORIENTED_EDGE('',*,*,#53734,.F.);
#77909=ORIENTED_EDGE('',*,*,#53735,.T.);
#77910=ORIENTED_EDGE('',*,*,#53736,.F.);
#77911=ORIENTED_EDGE('',*,*,#53737,.T.);
#77912=ORIENTED_EDGE('',*,*,#53738,.F.);
#77913=ORIENTED_EDGE('',*,*,#53735,.F.);
#77914=ORIENTED_EDGE('',*,*,#53739,.F.);
#77915=ORIENTED_EDGE('',*,*,#53740,.T.);
#77916=ORIENTED_EDGE('',*,*,#53741,.F.);
#77917=ORIENTED_EDGE('',*,*,#53733,.F.);
#77918=ORIENTED_EDGE('',*,*,#53742,.F.);
#77919=ORIENTED_EDGE('',*,*,#53743,.T.);
#77920=ORIENTED_EDGE('',*,*,#53744,.F.);
#77921=ORIENTED_EDGE('',*,*,#53737,.F.);
#77922=ORIENTED_EDGE('',*,*,#53745,.F.);
#77923=ORIENTED_EDGE('',*,*,#53746,.T.);
#77924=ORIENTED_EDGE('',*,*,#53747,.F.);
#77925=ORIENTED_EDGE('',*,*,#53740,.F.);
#77926=ORIENTED_EDGE('',*,*,#53748,.F.);
#77927=ORIENTED_EDGE('',*,*,#53749,.T.);
#77928=ORIENTED_EDGE('',*,*,#53750,.F.);
#77929=ORIENTED_EDGE('',*,*,#53743,.F.);
#77930=ORIENTED_EDGE('',*,*,#53751,.F.);
#77931=ORIENTED_EDGE('',*,*,#53752,.T.);
#77932=ORIENTED_EDGE('',*,*,#53753,.F.);
#77933=ORIENTED_EDGE('',*,*,#53746,.F.);
#77934=ORIENTED_EDGE('',*,*,#53754,.F.);
#77935=ORIENTED_EDGE('',*,*,#53749,.F.);
#77936=ORIENTED_EDGE('',*,*,#53755,.F.);
#77937=ORIENTED_EDGE('',*,*,#53752,.F.);
#77938=ORIENTED_EDGE('',*,*,#53756,.F.);
#77939=ORIENTED_EDGE('',*,*,#53757,.T.);
#77940=ORIENTED_EDGE('',*,*,#53754,.T.);
#77941=ORIENTED_EDGE('',*,*,#53758,.F.);
#77942=ORIENTED_EDGE('',*,*,#53759,.F.);
#77943=ORIENTED_EDGE('',*,*,#53760,.T.);
#77944=ORIENTED_EDGE('',*,*,#53756,.T.);
#77945=ORIENTED_EDGE('',*,*,#53757,.F.);
#77946=ORIENTED_EDGE('',*,*,#53761,.F.);
#77947=ORIENTED_EDGE('',*,*,#53758,.T.);
#77948=ORIENTED_EDGE('',*,*,#53748,.T.);
#77949=ORIENTED_EDGE('',*,*,#53762,.F.);
#77950=ORIENTED_EDGE('',*,*,#53763,.F.);
#77951=ORIENTED_EDGE('',*,*,#53764,.F.);
#77952=ORIENTED_EDGE('',*,*,#53765,.F.);
#77953=ORIENTED_EDGE('',*,*,#53766,.F.);
#77954=ORIENTED_EDGE('',*,*,#53767,.F.);
#77955=ORIENTED_EDGE('',*,*,#53768,.F.);
#77956=ORIENTED_EDGE('',*,*,#53769,.F.);
#77957=ORIENTED_EDGE('',*,*,#53770,.F.);
#77958=ORIENTED_EDGE('',*,*,#53771,.T.);
#77959=ORIENTED_EDGE('',*,*,#53772,.T.);
#77960=ORIENTED_EDGE('',*,*,#53773,.T.);
#77961=ORIENTED_EDGE('',*,*,#53774,.F.);
#77962=ORIENTED_EDGE('',*,*,#53765,.T.);
#77963=ORIENTED_EDGE('',*,*,#53770,.T.);
#77964=ORIENTED_EDGE('',*,*,#53775,.T.);
#77965=ORIENTED_EDGE('',*,*,#53776,.F.);
#77966=ORIENTED_EDGE('',*,*,#53777,.T.);
#77967=ORIENTED_EDGE('',*,*,#53774,.T.);
#77968=ORIENTED_EDGE('',*,*,#53778,.T.);
#77969=ORIENTED_EDGE('',*,*,#53766,.T.);
#77970=ORIENTED_EDGE('',*,*,#53777,.F.);
#77971=ORIENTED_EDGE('',*,*,#53779,.T.);
#77972=ORIENTED_EDGE('',*,*,#53780,.F.);
#77973=ORIENTED_EDGE('',*,*,#53781,.F.);
#77974=ORIENTED_EDGE('',*,*,#53782,.T.);
#77975=ORIENTED_EDGE('',*,*,#53783,.T.);
#77976=ORIENTED_EDGE('',*,*,#53780,.T.);
#77977=ORIENTED_EDGE('',*,*,#53784,.F.);
#77978=ORIENTED_EDGE('',*,*,#53785,.T.);
#77979=ORIENTED_EDGE('',*,*,#53786,.T.);
#77980=ORIENTED_EDGE('',*,*,#53787,.T.);
#77981=ORIENTED_EDGE('',*,*,#53783,.F.);
#77982=ORIENTED_EDGE('',*,*,#53788,.T.);
#77983=ORIENTED_EDGE('',*,*,#53784,.T.);
#77984=ORIENTED_EDGE('',*,*,#53767,.T.);
#77985=ORIENTED_EDGE('',*,*,#53789,.T.);
#77986=ORIENTED_EDGE('',*,*,#53771,.F.);
#77987=ORIENTED_EDGE('',*,*,#53764,.T.);
#77988=ORIENTED_EDGE('',*,*,#53787,.F.);
#77989=ORIENTED_EDGE('',*,*,#53790,.F.);
#77990=ORIENTED_EDGE('',*,*,#53791,.T.);
#77991=ORIENTED_EDGE('',*,*,#53792,.F.);
#77992=ORIENTED_EDGE('',*,*,#53793,.T.);
#77993=ORIENTED_EDGE('',*,*,#53794,.T.);
#77994=ORIENTED_EDGE('',*,*,#53795,.F.);
#77995=ORIENTED_EDGE('',*,*,#53796,.F.);
#77996=ORIENTED_EDGE('',*,*,#53797,.F.);
#77997=ORIENTED_EDGE('',*,*,#53796,.T.);
#77998=ORIENTED_EDGE('',*,*,#53791,.F.);
#77999=ORIENTED_EDGE('',*,*,#53798,.F.);
#78000=ORIENTED_EDGE('',*,*,#53799,.F.);
#78001=ORIENTED_EDGE('',*,*,#53800,.T.);
#78002=ORIENTED_EDGE('',*,*,#53801,.F.);
#78003=ORIENTED_EDGE('',*,*,#53794,.F.);
#78004=ORIENTED_EDGE('',*,*,#53802,.F.);
#78005=ORIENTED_EDGE('',*,*,#53803,.F.);
#78006=ORIENTED_EDGE('',*,*,#53801,.T.);
#78007=ORIENTED_EDGE('',*,*,#53804,.F.);
#78008=ORIENTED_EDGE('',*,*,#53805,.T.);
#78009=ORIENTED_EDGE('',*,*,#53806,.T.);
#78010=ORIENTED_EDGE('',*,*,#53807,.F.);
#78011=ORIENTED_EDGE('',*,*,#53808,.F.);
#78012=ORIENTED_EDGE('',*,*,#53805,.F.);
#78013=ORIENTED_EDGE('',*,*,#53808,.T.);
#78014=ORIENTED_EDGE('',*,*,#53809,.F.);
#78015=ORIENTED_EDGE('',*,*,#53810,.F.);
#78016=ORIENTED_EDGE('',*,*,#53811,.F.);
#78017=ORIENTED_EDGE('',*,*,#53810,.T.);
#78018=ORIENTED_EDGE('',*,*,#53812,.F.);
#78019=ORIENTED_EDGE('',*,*,#53813,.F.);
#78020=ORIENTED_EDGE('',*,*,#53793,.F.);
#78021=ORIENTED_EDGE('',*,*,#53792,.T.);
#78022=ORIENTED_EDGE('',*,*,#53795,.T.);
#78023=ORIENTED_EDGE('',*,*,#53803,.T.);
#78024=ORIENTED_EDGE('',*,*,#53811,.T.);
#78025=ORIENTED_EDGE('',*,*,#53814,.T.);
#78026=ORIENTED_EDGE('',*,*,#53815,.T.);
#78027=ORIENTED_EDGE('',*,*,#53816,.T.);
#78028=ORIENTED_EDGE('',*,*,#53736,.T.);
#78029=ORIENTED_EDGE('',*,*,#53817,.F.);
#78030=ORIENTED_EDGE('',*,*,#53818,.T.);
#78031=ORIENTED_EDGE('',*,*,#53819,.T.);
#78032=ORIENTED_EDGE('',*,*,#53744,.T.);
#78033=ORIENTED_EDGE('',*,*,#53820,.F.);
#78034=ORIENTED_EDGE('',*,*,#53821,.T.);
#78035=ORIENTED_EDGE('',*,*,#53822,.F.);
#78036=ORIENTED_EDGE('',*,*,#53772,.F.);
#78037=ORIENTED_EDGE('',*,*,#53823,.F.);
#78038=ORIENTED_EDGE('',*,*,#53813,.T.);
#78039=ORIENTED_EDGE('',*,*,#53823,.T.);
#78040=ORIENTED_EDGE('',*,*,#53789,.F.);
#78041=ORIENTED_EDGE('',*,*,#53824,.T.);
#78042=ORIENTED_EDGE('',*,*,#53790,.T.);
#78043=ORIENTED_EDGE('',*,*,#53824,.F.);
#78044=ORIENTED_EDGE('',*,*,#53786,.F.);
#78045=ORIENTED_EDGE('',*,*,#53825,.F.);
#78046=ORIENTED_EDGE('',*,*,#53798,.T.);
#78047=ORIENTED_EDGE('',*,*,#53799,.T.);
#78048=ORIENTED_EDGE('',*,*,#53825,.T.);
#78049=ORIENTED_EDGE('',*,*,#53785,.F.);
#78050=ORIENTED_EDGE('',*,*,#53788,.F.);
#78051=ORIENTED_EDGE('',*,*,#53782,.F.);
#78052=ORIENTED_EDGE('',*,*,#53826,.T.);
#78053=ORIENTED_EDGE('',*,*,#53802,.T.);
#78054=ORIENTED_EDGE('',*,*,#53797,.T.);
#78055=ORIENTED_EDGE('',*,*,#53826,.F.);
#78056=ORIENTED_EDGE('',*,*,#53781,.T.);
#78057=ORIENTED_EDGE('',*,*,#53827,.F.);
#78058=ORIENTED_EDGE('',*,*,#53800,.F.);
#78059=ORIENTED_EDGE('',*,*,#53804,.T.);
#78060=ORIENTED_EDGE('',*,*,#53827,.T.);
#78061=ORIENTED_EDGE('',*,*,#53779,.F.);
#78062=ORIENTED_EDGE('',*,*,#53828,.T.);
#78063=ORIENTED_EDGE('',*,*,#53828,.F.);
#78064=ORIENTED_EDGE('',*,*,#53776,.T.);
#78065=ORIENTED_EDGE('',*,*,#53829,.F.);
#78066=ORIENTED_EDGE('',*,*,#53806,.F.);
#78067=ORIENTED_EDGE('',*,*,#53739,.T.);
#78068=ORIENTED_EDGE('',*,*,#53734,.T.);
#78069=ORIENTED_EDGE('',*,*,#53741,.T.);
#78070=ORIENTED_EDGE('',*,*,#53747,.T.);
#78071=ORIENTED_EDGE('',*,*,#53753,.T.);
#78072=ORIENTED_EDGE('',*,*,#53755,.T.);
#78073=ORIENTED_EDGE('',*,*,#53751,.T.);
#78074=ORIENTED_EDGE('',*,*,#53745,.T.);
#78075=ORIENTED_EDGE('',*,*,#53829,.T.);
#78076=ORIENTED_EDGE('',*,*,#53778,.F.);
#78077=ORIENTED_EDGE('',*,*,#53775,.F.);
#78078=ORIENTED_EDGE('',*,*,#53773,.F.);
#78079=ORIENTED_EDGE('',*,*,#53822,.T.);
#78080=ORIENTED_EDGE('',*,*,#53812,.T.);
#78081=ORIENTED_EDGE('',*,*,#53809,.T.);
#78082=ORIENTED_EDGE('',*,*,#53807,.T.);
#78083=ORIENTED_EDGE('',*,*,#53820,.T.);
#78084=ORIENTED_EDGE('',*,*,#53750,.T.);
#78085=ORIENTED_EDGE('',*,*,#53760,.F.);
#78086=ORIENTED_EDGE('',*,*,#53830,.T.);
#78087=ORIENTED_EDGE('',*,*,#53762,.T.);
#78088=ORIENTED_EDGE('',*,*,#53742,.T.);
#78089=ORIENTED_EDGE('',*,*,#53816,.F.);
#78090=ORIENTED_EDGE('',*,*,#53831,.T.);
#78091=ORIENTED_EDGE('',*,*,#53814,.F.);
#78092=ORIENTED_EDGE('',*,*,#53832,.T.);
#78093=ORIENTED_EDGE('',*,*,#53768,.T.);
#78094=ORIENTED_EDGE('',*,*,#53832,.F.);
#78095=ORIENTED_EDGE('',*,*,#53815,.F.);
#78096=ORIENTED_EDGE('',*,*,#53833,.T.);
#78097=ORIENTED_EDGE('',*,*,#53769,.T.);
#78098=ORIENTED_EDGE('',*,*,#53833,.F.);
#78099=ORIENTED_EDGE('',*,*,#53817,.T.);
#78100=ORIENTED_EDGE('',*,*,#53738,.T.);
#78101=ORIENTED_EDGE('',*,*,#53819,.F.);
#78102=ORIENTED_EDGE('',*,*,#53834,.T.);
#78103=ORIENTED_EDGE('',*,*,#53830,.F.);
#78104=ORIENTED_EDGE('',*,*,#53761,.T.);
#78105=ORIENTED_EDGE('',*,*,#53759,.T.);
#78106=ORIENTED_EDGE('',*,*,#53763,.T.);
#78107=ORIENTED_EDGE('',*,*,#53831,.F.);
#78108=ORIENTED_EDGE('',*,*,#53818,.F.);
#78109=ORIENTED_EDGE('',*,*,#53834,.F.);
#78110=ORIENTED_EDGE('',*,*,#53821,.F.);
#78111=ORIENTED_EDGE('',*,*,#53835,.T.);
#78112=ORIENTED_EDGE('',*,*,#53836,.F.);
#78113=ORIENTED_EDGE('',*,*,#53837,.F.);
#78114=ORIENTED_EDGE('',*,*,#53838,.F.);
#78115=ORIENTED_EDGE('',*,*,#53839,.F.);
#78116=ORIENTED_EDGE('',*,*,#53840,.F.);
#78117=ORIENTED_EDGE('',*,*,#53841,.F.);
#78118=ORIENTED_EDGE('',*,*,#53842,.T.);
#78119=ORIENTED_EDGE('',*,*,#53835,.F.);
#78120=ORIENTED_EDGE('',*,*,#53842,.F.);
#78121=ORIENTED_EDGE('',*,*,#53843,.F.);
#78122=ORIENTED_EDGE('',*,*,#53844,.T.);
#78123=ORIENTED_EDGE('',*,*,#53845,.F.);
#78124=ORIENTED_EDGE('',*,*,#53846,.F.);
#78125=ORIENTED_EDGE('',*,*,#53844,.F.);
#78126=ORIENTED_EDGE('',*,*,#53847,.F.);
#78127=ORIENTED_EDGE('',*,*,#53848,.F.);
#78128=ORIENTED_EDGE('',*,*,#53849,.F.);
#78129=ORIENTED_EDGE('',*,*,#53850,.F.);
#78130=ORIENTED_EDGE('',*,*,#53836,.T.);
#78131=ORIENTED_EDGE('',*,*,#53851,.T.);
#78132=ORIENTED_EDGE('',*,*,#53850,.T.);
#78133=ORIENTED_EDGE('',*,*,#53852,.F.);
#78134=ORIENTED_EDGE('',*,*,#53837,.T.);
#78135=ORIENTED_EDGE('',*,*,#53852,.T.);
#78136=ORIENTED_EDGE('',*,*,#53849,.T.);
#78137=ORIENTED_EDGE('',*,*,#53853,.F.);
#78138=ORIENTED_EDGE('',*,*,#53838,.T.);
#78139=ORIENTED_EDGE('',*,*,#53853,.T.);
#78140=ORIENTED_EDGE('',*,*,#53848,.T.);
#78141=ORIENTED_EDGE('',*,*,#53854,.F.);
#78142=ORIENTED_EDGE('',*,*,#53839,.T.);
#78143=ORIENTED_EDGE('',*,*,#53854,.T.);
#78144=ORIENTED_EDGE('',*,*,#53847,.T.);
#78145=ORIENTED_EDGE('',*,*,#53851,.F.);
#78146=ORIENTED_EDGE('',*,*,#53855,.T.);
#78147=ORIENTED_EDGE('',*,*,#53856,.T.);
#78148=ORIENTED_EDGE('',*,*,#53857,.T.);
#78149=ORIENTED_EDGE('',*,*,#53855,.F.);
#78150=ORIENTED_EDGE('',*,*,#53857,.F.);
#78151=ORIENTED_EDGE('',*,*,#53840,.T.);
#78152=ORIENTED_EDGE('',*,*,#53841,.T.);
#78153=ORIENTED_EDGE('',*,*,#53858,.T.);
#78154=ORIENTED_EDGE('',*,*,#53845,.T.);
#78155=ORIENTED_EDGE('',*,*,#53846,.T.);
#78156=ORIENTED_EDGE('',*,*,#53858,.F.);
#78157=ORIENTED_EDGE('',*,*,#53843,.T.);
#78158=ORIENTED_EDGE('',*,*,#53856,.F.);
#78159=ORIENTED_EDGE('',*,*,#53859,.T.);
#78160=ORIENTED_EDGE('',*,*,#53860,.F.);
#78161=ORIENTED_EDGE('',*,*,#53861,.F.);
#78162=ORIENTED_EDGE('',*,*,#53862,.F.);
#78163=ORIENTED_EDGE('',*,*,#53863,.T.);
#78164=ORIENTED_EDGE('',*,*,#53864,.F.);
#78165=ORIENTED_EDGE('',*,*,#53859,.F.);
#78166=ORIENTED_EDGE('',*,*,#53865,.F.);
#78167=ORIENTED_EDGE('',*,*,#53866,.T.);
#78168=ORIENTED_EDGE('',*,*,#53867,.F.);
#78169=ORIENTED_EDGE('',*,*,#53863,.F.);
#78170=ORIENTED_EDGE('',*,*,#53868,.F.);
#78171=ORIENTED_EDGE('',*,*,#53869,.T.);
#78172=ORIENTED_EDGE('',*,*,#53870,.F.);
#78173=ORIENTED_EDGE('',*,*,#53866,.F.);
#78174=ORIENTED_EDGE('',*,*,#53871,.F.);
#78175=ORIENTED_EDGE('',*,*,#53872,.F.);
#78176=ORIENTED_EDGE('',*,*,#53873,.F.);
#78177=ORIENTED_EDGE('',*,*,#53869,.F.);
#78178=ORIENTED_EDGE('',*,*,#53874,.F.);
#78179=ORIENTED_EDGE('',*,*,#53875,.T.);
#78180=ORIENTED_EDGE('',*,*,#53876,.F.);
#78181=ORIENTED_EDGE('',*,*,#53877,.F.);
#78182=ORIENTED_EDGE('',*,*,#53878,.F.);
#78183=ORIENTED_EDGE('',*,*,#53879,.T.);
#78184=ORIENTED_EDGE('',*,*,#53880,.F.);
#78185=ORIENTED_EDGE('',*,*,#53875,.F.);
#78186=ORIENTED_EDGE('',*,*,#53881,.F.);
#78187=ORIENTED_EDGE('',*,*,#53882,.T.);
#78188=ORIENTED_EDGE('',*,*,#53883,.F.);
#78189=ORIENTED_EDGE('',*,*,#53879,.F.);
#78190=ORIENTED_EDGE('',*,*,#53884,.F.);
#78191=ORIENTED_EDGE('',*,*,#53885,.T.);
#78192=ORIENTED_EDGE('',*,*,#53886,.F.);
#78193=ORIENTED_EDGE('',*,*,#53882,.F.);
#78194=ORIENTED_EDGE('',*,*,#53887,.F.);
#78195=ORIENTED_EDGE('',*,*,#53888,.F.);
#78196=ORIENTED_EDGE('',*,*,#53889,.F.);
#78197=ORIENTED_EDGE('',*,*,#53885,.F.);
#78198=ORIENTED_EDGE('',*,*,#53890,.F.);
#78199=ORIENTED_EDGE('',*,*,#53891,.T.);
#78200=ORIENTED_EDGE('',*,*,#53892,.F.);
#78201=ORIENTED_EDGE('',*,*,#53893,.F.);
#78202=ORIENTED_EDGE('',*,*,#53894,.F.);
#78203=ORIENTED_EDGE('',*,*,#53895,.T.);
#78204=ORIENTED_EDGE('',*,*,#53896,.F.);
#78205=ORIENTED_EDGE('',*,*,#53891,.F.);
#78206=ORIENTED_EDGE('',*,*,#53897,.F.);
#78207=ORIENTED_EDGE('',*,*,#53898,.T.);
#78208=ORIENTED_EDGE('',*,*,#53899,.F.);
#78209=ORIENTED_EDGE('',*,*,#53895,.F.);
#78210=ORIENTED_EDGE('',*,*,#53900,.F.);
#78211=ORIENTED_EDGE('',*,*,#53901,.T.);
#78212=ORIENTED_EDGE('',*,*,#53902,.F.);
#78213=ORIENTED_EDGE('',*,*,#53898,.F.);
#78214=ORIENTED_EDGE('',*,*,#53903,.F.);
#78215=ORIENTED_EDGE('',*,*,#53904,.T.);
#78216=ORIENTED_EDGE('',*,*,#53905,.F.);
#78217=ORIENTED_EDGE('',*,*,#53901,.F.);
#78218=ORIENTED_EDGE('',*,*,#53906,.F.);
#78219=ORIENTED_EDGE('',*,*,#53907,.T.);
#78220=ORIENTED_EDGE('',*,*,#53908,.F.);
#78221=ORIENTED_EDGE('',*,*,#53904,.F.);
#78222=ORIENTED_EDGE('',*,*,#53909,.F.);
#78223=ORIENTED_EDGE('',*,*,#53910,.T.);
#78224=ORIENTED_EDGE('',*,*,#53911,.F.);
#78225=ORIENTED_EDGE('',*,*,#53907,.F.);
#78226=ORIENTED_EDGE('',*,*,#53912,.F.);
#78227=ORIENTED_EDGE('',*,*,#53913,.T.);
#78228=ORIENTED_EDGE('',*,*,#53914,.F.);
#78229=ORIENTED_EDGE('',*,*,#53910,.F.);
#78230=ORIENTED_EDGE('',*,*,#53915,.F.);
#78231=ORIENTED_EDGE('',*,*,#53916,.F.);
#78232=ORIENTED_EDGE('',*,*,#53917,.F.);
#78233=ORIENTED_EDGE('',*,*,#53913,.F.);
#78234=ORIENTED_EDGE('',*,*,#53918,.F.);
#78235=ORIENTED_EDGE('',*,*,#53919,.F.);
#78236=ORIENTED_EDGE('',*,*,#53920,.F.);
#78237=ORIENTED_EDGE('',*,*,#53921,.T.);
#78238=ORIENTED_EDGE('',*,*,#53922,.F.);
#78239=ORIENTED_EDGE('',*,*,#53923,.T.);
#78240=ORIENTED_EDGE('',*,*,#53924,.F.);
#78241=ORIENTED_EDGE('',*,*,#53921,.F.);
#78242=ORIENTED_EDGE('',*,*,#53925,.F.);
#78243=ORIENTED_EDGE('',*,*,#53926,.T.);
#78244=ORIENTED_EDGE('',*,*,#53927,.F.);
#78245=ORIENTED_EDGE('',*,*,#53923,.F.);
#78246=ORIENTED_EDGE('',*,*,#53928,.F.);
#78247=ORIENTED_EDGE('',*,*,#53929,.T.);
#78248=ORIENTED_EDGE('',*,*,#53930,.F.);
#78249=ORIENTED_EDGE('',*,*,#53926,.F.);
#78250=ORIENTED_EDGE('',*,*,#53931,.F.);
#78251=ORIENTED_EDGE('',*,*,#53932,.F.);
#78252=ORIENTED_EDGE('',*,*,#53933,.F.);
#78253=ORIENTED_EDGE('',*,*,#53929,.F.);
#78254=ORIENTED_EDGE('',*,*,#53934,.F.);
#78255=ORIENTED_EDGE('',*,*,#53935,.T.);
#78256=ORIENTED_EDGE('',*,*,#53936,.F.);
#78257=ORIENTED_EDGE('',*,*,#53937,.F.);
#78258=ORIENTED_EDGE('',*,*,#53938,.F.);
#78259=ORIENTED_EDGE('',*,*,#53939,.T.);
#78260=ORIENTED_EDGE('',*,*,#53940,.F.);
#78261=ORIENTED_EDGE('',*,*,#53935,.F.);
#78262=ORIENTED_EDGE('',*,*,#53941,.F.);
#78263=ORIENTED_EDGE('',*,*,#53942,.T.);
#78264=ORIENTED_EDGE('',*,*,#53943,.F.);
#78265=ORIENTED_EDGE('',*,*,#53939,.F.);
#78266=ORIENTED_EDGE('',*,*,#53944,.F.);
#78267=ORIENTED_EDGE('',*,*,#53945,.T.);
#78268=ORIENTED_EDGE('',*,*,#53946,.F.);
#78269=ORIENTED_EDGE('',*,*,#53942,.F.);
#78270=ORIENTED_EDGE('',*,*,#53947,.F.);
#78271=ORIENTED_EDGE('',*,*,#53948,.T.);
#78272=ORIENTED_EDGE('',*,*,#53949,.F.);
#78273=ORIENTED_EDGE('',*,*,#53945,.F.);
#78274=ORIENTED_EDGE('',*,*,#53950,.F.);
#78275=ORIENTED_EDGE('',*,*,#53951,.T.);
#78276=ORIENTED_EDGE('',*,*,#53952,.F.);
#78277=ORIENTED_EDGE('',*,*,#53948,.F.);
#78278=ORIENTED_EDGE('',*,*,#53953,.F.);
#78279=ORIENTED_EDGE('',*,*,#53954,.T.);
#78280=ORIENTED_EDGE('',*,*,#53955,.F.);
#78281=ORIENTED_EDGE('',*,*,#53951,.F.);
#78282=ORIENTED_EDGE('',*,*,#53956,.F.);
#78283=ORIENTED_EDGE('',*,*,#53957,.T.);
#78284=ORIENTED_EDGE('',*,*,#53958,.F.);
#78285=ORIENTED_EDGE('',*,*,#53954,.F.);
#78286=ORIENTED_EDGE('',*,*,#53959,.F.);
#78287=ORIENTED_EDGE('',*,*,#53960,.T.);
#78288=ORIENTED_EDGE('',*,*,#53961,.F.);
#78289=ORIENTED_EDGE('',*,*,#53957,.F.);
#78290=ORIENTED_EDGE('',*,*,#53962,.F.);
#78291=ORIENTED_EDGE('',*,*,#53963,.F.);
#78292=ORIENTED_EDGE('',*,*,#53964,.F.);
#78293=ORIENTED_EDGE('',*,*,#53960,.F.);
#78294=ORIENTED_EDGE('',*,*,#53965,.F.);
#78295=ORIENTED_EDGE('',*,*,#53966,.T.);
#78296=ORIENTED_EDGE('',*,*,#53967,.F.);
#78297=ORIENTED_EDGE('',*,*,#53968,.F.);
#78298=ORIENTED_EDGE('',*,*,#53969,.F.);
#78299=ORIENTED_EDGE('',*,*,#53970,.T.);
#78300=ORIENTED_EDGE('',*,*,#53971,.F.);
#78301=ORIENTED_EDGE('',*,*,#53966,.F.);
#78302=ORIENTED_EDGE('',*,*,#53972,.F.);
#78303=ORIENTED_EDGE('',*,*,#53973,.T.);
#78304=ORIENTED_EDGE('',*,*,#53974,.F.);
#78305=ORIENTED_EDGE('',*,*,#53970,.F.);
#78306=ORIENTED_EDGE('',*,*,#53975,.F.);
#78307=ORIENTED_EDGE('',*,*,#53976,.T.);
#78308=ORIENTED_EDGE('',*,*,#53977,.F.);
#78309=ORIENTED_EDGE('',*,*,#53973,.F.);
#78310=ORIENTED_EDGE('',*,*,#53978,.F.);
#78311=ORIENTED_EDGE('',*,*,#53979,.T.);
#78312=ORIENTED_EDGE('',*,*,#53980,.F.);
#78313=ORIENTED_EDGE('',*,*,#53976,.F.);
#78314=ORIENTED_EDGE('',*,*,#53981,.F.);
#78315=ORIENTED_EDGE('',*,*,#53982,.T.);
#78316=ORIENTED_EDGE('',*,*,#53983,.F.);
#78317=ORIENTED_EDGE('',*,*,#53979,.F.);
#78318=ORIENTED_EDGE('',*,*,#53984,.F.);
#78319=ORIENTED_EDGE('',*,*,#53985,.T.);
#78320=ORIENTED_EDGE('',*,*,#53986,.F.);
#78321=ORIENTED_EDGE('',*,*,#53982,.F.);
#78322=ORIENTED_EDGE('',*,*,#53987,.F.);
#78323=ORIENTED_EDGE('',*,*,#53988,.T.);
#78324=ORIENTED_EDGE('',*,*,#53989,.F.);
#78325=ORIENTED_EDGE('',*,*,#53985,.F.);
#78326=ORIENTED_EDGE('',*,*,#53990,.F.);
#78327=ORIENTED_EDGE('',*,*,#53991,.F.);
#78328=ORIENTED_EDGE('',*,*,#53992,.F.);
#78329=ORIENTED_EDGE('',*,*,#53988,.F.);
#78330=ORIENTED_EDGE('',*,*,#53993,.F.);
#78331=ORIENTED_EDGE('',*,*,#53994,.T.);
#78332=ORIENTED_EDGE('',*,*,#53995,.F.);
#78333=ORIENTED_EDGE('',*,*,#53996,.F.);
#78334=ORIENTED_EDGE('',*,*,#53997,.F.);
#78335=ORIENTED_EDGE('',*,*,#53998,.T.);
#78336=ORIENTED_EDGE('',*,*,#53999,.F.);
#78337=ORIENTED_EDGE('',*,*,#53994,.F.);
#78338=ORIENTED_EDGE('',*,*,#54000,.F.);
#78339=ORIENTED_EDGE('',*,*,#54001,.T.);
#78340=ORIENTED_EDGE('',*,*,#54002,.F.);
#78341=ORIENTED_EDGE('',*,*,#53998,.F.);
#78342=ORIENTED_EDGE('',*,*,#54003,.F.);
#78343=ORIENTED_EDGE('',*,*,#54004,.T.);
#78344=ORIENTED_EDGE('',*,*,#54005,.F.);
#78345=ORIENTED_EDGE('',*,*,#54001,.F.);
#78346=ORIENTED_EDGE('',*,*,#54006,.F.);
#78347=ORIENTED_EDGE('',*,*,#54007,.T.);
#78348=ORIENTED_EDGE('',*,*,#54008,.F.);
#78349=ORIENTED_EDGE('',*,*,#54004,.F.);
#78350=ORIENTED_EDGE('',*,*,#54009,.F.);
#78351=ORIENTED_EDGE('',*,*,#54010,.T.);
#78352=ORIENTED_EDGE('',*,*,#54011,.F.);
#78353=ORIENTED_EDGE('',*,*,#54007,.F.);
#78354=ORIENTED_EDGE('',*,*,#54012,.F.);
#78355=ORIENTED_EDGE('',*,*,#54013,.T.);
#78356=ORIENTED_EDGE('',*,*,#54014,.F.);
#78357=ORIENTED_EDGE('',*,*,#54010,.F.);
#78358=ORIENTED_EDGE('',*,*,#54015,.F.);
#78359=ORIENTED_EDGE('',*,*,#54016,.T.);
#78360=ORIENTED_EDGE('',*,*,#54017,.F.);
#78361=ORIENTED_EDGE('',*,*,#54013,.F.);
#78362=ORIENTED_EDGE('',*,*,#54018,.F.);
#78363=ORIENTED_EDGE('',*,*,#54019,.F.);
#78364=ORIENTED_EDGE('',*,*,#54020,.F.);
#78365=ORIENTED_EDGE('',*,*,#54016,.F.);
#78366=ORIENTED_EDGE('',*,*,#54021,.F.);
#78367=ORIENTED_EDGE('',*,*,#54022,.T.);
#78368=ORIENTED_EDGE('',*,*,#54023,.F.);
#78369=ORIENTED_EDGE('',*,*,#54024,.F.);
#78370=ORIENTED_EDGE('',*,*,#54025,.F.);
#78371=ORIENTED_EDGE('',*,*,#54026,.T.);
#78372=ORIENTED_EDGE('',*,*,#54027,.F.);
#78373=ORIENTED_EDGE('',*,*,#54022,.F.);
#78374=ORIENTED_EDGE('',*,*,#54028,.F.);
#78375=ORIENTED_EDGE('',*,*,#54029,.T.);
#78376=ORIENTED_EDGE('',*,*,#54030,.F.);
#78377=ORIENTED_EDGE('',*,*,#54026,.F.);
#78378=ORIENTED_EDGE('',*,*,#54031,.F.);
#78379=ORIENTED_EDGE('',*,*,#54032,.T.);
#78380=ORIENTED_EDGE('',*,*,#54033,.F.);
#78381=ORIENTED_EDGE('',*,*,#54029,.F.);
#78382=ORIENTED_EDGE('',*,*,#54034,.F.);
#78383=ORIENTED_EDGE('',*,*,#54035,.T.);
#78384=ORIENTED_EDGE('',*,*,#54036,.F.);
#78385=ORIENTED_EDGE('',*,*,#54032,.F.);
#78386=ORIENTED_EDGE('',*,*,#54037,.F.);
#78387=ORIENTED_EDGE('',*,*,#54038,.T.);
#78388=ORIENTED_EDGE('',*,*,#54039,.F.);
#78389=ORIENTED_EDGE('',*,*,#54035,.F.);
#78390=ORIENTED_EDGE('',*,*,#54040,.F.);
#78391=ORIENTED_EDGE('',*,*,#54041,.T.);
#78392=ORIENTED_EDGE('',*,*,#54042,.F.);
#78393=ORIENTED_EDGE('',*,*,#54038,.F.);
#78394=ORIENTED_EDGE('',*,*,#54043,.F.);
#78395=ORIENTED_EDGE('',*,*,#54044,.T.);
#78396=ORIENTED_EDGE('',*,*,#54045,.F.);
#78397=ORIENTED_EDGE('',*,*,#54041,.F.);
#78398=ORIENTED_EDGE('',*,*,#54046,.F.);
#78399=ORIENTED_EDGE('',*,*,#54047,.F.);
#78400=ORIENTED_EDGE('',*,*,#54048,.F.);
#78401=ORIENTED_EDGE('',*,*,#54044,.F.);
#78402=ORIENTED_EDGE('',*,*,#54049,.F.);
#78403=ORIENTED_EDGE('',*,*,#54050,.T.);
#78404=ORIENTED_EDGE('',*,*,#54051,.F.);
#78405=ORIENTED_EDGE('',*,*,#54052,.F.);
#78406=ORIENTED_EDGE('',*,*,#54053,.F.);
#78407=ORIENTED_EDGE('',*,*,#54054,.T.);
#78408=ORIENTED_EDGE('',*,*,#54055,.F.);
#78409=ORIENTED_EDGE('',*,*,#54050,.F.);
#78410=ORIENTED_EDGE('',*,*,#54056,.F.);
#78411=ORIENTED_EDGE('',*,*,#54057,.T.);
#78412=ORIENTED_EDGE('',*,*,#54058,.F.);
#78413=ORIENTED_EDGE('',*,*,#54054,.F.);
#78414=ORIENTED_EDGE('',*,*,#54059,.F.);
#78415=ORIENTED_EDGE('',*,*,#54060,.T.);
#78416=ORIENTED_EDGE('',*,*,#54061,.F.);
#78417=ORIENTED_EDGE('',*,*,#54057,.F.);
#78418=ORIENTED_EDGE('',*,*,#54062,.F.);
#78419=ORIENTED_EDGE('',*,*,#54063,.T.);
#78420=ORIENTED_EDGE('',*,*,#54064,.F.);
#78421=ORIENTED_EDGE('',*,*,#54060,.F.);
#78422=ORIENTED_EDGE('',*,*,#54065,.F.);
#78423=ORIENTED_EDGE('',*,*,#54066,.T.);
#78424=ORIENTED_EDGE('',*,*,#54067,.F.);
#78425=ORIENTED_EDGE('',*,*,#54063,.F.);
#78426=ORIENTED_EDGE('',*,*,#54068,.F.);
#78427=ORIENTED_EDGE('',*,*,#54069,.T.);
#78428=ORIENTED_EDGE('',*,*,#54070,.F.);
#78429=ORIENTED_EDGE('',*,*,#54066,.F.);
#78430=ORIENTED_EDGE('',*,*,#54071,.F.);
#78431=ORIENTED_EDGE('',*,*,#54072,.T.);
#78432=ORIENTED_EDGE('',*,*,#54073,.F.);
#78433=ORIENTED_EDGE('',*,*,#54069,.F.);
#78434=ORIENTED_EDGE('',*,*,#54074,.F.);
#78435=ORIENTED_EDGE('',*,*,#54075,.F.);
#78436=ORIENTED_EDGE('',*,*,#54076,.F.);
#78437=ORIENTED_EDGE('',*,*,#54072,.F.);
#78438=ORIENTED_EDGE('',*,*,#54077,.F.);
#78439=ORIENTED_EDGE('',*,*,#54078,.T.);
#78440=ORIENTED_EDGE('',*,*,#54079,.F.);
#78441=ORIENTED_EDGE('',*,*,#54080,.F.);
#78442=ORIENTED_EDGE('',*,*,#54081,.F.);
#78443=ORIENTED_EDGE('',*,*,#54082,.T.);
#78444=ORIENTED_EDGE('',*,*,#54083,.F.);
#78445=ORIENTED_EDGE('',*,*,#54078,.F.);
#78446=ORIENTED_EDGE('',*,*,#54084,.F.);
#78447=ORIENTED_EDGE('',*,*,#54085,.T.);
#78448=ORIENTED_EDGE('',*,*,#54086,.F.);
#78449=ORIENTED_EDGE('',*,*,#54082,.F.);
#78450=ORIENTED_EDGE('',*,*,#54087,.F.);
#78451=ORIENTED_EDGE('',*,*,#54088,.T.);
#78452=ORIENTED_EDGE('',*,*,#54089,.F.);
#78453=ORIENTED_EDGE('',*,*,#54085,.F.);
#78454=ORIENTED_EDGE('',*,*,#54090,.F.);
#78455=ORIENTED_EDGE('',*,*,#54091,.T.);
#78456=ORIENTED_EDGE('',*,*,#54092,.F.);
#78457=ORIENTED_EDGE('',*,*,#54088,.F.);
#78458=ORIENTED_EDGE('',*,*,#54093,.F.);
#78459=ORIENTED_EDGE('',*,*,#54094,.T.);
#78460=ORIENTED_EDGE('',*,*,#54095,.F.);
#78461=ORIENTED_EDGE('',*,*,#54091,.F.);
#78462=ORIENTED_EDGE('',*,*,#54096,.F.);
#78463=ORIENTED_EDGE('',*,*,#54097,.T.);
#78464=ORIENTED_EDGE('',*,*,#54098,.F.);
#78465=ORIENTED_EDGE('',*,*,#54094,.F.);
#78466=ORIENTED_EDGE('',*,*,#54099,.F.);
#78467=ORIENTED_EDGE('',*,*,#54100,.T.);
#78468=ORIENTED_EDGE('',*,*,#54101,.F.);
#78469=ORIENTED_EDGE('',*,*,#54097,.F.);
#78470=ORIENTED_EDGE('',*,*,#54102,.F.);
#78471=ORIENTED_EDGE('',*,*,#54103,.F.);
#78472=ORIENTED_EDGE('',*,*,#54104,.F.);
#78473=ORIENTED_EDGE('',*,*,#54100,.F.);
#78474=ORIENTED_EDGE('',*,*,#54105,.F.);
#78475=ORIENTED_EDGE('',*,*,#54106,.T.);
#78476=ORIENTED_EDGE('',*,*,#54107,.F.);
#78477=ORIENTED_EDGE('',*,*,#54108,.F.);
#78478=ORIENTED_EDGE('',*,*,#54109,.F.);
#78479=ORIENTED_EDGE('',*,*,#54110,.T.);
#78480=ORIENTED_EDGE('',*,*,#54111,.F.);
#78481=ORIENTED_EDGE('',*,*,#54106,.F.);
#78482=ORIENTED_EDGE('',*,*,#54112,.F.);
#78483=ORIENTED_EDGE('',*,*,#54113,.T.);
#78484=ORIENTED_EDGE('',*,*,#54114,.F.);
#78485=ORIENTED_EDGE('',*,*,#54110,.F.);
#78486=ORIENTED_EDGE('',*,*,#54115,.F.);
#78487=ORIENTED_EDGE('',*,*,#54116,.T.);
#78488=ORIENTED_EDGE('',*,*,#54117,.F.);
#78489=ORIENTED_EDGE('',*,*,#54113,.F.);
#78490=ORIENTED_EDGE('',*,*,#54118,.F.);
#78491=ORIENTED_EDGE('',*,*,#54119,.T.);
#78492=ORIENTED_EDGE('',*,*,#54120,.F.);
#78493=ORIENTED_EDGE('',*,*,#54116,.F.);
#78494=ORIENTED_EDGE('',*,*,#54121,.F.);
#78495=ORIENTED_EDGE('',*,*,#54122,.T.);
#78496=ORIENTED_EDGE('',*,*,#54123,.F.);
#78497=ORIENTED_EDGE('',*,*,#54119,.F.);
#78498=ORIENTED_EDGE('',*,*,#54124,.F.);
#78499=ORIENTED_EDGE('',*,*,#54125,.T.);
#78500=ORIENTED_EDGE('',*,*,#54126,.F.);
#78501=ORIENTED_EDGE('',*,*,#54122,.F.);
#78502=ORIENTED_EDGE('',*,*,#54127,.F.);
#78503=ORIENTED_EDGE('',*,*,#54128,.T.);
#78504=ORIENTED_EDGE('',*,*,#54129,.F.);
#78505=ORIENTED_EDGE('',*,*,#54125,.F.);
#78506=ORIENTED_EDGE('',*,*,#54130,.F.);
#78507=ORIENTED_EDGE('',*,*,#54131,.F.);
#78508=ORIENTED_EDGE('',*,*,#54132,.F.);
#78509=ORIENTED_EDGE('',*,*,#54128,.F.);
#78510=ORIENTED_EDGE('',*,*,#54133,.F.);
#78511=ORIENTED_EDGE('',*,*,#54134,.T.);
#78512=ORIENTED_EDGE('',*,*,#54135,.F.);
#78513=ORIENTED_EDGE('',*,*,#54136,.F.);
#78514=ORIENTED_EDGE('',*,*,#54137,.F.);
#78515=ORIENTED_EDGE('',*,*,#54138,.T.);
#78516=ORIENTED_EDGE('',*,*,#54139,.F.);
#78517=ORIENTED_EDGE('',*,*,#54134,.F.);
#78518=ORIENTED_EDGE('',*,*,#54140,.F.);
#78519=ORIENTED_EDGE('',*,*,#54141,.T.);
#78520=ORIENTED_EDGE('',*,*,#54142,.F.);
#78521=ORIENTED_EDGE('',*,*,#54138,.F.);
#78522=ORIENTED_EDGE('',*,*,#54143,.F.);
#78523=ORIENTED_EDGE('',*,*,#54144,.T.);
#78524=ORIENTED_EDGE('',*,*,#54145,.F.);
#78525=ORIENTED_EDGE('',*,*,#54141,.F.);
#78526=ORIENTED_EDGE('',*,*,#54146,.F.);
#78527=ORIENTED_EDGE('',*,*,#54147,.T.);
#78528=ORIENTED_EDGE('',*,*,#54148,.F.);
#78529=ORIENTED_EDGE('',*,*,#54144,.F.);
#78530=ORIENTED_EDGE('',*,*,#54149,.F.);
#78531=ORIENTED_EDGE('',*,*,#54150,.T.);
#78532=ORIENTED_EDGE('',*,*,#54151,.F.);
#78533=ORIENTED_EDGE('',*,*,#54147,.F.);
#78534=ORIENTED_EDGE('',*,*,#54152,.F.);
#78535=ORIENTED_EDGE('',*,*,#54153,.T.);
#78536=ORIENTED_EDGE('',*,*,#54154,.F.);
#78537=ORIENTED_EDGE('',*,*,#54150,.F.);
#78538=ORIENTED_EDGE('',*,*,#54155,.F.);
#78539=ORIENTED_EDGE('',*,*,#54156,.T.);
#78540=ORIENTED_EDGE('',*,*,#54157,.F.);
#78541=ORIENTED_EDGE('',*,*,#54153,.F.);
#78542=ORIENTED_EDGE('',*,*,#54158,.F.);
#78543=ORIENTED_EDGE('',*,*,#54159,.T.);
#78544=ORIENTED_EDGE('',*,*,#54160,.F.);
#78545=ORIENTED_EDGE('',*,*,#54156,.F.);
#78546=ORIENTED_EDGE('',*,*,#54161,.F.);
#78547=ORIENTED_EDGE('',*,*,#54162,.F.);
#78548=ORIENTED_EDGE('',*,*,#54163,.F.);
#78549=ORIENTED_EDGE('',*,*,#54159,.F.);
#78550=ORIENTED_EDGE('',*,*,#54164,.F.);
#78551=ORIENTED_EDGE('',*,*,#54165,.T.);
#78552=ORIENTED_EDGE('',*,*,#54166,.F.);
#78553=ORIENTED_EDGE('',*,*,#54167,.F.);
#78554=ORIENTED_EDGE('',*,*,#54168,.F.);
#78555=ORIENTED_EDGE('',*,*,#54169,.T.);
#78556=ORIENTED_EDGE('',*,*,#54170,.F.);
#78557=ORIENTED_EDGE('',*,*,#54165,.F.);
#78558=ORIENTED_EDGE('',*,*,#54171,.F.);
#78559=ORIENTED_EDGE('',*,*,#54172,.T.);
#78560=ORIENTED_EDGE('',*,*,#54173,.F.);
#78561=ORIENTED_EDGE('',*,*,#54169,.F.);
#78562=ORIENTED_EDGE('',*,*,#54174,.F.);
#78563=ORIENTED_EDGE('',*,*,#54175,.T.);
#78564=ORIENTED_EDGE('',*,*,#54176,.F.);
#78565=ORIENTED_EDGE('',*,*,#54172,.F.);
#78566=ORIENTED_EDGE('',*,*,#54177,.F.);
#78567=ORIENTED_EDGE('',*,*,#54178,.T.);
#78568=ORIENTED_EDGE('',*,*,#54179,.F.);
#78569=ORIENTED_EDGE('',*,*,#54175,.F.);
#78570=ORIENTED_EDGE('',*,*,#54180,.F.);
#78571=ORIENTED_EDGE('',*,*,#54181,.T.);
#78572=ORIENTED_EDGE('',*,*,#54182,.F.);
#78573=ORIENTED_EDGE('',*,*,#54178,.F.);
#78574=ORIENTED_EDGE('',*,*,#54183,.F.);
#78575=ORIENTED_EDGE('',*,*,#54184,.T.);
#78576=ORIENTED_EDGE('',*,*,#54185,.F.);
#78577=ORIENTED_EDGE('',*,*,#54181,.F.);
#78578=ORIENTED_EDGE('',*,*,#54186,.F.);
#78579=ORIENTED_EDGE('',*,*,#54187,.T.);
#78580=ORIENTED_EDGE('',*,*,#54188,.F.);
#78581=ORIENTED_EDGE('',*,*,#54184,.F.);
#78582=ORIENTED_EDGE('',*,*,#54189,.F.);
#78583=ORIENTED_EDGE('',*,*,#54190,.F.);
#78584=ORIENTED_EDGE('',*,*,#54191,.F.);
#78585=ORIENTED_EDGE('',*,*,#54187,.F.);
#78586=ORIENTED_EDGE('',*,*,#54192,.F.);
#78587=ORIENTED_EDGE('',*,*,#54193,.F.);
#78588=ORIENTED_EDGE('',*,*,#54194,.F.);
#78589=ORIENTED_EDGE('',*,*,#54195,.T.);
#78590=ORIENTED_EDGE('',*,*,#54196,.F.);
#78591=ORIENTED_EDGE('',*,*,#54197,.T.);
#78592=ORIENTED_EDGE('',*,*,#54198,.F.);
#78593=ORIENTED_EDGE('',*,*,#54195,.F.);
#78594=ORIENTED_EDGE('',*,*,#54199,.F.);
#78595=ORIENTED_EDGE('',*,*,#54200,.T.);
#78596=ORIENTED_EDGE('',*,*,#54201,.F.);
#78597=ORIENTED_EDGE('',*,*,#54197,.F.);
#78598=ORIENTED_EDGE('',*,*,#54202,.F.);
#78599=ORIENTED_EDGE('',*,*,#54203,.T.);
#78600=ORIENTED_EDGE('',*,*,#54204,.F.);
#78601=ORIENTED_EDGE('',*,*,#54200,.F.);
#78602=ORIENTED_EDGE('',*,*,#54205,.F.);
#78603=ORIENTED_EDGE('',*,*,#54206,.F.);
#78604=ORIENTED_EDGE('',*,*,#54207,.F.);
#78605=ORIENTED_EDGE('',*,*,#54203,.F.);
#78606=ORIENTED_EDGE('',*,*,#54208,.F.);
#78607=ORIENTED_EDGE('',*,*,#54209,.F.);
#78608=ORIENTED_EDGE('',*,*,#53930,.T.);
#78609=ORIENTED_EDGE('',*,*,#54210,.F.);
#78610=ORIENTED_EDGE('',*,*,#54211,.F.);
#78611=ORIENTED_EDGE('',*,*,#54212,.F.);
#78612=ORIENTED_EDGE('',*,*,#53887,.T.);
#78613=ORIENTED_EDGE('',*,*,#54213,.F.);
#78614=ORIENTED_EDGE('',*,*,#54214,.F.);
#78615=ORIENTED_EDGE('',*,*,#54215,.F.);
#78616=ORIENTED_EDGE('',*,*,#54198,.T.);
#78617=ORIENTED_EDGE('',*,*,#54216,.F.);
#78618=ORIENTED_EDGE('',*,*,#54217,.F.);
#78619=ORIENTED_EDGE('',*,*,#54218,.F.);
#78620=ORIENTED_EDGE('',*,*,#53865,.T.);
#78621=ORIENTED_EDGE('',*,*,#54219,.F.);
#78622=ORIENTED_EDGE('',*,*,#54220,.F.);
#78623=ORIENTED_EDGE('',*,*,#54221,.F.);
#78624=ORIENTED_EDGE('',*,*,#53871,.T.);
#78625=ORIENTED_EDGE('',*,*,#54222,.F.);
#78626=ORIENTED_EDGE('',*,*,#54223,.F.);
#78627=ORIENTED_EDGE('',*,*,#54224,.F.);
#78628=ORIENTED_EDGE('',*,*,#54176,.T.);
#78629=ORIENTED_EDGE('',*,*,#54225,.F.);
#78630=ORIENTED_EDGE('',*,*,#54226,.F.);
#78631=ORIENTED_EDGE('',*,*,#54227,.F.);
#78632=ORIENTED_EDGE('',*,*,#54145,.T.);
#78633=ORIENTED_EDGE('',*,*,#54228,.F.);
#78634=ORIENTED_EDGE('',*,*,#54229,.F.);
#78635=ORIENTED_EDGE('',*,*,#54230,.F.);
#78636=ORIENTED_EDGE('',*,*,#54117,.T.);
#78637=ORIENTED_EDGE('',*,*,#54231,.F.);
#78638=ORIENTED_EDGE('',*,*,#54232,.F.);
#78639=ORIENTED_EDGE('',*,*,#54233,.F.);
#78640=ORIENTED_EDGE('',*,*,#54089,.T.);
#78641=ORIENTED_EDGE('',*,*,#54234,.F.);
#78642=ORIENTED_EDGE('',*,*,#54235,.F.);
#78643=ORIENTED_EDGE('',*,*,#54236,.F.);
#78644=ORIENTED_EDGE('',*,*,#54061,.T.);
#78645=ORIENTED_EDGE('',*,*,#54237,.F.);
#78646=ORIENTED_EDGE('',*,*,#54238,.F.);
#78647=ORIENTED_EDGE('',*,*,#54239,.F.);
#78648=ORIENTED_EDGE('',*,*,#54033,.T.);
#78649=ORIENTED_EDGE('',*,*,#54240,.F.);
#78650=ORIENTED_EDGE('',*,*,#54241,.F.);
#78651=ORIENTED_EDGE('',*,*,#54242,.F.);
#78652=ORIENTED_EDGE('',*,*,#54067,.T.);
#78653=ORIENTED_EDGE('',*,*,#54243,.F.);
#78654=ORIENTED_EDGE('',*,*,#54244,.F.);
#78655=ORIENTED_EDGE('',*,*,#54245,.F.);
#78656=ORIENTED_EDGE('',*,*,#54095,.T.);
#78657=ORIENTED_EDGE('',*,*,#54246,.F.);
#78658=ORIENTED_EDGE('',*,*,#54247,.F.);
#78659=ORIENTED_EDGE('',*,*,#54248,.F.);
#78660=ORIENTED_EDGE('',*,*,#54123,.T.);
#78661=ORIENTED_EDGE('',*,*,#54249,.F.);
#78662=ORIENTED_EDGE('',*,*,#54250,.F.);
#78663=ORIENTED_EDGE('',*,*,#54251,.F.);
#78664=ORIENTED_EDGE('',*,*,#54154,.T.);
#78665=ORIENTED_EDGE('',*,*,#54252,.F.);
#78666=ORIENTED_EDGE('',*,*,#54253,.F.);
#78667=ORIENTED_EDGE('',*,*,#54254,.F.);
#78668=ORIENTED_EDGE('',*,*,#54182,.T.);
#78669=ORIENTED_EDGE('',*,*,#54255,.F.);
#78670=ORIENTED_EDGE('',*,*,#54256,.F.);
#78671=ORIENTED_EDGE('',*,*,#54257,.F.);
#78672=ORIENTED_EDGE('',*,*,#54039,.T.);
#78673=ORIENTED_EDGE('',*,*,#54258,.F.);
#78674=ORIENTED_EDGE('',*,*,#54259,.F.);
#78675=ORIENTED_EDGE('',*,*,#54260,.F.);
#78676=ORIENTED_EDGE('',*,*,#54005,.T.);
#78677=ORIENTED_EDGE('',*,*,#54261,.F.);
#78678=ORIENTED_EDGE('',*,*,#54262,.F.);
#78679=ORIENTED_EDGE('',*,*,#54263,.F.);
#78680=ORIENTED_EDGE('',*,*,#54011,.T.);
#78681=ORIENTED_EDGE('',*,*,#54264,.F.);
#78682=ORIENTED_EDGE('',*,*,#54265,.F.);
#78683=ORIENTED_EDGE('',*,*,#54266,.F.);
#78684=ORIENTED_EDGE('',*,*,#53977,.T.);
#78685=ORIENTED_EDGE('',*,*,#54267,.F.);
#78686=ORIENTED_EDGE('',*,*,#54268,.F.);
#78687=ORIENTED_EDGE('',*,*,#54269,.F.);
#78688=ORIENTED_EDGE('',*,*,#53946,.T.);
#78689=ORIENTED_EDGE('',*,*,#54270,.F.);
#78690=ORIENTED_EDGE('',*,*,#54271,.F.);
#78691=ORIENTED_EDGE('',*,*,#54272,.F.);
#78692=ORIENTED_EDGE('',*,*,#53983,.T.);
#78693=ORIENTED_EDGE('',*,*,#54273,.F.);
#78694=ORIENTED_EDGE('',*,*,#54274,.F.);
#78695=ORIENTED_EDGE('',*,*,#54275,.F.);
#78696=ORIENTED_EDGE('',*,*,#53955,.T.);
#78697=ORIENTED_EDGE('',*,*,#54276,.F.);
#78698=ORIENTED_EDGE('',*,*,#54277,.F.);
#78699=ORIENTED_EDGE('',*,*,#54278,.F.);
#78700=ORIENTED_EDGE('',*,*,#53902,.T.);
#78701=ORIENTED_EDGE('',*,*,#54279,.F.);
#78702=ORIENTED_EDGE('',*,*,#54280,.F.);
#78703=ORIENTED_EDGE('',*,*,#54281,.F.);
#78704=ORIENTED_EDGE('',*,*,#53908,.T.);
#78705=ORIENTED_EDGE('',*,*,#54282,.F.);
#78706=ORIENTED_EDGE('',*,*,#54283,.F.);
#78707=ORIENTED_EDGE('',*,*,#54284,.F.);
#78708=ORIENTED_EDGE('',*,*,#53881,.T.);
#78709=ORIENTED_EDGE('',*,*,#54285,.F.);
#78710=ORIENTED_EDGE('',*,*,#54286,.F.);
#78711=ORIENTED_EDGE('',*,*,#54199,.T.);
#78712=ORIENTED_EDGE('',*,*,#54194,.T.);
#78713=ORIENTED_EDGE('',*,*,#54287,.F.);
#78714=ORIENTED_EDGE('',*,*,#53860,.T.);
#78715=ORIENTED_EDGE('',*,*,#53864,.T.);
#78716=ORIENTED_EDGE('',*,*,#53867,.T.);
#78717=ORIENTED_EDGE('',*,*,#53870,.T.);
#78718=ORIENTED_EDGE('',*,*,#53873,.T.);
#78719=ORIENTED_EDGE('',*,*,#54288,.F.);
#78720=ORIENTED_EDGE('',*,*,#54289,.F.);
#78721=ORIENTED_EDGE('',*,*,#54290,.F.);
#78722=ORIENTED_EDGE('',*,*,#53876,.T.);
#78723=ORIENTED_EDGE('',*,*,#53880,.T.);
#78724=ORIENTED_EDGE('',*,*,#53883,.T.);
#78725=ORIENTED_EDGE('',*,*,#53886,.T.);
#78726=ORIENTED_EDGE('',*,*,#53889,.T.);
#78727=ORIENTED_EDGE('',*,*,#54291,.F.);
#78728=ORIENTED_EDGE('',*,*,#53934,.T.);
#78729=ORIENTED_EDGE('',*,*,#53931,.T.);
#78730=ORIENTED_EDGE('',*,*,#53928,.T.);
#78731=ORIENTED_EDGE('',*,*,#54292,.T.);
#78732=ORIENTED_EDGE('',*,*,#53912,.T.);
#78733=ORIENTED_EDGE('',*,*,#53909,.T.);
#78734=ORIENTED_EDGE('',*,*,#53906,.T.);
#78735=ORIENTED_EDGE('',*,*,#53903,.T.);
#78736=ORIENTED_EDGE('',*,*,#53900,.T.);
#78737=ORIENTED_EDGE('',*,*,#54293,.T.);
#78738=ORIENTED_EDGE('',*,*,#53959,.T.);
#78739=ORIENTED_EDGE('',*,*,#53956,.T.);
#78740=ORIENTED_EDGE('',*,*,#53953,.T.);
#78741=ORIENTED_EDGE('',*,*,#53950,.T.);
#78742=ORIENTED_EDGE('',*,*,#53947,.T.);
#78743=ORIENTED_EDGE('',*,*,#53944,.T.);
#78744=ORIENTED_EDGE('',*,*,#54294,.T.);
#78745=ORIENTED_EDGE('',*,*,#53987,.T.);
#78746=ORIENTED_EDGE('',*,*,#53984,.T.);
#78747=ORIENTED_EDGE('',*,*,#53981,.T.);
#78748=ORIENTED_EDGE('',*,*,#53978,.T.);
#78749=ORIENTED_EDGE('',*,*,#53975,.T.);
#78750=ORIENTED_EDGE('',*,*,#54295,.T.);
#78751=ORIENTED_EDGE('',*,*,#54015,.T.);
#78752=ORIENTED_EDGE('',*,*,#54012,.T.);
#78753=ORIENTED_EDGE('',*,*,#54009,.T.);
#78754=ORIENTED_EDGE('',*,*,#54006,.T.);
#78755=ORIENTED_EDGE('',*,*,#54003,.T.);
#78756=ORIENTED_EDGE('',*,*,#54296,.T.);
#78757=ORIENTED_EDGE('',*,*,#54043,.T.);
#78758=ORIENTED_EDGE('',*,*,#54040,.T.);
#78759=ORIENTED_EDGE('',*,*,#54037,.T.);
#78760=ORIENTED_EDGE('',*,*,#54034,.T.);
#78761=ORIENTED_EDGE('',*,*,#54031,.T.);
#78762=ORIENTED_EDGE('',*,*,#54297,.T.);
#78763=ORIENTED_EDGE('',*,*,#54071,.T.);
#78764=ORIENTED_EDGE('',*,*,#54068,.T.);
#78765=ORIENTED_EDGE('',*,*,#54065,.T.);
#78766=ORIENTED_EDGE('',*,*,#54062,.T.);
#78767=ORIENTED_EDGE('',*,*,#54059,.T.);
#78768=ORIENTED_EDGE('',*,*,#54298,.T.);
#78769=ORIENTED_EDGE('',*,*,#54099,.T.);
#78770=ORIENTED_EDGE('',*,*,#54096,.T.);
#78771=ORIENTED_EDGE('',*,*,#54093,.T.);
#78772=ORIENTED_EDGE('',*,*,#54090,.T.);
#78773=ORIENTED_EDGE('',*,*,#54087,.T.);
#78774=ORIENTED_EDGE('',*,*,#54299,.T.);
#78775=ORIENTED_EDGE('',*,*,#54127,.T.);
#78776=ORIENTED_EDGE('',*,*,#54124,.T.);
#78777=ORIENTED_EDGE('',*,*,#54121,.T.);
#78778=ORIENTED_EDGE('',*,*,#54118,.T.);
#78779=ORIENTED_EDGE('',*,*,#54115,.T.);
#78780=ORIENTED_EDGE('',*,*,#54300,.T.);
#78781=ORIENTED_EDGE('',*,*,#54158,.T.);
#78782=ORIENTED_EDGE('',*,*,#54155,.T.);
#78783=ORIENTED_EDGE('',*,*,#54152,.T.);
#78784=ORIENTED_EDGE('',*,*,#54149,.T.);
#78785=ORIENTED_EDGE('',*,*,#54146,.T.);
#78786=ORIENTED_EDGE('',*,*,#54143,.T.);
#78787=ORIENTED_EDGE('',*,*,#54301,.T.);
#78788=ORIENTED_EDGE('',*,*,#54186,.T.);
#78789=ORIENTED_EDGE('',*,*,#54183,.T.);
#78790=ORIENTED_EDGE('',*,*,#54180,.T.);
#78791=ORIENTED_EDGE('',*,*,#54177,.T.);
#78792=ORIENTED_EDGE('',*,*,#54174,.T.);
#78793=ORIENTED_EDGE('',*,*,#54302,.T.);
#78794=ORIENTED_EDGE('',*,*,#54202,.T.);
#78795=ORIENTED_EDGE('',*,*,#54303,.F.);
#78796=ORIENTED_EDGE('',*,*,#53922,.T.);
#78797=ORIENTED_EDGE('',*,*,#53924,.T.);
#78798=ORIENTED_EDGE('',*,*,#53927,.T.);
#78799=ORIENTED_EDGE('',*,*,#54209,.T.);
#78800=ORIENTED_EDGE('',*,*,#54288,.T.);
#78801=ORIENTED_EDGE('',*,*,#53872,.T.);
#78802=ORIENTED_EDGE('',*,*,#54304,.F.);
#78803=ORIENTED_EDGE('',*,*,#54305,.F.);
#78804=ORIENTED_EDGE('',*,*,#54306,.T.);
#78805=ORIENTED_EDGE('',*,*,#54304,.T.);
#78806=ORIENTED_EDGE('',*,*,#53874,.T.);
#78807=ORIENTED_EDGE('',*,*,#54221,.T.);
#78808=ORIENTED_EDGE('',*,*,#54307,.F.);
#78809=ORIENTED_EDGE('',*,*,#54213,.T.);
#78810=ORIENTED_EDGE('',*,*,#53884,.T.);
#78811=ORIENTED_EDGE('',*,*,#54284,.T.);
#78812=ORIENTED_EDGE('',*,*,#54308,.F.);
#78813=ORIENTED_EDGE('',*,*,#54285,.T.);
#78814=ORIENTED_EDGE('',*,*,#53878,.T.);
#78815=ORIENTED_EDGE('',*,*,#54309,.F.);
#78816=ORIENTED_EDGE('',*,*,#54310,.F.);
#78817=ORIENTED_EDGE('',*,*,#54282,.T.);
#78818=ORIENTED_EDGE('',*,*,#53911,.T.);
#78819=ORIENTED_EDGE('',*,*,#53914,.T.);
#78820=ORIENTED_EDGE('',*,*,#53917,.T.);
#78821=ORIENTED_EDGE('',*,*,#54311,.F.);
#78822=ORIENTED_EDGE('',*,*,#54312,.F.);
#78823=ORIENTED_EDGE('',*,*,#53892,.T.);
#78824=ORIENTED_EDGE('',*,*,#53896,.T.);
#78825=ORIENTED_EDGE('',*,*,#53899,.T.);
#78826=ORIENTED_EDGE('',*,*,#54278,.T.);
#78827=ORIENTED_EDGE('',*,*,#54246,.T.);
#78828=ORIENTED_EDGE('',*,*,#54098,.T.);
#78829=ORIENTED_EDGE('',*,*,#54101,.T.);
#78830=ORIENTED_EDGE('',*,*,#54104,.T.);
#78831=ORIENTED_EDGE('',*,*,#54313,.F.);
#78832=ORIENTED_EDGE('',*,*,#54314,.F.);
#78833=ORIENTED_EDGE('',*,*,#54079,.T.);
#78834=ORIENTED_EDGE('',*,*,#54083,.T.);
#78835=ORIENTED_EDGE('',*,*,#54086,.T.);
#78836=ORIENTED_EDGE('',*,*,#54233,.T.);
#78837=ORIENTED_EDGE('',*,*,#54249,.T.);
#78838=ORIENTED_EDGE('',*,*,#54126,.T.);
#78839=ORIENTED_EDGE('',*,*,#54129,.T.);
#78840=ORIENTED_EDGE('',*,*,#54132,.T.);
#78841=ORIENTED_EDGE('',*,*,#54315,.F.);
#78842=ORIENTED_EDGE('',*,*,#54316,.F.);
#78843=ORIENTED_EDGE('',*,*,#54107,.T.);
#78844=ORIENTED_EDGE('',*,*,#54111,.T.);
#78845=ORIENTED_EDGE('',*,*,#54114,.T.);
#78846=ORIENTED_EDGE('',*,*,#54230,.T.);
#78847=ORIENTED_EDGE('',*,*,#54317,.F.);
#78848=ORIENTED_EDGE('',*,*,#54135,.T.);
#78849=ORIENTED_EDGE('',*,*,#54139,.T.);
#78850=ORIENTED_EDGE('',*,*,#54142,.T.);
#78851=ORIENTED_EDGE('',*,*,#54227,.T.);
#78852=ORIENTED_EDGE('',*,*,#54276,.T.);
#78853=ORIENTED_EDGE('',*,*,#53958,.T.);
#78854=ORIENTED_EDGE('',*,*,#53961,.T.);
#78855=ORIENTED_EDGE('',*,*,#53964,.T.);
#78856=ORIENTED_EDGE('',*,*,#54318,.F.);
#78857=ORIENTED_EDGE('',*,*,#54243,.T.);
#78858=ORIENTED_EDGE('',*,*,#54070,.T.);
#78859=ORIENTED_EDGE('',*,*,#54073,.T.);
#78860=ORIENTED_EDGE('',*,*,#54076,.T.);
#78861=ORIENTED_EDGE('',*,*,#54319,.F.);
#78862=ORIENTED_EDGE('',*,*,#54320,.F.);
#78863=ORIENTED_EDGE('',*,*,#54051,.T.);
#78864=ORIENTED_EDGE('',*,*,#54055,.T.);
#78865=ORIENTED_EDGE('',*,*,#54058,.T.);
#78866=ORIENTED_EDGE('',*,*,#54236,.T.);
#78867=ORIENTED_EDGE('',*,*,#54321,.F.);
#78868=ORIENTED_EDGE('',*,*,#54105,.T.);
#78869=ORIENTED_EDGE('',*,*,#54322,.T.);
#78870=ORIENTED_EDGE('',*,*,#54053,.T.);
#78871=ORIENTED_EDGE('',*,*,#54322,.F.);
#78872=ORIENTED_EDGE('',*,*,#54102,.T.);
#78873=ORIENTED_EDGE('',*,*,#54298,.F.);
#78874=ORIENTED_EDGE('',*,*,#54056,.T.);
#78875=ORIENTED_EDGE('',*,*,#54237,.T.);
#78876=ORIENTED_EDGE('',*,*,#54064,.T.);
#78877=ORIENTED_EDGE('',*,*,#54242,.T.);
#78878=ORIENTED_EDGE('',*,*,#54323,.F.);
#78879=ORIENTED_EDGE('',*,*,#54258,.T.);
#78880=ORIENTED_EDGE('',*,*,#54042,.T.);
#78881=ORIENTED_EDGE('',*,*,#54045,.T.);
#78882=ORIENTED_EDGE('',*,*,#54048,.T.);
#78883=ORIENTED_EDGE('',*,*,#54324,.F.);
#78884=ORIENTED_EDGE('',*,*,#54325,.F.);
#78885=ORIENTED_EDGE('',*,*,#54023,.T.);
#78886=ORIENTED_EDGE('',*,*,#54027,.T.);
#78887=ORIENTED_EDGE('',*,*,#54030,.T.);
#78888=ORIENTED_EDGE('',*,*,#54239,.T.);
#78889=ORIENTED_EDGE('',*,*,#54326,.F.);
#78890=ORIENTED_EDGE('',*,*,#54077,.T.);
#78891=ORIENTED_EDGE('',*,*,#54327,.T.);
#78892=ORIENTED_EDGE('',*,*,#54025,.T.);
#78893=ORIENTED_EDGE('',*,*,#54327,.F.);
#78894=ORIENTED_EDGE('',*,*,#54074,.T.);
#78895=ORIENTED_EDGE('',*,*,#54297,.F.);
#78896=ORIENTED_EDGE('',*,*,#54028,.T.);
#78897=ORIENTED_EDGE('',*,*,#54240,.T.);
#78898=ORIENTED_EDGE('',*,*,#54036,.T.);
#78899=ORIENTED_EDGE('',*,*,#54257,.T.);
#78900=ORIENTED_EDGE('',*,*,#54328,.F.);
#78901=ORIENTED_EDGE('',*,*,#54264,.T.);
#78902=ORIENTED_EDGE('',*,*,#54014,.T.);
#78903=ORIENTED_EDGE('',*,*,#54017,.T.);
#78904=ORIENTED_EDGE('',*,*,#54020,.T.);
#78905=ORIENTED_EDGE('',*,*,#54329,.F.);
#78906=ORIENTED_EDGE('',*,*,#54330,.F.);
#78907=ORIENTED_EDGE('',*,*,#53995,.T.);
#78908=ORIENTED_EDGE('',*,*,#53999,.T.);
#78909=ORIENTED_EDGE('',*,*,#54002,.T.);
#78910=ORIENTED_EDGE('',*,*,#54260,.T.);
#78911=ORIENTED_EDGE('',*,*,#54331,.F.);
#78912=ORIENTED_EDGE('',*,*,#54049,.T.);
#78913=ORIENTED_EDGE('',*,*,#54332,.T.);
#78914=ORIENTED_EDGE('',*,*,#53997,.T.);
#78915=ORIENTED_EDGE('',*,*,#54332,.F.);
#78916=ORIENTED_EDGE('',*,*,#54046,.T.);
#78917=ORIENTED_EDGE('',*,*,#54296,.F.);
#78918=ORIENTED_EDGE('',*,*,#54000,.T.);
#78919=ORIENTED_EDGE('',*,*,#54261,.T.);
#78920=ORIENTED_EDGE('',*,*,#54008,.T.);
#78921=ORIENTED_EDGE('',*,*,#54263,.T.);
#78922=ORIENTED_EDGE('',*,*,#54333,.F.);
#78923=ORIENTED_EDGE('',*,*,#54273,.T.);
#78924=ORIENTED_EDGE('',*,*,#53986,.T.);
#78925=ORIENTED_EDGE('',*,*,#53989,.T.);
#78926=ORIENTED_EDGE('',*,*,#53992,.T.);
#78927=ORIENTED_EDGE('',*,*,#54334,.F.);
#78928=ORIENTED_EDGE('',*,*,#54335,.F.);
#78929=ORIENTED_EDGE('',*,*,#53967,.T.);
#78930=ORIENTED_EDGE('',*,*,#53971,.T.);
#78931=ORIENTED_EDGE('',*,*,#53974,.T.);
#78932=ORIENTED_EDGE('',*,*,#54266,.T.);
#78933=ORIENTED_EDGE('',*,*,#54336,.F.);
#78934=ORIENTED_EDGE('',*,*,#54021,.T.);
#78935=ORIENTED_EDGE('',*,*,#54337,.T.);
#78936=ORIENTED_EDGE('',*,*,#53969,.T.);
#78937=ORIENTED_EDGE('',*,*,#54337,.F.);
#78938=ORIENTED_EDGE('',*,*,#54018,.T.);
#78939=ORIENTED_EDGE('',*,*,#54295,.F.);
#78940=ORIENTED_EDGE('',*,*,#53972,.T.);
#78941=ORIENTED_EDGE('',*,*,#54267,.T.);
#78942=ORIENTED_EDGE('',*,*,#53980,.T.);
#78943=ORIENTED_EDGE('',*,*,#54272,.T.);
#78944=ORIENTED_EDGE('',*,*,#54338,.F.);
#78945=ORIENTED_EDGE('',*,*,#54255,.T.);
#78946=ORIENTED_EDGE('',*,*,#54185,.T.);
#78947=ORIENTED_EDGE('',*,*,#54188,.T.);
#78948=ORIENTED_EDGE('',*,*,#54191,.T.);
#78949=ORIENTED_EDGE('',*,*,#54339,.F.);
#78950=ORIENTED_EDGE('',*,*,#54340,.F.);
#78951=ORIENTED_EDGE('',*,*,#54166,.T.);
#78952=ORIENTED_EDGE('',*,*,#54170,.T.);
#78953=ORIENTED_EDGE('',*,*,#54173,.T.);
#78954=ORIENTED_EDGE('',*,*,#54224,.T.);
#78955=ORIENTED_EDGE('',*,*,#54341,.F.);
#78956=ORIENTED_EDGE('',*,*,#54208,.T.);
#78957=ORIENTED_EDGE('',*,*,#54342,.T.);
#78958=ORIENTED_EDGE('',*,*,#54168,.T.);
#78959=ORIENTED_EDGE('',*,*,#54342,.F.);
#78960=ORIENTED_EDGE('',*,*,#54205,.T.);
#78961=ORIENTED_EDGE('',*,*,#54302,.F.);
#78962=ORIENTED_EDGE('',*,*,#54171,.T.);
#78963=ORIENTED_EDGE('',*,*,#54225,.T.);
#78964=ORIENTED_EDGE('',*,*,#54179,.T.);
#78965=ORIENTED_EDGE('',*,*,#54254,.T.);
#78966=ORIENTED_EDGE('',*,*,#54343,.F.);
#78967=ORIENTED_EDGE('',*,*,#54270,.T.);
#78968=ORIENTED_EDGE('',*,*,#53949,.T.);
#78969=ORIENTED_EDGE('',*,*,#54344,.F.);
#78970=ORIENTED_EDGE('',*,*,#54345,.F.);
#78971=ORIENTED_EDGE('',*,*,#54344,.T.);
#78972=ORIENTED_EDGE('',*,*,#53952,.T.);
#78973=ORIENTED_EDGE('',*,*,#54275,.T.);
#78974=ORIENTED_EDGE('',*,*,#54346,.F.);
#78975=ORIENTED_EDGE('',*,*,#54347,.F.);
#78976=ORIENTED_EDGE('',*,*,#54151,.T.);
#78977=ORIENTED_EDGE('',*,*,#54251,.T.);
#78978=ORIENTED_EDGE('',*,*,#54348,.F.);
#78979=ORIENTED_EDGE('',*,*,#54252,.T.);
#78980=ORIENTED_EDGE('',*,*,#54157,.T.);
#78981=ORIENTED_EDGE('',*,*,#54160,.T.);
#78982=ORIENTED_EDGE('',*,*,#54163,.T.);
#78983=ORIENTED_EDGE('',*,*,#54349,.F.);
#78984=ORIENTED_EDGE('',*,*,#54350,.T.);
#78985=ORIENTED_EDGE('',*,*,#54206,.T.);
#78986=ORIENTED_EDGE('',*,*,#54341,.T.);
#78987=ORIENTED_EDGE('',*,*,#54167,.T.);
#78988=ORIENTED_EDGE('',*,*,#54340,.T.);
#78989=ORIENTED_EDGE('',*,*,#54226,.T.);
#78990=ORIENTED_EDGE('',*,*,#54343,.T.);
#78991=ORIENTED_EDGE('',*,*,#54256,.T.);
#78992=ORIENTED_EDGE('',*,*,#54339,.T.);
#78993=ORIENTED_EDGE('',*,*,#54190,.T.);
#78994=ORIENTED_EDGE('',*,*,#54351,.T.);
#78995=ORIENTED_EDGE('',*,*,#54136,.T.);
#78996=ORIENTED_EDGE('',*,*,#54317,.T.);
#78997=ORIENTED_EDGE('',*,*,#54229,.T.);
#78998=ORIENTED_EDGE('',*,*,#54352,.T.);
#78999=ORIENTED_EDGE('',*,*,#54348,.T.);
#79000=ORIENTED_EDGE('',*,*,#54253,.T.);
#79001=ORIENTED_EDGE('',*,*,#54349,.T.);
#79002=ORIENTED_EDGE('',*,*,#54162,.T.);
#79003=ORIENTED_EDGE('',*,*,#54353,.T.);
#79004=ORIENTED_EDGE('',*,*,#54108,.T.);
#79005=ORIENTED_EDGE('',*,*,#54316,.T.);
#79006=ORIENTED_EDGE('',*,*,#54232,.T.);
#79007=ORIENTED_EDGE('',*,*,#54354,.T.);
#79008=ORIENTED_EDGE('',*,*,#54250,.T.);
#79009=ORIENTED_EDGE('',*,*,#54315,.T.);
#79010=ORIENTED_EDGE('',*,*,#54131,.T.);
#79011=ORIENTED_EDGE('',*,*,#54355,.T.);
#79012=ORIENTED_EDGE('',*,*,#54080,.T.);
#79013=ORIENTED_EDGE('',*,*,#54314,.T.);
#79014=ORIENTED_EDGE('',*,*,#54235,.T.);
#79015=ORIENTED_EDGE('',*,*,#54356,.T.);
#79016=ORIENTED_EDGE('',*,*,#54247,.T.);
#79017=ORIENTED_EDGE('',*,*,#54313,.T.);
#79018=ORIENTED_EDGE('',*,*,#54103,.T.);
#79019=ORIENTED_EDGE('',*,*,#54321,.T.);
#79020=ORIENTED_EDGE('',*,*,#54052,.T.);
#79021=ORIENTED_EDGE('',*,*,#54320,.T.);
#79022=ORIENTED_EDGE('',*,*,#54238,.T.);
#79023=ORIENTED_EDGE('',*,*,#54323,.T.);
#79024=ORIENTED_EDGE('',*,*,#54244,.T.);
#79025=ORIENTED_EDGE('',*,*,#54319,.T.);
#79026=ORIENTED_EDGE('',*,*,#54075,.T.);
#79027=ORIENTED_EDGE('',*,*,#54326,.T.);
#79028=ORIENTED_EDGE('',*,*,#54024,.T.);
#79029=ORIENTED_EDGE('',*,*,#54325,.T.);
#79030=ORIENTED_EDGE('',*,*,#54241,.T.);
#79031=ORIENTED_EDGE('',*,*,#54328,.T.);
#79032=ORIENTED_EDGE('',*,*,#54259,.T.);
#79033=ORIENTED_EDGE('',*,*,#54324,.T.);
#79034=ORIENTED_EDGE('',*,*,#54047,.T.);
#79035=ORIENTED_EDGE('',*,*,#54331,.T.);
#79036=ORIENTED_EDGE('',*,*,#53996,.T.);
#79037=ORIENTED_EDGE('',*,*,#54330,.T.);
#79038=ORIENTED_EDGE('',*,*,#54262,.T.);
#79039=ORIENTED_EDGE('',*,*,#54333,.T.);
#79040=ORIENTED_EDGE('',*,*,#54265,.T.);
#79041=ORIENTED_EDGE('',*,*,#54329,.T.);
#79042=ORIENTED_EDGE('',*,*,#54019,.T.);
#79043=ORIENTED_EDGE('',*,*,#54336,.T.);
#79044=ORIENTED_EDGE('',*,*,#53968,.T.);
#79045=ORIENTED_EDGE('',*,*,#54335,.T.);
#79046=ORIENTED_EDGE('',*,*,#54268,.T.);
#79047=ORIENTED_EDGE('',*,*,#54338,.T.);
#79048=ORIENTED_EDGE('',*,*,#54274,.T.);
#79049=ORIENTED_EDGE('',*,*,#54334,.T.);
#79050=ORIENTED_EDGE('',*,*,#53991,.T.);
#79051=ORIENTED_EDGE('',*,*,#54357,.T.);
#79052=ORIENTED_EDGE('',*,*,#53937,.T.);
#79053=ORIENTED_EDGE('',*,*,#54358,.T.);
#79054=ORIENTED_EDGE('',*,*,#54271,.T.);
#79055=ORIENTED_EDGE('',*,*,#54345,.T.);
#79056=ORIENTED_EDGE('',*,*,#54346,.T.);
#79057=ORIENTED_EDGE('',*,*,#54277,.T.);
#79058=ORIENTED_EDGE('',*,*,#54318,.T.);
#79059=ORIENTED_EDGE('',*,*,#53963,.T.);
#79060=ORIENTED_EDGE('',*,*,#54359,.T.);
#79061=ORIENTED_EDGE('',*,*,#53893,.T.);
#79062=ORIENTED_EDGE('',*,*,#54312,.T.);
#79063=ORIENTED_EDGE('',*,*,#54280,.T.);
#79064=ORIENTED_EDGE('',*,*,#54360,.T.);
#79065=ORIENTED_EDGE('',*,*,#54283,.T.);
#79066=ORIENTED_EDGE('',*,*,#54311,.T.);
#79067=ORIENTED_EDGE('',*,*,#53916,.T.);
#79068=ORIENTED_EDGE('',*,*,#54361,.T.);
#79069=ORIENTED_EDGE('',*,*,#53919,.T.);
#79070=ORIENTED_EDGE('',*,*,#54303,.T.);
#79071=ORIENTED_EDGE('',*,*,#54211,.T.);
#79072=ORIENTED_EDGE('',*,*,#54362,.T.);
#79073=ORIENTED_EDGE('',*,*,#54363,.T.);
#79074=ORIENTED_EDGE('',*,*,#54364,.T.);
#79075=ORIENTED_EDGE('',*,*,#54214,.T.);
#79076=ORIENTED_EDGE('',*,*,#54308,.T.);
#79077=ORIENTED_EDGE('',*,*,#54286,.T.);
#79078=ORIENTED_EDGE('',*,*,#54310,.T.);
#79079=ORIENTED_EDGE('',*,*,#54365,.T.);
#79080=ORIENTED_EDGE('',*,*,#54366,.T.);
#79081=ORIENTED_EDGE('',*,*,#54305,.T.);
#79082=ORIENTED_EDGE('',*,*,#54307,.T.);
#79083=ORIENTED_EDGE('',*,*,#54223,.T.);
#79084=ORIENTED_EDGE('',*,*,#54367,.T.);
#79085=ORIENTED_EDGE('',*,*,#54220,.T.);
#79086=ORIENTED_EDGE('',*,*,#54368,.T.);
#79087=ORIENTED_EDGE('',*,*,#54369,.T.);
#79088=ORIENTED_EDGE('',*,*,#54370,.T.);
#79089=ORIENTED_EDGE('',*,*,#54217,.T.);
#79090=ORIENTED_EDGE('',*,*,#54228,.T.);
#79091=ORIENTED_EDGE('',*,*,#54148,.T.);
#79092=ORIENTED_EDGE('',*,*,#54347,.T.);
#79093=ORIENTED_EDGE('',*,*,#54352,.F.);
#79094=ORIENTED_EDGE('',*,*,#54358,.F.);
#79095=ORIENTED_EDGE('',*,*,#53936,.T.);
#79096=ORIENTED_EDGE('',*,*,#53940,.T.);
#79097=ORIENTED_EDGE('',*,*,#53943,.T.);
#79098=ORIENTED_EDGE('',*,*,#54269,.T.);
#79099=ORIENTED_EDGE('',*,*,#54301,.F.);
#79100=ORIENTED_EDGE('',*,*,#54140,.T.);
#79101=ORIENTED_EDGE('',*,*,#54371,.F.);
#79102=ORIENTED_EDGE('',*,*,#54189,.T.);
#79103=ORIENTED_EDGE('',*,*,#54351,.F.);
#79104=ORIENTED_EDGE('',*,*,#54192,.T.);
#79105=ORIENTED_EDGE('',*,*,#54371,.T.);
#79106=ORIENTED_EDGE('',*,*,#54137,.T.);
#79107=ORIENTED_EDGE('',*,*,#54294,.F.);
#79108=ORIENTED_EDGE('',*,*,#53941,.T.);
#79109=ORIENTED_EDGE('',*,*,#54372,.F.);
#79110=ORIENTED_EDGE('',*,*,#53990,.T.);
#79111=ORIENTED_EDGE('',*,*,#54357,.F.);
#79112=ORIENTED_EDGE('',*,*,#53993,.T.);
#79113=ORIENTED_EDGE('',*,*,#54372,.T.);
#79114=ORIENTED_EDGE('',*,*,#53938,.T.);
#79115=ORIENTED_EDGE('',*,*,#54293,.F.);
#79116=ORIENTED_EDGE('',*,*,#53897,.T.);
#79117=ORIENTED_EDGE('',*,*,#54373,.F.);
#79118=ORIENTED_EDGE('',*,*,#53962,.T.);
#79119=ORIENTED_EDGE('',*,*,#54359,.F.);
#79120=ORIENTED_EDGE('',*,*,#53965,.T.);
#79121=ORIENTED_EDGE('',*,*,#54373,.T.);
#79122=ORIENTED_EDGE('',*,*,#53894,.T.);
#79123=ORIENTED_EDGE('',*,*,#54300,.F.);
#79124=ORIENTED_EDGE('',*,*,#54112,.T.);
#79125=ORIENTED_EDGE('',*,*,#54374,.F.);
#79126=ORIENTED_EDGE('',*,*,#54161,.T.);
#79127=ORIENTED_EDGE('',*,*,#54353,.F.);
#79128=ORIENTED_EDGE('',*,*,#54164,.T.);
#79129=ORIENTED_EDGE('',*,*,#54374,.T.);
#79130=ORIENTED_EDGE('',*,*,#54109,.T.);
#79131=ORIENTED_EDGE('',*,*,#54231,.T.);
#79132=ORIENTED_EDGE('',*,*,#54120,.T.);
#79133=ORIENTED_EDGE('',*,*,#54248,.T.);
#79134=ORIENTED_EDGE('',*,*,#54354,.F.);
#79135=ORIENTED_EDGE('',*,*,#54299,.F.);
#79136=ORIENTED_EDGE('',*,*,#54084,.T.);
#79137=ORIENTED_EDGE('',*,*,#54375,.F.);
#79138=ORIENTED_EDGE('',*,*,#54130,.T.);
#79139=ORIENTED_EDGE('',*,*,#54355,.F.);
#79140=ORIENTED_EDGE('',*,*,#54133,.T.);
#79141=ORIENTED_EDGE('',*,*,#54375,.T.);
#79142=ORIENTED_EDGE('',*,*,#54081,.T.);
#79143=ORIENTED_EDGE('',*,*,#54234,.T.);
#79144=ORIENTED_EDGE('',*,*,#54092,.T.);
#79145=ORIENTED_EDGE('',*,*,#54245,.T.);
#79146=ORIENTED_EDGE('',*,*,#54356,.F.);
#79147=ORIENTED_EDGE('',*,*,#54279,.T.);
#79148=ORIENTED_EDGE('',*,*,#53905,.T.);
#79149=ORIENTED_EDGE('',*,*,#54281,.T.);
#79150=ORIENTED_EDGE('',*,*,#54360,.F.);
#79151=ORIENTED_EDGE('',*,*,#54292,.F.);
#79152=ORIENTED_EDGE('',*,*,#53925,.T.);
#79153=ORIENTED_EDGE('',*,*,#54376,.F.);
#79154=ORIENTED_EDGE('',*,*,#53915,.T.);
#79155=ORIENTED_EDGE('',*,*,#54376,.T.);
#79156=ORIENTED_EDGE('',*,*,#53920,.T.);
#79157=ORIENTED_EDGE('',*,*,#54361,.F.);
#79158=ORIENTED_EDGE('',*,*,#53918,.T.);
#79159=ORIENTED_EDGE('',*,*,#54377,.T.);
#79160=ORIENTED_EDGE('',*,*,#53890,.T.);
#79161=ORIENTED_EDGE('',*,*,#54212,.T.);
#79162=ORIENTED_EDGE('',*,*,#54364,.F.);
#79163=ORIENTED_EDGE('',*,*,#54309,.T.);
#79164=ORIENTED_EDGE('',*,*,#53877,.T.);
#79165=ORIENTED_EDGE('',*,*,#54290,.T.);
#79166=ORIENTED_EDGE('',*,*,#54378,.F.);
#79167=ORIENTED_EDGE('',*,*,#54365,.F.);
#79168=ORIENTED_EDGE('',*,*,#54378,.T.);
#79169=ORIENTED_EDGE('',*,*,#54289,.T.);
#79170=ORIENTED_EDGE('',*,*,#54306,.F.);
#79171=ORIENTED_EDGE('',*,*,#54366,.F.);
#79172=ORIENTED_EDGE('',*,*,#54222,.T.);
#79173=ORIENTED_EDGE('',*,*,#53868,.T.);
#79174=ORIENTED_EDGE('',*,*,#54218,.T.);
#79175=ORIENTED_EDGE('',*,*,#54367,.F.);
#79176=ORIENTED_EDGE('',*,*,#54219,.T.);
#79177=ORIENTED_EDGE('',*,*,#53862,.T.);
#79178=ORIENTED_EDGE('',*,*,#54379,.F.);
#79179=ORIENTED_EDGE('',*,*,#54368,.F.);
#79180=ORIENTED_EDGE('',*,*,#54287,.T.);
#79181=ORIENTED_EDGE('',*,*,#54193,.T.);
#79182=ORIENTED_EDGE('',*,*,#54380,.F.);
#79183=ORIENTED_EDGE('',*,*,#54369,.F.);
#79184=ORIENTED_EDGE('',*,*,#54379,.T.);
#79185=ORIENTED_EDGE('',*,*,#53861,.T.);
#79186=ORIENTED_EDGE('',*,*,#54380,.T.);
#79187=ORIENTED_EDGE('',*,*,#54196,.T.);
#79188=ORIENTED_EDGE('',*,*,#54215,.T.);
#79189=ORIENTED_EDGE('',*,*,#54370,.F.);
#79190=ORIENTED_EDGE('',*,*,#54216,.T.);
#79191=ORIENTED_EDGE('',*,*,#54201,.T.);
#79192=ORIENTED_EDGE('',*,*,#54204,.T.);
#79193=ORIENTED_EDGE('',*,*,#54207,.T.);
#79194=ORIENTED_EDGE('',*,*,#54350,.F.);
#79195=ORIENTED_EDGE('',*,*,#54210,.T.);
#79196=ORIENTED_EDGE('',*,*,#53933,.T.);
#79197=ORIENTED_EDGE('',*,*,#54381,.F.);
#79198=ORIENTED_EDGE('',*,*,#54362,.F.);
#79199=ORIENTED_EDGE('',*,*,#54381,.T.);
#79200=ORIENTED_EDGE('',*,*,#53932,.T.);
#79201=ORIENTED_EDGE('',*,*,#54291,.T.);
#79202=ORIENTED_EDGE('',*,*,#53888,.T.);
#79203=ORIENTED_EDGE('',*,*,#54377,.F.);
#79204=ORIENTED_EDGE('',*,*,#54363,.F.);
#79205=ORIENTED_EDGE('',*,*,#54382,.T.);
#79206=ORIENTED_EDGE('',*,*,#54383,.T.);
#79207=ORIENTED_EDGE('',*,*,#54384,.T.);
#79208=ORIENTED_EDGE('',*,*,#54385,.T.);
#79209=ORIENTED_EDGE('',*,*,#54386,.T.);
#79210=ORIENTED_EDGE('',*,*,#54387,.T.);
#79211=ORIENTED_EDGE('',*,*,#54388,.T.);
#79212=ORIENTED_EDGE('',*,*,#54383,.F.);
#79213=ORIENTED_EDGE('',*,*,#54389,.T.);
#79214=ORIENTED_EDGE('',*,*,#54390,.T.);
#79215=ORIENTED_EDGE('',*,*,#54391,.T.);
#79216=ORIENTED_EDGE('',*,*,#54384,.F.);
#79217=ORIENTED_EDGE('',*,*,#54392,.T.);
#79218=ORIENTED_EDGE('',*,*,#54393,.T.);
#79219=ORIENTED_EDGE('',*,*,#54385,.F.);
#79220=ORIENTED_EDGE('',*,*,#54394,.T.);
#79221=ORIENTED_EDGE('',*,*,#54395,.T.);
#79222=ORIENTED_EDGE('',*,*,#54386,.F.);
#79223=ORIENTED_EDGE('',*,*,#54396,.T.);
#79224=ORIENTED_EDGE('',*,*,#54397,.T.);
#79225=ORIENTED_EDGE('',*,*,#54387,.F.);
#79226=ORIENTED_EDGE('',*,*,#54398,.T.);
#79227=ORIENTED_EDGE('',*,*,#54399,.T.);
#79228=ORIENTED_EDGE('',*,*,#54382,.F.);
#79229=ORIENTED_EDGE('',*,*,#54400,.F.);
#79230=ORIENTED_EDGE('',*,*,#54401,.T.);
#79231=ORIENTED_EDGE('',*,*,#54402,.T.);
#79232=ORIENTED_EDGE('',*,*,#54403,.T.);
#79233=ORIENTED_EDGE('',*,*,#54404,.T.);
#79234=ORIENTED_EDGE('',*,*,#54405,.T.);
#79235=ORIENTED_EDGE('',*,*,#54401,.F.);
#79236=ORIENTED_EDGE('',*,*,#54406,.F.);
#79237=ORIENTED_EDGE('',*,*,#54407,.F.);
#79238=ORIENTED_EDGE('',*,*,#54402,.F.);
#79239=ORIENTED_EDGE('',*,*,#54408,.F.);
#79240=ORIENTED_EDGE('',*,*,#54409,.F.);
#79241=ORIENTED_EDGE('',*,*,#54403,.F.);
#79242=ORIENTED_EDGE('',*,*,#54410,.F.);
#79243=ORIENTED_EDGE('',*,*,#54411,.F.);
#79244=ORIENTED_EDGE('',*,*,#54404,.F.);
#79245=ORIENTED_EDGE('',*,*,#54412,.F.);
#79246=ORIENTED_EDGE('',*,*,#54413,.F.);
#79247=ORIENTED_EDGE('',*,*,#54405,.F.);
#79248=ORIENTED_EDGE('',*,*,#54414,.F.);
#79249=ORIENTED_EDGE('',*,*,#54415,.F.);
#79250=ORIENTED_EDGE('',*,*,#54416,.F.);
#79251=ORIENTED_EDGE('',*,*,#54400,.T.);
#79252=ORIENTED_EDGE('',*,*,#54417,.F.);
#79253=ORIENTED_EDGE('',*,*,#54399,.F.);
#79254=ORIENTED_EDGE('',*,*,#54418,.T.);
#79255=ORIENTED_EDGE('',*,*,#54406,.T.);
#79256=ORIENTED_EDGE('',*,*,#54416,.T.);
#79257=ORIENTED_EDGE('',*,*,#54419,.F.);
#79258=ORIENTED_EDGE('',*,*,#54389,.F.);
#79259=ORIENTED_EDGE('',*,*,#54397,.F.);
#79260=ORIENTED_EDGE('',*,*,#54420,.T.);
#79261=ORIENTED_EDGE('',*,*,#54408,.T.);
#79262=ORIENTED_EDGE('',*,*,#54407,.T.);
#79263=ORIENTED_EDGE('',*,*,#54418,.F.);
#79264=ORIENTED_EDGE('',*,*,#54398,.F.);
#79265=ORIENTED_EDGE('',*,*,#54395,.F.);
#79266=ORIENTED_EDGE('',*,*,#54421,.T.);
#79267=ORIENTED_EDGE('',*,*,#54410,.T.);
#79268=ORIENTED_EDGE('',*,*,#54409,.T.);
#79269=ORIENTED_EDGE('',*,*,#54420,.F.);
#79270=ORIENTED_EDGE('',*,*,#54396,.F.);
#79271=ORIENTED_EDGE('',*,*,#54393,.F.);
#79272=ORIENTED_EDGE('',*,*,#54422,.T.);
#79273=ORIENTED_EDGE('',*,*,#54412,.T.);
#79274=ORIENTED_EDGE('',*,*,#54411,.T.);
#79275=ORIENTED_EDGE('',*,*,#54421,.F.);
#79276=ORIENTED_EDGE('',*,*,#54394,.F.);
#79277=ORIENTED_EDGE('',*,*,#54391,.F.);
#79278=ORIENTED_EDGE('',*,*,#54423,.T.);
#79279=ORIENTED_EDGE('',*,*,#54414,.T.);
#79280=ORIENTED_EDGE('',*,*,#54413,.T.);
#79281=ORIENTED_EDGE('',*,*,#54422,.F.);
#79282=ORIENTED_EDGE('',*,*,#54392,.F.);
#79283=ORIENTED_EDGE('',*,*,#54388,.F.);
#79284=ORIENTED_EDGE('',*,*,#54419,.T.);
#79285=ORIENTED_EDGE('',*,*,#54417,.T.);
#79286=ORIENTED_EDGE('',*,*,#54415,.T.);
#79287=ORIENTED_EDGE('',*,*,#54423,.F.);
#79288=ORIENTED_EDGE('',*,*,#54390,.F.);
#79289=ORIENTED_EDGE('',*,*,#54424,.T.);
#79290=ORIENTED_EDGE('',*,*,#54425,.T.);
#79291=ORIENTED_EDGE('',*,*,#54426,.T.);
#79292=ORIENTED_EDGE('',*,*,#54427,.T.);
#79293=ORIENTED_EDGE('',*,*,#54428,.T.);
#79294=ORIENTED_EDGE('',*,*,#54429,.T.);
#79295=ORIENTED_EDGE('',*,*,#54430,.T.);
#79296=ORIENTED_EDGE('',*,*,#54425,.F.);
#79297=ORIENTED_EDGE('',*,*,#54431,.T.);
#79298=ORIENTED_EDGE('',*,*,#54432,.T.);
#79299=ORIENTED_EDGE('',*,*,#54433,.T.);
#79300=ORIENTED_EDGE('',*,*,#54426,.F.);
#79301=ORIENTED_EDGE('',*,*,#54434,.T.);
#79302=ORIENTED_EDGE('',*,*,#54435,.T.);
#79303=ORIENTED_EDGE('',*,*,#54427,.F.);
#79304=ORIENTED_EDGE('',*,*,#54436,.T.);
#79305=ORIENTED_EDGE('',*,*,#54437,.T.);
#79306=ORIENTED_EDGE('',*,*,#54428,.F.);
#79307=ORIENTED_EDGE('',*,*,#54438,.T.);
#79308=ORIENTED_EDGE('',*,*,#54439,.T.);
#79309=ORIENTED_EDGE('',*,*,#54429,.F.);
#79310=ORIENTED_EDGE('',*,*,#54440,.T.);
#79311=ORIENTED_EDGE('',*,*,#54441,.T.);
#79312=ORIENTED_EDGE('',*,*,#54424,.F.);
#79313=ORIENTED_EDGE('',*,*,#54442,.F.);
#79314=ORIENTED_EDGE('',*,*,#54443,.T.);
#79315=ORIENTED_EDGE('',*,*,#54444,.T.);
#79316=ORIENTED_EDGE('',*,*,#54445,.T.);
#79317=ORIENTED_EDGE('',*,*,#54446,.T.);
#79318=ORIENTED_EDGE('',*,*,#54447,.T.);
#79319=ORIENTED_EDGE('',*,*,#54443,.F.);
#79320=ORIENTED_EDGE('',*,*,#54448,.F.);
#79321=ORIENTED_EDGE('',*,*,#54449,.F.);
#79322=ORIENTED_EDGE('',*,*,#54444,.F.);
#79323=ORIENTED_EDGE('',*,*,#54450,.F.);
#79324=ORIENTED_EDGE('',*,*,#54451,.F.);
#79325=ORIENTED_EDGE('',*,*,#54445,.F.);
#79326=ORIENTED_EDGE('',*,*,#54452,.F.);
#79327=ORIENTED_EDGE('',*,*,#54453,.F.);
#79328=ORIENTED_EDGE('',*,*,#54446,.F.);
#79329=ORIENTED_EDGE('',*,*,#54454,.F.);
#79330=ORIENTED_EDGE('',*,*,#54455,.F.);
#79331=ORIENTED_EDGE('',*,*,#54447,.F.);
#79332=ORIENTED_EDGE('',*,*,#54456,.F.);
#79333=ORIENTED_EDGE('',*,*,#54457,.F.);
#79334=ORIENTED_EDGE('',*,*,#54458,.F.);
#79335=ORIENTED_EDGE('',*,*,#54442,.T.);
#79336=ORIENTED_EDGE('',*,*,#54459,.F.);
#79337=ORIENTED_EDGE('',*,*,#54441,.F.);
#79338=ORIENTED_EDGE('',*,*,#54460,.T.);
#79339=ORIENTED_EDGE('',*,*,#54448,.T.);
#79340=ORIENTED_EDGE('',*,*,#54458,.T.);
#79341=ORIENTED_EDGE('',*,*,#54461,.F.);
#79342=ORIENTED_EDGE('',*,*,#54431,.F.);
#79343=ORIENTED_EDGE('',*,*,#54439,.F.);
#79344=ORIENTED_EDGE('',*,*,#54462,.T.);
#79345=ORIENTED_EDGE('',*,*,#54450,.T.);
#79346=ORIENTED_EDGE('',*,*,#54449,.T.);
#79347=ORIENTED_EDGE('',*,*,#54460,.F.);
#79348=ORIENTED_EDGE('',*,*,#54440,.F.);
#79349=ORIENTED_EDGE('',*,*,#54437,.F.);
#79350=ORIENTED_EDGE('',*,*,#54463,.T.);
#79351=ORIENTED_EDGE('',*,*,#54452,.T.);
#79352=ORIENTED_EDGE('',*,*,#54451,.T.);
#79353=ORIENTED_EDGE('',*,*,#54462,.F.);
#79354=ORIENTED_EDGE('',*,*,#54438,.F.);
#79355=ORIENTED_EDGE('',*,*,#54435,.F.);
#79356=ORIENTED_EDGE('',*,*,#54464,.T.);
#79357=ORIENTED_EDGE('',*,*,#54454,.T.);
#79358=ORIENTED_EDGE('',*,*,#54453,.T.);
#79359=ORIENTED_EDGE('',*,*,#54463,.F.);
#79360=ORIENTED_EDGE('',*,*,#54436,.F.);
#79361=ORIENTED_EDGE('',*,*,#54433,.F.);
#79362=ORIENTED_EDGE('',*,*,#54465,.T.);
#79363=ORIENTED_EDGE('',*,*,#54456,.T.);
#79364=ORIENTED_EDGE('',*,*,#54455,.T.);
#79365=ORIENTED_EDGE('',*,*,#54464,.F.);
#79366=ORIENTED_EDGE('',*,*,#54434,.F.);
#79367=ORIENTED_EDGE('',*,*,#54430,.F.);
#79368=ORIENTED_EDGE('',*,*,#54461,.T.);
#79369=ORIENTED_EDGE('',*,*,#54459,.T.);
#79370=ORIENTED_EDGE('',*,*,#54457,.T.);
#79371=ORIENTED_EDGE('',*,*,#54465,.F.);
#79372=ORIENTED_EDGE('',*,*,#54432,.F.);
#79373=ORIENTED_EDGE('',*,*,#54466,.F.);
#79374=ORIENTED_EDGE('',*,*,#54467,.F.);
#79375=ORIENTED_EDGE('',*,*,#54468,.T.);
#79376=ORIENTED_EDGE('',*,*,#54469,.F.);
#79377=ORIENTED_EDGE('',*,*,#54470,.F.);
#79378=ORIENTED_EDGE('',*,*,#54471,.F.);
#79379=ORIENTED_EDGE('',*,*,#54466,.T.);
#79380=ORIENTED_EDGE('',*,*,#54472,.F.);
#79381=ORIENTED_EDGE('',*,*,#54473,.F.);
#79382=ORIENTED_EDGE('',*,*,#54474,.F.);
#79383=ORIENTED_EDGE('',*,*,#54470,.T.);
#79384=ORIENTED_EDGE('',*,*,#54475,.F.);
#79385=ORIENTED_EDGE('',*,*,#54476,.F.);
#79386=ORIENTED_EDGE('',*,*,#54477,.F.);
#79387=ORIENTED_EDGE('',*,*,#54473,.T.);
#79388=ORIENTED_EDGE('',*,*,#54478,.F.);
#79389=ORIENTED_EDGE('',*,*,#54479,.F.);
#79390=ORIENTED_EDGE('',*,*,#54480,.F.);
#79391=ORIENTED_EDGE('',*,*,#54476,.T.);
#79392=ORIENTED_EDGE('',*,*,#54481,.F.);
#79393=ORIENTED_EDGE('',*,*,#54468,.F.);
#79394=ORIENTED_EDGE('',*,*,#54482,.F.);
#79395=ORIENTED_EDGE('',*,*,#54479,.T.);
#79396=ORIENTED_EDGE('',*,*,#54483,.F.);
#79397=ORIENTED_EDGE('',*,*,#54484,.T.);
#79398=ORIENTED_EDGE('',*,*,#54477,.T.);
#79399=ORIENTED_EDGE('',*,*,#54480,.T.);
#79400=ORIENTED_EDGE('',*,*,#54482,.T.);
#79401=ORIENTED_EDGE('',*,*,#54467,.T.);
#79402=ORIENTED_EDGE('',*,*,#54471,.T.);
#79403=ORIENTED_EDGE('',*,*,#54474,.T.);
#79404=ORIENTED_EDGE('',*,*,#54484,.F.);
#79405=ORIENTED_EDGE('',*,*,#54485,.F.);
#79406=ORIENTED_EDGE('',*,*,#54469,.T.);
#79407=ORIENTED_EDGE('',*,*,#54486,.F.);
#79408=ORIENTED_EDGE('',*,*,#54472,.T.);
#79409=ORIENTED_EDGE('',*,*,#54487,.F.);
#79410=ORIENTED_EDGE('',*,*,#54475,.T.);
#79411=ORIENTED_EDGE('',*,*,#54488,.F.);
#79412=ORIENTED_EDGE('',*,*,#54478,.T.);
#79413=ORIENTED_EDGE('',*,*,#54489,.F.);
#79414=ORIENTED_EDGE('',*,*,#54481,.T.);
#79415=ORIENTED_EDGE('',*,*,#54490,.F.);
#79416=ORIENTED_EDGE('',*,*,#54483,.T.);
#79417=ORIENTED_EDGE('',*,*,#54491,.T.);
#79418=ORIENTED_EDGE('',*,*,#54492,.T.);
#79419=ORIENTED_EDGE('',*,*,#54493,.T.);
#79420=ORIENTED_EDGE('',*,*,#54494,.T.);
#79421=ORIENTED_EDGE('',*,*,#54492,.F.);
#79422=ORIENTED_EDGE('',*,*,#54495,.T.);
#79423=ORIENTED_EDGE('',*,*,#54491,.F.);
#79424=ORIENTED_EDGE('',*,*,#54490,.T.);
#79425=ORIENTED_EDGE('',*,*,#54489,.T.);
#79426=ORIENTED_EDGE('',*,*,#54488,.T.);
#79427=ORIENTED_EDGE('',*,*,#54487,.T.);
#79428=ORIENTED_EDGE('',*,*,#54486,.T.);
#79429=ORIENTED_EDGE('',*,*,#54485,.T.);
#79430=ORIENTED_EDGE('',*,*,#54495,.F.);
#79431=ORIENTED_EDGE('',*,*,#54496,.T.);
#79432=ORIENTED_EDGE('',*,*,#54493,.F.);
#79433=ORIENTED_EDGE('',*,*,#54494,.F.);
#79434=ORIENTED_EDGE('',*,*,#54496,.F.);
#79435=ORIENTED_EDGE('',*,*,#54497,.T.);
#79436=ORIENTED_EDGE('',*,*,#54498,.T.);
#79437=ORIENTED_EDGE('',*,*,#54499,.T.);
#79438=ORIENTED_EDGE('',*,*,#54500,.T.);
#79439=ORIENTED_EDGE('',*,*,#54501,.T.);
#79440=ORIENTED_EDGE('',*,*,#54502,.F.);
#79441=ORIENTED_EDGE('',*,*,#54502,.T.);
#79442=ORIENTED_EDGE('',*,*,#54503,.T.);
#79443=ORIENTED_EDGE('',*,*,#54504,.F.);
#79444=ORIENTED_EDGE('',*,*,#54505,.F.);
#79445=ORIENTED_EDGE('',*,*,#54504,.T.);
#79446=ORIENTED_EDGE('',*,*,#54506,.T.);
#79447=ORIENTED_EDGE('',*,*,#54507,.F.);
#79448=ORIENTED_EDGE('',*,*,#54508,.T.);
#79449=ORIENTED_EDGE('',*,*,#54507,.T.);
#79450=ORIENTED_EDGE('',*,*,#54509,.T.);
#79451=ORIENTED_EDGE('',*,*,#54510,.T.);
#79452=ORIENTED_EDGE('',*,*,#54511,.F.);
#79453=ORIENTED_EDGE('',*,*,#54512,.T.);
#79454=ORIENTED_EDGE('',*,*,#54513,.F.);
#79455=ORIENTED_EDGE('',*,*,#54514,.T.);
#79456=ORIENTED_EDGE('',*,*,#54515,.F.);
#79457=ORIENTED_EDGE('',*,*,#54516,.T.);
#79458=ORIENTED_EDGE('',*,*,#54511,.T.);
#79459=ORIENTED_EDGE('',*,*,#54517,.T.);
#79460=ORIENTED_EDGE('',*,*,#54518,.T.);
#79461=ORIENTED_EDGE('',*,*,#54515,.T.);
#79462=ORIENTED_EDGE('',*,*,#54519,.F.);
#79463=ORIENTED_EDGE('',*,*,#54520,.T.);
#79464=ORIENTED_EDGE('',*,*,#54521,.T.);
#79465=ORIENTED_EDGE('',*,*,#54522,.F.);
#79466=ORIENTED_EDGE('',*,*,#54523,.T.);
#79467=ORIENTED_EDGE('',*,*,#54519,.T.);
#79468=ORIENTED_EDGE('',*,*,#54524,.F.);
#79469=ORIENTED_EDGE('',*,*,#54525,.T.);
#79470=ORIENTED_EDGE('',*,*,#54522,.T.);
#79471=ORIENTED_EDGE('',*,*,#54526,.T.);
#79472=ORIENTED_EDGE('',*,*,#54527,.T.);
#79473=ORIENTED_EDGE('',*,*,#54528,.T.);
#79474=ORIENTED_EDGE('',*,*,#54529,.T.);
#79475=ORIENTED_EDGE('',*,*,#54510,.F.);
#79476=ORIENTED_EDGE('',*,*,#54530,.T.);
#79477=ORIENTED_EDGE('',*,*,#54531,.T.);
#79478=ORIENTED_EDGE('',*,*,#54532,.T.);
#79479=ORIENTED_EDGE('',*,*,#54533,.F.);
#79480=ORIENTED_EDGE('',*,*,#54534,.T.);
#79481=ORIENTED_EDGE('',*,*,#54535,.T.);
#79482=ORIENTED_EDGE('',*,*,#54536,.T.);
#79483=ORIENTED_EDGE('',*,*,#54537,.F.);
#79484=ORIENTED_EDGE('',*,*,#54538,.T.);
#79485=ORIENTED_EDGE('',*,*,#54539,.F.);
#79486=ORIENTED_EDGE('',*,*,#54540,.T.);
#79487=ORIENTED_EDGE('',*,*,#54541,.F.);
#79488=ORIENTED_EDGE('',*,*,#54500,.F.);
#79489=ORIENTED_EDGE('',*,*,#54542,.F.);
#79490=ORIENTED_EDGE('',*,*,#54538,.F.);
#79491=ORIENTED_EDGE('',*,*,#54543,.F.);
#79492=ORIENTED_EDGE('',*,*,#54536,.F.);
#79493=ORIENTED_EDGE('',*,*,#54544,.T.);
#79494=ORIENTED_EDGE('',*,*,#54499,.F.);
#79495=ORIENTED_EDGE('',*,*,#54545,.F.);
#79496=ORIENTED_EDGE('',*,*,#54517,.F.);
#79497=ORIENTED_EDGE('',*,*,#54514,.F.);
#79498=ORIENTED_EDGE('',*,*,#54546,.F.);
#79499=ORIENTED_EDGE('',*,*,#54547,.T.);
#79500=ORIENTED_EDGE('',*,*,#54548,.T.);
#79501=ORIENTED_EDGE('',*,*,#54549,.F.);
#79502=ORIENTED_EDGE('',*,*,#54550,.F.);
#79503=ORIENTED_EDGE('',*,*,#54526,.F.);
#79504=ORIENTED_EDGE('',*,*,#54521,.F.);
#79505=ORIENTED_EDGE('',*,*,#54551,.F.);
#79506=ORIENTED_EDGE('',*,*,#54552,.T.);
#79507=ORIENTED_EDGE('',*,*,#54553,.F.);
#79508=ORIENTED_EDGE('',*,*,#54554,.T.);
#79509=ORIENTED_EDGE('',*,*,#54555,.T.);
#79510=ORIENTED_EDGE('',*,*,#54556,.F.);
#79511=ORIENTED_EDGE('',*,*,#54557,.T.);
#79512=ORIENTED_EDGE('',*,*,#54558,.T.);
#79513=ORIENTED_EDGE('',*,*,#54554,.F.);
#79514=ORIENTED_EDGE('',*,*,#54559,.T.);
#79515=ORIENTED_EDGE('',*,*,#54560,.T.);
#79516=ORIENTED_EDGE('',*,*,#54561,.T.);
#79517=ORIENTED_EDGE('',*,*,#54557,.F.);
#79518=ORIENTED_EDGE('',*,*,#54562,.F.);
#79519=ORIENTED_EDGE('',*,*,#54563,.F.);
#79520=ORIENTED_EDGE('',*,*,#54564,.T.);
#79521=ORIENTED_EDGE('',*,*,#54560,.F.);
#79522=ORIENTED_EDGE('',*,*,#54565,.T.);
#79523=ORIENTED_EDGE('',*,*,#54566,.T.);
#79524=ORIENTED_EDGE('',*,*,#54567,.T.);
#79525=ORIENTED_EDGE('',*,*,#54568,.F.);
#79526=ORIENTED_EDGE('',*,*,#54567,.F.);
#79527=ORIENTED_EDGE('',*,*,#54569,.T.);
#79528=ORIENTED_EDGE('',*,*,#54570,.T.);
#79529=ORIENTED_EDGE('',*,*,#54570,.F.);
#79530=ORIENTED_EDGE('',*,*,#54571,.T.);
#79531=ORIENTED_EDGE('',*,*,#54572,.F.);
#79532=ORIENTED_EDGE('',*,*,#54573,.F.);
#79533=ORIENTED_EDGE('',*,*,#54574,.T.);
#79534=ORIENTED_EDGE('',*,*,#54575,.T.);
#79535=ORIENTED_EDGE('',*,*,#54575,.F.);
#79536=ORIENTED_EDGE('',*,*,#54576,.T.);
#79537=ORIENTED_EDGE('',*,*,#54577,.T.);
#79538=ORIENTED_EDGE('',*,*,#54577,.F.);
#79539=ORIENTED_EDGE('',*,*,#54578,.T.);
#79540=ORIENTED_EDGE('',*,*,#54579,.T.);
#79541=ORIENTED_EDGE('',*,*,#54580,.F.);
#79542=ORIENTED_EDGE('',*,*,#54581,.F.);
#79543=ORIENTED_EDGE('',*,*,#54582,.T.);
#79544=ORIENTED_EDGE('',*,*,#54583,.F.);
#79545=ORIENTED_EDGE('',*,*,#54584,.F.);
#79546=ORIENTED_EDGE('',*,*,#54585,.T.);
#79547=ORIENTED_EDGE('',*,*,#54563,.T.);
#79548=ORIENTED_EDGE('',*,*,#54586,.F.);
#79549=ORIENTED_EDGE('',*,*,#54587,.F.);
#79550=ORIENTED_EDGE('',*,*,#54588,.F.);
#79551=ORIENTED_EDGE('',*,*,#54589,.F.);
#79552=ORIENTED_EDGE('',*,*,#54590,.F.);
#79553=ORIENTED_EDGE('',*,*,#54591,.F.);
#79554=ORIENTED_EDGE('',*,*,#54592,.F.);
#79555=ORIENTED_EDGE('',*,*,#54593,.T.);
#79556=ORIENTED_EDGE('',*,*,#54594,.F.);
#79557=ORIENTED_EDGE('',*,*,#54595,.F.);
#79558=ORIENTED_EDGE('',*,*,#54551,.T.);
#79559=ORIENTED_EDGE('',*,*,#54596,.F.);
#79560=ORIENTED_EDGE('',*,*,#54588,.T.);
#79561=ORIENTED_EDGE('',*,*,#54597,.F.);
#79562=ORIENTED_EDGE('',*,*,#54594,.T.);
#79563=ORIENTED_EDGE('',*,*,#54598,.T.);
#79564=ORIENTED_EDGE('',*,*,#54556,.T.);
#79565=ORIENTED_EDGE('',*,*,#54534,.F.);
#79566=ORIENTED_EDGE('',*,*,#54599,.T.);
#79567=ORIENTED_EDGE('',*,*,#54590,.T.);
#79568=ORIENTED_EDGE('',*,*,#54600,.T.);
#79569=ORIENTED_EDGE('',*,*,#54592,.T.);
#79570=ORIENTED_EDGE('',*,*,#54601,.T.);
#79571=ORIENTED_EDGE('',*,*,#54540,.F.);
#79572=ORIENTED_EDGE('',*,*,#54602,.T.);
#79573=ORIENTED_EDGE('',*,*,#54603,.F.);
#79574=ORIENTED_EDGE('',*,*,#54573,.T.);
#79575=ORIENTED_EDGE('',*,*,#54580,.T.);
#79576=ORIENTED_EDGE('',*,*,#54604,.T.);
#79577=ORIENTED_EDGE('',*,*,#54605,.T.);
#79578=ORIENTED_EDGE('',*,*,#54606,.F.);
#79579=ORIENTED_EDGE('',*,*,#54607,.F.);
#79580=ORIENTED_EDGE('',*,*,#54608,.T.);
#79581=ORIENTED_EDGE('',*,*,#54568,.T.);
#79582=ORIENTED_EDGE('',*,*,#54572,.T.);
#79583=ORIENTED_EDGE('',*,*,#54609,.F.);
#79584=ORIENTED_EDGE('',*,*,#54542,.T.);
#79585=ORIENTED_EDGE('',*,*,#54505,.T.);
#79586=ORIENTED_EDGE('',*,*,#54610,.T.);
#79587=ORIENTED_EDGE('',*,*,#54611,.F.);
#79588=ORIENTED_EDGE('',*,*,#54539,.T.);
#79589=ORIENTED_EDGE('',*,*,#54609,.T.);
#79590=ORIENTED_EDGE('',*,*,#54612,.T.);
#79591=ORIENTED_EDGE('',*,*,#54613,.F.);
#79592=ORIENTED_EDGE('',*,*,#54546,.T.);
#79593=ORIENTED_EDGE('',*,*,#54513,.T.);
#79594=ORIENTED_EDGE('',*,*,#54614,.T.);
#79595=ORIENTED_EDGE('',*,*,#54615,.F.);
#79596=ORIENTED_EDGE('',*,*,#54616,.T.);
#79597=ORIENTED_EDGE('',*,*,#54613,.T.);
#79598=ORIENTED_EDGE('',*,*,#54617,.T.);
#79599=ORIENTED_EDGE('',*,*,#54527,.F.);
#79600=ORIENTED_EDGE('',*,*,#54618,.T.);
#79601=ORIENTED_EDGE('',*,*,#54615,.T.);
#79602=ORIENTED_EDGE('',*,*,#54619,.T.);
#79603=ORIENTED_EDGE('',*,*,#54620,.F.);
#79604=ORIENTED_EDGE('',*,*,#54621,.T.);
#79605=ORIENTED_EDGE('',*,*,#54524,.T.);
#79606=ORIENTED_EDGE('',*,*,#54550,.T.);
#79607=ORIENTED_EDGE('',*,*,#54622,.F.);
#79608=ORIENTED_EDGE('',*,*,#54623,.T.);
#79609=ORIENTED_EDGE('',*,*,#54620,.T.);
#79610=ORIENTED_EDGE('',*,*,#54624,.T.);
#79611=ORIENTED_EDGE('',*,*,#54531,.F.);
#79612=ORIENTED_EDGE('',*,*,#54625,.T.);
#79613=ORIENTED_EDGE('',*,*,#54622,.T.);
#79614=ORIENTED_EDGE('',*,*,#54626,.T.);
#79615=ORIENTED_EDGE('',*,*,#54627,.T.);
#79616=ORIENTED_EDGE('',*,*,#54628,.F.);
#79617=ORIENTED_EDGE('',*,*,#54624,.F.);
#79618=ORIENTED_EDGE('',*,*,#54549,.T.);
#79619=ORIENTED_EDGE('',*,*,#54629,.T.);
#79620=ORIENTED_EDGE('',*,*,#54547,.F.);
#79621=ORIENTED_EDGE('',*,*,#54616,.F.);
#79622=ORIENTED_EDGE('',*,*,#54630,.T.);
#79623=ORIENTED_EDGE('',*,*,#54631,.T.);
#79624=ORIENTED_EDGE('',*,*,#54632,.T.);
#79625=ORIENTED_EDGE('',*,*,#54606,.T.);
#79626=ORIENTED_EDGE('',*,*,#54633,.T.);
#79627=ORIENTED_EDGE('',*,*,#54634,.T.);
#79628=ORIENTED_EDGE('',*,*,#54627,.F.);
#79629=ORIENTED_EDGE('',*,*,#54548,.F.);
#79630=ORIENTED_EDGE('',*,*,#54629,.F.);
#79631=ORIENTED_EDGE('',*,*,#54635,.T.);
#79632=ORIENTED_EDGE('',*,*,#54636,.F.);
#79633=ORIENTED_EDGE('',*,*,#54559,.F.);
#79634=ORIENTED_EDGE('',*,*,#54598,.F.);
#79635=ORIENTED_EDGE('',*,*,#54637,.T.);
#79636=ORIENTED_EDGE('',*,*,#54638,.F.);
#79637=ORIENTED_EDGE('',*,*,#54635,.F.);
#79638=ORIENTED_EDGE('',*,*,#54593,.F.);
#79639=ORIENTED_EDGE('',*,*,#54602,.F.);
#79640=ORIENTED_EDGE('',*,*,#54611,.T.);
#79641=ORIENTED_EDGE('',*,*,#54639,.F.);
#79642=ORIENTED_EDGE('',*,*,#54637,.F.);
#79643=ORIENTED_EDGE('',*,*,#54640,.T.);
#79644=ORIENTED_EDGE('',*,*,#54641,.F.);
#79645=ORIENTED_EDGE('',*,*,#54565,.F.);
#79646=ORIENTED_EDGE('',*,*,#54608,.F.);
#79647=ORIENTED_EDGE('',*,*,#54642,.T.);
#79648=ORIENTED_EDGE('',*,*,#54643,.F.);
#79649=ORIENTED_EDGE('',*,*,#54640,.F.);
#79650=ORIENTED_EDGE('',*,*,#54644,.F.);
#79651=ORIENTED_EDGE('',*,*,#54583,.T.);
#79652=ORIENTED_EDGE('',*,*,#54645,.F.);
#79653=ORIENTED_EDGE('',*,*,#54642,.F.);
#79654=ORIENTED_EDGE('',*,*,#54646,.F.);
#79655=ORIENTED_EDGE('',*,*,#54647,.T.);
#79656=ORIENTED_EDGE('',*,*,#54604,.F.);
#79657=ORIENTED_EDGE('',*,*,#54579,.F.);
#79658=ORIENTED_EDGE('',*,*,#54648,.F.);
#79659=ORIENTED_EDGE('',*,*,#54649,.T.);
#79660=ORIENTED_EDGE('',*,*,#54650,.F.);
#79661=ORIENTED_EDGE('',*,*,#54647,.F.);
#79662=ORIENTED_EDGE('',*,*,#54651,.F.);
#79663=ORIENTED_EDGE('',*,*,#54584,.T.);
#79664=ORIENTED_EDGE('',*,*,#54652,.F.);
#79665=ORIENTED_EDGE('',*,*,#54649,.F.);
#79666=ORIENTED_EDGE('',*,*,#54653,.F.);
#79667=ORIENTED_EDGE('',*,*,#54625,.F.);
#79668=ORIENTED_EDGE('',*,*,#54530,.F.);
#79669=ORIENTED_EDGE('',*,*,#54509,.F.);
#79670=ORIENTED_EDGE('',*,*,#54506,.F.);
#79671=ORIENTED_EDGE('',*,*,#54503,.F.);
#79672=ORIENTED_EDGE('',*,*,#54501,.F.);
#79673=ORIENTED_EDGE('',*,*,#54541,.T.);
#79674=ORIENTED_EDGE('',*,*,#54537,.T.);
#79675=ORIENTED_EDGE('',*,*,#54601,.F.);
#79676=ORIENTED_EDGE('',*,*,#54591,.T.);
#79677=ORIENTED_EDGE('',*,*,#54597,.T.);
#79678=ORIENTED_EDGE('',*,*,#54555,.F.);
#79679=ORIENTED_EDGE('',*,*,#54558,.F.);
#79680=ORIENTED_EDGE('',*,*,#54561,.F.);
#79681=ORIENTED_EDGE('',*,*,#54564,.F.);
#79682=ORIENTED_EDGE('',*,*,#54585,.F.);
#79683=ORIENTED_EDGE('',*,*,#54653,.T.);
#79684=ORIENTED_EDGE('',*,*,#54651,.T.);
#79685=ORIENTED_EDGE('',*,*,#54648,.T.);
#79686=ORIENTED_EDGE('',*,*,#54578,.F.);
#79687=ORIENTED_EDGE('',*,*,#54576,.F.);
#79688=ORIENTED_EDGE('',*,*,#54574,.F.);
#79689=ORIENTED_EDGE('',*,*,#54603,.T.);
#79690=ORIENTED_EDGE('',*,*,#54571,.F.);
#79691=ORIENTED_EDGE('',*,*,#54569,.F.);
#79692=ORIENTED_EDGE('',*,*,#54566,.F.);
#79693=ORIENTED_EDGE('',*,*,#54641,.T.);
#79694=ORIENTED_EDGE('',*,*,#54643,.T.);
#79695=ORIENTED_EDGE('',*,*,#54645,.T.);
#79696=ORIENTED_EDGE('',*,*,#54582,.F.);
#79697=ORIENTED_EDGE('',*,*,#54654,.F.);
#79698=ORIENTED_EDGE('',*,*,#54552,.F.);
#79699=ORIENTED_EDGE('',*,*,#54595,.T.);
#79700=ORIENTED_EDGE('',*,*,#54587,.T.);
#79701=ORIENTED_EDGE('',*,*,#54599,.F.);
#79702=ORIENTED_EDGE('',*,*,#54533,.T.);
#79703=ORIENTED_EDGE('',*,*,#54543,.T.);
#79704=ORIENTED_EDGE('',*,*,#54498,.F.);
#79705=ORIENTED_EDGE('',*,*,#54655,.T.);
#79706=ORIENTED_EDGE('',*,*,#54528,.F.);
#79707=ORIENTED_EDGE('',*,*,#54619,.F.);
#79708=ORIENTED_EDGE('',*,*,#54617,.F.);
#79709=ORIENTED_EDGE('',*,*,#54614,.F.);
#79710=ORIENTED_EDGE('',*,*,#54512,.F.);
#79711=ORIENTED_EDGE('',*,*,#54516,.F.);
#79712=ORIENTED_EDGE('',*,*,#54518,.F.);
#79713=ORIENTED_EDGE('',*,*,#54545,.T.);
#79714=ORIENTED_EDGE('',*,*,#54520,.F.);
#79715=ORIENTED_EDGE('',*,*,#54523,.F.);
#79716=ORIENTED_EDGE('',*,*,#54525,.F.);
#79717=ORIENTED_EDGE('',*,*,#54621,.F.);
#79718=ORIENTED_EDGE('',*,*,#54623,.F.);
#79719=ORIENTED_EDGE('',*,*,#54631,.F.);
#79720=ORIENTED_EDGE('',*,*,#54630,.F.);
#79721=ORIENTED_EDGE('',*,*,#54618,.F.);
#79722=ORIENTED_EDGE('',*,*,#54529,.F.);
#79723=ORIENTED_EDGE('',*,*,#54655,.F.);
#79724=ORIENTED_EDGE('',*,*,#54497,.F.);
#79725=ORIENTED_EDGE('',*,*,#54544,.F.);
#79726=ORIENTED_EDGE('',*,*,#54535,.F.);
#79727=ORIENTED_EDGE('',*,*,#54600,.F.);
#79728=ORIENTED_EDGE('',*,*,#54589,.T.);
#79729=ORIENTED_EDGE('',*,*,#54596,.T.);
#79730=ORIENTED_EDGE('',*,*,#54553,.T.);
#79731=ORIENTED_EDGE('',*,*,#54654,.T.);
#79732=ORIENTED_EDGE('',*,*,#54581,.T.);
#79733=ORIENTED_EDGE('',*,*,#54646,.T.);
#79734=ORIENTED_EDGE('',*,*,#54656,.T.);
#79735=ORIENTED_EDGE('',*,*,#54634,.F.);
#79736=ORIENTED_EDGE('',*,*,#54657,.F.);
#79737=ORIENTED_EDGE('',*,*,#54652,.T.);
#79738=ORIENTED_EDGE('',*,*,#54586,.T.);
#79739=ORIENTED_EDGE('',*,*,#54562,.T.);
#79740=ORIENTED_EDGE('',*,*,#54636,.T.);
#79741=ORIENTED_EDGE('',*,*,#54638,.T.);
#79742=ORIENTED_EDGE('',*,*,#54639,.T.);
#79743=ORIENTED_EDGE('',*,*,#54612,.F.);
#79744=ORIENTED_EDGE('',*,*,#54610,.F.);
#79745=ORIENTED_EDGE('',*,*,#54508,.F.);
#79746=ORIENTED_EDGE('',*,*,#54532,.F.);
#79747=ORIENTED_EDGE('',*,*,#54626,.F.);
#79748=ORIENTED_EDGE('',*,*,#54628,.T.);
#79749=ORIENTED_EDGE('',*,*,#54633,.F.);
#79750=ORIENTED_EDGE('',*,*,#54605,.F.);
#79751=ORIENTED_EDGE('',*,*,#54650,.T.);
#79752=ORIENTED_EDGE('',*,*,#54657,.T.);
#79753=ORIENTED_EDGE('',*,*,#54632,.F.);
#79754=ORIENTED_EDGE('',*,*,#54656,.F.);
#79755=ORIENTED_EDGE('',*,*,#54644,.T.);
#79756=ORIENTED_EDGE('',*,*,#54607,.T.);
#79757=ORIENTED_EDGE('',*,*,#54658,.T.);
#79758=ORIENTED_EDGE('',*,*,#54659,.T.);
#79759=ORIENTED_EDGE('',*,*,#54660,.F.);
#79760=ORIENTED_EDGE('',*,*,#54661,.T.);
#79761=ORIENTED_EDGE('',*,*,#54662,.T.);
#79762=ORIENTED_EDGE('',*,*,#54663,.T.);
#79763=ORIENTED_EDGE('',*,*,#54658,.F.);
#79764=ORIENTED_EDGE('',*,*,#54664,.T.);
#79765=ORIENTED_EDGE('',*,*,#54665,.T.);
#79766=ORIENTED_EDGE('',*,*,#54666,.T.);
#79767=ORIENTED_EDGE('',*,*,#54662,.F.);
#79768=ORIENTED_EDGE('',*,*,#54667,.T.);
#79769=ORIENTED_EDGE('',*,*,#54668,.T.);
#79770=ORIENTED_EDGE('',*,*,#54669,.T.);
#79771=ORIENTED_EDGE('',*,*,#54665,.F.);
#79772=ORIENTED_EDGE('',*,*,#54670,.T.);
#79773=ORIENTED_EDGE('',*,*,#54671,.T.);
#79774=ORIENTED_EDGE('',*,*,#54672,.T.);
#79775=ORIENTED_EDGE('',*,*,#54668,.F.);
#79776=ORIENTED_EDGE('',*,*,#54673,.T.);
#79777=ORIENTED_EDGE('',*,*,#54674,.T.);
#79778=ORIENTED_EDGE('',*,*,#54675,.T.);
#79779=ORIENTED_EDGE('',*,*,#54671,.F.);
#79780=ORIENTED_EDGE('',*,*,#54676,.T.);
#79781=ORIENTED_EDGE('',*,*,#54677,.T.);
#79782=ORIENTED_EDGE('',*,*,#54678,.T.);
#79783=ORIENTED_EDGE('',*,*,#54674,.F.);
#79784=ORIENTED_EDGE('',*,*,#54679,.T.);
#79785=ORIENTED_EDGE('',*,*,#54680,.T.);
#79786=ORIENTED_EDGE('',*,*,#54681,.T.);
#79787=ORIENTED_EDGE('',*,*,#54677,.F.);
#79788=ORIENTED_EDGE('',*,*,#54682,.T.);
#79789=ORIENTED_EDGE('',*,*,#54683,.T.);
#79790=ORIENTED_EDGE('',*,*,#54684,.T.);
#79791=ORIENTED_EDGE('',*,*,#54680,.F.);
#79792=ORIENTED_EDGE('',*,*,#54685,.T.);
#79793=ORIENTED_EDGE('',*,*,#54686,.T.);
#79794=ORIENTED_EDGE('',*,*,#54687,.T.);
#79795=ORIENTED_EDGE('',*,*,#54683,.F.);
#79796=ORIENTED_EDGE('',*,*,#54688,.T.);
#79797=ORIENTED_EDGE('',*,*,#54689,.T.);
#79798=ORIENTED_EDGE('',*,*,#54690,.T.);
#79799=ORIENTED_EDGE('',*,*,#54686,.F.);
#79800=ORIENTED_EDGE('',*,*,#54691,.T.);
#79801=ORIENTED_EDGE('',*,*,#54692,.T.);
#79802=ORIENTED_EDGE('',*,*,#54693,.T.);
#79803=ORIENTED_EDGE('',*,*,#54689,.F.);
#79804=ORIENTED_EDGE('',*,*,#54694,.T.);
#79805=ORIENTED_EDGE('',*,*,#54695,.T.);
#79806=ORIENTED_EDGE('',*,*,#54696,.T.);
#79807=ORIENTED_EDGE('',*,*,#54692,.F.);
#79808=ORIENTED_EDGE('',*,*,#54697,.T.);
#79809=ORIENTED_EDGE('',*,*,#54698,.T.);
#79810=ORIENTED_EDGE('',*,*,#54699,.T.);
#79811=ORIENTED_EDGE('',*,*,#54695,.F.);
#79812=ORIENTED_EDGE('',*,*,#54700,.T.);
#79813=ORIENTED_EDGE('',*,*,#54701,.T.);
#79814=ORIENTED_EDGE('',*,*,#54702,.T.);
#79815=ORIENTED_EDGE('',*,*,#54698,.F.);
#79816=ORIENTED_EDGE('',*,*,#54703,.T.);
#79817=ORIENTED_EDGE('',*,*,#54704,.T.);
#79818=ORIENTED_EDGE('',*,*,#54705,.T.);
#79819=ORIENTED_EDGE('',*,*,#54701,.F.);
#79820=ORIENTED_EDGE('',*,*,#54706,.T.);
#79821=ORIENTED_EDGE('',*,*,#54707,.T.);
#79822=ORIENTED_EDGE('',*,*,#54708,.T.);
#79823=ORIENTED_EDGE('',*,*,#54704,.F.);
#79824=ORIENTED_EDGE('',*,*,#54709,.T.);
#79825=ORIENTED_EDGE('',*,*,#54710,.T.);
#79826=ORIENTED_EDGE('',*,*,#54711,.T.);
#79827=ORIENTED_EDGE('',*,*,#54707,.F.);
#79828=ORIENTED_EDGE('',*,*,#54712,.T.);
#79829=ORIENTED_EDGE('',*,*,#54713,.F.);
#79830=ORIENTED_EDGE('',*,*,#54714,.T.);
#79831=ORIENTED_EDGE('',*,*,#54715,.T.);
#79832=ORIENTED_EDGE('',*,*,#54716,.T.);
#79833=ORIENTED_EDGE('',*,*,#54717,.T.);
#79834=ORIENTED_EDGE('',*,*,#54718,.T.);
#79835=ORIENTED_EDGE('',*,*,#54719,.T.);
#79836=ORIENTED_EDGE('',*,*,#54720,.T.);
#79837=ORIENTED_EDGE('',*,*,#54721,.T.);
#79838=ORIENTED_EDGE('',*,*,#54722,.T.);
#79839=ORIENTED_EDGE('',*,*,#54717,.F.);
#79840=ORIENTED_EDGE('',*,*,#54723,.T.);
#79841=ORIENTED_EDGE('',*,*,#54724,.T.);
#79842=ORIENTED_EDGE('',*,*,#54725,.T.);
#79843=ORIENTED_EDGE('',*,*,#54721,.F.);
#79844=ORIENTED_EDGE('',*,*,#54726,.T.);
#79845=ORIENTED_EDGE('',*,*,#54727,.T.);
#79846=ORIENTED_EDGE('',*,*,#54728,.T.);
#79847=ORIENTED_EDGE('',*,*,#54724,.F.);
#79848=ORIENTED_EDGE('',*,*,#54729,.T.);
#79849=ORIENTED_EDGE('',*,*,#54730,.T.);
#79850=ORIENTED_EDGE('',*,*,#54731,.T.);
#79851=ORIENTED_EDGE('',*,*,#54727,.F.);
#79852=ORIENTED_EDGE('',*,*,#54732,.T.);
#79853=ORIENTED_EDGE('',*,*,#54733,.T.);
#79854=ORIENTED_EDGE('',*,*,#54734,.T.);
#79855=ORIENTED_EDGE('',*,*,#54730,.F.);
#79856=ORIENTED_EDGE('',*,*,#54735,.T.);
#79857=ORIENTED_EDGE('',*,*,#54736,.T.);
#79858=ORIENTED_EDGE('',*,*,#54737,.T.);
#79859=ORIENTED_EDGE('',*,*,#54733,.F.);
#79860=ORIENTED_EDGE('',*,*,#54738,.T.);
#79861=ORIENTED_EDGE('',*,*,#54739,.T.);
#79862=ORIENTED_EDGE('',*,*,#54740,.T.);
#79863=ORIENTED_EDGE('',*,*,#54736,.F.);
#79864=ORIENTED_EDGE('',*,*,#54741,.T.);
#79865=ORIENTED_EDGE('',*,*,#54742,.T.);
#79866=ORIENTED_EDGE('',*,*,#54743,.T.);
#79867=ORIENTED_EDGE('',*,*,#54739,.F.);
#79868=ORIENTED_EDGE('',*,*,#54744,.T.);
#79869=ORIENTED_EDGE('',*,*,#54745,.T.);
#79870=ORIENTED_EDGE('',*,*,#54746,.T.);
#79871=ORIENTED_EDGE('',*,*,#54742,.F.);
#79872=ORIENTED_EDGE('',*,*,#54747,.T.);
#79873=ORIENTED_EDGE('',*,*,#54748,.T.);
#79874=ORIENTED_EDGE('',*,*,#54749,.T.);
#79875=ORIENTED_EDGE('',*,*,#54745,.F.);
#79876=ORIENTED_EDGE('',*,*,#54750,.T.);
#79877=ORIENTED_EDGE('',*,*,#54751,.T.);
#79878=ORIENTED_EDGE('',*,*,#54752,.T.);
#79879=ORIENTED_EDGE('',*,*,#54748,.F.);
#79880=ORIENTED_EDGE('',*,*,#54753,.T.);
#79881=ORIENTED_EDGE('',*,*,#54754,.T.);
#79882=ORIENTED_EDGE('',*,*,#54755,.T.);
#79883=ORIENTED_EDGE('',*,*,#54751,.F.);
#79884=ORIENTED_EDGE('',*,*,#54756,.T.);
#79885=ORIENTED_EDGE('',*,*,#54757,.T.);
#79886=ORIENTED_EDGE('',*,*,#54758,.T.);
#79887=ORIENTED_EDGE('',*,*,#54754,.F.);
#79888=ORIENTED_EDGE('',*,*,#54759,.T.);
#79889=ORIENTED_EDGE('',*,*,#54760,.T.);
#79890=ORIENTED_EDGE('',*,*,#54761,.T.);
#79891=ORIENTED_EDGE('',*,*,#54757,.F.);
#79892=ORIENTED_EDGE('',*,*,#54762,.T.);
#79893=ORIENTED_EDGE('',*,*,#54763,.T.);
#79894=ORIENTED_EDGE('',*,*,#54764,.T.);
#79895=ORIENTED_EDGE('',*,*,#54760,.F.);
#79896=ORIENTED_EDGE('',*,*,#54765,.T.);
#79897=ORIENTED_EDGE('',*,*,#54766,.T.);
#79898=ORIENTED_EDGE('',*,*,#54767,.T.);
#79899=ORIENTED_EDGE('',*,*,#54763,.F.);
#79900=ORIENTED_EDGE('',*,*,#54768,.T.);
#79901=ORIENTED_EDGE('',*,*,#54769,.T.);
#79902=ORIENTED_EDGE('',*,*,#54770,.T.);
#79903=ORIENTED_EDGE('',*,*,#54766,.F.);
#79904=ORIENTED_EDGE('',*,*,#54771,.T.);
#79905=ORIENTED_EDGE('',*,*,#54772,.F.);
#79906=ORIENTED_EDGE('',*,*,#54773,.T.);
#79907=ORIENTED_EDGE('',*,*,#54774,.F.);
#79908=ORIENTED_EDGE('',*,*,#54775,.T.);
#79909=ORIENTED_EDGE('',*,*,#54776,.T.);
#79910=ORIENTED_EDGE('',*,*,#54777,.T.);
#79911=ORIENTED_EDGE('',*,*,#54778,.F.);
#79912=ORIENTED_EDGE('',*,*,#54779,.F.);
#79913=ORIENTED_EDGE('',*,*,#54780,.T.);
#79914=ORIENTED_EDGE('',*,*,#54781,.T.);
#79915=ORIENTED_EDGE('',*,*,#54782,.F.);
#79916=ORIENTED_EDGE('',*,*,#54783,.T.);
#79917=ORIENTED_EDGE('',*,*,#54776,.F.);
#79918=ORIENTED_EDGE('',*,*,#54784,.F.);
#79919=ORIENTED_EDGE('',*,*,#54785,.T.);
#79920=ORIENTED_EDGE('',*,*,#54786,.T.);
#79921=ORIENTED_EDGE('',*,*,#54780,.F.);
#79922=ORIENTED_EDGE('',*,*,#54787,.F.);
#79923=ORIENTED_EDGE('',*,*,#54788,.T.);
#79924=ORIENTED_EDGE('',*,*,#54789,.T.);
#79925=ORIENTED_EDGE('',*,*,#54785,.F.);
#79926=ORIENTED_EDGE('',*,*,#54790,.F.);
#79927=ORIENTED_EDGE('',*,*,#54791,.T.);
#79928=ORIENTED_EDGE('',*,*,#54792,.T.);
#79929=ORIENTED_EDGE('',*,*,#54788,.F.);
#79930=ORIENTED_EDGE('',*,*,#54793,.F.);
#79931=ORIENTED_EDGE('',*,*,#54794,.T.);
#79932=ORIENTED_EDGE('',*,*,#54795,.T.);
#79933=ORIENTED_EDGE('',*,*,#54791,.F.);
#79934=ORIENTED_EDGE('',*,*,#54796,.F.);
#79935=ORIENTED_EDGE('',*,*,#54797,.T.);
#79936=ORIENTED_EDGE('',*,*,#54798,.T.);
#79937=ORIENTED_EDGE('',*,*,#54794,.F.);
#79938=ORIENTED_EDGE('',*,*,#54799,.F.);
#79939=ORIENTED_EDGE('',*,*,#54800,.T.);
#79940=ORIENTED_EDGE('',*,*,#54801,.T.);
#79941=ORIENTED_EDGE('',*,*,#54797,.F.);
#79942=ORIENTED_EDGE('',*,*,#54802,.F.);
#79943=ORIENTED_EDGE('',*,*,#54803,.T.);
#79944=ORIENTED_EDGE('',*,*,#54804,.T.);
#79945=ORIENTED_EDGE('',*,*,#54800,.F.);
#79946=ORIENTED_EDGE('',*,*,#54805,.F.);
#79947=ORIENTED_EDGE('',*,*,#54806,.T.);
#79948=ORIENTED_EDGE('',*,*,#54807,.T.);
#79949=ORIENTED_EDGE('',*,*,#54803,.F.);
#79950=ORIENTED_EDGE('',*,*,#54808,.F.);
#79951=ORIENTED_EDGE('',*,*,#54809,.T.);
#79952=ORIENTED_EDGE('',*,*,#54810,.T.);
#79953=ORIENTED_EDGE('',*,*,#54806,.F.);
#79954=ORIENTED_EDGE('',*,*,#54811,.F.);
#79955=ORIENTED_EDGE('',*,*,#54812,.T.);
#79956=ORIENTED_EDGE('',*,*,#54813,.T.);
#79957=ORIENTED_EDGE('',*,*,#54809,.F.);
#79958=ORIENTED_EDGE('',*,*,#54814,.F.);
#79959=ORIENTED_EDGE('',*,*,#54815,.T.);
#79960=ORIENTED_EDGE('',*,*,#54816,.T.);
#79961=ORIENTED_EDGE('',*,*,#54812,.F.);
#79962=ORIENTED_EDGE('',*,*,#54817,.F.);
#79963=ORIENTED_EDGE('',*,*,#54818,.T.);
#79964=ORIENTED_EDGE('',*,*,#54819,.T.);
#79965=ORIENTED_EDGE('',*,*,#54815,.F.);
#79966=ORIENTED_EDGE('',*,*,#54820,.F.);
#79967=ORIENTED_EDGE('',*,*,#54821,.T.);
#79968=ORIENTED_EDGE('',*,*,#54822,.T.);
#79969=ORIENTED_EDGE('',*,*,#54818,.F.);
#79970=ORIENTED_EDGE('',*,*,#54823,.F.);
#79971=ORIENTED_EDGE('',*,*,#54824,.T.);
#79972=ORIENTED_EDGE('',*,*,#54825,.T.);
#79973=ORIENTED_EDGE('',*,*,#54821,.F.);
#79974=ORIENTED_EDGE('',*,*,#54826,.F.);
#79975=ORIENTED_EDGE('',*,*,#54827,.T.);
#79976=ORIENTED_EDGE('',*,*,#54828,.T.);
#79977=ORIENTED_EDGE('',*,*,#54824,.F.);
#79978=ORIENTED_EDGE('',*,*,#54829,.F.);
#79979=ORIENTED_EDGE('',*,*,#54830,.T.);
#79980=ORIENTED_EDGE('',*,*,#54831,.T.);
#79981=ORIENTED_EDGE('',*,*,#54827,.F.);
#79982=ORIENTED_EDGE('',*,*,#54832,.F.);
#79983=ORIENTED_EDGE('',*,*,#54833,.F.);
#79984=ORIENTED_EDGE('',*,*,#54834,.F.);
#79985=ORIENTED_EDGE('',*,*,#54835,.T.);
#79986=ORIENTED_EDGE('',*,*,#54836,.T.);
#79987=ORIENTED_EDGE('',*,*,#54837,.T.);
#79988=ORIENTED_EDGE('',*,*,#54838,.F.);
#79989=ORIENTED_EDGE('',*,*,#54839,.T.);
#79990=ORIENTED_EDGE('',*,*,#54840,.T.);
#79991=ORIENTED_EDGE('',*,*,#54841,.T.);
#79992=ORIENTED_EDGE('',*,*,#54836,.F.);
#79993=ORIENTED_EDGE('',*,*,#54842,.T.);
#79994=ORIENTED_EDGE('',*,*,#54843,.T.);
#79995=ORIENTED_EDGE('',*,*,#54844,.T.);
#79996=ORIENTED_EDGE('',*,*,#54840,.F.);
#79997=ORIENTED_EDGE('',*,*,#54845,.T.);
#79998=ORIENTED_EDGE('',*,*,#54846,.T.);
#79999=ORIENTED_EDGE('',*,*,#54847,.T.);
#80000=ORIENTED_EDGE('',*,*,#54843,.F.);
#80001=ORIENTED_EDGE('',*,*,#54848,.T.);
#80002=ORIENTED_EDGE('',*,*,#54849,.T.);
#80003=ORIENTED_EDGE('',*,*,#54850,.T.);
#80004=ORIENTED_EDGE('',*,*,#54846,.F.);
#80005=ORIENTED_EDGE('',*,*,#54851,.T.);
#80006=ORIENTED_EDGE('',*,*,#54852,.T.);
#80007=ORIENTED_EDGE('',*,*,#54853,.T.);
#80008=ORIENTED_EDGE('',*,*,#54849,.F.);
#80009=ORIENTED_EDGE('',*,*,#54854,.T.);
#80010=ORIENTED_EDGE('',*,*,#54855,.T.);
#80011=ORIENTED_EDGE('',*,*,#54856,.T.);
#80012=ORIENTED_EDGE('',*,*,#54852,.F.);
#80013=ORIENTED_EDGE('',*,*,#54857,.T.);
#80014=ORIENTED_EDGE('',*,*,#54858,.T.);
#80015=ORIENTED_EDGE('',*,*,#54859,.T.);
#80016=ORIENTED_EDGE('',*,*,#54855,.F.);
#80017=ORIENTED_EDGE('',*,*,#54860,.T.);
#80018=ORIENTED_EDGE('',*,*,#54861,.T.);
#80019=ORIENTED_EDGE('',*,*,#54862,.T.);
#80020=ORIENTED_EDGE('',*,*,#54858,.F.);
#80021=ORIENTED_EDGE('',*,*,#54863,.T.);
#80022=ORIENTED_EDGE('',*,*,#54864,.T.);
#80023=ORIENTED_EDGE('',*,*,#54865,.T.);
#80024=ORIENTED_EDGE('',*,*,#54861,.F.);
#80025=ORIENTED_EDGE('',*,*,#54866,.T.);
#80026=ORIENTED_EDGE('',*,*,#54867,.T.);
#80027=ORIENTED_EDGE('',*,*,#54868,.T.);
#80028=ORIENTED_EDGE('',*,*,#54864,.F.);
#80029=ORIENTED_EDGE('',*,*,#54869,.T.);
#80030=ORIENTED_EDGE('',*,*,#54870,.T.);
#80031=ORIENTED_EDGE('',*,*,#54871,.T.);
#80032=ORIENTED_EDGE('',*,*,#54867,.F.);
#80033=ORIENTED_EDGE('',*,*,#54872,.T.);
#80034=ORIENTED_EDGE('',*,*,#54873,.T.);
#80035=ORIENTED_EDGE('',*,*,#54874,.T.);
#80036=ORIENTED_EDGE('',*,*,#54870,.F.);
#80037=ORIENTED_EDGE('',*,*,#54875,.T.);
#80038=ORIENTED_EDGE('',*,*,#54876,.T.);
#80039=ORIENTED_EDGE('',*,*,#54877,.T.);
#80040=ORIENTED_EDGE('',*,*,#54873,.F.);
#80041=ORIENTED_EDGE('',*,*,#54878,.T.);
#80042=ORIENTED_EDGE('',*,*,#54879,.T.);
#80043=ORIENTED_EDGE('',*,*,#54880,.T.);
#80044=ORIENTED_EDGE('',*,*,#54876,.F.);
#80045=ORIENTED_EDGE('',*,*,#54881,.T.);
#80046=ORIENTED_EDGE('',*,*,#54882,.T.);
#80047=ORIENTED_EDGE('',*,*,#54883,.T.);
#80048=ORIENTED_EDGE('',*,*,#54879,.F.);
#80049=ORIENTED_EDGE('',*,*,#54884,.T.);
#80050=ORIENTED_EDGE('',*,*,#54885,.T.);
#80051=ORIENTED_EDGE('',*,*,#54886,.T.);
#80052=ORIENTED_EDGE('',*,*,#54882,.F.);
#80053=ORIENTED_EDGE('',*,*,#54887,.T.);
#80054=ORIENTED_EDGE('',*,*,#54888,.F.);
#80055=ORIENTED_EDGE('',*,*,#54889,.T.);
#80056=ORIENTED_EDGE('',*,*,#54890,.T.);
#80057=ORIENTED_EDGE('',*,*,#54891,.T.);
#80058=ORIENTED_EDGE('',*,*,#54892,.T.);
#80059=ORIENTED_EDGE('',*,*,#54893,.T.);
#80060=ORIENTED_EDGE('',*,*,#54894,.T.);
#80061=ORIENTED_EDGE('',*,*,#54895,.T.);
#80062=ORIENTED_EDGE('',*,*,#54896,.F.);
#80063=ORIENTED_EDGE('',*,*,#54897,.F.);
#80064=ORIENTED_EDGE('',*,*,#54898,.T.);
#80065=ORIENTED_EDGE('',*,*,#54899,.T.);
#80066=ORIENTED_EDGE('',*,*,#54900,.F.);
#80067=ORIENTED_EDGE('',*,*,#54901,.T.);
#80068=ORIENTED_EDGE('',*,*,#54894,.F.);
#80069=ORIENTED_EDGE('',*,*,#54902,.F.);
#80070=ORIENTED_EDGE('',*,*,#54903,.T.);
#80071=ORIENTED_EDGE('',*,*,#54904,.T.);
#80072=ORIENTED_EDGE('',*,*,#54898,.F.);
#80073=ORIENTED_EDGE('',*,*,#54905,.F.);
#80074=ORIENTED_EDGE('',*,*,#54906,.T.);
#80075=ORIENTED_EDGE('',*,*,#54907,.T.);
#80076=ORIENTED_EDGE('',*,*,#54903,.F.);
#80077=ORIENTED_EDGE('',*,*,#54908,.F.);
#80078=ORIENTED_EDGE('',*,*,#54909,.T.);
#80079=ORIENTED_EDGE('',*,*,#54910,.T.);
#80080=ORIENTED_EDGE('',*,*,#54906,.F.);
#80081=ORIENTED_EDGE('',*,*,#54911,.F.);
#80082=ORIENTED_EDGE('',*,*,#54912,.T.);
#80083=ORIENTED_EDGE('',*,*,#54913,.T.);
#80084=ORIENTED_EDGE('',*,*,#54909,.F.);
#80085=ORIENTED_EDGE('',*,*,#54914,.F.);
#80086=ORIENTED_EDGE('',*,*,#54915,.T.);
#80087=ORIENTED_EDGE('',*,*,#54916,.T.);
#80088=ORIENTED_EDGE('',*,*,#54912,.F.);
#80089=ORIENTED_EDGE('',*,*,#54917,.F.);
#80090=ORIENTED_EDGE('',*,*,#54918,.T.);
#80091=ORIENTED_EDGE('',*,*,#54919,.T.);
#80092=ORIENTED_EDGE('',*,*,#54915,.F.);
#80093=ORIENTED_EDGE('',*,*,#54920,.F.);
#80094=ORIENTED_EDGE('',*,*,#54921,.T.);
#80095=ORIENTED_EDGE('',*,*,#54922,.T.);
#80096=ORIENTED_EDGE('',*,*,#54918,.F.);
#80097=ORIENTED_EDGE('',*,*,#54923,.F.);
#80098=ORIENTED_EDGE('',*,*,#54924,.T.);
#80099=ORIENTED_EDGE('',*,*,#54925,.T.);
#80100=ORIENTED_EDGE('',*,*,#54921,.F.);
#80101=ORIENTED_EDGE('',*,*,#54926,.F.);
#80102=ORIENTED_EDGE('',*,*,#54927,.T.);
#80103=ORIENTED_EDGE('',*,*,#54928,.T.);
#80104=ORIENTED_EDGE('',*,*,#54924,.F.);
#80105=ORIENTED_EDGE('',*,*,#54929,.F.);
#80106=ORIENTED_EDGE('',*,*,#54930,.T.);
#80107=ORIENTED_EDGE('',*,*,#54931,.T.);
#80108=ORIENTED_EDGE('',*,*,#54927,.F.);
#80109=ORIENTED_EDGE('',*,*,#54932,.F.);
#80110=ORIENTED_EDGE('',*,*,#54933,.T.);
#80111=ORIENTED_EDGE('',*,*,#54934,.T.);
#80112=ORIENTED_EDGE('',*,*,#54930,.F.);
#80113=ORIENTED_EDGE('',*,*,#54935,.F.);
#80114=ORIENTED_EDGE('',*,*,#54936,.T.);
#80115=ORIENTED_EDGE('',*,*,#54937,.T.);
#80116=ORIENTED_EDGE('',*,*,#54933,.F.);
#80117=ORIENTED_EDGE('',*,*,#54938,.F.);
#80118=ORIENTED_EDGE('',*,*,#54939,.T.);
#80119=ORIENTED_EDGE('',*,*,#54940,.T.);
#80120=ORIENTED_EDGE('',*,*,#54936,.F.);
#80121=ORIENTED_EDGE('',*,*,#54941,.F.);
#80122=ORIENTED_EDGE('',*,*,#54942,.T.);
#80123=ORIENTED_EDGE('',*,*,#54943,.T.);
#80124=ORIENTED_EDGE('',*,*,#54939,.F.);
#80125=ORIENTED_EDGE('',*,*,#54944,.F.);
#80126=ORIENTED_EDGE('',*,*,#54945,.T.);
#80127=ORIENTED_EDGE('',*,*,#54946,.T.);
#80128=ORIENTED_EDGE('',*,*,#54942,.F.);
#80129=ORIENTED_EDGE('',*,*,#54947,.F.);
#80130=ORIENTED_EDGE('',*,*,#54948,.T.);
#80131=ORIENTED_EDGE('',*,*,#54949,.T.);
#80132=ORIENTED_EDGE('',*,*,#54945,.F.);
#80133=ORIENTED_EDGE('',*,*,#54950,.F.);
#80134=ORIENTED_EDGE('',*,*,#54951,.F.);
#80135=ORIENTED_EDGE('',*,*,#54952,.F.);
#80136=ORIENTED_EDGE('',*,*,#54953,.T.);
#80137=ORIENTED_EDGE('',*,*,#54954,.T.);
#80138=ORIENTED_EDGE('',*,*,#54955,.T.);
#80139=ORIENTED_EDGE('',*,*,#54956,.T.);
#80140=ORIENTED_EDGE('',*,*,#54957,.T.);
#80141=ORIENTED_EDGE('',*,*,#54958,.T.);
#80142=ORIENTED_EDGE('',*,*,#54954,.F.);
#80143=ORIENTED_EDGE('',*,*,#54959,.T.);
#80144=ORIENTED_EDGE('',*,*,#54960,.T.);
#80145=ORIENTED_EDGE('',*,*,#54961,.T.);
#80146=ORIENTED_EDGE('',*,*,#54957,.F.);
#80147=ORIENTED_EDGE('',*,*,#54962,.T.);
#80148=ORIENTED_EDGE('',*,*,#54963,.T.);
#80149=ORIENTED_EDGE('',*,*,#54964,.T.);
#80150=ORIENTED_EDGE('',*,*,#54960,.F.);
#80151=ORIENTED_EDGE('',*,*,#54965,.T.);
#80152=ORIENTED_EDGE('',*,*,#54966,.T.);
#80153=ORIENTED_EDGE('',*,*,#54967,.T.);
#80154=ORIENTED_EDGE('',*,*,#54963,.F.);
#80155=ORIENTED_EDGE('',*,*,#54968,.T.);
#80156=ORIENTED_EDGE('',*,*,#54969,.T.);
#80157=ORIENTED_EDGE('',*,*,#54970,.T.);
#80158=ORIENTED_EDGE('',*,*,#54966,.F.);
#80159=ORIENTED_EDGE('',*,*,#54971,.T.);
#80160=ORIENTED_EDGE('',*,*,#54972,.T.);
#80161=ORIENTED_EDGE('',*,*,#54973,.T.);
#80162=ORIENTED_EDGE('',*,*,#54969,.F.);
#80163=ORIENTED_EDGE('',*,*,#54974,.T.);
#80164=ORIENTED_EDGE('',*,*,#54975,.T.);
#80165=ORIENTED_EDGE('',*,*,#54976,.T.);
#80166=ORIENTED_EDGE('',*,*,#54972,.F.);
#80167=ORIENTED_EDGE('',*,*,#54977,.T.);
#80168=ORIENTED_EDGE('',*,*,#54978,.T.);
#80169=ORIENTED_EDGE('',*,*,#54979,.T.);
#80170=ORIENTED_EDGE('',*,*,#54975,.F.);
#80171=ORIENTED_EDGE('',*,*,#54980,.T.);
#80172=ORIENTED_EDGE('',*,*,#54981,.T.);
#80173=ORIENTED_EDGE('',*,*,#54982,.T.);
#80174=ORIENTED_EDGE('',*,*,#54978,.F.);
#80175=ORIENTED_EDGE('',*,*,#54983,.T.);
#80176=ORIENTED_EDGE('',*,*,#54984,.T.);
#80177=ORIENTED_EDGE('',*,*,#54985,.T.);
#80178=ORIENTED_EDGE('',*,*,#54981,.F.);
#80179=ORIENTED_EDGE('',*,*,#54986,.T.);
#80180=ORIENTED_EDGE('',*,*,#54987,.T.);
#80181=ORIENTED_EDGE('',*,*,#54988,.T.);
#80182=ORIENTED_EDGE('',*,*,#54984,.F.);
#80183=ORIENTED_EDGE('',*,*,#54989,.T.);
#80184=ORIENTED_EDGE('',*,*,#54990,.T.);
#80185=ORIENTED_EDGE('',*,*,#54991,.T.);
#80186=ORIENTED_EDGE('',*,*,#54987,.F.);
#80187=ORIENTED_EDGE('',*,*,#54992,.T.);
#80188=ORIENTED_EDGE('',*,*,#54993,.T.);
#80189=ORIENTED_EDGE('',*,*,#54994,.T.);
#80190=ORIENTED_EDGE('',*,*,#54990,.F.);
#80191=ORIENTED_EDGE('',*,*,#54995,.T.);
#80192=ORIENTED_EDGE('',*,*,#54996,.T.);
#80193=ORIENTED_EDGE('',*,*,#54997,.T.);
#80194=ORIENTED_EDGE('',*,*,#54993,.F.);
#80195=ORIENTED_EDGE('',*,*,#54998,.T.);
#80196=ORIENTED_EDGE('',*,*,#54999,.T.);
#80197=ORIENTED_EDGE('',*,*,#55000,.T.);
#80198=ORIENTED_EDGE('',*,*,#54996,.F.);
#80199=ORIENTED_EDGE('',*,*,#55001,.T.);
#80200=ORIENTED_EDGE('',*,*,#55002,.T.);
#80201=ORIENTED_EDGE('',*,*,#55003,.T.);
#80202=ORIENTED_EDGE('',*,*,#54999,.F.);
#80203=ORIENTED_EDGE('',*,*,#55004,.T.);
#80204=ORIENTED_EDGE('',*,*,#55005,.T.);
#80205=ORIENTED_EDGE('',*,*,#55006,.T.);
#80206=ORIENTED_EDGE('',*,*,#55002,.F.);
#80207=ORIENTED_EDGE('',*,*,#55007,.T.);
#80208=ORIENTED_EDGE('',*,*,#55008,.F.);
#80209=ORIENTED_EDGE('',*,*,#55009,.T.);
#80210=ORIENTED_EDGE('',*,*,#55010,.F.);
#80211=ORIENTED_EDGE('',*,*,#55011,.T.);
#80212=ORIENTED_EDGE('',*,*,#55012,.T.);
#80213=ORIENTED_EDGE('',*,*,#55013,.T.);
#80214=ORIENTED_EDGE('',*,*,#55014,.F.);
#80215=ORIENTED_EDGE('',*,*,#55015,.F.);
#80216=ORIENTED_EDGE('',*,*,#55016,.T.);
#80217=ORIENTED_EDGE('',*,*,#55017,.T.);
#80218=ORIENTED_EDGE('',*,*,#55018,.F.);
#80219=ORIENTED_EDGE('',*,*,#55019,.T.);
#80220=ORIENTED_EDGE('',*,*,#55012,.F.);
#80221=ORIENTED_EDGE('',*,*,#55020,.F.);
#80222=ORIENTED_EDGE('',*,*,#55021,.T.);
#80223=ORIENTED_EDGE('',*,*,#55022,.T.);
#80224=ORIENTED_EDGE('',*,*,#55016,.F.);
#80225=ORIENTED_EDGE('',*,*,#55023,.F.);
#80226=ORIENTED_EDGE('',*,*,#55024,.T.);
#80227=ORIENTED_EDGE('',*,*,#55025,.T.);
#80228=ORIENTED_EDGE('',*,*,#55021,.F.);
#80229=ORIENTED_EDGE('',*,*,#55026,.F.);
#80230=ORIENTED_EDGE('',*,*,#55027,.T.);
#80231=ORIENTED_EDGE('',*,*,#55028,.T.);
#80232=ORIENTED_EDGE('',*,*,#55024,.F.);
#80233=ORIENTED_EDGE('',*,*,#55029,.F.);
#80234=ORIENTED_EDGE('',*,*,#55030,.T.);
#80235=ORIENTED_EDGE('',*,*,#55031,.T.);
#80236=ORIENTED_EDGE('',*,*,#55027,.F.);
#80237=ORIENTED_EDGE('',*,*,#55032,.F.);
#80238=ORIENTED_EDGE('',*,*,#55033,.T.);
#80239=ORIENTED_EDGE('',*,*,#55034,.T.);
#80240=ORIENTED_EDGE('',*,*,#55030,.F.);
#80241=ORIENTED_EDGE('',*,*,#55035,.F.);
#80242=ORIENTED_EDGE('',*,*,#55036,.T.);
#80243=ORIENTED_EDGE('',*,*,#55037,.T.);
#80244=ORIENTED_EDGE('',*,*,#55033,.F.);
#80245=ORIENTED_EDGE('',*,*,#55038,.F.);
#80246=ORIENTED_EDGE('',*,*,#55039,.T.);
#80247=ORIENTED_EDGE('',*,*,#55040,.T.);
#80248=ORIENTED_EDGE('',*,*,#55036,.F.);
#80249=ORIENTED_EDGE('',*,*,#55041,.F.);
#80250=ORIENTED_EDGE('',*,*,#55042,.T.);
#80251=ORIENTED_EDGE('',*,*,#55043,.T.);
#80252=ORIENTED_EDGE('',*,*,#55039,.F.);
#80253=ORIENTED_EDGE('',*,*,#55044,.F.);
#80254=ORIENTED_EDGE('',*,*,#55045,.T.);
#80255=ORIENTED_EDGE('',*,*,#55046,.T.);
#80256=ORIENTED_EDGE('',*,*,#55042,.F.);
#80257=ORIENTED_EDGE('',*,*,#55047,.F.);
#80258=ORIENTED_EDGE('',*,*,#55048,.T.);
#80259=ORIENTED_EDGE('',*,*,#55049,.T.);
#80260=ORIENTED_EDGE('',*,*,#55045,.F.);
#80261=ORIENTED_EDGE('',*,*,#55050,.F.);
#80262=ORIENTED_EDGE('',*,*,#55051,.T.);
#80263=ORIENTED_EDGE('',*,*,#55052,.T.);
#80264=ORIENTED_EDGE('',*,*,#55048,.F.);
#80265=ORIENTED_EDGE('',*,*,#55053,.F.);
#80266=ORIENTED_EDGE('',*,*,#55054,.T.);
#80267=ORIENTED_EDGE('',*,*,#55055,.T.);
#80268=ORIENTED_EDGE('',*,*,#55051,.F.);
#80269=ORIENTED_EDGE('',*,*,#55056,.F.);
#80270=ORIENTED_EDGE('',*,*,#55057,.T.);
#80271=ORIENTED_EDGE('',*,*,#55058,.T.);
#80272=ORIENTED_EDGE('',*,*,#55054,.F.);
#80273=ORIENTED_EDGE('',*,*,#55059,.F.);
#80274=ORIENTED_EDGE('',*,*,#55060,.T.);
#80275=ORIENTED_EDGE('',*,*,#55061,.T.);
#80276=ORIENTED_EDGE('',*,*,#55057,.F.);
#80277=ORIENTED_EDGE('',*,*,#55062,.F.);
#80278=ORIENTED_EDGE('',*,*,#55063,.T.);
#80279=ORIENTED_EDGE('',*,*,#55064,.T.);
#80280=ORIENTED_EDGE('',*,*,#55060,.F.);
#80281=ORIENTED_EDGE('',*,*,#55065,.F.);
#80282=ORIENTED_EDGE('',*,*,#55066,.T.);
#80283=ORIENTED_EDGE('',*,*,#55067,.T.);
#80284=ORIENTED_EDGE('',*,*,#55063,.F.);
#80285=ORIENTED_EDGE('',*,*,#55068,.F.);
#80286=ORIENTED_EDGE('',*,*,#55069,.F.);
#80287=ORIENTED_EDGE('',*,*,#55070,.F.);
#80288=ORIENTED_EDGE('',*,*,#55071,.T.);
#80289=ORIENTED_EDGE('',*,*,#55072,.T.);
#80290=ORIENTED_EDGE('',*,*,#55073,.T.);
#80291=ORIENTED_EDGE('',*,*,#55074,.F.);
#80292=ORIENTED_EDGE('',*,*,#55075,.F.);
#80293=ORIENTED_EDGE('',*,*,#55076,.T.);
#80294=ORIENTED_EDGE('',*,*,#55077,.T.);
#80295=ORIENTED_EDGE('',*,*,#55078,.F.);
#80296=ORIENTED_EDGE('',*,*,#55079,.T.);
#80297=ORIENTED_EDGE('',*,*,#55072,.F.);
#80298=ORIENTED_EDGE('',*,*,#55080,.F.);
#80299=ORIENTED_EDGE('',*,*,#55081,.T.);
#80300=ORIENTED_EDGE('',*,*,#55082,.T.);
#80301=ORIENTED_EDGE('',*,*,#55076,.F.);
#80302=ORIENTED_EDGE('',*,*,#55083,.F.);
#80303=ORIENTED_EDGE('',*,*,#55084,.T.);
#80304=ORIENTED_EDGE('',*,*,#55085,.T.);
#80305=ORIENTED_EDGE('',*,*,#55081,.F.);
#80306=ORIENTED_EDGE('',*,*,#55086,.F.);
#80307=ORIENTED_EDGE('',*,*,#55087,.T.);
#80308=ORIENTED_EDGE('',*,*,#55088,.T.);
#80309=ORIENTED_EDGE('',*,*,#55084,.F.);
#80310=ORIENTED_EDGE('',*,*,#55089,.F.);
#80311=ORIENTED_EDGE('',*,*,#55090,.T.);
#80312=ORIENTED_EDGE('',*,*,#55091,.T.);
#80313=ORIENTED_EDGE('',*,*,#55087,.F.);
#80314=ORIENTED_EDGE('',*,*,#55092,.F.);
#80315=ORIENTED_EDGE('',*,*,#55093,.T.);
#80316=ORIENTED_EDGE('',*,*,#55094,.T.);
#80317=ORIENTED_EDGE('',*,*,#55090,.F.);
#80318=ORIENTED_EDGE('',*,*,#55095,.F.);
#80319=ORIENTED_EDGE('',*,*,#55096,.T.);
#80320=ORIENTED_EDGE('',*,*,#55097,.T.);
#80321=ORIENTED_EDGE('',*,*,#55093,.F.);
#80322=ORIENTED_EDGE('',*,*,#55098,.F.);
#80323=ORIENTED_EDGE('',*,*,#55099,.T.);
#80324=ORIENTED_EDGE('',*,*,#55100,.T.);
#80325=ORIENTED_EDGE('',*,*,#55096,.F.);
#80326=ORIENTED_EDGE('',*,*,#55101,.F.);
#80327=ORIENTED_EDGE('',*,*,#55102,.T.);
#80328=ORIENTED_EDGE('',*,*,#55103,.T.);
#80329=ORIENTED_EDGE('',*,*,#55099,.F.);
#80330=ORIENTED_EDGE('',*,*,#55104,.F.);
#80331=ORIENTED_EDGE('',*,*,#55105,.T.);
#80332=ORIENTED_EDGE('',*,*,#55106,.T.);
#80333=ORIENTED_EDGE('',*,*,#55102,.F.);
#80334=ORIENTED_EDGE('',*,*,#55107,.F.);
#80335=ORIENTED_EDGE('',*,*,#55108,.T.);
#80336=ORIENTED_EDGE('',*,*,#55109,.T.);
#80337=ORIENTED_EDGE('',*,*,#55105,.F.);
#80338=ORIENTED_EDGE('',*,*,#55110,.F.);
#80339=ORIENTED_EDGE('',*,*,#55111,.T.);
#80340=ORIENTED_EDGE('',*,*,#55112,.T.);
#80341=ORIENTED_EDGE('',*,*,#55108,.F.);
#80342=ORIENTED_EDGE('',*,*,#55113,.F.);
#80343=ORIENTED_EDGE('',*,*,#55114,.T.);
#80344=ORIENTED_EDGE('',*,*,#55115,.T.);
#80345=ORIENTED_EDGE('',*,*,#55111,.F.);
#80346=ORIENTED_EDGE('',*,*,#55116,.F.);
#80347=ORIENTED_EDGE('',*,*,#55117,.T.);
#80348=ORIENTED_EDGE('',*,*,#55118,.T.);
#80349=ORIENTED_EDGE('',*,*,#55114,.F.);
#80350=ORIENTED_EDGE('',*,*,#55119,.F.);
#80351=ORIENTED_EDGE('',*,*,#55120,.T.);
#80352=ORIENTED_EDGE('',*,*,#55121,.T.);
#80353=ORIENTED_EDGE('',*,*,#55117,.F.);
#80354=ORIENTED_EDGE('',*,*,#55122,.F.);
#80355=ORIENTED_EDGE('',*,*,#55123,.T.);
#80356=ORIENTED_EDGE('',*,*,#55124,.T.);
#80357=ORIENTED_EDGE('',*,*,#55120,.F.);
#80358=ORIENTED_EDGE('',*,*,#55125,.F.);
#80359=ORIENTED_EDGE('',*,*,#55126,.T.);
#80360=ORIENTED_EDGE('',*,*,#55127,.T.);
#80361=ORIENTED_EDGE('',*,*,#55123,.F.);
#80362=ORIENTED_EDGE('',*,*,#55128,.F.);
#80363=ORIENTED_EDGE('',*,*,#55129,.F.);
#80364=ORIENTED_EDGE('',*,*,#55130,.F.);
#80365=ORIENTED_EDGE('',*,*,#55131,.T.);
#80366=ORIENTED_EDGE('',*,*,#55132,.T.);
#80367=ORIENTED_EDGE('',*,*,#55133,.T.);
#80368=ORIENTED_EDGE('',*,*,#55134,.F.);
#80369=ORIENTED_EDGE('',*,*,#55135,.F.);
#80370=ORIENTED_EDGE('',*,*,#55136,.F.);
#80371=ORIENTED_EDGE('',*,*,#55137,.F.);
#80372=ORIENTED_EDGE('',*,*,#55138,.F.);
#80373=ORIENTED_EDGE('',*,*,#55139,.T.);
#80374=ORIENTED_EDGE('',*,*,#55140,.T.);
#80375=ORIENTED_EDGE('',*,*,#55141,.T.);
#80376=ORIENTED_EDGE('',*,*,#55142,.T.);
#80377=ORIENTED_EDGE('',*,*,#55139,.F.);
#80378=ORIENTED_EDGE('',*,*,#55143,.F.);
#80379=ORIENTED_EDGE('',*,*,#55144,.T.);
#80380=ORIENTED_EDGE('',*,*,#55145,.T.);
#80381=ORIENTED_EDGE('',*,*,#55146,.T.);
#80382=ORIENTED_EDGE('',*,*,#55140,.F.);
#80383=ORIENTED_EDGE('',*,*,#55147,.T.);
#80384=ORIENTED_EDGE('',*,*,#55148,.T.);
#80385=ORIENTED_EDGE('',*,*,#55149,.T.);
#80386=ORIENTED_EDGE('',*,*,#55150,.T.);
#80387=ORIENTED_EDGE('',*,*,#55151,.T.);
#80388=ORIENTED_EDGE('',*,*,#55152,.T.);
#80389=ORIENTED_EDGE('',*,*,#55153,.T.);
#80390=ORIENTED_EDGE('',*,*,#55154,.T.);
#80391=ORIENTED_EDGE('',*,*,#55155,.F.);
#80392=ORIENTED_EDGE('',*,*,#55156,.F.);
#80393=ORIENTED_EDGE('',*,*,#55157,.T.);
#80394=ORIENTED_EDGE('',*,*,#55135,.T.);
#80395=ORIENTED_EDGE('',*,*,#55158,.F.);
#80396=ORIENTED_EDGE('',*,*,#55137,.T.);
#80397=ORIENTED_EDGE('',*,*,#55159,.F.);
#80398=ORIENTED_EDGE('',*,*,#55160,.F.);
#80399=ORIENTED_EDGE('',*,*,#55156,.T.);
#80400=ORIENTED_EDGE('',*,*,#55161,.F.);
#80401=ORIENTED_EDGE('',*,*,#55160,.T.);
#80402=ORIENTED_EDGE('',*,*,#55162,.T.);
#80403=ORIENTED_EDGE('',*,*,#55142,.F.);
#80404=ORIENTED_EDGE('',*,*,#55163,.T.);
#80405=ORIENTED_EDGE('',*,*,#55164,.F.);
#80406=ORIENTED_EDGE('',*,*,#55165,.T.);
#80407=ORIENTED_EDGE('',*,*,#55166,.T.);
#80408=ORIENTED_EDGE('',*,*,#55167,.F.);
#80409=ORIENTED_EDGE('',*,*,#55168,.T.);
#80410=ORIENTED_EDGE('',*,*,#55132,.F.);
#80411=ORIENTED_EDGE('',*,*,#55169,.F.);
#80412=ORIENTED_EDGE('',*,*,#55170,.F.);
#80413=ORIENTED_EDGE('',*,*,#55171,.T.);
#80414=ORIENTED_EDGE('',*,*,#55172,.F.);
#80415=ORIENTED_EDGE('',*,*,#55173,.F.);
#80416=ORIENTED_EDGE('',*,*,#55174,.F.);
#80417=ORIENTED_EDGE('',*,*,#55175,.F.);
#80418=ORIENTED_EDGE('',*,*,#55176,.T.);
#80419=ORIENTED_EDGE('',*,*,#55177,.T.);
#80420=ORIENTED_EDGE('',*,*,#55178,.T.);
#80421=ORIENTED_EDGE('',*,*,#55179,.F.);
#80422=ORIENTED_EDGE('',*,*,#55180,.F.);
#80423=ORIENTED_EDGE('',*,*,#55181,.F.);
#80424=ORIENTED_EDGE('',*,*,#55182,.F.);
#80425=ORIENTED_EDGE('',*,*,#55183,.T.);
#80426=ORIENTED_EDGE('',*,*,#55184,.T.);
#80427=ORIENTED_EDGE('',*,*,#55185,.T.);
#80428=ORIENTED_EDGE('',*,*,#55186,.F.);
#80429=ORIENTED_EDGE('',*,*,#55186,.T.);
#80430=ORIENTED_EDGE('',*,*,#55187,.T.);
#80431=ORIENTED_EDGE('',*,*,#55188,.F.);
#80432=ORIENTED_EDGE('',*,*,#55187,.F.);
#80433=ORIENTED_EDGE('',*,*,#55170,.T.);
#80434=ORIENTED_EDGE('',*,*,#55189,.T.);
#80435=ORIENTED_EDGE('',*,*,#55185,.F.);
#80436=ORIENTED_EDGE('',*,*,#55189,.F.);
#80437=ORIENTED_EDGE('',*,*,#55188,.T.);
#80438=ORIENTED_EDGE('',*,*,#55190,.T.);
#80439=ORIENTED_EDGE('',*,*,#55191,.F.);
#80440=ORIENTED_EDGE('',*,*,#55191,.T.);
#80441=ORIENTED_EDGE('',*,*,#55192,.T.);
#80442=ORIENTED_EDGE('',*,*,#55193,.F.);
#80443=ORIENTED_EDGE('',*,*,#55192,.F.);
#80444=ORIENTED_EDGE('',*,*,#55169,.T.);
#80445=ORIENTED_EDGE('',*,*,#55194,.T.);
#80446=ORIENTED_EDGE('',*,*,#55190,.F.);
#80447=ORIENTED_EDGE('',*,*,#55194,.F.);
#80448=ORIENTED_EDGE('',*,*,#55193,.T.);
#80449=ORIENTED_EDGE('',*,*,#55195,.T.);
#80450=ORIENTED_EDGE('',*,*,#55196,.F.);
#80451=ORIENTED_EDGE('',*,*,#55196,.T.);
#80452=ORIENTED_EDGE('',*,*,#55197,.T.);
#80453=ORIENTED_EDGE('',*,*,#55198,.F.);
#80454=ORIENTED_EDGE('',*,*,#55197,.F.);
#80455=ORIENTED_EDGE('',*,*,#55167,.T.);
#80456=ORIENTED_EDGE('',*,*,#55199,.T.);
#80457=ORIENTED_EDGE('',*,*,#55200,.T.);
#80458=ORIENTED_EDGE('',*,*,#55195,.F.);
#80459=ORIENTED_EDGE('',*,*,#55200,.F.);
#80460=ORIENTED_EDGE('',*,*,#55201,.T.);
#80461=ORIENTED_EDGE('',*,*,#55198,.T.);
#80462=ORIENTED_EDGE('',*,*,#55202,.T.);
#80463=ORIENTED_EDGE('',*,*,#55203,.F.);
#80464=ORIENTED_EDGE('',*,*,#55203,.T.);
#80465=ORIENTED_EDGE('',*,*,#55204,.T.);
#80466=ORIENTED_EDGE('',*,*,#55205,.F.);
#80467=ORIENTED_EDGE('',*,*,#55204,.F.);
#80468=ORIENTED_EDGE('',*,*,#55164,.T.);
#80469=ORIENTED_EDGE('',*,*,#55206,.T.);
#80470=ORIENTED_EDGE('',*,*,#55207,.T.);
#80471=ORIENTED_EDGE('',*,*,#55202,.F.);
#80472=ORIENTED_EDGE('',*,*,#55207,.F.);
#80473=ORIENTED_EDGE('',*,*,#55208,.T.);
#80474=ORIENTED_EDGE('',*,*,#55205,.T.);
#80475=ORIENTED_EDGE('',*,*,#55171,.F.);
#80476=ORIENTED_EDGE('',*,*,#55209,.F.);
#80477=ORIENTED_EDGE('',*,*,#55210,.F.);
#80478=ORIENTED_EDGE('',*,*,#55183,.F.);
#80479=ORIENTED_EDGE('',*,*,#55211,.F.);
#80480=ORIENTED_EDGE('',*,*,#55212,.F.);
#80481=ORIENTED_EDGE('',*,*,#55213,.T.);
#80482=ORIENTED_EDGE('',*,*,#55214,.F.);
#80483=ORIENTED_EDGE('',*,*,#55215,.F.);
#80484=ORIENTED_EDGE('',*,*,#55213,.F.);
#80485=ORIENTED_EDGE('',*,*,#55216,.F.);
#80486=ORIENTED_EDGE('',*,*,#55217,.F.);
#80487=ORIENTED_EDGE('',*,*,#55218,.T.);
#80488=ORIENTED_EDGE('',*,*,#55219,.F.);
#80489=ORIENTED_EDGE('',*,*,#55220,.F.);
#80490=ORIENTED_EDGE('',*,*,#55218,.F.);
#80491=ORIENTED_EDGE('',*,*,#55221,.T.);
#80492=ORIENTED_EDGE('',*,*,#55222,.T.);
#80493=ORIENTED_EDGE('',*,*,#55223,.F.);
#80494=ORIENTED_EDGE('',*,*,#55224,.T.);
#80495=ORIENTED_EDGE('',*,*,#55225,.T.);
#80496=ORIENTED_EDGE('',*,*,#55226,.T.);
#80497=ORIENTED_EDGE('',*,*,#55221,.F.);
#80498=ORIENTED_EDGE('',*,*,#55227,.T.);
#80499=ORIENTED_EDGE('',*,*,#55228,.T.);
#80500=ORIENTED_EDGE('',*,*,#55229,.T.);
#80501=ORIENTED_EDGE('',*,*,#55225,.F.);
#80502=ORIENTED_EDGE('',*,*,#55230,.T.);
#80503=ORIENTED_EDGE('',*,*,#55231,.T.);
#80504=ORIENTED_EDGE('',*,*,#55232,.T.);
#80505=ORIENTED_EDGE('',*,*,#55228,.F.);
#80506=ORIENTED_EDGE('',*,*,#55233,.T.);
#80507=ORIENTED_EDGE('',*,*,#55234,.T.);
#80508=ORIENTED_EDGE('',*,*,#55235,.T.);
#80509=ORIENTED_EDGE('',*,*,#55231,.F.);
#80510=ORIENTED_EDGE('',*,*,#55236,.T.);
#80511=ORIENTED_EDGE('',*,*,#55223,.T.);
#80512=ORIENTED_EDGE('',*,*,#55237,.T.);
#80513=ORIENTED_EDGE('',*,*,#55234,.F.);
#80514=ORIENTED_EDGE('',*,*,#55238,.T.);
#80515=ORIENTED_EDGE('',*,*,#55239,.T.);
#80516=ORIENTED_EDGE('',*,*,#55238,.F.);
#80517=ORIENTED_EDGE('',*,*,#55236,.F.);
#80518=ORIENTED_EDGE('',*,*,#55233,.F.);
#80519=ORIENTED_EDGE('',*,*,#55230,.F.);
#80520=ORIENTED_EDGE('',*,*,#55227,.F.);
#80521=ORIENTED_EDGE('',*,*,#55224,.F.);
#80522=ORIENTED_EDGE('',*,*,#55239,.F.);
#80523=ORIENTED_EDGE('',*,*,#55240,.T.);
#80524=ORIENTED_EDGE('',*,*,#55222,.F.);
#80525=ORIENTED_EDGE('',*,*,#55241,.T.);
#80526=ORIENTED_EDGE('',*,*,#55226,.F.);
#80527=ORIENTED_EDGE('',*,*,#55242,.T.);
#80528=ORIENTED_EDGE('',*,*,#55229,.F.);
#80529=ORIENTED_EDGE('',*,*,#55243,.T.);
#80530=ORIENTED_EDGE('',*,*,#55232,.F.);
#80531=ORIENTED_EDGE('',*,*,#55244,.T.);
#80532=ORIENTED_EDGE('',*,*,#55235,.F.);
#80533=ORIENTED_EDGE('',*,*,#55245,.T.);
#80534=ORIENTED_EDGE('',*,*,#55237,.F.);
#80535=ORIENTED_EDGE('',*,*,#55216,.T.);
#80536=ORIENTED_EDGE('',*,*,#55217,.T.);
#80537=ORIENTED_EDGE('',*,*,#55246,.T.);
#80538=ORIENTED_EDGE('',*,*,#55214,.T.);
#80539=ORIENTED_EDGE('',*,*,#55215,.T.);
#80540=ORIENTED_EDGE('',*,*,#55246,.F.);
#80541=ORIENTED_EDGE('',*,*,#55212,.T.);
#80542=ORIENTED_EDGE('',*,*,#55242,.F.);
#80543=ORIENTED_EDGE('',*,*,#55243,.F.);
#80544=ORIENTED_EDGE('',*,*,#55244,.F.);
#80545=ORIENTED_EDGE('',*,*,#55245,.F.);
#80546=ORIENTED_EDGE('',*,*,#55240,.F.);
#80547=ORIENTED_EDGE('',*,*,#55241,.F.);
#80548=ORIENTED_EDGE('',*,*,#55210,.T.);
#80549=ORIENTED_EDGE('',*,*,#55247,.T.);
#80550=ORIENTED_EDGE('',*,*,#55219,.T.);
#80551=ORIENTED_EDGE('',*,*,#55220,.T.);
#80552=ORIENTED_EDGE('',*,*,#55247,.F.);
#80553=ORIENTED_EDGE('',*,*,#55209,.T.);
#80554=ORIENTED_EDGE('',*,*,#55184,.F.);
#80555=ORIENTED_EDGE('',*,*,#55248,.F.);
#80556=ORIENTED_EDGE('',*,*,#55249,.T.);
#80557=ORIENTED_EDGE('',*,*,#55249,.F.);
#80558=ORIENTED_EDGE('',*,*,#55250,.T.);
#80559=ORIENTED_EDGE('',*,*,#55251,.T.);
#80560=ORIENTED_EDGE('',*,*,#55252,.T.);
#80561=ORIENTED_EDGE('',*,*,#55252,.F.);
#80562=ORIENTED_EDGE('',*,*,#55253,.T.);
#80563=ORIENTED_EDGE('',*,*,#55254,.F.);
#80564=ORIENTED_EDGE('',*,*,#55255,.F.);
#80565=ORIENTED_EDGE('',*,*,#55256,.T.);
#80566=ORIENTED_EDGE('',*,*,#55257,.T.);
#80567=ORIENTED_EDGE('',*,*,#55258,.F.);
#80568=ORIENTED_EDGE('',*,*,#55256,.F.);
#80569=ORIENTED_EDGE('',*,*,#55259,.F.);
#80570=ORIENTED_EDGE('',*,*,#55260,.F.);
#80571=ORIENTED_EDGE('',*,*,#55261,.F.);
#80572=ORIENTED_EDGE('',*,*,#55262,.T.);
#80573=ORIENTED_EDGE('',*,*,#55263,.F.);
#80574=ORIENTED_EDGE('',*,*,#55257,.F.);
#80575=ORIENTED_EDGE('',*,*,#55264,.F.);
#80576=ORIENTED_EDGE('',*,*,#55265,.T.);
#80577=ORIENTED_EDGE('',*,*,#55266,.F.);
#80578=ORIENTED_EDGE('',*,*,#55262,.F.);
#80579=ORIENTED_EDGE('',*,*,#55267,.F.);
#80580=ORIENTED_EDGE('',*,*,#55268,.T.);
#80581=ORIENTED_EDGE('',*,*,#55269,.F.);
#80582=ORIENTED_EDGE('',*,*,#55265,.F.);
#80583=ORIENTED_EDGE('',*,*,#55270,.F.);
#80584=ORIENTED_EDGE('',*,*,#55271,.F.);
#80585=ORIENTED_EDGE('',*,*,#55272,.F.);
#80586=ORIENTED_EDGE('',*,*,#55268,.F.);
#80587=ORIENTED_EDGE('',*,*,#55273,.F.);
#80588=ORIENTED_EDGE('',*,*,#55274,.F.);
#80589=ORIENTED_EDGE('',*,*,#55275,.F.);
#80590=ORIENTED_EDGE('',*,*,#55175,.T.);
#80591=ORIENTED_EDGE('',*,*,#55276,.T.);
#80592=ORIENTED_EDGE('',*,*,#55276,.F.);
#80593=ORIENTED_EDGE('',*,*,#55174,.T.);
#80594=ORIENTED_EDGE('',*,*,#55277,.T.);
#80595=ORIENTED_EDGE('',*,*,#55278,.F.);
#80596=ORIENTED_EDGE('',*,*,#55277,.F.);
#80597=ORIENTED_EDGE('',*,*,#55173,.T.);
#80598=ORIENTED_EDGE('',*,*,#55279,.F.);
#80599=ORIENTED_EDGE('',*,*,#55280,.F.);
#80600=ORIENTED_EDGE('',*,*,#55181,.T.);
#80601=ORIENTED_EDGE('',*,*,#55281,.T.);
#80602=ORIENTED_EDGE('',*,*,#55281,.F.);
#80603=ORIENTED_EDGE('',*,*,#55180,.T.);
#80604=ORIENTED_EDGE('',*,*,#55282,.T.);
#80605=ORIENTED_EDGE('',*,*,#55283,.F.);
#80606=ORIENTED_EDGE('',*,*,#55282,.F.);
#80607=ORIENTED_EDGE('',*,*,#55179,.T.);
#80608=ORIENTED_EDGE('',*,*,#55284,.F.);
#80609=ORIENTED_EDGE('',*,*,#55285,.F.);
#80610=ORIENTED_EDGE('',*,*,#55260,.T.);
#80611=ORIENTED_EDGE('',*,*,#55286,.F.);
#80612=ORIENTED_EDGE('',*,*,#55287,.F.);
#80613=ORIENTED_EDGE('',*,*,#55288,.F.);
#80614=ORIENTED_EDGE('',*,*,#55289,.T.);
#80615=ORIENTED_EDGE('',*,*,#55290,.F.);
#80616=ORIENTED_EDGE('',*,*,#55291,.F.);
#80617=ORIENTED_EDGE('',*,*,#55271,.T.);
#80618=ORIENTED_EDGE('',*,*,#55292,.F.);
#80619=ORIENTED_EDGE('',*,*,#55293,.T.);
#80620=ORIENTED_EDGE('',*,*,#55294,.F.);
#80621=ORIENTED_EDGE('',*,*,#55289,.F.);
#80622=ORIENTED_EDGE('',*,*,#55295,.F.);
#80623=ORIENTED_EDGE('',*,*,#55296,.T.);
#80624=ORIENTED_EDGE('',*,*,#55297,.F.);
#80625=ORIENTED_EDGE('',*,*,#55283,.T.);
#80626=ORIENTED_EDGE('',*,*,#55284,.T.);
#80627=ORIENTED_EDGE('',*,*,#55298,.F.);
#80628=ORIENTED_EDGE('',*,*,#55293,.F.);
#80629=ORIENTED_EDGE('',*,*,#55296,.F.);
#80630=ORIENTED_EDGE('',*,*,#55299,.F.);
#80631=ORIENTED_EDGE('',*,*,#55300,.F.);
#80632=ORIENTED_EDGE('',*,*,#55301,.T.);
#80633=ORIENTED_EDGE('',*,*,#55302,.F.);
#80634=ORIENTED_EDGE('',*,*,#55303,.F.);
#80635=ORIENTED_EDGE('',*,*,#55288,.T.);
#80636=ORIENTED_EDGE('',*,*,#55304,.T.);
#80637=ORIENTED_EDGE('',*,*,#55305,.F.);
#80638=ORIENTED_EDGE('',*,*,#55301,.F.);
#80639=ORIENTED_EDGE('',*,*,#55306,.F.);
#80640=ORIENTED_EDGE('',*,*,#55307,.F.);
#80641=ORIENTED_EDGE('',*,*,#55275,.T.);
#80642=ORIENTED_EDGE('',*,*,#55278,.T.);
#80643=ORIENTED_EDGE('',*,*,#55308,.F.);
#80644=ORIENTED_EDGE('',*,*,#55304,.F.);
#80645=ORIENTED_EDGE('',*,*,#55309,.F.);
#80646=ORIENTED_EDGE('',*,*,#55290,.T.);
#80647=ORIENTED_EDGE('',*,*,#55310,.F.);
#80648=ORIENTED_EDGE('',*,*,#55311,.T.);
#80649=ORIENTED_EDGE('',*,*,#55312,.T.);
#80650=ORIENTED_EDGE('',*,*,#55313,.F.);
#80651=ORIENTED_EDGE('',*,*,#55311,.F.);
#80652=ORIENTED_EDGE('',*,*,#55314,.F.);
#80653=ORIENTED_EDGE('',*,*,#55315,.T.);
#80654=ORIENTED_EDGE('',*,*,#55316,.F.);
#80655=ORIENTED_EDGE('',*,*,#55312,.F.);
#80656=ORIENTED_EDGE('',*,*,#55317,.T.);
#80657=ORIENTED_EDGE('',*,*,#55318,.F.);
#80658=ORIENTED_EDGE('',*,*,#55315,.F.);
#80659=ORIENTED_EDGE('',*,*,#55319,.F.);
#80660=ORIENTED_EDGE('',*,*,#55320,.T.);
#80661=ORIENTED_EDGE('',*,*,#55321,.F.);
#80662=ORIENTED_EDGE('',*,*,#55317,.F.);
#80663=ORIENTED_EDGE('',*,*,#55322,.F.);
#80664=ORIENTED_EDGE('',*,*,#55323,.F.);
#80665=ORIENTED_EDGE('',*,*,#55298,.T.);
#80666=ORIENTED_EDGE('',*,*,#55178,.F.);
#80667=ORIENTED_EDGE('',*,*,#55320,.F.);
#80668=ORIENTED_EDGE('',*,*,#55324,.F.);
#80669=ORIENTED_EDGE('',*,*,#55300,.T.);
#80670=ORIENTED_EDGE('',*,*,#55325,.F.);
#80671=ORIENTED_EDGE('',*,*,#55326,.T.);
#80672=ORIENTED_EDGE('',*,*,#55327,.F.);
#80673=ORIENTED_EDGE('',*,*,#55328,.T.);
#80674=ORIENTED_EDGE('',*,*,#55326,.F.);
#80675=ORIENTED_EDGE('',*,*,#55329,.T.);
#80676=ORIENTED_EDGE('',*,*,#55330,.F.);
#80677=ORIENTED_EDGE('',*,*,#55328,.F.);
#80678=ORIENTED_EDGE('',*,*,#55331,.F.);
#80679=ORIENTED_EDGE('',*,*,#55332,.T.);
#80680=ORIENTED_EDGE('',*,*,#55333,.F.);
#80681=ORIENTED_EDGE('',*,*,#55329,.F.);
#80682=ORIENTED_EDGE('',*,*,#55334,.F.);
#80683=ORIENTED_EDGE('',*,*,#55176,.F.);
#80684=ORIENTED_EDGE('',*,*,#55307,.T.);
#80685=ORIENTED_EDGE('',*,*,#55335,.F.);
#80686=ORIENTED_EDGE('',*,*,#55332,.F.);
#80687=ORIENTED_EDGE('',*,*,#55286,.T.);
#80688=ORIENTED_EDGE('',*,*,#55259,.T.);
#80689=ORIENTED_EDGE('',*,*,#55255,.T.);
#80690=ORIENTED_EDGE('',*,*,#55336,.F.);
#80691=ORIENTED_EDGE('',*,*,#55264,.T.);
#80692=ORIENTED_EDGE('',*,*,#55261,.T.);
#80693=ORIENTED_EDGE('',*,*,#55285,.T.);
#80694=ORIENTED_EDGE('',*,*,#55303,.T.);
#80695=ORIENTED_EDGE('',*,*,#55337,.F.);
#80696=ORIENTED_EDGE('',*,*,#55273,.T.);
#80697=ORIENTED_EDGE('',*,*,#55270,.T.);
#80698=ORIENTED_EDGE('',*,*,#55267,.T.);
#80699=ORIENTED_EDGE('',*,*,#55335,.T.);
#80700=ORIENTED_EDGE('',*,*,#55306,.T.);
#80701=ORIENTED_EDGE('',*,*,#55324,.T.);
#80702=ORIENTED_EDGE('',*,*,#55330,.T.);
#80703=ORIENTED_EDGE('',*,*,#55333,.T.);
#80704=ORIENTED_EDGE('',*,*,#55310,.T.);
#80705=ORIENTED_EDGE('',*,*,#55294,.T.);
#80706=ORIENTED_EDGE('',*,*,#55323,.T.);
#80707=ORIENTED_EDGE('',*,*,#55322,.T.);
#80708=ORIENTED_EDGE('',*,*,#55319,.T.);
#80709=ORIENTED_EDGE('',*,*,#55314,.T.);
#80710=ORIENTED_EDGE('',*,*,#55172,.T.);
#80711=ORIENTED_EDGE('',*,*,#55211,.T.);
#80712=ORIENTED_EDGE('',*,*,#55182,.T.);
#80713=ORIENTED_EDGE('',*,*,#55280,.T.);
#80714=ORIENTED_EDGE('',*,*,#55297,.T.);
#80715=ORIENTED_EDGE('',*,*,#55295,.T.);
#80716=ORIENTED_EDGE('',*,*,#55292,.T.);
#80717=ORIENTED_EDGE('',*,*,#55274,.T.);
#80718=ORIENTED_EDGE('',*,*,#55337,.T.);
#80719=ORIENTED_EDGE('',*,*,#55302,.T.);
#80720=ORIENTED_EDGE('',*,*,#55305,.T.);
#80721=ORIENTED_EDGE('',*,*,#55308,.T.);
#80722=ORIENTED_EDGE('',*,*,#55279,.T.);
#80723=ORIENTED_EDGE('',*,*,#55338,.T.);
#80724=ORIENTED_EDGE('',*,*,#55339,.T.);
#80725=ORIENTED_EDGE('',*,*,#55340,.T.);
#80726=ORIENTED_EDGE('',*,*,#55341,.F.);
#80727=ORIENTED_EDGE('',*,*,#55342,.T.);
#80728=ORIENTED_EDGE('',*,*,#55343,.T.);
#80729=ORIENTED_EDGE('',*,*,#55344,.T.);
#80730=ORIENTED_EDGE('',*,*,#55345,.F.);
#80731=ORIENTED_EDGE('',*,*,#55346,.T.);
#80732=ORIENTED_EDGE('',*,*,#55347,.T.);
#80733=ORIENTED_EDGE('',*,*,#55348,.T.);
#80734=ORIENTED_EDGE('',*,*,#55349,.F.);
#80735=ORIENTED_EDGE('',*,*,#55350,.F.);
#80736=ORIENTED_EDGE('',*,*,#55349,.T.);
#80737=ORIENTED_EDGE('',*,*,#55351,.T.);
#80738=ORIENTED_EDGE('',*,*,#55352,.T.);
#80739=ORIENTED_EDGE('',*,*,#55353,.T.);
#80740=ORIENTED_EDGE('',*,*,#55354,.T.);
#80741=ORIENTED_EDGE('',*,*,#55355,.T.);
#80742=ORIENTED_EDGE('',*,*,#55356,.F.);
#80743=ORIENTED_EDGE('',*,*,#55357,.T.);
#80744=ORIENTED_EDGE('',*,*,#55358,.T.);
#80745=ORIENTED_EDGE('',*,*,#55359,.T.);
#80746=ORIENTED_EDGE('',*,*,#55360,.F.);
#80747=ORIENTED_EDGE('',*,*,#55348,.F.);
#80748=ORIENTED_EDGE('',*,*,#55361,.F.);
#80749=ORIENTED_EDGE('',*,*,#55357,.F.);
#80750=ORIENTED_EDGE('',*,*,#55362,.F.);
#80751=ORIENTED_EDGE('',*,*,#55363,.F.);
#80752=ORIENTED_EDGE('',*,*,#55360,.T.);
#80753=ORIENTED_EDGE('',*,*,#55364,.T.);
#80754=ORIENTED_EDGE('',*,*,#55365,.T.);
#80755=ORIENTED_EDGE('',*,*,#55359,.F.);
#80756=ORIENTED_EDGE('',*,*,#55366,.F.);
#80757=ORIENTED_EDGE('',*,*,#55353,.F.);
#80758=ORIENTED_EDGE('',*,*,#55367,.F.);
#80759=ORIENTED_EDGE('',*,*,#55368,.F.);
#80760=ORIENTED_EDGE('',*,*,#55356,.T.);
#80761=ORIENTED_EDGE('',*,*,#55369,.T.);
#80762=ORIENTED_EDGE('',*,*,#55370,.T.);
#80763=ORIENTED_EDGE('',*,*,#55355,.F.);
#80764=ORIENTED_EDGE('',*,*,#55371,.F.);
#80765=ORIENTED_EDGE('',*,*,#55342,.F.);
#80766=ORIENTED_EDGE('',*,*,#55372,.F.);
#80767=ORIENTED_EDGE('',*,*,#55373,.F.);
#80768=ORIENTED_EDGE('',*,*,#55345,.T.);
#80769=ORIENTED_EDGE('',*,*,#55374,.T.);
#80770=ORIENTED_EDGE('',*,*,#55375,.T.);
#80771=ORIENTED_EDGE('',*,*,#55376,.T.);
#80772=ORIENTED_EDGE('',*,*,#55377,.T.);
#80773=ORIENTED_EDGE('',*,*,#55378,.T.);
#80774=ORIENTED_EDGE('',*,*,#55379,.F.);
#80775=ORIENTED_EDGE('',*,*,#55380,.T.);
#80776=ORIENTED_EDGE('',*,*,#55381,.T.);
#80777=ORIENTED_EDGE('',*,*,#55382,.T.);
#80778=ORIENTED_EDGE('',*,*,#55383,.F.);
#80779=ORIENTED_EDGE('',*,*,#55384,.F.);
#80780=ORIENTED_EDGE('',*,*,#55263,.T.);
#80781=ORIENTED_EDGE('',*,*,#55385,.F.);
#80782=ORIENTED_EDGE('',*,*,#55386,.F.);
#80783=ORIENTED_EDGE('',*,*,#55380,.F.);
#80784=ORIENTED_EDGE('',*,*,#55387,.F.);
#80785=ORIENTED_EDGE('',*,*,#55383,.T.);
#80786=ORIENTED_EDGE('',*,*,#55388,.T.);
#80787=ORIENTED_EDGE('',*,*,#55389,.T.);
#80788=ORIENTED_EDGE('',*,*,#55382,.F.);
#80789=ORIENTED_EDGE('',*,*,#55390,.F.);
#80790=ORIENTED_EDGE('',*,*,#55376,.F.);
#80791=ORIENTED_EDGE('',*,*,#55391,.F.);
#80792=ORIENTED_EDGE('',*,*,#55392,.F.);
#80793=ORIENTED_EDGE('',*,*,#55379,.T.);
#80794=ORIENTED_EDGE('',*,*,#55393,.T.);
#80795=ORIENTED_EDGE('',*,*,#55394,.T.);
#80796=ORIENTED_EDGE('',*,*,#55378,.F.);
#80797=ORIENTED_EDGE('',*,*,#55395,.F.);
#80798=ORIENTED_EDGE('',*,*,#55338,.F.);
#80799=ORIENTED_EDGE('',*,*,#55396,.F.);
#80800=ORIENTED_EDGE('',*,*,#55397,.F.);
#80801=ORIENTED_EDGE('',*,*,#55341,.T.);
#80802=ORIENTED_EDGE('',*,*,#55398,.T.);
#80803=ORIENTED_EDGE('',*,*,#55399,.T.);
#80804=ORIENTED_EDGE('',*,*,#55393,.F.);
#80805=ORIENTED_EDGE('',*,*,#55396,.T.);
#80806=ORIENTED_EDGE('',*,*,#55397,.T.);
#80807=ORIENTED_EDGE('',*,*,#55400,.T.);
#80808=ORIENTED_EDGE('',*,*,#55388,.F.);
#80809=ORIENTED_EDGE('',*,*,#55391,.T.);
#80810=ORIENTED_EDGE('',*,*,#55392,.T.);
#80811=ORIENTED_EDGE('',*,*,#55401,.T.);
#80812=ORIENTED_EDGE('',*,*,#55369,.F.);
#80813=ORIENTED_EDGE('',*,*,#55372,.T.);
#80814=ORIENTED_EDGE('',*,*,#55373,.T.);
#80815=ORIENTED_EDGE('',*,*,#55402,.T.);
#80816=ORIENTED_EDGE('',*,*,#55364,.F.);
#80817=ORIENTED_EDGE('',*,*,#55367,.T.);
#80818=ORIENTED_EDGE('',*,*,#55368,.T.);
#80819=ORIENTED_EDGE('',*,*,#55403,.T.);
#80820=ORIENTED_EDGE('',*,*,#55351,.F.);
#80821=ORIENTED_EDGE('',*,*,#55362,.T.);
#80822=ORIENTED_EDGE('',*,*,#55363,.T.);
#80823=ORIENTED_EDGE('',*,*,#55404,.T.);
#80824=ORIENTED_EDGE('',*,*,#55405,.F.);
#80825=ORIENTED_EDGE('',*,*,#55406,.T.);
#80826=ORIENTED_EDGE('',*,*,#55407,.F.);
#80827=ORIENTED_EDGE('',*,*,#55408,.F.);
#80828=ORIENTED_EDGE('',*,*,#55409,.F.);
#80829=ORIENTED_EDGE('',*,*,#55410,.T.);
#80830=ORIENTED_EDGE('',*,*,#55411,.F.);
#80831=ORIENTED_EDGE('',*,*,#55412,.F.);
#80832=ORIENTED_EDGE('',*,*,#55413,.F.);
#80833=ORIENTED_EDGE('',*,*,#55414,.T.);
#80834=ORIENTED_EDGE('',*,*,#55415,.F.);
#80835=ORIENTED_EDGE('',*,*,#55416,.F.);
#80836=ORIENTED_EDGE('',*,*,#55417,.F.);
#80837=ORIENTED_EDGE('',*,*,#55418,.T.);
#80838=ORIENTED_EDGE('',*,*,#55419,.F.);
#80839=ORIENTED_EDGE('',*,*,#55420,.F.);
#80840=ORIENTED_EDGE('',*,*,#55421,.T.);
#80841=ORIENTED_EDGE('',*,*,#55417,.T.);
#80842=ORIENTED_EDGE('',*,*,#55422,.T.);
#80843=ORIENTED_EDGE('',*,*,#55346,.F.);
#80844=ORIENTED_EDGE('',*,*,#55423,.T.);
#80845=ORIENTED_EDGE('',*,*,#55424,.F.);
#80846=ORIENTED_EDGE('',*,*,#55425,.F.);
#80847=ORIENTED_EDGE('',*,*,#55418,.F.);
#80848=ORIENTED_EDGE('',*,*,#55426,.F.);
#80849=ORIENTED_EDGE('',*,*,#55427,.T.);
#80850=ORIENTED_EDGE('',*,*,#55428,.F.);
#80851=ORIENTED_EDGE('',*,*,#55429,.F.);
#80852=ORIENTED_EDGE('',*,*,#55430,.F.);
#80853=ORIENTED_EDGE('',*,*,#55431,.T.);
#80854=ORIENTED_EDGE('',*,*,#55432,.F.);
#80855=ORIENTED_EDGE('',*,*,#55433,.F.);
#80856=ORIENTED_EDGE('',*,*,#55419,.T.);
#80857=ORIENTED_EDGE('',*,*,#55434,.T.);
#80858=ORIENTED_EDGE('',*,*,#55430,.T.);
#80859=ORIENTED_EDGE('',*,*,#55435,.T.);
#80860=ORIENTED_EDGE('',*,*,#55436,.T.);
#80861=ORIENTED_EDGE('',*,*,#55437,.F.);
#80862=ORIENTED_EDGE('',*,*,#55438,.F.);
#80863=ORIENTED_EDGE('',*,*,#55431,.F.);
#80864=ORIENTED_EDGE('',*,*,#55432,.T.);
#80865=ORIENTED_EDGE('',*,*,#55439,.T.);
#80866=ORIENTED_EDGE('',*,*,#55426,.T.);
#80867=ORIENTED_EDGE('',*,*,#55440,.T.);
#80868=ORIENTED_EDGE('',*,*,#55441,.T.);
#80869=ORIENTED_EDGE('',*,*,#55442,.F.);
#80870=ORIENTED_EDGE('',*,*,#55443,.F.);
#80871=ORIENTED_EDGE('',*,*,#55427,.F.);
#80872=ORIENTED_EDGE('',*,*,#55428,.T.);
#80873=ORIENTED_EDGE('',*,*,#55444,.T.);
#80874=ORIENTED_EDGE('',*,*,#55413,.T.);
#80875=ORIENTED_EDGE('',*,*,#55445,.T.);
#80876=ORIENTED_EDGE('',*,*,#55446,.T.);
#80877=ORIENTED_EDGE('',*,*,#55447,.F.);
#80878=ORIENTED_EDGE('',*,*,#55448,.F.);
#80879=ORIENTED_EDGE('',*,*,#55414,.F.);
#80880=ORIENTED_EDGE('',*,*,#55449,.T.);
#80881=ORIENTED_EDGE('',*,*,#55415,.T.);
#80882=ORIENTED_EDGE('',*,*,#55450,.T.);
#80883=ORIENTED_EDGE('',*,*,#55409,.T.);
#80884=ORIENTED_EDGE('',*,*,#55451,.T.);
#80885=ORIENTED_EDGE('',*,*,#55452,.F.);
#80886=ORIENTED_EDGE('',*,*,#55453,.F.);
#80887=ORIENTED_EDGE('',*,*,#55410,.F.);
#80888=ORIENTED_EDGE('',*,*,#55454,.F.);
#80889=ORIENTED_EDGE('',*,*,#55455,.T.);
#80890=ORIENTED_EDGE('',*,*,#55456,.F.);
#80891=ORIENTED_EDGE('',*,*,#55457,.F.);
#80892=ORIENTED_EDGE('',*,*,#55458,.F.);
#80893=ORIENTED_EDGE('',*,*,#55459,.T.);
#80894=ORIENTED_EDGE('',*,*,#55460,.F.);
#80895=ORIENTED_EDGE('',*,*,#55461,.F.);
#80896=ORIENTED_EDGE('',*,*,#55411,.T.);
#80897=ORIENTED_EDGE('',*,*,#55462,.T.);
#80898=ORIENTED_EDGE('',*,*,#55458,.T.);
#80899=ORIENTED_EDGE('',*,*,#55463,.T.);
#80900=ORIENTED_EDGE('',*,*,#55464,.T.);
#80901=ORIENTED_EDGE('',*,*,#55465,.F.);
#80902=ORIENTED_EDGE('',*,*,#55466,.F.);
#80903=ORIENTED_EDGE('',*,*,#55459,.F.);
#80904=ORIENTED_EDGE('',*,*,#55460,.T.);
#80905=ORIENTED_EDGE('',*,*,#55467,.T.);
#80906=ORIENTED_EDGE('',*,*,#55454,.T.);
#80907=ORIENTED_EDGE('',*,*,#55468,.T.);
#80908=ORIENTED_EDGE('',*,*,#55469,.T.);
#80909=ORIENTED_EDGE('',*,*,#55470,.F.);
#80910=ORIENTED_EDGE('',*,*,#55471,.F.);
#80911=ORIENTED_EDGE('',*,*,#55455,.F.);
#80912=ORIENTED_EDGE('',*,*,#55456,.T.);
#80913=ORIENTED_EDGE('',*,*,#55472,.T.);
#80914=ORIENTED_EDGE('',*,*,#55405,.T.);
#80915=ORIENTED_EDGE('',*,*,#55473,.T.);
#80916=ORIENTED_EDGE('',*,*,#55474,.T.);
#80917=ORIENTED_EDGE('',*,*,#55475,.F.);
#80918=ORIENTED_EDGE('',*,*,#55476,.F.);
#80919=ORIENTED_EDGE('',*,*,#55406,.F.);
#80920=ORIENTED_EDGE('',*,*,#55477,.T.);
#80921=ORIENTED_EDGE('',*,*,#55340,.F.);
#80922=ORIENTED_EDGE('',*,*,#55478,.T.);
#80923=ORIENTED_EDGE('',*,*,#55407,.T.);
#80924=ORIENTED_EDGE('',*,*,#55477,.F.);
#80925=ORIENTED_EDGE('',*,*,#55476,.T.);
#80926=ORIENTED_EDGE('',*,*,#55479,.F.);
#80927=ORIENTED_EDGE('',*,*,#55398,.F.);
#80928=ORIENTED_EDGE('',*,*,#55480,.F.);
#80929=ORIENTED_EDGE('',*,*,#55316,.T.);
#80930=ORIENTED_EDGE('',*,*,#55481,.F.);
#80931=ORIENTED_EDGE('',*,*,#55327,.T.);
#80932=ORIENTED_EDGE('',*,*,#55482,.F.);
#80933=ORIENTED_EDGE('',*,*,#55321,.T.);
#80934=ORIENTED_EDGE('',*,*,#55177,.F.);
#80935=ORIENTED_EDGE('',*,*,#55334,.T.);
#80936=ORIENTED_EDGE('',*,*,#55421,.F.);
#80937=ORIENTED_EDGE('',*,*,#55350,.T.);
#80938=ORIENTED_EDGE('',*,*,#55483,.F.);
#80939=ORIENTED_EDGE('',*,*,#55423,.F.);
#80940=ORIENTED_EDGE('',*,*,#55448,.T.);
#80941=ORIENTED_EDGE('',*,*,#55484,.F.);
#80942=ORIENTED_EDGE('',*,*,#55451,.F.);
#80943=ORIENTED_EDGE('',*,*,#55450,.F.);
#80944=ORIENTED_EDGE('',*,*,#55471,.T.);
#80945=ORIENTED_EDGE('',*,*,#55485,.F.);
#80946=ORIENTED_EDGE('',*,*,#55474,.F.);
#80947=ORIENTED_EDGE('',*,*,#55472,.F.);
#80948=ORIENTED_EDGE('',*,*,#55466,.T.);
#80949=ORIENTED_EDGE('',*,*,#55486,.F.);
#80950=ORIENTED_EDGE('',*,*,#55469,.F.);
#80951=ORIENTED_EDGE('',*,*,#55467,.F.);
#80952=ORIENTED_EDGE('',*,*,#55453,.T.);
#80953=ORIENTED_EDGE('',*,*,#55487,.F.);
#80954=ORIENTED_EDGE('',*,*,#55464,.F.);
#80955=ORIENTED_EDGE('',*,*,#55462,.F.);
#80956=ORIENTED_EDGE('',*,*,#55443,.T.);
#80957=ORIENTED_EDGE('',*,*,#55488,.F.);
#80958=ORIENTED_EDGE('',*,*,#55446,.F.);
#80959=ORIENTED_EDGE('',*,*,#55444,.F.);
#80960=ORIENTED_EDGE('',*,*,#55438,.T.);
#80961=ORIENTED_EDGE('',*,*,#55489,.F.);
#80962=ORIENTED_EDGE('',*,*,#55441,.F.);
#80963=ORIENTED_EDGE('',*,*,#55439,.F.);
#80964=ORIENTED_EDGE('',*,*,#55425,.T.);
#80965=ORIENTED_EDGE('',*,*,#55490,.F.);
#80966=ORIENTED_EDGE('',*,*,#55436,.F.);
#80967=ORIENTED_EDGE('',*,*,#55434,.F.);
#80968=ORIENTED_EDGE('',*,*,#55385,.T.);
#80969=ORIENTED_EDGE('',*,*,#55266,.T.);
#80970=ORIENTED_EDGE('',*,*,#55491,.T.);
#80971=ORIENTED_EDGE('',*,*,#55492,.T.);
#80972=ORIENTED_EDGE('',*,*,#55491,.F.);
#80973=ORIENTED_EDGE('',*,*,#55269,.T.);
#80974=ORIENTED_EDGE('',*,*,#55493,.F.);
#80975=ORIENTED_EDGE('',*,*,#55344,.F.);
#80976=ORIENTED_EDGE('',*,*,#55494,.F.);
#80977=ORIENTED_EDGE('',*,*,#55493,.T.);
#80978=ORIENTED_EDGE('',*,*,#55272,.T.);
#80979=ORIENTED_EDGE('',*,*,#55291,.T.);
#80980=ORIENTED_EDGE('',*,*,#55309,.T.);
#80981=ORIENTED_EDGE('',*,*,#55495,.T.);
#80982=ORIENTED_EDGE('',*,*,#55374,.F.);
#80983=ORIENTED_EDGE('',*,*,#55496,.T.);
#80984=ORIENTED_EDGE('',*,*,#55258,.T.);
#80985=ORIENTED_EDGE('',*,*,#55384,.T.);
#80986=ORIENTED_EDGE('',*,*,#55387,.T.);
#80987=ORIENTED_EDGE('',*,*,#55497,.T.);
#80988=ORIENTED_EDGE('',*,*,#55498,.T.);
#80989=ORIENTED_EDGE('',*,*,#55499,.F.);
#80990=ORIENTED_EDGE('',*,*,#55498,.F.);
#80991=ORIENTED_EDGE('',*,*,#55500,.T.);
#80992=ORIENTED_EDGE('',*,*,#55501,.T.);
#80993=ORIENTED_EDGE('',*,*,#55502,.T.);
#80994=ORIENTED_EDGE('',*,*,#55499,.T.);
#80995=ORIENTED_EDGE('',*,*,#55503,.T.);
#80996=ORIENTED_EDGE('',*,*,#55078,.T.);
#80997=ORIENTED_EDGE('',*,*,#55504,.F.);
#80998=ORIENTED_EDGE('',*,*,#55505,.T.);
#80999=ORIENTED_EDGE('',*,*,#55506,.T.);
#81000=ORIENTED_EDGE('',*,*,#55507,.F.);
#81001=ORIENTED_EDGE('',*,*,#55508,.T.);
#81002=ORIENTED_EDGE('',*,*,#55509,.T.);
#81003=ORIENTED_EDGE('',*,*,#55510,.T.);
#81004=ORIENTED_EDGE('',*,*,#55511,.T.);
#81005=ORIENTED_EDGE('',*,*,#55512,.F.);
#81006=ORIENTED_EDGE('',*,*,#55513,.F.);
#81007=ORIENTED_EDGE('',*,*,#55514,.T.);
#81008=ORIENTED_EDGE('',*,*,#55515,.F.);
#81009=ORIENTED_EDGE('',*,*,#54715,.F.);
#81010=ORIENTED_EDGE('',*,*,#55510,.F.);
#81011=ORIENTED_EDGE('',*,*,#55500,.F.);
#81012=ORIENTED_EDGE('',*,*,#55497,.F.);
#81013=ORIENTED_EDGE('',*,*,#55502,.F.);
#81014=ORIENTED_EDGE('',*,*,#55508,.F.);
#81015=ORIENTED_EDGE('',*,*,#55129,.T.);
#81016=ORIENTED_EDGE('',*,*,#55516,.T.);
#81017=ORIENTED_EDGE('',*,*,#55126,.F.);
#81018=ORIENTED_EDGE('',*,*,#55517,.F.);
#81019=ORIENTED_EDGE('',*,*,#55501,.F.);
#81020=ORIENTED_EDGE('',*,*,#55509,.F.);
#81021=ORIENTED_EDGE('',*,*,#54716,.F.);
#81022=ORIENTED_EDGE('',*,*,#55518,.F.);
#81023=ORIENTED_EDGE('',*,*,#55073,.F.);
#81024=ORIENTED_EDGE('',*,*,#55079,.F.);
#81025=ORIENTED_EDGE('',*,*,#55503,.F.);
#81026=ORIENTED_EDGE('',*,*,#55077,.F.);
#81027=ORIENTED_EDGE('',*,*,#55082,.F.);
#81028=ORIENTED_EDGE('',*,*,#55085,.F.);
#81029=ORIENTED_EDGE('',*,*,#55088,.F.);
#81030=ORIENTED_EDGE('',*,*,#55091,.F.);
#81031=ORIENTED_EDGE('',*,*,#55094,.F.);
#81032=ORIENTED_EDGE('',*,*,#55097,.F.);
#81033=ORIENTED_EDGE('',*,*,#55100,.F.);
#81034=ORIENTED_EDGE('',*,*,#55103,.F.);
#81035=ORIENTED_EDGE('',*,*,#55106,.F.);
#81036=ORIENTED_EDGE('',*,*,#55109,.F.);
#81037=ORIENTED_EDGE('',*,*,#55112,.F.);
#81038=ORIENTED_EDGE('',*,*,#55115,.F.);
#81039=ORIENTED_EDGE('',*,*,#55118,.F.);
#81040=ORIENTED_EDGE('',*,*,#55121,.F.);
#81041=ORIENTED_EDGE('',*,*,#55124,.F.);
#81042=ORIENTED_EDGE('',*,*,#55127,.F.);
#81043=ORIENTED_EDGE('',*,*,#55516,.F.);
#81044=ORIENTED_EDGE('',*,*,#55131,.F.);
#81045=ORIENTED_EDGE('',*,*,#55519,.F.);
#81046=ORIENTED_EDGE('',*,*,#54659,.F.);
#81047=ORIENTED_EDGE('',*,*,#54663,.F.);
#81048=ORIENTED_EDGE('',*,*,#54666,.F.);
#81049=ORIENTED_EDGE('',*,*,#54669,.F.);
#81050=ORIENTED_EDGE('',*,*,#54672,.F.);
#81051=ORIENTED_EDGE('',*,*,#54675,.F.);
#81052=ORIENTED_EDGE('',*,*,#54678,.F.);
#81053=ORIENTED_EDGE('',*,*,#54681,.F.);
#81054=ORIENTED_EDGE('',*,*,#54684,.F.);
#81055=ORIENTED_EDGE('',*,*,#54687,.F.);
#81056=ORIENTED_EDGE('',*,*,#54690,.F.);
#81057=ORIENTED_EDGE('',*,*,#54693,.F.);
#81058=ORIENTED_EDGE('',*,*,#54696,.F.);
#81059=ORIENTED_EDGE('',*,*,#54699,.F.);
#81060=ORIENTED_EDGE('',*,*,#54702,.F.);
#81061=ORIENTED_EDGE('',*,*,#54705,.F.);
#81062=ORIENTED_EDGE('',*,*,#54708,.F.);
#81063=ORIENTED_EDGE('',*,*,#54711,.F.);
#81064=ORIENTED_EDGE('',*,*,#55520,.F.);
#81065=ORIENTED_EDGE('',*,*,#55521,.F.);
#81066=ORIENTED_EDGE('',*,*,#55522,.F.);
#81067=ORIENTED_EDGE('',*,*,#55511,.F.);
#81068=ORIENTED_EDGE('',*,*,#54714,.F.);
#81069=ORIENTED_EDGE('',*,*,#54661,.F.);
#81070=ORIENTED_EDGE('',*,*,#55523,.F.);
#81071=ORIENTED_EDGE('',*,*,#55517,.T.);
#81072=ORIENTED_EDGE('',*,*,#55128,.T.);
#81073=ORIENTED_EDGE('',*,*,#55125,.T.);
#81074=ORIENTED_EDGE('',*,*,#55122,.T.);
#81075=ORIENTED_EDGE('',*,*,#55119,.T.);
#81076=ORIENTED_EDGE('',*,*,#55116,.T.);
#81077=ORIENTED_EDGE('',*,*,#55113,.T.);
#81078=ORIENTED_EDGE('',*,*,#55110,.T.);
#81079=ORIENTED_EDGE('',*,*,#55107,.T.);
#81080=ORIENTED_EDGE('',*,*,#55104,.T.);
#81081=ORIENTED_EDGE('',*,*,#55101,.T.);
#81082=ORIENTED_EDGE('',*,*,#55098,.T.);
#81083=ORIENTED_EDGE('',*,*,#55095,.T.);
#81084=ORIENTED_EDGE('',*,*,#55092,.T.);
#81085=ORIENTED_EDGE('',*,*,#55089,.T.);
#81086=ORIENTED_EDGE('',*,*,#55086,.T.);
#81087=ORIENTED_EDGE('',*,*,#55083,.T.);
#81088=ORIENTED_EDGE('',*,*,#55080,.T.);
#81089=ORIENTED_EDGE('',*,*,#55075,.T.);
#81090=ORIENTED_EDGE('',*,*,#55524,.F.);
#81091=ORIENTED_EDGE('',*,*,#55506,.F.);
#81092=ORIENTED_EDGE('',*,*,#55525,.F.);
#81093=ORIENTED_EDGE('',*,*,#54712,.F.);
#81094=ORIENTED_EDGE('',*,*,#54709,.F.);
#81095=ORIENTED_EDGE('',*,*,#54706,.F.);
#81096=ORIENTED_EDGE('',*,*,#54703,.F.);
#81097=ORIENTED_EDGE('',*,*,#54700,.F.);
#81098=ORIENTED_EDGE('',*,*,#54697,.F.);
#81099=ORIENTED_EDGE('',*,*,#54694,.F.);
#81100=ORIENTED_EDGE('',*,*,#54691,.F.);
#81101=ORIENTED_EDGE('',*,*,#54688,.F.);
#81102=ORIENTED_EDGE('',*,*,#54685,.F.);
#81103=ORIENTED_EDGE('',*,*,#54682,.F.);
#81104=ORIENTED_EDGE('',*,*,#54679,.F.);
#81105=ORIENTED_EDGE('',*,*,#54676,.F.);
#81106=ORIENTED_EDGE('',*,*,#54673,.F.);
#81107=ORIENTED_EDGE('',*,*,#54670,.F.);
#81108=ORIENTED_EDGE('',*,*,#54667,.F.);
#81109=ORIENTED_EDGE('',*,*,#54664,.F.);
#81110=ORIENTED_EDGE('',*,*,#55526,.F.);
#81111=ORIENTED_EDGE('',*,*,#55527,.T.);
#81112=ORIENTED_EDGE('',*,*,#55528,.T.);
#81113=ORIENTED_EDGE('',*,*,#55018,.T.);
#81114=ORIENTED_EDGE('',*,*,#55529,.T.);
#81115=ORIENTED_EDGE('',*,*,#55530,.T.);
#81116=ORIENTED_EDGE('',*,*,#55014,.T.);
#81117=ORIENTED_EDGE('',*,*,#55531,.T.);
#81118=ORIENTED_EDGE('',*,*,#55532,.F.);
#81119=ORIENTED_EDGE('',*,*,#55533,.T.);
#81120=ORIENTED_EDGE('',*,*,#55534,.T.);
#81121=ORIENTED_EDGE('',*,*,#55535,.F.);
#81122=ORIENTED_EDGE('',*,*,#55536,.T.);
#81123=ORIENTED_EDGE('',*,*,#55537,.T.);
#81124=ORIENTED_EDGE('',*,*,#55538,.F.);
#81125=ORIENTED_EDGE('',*,*,#55539,.T.);
#81126=ORIENTED_EDGE('',*,*,#55529,.F.);
#81127=ORIENTED_EDGE('',*,*,#54774,.T.);
#81128=ORIENTED_EDGE('',*,*,#55533,.F.);
#81129=ORIENTED_EDGE('',*,*,#55069,.T.);
#81130=ORIENTED_EDGE('',*,*,#55540,.T.);
#81131=ORIENTED_EDGE('',*,*,#55066,.F.);
#81132=ORIENTED_EDGE('',*,*,#55541,.F.);
#81133=ORIENTED_EDGE('',*,*,#55527,.F.);
#81134=ORIENTED_EDGE('',*,*,#55542,.F.);
#81135=ORIENTED_EDGE('',*,*,#54775,.F.);
#81136=ORIENTED_EDGE('',*,*,#55531,.F.);
#81137=ORIENTED_EDGE('',*,*,#55013,.F.);
#81138=ORIENTED_EDGE('',*,*,#55019,.F.);
#81139=ORIENTED_EDGE('',*,*,#55528,.F.);
#81140=ORIENTED_EDGE('',*,*,#55017,.F.);
#81141=ORIENTED_EDGE('',*,*,#55022,.F.);
#81142=ORIENTED_EDGE('',*,*,#55025,.F.);
#81143=ORIENTED_EDGE('',*,*,#55028,.F.);
#81144=ORIENTED_EDGE('',*,*,#55031,.F.);
#81145=ORIENTED_EDGE('',*,*,#55034,.F.);
#81146=ORIENTED_EDGE('',*,*,#55037,.F.);
#81147=ORIENTED_EDGE('',*,*,#55040,.F.);
#81148=ORIENTED_EDGE('',*,*,#55043,.F.);
#81149=ORIENTED_EDGE('',*,*,#55046,.F.);
#81150=ORIENTED_EDGE('',*,*,#55049,.F.);
#81151=ORIENTED_EDGE('',*,*,#55052,.F.);
#81152=ORIENTED_EDGE('',*,*,#55055,.F.);
#81153=ORIENTED_EDGE('',*,*,#55058,.F.);
#81154=ORIENTED_EDGE('',*,*,#55061,.F.);
#81155=ORIENTED_EDGE('',*,*,#55064,.F.);
#81156=ORIENTED_EDGE('',*,*,#55067,.F.);
#81157=ORIENTED_EDGE('',*,*,#55540,.F.);
#81158=ORIENTED_EDGE('',*,*,#55071,.F.);
#81159=ORIENTED_EDGE('',*,*,#55543,.F.);
#81160=ORIENTED_EDGE('',*,*,#54718,.F.);
#81161=ORIENTED_EDGE('',*,*,#54722,.F.);
#81162=ORIENTED_EDGE('',*,*,#54725,.F.);
#81163=ORIENTED_EDGE('',*,*,#54728,.F.);
#81164=ORIENTED_EDGE('',*,*,#54731,.F.);
#81165=ORIENTED_EDGE('',*,*,#54734,.F.);
#81166=ORIENTED_EDGE('',*,*,#54737,.F.);
#81167=ORIENTED_EDGE('',*,*,#54740,.F.);
#81168=ORIENTED_EDGE('',*,*,#54743,.F.);
#81169=ORIENTED_EDGE('',*,*,#54746,.F.);
#81170=ORIENTED_EDGE('',*,*,#54749,.F.);
#81171=ORIENTED_EDGE('',*,*,#54752,.F.);
#81172=ORIENTED_EDGE('',*,*,#54755,.F.);
#81173=ORIENTED_EDGE('',*,*,#54758,.F.);
#81174=ORIENTED_EDGE('',*,*,#54761,.F.);
#81175=ORIENTED_EDGE('',*,*,#54764,.F.);
#81176=ORIENTED_EDGE('',*,*,#54767,.F.);
#81177=ORIENTED_EDGE('',*,*,#54770,.F.);
#81178=ORIENTED_EDGE('',*,*,#55544,.F.);
#81179=ORIENTED_EDGE('',*,*,#55545,.F.);
#81180=ORIENTED_EDGE('',*,*,#55546,.F.);
#81181=ORIENTED_EDGE('',*,*,#55547,.F.);
#81182=ORIENTED_EDGE('',*,*,#55534,.F.);
#81183=ORIENTED_EDGE('',*,*,#54773,.F.);
#81184=ORIENTED_EDGE('',*,*,#54720,.F.);
#81185=ORIENTED_EDGE('',*,*,#55548,.F.);
#81186=ORIENTED_EDGE('',*,*,#55541,.T.);
#81187=ORIENTED_EDGE('',*,*,#55068,.T.);
#81188=ORIENTED_EDGE('',*,*,#55065,.T.);
#81189=ORIENTED_EDGE('',*,*,#55062,.T.);
#81190=ORIENTED_EDGE('',*,*,#55059,.T.);
#81191=ORIENTED_EDGE('',*,*,#55056,.T.);
#81192=ORIENTED_EDGE('',*,*,#55053,.T.);
#81193=ORIENTED_EDGE('',*,*,#55050,.T.);
#81194=ORIENTED_EDGE('',*,*,#55047,.T.);
#81195=ORIENTED_EDGE('',*,*,#55044,.T.);
#81196=ORIENTED_EDGE('',*,*,#55041,.T.);
#81197=ORIENTED_EDGE('',*,*,#55038,.T.);
#81198=ORIENTED_EDGE('',*,*,#55035,.T.);
#81199=ORIENTED_EDGE('',*,*,#55032,.T.);
#81200=ORIENTED_EDGE('',*,*,#55029,.T.);
#81201=ORIENTED_EDGE('',*,*,#55026,.T.);
#81202=ORIENTED_EDGE('',*,*,#55023,.T.);
#81203=ORIENTED_EDGE('',*,*,#55020,.T.);
#81204=ORIENTED_EDGE('',*,*,#55015,.T.);
#81205=ORIENTED_EDGE('',*,*,#55530,.F.);
#81206=ORIENTED_EDGE('',*,*,#55549,.F.);
#81207=ORIENTED_EDGE('',*,*,#54771,.F.);
#81208=ORIENTED_EDGE('',*,*,#54768,.F.);
#81209=ORIENTED_EDGE('',*,*,#54765,.F.);
#81210=ORIENTED_EDGE('',*,*,#54762,.F.);
#81211=ORIENTED_EDGE('',*,*,#54759,.F.);
#81212=ORIENTED_EDGE('',*,*,#54756,.F.);
#81213=ORIENTED_EDGE('',*,*,#54753,.F.);
#81214=ORIENTED_EDGE('',*,*,#54750,.F.);
#81215=ORIENTED_EDGE('',*,*,#54747,.F.);
#81216=ORIENTED_EDGE('',*,*,#54744,.F.);
#81217=ORIENTED_EDGE('',*,*,#54741,.F.);
#81218=ORIENTED_EDGE('',*,*,#54738,.F.);
#81219=ORIENTED_EDGE('',*,*,#54735,.F.);
#81220=ORIENTED_EDGE('',*,*,#54732,.F.);
#81221=ORIENTED_EDGE('',*,*,#54729,.F.);
#81222=ORIENTED_EDGE('',*,*,#54726,.F.);
#81223=ORIENTED_EDGE('',*,*,#54723,.F.);
#81224=ORIENTED_EDGE('',*,*,#55550,.F.);
#81225=ORIENTED_EDGE('',*,*,#55551,.T.);
#81226=ORIENTED_EDGE('',*,*,#55552,.F.);
#81227=ORIENTED_EDGE('',*,*,#55250,.F.);
#81228=ORIENTED_EDGE('',*,*,#55008,.T.);
#81229=ORIENTED_EDGE('',*,*,#55553,.T.);
#81230=ORIENTED_EDGE('',*,*,#55005,.F.);
#81231=ORIENTED_EDGE('',*,*,#55554,.T.);
#81232=ORIENTED_EDGE('',*,*,#55555,.F.);
#81233=ORIENTED_EDGE('',*,*,#55556,.T.);
#81234=ORIENTED_EDGE('',*,*,#55557,.T.);
#81235=ORIENTED_EDGE('',*,*,#54900,.T.);
#81236=ORIENTED_EDGE('',*,*,#55558,.T.);
#81237=ORIENTED_EDGE('',*,*,#55559,.T.);
#81238=ORIENTED_EDGE('',*,*,#54896,.T.);
#81239=ORIENTED_EDGE('',*,*,#55560,.T.);
#81240=ORIENTED_EDGE('',*,*,#55561,.F.);
#81241=ORIENTED_EDGE('',*,*,#55562,.T.);
#81242=ORIENTED_EDGE('',*,*,#55563,.T.);
#81243=ORIENTED_EDGE('',*,*,#55564,.F.);
#81244=ORIENTED_EDGE('',*,*,#55565,.T.);
#81245=ORIENTED_EDGE('',*,*,#55566,.T.);
#81246=ORIENTED_EDGE('',*,*,#55567,.F.);
#81247=ORIENTED_EDGE('',*,*,#55555,.T.);
#81248=ORIENTED_EDGE('',*,*,#55558,.F.);
#81249=ORIENTED_EDGE('',*,*,#55010,.T.);
#81250=ORIENTED_EDGE('',*,*,#55562,.F.);
#81251=ORIENTED_EDGE('',*,*,#54951,.T.);
#81252=ORIENTED_EDGE('',*,*,#55568,.T.);
#81253=ORIENTED_EDGE('',*,*,#54948,.F.);
#81254=ORIENTED_EDGE('',*,*,#55569,.F.);
#81255=ORIENTED_EDGE('',*,*,#55551,.F.);
#81256=ORIENTED_EDGE('',*,*,#55570,.F.);
#81257=ORIENTED_EDGE('',*,*,#55011,.F.);
#81258=ORIENTED_EDGE('',*,*,#55560,.F.);
#81259=ORIENTED_EDGE('',*,*,#54895,.F.);
#81260=ORIENTED_EDGE('',*,*,#54901,.F.);
#81261=ORIENTED_EDGE('',*,*,#55557,.F.);
#81262=ORIENTED_EDGE('',*,*,#54899,.F.);
#81263=ORIENTED_EDGE('',*,*,#54904,.F.);
#81264=ORIENTED_EDGE('',*,*,#54907,.F.);
#81265=ORIENTED_EDGE('',*,*,#54910,.F.);
#81266=ORIENTED_EDGE('',*,*,#54913,.F.);
#81267=ORIENTED_EDGE('',*,*,#54916,.F.);
#81268=ORIENTED_EDGE('',*,*,#54919,.F.);
#81269=ORIENTED_EDGE('',*,*,#54922,.F.);
#81270=ORIENTED_EDGE('',*,*,#54925,.F.);
#81271=ORIENTED_EDGE('',*,*,#54928,.F.);
#81272=ORIENTED_EDGE('',*,*,#54931,.F.);
#81273=ORIENTED_EDGE('',*,*,#54934,.F.);
#81274=ORIENTED_EDGE('',*,*,#54937,.F.);
#81275=ORIENTED_EDGE('',*,*,#54940,.F.);
#81276=ORIENTED_EDGE('',*,*,#54943,.F.);
#81277=ORIENTED_EDGE('',*,*,#54946,.F.);
#81278=ORIENTED_EDGE('',*,*,#54949,.F.);
#81279=ORIENTED_EDGE('',*,*,#55568,.F.);
#81280=ORIENTED_EDGE('',*,*,#54953,.F.);
#81281=ORIENTED_EDGE('',*,*,#55571,.F.);
#81282=ORIENTED_EDGE('',*,*,#54958,.F.);
#81283=ORIENTED_EDGE('',*,*,#54961,.F.);
#81284=ORIENTED_EDGE('',*,*,#54964,.F.);
#81285=ORIENTED_EDGE('',*,*,#54967,.F.);
#81286=ORIENTED_EDGE('',*,*,#54970,.F.);
#81287=ORIENTED_EDGE('',*,*,#54973,.F.);
#81288=ORIENTED_EDGE('',*,*,#54976,.F.);
#81289=ORIENTED_EDGE('',*,*,#54979,.F.);
#81290=ORIENTED_EDGE('',*,*,#54982,.F.);
#81291=ORIENTED_EDGE('',*,*,#54985,.F.);
#81292=ORIENTED_EDGE('',*,*,#54988,.F.);
#81293=ORIENTED_EDGE('',*,*,#54991,.F.);
#81294=ORIENTED_EDGE('',*,*,#54994,.F.);
#81295=ORIENTED_EDGE('',*,*,#54997,.F.);
#81296=ORIENTED_EDGE('',*,*,#55000,.F.);
#81297=ORIENTED_EDGE('',*,*,#55003,.F.);
#81298=ORIENTED_EDGE('',*,*,#55006,.F.);
#81299=ORIENTED_EDGE('',*,*,#55553,.F.);
#81300=ORIENTED_EDGE('',*,*,#55556,.F.);
#81301=ORIENTED_EDGE('',*,*,#55572,.F.);
#81302=ORIENTED_EDGE('',*,*,#55573,.F.);
#81303=ORIENTED_EDGE('',*,*,#55563,.F.);
#81304=ORIENTED_EDGE('',*,*,#55009,.F.);
#81305=ORIENTED_EDGE('',*,*,#54956,.F.);
#81306=ORIENTED_EDGE('',*,*,#55574,.F.);
#81307=ORIENTED_EDGE('',*,*,#55569,.T.);
#81308=ORIENTED_EDGE('',*,*,#54950,.T.);
#81309=ORIENTED_EDGE('',*,*,#54947,.T.);
#81310=ORIENTED_EDGE('',*,*,#54944,.T.);
#81311=ORIENTED_EDGE('',*,*,#54941,.T.);
#81312=ORIENTED_EDGE('',*,*,#54938,.T.);
#81313=ORIENTED_EDGE('',*,*,#54935,.T.);
#81314=ORIENTED_EDGE('',*,*,#54932,.T.);
#81315=ORIENTED_EDGE('',*,*,#54929,.T.);
#81316=ORIENTED_EDGE('',*,*,#54926,.T.);
#81317=ORIENTED_EDGE('',*,*,#54923,.T.);
#81318=ORIENTED_EDGE('',*,*,#54920,.T.);
#81319=ORIENTED_EDGE('',*,*,#54917,.T.);
#81320=ORIENTED_EDGE('',*,*,#54914,.T.);
#81321=ORIENTED_EDGE('',*,*,#54911,.T.);
#81322=ORIENTED_EDGE('',*,*,#54908,.T.);
#81323=ORIENTED_EDGE('',*,*,#54905,.T.);
#81324=ORIENTED_EDGE('',*,*,#54902,.T.);
#81325=ORIENTED_EDGE('',*,*,#54897,.T.);
#81326=ORIENTED_EDGE('',*,*,#55559,.F.);
#81327=ORIENTED_EDGE('',*,*,#55554,.F.);
#81328=ORIENTED_EDGE('',*,*,#55007,.F.);
#81329=ORIENTED_EDGE('',*,*,#55004,.F.);
#81330=ORIENTED_EDGE('',*,*,#55001,.F.);
#81331=ORIENTED_EDGE('',*,*,#54998,.F.);
#81332=ORIENTED_EDGE('',*,*,#54995,.F.);
#81333=ORIENTED_EDGE('',*,*,#54992,.F.);
#81334=ORIENTED_EDGE('',*,*,#54989,.F.);
#81335=ORIENTED_EDGE('',*,*,#54986,.F.);
#81336=ORIENTED_EDGE('',*,*,#54983,.F.);
#81337=ORIENTED_EDGE('',*,*,#54980,.F.);
#81338=ORIENTED_EDGE('',*,*,#54977,.F.);
#81339=ORIENTED_EDGE('',*,*,#54974,.F.);
#81340=ORIENTED_EDGE('',*,*,#54971,.F.);
#81341=ORIENTED_EDGE('',*,*,#54968,.F.);
#81342=ORIENTED_EDGE('',*,*,#54965,.F.);
#81343=ORIENTED_EDGE('',*,*,#54962,.F.);
#81344=ORIENTED_EDGE('',*,*,#54959,.F.);
#81345=ORIENTED_EDGE('',*,*,#55575,.T.);
#81346=ORIENTED_EDGE('',*,*,#55253,.F.);
#81347=ORIENTED_EDGE('',*,*,#55576,.T.);
#81348=ORIENTED_EDGE('',*,*,#55577,.T.);
#81349=ORIENTED_EDGE('',*,*,#54888,.T.);
#81350=ORIENTED_EDGE('',*,*,#55578,.T.);
#81351=ORIENTED_EDGE('',*,*,#54885,.F.);
#81352=ORIENTED_EDGE('',*,*,#55579,.T.);
#81353=ORIENTED_EDGE('',*,*,#55580,.T.);
#81354=ORIENTED_EDGE('',*,*,#54782,.T.);
#81355=ORIENTED_EDGE('',*,*,#55581,.F.);
#81356=ORIENTED_EDGE('',*,*,#55582,.T.);
#81357=ORIENTED_EDGE('',*,*,#55583,.T.);
#81358=ORIENTED_EDGE('',*,*,#55584,.F.);
#81359=ORIENTED_EDGE('',*,*,#55585,.T.);
#81360=ORIENTED_EDGE('',*,*,#55586,.T.);
#81361=ORIENTED_EDGE('',*,*,#55587,.T.);
#81362=ORIENTED_EDGE('',*,*,#55588,.T.);
#81363=ORIENTED_EDGE('',*,*,#55589,.F.);
#81364=ORIENTED_EDGE('',*,*,#55590,.F.);
#81365=ORIENTED_EDGE('',*,*,#55591,.T.);
#81366=ORIENTED_EDGE('',*,*,#55592,.F.);
#81367=ORIENTED_EDGE('',*,*,#54892,.F.);
#81368=ORIENTED_EDGE('',*,*,#55587,.F.);
#81369=ORIENTED_EDGE('',*,*,#55576,.F.);
#81370=ORIENTED_EDGE('',*,*,#55251,.F.);
#81371=ORIENTED_EDGE('',*,*,#55575,.F.);
#81372=ORIENTED_EDGE('',*,*,#55585,.F.);
#81373=ORIENTED_EDGE('',*,*,#55468,.F.);
#81374=ORIENTED_EDGE('',*,*,#55457,.T.);
#81375=ORIENTED_EDGE('',*,*,#55473,.F.);
#81376=ORIENTED_EDGE('',*,*,#55408,.T.);
#81377=ORIENTED_EDGE('',*,*,#55478,.F.);
#81378=ORIENTED_EDGE('',*,*,#55339,.F.);
#81379=ORIENTED_EDGE('',*,*,#55395,.T.);
#81380=ORIENTED_EDGE('',*,*,#55377,.F.);
#81381=ORIENTED_EDGE('',*,*,#55390,.T.);
#81382=ORIENTED_EDGE('',*,*,#55381,.F.);
#81383=ORIENTED_EDGE('',*,*,#55386,.T.);
#81384=ORIENTED_EDGE('',*,*,#55492,.F.);
#81385=ORIENTED_EDGE('',*,*,#55494,.T.);
#81386=ORIENTED_EDGE('',*,*,#55343,.F.);
#81387=ORIENTED_EDGE('',*,*,#55371,.T.);
#81388=ORIENTED_EDGE('',*,*,#55354,.F.);
#81389=ORIENTED_EDGE('',*,*,#55366,.T.);
#81390=ORIENTED_EDGE('',*,*,#55358,.F.);
#81391=ORIENTED_EDGE('',*,*,#55361,.T.);
#81392=ORIENTED_EDGE('',*,*,#55347,.F.);
#81393=ORIENTED_EDGE('',*,*,#55422,.F.);
#81394=ORIENTED_EDGE('',*,*,#55420,.T.);
#81395=ORIENTED_EDGE('',*,*,#55435,.F.);
#81396=ORIENTED_EDGE('',*,*,#55433,.T.);
#81397=ORIENTED_EDGE('',*,*,#55440,.F.);
#81398=ORIENTED_EDGE('',*,*,#55429,.T.);
#81399=ORIENTED_EDGE('',*,*,#55445,.F.);
#81400=ORIENTED_EDGE('',*,*,#55416,.T.);
#81401=ORIENTED_EDGE('',*,*,#55449,.F.);
#81402=ORIENTED_EDGE('',*,*,#55412,.T.);
#81403=ORIENTED_EDGE('',*,*,#55463,.F.);
#81404=ORIENTED_EDGE('',*,*,#55461,.T.);
#81405=ORIENTED_EDGE('',*,*,#54955,.F.);
#81406=ORIENTED_EDGE('',*,*,#55571,.T.);
#81407=ORIENTED_EDGE('',*,*,#54952,.T.);
#81408=ORIENTED_EDGE('',*,*,#55574,.T.);
#81409=ORIENTED_EDGE('',*,*,#55523,.T.);
#81410=ORIENTED_EDGE('',*,*,#54660,.T.);
#81411=ORIENTED_EDGE('',*,*,#55519,.T.);
#81412=ORIENTED_EDGE('',*,*,#55130,.T.);
#81413=ORIENTED_EDGE('',*,*,#54719,.F.);
#81414=ORIENTED_EDGE('',*,*,#55543,.T.);
#81415=ORIENTED_EDGE('',*,*,#55070,.T.);
#81416=ORIENTED_EDGE('',*,*,#55548,.T.);
#81417=ORIENTED_EDGE('',*,*,#55593,.T.);
#81418=ORIENTED_EDGE('',*,*,#54838,.T.);
#81419=ORIENTED_EDGE('',*,*,#55594,.T.);
#81420=ORIENTED_EDGE('',*,*,#54834,.T.);
#81421=ORIENTED_EDGE('',*,*,#54833,.T.);
#81422=ORIENTED_EDGE('',*,*,#55595,.T.);
#81423=ORIENTED_EDGE('',*,*,#54830,.F.);
#81424=ORIENTED_EDGE('',*,*,#55596,.F.);
#81425=ORIENTED_EDGE('',*,*,#55577,.F.);
#81426=ORIENTED_EDGE('',*,*,#55586,.F.);
#81427=ORIENTED_EDGE('',*,*,#54893,.F.);
#81428=ORIENTED_EDGE('',*,*,#55597,.F.);
#81429=ORIENTED_EDGE('',*,*,#54777,.F.);
#81430=ORIENTED_EDGE('',*,*,#54783,.F.);
#81431=ORIENTED_EDGE('',*,*,#55580,.F.);
#81432=ORIENTED_EDGE('',*,*,#54781,.F.);
#81433=ORIENTED_EDGE('',*,*,#54786,.F.);
#81434=ORIENTED_EDGE('',*,*,#54789,.F.);
#81435=ORIENTED_EDGE('',*,*,#54792,.F.);
#81436=ORIENTED_EDGE('',*,*,#54795,.F.);
#81437=ORIENTED_EDGE('',*,*,#54798,.F.);
#81438=ORIENTED_EDGE('',*,*,#54801,.F.);
#81439=ORIENTED_EDGE('',*,*,#54804,.F.);
#81440=ORIENTED_EDGE('',*,*,#54807,.F.);
#81441=ORIENTED_EDGE('',*,*,#54810,.F.);
#81442=ORIENTED_EDGE('',*,*,#54813,.F.);
#81443=ORIENTED_EDGE('',*,*,#54816,.F.);
#81444=ORIENTED_EDGE('',*,*,#54819,.F.);
#81445=ORIENTED_EDGE('',*,*,#54822,.F.);
#81446=ORIENTED_EDGE('',*,*,#54825,.F.);
#81447=ORIENTED_EDGE('',*,*,#54828,.F.);
#81448=ORIENTED_EDGE('',*,*,#54831,.F.);
#81449=ORIENTED_EDGE('',*,*,#55595,.F.);
#81450=ORIENTED_EDGE('',*,*,#54835,.F.);
#81451=ORIENTED_EDGE('',*,*,#55594,.F.);
#81452=ORIENTED_EDGE('',*,*,#54837,.F.);
#81453=ORIENTED_EDGE('',*,*,#54841,.F.);
#81454=ORIENTED_EDGE('',*,*,#54844,.F.);
#81455=ORIENTED_EDGE('',*,*,#54847,.F.);
#81456=ORIENTED_EDGE('',*,*,#54850,.F.);
#81457=ORIENTED_EDGE('',*,*,#54853,.F.);
#81458=ORIENTED_EDGE('',*,*,#54856,.F.);
#81459=ORIENTED_EDGE('',*,*,#54859,.F.);
#81460=ORIENTED_EDGE('',*,*,#54862,.F.);
#81461=ORIENTED_EDGE('',*,*,#54865,.F.);
#81462=ORIENTED_EDGE('',*,*,#54868,.F.);
#81463=ORIENTED_EDGE('',*,*,#54871,.F.);
#81464=ORIENTED_EDGE('',*,*,#54874,.F.);
#81465=ORIENTED_EDGE('',*,*,#54877,.F.);
#81466=ORIENTED_EDGE('',*,*,#54880,.F.);
#81467=ORIENTED_EDGE('',*,*,#54883,.F.);
#81468=ORIENTED_EDGE('',*,*,#54886,.F.);
#81469=ORIENTED_EDGE('',*,*,#55578,.F.);
#81470=ORIENTED_EDGE('',*,*,#54891,.F.);
#81471=ORIENTED_EDGE('',*,*,#55598,.F.);
#81472=ORIENTED_EDGE('',*,*,#55588,.F.);
#81473=ORIENTED_EDGE('',*,*,#54839,.F.);
#81474=ORIENTED_EDGE('',*,*,#55593,.F.);
#81475=ORIENTED_EDGE('',*,*,#55596,.T.);
#81476=ORIENTED_EDGE('',*,*,#54832,.T.);
#81477=ORIENTED_EDGE('',*,*,#54829,.T.);
#81478=ORIENTED_EDGE('',*,*,#54826,.T.);
#81479=ORIENTED_EDGE('',*,*,#54823,.T.);
#81480=ORIENTED_EDGE('',*,*,#54820,.T.);
#81481=ORIENTED_EDGE('',*,*,#54817,.T.);
#81482=ORIENTED_EDGE('',*,*,#54814,.T.);
#81483=ORIENTED_EDGE('',*,*,#54811,.T.);
#81484=ORIENTED_EDGE('',*,*,#54808,.T.);
#81485=ORIENTED_EDGE('',*,*,#54805,.T.);
#81486=ORIENTED_EDGE('',*,*,#54802,.T.);
#81487=ORIENTED_EDGE('',*,*,#54799,.T.);
#81488=ORIENTED_EDGE('',*,*,#54796,.T.);
#81489=ORIENTED_EDGE('',*,*,#54793,.T.);
#81490=ORIENTED_EDGE('',*,*,#54790,.T.);
#81491=ORIENTED_EDGE('',*,*,#54787,.T.);
#81492=ORIENTED_EDGE('',*,*,#54784,.T.);
#81493=ORIENTED_EDGE('',*,*,#54779,.T.);
#81494=ORIENTED_EDGE('',*,*,#55599,.F.);
#81495=ORIENTED_EDGE('',*,*,#55583,.F.);
#81496=ORIENTED_EDGE('',*,*,#54889,.F.);
#81497=ORIENTED_EDGE('',*,*,#55579,.F.);
#81498=ORIENTED_EDGE('',*,*,#54887,.F.);
#81499=ORIENTED_EDGE('',*,*,#54884,.F.);
#81500=ORIENTED_EDGE('',*,*,#54881,.F.);
#81501=ORIENTED_EDGE('',*,*,#54878,.F.);
#81502=ORIENTED_EDGE('',*,*,#54875,.F.);
#81503=ORIENTED_EDGE('',*,*,#54872,.F.);
#81504=ORIENTED_EDGE('',*,*,#54869,.F.);
#81505=ORIENTED_EDGE('',*,*,#54866,.F.);
#81506=ORIENTED_EDGE('',*,*,#54863,.F.);
#81507=ORIENTED_EDGE('',*,*,#54860,.F.);
#81508=ORIENTED_EDGE('',*,*,#54857,.F.);
#81509=ORIENTED_EDGE('',*,*,#54854,.F.);
#81510=ORIENTED_EDGE('',*,*,#54851,.F.);
#81511=ORIENTED_EDGE('',*,*,#54848,.F.);
#81512=ORIENTED_EDGE('',*,*,#54845,.F.);
#81513=ORIENTED_EDGE('',*,*,#54842,.F.);
#81514=ORIENTED_EDGE('',*,*,#54772,.T.);
#81515=ORIENTED_EDGE('',*,*,#55544,.T.);
#81516=ORIENTED_EDGE('',*,*,#54769,.F.);
#81517=ORIENTED_EDGE('',*,*,#55549,.T.);
#81518=ORIENTED_EDGE('',*,*,#55539,.F.);
#81519=ORIENTED_EDGE('',*,*,#55545,.T.);
#81520=ORIENTED_EDGE('',*,*,#54713,.T.);
#81521=ORIENTED_EDGE('',*,*,#55520,.T.);
#81522=ORIENTED_EDGE('',*,*,#54710,.F.);
#81523=ORIENTED_EDGE('',*,*,#55525,.T.);
#81524=ORIENTED_EDGE('',*,*,#55600,.T.);
#81525=ORIENTED_EDGE('',*,*,#55521,.T.);
#81526=ORIENTED_EDGE('',*,*,#55480,.T.);
#81527=ORIENTED_EDGE('',*,*,#55325,.T.);
#81528=ORIENTED_EDGE('',*,*,#55299,.T.);
#81529=ORIENTED_EDGE('',*,*,#55287,.T.);
#81530=ORIENTED_EDGE('',*,*,#55336,.T.);
#81531=ORIENTED_EDGE('',*,*,#55254,.T.);
#81532=ORIENTED_EDGE('',*,*,#55496,.F.);
#81533=ORIENTED_EDGE('',*,*,#55389,.F.);
#81534=ORIENTED_EDGE('',*,*,#55401,.F.);
#81535=ORIENTED_EDGE('',*,*,#55394,.F.);
#81536=ORIENTED_EDGE('',*,*,#55400,.F.);
#81537=ORIENTED_EDGE('',*,*,#55399,.F.);
#81538=ORIENTED_EDGE('',*,*,#55479,.T.);
#81539=ORIENTED_EDGE('',*,*,#55475,.T.);
#81540=ORIENTED_EDGE('',*,*,#55485,.T.);
#81541=ORIENTED_EDGE('',*,*,#55470,.T.);
#81542=ORIENTED_EDGE('',*,*,#55486,.T.);
#81543=ORIENTED_EDGE('',*,*,#55465,.T.);
#81544=ORIENTED_EDGE('',*,*,#55487,.T.);
#81545=ORIENTED_EDGE('',*,*,#55452,.T.);
#81546=ORIENTED_EDGE('',*,*,#55484,.T.);
#81547=ORIENTED_EDGE('',*,*,#55447,.T.);
#81548=ORIENTED_EDGE('',*,*,#55488,.T.);
#81549=ORIENTED_EDGE('',*,*,#55442,.T.);
#81550=ORIENTED_EDGE('',*,*,#55489,.T.);
#81551=ORIENTED_EDGE('',*,*,#55437,.T.);
#81552=ORIENTED_EDGE('',*,*,#55490,.T.);
#81553=ORIENTED_EDGE('',*,*,#55424,.T.);
#81554=ORIENTED_EDGE('',*,*,#55483,.T.);
#81555=ORIENTED_EDGE('',*,*,#55352,.F.);
#81556=ORIENTED_EDGE('',*,*,#55404,.F.);
#81557=ORIENTED_EDGE('',*,*,#55365,.F.);
#81558=ORIENTED_EDGE('',*,*,#55403,.F.);
#81559=ORIENTED_EDGE('',*,*,#55370,.F.);
#81560=ORIENTED_EDGE('',*,*,#55402,.F.);
#81561=ORIENTED_EDGE('',*,*,#55375,.F.);
#81562=ORIENTED_EDGE('',*,*,#55495,.F.);
#81563=ORIENTED_EDGE('',*,*,#55313,.T.);
#81564=ORIENTED_EDGE('',*,*,#55601,.F.);
#81565=ORIENTED_EDGE('',*,*,#55565,.F.);
#81566=ORIENTED_EDGE('',*,*,#55590,.T.);
#81567=ORIENTED_EDGE('',*,*,#55602,.T.);
#81568=ORIENTED_EDGE('',*,*,#55513,.T.);
#81569=ORIENTED_EDGE('',*,*,#55603,.T.);
#81570=ORIENTED_EDGE('',*,*,#55604,.F.);
#81571=ORIENTED_EDGE('',*,*,#55536,.F.);
#81572=ORIENTED_EDGE('',*,*,#55482,.T.);
#81573=ORIENTED_EDGE('',*,*,#55331,.T.);
#81574=ORIENTED_EDGE('',*,*,#55481,.T.);
#81575=ORIENTED_EDGE('',*,*,#55318,.T.);
#81576=ORIENTED_EDGE('',*,*,#55602,.F.);
#81577=ORIENTED_EDGE('',*,*,#55589,.T.);
#81578=ORIENTED_EDGE('',*,*,#55605,.F.);
#81579=ORIENTED_EDGE('',*,*,#54890,.F.);
#81580=ORIENTED_EDGE('',*,*,#55582,.F.);
#81581=ORIENTED_EDGE('',*,*,#55591,.F.);
#81582=ORIENTED_EDGE('',*,*,#55605,.T.);
#81583=ORIENTED_EDGE('',*,*,#55584,.T.);
#81584=ORIENTED_EDGE('',*,*,#55598,.T.);
#81585=ORIENTED_EDGE('',*,*,#55592,.T.);
#81586=ORIENTED_EDGE('',*,*,#55581,.T.);
#81587=ORIENTED_EDGE('',*,*,#55599,.T.);
#81588=ORIENTED_EDGE('',*,*,#54778,.T.);
#81589=ORIENTED_EDGE('',*,*,#55597,.T.);
#81590=ORIENTED_EDGE('',*,*,#55601,.T.);
#81591=ORIENTED_EDGE('',*,*,#55564,.T.);
#81592=ORIENTED_EDGE('',*,*,#55606,.F.);
#81593=ORIENTED_EDGE('',*,*,#55550,.T.);
#81594=ORIENTED_EDGE('',*,*,#55248,.T.);
#81595=ORIENTED_EDGE('',*,*,#55552,.T.);
#81596=ORIENTED_EDGE('',*,*,#55607,.F.);
#81597=ORIENTED_EDGE('',*,*,#55566,.F.);
#81598=ORIENTED_EDGE('',*,*,#55567,.T.);
#81599=ORIENTED_EDGE('',*,*,#55608,.T.);
#81600=ORIENTED_EDGE('',*,*,#55572,.T.);
#81601=ORIENTED_EDGE('',*,*,#55606,.T.);
#81602=ORIENTED_EDGE('',*,*,#55561,.T.);
#81603=ORIENTED_EDGE('',*,*,#55573,.T.);
#81604=ORIENTED_EDGE('',*,*,#55608,.F.);
#81605=ORIENTED_EDGE('',*,*,#55607,.T.);
#81606=ORIENTED_EDGE('',*,*,#55570,.T.);
#81607=ORIENTED_EDGE('',*,*,#55604,.T.);
#81608=ORIENTED_EDGE('',*,*,#55535,.T.);
#81609=ORIENTED_EDGE('',*,*,#55609,.F.);
#81610=ORIENTED_EDGE('',*,*,#55526,.T.);
#81611=ORIENTED_EDGE('',*,*,#55610,.F.);
#81612=ORIENTED_EDGE('',*,*,#55537,.F.);
#81613=ORIENTED_EDGE('',*,*,#55538,.T.);
#81614=ORIENTED_EDGE('',*,*,#55611,.T.);
#81615=ORIENTED_EDGE('',*,*,#55546,.T.);
#81616=ORIENTED_EDGE('',*,*,#55609,.T.);
#81617=ORIENTED_EDGE('',*,*,#55532,.T.);
#81618=ORIENTED_EDGE('',*,*,#55547,.T.);
#81619=ORIENTED_EDGE('',*,*,#55611,.F.);
#81620=ORIENTED_EDGE('',*,*,#55610,.T.);
#81621=ORIENTED_EDGE('',*,*,#55542,.T.);
#81622=ORIENTED_EDGE('',*,*,#55603,.F.);
#81623=ORIENTED_EDGE('',*,*,#55512,.T.);
#81624=ORIENTED_EDGE('',*,*,#55612,.F.);
#81625=ORIENTED_EDGE('',*,*,#55600,.F.);
#81626=ORIENTED_EDGE('',*,*,#55505,.F.);
#81627=ORIENTED_EDGE('',*,*,#55514,.F.);
#81628=ORIENTED_EDGE('',*,*,#55612,.T.);
#81629=ORIENTED_EDGE('',*,*,#55507,.T.);
#81630=ORIENTED_EDGE('',*,*,#55522,.T.);
#81631=ORIENTED_EDGE('',*,*,#55515,.T.);
#81632=ORIENTED_EDGE('',*,*,#55504,.T.);
#81633=ORIENTED_EDGE('',*,*,#55524,.T.);
#81634=ORIENTED_EDGE('',*,*,#55074,.T.);
#81635=ORIENTED_EDGE('',*,*,#55518,.T.);
#81636=ORIENTED_EDGE('',*,*,#55162,.F.);
#81637=ORIENTED_EDGE('',*,*,#55159,.T.);
#81638=ORIENTED_EDGE('',*,*,#55136,.T.);
#81639=ORIENTED_EDGE('',*,*,#55157,.F.);
#81640=ORIENTED_EDGE('',*,*,#55613,.T.);
#81641=ORIENTED_EDGE('',*,*,#55614,.T.);
#81642=ORIENTED_EDGE('',*,*,#55143,.T.);
#81643=ORIENTED_EDGE('',*,*,#55138,.T.);
#81644=ORIENTED_EDGE('',*,*,#55158,.T.);
#81645=ORIENTED_EDGE('',*,*,#55161,.T.);
#81646=ORIENTED_EDGE('',*,*,#55155,.T.);
#81647=ORIENTED_EDGE('',*,*,#55134,.T.);
#81648=ORIENTED_EDGE('',*,*,#55141,.F.);
#81649=ORIENTED_EDGE('',*,*,#55146,.F.);
#81650=ORIENTED_EDGE('',*,*,#55615,.F.);
#81651=ORIENTED_EDGE('',*,*,#55163,.F.);
#81652=ORIENTED_EDGE('',*,*,#55615,.T.);
#81653=ORIENTED_EDGE('',*,*,#55145,.F.);
#81654=ORIENTED_EDGE('',*,*,#55616,.F.);
#81655=ORIENTED_EDGE('',*,*,#55206,.F.);
#81656=ORIENTED_EDGE('',*,*,#55616,.T.);
#81657=ORIENTED_EDGE('',*,*,#55150,.F.);
#81658=ORIENTED_EDGE('',*,*,#55617,.F.);
#81659=ORIENTED_EDGE('',*,*,#55208,.F.);
#81660=ORIENTED_EDGE('',*,*,#55144,.F.);
#81661=ORIENTED_EDGE('',*,*,#55614,.F.);
#81662=ORIENTED_EDGE('',*,*,#55618,.F.);
#81663=ORIENTED_EDGE('',*,*,#55147,.F.);
#81664=ORIENTED_EDGE('',*,*,#55619,.F.);
#81665=ORIENTED_EDGE('',*,*,#55148,.F.);
#81666=ORIENTED_EDGE('',*,*,#55620,.F.);
#81667=ORIENTED_EDGE('',*,*,#55154,.F.);
#81668=ORIENTED_EDGE('',*,*,#55617,.T.);
#81669=ORIENTED_EDGE('',*,*,#55149,.F.);
#81670=ORIENTED_EDGE('',*,*,#55621,.F.);
#81671=ORIENTED_EDGE('',*,*,#55165,.F.);
#81672=ORIENTED_EDGE('',*,*,#55620,.T.);
#81673=ORIENTED_EDGE('',*,*,#55618,.T.);
#81674=ORIENTED_EDGE('',*,*,#55622,.F.);
#81675=ORIENTED_EDGE('',*,*,#55621,.T.);
#81676=ORIENTED_EDGE('',*,*,#55619,.T.);
#81677=ORIENTED_EDGE('',*,*,#55623,.F.);
#81678=ORIENTED_EDGE('',*,*,#55622,.T.);
#81679=ORIENTED_EDGE('',*,*,#55613,.F.);
#81680=ORIENTED_EDGE('',*,*,#55624,.F.);
#81681=ORIENTED_EDGE('',*,*,#55151,.F.);
#81682=ORIENTED_EDGE('',*,*,#55623,.T.);
#81683=ORIENTED_EDGE('',*,*,#55153,.F.);
#81684=ORIENTED_EDGE('',*,*,#55625,.F.);
#81685=ORIENTED_EDGE('',*,*,#55168,.F.);
#81686=ORIENTED_EDGE('',*,*,#55201,.F.);
#81687=ORIENTED_EDGE('',*,*,#55199,.F.);
#81688=ORIENTED_EDGE('',*,*,#55166,.F.);
#81689=ORIENTED_EDGE('',*,*,#55624,.T.);
#81690=ORIENTED_EDGE('',*,*,#55133,.F.);
#81691=ORIENTED_EDGE('',*,*,#55625,.T.);
#81692=ORIENTED_EDGE('',*,*,#55152,.F.);
#85787=CYLINDRICAL_SURFACE('',#94087,2.);
#85788=CYLINDRICAL_SURFACE('',#94091,2.5);
#85789=CYLINDRICAL_SURFACE('',#94098,2.);
#85790=CYLINDRICAL_SURFACE('',#94102,2.5);
#85791=CYLINDRICAL_SURFACE('',#94105,5.);
#85792=CYLINDRICAL_SURFACE('',#94108,3.);
#85793=CYLINDRICAL_SURFACE('',#94116,3.);
#85794=CYLINDRICAL_SURFACE('',#94124,3.);
#85795=CYLINDRICAL_SURFACE('',#94136,0.5);
#85796=CYLINDRICAL_SURFACE('',#94143,0.5);
#85797=CYLINDRICAL_SURFACE('',#94153,0.5);
#85798=CYLINDRICAL_SURFACE('',#94160,0.5);
#85799=CYLINDRICAL_SURFACE('',#94170,0.5);
#85800=CYLINDRICAL_SURFACE('',#94177,0.5);
#85801=CYLINDRICAL_SURFACE('',#94184,5.);
#85802=CYLINDRICAL_SURFACE('',#94190,0.5);
#85803=CYLINDRICAL_SURFACE('',#94199,0.5);
#85804=CYLINDRICAL_SURFACE('',#94206,0.5);
#85805=CYLINDRICAL_SURFACE('',#94214,0.5);
#85806=CYLINDRICAL_SURFACE('',#94221,0.5);
#85807=CYLINDRICAL_SURFACE('',#94229,0.5);
#85808=CYLINDRICAL_SURFACE('',#94237,5.);
#85809=CYLINDRICAL_SURFACE('',#94241,58.3875000000282);
#85810=CYLINDRICAL_SURFACE('',#94260,3.);
#85811=CYLINDRICAL_SURFACE('',#94269,3.);
#85812=CYLINDRICAL_SURFACE('',#94279,0.5);
#85813=CYLINDRICAL_SURFACE('',#94285,0.5);
#85814=CYLINDRICAL_SURFACE('',#94293,0.5);
#85815=CYLINDRICAL_SURFACE('',#94299,0.5);
#85816=CYLINDRICAL_SURFACE('',#94306,0.5);
#85817=CYLINDRICAL_SURFACE('',#94312,0.5);
#85818=CYLINDRICAL_SURFACE('',#94319,0.5);
#85819=CYLINDRICAL_SURFACE('',#94325,0.5);
#85820=CYLINDRICAL_SURFACE('',#94332,0.5);
#85821=CYLINDRICAL_SURFACE('',#94338,0.5);
#85822=CYLINDRICAL_SURFACE('',#94346,0.5);
#85823=CYLINDRICAL_SURFACE('',#94352,0.5);
#85824=CYLINDRICAL_SURFACE('',#94355,0.999999999999996);
#85825=CYLINDRICAL_SURFACE('',#94356,0.5);
#85826=CYLINDRICAL_SURFACE('',#94360,0.500000000000005);
#85827=CYLINDRICAL_SURFACE('',#94363,0.5);
#85828=CYLINDRICAL_SURFACE('',#94365,0.999999999999996);
#85829=CYLINDRICAL_SURFACE('',#94367,0.5);
#85830=CYLINDRICAL_SURFACE('',#94370,0.999999999999996);
#85831=CYLINDRICAL_SURFACE('',#94371,0.5);
#85832=CYLINDRICAL_SURFACE('',#94375,0.500000000000005);
#85833=CYLINDRICAL_SURFACE('',#94378,0.5);
#85834=CYLINDRICAL_SURFACE('',#94380,0.999999999999996);
#85835=CYLINDRICAL_SURFACE('',#94382,0.999999999999997);
#85836=CYLINDRICAL_SURFACE('',#94383,0.5);
#85837=CYLINDRICAL_SURFACE('',#94387,0.499999999999999);
#85838=CYLINDRICAL_SURFACE('',#94390,0.5);
#85839=CYLINDRICAL_SURFACE('',#94392,0.999999999999997);
#85840=CYLINDRICAL_SURFACE('',#94393,0.5);
#85841=CYLINDRICAL_SURFACE('',#94397,0.499999999999999);
#85842=CYLINDRICAL_SURFACE('',#94400,0.5);
#85843=CYLINDRICAL_SURFACE('',#94402,0.999999999999996);
#85844=CYLINDRICAL_SURFACE('',#94403,0.999999999999997);
#85845=CYLINDRICAL_SURFACE('',#94404,0.5);
#85846=CYLINDRICAL_SURFACE('',#94408,0.499999999999999);
#85847=CYLINDRICAL_SURFACE('',#94411,0.5);
#85848=CYLINDRICAL_SURFACE('',#94413,0.999999999999997);
#85849=CYLINDRICAL_SURFACE('',#94416,0.5);
#85850=CYLINDRICAL_SURFACE('',#94420,0.999999999999997);
#85851=CYLINDRICAL_SURFACE('',#94421,0.5);
#85852=CYLINDRICAL_SURFACE('',#94425,0.499999999999999);
#85853=CYLINDRICAL_SURFACE('',#94428,0.5);
#85854=CYLINDRICAL_SURFACE('',#94431,0.5);
#85855=CYLINDRICAL_SURFACE('',#94435,1.);
#85856=CYLINDRICAL_SURFACE('',#94436,0.5);
#85857=CYLINDRICAL_SURFACE('',#94440,0.499999999999998);
#85858=CYLINDRICAL_SURFACE('',#94443,0.5);
#85859=CYLINDRICAL_SURFACE('',#94445,1.);
#85860=CYLINDRICAL_SURFACE('',#94446,0.5);
#85861=CYLINDRICAL_SURFACE('',#94450,0.499999999999998);
#85862=CYLINDRICAL_SURFACE('',#94454,0.5);
#85863=CYLINDRICAL_SURFACE('',#94457,1.);
#85864=CYLINDRICAL_SURFACE('',#94467,0.5);
#85865=CYLINDRICAL_SURFACE('',#94479,0.5);
#85866=CYLINDRICAL_SURFACE('',#94481,3.);
#85867=CYLINDRICAL_SURFACE('',#94484,0.5);
#85868=CYLINDRICAL_SURFACE('',#94490,0.5);
#85869=CYLINDRICAL_SURFACE('',#94496,0.5);
#85870=CYLINDRICAL_SURFACE('',#94503,0.5);
#85871=CYLINDRICAL_SURFACE('',#94510,0.5);
#85872=CYLINDRICAL_SURFACE('',#94516,0.5);
#85873=CYLINDRICAL_SURFACE('',#94523,1.);
#85874=CYLINDRICAL_SURFACE('',#94525,0.5);
#85875=CYLINDRICAL_SURFACE('',#94532,0.5);
#85876=CYLINDRICAL_SURFACE('',#94538,0.5);
#85877=CYLINDRICAL_SURFACE('',#94540,1.);
#85878=CYLINDRICAL_SURFACE('',#94543,0.5);
#85879=CYLINDRICAL_SURFACE('',#94550,0.5);
#85880=CYLINDRICAL_SURFACE('',#94556,0.5);
#85881=CYLINDRICAL_SURFACE('',#94558,1.);
#85882=CYLINDRICAL_SURFACE('',#94561,0.5);
#85883=CYLINDRICAL_SURFACE('',#94564,3.);
#85884=CYLINDRICAL_SURFACE('',#94571,0.499999999999999);
#85885=CYLINDRICAL_SURFACE('',#94573,5.);
#85886=CYLINDRICAL_SURFACE('',#94579,0.250000000000003);
#85887=CYLINDRICAL_SURFACE('',#94593,0.249999999999997);
#85888=CYLINDRICAL_SURFACE('',#94607,0.250000000000003);
#85889=CYLINDRICAL_SURFACE('',#94621,0.250000000000003);
#85890=CYLINDRICAL_SURFACE('',#94627,2.75);
#85891=CYLINDRICAL_SURFACE('',#94632,2.75);
#85892=CYLINDRICAL_SURFACE('',#94638,0.5);
#85893=CYLINDRICAL_SURFACE('',#94645,0.5);
#85894=CYLINDRICAL_SURFACE('',#94654,0.5);
#85895=CYLINDRICAL_SURFACE('',#94661,0.5);
#85896=CYLINDRICAL_SURFACE('',#94669,0.5);
#85897=CYLINDRICAL_SURFACE('',#94676,0.5);
#85898=CYLINDRICAL_SURFACE('',#94680,3.);
#85899=CYLINDRICAL_SURFACE('',#94687,0.5);
#85900=CYLINDRICAL_SURFACE('',#94713,0.5);
#85901=CYLINDRICAL_SURFACE('',#94716,0.5);
#85902=CYLINDRICAL_SURFACE('',#94731,0.5);
#85903=CYLINDRICAL_SURFACE('',#94742,0.5);
#85904=CYLINDRICAL_SURFACE('',#94745,0.5);
#85905=CYLINDRICAL_SURFACE('',#94770,0.5);
#85906=CYLINDRICAL_SURFACE('',#94773,0.5);
#85907=CYLINDRICAL_SURFACE('',#94775,0.5);
#85908=CYLINDRICAL_SURFACE('',#94778,0.5);
#85909=CYLINDRICAL_SURFACE('',#94793,0.5);
#85910=CYLINDRICAL_SURFACE('',#94796,0.5);
#85911=CYLINDRICAL_SURFACE('',#94849,0.5);
#85912=CYLINDRICAL_SURFACE('',#94852,0.5);
#85913=CYLINDRICAL_SURFACE('',#94874,0.5);
#85914=CYLINDRICAL_SURFACE('',#94877,0.5);
#85915=CYLINDRICAL_SURFACE('',#94897,0.5);
#85916=CYLINDRICAL_SURFACE('',#94900,0.5);
#85917=CYLINDRICAL_SURFACE('',#94912,0.5);
#85918=CYLINDRICAL_SURFACE('',#94915,0.5);
#85919=CYLINDRICAL_SURFACE('',#94924,0.5);
#85920=CYLINDRICAL_SURFACE('',#94927,0.5);
#85921=CYLINDRICAL_SURFACE('',#94939,0.5);
#85922=CYLINDRICAL_SURFACE('',#94942,0.5);
#85923=CYLINDRICAL_SURFACE('',#94965,0.5);
#85924=CYLINDRICAL_SURFACE('',#94968,0.5);
#85925=CYLINDRICAL_SURFACE('',#94986,0.5);
#85926=CYLINDRICAL_SURFACE('',#94989,0.5);
#85927=CYLINDRICAL_SURFACE('',#95001,0.5);
#85928=CYLINDRICAL_SURFACE('',#95004,0.5);
#85929=CYLINDRICAL_SURFACE('',#95011,0.5);
#85930=CYLINDRICAL_SURFACE('',#95013,2.);
#85931=CYLINDRICAL_SURFACE('',#95018,2.75);
#85932=CYLINDRICAL_SURFACE('',#95019,0.5);
#85933=CYLINDRICAL_SURFACE('',#95029,0.5);
#85934=CYLINDRICAL_SURFACE('',#95030,0.5);
#85935=CYLINDRICAL_SURFACE('',#95032,2.);
#85936=CYLINDRICAL_SURFACE('',#95037,2.75);
#85937=CYLINDRICAL_SURFACE('',#95039,0.5);
#85938=CYLINDRICAL_SURFACE('',#95041,3.);
#85939=CYLINDRICAL_SURFACE('',#95046,0.5);
#85940=CYLINDRICAL_SURFACE('',#95054,0.5);
#85941=CYLINDRICAL_SURFACE('',#95057,0.5);
#85942=CYLINDRICAL_SURFACE('',#95059,0.5);
#85943=CYLINDRICAL_SURFACE('',#95062,0.5);
#85944=CYLINDRICAL_SURFACE('',#95064,0.5);
#85945=CYLINDRICAL_SURFACE('',#95071,0.5);
#85946=CYLINDRICAL_SURFACE('',#95074,0.5);
#85947=CYLINDRICAL_SURFACE('',#95079,0.5);
#85948=CYLINDRICAL_SURFACE('',#95082,0.5);
#85949=CYLINDRICAL_SURFACE('',#95087,0.5);
#85950=CYLINDRICAL_SURFACE('',#95089,0.5);
#85951=CYLINDRICAL_SURFACE('',#95093,0.5);
#85952=CYLINDRICAL_SURFACE('',#95096,0.5);
#85953=CYLINDRICAL_SURFACE('',#95099,3.);
#85954=CYLINDRICAL_SURFACE('',#95101,67.5);
#85955=CYLINDRICAL_SURFACE('',#95103,3.);
#85956=CYLINDRICAL_SURFACE('',#95106,5.);
#85957=CYLINDRICAL_SURFACE('',#95107,58.5);
#85958=CYLINDRICAL_SURFACE('',#95123,5.);
#85959=CYLINDRICAL_SURFACE('',#95125,3.);
#85960=CYLINDRICAL_SURFACE('',#95127,67.5);
#85961=CYLINDRICAL_SURFACE('',#95129,3.);
#85962=CYLINDRICAL_SURFACE('',#95149,0.5);
#85963=CYLINDRICAL_SURFACE('',#95154,0.5);
#85964=CYLINDRICAL_SURFACE('',#95157,0.5);
#85965=CYLINDRICAL_SURFACE('',#95167,0.5);
#85966=CYLINDRICAL_SURFACE('',#95171,0.5);
#85967=CYLINDRICAL_SURFACE('',#95178,0.5);
#85968=CYLINDRICAL_SURFACE('',#95183,0.5);
#85969=CYLINDRICAL_SURFACE('',#95186,0.5);
#85970=CYLINDRICAL_SURFACE('',#95188,0.5);
#85971=CYLINDRICAL_SURFACE('',#95192,0.5);
#85972=CYLINDRICAL_SURFACE('',#95196,0.5);
#85973=CYLINDRICAL_SURFACE('',#95202,0.5);
#85974=CYLINDRICAL_SURFACE('',#95206,3.);
#85975=CYLINDRICAL_SURFACE('',#95213,0.5);
#85976=CYLINDRICAL_SURFACE('',#95215,0.5);
#85977=CYLINDRICAL_SURFACE('',#95221,0.5);
#85978=CYLINDRICAL_SURFACE('',#95227,0.5);
#85979=CYLINDRICAL_SURFACE('',#95235,0.5);
#85980=CYLINDRICAL_SURFACE('',#95238,3.);
#85981=CYLINDRICAL_SURFACE('',#95241,0.5);
#85982=CYLINDRICAL_SURFACE('',#95248,3.);
#85983=CYLINDRICAL_SURFACE('',#95255,3.);
#85984=CYLINDRICAL_SURFACE('',#95259,0.5);
#85985=CYLINDRICAL_SURFACE('',#95261,0.5);
#85986=CYLINDRICAL_SURFACE('',#95268,0.5);
#85987=CYLINDRICAL_SURFACE('',#95271,0.5);
#85988=CYLINDRICAL_SURFACE('',#95277,0.5);
#85989=CYLINDRICAL_SURFACE('',#95283,0.5);
#85990=CYLINDRICAL_SURFACE('',#95285,0.5);
#85991=CYLINDRICAL_SURFACE('',#95290,0.5);
#85992=CYLINDRICAL_SURFACE('',#95294,3.);
#85993=CYLINDRICAL_SURFACE('',#95299,0.5);
#85994=CYLINDRICAL_SURFACE('',#95304,0.5);
#85995=CYLINDRICAL_SURFACE('',#95311,0.5);
#85996=CYLINDRICAL_SURFACE('',#95315,0.5);
#85997=CYLINDRICAL_SURFACE('',#95321,0.5);
#85998=CYLINDRICAL_SURFACE('',#95324,0.5);
#85999=CYLINDRICAL_SURFACE('',#95326,0.5);
#86000=CYLINDRICAL_SURFACE('',#95329,0.5);
#86001=CYLINDRICAL_SURFACE('',#95336,0.5);
#86002=CYLINDRICAL_SURFACE('',#95341,0.5);
#86003=CYLINDRICAL_SURFACE('',#95348,0.5);
#86004=CYLINDRICAL_SURFACE('',#95351,0.5);
#86005=CYLINDRICAL_SURFACE('',#95354,0.5);
#86006=CYLINDRICAL_SURFACE('',#95357,0.5);
#86007=CYLINDRICAL_SURFACE('',#95365,0.5);
#86008=CYLINDRICAL_SURFACE('',#95370,0.5);
#86009=CYLINDRICAL_SURFACE('',#95376,0.5);
#86010=CYLINDRICAL_SURFACE('',#95379,0.5);
#86011=CYLINDRICAL_SURFACE('',#95381,0.5);
#86012=CYLINDRICAL_SURFACE('',#95384,0.5);
#86013=CYLINDRICAL_SURFACE('',#95391,0.5);
#86014=CYLINDRICAL_SURFACE('',#95395,0.5);
#86015=CYLINDRICAL_SURFACE('',#95401,0.5);
#86016=CYLINDRICAL_SURFACE('',#95407,0.5);
#86017=CYLINDRICAL_SURFACE('',#95411,3.);
#86018=CYLINDRICAL_SURFACE('',#95416,0.5);
#86019=CYLINDRICAL_SURFACE('',#95421,0.5);
#86020=CYLINDRICAL_SURFACE('',#95422,0.5);
#86021=CYLINDRICAL_SURFACE('',#95429,0.5);
#86022=CYLINDRICAL_SURFACE('',#95435,0.5);
#86023=CYLINDRICAL_SURFACE('',#95437,0.5);
#86024=CYLINDRICAL_SURFACE('',#95442,0.5);
#86025=CYLINDRICAL_SURFACE('',#95444,0.5);
#86026=CYLINDRICAL_SURFACE('',#95448,0.5);
#86027=CYLINDRICAL_SURFACE('',#95450,0.5);
#86028=CYLINDRICAL_SURFACE('',#95457,0.5);
#86029=CYLINDRICAL_SURFACE('',#95459,0.5);
#86030=CYLINDRICAL_SURFACE('',#95464,0.5);
#86031=CYLINDRICAL_SURFACE('',#95470,0.5);
#86032=CYLINDRICAL_SURFACE('',#95476,0.5);
#86033=CYLINDRICAL_SURFACE('',#95477,3.);
#86034=CYLINDRICAL_SURFACE('',#95481,0.5);
#86035=CYLINDRICAL_SURFACE('',#95483,1.);
#86036=CYLINDRICAL_SURFACE('',#95486,0.5);
#86037=CYLINDRICAL_SURFACE('',#95489,0.5);
#86038=CYLINDRICAL_SURFACE('',#95494,0.5);
#86039=CYLINDRICAL_SURFACE('',#95495,0.5);
#86040=CYLINDRICAL_SURFACE('',#95499,0.5);
#86041=CYLINDRICAL_SURFACE('',#95506,0.5);
#86042=CYLINDRICAL_SURFACE('',#95509,0.5);
#86043=CYLINDRICAL_SURFACE('',#95516,0.5);
#86044=CYLINDRICAL_SURFACE('',#95519,0.5);
#86045=CYLINDRICAL_SURFACE('',#95524,0.5);
#86046=CYLINDRICAL_SURFACE('',#95527,0.5);
#86047=CYLINDRICAL_SURFACE('',#95529,0.5);
#86048=CYLINDRICAL_SURFACE('',#95534,0.5);
#86049=CYLINDRICAL_SURFACE('',#95538,3.);
#86050=CYLINDRICAL_SURFACE('',#95542,0.5);
#86051=CYLINDRICAL_SURFACE('',#95544,0.5);
#86052=CYLINDRICAL_SURFACE('',#95548,0.5);
#86053=CYLINDRICAL_SURFACE('',#95553,0.5);
#86054=CYLINDRICAL_SURFACE('',#95557,0.5);
#86055=CYLINDRICAL_SURFACE('',#95563,0.5);
#86056=CYLINDRICAL_SURFACE('',#95565,0.5);
#86057=CYLINDRICAL_SURFACE('',#95570,0.5);
#86058=CYLINDRICAL_SURFACE('',#95573,3.);
#86059=CYLINDRICAL_SURFACE('',#95576,0.5);
#86060=CYLINDRICAL_SURFACE('',#95579,1.);
#86061=CYLINDRICAL_SURFACE('',#95580,0.5);
#86062=CYLINDRICAL_SURFACE('',#95584,3.);
#86063=CYLINDRICAL_SURFACE('',#95587,0.5);
#86064=CYLINDRICAL_SURFACE('',#95593,0.5);
#86065=CYLINDRICAL_SURFACE('',#95595,0.5);
#86066=CYLINDRICAL_SURFACE('',#95600,0.5);
#86067=CYLINDRICAL_SURFACE('',#95602,0.5);
#86068=CYLINDRICAL_SURFACE('',#95607,0.5);
#86069=CYLINDRICAL_SURFACE('',#95614,0.5);
#86070=CYLINDRICAL_SURFACE('',#95619,0.5);
#86071=CYLINDRICAL_SURFACE('',#95620,3.);
#86072=CYLINDRICAL_SURFACE('',#95624,1.);
#86073=CYLINDRICAL_SURFACE('',#95625,0.5);
#86074=CYLINDRICAL_SURFACE('',#95630,0.5);
#86075=CYLINDRICAL_SURFACE('',#95631,0.5);
#86076=CYLINDRICAL_SURFACE('',#95635,0.5);
#86077=CYLINDRICAL_SURFACE('',#95636,0.5);
#86078=CYLINDRICAL_SURFACE('',#95638,0.5);
#86079=CYLINDRICAL_SURFACE('',#95640,0.5);
#86080=CYLINDRICAL_SURFACE('',#95648,0.5);
#86081=CYLINDRICAL_SURFACE('',#95653,0.5);
#86082=CYLINDRICAL_SURFACE('',#95660,0.5);
#86083=CYLINDRICAL_SURFACE('',#95663,0.5);
#86084=CYLINDRICAL_SURFACE('',#95668,0.5);
#86085=CYLINDRICAL_SURFACE('',#95671,0.5);
#86086=CYLINDRICAL_SURFACE('',#95673,0.5);
#86087=CYLINDRICAL_SURFACE('',#95678,0.5);
#86088=CYLINDRICAL_SURFACE('',#95682,3.);
#86089=CYLINDRICAL_SURFACE('',#95686,0.5);
#86090=CYLINDRICAL_SURFACE('',#95688,0.5);
#86091=CYLINDRICAL_SURFACE('',#95692,0.5);
#86092=CYLINDRICAL_SURFACE('',#95697,0.5);
#86093=CYLINDRICAL_SURFACE('',#95701,0.5);
#86094=CYLINDRICAL_SURFACE('',#95711,0.5);
#86095=CYLINDRICAL_SURFACE('',#95713,0.5);
#86096=CYLINDRICAL_SURFACE('',#95719,0.5);
#86097=CYLINDRICAL_SURFACE('',#95722,0.5);
#86098=CYLINDRICAL_SURFACE('',#95729,0.5);
#86099=CYLINDRICAL_SURFACE('',#95731,0.5);
#86100=CYLINDRICAL_SURFACE('',#95736,0.5);
#86101=CYLINDRICAL_SURFACE('',#95741,0.5);
#86102=CYLINDRICAL_SURFACE('',#95743,0.5);
#86103=CYLINDRICAL_SURFACE('',#95745,0.5);
#86104=CYLINDRICAL_SURFACE('',#95746,3.);
#86105=CYLINDRICAL_SURFACE('',#95750,0.5);
#86106=CYLINDRICAL_SURFACE('',#95752,0.5);
#86107=CYLINDRICAL_SURFACE('',#95757,0.5);
#86108=CYLINDRICAL_SURFACE('',#95762,0.5);
#86109=CYLINDRICAL_SURFACE('',#95767,0.5);
#86110=CYLINDRICAL_SURFACE('',#95768,0.5);
#86111=CYLINDRICAL_SURFACE('',#95774,0.5);
#86112=CYLINDRICAL_SURFACE('',#95779,0.5);
#86113=CYLINDRICAL_SURFACE('',#95784,0.5);
#86114=CYLINDRICAL_SURFACE('',#95787,0.5);
#86115=CYLINDRICAL_SURFACE('',#95789,0.5);
#86116=CYLINDRICAL_SURFACE('',#95794,0.5);
#86117=CYLINDRICAL_SURFACE('',#95798,3.);
#86118=CYLINDRICAL_SURFACE('',#95802,0.5);
#86119=CYLINDRICAL_SURFACE('',#95803,0.5);
#86120=CYLINDRICAL_SURFACE('',#95805,0.5);
#86121=CYLINDRICAL_SURFACE('',#95810,0.5);
#86122=CYLINDRICAL_SURFACE('',#95815,0.5);
#86123=CYLINDRICAL_SURFACE('',#95818,0.5);
#86124=CYLINDRICAL_SURFACE('',#95824,58.5);
#86125=CYLINDRICAL_SURFACE('',#95827,0.999999999999999);
#86126=CYLINDRICAL_SURFACE('',#95835,1.);
#86127=CYLINDRICAL_SURFACE('',#95837,0.5);
#86128=CYLINDRICAL_SURFACE('',#95839,1.);
#86129=CYLINDRICAL_SURFACE('',#95841,0.5);
#86130=CYLINDRICAL_SURFACE('',#95843,1.);
#86131=CYLINDRICAL_SURFACE('',#95888,1.);
#86132=CYLINDRICAL_SURFACE('',#95890,0.5);
#86133=CYLINDRICAL_SURFACE('',#95892,1.);
#86134=CYLINDRICAL_SURFACE('',#95895,1.);
#86135=CYLINDRICAL_SURFACE('',#95897,0.5);
#86136=CYLINDRICAL_SURFACE('',#95905,0.999999999999999);
#86137=CYLINDRICAL_SURFACE('',#95907,0.500000000000006);
#86138=CYLINDRICAL_SURFACE('',#95909,0.999999999999999);
#86139=CYLINDRICAL_SURFACE('',#95911,0.500000000000006);
#86140=CYLINDRICAL_SURFACE('',#95913,0.999999999999999);
#86141=CYLINDRICAL_SURFACE('',#95915,3.);
#86142=CYLINDRICAL_SURFACE('',#95919,3.);
#86143=CYLINDRICAL_SURFACE('',#95929,3.);
#86144=CYLINDRICAL_SURFACE('',#95931,3.);
#86145=CYLINDRICAL_SURFACE('',#95933,0.5);
#86146=CYLINDRICAL_SURFACE('',#95942,0.5);
#86147=CYLINDRICAL_SURFACE('',#95943,3.);
#86148=CYLINDRICAL_SURFACE('',#95949,3.);
#86149=CYLINDRICAL_SURFACE('',#95952,3.);
#86150=CYLINDRICAL_SURFACE('',#95965,3.);
#86151=CYLINDRICAL_SURFACE('',#95971,3.);
#86152=CYLINDRICAL_SURFACE('',#95986,3.);
#86153=CYLINDRICAL_SURFACE('',#95994,3.);
#86154=CYLINDRICAL_SURFACE('',#96004,3.);
#86155=CYLINDRICAL_SURFACE('',#96010,3.);
#86156=CYLINDRICAL_SURFACE('',#96023,3.);
#86157=CYLINDRICAL_SURFACE('',#96033,3.);
#86158=CYLINDRICAL_SURFACE('',#96051,3.);
#86159=CYLINDRICAL_SURFACE('',#96062,3.);
#86160=CYLINDRICAL_SURFACE('',#96083,3.);
#86161=CYLINDRICAL_SURFACE('',#96089,3.);
#86162=CYLINDRICAL_SURFACE('',#96100,3.);
#86163=CYLINDRICAL_SURFACE('',#96103,0.5);
#86164=CYLINDRICAL_SURFACE('',#96123,0.5);
#86165=CYLINDRICAL_SURFACE('',#96126,3.);
#86166=CYLINDRICAL_SURFACE('',#96131,3.);
#86167=CYLINDRICAL_SURFACE('',#96145,3.);
#86168=CYLINDRICAL_SURFACE('',#96151,3.);
#86169=CYLINDRICAL_SURFACE('',#96160,0.999999999999999);
#86170=CYLINDRICAL_SURFACE('',#96163,0.500000000000006);
#86171=CYLINDRICAL_SURFACE('',#96166,0.999999999999999);
#86172=CYLINDRICAL_SURFACE('',#96169,0.500000000000006);
#86173=CYLINDRICAL_SURFACE('',#96172,0.999999999999999);
#86174=CYLINDRICAL_SURFACE('',#96188,0.5);
#86175=CYLINDRICAL_SURFACE('',#96191,1.);
#86176=CYLINDRICAL_SURFACE('',#96194,1.);
#86177=CYLINDRICAL_SURFACE('',#96197,0.5);
#86178=CYLINDRICAL_SURFACE('',#96200,1.);
#86179=CYLINDRICAL_SURFACE('',#96273,1.);
#86180=CYLINDRICAL_SURFACE('',#96276,0.5);
#86181=CYLINDRICAL_SURFACE('',#96279,1.);
#86182=CYLINDRICAL_SURFACE('',#96282,0.5);
#86183=CYLINDRICAL_SURFACE('',#96285,1.);
#86184=CYLINDRICAL_SURFACE('',#96299,0.999999999999999);
#86185=CYLINDRICAL_SURFACE('',#96305,58.5);
#86186=CYLINDRICAL_SURFACE('',#96313,0.5);
#86187=CYLINDRICAL_SURFACE('',#96318,0.5);
#86188=CYLINDRICAL_SURFACE('',#96323,0.5);
#86189=CYLINDRICAL_SURFACE('',#96327,0.5);
#86190=CYLINDRICAL_SURFACE('',#96328,0.5);
#86191=CYLINDRICAL_SURFACE('',#96329,0.5);
#86192=CYLINDRICAL_SURFACE('',#96336,3.);
#86193=CYLINDRICAL_SURFACE('',#96342,0.5);
#86194=CYLINDRICAL_SURFACE('',#96347,0.5);
#86195=CYLINDRICAL_SURFACE('',#96348,0.5);
#86196=CYLINDRICAL_SURFACE('',#96351,0.5);
#86197=CYLINDRICAL_SURFACE('',#96356,0.5);
#86198=CYLINDRICAL_SURFACE('',#96361,0.5);
#86199=CYLINDRICAL_SURFACE('',#96369,0.5);
#86200=CYLINDRICAL_SURFACE('',#96371,0.5);
#86201=CYLINDRICAL_SURFACE('',#96377,0.5);
#86202=CYLINDRICAL_SURFACE('',#96382,0.5);
#86203=CYLINDRICAL_SURFACE('',#96386,0.5);
#86204=CYLINDRICAL_SURFACE('',#96387,0.5);
#86205=CYLINDRICAL_SURFACE('',#96392,3.);
#86206=CYLINDRICAL_SURFACE('',#96394,0.5);
#86207=CYLINDRICAL_SURFACE('',#96397,0.5);
#86208=CYLINDRICAL_SURFACE('',#96399,0.5);
#86209=CYLINDRICAL_SURFACE('',#96406,0.5);
#86210=CYLINDRICAL_SURFACE('',#96411,0.5);
#86211=CYLINDRICAL_SURFACE('',#96412,0.5);
#86212=CYLINDRICAL_SURFACE('',#96418,0.5);
#86213=CYLINDRICAL_SURFACE('',#96422,0.5);
#86214=CYLINDRICAL_SURFACE('',#96428,0.5);
#86215=CYLINDRICAL_SURFACE('',#96429,0.5);
#86216=CYLINDRICAL_SURFACE('',#96440,0.5);
#86217=CYLINDRICAL_SURFACE('',#96446,0.5);
#86218=CYLINDRICAL_SURFACE('',#96451,0.5);
#86219=CYLINDRICAL_SURFACE('',#96454,0.5);
#86220=CYLINDRICAL_SURFACE('',#96455,0.5);
#86221=CYLINDRICAL_SURFACE('',#96460,3.);
#86222=CYLINDRICAL_SURFACE('',#96466,0.5);
#86223=CYLINDRICAL_SURFACE('',#96471,0.5);
#86224=CYLINDRICAL_SURFACE('',#96472,0.5);
#86225=CYLINDRICAL_SURFACE('',#96475,0.5);
#86226=CYLINDRICAL_SURFACE('',#96480,0.5);
#86227=CYLINDRICAL_SURFACE('',#96484,0.5);
#86228=CYLINDRICAL_SURFACE('',#96493,0.5);
#86229=CYLINDRICAL_SURFACE('',#96503,0.5);
#86230=CYLINDRICAL_SURFACE('',#96509,0.5);
#86231=CYLINDRICAL_SURFACE('',#96510,0.5);
#86232=CYLINDRICAL_SURFACE('',#96511,0.5);
#86233=CYLINDRICAL_SURFACE('',#96513,0.5);
#86234=CYLINDRICAL_SURFACE('',#96517,0.5);
#86235=CYLINDRICAL_SURFACE('',#96518,0.5);
#86236=CYLINDRICAL_SURFACE('',#96523,0.5);
#86237=CYLINDRICAL_SURFACE('',#96527,1.);
#86238=CYLINDRICAL_SURFACE('',#96533,3.);
#86239=CYLINDRICAL_SURFACE('',#96535,0.5);
#86240=CYLINDRICAL_SURFACE('',#96541,0.5);
#86241=CYLINDRICAL_SURFACE('',#96550,0.5);
#86242=CYLINDRICAL_SURFACE('',#96555,0.5);
#86243=CYLINDRICAL_SURFACE('',#96556,0.5);
#86244=CYLINDRICAL_SURFACE('',#96559,0.5);
#86245=CYLINDRICAL_SURFACE('',#96561,0.5);
#86246=CYLINDRICAL_SURFACE('',#96569,0.5);
#86247=CYLINDRICAL_SURFACE('',#96576,3.);
#86248=CYLINDRICAL_SURFACE('',#96582,0.5);
#86249=CYLINDRICAL_SURFACE('',#96583,1.);
#86250=CYLINDRICAL_SURFACE('',#96588,0.5);
#86251=CYLINDRICAL_SURFACE('',#96595,3.);
#86252=CYLINDRICAL_SURFACE('',#96601,0.5);
#86253=CYLINDRICAL_SURFACE('',#96607,0.5);
#86254=CYLINDRICAL_SURFACE('',#96609,0.5);
#86255=CYLINDRICAL_SURFACE('',#96617,0.5);
#86256=CYLINDRICAL_SURFACE('',#96623,0.5);
#86257=CYLINDRICAL_SURFACE('',#96628,0.5);
#86258=CYLINDRICAL_SURFACE('',#96631,0.5);
#86259=CYLINDRICAL_SURFACE('',#96632,0.5);
#86260=CYLINDRICAL_SURFACE('',#96637,3.);
#86261=CYLINDRICAL_SURFACE('',#96643,0.5);
#86262=CYLINDRICAL_SURFACE('',#96648,0.5);
#86263=CYLINDRICAL_SURFACE('',#96649,0.5);
#86264=CYLINDRICAL_SURFACE('',#96652,0.5);
#86265=CYLINDRICAL_SURFACE('',#96657,0.5);
#86266=CYLINDRICAL_SURFACE('',#96661,0.5);
#86267=CYLINDRICAL_SURFACE('',#96670,0.5);
#86268=CYLINDRICAL_SURFACE('',#96675,0.5);
#86269=CYLINDRICAL_SURFACE('',#96683,0.5);
#86270=CYLINDRICAL_SURFACE('',#96687,0.5);
#86271=CYLINDRICAL_SURFACE('',#96688,0.5);
#86272=CYLINDRICAL_SURFACE('',#96693,0.5);
#86273=CYLINDRICAL_SURFACE('',#96697,0.5);
#86274=CYLINDRICAL_SURFACE('',#96698,1.);
#86275=CYLINDRICAL_SURFACE('',#96699,0.5);
#86276=CYLINDRICAL_SURFACE('',#96705,3.);
#86277=CYLINDRICAL_SURFACE('',#96707,0.5);
#86278=CYLINDRICAL_SURFACE('',#96713,0.5);
#86279=CYLINDRICAL_SURFACE('',#96721,0.5);
#86280=CYLINDRICAL_SURFACE('',#96726,0.5);
#86281=CYLINDRICAL_SURFACE('',#96727,0.5);
#86282=CYLINDRICAL_SURFACE('',#96733,0.5);
#86283=CYLINDRICAL_SURFACE('',#96735,0.5);
#86284=CYLINDRICAL_SURFACE('',#96740,0.5);
#86285=CYLINDRICAL_SURFACE('',#96743,0.5);
#86286=CYLINDRICAL_SURFACE('',#96749,0.5);
#86287=CYLINDRICAL_SURFACE('',#96750,0.5);
#86288=CYLINDRICAL_SURFACE('',#96756,0.5);
#86289=CYLINDRICAL_SURFACE('',#96762,0.5);
#86290=CYLINDRICAL_SURFACE('',#96763,0.5);
#86291=CYLINDRICAL_SURFACE('',#96768,0.5);
#86292=CYLINDRICAL_SURFACE('',#96775,3.);
#86293=CYLINDRICAL_SURFACE('',#96781,0.5);
#86294=CYLINDRICAL_SURFACE('',#96785,0.5);
#86295=CYLINDRICAL_SURFACE('',#96791,0.5);
#86296=CYLINDRICAL_SURFACE('',#96797,0.5);
#86297=CYLINDRICAL_SURFACE('',#96803,0.5);
#86298=CYLINDRICAL_SURFACE('',#96806,0.5);
#86299=CYLINDRICAL_SURFACE('',#96809,0.5);
#86300=CYLINDRICAL_SURFACE('',#96812,0.5);
#86301=CYLINDRICAL_SURFACE('',#96818,0.5);
#86302=CYLINDRICAL_SURFACE('',#96826,0.5);
#86303=CYLINDRICAL_SURFACE('',#96833,0.5);
#86304=CYLINDRICAL_SURFACE('',#96836,0.5);
#86305=CYLINDRICAL_SURFACE('',#96840,0.5);
#86306=CYLINDRICAL_SURFACE('',#96843,0.5);
#86307=CYLINDRICAL_SURFACE('',#96850,0.5);
#86308=CYLINDRICAL_SURFACE('',#96858,0.5);
#86309=CYLINDRICAL_SURFACE('',#96864,0.5);
#86310=CYLINDRICAL_SURFACE('',#96867,0.5);
#86311=CYLINDRICAL_SURFACE('',#96870,0.5);
#86312=CYLINDRICAL_SURFACE('',#96873,0.5);
#86313=CYLINDRICAL_SURFACE('',#96879,0.5);
#86314=CYLINDRICAL_SURFACE('',#96885,0.5);
#86315=CYLINDRICAL_SURFACE('',#96891,0.5);
#86316=CYLINDRICAL_SURFACE('',#96895,0.5);
#86317=CYLINDRICAL_SURFACE('',#96902,3.);
#86318=CYLINDRICAL_SURFACE('',#96908,0.5);
#86319=CYLINDRICAL_SURFACE('',#96913,0.5);
#86320=CYLINDRICAL_SURFACE('',#96914,0.5);
#86321=CYLINDRICAL_SURFACE('',#96920,0.5);
#86322=CYLINDRICAL_SURFACE('',#96928,0.5);
#86323=CYLINDRICAL_SURFACE('',#96933,0.5);
#86324=CYLINDRICAL_SURFACE('',#96939,0.5);
#86325=CYLINDRICAL_SURFACE('',#96940,0.5);
#86326=CYLINDRICAL_SURFACE('',#96945,3.);
#86327=CYLINDRICAL_SURFACE('',#96954,3.);
#86328=CYLINDRICAL_SURFACE('',#96970,0.5);
#86329=CYLINDRICAL_SURFACE('',#96977,3.);
#86330=CYLINDRICAL_SURFACE('',#96983,0.5);
#86331=CYLINDRICAL_SURFACE('',#96999,0.5);
#86332=CYLINDRICAL_SURFACE('',#97007,0.5);
#86333=CYLINDRICAL_SURFACE('',#97015,0.5);
#86334=CYLINDRICAL_SURFACE('',#97019,0.5);
#86335=CYLINDRICAL_SURFACE('',#97028,3.);
#86336=CYLINDRICAL_SURFACE('',#97034,0.5);
#86337=CYLINDRICAL_SURFACE('',#97042,0.5);
#86338=CYLINDRICAL_SURFACE('',#97048,0.5);
#86339=CYLINDRICAL_SURFACE('',#97053,0.5);
#86340=CYLINDRICAL_SURFACE('',#97057,0.5);
#86341=CYLINDRICAL_SURFACE('',#97063,0.5);
#86342=CYLINDRICAL_SURFACE('',#97071,0.5);
#86343=CYLINDRICAL_SURFACE('',#97079,0.5);
#86344=CYLINDRICAL_SURFACE('',#97082,0.5);
#86345=CYLINDRICAL_SURFACE('',#97100,0.5);
#86346=CYLINDRICAL_SURFACE('',#97103,0.5);
#86347=CYLINDRICAL_SURFACE('',#97112,0.5);
#86348=CYLINDRICAL_SURFACE('',#97123,3.);
#86349=CYLINDRICAL_SURFACE('',#97125,67.5);
#86350=CYLINDRICAL_SURFACE('',#97127,3.);
#86351=CYLINDRICAL_SURFACE('',#97130,5.);
#86352=CYLINDRICAL_SURFACE('',#97132,58.5);
#86353=CYLINDRICAL_SURFACE('',#97134,5.);
#86354=CYLINDRICAL_SURFACE('',#97137,3.);
#86355=CYLINDRICAL_SURFACE('',#97139,67.5);
#86356=CYLINDRICAL_SURFACE('',#97141,3.);
#86357=CYLINDRICAL_SURFACE('',#97146,0.5);
#86358=CYLINDRICAL_SURFACE('',#97149,0.5);
#86359=CYLINDRICAL_SURFACE('',#97152,0.5);
#86360=CYLINDRICAL_SURFACE('',#97153,0.5);
#86361=CYLINDRICAL_SURFACE('',#97162,0.5);
#86362=CYLINDRICAL_SURFACE('',#97165,0.5);
#86363=CYLINDRICAL_SURFACE('',#97174,0.5);
#86364=CYLINDRICAL_SURFACE('',#97177,0.5);
#86365=CYLINDRICAL_SURFACE('',#97188,0.5);
#86366=CYLINDRICAL_SURFACE('',#97193,0.5);
#86367=CYLINDRICAL_SURFACE('',#97200,0.5);
#86368=CYLINDRICAL_SURFACE('',#97204,0.5);
#86369=CYLINDRICAL_SURFACE('',#97210,0.5);
#86370=CYLINDRICAL_SURFACE('',#97218,0.5);
#86371=CYLINDRICAL_SURFACE('',#97224,3.);
#86372=CYLINDRICAL_SURFACE('',#97225,0.5);
#86373=CYLINDRICAL_SURFACE('',#97227,2.75);
#86374=CYLINDRICAL_SURFACE('',#97233,2.);
#86375=CYLINDRICAL_SURFACE('',#97235,0.5);
#86376=CYLINDRICAL_SURFACE('',#97237,0.5);
#86377=CYLINDRICAL_SURFACE('',#97247,0.5);
#86378=CYLINDRICAL_SURFACE('',#97248,2.75);
#86379=CYLINDRICAL_SURFACE('',#97253,2.);
#86380=CYLINDRICAL_SURFACE('',#97255,0.5);
#86381=CYLINDRICAL_SURFACE('',#97262,0.5);
#86382=CYLINDRICAL_SURFACE('',#97264,0.5);
#86383=CYLINDRICAL_SURFACE('',#97270,0.5);
#86384=CYLINDRICAL_SURFACE('',#97272,0.5);
#86385=CYLINDRICAL_SURFACE('',#97279,0.5);
#86386=CYLINDRICAL_SURFACE('',#97281,0.5);
#86387=CYLINDRICAL_SURFACE('',#97293,0.5);
#86388=CYLINDRICAL_SURFACE('',#97295,0.5);
#86389=CYLINDRICAL_SURFACE('',#97301,0.5);
#86390=CYLINDRICAL_SURFACE('',#97303,0.5);
#86391=CYLINDRICAL_SURFACE('',#97308,0.5);
#86392=CYLINDRICAL_SURFACE('',#97310,0.5);
#86393=CYLINDRICAL_SURFACE('',#97316,0.5);
#86394=CYLINDRICAL_SURFACE('',#97318,0.5);
#86395=CYLINDRICAL_SURFACE('',#97328,0.5);
#86396=CYLINDRICAL_SURFACE('',#97330,0.5);
#86397=CYLINDRICAL_SURFACE('',#97345,0.5);
#86398=CYLINDRICAL_SURFACE('',#97348,0.5);
#86399=CYLINDRICAL_SURFACE('',#97392,0.5);
#86400=CYLINDRICAL_SURFACE('',#97395,0.5);
#86401=CYLINDRICAL_SURFACE('',#97405,0.5);
#86402=CYLINDRICAL_SURFACE('',#97408,0.5);
#86403=CYLINDRICAL_SURFACE('',#97410,0.5);
#86404=CYLINDRICAL_SURFACE('',#97414,0.5);
#86405=CYLINDRICAL_SURFACE('',#97440,0.5);
#86406=CYLINDRICAL_SURFACE('',#97443,0.5);
#86407=CYLINDRICAL_SURFACE('',#97449,0.5);
#86408=CYLINDRICAL_SURFACE('',#97460,0.5);
#86409=CYLINDRICAL_SURFACE('',#97463,0.5);
#86410=CYLINDRICAL_SURFACE('',#97488,0.5);
#86411=CYLINDRICAL_SURFACE('',#97494,3.);
#86412=CYLINDRICAL_SURFACE('',#97498,0.5);
#86413=CYLINDRICAL_SURFACE('',#97501,0.5);
#86414=CYLINDRICAL_SURFACE('',#97507,0.5);
#86415=CYLINDRICAL_SURFACE('',#97510,0.5);
#86416=CYLINDRICAL_SURFACE('',#97517,0.5);
#86417=CYLINDRICAL_SURFACE('',#97520,0.5);
#86418=CYLINDRICAL_SURFACE('',#97522,2.75);
#86419=CYLINDRICAL_SURFACE('',#97524,2.75);
#86420=CYLINDRICAL_SURFACE('',#97530,0.250000000000003);
#86421=CYLINDRICAL_SURFACE('',#97541,0.250000000000003);
#86422=CYLINDRICAL_SURFACE('',#97552,0.249999999999997);
#86423=CYLINDRICAL_SURFACE('',#97563,0.250000000000003);
#86424=CYLINDRICAL_SURFACE('',#97569,5.);
#86425=CYLINDRICAL_SURFACE('',#97571,0.499999999999999);
#86426=CYLINDRICAL_SURFACE('',#97576,3.);
#86427=CYLINDRICAL_SURFACE('',#97579,0.5);
#86428=CYLINDRICAL_SURFACE('',#97581,1.);
#86429=CYLINDRICAL_SURFACE('',#97582,0.5);
#86430=CYLINDRICAL_SURFACE('',#97587,0.5);
#86431=CYLINDRICAL_SURFACE('',#97592,0.5);
#86432=CYLINDRICAL_SURFACE('',#97593,1.);
#86433=CYLINDRICAL_SURFACE('',#97594,0.5);
#86434=CYLINDRICAL_SURFACE('',#97599,0.5);
#86435=CYLINDRICAL_SURFACE('',#97604,0.5);
#86436=CYLINDRICAL_SURFACE('',#97605,1.);
#86437=CYLINDRICAL_SURFACE('',#97610,0.5);
#86438=CYLINDRICAL_SURFACE('',#97615,0.5);
#86439=CYLINDRICAL_SURFACE('',#97620,0.5);
#86440=CYLINDRICAL_SURFACE('',#97623,0.5);
#86441=CYLINDRICAL_SURFACE('',#97628,0.5);
#86442=CYLINDRICAL_SURFACE('',#97633,0.5);
#86443=CYLINDRICAL_SURFACE('',#97635,3.);
#86444=CYLINDRICAL_SURFACE('',#97637,0.5);
#86445=CYLINDRICAL_SURFACE('',#97646,0.5);
#86446=CYLINDRICAL_SURFACE('',#97656,1.);
#86447=CYLINDRICAL_SURFACE('',#97658,0.5);
#86448=CYLINDRICAL_SURFACE('',#97662,0.499999999999998);
#86449=CYLINDRICAL_SURFACE('',#97665,0.5);
#86450=CYLINDRICAL_SURFACE('',#97666,1.);
#86451=CYLINDRICAL_SURFACE('',#97667,0.5);
#86452=CYLINDRICAL_SURFACE('',#97670,0.499999999999998);
#86453=CYLINDRICAL_SURFACE('',#97673,0.5);
#86454=CYLINDRICAL_SURFACE('',#97674,1.);
#86455=CYLINDRICAL_SURFACE('',#97679,0.5);
#86456=CYLINDRICAL_SURFACE('',#97680,0.5);
#86457=CYLINDRICAL_SURFACE('',#97683,0.499999999999999);
#86458=CYLINDRICAL_SURFACE('',#97686,0.5);
#86459=CYLINDRICAL_SURFACE('',#97687,0.999999999999997);
#86460=CYLINDRICAL_SURFACE('',#97689,0.5);
#86461=CYLINDRICAL_SURFACE('',#97693,0.999999999999997);
#86462=CYLINDRICAL_SURFACE('',#97695,0.5);
#86463=CYLINDRICAL_SURFACE('',#97698,0.499999999999999);
#86464=CYLINDRICAL_SURFACE('',#97701,0.5);
#86465=CYLINDRICAL_SURFACE('',#97702,0.999999999999997);
#86466=CYLINDRICAL_SURFACE('',#97703,0.999999999999996);
#86467=CYLINDRICAL_SURFACE('',#97706,0.5);
#86468=CYLINDRICAL_SURFACE('',#97709,0.499999999999999);
#86469=CYLINDRICAL_SURFACE('',#97712,0.5);
#86470=CYLINDRICAL_SURFACE('',#97713,0.999999999999997);
#86471=CYLINDRICAL_SURFACE('',#97716,0.5);
#86472=CYLINDRICAL_SURFACE('',#97719,0.499999999999999);
#86473=CYLINDRICAL_SURFACE('',#97722,0.5);
#86474=CYLINDRICAL_SURFACE('',#97723,0.999999999999997);
#86475=CYLINDRICAL_SURFACE('',#97725,0.999999999999996);
#86476=CYLINDRICAL_SURFACE('',#97728,0.5);
#86477=CYLINDRICAL_SURFACE('',#97731,0.500000000000005);
#86478=CYLINDRICAL_SURFACE('',#97734,0.5);
#86479=CYLINDRICAL_SURFACE('',#97735,0.999999999999996);
#86480=CYLINDRICAL_SURFACE('',#97737,0.5);
#86481=CYLINDRICAL_SURFACE('',#97740,0.999999999999996);
#86482=CYLINDRICAL_SURFACE('',#97742,0.5);
#86483=CYLINDRICAL_SURFACE('',#97745,0.500000000000005);
#86484=CYLINDRICAL_SURFACE('',#97748,0.5);
#86485=CYLINDRICAL_SURFACE('',#97749,0.999999999999996);
#86486=CYLINDRICAL_SURFACE('',#97752,0.5);
#86487=CYLINDRICAL_SURFACE('',#97755,0.5);
#86488=CYLINDRICAL_SURFACE('',#97762,0.5);
#86489=CYLINDRICAL_SURFACE('',#97765,0.5);
#86490=CYLINDRICAL_SURFACE('',#97771,0.5);
#86491=CYLINDRICAL_SURFACE('',#97774,0.5);
#86492=CYLINDRICAL_SURFACE('',#97780,0.5);
#86493=CYLINDRICAL_SURFACE('',#97783,0.5);
#86494=CYLINDRICAL_SURFACE('',#97789,0.5);
#86495=CYLINDRICAL_SURFACE('',#97792,0.5);
#86496=CYLINDRICAL_SURFACE('',#97799,0.5);
#86497=CYLINDRICAL_SURFACE('',#97802,0.5);
#86498=CYLINDRICAL_SURFACE('',#97809,3.);
#86499=CYLINDRICAL_SURFACE('',#97814,3.);
#86500=CYLINDRICAL_SURFACE('',#97821,58.3875000000282);
#86501=CYLINDRICAL_SURFACE('',#97823,5.);
#86502=CYLINDRICAL_SURFACE('',#97829,0.5);
#86503=CYLINDRICAL_SURFACE('',#97835,0.5);
#86504=CYLINDRICAL_SURFACE('',#97838,0.5);
#86505=CYLINDRICAL_SURFACE('',#97844,0.5);
#86506=CYLINDRICAL_SURFACE('',#97847,0.5);
#86507=CYLINDRICAL_SURFACE('',#97854,0.5);
#86508=CYLINDRICAL_SURFACE('',#97857,5.);
#86509=CYLINDRICAL_SURFACE('',#97864,0.5);
#86510=CYLINDRICAL_SURFACE('',#97867,0.5);
#86511=CYLINDRICAL_SURFACE('',#97874,0.5);
#86512=CYLINDRICAL_SURFACE('',#97877,0.5);
#86513=CYLINDRICAL_SURFACE('',#97884,0.5);
#86514=CYLINDRICAL_SURFACE('',#97887,0.5);
#86515=CYLINDRICAL_SURFACE('',#97890,58.3875000000282);
#86516=CYLINDRICAL_SURFACE('',#97897,3.);
#86517=CYLINDRICAL_SURFACE('',#97902,3.);
#86518=CYLINDRICAL_SURFACE('',#97907,3.);
#86519=CYLINDRICAL_SURFACE('',#97915,58.5);
#86520=CYLINDRICAL_SURFACE('',#97923,58.5);
#86521=CYLINDRICAL_SURFACE('',#97937,58.3875000000282);
#86522=CYLINDRICAL_SURFACE('',#97939,5.);
#86523=CYLINDRICAL_SURFACE('',#97969,3.25);
#86524=CYLINDRICAL_SURFACE('',#97974,2.);
#86525=CYLINDRICAL_SURFACE('',#97978,2.5);
#86526=CYLINDRICAL_SURFACE('',#98110,0.75);
#86527=CYLINDRICAL_SURFACE('',#98123,0.75);
#86528=CYLINDRICAL_SURFACE('',#98124,0.75);
#86529=CYLINDRICAL_SURFACE('',#98136,0.750000000000001);
#86530=CYLINDRICAL_SURFACE('',#98137,0.750000000000001);
#86531=CYLINDRICAL_SURFACE('',#98149,0.749999999999998);
#86532=CYLINDRICAL_SURFACE('',#98150,0.749999999999999);
#86533=CYLINDRICAL_SURFACE('',#98162,0.75);
#86534=CYLINDRICAL_SURFACE('',#98163,1.5);
#86535=CYLINDRICAL_SURFACE('',#98164,1.5);
#86536=CYLINDRICAL_SURFACE('',#98165,1.5);
#86537=CYLINDRICAL_SURFACE('',#98166,1.5);
#86538=CYLINDRICAL_SURFACE('',#98167,1.49999999999999);
#86539=CYLINDRICAL_SURFACE('',#98168,1.5);
#86540=CYLINDRICAL_SURFACE('',#98169,1.5);
#86541=CYLINDRICAL_SURFACE('',#98170,1.5);
#86542=CYLINDRICAL_SURFACE('',#98176,0.450000000000006);
#86543=CYLINDRICAL_SURFACE('',#98190,0.449999999999999);
#86544=CYLINDRICAL_SURFACE('',#98204,0.450000000000006);
#86545=CYLINDRICAL_SURFACE('',#98210,0.450000000000006);
#86546=CYLINDRICAL_SURFACE('',#98224,0.449999999999999);
#86547=CYLINDRICAL_SURFACE('',#98226,0.450000000000006);
#86548=CYLINDRICAL_SURFACE('',#98236,0.450000000000006);
#86549=CYLINDRICAL_SURFACE('',#98250,0.449999999999999);
#86550=CYLINDRICAL_SURFACE('',#98252,0.450000000000001);
#86551=CYLINDRICAL_SURFACE('',#98262,0.450000000000006);
#86552=CYLINDRICAL_SURFACE('',#98264,0.449999999999999);
#86553=CYLINDRICAL_SURFACE('',#98274,0.450000000000001);
#86554=CYLINDRICAL_SURFACE('',#98276,0.450000000000001);
#86555=CYLINDRICAL_SURFACE('',#98286,0.450000000000006);
#86556=CYLINDRICAL_SURFACE('',#98288,0.450000000000001);
#86557=CYLINDRICAL_SURFACE('',#98302,0.450000000000001);
#86558=CYLINDRICAL_SURFACE('',#98316,0.450000000000006);
#86559=CYLINDRICAL_SURFACE('',#98318,0.450000000000001);
#86560=CYLINDRICAL_SURFACE('',#98328,0.45);
#86561=CYLINDRICAL_SURFACE('',#98330,0.450000000000006);
#86562=CYLINDRICAL_SURFACE('',#98340,0.450000000000006);
#86563=CYLINDRICAL_SURFACE('',#98342,0.449999999999999);
#86564=CYLINDRICAL_SURFACE('',#98352,0.450000000000001);
#86565=CYLINDRICAL_SURFACE('',#98354,0.450000000000006);
#86566=CYLINDRICAL_SURFACE('',#98364,0.450000000000006);
#86567=CYLINDRICAL_SURFACE('',#98366,0.449999999999999);
#86568=CYLINDRICAL_SURFACE('',#98376,0.450000000000001);
#86569=CYLINDRICAL_SURFACE('',#98378,0.450000000000006);
#86570=CYLINDRICAL_SURFACE('',#98388,0.450000000000006);
#86571=CYLINDRICAL_SURFACE('',#98390,0.450000000000001);
#86572=CYLINDRICAL_SURFACE('',#98400,0.45);
#86573=CYLINDRICAL_SURFACE('',#98402,0.450000000000006);
#86574=CYLINDRICAL_SURFACE('',#98412,0.450000000000006);
#86575=CYLINDRICAL_SURFACE('',#98414,0.450000000000001);
#86576=CYLINDRICAL_SURFACE('',#98424,0.45);
#86577=CYLINDRICAL_SURFACE('',#98438,0.450000000000006);
#86578=CYLINDRICAL_SURFACE('',#98440,0.449999999999999);
#86579=CYLINDRICAL_SURFACE('',#98450,0.450000000000001);
#86580=CYLINDRICAL_SURFACE('',#98472,0.450000000000006);
#86581=CYLINDRICAL_SURFACE('',#98474,0.45);
#86582=CYLINDRICAL_SURFACE('',#98484,0.450000000000001);
#86583=CYLINDRICAL_SURFACE('',#98498,0.450000000000006);
#86584=CYLINDRICAL_SURFACE('',#98500,0.45);
#86585=CYLINDRICAL_SURFACE('',#98510,0.450000000000001);
#86586=CYLINDRICAL_SURFACE('',#98512,0.450000000000006);
#86587=CYLINDRICAL_SURFACE('',#98522,0.450000000000001);
#86588=CYLINDRICAL_SURFACE('',#98536,0.450000000000006);
#86589=CYLINDRICAL_SURFACE('',#98538,0.450000000000006);
#86590=CYLINDRICAL_SURFACE('',#98548,0.45);
#86591=CYLINDRICAL_SURFACE('',#98554,0.449999999999999);
#86592=CYLINDRICAL_SURFACE('',#98556,0.450000000000006);
#86593=CYLINDRICAL_SURFACE('',#98566,0.450000000000006);
#86594=CYLINDRICAL_SURFACE('',#98580,0.450000000000001);
#86595=CYLINDRICAL_SURFACE('',#98586,0.449999999999999);
#86596=CYLINDRICAL_SURFACE('',#98588,0.450000000000006);
#86597=CYLINDRICAL_SURFACE('',#98598,0.450000000000006);
#86598=CYLINDRICAL_SURFACE('',#98600,0.450000000000001);
#86599=CYLINDRICAL_SURFACE('',#98610,0.449999999999999);
#86600=CYLINDRICAL_SURFACE('',#98612,0.450000000000006);
#86601=CYLINDRICAL_SURFACE('',#98626,0.450000000000001);
#86602=CYLINDRICAL_SURFACE('',#98636,0.449999999999999);
#86603=CYLINDRICAL_SURFACE('',#98638,0.450000000000006);
#86604=CYLINDRICAL_SURFACE('',#98648,0.450000000000006);
#86605=CYLINDRICAL_SURFACE('',#98650,0.449999999999999);
#86606=CYLINDRICAL_SURFACE('',#98660,0.449999999999999);
#86607=CYLINDRICAL_SURFACE('',#98662,0.450000000000006);
#86608=CYLINDRICAL_SURFACE('',#98672,0.450000000000006);
#86609=CYLINDRICAL_SURFACE('',#98674,0.449999999999999);
#86610=CYLINDRICAL_SURFACE('',#98684,0.449999999999999);
#86611=CYLINDRICAL_SURFACE('',#98686,0.450000000000006);
#86612=CYLINDRICAL_SURFACE('',#98696,0.450000000000001);
#86613=CYLINDRICAL_SURFACE('',#98714,0.449999999999999);
#86614=CYLINDRICAL_SURFACE('',#98716,0.450000000000006);
#86615=CYLINDRICAL_SURFACE('',#98730,0.449999999999999);
#86616=CYLINDRICAL_SURFACE('',#98740,0.449999999999999);
#86617=CYLINDRICAL_SURFACE('',#98742,0.450000000000006);
#86618=CYLINDRICAL_SURFACE('',#98756,0.449999999999999);
#86619=CYLINDRICAL_SURFACE('',#98774,0.449999999999999);
#86620=CYLINDRICAL_SURFACE('',#98776,0.450000000000006);
#86621=CYLINDRICAL_SURFACE('',#98786,0.450000000000006);
#86622=CYLINDRICAL_SURFACE('',#98788,0.449999999999999);
#86623=CYLINDRICAL_SURFACE('',#98798,0.449999999999999);
#86624=CYLINDRICAL_SURFACE('',#98800,0.450000000000006);
#86625=CYLINDRICAL_SURFACE('',#98810,0.450000000000006);
#86626=CYLINDRICAL_SURFACE('',#98832,0.449999999999999);
#86627=CYLINDRICAL_SURFACE('',#98834,0.450000000000006);
#86628=CYLINDRICAL_SURFACE('',#98844,0.450000000000006);
#86629=CYLINDRICAL_SURFACE('',#98858,0.449999999999999);
#86630=CYLINDRICAL_SURFACE('',#98860,0.450000000000006);
#86631=CYLINDRICAL_SURFACE('',#98870,0.450000000000006);
#86632=CYLINDRICAL_SURFACE('',#98872,0.449999999999999);
#86633=CYLINDRICAL_SURFACE('',#98882,0.449999999999999);
#86634=CYLINDRICAL_SURFACE('',#98884,0.450000000000001);
#86635=CYLINDRICAL_SURFACE('',#98894,0.450000000000006);
#86636=CYLINDRICAL_SURFACE('',#98908,0.449999999999999);
#86637=CYLINDRICAL_SURFACE('',#98910,0.450000000000006);
#86638=CYLINDRICAL_SURFACE('',#98920,0.450000000000001);
#86639=CYLINDRICAL_SURFACE('',#98922,0.449999999999999);
#86640=CYLINDRICAL_SURFACE('',#98932,0.449999999999999);
#86641=CYLINDRICAL_SURFACE('',#98946,0.450000000000006);
#86642=CYLINDRICAL_SURFACE('',#98952,0.450000000000006);
#86643=CYLINDRICAL_SURFACE('',#98966,0.449999999999999);
#86644=CYLINDRICAL_SURFACE('',#99029,0.44999999999999);
#86645=CYLINDRICAL_SURFACE('',#99043,0.450000000000001);
#86646=CYLINDRICAL_SURFACE('',#99052,0.450000000000001);
#86647=CYLINDRICAL_SURFACE('',#99066,0.45);
#86648=CYLINDRICAL_SURFACE('',#99075,0.450000000000006);
#86649=CYLINDRICAL_SURFACE('',#99089,0.44999999999999);
#86650=CYLINDRICAL_SURFACE('',#99098,0.45);
#86651=CYLINDRICAL_SURFACE('',#99112,0.450000000000006);
#86652=CYLINDRICAL_SURFACE('',#99220,0.75);
#86653=CYLINDRICAL_SURFACE('',#99222,0.750000000000001);
#86654=CYLINDRICAL_SURFACE('',#99224,0.750000000000001);
#86655=CYLINDRICAL_SURFACE('',#99226,0.750000000000001);
#86656=CYLINDRICAL_SURFACE('',#99228,0.750000000000001);
#86657=CYLINDRICAL_SURFACE('',#99230,0.750000000000001);
#86658=CYLINDRICAL_SURFACE('',#99232,0.75);
#86659=CYLINDRICAL_SURFACE('',#99234,0.75);
#86660=CYLINDRICAL_SURFACE('',#99236,0.75);
#86661=CYLINDRICAL_SURFACE('',#99238,0.750000000000001);
#86662=CYLINDRICAL_SURFACE('',#99240,0.750000000000001);
#86663=CYLINDRICAL_SURFACE('',#99242,0.750000000000001);
#86664=CYLINDRICAL_SURFACE('',#99244,0.750000000000001);
#86665=CYLINDRICAL_SURFACE('',#99246,0.750000000000001);
#86666=CYLINDRICAL_SURFACE('',#99248,0.750000000000001);
#86667=CYLINDRICAL_SURFACE('',#99250,0.750000000000001);
#86668=CYLINDRICAL_SURFACE('',#99252,0.75);
#86669=CYLINDRICAL_SURFACE('',#99254,0.75);
#86670=CYLINDRICAL_SURFACE('',#99256,0.75);
#86671=CYLINDRICAL_SURFACE('',#99258,0.75);
#86672=CYLINDRICAL_SURFACE('',#99260,0.750000000000001);
#86673=CYLINDRICAL_SURFACE('',#99262,0.75);
#86674=CYLINDRICAL_SURFACE('',#99264,0.750000000000001);
#86675=CYLINDRICAL_SURFACE('',#99266,0.750000000000001);
#86676=CYLINDRICAL_SURFACE('',#99268,0.750000000000001);
#86677=CYLINDRICAL_SURFACE('',#99270,0.750000000000001);
#86678=CYLINDRICAL_SURFACE('',#99272,0.750000000000001);
#86679=CYLINDRICAL_SURFACE('',#99274,0.750000000000001);
#86680=CYLINDRICAL_SURFACE('',#99276,0.750000000000001);
#86681=CYLINDRICAL_SURFACE('',#99278,0.750000000000001);
#86682=CYLINDRICAL_SURFACE('',#99280,0.750000000000001);
#86683=CYLINDRICAL_SURFACE('',#99282,0.750000000000001);
#86684=CYLINDRICAL_SURFACE('',#99284,0.75);
#86685=CYLINDRICAL_SURFACE('',#99286,0.750000000000001);
#86686=CYLINDRICAL_SURFACE('',#99288,0.75);
#86687=CYLINDRICAL_SURFACE('',#99290,0.75);
#86688=CYLINDRICAL_SURFACE('',#99292,0.750000000000001);
#86689=CYLINDRICAL_SURFACE('',#99294,0.750000000000001);
#86690=CYLINDRICAL_SURFACE('',#99296,0.750000000000001);
#86691=CYLINDRICAL_SURFACE('',#99298,0.750000000000001);
#86692=CYLINDRICAL_SURFACE('',#99300,0.750000000000001);
#86693=CYLINDRICAL_SURFACE('',#99302,0.750000000000001);
#86694=CYLINDRICAL_SURFACE('',#99304,0.750000000000001);
#86695=CYLINDRICAL_SURFACE('',#99306,0.750000000000001);
#86696=CYLINDRICAL_SURFACE('',#99308,0.75);
#86697=CYLINDRICAL_SURFACE('',#99310,0.75);
#86698=CYLINDRICAL_SURFACE('',#99312,0.750000000000001);
#86699=CYLINDRICAL_SURFACE('',#99314,0.750000000000001);
#86700=CYLINDRICAL_SURFACE('',#99316,0.750000000000001);
#86701=CYLINDRICAL_SURFACE('',#99318,0.750000000000001);
#86702=CYLINDRICAL_SURFACE('',#99320,0.750000000000001);
#86703=CYLINDRICAL_SURFACE('',#99322,0.750000000000001);
#86704=CYLINDRICAL_SURFACE('',#99324,0.750000000000001);
#86705=CYLINDRICAL_SURFACE('',#99326,0.750000000000001);
#86706=CYLINDRICAL_SURFACE('',#99328,0.750000000000001);
#86707=CYLINDRICAL_SURFACE('',#99330,0.750000000000001);
#86708=CYLINDRICAL_SURFACE('',#99332,0.750000000000001);
#86709=CYLINDRICAL_SURFACE('',#99334,0.750000000000001);
#86710=CYLINDRICAL_SURFACE('',#99336,0.750000000000001);
#86711=CYLINDRICAL_SURFACE('',#99338,0.750000000000001);
#86712=CYLINDRICAL_SURFACE('',#99340,0.750000000000001);
#86713=CYLINDRICAL_SURFACE('',#99342,0.750000000000001);
#86714=CYLINDRICAL_SURFACE('',#99344,0.750000000000001);
#86715=CYLINDRICAL_SURFACE('',#99346,0.750000000000001);
#86716=CYLINDRICAL_SURFACE('',#99348,0.750000000000001);
#86717=CYLINDRICAL_SURFACE('',#99350,0.750000000000001);
#86718=CYLINDRICAL_SURFACE('',#99352,0.750000000000001);
#86719=CYLINDRICAL_SURFACE('',#99354,0.750000000000001);
#86720=CYLINDRICAL_SURFACE('',#99356,0.750000000000001);
#86721=CYLINDRICAL_SURFACE('',#99358,0.750000000000001);
#86722=CYLINDRICAL_SURFACE('',#99360,0.750000000000001);
#86723=CYLINDRICAL_SURFACE('',#99362,0.75);
#86724=CYLINDRICAL_SURFACE('',#99364,0.750000000000001);
#86725=CYLINDRICAL_SURFACE('',#99366,0.750000000000001);
#86726=CYLINDRICAL_SURFACE('',#99368,0.75);
#86727=CYLINDRICAL_SURFACE('',#99370,0.750000000000001);
#86728=CYLINDRICAL_SURFACE('',#99372,0.75);
#86729=CYLINDRICAL_SURFACE('',#99374,0.75);
#86730=CYLINDRICAL_SURFACE('',#99376,0.750000000000001);
#86731=CYLINDRICAL_SURFACE('',#99378,0.750000000000001);
#86732=CYLINDRICAL_SURFACE('',#99380,0.750000000000001);
#86733=CYLINDRICAL_SURFACE('',#99382,0.750000000000001);
#86734=CYLINDRICAL_SURFACE('',#99384,0.750000000000001);
#86735=CYLINDRICAL_SURFACE('',#99386,0.750000000000001);
#86736=CYLINDRICAL_SURFACE('',#99388,0.750000000000001);
#86737=CYLINDRICAL_SURFACE('',#99390,0.750000000000001);
#86738=CYLINDRICAL_SURFACE('',#99392,0.750000000000001);
#86739=CYLINDRICAL_SURFACE('',#99394,0.750000000000001);
#86740=CYLINDRICAL_SURFACE('',#99396,0.750000000000001);
#86741=CYLINDRICAL_SURFACE('',#99398,0.750000000000001);
#86742=CYLINDRICAL_SURFACE('',#99400,0.750000000000001);
#86743=CYLINDRICAL_SURFACE('',#99402,0.750000000000001);
#86744=CYLINDRICAL_SURFACE('',#99404,0.750000000000001);
#86745=CYLINDRICAL_SURFACE('',#99406,0.750000000000001);
#86746=CYLINDRICAL_SURFACE('',#99408,0.750000000000001);
#86747=CYLINDRICAL_SURFACE('',#99410,0.75);
#86748=CYLINDRICAL_SURFACE('',#99412,0.750000000000001);
#86749=CYLINDRICAL_SURFACE('',#99414,0.75);
#86750=CYLINDRICAL_SURFACE('',#99416,0.75);
#86751=CYLINDRICAL_SURFACE('',#99418,0.750000000000001);
#86752=CYLINDRICAL_SURFACE('',#99420,0.750000000000001);
#86753=CYLINDRICAL_SURFACE('',#99422,0.750000000000001);
#86754=CYLINDRICAL_SURFACE('',#99424,0.750000000000001);
#86755=CYLINDRICAL_SURFACE('',#99426,0.750000000000001);
#86756=CYLINDRICAL_SURFACE('',#99428,0.750000000000001);
#86757=CYLINDRICAL_SURFACE('',#99430,0.750000000000001);
#86758=CYLINDRICAL_SURFACE('',#99432,0.750000000000001);
#86759=CYLINDRICAL_SURFACE('',#99434,0.750000000000001);
#86760=CYLINDRICAL_SURFACE('',#99436,0.750000000000001);
#86761=CYLINDRICAL_SURFACE('',#99438,0.750000000000001);
#86762=CYLINDRICAL_SURFACE('',#99440,0.750000000000001);
#86763=CYLINDRICAL_SURFACE('',#99442,0.750000000000001);
#86764=CYLINDRICAL_SURFACE('',#99444,0.750000000000001);
#86765=CYLINDRICAL_SURFACE('',#99446,0.750000000000001);
#86766=CYLINDRICAL_SURFACE('',#99448,0.750000000000001);
#86767=CYLINDRICAL_SURFACE('',#99450,0.750000000000001);
#86768=CYLINDRICAL_SURFACE('',#99452,0.750000000000001);
#86769=CYLINDRICAL_SURFACE('',#99454,0.750000000000001);
#86770=CYLINDRICAL_SURFACE('',#99456,0.750000000000001);
#86771=CYLINDRICAL_SURFACE('',#99458,0.750000000000001);
#86772=CYLINDRICAL_SURFACE('',#99460,0.750000000000001);
#86773=CYLINDRICAL_SURFACE('',#99462,0.750000000000001);
#86774=CYLINDRICAL_SURFACE('',#99464,0.750000000000001);
#86775=CYLINDRICAL_SURFACE('',#99466,0.750000000000001);
#86776=CYLINDRICAL_SURFACE('',#99468,0.750000000000001);
#86777=CYLINDRICAL_SURFACE('',#99470,0.750000000000001);
#86778=CYLINDRICAL_SURFACE('',#99472,0.750000000000001);
#86779=CYLINDRICAL_SURFACE('',#99474,0.750000000000001);
#86780=CYLINDRICAL_SURFACE('',#99476,0.750000000000001);
#86781=CYLINDRICAL_SURFACE('',#99478,0.75);
#86782=CYLINDRICAL_SURFACE('',#99480,0.75);
#86783=CYLINDRICAL_SURFACE('',#99482,0.750000000000001);
#86784=CYLINDRICAL_SURFACE('',#99484,0.750000000000001);
#86785=CYLINDRICAL_SURFACE('',#99486,0.750000000000001);
#86786=CYLINDRICAL_SURFACE('',#99488,10.);
#86787=CYLINDRICAL_SURFACE('',#99490,10.);
#86788=CYLINDRICAL_SURFACE('',#99492,10.);
#86789=CYLINDRICAL_SURFACE('',#99494,10.);
#86790=CYLINDRICAL_SURFACE('',#99496,13.1055395526668);
#86791=CYLINDRICAL_SURFACE('',#99498,13.1055395526668);
#86792=CYLINDRICAL_SURFACE('',#99500,11.1055395526669);
#86793=CYLINDRICAL_SURFACE('',#99504,11.1055395526669);
#86794=CYLINDRICAL_SURFACE('',#99506,12.1055395526668);
#86795=CYLINDRICAL_SURFACE('',#99508,11.1055395526669);
#86796=CYLINDRICAL_SURFACE('',#99512,11.1055395526669);
#86797=CYLINDRICAL_SURFACE('',#99514,12.1055395526668);
#86798=CYLINDRICAL_SURFACE('',#99573,3.5);
#86799=CYLINDRICAL_SURFACE('',#99576,50.5);
#86800=CYLINDRICAL_SURFACE('',#99579,3.5);
#86801=CYLINDRICAL_SURFACE('',#99582,679.934816028482);
#86802=CYLINDRICAL_SURFACE('',#99585,3.5);
#86803=CYLINDRICAL_SURFACE('',#99588,50.5);
#86804=CYLINDRICAL_SURFACE('',#99591,3.49999999999996);
#86805=CYLINDRICAL_SURFACE('',#99602,74.6139048513169);
#86806=CYLINDRICAL_SURFACE('',#99607,74.6139048513167);
#86807=CYLINDRICAL_SURFACE('',#99610,8.5);
#86808=CYLINDRICAL_SURFACE('',#99613,8.5);
#86809=CYLINDRICAL_SURFACE('',#99616,55.5);
#86810=CYLINDRICAL_SURFACE('',#99619,8.5);
#86811=CYLINDRICAL_SURFACE('',#99622,684.934816028482);
#86812=CYLINDRICAL_SURFACE('',#99625,8.5);
#86813=CYLINDRICAL_SURFACE('',#99628,55.5);
#86814=CYLINDRICAL_SURFACE('',#99692,684.934816028482);
#86815=CYLINDRICAL_SURFACE('',#99694,684.934816028482);
#86816=CYLINDRICAL_SURFACE('',#99696,684.934816028482);
#86817=CYLINDRICAL_SURFACE('',#99698,684.934816028482);
#86818=CYLINDRICAL_SURFACE('',#99700,684.934816028482);
#86819=CYLINDRICAL_SURFACE('',#99706,1.);
#86820=CYLINDRICAL_SURFACE('',#99708,48.);
#86821=CYLINDRICAL_SURFACE('',#99710,0.999999999999999);
#86822=CYLINDRICAL_SURFACE('',#99712,677.434816028482);
#86823=CYLINDRICAL_SURFACE('',#99714,1.);
#86824=CYLINDRICAL_SURFACE('',#99716,48.);
#86825=CYLINDRICAL_SURFACE('',#99718,0.999999999999959);
#86826=CYLINDRICAL_SURFACE('',#99731,73.8);
#86827=CYLINDRICAL_SURFACE('',#99736,73.8);
#86828=CYLINDRICAL_SURFACE('',#99739,77.1139048513169);
#86829=CYLINDRICAL_SURFACE('',#99742,77.1139048513167);
#86830=CYLINDRICAL_SURFACE('',#99743,51.8);
#86831=CYLINDRICAL_SURFACE('',#99745,4.8);
#86832=CYLINDRICAL_SURFACE('',#99747,681.234816028482);
#86833=CYLINDRICAL_SURFACE('',#99749,4.8);
#86834=CYLINDRICAL_SURFACE('',#99751,51.8);
#86835=CYLINDRICAL_SURFACE('',#99753,4.8);
#86836=CYLINDRICAL_SURFACE('',#99755,4.8);
#86837=CYLINDRICAL_SURFACE('',#99757,5.99999999999992);
#86838=CYLINDRICAL_SURFACE('',#99759,6.);
#86839=CYLINDRICAL_SURFACE('',#99761,53.);
#86840=CYLINDRICAL_SURFACE('',#99763,6.);
#86841=CYLINDRICAL_SURFACE('',#99765,682.434816028482);
#86842=CYLINDRICAL_SURFACE('',#99767,6.);
#86843=CYLINDRICAL_SURFACE('',#99769,53.);
#86844=CYLINDRICAL_SURFACE('',#99794,677.434816028482);
#86845=CYLINDRICAL_SURFACE('',#99796,677.434816028482);
#86846=CYLINDRICAL_SURFACE('',#99798,677.434816028482);
#86847=CYLINDRICAL_SURFACE('',#99800,677.434816028482);
#86848=CYLINDRICAL_SURFACE('',#99802,677.434816028482);
#86849=CYLINDRICAL_SURFACE('',#99814,204.49569081556);
#86850=CYLINDRICAL_SURFACE('',#99816,677.434816028482);
#86851=CYLINDRICAL_SURFACE('',#99818,206.99569081556);
#86852=CYLINDRICAL_SURFACE('',#99835,204.49569081556);
#86853=CYLINDRICAL_SURFACE('',#99837,204.49569081556);
#86854=CYLINDRICAL_SURFACE('',#99839,677.434816028482);
#86855=CYLINDRICAL_SURFACE('',#99841,677.434816028482);
#86856=CYLINDRICAL_SURFACE('',#99843,48.);
#86857=CYLINDRICAL_SURFACE('',#99845,48.);
#86858=CYLINDRICAL_SURFACE('',#99847,48.);
#86859=CYLINDRICAL_SURFACE('',#99849,48.);
#86860=CYLINDRICAL_SURFACE('',#100018,0.75);
#86861=CYLINDRICAL_SURFACE('',#100031,0.75);
#86862=CYLINDRICAL_SURFACE('',#100032,0.75);
#86863=CYLINDRICAL_SURFACE('',#100044,0.750000000000001);
#86864=CYLINDRICAL_SURFACE('',#100045,0.750000000000001);
#86865=CYLINDRICAL_SURFACE('',#100057,0.749999999999998);
#86866=CYLINDRICAL_SURFACE('',#100058,0.749999999999999);
#86867=CYLINDRICAL_SURFACE('',#100070,0.75);
#86868=CYLINDRICAL_SURFACE('',#100071,1.5);
#86869=CYLINDRICAL_SURFACE('',#100072,1.5);
#86870=CYLINDRICAL_SURFACE('',#100073,1.5);
#86871=CYLINDRICAL_SURFACE('',#100074,1.5);
#86872=CYLINDRICAL_SURFACE('',#100075,1.49999999999999);
#86873=CYLINDRICAL_SURFACE('',#100076,1.5);
#86874=CYLINDRICAL_SURFACE('',#100077,1.5);
#86875=CYLINDRICAL_SURFACE('',#100078,1.5);
#86876=CYLINDRICAL_SURFACE('',#100084,0.450000000000006);
#86877=CYLINDRICAL_SURFACE('',#100098,0.449999999999999);
#86878=CYLINDRICAL_SURFACE('',#100112,0.450000000000006);
#86879=CYLINDRICAL_SURFACE('',#100118,0.450000000000006);
#86880=CYLINDRICAL_SURFACE('',#100132,0.449999999999999);
#86881=CYLINDRICAL_SURFACE('',#100134,0.450000000000006);
#86882=CYLINDRICAL_SURFACE('',#100144,0.450000000000006);
#86883=CYLINDRICAL_SURFACE('',#100158,0.449999999999999);
#86884=CYLINDRICAL_SURFACE('',#100160,0.450000000000001);
#86885=CYLINDRICAL_SURFACE('',#100170,0.450000000000006);
#86886=CYLINDRICAL_SURFACE('',#100172,0.449999999999999);
#86887=CYLINDRICAL_SURFACE('',#100182,0.450000000000001);
#86888=CYLINDRICAL_SURFACE('',#100184,0.450000000000001);
#86889=CYLINDRICAL_SURFACE('',#100194,0.450000000000006);
#86890=CYLINDRICAL_SURFACE('',#100196,0.450000000000001);
#86891=CYLINDRICAL_SURFACE('',#100210,0.450000000000001);
#86892=CYLINDRICAL_SURFACE('',#100224,0.450000000000006);
#86893=CYLINDRICAL_SURFACE('',#100226,0.450000000000001);
#86894=CYLINDRICAL_SURFACE('',#100236,0.45);
#86895=CYLINDRICAL_SURFACE('',#100238,0.450000000000006);
#86896=CYLINDRICAL_SURFACE('',#100248,0.450000000000006);
#86897=CYLINDRICAL_SURFACE('',#100250,0.449999999999999);
#86898=CYLINDRICAL_SURFACE('',#100260,0.450000000000001);
#86899=CYLINDRICAL_SURFACE('',#100262,0.450000000000006);
#86900=CYLINDRICAL_SURFACE('',#100272,0.450000000000006);
#86901=CYLINDRICAL_SURFACE('',#100274,0.449999999999999);
#86902=CYLINDRICAL_SURFACE('',#100284,0.450000000000001);
#86903=CYLINDRICAL_SURFACE('',#100286,0.450000000000006);
#86904=CYLINDRICAL_SURFACE('',#100296,0.450000000000006);
#86905=CYLINDRICAL_SURFACE('',#100298,0.450000000000001);
#86906=CYLINDRICAL_SURFACE('',#100308,0.45);
#86907=CYLINDRICAL_SURFACE('',#100310,0.450000000000006);
#86908=CYLINDRICAL_SURFACE('',#100320,0.450000000000006);
#86909=CYLINDRICAL_SURFACE('',#100322,0.450000000000001);
#86910=CYLINDRICAL_SURFACE('',#100332,0.45);
#86911=CYLINDRICAL_SURFACE('',#100346,0.450000000000006);
#86912=CYLINDRICAL_SURFACE('',#100348,0.449999999999999);
#86913=CYLINDRICAL_SURFACE('',#100358,0.450000000000001);
#86914=CYLINDRICAL_SURFACE('',#100380,0.450000000000006);
#86915=CYLINDRICAL_SURFACE('',#100382,0.45);
#86916=CYLINDRICAL_SURFACE('',#100392,0.450000000000001);
#86917=CYLINDRICAL_SURFACE('',#100406,0.450000000000006);
#86918=CYLINDRICAL_SURFACE('',#100408,0.45);
#86919=CYLINDRICAL_SURFACE('',#100418,0.450000000000001);
#86920=CYLINDRICAL_SURFACE('',#100420,0.450000000000006);
#86921=CYLINDRICAL_SURFACE('',#100430,0.450000000000001);
#86922=CYLINDRICAL_SURFACE('',#100444,0.450000000000006);
#86923=CYLINDRICAL_SURFACE('',#100446,0.450000000000006);
#86924=CYLINDRICAL_SURFACE('',#100456,0.45);
#86925=CYLINDRICAL_SURFACE('',#100462,0.449999999999999);
#86926=CYLINDRICAL_SURFACE('',#100464,0.450000000000006);
#86927=CYLINDRICAL_SURFACE('',#100474,0.450000000000006);
#86928=CYLINDRICAL_SURFACE('',#100488,0.450000000000001);
#86929=CYLINDRICAL_SURFACE('',#100494,0.449999999999999);
#86930=CYLINDRICAL_SURFACE('',#100496,0.450000000000006);
#86931=CYLINDRICAL_SURFACE('',#100506,0.450000000000006);
#86932=CYLINDRICAL_SURFACE('',#100508,0.450000000000001);
#86933=CYLINDRICAL_SURFACE('',#100518,0.449999999999999);
#86934=CYLINDRICAL_SURFACE('',#100520,0.450000000000006);
#86935=CYLINDRICAL_SURFACE('',#100534,0.450000000000001);
#86936=CYLINDRICAL_SURFACE('',#100544,0.449999999999999);
#86937=CYLINDRICAL_SURFACE('',#100546,0.450000000000006);
#86938=CYLINDRICAL_SURFACE('',#100556,0.450000000000006);
#86939=CYLINDRICAL_SURFACE('',#100558,0.449999999999999);
#86940=CYLINDRICAL_SURFACE('',#100568,0.449999999999999);
#86941=CYLINDRICAL_SURFACE('',#100570,0.450000000000006);
#86942=CYLINDRICAL_SURFACE('',#100580,0.450000000000006);
#86943=CYLINDRICAL_SURFACE('',#100582,0.449999999999999);
#86944=CYLINDRICAL_SURFACE('',#100592,0.449999999999999);
#86945=CYLINDRICAL_SURFACE('',#100594,0.450000000000006);
#86946=CYLINDRICAL_SURFACE('',#100604,0.450000000000001);
#86947=CYLINDRICAL_SURFACE('',#100622,0.449999999999999);
#86948=CYLINDRICAL_SURFACE('',#100624,0.450000000000006);
#86949=CYLINDRICAL_SURFACE('',#100638,0.449999999999999);
#86950=CYLINDRICAL_SURFACE('',#100648,0.449999999999999);
#86951=CYLINDRICAL_SURFACE('',#100650,0.450000000000006);
#86952=CYLINDRICAL_SURFACE('',#100664,0.449999999999999);
#86953=CYLINDRICAL_SURFACE('',#100682,0.449999999999999);
#86954=CYLINDRICAL_SURFACE('',#100684,0.450000000000006);
#86955=CYLINDRICAL_SURFACE('',#100694,0.450000000000006);
#86956=CYLINDRICAL_SURFACE('',#100696,0.449999999999999);
#86957=CYLINDRICAL_SURFACE('',#100706,0.449999999999999);
#86958=CYLINDRICAL_SURFACE('',#100708,0.450000000000006);
#86959=CYLINDRICAL_SURFACE('',#100718,0.450000000000006);
#86960=CYLINDRICAL_SURFACE('',#100740,0.449999999999999);
#86961=CYLINDRICAL_SURFACE('',#100742,0.450000000000006);
#86962=CYLINDRICAL_SURFACE('',#100752,0.450000000000006);
#86963=CYLINDRICAL_SURFACE('',#100766,0.449999999999999);
#86964=CYLINDRICAL_SURFACE('',#100768,0.450000000000006);
#86965=CYLINDRICAL_SURFACE('',#100778,0.450000000000006);
#86966=CYLINDRICAL_SURFACE('',#100780,0.449999999999999);
#86967=CYLINDRICAL_SURFACE('',#100790,0.449999999999999);
#86968=CYLINDRICAL_SURFACE('',#100792,0.450000000000001);
#86969=CYLINDRICAL_SURFACE('',#100802,0.450000000000006);
#86970=CYLINDRICAL_SURFACE('',#100816,0.449999999999999);
#86971=CYLINDRICAL_SURFACE('',#100818,0.450000000000006);
#86972=CYLINDRICAL_SURFACE('',#100828,0.450000000000001);
#86973=CYLINDRICAL_SURFACE('',#100830,0.449999999999999);
#86974=CYLINDRICAL_SURFACE('',#100840,0.449999999999999);
#86975=CYLINDRICAL_SURFACE('',#100854,0.450000000000006);
#86976=CYLINDRICAL_SURFACE('',#100860,0.450000000000006);
#86977=CYLINDRICAL_SURFACE('',#100874,0.449999999999999);
#86978=CYLINDRICAL_SURFACE('',#100957,0.44999999999999);
#86979=CYLINDRICAL_SURFACE('',#100971,0.450000000000001);
#86980=CYLINDRICAL_SURFACE('',#100980,0.450000000000001);
#86981=CYLINDRICAL_SURFACE('',#100994,0.45);
#86982=CYLINDRICAL_SURFACE('',#101003,0.450000000000006);
#86983=CYLINDRICAL_SURFACE('',#101017,0.44999999999999);
#86984=CYLINDRICAL_SURFACE('',#101026,0.45);
#86985=CYLINDRICAL_SURFACE('',#101040,0.450000000000006);
#86986=CYLINDRICAL_SURFACE('',#101154,0.75);
#86987=CYLINDRICAL_SURFACE('',#101156,0.750000000000001);
#86988=CYLINDRICAL_SURFACE('',#101158,0.750000000000001);
#86989=CYLINDRICAL_SURFACE('',#101160,0.750000000000001);
#86990=CYLINDRICAL_SURFACE('',#101162,0.750000000000001);
#86991=CYLINDRICAL_SURFACE('',#101164,0.750000000000001);
#86992=CYLINDRICAL_SURFACE('',#101166,0.75);
#86993=CYLINDRICAL_SURFACE('',#101168,0.75);
#86994=CYLINDRICAL_SURFACE('',#101170,0.75);
#86995=CYLINDRICAL_SURFACE('',#101172,0.750000000000001);
#86996=CYLINDRICAL_SURFACE('',#101174,0.750000000000001);
#86997=CYLINDRICAL_SURFACE('',#101176,0.750000000000001);
#86998=CYLINDRICAL_SURFACE('',#101178,0.750000000000001);
#86999=CYLINDRICAL_SURFACE('',#101180,0.750000000000001);
#87000=CYLINDRICAL_SURFACE('',#101182,0.750000000000001);
#87001=CYLINDRICAL_SURFACE('',#101184,0.750000000000001);
#87002=CYLINDRICAL_SURFACE('',#101186,0.75);
#87003=CYLINDRICAL_SURFACE('',#101188,0.75);
#87004=CYLINDRICAL_SURFACE('',#101190,0.75);
#87005=CYLINDRICAL_SURFACE('',#101192,0.75);
#87006=CYLINDRICAL_SURFACE('',#101194,0.750000000000001);
#87007=CYLINDRICAL_SURFACE('',#101196,0.75);
#87008=CYLINDRICAL_SURFACE('',#101198,0.750000000000001);
#87009=CYLINDRICAL_SURFACE('',#101200,0.750000000000001);
#87010=CYLINDRICAL_SURFACE('',#101202,0.750000000000001);
#87011=CYLINDRICAL_SURFACE('',#101204,0.750000000000001);
#87012=CYLINDRICAL_SURFACE('',#101206,0.750000000000001);
#87013=CYLINDRICAL_SURFACE('',#101208,0.750000000000001);
#87014=CYLINDRICAL_SURFACE('',#101210,0.750000000000001);
#87015=CYLINDRICAL_SURFACE('',#101212,0.750000000000001);
#87016=CYLINDRICAL_SURFACE('',#101214,0.750000000000001);
#87017=CYLINDRICAL_SURFACE('',#101216,0.750000000000001);
#87018=CYLINDRICAL_SURFACE('',#101218,0.75);
#87019=CYLINDRICAL_SURFACE('',#101220,0.750000000000001);
#87020=CYLINDRICAL_SURFACE('',#101222,0.75);
#87021=CYLINDRICAL_SURFACE('',#101224,0.75);
#87022=CYLINDRICAL_SURFACE('',#101226,0.750000000000001);
#87023=CYLINDRICAL_SURFACE('',#101228,0.750000000000001);
#87024=CYLINDRICAL_SURFACE('',#101230,0.750000000000001);
#87025=CYLINDRICAL_SURFACE('',#101232,0.750000000000001);
#87026=CYLINDRICAL_SURFACE('',#101234,0.750000000000001);
#87027=CYLINDRICAL_SURFACE('',#101236,0.750000000000001);
#87028=CYLINDRICAL_SURFACE('',#101238,0.750000000000001);
#87029=CYLINDRICAL_SURFACE('',#101240,0.750000000000001);
#87030=CYLINDRICAL_SURFACE('',#101242,0.75);
#87031=CYLINDRICAL_SURFACE('',#101244,0.75);
#87032=CYLINDRICAL_SURFACE('',#101246,0.750000000000001);
#87033=CYLINDRICAL_SURFACE('',#101248,0.750000000000001);
#87034=CYLINDRICAL_SURFACE('',#101250,0.750000000000001);
#87035=CYLINDRICAL_SURFACE('',#101252,0.750000000000001);
#87036=CYLINDRICAL_SURFACE('',#101254,0.750000000000001);
#87037=CYLINDRICAL_SURFACE('',#101256,0.750000000000001);
#87038=CYLINDRICAL_SURFACE('',#101258,0.750000000000001);
#87039=CYLINDRICAL_SURFACE('',#101260,0.750000000000001);
#87040=CYLINDRICAL_SURFACE('',#101262,0.750000000000001);
#87041=CYLINDRICAL_SURFACE('',#101264,0.750000000000001);
#87042=CYLINDRICAL_SURFACE('',#101266,0.750000000000001);
#87043=CYLINDRICAL_SURFACE('',#101268,0.750000000000001);
#87044=CYLINDRICAL_SURFACE('',#101270,0.750000000000001);
#87045=CYLINDRICAL_SURFACE('',#101272,0.750000000000001);
#87046=CYLINDRICAL_SURFACE('',#101274,0.750000000000001);
#87047=CYLINDRICAL_SURFACE('',#101276,0.750000000000001);
#87048=CYLINDRICAL_SURFACE('',#101278,0.750000000000001);
#87049=CYLINDRICAL_SURFACE('',#101280,0.750000000000001);
#87050=CYLINDRICAL_SURFACE('',#101282,0.750000000000001);
#87051=CYLINDRICAL_SURFACE('',#101284,0.750000000000001);
#87052=CYLINDRICAL_SURFACE('',#101286,0.750000000000001);
#87053=CYLINDRICAL_SURFACE('',#101288,0.750000000000001);
#87054=CYLINDRICAL_SURFACE('',#101290,0.750000000000001);
#87055=CYLINDRICAL_SURFACE('',#101292,0.750000000000001);
#87056=CYLINDRICAL_SURFACE('',#101294,0.750000000000001);
#87057=CYLINDRICAL_SURFACE('',#101296,0.75);
#87058=CYLINDRICAL_SURFACE('',#101298,0.750000000000001);
#87059=CYLINDRICAL_SURFACE('',#101300,0.750000000000001);
#87060=CYLINDRICAL_SURFACE('',#101302,0.75);
#87061=CYLINDRICAL_SURFACE('',#101304,0.750000000000001);
#87062=CYLINDRICAL_SURFACE('',#101306,0.75);
#87063=CYLINDRICAL_SURFACE('',#101308,0.75);
#87064=CYLINDRICAL_SURFACE('',#101310,0.750000000000001);
#87065=CYLINDRICAL_SURFACE('',#101312,0.750000000000001);
#87066=CYLINDRICAL_SURFACE('',#101314,0.750000000000001);
#87067=CYLINDRICAL_SURFACE('',#101316,0.750000000000001);
#87068=CYLINDRICAL_SURFACE('',#101318,0.750000000000001);
#87069=CYLINDRICAL_SURFACE('',#101320,0.750000000000001);
#87070=CYLINDRICAL_SURFACE('',#101322,0.750000000000001);
#87071=CYLINDRICAL_SURFACE('',#101324,0.750000000000001);
#87072=CYLINDRICAL_SURFACE('',#101326,0.750000000000001);
#87073=CYLINDRICAL_SURFACE('',#101328,0.750000000000001);
#87074=CYLINDRICAL_SURFACE('',#101330,0.750000000000001);
#87075=CYLINDRICAL_SURFACE('',#101332,0.750000000000001);
#87076=CYLINDRICAL_SURFACE('',#101334,0.750000000000001);
#87077=CYLINDRICAL_SURFACE('',#101336,0.750000000000001);
#87078=CYLINDRICAL_SURFACE('',#101338,0.750000000000001);
#87079=CYLINDRICAL_SURFACE('',#101340,0.750000000000001);
#87080=CYLINDRICAL_SURFACE('',#101342,0.750000000000001);
#87081=CYLINDRICAL_SURFACE('',#101344,0.75);
#87082=CYLINDRICAL_SURFACE('',#101346,0.750000000000001);
#87083=CYLINDRICAL_SURFACE('',#101348,0.75);
#87084=CYLINDRICAL_SURFACE('',#101350,0.75);
#87085=CYLINDRICAL_SURFACE('',#101352,0.750000000000001);
#87086=CYLINDRICAL_SURFACE('',#101354,0.750000000000001);
#87087=CYLINDRICAL_SURFACE('',#101356,0.750000000000001);
#87088=CYLINDRICAL_SURFACE('',#101358,0.750000000000001);
#87089=CYLINDRICAL_SURFACE('',#101360,0.750000000000001);
#87090=CYLINDRICAL_SURFACE('',#101362,0.750000000000001);
#87091=CYLINDRICAL_SURFACE('',#101364,0.750000000000001);
#87092=CYLINDRICAL_SURFACE('',#101366,0.750000000000001);
#87093=CYLINDRICAL_SURFACE('',#101368,0.750000000000001);
#87094=CYLINDRICAL_SURFACE('',#101370,0.750000000000001);
#87095=CYLINDRICAL_SURFACE('',#101372,0.750000000000001);
#87096=CYLINDRICAL_SURFACE('',#101374,0.750000000000001);
#87097=CYLINDRICAL_SURFACE('',#101376,0.750000000000001);
#87098=CYLINDRICAL_SURFACE('',#101378,0.750000000000001);
#87099=CYLINDRICAL_SURFACE('',#101380,0.750000000000001);
#87100=CYLINDRICAL_SURFACE('',#101382,0.750000000000001);
#87101=CYLINDRICAL_SURFACE('',#101384,0.750000000000001);
#87102=CYLINDRICAL_SURFACE('',#101386,0.750000000000001);
#87103=CYLINDRICAL_SURFACE('',#101388,0.750000000000001);
#87104=CYLINDRICAL_SURFACE('',#101390,0.750000000000001);
#87105=CYLINDRICAL_SURFACE('',#101392,0.750000000000001);
#87106=CYLINDRICAL_SURFACE('',#101394,0.750000000000001);
#87107=CYLINDRICAL_SURFACE('',#101396,0.750000000000001);
#87108=CYLINDRICAL_SURFACE('',#101398,0.750000000000001);
#87109=CYLINDRICAL_SURFACE('',#101400,0.750000000000001);
#87110=CYLINDRICAL_SURFACE('',#101402,0.750000000000001);
#87111=CYLINDRICAL_SURFACE('',#101404,0.750000000000001);
#87112=CYLINDRICAL_SURFACE('',#101406,0.750000000000001);
#87113=CYLINDRICAL_SURFACE('',#101408,0.750000000000001);
#87114=CYLINDRICAL_SURFACE('',#101410,0.750000000000001);
#87115=CYLINDRICAL_SURFACE('',#101412,0.75);
#87116=CYLINDRICAL_SURFACE('',#101414,0.75);
#87117=CYLINDRICAL_SURFACE('',#101416,0.750000000000001);
#87118=CYLINDRICAL_SURFACE('',#101418,0.750000000000001);
#87119=CYLINDRICAL_SURFACE('',#101420,0.750000000000001);
#87120=CYLINDRICAL_SURFACE('',#101422,10.);
#87121=CYLINDRICAL_SURFACE('',#101424,10.);
#87122=CYLINDRICAL_SURFACE('',#101426,10.);
#87123=CYLINDRICAL_SURFACE('',#101428,10.);
#87124=CYLINDRICAL_SURFACE('',#101432,4.62535);
#87125=CYLINDRICAL_SURFACE('',#101434,13.1055395526668);
#87126=CYLINDRICAL_SURFACE('',#101436,13.1055395526668);
#87127=CYLINDRICAL_SURFACE('',#101438,8.10553955266686);
#87128=CYLINDRICAL_SURFACE('',#101456,11.1055395526669);
#87129=CYLINDRICAL_SURFACE('',#101460,11.1055395526669);
#87130=CYLINDRICAL_SURFACE('',#101462,12.1055395526668);
#87131=CYLINDRICAL_SURFACE('',#101464,11.1055395526669);
#87132=CYLINDRICAL_SURFACE('',#101468,11.1055395526669);
#87133=CYLINDRICAL_SURFACE('',#101470,12.1055395526668);
#87134=CYLINDRICAL_SURFACE('',#101562,3.5);
#87135=CYLINDRICAL_SURFACE('',#101564,50.5);
#87136=CYLINDRICAL_SURFACE('',#101566,3.5);
#87137=CYLINDRICAL_SURFACE('',#101568,679.934816028482);
#87138=CYLINDRICAL_SURFACE('',#101570,3.5);
#87139=CYLINDRICAL_SURFACE('',#101572,50.5);
#87140=CYLINDRICAL_SURFACE('',#101574,3.49999999999996);
#87141=CYLINDRICAL_SURFACE('',#101576,679.934816028482);
#87142=CYLINDRICAL_SURFACE('',#101586,74.6139048513169);
#87143=CYLINDRICAL_SURFACE('',#101591,74.6139048513167);
#87144=CYLINDRICAL_SURFACE('',#101594,8.5);
#87145=CYLINDRICAL_SURFACE('',#101597,684.934816028482);
#87146=CYLINDRICAL_SURFACE('',#101600,211.99569081556);
#87147=CYLINDRICAL_SURFACE('',#101605,8.5);
#87148=CYLINDRICAL_SURFACE('',#101608,55.5);
#87149=CYLINDRICAL_SURFACE('',#101611,8.5);
#87150=CYLINDRICAL_SURFACE('',#101614,684.934816028482);
#87151=CYLINDRICAL_SURFACE('',#101617,8.5);
#87152=CYLINDRICAL_SURFACE('',#101620,55.5);
#87153=CYLINDRICAL_SURFACE('',#101695,684.934816028482);
#87154=CYLINDRICAL_SURFACE('',#101697,684.934816028482);
#87155=CYLINDRICAL_SURFACE('',#101699,684.934816028482);
#87156=CYLINDRICAL_SURFACE('',#101701,684.934816028482);
#87157=CYLINDRICAL_SURFACE('',#101703,684.934816028482);
#87158=CYLINDRICAL_SURFACE('',#101709,1.);
#87159=CYLINDRICAL_SURFACE('',#101710,48.);
#87160=CYLINDRICAL_SURFACE('',#101711,0.999999999999999);
#87161=CYLINDRICAL_SURFACE('',#101712,677.434816028482);
#87162=CYLINDRICAL_SURFACE('',#101713,1.);
#87163=CYLINDRICAL_SURFACE('',#101714,48.);
#87164=CYLINDRICAL_SURFACE('',#101715,0.999999999999959);
#87165=CYLINDRICAL_SURFACE('',#101725,73.8);
#87166=CYLINDRICAL_SURFACE('',#101729,73.8);
#87167=CYLINDRICAL_SURFACE('',#101732,77.1139048513169);
#87168=CYLINDRICAL_SURFACE('',#101735,77.1139048513167);
#87169=CYLINDRICAL_SURFACE('',#101737,51.8);
#87170=CYLINDRICAL_SURFACE('',#101739,4.8);
#87171=CYLINDRICAL_SURFACE('',#101741,681.234816028482);
#87172=CYLINDRICAL_SURFACE('',#101743,4.8);
#87173=CYLINDRICAL_SURFACE('',#101745,51.8);
#87174=CYLINDRICAL_SURFACE('',#101747,4.8);
#87175=CYLINDRICAL_SURFACE('',#101749,681.234816028482);
#87176=CYLINDRICAL_SURFACE('',#101751,208.29569081556);
#87177=CYLINDRICAL_SURFACE('',#101753,4.8);
#87178=CYLINDRICAL_SURFACE('',#101765,5.99999999999992);
#87179=CYLINDRICAL_SURFACE('',#101766,682.434816028482);
#87180=CYLINDRICAL_SURFACE('',#101767,209.495690815561);
#87181=CYLINDRICAL_SURFACE('',#101768,6.);
#87182=CYLINDRICAL_SURFACE('',#101769,53.);
#87183=CYLINDRICAL_SURFACE('',#101770,6.);
#87184=CYLINDRICAL_SURFACE('',#101771,682.434816028482);
#87185=CYLINDRICAL_SURFACE('',#101772,6.);
#87186=CYLINDRICAL_SURFACE('',#101773,53.);
#87187=CYLINDRICAL_SURFACE('',#101806,677.434816028482);
#87188=CYLINDRICAL_SURFACE('',#101807,677.434816028482);
#87189=CYLINDRICAL_SURFACE('',#101808,677.434816028482);
#87190=CYLINDRICAL_SURFACE('',#101809,677.434816028482);
#87191=CYLINDRICAL_SURFACE('',#101810,677.434816028482);
#87192=CYLINDRICAL_SURFACE('',#101821,204.49569081556);
#87193=CYLINDRICAL_SURFACE('',#101822,677.434816028482);
#87194=CYLINDRICAL_SURFACE('',#101823,206.99569081556);
#87195=CYLINDRICAL_SURFACE('',#101825,206.99569081556);
#87196=CYLINDRICAL_SURFACE('',#101842,204.49569081556);
#87197=CYLINDRICAL_SURFACE('',#101843,204.49569081556);
#87198=CYLINDRICAL_SURFACE('',#101844,677.434816028482);
#87199=CYLINDRICAL_SURFACE('',#101845,677.434816028482);
#87200=CYLINDRICAL_SURFACE('',#101846,48.);
#87201=CYLINDRICAL_SURFACE('',#101847,48.);
#87202=CYLINDRICAL_SURFACE('',#101848,48.);
#87203=CYLINDRICAL_SURFACE('',#101849,48.);
#87204=CYLINDRICAL_SURFACE('',#101906,3.25);
#87205=CYLINDRICAL_SURFACE('',#101998,3.25);
#87206=CYLINDRICAL_SURFACE('',#102021,7.8);
#87207=CYLINDRICAL_SURFACE('',#102023,8.8);
#87208=CYLINDRICAL_SURFACE('',#102029,2.);
#87209=CYLINDRICAL_SURFACE('',#102033,2.5);
#87210=CYLINDRICAL_SURFACE('',#102041,0.5);
#87211=CYLINDRICAL_SURFACE('',#102043,0.5);
#87212=CYLINDRICAL_SURFACE('',#102053,0.5);
#87213=CYLINDRICAL_SURFACE('',#102055,0.5);
#87214=CYLINDRICAL_SURFACE('',#102061,7.00000000000001);
#87215=CYLINDRICAL_SURFACE('',#102063,7.00000000000001);
#87216=CYLINDRICAL_SURFACE('',#102073,1.);
#87217=CYLINDRICAL_SURFACE('',#102079,4.);
#87218=CYLINDRICAL_SURFACE('',#102090,1.);
#87219=CYLINDRICAL_SURFACE('',#102091,4.);
#87220=CYLINDRICAL_SURFACE('',#102092,4.);
#87221=CYLINDRICAL_SURFACE('',#102095,1.);
#87222=CYLINDRICAL_SURFACE('',#102105,4.);
#87223=CYLINDRICAL_SURFACE('',#102111,1.);
#87224=CYLINDRICAL_SURFACE('',#102119,7.00000000000001);
#87225=CYLINDRICAL_SURFACE('',#102121,7.00000000000001);
#87226=CYLINDRICAL_SURFACE('',#102123,1.);
#87227=CYLINDRICAL_SURFACE('',#102125,1.);
#87228=CYLINDRICAL_SURFACE('',#102127,1.);
#87229=CYLINDRICAL_SURFACE('',#102129,1.);
#87230=CYLINDRICAL_SURFACE('',#102133,7.8);
#87231=CYLINDRICAL_SURFACE('',#102134,7.8);
#87232=CYLINDRICAL_SURFACE('',#102159,7.8);
#87233=CYLINDRICAL_SURFACE('',#102161,8.8);
#87234=CYLINDRICAL_SURFACE('',#102163,0.499999999999998);
#87235=CYLINDRICAL_SURFACE('',#102169,0.5);
#87236=CYLINDRICAL_SURFACE('',#102175,0.5);
#87237=CYLINDRICAL_SURFACE('',#102176,0.5);
#87238=CYLINDRICAL_SURFACE('',#102183,0.5);
#87239=CYLINDRICAL_SURFACE('',#102189,0.499999999999998);
#87240=CYLINDRICAL_SURFACE('',#102190,0.5);
#87241=CYLINDRICAL_SURFACE('',#102197,0.5);
#87242=CYLINDRICAL_SURFACE('',#102203,0.5);
#87243=CYLINDRICAL_SURFACE('',#102209,0.5);
#87244=CYLINDRICAL_SURFACE('',#102215,0.5);
#87245=CYLINDRICAL_SURFACE('',#102217,0.5);
#87246=CYLINDRICAL_SURFACE('',#102224,0.5);
#87247=CYLINDRICAL_SURFACE('',#102230,0.500000000000003);
#87248=CYLINDRICAL_SURFACE('',#102231,0.5);
#87249=CYLINDRICAL_SURFACE('',#102238,0.5);
#87250=CYLINDRICAL_SURFACE('',#102248,0.5);
#87251=CYLINDRICAL_SURFACE('',#102254,0.5);
#87252=CYLINDRICAL_SURFACE('',#102260,0.5);
#87253=CYLINDRICAL_SURFACE('',#102262,0.5);
#87254=CYLINDRICAL_SURFACE('',#102269,0.5);
#87255=CYLINDRICAL_SURFACE('',#102283,0.5);
#87256=CYLINDRICAL_SURFACE('',#102289,0.5);
#87257=CYLINDRICAL_SURFACE('',#102291,0.5);
#87258=CYLINDRICAL_SURFACE('',#102298,0.5);
#87259=CYLINDRICAL_SURFACE('',#102312,0.5);
#87260=CYLINDRICAL_SURFACE('',#102318,0.5);
#87261=CYLINDRICAL_SURFACE('',#102320,0.5);
#87262=CYLINDRICAL_SURFACE('',#102327,0.5);
#87263=CYLINDRICAL_SURFACE('',#102341,0.5);
#87264=CYLINDRICAL_SURFACE('',#102347,0.5);
#87265=CYLINDRICAL_SURFACE('',#102349,0.5);
#87266=CYLINDRICAL_SURFACE('',#102356,0.5);
#87267=CYLINDRICAL_SURFACE('',#102370,0.5);
#87268=CYLINDRICAL_SURFACE('',#102376,0.5);
#87269=CYLINDRICAL_SURFACE('',#102378,0.5);
#87270=CYLINDRICAL_SURFACE('',#102385,0.5);
#87271=CYLINDRICAL_SURFACE('',#102399,0.5);
#87272=CYLINDRICAL_SURFACE('',#102405,0.5);
#87273=CYLINDRICAL_SURFACE('',#102407,0.5);
#87274=CYLINDRICAL_SURFACE('',#102414,0.5);
#87275=CYLINDRICAL_SURFACE('',#102428,0.5);
#87276=CYLINDRICAL_SURFACE('',#102434,0.5);
#87277=CYLINDRICAL_SURFACE('',#102436,0.5);
#87278=CYLINDRICAL_SURFACE('',#102443,0.5);
#87279=CYLINDRICAL_SURFACE('',#102449,0.5);
#87280=CYLINDRICAL_SURFACE('',#102459,0.5);
#87281=CYLINDRICAL_SURFACE('',#102465,0.5);
#87282=CYLINDRICAL_SURFACE('',#102467,0.5);
#87283=CYLINDRICAL_SURFACE('',#102474,0.5);
#87284=CYLINDRICAL_SURFACE('',#102480,0.5);
#87285=CYLINDRICAL_SURFACE('',#102486,0.5);
#87286=CYLINDRICAL_SURFACE('',#102492,0.5);
#87287=CYLINDRICAL_SURFACE('',#102494,0.499999999999998);
#87288=CYLINDRICAL_SURFACE('',#102500,0.5);
#87289=CYLINDRICAL_SURFACE('',#102506,0.5);
#87290=CYLINDRICAL_SURFACE('',#102508,0.5);
#87291=CYLINDRICAL_SURFACE('',#102510,0.5);
#87292=CYLINDRICAL_SURFACE('',#102512,0.5);
#87293=CYLINDRICAL_SURFACE('',#102514,0.5);
#87294=CYLINDRICAL_SURFACE('',#102516,0.5);
#87295=CYLINDRICAL_SURFACE('',#102518,0.5);
#87296=CYLINDRICAL_SURFACE('',#102520,0.5);
#87297=CYLINDRICAL_SURFACE('',#102522,0.5);
#87298=CYLINDRICAL_SURFACE('',#102524,0.5);
#87299=CYLINDRICAL_SURFACE('',#102526,0.5);
#87300=CYLINDRICAL_SURFACE('',#102528,0.5);
#87301=CYLINDRICAL_SURFACE('',#102530,0.5);
#87302=CYLINDRICAL_SURFACE('',#102532,0.5);
#87303=CYLINDRICAL_SURFACE('',#102534,0.5);
#87304=CYLINDRICAL_SURFACE('',#102536,0.5);
#87305=CYLINDRICAL_SURFACE('',#102538,0.5);
#87306=CYLINDRICAL_SURFACE('',#102540,0.5);
#87307=CYLINDRICAL_SURFACE('',#102542,0.5);
#87308=CYLINDRICAL_SURFACE('',#102544,0.5);
#87309=CYLINDRICAL_SURFACE('',#102546,0.5);
#87310=CYLINDRICAL_SURFACE('',#102548,0.5);
#87311=CYLINDRICAL_SURFACE('',#102550,0.5);
#87312=CYLINDRICAL_SURFACE('',#102552,0.5);
#87313=CYLINDRICAL_SURFACE('',#102554,0.5);
#87314=CYLINDRICAL_SURFACE('',#102556,0.5);
#87315=CYLINDRICAL_SURFACE('',#102558,0.5);
#87316=CYLINDRICAL_SURFACE('',#102565,231.99961917989);
#87317=CYLINDRICAL_SURFACE('',#102581,3.);
#87318=CYLINDRICAL_SURFACE('',#102582,58.5);
#87319=CYLINDRICAL_SURFACE('',#102587,3.);
#87320=CYLINDRICAL_SURFACE('',#102588,58.5);
#87321=CYLINDRICAL_SURFACE('',#102593,3.);
#87322=CYLINDRICAL_SURFACE('',#102594,58.5);
#87323=CYLINDRICAL_SURFACE('',#102599,3.);
#87324=CYLINDRICAL_SURFACE('',#102600,58.5);
#87325=CYLINDRICAL_SURFACE('',#102605,3.);
#87326=CYLINDRICAL_SURFACE('',#102607,5.);
#87327=CYLINDRICAL_SURFACE('',#102610,5.);
#87328=CYLINDRICAL_SURFACE('',#102620,3.);
#87329=CYLINDRICAL_SURFACE('',#102622,3.);
#87330=CYLINDRICAL_SURFACE('',#102624,3.);
#87331=CYLINDRICAL_SURFACE('',#102626,3.);
#87332=CYLINDRICAL_SURFACE('',#102628,58.5);
#87333=CYLINDRICAL_SURFACE('',#102629,3.);
#87334=CYLINDRICAL_SURFACE('',#102631,58.5);
#87335=CYLINDRICAL_SURFACE('',#102633,3.);
#87336=CYLINDRICAL_SURFACE('',#102640,77.1121191998622);
#87337=CYLINDRICAL_SURFACE('',#102644,77.1121191998622);
#87338=CYLINDRICAL_SURFACE('',#102736,3.25);
#87339=CYLINDRICAL_SURFACE('',#102737,0.749999999999997);
#87340=CYLINDRICAL_SURFACE('',#102740,0.75);
#87341=CYLINDRICAL_SURFACE('',#102747,0.750000000000001);
#87342=CYLINDRICAL_SURFACE('',#102776,0.499999999999987);
#87343=CYLINDRICAL_SURFACE('',#102779,0.500000000000001);
#87344=CYLINDRICAL_SURFACE('',#102784,0.749999999999997);
#87345=CYLINDRICAL_SURFACE('',#102787,0.75);
#87346=CYLINDRICAL_SURFACE('',#102794,0.750000000000001);
#87347=CYLINDRICAL_SURFACE('',#102823,0.499999999999987);
#87348=CYLINDRICAL_SURFACE('',#102826,0.500000000000001);
#87349=CYLINDRICAL_SURFACE('',#102833,0.750000000000001);
#87350=CYLINDRICAL_SURFACE('',#102836,0.750000000000001);
#87351=CYLINDRICAL_SURFACE('',#102842,0.750000000000001);
#87352=CYLINDRICAL_SURFACE('',#102843,0.750000000000001);
#87353=CYLINDRICAL_SURFACE('',#102849,0.750000000000001);
#87354=CYLINDRICAL_SURFACE('',#102850,7.00000000000001);
#87355=CYLINDRICAL_SURFACE('',#102852,7.00000000000001);
#87356=CYLINDRICAL_SURFACE('',#102857,0.750000000000001);
#87357=CYLINDRICAL_SURFACE('',#102860,0.750000000000001);
#87358=CYLINDRICAL_SURFACE('',#102861,0.750000000000001);
#87359=CYLINDRICAL_SURFACE('',#102867,0.750000000000001);
#87360=CYLINDRICAL_SURFACE('',#102868,0.750000000000001);
#87361=CYLINDRICAL_SURFACE('',#102874,0.750000000000001);
#87362=CYLINDRICAL_SURFACE('',#102878,7.00000000000001);
#87363=CYLINDRICAL_SURFACE('',#102879,7.00000000000001);
#87364=CYLINDRICAL_SURFACE('',#102880,2.);
#87365=CYLINDRICAL_SURFACE('',#102882,2.);
#87366=CYLINDRICAL_SURFACE('',#102883,2.);
#87367=CYLINDRICAL_SURFACE('',#102884,2.);
#87368=CYLINDRICAL_SURFACE('',#102885,2.);
#87369=CYLINDRICAL_SURFACE('',#102886,2.);
#87370=CYLINDRICAL_SURFACE('',#102887,2.);
#87371=CYLINDRICAL_SURFACE('',#102888,2.);
#87372=CYLINDRICAL_SURFACE('',#102889,2.);
#87373=CYLINDRICAL_SURFACE('',#102890,2.);
#87374=CYLINDRICAL_SURFACE('',#102891,2.);
#87375=CYLINDRICAL_SURFACE('',#102892,2.);
#87376=CYLINDRICAL_SURFACE('',#102893,2.);
#87377=CYLINDRICAL_SURFACE('',#102894,2.);
#87378=CYLINDRICAL_SURFACE('',#102895,2.);
#87379=CYLINDRICAL_SURFACE('',#102896,2.);
#87380=CYLINDRICAL_SURFACE('',#102897,2.);
#87381=CYLINDRICAL_SURFACE('',#102898,2.);
#87382=CYLINDRICAL_SURFACE('',#102899,2.);
#87383=CYLINDRICAL_SURFACE('',#102900,2.);
#87384=CYLINDRICAL_SURFACE('',#102902,2.);
#87385=CYLINDRICAL_SURFACE('',#102903,2.);
#87386=CYLINDRICAL_SURFACE('',#102904,2.);
#87387=CYLINDRICAL_SURFACE('',#102905,2.);
#87388=CYLINDRICAL_SURFACE('',#102906,2.);
#87389=CYLINDRICAL_SURFACE('',#102907,2.);
#87390=CYLINDRICAL_SURFACE('',#102908,2.);
#87391=CYLINDRICAL_SURFACE('',#102909,2.);
#87392=CYLINDRICAL_SURFACE('',#102910,2.);
#87393=CYLINDRICAL_SURFACE('',#102911,2.);
#87394=CYLINDRICAL_SURFACE('',#102912,2.);
#87395=CYLINDRICAL_SURFACE('',#102913,2.);
#87396=CYLINDRICAL_SURFACE('',#102914,2.);
#87397=CYLINDRICAL_SURFACE('',#102915,2.);
#87398=CYLINDRICAL_SURFACE('',#102916,2.);
#87399=CYLINDRICAL_SURFACE('',#102917,2.);
#87400=CYLINDRICAL_SURFACE('',#102918,2.);
#87401=CYLINDRICAL_SURFACE('',#102919,2.);
#87402=CYLINDRICAL_SURFACE('',#102920,1.66874528305244);
#87403=CYLINDRICAL_SURFACE('',#102921,1.66874528305244);
#87404=CYLINDRICAL_SURFACE('',#102922,1.66874528305244);
#87405=CYLINDRICAL_SURFACE('',#102923,1.66874528305244);
#87406=CYLINDRICAL_SURFACE('',#102924,1.66874528305244);
#87407=CYLINDRICAL_SURFACE('',#102925,1.66874528305244);
#87408=CYLINDRICAL_SURFACE('',#102926,1.66874528305244);
#87409=CYLINDRICAL_SURFACE('',#102927,1.66874528305244);
#87410=CYLINDRICAL_SURFACE('',#102928,1.66874528305244);
#87411=CYLINDRICAL_SURFACE('',#102929,1.66874528305244);
#87412=CYLINDRICAL_SURFACE('',#102930,1.66874528305244);
#87413=CYLINDRICAL_SURFACE('',#102931,1.66874528305244);
#87414=CYLINDRICAL_SURFACE('',#102932,1.66874528305244);
#87415=CYLINDRICAL_SURFACE('',#102933,1.66874528305244);
#87416=CYLINDRICAL_SURFACE('',#102934,1.66874528305244);
#87417=CYLINDRICAL_SURFACE('',#102935,1.66874528305244);
#87418=CYLINDRICAL_SURFACE('',#102936,1.66874528305244);
#87419=CYLINDRICAL_SURFACE('',#102937,1.66874528305244);
#87420=CYLINDRICAL_SURFACE('',#102938,1.66874528305244);
#87421=CYLINDRICAL_SURFACE('',#102940,2.);
#87422=CYLINDRICAL_SURFACE('',#102942,2.);
#87423=CYLINDRICAL_SURFACE('',#102943,2.);
#87424=CYLINDRICAL_SURFACE('',#102944,2.);
#87425=CYLINDRICAL_SURFACE('',#102945,2.);
#87426=CYLINDRICAL_SURFACE('',#102946,2.);
#87427=CYLINDRICAL_SURFACE('',#102947,2.);
#87428=CYLINDRICAL_SURFACE('',#102948,2.);
#87429=CYLINDRICAL_SURFACE('',#102949,2.);
#87430=CYLINDRICAL_SURFACE('',#102950,2.);
#87431=CYLINDRICAL_SURFACE('',#102951,2.);
#87432=CYLINDRICAL_SURFACE('',#102952,2.);
#87433=CYLINDRICAL_SURFACE('',#102953,2.);
#87434=CYLINDRICAL_SURFACE('',#102954,2.);
#87435=CYLINDRICAL_SURFACE('',#102955,2.);
#87436=CYLINDRICAL_SURFACE('',#102956,2.);
#87437=CYLINDRICAL_SURFACE('',#102957,2.);
#87438=CYLINDRICAL_SURFACE('',#102958,2.);
#87439=CYLINDRICAL_SURFACE('',#102960,1.66874528305248);
#87440=CYLINDRICAL_SURFACE('',#102961,1.66874528305248);
#87441=CYLINDRICAL_SURFACE('',#102962,1.66874528305248);
#87442=CYLINDRICAL_SURFACE('',#102963,1.66874528305248);
#87443=CYLINDRICAL_SURFACE('',#102964,1.66874528305248);
#87444=CYLINDRICAL_SURFACE('',#102965,1.66874528305248);
#87445=CYLINDRICAL_SURFACE('',#102966,1.66874528305248);
#87446=CYLINDRICAL_SURFACE('',#102967,1.66874528305248);
#87447=CYLINDRICAL_SURFACE('',#102968,1.66874528305248);
#87448=CYLINDRICAL_SURFACE('',#102969,1.66874528305248);
#87449=CYLINDRICAL_SURFACE('',#102970,1.66874528305248);
#87450=CYLINDRICAL_SURFACE('',#102971,1.66874528305248);
#87451=CYLINDRICAL_SURFACE('',#102972,1.66874528305248);
#87452=CYLINDRICAL_SURFACE('',#102973,1.66874528305248);
#87453=CYLINDRICAL_SURFACE('',#102974,1.66874528305248);
#87454=CYLINDRICAL_SURFACE('',#102975,1.66874528305248);
#87455=CYLINDRICAL_SURFACE('',#102976,1.66874528305248);
#87456=CYLINDRICAL_SURFACE('',#102977,1.66874528305248);
#87457=CYLINDRICAL_SURFACE('',#102978,1.66874528305248);
#87458=CYLINDRICAL_SURFACE('',#102980,2.);
#87459=CYLINDRICAL_SURFACE('',#102982,2.);
#87460=CYLINDRICAL_SURFACE('',#102983,2.);
#87461=CYLINDRICAL_SURFACE('',#102984,2.);
#87462=CYLINDRICAL_SURFACE('',#102985,2.);
#87463=CYLINDRICAL_SURFACE('',#102986,2.);
#87464=CYLINDRICAL_SURFACE('',#102987,2.);
#87465=CYLINDRICAL_SURFACE('',#102988,2.);
#87466=CYLINDRICAL_SURFACE('',#102989,2.);
#87467=CYLINDRICAL_SURFACE('',#102990,2.);
#87468=CYLINDRICAL_SURFACE('',#102991,2.);
#87469=CYLINDRICAL_SURFACE('',#102992,2.);
#87470=CYLINDRICAL_SURFACE('',#102993,2.);
#87471=CYLINDRICAL_SURFACE('',#102994,2.);
#87472=CYLINDRICAL_SURFACE('',#102995,2.);
#87473=CYLINDRICAL_SURFACE('',#102996,2.);
#87474=CYLINDRICAL_SURFACE('',#102997,2.);
#87475=CYLINDRICAL_SURFACE('',#102998,2.);
#87476=CYLINDRICAL_SURFACE('',#102999,2.);
#87477=CYLINDRICAL_SURFACE('',#103000,1.66874528305242);
#87478=CYLINDRICAL_SURFACE('',#103001,1.66874528305242);
#87479=CYLINDRICAL_SURFACE('',#103002,1.66874528305242);
#87480=CYLINDRICAL_SURFACE('',#103003,1.66874528305242);
#87481=CYLINDRICAL_SURFACE('',#103004,1.66874528305242);
#87482=CYLINDRICAL_SURFACE('',#103005,1.66874528305242);
#87483=CYLINDRICAL_SURFACE('',#103006,1.66874528305242);
#87484=CYLINDRICAL_SURFACE('',#103007,1.66874528305242);
#87485=CYLINDRICAL_SURFACE('',#103008,1.66874528305242);
#87486=CYLINDRICAL_SURFACE('',#103009,1.66874528305242);
#87487=CYLINDRICAL_SURFACE('',#103010,1.66874528305242);
#87488=CYLINDRICAL_SURFACE('',#103011,1.66874528305242);
#87489=CYLINDRICAL_SURFACE('',#103012,1.66874528305242);
#87490=CYLINDRICAL_SURFACE('',#103013,1.66874528305242);
#87491=CYLINDRICAL_SURFACE('',#103014,1.66874528305242);
#87492=CYLINDRICAL_SURFACE('',#103015,1.66874528305242);
#87493=CYLINDRICAL_SURFACE('',#103016,1.66874528305242);
#87494=CYLINDRICAL_SURFACE('',#103017,1.66874528305242);
#87495=CYLINDRICAL_SURFACE('',#103018,1.66874528305242);
#87496=CYLINDRICAL_SURFACE('',#103020,1.66874528305242);
#87497=CYLINDRICAL_SURFACE('',#103021,1.66874528305242);
#87498=CYLINDRICAL_SURFACE('',#103022,1.66874528305242);
#87499=CYLINDRICAL_SURFACE('',#103023,1.66874528305242);
#87500=CYLINDRICAL_SURFACE('',#103024,1.66874528305242);
#87501=CYLINDRICAL_SURFACE('',#103025,1.66874528305242);
#87502=CYLINDRICAL_SURFACE('',#103026,1.66874528305242);
#87503=CYLINDRICAL_SURFACE('',#103027,1.66874528305242);
#87504=CYLINDRICAL_SURFACE('',#103028,1.66874528305242);
#87505=CYLINDRICAL_SURFACE('',#103029,1.66874528305242);
#87506=CYLINDRICAL_SURFACE('',#103030,1.66874528305242);
#87507=CYLINDRICAL_SURFACE('',#103031,1.66874528305242);
#87508=CYLINDRICAL_SURFACE('',#103032,1.66874528305242);
#87509=CYLINDRICAL_SURFACE('',#103033,1.66874528305242);
#87510=CYLINDRICAL_SURFACE('',#103034,1.66874528305242);
#87511=CYLINDRICAL_SURFACE('',#103035,1.66874528305242);
#87512=CYLINDRICAL_SURFACE('',#103036,1.66874528305242);
#87513=CYLINDRICAL_SURFACE('',#103037,1.66874528305242);
#87514=CYLINDRICAL_SURFACE('',#103038,1.66874528305242);
#87515=CYLINDRICAL_SURFACE('',#103059,3.);
#87516=CYLINDRICAL_SURFACE('',#103061,6.);
#87517=CYLINDRICAL_SURFACE('',#103066,3.);
#87518=CYLINDRICAL_SURFACE('',#103068,6.);
#87519=CYLINDRICAL_SURFACE('',#103073,3.);
#87520=CYLINDRICAL_SURFACE('',#103075,6.);
#87521=CYLINDRICAL_SURFACE('',#103080,3.);
#87522=CYLINDRICAL_SURFACE('',#103082,6.00000000000001);
#87523=CYLINDRICAL_SURFACE('',#103122,7.);
#87524=CYLINDRICAL_SURFACE('',#103138,0.999999999999999);
#87525=CYLINDRICAL_SURFACE('',#103143,0.999999999999997);
#87526=CYLINDRICAL_SURFACE('',#103154,1.);
#87527=CYLINDRICAL_SURFACE('',#103157,1.);
#87528=CYLINDRICAL_SURFACE('',#103164,1.);
#87529=CYLINDRICAL_SURFACE('',#103167,1.);
#87530=CYLINDRICAL_SURFACE('',#103169,20.);
#87531=CYLINDRICAL_SURFACE('',#103174,3.);
#87532=CYLINDRICAL_SURFACE('',#103176,3.);
#87533=CYLINDRICAL_SURFACE('',#103178,3.);
#87534=CYLINDRICAL_SURFACE('',#103182,3.);
#87535=CYLINDRICAL_SURFACE('',#103184,3.);
#87536=CYLINDRICAL_SURFACE('',#103189,67.5);
#87537=CYLINDRICAL_SURFACE('',#103197,3.);
#87538=CYLINDRICAL_SURFACE('',#103199,3.);
#87539=CYLINDRICAL_SURFACE('',#103204,67.5);
#87540=CYLINDRICAL_SURFACE('',#103216,3.);
#87541=CYLINDRICAL_SURFACE('',#103218,3.);
#87542=CYLINDRICAL_SURFACE('',#103220,3.);
#87543=CYLINDRICAL_SURFACE('',#103222,3.);
#87544=CYLINDRICAL_SURFACE('',#103224,58.3875000000282);
#87545=CYLINDRICAL_SURFACE('',#103229,3.);
#87546=CYLINDRICAL_SURFACE('',#103231,3.);
#87547=CYLINDRICAL_SURFACE('',#103236,67.5);
#87548=CYLINDRICAL_SURFACE('',#103244,58.3875000000282);
#87549=CYLINDRICAL_SURFACE('',#103249,3.);
#87550=CYLINDRICAL_SURFACE('',#103251,3.);
#87551=CYLINDRICAL_SURFACE('',#103256,67.5);
#87552=CYLINDRICAL_SURFACE('',#103264,58.3875000000282);
#87553=CYLINDRICAL_SURFACE('',#103282,3.);
#87554=CYLINDRICAL_SURFACE('',#103284,58.3875000000282);
#87555=CYLINDRICAL_SURFACE('',#103289,2.);
#87556=CYLINDRICAL_SURFACE('',#103292,1.66874528305242);
#87557=CYLINDRICAL_SURFACE('',#103293,2.);
#87558=CYLINDRICAL_SURFACE('',#103295,1.66874528305242);
#87559=CYLINDRICAL_SURFACE('',#103296,2.);
#87560=CYLINDRICAL_SURFACE('',#103297,2.);
#87561=CYLINDRICAL_SURFACE('',#103299,1.66874528305248);
#87562=CYLINDRICAL_SURFACE('',#103300,2.);
#87563=CYLINDRICAL_SURFACE('',#103301,2.);
#87564=CYLINDRICAL_SURFACE('',#103305,1.66874528305244);
#87565=CYLINDRICAL_SURFACE('',#103306,2.);
#87566=CYLINDRICAL_SURFACE('',#103307,2.);
#87567=CYLINDRICAL_SURFACE('',#103309,53.8875000000282);
#87568=CYLINDRICAL_SURFACE('',#103312,10.);
#87569=CYLINDRICAL_SURFACE('',#103316,10.);
#87570=CYLINDRICAL_SURFACE('',#103318,10.);
#87571=CYLINDRICAL_SURFACE('',#103321,10.);
#87572=CYLINDRICAL_SURFACE('',#103327,10.);
#87573=CYLINDRICAL_SURFACE('',#103329,10.);
#87574=CYLINDRICAL_SURFACE('',#103331,10.);
#88019=ADVANCED_FACE('',(#8740),#6929,.T.);
#88020=ADVANCED_FACE('',(#8741),#7726,.T.);
#88021=ADVANCED_FACE('',(#8742),#85787,.T.);
#88022=ADVANCED_FACE('',(#8743,#7439),#7727,.F.);
#88023=ADVANCED_FACE('',(#8744),#85788,.T.);
#88024=ADVANCED_FACE('',(#8745),#7728,.F.);
#88025=ADVANCED_FACE('',(#8746),#6930,.T.);
#88026=ADVANCED_FACE('',(#8747),#7729,.T.);
#88027=ADVANCED_FACE('',(#8748),#85789,.T.);
#88028=ADVANCED_FACE('',(#8749,#7440),#7730,.F.);
#88029=ADVANCED_FACE('',(#8750),#85790,.T.);
#88030=ADVANCED_FACE('',(#8751),#7731,.F.);
#88031=ADVANCED_FACE('',(#8752),#85791,.F.);
#88032=ADVANCED_FACE('',(#8753),#85792,.F.);
#88033=ADVANCED_FACE('',(#8754),#3206,.F.);
#88034=ADVANCED_FACE('',(#8755),#2038,.F.);
#88035=ADVANCED_FACE('',(#8756),#85793,.T.);
#88036=ADVANCED_FACE('',(#8757),#7732,.T.);
#88037=ADVANCED_FACE('',(#8758),#3207,.T.);
#88038=ADVANCED_FACE('',(#8759),#85794,.T.);
#88039=ADVANCED_FACE('',(#8760),#7733,.T.);
#88040=ADVANCED_FACE('',(#8761),#3208,.T.);
#88041=ADVANCED_FACE('',(#8762),#7734,.T.);
#88042=ADVANCED_FACE('',(#8763),#2039,.F.);
#88043=ADVANCED_FACE('',(#8764),#85795,.F.);
#88044=ADVANCED_FACE('',(#8765),#3209,.T.);
#88045=ADVANCED_FACE('',(#8766),#85796,.F.);
#88046=ADVANCED_FACE('',(#8767),#2040,.F.);
#88047=ADVANCED_FACE('',(#8768),#2041,.F.);
#88048=ADVANCED_FACE('',(#8769),#2042,.F.);
#88049=ADVANCED_FACE('',(#8770),#85797,.F.);
#88050=ADVANCED_FACE('',(#8771),#3210,.T.);
#88051=ADVANCED_FACE('',(#8772),#85798,.F.);
#88052=ADVANCED_FACE('',(#8773),#2043,.F.);
#88053=ADVANCED_FACE('',(#8774),#3211,.F.);
#88054=ADVANCED_FACE('',(#8775),#2044,.F.);
#88055=ADVANCED_FACE('',(#8776),#85799,.F.);
#88056=ADVANCED_FACE('',(#8777),#3212,.T.);
#88057=ADVANCED_FACE('',(#8778),#85800,.F.);
#88058=ADVANCED_FACE('',(#8779),#2045,.F.);
#88059=ADVANCED_FACE('',(#8780),#3213,.F.);
#88060=ADVANCED_FACE('',(#8781),#85801,.F.);
#88061=ADVANCED_FACE('',(#8782),#3214,.T.);
#88062=ADVANCED_FACE('',(#8783),#85802,.F.);
#88063=ADVANCED_FACE('',(#8784),#2046,.F.);
#88064=ADVANCED_FACE('',(#8785),#3215,.F.);
#88065=ADVANCED_FACE('',(#8786),#2047,.F.);
#88066=ADVANCED_FACE('',(#8787),#85803,.F.);
#88067=ADVANCED_FACE('',(#8788),#3216,.T.);
#88068=ADVANCED_FACE('',(#8789),#85804,.F.);
#88069=ADVANCED_FACE('',(#8790),#2048,.F.);
#88070=ADVANCED_FACE('',(#8791),#2049,.F.);
#88071=ADVANCED_FACE('',(#8792),#2050,.F.);
#88072=ADVANCED_FACE('',(#8793),#85805,.F.);
#88073=ADVANCED_FACE('',(#8794),#3217,.T.);
#88074=ADVANCED_FACE('',(#8795),#85806,.F.);
#88075=ADVANCED_FACE('',(#8796),#2051,.F.);
#88076=ADVANCED_FACE('',(#8797),#2052,.F.);
#88077=ADVANCED_FACE('',(#8798),#2053,.F.);
#88078=ADVANCED_FACE('',(#8799),#85807,.F.);
#88079=ADVANCED_FACE('',(#8800),#2054,.F.);
#88080=ADVANCED_FACE('',(#8801),#3218,.F.);
#88081=ADVANCED_FACE('',(#8802),#2055,.F.);
#88082=ADVANCED_FACE('',(#8803),#85808,.F.);
#88083=ADVANCED_FACE('',(#8804),#85809,.T.);
#88084=ADVANCED_FACE('',(#8805),#2056,.F.);
#88085=ADVANCED_FACE('',(#8806),#3219,.F.);
#88086=ADVANCED_FACE('',(#8807),#2057,.F.);
#88087=ADVANCED_FACE('',(#8808),#85810,.T.);
#88088=ADVANCED_FACE('',(#8809),#7735,.T.);
#88089=ADVANCED_FACE('',(#8810),#3220,.T.);
#88090=ADVANCED_FACE('',(#8811),#85811,.T.);
#88091=ADVANCED_FACE('',(#8812),#7736,.T.);
#88092=ADVANCED_FACE('',(#8813),#3221,.T.);
#88093=ADVANCED_FACE('',(#8814),#7737,.T.);
#88094=ADVANCED_FACE('',(#8815),#2058,.F.);
#88095=ADVANCED_FACE('',(#8816),#85812,.F.);
#88096=ADVANCED_FACE('',(#8817),#3222,.T.);
#88097=ADVANCED_FACE('',(#8818),#85813,.F.);
#88098=ADVANCED_FACE('',(#8819),#2059,.F.);
#88099=ADVANCED_FACE('',(#8820),#3223,.F.);
#88100=ADVANCED_FACE('',(#8821),#2060,.F.);
#88101=ADVANCED_FACE('',(#8822),#85814,.F.);
#88102=ADVANCED_FACE('',(#8823),#3224,.T.);
#88103=ADVANCED_FACE('',(#8824),#85815,.F.);
#88104=ADVANCED_FACE('',(#8825),#2061,.F.);
#88105=ADVANCED_FACE('',(#8826),#2062,.F.);
#88106=ADVANCED_FACE('',(#8827),#2063,.F.);
#88107=ADVANCED_FACE('',(#8828),#85816,.F.);
#88108=ADVANCED_FACE('',(#8829),#3225,.T.);
#88109=ADVANCED_FACE('',(#8830),#85817,.F.);
#88110=ADVANCED_FACE('',(#8831),#2064,.F.);
#88111=ADVANCED_FACE('',(#8832),#2065,.F.);
#88112=ADVANCED_FACE('',(#8833),#2066,.F.);
#88113=ADVANCED_FACE('',(#8834),#85818,.F.);
#88114=ADVANCED_FACE('',(#8835),#3226,.T.);
#88115=ADVANCED_FACE('',(#8836),#85819,.F.);
#88116=ADVANCED_FACE('',(#8837),#2067,.F.);
#88117=ADVANCED_FACE('',(#8838),#2068,.F.);
#88118=ADVANCED_FACE('',(#8839),#2069,.F.);
#88119=ADVANCED_FACE('',(#8840),#85820,.F.);
#88120=ADVANCED_FACE('',(#8841),#3227,.T.);
#88121=ADVANCED_FACE('',(#8842),#85821,.F.);
#88122=ADVANCED_FACE('',(#8843),#2070,.F.);
#88123=ADVANCED_FACE('',(#8844),#3228,.F.);
#88124=ADVANCED_FACE('',(#8845),#2071,.F.);
#88125=ADVANCED_FACE('',(#8846),#85822,.F.);
#88126=ADVANCED_FACE('',(#8847),#3229,.T.);
#88127=ADVANCED_FACE('',(#8848),#85823,.F.);
#88128=ADVANCED_FACE('',(#8849),#2072,.F.);
#88129=ADVANCED_FACE('',(#8850),#85824,.T.);
#88130=ADVANCED_FACE('',(#8851),#85825,.F.);
#88131=ADVANCED_FACE('',(#8852),#2073,.F.);
#88132=ADVANCED_FACE('',(#8853),#85826,.F.);
#88133=ADVANCED_FACE('',(#8854),#2074,.F.);
#88134=ADVANCED_FACE('',(#8855),#85827,.F.);
#88135=ADVANCED_FACE('',(#8856),#85828,.T.);
#88136=ADVANCED_FACE('',(#8857),#2075,.F.);
#88137=ADVANCED_FACE('',(#8858),#85829,.F.);
#88138=ADVANCED_FACE('',(#8859),#2076,.T.);
#88139=ADVANCED_FACE('',(#8860),#85830,.T.);
#88140=ADVANCED_FACE('',(#8861),#85831,.F.);
#88141=ADVANCED_FACE('',(#8862),#2077,.F.);
#88142=ADVANCED_FACE('',(#8863),#85832,.F.);
#88143=ADVANCED_FACE('',(#8864),#2078,.F.);
#88144=ADVANCED_FACE('',(#8865),#85833,.F.);
#88145=ADVANCED_FACE('',(#8866),#85834,.T.);
#88146=ADVANCED_FACE('',(#8867),#2079,.T.);
#88147=ADVANCED_FACE('',(#8868),#85835,.T.);
#88148=ADVANCED_FACE('',(#8869),#85836,.F.);
#88149=ADVANCED_FACE('',(#8870),#2080,.F.);
#88150=ADVANCED_FACE('',(#8871),#85837,.F.);
#88151=ADVANCED_FACE('',(#8872),#2081,.F.);
#88152=ADVANCED_FACE('',(#8873),#85838,.F.);
#88153=ADVANCED_FACE('',(#8874),#2082,.T.);
#88154=ADVANCED_FACE('',(#8875),#85839,.T.);
#88155=ADVANCED_FACE('',(#8876),#85840,.F.);
#88156=ADVANCED_FACE('',(#8877),#2083,.F.);
#88157=ADVANCED_FACE('',(#8878),#85841,.F.);
#88158=ADVANCED_FACE('',(#8879),#2084,.F.);
#88159=ADVANCED_FACE('',(#8880),#85842,.F.);
#88160=ADVANCED_FACE('',(#8881),#85843,.T.);
#88161=ADVANCED_FACE('',(#8882),#85844,.T.);
#88162=ADVANCED_FACE('',(#8883),#85845,.F.);
#88163=ADVANCED_FACE('',(#8884),#2085,.F.);
#88164=ADVANCED_FACE('',(#8885),#85846,.F.);
#88165=ADVANCED_FACE('',(#8886),#2086,.F.);
#88166=ADVANCED_FACE('',(#8887),#85847,.F.);
#88167=ADVANCED_FACE('',(#8888),#85848,.T.);
#88168=ADVANCED_FACE('',(#8889),#2087,.F.);
#88169=ADVANCED_FACE('',(#8890),#85849,.F.);
#88170=ADVANCED_FACE('',(#8891),#2088,.T.);
#88171=ADVANCED_FACE('',(#8892),#85850,.T.);
#88172=ADVANCED_FACE('',(#8893),#85851,.F.);
#88173=ADVANCED_FACE('',(#8894),#2089,.F.);
#88174=ADVANCED_FACE('',(#8895),#85852,.F.);
#88175=ADVANCED_FACE('',(#8896),#2090,.F.);
#88176=ADVANCED_FACE('',(#8897),#85853,.F.);
#88177=ADVANCED_FACE('',(#8898),#2091,.T.);
#88178=ADVANCED_FACE('',(#8899),#85854,.F.);
#88179=ADVANCED_FACE('',(#8900),#2092,.F.);
#88180=ADVANCED_FACE('',(#8901),#85855,.T.);
#88181=ADVANCED_FACE('',(#8902),#85856,.F.);
#88182=ADVANCED_FACE('',(#8903),#2093,.F.);
#88183=ADVANCED_FACE('',(#8904),#85857,.F.);
#88184=ADVANCED_FACE('',(#8905),#2094,.F.);
#88185=ADVANCED_FACE('',(#8906),#85858,.F.);
#88186=ADVANCED_FACE('',(#8907),#85859,.T.);
#88187=ADVANCED_FACE('',(#8908),#85860,.F.);
#88188=ADVANCED_FACE('',(#8909),#2095,.F.);
#88189=ADVANCED_FACE('',(#8910),#85861,.F.);
#88190=ADVANCED_FACE('',(#8911),#2096,.F.);
#88191=ADVANCED_FACE('',(#8912),#85862,.F.);
#88192=ADVANCED_FACE('',(#8913),#85863,.T.);
#88193=ADVANCED_FACE('',(#8914),#7738,.T.);
#88194=ADVANCED_FACE('',(#8915),#7739,.T.);
#88195=ADVANCED_FACE('',(#8916),#7740,.F.);
#88196=ADVANCED_FACE('',(#8917),#85864,.T.);
#88197=ADVANCED_FACE('',(#8918),#2097,.F.);
#88198=ADVANCED_FACE('',(#8919),#2098,.F.);
#88199=ADVANCED_FACE('',(#8920),#2099,.F.);
#88200=ADVANCED_FACE('',(#8921),#3230,.F.);
#88201=ADVANCED_FACE('',(#8922),#85865,.F.);
#88202=ADVANCED_FACE('',(#8923),#85866,.T.);
#88203=ADVANCED_FACE('',(#8924),#85867,.F.);
#88204=ADVANCED_FACE('',(#8925),#3231,.F.);
#88205=ADVANCED_FACE('',(#8926),#85868,.F.);
#88206=ADVANCED_FACE('',(#8927),#3232,.F.);
#88207=ADVANCED_FACE('',(#8928),#85869,.F.);
#88208=ADVANCED_FACE('',(#8929),#3233,.F.);
#88209=ADVANCED_FACE('',(#8930),#85870,.F.);
#88210=ADVANCED_FACE('',(#8931),#3234,.F.);
#88211=ADVANCED_FACE('',(#8932),#85871,.F.);
#88212=ADVANCED_FACE('',(#8933),#3235,.F.);
#88213=ADVANCED_FACE('',(#8934),#85872,.F.);
#88214=ADVANCED_FACE('',(#8935),#3236,.F.);
#88215=ADVANCED_FACE('',(#8936),#2100,.F.);
#88216=ADVANCED_FACE('',(#8937),#85873,.F.);
#88217=ADVANCED_FACE('',(#8938),#85874,.F.);
#88218=ADVANCED_FACE('',(#8939),#3237,.F.);
#88219=ADVANCED_FACE('',(#8940),#85875,.F.);
#88220=ADVANCED_FACE('',(#8941),#3238,.F.);
#88221=ADVANCED_FACE('',(#8942),#85876,.F.);
#88222=ADVANCED_FACE('',(#8943),#85877,.F.);
#88223=ADVANCED_FACE('',(#8944),#85878,.F.);
#88224=ADVANCED_FACE('',(#8945),#3239,.F.);
#88225=ADVANCED_FACE('',(#8946),#85879,.F.);
#88226=ADVANCED_FACE('',(#8947),#3240,.F.);
#88227=ADVANCED_FACE('',(#8948),#85880,.F.);
#88228=ADVANCED_FACE('',(#8949),#85881,.F.);
#88229=ADVANCED_FACE('',(#8950),#85882,.F.);
#88230=ADVANCED_FACE('',(#8951),#7741,.F.);
#88231=ADVANCED_FACE('',(#8952),#85883,.T.);
#88232=ADVANCED_FACE('',(#8953),#3241,.F.);
#88233=ADVANCED_FACE('',(#8954),#85884,.F.);
#88234=ADVANCED_FACE('',(#8955),#85885,.F.);
#88235=ADVANCED_FACE('',(#8956),#3242,.T.);
#88236=ADVANCED_FACE('',(#8957),#85886,.T.);
#88237=ADVANCED_FACE('',(#8958),#3243,.T.);
#88238=ADVANCED_FACE('',(#8959),#3244,.T.);
#88239=ADVANCED_FACE('',(#8960),#3245,.T.);
#88240=ADVANCED_FACE('',(#8961),#85887,.T.);
#88241=ADVANCED_FACE('',(#8962),#3246,.T.);
#88242=ADVANCED_FACE('',(#8963),#3247,.T.);
#88243=ADVANCED_FACE('',(#8964),#3248,.T.);
#88244=ADVANCED_FACE('',(#8965),#85888,.T.);
#88245=ADVANCED_FACE('',(#8966),#3249,.T.);
#88246=ADVANCED_FACE('',(#8967),#3250,.T.);
#88247=ADVANCED_FACE('',(#8968),#3251,.T.);
#88248=ADVANCED_FACE('',(#8969),#85889,.T.);
#88249=ADVANCED_FACE('',(#8970),#3252,.T.);
#88250=ADVANCED_FACE('',(#8971),#85890,.F.);
#88251=ADVANCED_FACE('',(#8972),#85891,.F.);
#88252=ADVANCED_FACE('',(#8973),#2101,.F.);
#88253=ADVANCED_FACE('',(#8974),#85892,.F.);
#88254=ADVANCED_FACE('',(#8975),#3253,.T.);
#88255=ADVANCED_FACE('',(#8976),#85893,.F.);
#88256=ADVANCED_FACE('',(#8977),#2102,.F.);
#88257=ADVANCED_FACE('',(#8978),#3254,.F.);
#88258=ADVANCED_FACE('',(#8979),#2103,.F.);
#88259=ADVANCED_FACE('',(#8980),#85894,.F.);
#88260=ADVANCED_FACE('',(#8981),#3255,.T.);
#88261=ADVANCED_FACE('',(#8982),#85895,.F.);
#88262=ADVANCED_FACE('',(#8983),#2104,.F.);
#88263=ADVANCED_FACE('',(#8984),#2105,.F.);
#88264=ADVANCED_FACE('',(#8985),#2106,.F.);
#88265=ADVANCED_FACE('',(#8986),#85896,.F.);
#88266=ADVANCED_FACE('',(#8987),#3256,.T.);
#88267=ADVANCED_FACE('',(#8988),#85897,.F.);
#88268=ADVANCED_FACE('',(#8989),#2107,.F.);
#88269=ADVANCED_FACE('',(#8990),#85898,.F.);
#88270=ADVANCED_FACE('',(#8991),#2108,.F.);
#88271=ADVANCED_FACE('',(#8992),#3257,.F.);
#88272=ADVANCED_FACE('',(#8993),#2109,.T.);
#88273=ADVANCED_FACE('',(#8994),#85899,.T.);
#88274=ADVANCED_FACE('',(#8995),#2110,.T.);
#88275=ADVANCED_FACE('',(#8996),#2111,.F.);
#88276=ADVANCED_FACE('',(#8997),#7742,.F.);
#88277=ADVANCED_FACE('',(#8998),#6931,.T.);
#88278=ADVANCED_FACE('',(#8999),#2112,.F.);
#88279=ADVANCED_FACE('',(#9000),#7743,.F.);
#88280=ADVANCED_FACE('',(#9001),#2113,.T.);
#88281=ADVANCED_FACE('',(#9002),#2114,.T.);
#88282=ADVANCED_FACE('',(#9003),#2115,.T.);
#88283=ADVANCED_FACE('',(#9004),#2116,.F.);
#88284=ADVANCED_FACE('',(#9005),#7744,.F.);
#88285=ADVANCED_FACE('',(#9006),#6932,.T.);
#88286=ADVANCED_FACE('',(#9007),#2117,.F.);
#88287=ADVANCED_FACE('',(#9008),#7745,.F.);
#88288=ADVANCED_FACE('',(#9009),#85900,.T.);
#88289=ADVANCED_FACE('',(#9010),#7746,.F.);
#88290=ADVANCED_FACE('',(#9011),#85901,.T.);
#88291=ADVANCED_FACE('',(#9012),#2118,.F.);
#88292=ADVANCED_FACE('',(#9013),#7747,.F.);
#88293=ADVANCED_FACE('',(#9014),#6933,.T.);
#88294=ADVANCED_FACE('',(#9015),#2119,.F.);
#88295=ADVANCED_FACE('',(#9016),#7748,.F.);
#88296=ADVANCED_FACE('',(#9017),#85902,.T.);
#88297=ADVANCED_FACE('',(#9018),#3258,.F.);
#88298=ADVANCED_FACE('',(#9019),#2120,.F.);
#88299=ADVANCED_FACE('',(#9020),#7749,.F.);
#88300=ADVANCED_FACE('',(#9021),#85903,.T.);
#88301=ADVANCED_FACE('',(#9022),#7750,.T.);
#88302=ADVANCED_FACE('',(#9023),#85904,.T.);
#88303=ADVANCED_FACE('',(#9024),#7751,.F.);
#88304=ADVANCED_FACE('',(#9025),#2121,.F.);
#88305=ADVANCED_FACE('',(#9026),#6934,.T.);
#88306=ADVANCED_FACE('',(#9027),#2122,.F.);
#88307=ADVANCED_FACE('',(#9028),#7752,.F.);
#88308=ADVANCED_FACE('',(#9029),#2123,.T.);
#88309=ADVANCED_FACE('',(#9030),#2124,.T.);
#88310=ADVANCED_FACE('',(#9031),#2125,.T.);
#88311=ADVANCED_FACE('',(#9032),#2126,.F.);
#88312=ADVANCED_FACE('',(#9033),#7753,.F.);
#88313=ADVANCED_FACE('',(#9034),#6935,.T.);
#88314=ADVANCED_FACE('',(#9035),#2127,.F.);
#88315=ADVANCED_FACE('',(#9036),#7754,.F.);
#88316=ADVANCED_FACE('',(#9037),#2128,.T.);
#88317=ADVANCED_FACE('',(#9038),#2129,.T.);
#88318=ADVANCED_FACE('',(#9039),#2130,.T.);
#88319=ADVANCED_FACE('',(#9040),#7755,.F.);
#88320=ADVANCED_FACE('',(#9041),#85905,.T.);
#88321=ADVANCED_FACE('',(#9042),#7756,.F.);
#88322=ADVANCED_FACE('',(#9043),#85906,.T.);
#88323=ADVANCED_FACE('',(#9044),#85907,.T.);
#88324=ADVANCED_FACE('',(#9045),#7757,.F.);
#88325=ADVANCED_FACE('',(#9046),#85908,.T.);
#88326=ADVANCED_FACE('',(#9047),#7758,.F.);
#88327=ADVANCED_FACE('',(#9048),#2131,.F.);
#88328=ADVANCED_FACE('',(#9049),#6936,.T.);
#88329=ADVANCED_FACE('',(#9050),#2132,.F.);
#88330=ADVANCED_FACE('',(#9051),#7759,.F.);
#88331=ADVANCED_FACE('',(#9052),#85909,.T.);
#88332=ADVANCED_FACE('',(#9053),#7760,.F.);
#88333=ADVANCED_FACE('',(#9054),#85910,.T.);
#88334=ADVANCED_FACE('',(#9055),#2133,.F.);
#88335=ADVANCED_FACE('',(#9056),#7761,.F.);
#88336=ADVANCED_FACE('',(#9057),#6937,.T.);
#88337=ADVANCED_FACE('',(#9058),#2134,.F.);
#88338=ADVANCED_FACE('',(#9059),#7762,.F.);
#88339=ADVANCED_FACE('',(#9060),#2135,.T.);
#88340=ADVANCED_FACE('',(#9061),#2136,.T.);
#88341=ADVANCED_FACE('',(#9062),#2137,.T.);
#88342=ADVANCED_FACE('',(#9063),#2138,.F.);
#88343=ADVANCED_FACE('',(#9064),#7763,.F.);
#88344=ADVANCED_FACE('',(#9065),#6938,.T.);
#88345=ADVANCED_FACE('',(#9066),#2139,.F.);
#88346=ADVANCED_FACE('',(#9067),#7764,.F.);
#88347=ADVANCED_FACE('',(#9068),#2140,.T.);
#88348=ADVANCED_FACE('',(#9069),#2141,.T.);
#88349=ADVANCED_FACE('',(#9070),#2142,.T.);
#88350=ADVANCED_FACE('',(#9071),#2143,.F.);
#88351=ADVANCED_FACE('',(#9072),#7765,.F.);
#88352=ADVANCED_FACE('',(#9073),#6939,.T.);
#88353=ADVANCED_FACE('',(#9074),#2144,.F.);
#88354=ADVANCED_FACE('',(#9075),#7766,.F.);
#88355=ADVANCED_FACE('',(#9076),#2145,.T.);
#88356=ADVANCED_FACE('',(#9077),#2146,.T.);
#88357=ADVANCED_FACE('',(#9078),#2147,.T.);
#88358=ADVANCED_FACE('',(#9079),#2148,.F.);
#88359=ADVANCED_FACE('',(#9080),#7767,.F.);
#88360=ADVANCED_FACE('',(#9081),#6940,.T.);
#88361=ADVANCED_FACE('',(#9082),#2149,.F.);
#88362=ADVANCED_FACE('',(#9083),#7768,.F.);
#88363=ADVANCED_FACE('',(#9084),#85911,.T.);
#88364=ADVANCED_FACE('',(#9085),#7769,.F.);
#88365=ADVANCED_FACE('',(#9086),#85912,.T.);
#88366=ADVANCED_FACE('',(#9087),#2150,.F.);
#88367=ADVANCED_FACE('',(#9088),#7770,.F.);
#88368=ADVANCED_FACE('',(#9089),#6941,.T.);
#88369=ADVANCED_FACE('',(#9090),#2151,.F.);
#88370=ADVANCED_FACE('',(#9091),#7771,.F.);
#88371=ADVANCED_FACE('',(#9092),#7772,.T.);
#88372=ADVANCED_FACE('',(#9093),#2152,.F.);
#88373=ADVANCED_FACE('',(#9094),#2153,.F.);
#88374=ADVANCED_FACE('',(#9095),#7773,.F.);
#88375=ADVANCED_FACE('',(#9096),#85913,.T.);
#88376=ADVANCED_FACE('',(#9097),#7774,.F.);
#88377=ADVANCED_FACE('',(#9098),#85914,.T.);
#88378=ADVANCED_FACE('',(#9099),#7775,.F.);
#88379=ADVANCED_FACE('',(#9100),#2154,.F.);
#88380=ADVANCED_FACE('',(#9101),#2155,.F.);
#88381=ADVANCED_FACE('',(#9102),#7776,.F.);
#88382=ADVANCED_FACE('',(#9103),#3259,.F.);
#88383=ADVANCED_FACE('',(#9104),#7777,.T.);
#88384=ADVANCED_FACE('',(#9105),#2156,.F.);
#88385=ADVANCED_FACE('',(#9106),#7778,.F.);
#88386=ADVANCED_FACE('',(#9107),#85915,.T.);
#88387=ADVANCED_FACE('',(#9108),#7779,.F.);
#88388=ADVANCED_FACE('',(#9109),#85916,.T.);
#88389=ADVANCED_FACE('',(#9110),#7780,.F.);
#88390=ADVANCED_FACE('',(#9111),#7781,.T.);
#88391=ADVANCED_FACE('',(#9112),#2157,.F.);
#88392=ADVANCED_FACE('',(#9113),#2158,.F.);
#88393=ADVANCED_FACE('',(#9114),#7782,.F.);
#88394=ADVANCED_FACE('',(#9115),#85917,.T.);
#88395=ADVANCED_FACE('',(#9116),#7783,.T.);
#88396=ADVANCED_FACE('',(#9117),#85918,.T.);
#88397=ADVANCED_FACE('',(#9118),#7784,.F.);
#88398=ADVANCED_FACE('',(#9119),#2159,.F.);
#88399=ADVANCED_FACE('',(#9120),#2160,.F.);
#88400=ADVANCED_FACE('',(#9121),#7785,.T.);
#88401=ADVANCED_FACE('',(#9122),#85919,.T.);
#88402=ADVANCED_FACE('',(#9123),#7786,.T.);
#88403=ADVANCED_FACE('',(#9124),#85920,.T.);
#88404=ADVANCED_FACE('',(#9125),#7787,.F.);
#88405=ADVANCED_FACE('',(#9126),#7788,.T.);
#88406=ADVANCED_FACE('',(#9127),#2161,.F.);
#88407=ADVANCED_FACE('',(#9128),#2162,.F.);
#88408=ADVANCED_FACE('',(#9129),#7789,.F.);
#88409=ADVANCED_FACE('',(#9130),#85921,.T.);
#88410=ADVANCED_FACE('',(#9131),#7790,.F.);
#88411=ADVANCED_FACE('',(#9132),#85922,.T.);
#88412=ADVANCED_FACE('',(#9133),#2163,.F.);
#88413=ADVANCED_FACE('',(#9134),#7791,.F.);
#88414=ADVANCED_FACE('',(#9135),#7792,.F.);
#88415=ADVANCED_FACE('',(#9136),#2164,.F.);
#88416=ADVANCED_FACE('',(#9137),#2165,.T.);
#88417=ADVANCED_FACE('',(#9138),#3260,.F.);
#88418=ADVANCED_FACE('',(#9139),#7793,.T.);
#88419=ADVANCED_FACE('',(#9140),#2166,.F.);
#88420=ADVANCED_FACE('',(#9141),#7794,.F.);
#88421=ADVANCED_FACE('',(#9142),#85923,.T.);
#88422=ADVANCED_FACE('',(#9143),#7795,.F.);
#88423=ADVANCED_FACE('',(#9144),#85924,.T.);
#88424=ADVANCED_FACE('',(#9145),#7796,.F.);
#88425=ADVANCED_FACE('',(#9146),#3261,.F.);
#88426=ADVANCED_FACE('',(#9147),#2167,.F.);
#88427=ADVANCED_FACE('',(#9148),#7797,.F.);
#88428=ADVANCED_FACE('',(#9149),#2168,.F.);
#88429=ADVANCED_FACE('',(#9150),#7798,.F.);
#88430=ADVANCED_FACE('',(#9151),#85925,.T.);
#88431=ADVANCED_FACE('',(#9152),#7799,.F.);
#88432=ADVANCED_FACE('',(#9153),#85926,.T.);
#88433=ADVANCED_FACE('',(#9154),#7800,.F.);
#88434=ADVANCED_FACE('',(#9155),#2169,.F.);
#88435=ADVANCED_FACE('',(#9156),#7801,.T.);
#88436=ADVANCED_FACE('',(#9157),#2170,.F.);
#88437=ADVANCED_FACE('',(#9158),#7802,.F.);
#88438=ADVANCED_FACE('',(#9159),#85927,.T.);
#88439=ADVANCED_FACE('',(#9160),#7803,.F.);
#88440=ADVANCED_FACE('',(#9161),#85928,.T.);
#88441=ADVANCED_FACE('',(#9162),#2171,.F.);
#88442=ADVANCED_FACE('',(#9163),#7804,.F.);
#88443=ADVANCED_FACE('',(#9164),#7805,.T.);
#88444=ADVANCED_FACE('',(#9165),#85929,.F.);
#88445=ADVANCED_FACE('',(#9166),#85930,.F.);
#88446=ADVANCED_FACE('',(#9167,#7441),#7806,.T.);
#88447=ADVANCED_FACE('',(#9168),#85931,.F.);
#88448=ADVANCED_FACE('',(#9169),#85932,.F.);
#88449=ADVANCED_FACE('',(#9170),#2172,.T.);
#88450=ADVANCED_FACE('',(#9171),#3262,.F.);
#88451=ADVANCED_FACE('',(#9172),#2173,.T.);
#88452=ADVANCED_FACE('',(#9173),#85933,.F.);
#88453=ADVANCED_FACE('',(#9174),#85934,.F.);
#88454=ADVANCED_FACE('',(#9175),#85935,.F.);
#88455=ADVANCED_FACE('',(#9176,#7442),#7807,.T.);
#88456=ADVANCED_FACE('',(#9177),#85936,.F.);
#88457=ADVANCED_FACE('',(#9178),#85937,.F.);
#88458=ADVANCED_FACE('',(#9179),#85938,.T.);
#88459=ADVANCED_FACE('',(#9180),#3263,.T.);
#88460=ADVANCED_FACE('',(#9181),#85939,.T.);
#88461=ADVANCED_FACE('',(#9182),#7808,.T.);
#88462=ADVANCED_FACE('',(#9183),#2174,.F.);
#88463=ADVANCED_FACE('',(#9184),#2175,.F.);
#88464=ADVANCED_FACE('',(#9185),#3264,.F.);
#88465=ADVANCED_FACE('',(#9186),#85940,.F.);
#88466=ADVANCED_FACE('',(#9187),#2176,.F.);
#88467=ADVANCED_FACE('',(#9188),#2177,.F.);
#88468=ADVANCED_FACE('',(#9189),#85941,.T.);
#88469=ADVANCED_FACE('',(#9190),#7809,.T.);
#88470=ADVANCED_FACE('',(#9191),#85942,.T.);
#88471=ADVANCED_FACE('',(#9192),#2178,.F.);
#88472=ADVANCED_FACE('',(#9193),#2179,.F.);
#88473=ADVANCED_FACE('',(#9194),#85943,.T.);
#88474=ADVANCED_FACE('',(#9195),#7810,.T.);
#88475=ADVANCED_FACE('',(#9196),#85944,.T.);
#88476=ADVANCED_FACE('',(#9197),#2180,.F.);
#88477=ADVANCED_FACE('',(#9198),#2181,.F.);
#88478=ADVANCED_FACE('',(#9199),#2182,.F.);
#88479=ADVANCED_FACE('',(#9200),#7811,.F.);
#88480=ADVANCED_FACE('',(#9201),#2183,.T.);
#88481=ADVANCED_FACE('',(#9202),#85945,.T.);
#88482=ADVANCED_FACE('',(#9203),#7812,.T.);
#88483=ADVANCED_FACE('',(#9204),#85946,.T.);
#88484=ADVANCED_FACE('',(#9205),#2184,.T.);
#88485=ADVANCED_FACE('',(#9206),#7813,.F.);
#88486=ADVANCED_FACE('',(#9207),#2185,.T.);
#88487=ADVANCED_FACE('',(#9208),#85947,.T.);
#88488=ADVANCED_FACE('',(#9209),#7814,.T.);
#88489=ADVANCED_FACE('',(#9210),#85948,.T.);
#88490=ADVANCED_FACE('',(#9211),#2186,.T.);
#88491=ADVANCED_FACE('',(#9212),#7815,.F.);
#88492=ADVANCED_FACE('',(#9213),#2187,.T.);
#88493=ADVANCED_FACE('',(#9214),#85949,.F.);
#88494=ADVANCED_FACE('',(#9215),#85950,.F.);
#88495=ADVANCED_FACE('',(#9216),#2188,.F.);
#88496=ADVANCED_FACE('',(#9217),#85951,.F.);
#88497=ADVANCED_FACE('',(#9218),#2189,.F.);
#88498=ADVANCED_FACE('',(#9219),#85952,.F.);
#88499=ADVANCED_FACE('',(#9220),#2190,.F.);
#88500=ADVANCED_FACE('',(#9221),#7816,.T.);
#88501=ADVANCED_FACE('',(#9222),#85953,.T.);
#88502=ADVANCED_FACE('',(#9223),#85954,.T.);
#88503=ADVANCED_FACE('',(#9224),#85955,.T.);
#88504=ADVANCED_FACE('',(#9225),#7817,.T.);
#88505=ADVANCED_FACE('',(#9226),#85956,.F.);
#88506=ADVANCED_FACE('',(#9227),#85957,.T.);
#88507=ADVANCED_FACE('',(#9228),#85958,.F.);
#88508=ADVANCED_FACE('',(#9229),#7818,.T.);
#88509=ADVANCED_FACE('',(#9230),#85959,.T.);
#88510=ADVANCED_FACE('',(#9231),#85960,.T.);
#88511=ADVANCED_FACE('',(#9232),#85961,.T.);
#88512=ADVANCED_FACE('',(#9233),#7819,.T.);
#88513=ADVANCED_FACE('',(#9234),#2191,.F.);
#88514=ADVANCED_FACE('',(#9235),#7820,.F.);
#88515=ADVANCED_FACE('',(#9236),#2192,.F.);
#88516=ADVANCED_FACE('',(#9237),#7821,.F.);
#88517=ADVANCED_FACE('',(#9238),#2193,.F.);
#88518=ADVANCED_FACE('',(#9239),#7822,.F.);
#88519=ADVANCED_FACE('',(#9240),#7823,.F.);
#88520=ADVANCED_FACE('',(#9241),#85962,.T.);
#88521=ADVANCED_FACE('',(#9242),#2194,.F.);
#88522=ADVANCED_FACE('',(#9243),#6942,.T.);
#88523=ADVANCED_FACE('',(#9244),#2195,.F.);
#88524=ADVANCED_FACE('',(#9245),#85963,.T.);
#88525=ADVANCED_FACE('',(#9246),#7824,.F.);
#88526=ADVANCED_FACE('',(#9247),#85964,.T.);
#88527=ADVANCED_FACE('',(#9248),#2196,.F.);
#88528=ADVANCED_FACE('',(#9249),#6943,.T.);
#88529=ADVANCED_FACE('',(#9250),#2197,.F.);
#88530=ADVANCED_FACE('',(#9251),#2198,.T.);
#88531=ADVANCED_FACE('',(#9252),#2199,.T.);
#88532=ADVANCED_FACE('',(#9253),#2200,.T.);
#88533=ADVANCED_FACE('',(#9254),#2201,.F.);
#88534=ADVANCED_FACE('',(#9255),#6944,.T.);
#88535=ADVANCED_FACE('',(#9256),#2202,.F.);
#88536=ADVANCED_FACE('',(#9257),#85965,.F.);
#88537=ADVANCED_FACE('',(#9258),#2203,.F.);
#88538=ADVANCED_FACE('',(#9259),#2204,.T.);
#88539=ADVANCED_FACE('',(#9260),#85966,.T.);
#88540=ADVANCED_FACE('',(#9261),#7825,.F.);
#88541=ADVANCED_FACE('',(#9262),#2205,.F.);
#88542=ADVANCED_FACE('',(#9263),#2206,.F.);
#88543=ADVANCED_FACE('',(#9264),#2207,.F.);
#88544=ADVANCED_FACE('',(#9265),#85967,.F.);
#88545=ADVANCED_FACE('',(#9266),#2208,.F.);
#88546=ADVANCED_FACE('',(#9267),#2209,.F.);
#88547=ADVANCED_FACE('',(#9268),#2210,.F.);
#88548=ADVANCED_FACE('',(#9269),#2211,.F.);
#88549=ADVANCED_FACE('',(#9270),#85968,.F.);
#88550=ADVANCED_FACE('',(#9271),#2212,.F.);
#88551=ADVANCED_FACE('',(#9272),#2213,.F.);
#88552=ADVANCED_FACE('',(#9273),#85969,.T.);
#88553=ADVANCED_FACE('',(#9274),#7826,.T.);
#88554=ADVANCED_FACE('',(#9275),#85970,.T.);
#88555=ADVANCED_FACE('',(#9276),#2214,.F.);
#88556=ADVANCED_FACE('',(#9277),#2215,.F.);
#88557=ADVANCED_FACE('',(#9278),#2216,.F.);
#88558=ADVANCED_FACE('',(#9279),#85971,.F.);
#88559=ADVANCED_FACE('',(#9280),#2217,.F.);
#88560=ADVANCED_FACE('',(#9281),#2218,.F.);
#88561=ADVANCED_FACE('',(#9282),#2219,.F.);
#88562=ADVANCED_FACE('',(#9283),#2220,.F.);
#88563=ADVANCED_FACE('',(#9284),#85972,.F.);
#88564=ADVANCED_FACE('',(#9285),#2221,.F.);
#88565=ADVANCED_FACE('',(#9286),#2222,.F.);
#88566=ADVANCED_FACE('',(#9287),#3265,.T.);
#88567=ADVANCED_FACE('',(#9288),#85973,.T.);
#88568=ADVANCED_FACE('',(#9289),#3266,.T.);
#88569=ADVANCED_FACE('',(#9290),#85974,.T.);
#88570=ADVANCED_FACE('',(#9291),#3267,.T.);
#88571=ADVANCED_FACE('',(#9292),#2223,.F.);
#88572=ADVANCED_FACE('',(#9293),#2224,.F.);
#88573=ADVANCED_FACE('',(#9294),#2225,.F.);
#88574=ADVANCED_FACE('',(#9295),#85975,.F.);
#88575=ADVANCED_FACE('',(#9296),#2226,.F.);
#88576=ADVANCED_FACE('',(#9297),#85976,.T.);
#88577=ADVANCED_FACE('',(#9298),#3268,.T.);
#88578=ADVANCED_FACE('',(#9299),#2227,.F.);
#88579=ADVANCED_FACE('',(#9300),#2228,.F.);
#88580=ADVANCED_FACE('',(#9301),#2229,.F.);
#88581=ADVANCED_FACE('',(#9302),#85977,.F.);
#88582=ADVANCED_FACE('',(#9303),#2230,.F.);
#88583=ADVANCED_FACE('',(#9304),#2231,.F.);
#88584=ADVANCED_FACE('',(#9305),#3269,.T.);
#88585=ADVANCED_FACE('',(#9306),#85978,.T.);
#88586=ADVANCED_FACE('',(#9307),#3270,.T.);
#88587=ADVANCED_FACE('',(#9308),#6945,.T.);
#88588=ADVANCED_FACE('',(#9309),#2232,.F.);
#88589=ADVANCED_FACE('',(#9310),#2233,.F.);
#88590=ADVANCED_FACE('',(#9311),#2234,.F.);
#88591=ADVANCED_FACE('',(#9312),#2235,.F.);
#88592=ADVANCED_FACE('',(#9313),#85979,.F.);
#88593=ADVANCED_FACE('',(#9314),#3271,.T.);
#88594=ADVANCED_FACE('',(#9315),#85980,.T.);
#88595=ADVANCED_FACE('',(#9316),#3272,.T.);
#88596=ADVANCED_FACE('',(#9317),#85981,.F.);
#88597=ADVANCED_FACE('',(#9318),#2236,.F.);
#88598=ADVANCED_FACE('',(#9319),#2237,.F.);
#88599=ADVANCED_FACE('',(#9320),#2238,.F.);
#88600=ADVANCED_FACE('',(#9321),#2239,.F.);
#88601=ADVANCED_FACE('',(#9322),#2240,.F.);
#88602=ADVANCED_FACE('',(#9323),#2241,.F.);
#88603=ADVANCED_FACE('',(#9324),#3273,.T.);
#88604=ADVANCED_FACE('',(#9325),#85982,.T.);
#88605=ADVANCED_FACE('',(#9326),#3274,.T.);
#88606=ADVANCED_FACE('',(#9327),#3275,.T.);
#88607=ADVANCED_FACE('',(#9328),#85983,.T.);
#88608=ADVANCED_FACE('',(#9329),#3276,.T.);
#88609=ADVANCED_FACE('',(#9330),#85984,.T.);
#88610=ADVANCED_FACE('',(#9331),#85985,.F.);
#88611=ADVANCED_FACE('',(#9332),#2242,.F.);
#88612=ADVANCED_FACE('',(#9333),#2243,.F.);
#88613=ADVANCED_FACE('',(#9334),#2244,.F.);
#88614=ADVANCED_FACE('',(#9335),#85986,.F.);
#88615=ADVANCED_FACE('',(#9336),#2245,.F.);
#88616=ADVANCED_FACE('',(#9337),#2246,.F.);
#88617=ADVANCED_FACE('',(#9338),#85987,.T.);
#88618=ADVANCED_FACE('',(#9339),#3277,.T.);
#88619=ADVANCED_FACE('',(#9340),#2247,.F.);
#88620=ADVANCED_FACE('',(#9341),#2248,.F.);
#88621=ADVANCED_FACE('',(#9342),#2249,.F.);
#88622=ADVANCED_FACE('',(#9343),#85988,.F.);
#88623=ADVANCED_FACE('',(#9344),#2250,.F.);
#88624=ADVANCED_FACE('',(#9345),#2251,.F.);
#88625=ADVANCED_FACE('',(#9346),#2252,.F.);
#88626=ADVANCED_FACE('',(#9347),#85989,.F.);
#88627=ADVANCED_FACE('',(#9348),#85990,.T.);
#88628=ADVANCED_FACE('',(#9349),#3278,.T.);
#88629=ADVANCED_FACE('',(#9350),#85991,.T.);
#88630=ADVANCED_FACE('',(#9351),#3279,.T.);
#88631=ADVANCED_FACE('',(#9352),#85992,.T.);
#88632=ADVANCED_FACE('',(#9353),#3280,.T.);
#88633=ADVANCED_FACE('',(#9354),#2253,.F.);
#88634=ADVANCED_FACE('',(#9355),#85993,.T.);
#88635=ADVANCED_FACE('',(#9356),#3281,.T.);
#88636=ADVANCED_FACE('',(#9357),#85994,.F.);
#88637=ADVANCED_FACE('',(#9358),#2254,.F.);
#88638=ADVANCED_FACE('',(#9359),#2255,.F.);
#88639=ADVANCED_FACE('',(#9360),#2256,.F.);
#88640=ADVANCED_FACE('',(#9361),#85995,.F.);
#88641=ADVANCED_FACE('',(#9362),#2257,.F.);
#88642=ADVANCED_FACE('',(#9363),#2258,.F.);
#88643=ADVANCED_FACE('',(#9364),#2259,.F.);
#88644=ADVANCED_FACE('',(#9365),#2260,.F.);
#88645=ADVANCED_FACE('',(#9366),#85996,.F.);
#88646=ADVANCED_FACE('',(#9367),#2261,.F.);
#88647=ADVANCED_FACE('',(#9368),#2262,.F.);
#88648=ADVANCED_FACE('',(#9369),#2263,.F.);
#88649=ADVANCED_FACE('',(#9370),#85997,.F.);
#88650=ADVANCED_FACE('',(#9371),#2264,.T.);
#88651=ADVANCED_FACE('',(#9372),#85998,.T.);
#88652=ADVANCED_FACE('',(#9373),#7827,.T.);
#88653=ADVANCED_FACE('',(#9374),#85999,.T.);
#88654=ADVANCED_FACE('',(#9375),#2265,.F.);
#88655=ADVANCED_FACE('',(#9376),#2266,.T.);
#88656=ADVANCED_FACE('',(#9377),#86000,.F.);
#88657=ADVANCED_FACE('',(#9378),#2267,.F.);
#88658=ADVANCED_FACE('',(#9379),#2268,.F.);
#88659=ADVANCED_FACE('',(#9380),#2269,.F.);
#88660=ADVANCED_FACE('',(#9381),#86001,.F.);
#88661=ADVANCED_FACE('',(#9382),#2270,.F.);
#88662=ADVANCED_FACE('',(#9383),#2271,.F.);
#88663=ADVANCED_FACE('',(#9384),#2272,.F.);
#88664=ADVANCED_FACE('',(#9385),#2273,.F.);
#88665=ADVANCED_FACE('',(#9386),#86002,.F.);
#88666=ADVANCED_FACE('',(#9387),#2274,.F.);
#88667=ADVANCED_FACE('',(#9388),#2275,.F.);
#88668=ADVANCED_FACE('',(#9389),#2276,.F.);
#88669=ADVANCED_FACE('',(#9390),#86003,.F.);
#88670=ADVANCED_FACE('',(#9391),#2277,.T.);
#88671=ADVANCED_FACE('',(#9392),#86004,.T.);
#88672=ADVANCED_FACE('',(#9393),#7828,.T.);
#88673=ADVANCED_FACE('',(#9394),#86005,.T.);
#88674=ADVANCED_FACE('',(#9395),#2278,.F.);
#88675=ADVANCED_FACE('',(#9396),#2279,.T.);
#88676=ADVANCED_FACE('',(#9397),#86006,.F.);
#88677=ADVANCED_FACE('',(#9398),#2280,.F.);
#88678=ADVANCED_FACE('',(#9399),#2281,.F.);
#88679=ADVANCED_FACE('',(#9400),#2282,.F.);
#88680=ADVANCED_FACE('',(#9401),#86007,.F.);
#88681=ADVANCED_FACE('',(#9402),#2283,.F.);
#88682=ADVANCED_FACE('',(#9403),#2284,.F.);
#88683=ADVANCED_FACE('',(#9404),#2285,.F.);
#88684=ADVANCED_FACE('',(#9405),#2286,.F.);
#88685=ADVANCED_FACE('',(#9406),#86008,.F.);
#88686=ADVANCED_FACE('',(#9407),#2287,.F.);
#88687=ADVANCED_FACE('',(#9408),#2288,.F.);
#88688=ADVANCED_FACE('',(#9409),#2289,.F.);
#88689=ADVANCED_FACE('',(#9410),#86009,.F.);
#88690=ADVANCED_FACE('',(#9411),#2290,.T.);
#88691=ADVANCED_FACE('',(#9412),#86010,.T.);
#88692=ADVANCED_FACE('',(#9413),#7829,.T.);
#88693=ADVANCED_FACE('',(#9414),#86011,.T.);
#88694=ADVANCED_FACE('',(#9415),#2291,.F.);
#88695=ADVANCED_FACE('',(#9416),#2292,.T.);
#88696=ADVANCED_FACE('',(#9417),#86012,.F.);
#88697=ADVANCED_FACE('',(#9418),#2293,.F.);
#88698=ADVANCED_FACE('',(#9419),#2294,.F.);
#88699=ADVANCED_FACE('',(#9420),#2295,.F.);
#88700=ADVANCED_FACE('',(#9421),#86013,.F.);
#88701=ADVANCED_FACE('',(#9422),#2296,.F.);
#88702=ADVANCED_FACE('',(#9423),#2297,.F.);
#88703=ADVANCED_FACE('',(#9424),#2298,.F.);
#88704=ADVANCED_FACE('',(#9425),#2299,.F.);
#88705=ADVANCED_FACE('',(#9426),#86014,.F.);
#88706=ADVANCED_FACE('',(#9427),#2300,.F.);
#88707=ADVANCED_FACE('',(#9428),#2301,.F.);
#88708=ADVANCED_FACE('',(#9429),#2302,.F.);
#88709=ADVANCED_FACE('',(#9430),#86015,.F.);
#88710=ADVANCED_FACE('',(#9431),#3282,.T.);
#88711=ADVANCED_FACE('',(#9432),#86016,.T.);
#88712=ADVANCED_FACE('',(#9433),#3283,.T.);
#88713=ADVANCED_FACE('',(#9434),#86017,.T.);
#88714=ADVANCED_FACE('',(#9435),#3284,.T.);
#88715=ADVANCED_FACE('',(#9436),#2303,.F.);
#88716=ADVANCED_FACE('',(#9437),#86018,.T.);
#88717=ADVANCED_FACE('',(#9438),#3285,.T.);
#88718=ADVANCED_FACE('',(#9439),#86019,.T.);
#88719=ADVANCED_FACE('',(#9440),#86020,.F.);
#88720=ADVANCED_FACE('',(#9441),#2304,.F.);
#88721=ADVANCED_FACE('',(#9442),#2305,.F.);
#88722=ADVANCED_FACE('',(#9443),#2306,.F.);
#88723=ADVANCED_FACE('',(#9444),#86021,.F.);
#88724=ADVANCED_FACE('',(#9445),#2307,.F.);
#88725=ADVANCED_FACE('',(#9446),#2308,.F.);
#88726=ADVANCED_FACE('',(#9447),#2309,.F.);
#88727=ADVANCED_FACE('',(#9448),#2310,.F.);
#88728=ADVANCED_FACE('',(#9449),#86022,.F.);
#88729=ADVANCED_FACE('',(#9450),#86023,.T.);
#88730=ADVANCED_FACE('',(#9451),#3286,.T.);
#88731=ADVANCED_FACE('',(#9452),#86024,.T.);
#88732=ADVANCED_FACE('',(#9453),#2311,.F.);
#88733=ADVANCED_FACE('',(#9454),#86025,.F.);
#88734=ADVANCED_FACE('',(#9455),#2312,.F.);
#88735=ADVANCED_FACE('',(#9456),#2313,.F.);
#88736=ADVANCED_FACE('',(#9457),#2314,.F.);
#88737=ADVANCED_FACE('',(#9458),#86026,.F.);
#88738=ADVANCED_FACE('',(#9459),#86027,.F.);
#88739=ADVANCED_FACE('',(#9460),#3287,.F.);
#88740=ADVANCED_FACE('',(#9461),#2315,.F.);
#88741=ADVANCED_FACE('',(#9462),#86028,.F.);
#88742=ADVANCED_FACE('',(#9463),#86029,.T.);
#88743=ADVANCED_FACE('',(#9464),#3288,.T.);
#88744=ADVANCED_FACE('',(#9465),#86030,.T.);
#88745=ADVANCED_FACE('',(#9466),#3289,.T.);
#88746=ADVANCED_FACE('',(#9467),#2316,.F.);
#88747=ADVANCED_FACE('',(#9468),#2317,.F.);
#88748=ADVANCED_FACE('',(#9469),#86031,.F.);
#88749=ADVANCED_FACE('',(#9470),#2318,.F.);
#88750=ADVANCED_FACE('',(#9471),#2319,.F.);
#88751=ADVANCED_FACE('',(#9472),#2320,.F.);
#88752=ADVANCED_FACE('',(#9473),#86032,.F.);
#88753=ADVANCED_FACE('',(#9474),#86033,.T.);
#88754=ADVANCED_FACE('',(#9475),#3290,.T.);
#88755=ADVANCED_FACE('',(#9476),#86034,.F.);
#88756=ADVANCED_FACE('',(#9477),#86035,.F.);
#88757=ADVANCED_FACE('',(#9478),#86036,.F.);
#88758=ADVANCED_FACE('',(#9479),#2321,.F.);
#88759=ADVANCED_FACE('',(#9480),#86037,.T.);
#88760=ADVANCED_FACE('',(#9481),#3291,.T.);
#88761=ADVANCED_FACE('',(#9482),#86038,.T.);
#88762=ADVANCED_FACE('',(#9483),#86039,.F.);
#88763=ADVANCED_FACE('',(#9484),#2322,.F.);
#88764=ADVANCED_FACE('',(#9485),#86040,.F.);
#88765=ADVANCED_FACE('',(#9486),#2323,.F.);
#88766=ADVANCED_FACE('',(#9487),#2324,.F.);
#88767=ADVANCED_FACE('',(#9488),#2325,.F.);
#88768=ADVANCED_FACE('',(#9489),#2326,.F.);
#88769=ADVANCED_FACE('',(#9490),#2327,.F.);
#88770=ADVANCED_FACE('',(#9491),#86041,.F.);
#88771=ADVANCED_FACE('',(#9492),#2328,.F.);
#88772=ADVANCED_FACE('',(#9493),#2329,.F.);
#88773=ADVANCED_FACE('',(#9494),#86042,.T.);
#88774=ADVANCED_FACE('',(#9495),#3292,.T.);
#88775=ADVANCED_FACE('',(#9496),#6946,.T.);
#88776=ADVANCED_FACE('',(#9497),#2330,.F.);
#88777=ADVANCED_FACE('',(#9498),#86043,.F.);
#88778=ADVANCED_FACE('',(#9499),#2331,.F.);
#88779=ADVANCED_FACE('',(#9500),#2332,.F.);
#88780=ADVANCED_FACE('',(#9501),#86044,.F.);
#88781=ADVANCED_FACE('',(#9502),#2333,.F.);
#88782=ADVANCED_FACE('',(#9503),#2334,.F.);
#88783=ADVANCED_FACE('',(#9504),#2335,.F.);
#88784=ADVANCED_FACE('',(#9505),#86045,.F.);
#88785=ADVANCED_FACE('',(#9506),#2336,.F.);
#88786=ADVANCED_FACE('',(#9507),#86046,.F.);
#88787=ADVANCED_FACE('',(#9508),#86047,.T.);
#88788=ADVANCED_FACE('',(#9509),#3293,.T.);
#88789=ADVANCED_FACE('',(#9510),#86048,.T.);
#88790=ADVANCED_FACE('',(#9511),#3294,.T.);
#88791=ADVANCED_FACE('',(#9512),#86049,.T.);
#88792=ADVANCED_FACE('',(#9513),#3295,.T.);
#88793=ADVANCED_FACE('',(#9514),#86050,.T.);
#88794=ADVANCED_FACE('',(#9515),#86051,.F.);
#88795=ADVANCED_FACE('',(#9516),#2337,.F.);
#88796=ADVANCED_FACE('',(#9517),#86052,.F.);
#88797=ADVANCED_FACE('',(#9518),#2338,.F.);
#88798=ADVANCED_FACE('',(#9519),#2339,.F.);
#88799=ADVANCED_FACE('',(#9520),#2340,.F.);
#88800=ADVANCED_FACE('',(#9521),#86053,.F.);
#88801=ADVANCED_FACE('',(#9522),#2341,.F.);
#88802=ADVANCED_FACE('',(#9523),#2342,.F.);
#88803=ADVANCED_FACE('',(#9524),#2343,.F.);
#88804=ADVANCED_FACE('',(#9525),#86054,.T.);
#88805=ADVANCED_FACE('',(#9526),#3296,.T.);
#88806=ADVANCED_FACE('',(#9527),#3297,.F.);
#88807=ADVANCED_FACE('',(#9528),#86055,.F.);
#88808=ADVANCED_FACE('',(#9529),#86056,.F.);
#88809=ADVANCED_FACE('',(#9530),#2344,.F.);
#88810=ADVANCED_FACE('',(#9531),#2345,.F.);
#88811=ADVANCED_FACE('',(#9532),#2346,.F.);
#88812=ADVANCED_FACE('',(#9533),#86057,.F.);
#88813=ADVANCED_FACE('',(#9534),#3298,.T.);
#88814=ADVANCED_FACE('',(#9535),#86058,.T.);
#88815=ADVANCED_FACE('',(#9536),#3299,.T.);
#88816=ADVANCED_FACE('',(#9537),#86059,.F.);
#88817=ADVANCED_FACE('',(#9538),#2347,.F.);
#88818=ADVANCED_FACE('',(#9539),#2348,.F.);
#88819=ADVANCED_FACE('',(#9540),#86060,.F.);
#88820=ADVANCED_FACE('',(#9541),#86061,.T.);
#88821=ADVANCED_FACE('',(#9542),#3300,.T.);
#88822=ADVANCED_FACE('',(#9543),#86062,.T.);
#88823=ADVANCED_FACE('',(#9544),#3301,.T.);
#88824=ADVANCED_FACE('',(#9545),#86063,.F.);
#88825=ADVANCED_FACE('',(#9546),#2349,.F.);
#88826=ADVANCED_FACE('',(#9547),#2350,.F.);
#88827=ADVANCED_FACE('',(#9548),#2351,.F.);
#88828=ADVANCED_FACE('',(#9549),#3302,.F.);
#88829=ADVANCED_FACE('',(#9550),#86064,.F.);
#88830=ADVANCED_FACE('',(#9551),#86065,.F.);
#88831=ADVANCED_FACE('',(#9552),#2352,.F.);
#88832=ADVANCED_FACE('',(#9553),#86066,.F.);
#88833=ADVANCED_FACE('',(#9554),#86067,.T.);
#88834=ADVANCED_FACE('',(#9555),#3303,.T.);
#88835=ADVANCED_FACE('',(#9556),#86068,.T.);
#88836=ADVANCED_FACE('',(#9557),#3304,.T.);
#88837=ADVANCED_FACE('',(#9558),#2353,.F.);
#88838=ADVANCED_FACE('',(#9559),#2354,.F.);
#88839=ADVANCED_FACE('',(#9560),#2355,.F.);
#88840=ADVANCED_FACE('',(#9561),#86069,.F.);
#88841=ADVANCED_FACE('',(#9562),#2356,.F.);
#88842=ADVANCED_FACE('',(#9563),#2357,.F.);
#88843=ADVANCED_FACE('',(#9564),#2358,.F.);
#88844=ADVANCED_FACE('',(#9565),#86070,.F.);
#88845=ADVANCED_FACE('',(#9566),#86071,.T.);
#88846=ADVANCED_FACE('',(#9567),#3305,.T.);
#88847=ADVANCED_FACE('',(#9568),#86072,.F.);
#88848=ADVANCED_FACE('',(#9569),#2359,.F.);
#88849=ADVANCED_FACE('',(#9570),#86073,.T.);
#88850=ADVANCED_FACE('',(#9571),#3306,.T.);
#88851=ADVANCED_FACE('',(#9572),#86074,.T.);
#88852=ADVANCED_FACE('',(#9573),#86075,.F.);
#88853=ADVANCED_FACE('',(#9574),#2360,.F.);
#88854=ADVANCED_FACE('',(#9575),#86076,.F.);
#88855=ADVANCED_FACE('',(#9576),#86077,.F.);
#88856=ADVANCED_FACE('',(#9577),#86078,.T.);
#88857=ADVANCED_FACE('',(#9578),#86079,.F.);
#88858=ADVANCED_FACE('',(#9579),#2361,.F.);
#88859=ADVANCED_FACE('',(#9580),#2362,.F.);
#88860=ADVANCED_FACE('',(#9581),#2363,.F.);
#88861=ADVANCED_FACE('',(#9582),#2364,.F.);
#88862=ADVANCED_FACE('',(#9583),#86080,.F.);
#88863=ADVANCED_FACE('',(#9584),#2365,.F.);
#88864=ADVANCED_FACE('',(#9585),#2366,.F.);
#88865=ADVANCED_FACE('',(#9586),#2367,.F.);
#88866=ADVANCED_FACE('',(#9587),#2368,.F.);
#88867=ADVANCED_FACE('',(#9588),#86081,.T.);
#88868=ADVANCED_FACE('',(#9589),#3307,.T.);
#88869=ADVANCED_FACE('',(#9590),#6947,.T.);
#88870=ADVANCED_FACE('',(#9591),#2369,.F.);
#88871=ADVANCED_FACE('',(#9592),#86082,.F.);
#88872=ADVANCED_FACE('',(#9593),#2370,.F.);
#88873=ADVANCED_FACE('',(#9594),#2371,.F.);
#88874=ADVANCED_FACE('',(#9595),#86083,.F.);
#88875=ADVANCED_FACE('',(#9596),#2372,.F.);
#88876=ADVANCED_FACE('',(#9597),#2373,.F.);
#88877=ADVANCED_FACE('',(#9598),#2374,.F.);
#88878=ADVANCED_FACE('',(#9599),#86084,.F.);
#88879=ADVANCED_FACE('',(#9600),#2375,.F.);
#88880=ADVANCED_FACE('',(#9601),#86085,.F.);
#88881=ADVANCED_FACE('',(#9602),#86086,.T.);
#88882=ADVANCED_FACE('',(#9603),#3308,.T.);
#88883=ADVANCED_FACE('',(#9604),#86087,.T.);
#88884=ADVANCED_FACE('',(#9605),#3309,.T.);
#88885=ADVANCED_FACE('',(#9606),#86088,.T.);
#88886=ADVANCED_FACE('',(#9607),#3310,.T.);
#88887=ADVANCED_FACE('',(#9608),#86089,.T.);
#88888=ADVANCED_FACE('',(#9609),#86090,.F.);
#88889=ADVANCED_FACE('',(#9610),#2376,.F.);
#88890=ADVANCED_FACE('',(#9611),#86091,.F.);
#88891=ADVANCED_FACE('',(#9612),#2377,.F.);
#88892=ADVANCED_FACE('',(#9613),#2378,.F.);
#88893=ADVANCED_FACE('',(#9614),#2379,.F.);
#88894=ADVANCED_FACE('',(#9615),#86092,.F.);
#88895=ADVANCED_FACE('',(#9616),#2380,.F.);
#88896=ADVANCED_FACE('',(#9617),#2381,.F.);
#88897=ADVANCED_FACE('',(#9618),#2382,.F.);
#88898=ADVANCED_FACE('',(#9619),#86093,.T.);
#88899=ADVANCED_FACE('',(#9620),#3311,.T.);
#88900=ADVANCED_FACE('',(#9621),#6948,.T.);
#88901=ADVANCED_FACE('',(#9622),#2383,.F.);
#88902=ADVANCED_FACE('',(#9623),#2384,.F.);
#88903=ADVANCED_FACE('',(#9624),#2385,.F.);
#88904=ADVANCED_FACE('',(#9625),#86094,.F.);
#88905=ADVANCED_FACE('',(#9626),#86095,.T.);
#88906=ADVANCED_FACE('',(#9627),#3312,.T.);
#88907=ADVANCED_FACE('',(#9628),#86096,.T.);
#88908=ADVANCED_FACE('',(#9629),#2386,.F.);
#88909=ADVANCED_FACE('',(#9630),#2387,.F.);
#88910=ADVANCED_FACE('',(#9631),#86097,.F.);
#88911=ADVANCED_FACE('',(#9632),#2388,.F.);
#88912=ADVANCED_FACE('',(#9633),#2389,.F.);
#88913=ADVANCED_FACE('',(#9634),#2390,.F.);
#88914=ADVANCED_FACE('',(#9635),#2391,.F.);
#88915=ADVANCED_FACE('',(#9636),#86098,.F.);
#88916=ADVANCED_FACE('',(#9637),#86099,.T.);
#88917=ADVANCED_FACE('',(#9638),#3313,.T.);
#88918=ADVANCED_FACE('',(#9639),#86100,.T.);
#88919=ADVANCED_FACE('',(#9640),#3314,.T.);
#88920=ADVANCED_FACE('',(#9641),#2392,.F.);
#88921=ADVANCED_FACE('',(#9642),#86101,.F.);
#88922=ADVANCED_FACE('',(#9643),#86102,.F.);
#88923=ADVANCED_FACE('',(#9644),#86103,.F.);
#88924=ADVANCED_FACE('',(#9645),#86104,.T.);
#88925=ADVANCED_FACE('',(#9646),#3315,.T.);
#88926=ADVANCED_FACE('',(#9647),#86105,.T.);
#88927=ADVANCED_FACE('',(#9648),#86106,.F.);
#88928=ADVANCED_FACE('',(#9649),#2393,.F.);
#88929=ADVANCED_FACE('',(#9650),#86107,.F.);
#88930=ADVANCED_FACE('',(#9651),#2394,.F.);
#88931=ADVANCED_FACE('',(#9652),#2395,.F.);
#88932=ADVANCED_FACE('',(#9653),#2396,.F.);
#88933=ADVANCED_FACE('',(#9654),#86108,.F.);
#88934=ADVANCED_FACE('',(#9655),#2397,.F.);
#88935=ADVANCED_FACE('',(#9656),#2398,.F.);
#88936=ADVANCED_FACE('',(#9657),#2399,.F.);
#88937=ADVANCED_FACE('',(#9658),#86109,.F.);
#88938=ADVANCED_FACE('',(#9659),#86110,.T.);
#88939=ADVANCED_FACE('',(#9660),#3316,.T.);
#88940=ADVANCED_FACE('',(#9661),#3317,.F.);
#88941=ADVANCED_FACE('',(#9662),#86111,.F.);
#88942=ADVANCED_FACE('',(#9663),#2400,.F.);
#88943=ADVANCED_FACE('',(#9664),#2401,.F.);
#88944=ADVANCED_FACE('',(#9665),#2402,.F.);
#88945=ADVANCED_FACE('',(#9666),#86112,.F.);
#88946=ADVANCED_FACE('',(#9667),#2403,.F.);
#88947=ADVANCED_FACE('',(#9668),#2404,.F.);
#88948=ADVANCED_FACE('',(#9669),#2405,.F.);
#88949=ADVANCED_FACE('',(#9670),#86113,.F.);
#88950=ADVANCED_FACE('',(#9671),#2406,.F.);
#88951=ADVANCED_FACE('',(#9672),#86114,.F.);
#88952=ADVANCED_FACE('',(#9673),#86115,.T.);
#88953=ADVANCED_FACE('',(#9674),#3318,.T.);
#88954=ADVANCED_FACE('',(#9675),#86116,.T.);
#88955=ADVANCED_FACE('',(#9676),#3319,.T.);
#88956=ADVANCED_FACE('',(#9677),#86117,.T.);
#88957=ADVANCED_FACE('',(#9678),#3320,.T.);
#88958=ADVANCED_FACE('',(#9679),#86118,.F.);
#88959=ADVANCED_FACE('',(#9680),#86119,.T.);
#88960=ADVANCED_FACE('',(#9681),#86120,.F.);
#88961=ADVANCED_FACE('',(#9682),#2407,.F.);
#88962=ADVANCED_FACE('',(#9683),#86121,.F.);
#88963=ADVANCED_FACE('',(#9684),#2408,.F.);
#88964=ADVANCED_FACE('',(#9685),#2409,.F.);
#88965=ADVANCED_FACE('',(#9686),#2410,.F.);
#88966=ADVANCED_FACE('',(#9687),#86122,.F.);
#88967=ADVANCED_FACE('',(#9688),#2411,.F.);
#88968=ADVANCED_FACE('',(#9689),#2412,.F.);
#88969=ADVANCED_FACE('',(#9690),#86123,.T.);
#88970=ADVANCED_FACE('',(#9691),#3321,.T.);
#88971=ADVANCED_FACE('',(#9692),#7830,.T.);
#88972=ADVANCED_FACE('',(#9693),#86124,.T.);
#88973=ADVANCED_FACE('',(#9694),#7831,.T.);
#88974=ADVANCED_FACE('',(#9695),#2413,.F.);
#88975=ADVANCED_FACE('',(#9696),#2414,.F.);
#88976=ADVANCED_FACE('',(#9697),#1016,.F.);
#88977=ADVANCED_FACE('',(#9698),#86125,.T.);
#88978=ADVANCED_FACE('',(#9699),#3322,.T.);
#88979=ADVANCED_FACE('',(#9700),#3323,.T.);
#88980=ADVANCED_FACE('',(#9701),#3324,.T.);
#88981=ADVANCED_FACE('',(#9702),#86126,.T.);
#88982=ADVANCED_FACE('',(#9703),#2415,.F.);
#88983=ADVANCED_FACE('',(#9704),#86127,.F.);
#88984=ADVANCED_FACE('',(#9705),#2416,.F.);
#88985=ADVANCED_FACE('',(#9706),#86128,.T.);
#88986=ADVANCED_FACE('',(#9707),#2417,.F.);
#88987=ADVANCED_FACE('',(#9708),#86129,.F.);
#88988=ADVANCED_FACE('',(#9709),#2418,.F.);
#88989=ADVANCED_FACE('',(#9710),#86130,.T.);
#88990=ADVANCED_FACE('',(#9711),#2419,.T.);
#88991=ADVANCED_FACE('',(#9712),#2420,.F.);
#88992=ADVANCED_FACE('',(#9713),#2421,.T.);
#88993=ADVANCED_FACE('',(#9714),#2422,.F.);
#88994=ADVANCED_FACE('',(#9715),#3325,.F.);
#88995=ADVANCED_FACE('',(#9716),#2423,.F.);
#88996=ADVANCED_FACE('',(#9717),#3326,.T.);
#88997=ADVANCED_FACE('',(#9718),#2424,.F.);
#88998=ADVANCED_FACE('',(#9719),#3327,.F.);
#88999=ADVANCED_FACE('',(#9720),#2425,.F.);
#89000=ADVANCED_FACE('',(#9721),#2426,.F.);
#89001=ADVANCED_FACE('',(#9722),#3328,.T.);
#89002=ADVANCED_FACE('',(#9723),#2427,.F.);
#89003=ADVANCED_FACE('',(#9724),#2428,.F.);
#89004=ADVANCED_FACE('',(#9725),#2429,.F.);
#89005=ADVANCED_FACE('',(#9726),#3329,.T.);
#89006=ADVANCED_FACE('',(#9727),#2430,.F.);
#89007=ADVANCED_FACE('',(#9728),#2431,.F.);
#89008=ADVANCED_FACE('',(#9729),#2432,.F.);
#89009=ADVANCED_FACE('',(#9730),#3330,.T.);
#89010=ADVANCED_FACE('',(#9731),#2433,.F.);
#89011=ADVANCED_FACE('',(#9732),#2434,.F.);
#89012=ADVANCED_FACE('',(#9733),#2435,.F.);
#89013=ADVANCED_FACE('',(#9734),#3331,.T.);
#89014=ADVANCED_FACE('',(#9735),#2436,.F.);
#89015=ADVANCED_FACE('',(#9736),#2437,.F.);
#89016=ADVANCED_FACE('',(#9737),#3332,.F.);
#89017=ADVANCED_FACE('',(#9738),#2438,.F.);
#89018=ADVANCED_FACE('',(#9739),#3333,.T.);
#89019=ADVANCED_FACE('',(#9740),#2439,.F.);
#89020=ADVANCED_FACE('',(#9741),#3334,.F.);
#89021=ADVANCED_FACE('',(#9742),#2440,.F.);
#89022=ADVANCED_FACE('',(#9743),#2441,.F.);
#89023=ADVANCED_FACE('',(#9744),#2442,.T.);
#89024=ADVANCED_FACE('',(#9745),#86131,.T.);
#89025=ADVANCED_FACE('',(#9746),#2443,.F.);
#89026=ADVANCED_FACE('',(#9747),#86132,.F.);
#89027=ADVANCED_FACE('',(#9748),#2444,.F.);
#89028=ADVANCED_FACE('',(#9749),#86133,.T.);
#89029=ADVANCED_FACE('',(#9750),#2445,.T.);
#89030=ADVANCED_FACE('',(#9751),#86134,.T.);
#89031=ADVANCED_FACE('',(#9752),#2446,.F.);
#89032=ADVANCED_FACE('',(#9753),#86135,.F.);
#89033=ADVANCED_FACE('',(#9754),#2447,.F.);
#89034=ADVANCED_FACE('',(#9755),#3335,.T.);
#89035=ADVANCED_FACE('',(#9756),#3336,.T.);
#89036=ADVANCED_FACE('',(#9757),#3337,.T.);
#89037=ADVANCED_FACE('',(#9758),#86136,.T.);
#89038=ADVANCED_FACE('',(#9759),#2448,.F.);
#89039=ADVANCED_FACE('',(#9760),#86137,.F.);
#89040=ADVANCED_FACE('',(#9761),#2449,.F.);
#89041=ADVANCED_FACE('',(#9762),#86138,.T.);
#89042=ADVANCED_FACE('',(#9763),#2450,.F.);
#89043=ADVANCED_FACE('',(#9764),#86139,.F.);
#89044=ADVANCED_FACE('',(#9765),#2451,.F.);
#89045=ADVANCED_FACE('',(#9766),#86140,.T.);
#89046=ADVANCED_FACE('',(#9767),#2452,.T.);
#89047=ADVANCED_FACE('',(#9768),#2453,.T.);
#89048=ADVANCED_FACE('',(#9769),#2454,.F.);
#89049=ADVANCED_FACE('',(#9770),#86141,.T.);
#89050=ADVANCED_FACE('',(#9771),#2455,.F.);
#89051=ADVANCED_FACE('',(#9772),#2456,.F.);
#89052=ADVANCED_FACE('',(#9773),#3338,.F.);
#89053=ADVANCED_FACE('',(#9774),#86142,.T.);
#89054=ADVANCED_FACE('',(#9775),#7832,.F.);
#89055=ADVANCED_FACE('',(#9776),#7833,.F.);
#89056=ADVANCED_FACE('',(#9777),#7834,.T.);
#89057=ADVANCED_FACE('',(#9778),#7835,.F.);
#89058=ADVANCED_FACE('',(#9779),#7836,.T.);
#89059=ADVANCED_FACE('',(#9780),#7837,.T.);
#89060=ADVANCED_FACE('',(#9781),#7838,.F.);
#89061=ADVANCED_FACE('',(#9782),#6949,.T.);
#89062=ADVANCED_FACE('',(#9783),#2457,.F.);
#89063=ADVANCED_FACE('',(#9784),#7839,.T.);
#89064=ADVANCED_FACE('',(#9785),#86143,.T.);
#89065=ADVANCED_FACE('',(#9786),#7840,.F.);
#89066=ADVANCED_FACE('',(#9787),#86144,.T.);
#89067=ADVANCED_FACE('',(#9788),#7841,.T.);
#89068=ADVANCED_FACE('',(#9789),#86145,.T.);
#89069=ADVANCED_FACE('',(#9790),#6950,.T.);
#89070=ADVANCED_FACE('',(#9791),#2458,.F.);
#89071=ADVANCED_FACE('',(#9792),#7842,.T.);
#89072=ADVANCED_FACE('',(#9793),#2459,.T.);
#89073=ADVANCED_FACE('',(#9794),#6951,.T.);
#89074=ADVANCED_FACE('',(#9795),#2460,.F.);
#89075=ADVANCED_FACE('',(#9796),#7843,.T.);
#89076=ADVANCED_FACE('',(#9797),#2461,.T.);
#89077=ADVANCED_FACE('',(#9798),#6952,.T.);
#89078=ADVANCED_FACE('',(#9799),#2462,.F.);
#89079=ADVANCED_FACE('',(#9800),#7844,.T.);
#89080=ADVANCED_FACE('',(#9801),#2463,.T.);
#89081=ADVANCED_FACE('',(#9802),#6953,.T.);
#89082=ADVANCED_FACE('',(#9803),#2464,.F.);
#89083=ADVANCED_FACE('',(#9804),#7845,.T.);
#89084=ADVANCED_FACE('',(#9805),#86146,.T.);
#89085=ADVANCED_FACE('',(#9806),#86147,.T.);
#89086=ADVANCED_FACE('',(#9807),#7846,.T.);
#89087=ADVANCED_FACE('',(#9808),#7847,.F.);
#89088=ADVANCED_FACE('',(#9809),#6954,.T.);
#89089=ADVANCED_FACE('',(#9810),#2465,.F.);
#89090=ADVANCED_FACE('',(#9811),#7848,.T.);
#89091=ADVANCED_FACE('',(#9812),#7849,.F.);
#89092=ADVANCED_FACE('',(#9813),#86148,.T.);
#89093=ADVANCED_FACE('',(#9814),#2466,.F.);
#89094=ADVANCED_FACE('',(#9815),#6955,.T.);
#89095=ADVANCED_FACE('',(#9816),#7850,.F.);
#89096=ADVANCED_FACE('',(#9817),#86149,.T.);
#89097=ADVANCED_FACE('',(#9818),#7851,.T.);
#89098=ADVANCED_FACE('',(#9819),#7852,.F.);
#89099=ADVANCED_FACE('',(#9820),#2467,.F.);
#89100=ADVANCED_FACE('',(#9821),#2468,.F.);
#89101=ADVANCED_FACE('',(#9822),#3339,.F.);
#89102=ADVANCED_FACE('',(#9823),#7853,.F.);
#89103=ADVANCED_FACE('',(#9824),#2469,.T.);
#89104=ADVANCED_FACE('',(#9825),#6956,.T.);
#89105=ADVANCED_FACE('',(#9826),#2470,.F.);
#89106=ADVANCED_FACE('',(#9827),#7854,.F.);
#89107=ADVANCED_FACE('',(#9828),#2471,.F.);
#89108=ADVANCED_FACE('',(#9829),#7855,.F.);
#89109=ADVANCED_FACE('',(#9830),#7856,.F.);
#89110=ADVANCED_FACE('',(#9831),#86150,.T.);
#89111=ADVANCED_FACE('',(#9832),#7857,.T.);
#89112=ADVANCED_FACE('',(#9833),#6957,.T.);
#89113=ADVANCED_FACE('',(#9834),#6958,.T.);
#89114=ADVANCED_FACE('',(#9835),#6959,.T.);
#89115=ADVANCED_FACE('',(#9836),#7858,.F.);
#89116=ADVANCED_FACE('',(#9837),#86151,.T.);
#89117=ADVANCED_FACE('',(#9838),#7859,.T.);
#89118=ADVANCED_FACE('',(#9839),#2472,.F.);
#89119=ADVANCED_FACE('',(#9840),#7860,.T.);
#89120=ADVANCED_FACE('',(#9841),#2473,.F.);
#89121=ADVANCED_FACE('',(#9842),#6960,.T.);
#89122=ADVANCED_FACE('',(#9843),#3340,.F.);
#89123=ADVANCED_FACE('',(#9844),#7861,.F.);
#89124=ADVANCED_FACE('',(#9845),#3341,.F.);
#89125=ADVANCED_FACE('',(#9846),#6961,.T.);
#89126=ADVANCED_FACE('',(#9847),#2474,.F.);
#89127=ADVANCED_FACE('',(#9848),#7862,.T.);
#89128=ADVANCED_FACE('',(#9849),#2475,.F.);
#89129=ADVANCED_FACE('',(#9850),#7863,.F.);
#89130=ADVANCED_FACE('',(#9851),#7864,.F.);
#89131=ADVANCED_FACE('',(#9852),#86152,.T.);
#89132=ADVANCED_FACE('',(#9853),#7865,.T.);
#89133=ADVANCED_FACE('',(#9854),#2476,.F.);
#89134=ADVANCED_FACE('',(#9855),#7866,.T.);
#89135=ADVANCED_FACE('',(#9856),#2477,.F.);
#89136=ADVANCED_FACE('',(#9857),#6962,.T.);
#89137=ADVANCED_FACE('',(#9858),#3342,.F.);
#89138=ADVANCED_FACE('',(#9859),#7867,.F.);
#89139=ADVANCED_FACE('',(#9860),#86153,.T.);
#89140=ADVANCED_FACE('',(#9861),#7868,.T.);
#89141=ADVANCED_FACE('',(#9862),#7869,.F.);
#89142=ADVANCED_FACE('',(#9863),#3343,.F.);
#89143=ADVANCED_FACE('',(#9864),#6963,.T.);
#89144=ADVANCED_FACE('',(#9865),#2478,.F.);
#89145=ADVANCED_FACE('',(#9866),#7870,.T.);
#89146=ADVANCED_FACE('',(#9867),#2479,.F.);
#89147=ADVANCED_FACE('',(#9868),#6964,.T.);
#89148=ADVANCED_FACE('',(#9869),#7871,.F.);
#89149=ADVANCED_FACE('',(#9870),#86154,.T.);
#89150=ADVANCED_FACE('',(#9871),#7872,.T.);
#89151=ADVANCED_FACE('',(#9872),#7873,.F.);
#89152=ADVANCED_FACE('',(#9873),#7874,.F.);
#89153=ADVANCED_FACE('',(#9874),#7875,.T.);
#89154=ADVANCED_FACE('',(#9875),#86155,.T.);
#89155=ADVANCED_FACE('',(#9876),#7876,.F.);
#89156=ADVANCED_FACE('',(#9877),#6965,.T.);
#89157=ADVANCED_FACE('',(#9878),#2480,.F.);
#89158=ADVANCED_FACE('',(#9879),#7877,.T.);
#89159=ADVANCED_FACE('',(#9880),#2481,.F.);
#89160=ADVANCED_FACE('',(#9881),#6966,.T.);
#89161=ADVANCED_FACE('',(#9882),#3344,.F.);
#89162=ADVANCED_FACE('',(#9883),#7878,.F.);
#89163=ADVANCED_FACE('',(#9884),#7879,.T.);
#89164=ADVANCED_FACE('',(#9885),#86156,.T.);
#89165=ADVANCED_FACE('',(#9886),#7880,.F.);
#89166=ADVANCED_FACE('',(#9887),#3345,.F.);
#89167=ADVANCED_FACE('',(#9888),#6967,.T.);
#89168=ADVANCED_FACE('',(#9889),#2482,.F.);
#89169=ADVANCED_FACE('',(#9890),#7881,.T.);
#89170=ADVANCED_FACE('',(#9891),#2483,.F.);
#89171=ADVANCED_FACE('',(#9892),#7882,.T.);
#89172=ADVANCED_FACE('',(#9893),#86157,.T.);
#89173=ADVANCED_FACE('',(#9894),#7883,.F.);
#89174=ADVANCED_FACE('',(#9895),#7884,.F.);
#89175=ADVANCED_FACE('',(#9896),#2484,.F.);
#89176=ADVANCED_FACE('',(#9897),#7885,.T.);
#89177=ADVANCED_FACE('',(#9898),#2485,.F.);
#89178=ADVANCED_FACE('',(#9899),#6968,.T.);
#89179=ADVANCED_FACE('',(#9900),#3346,.F.);
#89180=ADVANCED_FACE('',(#9901),#7886,.F.);
#89181=ADVANCED_FACE('',(#9902),#3347,.F.);
#89182=ADVANCED_FACE('',(#9903),#6969,.T.);
#89183=ADVANCED_FACE('',(#9904),#2486,.F.);
#89184=ADVANCED_FACE('',(#9905),#7887,.T.);
#89185=ADVANCED_FACE('',(#9906),#2487,.F.);
#89186=ADVANCED_FACE('',(#9907),#7888,.T.);
#89187=ADVANCED_FACE('',(#9908),#86158,.T.);
#89188=ADVANCED_FACE('',(#9909),#7889,.F.);
#89189=ADVANCED_FACE('',(#9910),#6970,.T.);
#89190=ADVANCED_FACE('',(#9911),#6971,.T.);
#89191=ADVANCED_FACE('',(#9912),#6972,.T.);
#89192=ADVANCED_FACE('',(#9913),#7890,.T.);
#89193=ADVANCED_FACE('',(#9914),#86159,.T.);
#89194=ADVANCED_FACE('',(#9915),#7891,.F.);
#89195=ADVANCED_FACE('',(#9916),#7892,.F.);
#89196=ADVANCED_FACE('',(#9917),#2488,.F.);
#89197=ADVANCED_FACE('',(#9918),#7893,.F.);
#89198=ADVANCED_FACE('',(#9919),#2489,.F.);
#89199=ADVANCED_FACE('',(#9920),#6973,.T.);
#89200=ADVANCED_FACE('',(#9921),#2490,.T.);
#89201=ADVANCED_FACE('',(#9922),#7894,.F.);
#89202=ADVANCED_FACE('',(#9923),#3348,.F.);
#89203=ADVANCED_FACE('',(#9924),#2491,.F.);
#89204=ADVANCED_FACE('',(#9925),#2492,.F.);
#89205=ADVANCED_FACE('',(#9926),#7895,.F.);
#89206=ADVANCED_FACE('',(#9927),#7896,.T.);
#89207=ADVANCED_FACE('',(#9928),#86160,.T.);
#89208=ADVANCED_FACE('',(#9929),#7897,.F.);
#89209=ADVANCED_FACE('',(#9930),#6974,.T.);
#89210=ADVANCED_FACE('',(#9931),#2493,.F.);
#89211=ADVANCED_FACE('',(#9932),#86161,.T.);
#89212=ADVANCED_FACE('',(#9933),#7898,.F.);
#89213=ADVANCED_FACE('',(#9934),#7899,.T.);
#89214=ADVANCED_FACE('',(#9935),#2494,.F.);
#89215=ADVANCED_FACE('',(#9936),#6975,.T.);
#89216=ADVANCED_FACE('',(#9937),#7900,.F.);
#89217=ADVANCED_FACE('',(#9938),#7901,.T.);
#89218=ADVANCED_FACE('',(#9939),#86162,.T.);
#89219=ADVANCED_FACE('',(#9940),#86163,.T.);
#89220=ADVANCED_FACE('',(#9941),#7902,.T.);
#89221=ADVANCED_FACE('',(#9942),#2495,.F.);
#89222=ADVANCED_FACE('',(#9943),#6976,.T.);
#89223=ADVANCED_FACE('',(#9944),#2496,.T.);
#89224=ADVANCED_FACE('',(#9945),#7903,.T.);
#89225=ADVANCED_FACE('',(#9946),#2497,.F.);
#89226=ADVANCED_FACE('',(#9947),#6977,.T.);
#89227=ADVANCED_FACE('',(#9948),#2498,.T.);
#89228=ADVANCED_FACE('',(#9949),#7904,.T.);
#89229=ADVANCED_FACE('',(#9950),#2499,.F.);
#89230=ADVANCED_FACE('',(#9951),#6978,.T.);
#89231=ADVANCED_FACE('',(#9952),#2500,.T.);
#89232=ADVANCED_FACE('',(#9953),#7905,.T.);
#89233=ADVANCED_FACE('',(#9954),#2501,.F.);
#89234=ADVANCED_FACE('',(#9955),#6979,.T.);
#89235=ADVANCED_FACE('',(#9956),#86164,.T.);
#89236=ADVANCED_FACE('',(#9957),#7906,.T.);
#89237=ADVANCED_FACE('',(#9958),#86165,.T.);
#89238=ADVANCED_FACE('',(#9959),#7907,.F.);
#89239=ADVANCED_FACE('',(#9960),#86166,.T.);
#89240=ADVANCED_FACE('',(#9961),#7908,.T.);
#89241=ADVANCED_FACE('',(#9962),#2502,.F.);
#89242=ADVANCED_FACE('',(#9963),#6980,.T.);
#89243=ADVANCED_FACE('',(#9964),#7909,.F.);
#89244=ADVANCED_FACE('',(#9965),#7910,.T.);
#89245=ADVANCED_FACE('',(#9966),#7911,.T.);
#89246=ADVANCED_FACE('',(#9967),#7912,.F.);
#89247=ADVANCED_FACE('',(#9968),#7913,.T.);
#89248=ADVANCED_FACE('',(#9969),#7914,.F.);
#89249=ADVANCED_FACE('',(#9970),#7915,.F.);
#89250=ADVANCED_FACE('',(#9971),#86167,.T.);
#89251=ADVANCED_FACE('',(#9972),#3349,.F.);
#89252=ADVANCED_FACE('',(#9973),#2503,.F.);
#89253=ADVANCED_FACE('',(#9974),#2504,.F.);
#89254=ADVANCED_FACE('',(#9975),#86168,.T.);
#89255=ADVANCED_FACE('',(#9976),#2505,.F.);
#89256=ADVANCED_FACE('',(#9977),#2506,.T.);
#89257=ADVANCED_FACE('',(#9978),#2507,.T.);
#89258=ADVANCED_FACE('',(#9979),#86169,.T.);
#89259=ADVANCED_FACE('',(#9980),#2508,.F.);
#89260=ADVANCED_FACE('',(#9981),#86170,.F.);
#89261=ADVANCED_FACE('',(#9982),#2509,.F.);
#89262=ADVANCED_FACE('',(#9983),#86171,.T.);
#89263=ADVANCED_FACE('',(#9984),#2510,.F.);
#89264=ADVANCED_FACE('',(#9985),#86172,.F.);
#89265=ADVANCED_FACE('',(#9986),#2511,.F.);
#89266=ADVANCED_FACE('',(#9987),#86173,.T.);
#89267=ADVANCED_FACE('',(#9988),#3350,.T.);
#89268=ADVANCED_FACE('',(#9989),#3351,.T.);
#89269=ADVANCED_FACE('',(#9990),#3352,.T.);
#89270=ADVANCED_FACE('',(#9991),#2512,.F.);
#89271=ADVANCED_FACE('',(#9992),#86174,.F.);
#89272=ADVANCED_FACE('',(#9993),#2513,.F.);
#89273=ADVANCED_FACE('',(#9994),#86175,.T.);
#89274=ADVANCED_FACE('',(#9995),#2514,.T.);
#89275=ADVANCED_FACE('',(#9996),#86176,.T.);
#89276=ADVANCED_FACE('',(#9997),#2515,.F.);
#89277=ADVANCED_FACE('',(#9998),#86177,.F.);
#89278=ADVANCED_FACE('',(#9999),#2516,.F.);
#89279=ADVANCED_FACE('',(#10000),#86178,.T.);
#89280=ADVANCED_FACE('',(#10001),#2517,.T.);
#89281=ADVANCED_FACE('',(#10002),#2518,.F.);
#89282=ADVANCED_FACE('',(#10003),#2519,.F.);
#89283=ADVANCED_FACE('',(#10004),#3353,.F.);
#89284=ADVANCED_FACE('',(#10005),#2520,.F.);
#89285=ADVANCED_FACE('',(#10006),#3354,.T.);
#89286=ADVANCED_FACE('',(#10007),#2521,.F.);
#89287=ADVANCED_FACE('',(#10008),#3355,.F.);
#89288=ADVANCED_FACE('',(#10009),#2522,.F.);
#89289=ADVANCED_FACE('',(#10010),#2523,.F.);
#89290=ADVANCED_FACE('',(#10011),#3356,.T.);
#89291=ADVANCED_FACE('',(#10012),#2524,.F.);
#89292=ADVANCED_FACE('',(#10013),#2525,.F.);
#89293=ADVANCED_FACE('',(#10014),#2526,.F.);
#89294=ADVANCED_FACE('',(#10015),#3357,.T.);
#89295=ADVANCED_FACE('',(#10016),#2527,.F.);
#89296=ADVANCED_FACE('',(#10017),#2528,.F.);
#89297=ADVANCED_FACE('',(#10018),#2529,.F.);
#89298=ADVANCED_FACE('',(#10019),#3358,.T.);
#89299=ADVANCED_FACE('',(#10020),#2530,.F.);
#89300=ADVANCED_FACE('',(#10021),#2531,.F.);
#89301=ADVANCED_FACE('',(#10022),#2532,.F.);
#89302=ADVANCED_FACE('',(#10023),#3359,.T.);
#89303=ADVANCED_FACE('',(#10024),#2533,.F.);
#89304=ADVANCED_FACE('',(#10025),#2534,.F.);
#89305=ADVANCED_FACE('',(#10026),#3360,.F.);
#89306=ADVANCED_FACE('',(#10027),#2535,.F.);
#89307=ADVANCED_FACE('',(#10028),#3361,.T.);
#89308=ADVANCED_FACE('',(#10029),#2536,.F.);
#89309=ADVANCED_FACE('',(#10030),#3362,.F.);
#89310=ADVANCED_FACE('',(#10031),#2537,.F.);
#89311=ADVANCED_FACE('',(#10032),#2538,.T.);
#89312=ADVANCED_FACE('',(#10033),#2539,.F.);
#89313=ADVANCED_FACE('',(#10034),#2540,.T.);
#89314=ADVANCED_FACE('',(#10035),#86179,.T.);
#89315=ADVANCED_FACE('',(#10036),#2541,.F.);
#89316=ADVANCED_FACE('',(#10037),#86180,.F.);
#89317=ADVANCED_FACE('',(#10038),#2542,.F.);
#89318=ADVANCED_FACE('',(#10039),#86181,.T.);
#89319=ADVANCED_FACE('',(#10040),#2543,.F.);
#89320=ADVANCED_FACE('',(#10041),#86182,.F.);
#89321=ADVANCED_FACE('',(#10042),#2544,.F.);
#89322=ADVANCED_FACE('',(#10043),#86183,.T.);
#89323=ADVANCED_FACE('',(#10044),#3363,.T.);
#89324=ADVANCED_FACE('',(#10045),#3364,.T.);
#89325=ADVANCED_FACE('',(#10046),#3365,.T.);
#89326=ADVANCED_FACE('',(#10047),#86184,.T.);
#89327=ADVANCED_FACE('',(#10048),#1017,.F.);
#89328=ADVANCED_FACE('',(#10049),#2545,.F.);
#89329=ADVANCED_FACE('',(#10050),#2546,.F.);
#89330=ADVANCED_FACE('',(#10051),#7916,.T.);
#89331=ADVANCED_FACE('',(#10052),#86185,.T.);
#89332=ADVANCED_FACE('',(#10053),#7917,.T.);
#89333=ADVANCED_FACE('',(#10054),#3366,.T.);
#89334=ADVANCED_FACE('',(#10055),#86186,.T.);
#89335=ADVANCED_FACE('',(#10056),#2547,.F.);
#89336=ADVANCED_FACE('',(#10057),#2548,.F.);
#89337=ADVANCED_FACE('',(#10058),#86187,.F.);
#89338=ADVANCED_FACE('',(#10059),#2549,.F.);
#89339=ADVANCED_FACE('',(#10060),#2550,.F.);
#89340=ADVANCED_FACE('',(#10061),#2551,.F.);
#89341=ADVANCED_FACE('',(#10062),#86188,.F.);
#89342=ADVANCED_FACE('',(#10063),#2552,.F.);
#89343=ADVANCED_FACE('',(#10064),#86189,.F.);
#89344=ADVANCED_FACE('',(#10065),#86190,.T.);
#89345=ADVANCED_FACE('',(#10066),#86191,.F.);
#89346=ADVANCED_FACE('',(#10067),#3367,.T.);
#89347=ADVANCED_FACE('',(#10068),#86192,.T.);
#89348=ADVANCED_FACE('',(#10069),#3368,.T.);
#89349=ADVANCED_FACE('',(#10070),#86193,.T.);
#89350=ADVANCED_FACE('',(#10071),#3369,.T.);
#89351=ADVANCED_FACE('',(#10072),#86194,.T.);
#89352=ADVANCED_FACE('',(#10073),#86195,.F.);
#89353=ADVANCED_FACE('',(#10074),#2553,.F.);
#89354=ADVANCED_FACE('',(#10075),#86196,.F.);
#89355=ADVANCED_FACE('',(#10076),#2554,.F.);
#89356=ADVANCED_FACE('',(#10077),#2555,.F.);
#89357=ADVANCED_FACE('',(#10078),#2556,.F.);
#89358=ADVANCED_FACE('',(#10079),#86197,.F.);
#89359=ADVANCED_FACE('',(#10080),#2557,.F.);
#89360=ADVANCED_FACE('',(#10081),#2558,.F.);
#89361=ADVANCED_FACE('',(#10082),#2559,.F.);
#89362=ADVANCED_FACE('',(#10083),#86198,.F.);
#89363=ADVANCED_FACE('',(#10084),#3370,.F.);
#89364=ADVANCED_FACE('',(#10085),#3371,.T.);
#89365=ADVANCED_FACE('',(#10086),#86199,.T.);
#89366=ADVANCED_FACE('',(#10087),#86200,.F.);
#89367=ADVANCED_FACE('',(#10088),#2560,.F.);
#89368=ADVANCED_FACE('',(#10089),#2561,.F.);
#89369=ADVANCED_FACE('',(#10090),#2562,.F.);
#89370=ADVANCED_FACE('',(#10091),#86201,.F.);
#89371=ADVANCED_FACE('',(#10092),#2563,.F.);
#89372=ADVANCED_FACE('',(#10093),#2564,.F.);
#89373=ADVANCED_FACE('',(#10094),#2565,.F.);
#89374=ADVANCED_FACE('',(#10095),#86202,.F.);
#89375=ADVANCED_FACE('',(#10096),#2566,.F.);
#89376=ADVANCED_FACE('',(#10097),#86203,.F.);
#89377=ADVANCED_FACE('',(#10098),#86204,.T.);
#89378=ADVANCED_FACE('',(#10099),#3372,.T.);
#89379=ADVANCED_FACE('',(#10100),#86205,.T.);
#89380=ADVANCED_FACE('',(#10101),#86206,.F.);
#89381=ADVANCED_FACE('',(#10102),#86207,.F.);
#89382=ADVANCED_FACE('',(#10103),#86208,.F.);
#89383=ADVANCED_FACE('',(#10104),#2567,.F.);
#89384=ADVANCED_FACE('',(#10105),#3373,.T.);
#89385=ADVANCED_FACE('',(#10106),#86209,.T.);
#89386=ADVANCED_FACE('',(#10107),#3374,.T.);
#89387=ADVANCED_FACE('',(#10108),#86210,.T.);
#89388=ADVANCED_FACE('',(#10109),#86211,.F.);
#89389=ADVANCED_FACE('',(#10110),#2568,.F.);
#89390=ADVANCED_FACE('',(#10111),#2569,.F.);
#89391=ADVANCED_FACE('',(#10112),#2570,.F.);
#89392=ADVANCED_FACE('',(#10113),#2571,.F.);
#89393=ADVANCED_FACE('',(#10114),#86212,.F.);
#89394=ADVANCED_FACE('',(#10115),#2572,.F.);
#89395=ADVANCED_FACE('',(#10116),#2573,.F.);
#89396=ADVANCED_FACE('',(#10117),#86213,.T.);
#89397=ADVANCED_FACE('',(#10118),#3375,.T.);
#89398=ADVANCED_FACE('',(#10119),#86214,.T.);
#89399=ADVANCED_FACE('',(#10120),#86215,.F.);
#89400=ADVANCED_FACE('',(#10121),#2574,.F.);
#89401=ADVANCED_FACE('',(#10122),#2575,.F.);
#89402=ADVANCED_FACE('',(#10123),#2576,.F.);
#89403=ADVANCED_FACE('',(#10124),#6981,.T.);
#89404=ADVANCED_FACE('',(#10125),#3376,.T.);
#89405=ADVANCED_FACE('',(#10126),#86216,.T.);
#89406=ADVANCED_FACE('',(#10127),#2577,.F.);
#89407=ADVANCED_FACE('',(#10128),#2578,.F.);
#89408=ADVANCED_FACE('',(#10129),#2579,.F.);
#89409=ADVANCED_FACE('',(#10130),#86217,.F.);
#89410=ADVANCED_FACE('',(#10131),#2580,.F.);
#89411=ADVANCED_FACE('',(#10132),#2581,.F.);
#89412=ADVANCED_FACE('',(#10133),#2582,.F.);
#89413=ADVANCED_FACE('',(#10134),#86218,.F.);
#89414=ADVANCED_FACE('',(#10135),#2583,.F.);
#89415=ADVANCED_FACE('',(#10136),#86219,.F.);
#89416=ADVANCED_FACE('',(#10137),#86220,.T.);
#89417=ADVANCED_FACE('',(#10138),#3377,.T.);
#89418=ADVANCED_FACE('',(#10139),#86221,.T.);
#89419=ADVANCED_FACE('',(#10140),#3378,.T.);
#89420=ADVANCED_FACE('',(#10141),#86222,.T.);
#89421=ADVANCED_FACE('',(#10142),#3379,.T.);
#89422=ADVANCED_FACE('',(#10143),#86223,.T.);
#89423=ADVANCED_FACE('',(#10144),#86224,.F.);
#89424=ADVANCED_FACE('',(#10145),#2584,.F.);
#89425=ADVANCED_FACE('',(#10146),#86225,.F.);
#89426=ADVANCED_FACE('',(#10147),#2585,.F.);
#89427=ADVANCED_FACE('',(#10148),#2586,.F.);
#89428=ADVANCED_FACE('',(#10149),#2587,.F.);
#89429=ADVANCED_FACE('',(#10150),#86226,.F.);
#89430=ADVANCED_FACE('',(#10151),#2588,.F.);
#89431=ADVANCED_FACE('',(#10152),#2589,.F.);
#89432=ADVANCED_FACE('',(#10153),#86227,.F.);
#89433=ADVANCED_FACE('',(#10154),#2590,.F.);
#89434=ADVANCED_FACE('',(#10155),#6982,.T.);
#89435=ADVANCED_FACE('',(#10156),#3380,.T.);
#89436=ADVANCED_FACE('',(#10157),#86228,.T.);
#89437=ADVANCED_FACE('',(#10158),#2591,.F.);
#89438=ADVANCED_FACE('',(#10159),#2592,.F.);
#89439=ADVANCED_FACE('',(#10160),#2593,.F.);
#89440=ADVANCED_FACE('',(#10161),#2594,.F.);
#89441=ADVANCED_FACE('',(#10162),#86229,.F.);
#89442=ADVANCED_FACE('',(#10163),#2595,.F.);
#89443=ADVANCED_FACE('',(#10164),#2596,.F.);
#89444=ADVANCED_FACE('',(#10165),#2597,.F.);
#89445=ADVANCED_FACE('',(#10166),#2598,.F.);
#89446=ADVANCED_FACE('',(#10167),#86230,.F.);
#89447=ADVANCED_FACE('',(#10168),#86231,.T.);
#89448=ADVANCED_FACE('',(#10169),#86232,.F.);
#89449=ADVANCED_FACE('',(#10170),#86233,.F.);
#89450=ADVANCED_FACE('',(#10171),#2599,.F.);
#89451=ADVANCED_FACE('',(#10172),#86234,.F.);
#89452=ADVANCED_FACE('',(#10173),#86235,.T.);
#89453=ADVANCED_FACE('',(#10174),#3381,.T.);
#89454=ADVANCED_FACE('',(#10175),#86236,.T.);
#89455=ADVANCED_FACE('',(#10176),#2600,.F.);
#89456=ADVANCED_FACE('',(#10177),#86237,.F.);
#89457=ADVANCED_FACE('',(#10178),#3382,.T.);
#89458=ADVANCED_FACE('',(#10179),#86238,.T.);
#89459=ADVANCED_FACE('',(#10180),#86239,.F.);
#89460=ADVANCED_FACE('',(#10181),#2601,.F.);
#89461=ADVANCED_FACE('',(#10182),#2602,.F.);
#89462=ADVANCED_FACE('',(#10183),#2603,.F.);
#89463=ADVANCED_FACE('',(#10184),#86240,.F.);
#89464=ADVANCED_FACE('',(#10185),#2604,.F.);
#89465=ADVANCED_FACE('',(#10186),#2605,.F.);
#89466=ADVANCED_FACE('',(#10187),#2606,.F.);
#89467=ADVANCED_FACE('',(#10188),#3383,.T.);
#89468=ADVANCED_FACE('',(#10189),#86241,.T.);
#89469=ADVANCED_FACE('',(#10190),#3384,.T.);
#89470=ADVANCED_FACE('',(#10191),#86242,.T.);
#89471=ADVANCED_FACE('',(#10192),#86243,.F.);
#89472=ADVANCED_FACE('',(#10193),#2607,.F.);
#89473=ADVANCED_FACE('',(#10194),#86244,.F.);
#89474=ADVANCED_FACE('',(#10195),#86245,.F.);
#89475=ADVANCED_FACE('',(#10196),#3385,.F.);
#89476=ADVANCED_FACE('',(#10197),#2608,.F.);
#89477=ADVANCED_FACE('',(#10198),#2609,.F.);
#89478=ADVANCED_FACE('',(#10199),#2610,.F.);
#89479=ADVANCED_FACE('',(#10200),#86246,.F.);
#89480=ADVANCED_FACE('',(#10201),#3386,.T.);
#89481=ADVANCED_FACE('',(#10202),#86247,.T.);
#89482=ADVANCED_FACE('',(#10203),#3387,.T.);
#89483=ADVANCED_FACE('',(#10204),#86248,.T.);
#89484=ADVANCED_FACE('',(#10205),#86249,.F.);
#89485=ADVANCED_FACE('',(#10206),#2611,.F.);
#89486=ADVANCED_FACE('',(#10207),#2612,.F.);
#89487=ADVANCED_FACE('',(#10208),#86250,.F.);
#89488=ADVANCED_FACE('',(#10209),#3388,.T.);
#89489=ADVANCED_FACE('',(#10210),#86251,.T.);
#89490=ADVANCED_FACE('',(#10211),#3389,.T.);
#89491=ADVANCED_FACE('',(#10212),#86252,.F.);
#89492=ADVANCED_FACE('',(#10213),#2613,.F.);
#89493=ADVANCED_FACE('',(#10214),#2614,.F.);
#89494=ADVANCED_FACE('',(#10215),#2615,.F.);
#89495=ADVANCED_FACE('',(#10216),#86253,.F.);
#89496=ADVANCED_FACE('',(#10217),#86254,.F.);
#89497=ADVANCED_FACE('',(#10218),#3390,.F.);
#89498=ADVANCED_FACE('',(#10219),#3391,.T.);
#89499=ADVANCED_FACE('',(#10220),#86255,.T.);
#89500=ADVANCED_FACE('',(#10221),#2616,.F.);
#89501=ADVANCED_FACE('',(#10222),#2617,.F.);
#89502=ADVANCED_FACE('',(#10223),#2618,.F.);
#89503=ADVANCED_FACE('',(#10224),#86256,.F.);
#89504=ADVANCED_FACE('',(#10225),#2619,.F.);
#89505=ADVANCED_FACE('',(#10226),#2620,.F.);
#89506=ADVANCED_FACE('',(#10227),#2621,.F.);
#89507=ADVANCED_FACE('',(#10228),#86257,.F.);
#89508=ADVANCED_FACE('',(#10229),#2622,.F.);
#89509=ADVANCED_FACE('',(#10230),#86258,.F.);
#89510=ADVANCED_FACE('',(#10231),#86259,.T.);
#89511=ADVANCED_FACE('',(#10232),#3392,.T.);
#89512=ADVANCED_FACE('',(#10233),#86260,.T.);
#89513=ADVANCED_FACE('',(#10234),#3393,.T.);
#89514=ADVANCED_FACE('',(#10235),#86261,.T.);
#89515=ADVANCED_FACE('',(#10236),#3394,.T.);
#89516=ADVANCED_FACE('',(#10237),#86262,.T.);
#89517=ADVANCED_FACE('',(#10238),#86263,.F.);
#89518=ADVANCED_FACE('',(#10239),#2623,.F.);
#89519=ADVANCED_FACE('',(#10240),#86264,.F.);
#89520=ADVANCED_FACE('',(#10241),#2624,.F.);
#89521=ADVANCED_FACE('',(#10242),#2625,.F.);
#89522=ADVANCED_FACE('',(#10243),#2626,.F.);
#89523=ADVANCED_FACE('',(#10244),#86265,.F.);
#89524=ADVANCED_FACE('',(#10245),#2627,.F.);
#89525=ADVANCED_FACE('',(#10246),#2628,.F.);
#89526=ADVANCED_FACE('',(#10247),#86266,.F.);
#89527=ADVANCED_FACE('',(#10248),#2629,.F.);
#89528=ADVANCED_FACE('',(#10249),#6983,.T.);
#89529=ADVANCED_FACE('',(#10250),#3395,.T.);
#89530=ADVANCED_FACE('',(#10251),#86267,.T.);
#89531=ADVANCED_FACE('',(#10252),#2630,.F.);
#89532=ADVANCED_FACE('',(#10253),#2631,.F.);
#89533=ADVANCED_FACE('',(#10254),#86268,.F.);
#89534=ADVANCED_FACE('',(#10255),#2632,.F.);
#89535=ADVANCED_FACE('',(#10256),#2633,.F.);
#89536=ADVANCED_FACE('',(#10257),#2634,.F.);
#89537=ADVANCED_FACE('',(#10258),#2635,.F.);
#89538=ADVANCED_FACE('',(#10259),#2636,.F.);
#89539=ADVANCED_FACE('',(#10260),#86269,.F.);
#89540=ADVANCED_FACE('',(#10261),#2637,.F.);
#89541=ADVANCED_FACE('',(#10262),#86270,.F.);
#89542=ADVANCED_FACE('',(#10263),#86271,.T.);
#89543=ADVANCED_FACE('',(#10264),#3396,.T.);
#89544=ADVANCED_FACE('',(#10265),#86272,.T.);
#89545=ADVANCED_FACE('',(#10266),#2638,.F.);
#89546=ADVANCED_FACE('',(#10267),#86273,.F.);
#89547=ADVANCED_FACE('',(#10268),#86274,.F.);
#89548=ADVANCED_FACE('',(#10269),#86275,.F.);
#89549=ADVANCED_FACE('',(#10270),#3397,.T.);
#89550=ADVANCED_FACE('',(#10271),#86276,.T.);
#89551=ADVANCED_FACE('',(#10272),#86277,.F.);
#89552=ADVANCED_FACE('',(#10273),#2639,.F.);
#89553=ADVANCED_FACE('',(#10274),#2640,.F.);
#89554=ADVANCED_FACE('',(#10275),#2641,.F.);
#89555=ADVANCED_FACE('',(#10276),#86278,.F.);
#89556=ADVANCED_FACE('',(#10277),#2642,.F.);
#89557=ADVANCED_FACE('',(#10278),#2643,.F.);
#89558=ADVANCED_FACE('',(#10279),#3398,.T.);
#89559=ADVANCED_FACE('',(#10280),#86279,.T.);
#89560=ADVANCED_FACE('',(#10281),#3399,.T.);
#89561=ADVANCED_FACE('',(#10282),#86280,.T.);
#89562=ADVANCED_FACE('',(#10283),#86281,.F.);
#89563=ADVANCED_FACE('',(#10284),#2644,.F.);
#89564=ADVANCED_FACE('',(#10285),#3400,.F.);
#89565=ADVANCED_FACE('',(#10286),#86282,.F.);
#89566=ADVANCED_FACE('',(#10287),#86283,.F.);
#89567=ADVANCED_FACE('',(#10288),#2645,.F.);
#89568=ADVANCED_FACE('',(#10289),#2646,.F.);
#89569=ADVANCED_FACE('',(#10290),#2647,.F.);
#89570=ADVANCED_FACE('',(#10291),#86284,.F.);
#89571=ADVANCED_FACE('',(#10292),#2648,.F.);
#89572=ADVANCED_FACE('',(#10293),#86285,.T.);
#89573=ADVANCED_FACE('',(#10294),#3401,.T.);
#89574=ADVANCED_FACE('',(#10295),#86286,.T.);
#89575=ADVANCED_FACE('',(#10296),#86287,.F.);
#89576=ADVANCED_FACE('',(#10297),#2649,.F.);
#89577=ADVANCED_FACE('',(#10298),#2650,.F.);
#89578=ADVANCED_FACE('',(#10299),#2651,.F.);
#89579=ADVANCED_FACE('',(#10300),#2652,.F.);
#89580=ADVANCED_FACE('',(#10301),#86288,.F.);
#89581=ADVANCED_FACE('',(#10302),#2653,.F.);
#89582=ADVANCED_FACE('',(#10303),#2654,.F.);
#89583=ADVANCED_FACE('',(#10304),#2655,.F.);
#89584=ADVANCED_FACE('',(#10305),#86289,.F.);
#89585=ADVANCED_FACE('',(#10306),#86290,.T.);
#89586=ADVANCED_FACE('',(#10307),#3402,.T.);
#89587=ADVANCED_FACE('',(#10308),#86291,.T.);
#89588=ADVANCED_FACE('',(#10309),#2656,.F.);
#89589=ADVANCED_FACE('',(#10310),#3403,.T.);
#89590=ADVANCED_FACE('',(#10311),#86292,.T.);
#89591=ADVANCED_FACE('',(#10312),#3404,.T.);
#89592=ADVANCED_FACE('',(#10313),#86293,.T.);
#89593=ADVANCED_FACE('',(#10314),#3405,.T.);
#89594=ADVANCED_FACE('',(#10315),#86294,.F.);
#89595=ADVANCED_FACE('',(#10316),#2657,.F.);
#89596=ADVANCED_FACE('',(#10317),#2658,.F.);
#89597=ADVANCED_FACE('',(#10318),#2659,.F.);
#89598=ADVANCED_FACE('',(#10319),#86295,.F.);
#89599=ADVANCED_FACE('',(#10320),#2660,.F.);
#89600=ADVANCED_FACE('',(#10321),#2661,.F.);
#89601=ADVANCED_FACE('',(#10322),#2662,.F.);
#89602=ADVANCED_FACE('',(#10323),#2663,.F.);
#89603=ADVANCED_FACE('',(#10324),#86296,.F.);
#89604=ADVANCED_FACE('',(#10325),#2664,.F.);
#89605=ADVANCED_FACE('',(#10326),#2665,.F.);
#89606=ADVANCED_FACE('',(#10327),#2666,.F.);
#89607=ADVANCED_FACE('',(#10328),#86297,.F.);
#89608=ADVANCED_FACE('',(#10329),#2667,.T.);
#89609=ADVANCED_FACE('',(#10330),#2668,.F.);
#89610=ADVANCED_FACE('',(#10331),#86298,.T.);
#89611=ADVANCED_FACE('',(#10332),#7918,.T.);
#89612=ADVANCED_FACE('',(#10333),#86299,.T.);
#89613=ADVANCED_FACE('',(#10334),#2669,.T.);
#89614=ADVANCED_FACE('',(#10335),#86300,.F.);
#89615=ADVANCED_FACE('',(#10336),#2670,.F.);
#89616=ADVANCED_FACE('',(#10337),#2671,.F.);
#89617=ADVANCED_FACE('',(#10338),#2672,.F.);
#89618=ADVANCED_FACE('',(#10339),#86301,.F.);
#89619=ADVANCED_FACE('',(#10340),#2673,.F.);
#89620=ADVANCED_FACE('',(#10341),#2674,.F.);
#89621=ADVANCED_FACE('',(#10342),#2675,.F.);
#89622=ADVANCED_FACE('',(#10343),#2676,.F.);
#89623=ADVANCED_FACE('',(#10344),#86302,.F.);
#89624=ADVANCED_FACE('',(#10345),#2677,.F.);
#89625=ADVANCED_FACE('',(#10346),#2678,.F.);
#89626=ADVANCED_FACE('',(#10347),#2679,.F.);
#89627=ADVANCED_FACE('',(#10348),#86303,.F.);
#89628=ADVANCED_FACE('',(#10349),#2680,.T.);
#89629=ADVANCED_FACE('',(#10350),#2681,.F.);
#89630=ADVANCED_FACE('',(#10351),#86304,.T.);
#89631=ADVANCED_FACE('',(#10352),#7919,.T.);
#89632=ADVANCED_FACE('',(#10353),#86305,.T.);
#89633=ADVANCED_FACE('',(#10354),#2682,.T.);
#89634=ADVANCED_FACE('',(#10355),#86306,.F.);
#89635=ADVANCED_FACE('',(#10356),#2683,.F.);
#89636=ADVANCED_FACE('',(#10357),#2684,.F.);
#89637=ADVANCED_FACE('',(#10358),#2685,.F.);
#89638=ADVANCED_FACE('',(#10359),#86307,.F.);
#89639=ADVANCED_FACE('',(#10360),#2686,.F.);
#89640=ADVANCED_FACE('',(#10361),#2687,.F.);
#89641=ADVANCED_FACE('',(#10362),#2688,.F.);
#89642=ADVANCED_FACE('',(#10363),#2689,.F.);
#89643=ADVANCED_FACE('',(#10364),#86308,.F.);
#89644=ADVANCED_FACE('',(#10365),#2690,.F.);
#89645=ADVANCED_FACE('',(#10366),#2691,.F.);
#89646=ADVANCED_FACE('',(#10367),#2692,.F.);
#89647=ADVANCED_FACE('',(#10368),#86309,.F.);
#89648=ADVANCED_FACE('',(#10369),#2693,.T.);
#89649=ADVANCED_FACE('',(#10370),#2694,.F.);
#89650=ADVANCED_FACE('',(#10371),#86310,.T.);
#89651=ADVANCED_FACE('',(#10372),#7920,.T.);
#89652=ADVANCED_FACE('',(#10373),#86311,.T.);
#89653=ADVANCED_FACE('',(#10374),#2695,.T.);
#89654=ADVANCED_FACE('',(#10375),#86312,.F.);
#89655=ADVANCED_FACE('',(#10376),#2696,.F.);
#89656=ADVANCED_FACE('',(#10377),#2697,.F.);
#89657=ADVANCED_FACE('',(#10378),#2698,.F.);
#89658=ADVANCED_FACE('',(#10379),#86313,.F.);
#89659=ADVANCED_FACE('',(#10380),#2699,.F.);
#89660=ADVANCED_FACE('',(#10381),#2700,.F.);
#89661=ADVANCED_FACE('',(#10382),#2701,.F.);
#89662=ADVANCED_FACE('',(#10383),#2702,.F.);
#89663=ADVANCED_FACE('',(#10384),#86314,.F.);
#89664=ADVANCED_FACE('',(#10385),#2703,.F.);
#89665=ADVANCED_FACE('',(#10386),#2704,.F.);
#89666=ADVANCED_FACE('',(#10387),#2705,.F.);
#89667=ADVANCED_FACE('',(#10388),#86315,.F.);
#89668=ADVANCED_FACE('',(#10389),#3406,.T.);
#89669=ADVANCED_FACE('',(#10390),#86316,.T.);
#89670=ADVANCED_FACE('',(#10391),#2706,.F.);
#89671=ADVANCED_FACE('',(#10392),#3407,.T.);
#89672=ADVANCED_FACE('',(#10393),#86317,.T.);
#89673=ADVANCED_FACE('',(#10394),#3408,.T.);
#89674=ADVANCED_FACE('',(#10395),#86318,.T.);
#89675=ADVANCED_FACE('',(#10396),#3409,.T.);
#89676=ADVANCED_FACE('',(#10397),#86319,.T.);
#89677=ADVANCED_FACE('',(#10398),#86320,.F.);
#89678=ADVANCED_FACE('',(#10399),#2707,.F.);
#89679=ADVANCED_FACE('',(#10400),#2708,.F.);
#89680=ADVANCED_FACE('',(#10401),#2709,.F.);
#89681=ADVANCED_FACE('',(#10402),#86321,.F.);
#89682=ADVANCED_FACE('',(#10403),#2710,.F.);
#89683=ADVANCED_FACE('',(#10404),#2711,.F.);
#89684=ADVANCED_FACE('',(#10405),#2712,.F.);
#89685=ADVANCED_FACE('',(#10406),#3410,.T.);
#89686=ADVANCED_FACE('',(#10407),#86322,.T.);
#89687=ADVANCED_FACE('',(#10408),#2713,.F.);
#89688=ADVANCED_FACE('',(#10409),#2714,.F.);
#89689=ADVANCED_FACE('',(#10410),#86323,.F.);
#89690=ADVANCED_FACE('',(#10411),#2715,.F.);
#89691=ADVANCED_FACE('',(#10412),#2716,.F.);
#89692=ADVANCED_FACE('',(#10413),#2717,.F.);
#89693=ADVANCED_FACE('',(#10414),#86324,.F.);
#89694=ADVANCED_FACE('',(#10415),#86325,.T.);
#89695=ADVANCED_FACE('',(#10416),#3411,.T.);
#89696=ADVANCED_FACE('',(#10417),#86326,.T.);
#89697=ADVANCED_FACE('',(#10418),#3412,.T.);
#89698=ADVANCED_FACE('',(#10419),#3413,.T.);
#89699=ADVANCED_FACE('',(#10420),#86327,.T.);
#89700=ADVANCED_FACE('',(#10421),#3414,.T.);
#89701=ADVANCED_FACE('',(#10422),#2718,.F.);
#89702=ADVANCED_FACE('',(#10423),#2719,.F.);
#89703=ADVANCED_FACE('',(#10424),#2720,.F.);
#89704=ADVANCED_FACE('',(#10425),#2721,.F.);
#89705=ADVANCED_FACE('',(#10426),#2722,.F.);
#89706=ADVANCED_FACE('',(#10427),#2723,.F.);
#89707=ADVANCED_FACE('',(#10428),#86328,.F.);
#89708=ADVANCED_FACE('',(#10429),#3415,.T.);
#89709=ADVANCED_FACE('',(#10430),#86329,.T.);
#89710=ADVANCED_FACE('',(#10431),#3416,.T.);
#89711=ADVANCED_FACE('',(#10432),#86330,.F.);
#89712=ADVANCED_FACE('',(#10433),#2724,.F.);
#89713=ADVANCED_FACE('',(#10434),#2725,.F.);
#89714=ADVANCED_FACE('',(#10435),#2726,.F.);
#89715=ADVANCED_FACE('',(#10436),#2727,.F.);
#89716=ADVANCED_FACE('',(#10437),#6984,.T.);
#89717=ADVANCED_FACE('',(#10438),#3417,.T.);
#89718=ADVANCED_FACE('',(#10439),#86331,.T.);
#89719=ADVANCED_FACE('',(#10440),#3418,.T.);
#89720=ADVANCED_FACE('',(#10441),#2728,.F.);
#89721=ADVANCED_FACE('',(#10442),#2729,.F.);
#89722=ADVANCED_FACE('',(#10443),#86332,.F.);
#89723=ADVANCED_FACE('',(#10444),#2730,.F.);
#89724=ADVANCED_FACE('',(#10445),#2731,.F.);
#89725=ADVANCED_FACE('',(#10446),#2732,.F.);
#89726=ADVANCED_FACE('',(#10447),#3419,.T.);
#89727=ADVANCED_FACE('',(#10448),#86333,.T.);
#89728=ADVANCED_FACE('',(#10449),#2733,.F.);
#89729=ADVANCED_FACE('',(#10450),#86334,.F.);
#89730=ADVANCED_FACE('',(#10451),#2734,.F.);
#89731=ADVANCED_FACE('',(#10452),#2735,.F.);
#89732=ADVANCED_FACE('',(#10453),#2736,.F.);
#89733=ADVANCED_FACE('',(#10454),#3420,.T.);
#89734=ADVANCED_FACE('',(#10455),#86335,.T.);
#89735=ADVANCED_FACE('',(#10456),#3421,.T.);
#89736=ADVANCED_FACE('',(#10457),#86336,.T.);
#89737=ADVANCED_FACE('',(#10458),#3422,.T.);
#89738=ADVANCED_FACE('',(#10459),#2737,.F.);
#89739=ADVANCED_FACE('',(#10460),#2738,.F.);
#89740=ADVANCED_FACE('',(#10461),#86337,.F.);
#89741=ADVANCED_FACE('',(#10462),#2739,.F.);
#89742=ADVANCED_FACE('',(#10463),#2740,.F.);
#89743=ADVANCED_FACE('',(#10464),#2741,.F.);
#89744=ADVANCED_FACE('',(#10465),#2742,.F.);
#89745=ADVANCED_FACE('',(#10466),#86338,.F.);
#89746=ADVANCED_FACE('',(#10467),#2743,.F.);
#89747=ADVANCED_FACE('',(#10468),#2744,.F.);
#89748=ADVANCED_FACE('',(#10469),#2745,.F.);
#89749=ADVANCED_FACE('',(#10470),#86339,.T.);
#89750=ADVANCED_FACE('',(#10471),#7921,.T.);
#89751=ADVANCED_FACE('',(#10472),#86340,.T.);
#89752=ADVANCED_FACE('',(#10473),#2746,.F.);
#89753=ADVANCED_FACE('',(#10474),#2747,.F.);
#89754=ADVANCED_FACE('',(#10475),#86341,.F.);
#89755=ADVANCED_FACE('',(#10476),#2748,.F.);
#89756=ADVANCED_FACE('',(#10477),#2749,.F.);
#89757=ADVANCED_FACE('',(#10478),#2750,.F.);
#89758=ADVANCED_FACE('',(#10479),#2751,.F.);
#89759=ADVANCED_FACE('',(#10480),#86342,.F.);
#89760=ADVANCED_FACE('',(#10481),#2752,.F.);
#89761=ADVANCED_FACE('',(#10482),#2753,.F.);
#89762=ADVANCED_FACE('',(#10483),#2754,.F.);
#89763=ADVANCED_FACE('',(#10484),#7922,.F.);
#89764=ADVANCED_FACE('',(#10485),#86343,.T.);
#89765=ADVANCED_FACE('',(#10486),#2755,.T.);
#89766=ADVANCED_FACE('',(#10487),#2756,.F.);
#89767=ADVANCED_FACE('',(#10488),#86344,.F.);
#89768=ADVANCED_FACE('',(#10489),#2757,.F.);
#89769=ADVANCED_FACE('',(#10490),#6985,.T.);
#89770=ADVANCED_FACE('',(#10491),#2758,.F.);
#89771=ADVANCED_FACE('',(#10492),#2759,.T.);
#89772=ADVANCED_FACE('',(#10493),#2760,.T.);
#89773=ADVANCED_FACE('',(#10494),#2761,.T.);
#89774=ADVANCED_FACE('',(#10495),#2762,.F.);
#89775=ADVANCED_FACE('',(#10496),#6986,.T.);
#89776=ADVANCED_FACE('',(#10497),#2763,.F.);
#89777=ADVANCED_FACE('',(#10498),#86345,.T.);
#89778=ADVANCED_FACE('',(#10499),#7923,.F.);
#89779=ADVANCED_FACE('',(#10500),#86346,.T.);
#89780=ADVANCED_FACE('',(#10501),#2764,.F.);
#89781=ADVANCED_FACE('',(#10502),#6987,.T.);
#89782=ADVANCED_FACE('',(#10503),#2765,.F.);
#89783=ADVANCED_FACE('',(#10504),#86347,.T.);
#89784=ADVANCED_FACE('',(#10505),#7924,.F.);
#89785=ADVANCED_FACE('',(#10506),#7925,.F.);
#89786=ADVANCED_FACE('',(#10507),#2766,.F.);
#89787=ADVANCED_FACE('',(#10508),#7926,.F.);
#89788=ADVANCED_FACE('',(#10509),#2767,.F.);
#89789=ADVANCED_FACE('',(#10510),#7927,.F.);
#89790=ADVANCED_FACE('',(#10511),#2768,.F.);
#89791=ADVANCED_FACE('',(#10512),#7928,.T.);
#89792=ADVANCED_FACE('',(#10513),#86348,.T.);
#89793=ADVANCED_FACE('',(#10514),#86349,.T.);
#89794=ADVANCED_FACE('',(#10515),#86350,.T.);
#89795=ADVANCED_FACE('',(#10516),#7929,.T.);
#89796=ADVANCED_FACE('',(#10517),#86351,.F.);
#89797=ADVANCED_FACE('',(#10518),#86352,.T.);
#89798=ADVANCED_FACE('',(#10519),#86353,.F.);
#89799=ADVANCED_FACE('',(#10520),#7930,.T.);
#89800=ADVANCED_FACE('',(#10521),#86354,.T.);
#89801=ADVANCED_FACE('',(#10522),#86355,.T.);
#89802=ADVANCED_FACE('',(#10523),#86356,.T.);
#89803=ADVANCED_FACE('',(#10524),#7931,.T.);
#89804=ADVANCED_FACE('',(#10525),#2769,.F.);
#89805=ADVANCED_FACE('',(#10526),#86357,.F.);
#89806=ADVANCED_FACE('',(#10527),#2770,.F.);
#89807=ADVANCED_FACE('',(#10528),#86358,.F.);
#89808=ADVANCED_FACE('',(#10529),#2771,.F.);
#89809=ADVANCED_FACE('',(#10530),#86359,.F.);
#89810=ADVANCED_FACE('',(#10531),#86360,.F.);
#89811=ADVANCED_FACE('',(#10532),#2772,.T.);
#89812=ADVANCED_FACE('',(#10533),#7932,.F.);
#89813=ADVANCED_FACE('',(#10534),#2773,.T.);
#89814=ADVANCED_FACE('',(#10535),#86361,.T.);
#89815=ADVANCED_FACE('',(#10536),#7933,.T.);
#89816=ADVANCED_FACE('',(#10537),#86362,.T.);
#89817=ADVANCED_FACE('',(#10538),#2774,.T.);
#89818=ADVANCED_FACE('',(#10539),#7934,.F.);
#89819=ADVANCED_FACE('',(#10540),#2775,.T.);
#89820=ADVANCED_FACE('',(#10541),#86363,.T.);
#89821=ADVANCED_FACE('',(#10542),#7935,.T.);
#89822=ADVANCED_FACE('',(#10543),#86364,.T.);
#89823=ADVANCED_FACE('',(#10544),#2776,.T.);
#89824=ADVANCED_FACE('',(#10545),#7936,.F.);
#89825=ADVANCED_FACE('',(#10546),#2777,.F.);
#89826=ADVANCED_FACE('',(#10547),#2778,.F.);
#89827=ADVANCED_FACE('',(#10548),#2779,.F.);
#89828=ADVANCED_FACE('',(#10549),#86365,.T.);
#89829=ADVANCED_FACE('',(#10550),#7937,.T.);
#89830=ADVANCED_FACE('',(#10551),#86366,.T.);
#89831=ADVANCED_FACE('',(#10552),#2780,.F.);
#89832=ADVANCED_FACE('',(#10553),#2781,.F.);
#89833=ADVANCED_FACE('',(#10554),#86367,.T.);
#89834=ADVANCED_FACE('',(#10555),#7938,.T.);
#89835=ADVANCED_FACE('',(#10556),#86368,.T.);
#89836=ADVANCED_FACE('',(#10557),#2782,.F.);
#89837=ADVANCED_FACE('',(#10558),#2783,.F.);
#89838=ADVANCED_FACE('',(#10559),#86369,.F.);
#89839=ADVANCED_FACE('',(#10560),#3423,.F.);
#89840=ADVANCED_FACE('',(#10561),#2784,.F.);
#89841=ADVANCED_FACE('',(#10562),#2785,.F.);
#89842=ADVANCED_FACE('',(#10563),#7939,.T.);
#89843=ADVANCED_FACE('',(#10564),#86370,.T.);
#89844=ADVANCED_FACE('',(#10565),#3424,.T.);
#89845=ADVANCED_FACE('',(#10566),#86371,.T.);
#89846=ADVANCED_FACE('',(#10567),#86372,.F.);
#89847=ADVANCED_FACE('',(#10568),#86373,.F.);
#89848=ADVANCED_FACE('',(#10569,#7443),#7940,.T.);
#89849=ADVANCED_FACE('',(#10570),#86374,.F.);
#89850=ADVANCED_FACE('',(#10571),#86375,.F.);
#89851=ADVANCED_FACE('',(#10572),#86376,.F.);
#89852=ADVANCED_FACE('',(#10573),#2786,.T.);
#89853=ADVANCED_FACE('',(#10574),#3425,.F.);
#89854=ADVANCED_FACE('',(#10575),#2787,.T.);
#89855=ADVANCED_FACE('',(#10576),#86377,.F.);
#89856=ADVANCED_FACE('',(#10577),#86378,.F.);
#89857=ADVANCED_FACE('',(#10578,#7444),#7941,.T.);
#89858=ADVANCED_FACE('',(#10579),#86379,.F.);
#89859=ADVANCED_FACE('',(#10580),#86380,.F.);
#89860=ADVANCED_FACE('',(#10581),#7942,.T.);
#89861=ADVANCED_FACE('',(#10582),#7943,.F.);
#89862=ADVANCED_FACE('',(#10583),#2788,.F.);
#89863=ADVANCED_FACE('',(#10584),#86381,.T.);
#89864=ADVANCED_FACE('',(#10585),#7944,.F.);
#89865=ADVANCED_FACE('',(#10586),#86382,.T.);
#89866=ADVANCED_FACE('',(#10587),#7945,.F.);
#89867=ADVANCED_FACE('',(#10588),#2789,.F.);
#89868=ADVANCED_FACE('',(#10589),#7946,.T.);
#89869=ADVANCED_FACE('',(#10590),#2790,.F.);
#89870=ADVANCED_FACE('',(#10591),#7947,.F.);
#89871=ADVANCED_FACE('',(#10592),#86383,.T.);
#89872=ADVANCED_FACE('',(#10593),#7948,.F.);
#89873=ADVANCED_FACE('',(#10594),#86384,.T.);
#89874=ADVANCED_FACE('',(#10595),#7949,.F.);
#89875=ADVANCED_FACE('',(#10596),#2791,.F.);
#89876=ADVANCED_FACE('',(#10597),#7950,.F.);
#89877=ADVANCED_FACE('',(#10598),#2792,.F.);
#89878=ADVANCED_FACE('',(#10599),#3426,.F.);
#89879=ADVANCED_FACE('',(#10600),#7951,.F.);
#89880=ADVANCED_FACE('',(#10601),#86385,.T.);
#89881=ADVANCED_FACE('',(#10602),#7952,.F.);
#89882=ADVANCED_FACE('',(#10603),#86386,.T.);
#89883=ADVANCED_FACE('',(#10604),#7953,.F.);
#89884=ADVANCED_FACE('',(#10605),#2793,.F.);
#89885=ADVANCED_FACE('',(#10606),#7954,.T.);
#89886=ADVANCED_FACE('',(#10607),#3427,.F.);
#89887=ADVANCED_FACE('',(#10608),#2794,.T.);
#89888=ADVANCED_FACE('',(#10609),#2795,.F.);
#89889=ADVANCED_FACE('',(#10610),#7955,.F.);
#89890=ADVANCED_FACE('',(#10611),#7956,.F.);
#89891=ADVANCED_FACE('',(#10612),#2796,.F.);
#89892=ADVANCED_FACE('',(#10613),#86387,.T.);
#89893=ADVANCED_FACE('',(#10614),#7957,.F.);
#89894=ADVANCED_FACE('',(#10615),#86388,.T.);
#89895=ADVANCED_FACE('',(#10616),#7958,.F.);
#89896=ADVANCED_FACE('',(#10617),#2797,.F.);
#89897=ADVANCED_FACE('',(#10618),#2798,.F.);
#89898=ADVANCED_FACE('',(#10619),#7959,.T.);
#89899=ADVANCED_FACE('',(#10620),#7960,.F.);
#89900=ADVANCED_FACE('',(#10621),#86389,.T.);
#89901=ADVANCED_FACE('',(#10622),#7961,.T.);
#89902=ADVANCED_FACE('',(#10623),#86390,.T.);
#89903=ADVANCED_FACE('',(#10624),#7962,.T.);
#89904=ADVANCED_FACE('',(#10625),#2799,.F.);
#89905=ADVANCED_FACE('',(#10626),#2800,.F.);
#89906=ADVANCED_FACE('',(#10627),#7963,.F.);
#89907=ADVANCED_FACE('',(#10628),#86391,.T.);
#89908=ADVANCED_FACE('',(#10629),#7964,.T.);
#89909=ADVANCED_FACE('',(#10630),#86392,.T.);
#89910=ADVANCED_FACE('',(#10631),#7965,.F.);
#89911=ADVANCED_FACE('',(#10632),#2801,.F.);
#89912=ADVANCED_FACE('',(#10633),#2802,.F.);
#89913=ADVANCED_FACE('',(#10634),#7966,.T.);
#89914=ADVANCED_FACE('',(#10635),#7967,.F.);
#89915=ADVANCED_FACE('',(#10636),#86393,.T.);
#89916=ADVANCED_FACE('',(#10637),#7968,.F.);
#89917=ADVANCED_FACE('',(#10638),#86394,.T.);
#89918=ADVANCED_FACE('',(#10639),#7969,.F.);
#89919=ADVANCED_FACE('',(#10640),#2803,.F.);
#89920=ADVANCED_FACE('',(#10641),#7970,.T.);
#89921=ADVANCED_FACE('',(#10642),#3428,.F.);
#89922=ADVANCED_FACE('',(#10643),#7971,.F.);
#89923=ADVANCED_FACE('',(#10644),#2804,.F.);
#89924=ADVANCED_FACE('',(#10645),#2805,.F.);
#89925=ADVANCED_FACE('',(#10646),#7972,.F.);
#89926=ADVANCED_FACE('',(#10647),#86395,.T.);
#89927=ADVANCED_FACE('',(#10648),#7973,.F.);
#89928=ADVANCED_FACE('',(#10649),#86396,.T.);
#89929=ADVANCED_FACE('',(#10650),#7974,.F.);
#89930=ADVANCED_FACE('',(#10651),#2806,.F.);
#89931=ADVANCED_FACE('',(#10652),#2807,.F.);
#89932=ADVANCED_FACE('',(#10653),#7975,.T.);
#89933=ADVANCED_FACE('',(#10654),#7976,.F.);
#89934=ADVANCED_FACE('',(#10655),#2808,.F.);
#89935=ADVANCED_FACE('',(#10656),#6988,.T.);
#89936=ADVANCED_FACE('',(#10657),#7977,.F.);
#89937=ADVANCED_FACE('',(#10658),#2809,.F.);
#89938=ADVANCED_FACE('',(#10659),#86397,.T.);
#89939=ADVANCED_FACE('',(#10660),#7978,.F.);
#89940=ADVANCED_FACE('',(#10661),#86398,.T.);
#89941=ADVANCED_FACE('',(#10662),#7979,.F.);
#89942=ADVANCED_FACE('',(#10663),#2810,.F.);
#89943=ADVANCED_FACE('',(#10664),#6989,.T.);
#89944=ADVANCED_FACE('',(#10665),#7980,.F.);
#89945=ADVANCED_FACE('',(#10666),#2811,.F.);
#89946=ADVANCED_FACE('',(#10667),#2812,.T.);
#89947=ADVANCED_FACE('',(#10668),#2813,.T.);
#89948=ADVANCED_FACE('',(#10669),#2814,.T.);
#89949=ADVANCED_FACE('',(#10670),#7981,.F.);
#89950=ADVANCED_FACE('',(#10671),#2815,.F.);
#89951=ADVANCED_FACE('',(#10672),#6990,.T.);
#89952=ADVANCED_FACE('',(#10673),#7982,.F.);
#89953=ADVANCED_FACE('',(#10674),#2816,.F.);
#89954=ADVANCED_FACE('',(#10675),#2817,.T.);
#89955=ADVANCED_FACE('',(#10676),#2818,.T.);
#89956=ADVANCED_FACE('',(#10677),#2819,.T.);
#89957=ADVANCED_FACE('',(#10678),#7983,.F.);
#89958=ADVANCED_FACE('',(#10679),#2820,.F.);
#89959=ADVANCED_FACE('',(#10680),#6991,.T.);
#89960=ADVANCED_FACE('',(#10681),#7984,.F.);
#89961=ADVANCED_FACE('',(#10682),#2821,.F.);
#89962=ADVANCED_FACE('',(#10683),#2822,.T.);
#89963=ADVANCED_FACE('',(#10684),#2823,.T.);
#89964=ADVANCED_FACE('',(#10685),#2824,.T.);
#89965=ADVANCED_FACE('',(#10686),#7985,.F.);
#89966=ADVANCED_FACE('',(#10687),#2825,.F.);
#89967=ADVANCED_FACE('',(#10688),#6992,.T.);
#89968=ADVANCED_FACE('',(#10689),#7986,.F.);
#89969=ADVANCED_FACE('',(#10690),#2826,.F.);
#89970=ADVANCED_FACE('',(#10691),#86399,.T.);
#89971=ADVANCED_FACE('',(#10692),#7987,.F.);
#89972=ADVANCED_FACE('',(#10693),#86400,.T.);
#89973=ADVANCED_FACE('',(#10694),#7988,.F.);
#89974=ADVANCED_FACE('',(#10695),#2827,.F.);
#89975=ADVANCED_FACE('',(#10696),#6993,.T.);
#89976=ADVANCED_FACE('',(#10697),#2828,.F.);
#89977=ADVANCED_FACE('',(#10698),#7989,.F.);
#89978=ADVANCED_FACE('',(#10699),#86401,.T.);
#89979=ADVANCED_FACE('',(#10700),#7990,.F.);
#89980=ADVANCED_FACE('',(#10701),#86402,.T.);
#89981=ADVANCED_FACE('',(#10702),#86403,.T.);
#89982=ADVANCED_FACE('',(#10703),#7991,.F.);
#89983=ADVANCED_FACE('',(#10704),#86404,.T.);
#89984=ADVANCED_FACE('',(#10705),#7992,.F.);
#89985=ADVANCED_FACE('',(#10706),#2829,.T.);
#89986=ADVANCED_FACE('',(#10707),#2830,.T.);
#89987=ADVANCED_FACE('',(#10708),#2831,.T.);
#89988=ADVANCED_FACE('',(#10709),#7993,.F.);
#89989=ADVANCED_FACE('',(#10710),#2832,.F.);
#89990=ADVANCED_FACE('',(#10711),#6994,.T.);
#89991=ADVANCED_FACE('',(#10712),#7994,.F.);
#89992=ADVANCED_FACE('',(#10713),#2833,.F.);
#89993=ADVANCED_FACE('',(#10714),#2834,.T.);
#89994=ADVANCED_FACE('',(#10715),#2835,.T.);
#89995=ADVANCED_FACE('',(#10716),#2836,.T.);
#89996=ADVANCED_FACE('',(#10717),#7995,.F.);
#89997=ADVANCED_FACE('',(#10718),#2837,.F.);
#89998=ADVANCED_FACE('',(#10719),#6995,.T.);
#89999=ADVANCED_FACE('',(#10720),#2838,.F.);
#90000=ADVANCED_FACE('',(#10721),#7996,.F.);
#90001=ADVANCED_FACE('',(#10722),#86405,.T.);
#90002=ADVANCED_FACE('',(#10723),#7997,.T.);
#90003=ADVANCED_FACE('',(#10724),#86406,.T.);
#90004=ADVANCED_FACE('',(#10725),#7998,.F.);
#90005=ADVANCED_FACE('',(#10726),#2839,.F.);
#90006=ADVANCED_FACE('',(#10727),#3429,.F.);
#90007=ADVANCED_FACE('',(#10728),#86407,.T.);
#90008=ADVANCED_FACE('',(#10729),#7999,.F.);
#90009=ADVANCED_FACE('',(#10730),#2840,.F.);
#90010=ADVANCED_FACE('',(#10731),#6996,.T.);
#90011=ADVANCED_FACE('',(#10732),#8000,.F.);
#90012=ADVANCED_FACE('',(#10733),#2841,.F.);
#90013=ADVANCED_FACE('',(#10734),#86408,.T.);
#90014=ADVANCED_FACE('',(#10735),#8001,.F.);
#90015=ADVANCED_FACE('',(#10736),#86409,.T.);
#90016=ADVANCED_FACE('',(#10737),#8002,.F.);
#90017=ADVANCED_FACE('',(#10738),#2842,.F.);
#90018=ADVANCED_FACE('',(#10739),#6997,.T.);
#90019=ADVANCED_FACE('',(#10740),#8003,.F.);
#90020=ADVANCED_FACE('',(#10741),#2843,.F.);
#90021=ADVANCED_FACE('',(#10742),#2844,.T.);
#90022=ADVANCED_FACE('',(#10743),#2845,.T.);
#90023=ADVANCED_FACE('',(#10744),#2846,.T.);
#90024=ADVANCED_FACE('',(#10745),#8004,.F.);
#90025=ADVANCED_FACE('',(#10746),#2847,.F.);
#90026=ADVANCED_FACE('',(#10747),#6998,.T.);
#90027=ADVANCED_FACE('',(#10748),#8005,.F.);
#90028=ADVANCED_FACE('',(#10749),#2848,.F.);
#90029=ADVANCED_FACE('',(#10750),#2849,.T.);
#90030=ADVANCED_FACE('',(#10751),#86410,.T.);
#90031=ADVANCED_FACE('',(#10752),#2850,.T.);
#90032=ADVANCED_FACE('',(#10753),#3430,.F.);
#90033=ADVANCED_FACE('',(#10754),#2851,.F.);
#90034=ADVANCED_FACE('',(#10755),#86411,.F.);
#90035=ADVANCED_FACE('',(#10756),#2852,.F.);
#90036=ADVANCED_FACE('',(#10757),#86412,.F.);
#90037=ADVANCED_FACE('',(#10758),#3431,.T.);
#90038=ADVANCED_FACE('',(#10759),#86413,.F.);
#90039=ADVANCED_FACE('',(#10760),#2853,.F.);
#90040=ADVANCED_FACE('',(#10761),#2854,.F.);
#90041=ADVANCED_FACE('',(#10762),#2855,.F.);
#90042=ADVANCED_FACE('',(#10763),#86414,.F.);
#90043=ADVANCED_FACE('',(#10764),#3432,.T.);
#90044=ADVANCED_FACE('',(#10765),#86415,.F.);
#90045=ADVANCED_FACE('',(#10766),#2856,.F.);
#90046=ADVANCED_FACE('',(#10767),#3433,.F.);
#90047=ADVANCED_FACE('',(#10768),#2857,.F.);
#90048=ADVANCED_FACE('',(#10769),#86416,.F.);
#90049=ADVANCED_FACE('',(#10770),#3434,.T.);
#90050=ADVANCED_FACE('',(#10771),#86417,.F.);
#90051=ADVANCED_FACE('',(#10772),#2858,.F.);
#90052=ADVANCED_FACE('',(#10773),#86418,.F.);
#90053=ADVANCED_FACE('',(#10774),#86419,.F.);
#90054=ADVANCED_FACE('',(#10775),#3435,.T.);
#90055=ADVANCED_FACE('',(#10776),#86420,.T.);
#90056=ADVANCED_FACE('',(#10777),#3436,.T.);
#90057=ADVANCED_FACE('',(#10778),#3437,.T.);
#90058=ADVANCED_FACE('',(#10779),#3438,.T.);
#90059=ADVANCED_FACE('',(#10780),#86421,.T.);
#90060=ADVANCED_FACE('',(#10781),#3439,.T.);
#90061=ADVANCED_FACE('',(#10782),#3440,.T.);
#90062=ADVANCED_FACE('',(#10783),#3441,.T.);
#90063=ADVANCED_FACE('',(#10784),#86422,.T.);
#90064=ADVANCED_FACE('',(#10785),#3442,.T.);
#90065=ADVANCED_FACE('',(#10786),#3443,.T.);
#90066=ADVANCED_FACE('',(#10787),#3444,.T.);
#90067=ADVANCED_FACE('',(#10788),#86423,.T.);
#90068=ADVANCED_FACE('',(#10789),#3445,.T.);
#90069=ADVANCED_FACE('',(#10790),#86424,.F.);
#90070=ADVANCED_FACE('',(#10791),#86425,.F.);
#90071=ADVANCED_FACE('',(#10792),#3446,.F.);
#90072=ADVANCED_FACE('',(#10793),#86426,.T.);
#90073=ADVANCED_FACE('',(#10794),#8006,.F.);
#90074=ADVANCED_FACE('',(#10795),#86427,.F.);
#90075=ADVANCED_FACE('',(#10796),#86428,.F.);
#90076=ADVANCED_FACE('',(#10797),#86429,.F.);
#90077=ADVANCED_FACE('',(#10798),#3447,.F.);
#90078=ADVANCED_FACE('',(#10799),#86430,.F.);
#90079=ADVANCED_FACE('',(#10800),#3448,.F.);
#90080=ADVANCED_FACE('',(#10801),#86431,.F.);
#90081=ADVANCED_FACE('',(#10802),#86432,.F.);
#90082=ADVANCED_FACE('',(#10803),#86433,.F.);
#90083=ADVANCED_FACE('',(#10804),#3449,.F.);
#90084=ADVANCED_FACE('',(#10805),#86434,.F.);
#90085=ADVANCED_FACE('',(#10806),#3450,.F.);
#90086=ADVANCED_FACE('',(#10807),#86435,.F.);
#90087=ADVANCED_FACE('',(#10808),#86436,.F.);
#90088=ADVANCED_FACE('',(#10809),#2859,.F.);
#90089=ADVANCED_FACE('',(#10810),#3451,.F.);
#90090=ADVANCED_FACE('',(#10811),#86437,.F.);
#90091=ADVANCED_FACE('',(#10812),#3452,.F.);
#90092=ADVANCED_FACE('',(#10813),#86438,.F.);
#90093=ADVANCED_FACE('',(#10814),#3453,.F.);
#90094=ADVANCED_FACE('',(#10815),#86439,.F.);
#90095=ADVANCED_FACE('',(#10816),#3454,.F.);
#90096=ADVANCED_FACE('',(#10817),#86440,.F.);
#90097=ADVANCED_FACE('',(#10818),#3455,.F.);
#90098=ADVANCED_FACE('',(#10819),#86441,.F.);
#90099=ADVANCED_FACE('',(#10820),#3456,.F.);
#90100=ADVANCED_FACE('',(#10821),#86442,.F.);
#90101=ADVANCED_FACE('',(#10822),#86443,.T.);
#90102=ADVANCED_FACE('',(#10823),#86444,.F.);
#90103=ADVANCED_FACE('',(#10824),#3457,.F.);
#90104=ADVANCED_FACE('',(#10825),#2860,.F.);
#90105=ADVANCED_FACE('',(#10826),#2861,.F.);
#90106=ADVANCED_FACE('',(#10827),#2862,.F.);
#90107=ADVANCED_FACE('',(#10828),#86445,.T.);
#90108=ADVANCED_FACE('',(#10829),#8007,.F.);
#90109=ADVANCED_FACE('',(#10830),#8008,.T.);
#90110=ADVANCED_FACE('',(#10831),#8009,.T.);
#90111=ADVANCED_FACE('',(#10832),#86446,.T.);
#90112=ADVANCED_FACE('',(#10833),#86447,.F.);
#90113=ADVANCED_FACE('',(#10834),#2863,.F.);
#90114=ADVANCED_FACE('',(#10835),#86448,.F.);
#90115=ADVANCED_FACE('',(#10836),#2864,.F.);
#90116=ADVANCED_FACE('',(#10837),#86449,.F.);
#90117=ADVANCED_FACE('',(#10838),#86450,.T.);
#90118=ADVANCED_FACE('',(#10839),#86451,.F.);
#90119=ADVANCED_FACE('',(#10840),#2865,.F.);
#90120=ADVANCED_FACE('',(#10841),#86452,.F.);
#90121=ADVANCED_FACE('',(#10842),#2866,.F.);
#90122=ADVANCED_FACE('',(#10843),#86453,.F.);
#90123=ADVANCED_FACE('',(#10844),#86454,.T.);
#90124=ADVANCED_FACE('',(#10845),#2867,.F.);
#90125=ADVANCED_FACE('',(#10846),#86455,.F.);
#90126=ADVANCED_FACE('',(#10847),#2868,.T.);
#90127=ADVANCED_FACE('',(#10848),#86456,.F.);
#90128=ADVANCED_FACE('',(#10849),#2869,.F.);
#90129=ADVANCED_FACE('',(#10850),#86457,.F.);
#90130=ADVANCED_FACE('',(#10851),#2870,.F.);
#90131=ADVANCED_FACE('',(#10852),#86458,.F.);
#90132=ADVANCED_FACE('',(#10853),#86459,.T.);
#90133=ADVANCED_FACE('',(#10854),#2871,.T.);
#90134=ADVANCED_FACE('',(#10855),#86460,.F.);
#90135=ADVANCED_FACE('',(#10856),#2872,.F.);
#90136=ADVANCED_FACE('',(#10857),#86461,.T.);
#90137=ADVANCED_FACE('',(#10858),#86462,.F.);
#90138=ADVANCED_FACE('',(#10859),#2873,.F.);
#90139=ADVANCED_FACE('',(#10860),#86463,.F.);
#90140=ADVANCED_FACE('',(#10861),#2874,.F.);
#90141=ADVANCED_FACE('',(#10862),#86464,.F.);
#90142=ADVANCED_FACE('',(#10863),#86465,.T.);
#90143=ADVANCED_FACE('',(#10864),#86466,.T.);
#90144=ADVANCED_FACE('',(#10865),#86467,.F.);
#90145=ADVANCED_FACE('',(#10866),#2875,.F.);
#90146=ADVANCED_FACE('',(#10867),#86468,.F.);
#90147=ADVANCED_FACE('',(#10868),#2876,.F.);
#90148=ADVANCED_FACE('',(#10869),#86469,.F.);
#90149=ADVANCED_FACE('',(#10870),#86470,.T.);
#90150=ADVANCED_FACE('',(#10871),#2877,.T.);
#90151=ADVANCED_FACE('',(#10872),#86471,.F.);
#90152=ADVANCED_FACE('',(#10873),#2878,.F.);
#90153=ADVANCED_FACE('',(#10874),#86472,.F.);
#90154=ADVANCED_FACE('',(#10875),#2879,.F.);
#90155=ADVANCED_FACE('',(#10876),#86473,.F.);
#90156=ADVANCED_FACE('',(#10877),#86474,.T.);
#90157=ADVANCED_FACE('',(#10878),#2880,.T.);
#90158=ADVANCED_FACE('',(#10879),#86475,.T.);
#90159=ADVANCED_FACE('',(#10880),#86476,.F.);
#90160=ADVANCED_FACE('',(#10881),#2881,.F.);
#90161=ADVANCED_FACE('',(#10882),#86477,.F.);
#90162=ADVANCED_FACE('',(#10883),#2882,.F.);
#90163=ADVANCED_FACE('',(#10884),#86478,.F.);
#90164=ADVANCED_FACE('',(#10885),#86479,.T.);
#90165=ADVANCED_FACE('',(#10886),#2883,.T.);
#90166=ADVANCED_FACE('',(#10887),#86480,.F.);
#90167=ADVANCED_FACE('',(#10888),#2884,.F.);
#90168=ADVANCED_FACE('',(#10889),#86481,.T.);
#90169=ADVANCED_FACE('',(#10890),#86482,.F.);
#90170=ADVANCED_FACE('',(#10891),#2885,.F.);
#90171=ADVANCED_FACE('',(#10892),#86483,.F.);
#90172=ADVANCED_FACE('',(#10893),#2886,.F.);
#90173=ADVANCED_FACE('',(#10894),#86484,.F.);
#90174=ADVANCED_FACE('',(#10895),#86485,.T.);
#90175=ADVANCED_FACE('',(#10896),#2887,.F.);
#90176=ADVANCED_FACE('',(#10897),#86486,.F.);
#90177=ADVANCED_FACE('',(#10898),#3458,.T.);
#90178=ADVANCED_FACE('',(#10899),#86487,.F.);
#90179=ADVANCED_FACE('',(#10900),#2888,.F.);
#90180=ADVANCED_FACE('',(#10901),#3459,.F.);
#90181=ADVANCED_FACE('',(#10902),#2889,.F.);
#90182=ADVANCED_FACE('',(#10903),#86488,.F.);
#90183=ADVANCED_FACE('',(#10904),#3460,.T.);
#90184=ADVANCED_FACE('',(#10905),#86489,.F.);
#90185=ADVANCED_FACE('',(#10906),#2890,.F.);
#90186=ADVANCED_FACE('',(#10907),#2891,.F.);
#90187=ADVANCED_FACE('',(#10908),#2892,.F.);
#90188=ADVANCED_FACE('',(#10909),#86490,.F.);
#90189=ADVANCED_FACE('',(#10910),#3461,.T.);
#90190=ADVANCED_FACE('',(#10911),#86491,.F.);
#90191=ADVANCED_FACE('',(#10912),#2893,.F.);
#90192=ADVANCED_FACE('',(#10913),#2894,.F.);
#90193=ADVANCED_FACE('',(#10914),#2895,.F.);
#90194=ADVANCED_FACE('',(#10915),#86492,.F.);
#90195=ADVANCED_FACE('',(#10916),#3462,.T.);
#90196=ADVANCED_FACE('',(#10917),#86493,.F.);
#90197=ADVANCED_FACE('',(#10918),#2896,.F.);
#90198=ADVANCED_FACE('',(#10919),#2897,.F.);
#90199=ADVANCED_FACE('',(#10920),#2898,.F.);
#90200=ADVANCED_FACE('',(#10921),#86494,.F.);
#90201=ADVANCED_FACE('',(#10922),#3463,.T.);
#90202=ADVANCED_FACE('',(#10923),#86495,.F.);
#90203=ADVANCED_FACE('',(#10924),#2899,.F.);
#90204=ADVANCED_FACE('',(#10925),#3464,.F.);
#90205=ADVANCED_FACE('',(#10926),#2900,.F.);
#90206=ADVANCED_FACE('',(#10927),#86496,.F.);
#90207=ADVANCED_FACE('',(#10928),#3465,.T.);
#90208=ADVANCED_FACE('',(#10929),#86497,.F.);
#90209=ADVANCED_FACE('',(#10930),#2901,.F.);
#90210=ADVANCED_FACE('',(#10931),#8010,.T.);
#90211=ADVANCED_FACE('',(#10932),#3466,.T.);
#90212=ADVANCED_FACE('',(#10933),#8011,.T.);
#90213=ADVANCED_FACE('',(#10934),#86498,.T.);
#90214=ADVANCED_FACE('',(#10935),#3467,.T.);
#90215=ADVANCED_FACE('',(#10936),#8012,.T.);
#90216=ADVANCED_FACE('',(#10937),#86499,.T.);
#90217=ADVANCED_FACE('',(#10938),#2902,.F.);
#90218=ADVANCED_FACE('',(#10939),#3468,.F.);
#90219=ADVANCED_FACE('',(#10940),#2903,.F.);
#90220=ADVANCED_FACE('',(#10941),#86500,.T.);
#90221=ADVANCED_FACE('',(#10942),#86501,.F.);
#90222=ADVANCED_FACE('',(#10943),#2904,.F.);
#90223=ADVANCED_FACE('',(#10944),#3469,.F.);
#90224=ADVANCED_FACE('',(#10945),#2905,.F.);
#90225=ADVANCED_FACE('',(#10946),#86502,.F.);
#90226=ADVANCED_FACE('',(#10947),#2906,.F.);
#90227=ADVANCED_FACE('',(#10948),#2907,.F.);
#90228=ADVANCED_FACE('',(#10949),#2908,.F.);
#90229=ADVANCED_FACE('',(#10950),#86503,.F.);
#90230=ADVANCED_FACE('',(#10951),#3470,.T.);
#90231=ADVANCED_FACE('',(#10952),#86504,.F.);
#90232=ADVANCED_FACE('',(#10953),#2909,.F.);
#90233=ADVANCED_FACE('',(#10954),#2910,.F.);
#90234=ADVANCED_FACE('',(#10955),#2911,.F.);
#90235=ADVANCED_FACE('',(#10956),#86505,.F.);
#90236=ADVANCED_FACE('',(#10957),#3471,.T.);
#90237=ADVANCED_FACE('',(#10958),#86506,.F.);
#90238=ADVANCED_FACE('',(#10959),#2912,.F.);
#90239=ADVANCED_FACE('',(#10960),#3472,.F.);
#90240=ADVANCED_FACE('',(#10961),#2913,.F.);
#90241=ADVANCED_FACE('',(#10962),#86507,.F.);
#90242=ADVANCED_FACE('',(#10963),#3473,.T.);
#90243=ADVANCED_FACE('',(#10964),#86508,.F.);
#90244=ADVANCED_FACE('',(#10965),#3474,.F.);
#90245=ADVANCED_FACE('',(#10966),#2914,.F.);
#90246=ADVANCED_FACE('',(#10967),#86509,.F.);
#90247=ADVANCED_FACE('',(#10968),#3475,.T.);
#90248=ADVANCED_FACE('',(#10969),#86510,.F.);
#90249=ADVANCED_FACE('',(#10970),#2915,.F.);
#90250=ADVANCED_FACE('',(#10971),#3476,.F.);
#90251=ADVANCED_FACE('',(#10972),#2916,.F.);
#90252=ADVANCED_FACE('',(#10973),#86511,.F.);
#90253=ADVANCED_FACE('',(#10974),#3477,.T.);
#90254=ADVANCED_FACE('',(#10975),#86512,.F.);
#90255=ADVANCED_FACE('',(#10976),#2917,.F.);
#90256=ADVANCED_FACE('',(#10977),#2918,.F.);
#90257=ADVANCED_FACE('',(#10978),#2919,.F.);
#90258=ADVANCED_FACE('',(#10979),#86513,.F.);
#90259=ADVANCED_FACE('',(#10980),#3478,.T.);
#90260=ADVANCED_FACE('',(#10981),#86514,.F.);
#90261=ADVANCED_FACE('',(#10982),#2920,.F.);
#90262=ADVANCED_FACE('',(#10983),#86515,.T.);
#90263=ADVANCED_FACE('',(#10984),#8013,.T.);
#90264=ADVANCED_FACE('',(#10985),#3479,.T.);
#90265=ADVANCED_FACE('',(#10986),#8014,.T.);
#90266=ADVANCED_FACE('',(#10987),#86516,.T.);
#90267=ADVANCED_FACE('',(#10988),#3480,.T.);
#90268=ADVANCED_FACE('',(#10989),#8015,.T.);
#90269=ADVANCED_FACE('',(#10990),#86517,.T.);
#90270=ADVANCED_FACE('',(#10991),#2921,.F.);
#90271=ADVANCED_FACE('',(#10992),#3481,.F.);
#90272=ADVANCED_FACE('',(#10993),#86518,.F.);
#90273=ADVANCED_FACE('',(#10994),#2922,.F.);
#90274=ADVANCED_FACE('',(#10995),#2923,.T.);
#90275=ADVANCED_FACE('',(#10996),#8016,.T.);
#90276=ADVANCED_FACE('',(#10997),#2924,.T.);
#90277=ADVANCED_FACE('',(#10998),#2925,.F.);
#90278=ADVANCED_FACE('',(#10999),#86519,.T.);
#90279=ADVANCED_FACE('',(#11000),#3482,.T.);
#90280=ADVANCED_FACE('',(#11001,#7445,#7446,#7447,#7448),#8017,.F.);
#90281=ADVANCED_FACE('',(#11002),#3483,.T.);
#90282=ADVANCED_FACE('',(#11003),#86520,.T.);
#90283=ADVANCED_FACE('',(#11004),#3484,.F.);
#90284=ADVANCED_FACE('',(#11005),#8018,.F.);
#90285=ADVANCED_FACE('',(#11006),#8019,.F.);
#90286=ADVANCED_FACE('',(#11007),#8020,.F.);
#90287=ADVANCED_FACE('',(#11008),#3485,.F.);
#90288=ADVANCED_FACE('',(#11009),#6999,.T.);
#90289=ADVANCED_FACE('',(#11010),#3486,.T.);
#90290=ADVANCED_FACE('',(#11011),#86521,.T.);
#90291=ADVANCED_FACE('',(#11012),#86522,.F.);
#90292=ADVANCED_FACE('',(#11013,#7449,#7450,#7451,#7452),#8021,.F.);
#90293=ADVANCED_FACE('',(#11014),#8022,.F.);
#90294=ADVANCED_FACE('',(#11015),#8023,.F.);
#90295=ADVANCED_FACE('',(#11016),#8024,.F.);
#90296=ADVANCED_FACE('',(#11017),#8025,.F.);
#90297=ADVANCED_FACE('',(#11018),#8026,.F.);
#90298=ADVANCED_FACE('',(#11019),#8027,.F.);
#90299=ADVANCED_FACE('',(#11020),#7000,.F.);
#90300=ADVANCED_FACE('',(#11021),#7001,.F.);
#90301=ADVANCED_FACE('',(#11022),#7002,.F.);
#90302=ADVANCED_FACE('',(#11023),#7003,.F.);
#90303=ADVANCED_FACE('',(#11024),#7004,.F.);
#90304=ADVANCED_FACE('',(#11025),#7005,.F.);
#90305=ADVANCED_FACE('',(#11026),#7006,.F.);
#90306=ADVANCED_FACE('',(#11027),#3487,.T.);
#90307=ADVANCED_FACE('',(#11028),#8028,.F.);
#90308=ADVANCED_FACE('',(#11029,#7453),#8029,.T.);
#90309=ADVANCED_FACE('',(#11030),#86523,.T.);
#90310=ADVANCED_FACE('',(#11031),#7007,.T.);
#90311=ADVANCED_FACE('',(#11032),#8030,.T.);
#90312=ADVANCED_FACE('',(#11033),#86524,.T.);
#90313=ADVANCED_FACE('',(#11034,#7454),#8031,.F.);
#90314=ADVANCED_FACE('',(#11035),#86525,.T.);
#90315=ADVANCED_FACE('',(#11036),#8032,.F.);
#90316=ADVANCED_FACE('',(#11037),#2926,.T.);
#90317=ADVANCED_FACE('',(#11038),#3488,.T.);
#90318=ADVANCED_FACE('',(#11039),#2927,.F.);
#90319=ADVANCED_FACE('',(#11040),#2928,.F.);
#90320=ADVANCED_FACE('',(#11041),#1018,.F.);
#90321=ADVANCED_FACE('',(#11042),#2929,.F.);
#90322=ADVANCED_FACE('',(#11043),#3489,.F.);
#90323=ADVANCED_FACE('',(#11044),#2930,.F.);
#90324=ADVANCED_FACE('',(#11045),#3490,.F.);
#90325=ADVANCED_FACE('',(#11046),#2931,.F.);
#90326=ADVANCED_FACE('',(#11047),#3491,.F.);
#90327=ADVANCED_FACE('',(#11048),#2932,.F.);
#90328=ADVANCED_FACE('',(#11049),#2933,.F.);
#90329=ADVANCED_FACE('',(#11050),#2934,.F.);
#90330=ADVANCED_FACE('',(#11051),#1019,.F.);
#90331=ADVANCED_FACE('',(#11052),#2935,.F.);
#90332=ADVANCED_FACE('',(#11053),#2936,.F.);
#90333=ADVANCED_FACE('',(#11054),#2937,.F.);
#90334=ADVANCED_FACE('',(#11055),#2938,.F.);
#90335=ADVANCED_FACE('',(#11056),#2939,.F.);
#90336=ADVANCED_FACE('',(#11057),#1020,.F.);
#90337=ADVANCED_FACE('',(#11058),#2940,.F.);
#90338=ADVANCED_FACE('',(#11059),#2941,.F.);
#90339=ADVANCED_FACE('',(#11060),#2942,.F.);
#90340=ADVANCED_FACE('',(#11061),#3492,.F.);
#90341=ADVANCED_FACE('',(#11062),#1021,.F.);
#90342=ADVANCED_FACE('',(#11063),#3493,.F.);
#90343=ADVANCED_FACE('',(#11064),#2943,.F.);
#90344=ADVANCED_FACE('',(#11065),#3494,.F.);
#90345=ADVANCED_FACE('',(#11066),#3495,.F.);
#90346=ADVANCED_FACE('',(#11067),#3496,.F.);
#90347=ADVANCED_FACE('',(#11068),#3497,.F.);
#90348=ADVANCED_FACE('',(#11069),#3498,.F.);
#90349=ADVANCED_FACE('',(#11070),#3499,.F.);
#90350=ADVANCED_FACE('',(#11071),#3500,.F.);
#90351=ADVANCED_FACE('',(#11072),#3501,.F.);
#90352=ADVANCED_FACE('',(#11073),#2944,.F.);
#90353=ADVANCED_FACE('',(#11074),#2945,.F.);
#90354=ADVANCED_FACE('',(#11075),#2946,.F.);
#90355=ADVANCED_FACE('',(#11076),#2947,.F.);
#90356=ADVANCED_FACE('',(#11077),#2948,.F.);
#90357=ADVANCED_FACE('',(#11078),#2949,.F.);
#90358=ADVANCED_FACE('',(#11079),#2950,.F.);
#90359=ADVANCED_FACE('',(#11080),#2951,.F.);
#90360=ADVANCED_FACE('',(#11081),#2952,.F.);
#90361=ADVANCED_FACE('',(#11082),#2953,.F.);
#90362=ADVANCED_FACE('',(#11083),#2954,.F.);
#90363=ADVANCED_FACE('',(#11084),#2955,.F.);
#90364=ADVANCED_FACE('',(#11085),#3502,.F.);
#90365=ADVANCED_FACE('',(#11086),#2956,.F.);
#90366=ADVANCED_FACE('',(#11087),#3503,.F.);
#90367=ADVANCED_FACE('',(#11088),#2957,.F.);
#90368=ADVANCED_FACE('',(#11089),#2958,.F.);
#90369=ADVANCED_FACE('',(#11090),#2959,.F.);
#90370=ADVANCED_FACE('',(#11091),#2960,.F.);
#90371=ADVANCED_FACE('',(#11092),#2961,.F.);
#90372=ADVANCED_FACE('',(#11093),#2962,.F.);
#90373=ADVANCED_FACE('',(#11094),#2963,.F.);
#90374=ADVANCED_FACE('',(#11095),#2964,.F.);
#90375=ADVANCED_FACE('',(#11096),#2965,.F.);
#90376=ADVANCED_FACE('',(#11097),#86526,.T.);
#90377=ADVANCED_FACE('',(#11098),#2966,.F.);
#90378=ADVANCED_FACE('',(#11099),#3504,.T.);
#90379=ADVANCED_FACE('',(#11100),#2967,.F.);
#90380=ADVANCED_FACE('',(#11101),#86527,.T.);
#90381=ADVANCED_FACE('',(#11102),#86528,.T.);
#90382=ADVANCED_FACE('',(#11103),#2968,.F.);
#90383=ADVANCED_FACE('',(#11104),#3505,.T.);
#90384=ADVANCED_FACE('',(#11105),#2969,.F.);
#90385=ADVANCED_FACE('',(#11106),#86529,.T.);
#90386=ADVANCED_FACE('',(#11107),#86530,.T.);
#90387=ADVANCED_FACE('',(#11108),#2970,.F.);
#90388=ADVANCED_FACE('',(#11109),#3506,.T.);
#90389=ADVANCED_FACE('',(#11110),#2971,.F.);
#90390=ADVANCED_FACE('',(#11111),#86531,.T.);
#90391=ADVANCED_FACE('',(#11112),#86532,.T.);
#90392=ADVANCED_FACE('',(#11113),#2972,.F.);
#90393=ADVANCED_FACE('',(#11114),#3507,.T.);
#90394=ADVANCED_FACE('',(#11115),#2973,.F.);
#90395=ADVANCED_FACE('',(#11116),#86533,.T.);
#90396=ADVANCED_FACE('',(#11117),#86534,.T.);
#90397=ADVANCED_FACE('',(#11118),#86535,.T.);
#90398=ADVANCED_FACE('',(#11119),#86536,.T.);
#90399=ADVANCED_FACE('',(#11120),#86537,.T.);
#90400=ADVANCED_FACE('',(#11121),#86538,.T.);
#90401=ADVANCED_FACE('',(#11122),#86539,.T.);
#90402=ADVANCED_FACE('',(#11123),#86540,.T.);
#90403=ADVANCED_FACE('',(#11124),#86541,.T.);
#90404=ADVANCED_FACE('',(#11125),#3508,.T.);
#90405=ADVANCED_FACE('',(#11126),#86542,.T.);
#90406=ADVANCED_FACE('',(#11127),#3509,.T.);
#90407=ADVANCED_FACE('',(#11128),#3510,.T.);
#90408=ADVANCED_FACE('',(#11129),#3511,.T.);
#90409=ADVANCED_FACE('',(#11130),#86543,.T.);
#90410=ADVANCED_FACE('',(#11131),#3512,.T.);
#90411=ADVANCED_FACE('',(#11132),#3513,.T.);
#90412=ADVANCED_FACE('',(#11133),#3514,.T.);
#90413=ADVANCED_FACE('',(#11134),#86544,.T.);
#90414=ADVANCED_FACE('',(#11135),#3515,.T.);
#90415=ADVANCED_FACE('',(#11136),#86545,.T.);
#90416=ADVANCED_FACE('',(#11137),#3516,.T.);
#90417=ADVANCED_FACE('',(#11138),#3517,.T.);
#90418=ADVANCED_FACE('',(#11139),#3518,.T.);
#90419=ADVANCED_FACE('',(#11140),#86546,.T.);
#90420=ADVANCED_FACE('',(#11141),#86547,.T.);
#90421=ADVANCED_FACE('',(#11142),#3519,.T.);
#90422=ADVANCED_FACE('',(#11143),#3520,.T.);
#90423=ADVANCED_FACE('',(#11144),#86548,.T.);
#90424=ADVANCED_FACE('',(#11145),#3521,.T.);
#90425=ADVANCED_FACE('',(#11146),#3522,.T.);
#90426=ADVANCED_FACE('',(#11147),#3523,.T.);
#90427=ADVANCED_FACE('',(#11148),#86549,.T.);
#90428=ADVANCED_FACE('',(#11149),#86550,.T.);
#90429=ADVANCED_FACE('',(#11150),#3524,.T.);
#90430=ADVANCED_FACE('',(#11151),#3525,.T.);
#90431=ADVANCED_FACE('',(#11152),#86551,.T.);
#90432=ADVANCED_FACE('',(#11153),#86552,.T.);
#90433=ADVANCED_FACE('',(#11154),#3526,.T.);
#90434=ADVANCED_FACE('',(#11155),#3527,.T.);
#90435=ADVANCED_FACE('',(#11156),#86553,.T.);
#90436=ADVANCED_FACE('',(#11157),#86554,.T.);
#90437=ADVANCED_FACE('',(#11158),#3528,.T.);
#90438=ADVANCED_FACE('',(#11159),#3529,.T.);
#90439=ADVANCED_FACE('',(#11160),#86555,.T.);
#90440=ADVANCED_FACE('',(#11161),#86556,.T.);
#90441=ADVANCED_FACE('',(#11162),#3530,.T.);
#90442=ADVANCED_FACE('',(#11163),#3531,.T.);
#90443=ADVANCED_FACE('',(#11164),#3532,.T.);
#90444=ADVANCED_FACE('',(#11165),#86557,.T.);
#90445=ADVANCED_FACE('',(#11166),#3533,.T.);
#90446=ADVANCED_FACE('',(#11167),#3534,.T.);
#90447=ADVANCED_FACE('',(#11168),#3535,.T.);
#90448=ADVANCED_FACE('',(#11169),#86558,.T.);
#90449=ADVANCED_FACE('',(#11170),#86559,.T.);
#90450=ADVANCED_FACE('',(#11171),#3536,.T.);
#90451=ADVANCED_FACE('',(#11172),#3537,.T.);
#90452=ADVANCED_FACE('',(#11173),#86560,.T.);
#90453=ADVANCED_FACE('',(#11174),#86561,.T.);
#90454=ADVANCED_FACE('',(#11175),#3538,.T.);
#90455=ADVANCED_FACE('',(#11176),#3539,.T.);
#90456=ADVANCED_FACE('',(#11177),#86562,.T.);
#90457=ADVANCED_FACE('',(#11178),#86563,.T.);
#90458=ADVANCED_FACE('',(#11179),#3540,.T.);
#90459=ADVANCED_FACE('',(#11180),#3541,.T.);
#90460=ADVANCED_FACE('',(#11181),#86564,.T.);
#90461=ADVANCED_FACE('',(#11182),#86565,.T.);
#90462=ADVANCED_FACE('',(#11183),#3542,.T.);
#90463=ADVANCED_FACE('',(#11184),#3543,.T.);
#90464=ADVANCED_FACE('',(#11185),#86566,.T.);
#90465=ADVANCED_FACE('',(#11186),#86567,.T.);
#90466=ADVANCED_FACE('',(#11187),#3544,.T.);
#90467=ADVANCED_FACE('',(#11188),#3545,.T.);
#90468=ADVANCED_FACE('',(#11189),#86568,.T.);
#90469=ADVANCED_FACE('',(#11190),#86569,.T.);
#90470=ADVANCED_FACE('',(#11191),#3546,.T.);
#90471=ADVANCED_FACE('',(#11192),#3547,.T.);
#90472=ADVANCED_FACE('',(#11193),#86570,.T.);
#90473=ADVANCED_FACE('',(#11194),#86571,.T.);
#90474=ADVANCED_FACE('',(#11195),#3548,.T.);
#90475=ADVANCED_FACE('',(#11196),#3549,.T.);
#90476=ADVANCED_FACE('',(#11197),#86572,.T.);
#90477=ADVANCED_FACE('',(#11198),#86573,.T.);
#90478=ADVANCED_FACE('',(#11199),#3550,.T.);
#90479=ADVANCED_FACE('',(#11200),#3551,.T.);
#90480=ADVANCED_FACE('',(#11201),#86574,.T.);
#90481=ADVANCED_FACE('',(#11202),#86575,.T.);
#90482=ADVANCED_FACE('',(#11203),#3552,.T.);
#90483=ADVANCED_FACE('',(#11204),#3553,.T.);
#90484=ADVANCED_FACE('',(#11205),#86576,.T.);
#90485=ADVANCED_FACE('',(#11206),#3554,.T.);
#90486=ADVANCED_FACE('',(#11207),#3555,.T.);
#90487=ADVANCED_FACE('',(#11208),#3556,.T.);
#90488=ADVANCED_FACE('',(#11209),#86577,.T.);
#90489=ADVANCED_FACE('',(#11210),#86578,.T.);
#90490=ADVANCED_FACE('',(#11211),#3557,.T.);
#90491=ADVANCED_FACE('',(#11212),#3558,.T.);
#90492=ADVANCED_FACE('',(#11213),#86579,.T.);
#90493=ADVANCED_FACE('',(#11214),#3559,.T.);
#90494=ADVANCED_FACE('',(#11215),#3560,.T.);
#90495=ADVANCED_FACE('',(#11216),#3561,.T.);
#90496=ADVANCED_FACE('',(#11217),#3562,.T.);
#90497=ADVANCED_FACE('',(#11218),#3563,.T.);
#90498=ADVANCED_FACE('',(#11219),#86580,.T.);
#90499=ADVANCED_FACE('',(#11220),#86581,.T.);
#90500=ADVANCED_FACE('',(#11221),#3564,.T.);
#90501=ADVANCED_FACE('',(#11222),#3565,.T.);
#90502=ADVANCED_FACE('',(#11223),#86582,.T.);
#90503=ADVANCED_FACE('',(#11224),#3566,.T.);
#90504=ADVANCED_FACE('',(#11225),#3567,.T.);
#90505=ADVANCED_FACE('',(#11226),#3568,.T.);
#90506=ADVANCED_FACE('',(#11227),#86583,.T.);
#90507=ADVANCED_FACE('',(#11228),#86584,.T.);
#90508=ADVANCED_FACE('',(#11229),#3569,.T.);
#90509=ADVANCED_FACE('',(#11230),#3570,.T.);
#90510=ADVANCED_FACE('',(#11231),#86585,.T.);
#90511=ADVANCED_FACE('',(#11232),#86586,.T.);
#90512=ADVANCED_FACE('',(#11233),#3571,.T.);
#90513=ADVANCED_FACE('',(#11234),#3572,.T.);
#90514=ADVANCED_FACE('',(#11235),#86587,.T.);
#90515=ADVANCED_FACE('',(#11236),#3573,.T.);
#90516=ADVANCED_FACE('',(#11237),#3574,.T.);
#90517=ADVANCED_FACE('',(#11238),#3575,.T.);
#90518=ADVANCED_FACE('',(#11239),#86588,.T.);
#90519=ADVANCED_FACE('',(#11240),#86589,.T.);
#90520=ADVANCED_FACE('',(#11241),#3576,.T.);
#90521=ADVANCED_FACE('',(#11242),#3577,.T.);
#90522=ADVANCED_FACE('',(#11243),#86590,.T.);
#90523=ADVANCED_FACE('',(#11244),#3578,.T.);
#90524=ADVANCED_FACE('',(#11245),#86591,.T.);
#90525=ADVANCED_FACE('',(#11246),#86592,.T.);
#90526=ADVANCED_FACE('',(#11247),#3579,.T.);
#90527=ADVANCED_FACE('',(#11248),#3580,.T.);
#90528=ADVANCED_FACE('',(#11249),#86593,.T.);
#90529=ADVANCED_FACE('',(#11250),#3581,.T.);
#90530=ADVANCED_FACE('',(#11251),#3582,.T.);
#90531=ADVANCED_FACE('',(#11252),#3583,.T.);
#90532=ADVANCED_FACE('',(#11253),#86594,.T.);
#90533=ADVANCED_FACE('',(#11254),#3584,.T.);
#90534=ADVANCED_FACE('',(#11255),#86595,.T.);
#90535=ADVANCED_FACE('',(#11256),#86596,.T.);
#90536=ADVANCED_FACE('',(#11257),#3585,.T.);
#90537=ADVANCED_FACE('',(#11258),#3586,.T.);
#90538=ADVANCED_FACE('',(#11259),#86597,.T.);
#90539=ADVANCED_FACE('',(#11260),#86598,.T.);
#90540=ADVANCED_FACE('',(#11261),#3587,.T.);
#90541=ADVANCED_FACE('',(#11262),#3588,.T.);
#90542=ADVANCED_FACE('',(#11263),#86599,.T.);
#90543=ADVANCED_FACE('',(#11264),#86600,.T.);
#90544=ADVANCED_FACE('',(#11265),#3589,.T.);
#90545=ADVANCED_FACE('',(#11266),#3590,.T.);
#90546=ADVANCED_FACE('',(#11267),#3591,.T.);
#90547=ADVANCED_FACE('',(#11268),#86601,.T.);
#90548=ADVANCED_FACE('',(#11269),#3592,.T.);
#90549=ADVANCED_FACE('',(#11270),#3593,.T.);
#90550=ADVANCED_FACE('',(#11271),#86602,.T.);
#90551=ADVANCED_FACE('',(#11272),#86603,.T.);
#90552=ADVANCED_FACE('',(#11273),#3594,.T.);
#90553=ADVANCED_FACE('',(#11274),#3595,.T.);
#90554=ADVANCED_FACE('',(#11275),#86604,.T.);
#90555=ADVANCED_FACE('',(#11276),#86605,.T.);
#90556=ADVANCED_FACE('',(#11277),#3596,.T.);
#90557=ADVANCED_FACE('',(#11278),#3597,.T.);
#90558=ADVANCED_FACE('',(#11279),#86606,.T.);
#90559=ADVANCED_FACE('',(#11280),#86607,.T.);
#90560=ADVANCED_FACE('',(#11281),#3598,.T.);
#90561=ADVANCED_FACE('',(#11282),#3599,.T.);
#90562=ADVANCED_FACE('',(#11283),#86608,.T.);
#90563=ADVANCED_FACE('',(#11284),#86609,.T.);
#90564=ADVANCED_FACE('',(#11285),#3600,.T.);
#90565=ADVANCED_FACE('',(#11286),#3601,.T.);
#90566=ADVANCED_FACE('',(#11287),#86610,.T.);
#90567=ADVANCED_FACE('',(#11288),#86611,.T.);
#90568=ADVANCED_FACE('',(#11289),#3602,.T.);
#90569=ADVANCED_FACE('',(#11290),#3603,.T.);
#90570=ADVANCED_FACE('',(#11291),#86612,.T.);
#90571=ADVANCED_FACE('',(#11292),#3604,.T.);
#90572=ADVANCED_FACE('',(#11293),#3605,.T.);
#90573=ADVANCED_FACE('',(#11294),#3606,.T.);
#90574=ADVANCED_FACE('',(#11295),#3607,.T.);
#90575=ADVANCED_FACE('',(#11296),#86613,.T.);
#90576=ADVANCED_FACE('',(#11297),#86614,.T.);
#90577=ADVANCED_FACE('',(#11298),#3608,.T.);
#90578=ADVANCED_FACE('',(#11299),#3609,.T.);
#90579=ADVANCED_FACE('',(#11300),#3610,.T.);
#90580=ADVANCED_FACE('',(#11301),#86615,.T.);
#90581=ADVANCED_FACE('',(#11302),#3611,.T.);
#90582=ADVANCED_FACE('',(#11303),#3612,.T.);
#90583=ADVANCED_FACE('',(#11304),#86616,.T.);
#90584=ADVANCED_FACE('',(#11305),#86617,.T.);
#90585=ADVANCED_FACE('',(#11306),#3613,.T.);
#90586=ADVANCED_FACE('',(#11307),#3614,.T.);
#90587=ADVANCED_FACE('',(#11308),#3615,.T.);
#90588=ADVANCED_FACE('',(#11309),#86618,.T.);
#90589=ADVANCED_FACE('',(#11310),#3616,.T.);
#90590=ADVANCED_FACE('',(#11311),#3617,.T.);
#90591=ADVANCED_FACE('',(#11312),#3618,.T.);
#90592=ADVANCED_FACE('',(#11313),#3619,.T.);
#90593=ADVANCED_FACE('',(#11314),#86619,.T.);
#90594=ADVANCED_FACE('',(#11315),#86620,.T.);
#90595=ADVANCED_FACE('',(#11316),#3620,.T.);
#90596=ADVANCED_FACE('',(#11317),#3621,.T.);
#90597=ADVANCED_FACE('',(#11318),#86621,.T.);
#90598=ADVANCED_FACE('',(#11319),#86622,.T.);
#90599=ADVANCED_FACE('',(#11320),#3622,.T.);
#90600=ADVANCED_FACE('',(#11321),#3623,.T.);
#90601=ADVANCED_FACE('',(#11322),#86623,.T.);
#90602=ADVANCED_FACE('',(#11323),#86624,.T.);
#90603=ADVANCED_FACE('',(#11324),#3624,.T.);
#90604=ADVANCED_FACE('',(#11325),#3625,.T.);
#90605=ADVANCED_FACE('',(#11326),#86625,.T.);
#90606=ADVANCED_FACE('',(#11327),#3626,.T.);
#90607=ADVANCED_FACE('',(#11328),#3627,.T.);
#90608=ADVANCED_FACE('',(#11329),#3628,.T.);
#90609=ADVANCED_FACE('',(#11330),#3629,.T.);
#90610=ADVANCED_FACE('',(#11331),#3630,.T.);
#90611=ADVANCED_FACE('',(#11332),#86626,.T.);
#90612=ADVANCED_FACE('',(#11333),#86627,.T.);
#90613=ADVANCED_FACE('',(#11334),#3631,.T.);
#90614=ADVANCED_FACE('',(#11335),#3632,.T.);
#90615=ADVANCED_FACE('',(#11336),#86628,.T.);
#90616=ADVANCED_FACE('',(#11337),#3633,.T.);
#90617=ADVANCED_FACE('',(#11338),#3634,.T.);
#90618=ADVANCED_FACE('',(#11339),#3635,.T.);
#90619=ADVANCED_FACE('',(#11340),#86629,.T.);
#90620=ADVANCED_FACE('',(#11341),#86630,.T.);
#90621=ADVANCED_FACE('',(#11342),#3636,.T.);
#90622=ADVANCED_FACE('',(#11343),#3637,.T.);
#90623=ADVANCED_FACE('',(#11344),#86631,.T.);
#90624=ADVANCED_FACE('',(#11345),#86632,.T.);
#90625=ADVANCED_FACE('',(#11346),#3638,.T.);
#90626=ADVANCED_FACE('',(#11347),#3639,.T.);
#90627=ADVANCED_FACE('',(#11348),#86633,.T.);
#90628=ADVANCED_FACE('',(#11349),#86634,.T.);
#90629=ADVANCED_FACE('',(#11350),#3640,.T.);
#90630=ADVANCED_FACE('',(#11351),#3641,.T.);
#90631=ADVANCED_FACE('',(#11352),#86635,.T.);
#90632=ADVANCED_FACE('',(#11353),#3642,.T.);
#90633=ADVANCED_FACE('',(#11354),#3643,.T.);
#90634=ADVANCED_FACE('',(#11355),#3644,.T.);
#90635=ADVANCED_FACE('',(#11356),#86636,.T.);
#90636=ADVANCED_FACE('',(#11357),#86637,.T.);
#90637=ADVANCED_FACE('',(#11358),#3645,.T.);
#90638=ADVANCED_FACE('',(#11359),#3646,.T.);
#90639=ADVANCED_FACE('',(#11360),#86638,.T.);
#90640=ADVANCED_FACE('',(#11361),#86639,.T.);
#90641=ADVANCED_FACE('',(#11362),#3647,.T.);
#90642=ADVANCED_FACE('',(#11363),#3648,.T.);
#90643=ADVANCED_FACE('',(#11364),#86640,.T.);
#90644=ADVANCED_FACE('',(#11365),#3649,.T.);
#90645=ADVANCED_FACE('',(#11366),#3650,.T.);
#90646=ADVANCED_FACE('',(#11367),#3651,.T.);
#90647=ADVANCED_FACE('',(#11368),#86641,.T.);
#90648=ADVANCED_FACE('',(#11369),#3652,.T.);
#90649=ADVANCED_FACE('',(#11370),#86642,.T.);
#90650=ADVANCED_FACE('',(#11371),#3653,.T.);
#90651=ADVANCED_FACE('',(#11372),#3654,.T.);
#90652=ADVANCED_FACE('',(#11373),#3655,.T.);
#90653=ADVANCED_FACE('',(#11374),#86643,.T.);
#90654=ADVANCED_FACE('',(#11375),#3656,.T.);
#90655=ADVANCED_FACE('',(#11376),#3657,.T.);
#90656=ADVANCED_FACE('',(#11377),#3658,.T.);
#90657=ADVANCED_FACE('',(#11378),#3659,.T.);
#90658=ADVANCED_FACE('',(#11379),#3660,.T.);
#90659=ADVANCED_FACE('',(#11380),#3661,.T.);
#90660=ADVANCED_FACE('',(#11381),#3662,.T.);
#90661=ADVANCED_FACE('',(#11382),#3663,.T.);
#90662=ADVANCED_FACE('',(#11383),#3664,.T.);
#90663=ADVANCED_FACE('',(#11384),#3665,.T.);
#90664=ADVANCED_FACE('',(#11385),#3666,.T.);
#90665=ADVANCED_FACE('',(#11386),#3667,.T.);
#90666=ADVANCED_FACE('',(#11387),#3668,.T.);
#90667=ADVANCED_FACE('',(#11388),#3669,.T.);
#90668=ADVANCED_FACE('',(#11389),#3670,.T.);
#90669=ADVANCED_FACE('',(#11390),#86644,.T.);
#90670=ADVANCED_FACE('',(#11391),#3671,.T.);
#90671=ADVANCED_FACE('',(#11392),#3672,.T.);
#90672=ADVANCED_FACE('',(#11393),#3673,.T.);
#90673=ADVANCED_FACE('',(#11394),#86645,.T.);
#90674=ADVANCED_FACE('',(#11395),#3674,.T.);
#90675=ADVANCED_FACE('',(#11396),#3675,.T.);
#90676=ADVANCED_FACE('',(#11397),#86646,.T.);
#90677=ADVANCED_FACE('',(#11398),#3676,.T.);
#90678=ADVANCED_FACE('',(#11399),#3677,.T.);
#90679=ADVANCED_FACE('',(#11400),#3678,.T.);
#90680=ADVANCED_FACE('',(#11401),#86647,.T.);
#90681=ADVANCED_FACE('',(#11402),#3679,.T.);
#90682=ADVANCED_FACE('',(#11403),#3680,.T.);
#90683=ADVANCED_FACE('',(#11404),#86648,.T.);
#90684=ADVANCED_FACE('',(#11405),#3681,.T.);
#90685=ADVANCED_FACE('',(#11406),#3682,.T.);
#90686=ADVANCED_FACE('',(#11407),#3683,.T.);
#90687=ADVANCED_FACE('',(#11408),#86649,.T.);
#90688=ADVANCED_FACE('',(#11409),#3684,.T.);
#90689=ADVANCED_FACE('',(#11410),#3685,.T.);
#90690=ADVANCED_FACE('',(#11411),#86650,.T.);
#90691=ADVANCED_FACE('',(#11412),#3686,.T.);
#90692=ADVANCED_FACE('',(#11413),#3687,.T.);
#90693=ADVANCED_FACE('',(#11414),#3688,.T.);
#90694=ADVANCED_FACE('',(#11415),#86651,.T.);
#90695=ADVANCED_FACE('',(#11416),#3689,.T.);
#90696=ADVANCED_FACE('',(#11417),#3690,.T.);
#90697=ADVANCED_FACE('',(#11418),#3691,.T.);
#90698=ADVANCED_FACE('',(#11419),#3692,.T.);
#90699=ADVANCED_FACE('',(#11420),#3693,.T.);
#90700=ADVANCED_FACE('',(#11421),#3694,.T.);
#90701=ADVANCED_FACE('',(#11422),#3695,.T.);
#90702=ADVANCED_FACE('',(#11423),#3696,.T.);
#90703=ADVANCED_FACE('',(#11424),#2974,.T.);
#90704=ADVANCED_FACE('',(#11425),#2975,.T.);
#90705=ADVANCED_FACE('',(#11426),#2976,.T.);
#90706=ADVANCED_FACE('',(#11427),#2977,.T.);
#90707=ADVANCED_FACE('',(#11428),#2978,.T.);
#90708=ADVANCED_FACE('',(#11429),#2979,.T.);
#90709=ADVANCED_FACE('',(#11430),#2980,.T.);
#90710=ADVANCED_FACE('',(#11431),#2981,.T.);
#90711=ADVANCED_FACE('',(#11432),#2982,.T.);
#90712=ADVANCED_FACE('',(#11433),#2983,.T.);
#90713=ADVANCED_FACE('',(#11434),#2984,.T.);
#90714=ADVANCED_FACE('',(#11435),#2985,.T.);
#90715=ADVANCED_FACE('',(#11436),#2986,.T.);
#90716=ADVANCED_FACE('',(#11437),#2987,.T.);
#90717=ADVANCED_FACE('',(#11438),#2988,.T.);
#90718=ADVANCED_FACE('',(#11439),#2989,.T.);
#90719=ADVANCED_FACE('',(#11440),#2990,.T.);
#90720=ADVANCED_FACE('',(#11441),#2991,.T.);
#90721=ADVANCED_FACE('',(#11442),#2992,.T.);
#90722=ADVANCED_FACE('',(#11443),#2993,.T.);
#90723=ADVANCED_FACE('',(#11444),#2994,.T.);
#90724=ADVANCED_FACE('',(#11445),#2995,.T.);
#90725=ADVANCED_FACE('',(#11446),#2996,.T.);
#90726=ADVANCED_FACE('',(#11447),#2997,.T.);
#90727=ADVANCED_FACE('',(#11448),#2998,.T.);
#90728=ADVANCED_FACE('',(#11449),#2999,.T.);
#90729=ADVANCED_FACE('',(#11450),#3000,.T.);
#90730=ADVANCED_FACE('',(#11451),#3001,.T.);
#90731=ADVANCED_FACE('',(#11452),#3002,.T.);
#90732=ADVANCED_FACE('',(#11453),#3003,.T.);
#90733=ADVANCED_FACE('',(#11454),#3004,.T.);
#90734=ADVANCED_FACE('',(#11455),#3005,.T.);
#90735=ADVANCED_FACE('',(#11456),#3006,.T.);
#90736=ADVANCED_FACE('',(#11457),#3007,.T.);
#90737=ADVANCED_FACE('',(#11458),#3008,.T.);
#90738=ADVANCED_FACE('',(#11459),#3009,.T.);
#90739=ADVANCED_FACE('',(#11460),#3010,.T.);
#90740=ADVANCED_FACE('',(#11461),#3011,.T.);
#90741=ADVANCED_FACE('',(#11462),#3697,.T.);
#90742=ADVANCED_FACE('',(#11463),#3012,.T.);
#90743=ADVANCED_FACE('',(#11464),#3013,.T.);
#90744=ADVANCED_FACE('',(#11465),#3014,.T.);
#90745=ADVANCED_FACE('',(#11466),#3015,.T.);
#90746=ADVANCED_FACE('',(#11467),#3016,.T.);
#90747=ADVANCED_FACE('',(#11468),#3017,.T.);
#90748=ADVANCED_FACE('',(#11469),#3018,.T.);
#90749=ADVANCED_FACE('',(#11470),#3019,.T.);
#90750=ADVANCED_FACE('',(#11471),#3020,.T.);
#90751=ADVANCED_FACE('',(#11472),#3021,.T.);
#90752=ADVANCED_FACE('',(#11473),#3022,.T.);
#90753=ADVANCED_FACE('',(#11474),#3023,.T.);
#90754=ADVANCED_FACE('',(#11475),#86652,.F.);
#90755=ADVANCED_FACE('',(#11476),#86653,.F.);
#90756=ADVANCED_FACE('',(#11477),#86654,.F.);
#90757=ADVANCED_FACE('',(#11478),#86655,.F.);
#90758=ADVANCED_FACE('',(#11479),#86656,.F.);
#90759=ADVANCED_FACE('',(#11480),#86657,.F.);
#90760=ADVANCED_FACE('',(#11481),#86658,.F.);
#90761=ADVANCED_FACE('',(#11482),#86659,.F.);
#90762=ADVANCED_FACE('',(#11483),#86660,.F.);
#90763=ADVANCED_FACE('',(#11484),#86661,.F.);
#90764=ADVANCED_FACE('',(#11485),#86662,.F.);
#90765=ADVANCED_FACE('',(#11486),#86663,.F.);
#90766=ADVANCED_FACE('',(#11487),#86664,.F.);
#90767=ADVANCED_FACE('',(#11488),#86665,.F.);
#90768=ADVANCED_FACE('',(#11489),#86666,.F.);
#90769=ADVANCED_FACE('',(#11490),#86667,.F.);
#90770=ADVANCED_FACE('',(#11491),#86668,.F.);
#90771=ADVANCED_FACE('',(#11492),#86669,.F.);
#90772=ADVANCED_FACE('',(#11493),#86670,.F.);
#90773=ADVANCED_FACE('',(#11494),#86671,.F.);
#90774=ADVANCED_FACE('',(#11495),#86672,.F.);
#90775=ADVANCED_FACE('',(#11496),#86673,.F.);
#90776=ADVANCED_FACE('',(#11497),#86674,.F.);
#90777=ADVANCED_FACE('',(#11498),#86675,.F.);
#90778=ADVANCED_FACE('',(#11499),#86676,.F.);
#90779=ADVANCED_FACE('',(#11500),#86677,.F.);
#90780=ADVANCED_FACE('',(#11501),#86678,.F.);
#90781=ADVANCED_FACE('',(#11502),#86679,.F.);
#90782=ADVANCED_FACE('',(#11503),#86680,.F.);
#90783=ADVANCED_FACE('',(#11504),#86681,.F.);
#90784=ADVANCED_FACE('',(#11505),#86682,.F.);
#90785=ADVANCED_FACE('',(#11506),#86683,.F.);
#90786=ADVANCED_FACE('',(#11507),#86684,.F.);
#90787=ADVANCED_FACE('',(#11508),#86685,.F.);
#90788=ADVANCED_FACE('',(#11509),#86686,.F.);
#90789=ADVANCED_FACE('',(#11510),#86687,.F.);
#90790=ADVANCED_FACE('',(#11511),#86688,.F.);
#90791=ADVANCED_FACE('',(#11512),#86689,.F.);
#90792=ADVANCED_FACE('',(#11513),#86690,.F.);
#90793=ADVANCED_FACE('',(#11514),#86691,.F.);
#90794=ADVANCED_FACE('',(#11515),#86692,.F.);
#90795=ADVANCED_FACE('',(#11516),#86693,.F.);
#90796=ADVANCED_FACE('',(#11517),#86694,.F.);
#90797=ADVANCED_FACE('',(#11518),#86695,.F.);
#90798=ADVANCED_FACE('',(#11519),#86696,.F.);
#90799=ADVANCED_FACE('',(#11520),#86697,.F.);
#90800=ADVANCED_FACE('',(#11521),#86698,.F.);
#90801=ADVANCED_FACE('',(#11522),#86699,.F.);
#90802=ADVANCED_FACE('',(#11523),#86700,.F.);
#90803=ADVANCED_FACE('',(#11524),#86701,.F.);
#90804=ADVANCED_FACE('',(#11525),#86702,.F.);
#90805=ADVANCED_FACE('',(#11526),#86703,.F.);
#90806=ADVANCED_FACE('',(#11527),#86704,.F.);
#90807=ADVANCED_FACE('',(#11528),#86705,.F.);
#90808=ADVANCED_FACE('',(#11529),#86706,.F.);
#90809=ADVANCED_FACE('',(#11530),#86707,.F.);
#90810=ADVANCED_FACE('',(#11531),#86708,.F.);
#90811=ADVANCED_FACE('',(#11532),#86709,.F.);
#90812=ADVANCED_FACE('',(#11533),#86710,.F.);
#90813=ADVANCED_FACE('',(#11534),#86711,.F.);
#90814=ADVANCED_FACE('',(#11535),#86712,.F.);
#90815=ADVANCED_FACE('',(#11536),#86713,.F.);
#90816=ADVANCED_FACE('',(#11537),#86714,.F.);
#90817=ADVANCED_FACE('',(#11538),#86715,.F.);
#90818=ADVANCED_FACE('',(#11539),#86716,.F.);
#90819=ADVANCED_FACE('',(#11540),#86717,.F.);
#90820=ADVANCED_FACE('',(#11541),#86718,.F.);
#90821=ADVANCED_FACE('',(#11542),#86719,.F.);
#90822=ADVANCED_FACE('',(#11543),#86720,.F.);
#90823=ADVANCED_FACE('',(#11544),#86721,.F.);
#90824=ADVANCED_FACE('',(#11545),#86722,.F.);
#90825=ADVANCED_FACE('',(#11546),#86723,.F.);
#90826=ADVANCED_FACE('',(#11547),#86724,.F.);
#90827=ADVANCED_FACE('',(#11548),#86725,.F.);
#90828=ADVANCED_FACE('',(#11549),#86726,.F.);
#90829=ADVANCED_FACE('',(#11550),#86727,.F.);
#90830=ADVANCED_FACE('',(#11551),#86728,.F.);
#90831=ADVANCED_FACE('',(#11552),#86729,.F.);
#90832=ADVANCED_FACE('',(#11553),#86730,.F.);
#90833=ADVANCED_FACE('',(#11554),#86731,.F.);
#90834=ADVANCED_FACE('',(#11555),#86732,.F.);
#90835=ADVANCED_FACE('',(#11556),#86733,.F.);
#90836=ADVANCED_FACE('',(#11557),#86734,.F.);
#90837=ADVANCED_FACE('',(#11558),#86735,.F.);
#90838=ADVANCED_FACE('',(#11559),#86736,.F.);
#90839=ADVANCED_FACE('',(#11560),#86737,.F.);
#90840=ADVANCED_FACE('',(#11561),#86738,.F.);
#90841=ADVANCED_FACE('',(#11562),#86739,.F.);
#90842=ADVANCED_FACE('',(#11563),#86740,.F.);
#90843=ADVANCED_FACE('',(#11564),#86741,.F.);
#90844=ADVANCED_FACE('',(#11565),#86742,.F.);
#90845=ADVANCED_FACE('',(#11566),#86743,.F.);
#90846=ADVANCED_FACE('',(#11567),#86744,.F.);
#90847=ADVANCED_FACE('',(#11568),#86745,.F.);
#90848=ADVANCED_FACE('',(#11569),#86746,.F.);
#90849=ADVANCED_FACE('',(#11570),#86747,.F.);
#90850=ADVANCED_FACE('',(#11571),#86748,.F.);
#90851=ADVANCED_FACE('',(#11572),#86749,.F.);
#90852=ADVANCED_FACE('',(#11573),#86750,.F.);
#90853=ADVANCED_FACE('',(#11574),#86751,.F.);
#90854=ADVANCED_FACE('',(#11575),#86752,.F.);
#90855=ADVANCED_FACE('',(#11576),#86753,.F.);
#90856=ADVANCED_FACE('',(#11577),#86754,.F.);
#90857=ADVANCED_FACE('',(#11578),#86755,.F.);
#90858=ADVANCED_FACE('',(#11579),#86756,.F.);
#90859=ADVANCED_FACE('',(#11580),#86757,.F.);
#90860=ADVANCED_FACE('',(#11581),#86758,.F.);
#90861=ADVANCED_FACE('',(#11582),#86759,.F.);
#90862=ADVANCED_FACE('',(#11583),#86760,.F.);
#90863=ADVANCED_FACE('',(#11584),#86761,.F.);
#90864=ADVANCED_FACE('',(#11585),#86762,.F.);
#90865=ADVANCED_FACE('',(#11586),#86763,.F.);
#90866=ADVANCED_FACE('',(#11587),#86764,.F.);
#90867=ADVANCED_FACE('',(#11588),#86765,.F.);
#90868=ADVANCED_FACE('',(#11589),#86766,.F.);
#90869=ADVANCED_FACE('',(#11590),#86767,.F.);
#90870=ADVANCED_FACE('',(#11591),#86768,.F.);
#90871=ADVANCED_FACE('',(#11592),#86769,.F.);
#90872=ADVANCED_FACE('',(#11593),#86770,.F.);
#90873=ADVANCED_FACE('',(#11594),#86771,.F.);
#90874=ADVANCED_FACE('',(#11595),#86772,.F.);
#90875=ADVANCED_FACE('',(#11596),#86773,.F.);
#90876=ADVANCED_FACE('',(#11597),#86774,.F.);
#90877=ADVANCED_FACE('',(#11598),#86775,.F.);
#90878=ADVANCED_FACE('',(#11599),#86776,.F.);
#90879=ADVANCED_FACE('',(#11600),#86777,.F.);
#90880=ADVANCED_FACE('',(#11601),#86778,.F.);
#90881=ADVANCED_FACE('',(#11602),#86779,.F.);
#90882=ADVANCED_FACE('',(#11603),#86780,.F.);
#90883=ADVANCED_FACE('',(#11604),#86781,.F.);
#90884=ADVANCED_FACE('',(#11605),#86782,.F.);
#90885=ADVANCED_FACE('',(#11606),#86783,.F.);
#90886=ADVANCED_FACE('',(#11607),#86784,.F.);
#90887=ADVANCED_FACE('',(#11608),#86785,.F.);
#90888=ADVANCED_FACE('',(#11609),#86786,.F.);
#90889=ADVANCED_FACE('',(#11610),#86787,.F.);
#90890=ADVANCED_FACE('',(#11611),#86788,.F.);
#90891=ADVANCED_FACE('',(#11612),#86789,.F.);
#90892=ADVANCED_FACE('',(#11613),#86790,.T.);
#90893=ADVANCED_FACE('',(#11614),#86791,.T.);
#90894=ADVANCED_FACE('',(#11615),#86792,.F.);
#90895=ADVANCED_FACE('',(#11616),#8033,.F.);
#90896=ADVANCED_FACE('',(#11617),#8034,.F.);
#90897=ADVANCED_FACE('',(#11618),#86793,.F.);
#90898=ADVANCED_FACE('',(#11619),#86794,.T.);
#90899=ADVANCED_FACE('',(#11620),#86795,.F.);
#90900=ADVANCED_FACE('',(#11621),#8035,.T.);
#90901=ADVANCED_FACE('',(#11622),#8036,.T.);
#90902=ADVANCED_FACE('',(#11623),#86796,.F.);
#90903=ADVANCED_FACE('',(#11624),#86797,.T.);
#90904=ADVANCED_FACE('',(#11625),#8037,.F.);
#90905=ADVANCED_FACE('',(#11626),#8038,.F.);
#90906=ADVANCED_FACE('',(#11627),#8039,.F.);
#90907=ADVANCED_FACE('',(#11628),#8040,.F.);
#90908=ADVANCED_FACE('',(#11629),#8041,.F.);
#90909=ADVANCED_FACE('',(#11630),#8042,.F.);
#90910=ADVANCED_FACE('',(#11631),#8043,.F.);
#90911=ADVANCED_FACE('',(#11632),#8044,.F.);
#90912=ADVANCED_FACE('',(#11633),#8045,.F.);
#90913=ADVANCED_FACE('',(#11634),#8046,.F.);
#90914=ADVANCED_FACE('',(#11635),#8047,.F.);
#90915=ADVANCED_FACE('',(#11636),#8048,.F.);
#90916=ADVANCED_FACE('',(#11637),#8049,.F.);
#90917=ADVANCED_FACE('',(#11638),#8050,.F.);
#90918=ADVANCED_FACE('',(#11639),#8051,.F.);
#90919=ADVANCED_FACE('',(#11640),#8052,.F.);
#90920=ADVANCED_FACE('',(#11641),#8053,.F.);
#90921=ADVANCED_FACE('',(#11642),#8054,.F.);
#90922=ADVANCED_FACE('',(#11643),#8055,.F.);
#90923=ADVANCED_FACE('',(#11644),#8056,.F.);
#90924=ADVANCED_FACE('',(#11645),#8057,.F.);
#90925=ADVANCED_FACE('',(#11646),#8058,.F.);
#90926=ADVANCED_FACE('',(#11647),#8059,.F.);
#90927=ADVANCED_FACE('',(#11648),#8060,.F.);
#90928=ADVANCED_FACE('',(#11649),#8061,.F.);
#90929=ADVANCED_FACE('',(#11650),#8062,.F.);
#90930=ADVANCED_FACE('',(#11651),#8063,.F.);
#90931=ADVANCED_FACE('',(#11652),#8064,.F.);
#90932=ADVANCED_FACE('',(#11653),#8065,.F.);
#90933=ADVANCED_FACE('',(#11654),#8066,.F.);
#90934=ADVANCED_FACE('',(#11655),#8067,.F.);
#90935=ADVANCED_FACE('',(#11656),#8068,.F.);
#90936=ADVANCED_FACE('',(#11657),#8069,.F.);
#90937=ADVANCED_FACE('',(#11658),#8070,.F.);
#90938=ADVANCED_FACE('',(#11659),#8071,.F.);
#90939=ADVANCED_FACE('',(#11660),#8072,.F.);
#90940=ADVANCED_FACE('',(#11661),#8073,.F.);
#90941=ADVANCED_FACE('',(#11662),#8074,.F.);
#90942=ADVANCED_FACE('',(#11663),#8075,.F.);
#90943=ADVANCED_FACE('',(#11664),#8076,.F.);
#90944=ADVANCED_FACE('',(#11665),#8077,.F.);
#90945=ADVANCED_FACE('',(#11666),#8078,.F.);
#90946=ADVANCED_FACE('',(#11667),#8079,.F.);
#90947=ADVANCED_FACE('',(#11668),#8080,.F.);
#90948=ADVANCED_FACE('',(#11669),#8081,.F.);
#90949=ADVANCED_FACE('',(#11670),#8082,.F.);
#90950=ADVANCED_FACE('',(#11671),#8083,.F.);
#90951=ADVANCED_FACE('',(#11672),#8084,.F.);
#90952=ADVANCED_FACE('',(#11673),#8085,.F.);
#90953=ADVANCED_FACE('',(#11674),#8086,.F.);
#90954=ADVANCED_FACE('',(#11675),#8087,.F.);
#90955=ADVANCED_FACE('',(#11676),#8088,.F.);
#90956=ADVANCED_FACE('',(#11677),#8089,.F.);
#90957=ADVANCED_FACE('',(#11678),#8090,.F.);
#90958=ADVANCED_FACE('',(#11679),#8091,.F.);
#90959=ADVANCED_FACE('',(#11680),#8092,.F.);
#90960=ADVANCED_FACE('',(#11681),#8093,.F.);
#90961=ADVANCED_FACE('',(#11682),#86798,.T.);
#90962=ADVANCED_FACE('',(#11683),#86799,.T.);
#90963=ADVANCED_FACE('',(#11684),#86800,.T.);
#90964=ADVANCED_FACE('',(#11685),#86801,.T.);
#90965=ADVANCED_FACE('',(#11686),#86802,.T.);
#90966=ADVANCED_FACE('',(#11687),#86803,.T.);
#90967=ADVANCED_FACE('',(#11688),#86804,.T.);
#90968=ADVANCED_FACE('',(#11689),#8094,.T.);
#90969=ADVANCED_FACE('',(#11690),#8095,.T.);
#90970=ADVANCED_FACE('',(#11691),#8096,.F.);
#90971=ADVANCED_FACE('',(#11692),#8097,.T.);
#90972=ADVANCED_FACE('',(#11693),#8098,.F.);
#90973=ADVANCED_FACE('',(#11694),#8099,.F.);
#90974=ADVANCED_FACE('',(#11695),#86805,.F.);
#90975=ADVANCED_FACE('',(#11696),#8100,.F.);
#90976=ADVANCED_FACE('',(#11697),#8101,.F.);
#90977=ADVANCED_FACE('',(#11698),#86806,.F.);
#90978=ADVANCED_FACE('',(#11699),#86807,.T.);
#90979=ADVANCED_FACE('',(#11700),#86808,.T.);
#90980=ADVANCED_FACE('',(#11701),#86809,.T.);
#90981=ADVANCED_FACE('',(#11702),#86810,.T.);
#90982=ADVANCED_FACE('',(#11703),#86811,.T.);
#90983=ADVANCED_FACE('',(#11704),#86812,.T.);
#90984=ADVANCED_FACE('',(#11705),#86813,.T.);
#90985=ADVANCED_FACE('',(#11706),#905,.F.);
#90986=ADVANCED_FACE('',(#11707),#906,.F.);
#90987=ADVANCED_FACE('',(#11708),#907,.F.);
#90988=ADVANCED_FACE('',(#11709),#908,.F.);
#90989=ADVANCED_FACE('',(#11710),#7008,.F.);
#90990=ADVANCED_FACE('',(#11711),#7009,.F.);
#90991=ADVANCED_FACE('',(#11712),#7010,.F.);
#90992=ADVANCED_FACE('',(#11713),#7011,.F.);
#90993=ADVANCED_FACE('',(#11714),#7012,.F.);
#90994=ADVANCED_FACE('',(#11715),#7013,.F.);
#90995=ADVANCED_FACE('',(#11716),#7014,.F.);
#90996=ADVANCED_FACE('',(#11717),#7015,.F.);
#90997=ADVANCED_FACE('',(#11718),#7016,.F.);
#90998=ADVANCED_FACE('',(#11719),#7017,.F.);
#90999=ADVANCED_FACE('',(#11720),#7018,.F.);
#91000=ADVANCED_FACE('',(#11721),#7019,.F.);
#91001=ADVANCED_FACE('',(#11722),#7020,.F.);
#91002=ADVANCED_FACE('',(#11723),#909,.F.);
#91003=ADVANCED_FACE('',(#11724),#910,.F.);
#91004=ADVANCED_FACE('',(#11725),#7021,.F.);
#91005=ADVANCED_FACE('',(#11726),#911,.F.);
#91006=ADVANCED_FACE('',(#11727),#8102,.F.);
#91007=ADVANCED_FACE('',(#11728),#912,.F.);
#91008=ADVANCED_FACE('',(#11729),#8103,.F.);
#91009=ADVANCED_FACE('',(#11730),#913,.F.);
#91010=ADVANCED_FACE('',(#11731),#8104,.T.);
#91011=ADVANCED_FACE('',(#11732),#914,.F.);
#91012=ADVANCED_FACE('',(#11733),#8105,.F.);
#91013=ADVANCED_FACE('',(#11734),#8106,.F.);
#91014=ADVANCED_FACE('',(#11735),#8107,.F.);
#91015=ADVANCED_FACE('',(#11736),#8108,.F.);
#91016=ADVANCED_FACE('',(#11737),#8109,.F.);
#91017=ADVANCED_FACE('',(#11738),#8110,.F.);
#91018=ADVANCED_FACE('',(#11739),#8111,.F.);
#91019=ADVANCED_FACE('',(#11740),#86814,.T.);
#91020=ADVANCED_FACE('',(#11741),#86815,.T.);
#91021=ADVANCED_FACE('',(#11742),#86816,.T.);
#91022=ADVANCED_FACE('',(#11743),#86817,.T.);
#91023=ADVANCED_FACE('',(#11744),#86818,.T.);
#91024=ADVANCED_FACE('',(#11745),#8112,.T.);
#91025=ADVANCED_FACE('',(#11746),#7022,.T.);
#91026=ADVANCED_FACE('',(#11747),#8113,.T.);
#91027=ADVANCED_FACE('',(#11748),#915,.F.);
#91028=ADVANCED_FACE('',(#11749),#7023,.T.);
#91029=ADVANCED_FACE('',(#11750),#86819,.F.);
#91030=ADVANCED_FACE('',(#11751),#86820,.F.);
#91031=ADVANCED_FACE('',(#11752),#86821,.F.);
#91032=ADVANCED_FACE('',(#11753),#86822,.F.);
#91033=ADVANCED_FACE('',(#11754),#86823,.F.);
#91034=ADVANCED_FACE('',(#11755),#86824,.F.);
#91035=ADVANCED_FACE('',(#11756),#86825,.F.);
#91036=ADVANCED_FACE('',(#11757),#8114,.T.);
#91037=ADVANCED_FACE('',(#11758),#7024,.F.);
#91038=ADVANCED_FACE('',(#11759),#8115,.T.);
#91039=ADVANCED_FACE('',(#11760),#7025,.F.);
#91040=ADVANCED_FACE('',(#11761,#7455),#8116,.F.);
#91041=ADVANCED_FACE('',(#11762),#8117,.F.);
#91042=ADVANCED_FACE('',(#11763),#8118,.F.);
#91043=ADVANCED_FACE('',(#11764),#86826,.T.);
#91044=ADVANCED_FACE('',(#11765),#8119,.T.);
#91045=ADVANCED_FACE('',(#11766),#8120,.F.);
#91046=ADVANCED_FACE('',(#11767),#8121,.F.);
#91047=ADVANCED_FACE('',(#11768),#86827,.T.);
#91048=ADVANCED_FACE('',(#11769),#8122,.T.);
#91049=ADVANCED_FACE('',(#11770),#8123,.T.);
#91050=ADVANCED_FACE('',(#11771),#86828,.T.);
#91051=ADVANCED_FACE('',(#11772),#8124,.T.);
#91052=ADVANCED_FACE('',(#11773),#8125,.T.);
#91053=ADVANCED_FACE('',(#11774),#86829,.T.);
#91054=ADVANCED_FACE('',(#11775),#916,.F.);
#91055=ADVANCED_FACE('',(#11776),#86830,.T.);
#91056=ADVANCED_FACE('',(#11777),#86831,.T.);
#91057=ADVANCED_FACE('',(#11778),#86832,.T.);
#91058=ADVANCED_FACE('',(#11779),#86833,.T.);
#91059=ADVANCED_FACE('',(#11780),#86834,.T.);
#91060=ADVANCED_FACE('',(#11781),#86835,.T.);
#91061=ADVANCED_FACE('',(#11782),#86836,.T.);
#91062=ADVANCED_FACE('',(#11783),#86837,.F.);
#91063=ADVANCED_FACE('',(#11784),#86838,.F.);
#91064=ADVANCED_FACE('',(#11785),#86839,.F.);
#91065=ADVANCED_FACE('',(#11786),#86840,.F.);
#91066=ADVANCED_FACE('',(#11787),#86841,.F.);
#91067=ADVANCED_FACE('',(#11788),#86842,.F.);
#91068=ADVANCED_FACE('',(#11789),#86843,.F.);
#91069=ADVANCED_FACE('',(#11790),#917,.F.);
#91070=ADVANCED_FACE('',(#11791),#918,.F.);
#91071=ADVANCED_FACE('',(#11792),#919,.F.);
#91072=ADVANCED_FACE('',(#11793),#920,.F.);
#91073=ADVANCED_FACE('',(#11794),#7026,.T.);
#91074=ADVANCED_FACE('',(#11795),#7027,.T.);
#91075=ADVANCED_FACE('',(#11796),#7028,.T.);
#91076=ADVANCED_FACE('',(#11797),#7029,.T.);
#91077=ADVANCED_FACE('',(#11798),#7030,.T.);
#91078=ADVANCED_FACE('',(#11799),#7031,.T.);
#91079=ADVANCED_FACE('',(#11800),#7032,.T.);
#91080=ADVANCED_FACE('',(#11801),#7033,.T.);
#91081=ADVANCED_FACE('',(#11802),#7034,.T.);
#91082=ADVANCED_FACE('',(#11803),#7035,.T.);
#91083=ADVANCED_FACE('',(#11804),#7036,.T.);
#91084=ADVANCED_FACE('',(#11805),#7037,.T.);
#91085=ADVANCED_FACE('',(#11806),#7038,.T.);
#91086=ADVANCED_FACE('',(#11807),#921,.F.);
#91087=ADVANCED_FACE('',(#11808),#922,.F.);
#91088=ADVANCED_FACE('',(#11809),#7039,.T.);
#91089=ADVANCED_FACE('',(#11810),#923,.F.);
#91090=ADVANCED_FACE('',(#11811),#924,.F.);
#91091=ADVANCED_FACE('',(#11812),#8126,.T.);
#91092=ADVANCED_FACE('',(#11813),#925,.F.);
#91093=ADVANCED_FACE('',(#11814),#8127,.F.);
#91094=ADVANCED_FACE('',(#11815),#926,.F.);
#91095=ADVANCED_FACE('',(#11816),#86844,.F.);
#91096=ADVANCED_FACE('',(#11817),#86845,.F.);
#91097=ADVANCED_FACE('',(#11818),#86846,.F.);
#91098=ADVANCED_FACE('',(#11819),#86847,.F.);
#91099=ADVANCED_FACE('',(#11820),#86848,.F.);
#91100=ADVANCED_FACE('',(#11821),#8128,.T.);
#91101=ADVANCED_FACE('',(#11822),#8129,.T.);
#91102=ADVANCED_FACE('',(#11823),#8130,.T.);
#91103=ADVANCED_FACE('',(#11824),#8131,.T.);
#91104=ADVANCED_FACE('',(#11825),#8132,.T.);
#91105=ADVANCED_FACE('',(#11826),#8133,.T.);
#91106=ADVANCED_FACE('',(#11827),#8134,.T.);
#91107=ADVANCED_FACE('',(#11828),#8135,.T.);
#91108=ADVANCED_FACE('',(#11829),#8136,.T.);
#91109=ADVANCED_FACE('',(#11830),#8137,.T.);
#91110=ADVANCED_FACE('',(#11831),#86849,.F.);
#91111=ADVANCED_FACE('',(#11832),#86850,.F.);
#91112=ADVANCED_FACE('',(#11833),#86851,.T.);
#91113=ADVANCED_FACE('',(#11834),#8138,.T.);
#91114=ADVANCED_FACE('',(#11835),#8139,.T.);
#91115=ADVANCED_FACE('',(#11836),#8140,.T.);
#91116=ADVANCED_FACE('',(#11837),#8141,.T.);
#91117=ADVANCED_FACE('',(#11838),#8142,.T.);
#91118=ADVANCED_FACE('',(#11839),#8143,.T.);
#91119=ADVANCED_FACE('',(#11840),#8144,.T.);
#91120=ADVANCED_FACE('',(#11841),#8145,.T.);
#91121=ADVANCED_FACE('',(#11842),#8146,.T.);
#91122=ADVANCED_FACE('',(#11843),#8147,.T.);
#91123=ADVANCED_FACE('',(#11844),#8148,.T.);
#91124=ADVANCED_FACE('',(#11845),#8149,.T.);
#91125=ADVANCED_FACE('',(#11846),#8150,.T.);
#91126=ADVANCED_FACE('',(#11847),#8151,.T.);
#91127=ADVANCED_FACE('',(#11848),#86852,.F.);
#91128=ADVANCED_FACE('',(#11849),#86853,.F.);
#91129=ADVANCED_FACE('',(#11850),#86854,.F.);
#91130=ADVANCED_FACE('',(#11851),#86855,.F.);
#91131=ADVANCED_FACE('',(#11852),#86856,.F.);
#91132=ADVANCED_FACE('',(#11853),#86857,.F.);
#91133=ADVANCED_FACE('',(#11854),#86858,.F.);
#91134=ADVANCED_FACE('',(#11855),#86859,.F.);
#91135=ADVANCED_FACE('',(#11856),#8152,.T.);
#91136=ADVANCED_FACE('',(#11857),#8153,.T.);
#91137=ADVANCED_FACE('',(#11858),#8154,.T.);
#91138=ADVANCED_FACE('',(#11859),#8155,.T.);
#91139=ADVANCED_FACE('',(#11860),#8156,.T.);
#91140=ADVANCED_FACE('',(#11861),#8157,.T.);
#91141=ADVANCED_FACE('',(#11862),#8158,.T.);
#91142=ADVANCED_FACE('',(#11863),#8159,.T.);
#91143=ADVANCED_FACE('',(#11864),#8160,.T.);
#91144=ADVANCED_FACE('',(#11865),#8161,.T.);
#91145=ADVANCED_FACE('',(#11866),#8162,.T.);
#91146=ADVANCED_FACE('',(#11867),#8163,.T.);
#91147=ADVANCED_FACE('',(#11868),#8164,.T.);
#91148=ADVANCED_FACE('',(#11869),#8165,.T.);
#91149=ADVANCED_FACE('',(#11870),#8166,.T.);
#91150=ADVANCED_FACE('',(#11871),#8167,.T.);
#91151=ADVANCED_FACE('',(#11872),#8168,.T.);
#91152=ADVANCED_FACE('',(#11873),#8169,.T.);
#91153=ADVANCED_FACE('',(#11874),#8170,.T.);
#91154=ADVANCED_FACE('',(#11875),#8171,.T.);
#91155=ADVANCED_FACE('',(#11876),#8172,.T.);
#91156=ADVANCED_FACE('',(#11877),#8173,.T.);
#91157=ADVANCED_FACE('',(#11878),#8174,.T.);
#91158=ADVANCED_FACE('',(#11879),#8175,.T.);
#91159=ADVANCED_FACE('',(#11880),#8176,.T.);
#91160=ADVANCED_FACE('',(#11881),#8177,.T.);
#91161=ADVANCED_FACE('',(#11882),#8178,.T.);
#91162=ADVANCED_FACE('',(#11883),#8179,.T.);
#91163=ADVANCED_FACE('',(#11884),#3024,.T.);
#91164=ADVANCED_FACE('',(#11885),#3698,.T.);
#91165=ADVANCED_FACE('',(#11886),#3699,.T.);
#91166=ADVANCED_FACE('',(#11887),#3025,.F.);
#91167=ADVANCED_FACE('',(#11888),#3026,.F.);
#91168=ADVANCED_FACE('',(#11889),#1022,.F.);
#91169=ADVANCED_FACE('',(#11890),#3027,.F.);
#91170=ADVANCED_FACE('',(#11891),#3700,.F.);
#91171=ADVANCED_FACE('',(#11892),#3028,.F.);
#91172=ADVANCED_FACE('',(#11893),#3701,.F.);
#91173=ADVANCED_FACE('',(#11894),#3029,.F.);
#91174=ADVANCED_FACE('',(#11895),#3702,.F.);
#91175=ADVANCED_FACE('',(#11896),#3030,.F.);
#91176=ADVANCED_FACE('',(#11897),#3031,.F.);
#91177=ADVANCED_FACE('',(#11898),#3032,.F.);
#91178=ADVANCED_FACE('',(#11899),#1023,.F.);
#91179=ADVANCED_FACE('',(#11900),#3033,.F.);
#91180=ADVANCED_FACE('',(#11901),#3034,.F.);
#91181=ADVANCED_FACE('',(#11902),#3035,.F.);
#91182=ADVANCED_FACE('',(#11903),#3036,.F.);
#91183=ADVANCED_FACE('',(#11904),#3037,.F.);
#91184=ADVANCED_FACE('',(#11905),#1024,.F.);
#91185=ADVANCED_FACE('',(#11906),#3038,.F.);
#91186=ADVANCED_FACE('',(#11907),#3039,.F.);
#91187=ADVANCED_FACE('',(#11908),#3040,.F.);
#91188=ADVANCED_FACE('',(#11909),#3703,.F.);
#91189=ADVANCED_FACE('',(#11910),#1025,.F.);
#91190=ADVANCED_FACE('',(#11911),#3704,.F.);
#91191=ADVANCED_FACE('',(#11912),#3041,.F.);
#91192=ADVANCED_FACE('',(#11913),#3705,.F.);
#91193=ADVANCED_FACE('',(#11914),#3706,.F.);
#91194=ADVANCED_FACE('',(#11915),#3707,.F.);
#91195=ADVANCED_FACE('',(#11916),#3708,.F.);
#91196=ADVANCED_FACE('',(#11917),#3709,.F.);
#91197=ADVANCED_FACE('',(#11918),#3710,.F.);
#91198=ADVANCED_FACE('',(#11919),#3711,.F.);
#91199=ADVANCED_FACE('',(#11920),#3712,.F.);
#91200=ADVANCED_FACE('',(#11921),#3713,.F.);
#91201=ADVANCED_FACE('',(#11922),#3714,.F.);
#91202=ADVANCED_FACE('',(#11923),#3042,.F.);
#91203=ADVANCED_FACE('',(#11924),#3043,.F.);
#91204=ADVANCED_FACE('',(#11925),#3044,.F.);
#91205=ADVANCED_FACE('',(#11926),#3045,.F.);
#91206=ADVANCED_FACE('',(#11927),#3046,.F.);
#91207=ADVANCED_FACE('',(#11928),#3047,.F.);
#91208=ADVANCED_FACE('',(#11929),#3048,.F.);
#91209=ADVANCED_FACE('',(#11930),#3049,.F.);
#91210=ADVANCED_FACE('',(#11931),#3050,.F.);
#91211=ADVANCED_FACE('',(#11932),#3051,.F.);
#91212=ADVANCED_FACE('',(#11933),#3052,.F.);
#91213=ADVANCED_FACE('',(#11934),#3053,.F.);
#91214=ADVANCED_FACE('',(#11935),#3715,.F.);
#91215=ADVANCED_FACE('',(#11936),#3054,.F.);
#91216=ADVANCED_FACE('',(#11937),#3716,.F.);
#91217=ADVANCED_FACE('',(#11938),#3055,.F.);
#91218=ADVANCED_FACE('',(#11939),#3056,.F.);
#91219=ADVANCED_FACE('',(#11940),#3057,.F.);
#91220=ADVANCED_FACE('',(#11941),#3058,.F.);
#91221=ADVANCED_FACE('',(#11942),#3059,.F.);
#91222=ADVANCED_FACE('',(#11943),#3060,.F.);
#91223=ADVANCED_FACE('',(#11944),#3061,.F.);
#91224=ADVANCED_FACE('',(#11945),#3062,.F.);
#91225=ADVANCED_FACE('',(#11946),#3063,.F.);
#91226=ADVANCED_FACE('',(#11947),#86860,.T.);
#91227=ADVANCED_FACE('',(#11948),#3064,.F.);
#91228=ADVANCED_FACE('',(#11949),#3717,.T.);
#91229=ADVANCED_FACE('',(#11950),#3065,.F.);
#91230=ADVANCED_FACE('',(#11951),#86861,.T.);
#91231=ADVANCED_FACE('',(#11952),#86862,.T.);
#91232=ADVANCED_FACE('',(#11953),#3066,.F.);
#91233=ADVANCED_FACE('',(#11954),#3718,.T.);
#91234=ADVANCED_FACE('',(#11955),#3067,.F.);
#91235=ADVANCED_FACE('',(#11956),#86863,.T.);
#91236=ADVANCED_FACE('',(#11957),#86864,.T.);
#91237=ADVANCED_FACE('',(#11958),#3068,.F.);
#91238=ADVANCED_FACE('',(#11959),#3719,.T.);
#91239=ADVANCED_FACE('',(#11960),#3069,.F.);
#91240=ADVANCED_FACE('',(#11961),#86865,.T.);
#91241=ADVANCED_FACE('',(#11962),#86866,.T.);
#91242=ADVANCED_FACE('',(#11963),#3070,.F.);
#91243=ADVANCED_FACE('',(#11964),#3720,.T.);
#91244=ADVANCED_FACE('',(#11965),#3071,.F.);
#91245=ADVANCED_FACE('',(#11966),#86867,.T.);
#91246=ADVANCED_FACE('',(#11967),#86868,.T.);
#91247=ADVANCED_FACE('',(#11968),#86869,.T.);
#91248=ADVANCED_FACE('',(#11969),#86870,.T.);
#91249=ADVANCED_FACE('',(#11970),#86871,.T.);
#91250=ADVANCED_FACE('',(#11971),#86872,.T.);
#91251=ADVANCED_FACE('',(#11972),#86873,.T.);
#91252=ADVANCED_FACE('',(#11973),#86874,.T.);
#91253=ADVANCED_FACE('',(#11974),#86875,.T.);
#91254=ADVANCED_FACE('',(#11975),#3721,.T.);
#91255=ADVANCED_FACE('',(#11976),#86876,.T.);
#91256=ADVANCED_FACE('',(#11977),#3722,.T.);
#91257=ADVANCED_FACE('',(#11978),#3723,.T.);
#91258=ADVANCED_FACE('',(#11979),#3724,.T.);
#91259=ADVANCED_FACE('',(#11980),#86877,.T.);
#91260=ADVANCED_FACE('',(#11981),#3725,.T.);
#91261=ADVANCED_FACE('',(#11982),#3726,.T.);
#91262=ADVANCED_FACE('',(#11983),#3727,.T.);
#91263=ADVANCED_FACE('',(#11984),#86878,.T.);
#91264=ADVANCED_FACE('',(#11985),#3728,.T.);
#91265=ADVANCED_FACE('',(#11986),#86879,.T.);
#91266=ADVANCED_FACE('',(#11987),#3729,.T.);
#91267=ADVANCED_FACE('',(#11988),#3730,.T.);
#91268=ADVANCED_FACE('',(#11989),#3731,.T.);
#91269=ADVANCED_FACE('',(#11990),#86880,.T.);
#91270=ADVANCED_FACE('',(#11991),#86881,.T.);
#91271=ADVANCED_FACE('',(#11992),#3732,.T.);
#91272=ADVANCED_FACE('',(#11993),#3733,.T.);
#91273=ADVANCED_FACE('',(#11994),#86882,.T.);
#91274=ADVANCED_FACE('',(#11995),#3734,.T.);
#91275=ADVANCED_FACE('',(#11996),#3735,.T.);
#91276=ADVANCED_FACE('',(#11997),#3736,.T.);
#91277=ADVANCED_FACE('',(#11998),#86883,.T.);
#91278=ADVANCED_FACE('',(#11999),#86884,.T.);
#91279=ADVANCED_FACE('',(#12000),#3737,.T.);
#91280=ADVANCED_FACE('',(#12001),#3738,.T.);
#91281=ADVANCED_FACE('',(#12002),#86885,.T.);
#91282=ADVANCED_FACE('',(#12003),#86886,.T.);
#91283=ADVANCED_FACE('',(#12004),#3739,.T.);
#91284=ADVANCED_FACE('',(#12005),#3740,.T.);
#91285=ADVANCED_FACE('',(#12006),#86887,.T.);
#91286=ADVANCED_FACE('',(#12007),#86888,.T.);
#91287=ADVANCED_FACE('',(#12008),#3741,.T.);
#91288=ADVANCED_FACE('',(#12009),#3742,.T.);
#91289=ADVANCED_FACE('',(#12010),#86889,.T.);
#91290=ADVANCED_FACE('',(#12011),#86890,.T.);
#91291=ADVANCED_FACE('',(#12012),#3743,.T.);
#91292=ADVANCED_FACE('',(#12013),#3744,.T.);
#91293=ADVANCED_FACE('',(#12014),#3745,.T.);
#91294=ADVANCED_FACE('',(#12015),#86891,.T.);
#91295=ADVANCED_FACE('',(#12016),#3746,.T.);
#91296=ADVANCED_FACE('',(#12017),#3747,.T.);
#91297=ADVANCED_FACE('',(#12018),#3748,.T.);
#91298=ADVANCED_FACE('',(#12019),#86892,.T.);
#91299=ADVANCED_FACE('',(#12020),#86893,.T.);
#91300=ADVANCED_FACE('',(#12021),#3749,.T.);
#91301=ADVANCED_FACE('',(#12022),#3750,.T.);
#91302=ADVANCED_FACE('',(#12023),#86894,.T.);
#91303=ADVANCED_FACE('',(#12024),#86895,.T.);
#91304=ADVANCED_FACE('',(#12025),#3751,.T.);
#91305=ADVANCED_FACE('',(#12026),#3752,.T.);
#91306=ADVANCED_FACE('',(#12027),#86896,.T.);
#91307=ADVANCED_FACE('',(#12028),#86897,.T.);
#91308=ADVANCED_FACE('',(#12029),#3753,.T.);
#91309=ADVANCED_FACE('',(#12030),#3754,.T.);
#91310=ADVANCED_FACE('',(#12031),#86898,.T.);
#91311=ADVANCED_FACE('',(#12032),#86899,.T.);
#91312=ADVANCED_FACE('',(#12033),#3755,.T.);
#91313=ADVANCED_FACE('',(#12034),#3756,.T.);
#91314=ADVANCED_FACE('',(#12035),#86900,.T.);
#91315=ADVANCED_FACE('',(#12036),#86901,.T.);
#91316=ADVANCED_FACE('',(#12037),#3757,.T.);
#91317=ADVANCED_FACE('',(#12038),#3758,.T.);
#91318=ADVANCED_FACE('',(#12039),#86902,.T.);
#91319=ADVANCED_FACE('',(#12040),#86903,.T.);
#91320=ADVANCED_FACE('',(#12041),#3759,.T.);
#91321=ADVANCED_FACE('',(#12042),#3760,.T.);
#91322=ADVANCED_FACE('',(#12043),#86904,.T.);
#91323=ADVANCED_FACE('',(#12044),#86905,.T.);
#91324=ADVANCED_FACE('',(#12045),#3761,.T.);
#91325=ADVANCED_FACE('',(#12046),#3762,.T.);
#91326=ADVANCED_FACE('',(#12047),#86906,.T.);
#91327=ADVANCED_FACE('',(#12048),#86907,.T.);
#91328=ADVANCED_FACE('',(#12049),#3763,.T.);
#91329=ADVANCED_FACE('',(#12050),#3764,.T.);
#91330=ADVANCED_FACE('',(#12051),#86908,.T.);
#91331=ADVANCED_FACE('',(#12052),#86909,.T.);
#91332=ADVANCED_FACE('',(#12053),#3765,.T.);
#91333=ADVANCED_FACE('',(#12054),#3766,.T.);
#91334=ADVANCED_FACE('',(#12055),#86910,.T.);
#91335=ADVANCED_FACE('',(#12056),#3767,.T.);
#91336=ADVANCED_FACE('',(#12057),#3768,.T.);
#91337=ADVANCED_FACE('',(#12058),#3769,.T.);
#91338=ADVANCED_FACE('',(#12059),#86911,.T.);
#91339=ADVANCED_FACE('',(#12060),#86912,.T.);
#91340=ADVANCED_FACE('',(#12061),#3770,.T.);
#91341=ADVANCED_FACE('',(#12062),#3771,.T.);
#91342=ADVANCED_FACE('',(#12063),#86913,.T.);
#91343=ADVANCED_FACE('',(#12064),#3772,.T.);
#91344=ADVANCED_FACE('',(#12065),#3773,.T.);
#91345=ADVANCED_FACE('',(#12066),#3774,.T.);
#91346=ADVANCED_FACE('',(#12067),#3775,.T.);
#91347=ADVANCED_FACE('',(#12068),#3776,.T.);
#91348=ADVANCED_FACE('',(#12069),#86914,.T.);
#91349=ADVANCED_FACE('',(#12070),#86915,.T.);
#91350=ADVANCED_FACE('',(#12071),#3777,.T.);
#91351=ADVANCED_FACE('',(#12072),#3778,.T.);
#91352=ADVANCED_FACE('',(#12073),#86916,.T.);
#91353=ADVANCED_FACE('',(#12074),#3779,.T.);
#91354=ADVANCED_FACE('',(#12075),#3780,.T.);
#91355=ADVANCED_FACE('',(#12076),#3781,.T.);
#91356=ADVANCED_FACE('',(#12077),#86917,.T.);
#91357=ADVANCED_FACE('',(#12078),#86918,.T.);
#91358=ADVANCED_FACE('',(#12079),#3782,.T.);
#91359=ADVANCED_FACE('',(#12080),#3783,.T.);
#91360=ADVANCED_FACE('',(#12081),#86919,.T.);
#91361=ADVANCED_FACE('',(#12082),#86920,.T.);
#91362=ADVANCED_FACE('',(#12083),#3784,.T.);
#91363=ADVANCED_FACE('',(#12084),#3785,.T.);
#91364=ADVANCED_FACE('',(#12085),#86921,.T.);
#91365=ADVANCED_FACE('',(#12086),#3786,.T.);
#91366=ADVANCED_FACE('',(#12087),#3787,.T.);
#91367=ADVANCED_FACE('',(#12088),#3788,.T.);
#91368=ADVANCED_FACE('',(#12089),#86922,.T.);
#91369=ADVANCED_FACE('',(#12090),#86923,.T.);
#91370=ADVANCED_FACE('',(#12091),#3789,.T.);
#91371=ADVANCED_FACE('',(#12092),#3790,.T.);
#91372=ADVANCED_FACE('',(#12093),#86924,.T.);
#91373=ADVANCED_FACE('',(#12094),#3791,.T.);
#91374=ADVANCED_FACE('',(#12095),#86925,.T.);
#91375=ADVANCED_FACE('',(#12096),#86926,.T.);
#91376=ADVANCED_FACE('',(#12097),#3792,.T.);
#91377=ADVANCED_FACE('',(#12098),#3793,.T.);
#91378=ADVANCED_FACE('',(#12099),#86927,.T.);
#91379=ADVANCED_FACE('',(#12100),#3794,.T.);
#91380=ADVANCED_FACE('',(#12101),#3795,.T.);
#91381=ADVANCED_FACE('',(#12102),#3796,.T.);
#91382=ADVANCED_FACE('',(#12103),#86928,.T.);
#91383=ADVANCED_FACE('',(#12104),#3797,.T.);
#91384=ADVANCED_FACE('',(#12105),#86929,.T.);
#91385=ADVANCED_FACE('',(#12106),#86930,.T.);
#91386=ADVANCED_FACE('',(#12107),#3798,.T.);
#91387=ADVANCED_FACE('',(#12108),#3799,.T.);
#91388=ADVANCED_FACE('',(#12109),#86931,.T.);
#91389=ADVANCED_FACE('',(#12110),#86932,.T.);
#91390=ADVANCED_FACE('',(#12111),#3800,.T.);
#91391=ADVANCED_FACE('',(#12112),#3801,.T.);
#91392=ADVANCED_FACE('',(#12113),#86933,.T.);
#91393=ADVANCED_FACE('',(#12114),#86934,.T.);
#91394=ADVANCED_FACE('',(#12115),#3802,.T.);
#91395=ADVANCED_FACE('',(#12116),#3803,.T.);
#91396=ADVANCED_FACE('',(#12117),#3804,.T.);
#91397=ADVANCED_FACE('',(#12118),#86935,.T.);
#91398=ADVANCED_FACE('',(#12119),#3805,.T.);
#91399=ADVANCED_FACE('',(#12120),#3806,.T.);
#91400=ADVANCED_FACE('',(#12121),#86936,.T.);
#91401=ADVANCED_FACE('',(#12122),#86937,.T.);
#91402=ADVANCED_FACE('',(#12123),#3807,.T.);
#91403=ADVANCED_FACE('',(#12124),#3808,.T.);
#91404=ADVANCED_FACE('',(#12125),#86938,.T.);
#91405=ADVANCED_FACE('',(#12126),#86939,.T.);
#91406=ADVANCED_FACE('',(#12127),#3809,.T.);
#91407=ADVANCED_FACE('',(#12128),#3810,.T.);
#91408=ADVANCED_FACE('',(#12129),#86940,.T.);
#91409=ADVANCED_FACE('',(#12130),#86941,.T.);
#91410=ADVANCED_FACE('',(#12131),#3811,.T.);
#91411=ADVANCED_FACE('',(#12132),#3812,.T.);
#91412=ADVANCED_FACE('',(#12133),#86942,.T.);
#91413=ADVANCED_FACE('',(#12134),#86943,.T.);
#91414=ADVANCED_FACE('',(#12135),#3813,.T.);
#91415=ADVANCED_FACE('',(#12136),#3814,.T.);
#91416=ADVANCED_FACE('',(#12137),#86944,.T.);
#91417=ADVANCED_FACE('',(#12138),#86945,.T.);
#91418=ADVANCED_FACE('',(#12139),#3815,.T.);
#91419=ADVANCED_FACE('',(#12140),#3816,.T.);
#91420=ADVANCED_FACE('',(#12141),#86946,.T.);
#91421=ADVANCED_FACE('',(#12142),#3817,.T.);
#91422=ADVANCED_FACE('',(#12143),#3818,.T.);
#91423=ADVANCED_FACE('',(#12144),#3819,.T.);
#91424=ADVANCED_FACE('',(#12145),#3820,.T.);
#91425=ADVANCED_FACE('',(#12146),#86947,.T.);
#91426=ADVANCED_FACE('',(#12147),#86948,.T.);
#91427=ADVANCED_FACE('',(#12148),#3821,.T.);
#91428=ADVANCED_FACE('',(#12149),#3822,.T.);
#91429=ADVANCED_FACE('',(#12150),#3823,.T.);
#91430=ADVANCED_FACE('',(#12151),#86949,.T.);
#91431=ADVANCED_FACE('',(#12152),#3824,.T.);
#91432=ADVANCED_FACE('',(#12153),#3825,.T.);
#91433=ADVANCED_FACE('',(#12154),#86950,.T.);
#91434=ADVANCED_FACE('',(#12155),#86951,.T.);
#91435=ADVANCED_FACE('',(#12156),#3826,.T.);
#91436=ADVANCED_FACE('',(#12157),#3827,.T.);
#91437=ADVANCED_FACE('',(#12158),#3828,.T.);
#91438=ADVANCED_FACE('',(#12159),#86952,.T.);
#91439=ADVANCED_FACE('',(#12160),#3829,.T.);
#91440=ADVANCED_FACE('',(#12161),#3830,.T.);
#91441=ADVANCED_FACE('',(#12162),#3831,.T.);
#91442=ADVANCED_FACE('',(#12163),#3832,.T.);
#91443=ADVANCED_FACE('',(#12164),#86953,.T.);
#91444=ADVANCED_FACE('',(#12165),#86954,.T.);
#91445=ADVANCED_FACE('',(#12166),#3833,.T.);
#91446=ADVANCED_FACE('',(#12167),#3834,.T.);
#91447=ADVANCED_FACE('',(#12168),#86955,.T.);
#91448=ADVANCED_FACE('',(#12169),#86956,.T.);
#91449=ADVANCED_FACE('',(#12170),#3835,.T.);
#91450=ADVANCED_FACE('',(#12171),#3836,.T.);
#91451=ADVANCED_FACE('',(#12172),#86957,.T.);
#91452=ADVANCED_FACE('',(#12173),#86958,.T.);
#91453=ADVANCED_FACE('',(#12174),#3837,.T.);
#91454=ADVANCED_FACE('',(#12175),#3838,.T.);
#91455=ADVANCED_FACE('',(#12176),#86959,.T.);
#91456=ADVANCED_FACE('',(#12177),#3839,.T.);
#91457=ADVANCED_FACE('',(#12178),#3840,.T.);
#91458=ADVANCED_FACE('',(#12179),#3841,.T.);
#91459=ADVANCED_FACE('',(#12180),#3842,.T.);
#91460=ADVANCED_FACE('',(#12181),#3843,.T.);
#91461=ADVANCED_FACE('',(#12182),#86960,.T.);
#91462=ADVANCED_FACE('',(#12183),#86961,.T.);
#91463=ADVANCED_FACE('',(#12184),#3844,.T.);
#91464=ADVANCED_FACE('',(#12185),#3845,.T.);
#91465=ADVANCED_FACE('',(#12186),#86962,.T.);
#91466=ADVANCED_FACE('',(#12187),#3846,.T.);
#91467=ADVANCED_FACE('',(#12188),#3847,.T.);
#91468=ADVANCED_FACE('',(#12189),#3848,.T.);
#91469=ADVANCED_FACE('',(#12190),#86963,.T.);
#91470=ADVANCED_FACE('',(#12191),#86964,.T.);
#91471=ADVANCED_FACE('',(#12192),#3849,.T.);
#91472=ADVANCED_FACE('',(#12193),#3850,.T.);
#91473=ADVANCED_FACE('',(#12194),#86965,.T.);
#91474=ADVANCED_FACE('',(#12195),#86966,.T.);
#91475=ADVANCED_FACE('',(#12196),#3851,.T.);
#91476=ADVANCED_FACE('',(#12197),#3852,.T.);
#91477=ADVANCED_FACE('',(#12198),#86967,.T.);
#91478=ADVANCED_FACE('',(#12199),#86968,.T.);
#91479=ADVANCED_FACE('',(#12200),#3853,.T.);
#91480=ADVANCED_FACE('',(#12201),#3854,.T.);
#91481=ADVANCED_FACE('',(#12202),#86969,.T.);
#91482=ADVANCED_FACE('',(#12203),#3855,.T.);
#91483=ADVANCED_FACE('',(#12204),#3856,.T.);
#91484=ADVANCED_FACE('',(#12205),#3857,.T.);
#91485=ADVANCED_FACE('',(#12206),#86970,.T.);
#91486=ADVANCED_FACE('',(#12207),#86971,.T.);
#91487=ADVANCED_FACE('',(#12208),#3858,.T.);
#91488=ADVANCED_FACE('',(#12209),#3859,.T.);
#91489=ADVANCED_FACE('',(#12210),#86972,.T.);
#91490=ADVANCED_FACE('',(#12211),#86973,.T.);
#91491=ADVANCED_FACE('',(#12212),#3860,.T.);
#91492=ADVANCED_FACE('',(#12213),#3861,.T.);
#91493=ADVANCED_FACE('',(#12214),#86974,.T.);
#91494=ADVANCED_FACE('',(#12215),#3862,.T.);
#91495=ADVANCED_FACE('',(#12216),#3863,.T.);
#91496=ADVANCED_FACE('',(#12217),#3864,.T.);
#91497=ADVANCED_FACE('',(#12218),#86975,.T.);
#91498=ADVANCED_FACE('',(#12219),#3865,.T.);
#91499=ADVANCED_FACE('',(#12220),#86976,.T.);
#91500=ADVANCED_FACE('',(#12221),#3866,.T.);
#91501=ADVANCED_FACE('',(#12222),#3867,.T.);
#91502=ADVANCED_FACE('',(#12223),#3868,.T.);
#91503=ADVANCED_FACE('',(#12224),#86977,.T.);
#91504=ADVANCED_FACE('',(#12225),#3869,.T.);
#91505=ADVANCED_FACE('',(#12226),#3870,.T.);
#91506=ADVANCED_FACE('',(#12227),#3871,.T.);
#91507=ADVANCED_FACE('',(#12228),#3872,.T.);
#91508=ADVANCED_FACE('',(#12229),#3873,.T.);
#91509=ADVANCED_FACE('',(#12230),#3874,.T.);
#91510=ADVANCED_FACE('',(#12231),#3875,.T.);
#91511=ADVANCED_FACE('',(#12232),#3876,.T.);
#91512=ADVANCED_FACE('',(#12233),#3877,.T.);
#91513=ADVANCED_FACE('',(#12234),#3878,.T.);
#91514=ADVANCED_FACE('',(#12235),#3879,.T.);
#91515=ADVANCED_FACE('',(#12236),#3880,.T.);
#91516=ADVANCED_FACE('',(#12237),#3881,.T.);
#91517=ADVANCED_FACE('',(#12238),#3882,.T.);
#91518=ADVANCED_FACE('',(#12239),#3883,.T.);
#91519=ADVANCED_FACE('',(#12240),#3884,.T.);
#91520=ADVANCED_FACE('',(#12241),#3885,.T.);
#91521=ADVANCED_FACE('',(#12242),#3886,.T.);
#91522=ADVANCED_FACE('',(#12243),#3887,.T.);
#91523=ADVANCED_FACE('',(#12244),#3888,.T.);
#91524=ADVANCED_FACE('',(#12245),#3889,.T.);
#91525=ADVANCED_FACE('',(#12246),#86978,.T.);
#91526=ADVANCED_FACE('',(#12247),#3890,.T.);
#91527=ADVANCED_FACE('',(#12248),#3891,.T.);
#91528=ADVANCED_FACE('',(#12249),#3892,.T.);
#91529=ADVANCED_FACE('',(#12250),#86979,.T.);
#91530=ADVANCED_FACE('',(#12251),#3893,.T.);
#91531=ADVANCED_FACE('',(#12252),#3894,.T.);
#91532=ADVANCED_FACE('',(#12253),#86980,.T.);
#91533=ADVANCED_FACE('',(#12254),#3895,.T.);
#91534=ADVANCED_FACE('',(#12255),#3896,.T.);
#91535=ADVANCED_FACE('',(#12256),#3897,.T.);
#91536=ADVANCED_FACE('',(#12257),#86981,.T.);
#91537=ADVANCED_FACE('',(#12258),#3898,.T.);
#91538=ADVANCED_FACE('',(#12259),#3899,.T.);
#91539=ADVANCED_FACE('',(#12260),#86982,.T.);
#91540=ADVANCED_FACE('',(#12261),#3900,.T.);
#91541=ADVANCED_FACE('',(#12262),#3901,.T.);
#91542=ADVANCED_FACE('',(#12263),#3902,.T.);
#91543=ADVANCED_FACE('',(#12264),#86983,.T.);
#91544=ADVANCED_FACE('',(#12265),#3903,.T.);
#91545=ADVANCED_FACE('',(#12266),#3904,.T.);
#91546=ADVANCED_FACE('',(#12267),#86984,.T.);
#91547=ADVANCED_FACE('',(#12268),#3905,.T.);
#91548=ADVANCED_FACE('',(#12269),#3906,.T.);
#91549=ADVANCED_FACE('',(#12270),#3907,.T.);
#91550=ADVANCED_FACE('',(#12271),#86985,.T.);
#91551=ADVANCED_FACE('',(#12272),#3908,.T.);
#91552=ADVANCED_FACE('',(#12273),#3909,.T.);
#91553=ADVANCED_FACE('',(#12274),#3910,.T.);
#91554=ADVANCED_FACE('',(#12275),#3911,.T.);
#91555=ADVANCED_FACE('',(#12276),#3912,.T.);
#91556=ADVANCED_FACE('',(#12277),#3913,.T.);
#91557=ADVANCED_FACE('',(#12278),#3914,.T.);
#91558=ADVANCED_FACE('',(#12279),#3915,.T.);
#91559=ADVANCED_FACE('',(#12280),#3916,.T.);
#91560=ADVANCED_FACE('',(#12281),#3917,.T.);
#91561=ADVANCED_FACE('',(#12282),#3072,.T.);
#91562=ADVANCED_FACE('',(#12283),#3073,.T.);
#91563=ADVANCED_FACE('',(#12284),#3074,.T.);
#91564=ADVANCED_FACE('',(#12285),#3075,.T.);
#91565=ADVANCED_FACE('',(#12286),#3076,.T.);
#91566=ADVANCED_FACE('',(#12287),#3077,.T.);
#91567=ADVANCED_FACE('',(#12288),#3078,.T.);
#91568=ADVANCED_FACE('',(#12289),#3079,.T.);
#91569=ADVANCED_FACE('',(#12290),#3080,.T.);
#91570=ADVANCED_FACE('',(#12291),#3081,.T.);
#91571=ADVANCED_FACE('',(#12292),#3082,.T.);
#91572=ADVANCED_FACE('',(#12293),#3083,.T.);
#91573=ADVANCED_FACE('',(#12294),#3084,.T.);
#91574=ADVANCED_FACE('',(#12295),#3085,.T.);
#91575=ADVANCED_FACE('',(#12296),#3086,.T.);
#91576=ADVANCED_FACE('',(#12297),#3087,.T.);
#91577=ADVANCED_FACE('',(#12298),#3088,.T.);
#91578=ADVANCED_FACE('',(#12299),#3089,.T.);
#91579=ADVANCED_FACE('',(#12300),#3090,.T.);
#91580=ADVANCED_FACE('',(#12301),#3091,.T.);
#91581=ADVANCED_FACE('',(#12302),#3092,.T.);
#91582=ADVANCED_FACE('',(#12303),#3093,.T.);
#91583=ADVANCED_FACE('',(#12304),#3094,.T.);
#91584=ADVANCED_FACE('',(#12305),#3095,.T.);
#91585=ADVANCED_FACE('',(#12306),#3096,.T.);
#91586=ADVANCED_FACE('',(#12307),#3097,.T.);
#91587=ADVANCED_FACE('',(#12308),#3098,.T.);
#91588=ADVANCED_FACE('',(#12309),#3099,.T.);
#91589=ADVANCED_FACE('',(#12310),#3100,.T.);
#91590=ADVANCED_FACE('',(#12311),#3101,.T.);
#91591=ADVANCED_FACE('',(#12312),#3102,.T.);
#91592=ADVANCED_FACE('',(#12313),#3103,.T.);
#91593=ADVANCED_FACE('',(#12314),#3104,.T.);
#91594=ADVANCED_FACE('',(#12315),#3105,.T.);
#91595=ADVANCED_FACE('',(#12316),#3106,.T.);
#91596=ADVANCED_FACE('',(#12317),#3107,.T.);
#91597=ADVANCED_FACE('',(#12318),#3108,.T.);
#91598=ADVANCED_FACE('',(#12319),#3109,.T.);
#91599=ADVANCED_FACE('',(#12320),#3110,.T.);
#91600=ADVANCED_FACE('',(#12321),#3111,.T.);
#91601=ADVANCED_FACE('',(#12322),#3918,.T.);
#91602=ADVANCED_FACE('',(#12323),#3112,.T.);
#91603=ADVANCED_FACE('',(#12324),#3113,.T.);
#91604=ADVANCED_FACE('',(#12325),#3114,.T.);
#91605=ADVANCED_FACE('',(#12326),#3115,.T.);
#91606=ADVANCED_FACE('',(#12327),#3116,.T.);
#91607=ADVANCED_FACE('',(#12328),#3117,.T.);
#91608=ADVANCED_FACE('',(#12329),#3118,.T.);
#91609=ADVANCED_FACE('',(#12330),#3119,.T.);
#91610=ADVANCED_FACE('',(#12331),#3120,.T.);
#91611=ADVANCED_FACE('',(#12332),#3121,.T.);
#91612=ADVANCED_FACE('',(#12333),#3122,.T.);
#91613=ADVANCED_FACE('',(#12334),#3123,.T.);
#91614=ADVANCED_FACE('',(#12335),#86986,.F.);
#91615=ADVANCED_FACE('',(#12336),#86987,.F.);
#91616=ADVANCED_FACE('',(#12337),#86988,.F.);
#91617=ADVANCED_FACE('',(#12338),#86989,.F.);
#91618=ADVANCED_FACE('',(#12339),#86990,.F.);
#91619=ADVANCED_FACE('',(#12340),#86991,.F.);
#91620=ADVANCED_FACE('',(#12341),#86992,.F.);
#91621=ADVANCED_FACE('',(#12342),#86993,.F.);
#91622=ADVANCED_FACE('',(#12343),#86994,.F.);
#91623=ADVANCED_FACE('',(#12344),#86995,.F.);
#91624=ADVANCED_FACE('',(#12345),#86996,.F.);
#91625=ADVANCED_FACE('',(#12346),#86997,.F.);
#91626=ADVANCED_FACE('',(#12347),#86998,.F.);
#91627=ADVANCED_FACE('',(#12348),#86999,.F.);
#91628=ADVANCED_FACE('',(#12349),#87000,.F.);
#91629=ADVANCED_FACE('',(#12350),#87001,.F.);
#91630=ADVANCED_FACE('',(#12351),#87002,.F.);
#91631=ADVANCED_FACE('',(#12352),#87003,.F.);
#91632=ADVANCED_FACE('',(#12353),#87004,.F.);
#91633=ADVANCED_FACE('',(#12354),#87005,.F.);
#91634=ADVANCED_FACE('',(#12355),#87006,.F.);
#91635=ADVANCED_FACE('',(#12356),#87007,.F.);
#91636=ADVANCED_FACE('',(#12357),#87008,.F.);
#91637=ADVANCED_FACE('',(#12358),#87009,.F.);
#91638=ADVANCED_FACE('',(#12359),#87010,.F.);
#91639=ADVANCED_FACE('',(#12360),#87011,.F.);
#91640=ADVANCED_FACE('',(#12361),#87012,.F.);
#91641=ADVANCED_FACE('',(#12362),#87013,.F.);
#91642=ADVANCED_FACE('',(#12363),#87014,.F.);
#91643=ADVANCED_FACE('',(#12364),#87015,.F.);
#91644=ADVANCED_FACE('',(#12365),#87016,.F.);
#91645=ADVANCED_FACE('',(#12366),#87017,.F.);
#91646=ADVANCED_FACE('',(#12367),#87018,.F.);
#91647=ADVANCED_FACE('',(#12368),#87019,.F.);
#91648=ADVANCED_FACE('',(#12369),#87020,.F.);
#91649=ADVANCED_FACE('',(#12370),#87021,.F.);
#91650=ADVANCED_FACE('',(#12371),#87022,.F.);
#91651=ADVANCED_FACE('',(#12372),#87023,.F.);
#91652=ADVANCED_FACE('',(#12373),#87024,.F.);
#91653=ADVANCED_FACE('',(#12374),#87025,.F.);
#91654=ADVANCED_FACE('',(#12375),#87026,.F.);
#91655=ADVANCED_FACE('',(#12376),#87027,.F.);
#91656=ADVANCED_FACE('',(#12377),#87028,.F.);
#91657=ADVANCED_FACE('',(#12378),#87029,.F.);
#91658=ADVANCED_FACE('',(#12379),#87030,.F.);
#91659=ADVANCED_FACE('',(#12380),#87031,.F.);
#91660=ADVANCED_FACE('',(#12381),#87032,.F.);
#91661=ADVANCED_FACE('',(#12382),#87033,.F.);
#91662=ADVANCED_FACE('',(#12383),#87034,.F.);
#91663=ADVANCED_FACE('',(#12384),#87035,.F.);
#91664=ADVANCED_FACE('',(#12385),#87036,.F.);
#91665=ADVANCED_FACE('',(#12386),#87037,.F.);
#91666=ADVANCED_FACE('',(#12387),#87038,.F.);
#91667=ADVANCED_FACE('',(#12388),#87039,.F.);
#91668=ADVANCED_FACE('',(#12389),#87040,.F.);
#91669=ADVANCED_FACE('',(#12390),#87041,.F.);
#91670=ADVANCED_FACE('',(#12391),#87042,.F.);
#91671=ADVANCED_FACE('',(#12392),#87043,.F.);
#91672=ADVANCED_FACE('',(#12393),#87044,.F.);
#91673=ADVANCED_FACE('',(#12394),#87045,.F.);
#91674=ADVANCED_FACE('',(#12395),#87046,.F.);
#91675=ADVANCED_FACE('',(#12396),#87047,.F.);
#91676=ADVANCED_FACE('',(#12397),#87048,.F.);
#91677=ADVANCED_FACE('',(#12398),#87049,.F.);
#91678=ADVANCED_FACE('',(#12399),#87050,.F.);
#91679=ADVANCED_FACE('',(#12400),#87051,.F.);
#91680=ADVANCED_FACE('',(#12401),#87052,.F.);
#91681=ADVANCED_FACE('',(#12402),#87053,.F.);
#91682=ADVANCED_FACE('',(#12403),#87054,.F.);
#91683=ADVANCED_FACE('',(#12404),#87055,.F.);
#91684=ADVANCED_FACE('',(#12405),#87056,.F.);
#91685=ADVANCED_FACE('',(#12406),#87057,.F.);
#91686=ADVANCED_FACE('',(#12407),#87058,.F.);
#91687=ADVANCED_FACE('',(#12408),#87059,.F.);
#91688=ADVANCED_FACE('',(#12409),#87060,.F.);
#91689=ADVANCED_FACE('',(#12410),#87061,.F.);
#91690=ADVANCED_FACE('',(#12411),#87062,.F.);
#91691=ADVANCED_FACE('',(#12412),#87063,.F.);
#91692=ADVANCED_FACE('',(#12413),#87064,.F.);
#91693=ADVANCED_FACE('',(#12414),#87065,.F.);
#91694=ADVANCED_FACE('',(#12415),#87066,.F.);
#91695=ADVANCED_FACE('',(#12416),#87067,.F.);
#91696=ADVANCED_FACE('',(#12417),#87068,.F.);
#91697=ADVANCED_FACE('',(#12418),#87069,.F.);
#91698=ADVANCED_FACE('',(#12419),#87070,.F.);
#91699=ADVANCED_FACE('',(#12420),#87071,.F.);
#91700=ADVANCED_FACE('',(#12421),#87072,.F.);
#91701=ADVANCED_FACE('',(#12422),#87073,.F.);
#91702=ADVANCED_FACE('',(#12423),#87074,.F.);
#91703=ADVANCED_FACE('',(#12424),#87075,.F.);
#91704=ADVANCED_FACE('',(#12425),#87076,.F.);
#91705=ADVANCED_FACE('',(#12426),#87077,.F.);
#91706=ADVANCED_FACE('',(#12427),#87078,.F.);
#91707=ADVANCED_FACE('',(#12428),#87079,.F.);
#91708=ADVANCED_FACE('',(#12429),#87080,.F.);
#91709=ADVANCED_FACE('',(#12430),#87081,.F.);
#91710=ADVANCED_FACE('',(#12431),#87082,.F.);
#91711=ADVANCED_FACE('',(#12432),#87083,.F.);
#91712=ADVANCED_FACE('',(#12433),#87084,.F.);
#91713=ADVANCED_FACE('',(#12434),#87085,.F.);
#91714=ADVANCED_FACE('',(#12435),#87086,.F.);
#91715=ADVANCED_FACE('',(#12436),#87087,.F.);
#91716=ADVANCED_FACE('',(#12437),#87088,.F.);
#91717=ADVANCED_FACE('',(#12438),#87089,.F.);
#91718=ADVANCED_FACE('',(#12439),#87090,.F.);
#91719=ADVANCED_FACE('',(#12440),#87091,.F.);
#91720=ADVANCED_FACE('',(#12441),#87092,.F.);
#91721=ADVANCED_FACE('',(#12442),#87093,.F.);
#91722=ADVANCED_FACE('',(#12443),#87094,.F.);
#91723=ADVANCED_FACE('',(#12444),#87095,.F.);
#91724=ADVANCED_FACE('',(#12445),#87096,.F.);
#91725=ADVANCED_FACE('',(#12446),#87097,.F.);
#91726=ADVANCED_FACE('',(#12447),#87098,.F.);
#91727=ADVANCED_FACE('',(#12448),#87099,.F.);
#91728=ADVANCED_FACE('',(#12449),#87100,.F.);
#91729=ADVANCED_FACE('',(#12450),#87101,.F.);
#91730=ADVANCED_FACE('',(#12451),#87102,.F.);
#91731=ADVANCED_FACE('',(#12452),#87103,.F.);
#91732=ADVANCED_FACE('',(#12453),#87104,.F.);
#91733=ADVANCED_FACE('',(#12454),#87105,.F.);
#91734=ADVANCED_FACE('',(#12455),#87106,.F.);
#91735=ADVANCED_FACE('',(#12456),#87107,.F.);
#91736=ADVANCED_FACE('',(#12457),#87108,.F.);
#91737=ADVANCED_FACE('',(#12458),#87109,.F.);
#91738=ADVANCED_FACE('',(#12459),#87110,.F.);
#91739=ADVANCED_FACE('',(#12460),#87111,.F.);
#91740=ADVANCED_FACE('',(#12461),#87112,.F.);
#91741=ADVANCED_FACE('',(#12462),#87113,.F.);
#91742=ADVANCED_FACE('',(#12463),#87114,.F.);
#91743=ADVANCED_FACE('',(#12464),#87115,.F.);
#91744=ADVANCED_FACE('',(#12465),#87116,.F.);
#91745=ADVANCED_FACE('',(#12466),#87117,.F.);
#91746=ADVANCED_FACE('',(#12467),#87118,.F.);
#91747=ADVANCED_FACE('',(#12468),#87119,.F.);
#91748=ADVANCED_FACE('',(#12469),#87120,.F.);
#91749=ADVANCED_FACE('',(#12470),#87121,.F.);
#91750=ADVANCED_FACE('',(#12471),#87122,.F.);
#91751=ADVANCED_FACE('',(#12472),#87123,.F.);
#91752=ADVANCED_FACE('',(#12473),#8180,.T.);
#91753=ADVANCED_FACE('',(#12474),#87124,.F.);
#91754=ADVANCED_FACE('',(#12475,#7456),#8181,.T.);
#91755=ADVANCED_FACE('',(#12476),#87125,.T.);
#91756=ADVANCED_FACE('',(#12477),#87126,.T.);
#91757=ADVANCED_FACE('',(#12478),#87127,.T.);
#91758=ADVANCED_FACE('',(#12479),#87128,.F.);
#91759=ADVANCED_FACE('',(#12480),#8182,.F.);
#91760=ADVANCED_FACE('',(#12481),#8183,.F.);
#91761=ADVANCED_FACE('',(#12482),#87129,.F.);
#91762=ADVANCED_FACE('',(#12483),#87130,.T.);
#91763=ADVANCED_FACE('',(#12484),#87131,.F.);
#91764=ADVANCED_FACE('',(#12485),#8184,.T.);
#91765=ADVANCED_FACE('',(#12486),#8185,.T.);
#91766=ADVANCED_FACE('',(#12487),#87132,.F.);
#91767=ADVANCED_FACE('',(#12488),#87133,.T.);
#91768=ADVANCED_FACE('',(#12489),#8186,.F.);
#91769=ADVANCED_FACE('',(#12490),#8187,.F.);
#91770=ADVANCED_FACE('',(#12491),#8188,.F.);
#91771=ADVANCED_FACE('',(#12492),#8189,.F.);
#91772=ADVANCED_FACE('',(#12493),#8190,.F.);
#91773=ADVANCED_FACE('',(#12494),#8191,.F.);
#91774=ADVANCED_FACE('',(#12495),#8192,.F.);
#91775=ADVANCED_FACE('',(#12496),#8193,.F.);
#91776=ADVANCED_FACE('',(#12497),#8194,.F.);
#91777=ADVANCED_FACE('',(#12498),#8195,.F.);
#91778=ADVANCED_FACE('',(#12499),#8196,.F.);
#91779=ADVANCED_FACE('',(#12500),#8197,.F.);
#91780=ADVANCED_FACE('',(#12501),#8198,.F.);
#91781=ADVANCED_FACE('',(#12502),#8199,.F.);
#91782=ADVANCED_FACE('',(#12503),#8200,.F.);
#91783=ADVANCED_FACE('',(#12504),#8201,.F.);
#91784=ADVANCED_FACE('',(#12505),#8202,.F.);
#91785=ADVANCED_FACE('',(#12506),#8203,.F.);
#91786=ADVANCED_FACE('',(#12507),#8204,.F.);
#91787=ADVANCED_FACE('',(#12508),#8205,.F.);
#91788=ADVANCED_FACE('',(#12509),#8206,.F.);
#91789=ADVANCED_FACE('',(#12510),#8207,.F.);
#91790=ADVANCED_FACE('',(#12511),#8208,.F.);
#91791=ADVANCED_FACE('',(#12512),#8209,.F.);
#91792=ADVANCED_FACE('',(#12513),#8210,.F.);
#91793=ADVANCED_FACE('',(#12514),#8211,.F.);
#91794=ADVANCED_FACE('',(#12515),#8212,.F.);
#91795=ADVANCED_FACE('',(#12516),#8213,.F.);
#91796=ADVANCED_FACE('',(#12517),#8214,.F.);
#91797=ADVANCED_FACE('',(#12518),#8215,.F.);
#91798=ADVANCED_FACE('',(#12519),#8216,.F.);
#91799=ADVANCED_FACE('',(#12520),#8217,.F.);
#91800=ADVANCED_FACE('',(#12521),#8218,.F.);
#91801=ADVANCED_FACE('',(#12522),#8219,.F.);
#91802=ADVANCED_FACE('',(#12523),#8220,.F.);
#91803=ADVANCED_FACE('',(#12524),#8221,.F.);
#91804=ADVANCED_FACE('',(#12525),#8222,.F.);
#91805=ADVANCED_FACE('',(#12526),#8223,.F.);
#91806=ADVANCED_FACE('',(#12527),#8224,.F.);
#91807=ADVANCED_FACE('',(#12528),#8225,.F.);
#91808=ADVANCED_FACE('',(#12529),#8226,.F.);
#91809=ADVANCED_FACE('',(#12530),#8227,.F.);
#91810=ADVANCED_FACE('',(#12531),#8228,.F.);
#91811=ADVANCED_FACE('',(#12532),#8229,.F.);
#91812=ADVANCED_FACE('',(#12533),#8230,.F.);
#91813=ADVANCED_FACE('',(#12534),#8231,.F.);
#91814=ADVANCED_FACE('',(#12535),#8232,.F.);
#91815=ADVANCED_FACE('',(#12536),#8233,.F.);
#91816=ADVANCED_FACE('',(#12537),#8234,.F.);
#91817=ADVANCED_FACE('',(#12538),#8235,.F.);
#91818=ADVANCED_FACE('',(#12539),#8236,.F.);
#91819=ADVANCED_FACE('',(#12540),#8237,.F.);
#91820=ADVANCED_FACE('',(#12541),#8238,.F.);
#91821=ADVANCED_FACE('',(#12542),#8239,.F.);
#91822=ADVANCED_FACE('',(#12543),#8240,.F.);
#91823=ADVANCED_FACE('',(#12544),#8241,.F.);
#91824=ADVANCED_FACE('',(#12545),#8242,.F.);
#91825=ADVANCED_FACE('',(#12546,#7457,#7458,#7459,#7460,#7461,#7462,#7463,
#7464,#7465,#7466,#7467,#7468,#7469,#7470,#7471,#7472,#7473,#7474,#7475,
#7476,#7477,#7478,#7479,#7480,#7481,#7482,#7483,#7484,#7485,#7486,#7487,
#7488,#7489,#7490,#7491,#7492,#7493,#7494,#7495,#7496,#7497,#7498,#7499,
#7500,#7501,#7502,#7503,#7504,#7505,#7506,#7507,#7508,#7509,#7510,#7511,
#7512,#7513,#7514,#7515,#7516,#7517,#7518,#7519,#7520,#7521,#7522,#7523,
#7524),#8243,.F.);
#91826=ADVANCED_FACE('',(#12547),#87134,.T.);
#91827=ADVANCED_FACE('',(#12548),#87135,.T.);
#91828=ADVANCED_FACE('',(#12549),#87136,.T.);
#91829=ADVANCED_FACE('',(#12550),#87137,.T.);
#91830=ADVANCED_FACE('',(#12551),#87138,.T.);
#91831=ADVANCED_FACE('',(#12552),#87139,.T.);
#91832=ADVANCED_FACE('',(#12553),#87140,.T.);
#91833=ADVANCED_FACE('',(#12554),#87141,.T.);
#91834=ADVANCED_FACE('',(#12555),#8244,.T.);
#91835=ADVANCED_FACE('',(#12556),#8245,.T.);
#91836=ADVANCED_FACE('',(#12557),#8246,.F.);
#91837=ADVANCED_FACE('',(#12558),#8247,.T.);
#91838=ADVANCED_FACE('',(#12559),#8248,.F.);
#91839=ADVANCED_FACE('',(#12560),#8249,.F.);
#91840=ADVANCED_FACE('',(#12561),#87142,.F.);
#91841=ADVANCED_FACE('',(#12562),#8250,.F.);
#91842=ADVANCED_FACE('',(#12563),#8251,.F.);
#91843=ADVANCED_FACE('',(#12564),#87143,.F.);
#91844=ADVANCED_FACE('',(#12565),#927,.T.);
#91845=ADVANCED_FACE('',(#12566),#928,.F.);
#91846=ADVANCED_FACE('',(#12567),#87144,.T.);
#91847=ADVANCED_FACE('',(#12568),#87145,.T.);
#91848=ADVANCED_FACE('',(#12569),#87146,.T.);
#91849=ADVANCED_FACE('',(#12570),#87147,.T.);
#91850=ADVANCED_FACE('',(#12571),#87148,.T.);
#91851=ADVANCED_FACE('',(#12572),#87149,.T.);
#91852=ADVANCED_FACE('',(#12573),#87150,.T.);
#91853=ADVANCED_FACE('',(#12574),#87151,.T.);
#91854=ADVANCED_FACE('',(#12575),#87152,.T.);
#91855=ADVANCED_FACE('',(#12576),#929,.F.);
#91856=ADVANCED_FACE('',(#12577),#930,.F.);
#91857=ADVANCED_FACE('',(#12578),#931,.F.);
#91858=ADVANCED_FACE('',(#12579),#932,.F.);
#91859=ADVANCED_FACE('',(#12580),#7040,.F.);
#91860=ADVANCED_FACE('',(#12581),#7041,.F.);
#91861=ADVANCED_FACE('',(#12582),#7042,.F.);
#91862=ADVANCED_FACE('',(#12583),#7043,.F.);
#91863=ADVANCED_FACE('',(#12584),#7044,.F.);
#91864=ADVANCED_FACE('',(#12585),#7045,.F.);
#91865=ADVANCED_FACE('',(#12586),#7046,.F.);
#91866=ADVANCED_FACE('',(#12587,#7525),#8252,.T.);
#91867=ADVANCED_FACE('',(#12588),#7047,.F.);
#91868=ADVANCED_FACE('',(#12589),#7048,.F.);
#91869=ADVANCED_FACE('',(#12590),#7049,.F.);
#91870=ADVANCED_FACE('',(#12591),#7050,.F.);
#91871=ADVANCED_FACE('',(#12592),#7051,.F.);
#91872=ADVANCED_FACE('',(#12593),#7052,.F.);
#91873=ADVANCED_FACE('',(#12594),#7053,.F.);
#91874=ADVANCED_FACE('',(#12595),#7054,.F.);
#91875=ADVANCED_FACE('',(#12596),#7055,.F.);
#91876=ADVANCED_FACE('',(#12597),#933,.F.);
#91877=ADVANCED_FACE('',(#12598),#934,.F.);
#91878=ADVANCED_FACE('',(#12599),#7056,.F.);
#91879=ADVANCED_FACE('',(#12600),#935,.F.);
#91880=ADVANCED_FACE('',(#12601),#7057,.F.);
#91881=ADVANCED_FACE('',(#12602),#8253,.F.);
#91882=ADVANCED_FACE('',(#12603),#936,.F.);
#91883=ADVANCED_FACE('',(#12604),#8254,.F.);
#91884=ADVANCED_FACE('',(#12605),#937,.F.);
#91885=ADVANCED_FACE('',(#12606),#8255,.T.);
#91886=ADVANCED_FACE('',(#12607),#938,.F.);
#91887=ADVANCED_FACE('',(#12608),#8256,.F.);
#91888=ADVANCED_FACE('',(#12609),#8257,.F.);
#91889=ADVANCED_FACE('',(#12610),#8258,.F.);
#91890=ADVANCED_FACE('',(#12611),#8259,.F.);
#91891=ADVANCED_FACE('',(#12612),#8260,.F.);
#91892=ADVANCED_FACE('',(#12613),#8261,.F.);
#91893=ADVANCED_FACE('',(#12614),#8262,.F.);
#91894=ADVANCED_FACE('',(#12615),#8263,.F.);
#91895=ADVANCED_FACE('',(#12616),#8264,.F.);
#91896=ADVANCED_FACE('',(#12617),#87153,.T.);
#91897=ADVANCED_FACE('',(#12618),#87154,.T.);
#91898=ADVANCED_FACE('',(#12619),#87155,.T.);
#91899=ADVANCED_FACE('',(#12620),#87156,.T.);
#91900=ADVANCED_FACE('',(#12621),#87157,.T.);
#91901=ADVANCED_FACE('',(#12622),#8265,.T.);
#91902=ADVANCED_FACE('',(#12623),#7058,.T.);
#91903=ADVANCED_FACE('',(#12624),#8266,.T.);
#91904=ADVANCED_FACE('',(#12625),#939,.F.);
#91905=ADVANCED_FACE('',(#12626),#7059,.T.);
#91906=ADVANCED_FACE('',(#12627),#87158,.F.);
#91907=ADVANCED_FACE('',(#12628),#87159,.F.);
#91908=ADVANCED_FACE('',(#12629),#87160,.F.);
#91909=ADVANCED_FACE('',(#12630),#87161,.F.);
#91910=ADVANCED_FACE('',(#12631),#87162,.F.);
#91911=ADVANCED_FACE('',(#12632),#87163,.F.);
#91912=ADVANCED_FACE('',(#12633),#87164,.F.);
#91913=ADVANCED_FACE('',(#12634),#8267,.T.);
#91914=ADVANCED_FACE('',(#12635),#7060,.F.);
#91915=ADVANCED_FACE('',(#12636),#8268,.T.);
#91916=ADVANCED_FACE('',(#12637),#7061,.F.);
#91917=ADVANCED_FACE('',(#12638,#7526),#8269,.F.);
#91918=ADVANCED_FACE('',(#12639),#8270,.F.);
#91919=ADVANCED_FACE('',(#12640),#8271,.F.);
#91920=ADVANCED_FACE('',(#12641),#87165,.T.);
#91921=ADVANCED_FACE('',(#12642),#8272,.T.);
#91922=ADVANCED_FACE('',(#12643),#8273,.F.);
#91923=ADVANCED_FACE('',(#12644),#8274,.F.);
#91924=ADVANCED_FACE('',(#12645),#87166,.T.);
#91925=ADVANCED_FACE('',(#12646),#8275,.T.);
#91926=ADVANCED_FACE('',(#12647),#8276,.T.);
#91927=ADVANCED_FACE('',(#12648),#87167,.T.);
#91928=ADVANCED_FACE('',(#12649),#8277,.T.);
#91929=ADVANCED_FACE('',(#12650),#8278,.T.);
#91930=ADVANCED_FACE('',(#12651),#87168,.T.);
#91931=ADVANCED_FACE('',(#12652),#940,.F.);
#91932=ADVANCED_FACE('',(#12653),#941,.T.);
#91933=ADVANCED_FACE('',(#12654),#942,.T.);
#91934=ADVANCED_FACE('',(#12655,#7527,#7528,#7529,#7530,#7531,#7532,#7533,
#7534,#7535,#7536,#7537,#7538,#7539,#7540,#7541,#7542,#7543,#7544,#7545,
#7546,#7547,#7548,#7549,#7550,#7551,#7552,#7553,#7554,#7555,#7556,#7557,
#7558,#7559,#7560,#7561,#7562,#7563,#7564,#7565,#7566,#7567,#7568,#7569,
#7570,#7571,#7572,#7573,#7574,#7575,#7576,#7577,#7578,#7579,#7580,#7581,
#7582,#7583,#7584,#7585,#7586,#7587),#8279,.T.);
#91935=ADVANCED_FACE('',(#12656),#87169,.T.);
#91936=ADVANCED_FACE('',(#12657),#87170,.T.);
#91937=ADVANCED_FACE('',(#12658),#87171,.T.);
#91938=ADVANCED_FACE('',(#12659),#87172,.T.);
#91939=ADVANCED_FACE('',(#12660),#87173,.T.);
#91940=ADVANCED_FACE('',(#12661),#87174,.T.);
#91941=ADVANCED_FACE('',(#12662),#87175,.T.);
#91942=ADVANCED_FACE('',(#12663),#87176,.T.);
#91943=ADVANCED_FACE('',(#12664),#87177,.T.);
#91944=ADVANCED_FACE('',(#12665,#7588),#8280,.T.);
#91945=ADVANCED_FACE('',(#12666),#87178,.F.);
#91946=ADVANCED_FACE('',(#12667),#87179,.F.);
#91947=ADVANCED_FACE('',(#12668),#87180,.F.);
#91948=ADVANCED_FACE('',(#12669),#87181,.F.);
#91949=ADVANCED_FACE('',(#12670),#87182,.F.);
#91950=ADVANCED_FACE('',(#12671),#87183,.F.);
#91951=ADVANCED_FACE('',(#12672),#87184,.F.);
#91952=ADVANCED_FACE('',(#12673),#87185,.F.);
#91953=ADVANCED_FACE('',(#12674),#87186,.F.);
#91954=ADVANCED_FACE('',(#12675),#943,.T.);
#91955=ADVANCED_FACE('',(#12676),#944,.T.);
#91956=ADVANCED_FACE('',(#12677),#945,.T.);
#91957=ADVANCED_FACE('',(#12678),#946,.T.);
#91958=ADVANCED_FACE('',(#12679),#7062,.T.);
#91959=ADVANCED_FACE('',(#12680),#7063,.T.);
#91960=ADVANCED_FACE('',(#12681),#7064,.T.);
#91961=ADVANCED_FACE('',(#12682),#7065,.T.);
#91962=ADVANCED_FACE('',(#12683),#7066,.T.);
#91963=ADVANCED_FACE('',(#12684),#7067,.T.);
#91964=ADVANCED_FACE('',(#12685),#7068,.T.);
#91965=ADVANCED_FACE('',(#12686,#7589),#8281,.T.);
#91966=ADVANCED_FACE('',(#12687,#7590),#8282,.F.);
#91967=ADVANCED_FACE('',(#12688),#7069,.T.);
#91968=ADVANCED_FACE('',(#12689),#7070,.T.);
#91969=ADVANCED_FACE('',(#12690),#7071,.T.);
#91970=ADVANCED_FACE('',(#12691),#7072,.T.);
#91971=ADVANCED_FACE('',(#12692),#7073,.T.);
#91972=ADVANCED_FACE('',(#12693),#7074,.T.);
#91973=ADVANCED_FACE('',(#12694),#7075,.T.);
#91974=ADVANCED_FACE('',(#12695),#7076,.T.);
#91975=ADVANCED_FACE('',(#12696),#7077,.T.);
#91976=ADVANCED_FACE('',(#12697),#947,.T.);
#91977=ADVANCED_FACE('',(#12698),#948,.T.);
#91978=ADVANCED_FACE('',(#12699),#7078,.T.);
#91979=ADVANCED_FACE('',(#12700),#949,.T.);
#91980=ADVANCED_FACE('',(#12701),#7079,.T.);
#91981=ADVANCED_FACE('',(#12702,#7591),#8283,.T.);
#91982=ADVANCED_FACE('',(#12703),#950,.T.);
#91983=ADVANCED_FACE('',(#12704),#8284,.T.);
#91984=ADVANCED_FACE('',(#12705),#951,.T.);
#91985=ADVANCED_FACE('',(#12706),#8285,.F.);
#91986=ADVANCED_FACE('',(#12707),#952,.T.);
#91987=ADVANCED_FACE('',(#12708),#87187,.F.);
#91988=ADVANCED_FACE('',(#12709),#87188,.F.);
#91989=ADVANCED_FACE('',(#12710),#87189,.F.);
#91990=ADVANCED_FACE('',(#12711),#87190,.F.);
#91991=ADVANCED_FACE('',(#12712),#87191,.F.);
#91992=ADVANCED_FACE('',(#12713),#8286,.T.);
#91993=ADVANCED_FACE('',(#12714),#8287,.T.);
#91994=ADVANCED_FACE('',(#12715),#8288,.T.);
#91995=ADVANCED_FACE('',(#12716),#8289,.T.);
#91996=ADVANCED_FACE('',(#12717),#8290,.T.);
#91997=ADVANCED_FACE('',(#12718),#8291,.T.);
#91998=ADVANCED_FACE('',(#12719),#8292,.T.);
#91999=ADVANCED_FACE('',(#12720),#8293,.T.);
#92000=ADVANCED_FACE('',(#12721),#8294,.T.);
#92001=ADVANCED_FACE('',(#12722),#8295,.T.);
#92002=ADVANCED_FACE('',(#12723),#87192,.F.);
#92003=ADVANCED_FACE('',(#12724),#87193,.F.);
#92004=ADVANCED_FACE('',(#12725),#87194,.T.);
#92005=ADVANCED_FACE('',(#12726),#87195,.T.);
#92006=ADVANCED_FACE('',(#12727,#7592),#8296,.F.);
#92007=ADVANCED_FACE('',(#12728),#8297,.T.);
#92008=ADVANCED_FACE('',(#12729),#8298,.T.);
#92009=ADVANCED_FACE('',(#12730),#8299,.T.);
#92010=ADVANCED_FACE('',(#12731),#8300,.T.);
#92011=ADVANCED_FACE('',(#12732),#8301,.T.);
#92012=ADVANCED_FACE('',(#12733),#8302,.T.);
#92013=ADVANCED_FACE('',(#12734),#8303,.T.);
#92014=ADVANCED_FACE('',(#12735),#8304,.T.);
#92015=ADVANCED_FACE('',(#12736),#8305,.T.);
#92016=ADVANCED_FACE('',(#12737),#8306,.T.);
#92017=ADVANCED_FACE('',(#12738),#8307,.T.);
#92018=ADVANCED_FACE('',(#12739),#8308,.T.);
#92019=ADVANCED_FACE('',(#12740),#8309,.T.);
#92020=ADVANCED_FACE('',(#12741),#8310,.T.);
#92021=ADVANCED_FACE('',(#12742),#87196,.F.);
#92022=ADVANCED_FACE('',(#12743),#87197,.F.);
#92023=ADVANCED_FACE('',(#12744),#87198,.F.);
#92024=ADVANCED_FACE('',(#12745),#87199,.F.);
#92025=ADVANCED_FACE('',(#12746),#87200,.F.);
#92026=ADVANCED_FACE('',(#12747),#87201,.F.);
#92027=ADVANCED_FACE('',(#12748),#87202,.F.);
#92028=ADVANCED_FACE('',(#12749),#87203,.F.);
#92029=ADVANCED_FACE('',(#12750),#8311,.T.);
#92030=ADVANCED_FACE('',(#12751),#8312,.T.);
#92031=ADVANCED_FACE('',(#12752),#8313,.T.);
#92032=ADVANCED_FACE('',(#12753),#8314,.T.);
#92033=ADVANCED_FACE('',(#12754),#8315,.T.);
#92034=ADVANCED_FACE('',(#12755),#8316,.T.);
#92035=ADVANCED_FACE('',(#12756),#8317,.T.);
#92036=ADVANCED_FACE('',(#12757),#8318,.T.);
#92037=ADVANCED_FACE('',(#12758),#8319,.T.);
#92038=ADVANCED_FACE('',(#12759),#8320,.T.);
#92039=ADVANCED_FACE('',(#12760),#8321,.T.);
#92040=ADVANCED_FACE('',(#12761),#8322,.T.);
#92041=ADVANCED_FACE('',(#12762),#8323,.T.);
#92042=ADVANCED_FACE('',(#12763),#8324,.T.);
#92043=ADVANCED_FACE('',(#12764),#8325,.T.);
#92044=ADVANCED_FACE('',(#12765),#8326,.T.);
#92045=ADVANCED_FACE('',(#12766),#8327,.T.);
#92046=ADVANCED_FACE('',(#12767),#8328,.T.);
#92047=ADVANCED_FACE('',(#12768),#8329,.T.);
#92048=ADVANCED_FACE('',(#12769),#8330,.T.);
#92049=ADVANCED_FACE('',(#12770),#8331,.T.);
#92050=ADVANCED_FACE('',(#12771),#8332,.T.);
#92051=ADVANCED_FACE('',(#12772),#8333,.T.);
#92052=ADVANCED_FACE('',(#12773),#8334,.T.);
#92053=ADVANCED_FACE('',(#12774),#8335,.T.);
#92054=ADVANCED_FACE('',(#12775),#8336,.T.);
#92055=ADVANCED_FACE('',(#12776),#8337,.T.);
#92056=ADVANCED_FACE('',(#12777),#8338,.T.);
#92057=ADVANCED_FACE('',(#12778),#3919,.T.);
#92058=ADVANCED_FACE('',(#12779),#8339,.F.);
#92059=ADVANCED_FACE('',(#12780),#8340,.F.);
#92060=ADVANCED_FACE('',(#12781),#8341,.F.);
#92061=ADVANCED_FACE('',(#12782),#8342,.F.);
#92062=ADVANCED_FACE('',(#12783),#8343,.F.);
#92063=ADVANCED_FACE('',(#12784),#8344,.F.);
#92064=ADVANCED_FACE('',(#12785),#7080,.F.);
#92065=ADVANCED_FACE('',(#12786),#7081,.F.);
#92066=ADVANCED_FACE('',(#12787),#7082,.F.);
#92067=ADVANCED_FACE('',(#12788),#7083,.F.);
#92068=ADVANCED_FACE('',(#12789),#7084,.F.);
#92069=ADVANCED_FACE('',(#12790),#7085,.F.);
#92070=ADVANCED_FACE('',(#12791),#7086,.F.);
#92071=ADVANCED_FACE('',(#12792),#3920,.T.);
#92072=ADVANCED_FACE('',(#12793),#8345,.F.);
#92073=ADVANCED_FACE('',(#12794,#7593),#8346,.T.);
#92074=ADVANCED_FACE('',(#12795),#87204,.T.);
#92075=ADVANCED_FACE('',(#12796),#8347,.T.);
#92076=ADVANCED_FACE('',(#12797),#7087,.T.);
#92077=ADVANCED_FACE('',(#12798),#7088,.T.);
#92078=ADVANCED_FACE('',(#12799),#7089,.T.);
#92079=ADVANCED_FACE('',(#12800),#7090,.T.);
#92080=ADVANCED_FACE('',(#12801),#7091,.T.);
#92081=ADVANCED_FACE('',(#12802),#7092,.T.);
#92082=ADVANCED_FACE('',(#12803),#8348,.F.);
#92083=ADVANCED_FACE('',(#12804),#7093,.T.);
#92084=ADVANCED_FACE('',(#12805),#7094,.T.);
#92085=ADVANCED_FACE('',(#12806),#7095,.T.);
#92086=ADVANCED_FACE('',(#12807),#7096,.T.);
#92087=ADVANCED_FACE('',(#12808),#7097,.T.);
#92088=ADVANCED_FACE('',(#12809),#7098,.T.);
#92089=ADVANCED_FACE('',(#12810),#8349,.F.);
#92090=ADVANCED_FACE('',(#12811),#8350,.F.);
#92091=ADVANCED_FACE('',(#12812),#8351,.F.);
#92092=ADVANCED_FACE('',(#12813),#8352,.F.);
#92093=ADVANCED_FACE('',(#12814),#8353,.F.);
#92094=ADVANCED_FACE('',(#12815),#8354,.F.);
#92095=ADVANCED_FACE('',(#12816),#8355,.T.);
#92096=ADVANCED_FACE('',(#12817),#7099,.T.);
#92097=ADVANCED_FACE('',(#12818),#7100,.T.);
#92098=ADVANCED_FACE('',(#12819),#7101,.T.);
#92099=ADVANCED_FACE('',(#12820),#7102,.T.);
#92100=ADVANCED_FACE('',(#12821),#7103,.T.);
#92101=ADVANCED_FACE('',(#12822),#7104,.T.);
#92102=ADVANCED_FACE('',(#12823),#8356,.F.);
#92103=ADVANCED_FACE('',(#12824),#7105,.T.);
#92104=ADVANCED_FACE('',(#12825),#7106,.T.);
#92105=ADVANCED_FACE('',(#12826),#7107,.T.);
#92106=ADVANCED_FACE('',(#12827),#7108,.T.);
#92107=ADVANCED_FACE('',(#12828),#7109,.T.);
#92108=ADVANCED_FACE('',(#12829),#7110,.T.);
#92109=ADVANCED_FACE('',(#12830),#8357,.F.);
#92110=ADVANCED_FACE('',(#12831),#8358,.F.);
#92111=ADVANCED_FACE('',(#12832),#8359,.F.);
#92112=ADVANCED_FACE('',(#12833),#8360,.F.);
#92113=ADVANCED_FACE('',(#12834),#8361,.F.);
#92114=ADVANCED_FACE('',(#12835),#8362,.F.);
#92115=ADVANCED_FACE('',(#12836),#8363,.F.);
#92116=ADVANCED_FACE('',(#12837),#8364,.F.);
#92117=ADVANCED_FACE('',(#12838),#8365,.F.);
#92118=ADVANCED_FACE('',(#12839),#8366,.F.);
#92119=ADVANCED_FACE('',(#12840),#8367,.F.);
#92120=ADVANCED_FACE('',(#12841),#8368,.F.);
#92121=ADVANCED_FACE('',(#12842),#7111,.F.);
#92122=ADVANCED_FACE('',(#12843),#7112,.F.);
#92123=ADVANCED_FACE('',(#12844),#7113,.F.);
#92124=ADVANCED_FACE('',(#12845),#7114,.F.);
#92125=ADVANCED_FACE('',(#12846),#7115,.F.);
#92126=ADVANCED_FACE('',(#12847),#7116,.F.);
#92127=ADVANCED_FACE('',(#12848),#7117,.F.);
#92128=ADVANCED_FACE('',(#12849),#3921,.T.);
#92129=ADVANCED_FACE('',(#12850),#8369,.F.);
#92130=ADVANCED_FACE('',(#12851,#7594),#8370,.T.);
#92131=ADVANCED_FACE('',(#12852),#87205,.T.);
#92132=ADVANCED_FACE('',(#12853,#7595),#1026,.T.);
#92133=ADVANCED_FACE('',(#12854),#3922,.T.);
#92134=ADVANCED_FACE('',(#12855),#3923,.T.);
#92135=ADVANCED_FACE('',(#12856),#8371,.F.);
#92136=ADVANCED_FACE('',(#12857),#8372,.F.);
#92137=ADVANCED_FACE('',(#12858),#7118,.F.);
#92138=ADVANCED_FACE('',(#12859),#8373,.F.);
#92139=ADVANCED_FACE('',(#12860),#7119,.F.);
#92140=ADVANCED_FACE('',(#12861),#8374,.T.);
#92141=ADVANCED_FACE('',(#12862),#87206,.T.);
#92142=ADVANCED_FACE('',(#12863),#87207,.T.);
#92143=ADVANCED_FACE('',(#12864,#7596),#8375,.T.);
#92144=ADVANCED_FACE('',(#12865),#7120,.T.);
#92145=ADVANCED_FACE('',(#12866),#8376,.T.);
#92146=ADVANCED_FACE('',(#12867),#87208,.T.);
#92147=ADVANCED_FACE('',(#12868,#7597),#8377,.F.);
#92148=ADVANCED_FACE('',(#12869),#87209,.T.);
#92149=ADVANCED_FACE('',(#12870),#8378,.F.);
#92150=ADVANCED_FACE('',(#12871),#3924,.T.);
#92151=ADVANCED_FACE('',(#12872),#87210,.T.);
#92152=ADVANCED_FACE('',(#12873),#87211,.T.);
#92153=ADVANCED_FACE('',(#12874),#3925,.T.);
#92154=ADVANCED_FACE('',(#12875),#3926,.T.);
#92155=ADVANCED_FACE('',(#12876),#87212,.T.);
#92156=ADVANCED_FACE('',(#12877),#87213,.T.);
#92157=ADVANCED_FACE('',(#12878),#3927,.T.);
#92158=ADVANCED_FACE('',(#12879),#8379,.F.);
#92159=ADVANCED_FACE('',(#12880),#87214,.T.);
#92160=ADVANCED_FACE('',(#12881),#87215,.T.);
#92161=ADVANCED_FACE('',(#12882,#7598,#7599),#8380,.F.);
#92162=ADVANCED_FACE('',(#12883),#3928,.F.);
#92163=ADVANCED_FACE('',(#12884),#87216,.F.);
#92164=ADVANCED_FACE('',(#12885),#3929,.F.);
#92165=ADVANCED_FACE('',(#12886),#87217,.T.);
#92166=ADVANCED_FACE('',(#12887),#3930,.T.);
#92167=ADVANCED_FACE('',(#12888),#3931,.T.);
#92168=ADVANCED_FACE('',(#12889),#87218,.T.);
#92169=ADVANCED_FACE('',(#12890),#87219,.T.);
#92170=ADVANCED_FACE('',(#12891),#87220,.T.);
#92171=ADVANCED_FACE('',(#12892),#87221,.T.);
#92172=ADVANCED_FACE('',(#12893),#3932,.T.);
#92173=ADVANCED_FACE('',(#12894),#3933,.T.);
#92174=ADVANCED_FACE('',(#12895),#87222,.T.);
#92175=ADVANCED_FACE('',(#12896),#3934,.F.);
#92176=ADVANCED_FACE('',(#12897),#87223,.F.);
#92177=ADVANCED_FACE('',(#12898),#3935,.F.);
#92178=ADVANCED_FACE('',(#12899,#7600,#7601),#8381,.F.);
#92179=ADVANCED_FACE('',(#12900),#87224,.T.);
#92180=ADVANCED_FACE('',(#12901),#87225,.T.);
#92181=ADVANCED_FACE('',(#12902),#87226,.F.);
#92182=ADVANCED_FACE('',(#12903),#8382,.F.);
#92183=ADVANCED_FACE('',(#12904),#87227,.T.);
#92184=ADVANCED_FACE('',(#12905),#8383,.T.);
#92185=ADVANCED_FACE('',(#12906),#87228,.T.);
#92186=ADVANCED_FACE('',(#12907),#8384,.F.);
#92187=ADVANCED_FACE('',(#12908),#87229,.F.);
#92188=ADVANCED_FACE('',(#12909,#7602),#8385,.F.);
#92189=ADVANCED_FACE('',(#12910),#8386,.F.);
#92190=ADVANCED_FACE('',(#12911),#8387,.F.);
#92191=ADVANCED_FACE('',(#12912),#87230,.F.);
#92192=ADVANCED_FACE('',(#12913),#87231,.F.);
#92193=ADVANCED_FACE('',(#12914),#8388,.F.);
#92194=ADVANCED_FACE('',(#12915),#8389,.F.);
#92195=ADVANCED_FACE('',(#12916,#7603),#1027,.T.);
#92196=ADVANCED_FACE('',(#12917),#3936,.T.);
#92197=ADVANCED_FACE('',(#12918),#3937,.T.);
#92198=ADVANCED_FACE('',(#12919),#8390,.F.);
#92199=ADVANCED_FACE('',(#12920),#8391,.F.);
#92200=ADVANCED_FACE('',(#12921),#7121,.F.);
#92201=ADVANCED_FACE('',(#12922),#8392,.F.);
#92202=ADVANCED_FACE('',(#12923),#7122,.F.);
#92203=ADVANCED_FACE('',(#12924),#8393,.T.);
#92204=ADVANCED_FACE('',(#12925),#87232,.T.);
#92205=ADVANCED_FACE('',(#12926),#87233,.T.);
#92206=ADVANCED_FACE('',(#12927,#7604),#8394,.T.);
#92207=ADVANCED_FACE('',(#12928),#87234,.T.);
#92208=ADVANCED_FACE('',(#12929),#3938,.T.);
#92209=ADVANCED_FACE('',(#12930),#87235,.T.);
#92210=ADVANCED_FACE('',(#12931),#3939,.T.);
#92211=ADVANCED_FACE('',(#12932),#87236,.T.);
#92212=ADVANCED_FACE('',(#12933),#87237,.T.);
#92213=ADVANCED_FACE('',(#12934),#3940,.T.);
#92214=ADVANCED_FACE('',(#12935),#87238,.T.);
#92215=ADVANCED_FACE('',(#12936),#3941,.T.);
#92216=ADVANCED_FACE('',(#12937),#87239,.T.);
#92217=ADVANCED_FACE('',(#12938),#87240,.T.);
#92218=ADVANCED_FACE('',(#12939),#3942,.T.);
#92219=ADVANCED_FACE('',(#12940),#87241,.T.);
#92220=ADVANCED_FACE('',(#12941),#3943,.T.);
#92221=ADVANCED_FACE('',(#12942),#87242,.T.);
#92222=ADVANCED_FACE('',(#12943),#3944,.T.);
#92223=ADVANCED_FACE('',(#12944),#87243,.T.);
#92224=ADVANCED_FACE('',(#12945),#3945,.T.);
#92225=ADVANCED_FACE('',(#12946),#87244,.T.);
#92226=ADVANCED_FACE('',(#12947),#87245,.T.);
#92227=ADVANCED_FACE('',(#12948),#3946,.T.);
#92228=ADVANCED_FACE('',(#12949),#87246,.T.);
#92229=ADVANCED_FACE('',(#12950),#3947,.T.);
#92230=ADVANCED_FACE('',(#12951),#87247,.T.);
#92231=ADVANCED_FACE('',(#12952),#87248,.T.);
#92232=ADVANCED_FACE('',(#12953),#3948,.T.);
#92233=ADVANCED_FACE('',(#12954),#87249,.T.);
#92234=ADVANCED_FACE('',(#12955),#3949,.T.);
#92235=ADVANCED_FACE('',(#12956),#3950,.T.);
#92236=ADVANCED_FACE('',(#12957),#87250,.T.);
#92237=ADVANCED_FACE('',(#12958),#3951,.T.);
#92238=ADVANCED_FACE('',(#12959),#87251,.T.);
#92239=ADVANCED_FACE('',(#12960),#3952,.T.);
#92240=ADVANCED_FACE('',(#12961),#87252,.T.);
#92241=ADVANCED_FACE('',(#12962),#87253,.T.);
#92242=ADVANCED_FACE('',(#12963),#3953,.T.);
#92243=ADVANCED_FACE('',(#12964),#87254,.T.);
#92244=ADVANCED_FACE('',(#12965),#3954,.T.);
#92245=ADVANCED_FACE('',(#12966),#3955,.T.);
#92246=ADVANCED_FACE('',(#12967),#3956,.T.);
#92247=ADVANCED_FACE('',(#12968),#87255,.T.);
#92248=ADVANCED_FACE('',(#12969),#3957,.T.);
#92249=ADVANCED_FACE('',(#12970),#87256,.T.);
#92250=ADVANCED_FACE('',(#12971),#87257,.T.);
#92251=ADVANCED_FACE('',(#12972),#3958,.T.);
#92252=ADVANCED_FACE('',(#12973),#87258,.T.);
#92253=ADVANCED_FACE('',(#12974),#3959,.T.);
#92254=ADVANCED_FACE('',(#12975),#3960,.T.);
#92255=ADVANCED_FACE('',(#12976),#3961,.T.);
#92256=ADVANCED_FACE('',(#12977),#87259,.T.);
#92257=ADVANCED_FACE('',(#12978),#3962,.T.);
#92258=ADVANCED_FACE('',(#12979),#87260,.T.);
#92259=ADVANCED_FACE('',(#12980),#87261,.T.);
#92260=ADVANCED_FACE('',(#12981),#3963,.T.);
#92261=ADVANCED_FACE('',(#12982),#87262,.T.);
#92262=ADVANCED_FACE('',(#12983),#3964,.T.);
#92263=ADVANCED_FACE('',(#12984),#3965,.T.);
#92264=ADVANCED_FACE('',(#12985),#3966,.T.);
#92265=ADVANCED_FACE('',(#12986),#87263,.T.);
#92266=ADVANCED_FACE('',(#12987),#3967,.T.);
#92267=ADVANCED_FACE('',(#12988),#87264,.T.);
#92268=ADVANCED_FACE('',(#12989),#87265,.T.);
#92269=ADVANCED_FACE('',(#12990),#3968,.T.);
#92270=ADVANCED_FACE('',(#12991),#87266,.T.);
#92271=ADVANCED_FACE('',(#12992),#3969,.T.);
#92272=ADVANCED_FACE('',(#12993),#3970,.T.);
#92273=ADVANCED_FACE('',(#12994),#3971,.T.);
#92274=ADVANCED_FACE('',(#12995),#87267,.T.);
#92275=ADVANCED_FACE('',(#12996),#3972,.T.);
#92276=ADVANCED_FACE('',(#12997),#87268,.T.);
#92277=ADVANCED_FACE('',(#12998),#87269,.T.);
#92278=ADVANCED_FACE('',(#12999),#3973,.T.);
#92279=ADVANCED_FACE('',(#13000),#87270,.T.);
#92280=ADVANCED_FACE('',(#13001),#3974,.T.);
#92281=ADVANCED_FACE('',(#13002),#3975,.T.);
#92282=ADVANCED_FACE('',(#13003),#3976,.T.);
#92283=ADVANCED_FACE('',(#13004),#87271,.T.);
#92284=ADVANCED_FACE('',(#13005),#3977,.T.);
#92285=ADVANCED_FACE('',(#13006),#87272,.T.);
#92286=ADVANCED_FACE('',(#13007),#87273,.T.);
#92287=ADVANCED_FACE('',(#13008),#3978,.T.);
#92288=ADVANCED_FACE('',(#13009),#87274,.T.);
#92289=ADVANCED_FACE('',(#13010),#3979,.T.);
#92290=ADVANCED_FACE('',(#13011),#3980,.T.);
#92291=ADVANCED_FACE('',(#13012),#3981,.T.);
#92292=ADVANCED_FACE('',(#13013),#87275,.T.);
#92293=ADVANCED_FACE('',(#13014),#3982,.T.);
#92294=ADVANCED_FACE('',(#13015),#87276,.T.);
#92295=ADVANCED_FACE('',(#13016),#87277,.T.);
#92296=ADVANCED_FACE('',(#13017),#3983,.T.);
#92297=ADVANCED_FACE('',(#13018),#87278,.T.);
#92298=ADVANCED_FACE('',(#13019),#3984,.T.);
#92299=ADVANCED_FACE('',(#13020),#87279,.T.);
#92300=ADVANCED_FACE('',(#13021),#3985,.T.);
#92301=ADVANCED_FACE('',(#13022),#3986,.T.);
#92302=ADVANCED_FACE('',(#13023),#87280,.T.);
#92303=ADVANCED_FACE('',(#13024),#3987,.T.);
#92304=ADVANCED_FACE('',(#13025),#87281,.T.);
#92305=ADVANCED_FACE('',(#13026),#87282,.T.);
#92306=ADVANCED_FACE('',(#13027),#3988,.T.);
#92307=ADVANCED_FACE('',(#13028),#87283,.T.);
#92308=ADVANCED_FACE('',(#13029),#3989,.T.);
#92309=ADVANCED_FACE('',(#13030),#87284,.T.);
#92310=ADVANCED_FACE('',(#13031),#3990,.T.);
#92311=ADVANCED_FACE('',(#13032),#87285,.T.);
#92312=ADVANCED_FACE('',(#13033),#3991,.T.);
#92313=ADVANCED_FACE('',(#13034),#87286,.T.);
#92314=ADVANCED_FACE('',(#13035),#87287,.T.);
#92315=ADVANCED_FACE('',(#13036),#3992,.T.);
#92316=ADVANCED_FACE('',(#13037),#87288,.T.);
#92317=ADVANCED_FACE('',(#13038),#3993,.T.);
#92318=ADVANCED_FACE('',(#13039),#87289,.T.);
#92319=ADVANCED_FACE('',(#13040),#87290,.F.);
#92320=ADVANCED_FACE('',(#13041),#87291,.F.);
#92321=ADVANCED_FACE('',(#13042),#87292,.F.);
#92322=ADVANCED_FACE('',(#13043),#87293,.F.);
#92323=ADVANCED_FACE('',(#13044),#87294,.F.);
#92324=ADVANCED_FACE('',(#13045),#87295,.F.);
#92325=ADVANCED_FACE('',(#13046),#87296,.F.);
#92326=ADVANCED_FACE('',(#13047),#87297,.F.);
#92327=ADVANCED_FACE('',(#13048),#87298,.F.);
#92328=ADVANCED_FACE('',(#13049),#87299,.F.);
#92329=ADVANCED_FACE('',(#13050),#87300,.F.);
#92330=ADVANCED_FACE('',(#13051),#87301,.F.);
#92331=ADVANCED_FACE('',(#13052),#87302,.F.);
#92332=ADVANCED_FACE('',(#13053),#87303,.F.);
#92333=ADVANCED_FACE('',(#13054),#87304,.F.);
#92334=ADVANCED_FACE('',(#13055),#87305,.F.);
#92335=ADVANCED_FACE('',(#13056),#87306,.F.);
#92336=ADVANCED_FACE('',(#13057),#87307,.F.);
#92337=ADVANCED_FACE('',(#13058),#87308,.F.);
#92338=ADVANCED_FACE('',(#13059),#87309,.F.);
#92339=ADVANCED_FACE('',(#13060),#87310,.F.);
#92340=ADVANCED_FACE('',(#13061),#87311,.F.);
#92341=ADVANCED_FACE('',(#13062),#87312,.F.);
#92342=ADVANCED_FACE('',(#13063),#87313,.F.);
#92343=ADVANCED_FACE('',(#13064),#87314,.F.);
#92344=ADVANCED_FACE('',(#13065),#87315,.F.);
#92345=ADVANCED_FACE('',(#13066),#8395,.T.);
#92346=ADVANCED_FACE('',(#13067),#8396,.F.);
#92347=ADVANCED_FACE('',(#13068),#87316,.T.);
#92348=ADVANCED_FACE('',(#13069),#8397,.F.);
#92349=ADVANCED_FACE('',(#13070),#8398,.F.);
#92350=ADVANCED_FACE('',(#13071),#8399,.F.);
#92351=ADVANCED_FACE('',(#13072),#8400,.F.);
#92352=ADVANCED_FACE('',(#13073),#8401,.F.);
#92353=ADVANCED_FACE('',(#13074),#8402,.F.);
#92354=ADVANCED_FACE('',(#13075),#8403,.F.);
#92355=ADVANCED_FACE('',(#13076),#8404,.F.);
#92356=ADVANCED_FACE('',(#13077),#8405,.F.);
#92357=ADVANCED_FACE('',(#13078),#8406,.F.);
#92358=ADVANCED_FACE('',(#13079),#8407,.F.);
#92359=ADVANCED_FACE('',(#13080),#8408,.F.);
#92360=ADVANCED_FACE('',(#13081),#8409,.F.);
#92361=ADVANCED_FACE('',(#13082),#8410,.F.);
#92362=ADVANCED_FACE('',(#13083),#87317,.T.);
#92363=ADVANCED_FACE('',(#13084),#87318,.T.);
#92364=ADVANCED_FACE('',(#13085),#8411,.F.);
#92365=ADVANCED_FACE('',(#13086),#8412,.F.);
#92366=ADVANCED_FACE('',(#13087),#8413,.F.);
#92367=ADVANCED_FACE('',(#13088),#87319,.T.);
#92368=ADVANCED_FACE('',(#13089),#87320,.T.);
#92369=ADVANCED_FACE('',(#13090),#8414,.F.);
#92370=ADVANCED_FACE('',(#13091),#8415,.F.);
#92371=ADVANCED_FACE('',(#13092),#8416,.F.);
#92372=ADVANCED_FACE('',(#13093),#87321,.T.);
#92373=ADVANCED_FACE('',(#13094),#87322,.T.);
#92374=ADVANCED_FACE('',(#13095),#8417,.F.);
#92375=ADVANCED_FACE('',(#13096),#8418,.F.);
#92376=ADVANCED_FACE('',(#13097),#8419,.F.);
#92377=ADVANCED_FACE('',(#13098),#87323,.T.);
#92378=ADVANCED_FACE('',(#13099),#87324,.T.);
#92379=ADVANCED_FACE('',(#13100),#8420,.F.);
#92380=ADVANCED_FACE('',(#13101),#8421,.F.);
#92381=ADVANCED_FACE('',(#13102),#8422,.F.);
#92382=ADVANCED_FACE('',(#13103),#87325,.T.);
#92383=ADVANCED_FACE('',(#13104),#8423,.T.);
#92384=ADVANCED_FACE('',(#13105),#87326,.F.);
#92385=ADVANCED_FACE('',(#13106),#8424,.T.);
#92386=ADVANCED_FACE('',(#13107),#87327,.F.);
#92387=ADVANCED_FACE('',(#13108),#8425,.F.);
#92388=ADVANCED_FACE('',(#13109),#8426,.F.);
#92389=ADVANCED_FACE('',(#13110),#8427,.T.);
#92390=ADVANCED_FACE('',(#13111),#8428,.F.);
#92391=ADVANCED_FACE('',(#13112),#87328,.T.);
#92392=ADVANCED_FACE('',(#13113),#8429,.F.);
#92393=ADVANCED_FACE('',(#13114),#87329,.T.);
#92394=ADVANCED_FACE('',(#13115),#8430,.F.);
#92395=ADVANCED_FACE('',(#13116),#87330,.T.);
#92396=ADVANCED_FACE('',(#13117),#8431,.F.);
#92397=ADVANCED_FACE('',(#13118),#87331,.T.);
#92398=ADVANCED_FACE('',(#13119),#8432,.F.);
#92399=ADVANCED_FACE('',(#13120),#87332,.T.);
#92400=ADVANCED_FACE('',(#13121),#87333,.T.);
#92401=ADVANCED_FACE('',(#13122),#8433,.F.);
#92402=ADVANCED_FACE('',(#13123),#87334,.T.);
#92403=ADVANCED_FACE('',(#13124),#8434,.T.);
#92404=ADVANCED_FACE('',(#13125),#87335,.T.);
#92405=ADVANCED_FACE('',(#13126),#8435,.F.);
#92406=ADVANCED_FACE('',(#13127),#8436,.F.);
#92407=ADVANCED_FACE('',(#13128),#8437,.F.);
#92408=ADVANCED_FACE('',(#13129),#8438,.T.);
#92409=ADVANCED_FACE('',(#13130),#8439,.F.);
#92410=ADVANCED_FACE('',(#13131),#8440,.F.);
#92411=ADVANCED_FACE('',(#13132),#87336,.T.);
#92412=ADVANCED_FACE('',(#13133),#8441,.F.);
#92413=ADVANCED_FACE('',(#13134),#8442,.F.);
#92414=ADVANCED_FACE('',(#13135),#8443,.F.);
#92415=ADVANCED_FACE('',(#13136),#87337,.T.);
#92416=ADVANCED_FACE('',(#13137),#8444,.T.);
#92417=ADVANCED_FACE('',(#13138),#7123,.T.);
#92418=ADVANCED_FACE('',(#13139),#7124,.T.);
#92419=ADVANCED_FACE('',(#13140),#7125,.T.);
#92420=ADVANCED_FACE('',(#13141),#7126,.T.);
#92421=ADVANCED_FACE('',(#13142),#7127,.T.);
#92422=ADVANCED_FACE('',(#13143),#7128,.T.);
#92423=ADVANCED_FACE('',(#13144),#8445,.F.);
#92424=ADVANCED_FACE('',(#13145),#7129,.T.);
#92425=ADVANCED_FACE('',(#13146),#7130,.T.);
#92426=ADVANCED_FACE('',(#13147),#7131,.T.);
#92427=ADVANCED_FACE('',(#13148),#7132,.T.);
#92428=ADVANCED_FACE('',(#13149),#7133,.T.);
#92429=ADVANCED_FACE('',(#13150),#7134,.T.);
#92430=ADVANCED_FACE('',(#13151),#8446,.F.);
#92431=ADVANCED_FACE('',(#13152),#8447,.F.);
#92432=ADVANCED_FACE('',(#13153),#8448,.F.);
#92433=ADVANCED_FACE('',(#13154),#8449,.F.);
#92434=ADVANCED_FACE('',(#13155),#8450,.F.);
#92435=ADVANCED_FACE('',(#13156),#8451,.F.);
#92436=ADVANCED_FACE('',(#13157),#8452,.T.);
#92437=ADVANCED_FACE('',(#13158),#7135,.T.);
#92438=ADVANCED_FACE('',(#13159),#7136,.T.);
#92439=ADVANCED_FACE('',(#13160),#7137,.T.);
#92440=ADVANCED_FACE('',(#13161),#7138,.T.);
#92441=ADVANCED_FACE('',(#13162),#7139,.T.);
#92442=ADVANCED_FACE('',(#13163),#7140,.T.);
#92443=ADVANCED_FACE('',(#13164),#8453,.F.);
#92444=ADVANCED_FACE('',(#13165),#7141,.T.);
#92445=ADVANCED_FACE('',(#13166),#7142,.T.);
#92446=ADVANCED_FACE('',(#13167),#7143,.T.);
#92447=ADVANCED_FACE('',(#13168),#7144,.T.);
#92448=ADVANCED_FACE('',(#13169),#7145,.T.);
#92449=ADVANCED_FACE('',(#13170),#7146,.T.);
#92450=ADVANCED_FACE('',(#13171),#8454,.F.);
#92451=ADVANCED_FACE('',(#13172),#8455,.F.);
#92452=ADVANCED_FACE('',(#13173),#8456,.F.);
#92453=ADVANCED_FACE('',(#13174),#8457,.F.);
#92454=ADVANCED_FACE('',(#13175),#8458,.F.);
#92455=ADVANCED_FACE('',(#13176),#8459,.F.);
#92456=ADVANCED_FACE('',(#13177),#8460,.F.);
#92457=ADVANCED_FACE('',(#13178),#8461,.F.);
#92458=ADVANCED_FACE('',(#13179),#8462,.F.);
#92459=ADVANCED_FACE('',(#13180),#8463,.F.);
#92460=ADVANCED_FACE('',(#13181),#8464,.F.);
#92461=ADVANCED_FACE('',(#13182),#8465,.F.);
#92462=ADVANCED_FACE('',(#13183),#7147,.F.);
#92463=ADVANCED_FACE('',(#13184),#7148,.F.);
#92464=ADVANCED_FACE('',(#13185),#7149,.F.);
#92465=ADVANCED_FACE('',(#13186),#7150,.F.);
#92466=ADVANCED_FACE('',(#13187),#7151,.F.);
#92467=ADVANCED_FACE('',(#13188),#7152,.F.);
#92468=ADVANCED_FACE('',(#13189),#7153,.F.);
#92469=ADVANCED_FACE('',(#13190),#3994,.T.);
#92470=ADVANCED_FACE('',(#13191),#8466,.F.);
#92471=ADVANCED_FACE('',(#13192,#7605),#8467,.T.);
#92472=ADVANCED_FACE('',(#13193),#87338,.T.);
#92473=ADVANCED_FACE('',(#13194),#87339,.T.);
#92474=ADVANCED_FACE('',(#13195),#87340,.T.);
#92475=ADVANCED_FACE('',(#13196),#1028,.T.);
#92476=ADVANCED_FACE('',(#13197),#87341,.T.);
#92477=ADVANCED_FACE('',(#13198),#1029,.T.);
#92478=ADVANCED_FACE('',(#13199),#3995,.T.);
#92479=ADVANCED_FACE('',(#13200),#1030,.T.);
#92480=ADVANCED_FACE('',(#13201),#3996,.T.);
#92481=ADVANCED_FACE('',(#13202),#3997,.T.);
#92482=ADVANCED_FACE('',(#13203),#1031,.T.);
#92483=ADVANCED_FACE('',(#13204),#3998,.T.);
#92484=ADVANCED_FACE('',(#13205),#3999,.T.);
#92485=ADVANCED_FACE('',(#13206),#4000,.T.);
#92486=ADVANCED_FACE('',(#13207),#87342,.F.);
#92487=ADVANCED_FACE('',(#13208),#87343,.F.);
#92488=ADVANCED_FACE('',(#13209),#8468,.F.);
#92489=ADVANCED_FACE('',(#13210),#8469,.F.);
#92490=ADVANCED_FACE('',(#13211),#8470,.F.);
#92491=ADVANCED_FACE('',(#13212),#87344,.T.);
#92492=ADVANCED_FACE('',(#13213),#87345,.T.);
#92493=ADVANCED_FACE('',(#13214),#1032,.T.);
#92494=ADVANCED_FACE('',(#13215),#87346,.T.);
#92495=ADVANCED_FACE('',(#13216),#1033,.T.);
#92496=ADVANCED_FACE('',(#13217),#4001,.T.);
#92497=ADVANCED_FACE('',(#13218),#1034,.T.);
#92498=ADVANCED_FACE('',(#13219),#4002,.T.);
#92499=ADVANCED_FACE('',(#13220),#4003,.T.);
#92500=ADVANCED_FACE('',(#13221),#1035,.T.);
#92501=ADVANCED_FACE('',(#13222),#4004,.T.);
#92502=ADVANCED_FACE('',(#13223),#4005,.T.);
#92503=ADVANCED_FACE('',(#13224),#4006,.T.);
#92504=ADVANCED_FACE('',(#13225),#87347,.F.);
#92505=ADVANCED_FACE('',(#13226),#87348,.F.);
#92506=ADVANCED_FACE('',(#13227),#8471,.F.);
#92507=ADVANCED_FACE('',(#13228),#8472,.F.);
#92508=ADVANCED_FACE('',(#13229),#8473,.T.);
#92509=ADVANCED_FACE('',(#13230),#8474,.T.);
#92510=ADVANCED_FACE('',(#13231),#8475,.F.);
#92511=ADVANCED_FACE('',(#13232),#87349,.T.);
#92512=ADVANCED_FACE('',(#13233),#3124,.T.);
#92513=ADVANCED_FACE('',(#13234),#87350,.T.);
#92514=ADVANCED_FACE('',(#13235),#4007,.T.);
#92515=ADVANCED_FACE('',(#13236),#87351,.T.);
#92516=ADVANCED_FACE('',(#13237),#87352,.T.);
#92517=ADVANCED_FACE('',(#13238),#4008,.T.);
#92518=ADVANCED_FACE('',(#13239),#87353,.T.);
#92519=ADVANCED_FACE('',(#13240),#87354,.T.);
#92520=ADVANCED_FACE('',(#13241),#87355,.T.);
#92521=ADVANCED_FACE('',(#13242),#8476,.T.);
#92522=ADVANCED_FACE('',(#13243),#87356,.T.);
#92523=ADVANCED_FACE('',(#13244),#3125,.T.);
#92524=ADVANCED_FACE('',(#13245),#87357,.T.);
#92525=ADVANCED_FACE('',(#13246),#87358,.T.);
#92526=ADVANCED_FACE('',(#13247),#4009,.T.);
#92527=ADVANCED_FACE('',(#13248),#87359,.T.);
#92528=ADVANCED_FACE('',(#13249),#87360,.T.);
#92529=ADVANCED_FACE('',(#13250),#4010,.T.);
#92530=ADVANCED_FACE('',(#13251),#87361,.T.);
#92531=ADVANCED_FACE('',(#13252),#8477,.T.);
#92532=ADVANCED_FACE('',(#13253),#8478,.F.);
#92533=ADVANCED_FACE('',(#13254),#8479,.F.);
#92534=ADVANCED_FACE('',(#13255),#87362,.T.);
#92535=ADVANCED_FACE('',(#13256),#87363,.T.);
#92536=ADVANCED_FACE('',(#13257),#87364,.F.);
#92537=ADVANCED_FACE('',(#13258),#87365,.F.);
#92538=ADVANCED_FACE('',(#13259),#87366,.F.);
#92539=ADVANCED_FACE('',(#13260),#87367,.F.);
#92540=ADVANCED_FACE('',(#13261),#87368,.F.);
#92541=ADVANCED_FACE('',(#13262),#87369,.F.);
#92542=ADVANCED_FACE('',(#13263),#87370,.F.);
#92543=ADVANCED_FACE('',(#13264),#87371,.F.);
#92544=ADVANCED_FACE('',(#13265),#87372,.F.);
#92545=ADVANCED_FACE('',(#13266),#87373,.F.);
#92546=ADVANCED_FACE('',(#13267),#87374,.F.);
#92547=ADVANCED_FACE('',(#13268),#87375,.F.);
#92548=ADVANCED_FACE('',(#13269),#87376,.F.);
#92549=ADVANCED_FACE('',(#13270),#87377,.F.);
#92550=ADVANCED_FACE('',(#13271),#87378,.F.);
#92551=ADVANCED_FACE('',(#13272),#87379,.F.);
#92552=ADVANCED_FACE('',(#13273),#87380,.F.);
#92553=ADVANCED_FACE('',(#13274),#87381,.F.);
#92554=ADVANCED_FACE('',(#13275),#87382,.F.);
#92555=ADVANCED_FACE('',(#13276),#87383,.F.);
#92556=ADVANCED_FACE('',(#13277),#87384,.F.);
#92557=ADVANCED_FACE('',(#13278),#87385,.F.);
#92558=ADVANCED_FACE('',(#13279),#87386,.F.);
#92559=ADVANCED_FACE('',(#13280),#87387,.F.);
#92560=ADVANCED_FACE('',(#13281),#87388,.F.);
#92561=ADVANCED_FACE('',(#13282),#87389,.F.);
#92562=ADVANCED_FACE('',(#13283),#87390,.F.);
#92563=ADVANCED_FACE('',(#13284),#87391,.F.);
#92564=ADVANCED_FACE('',(#13285),#87392,.F.);
#92565=ADVANCED_FACE('',(#13286),#87393,.F.);
#92566=ADVANCED_FACE('',(#13287),#87394,.F.);
#92567=ADVANCED_FACE('',(#13288),#87395,.F.);
#92568=ADVANCED_FACE('',(#13289),#87396,.F.);
#92569=ADVANCED_FACE('',(#13290),#87397,.F.);
#92570=ADVANCED_FACE('',(#13291),#87398,.F.);
#92571=ADVANCED_FACE('',(#13292),#87399,.F.);
#92572=ADVANCED_FACE('',(#13293),#87400,.F.);
#92573=ADVANCED_FACE('',(#13294),#87401,.F.);
#92574=ADVANCED_FACE('',(#13295),#87402,.F.);
#92575=ADVANCED_FACE('',(#13296),#87403,.F.);
#92576=ADVANCED_FACE('',(#13297),#87404,.F.);
#92577=ADVANCED_FACE('',(#13298),#87405,.F.);
#92578=ADVANCED_FACE('',(#13299),#87406,.F.);
#92579=ADVANCED_FACE('',(#13300),#87407,.F.);
#92580=ADVANCED_FACE('',(#13301),#87408,.F.);
#92581=ADVANCED_FACE('',(#13302),#87409,.F.);
#92582=ADVANCED_FACE('',(#13303),#87410,.F.);
#92583=ADVANCED_FACE('',(#13304),#87411,.F.);
#92584=ADVANCED_FACE('',(#13305),#87412,.F.);
#92585=ADVANCED_FACE('',(#13306),#87413,.F.);
#92586=ADVANCED_FACE('',(#13307),#87414,.F.);
#92587=ADVANCED_FACE('',(#13308),#87415,.F.);
#92588=ADVANCED_FACE('',(#13309),#87416,.F.);
#92589=ADVANCED_FACE('',(#13310),#87417,.F.);
#92590=ADVANCED_FACE('',(#13311),#87418,.F.);
#92591=ADVANCED_FACE('',(#13312),#87419,.F.);
#92592=ADVANCED_FACE('',(#13313),#87420,.F.);
#92593=ADVANCED_FACE('',(#13314),#87421,.F.);
#92594=ADVANCED_FACE('',(#13315),#87422,.F.);
#92595=ADVANCED_FACE('',(#13316),#87423,.F.);
#92596=ADVANCED_FACE('',(#13317),#87424,.F.);
#92597=ADVANCED_FACE('',(#13318),#87425,.F.);
#92598=ADVANCED_FACE('',(#13319),#87426,.F.);
#92599=ADVANCED_FACE('',(#13320),#87427,.F.);
#92600=ADVANCED_FACE('',(#13321),#87428,.F.);
#92601=ADVANCED_FACE('',(#13322),#87429,.F.);
#92602=ADVANCED_FACE('',(#13323),#87430,.F.);
#92603=ADVANCED_FACE('',(#13324),#87431,.F.);
#92604=ADVANCED_FACE('',(#13325),#87432,.F.);
#92605=ADVANCED_FACE('',(#13326),#87433,.F.);
#92606=ADVANCED_FACE('',(#13327),#87434,.F.);
#92607=ADVANCED_FACE('',(#13328),#87435,.F.);
#92608=ADVANCED_FACE('',(#13329),#87436,.F.);
#92609=ADVANCED_FACE('',(#13330),#87437,.F.);
#92610=ADVANCED_FACE('',(#13331),#87438,.F.);
#92611=ADVANCED_FACE('',(#13332),#87439,.F.);
#92612=ADVANCED_FACE('',(#13333),#87440,.F.);
#92613=ADVANCED_FACE('',(#13334),#87441,.F.);
#92614=ADVANCED_FACE('',(#13335),#87442,.F.);
#92615=ADVANCED_FACE('',(#13336),#87443,.F.);
#92616=ADVANCED_FACE('',(#13337),#87444,.F.);
#92617=ADVANCED_FACE('',(#13338),#87445,.F.);
#92618=ADVANCED_FACE('',(#13339),#87446,.F.);
#92619=ADVANCED_FACE('',(#13340),#87447,.F.);
#92620=ADVANCED_FACE('',(#13341),#87448,.F.);
#92621=ADVANCED_FACE('',(#13342),#87449,.F.);
#92622=ADVANCED_FACE('',(#13343),#87450,.F.);
#92623=ADVANCED_FACE('',(#13344),#87451,.F.);
#92624=ADVANCED_FACE('',(#13345),#87452,.F.);
#92625=ADVANCED_FACE('',(#13346),#87453,.F.);
#92626=ADVANCED_FACE('',(#13347),#87454,.F.);
#92627=ADVANCED_FACE('',(#13348),#87455,.F.);
#92628=ADVANCED_FACE('',(#13349),#87456,.F.);
#92629=ADVANCED_FACE('',(#13350),#87457,.F.);
#92630=ADVANCED_FACE('',(#13351),#87458,.F.);
#92631=ADVANCED_FACE('',(#13352),#87459,.F.);
#92632=ADVANCED_FACE('',(#13353),#87460,.F.);
#92633=ADVANCED_FACE('',(#13354),#87461,.F.);
#92634=ADVANCED_FACE('',(#13355),#87462,.F.);
#92635=ADVANCED_FACE('',(#13356),#87463,.F.);
#92636=ADVANCED_FACE('',(#13357),#87464,.F.);
#92637=ADVANCED_FACE('',(#13358),#87465,.F.);
#92638=ADVANCED_FACE('',(#13359),#87466,.F.);
#92639=ADVANCED_FACE('',(#13360),#87467,.F.);
#92640=ADVANCED_FACE('',(#13361),#87468,.F.);
#92641=ADVANCED_FACE('',(#13362),#87469,.F.);
#92642=ADVANCED_FACE('',(#13363),#87470,.F.);
#92643=ADVANCED_FACE('',(#13364),#87471,.F.);
#92644=ADVANCED_FACE('',(#13365),#87472,.F.);
#92645=ADVANCED_FACE('',(#13366),#87473,.F.);
#92646=ADVANCED_FACE('',(#13367),#87474,.F.);
#92647=ADVANCED_FACE('',(#13368),#87475,.F.);
#92648=ADVANCED_FACE('',(#13369),#87476,.F.);
#92649=ADVANCED_FACE('',(#13370),#87477,.F.);
#92650=ADVANCED_FACE('',(#13371),#87478,.F.);
#92651=ADVANCED_FACE('',(#13372),#87479,.F.);
#92652=ADVANCED_FACE('',(#13373),#87480,.F.);
#92653=ADVANCED_FACE('',(#13374),#87481,.F.);
#92654=ADVANCED_FACE('',(#13375),#87482,.F.);
#92655=ADVANCED_FACE('',(#13376),#87483,.F.);
#92656=ADVANCED_FACE('',(#13377),#87484,.F.);
#92657=ADVANCED_FACE('',(#13378),#87485,.F.);
#92658=ADVANCED_FACE('',(#13379),#87486,.F.);
#92659=ADVANCED_FACE('',(#13380),#87487,.F.);
#92660=ADVANCED_FACE('',(#13381),#87488,.F.);
#92661=ADVANCED_FACE('',(#13382),#87489,.F.);
#92662=ADVANCED_FACE('',(#13383),#87490,.F.);
#92663=ADVANCED_FACE('',(#13384),#87491,.F.);
#92664=ADVANCED_FACE('',(#13385),#87492,.F.);
#92665=ADVANCED_FACE('',(#13386),#87493,.F.);
#92666=ADVANCED_FACE('',(#13387),#87494,.F.);
#92667=ADVANCED_FACE('',(#13388),#87495,.F.);
#92668=ADVANCED_FACE('',(#13389),#87496,.F.);
#92669=ADVANCED_FACE('',(#13390),#87497,.F.);
#92670=ADVANCED_FACE('',(#13391),#87498,.F.);
#92671=ADVANCED_FACE('',(#13392),#87499,.F.);
#92672=ADVANCED_FACE('',(#13393),#87500,.F.);
#92673=ADVANCED_FACE('',(#13394),#87501,.F.);
#92674=ADVANCED_FACE('',(#13395),#87502,.F.);
#92675=ADVANCED_FACE('',(#13396),#87503,.F.);
#92676=ADVANCED_FACE('',(#13397),#87504,.F.);
#92677=ADVANCED_FACE('',(#13398),#87505,.F.);
#92678=ADVANCED_FACE('',(#13399),#87506,.F.);
#92679=ADVANCED_FACE('',(#13400),#87507,.F.);
#92680=ADVANCED_FACE('',(#13401),#87508,.F.);
#92681=ADVANCED_FACE('',(#13402),#87509,.F.);
#92682=ADVANCED_FACE('',(#13403),#87510,.F.);
#92683=ADVANCED_FACE('',(#13404),#87511,.F.);
#92684=ADVANCED_FACE('',(#13405),#87512,.F.);
#92685=ADVANCED_FACE('',(#13406),#87513,.F.);
#92686=ADVANCED_FACE('',(#13407),#87514,.F.);
#92687=ADVANCED_FACE('',(#13408),#8480,.F.);
#92688=ADVANCED_FACE('',(#13409),#8481,.F.);
#92689=ADVANCED_FACE('',(#13410),#8482,.F.);
#92690=ADVANCED_FACE('',(#13411),#8483,.F.);
#92691=ADVANCED_FACE('',(#13412),#8484,.F.);
#92692=ADVANCED_FACE('',(#13413),#8485,.F.);
#92693=ADVANCED_FACE('',(#13414),#8486,.T.);
#92694=ADVANCED_FACE('',(#13415,#7606,#7607,#7608),#8487,.T.);
#92695=ADVANCED_FACE('',(#13416,#7609),#8488,.T.);
#92696=ADVANCED_FACE('',(#13417),#87515,.F.);
#92697=ADVANCED_FACE('',(#13418),#87516,.T.);
#92698=ADVANCED_FACE('',(#13419),#8489,.T.);
#92699=ADVANCED_FACE('',(#13420,#7610),#8490,.T.);
#92700=ADVANCED_FACE('',(#13421),#87517,.F.);
#92701=ADVANCED_FACE('',(#13422),#87518,.T.);
#92702=ADVANCED_FACE('',(#13423),#8491,.T.);
#92703=ADVANCED_FACE('',(#13424,#7611),#8492,.T.);
#92704=ADVANCED_FACE('',(#13425),#87519,.F.);
#92705=ADVANCED_FACE('',(#13426),#87520,.T.);
#92706=ADVANCED_FACE('',(#13427),#8493,.T.);
#92707=ADVANCED_FACE('',(#13428,#7612),#8494,.T.);
#92708=ADVANCED_FACE('',(#13429),#87521,.F.);
#92709=ADVANCED_FACE('',(#13430),#87522,.T.);
#92710=ADVANCED_FACE('',(#13431),#8495,.T.);
#92711=ADVANCED_FACE('',(#13432),#4011,.T.);
#92712=ADVANCED_FACE('',(#13433),#4012,.T.);
#92713=ADVANCED_FACE('',(#13434),#4013,.T.);
#92714=ADVANCED_FACE('',(#13435),#8496,.F.);
#92715=ADVANCED_FACE('',(#13436),#8497,.F.);
#92716=ADVANCED_FACE('',(#13437),#8498,.F.);
#92717=ADVANCED_FACE('',(#13438),#8499,.F.);
#92718=ADVANCED_FACE('',(#13439),#8500,.F.);
#92719=ADVANCED_FACE('',(#13440),#8501,.F.);
#92720=ADVANCED_FACE('',(#13441),#7154,.F.);
#92721=ADVANCED_FACE('',(#13442),#7155,.F.);
#92722=ADVANCED_FACE('',(#13443),#7156,.F.);
#92723=ADVANCED_FACE('',(#13444),#7157,.F.);
#92724=ADVANCED_FACE('',(#13445),#7158,.F.);
#92725=ADVANCED_FACE('',(#13446),#7159,.F.);
#92726=ADVANCED_FACE('',(#13447),#7160,.F.);
#92727=ADVANCED_FACE('',(#13448),#7161,.T.);
#92728=ADVANCED_FACE('',(#13449,#7613),#8502,.T.);
#92729=ADVANCED_FACE('',(#13450),#87523,.T.);
#92730=ADVANCED_FACE('',(#13451),#953,.F.);
#92731=ADVANCED_FACE('',(#13452),#3126,.F.);
#92732=ADVANCED_FACE('',(#13453),#954,.T.);
#92733=ADVANCED_FACE('',(#13454),#3127,.F.);
#92734=ADVANCED_FACE('',(#13455),#3128,.T.);
#92735=ADVANCED_FACE('',(#13456),#3129,.T.);
#92736=ADVANCED_FACE('',(#13457),#3130,.T.);
#92737=ADVANCED_FACE('',(#13458),#3131,.T.);
#92738=ADVANCED_FACE('',(#13459),#3132,.T.);
#92739=ADVANCED_FACE('',(#13460),#3133,.T.);
#92740=ADVANCED_FACE('',(#13461),#3134,.F.);
#92741=ADVANCED_FACE('',(#13462),#3135,.F.);
#92742=ADVANCED_FACE('',(#13463),#3136,.F.);
#92743=ADVANCED_FACE('',(#13464),#3137,.F.);
#92744=ADVANCED_FACE('',(#13465),#3138,.F.);
#92745=ADVANCED_FACE('',(#13466),#3139,.F.);
#92746=ADVANCED_FACE('',(#13467),#3140,.T.);
#92747=ADVANCED_FACE('',(#13468),#3141,.T.);
#92748=ADVANCED_FACE('',(#13469),#87524,.T.);
#92749=ADVANCED_FACE('',(#13470),#3142,.T.);
#92750=ADVANCED_FACE('',(#13471),#3143,.T.);
#92751=ADVANCED_FACE('',(#13472),#87525,.T.);
#92752=ADVANCED_FACE('',(#13473),#3144,.T.);
#92753=ADVANCED_FACE('',(#13474),#3145,.F.);
#92754=ADVANCED_FACE('',(#13475),#3146,.F.);
#92755=ADVANCED_FACE('',(#13476),#1036,.F.);
#92756=ADVANCED_FACE('',(#13477),#87526,.F.);
#92757=ADVANCED_FACE('',(#13478),#3147,.F.);
#92758=ADVANCED_FACE('',(#13479),#87527,.F.);
#92759=ADVANCED_FACE('',(#13480),#3148,.F.);
#92760=ADVANCED_FACE('',(#13481),#1037,.F.);
#92761=ADVANCED_FACE('',(#13482),#87528,.F.);
#92762=ADVANCED_FACE('',(#13483),#3149,.F.);
#92763=ADVANCED_FACE('',(#13484),#87529,.F.);
#92764=ADVANCED_FACE('',(#13485),#8503,.T.);
#92765=ADVANCED_FACE('',(#13486),#87530,.F.);
#92766=ADVANCED_FACE('',(#13487),#8504,.F.);
#92767=ADVANCED_FACE('',(#13488),#8505,.T.);
#92768=ADVANCED_FACE('',(#13489),#8506,.F.);
#92769=ADVANCED_FACE('',(#13490),#87531,.F.);
#92770=ADVANCED_FACE('',(#13491),#87532,.F.);
#92771=ADVANCED_FACE('',(#13492),#87533,.F.);
#92772=ADVANCED_FACE('',(#13493),#3150,.T.);
#92773=ADVANCED_FACE('',(#13494),#87534,.T.);
#92774=ADVANCED_FACE('',(#13495),#87535,.T.);
#92775=ADVANCED_FACE('',(#13496),#8507,.T.);
#92776=ADVANCED_FACE('',(#13497),#3151,.T.);
#92777=ADVANCED_FACE('',(#13498),#87536,.T.);
#92778=ADVANCED_FACE('',(#13499),#3152,.T.);
#92779=ADVANCED_FACE('',(#13500),#8508,.T.);
#92780=ADVANCED_FACE('',(#13501),#3153,.T.);
#92781=ADVANCED_FACE('',(#13502),#87537,.T.);
#92782=ADVANCED_FACE('',(#13503),#87538,.T.);
#92783=ADVANCED_FACE('',(#13504),#8509,.T.);
#92784=ADVANCED_FACE('',(#13505),#3154,.T.);
#92785=ADVANCED_FACE('',(#13506),#87539,.T.);
#92786=ADVANCED_FACE('',(#13507),#3155,.T.);
#92787=ADVANCED_FACE('',(#13508),#8510,.T.);
#92788=ADVANCED_FACE('',(#13509),#3156,.T.);
#92789=ADVANCED_FACE('',(#13510),#3157,.T.);
#92790=ADVANCED_FACE('',(#13511),#4014,.T.);
#92791=ADVANCED_FACE('',(#13512),#3158,.T.);
#92792=ADVANCED_FACE('',(#13513),#4015,.T.);
#92793=ADVANCED_FACE('',(#13514),#3159,.T.);
#92794=ADVANCED_FACE('',(#13515),#87540,.F.);
#92795=ADVANCED_FACE('',(#13516),#87541,.F.);
#92796=ADVANCED_FACE('',(#13517),#87542,.F.);
#92797=ADVANCED_FACE('',(#13518),#87543,.F.);
#92798=ADVANCED_FACE('',(#13519),#87544,.T.);
#92799=ADVANCED_FACE('',(#13520),#3160,.T.);
#92800=ADVANCED_FACE('',(#13521),#87545,.T.);
#92801=ADVANCED_FACE('',(#13522),#87546,.T.);
#92802=ADVANCED_FACE('',(#13523),#8511,.T.);
#92803=ADVANCED_FACE('',(#13524),#3161,.T.);
#92804=ADVANCED_FACE('',(#13525),#87547,.T.);
#92805=ADVANCED_FACE('',(#13526),#3162,.T.);
#92806=ADVANCED_FACE('',(#13527),#8512,.T.);
#92807=ADVANCED_FACE('',(#13528),#3163,.T.);
#92808=ADVANCED_FACE('',(#13529),#87548,.T.);
#92809=ADVANCED_FACE('',(#13530),#3164,.T.);
#92810=ADVANCED_FACE('',(#13531),#87549,.T.);
#92811=ADVANCED_FACE('',(#13532),#87550,.T.);
#92812=ADVANCED_FACE('',(#13533),#8513,.T.);
#92813=ADVANCED_FACE('',(#13534),#3165,.T.);
#92814=ADVANCED_FACE('',(#13535),#87551,.T.);
#92815=ADVANCED_FACE('',(#13536),#3166,.T.);
#92816=ADVANCED_FACE('',(#13537),#8514,.T.);
#92817=ADVANCED_FACE('',(#13538),#3167,.T.);
#92818=ADVANCED_FACE('',(#13539),#87552,.T.);
#92819=ADVANCED_FACE('',(#13540),#4016,.T.);
#92820=ADVANCED_FACE('',(#13541),#4017,.F.);
#92821=ADVANCED_FACE('',(#13542),#4018,.F.);
#92822=ADVANCED_FACE('',(#13543),#4019,.T.);
#92823=ADVANCED_FACE('',(#13544),#4020,.T.);
#92824=ADVANCED_FACE('',(#13545),#3168,.T.);
#92825=ADVANCED_FACE('',(#13546),#4021,.T.);
#92826=ADVANCED_FACE('',(#13547),#3169,.T.);
#92827=ADVANCED_FACE('',(#13548),#3170,.T.);
#92828=ADVANCED_FACE('',(#13549),#4022,.T.);
#92829=ADVANCED_FACE('',(#13550),#3171,.T.);
#92830=ADVANCED_FACE('',(#13551),#87553,.F.);
#92831=ADVANCED_FACE('',(#13552),#87554,.T.);
#92832=ADVANCED_FACE('',(#13553),#4023,.T.);
#92833=ADVANCED_FACE('',(#13554),#3172,.T.);
#92834=ADVANCED_FACE('',(#13555),#955,.T.);
#92835=ADVANCED_FACE('',(#13556),#3173,.F.);
#92836=ADVANCED_FACE('',(#13557),#87555,.F.);
#92837=ADVANCED_FACE('',(#13558),#956,.T.);
#92838=ADVANCED_FACE('',(#13559),#957,.T.);
#92839=ADVANCED_FACE('',(#13560),#958,.T.);
#92840=ADVANCED_FACE('',(#13561),#959,.T.);
#92841=ADVANCED_FACE('',(#13562),#87556,.F.);
#92842=ADVANCED_FACE('',(#13563),#3174,.F.);
#92843=ADVANCED_FACE('',(#13564),#3175,.F.);
#92844=ADVANCED_FACE('',(#13565),#3176,.F.);
#92845=ADVANCED_FACE('',(#13566),#3177,.F.);
#92846=ADVANCED_FACE('',(#13567),#87557,.F.);
#92847=ADVANCED_FACE('',(#13568),#960,.F.);
#92848=ADVANCED_FACE('',(#13569),#961,.F.);
#92849=ADVANCED_FACE('',(#13570),#962,.F.);
#92850=ADVANCED_FACE('',(#13571),#963,.F.);
#92851=ADVANCED_FACE('',(#13572),#87558,.F.);
#92852=ADVANCED_FACE('',(#13573),#3178,.F.);
#92853=ADVANCED_FACE('',(#13574),#3179,.F.);
#92854=ADVANCED_FACE('',(#13575),#3180,.F.);
#92855=ADVANCED_FACE('',(#13576),#3181,.F.);
#92856=ADVANCED_FACE('',(#13577),#87559,.F.);
#92857=ADVANCED_FACE('',(#13578),#87560,.F.);
#92858=ADVANCED_FACE('',(#13579),#964,.F.);
#92859=ADVANCED_FACE('',(#13580),#965,.F.);
#92860=ADVANCED_FACE('',(#13581),#966,.F.);
#92861=ADVANCED_FACE('',(#13582),#967,.F.);
#92862=ADVANCED_FACE('',(#13583),#87561,.F.);
#92863=ADVANCED_FACE('',(#13584),#3182,.F.);
#92864=ADVANCED_FACE('',(#13585),#3183,.F.);
#92865=ADVANCED_FACE('',(#13586),#3184,.F.);
#92866=ADVANCED_FACE('',(#13587),#3185,.F.);
#92867=ADVANCED_FACE('',(#13588),#87562,.F.);
#92868=ADVANCED_FACE('',(#13589),#87563,.F.);
#92869=ADVANCED_FACE('',(#13590),#968,.T.);
#92870=ADVANCED_FACE('',(#13591),#969,.T.);
#92871=ADVANCED_FACE('',(#13592),#970,.T.);
#92872=ADVANCED_FACE('',(#13593),#971,.T.);
#92873=ADVANCED_FACE('',(#13594,#7614,#7615,#7616,#7617),#8515,.T.);
#92874=ADVANCED_FACE('',(#13595),#87564,.F.);
#92875=ADVANCED_FACE('',(#13596),#3186,.F.);
#92876=ADVANCED_FACE('',(#13597),#3187,.F.);
#92877=ADVANCED_FACE('',(#13598),#3188,.F.);
#92878=ADVANCED_FACE('',(#13599),#3189,.F.);
#92879=ADVANCED_FACE('',(#13600),#87565,.F.);
#92880=ADVANCED_FACE('',(#13601),#87566,.F.);
#92881=ADVANCED_FACE('',(#13602,#7618,#7619,#7620,#7621),#7162,.T.);
#92882=ADVANCED_FACE('',(#13603),#87567,.T.);
#92883=ADVANCED_FACE('',(#13604),#972,.T.);
#92884=ADVANCED_FACE('',(#13605),#973,.T.);
#92885=ADVANCED_FACE('',(#13606),#974,.T.);
#92886=ADVANCED_FACE('',(#13607),#975,.F.);
#92887=ADVANCED_FACE('',(#13608),#976,.F.);
#92888=ADVANCED_FACE('',(#13609),#977,.F.);
#92889=ADVANCED_FACE('',(#13610),#978,.F.);
#92890=ADVANCED_FACE('',(#13611),#979,.F.);
#92891=ADVANCED_FACE('',(#13612),#980,.F.);
#92892=ADVANCED_FACE('',(#13613),#981,.T.);
#92893=ADVANCED_FACE('',(#13614),#982,.T.);
#92894=ADVANCED_FACE('',(#13615),#983,.T.);
#92895=ADVANCED_FACE('',(#13616),#8516,.F.);
#92896=ADVANCED_FACE('',(#13617),#8517,.T.);
#92897=ADVANCED_FACE('',(#13618),#87568,.T.);
#92898=ADVANCED_FACE('',(#13619),#3190,.T.);
#92899=ADVANCED_FACE('',(#13620),#3191,.T.);
#92900=ADVANCED_FACE('',(#13621),#87569,.T.);
#92901=ADVANCED_FACE('',(#13622),#87570,.T.);
#92902=ADVANCED_FACE('',(#13623),#87571,.T.);
#92903=ADVANCED_FACE('',(#13624),#1038,.T.);
#92904=ADVANCED_FACE('',(#13625),#1039,.T.);
#92905=ADVANCED_FACE('',(#13626),#87572,.T.);
#92906=ADVANCED_FACE('',(#13627),#87573,.T.);
#92907=ADVANCED_FACE('',(#13628),#87574,.T.);
#93708=CLOSED_SHELL('',(#88019,#88020,#88021,#88022,#88023,#88024));
#93709=CLOSED_SHELL('',(#88025,#88026,#88027,#88028,#88029,#88030));
#93710=CLOSED_SHELL('',(#88031,#88032,#88033,#88034,#88035,#88036,#88037,
#88038,#88039,#88040,#88041,#88042,#88043,#88044,#88045,#88046,#88047,#88048,
#88049,#88050,#88051,#88052,#88053,#88054,#88055,#88056,#88057,#88058,#88059,
#88060,#88061,#88062,#88063,#88064,#88065,#88066,#88067,#88068,#88069,#88070,
#88071,#88072,#88073,#88074,#88075,#88076,#88077,#88078,#88079,#88080,#88081,
#88082,#88083,#88084,#88085,#88086,#88087,#88088,#88089,#88090,#88091,#88092,
#88093,#88094,#88095,#88096,#88097,#88098,#88099,#88100,#88101,#88102,#88103,
#88104,#88105,#88106,#88107,#88108,#88109,#88110,#88111,#88112,#88113,#88114,
#88115,#88116,#88117,#88118,#88119,#88120,#88121,#88122,#88123,#88124,#88125,
#88126,#88127,#88128,#88129,#88130,#88131,#88132,#88133,#88134,#88135,#88136,
#88137,#88138,#88139,#88140,#88141,#88142,#88143,#88144,#88145,#88146,#88147,
#88148,#88149,#88150,#88151,#88152,#88153,#88154,#88155,#88156,#88157,#88158,
#88159,#88160,#88161,#88162,#88163,#88164,#88165,#88166,#88167,#88168,#88169,
#88170,#88171,#88172,#88173,#88174,#88175,#88176,#88177,#88178,#88179,#88180,
#88181,#88182,#88183,#88184,#88185,#88186,#88187,#88188,#88189,#88190,#88191,
#88192,#88193,#88194,#88195,#88196,#88197,#88198,#88199,#88200,#88201,#88202,
#88203,#88204,#88205,#88206,#88207,#88208,#88209,#88210,#88211,#88212,#88213,
#88214,#88215,#88216,#88217,#88218,#88219,#88220,#88221,#88222,#88223,#88224,
#88225,#88226,#88227,#88228,#88229,#88230,#88231,#88232,#88233,#88234,#88235,
#88236,#88237,#88238,#88239,#88240,#88241,#88242,#88243,#88244,#88245,#88246,
#88247,#88248,#88249,#88250,#88251,#88252,#88253,#88254,#88255,#88256,#88257,
#88258,#88259,#88260,#88261,#88262,#88263,#88264,#88265,#88266,#88267,#88268,
#88269,#88270,#88271,#88272,#88273,#88274,#88275,#88276,#88277,#88278,#88279,
#88280,#88281,#88282,#88283,#88284,#88285,#88286,#88287,#88288,#88289,#88290,
#88291,#88292,#88293,#88294,#88295,#88296,#88297,#88298,#88299,#88300,#88301,
#88302,#88303,#88304,#88305,#88306,#88307,#88308,#88309,#88310,#88311,#88312,
#88313,#88314,#88315,#88316,#88317,#88318,#88319,#88320,#88321,#88322,#88323,
#88324,#88325,#88326,#88327,#88328,#88329,#88330,#88331,#88332,#88333,#88334,
#88335,#88336,#88337,#88338,#88339,#88340,#88341,#88342,#88343,#88344,#88345,
#88346,#88347,#88348,#88349,#88350,#88351,#88352,#88353,#88354,#88355,#88356,
#88357,#88358,#88359,#88360,#88361,#88362,#88363,#88364,#88365,#88366,#88367,
#88368,#88369,#88370,#88371,#88372,#88373,#88374,#88375,#88376,#88377,#88378,
#88379,#88380,#88381,#88382,#88383,#88384,#88385,#88386,#88387,#88388,#88389,
#88390,#88391,#88392,#88393,#88394,#88395,#88396,#88397,#88398,#88399,#88400,
#88401,#88402,#88403,#88404,#88405,#88406,#88407,#88408,#88409,#88410,#88411,
#88412,#88413,#88414,#88415,#88416,#88417,#88418,#88419,#88420,#88421,#88422,
#88423,#88424,#88425,#88426,#88427,#88428,#88429,#88430,#88431,#88432,#88433,
#88434,#88435,#88436,#88437,#88438,#88439,#88440,#88441,#88442,#88443,#88444,
#88445,#88446,#88447,#88448,#88449,#88450,#88451,#88452,#88453,#88454,#88455,
#88456,#88457,#88458,#88459,#88460,#88461,#88462,#88463,#88464,#88465,#88466,
#88467,#88468,#88469,#88470,#88471,#88472,#88473,#88474,#88475,#88476,#88477,
#88478,#88479,#88480,#88481,#88482,#88483,#88484,#88485,#88486,#88487,#88488,
#88489,#88490,#88491,#88492,#88493,#88494,#88495,#88496,#88497,#88498,#88499,
#88500,#88501,#88502,#88503,#88504,#88505,#88506,#88507,#88508,#88509,#88510,
#88511,#88512,#88513,#88514,#88515,#88516,#88517,#88518,#88519,#88520,#88521,
#88522,#88523,#88524,#88525,#88526,#88527,#88528,#88529,#88530,#88531,#88532,
#88533,#88534,#88535,#88536,#88537,#88538,#88539,#88540,#88541,#88542,#88543,
#88544,#88545,#88546,#88547,#88548,#88549,#88550,#88551,#88552,#88553,#88554,
#88555,#88556,#88557,#88558,#88559,#88560,#88561,#88562,#88563,#88564,#88565,
#88566,#88567,#88568,#88569,#88570,#88571,#88572,#88573,#88574,#88575,#88576,
#88577,#88578,#88579,#88580,#88581,#88582,#88583,#88584,#88585,#88586,#88587,
#88588,#88589,#88590,#88591,#88592,#88593,#88594,#88595,#88596,#88597,#88598,
#88599,#88600,#88601,#88602,#88603,#88604,#88605,#88606,#88607,#88608,#88609,
#88610,#88611,#88612,#88613,#88614,#88615,#88616,#88617,#88618,#88619,#88620,
#88621,#88622,#88623,#88624,#88625,#88626,#88627,#88628,#88629,#88630,#88631,
#88632,#88633,#88634,#88635,#88636,#88637,#88638,#88639,#88640,#88641,#88642,
#88643,#88644,#88645,#88646,#88647,#88648,#88649,#88650,#88651,#88652,#88653,
#88654,#88655,#88656,#88657,#88658,#88659,#88660,#88661,#88662,#88663,#88664,
#88665,#88666,#88667,#88668,#88669,#88670,#88671,#88672,#88673,#88674,#88675,
#88676,#88677,#88678,#88679,#88680,#88681,#88682,#88683,#88684,#88685,#88686,
#88687,#88688,#88689,#88690,#88691,#88692,#88693,#88694,#88695,#88696,#88697,
#88698,#88699,#88700,#88701,#88702,#88703,#88704,#88705,#88706,#88707,#88708,
#88709,#88710,#88711,#88712,#88713,#88714,#88715,#88716,#88717,#88718,#88719,
#88720,#88721,#88722,#88723,#88724,#88725,#88726,#88727,#88728,#88729,#88730,
#88731,#88732,#88733,#88734,#88735,#88736,#88737,#88738,#88739,#88740,#88741,
#88742,#88743,#88744,#88745,#88746,#88747,#88748,#88749,#88750,#88751,#88752,
#88753,#88754,#88755,#88756,#88757,#88758,#88759,#88760,#88761,#88762,#88763,
#88764,#88765,#88766,#88767,#88768,#88769,#88770,#88771,#88772,#88773,#88774,
#88775,#88776,#88777,#88778,#88779,#88780,#88781,#88782,#88783,#88784,#88785,
#88786,#88787,#88788,#88789,#88790,#88791,#88792,#88793,#88794,#88795,#88796,
#88797,#88798,#88799,#88800,#88801,#88802,#88803,#88804,#88805,#88806,#88807,
#88808,#88809,#88810,#88811,#88812,#88813,#88814,#88815,#88816,#88817,#88818,
#88819,#88820,#88821,#88822,#88823,#88824,#88825,#88826,#88827,#88828,#88829,
#88830,#88831,#88832,#88833,#88834,#88835,#88836,#88837,#88838,#88839,#88840,
#88841,#88842,#88843,#88844,#88845,#88846,#88847,#88848,#88849,#88850,#88851,
#88852,#88853,#88854,#88855,#88856,#88857,#88858,#88859,#88860,#88861,#88862,
#88863,#88864,#88865,#88866,#88867,#88868,#88869,#88870,#88871,#88872,#88873,
#88874,#88875,#88876,#88877,#88878,#88879,#88880,#88881,#88882,#88883,#88884,
#88885,#88886,#88887,#88888,#88889,#88890,#88891,#88892,#88893,#88894,#88895,
#88896,#88897,#88898,#88899,#88900,#88901,#88902,#88903,#88904,#88905,#88906,
#88907,#88908,#88909,#88910,#88911,#88912,#88913,#88914,#88915,#88916,#88917,
#88918,#88919,#88920,#88921,#88922,#88923,#88924,#88925,#88926,#88927,#88928,
#88929,#88930,#88931,#88932,#88933,#88934,#88935,#88936,#88937,#88938,#88939,
#88940,#88941,#88942,#88943,#88944,#88945,#88946,#88947,#88948,#88949,#88950,
#88951,#88952,#88953,#88954,#88955,#88956,#88957,#88958,#88959,#88960,#88961,
#88962,#88963,#88964,#88965,#88966,#88967,#88968,#88969,#88970,#88971,#88972,
#88973,#88974,#88975,#88976,#88977,#88978,#88979,#88980,#88981,#88982,#88983,
#88984,#88985,#88986,#88987,#88988,#88989,#88990,#88991,#88992,#88993,#88994,
#88995,#88996,#88997,#88998,#88999,#89000,#89001,#89002,#89003,#89004,#89005,
#89006,#89007,#89008,#89009,#89010,#89011,#89012,#89013,#89014,#89015,#89016,
#89017,#89018,#89019,#89020,#89021,#89022,#89023,#89024,#89025,#89026,#89027,
#89028,#89029,#89030,#89031,#89032,#89033,#89034,#89035,#89036,#89037,#89038,
#89039,#89040,#89041,#89042,#89043,#89044,#89045,#89046,#89047,#89048,#89049,
#89050,#89051,#89052,#89053,#89054,#89055,#89056,#89057,#89058,#89059,#89060,
#89061,#89062,#89063,#89064,#89065,#89066,#89067,#89068,#89069,#89070,#89071,
#89072,#89073,#89074,#89075,#89076,#89077,#89078,#89079,#89080,#89081,#89082,
#89083,#89084,#89085,#89086,#89087,#89088,#89089,#89090,#89091,#89092,#89093,
#89094,#89095,#89096,#89097,#89098,#89099,#89100,#89101,#89102,#89103,#89104,
#89105,#89106,#89107,#89108,#89109,#89110,#89111,#89112,#89113,#89114,#89115,
#89116,#89117,#89118,#89119,#89120,#89121,#89122,#89123,#89124,#89125,#89126,
#89127,#89128,#89129,#89130,#89131,#89132,#89133,#89134,#89135,#89136,#89137,
#89138,#89139,#89140,#89141,#89142,#89143,#89144,#89145,#89146,#89147,#89148,
#89149,#89150,#89151,#89152,#89153,#89154,#89155,#89156,#89157,#89158,#89159,
#89160,#89161,#89162,#89163,#89164,#89165,#89166,#89167,#89168,#89169,#89170,
#89171,#89172,#89173,#89174,#89175,#89176,#89177,#89178,#89179,#89180,#89181,
#89182,#89183,#89184,#89185,#89186,#89187,#89188,#89189,#89190,#89191,#89192,
#89193,#89194,#89195,#89196,#89197,#89198,#89199,#89200,#89201,#89202,#89203,
#89204,#89205,#89206,#89207,#89208,#89209,#89210,#89211,#89212,#89213,#89214,
#89215,#89216,#89217,#89218,#89219,#89220,#89221,#89222,#89223,#89224,#89225,
#89226,#89227,#89228,#89229,#89230,#89231,#89232,#89233,#89234,#89235,#89236,
#89237,#89238,#89239,#89240,#89241,#89242,#89243,#89244,#89245,#89246,#89247,
#89248,#89249,#89250,#89251,#89252,#89253,#89254,#89255,#89256,#89257,#89258,
#89259,#89260,#89261,#89262,#89263,#89264,#89265,#89266,#89267,#89268,#89269,
#89270,#89271,#89272,#89273,#89274,#89275,#89276,#89277,#89278,#89279,#89280,
#89281,#89282,#89283,#89284,#89285,#89286,#89287,#89288,#89289,#89290,#89291,
#89292,#89293,#89294,#89295,#89296,#89297,#89298,#89299,#89300,#89301,#89302,
#89303,#89304,#89305,#89306,#89307,#89308,#89309,#89310,#89311,#89312,#89313,
#89314,#89315,#89316,#89317,#89318,#89319,#89320,#89321,#89322,#89323,#89324,
#89325,#89326,#89327,#89328,#89329,#89330,#89331,#89332,#89333,#89334,#89335,
#89336,#89337,#89338,#89339,#89340,#89341,#89342,#89343,#89344,#89345,#89346,
#89347,#89348,#89349,#89350,#89351,#89352,#89353,#89354,#89355,#89356,#89357,
#89358,#89359,#89360,#89361,#89362,#89363,#89364,#89365,#89366,#89367,#89368,
#89369,#89370,#89371,#89372,#89373,#89374,#89375,#89376,#89377,#89378,#89379,
#89380,#89381,#89382,#89383,#89384,#89385,#89386,#89387,#89388,#89389,#89390,
#89391,#89392,#89393,#89394,#89395,#89396,#89397,#89398,#89399,#89400,#89401,
#89402,#89403,#89404,#89405,#89406,#89407,#89408,#89409,#89410,#89411,#89412,
#89413,#89414,#89415,#89416,#89417,#89418,#89419,#89420,#89421,#89422,#89423,
#89424,#89425,#89426,#89427,#89428,#89429,#89430,#89431,#89432,#89433,#89434,
#89435,#89436,#89437,#89438,#89439,#89440,#89441,#89442,#89443,#89444,#89445,
#89446,#89447,#89448,#89449,#89450,#89451,#89452,#89453,#89454,#89455,#89456,
#89457,#89458,#89459,#89460,#89461,#89462,#89463,#89464,#89465,#89466,#89467,
#89468,#89469,#89470,#89471,#89472,#89473,#89474,#89475,#89476,#89477,#89478,
#89479,#89480,#89481,#89482,#89483,#89484,#89485,#89486,#89487,#89488,#89489,
#89490,#89491,#89492,#89493,#89494,#89495,#89496,#89497,#89498,#89499,#89500,
#89501,#89502,#89503,#89504,#89505,#89506,#89507,#89508,#89509,#89510,#89511,
#89512,#89513,#89514,#89515,#89516,#89517,#89518,#89519,#89520,#89521,#89522,
#89523,#89524,#89525,#89526,#89527,#89528,#89529,#89530,#89531,#89532,#89533,
#89534,#89535,#89536,#89537,#89538,#89539,#89540,#89541,#89542,#89543,#89544,
#89545,#89546,#89547,#89548,#89549,#89550,#89551,#89552,#89553,#89554,#89555,
#89556,#89557,#89558,#89559,#89560,#89561,#89562,#89563,#89564,#89565,#89566,
#89567,#89568,#89569,#89570,#89571,#89572,#89573,#89574,#89575,#89576,#89577,
#89578,#89579,#89580,#89581,#89582,#89583,#89584,#89585,#89586,#89587,#89588,
#89589,#89590,#89591,#89592,#89593,#89594,#89595,#89596,#89597,#89598,#89599,
#89600,#89601,#89602,#89603,#89604,#89605,#89606,#89607,#89608,#89609,#89610,
#89611,#89612,#89613,#89614,#89615,#89616,#89617,#89618,#89619,#89620,#89621,
#89622,#89623,#89624,#89625,#89626,#89627,#89628,#89629,#89630,#89631,#89632,
#89633,#89634,#89635,#89636,#89637,#89638,#89639,#89640,#89641,#89642,#89643,
#89644,#89645,#89646,#89647,#89648,#89649,#89650,#89651,#89652,#89653,#89654,
#89655,#89656,#89657,#89658,#89659,#89660,#89661,#89662,#89663,#89664,#89665,
#89666,#89667,#89668,#89669,#89670,#89671,#89672,#89673,#89674,#89675,#89676,
#89677,#89678,#89679,#89680,#89681,#89682,#89683,#89684,#89685,#89686,#89687,
#89688,#89689,#89690,#89691,#89692,#89693,#89694,#89695,#89696,#89697,#89698,
#89699,#89700,#89701,#89702,#89703,#89704,#89705,#89706,#89707,#89708,#89709,
#89710,#89711,#89712,#89713,#89714,#89715,#89716,#89717,#89718,#89719,#89720,
#89721,#89722,#89723,#89724,#89725,#89726,#89727,#89728,#89729,#89730,#89731,
#89732,#89733,#89734,#89735,#89736,#89737,#89738,#89739,#89740,#89741,#89742,
#89743,#89744,#89745,#89746,#89747,#89748,#89749,#89750,#89751,#89752,#89753,
#89754,#89755,#89756,#89757,#89758,#89759,#89760,#89761,#89762,#89763,#89764,
#89765,#89766,#89767,#89768,#89769,#89770,#89771,#89772,#89773,#89774,#89775,
#89776,#89777,#89778,#89779,#89780,#89781,#89782,#89783,#89784,#89785,#89786,
#89787,#89788,#89789,#89790,#89791,#89792,#89793,#89794,#89795,#89796,#89797,
#89798,#89799,#89800,#89801,#89802,#89803,#89804,#89805,#89806,#89807,#89808,
#89809,#89810,#89811,#89812,#89813,#89814,#89815,#89816,#89817,#89818,#89819,
#89820,#89821,#89822,#89823,#89824,#89825,#89826,#89827,#89828,#89829,#89830,
#89831,#89832,#89833,#89834,#89835,#89836,#89837,#89838,#89839,#89840,#89841,
#89842,#89843,#89844,#89845,#89846,#89847,#89848,#89849,#89850,#89851,#89852,
#89853,#89854,#89855,#89856,#89857,#89858,#89859,#89860,#89861,#89862,#89863,
#89864,#89865,#89866,#89867,#89868,#89869,#89870,#89871,#89872,#89873,#89874,
#89875,#89876,#89877,#89878,#89879,#89880,#89881,#89882,#89883,#89884,#89885,
#89886,#89887,#89888,#89889,#89890,#89891,#89892,#89893,#89894,#89895,#89896,
#89897,#89898,#89899,#89900,#89901,#89902,#89903,#89904,#89905,#89906,#89907,
#89908,#89909,#89910,#89911,#89912,#89913,#89914,#89915,#89916,#89917,#89918,
#89919,#89920,#89921,#89922,#89923,#89924,#89925,#89926,#89927,#89928,#89929,
#89930,#89931,#89932,#89933,#89934,#89935,#89936,#89937,#89938,#89939,#89940,
#89941,#89942,#89943,#89944,#89945,#89946,#89947,#89948,#89949,#89950,#89951,
#89952,#89953,#89954,#89955,#89956,#89957,#89958,#89959,#89960,#89961,#89962,
#89963,#89964,#89965,#89966,#89967,#89968,#89969,#89970,#89971,#89972,#89973,
#89974,#89975,#89976,#89977,#89978,#89979,#89980,#89981,#89982,#89983,#89984,
#89985,#89986,#89987,#89988,#89989,#89990,#89991,#89992,#89993,#89994,#89995,
#89996,#89997,#89998,#89999,#90000,#90001,#90002,#90003,#90004,#90005,#90006,
#90007,#90008,#90009,#90010,#90011,#90012,#90013,#90014,#90015,#90016,#90017,
#90018,#90019,#90020,#90021,#90022,#90023,#90024,#90025,#90026,#90027,#90028,
#90029,#90030,#90031,#90032,#90033,#90034,#90035,#90036,#90037,#90038,#90039,
#90040,#90041,#90042,#90043,#90044,#90045,#90046,#90047,#90048,#90049,#90050,
#90051,#90052,#90053,#90054,#90055,#90056,#90057,#90058,#90059,#90060,#90061,
#90062,#90063,#90064,#90065,#90066,#90067,#90068,#90069,#90070,#90071,#90072,
#90073,#90074,#90075,#90076,#90077,#90078,#90079,#90080,#90081,#90082,#90083,
#90084,#90085,#90086,#90087,#90088,#90089,#90090,#90091,#90092,#90093,#90094,
#90095,#90096,#90097,#90098,#90099,#90100,#90101,#90102,#90103,#90104,#90105,
#90106,#90107,#90108,#90109,#90110,#90111,#90112,#90113,#90114,#90115,#90116,
#90117,#90118,#90119,#90120,#90121,#90122,#90123,#90124,#90125,#90126,#90127,
#90128,#90129,#90130,#90131,#90132,#90133,#90134,#90135,#90136,#90137,#90138,
#90139,#90140,#90141,#90142,#90143,#90144,#90145,#90146,#90147,#90148,#90149,
#90150,#90151,#90152,#90153,#90154,#90155,#90156,#90157,#90158,#90159,#90160,
#90161,#90162,#90163,#90164,#90165,#90166,#90167,#90168,#90169,#90170,#90171,
#90172,#90173,#90174,#90175,#90176,#90177,#90178,#90179,#90180,#90181,#90182,
#90183,#90184,#90185,#90186,#90187,#90188,#90189,#90190,#90191,#90192,#90193,
#90194,#90195,#90196,#90197,#90198,#90199,#90200,#90201,#90202,#90203,#90204,
#90205,#90206,#90207,#90208,#90209,#90210,#90211,#90212,#90213,#90214,#90215,
#90216,#90217,#90218,#90219,#90220,#90221,#90222,#90223,#90224,#90225,#90226,
#90227,#90228,#90229,#90230,#90231,#90232,#90233,#90234,#90235,#90236,#90237,
#90238,#90239,#90240,#90241,#90242,#90243,#90244,#90245,#90246,#90247,#90248,
#90249,#90250,#90251,#90252,#90253,#90254,#90255,#90256,#90257,#90258,#90259,
#90260,#90261,#90262,#90263,#90264,#90265,#90266,#90267,#90268,#90269,#90270,
#90271,#90272,#90273,#90274,#90275,#90276,#90277,#90278,#90279,#90280,#90281,
#90282,#90283,#90284,#90285,#90286,#90287,#90288,#90289,#90290,#90291,#90292));
#93711=CLOSED_SHELL('',(#90293,#90294,#90295,#90296,#90297,#90298,#90299,
#90300,#90301,#90302,#90303,#90304,#90305,#90306,#90307,#90308,#90309));
#93712=CLOSED_SHELL('',(#90310,#90311,#90312,#90313,#90314,#90315));
#93713=CLOSED_SHELL('',(#90316,#90317,#90318,#90319,#90320,#90321,#90322,
#90323,#90324,#90325,#90326,#90327,#90328,#90329,#90330,#90331,#90332,#90333,
#90334,#90335,#90336,#90337,#90338,#90339,#90340,#90341,#90342,#90343,#90344,
#90345,#90346,#90347,#90348,#90349,#90350,#90351,#90352,#90353,#90354,#90355,
#90356,#90357,#90358,#90359,#90360,#90361,#90362,#90363,#90364,#90365,#90366,
#90367,#90368,#90369,#90370,#90371,#90372,#90373,#90374,#90375,#90376,#90377,
#90378,#90379,#90380,#90381,#90382,#90383,#90384,#90385,#90386,#90387,#90388,
#90389,#90390,#90391,#90392,#90393,#90394,#90395,#90396,#90397,#90398,#90399,
#90400,#90401,#90402,#90403,#90404,#90405,#90406,#90407,#90408,#90409,#90410,
#90411,#90412,#90413,#90414,#90415,#90416,#90417,#90418,#90419,#90420,#90421,
#90422,#90423,#90424,#90425,#90426,#90427,#90428,#90429,#90430,#90431,#90432,
#90433,#90434,#90435,#90436,#90437,#90438,#90439,#90440,#90441,#90442,#90443,
#90444,#90445,#90446,#90447,#90448,#90449,#90450,#90451,#90452,#90453,#90454,
#90455,#90456,#90457,#90458,#90459,#90460,#90461,#90462,#90463,#90464,#90465,
#90466,#90467,#90468,#90469,#90470,#90471,#90472,#90473,#90474,#90475,#90476,
#90477,#90478,#90479,#90480,#90481,#90482,#90483,#90484,#90485,#90486,#90487,
#90488,#90489,#90490,#90491,#90492,#90493,#90494,#90495,#90496,#90497,#90498,
#90499,#90500,#90501,#90502,#90503,#90504,#90505,#90506,#90507,#90508,#90509,
#90510,#90511,#90512,#90513,#90514,#90515,#90516,#90517,#90518,#90519,#90520,
#90521,#90522,#90523,#90524,#90525,#90526,#90527,#90528,#90529,#90530,#90531,
#90532,#90533,#90534,#90535,#90536,#90537,#90538,#90539,#90540,#90541,#90542,
#90543,#90544,#90545,#90546,#90547,#90548,#90549,#90550,#90551,#90552,#90553,
#90554,#90555,#90556,#90557,#90558,#90559,#90560,#90561,#90562,#90563,#90564,
#90565,#90566,#90567,#90568,#90569,#90570,#90571,#90572,#90573,#90574,#90575,
#90576,#90577,#90578,#90579,#90580,#90581,#90582,#90583,#90584,#90585,#90586,
#90587,#90588,#90589,#90590,#90591,#90592,#90593,#90594,#90595,#90596,#90597,
#90598,#90599,#90600,#90601,#90602,#90603,#90604,#90605,#90606,#90607,#90608,
#90609,#90610,#90611,#90612,#90613,#90614,#90615,#90616,#90617,#90618,#90619,
#90620,#90621,#90622,#90623,#90624,#90625,#90626,#90627,#90628,#90629,#90630,
#90631,#90632,#90633,#90634,#90635,#90636,#90637,#90638,#90639,#90640,#90641,
#90642,#90643,#90644,#90645,#90646,#90647,#90648,#90649,#90650,#90651,#90652,
#90653,#90654,#90655,#90656,#90657,#90658,#90659,#90660,#90661,#90662,#90663,
#90664,#90665,#90666,#90667,#90668,#90669,#90670,#90671,#90672,#90673,#90674,
#90675,#90676,#90677,#90678,#90679,#90680,#90681,#90682,#90683,#90684,#90685,
#90686,#90687,#90688,#90689,#90690,#90691,#90692,#90693,#90694,#90695,#90696,
#90697,#90698,#90699,#90700,#90701,#90702,#90703,#90704,#90705,#90706,#90707,
#90708,#90709,#90710,#90711,#90712,#90713,#90714,#90715,#90716,#90717,#90718,
#90719,#90720,#90721,#90722,#90723,#90724,#90725,#90726,#90727,#90728,#90729,
#90730,#90731,#90732,#90733,#90734,#90735,#90736,#90737,#90738,#90739,#90740,
#90741,#90742,#90743,#90744,#90745,#90746,#90747,#90748,#90749,#90750,#90751,
#90752,#90753,#90754,#90755,#90756,#90757,#90758,#90759,#90760,#90761,#90762,
#90763,#90764,#90765,#90766,#90767,#90768,#90769,#90770,#90771,#90772,#90773,
#90774,#90775,#90776,#90777,#90778,#90779,#90780,#90781,#90782,#90783,#90784,
#90785,#90786,#90787,#90788,#90789,#90790,#90791,#90792,#90793,#90794,#90795,
#90796,#90797,#90798,#90799,#90800,#90801,#90802,#90803,#90804,#90805,#90806,
#90807,#90808,#90809,#90810,#90811,#90812,#90813,#90814,#90815,#90816,#90817,
#90818,#90819,#90820,#90821,#90822,#90823,#90824,#90825,#90826,#90827,#90828,
#90829,#90830,#90831,#90832,#90833,#90834,#90835,#90836,#90837,#90838,#90839,
#90840,#90841,#90842,#90843,#90844,#90845,#90846,#90847,#90848,#90849,#90850,
#90851,#90852,#90853,#90854,#90855,#90856,#90857,#90858,#90859,#90860,#90861,
#90862,#90863,#90864,#90865,#90866,#90867,#90868,#90869,#90870,#90871,#90872,
#90873,#90874,#90875,#90876,#90877,#90878,#90879,#90880,#90881,#90882,#90883,
#90884,#90885,#90886,#90887,#90888,#90889,#90890,#90891,#90892,#90893,#90894,
#90895,#90896,#90897,#90898,#90899,#90900,#90901,#90902,#90903,#90904,#90905,
#90906,#90907,#90908,#90909,#90910,#90911,#90912,#90913,#90914,#90915,#90916,
#90917,#90918,#90919,#90920,#90921,#90922,#90923,#90924,#90925,#90926,#90927,
#90928,#90929,#90930,#90931,#90932,#90933,#90934,#90935,#90936,#90937,#90938,
#90939,#90940,#90941,#90942,#90943,#90944,#90945,#90946,#90947,#90948,#90949,
#90950,#90951,#90952,#90953,#90954,#90955,#90956,#90957,#90958,#90959,#90960,
#90961,#90962,#90963,#90964,#90965,#90966,#90967,#90968,#90969,#90970,#90971,
#90972,#90973,#90974,#90975,#90976,#90977,#90978,#90979,#90980,#90981,#90982,
#90983,#90984,#90985,#90986,#90987,#90988,#90989,#90990,#90991,#90992,#90993,
#90994,#90995,#90996,#90997,#90998,#90999,#91000,#91001,#91002,#91003,#91004,
#91005,#91006,#91007,#91008,#91009,#91010,#91011,#91012,#91013,#91014,#91015,
#91016,#91017,#91018,#91019,#91020,#91021,#91022,#91023,#91024,#91025,#91026,
#91027,#91028,#91029,#91030,#91031,#91032,#91033,#91034,#91035,#91036,#91037,
#91038,#91039,#91040,#91041,#91042,#91043,#91044,#91045,#91046,#91047,#91048,
#91049,#91050,#91051,#91052,#91053,#91054,#91055,#91056,#91057,#91058,#91059,
#91060,#91061,#91062,#91063,#91064,#91065,#91066,#91067,#91068,#91069,#91070,
#91071,#91072,#91073,#91074,#91075,#91076,#91077,#91078,#91079,#91080,#91081,
#91082,#91083,#91084,#91085,#91086,#91087,#91088,#91089,#91090,#91091,#91092,
#91093,#91094,#91095,#91096,#91097,#91098,#91099,#91100,#91101,#91102,#91103,
#91104,#91105,#91106,#91107,#91108,#91109,#91110,#91111,#91112,#91113,#91114,
#91115,#91116,#91117,#91118,#91119,#91120,#91121,#91122,#91123,#91124,#91125,
#91126,#91127,#91128,#91129,#91130,#91131,#91132,#91133,#91134,#91135,#91136,
#91137,#91138,#91139,#91140,#91141,#91142,#91143,#91144,#91145,#91146,#91147,
#91148,#91149,#91150,#91151,#91152,#91153,#91154,#91155,#91156,#91157,#91158,
#91159,#91160,#91161,#91162,#91163,#91164,#91165,#91166,#91167,#91168,#91169,
#91170,#91171,#91172,#91173,#91174,#91175,#91176,#91177,#91178,#91179,#91180,
#91181,#91182,#91183,#91184,#91185,#91186,#91187,#91188,#91189,#91190,#91191,
#91192,#91193,#91194,#91195,#91196,#91197,#91198,#91199,#91200,#91201,#91202,
#91203,#91204,#91205,#91206,#91207,#91208,#91209,#91210,#91211,#91212,#91213,
#91214,#91215,#91216,#91217,#91218,#91219,#91220,#91221,#91222,#91223,#91224,
#91225,#91226,#91227,#91228,#91229,#91230,#91231,#91232,#91233,#91234,#91235,
#91236,#91237,#91238,#91239,#91240,#91241,#91242,#91243,#91244,#91245,#91246,
#91247,#91248,#91249,#91250,#91251,#91252,#91253,#91254,#91255,#91256,#91257,
#91258,#91259,#91260,#91261,#91262,#91263,#91264,#91265,#91266,#91267,#91268,
#91269,#91270,#91271,#91272,#91273,#91274,#91275,#91276,#91277,#91278,#91279,
#91280,#91281,#91282,#91283,#91284,#91285,#91286,#91287,#91288,#91289,#91290,
#91291,#91292,#91293,#91294,#91295,#91296,#91297,#91298,#91299,#91300,#91301,
#91302,#91303,#91304,#91305,#91306,#91307,#91308,#91309,#91310,#91311,#91312,
#91313,#91314,#91315,#91316,#91317,#91318,#91319,#91320,#91321,#91322,#91323,
#91324,#91325,#91326,#91327,#91328,#91329,#91330,#91331,#91332,#91333,#91334,
#91335,#91336,#91337,#91338,#91339,#91340,#91341,#91342,#91343,#91344,#91345,
#91346,#91347,#91348,#91349,#91350,#91351,#91352,#91353,#91354,#91355,#91356,
#91357,#91358,#91359,#91360,#91361,#91362,#91363,#91364,#91365,#91366,#91367,
#91368,#91369,#91370,#91371,#91372,#91373,#91374,#91375,#91376,#91377,#91378,
#91379,#91380,#91381,#91382,#91383,#91384,#91385,#91386,#91387,#91388,#91389,
#91390,#91391,#91392,#91393,#91394,#91395,#91396,#91397,#91398,#91399,#91400,
#91401,#91402,#91403,#91404,#91405,#91406,#91407,#91408,#91409,#91410,#91411,
#91412,#91413,#91414,#91415,#91416,#91417,#91418,#91419,#91420,#91421,#91422,
#91423,#91424,#91425,#91426,#91427,#91428,#91429,#91430,#91431,#91432,#91433,
#91434,#91435,#91436,#91437,#91438,#91439,#91440,#91441,#91442,#91443,#91444,
#91445,#91446,#91447,#91448,#91449,#91450,#91451,#91452,#91453,#91454,#91455,
#91456,#91457,#91458,#91459,#91460,#91461,#91462,#91463,#91464,#91465,#91466,
#91467,#91468,#91469,#91470,#91471,#91472,#91473,#91474,#91475,#91476,#91477,
#91478,#91479,#91480,#91481,#91482,#91483,#91484,#91485,#91486,#91487,#91488,
#91489,#91490,#91491,#91492,#91493,#91494,#91495,#91496,#91497,#91498,#91499,
#91500,#91501,#91502,#91503,#91504,#91505,#91506,#91507,#91508,#91509,#91510,
#91511,#91512,#91513,#91514,#91515,#91516,#91517,#91518,#91519,#91520,#91521,
#91522,#91523,#91524,#91525,#91526,#91527,#91528,#91529,#91530,#91531,#91532,
#91533,#91534,#91535,#91536,#91537,#91538,#91539,#91540,#91541,#91542,#91543,
#91544,#91545,#91546,#91547,#91548,#91549,#91550,#91551,#91552,#91553,#91554,
#91555,#91556,#91557,#91558,#91559,#91560,#91561,#91562,#91563,#91564,#91565,
#91566,#91567,#91568,#91569,#91570,#91571,#91572,#91573,#91574,#91575,#91576,
#91577,#91578,#91579,#91580,#91581,#91582,#91583,#91584,#91585,#91586,#91587,
#91588,#91589,#91590,#91591,#91592,#91593,#91594,#91595,#91596,#91597,#91598,
#91599,#91600,#91601,#91602,#91603,#91604,#91605,#91606,#91607,#91608,#91609,
#91610,#91611,#91612,#91613,#91614,#91615,#91616,#91617,#91618,#91619,#91620,
#91621,#91622,#91623,#91624,#91625,#91626,#91627,#91628,#91629,#91630,#91631,
#91632,#91633,#91634,#91635,#91636,#91637,#91638,#91639,#91640,#91641,#91642,
#91643,#91644,#91645,#91646,#91647,#91648,#91649,#91650,#91651,#91652,#91653,
#91654,#91655,#91656,#91657,#91658,#91659,#91660,#91661,#91662,#91663,#91664,
#91665,#91666,#91667,#91668,#91669,#91670,#91671,#91672,#91673,#91674,#91675,
#91676,#91677,#91678,#91679,#91680,#91681,#91682,#91683,#91684,#91685,#91686,
#91687,#91688,#91689,#91690,#91691,#91692,#91693,#91694,#91695,#91696,#91697,
#91698,#91699,#91700,#91701,#91702,#91703,#91704,#91705,#91706,#91707,#91708,
#91709,#91710,#91711,#91712,#91713,#91714,#91715,#91716,#91717,#91718,#91719,
#91720,#91721,#91722,#91723,#91724,#91725,#91726,#91727,#91728,#91729,#91730,
#91731,#91732,#91733,#91734,#91735,#91736,#91737,#91738,#91739,#91740,#91741,
#91742,#91743,#91744,#91745,#91746,#91747,#91748,#91749,#91750,#91751,#91752,
#91753,#91754,#91755,#91756,#91757,#91758,#91759,#91760,#91761,#91762,#91763,
#91764,#91765,#91766,#91767,#91768,#91769,#91770,#91771,#91772,#91773,#91774,
#91775,#91776,#91777,#91778,#91779,#91780,#91781,#91782,#91783,#91784,#91785,
#91786,#91787,#91788,#91789,#91790,#91791,#91792,#91793,#91794,#91795,#91796,
#91797,#91798,#91799,#91800,#91801,#91802,#91803,#91804,#91805,#91806,#91807,
#91808,#91809,#91810,#91811,#91812,#91813,#91814,#91815,#91816,#91817,#91818,
#91819,#91820,#91821,#91822,#91823,#91824,#91825,#91826,#91827,#91828,#91829,
#91830,#91831,#91832,#91833,#91834,#91835,#91836,#91837,#91838,#91839,#91840,
#91841,#91842,#91843,#91844,#91845,#91846,#91847,#91848,#91849,#91850,#91851,
#91852,#91853,#91854,#91855,#91856,#91857,#91858,#91859,#91860,#91861,#91862,
#91863,#91864,#91865,#91866,#91867,#91868,#91869,#91870,#91871,#91872,#91873,
#91874,#91875,#91876,#91877,#91878,#91879,#91880,#91881,#91882,#91883,#91884,
#91885,#91886,#91887,#91888,#91889,#91890,#91891,#91892,#91893,#91894,#91895,
#91896,#91897,#91898,#91899,#91900,#91901,#91902,#91903,#91904,#91905,#91906,
#91907,#91908,#91909,#91910,#91911,#91912,#91913,#91914,#91915,#91916,#91917,
#91918,#91919,#91920,#91921,#91922,#91923,#91924,#91925,#91926,#91927,#91928,
#91929,#91930,#91931,#91932,#91933,#91934,#91935,#91936,#91937,#91938,#91939,
#91940,#91941,#91942,#91943,#91944,#91945,#91946,#91947,#91948,#91949,#91950,
#91951,#91952,#91953,#91954,#91955,#91956,#91957,#91958,#91959,#91960,#91961,
#91962,#91963,#91964,#91965,#91966,#91967,#91968,#91969,#91970,#91971,#91972,
#91973,#91974,#91975,#91976,#91977,#91978,#91979,#91980,#91981,#91982,#91983,
#91984,#91985,#91986,#91987,#91988,#91989,#91990,#91991,#91992,#91993,#91994,
#91995,#91996,#91997,#91998,#91999,#92000,#92001,#92002,#92003,#92004,#92005,
#92006,#92007,#92008,#92009,#92010,#92011,#92012,#92013,#92014,#92015,#92016,
#92017,#92018,#92019,#92020,#92021,#92022,#92023,#92024,#92025,#92026,#92027,
#92028,#92029,#92030,#92031,#92032,#92033,#92034,#92035,#92036,#92037,#92038,
#92039,#92040,#92041,#92042,#92043,#92044,#92045,#92046,#92047,#92048,#92049,
#92050,#92051,#92052,#92053,#92054,#92055,#92056,#92057));
#93714=CLOSED_SHELL('',(#92058,#92059,#92060,#92061,#92062,#92063,#92064,
#92065,#92066,#92067,#92068,#92069,#92070,#92071,#92072,#92073,#92074));
#93715=CLOSED_SHELL('',(#92075,#92076,#92077,#92078,#92079,#92080,#92081,
#92082,#92083,#92084,#92085,#92086,#92087,#92088,#92089,#92090,#92091,#92092,
#92093,#92094));
#93716=CLOSED_SHELL('',(#92095,#92096,#92097,#92098,#92099,#92100,#92101,
#92102,#92103,#92104,#92105,#92106,#92107,#92108,#92109,#92110,#92111,#92112,
#92113,#92114));
#93717=CLOSED_SHELL('',(#92115,#92116,#92117,#92118,#92119,#92120,#92121,
#92122,#92123,#92124,#92125,#92126,#92127,#92128,#92129,#92130,#92131));
#93718=CLOSED_SHELL('',(#92132,#92133,#92134,#92135,#92136,#92137,#92138,
#92139,#92140,#92141,#92142,#92143));
#93719=CLOSED_SHELL('',(#92144,#92145,#92146,#92147,#92148,#92149));
#93720=CLOSED_SHELL('',(#92150,#92151,#92152,#92153,#92154,#92155,#92156,
#92157,#92158,#92159,#92160,#92161,#92162,#92163,#92164,#92165,#92166,#92167,
#92168,#92169,#92170,#92171,#92172,#92173,#92174,#92175,#92176,#92177,#92178,
#92179,#92180,#92181,#92182,#92183,#92184,#92185,#92186,#92187,#92188,#92189,
#92190,#92191,#92192,#92193,#92194));
#93721=CLOSED_SHELL('',(#92195,#92196,#92197,#92198,#92199,#92200,#92201,
#92202,#92203,#92204,#92205,#92206));
#93722=CLOSED_SHELL('',(#92207,#92208,#92209,#92210,#92211,#92212,#92213,
#92214,#92215,#92216,#92217,#92218,#92219,#92220,#92221,#92222,#92223,#92224,
#92225,#92226,#92227,#92228,#92229,#92230,#92231,#92232,#92233,#92234,#92235,
#92236,#92237,#92238,#92239,#92240,#92241,#92242,#92243,#92244,#92245,#92246,
#92247,#92248,#92249,#92250,#92251,#92252,#92253,#92254,#92255,#92256,#92257,
#92258,#92259,#92260,#92261,#92262,#92263,#92264,#92265,#92266,#92267,#92268,
#92269,#92270,#92271,#92272,#92273,#92274,#92275,#92276,#92277,#92278,#92279,
#92280,#92281,#92282,#92283,#92284,#92285,#92286,#92287,#92288,#92289,#92290,
#92291,#92292,#92293,#92294,#92295,#92296,#92297,#92298,#92299,#92300,#92301,
#92302,#92303,#92304,#92305,#92306,#92307,#92308,#92309,#92310,#92311,#92312,
#92313,#92314,#92315,#92316,#92317,#92318,#92319,#92320,#92321,#92322,#92323,
#92324,#92325,#92326,#92327,#92328,#92329,#92330,#92331,#92332,#92333,#92334,
#92335,#92336,#92337,#92338,#92339,#92340,#92341,#92342,#92343,#92344,#92345,
#92346,#92347,#92348,#92349,#92350,#92351,#92352,#92353,#92354,#92355,#92356,
#92357,#92358,#92359,#92360,#92361,#92362,#92363,#92364,#92365,#92366,#92367,
#92368,#92369,#92370,#92371,#92372,#92373,#92374,#92375,#92376,#92377,#92378,
#92379,#92380,#92381,#92382,#92383,#92384,#92385,#92386,#92387,#92388,#92389,
#92390,#92391,#92392,#92393,#92394,#92395,#92396,#92397,#92398,#92399,#92400,
#92401,#92402,#92403,#92404,#92405,#92406,#92407,#92408,#92409,#92410,#92411,
#92412,#92413,#92414,#92415));
#93723=CLOSED_SHELL('',(#92416,#92417,#92418,#92419,#92420,#92421,#92422,
#92423,#92424,#92425,#92426,#92427,#92428,#92429,#92430,#92431,#92432,#92433,
#92434,#92435));
#93724=CLOSED_SHELL('',(#92436,#92437,#92438,#92439,#92440,#92441,#92442,
#92443,#92444,#92445,#92446,#92447,#92448,#92449,#92450,#92451,#92452,#92453,
#92454,#92455));
#93725=CLOSED_SHELL('',(#92456,#92457,#92458,#92459,#92460,#92461,#92462,
#92463,#92464,#92465,#92466,#92467,#92468,#92469,#92470,#92471,#92472));
#93726=CLOSED_SHELL('',(#92473,#92474,#92475,#92476,#92477,#92478,#92479,
#92480,#92481,#92482,#92483,#92484,#92485,#92486,#92487,#92488,#92489,#92490,
#92491,#92492,#92493,#92494,#92495,#92496,#92497,#92498,#92499,#92500,#92501,
#92502,#92503,#92504,#92505,#92506,#92507,#92508,#92509,#92510,#92511,#92512,
#92513,#92514,#92515,#92516,#92517,#92518,#92519,#92520,#92521,#92522,#92523,
#92524,#92525,#92526,#92527,#92528,#92529,#92530,#92531,#92532,#92533,#92534,
#92535));
#93727=CLOSED_SHELL('',(#92536,#92537,#92538,#92539,#92540,#92541,#92542,
#92543,#92544,#92545,#92546,#92547,#92548,#92549,#92550,#92551,#92552,#92553,
#92554,#92555,#92556,#92557,#92558,#92559,#92560,#92561,#92562,#92563,#92564,
#92565,#92566,#92567,#92568,#92569,#92570,#92571,#92572,#92573,#92574,#92575,
#92576,#92577,#92578,#92579,#92580,#92581,#92582,#92583,#92584,#92585,#92586,
#92587,#92588,#92589,#92590,#92591,#92592,#92593,#92594,#92595,#92596,#92597,
#92598,#92599,#92600,#92601,#92602,#92603,#92604,#92605,#92606,#92607,#92608,
#92609,#92610,#92611,#92612,#92613,#92614,#92615,#92616,#92617,#92618,#92619,
#92620,#92621,#92622,#92623,#92624,#92625,#92626,#92627,#92628,#92629,#92630,
#92631,#92632,#92633,#92634,#92635,#92636,#92637,#92638,#92639,#92640,#92641,
#92642,#92643,#92644,#92645,#92646,#92647,#92648,#92649,#92650,#92651,#92652,
#92653,#92654,#92655,#92656,#92657,#92658,#92659,#92660,#92661,#92662,#92663,
#92664,#92665,#92666,#92667,#92668,#92669,#92670,#92671,#92672,#92673,#92674,
#92675,#92676,#92677,#92678,#92679,#92680,#92681,#92682,#92683,#92684,#92685,
#92686,#92687,#92688,#92689,#92690,#92691,#92692,#92693,#92694,#92695,#92696,
#92697,#92698,#92699,#92700,#92701,#92702,#92703,#92704,#92705,#92706,#92707,
#92708,#92709,#92710,#92711,#92712,#92713,#92714,#92715,#92716,#92717,#92718,
#92719,#92720,#92721,#92722,#92723,#92724,#92725,#92726,#92727,#92728,#92729,
#92730,#92731,#92732,#92733,#92734,#92735,#92736,#92737,#92738,#92739,#92740,
#92741,#92742,#92743,#92744,#92745,#92746,#92747,#92748,#92749,#92750,#92751,
#92752,#92753,#92754,#92755,#92756,#92757,#92758,#92759,#92760,#92761,#92762,
#92763,#92764,#92765,#92766,#92767,#92768,#92769,#92770,#92771,#92772,#92773,
#92774,#92775,#92776,#92777,#92778,#92779,#92780,#92781,#92782,#92783,#92784,
#92785,#92786,#92787,#92788,#92789,#92790,#92791,#92792,#92793,#92794,#92795,
#92796,#92797,#92798,#92799,#92800,#92801,#92802,#92803,#92804,#92805,#92806,
#92807,#92808,#92809,#92810,#92811,#92812,#92813,#92814,#92815,#92816,#92817,
#92818,#92819,#92820,#92821,#92822,#92823,#92824,#92825,#92826,#92827,#92828,
#92829,#92830,#92831,#92832,#92833,#92834,#92835,#92836,#92837,#92838,#92839,
#92840,#92841,#92842,#92843,#92844,#92845,#92846,#92847,#92848,#92849,#92850,
#92851,#92852,#92853,#92854,#92855,#92856,#92857,#92858,#92859,#92860,#92861,
#92862,#92863,#92864,#92865,#92866,#92867,#92868,#92869,#92870,#92871,#92872,
#92873,#92874,#92875,#92876,#92877,#92878,#92879,#92880,#92881,#92882,#92883,
#92884,#92885,#92886,#92887,#92888,#92889,#92890,#92891,#92892,#92893,#92894,
#92895,#92896,#92897,#92898,#92899,#92900,#92901,#92902,#92903,#92904,#92905,
#92906,#92907));
#94082=AXIS2_PLACEMENT_3D('',#131308,#105182,#105183);
#94083=AXIS2_PLACEMENT_3D('',#131309,#105184,#105185);
#94084=AXIS2_PLACEMENT_3D('',#131311,#105186,#105187);
#94085=AXIS2_PLACEMENT_3D('',#131314,#105189,#105190);
#94086=AXIS2_PLACEMENT_3D('',#131315,#105191,#105192);
#94087=AXIS2_PLACEMENT_3D('',#131316,#105193,#105194);
#94088=AXIS2_PLACEMENT_3D('',#131318,#105195,#105196);
#94089=AXIS2_PLACEMENT_3D('',#131320,#105198,#105199);
#94090=AXIS2_PLACEMENT_3D('',#131322,#105200,#105201);
#94091=AXIS2_PLACEMENT_3D('',#131323,#105202,#105203);
#94092=AXIS2_PLACEMENT_3D('',#131325,#105204,#105205);
#94093=AXIS2_PLACEMENT_3D('',#131327,#105207,#105208);
#94094=AXIS2_PLACEMENT_3D('',#131328,#105209,#105210);
#94095=AXIS2_PLACEMENT_3D('',#131330,#105211,#105212);
#94096=AXIS2_PLACEMENT_3D('',#131333,#105214,#105215);
#94097=AXIS2_PLACEMENT_3D('',#131334,#105216,#105217);
#94098=AXIS2_PLACEMENT_3D('',#131335,#105218,#105219);
#94099=AXIS2_PLACEMENT_3D('',#131337,#105220,#105221);
#94100=AXIS2_PLACEMENT_3D('',#131339,#105223,#105224);
#94101=AXIS2_PLACEMENT_3D('',#131341,#105225,#105226);
#94102=AXIS2_PLACEMENT_3D('',#131342,#105227,#105228);
#94103=AXIS2_PLACEMENT_3D('',#131344,#105229,#105230);
#94104=AXIS2_PLACEMENT_3D('',#131346,#105232,#105233);
#94105=AXIS2_PLACEMENT_3D('',#131347,#105234,#105235);
#94106=AXIS2_PLACEMENT_3D('',#131352,#105237,#105238);
#94107=AXIS2_PLACEMENT_3D('',#131364,#105240,#105241);
#94108=AXIS2_PLACEMENT_3D('',#131369,#105242,#105243);
#94109=AXIS2_PLACEMENT_3D('',#131372,#105244,#105245);
#94110=AXIS2_PLACEMENT_3D('',#131376,#105247,#105248);
#94111=AXIS2_PLACEMENT_3D('',#131383,#105250,#105251);
#94112=AXIS2_PLACEMENT_3D('',#131385,#105252,#105253);
#94113=AXIS2_PLACEMENT_3D('',#131387,#105254,#105255);
#94114=AXIS2_PLACEMENT_3D('',#131388,#105256,#105257);
#94115=AXIS2_PLACEMENT_3D('',#131402,#105258,#105259);
#94116=AXIS2_PLACEMENT_3D('',#131413,#105260,#105261);
#94117=AXIS2_PLACEMENT_3D('',#131418,#105263,#105264);
#94118=AXIS2_PLACEMENT_3D('',#131421,#105266,#105267);
#94119=AXIS2_PLACEMENT_3D('',#131422,#105268,#105269);
#94120=AXIS2_PLACEMENT_3D('',#131533,#105281,#105282);
#94121=AXIS2_PLACEMENT_3D('',#131535,#105283,#105284);
#94122=AXIS2_PLACEMENT_3D('',#131537,#105285,#105286);
#94123=AXIS2_PLACEMENT_3D('',#131538,#105287,#105288);
#94124=AXIS2_PLACEMENT_3D('',#131539,#105289,#105290);
#94125=AXIS2_PLACEMENT_3D('',#131544,#105292,#105293);
#94126=AXIS2_PLACEMENT_3D('',#131547,#105295,#105296);
#94127=AXIS2_PLACEMENT_3D('',#131548,#105297,#105298);
#94128=AXIS2_PLACEMENT_3D('',#131551,#105301,#105302);
#94129=AXIS2_PLACEMENT_3D('',#131553,#105303,#105304);
#94130=AXIS2_PLACEMENT_3D('',#131555,#105305,#105306);
#94131=AXIS2_PLACEMENT_3D('',#131556,#105307,#105308);
#94132=AXIS2_PLACEMENT_3D('',#131557,#105309,#105310);
#94133=AXIS2_PLACEMENT_3D('',#131630,#105321,#105322);
#94134=AXIS2_PLACEMENT_3D('',#131658,#105324,#105325);
#94135=AXIS2_PLACEMENT_3D('',#131669,#105326,#105327);
#94136=AXIS2_PLACEMENT_3D('',#131678,#105328,#105329);
#94137=AXIS2_PLACEMENT_3D('',#131681,#105330,#105331);
#94138=AXIS2_PLACEMENT_3D('',#131684,#105334,#105335);
#94139=AXIS2_PLACEMENT_3D('',#131687,#105336,#105337);
#94140=AXIS2_PLACEMENT_3D('',#131688,#105338,#105339);
#94141=AXIS2_PLACEMENT_3D('',#131690,#105340,#105341);
#94142=AXIS2_PLACEMENT_3D('',#131691,#105342,#105343);
#94143=AXIS2_PLACEMENT_3D('',#131692,#105344,#105345);
#94144=AXIS2_PLACEMENT_3D('',#131695,#105346,#105347);
#94145=AXIS2_PLACEMENT_3D('',#131699,#105349,#105350);
#94146=AXIS2_PLACEMENT_3D('',#131700,#105351,#105352);
#94147=AXIS2_PLACEMENT_3D('',#131703,#105354,#105355);
#94148=AXIS2_PLACEMENT_3D('',#131782,#105356,#105357);
#94149=AXIS2_PLACEMENT_3D('',#131806,#105358,#105359);
#94150=AXIS2_PLACEMENT_3D('',#131808,#105360,#105361);
#94151=AXIS2_PLACEMENT_3D('',#131809,#105362,#105363);
#94152=AXIS2_PLACEMENT_3D('',#131879,#105364,#105365);
#94153=AXIS2_PLACEMENT_3D('',#131890,#105366,#105367);
#94154=AXIS2_PLACEMENT_3D('',#131893,#105368,#105369);
#94155=AXIS2_PLACEMENT_3D('',#131896,#105372,#105373);
#94156=AXIS2_PLACEMENT_3D('',#131899,#105374,#105375);
#94157=AXIS2_PLACEMENT_3D('',#131900,#105376,#105377);
#94158=AXIS2_PLACEMENT_3D('',#131902,#105378,#105379);
#94159=AXIS2_PLACEMENT_3D('',#131903,#105380,#105381);
#94160=AXIS2_PLACEMENT_3D('',#131904,#105382,#105383);
#94161=AXIS2_PLACEMENT_3D('',#131907,#105384,#105385);
#94162=AXIS2_PLACEMENT_3D('',#131911,#105387,#105388);
#94163=AXIS2_PLACEMENT_3D('',#131912,#105389,#105390);
#94164=AXIS2_PLACEMENT_3D('',#131940,#105392,#105393);
#94165=AXIS2_PLACEMENT_3D('',#131947,#105394,#105395);
#94166=AXIS2_PLACEMENT_3D('',#131949,#105396,#105397);
#94167=AXIS2_PLACEMENT_3D('',#131951,#105398,#105399);
#94168=AXIS2_PLACEMENT_3D('',#131952,#105400,#105401);
#94169=AXIS2_PLACEMENT_3D('',#132028,#105402,#105403);
#94170=AXIS2_PLACEMENT_3D('',#132066,#105404,#105405);
#94171=AXIS2_PLACEMENT_3D('',#132069,#105406,#105407);
#94172=AXIS2_PLACEMENT_3D('',#132072,#105410,#105411);
#94173=AXIS2_PLACEMENT_3D('',#132075,#105412,#105413);
#94174=AXIS2_PLACEMENT_3D('',#132076,#105414,#105415);
#94175=AXIS2_PLACEMENT_3D('',#132078,#105416,#105417);
#94176=AXIS2_PLACEMENT_3D('',#132079,#105418,#105419);
#94177=AXIS2_PLACEMENT_3D('',#132080,#105420,#105421);
#94178=AXIS2_PLACEMENT_3D('',#132083,#105422,#105423);
#94179=AXIS2_PLACEMENT_3D('',#132086,#105425,#105426);
#94180=AXIS2_PLACEMENT_3D('',#132163,#105428,#105429);
#94181=AXIS2_PLACEMENT_3D('',#132174,#105430,#105431);
#94182=AXIS2_PLACEMENT_3D('',#132175,#105432,#105433);
#94183=AXIS2_PLACEMENT_3D('',#132176,#105434,#105435);
#94184=AXIS2_PLACEMENT_3D('',#132177,#105436,#105437);
#94185=AXIS2_PLACEMENT_3D('',#132182,#105439,#105440);
#94186=AXIS2_PLACEMENT_3D('',#132204,#105442,#105443);
#94187=AXIS2_PLACEMENT_3D('',#132207,#105444,#105445);
#94188=AXIS2_PLACEMENT_3D('',#132208,#105446,#105447);
#94189=AXIS2_PLACEMENT_3D('',#132210,#105448,#105449);
#94190=AXIS2_PLACEMENT_3D('',#132215,#105450,#105451);
#94191=AXIS2_PLACEMENT_3D('',#132218,#105452,#105453);
#94192=AXIS2_PLACEMENT_3D('',#132221,#105455,#105456);
#94193=AXIS2_PLACEMENT_3D('',#132243,#105458,#105459);
#94194=AXIS2_PLACEMENT_3D('',#132256,#105460,#105461);
#94195=AXIS2_PLACEMENT_3D('',#132259,#105462,#105463);
#94196=AXIS2_PLACEMENT_3D('',#132260,#105464,#105465);
#94197=AXIS2_PLACEMENT_3D('',#132261,#105466,#105467);
#94198=AXIS2_PLACEMENT_3D('',#132294,#105468,#105469);
#94199=AXIS2_PLACEMENT_3D('',#132351,#105470,#105471);
#94200=AXIS2_PLACEMENT_3D('',#132355,#105473,#105474);
#94201=AXIS2_PLACEMENT_3D('',#132357,#105476,#105477);
#94202=AXIS2_PLACEMENT_3D('',#132360,#105478,#105479);
#94203=AXIS2_PLACEMENT_3D('',#132361,#105480,#105481);
#94204=AXIS2_PLACEMENT_3D('',#132363,#105482,#105483);
#94205=AXIS2_PLACEMENT_3D('',#132364,#105484,#105485);
#94206=AXIS2_PLACEMENT_3D('',#132365,#105486,#105487);
#94207=AXIS2_PLACEMENT_3D('',#132368,#105488,#105489);
#94208=AXIS2_PLACEMENT_3D('',#132371,#105491,#105492);
#94209=AXIS2_PLACEMENT_3D('',#132405,#105494,#105495);
#94210=AXIS2_PLACEMENT_3D('',#132473,#105496,#105497);
#94211=AXIS2_PLACEMENT_3D('',#132474,#105498,#105499);
#94212=AXIS2_PLACEMENT_3D('',#132475,#105500,#105501);
#94213=AXIS2_PLACEMENT_3D('',#132496,#105502,#105503);
#94214=AXIS2_PLACEMENT_3D('',#132509,#105504,#105505);
#94215=AXIS2_PLACEMENT_3D('',#132512,#105506,#105507);
#94216=AXIS2_PLACEMENT_3D('',#132515,#105510,#105511);
#94217=AXIS2_PLACEMENT_3D('',#132518,#105512,#105513);
#94218=AXIS2_PLACEMENT_3D('',#132519,#105514,#105515);
#94219=AXIS2_PLACEMENT_3D('',#132521,#105516,#105517);
#94220=AXIS2_PLACEMENT_3D('',#132522,#105518,#105519);
#94221=AXIS2_PLACEMENT_3D('',#132523,#105520,#105521);
#94222=AXIS2_PLACEMENT_3D('',#132526,#105522,#105523);
#94223=AXIS2_PLACEMENT_3D('',#132529,#105525,#105526);
#94224=AXIS2_PLACEMENT_3D('',#132563,#105528,#105529);
#94225=AXIS2_PLACEMENT_3D('',#132600,#105530,#105531);
#94226=AXIS2_PLACEMENT_3D('',#132601,#105532,#105533);
#94227=AXIS2_PLACEMENT_3D('',#132602,#105534,#105535);
#94228=AXIS2_PLACEMENT_3D('',#132641,#105536,#105537);
#94229=AXIS2_PLACEMENT_3D('',#132697,#105538,#105539);
#94230=AXIS2_PLACEMENT_3D('',#132700,#105540,#105541);
#94231=AXIS2_PLACEMENT_3D('',#132716,#105544,#105545);
#94232=AXIS2_PLACEMENT_3D('',#132718,#105546,#105547);
#94233=AXIS2_PLACEMENT_3D('',#132723,#105548,#105549);
#94234=AXIS2_PLACEMENT_3D('',#132725,#105550,#105551);
#94235=AXIS2_PLACEMENT_3D('',#132726,#105552,#105553);
#94236=AXIS2_PLACEMENT_3D('',#132740,#105554,#105555);
#94237=AXIS2_PLACEMENT_3D('',#132751,#105556,#105557);
#94238=AXIS2_PLACEMENT_3D('',#132756,#105559,#105560);
#94239=AXIS2_PLACEMENT_3D('',#132767,#105562,#105563);
#94240=AXIS2_PLACEMENT_3D('',#132768,#105564,#105565);
#94241=AXIS2_PLACEMENT_3D('',#132769,#105566,#105567);
#94242=AXIS2_PLACEMENT_3D('',#132770,#105568,#105569);
#94243=AXIS2_PLACEMENT_3D('',#132783,#105571,#105572);
#94244=AXIS2_PLACEMENT_3D('',#132831,#105574,#105575);
#94245=AXIS2_PLACEMENT_3D('',#132842,#105577,#105578);
#94246=AXIS2_PLACEMENT_3D('',#132855,#105580,#105581);
#94247=AXIS2_PLACEMENT_3D('',#132912,#105583,#105584);
#94248=AXIS2_PLACEMENT_3D('',#132927,#105586,#105587);
#94249=AXIS2_PLACEMENT_3D('',#132954,#105589,#105590);
#94250=AXIS2_PLACEMENT_3D('',#133002,#105592,#105593);
#94251=AXIS2_PLACEMENT_3D('',#133053,#105595,#105596);
#94252=AXIS2_PLACEMENT_3D('',#133101,#105598,#105599);
#94253=AXIS2_PLACEMENT_3D('',#133114,#105601,#105602);
#94254=AXIS2_PLACEMENT_3D('',#133136,#105604,#105605);
#94255=AXIS2_PLACEMENT_3D('',#133142,#105606,#105607);
#94256=AXIS2_PLACEMENT_3D('',#133143,#105608,#105609);
#94257=AXIS2_PLACEMENT_3D('',#133145,#105610,#105611);
#94258=AXIS2_PLACEMENT_3D('',#133146,#105612,#105613);
#94259=AXIS2_PLACEMENT_3D('',#133166,#105614,#105615);
#94260=AXIS2_PLACEMENT_3D('',#133173,#105616,#105617);
#94261=AXIS2_PLACEMENT_3D('',#133178,#105619,#105620);
#94262=AXIS2_PLACEMENT_3D('',#133181,#105622,#105623);
#94263=AXIS2_PLACEMENT_3D('',#133182,#105624,#105625);
#94264=AXIS2_PLACEMENT_3D('',#133232,#105632,#105633);
#94265=AXIS2_PLACEMENT_3D('',#133257,#105639,#105640);
#94266=AXIS2_PLACEMENT_3D('',#133259,#105641,#105642);
#94267=AXIS2_PLACEMENT_3D('',#133261,#105643,#105644);
#94268=AXIS2_PLACEMENT_3D('',#133262,#105645,#105646);
#94269=AXIS2_PLACEMENT_3D('',#133263,#105647,#105648);
#94270=AXIS2_PLACEMENT_3D('',#133268,#105650,#105651);
#94271=AXIS2_PLACEMENT_3D('',#133271,#105653,#105654);
#94272=AXIS2_PLACEMENT_3D('',#133272,#105655,#105656);
#94273=AXIS2_PLACEMENT_3D('',#133275,#105659,#105660);
#94274=AXIS2_PLACEMENT_3D('',#133277,#105661,#105662);
#94275=AXIS2_PLACEMENT_3D('',#133279,#105663,#105664);
#94276=AXIS2_PLACEMENT_3D('',#133280,#105665,#105666);
#94277=AXIS2_PLACEMENT_3D('',#133281,#105667,#105668);
#94278=AXIS2_PLACEMENT_3D('',#133366,#105678,#105679);
#94279=AXIS2_PLACEMENT_3D('',#133373,#105680,#105681);
#94280=AXIS2_PLACEMENT_3D('',#133375,#105682,#105683);
#94281=AXIS2_PLACEMENT_3D('',#133377,#105685,#105686);
#94282=AXIS2_PLACEMENT_3D('',#133380,#105687,#105688);
#94283=AXIS2_PLACEMENT_3D('',#133381,#105689,#105690);
#94284=AXIS2_PLACEMENT_3D('',#133382,#105691,#105692);
#94285=AXIS2_PLACEMENT_3D('',#133383,#105693,#105694);
#94286=AXIS2_PLACEMENT_3D('',#133385,#105695,#105696);
#94287=AXIS2_PLACEMENT_3D('',#133388,#105698,#105699);
#94288=AXIS2_PLACEMENT_3D('',#133414,#105700,#105701);
#94289=AXIS2_PLACEMENT_3D('',#133423,#105702,#105703);
#94290=AXIS2_PLACEMENT_3D('',#133425,#105704,#105705);
#94291=AXIS2_PLACEMENT_3D('',#133426,#105706,#105707);
#94292=AXIS2_PLACEMENT_3D('',#133458,#105708,#105709);
#94293=AXIS2_PLACEMENT_3D('',#133469,#105710,#105711);
#94294=AXIS2_PLACEMENT_3D('',#133471,#105712,#105713);
#94295=AXIS2_PLACEMENT_3D('',#133473,#105715,#105716);
#94296=AXIS2_PLACEMENT_3D('',#133476,#105717,#105718);
#94297=AXIS2_PLACEMENT_3D('',#133477,#105719,#105720);
#94298=AXIS2_PLACEMENT_3D('',#133478,#105721,#105722);
#94299=AXIS2_PLACEMENT_3D('',#133479,#105723,#105724);
#94300=AXIS2_PLACEMENT_3D('',#133481,#105725,#105726);
#94301=AXIS2_PLACEMENT_3D('',#133483,#105727,#105728);
#94302=AXIS2_PLACEMENT_3D('',#133516,#105730,#105731);
#94303=AXIS2_PLACEMENT_3D('',#133540,#105732,#105733);
#94304=AXIS2_PLACEMENT_3D('',#133541,#105734,#105735);
#94305=AXIS2_PLACEMENT_3D('',#133579,#105736,#105737);
#94306=AXIS2_PLACEMENT_3D('',#133629,#105738,#105739);
#94307=AXIS2_PLACEMENT_3D('',#133631,#105740,#105741);
#94308=AXIS2_PLACEMENT_3D('',#133633,#105743,#105744);
#94309=AXIS2_PLACEMENT_3D('',#133636,#105745,#105746);
#94310=AXIS2_PLACEMENT_3D('',#133637,#105747,#105748);
#94311=AXIS2_PLACEMENT_3D('',#133638,#105749,#105750);
#94312=AXIS2_PLACEMENT_3D('',#133639,#105751,#105752);
#94313=AXIS2_PLACEMENT_3D('',#133641,#105753,#105754);
#94314=AXIS2_PLACEMENT_3D('',#133643,#105755,#105756);
#94315=AXIS2_PLACEMENT_3D('',#133676,#105758,#105759);
#94316=AXIS2_PLACEMENT_3D('',#133739,#105760,#105761);
#94317=AXIS2_PLACEMENT_3D('',#133740,#105762,#105763);
#94318=AXIS2_PLACEMENT_3D('',#133772,#105764,#105765);
#94319=AXIS2_PLACEMENT_3D('',#133822,#105766,#105767);
#94320=AXIS2_PLACEMENT_3D('',#133824,#105768,#105769);
#94321=AXIS2_PLACEMENT_3D('',#133826,#105771,#105772);
#94322=AXIS2_PLACEMENT_3D('',#133829,#105773,#105774);
#94323=AXIS2_PLACEMENT_3D('',#133830,#105775,#105776);
#94324=AXIS2_PLACEMENT_3D('',#133831,#105777,#105778);
#94325=AXIS2_PLACEMENT_3D('',#133832,#105779,#105780);
#94326=AXIS2_PLACEMENT_3D('',#133834,#105781,#105782);
#94327=AXIS2_PLACEMENT_3D('',#133836,#105783,#105784);
#94328=AXIS2_PLACEMENT_3D('',#133869,#105786,#105787);
#94329=AXIS2_PLACEMENT_3D('',#133893,#105788,#105789);
#94330=AXIS2_PLACEMENT_3D('',#133894,#105790,#105791);
#94331=AXIS2_PLACEMENT_3D('',#133920,#105792,#105793);
#94332=AXIS2_PLACEMENT_3D('',#133929,#105794,#105795);
#94333=AXIS2_PLACEMENT_3D('',#133931,#105796,#105797);
#94334=AXIS2_PLACEMENT_3D('',#133933,#105799,#105800);
#94335=AXIS2_PLACEMENT_3D('',#133936,#105801,#105802);
#94336=AXIS2_PLACEMENT_3D('',#133937,#105803,#105804);
#94337=AXIS2_PLACEMENT_3D('',#133938,#105805,#105806);
#94338=AXIS2_PLACEMENT_3D('',#133939,#105807,#105808);
#94339=AXIS2_PLACEMENT_3D('',#133941,#105809,#105810);
#94340=AXIS2_PLACEMENT_3D('',#133944,#105812,#105813);
#94341=AXIS2_PLACEMENT_3D('',#133964,#105814,#105815);
#94342=AXIS2_PLACEMENT_3D('',#133971,#105816,#105817);
#94343=AXIS2_PLACEMENT_3D('',#133973,#105818,#105819);
#94344=AXIS2_PLACEMENT_3D('',#133974,#105820,#105821);
#94345=AXIS2_PLACEMENT_3D('',#134006,#105822,#105823);
#94346=AXIS2_PLACEMENT_3D('',#134044,#105824,#105825);
#94347=AXIS2_PLACEMENT_3D('',#134046,#105826,#105827);
#94348=AXIS2_PLACEMENT_3D('',#134048,#105829,#105830);
#94349=AXIS2_PLACEMENT_3D('',#134051,#105831,#105832);
#94350=AXIS2_PLACEMENT_3D('',#134052,#105833,#105834);
#94351=AXIS2_PLACEMENT_3D('',#134053,#105835,#105836);
#94352=AXIS2_PLACEMENT_3D('',#134054,#105837,#105838);
#94353=AXIS2_PLACEMENT_3D('',#134056,#105839,#105840);
#94354=AXIS2_PLACEMENT_3D('',#134059,#105842,#105843);
#94355=AXIS2_PLACEMENT_3D('',#134092,#105844,#105845);
#94356=AXIS2_PLACEMENT_3D('',#134116,#105847,#105848);
#94357=AXIS2_PLACEMENT_3D('',#134118,#105849,#105850);
#94358=AXIS2_PLACEMENT_3D('',#134120,#105851,#105852);
#94359=AXIS2_PLACEMENT_3D('',#134141,#105854,#105855);
#94360=AXIS2_PLACEMENT_3D('',#134148,#105856,#105857);
#94361=AXIS2_PLACEMENT_3D('',#134150,#105858,#105859);
#94362=AXIS2_PLACEMENT_3D('',#134171,#105861,#105862);
#94363=AXIS2_PLACEMENT_3D('',#134178,#105863,#105864);
#94364=AXIS2_PLACEMENT_3D('',#134180,#105865,#105866);
#94365=AXIS2_PLACEMENT_3D('',#134182,#105868,#105869);
#94366=AXIS2_PLACEMENT_3D('',#134214,#105871,#105872);
#94367=AXIS2_PLACEMENT_3D('',#134221,#105873,#105874);
#94368=AXIS2_PLACEMENT_3D('',#134223,#105875,#105876);
#94369=AXIS2_PLACEMENT_3D('',#134244,#105878,#105879);
#94370=AXIS2_PLACEMENT_3D('',#134258,#105880,#105881);
#94371=AXIS2_PLACEMENT_3D('',#134271,#105883,#105884);
#94372=AXIS2_PLACEMENT_3D('',#134273,#105885,#105886);
#94373=AXIS2_PLACEMENT_3D('',#134275,#105887,#105888);
#94374=AXIS2_PLACEMENT_3D('',#134296,#105890,#105891);
#94375=AXIS2_PLACEMENT_3D('',#134303,#105892,#105893);
#94376=AXIS2_PLACEMENT_3D('',#134305,#105894,#105895);
#94377=AXIS2_PLACEMENT_3D('',#134326,#105897,#105898);
#94378=AXIS2_PLACEMENT_3D('',#134333,#105899,#105900);
#94379=AXIS2_PLACEMENT_3D('',#134335,#105901,#105902);
#94380=AXIS2_PLACEMENT_3D('',#134337,#105904,#105905);
#94381=AXIS2_PLACEMENT_3D('',#134358,#105907,#105908);
#94382=AXIS2_PLACEMENT_3D('',#134365,#105909,#105910);
#94383=AXIS2_PLACEMENT_3D('',#134389,#105912,#105913);
#94384=AXIS2_PLACEMENT_3D('',#134391,#105914,#105915);
#94385=AXIS2_PLACEMENT_3D('',#134394,#105917,#105918);
#94386=AXIS2_PLACEMENT_3D('',#134414,#105919,#105920);
#94387=AXIS2_PLACEMENT_3D('',#134421,#105921,#105922);
#94388=AXIS2_PLACEMENT_3D('',#134423,#105923,#105924);
#94389=AXIS2_PLACEMENT_3D('',#134444,#105926,#105927);
#94390=AXIS2_PLACEMENT_3D('',#134451,#105928,#105929);
#94391=AXIS2_PLACEMENT_3D('',#134453,#105930,#105931);
#94392=AXIS2_PLACEMENT_3D('',#134492,#105933,#105934);
#94393=AXIS2_PLACEMENT_3D('',#134505,#105936,#105937);
#94394=AXIS2_PLACEMENT_3D('',#134507,#105938,#105939);
#94395=AXIS2_PLACEMENT_3D('',#134509,#105940,#105941);
#94396=AXIS2_PLACEMENT_3D('',#134530,#105943,#105944);
#94397=AXIS2_PLACEMENT_3D('',#134537,#105945,#105946);
#94398=AXIS2_PLACEMENT_3D('',#134539,#105947,#105948);
#94399=AXIS2_PLACEMENT_3D('',#134560,#105950,#105951);
#94400=AXIS2_PLACEMENT_3D('',#134567,#105952,#105953);
#94401=AXIS2_PLACEMENT_3D('',#134569,#105954,#105955);
#94402=AXIS2_PLACEMENT_3D('',#134571,#105957,#105958);
#94403=AXIS2_PLACEMENT_3D('',#134573,#105960,#105961);
#94404=AXIS2_PLACEMENT_3D('',#134597,#105963,#105964);
#94405=AXIS2_PLACEMENT_3D('',#134599,#105965,#105966);
#94406=AXIS2_PLACEMENT_3D('',#134602,#105968,#105969);
#94407=AXIS2_PLACEMENT_3D('',#134622,#105970,#105971);
#94408=AXIS2_PLACEMENT_3D('',#134629,#105972,#105973);
#94409=AXIS2_PLACEMENT_3D('',#134631,#105974,#105975);
#94410=AXIS2_PLACEMENT_3D('',#134652,#105977,#105978);
#94411=AXIS2_PLACEMENT_3D('',#134659,#105979,#105980);
#94412=AXIS2_PLACEMENT_3D('',#134661,#105981,#105982);
#94413=AXIS2_PLACEMENT_3D('',#134663,#105984,#105985);
#94414=AXIS2_PLACEMENT_3D('',#134689,#105987,#105988);
#94415=AXIS2_PLACEMENT_3D('',#134690,#105989,#105990);
#94416=AXIS2_PLACEMENT_3D('',#134691,#105991,#105992);
#94417=AXIS2_PLACEMENT_3D('',#134693,#105993,#105994);
#94418=AXIS2_PLACEMENT_3D('',#134714,#105996,#105997);
#94419=AXIS2_PLACEMENT_3D('',#134723,#105998,#105999);
#94420=AXIS2_PLACEMENT_3D('',#134737,#106000,#106001);
#94421=AXIS2_PLACEMENT_3D('',#134750,#106003,#106004);
#94422=AXIS2_PLACEMENT_3D('',#134752,#106005,#106006);
#94423=AXIS2_PLACEMENT_3D('',#134754,#106007,#106008);
#94424=AXIS2_PLACEMENT_3D('',#134775,#106010,#106011);
#94425=AXIS2_PLACEMENT_3D('',#134782,#106012,#106013);
#94426=AXIS2_PLACEMENT_3D('',#134784,#106014,#106015);
#94427=AXIS2_PLACEMENT_3D('',#134805,#106017,#106018);
#94428=AXIS2_PLACEMENT_3D('',#134812,#106019,#106020);
#94429=AXIS2_PLACEMENT_3D('',#134814,#106021,#106022);
#94430=AXIS2_PLACEMENT_3D('',#134842,#106024,#106025);
#94431=AXIS2_PLACEMENT_3D('',#134849,#106026,#106027);
#94432=AXIS2_PLACEMENT_3D('',#134851,#106028,#106029);
#94433=AXIS2_PLACEMENT_3D('',#134854,#106031,#106032);
#94434=AXIS2_PLACEMENT_3D('',#134867,#106033,#106034);
#94435=AXIS2_PLACEMENT_3D('',#134868,#106035,#106036);
#94436=AXIS2_PLACEMENT_3D('',#134881,#106038,#106039);
#94437=AXIS2_PLACEMENT_3D('',#134883,#106040,#106041);
#94438=AXIS2_PLACEMENT_3D('',#134885,#106042,#106043);
#94439=AXIS2_PLACEMENT_3D('',#134906,#106045,#106046);
#94440=AXIS2_PLACEMENT_3D('',#134913,#106047,#106048);
#94441=AXIS2_PLACEMENT_3D('',#134915,#106049,#106050);
#94442=AXIS2_PLACEMENT_3D('',#134936,#106052,#106053);
#94443=AXIS2_PLACEMENT_3D('',#134943,#106054,#106055);
#94444=AXIS2_PLACEMENT_3D('',#134945,#106056,#106057);
#94445=AXIS2_PLACEMENT_3D('',#134947,#106059,#106060);
#94446=AXIS2_PLACEMENT_3D('',#134971,#106062,#106063);
#94447=AXIS2_PLACEMENT_3D('',#134973,#106064,#106065);
#94448=AXIS2_PLACEMENT_3D('',#134975,#106066,#106067);
#94449=AXIS2_PLACEMENT_3D('',#134996,#106069,#106070);
#94450=AXIS2_PLACEMENT_3D('',#135003,#106071,#106072);
#94451=AXIS2_PLACEMENT_3D('',#135005,#106073,#106074);
#94452=AXIS2_PLACEMENT_3D('',#135026,#106076,#106077);
#94453=AXIS2_PLACEMENT_3D('',#135028,#106078,#106079);
#94454=AXIS2_PLACEMENT_3D('',#135035,#106080,#106081);
#94455=AXIS2_PLACEMENT_3D('',#135037,#106082,#106083);
#94456=AXIS2_PLACEMENT_3D('',#135039,#106084,#106085);
#94457=AXIS2_PLACEMENT_3D('',#135041,#106087,#106088);
#94458=AXIS2_PLACEMENT_3D('',#135054,#106090,#106091);
#94459=AXIS2_PLACEMENT_3D('',#135058,#106093,#106094);
#94460=AXIS2_PLACEMENT_3D('',#135060,#106095,#106096);
#94461=AXIS2_PLACEMENT_3D('',#135062,#106097,#106098);
#94462=AXIS2_PLACEMENT_3D('',#135066,#106100,#106101);
#94463=AXIS2_PLACEMENT_3D('',#135068,#106103,#106104);
#94464=AXIS2_PLACEMENT_3D('',#135072,#106106,#106107);
#94465=AXIS2_PLACEMENT_3D('',#135074,#106108,#106109);
#94466=AXIS2_PLACEMENT_3D('',#135076,#106111,#106112);
#94467=AXIS2_PLACEMENT_3D('',#135082,#106116,#106117);
#94468=AXIS2_PLACEMENT_3D('',#135085,#106119,#106120);
#94469=AXIS2_PLACEMENT_3D('',#135100,#106121,#106122);
#94470=AXIS2_PLACEMENT_3D('',#135101,#106123,#106124);
#94471=AXIS2_PLACEMENT_3D('',#135102,#106125,#106126);
#94472=AXIS2_PLACEMENT_3D('',#135121,#106127,#106128);
#94473=AXIS2_PLACEMENT_3D('',#135225,#106129,#106130);
#94474=AXIS2_PLACEMENT_3D('',#135232,#106131,#106132);
#94475=AXIS2_PLACEMENT_3D('',#135235,#106133,#106134);
#94476=AXIS2_PLACEMENT_3D('',#135237,#106135,#106136);
#94477=AXIS2_PLACEMENT_3D('',#135239,#106137,#106138);
#94478=AXIS2_PLACEMENT_3D('',#135240,#106139,#106140);
#94479=AXIS2_PLACEMENT_3D('',#135241,#106141,#106142);
#94480=AXIS2_PLACEMENT_3D('',#135245,#106144,#106145);
#94481=AXIS2_PLACEMENT_3D('',#135247,#106147,#106148);
#94482=AXIS2_PLACEMENT_3D('',#135283,#106151,#106152);
#94483=AXIS2_PLACEMENT_3D('',#135286,#106154,#106155);
#94484=AXIS2_PLACEMENT_3D('',#135287,#106156,#106157);
#94485=AXIS2_PLACEMENT_3D('',#135291,#106159,#106160);
#94486=AXIS2_PLACEMENT_3D('',#135293,#106162,#106163);
#94487=AXIS2_PLACEMENT_3D('',#135295,#106164,#106165);
#94488=AXIS2_PLACEMENT_3D('',#135297,#106166,#106167);
#94489=AXIS2_PLACEMENT_3D('',#135298,#106168,#106169);
#94490=AXIS2_PLACEMENT_3D('',#135299,#106170,#106171);
#94491=AXIS2_PLACEMENT_3D('',#135303,#106173,#106174);
#94492=AXIS2_PLACEMENT_3D('',#135305,#106176,#106177);
#94493=AXIS2_PLACEMENT_3D('',#135307,#106178,#106179);
#94494=AXIS2_PLACEMENT_3D('',#135309,#106180,#106181);
#94495=AXIS2_PLACEMENT_3D('',#135310,#106182,#106183);
#94496=AXIS2_PLACEMENT_3D('',#135311,#106184,#106185);
#94497=AXIS2_PLACEMENT_3D('',#135315,#106187,#106188);
#94498=AXIS2_PLACEMENT_3D('',#135317,#106190,#106191);
#94499=AXIS2_PLACEMENT_3D('',#135320,#106192,#106193);
#94500=AXIS2_PLACEMENT_3D('',#135322,#106194,#106195);
#94501=AXIS2_PLACEMENT_3D('',#135324,#106196,#106197);
#94502=AXIS2_PLACEMENT_3D('',#135338,#106198,#106199);
#94503=AXIS2_PLACEMENT_3D('',#135382,#106200,#106201);
#94504=AXIS2_PLACEMENT_3D('',#135384,#106202,#106203);
#94505=AXIS2_PLACEMENT_3D('',#135388,#106205,#106206);
#94506=AXIS2_PLACEMENT_3D('',#135390,#106208,#106209);
#94507=AXIS2_PLACEMENT_3D('',#135392,#106210,#106211);
#94508=AXIS2_PLACEMENT_3D('',#135394,#106212,#106213);
#94509=AXIS2_PLACEMENT_3D('',#135395,#106214,#106215);
#94510=AXIS2_PLACEMENT_3D('',#135396,#106216,#106217);
#94511=AXIS2_PLACEMENT_3D('',#135400,#106219,#106220);
#94512=AXIS2_PLACEMENT_3D('',#135402,#106222,#106223);
#94513=AXIS2_PLACEMENT_3D('',#135404,#106224,#106225);
#94514=AXIS2_PLACEMENT_3D('',#135406,#106226,#106227);
#94515=AXIS2_PLACEMENT_3D('',#135407,#106228,#106229);
#94516=AXIS2_PLACEMENT_3D('',#135408,#106230,#106231);
#94517=AXIS2_PLACEMENT_3D('',#135412,#106233,#106234);
#94518=AXIS2_PLACEMENT_3D('',#135414,#106236,#106237);
#94519=AXIS2_PLACEMENT_3D('',#135416,#106238,#106239);
#94520=AXIS2_PLACEMENT_3D('',#135418,#106240,#106241);
#94521=AXIS2_PLACEMENT_3D('',#135419,#106242,#106243);
#94522=AXIS2_PLACEMENT_3D('',#135446,#106244,#106245);
#94523=AXIS2_PLACEMENT_3D('',#135464,#106246,#106247);
#94524=AXIS2_PLACEMENT_3D('',#135469,#106250,#106251);
#94525=AXIS2_PLACEMENT_3D('',#135470,#106252,#106253);
#94526=AXIS2_PLACEMENT_3D('',#135472,#106254,#106255);
#94527=AXIS2_PLACEMENT_3D('',#135476,#106257,#106258);
#94528=AXIS2_PLACEMENT_3D('',#135478,#106260,#106261);
#94529=AXIS2_PLACEMENT_3D('',#135480,#106262,#106263);
#94530=AXIS2_PLACEMENT_3D('',#135482,#106264,#106265);
#94531=AXIS2_PLACEMENT_3D('',#135483,#106266,#106267);
#94532=AXIS2_PLACEMENT_3D('',#135484,#106268,#106269);
#94533=AXIS2_PLACEMENT_3D('',#135488,#106271,#106272);
#94534=AXIS2_PLACEMENT_3D('',#135490,#106274,#106275);
#94535=AXIS2_PLACEMENT_3D('',#135492,#106276,#106277);
#94536=AXIS2_PLACEMENT_3D('',#135494,#106278,#106279);
#94537=AXIS2_PLACEMENT_3D('',#135495,#106280,#106281);
#94538=AXIS2_PLACEMENT_3D('',#135496,#106282,#106283);
#94539=AXIS2_PLACEMENT_3D('',#135500,#106285,#106286);
#94540=AXIS2_PLACEMENT_3D('',#135502,#106288,#106289);
#94541=AXIS2_PLACEMENT_3D('',#135506,#106291,#106292);
#94542=AXIS2_PLACEMENT_3D('',#135509,#106294,#106295);
#94543=AXIS2_PLACEMENT_3D('',#135510,#106296,#106297);
#94544=AXIS2_PLACEMENT_3D('',#135512,#106298,#106299);
#94545=AXIS2_PLACEMENT_3D('',#135516,#106301,#106302);
#94546=AXIS2_PLACEMENT_3D('',#135518,#106304,#106305);
#94547=AXIS2_PLACEMENT_3D('',#135520,#106306,#106307);
#94548=AXIS2_PLACEMENT_3D('',#135522,#106308,#106309);
#94549=AXIS2_PLACEMENT_3D('',#135523,#106310,#106311);
#94550=AXIS2_PLACEMENT_3D('',#135524,#106312,#106313);
#94551=AXIS2_PLACEMENT_3D('',#135528,#106315,#106316);
#94552=AXIS2_PLACEMENT_3D('',#135530,#106318,#106319);
#94553=AXIS2_PLACEMENT_3D('',#135532,#106320,#106321);
#94554=AXIS2_PLACEMENT_3D('',#135534,#106322,#106323);
#94555=AXIS2_PLACEMENT_3D('',#135535,#106324,#106325);
#94556=AXIS2_PLACEMENT_3D('',#135536,#106326,#106327);
#94557=AXIS2_PLACEMENT_3D('',#135540,#106329,#106330);
#94558=AXIS2_PLACEMENT_3D('',#135542,#106332,#106333);
#94559=AXIS2_PLACEMENT_3D('',#135546,#106335,#106336);
#94560=AXIS2_PLACEMENT_3D('',#135549,#106338,#106339);
#94561=AXIS2_PLACEMENT_3D('',#135550,#106340,#106341);
#94562=AXIS2_PLACEMENT_3D('',#135552,#106342,#106343);
#94563=AXIS2_PLACEMENT_3D('',#135555,#106346,#106347);
#94564=AXIS2_PLACEMENT_3D('',#135610,#106354,#106355);
#94565=AXIS2_PLACEMENT_3D('',#135612,#106356,#106357);
#94566=AXIS2_PLACEMENT_3D('',#135625,#106359,#106360);
#94567=AXIS2_PLACEMENT_3D('',#135628,#106361,#106362);
#94568=AXIS2_PLACEMENT_3D('',#135630,#106363,#106364);
#94569=AXIS2_PLACEMENT_3D('',#135632,#106365,#106366);
#94570=AXIS2_PLACEMENT_3D('',#135633,#106367,#106368);
#94571=AXIS2_PLACEMENT_3D('',#135634,#106369,#106370);
#94572=AXIS2_PLACEMENT_3D('',#135636,#106371,#106372);
#94573=AXIS2_PLACEMENT_3D('',#135639,#106375,#106376);
#94574=AXIS2_PLACEMENT_3D('',#135643,#106378,#106379);
#94575=AXIS2_PLACEMENT_3D('',#135645,#106381,#106382);
#94576=AXIS2_PLACEMENT_3D('',#135647,#106383,#106384);
#94577=AXIS2_PLACEMENT_3D('',#135649,#106385,#106386);
#94578=AXIS2_PLACEMENT_3D('',#135650,#106387,#106388);
#94579=AXIS2_PLACEMENT_3D('',#135651,#106389,#106390);
#94580=AXIS2_PLACEMENT_3D('',#135654,#106391,#106392);
#94581=AXIS2_PLACEMENT_3D('',#135657,#106395,#106396);
#94582=AXIS2_PLACEMENT_3D('',#135660,#106397,#106398);
#94583=AXIS2_PLACEMENT_3D('',#135661,#106399,#106400);
#94584=AXIS2_PLACEMENT_3D('',#135662,#106401,#106402);
#94585=AXIS2_PLACEMENT_3D('',#135663,#106403,#106404);
#94586=AXIS2_PLACEMENT_3D('',#135666,#106405,#106406);
#94587=AXIS2_PLACEMENT_3D('',#135667,#106407,#106408);
#94588=AXIS2_PLACEMENT_3D('',#135668,#106409,#106410);
#94589=AXIS2_PLACEMENT_3D('',#135669,#106411,#106412);
#94590=AXIS2_PLACEMENT_3D('',#135672,#106413,#106414);
#94591=AXIS2_PLACEMENT_3D('',#135673,#106415,#106416);
#94592=AXIS2_PLACEMENT_3D('',#135674,#106417,#106418);
#94593=AXIS2_PLACEMENT_3D('',#135675,#106419,#106420);
#94594=AXIS2_PLACEMENT_3D('',#135678,#106421,#106422);
#94595=AXIS2_PLACEMENT_3D('',#135681,#106425,#106426);
#94596=AXIS2_PLACEMENT_3D('',#135684,#106427,#106428);
#94597=AXIS2_PLACEMENT_3D('',#135685,#106429,#106430);
#94598=AXIS2_PLACEMENT_3D('',#135686,#106431,#106432);
#94599=AXIS2_PLACEMENT_3D('',#135687,#106433,#106434);
#94600=AXIS2_PLACEMENT_3D('',#135690,#106435,#106436);
#94601=AXIS2_PLACEMENT_3D('',#135691,#106437,#106438);
#94602=AXIS2_PLACEMENT_3D('',#135692,#106439,#106440);
#94603=AXIS2_PLACEMENT_3D('',#135693,#106441,#106442);
#94604=AXIS2_PLACEMENT_3D('',#135696,#106443,#106444);
#94605=AXIS2_PLACEMENT_3D('',#135697,#106445,#106446);
#94606=AXIS2_PLACEMENT_3D('',#135698,#106447,#106448);
#94607=AXIS2_PLACEMENT_3D('',#135699,#106449,#106450);
#94608=AXIS2_PLACEMENT_3D('',#135702,#106451,#106452);
#94609=AXIS2_PLACEMENT_3D('',#135705,#106455,#106456);
#94610=AXIS2_PLACEMENT_3D('',#135708,#106457,#106458);
#94611=AXIS2_PLACEMENT_3D('',#135709,#106459,#106460);
#94612=AXIS2_PLACEMENT_3D('',#135710,#106461,#106462);
#94613=AXIS2_PLACEMENT_3D('',#135711,#106463,#106464);
#94614=AXIS2_PLACEMENT_3D('',#135714,#106465,#106466);
#94615=AXIS2_PLACEMENT_3D('',#135715,#106467,#106468);
#94616=AXIS2_PLACEMENT_3D('',#135716,#106469,#106470);
#94617=AXIS2_PLACEMENT_3D('',#135717,#106471,#106472);
#94618=AXIS2_PLACEMENT_3D('',#135720,#106473,#106474);
#94619=AXIS2_PLACEMENT_3D('',#135721,#106475,#106476);
#94620=AXIS2_PLACEMENT_3D('',#135722,#106477,#106478);
#94621=AXIS2_PLACEMENT_3D('',#135723,#106479,#106480);
#94622=AXIS2_PLACEMENT_3D('',#135726,#106481,#106482);
#94623=AXIS2_PLACEMENT_3D('',#135729,#106485,#106486);
#94624=AXIS2_PLACEMENT_3D('',#135732,#106487,#106488);
#94625=AXIS2_PLACEMENT_3D('',#135733,#106489,#106490);
#94626=AXIS2_PLACEMENT_3D('',#135734,#106491,#106492);
#94627=AXIS2_PLACEMENT_3D('',#135735,#106493,#106494);
#94628=AXIS2_PLACEMENT_3D('',#135765,#106495,#106496);
#94629=AXIS2_PLACEMENT_3D('',#135768,#106498,#106499);
#94630=AXIS2_PLACEMENT_3D('',#135770,#106500,#106501);
#94631=AXIS2_PLACEMENT_3D('',#135790,#106502,#106503);
#94632=AXIS2_PLACEMENT_3D('',#135791,#106504,#106505);
#94633=AXIS2_PLACEMENT_3D('',#135794,#106506,#106507);
#94634=AXIS2_PLACEMENT_3D('',#135806,#106509,#106510);
#94635=AXIS2_PLACEMENT_3D('',#135817,#106511,#106512);
#94636=AXIS2_PLACEMENT_3D('',#135868,#106513,#106514);
#94637=AXIS2_PLACEMENT_3D('',#135881,#106515,#106516);
#94638=AXIS2_PLACEMENT_3D('',#135925,#106517,#106518);
#94639=AXIS2_PLACEMENT_3D('',#135929,#106520,#106521);
#94640=AXIS2_PLACEMENT_3D('',#135931,#106523,#106524);
#94641=AXIS2_PLACEMENT_3D('',#135933,#106525,#106526);
#94642=AXIS2_PLACEMENT_3D('',#135935,#106527,#106528);
#94643=AXIS2_PLACEMENT_3D('',#135937,#106529,#106530);
#94644=AXIS2_PLACEMENT_3D('',#135938,#106531,#106532);
#94645=AXIS2_PLACEMENT_3D('',#135939,#106533,#106534);
#94646=AXIS2_PLACEMENT_3D('',#135942,#106535,#106536);
#94647=AXIS2_PLACEMENT_3D('',#135945,#106538,#106539);
#94648=AXIS2_PLACEMENT_3D('',#135979,#106541,#106542);
#94649=AXIS2_PLACEMENT_3D('',#136063,#106543,#106544);
#94650=AXIS2_PLACEMENT_3D('',#136066,#106545,#106546);
#94651=AXIS2_PLACEMENT_3D('',#136067,#106547,#106548);
#94652=AXIS2_PLACEMENT_3D('',#136068,#106549,#106550);
#94653=AXIS2_PLACEMENT_3D('',#136095,#106551,#106552);
#94654=AXIS2_PLACEMENT_3D('',#136102,#106553,#106554);
#94655=AXIS2_PLACEMENT_3D('',#136106,#106556,#106557);
#94656=AXIS2_PLACEMENT_3D('',#136108,#106559,#106560);
#94657=AXIS2_PLACEMENT_3D('',#136110,#106561,#106562);
#94658=AXIS2_PLACEMENT_3D('',#136112,#106563,#106564);
#94659=AXIS2_PLACEMENT_3D('',#136114,#106565,#106566);
#94660=AXIS2_PLACEMENT_3D('',#136115,#106567,#106568);
#94661=AXIS2_PLACEMENT_3D('',#136116,#106569,#106570);
#94662=AXIS2_PLACEMENT_3D('',#136119,#106571,#106572);
#94663=AXIS2_PLACEMENT_3D('',#136122,#106574,#106575);
#94664=AXIS2_PLACEMENT_3D('',#136150,#106577,#106578);
#94665=AXIS2_PLACEMENT_3D('',#136181,#106579,#106580);
#94666=AXIS2_PLACEMENT_3D('',#136182,#106581,#106582);
#94667=AXIS2_PLACEMENT_3D('',#136183,#106583,#106584);
#94668=AXIS2_PLACEMENT_3D('',#136268,#106585,#106586);
#94669=AXIS2_PLACEMENT_3D('',#136279,#106587,#106588);
#94670=AXIS2_PLACEMENT_3D('',#136283,#106590,#106591);
#94671=AXIS2_PLACEMENT_3D('',#136285,#106593,#106594);
#94672=AXIS2_PLACEMENT_3D('',#136287,#106595,#106596);
#94673=AXIS2_PLACEMENT_3D('',#136289,#106597,#106598);
#94674=AXIS2_PLACEMENT_3D('',#136291,#106599,#106600);
#94675=AXIS2_PLACEMENT_3D('',#136292,#106601,#106602);
#94676=AXIS2_PLACEMENT_3D('',#136293,#106603,#106604);
#94677=AXIS2_PLACEMENT_3D('',#136296,#106605,#106606);
#94678=AXIS2_PLACEMENT_3D('',#136299,#106608,#106609);
#94679=AXIS2_PLACEMENT_3D('',#136333,#106611,#106612);
#94680=AXIS2_PLACEMENT_3D('',#136393,#106613,#106614);
#94681=AXIS2_PLACEMENT_3D('',#136425,#106618,#106619);
#94682=AXIS2_PLACEMENT_3D('',#136431,#106620,#106621);
#94683=AXIS2_PLACEMENT_3D('',#136436,#106622,#106623);
#94684=AXIS2_PLACEMENT_3D('',#136437,#106624,#106625);
#94685=AXIS2_PLACEMENT_3D('',#136438,#106626,#106627);
#94686=AXIS2_PLACEMENT_3D('',#136481,#106628,#106629);
#94687=AXIS2_PLACEMENT_3D('',#136510,#106630,#106631);
#94688=AXIS2_PLACEMENT_3D('',#136514,#106633,#106634);
#94689=AXIS2_PLACEMENT_3D('',#136614,#106636,#106637);
#94690=AXIS2_PLACEMENT_3D('',#136615,#106638,#106639);
#94691=AXIS2_PLACEMENT_3D('',#136616,#106640,#106641);
#94692=AXIS2_PLACEMENT_3D('',#136623,#106642,#106643);
#94693=AXIS2_PLACEMENT_3D('',#136627,#106645,#106646);
#94694=AXIS2_PLACEMENT_3D('',#136633,#106647,#106648);
#94695=AXIS2_PLACEMENT_3D('',#136634,#106649,#106650);
#94696=AXIS2_PLACEMENT_3D('',#136673,#106651,#106652);
#94697=AXIS2_PLACEMENT_3D('',#136674,#106653,#106654);
#94698=AXIS2_PLACEMENT_3D('',#136675,#106655,#106656);
#94699=AXIS2_PLACEMENT_3D('',#136754,#106658,#106659);
#94700=AXIS2_PLACEMENT_3D('',#136851,#106661,#106662);
#94701=AXIS2_PLACEMENT_3D('',#136964,#106663,#106664);
#94702=AXIS2_PLACEMENT_3D('',#136978,#106665,#106666);
#94703=AXIS2_PLACEMENT_3D('',#136979,#106667,#106668);
#94704=AXIS2_PLACEMENT_3D('',#136980,#106669,#106670);
#94705=AXIS2_PLACEMENT_3D('',#137072,#106673,#106674);
#94706=AXIS2_PLACEMENT_3D('',#137073,#106675,#106676);
#94707=AXIS2_PLACEMENT_3D('',#137103,#106677,#106678);
#94708=AXIS2_PLACEMENT_3D('',#137104,#106679,#106680);
#94709=AXIS2_PLACEMENT_3D('',#137105,#106681,#106682);
#94710=AXIS2_PLACEMENT_3D('',#137109,#106684,#106685);
#94711=AXIS2_PLACEMENT_3D('',#137113,#106687,#106688);
#94712=AXIS2_PLACEMENT_3D('',#137116,#106690,#106691);
#94713=AXIS2_PLACEMENT_3D('',#137159,#106693,#106694);
#94714=AXIS2_PLACEMENT_3D('',#137162,#106696,#106697);
#94715=AXIS2_PLACEMENT_3D('',#137163,#106698,#106699);
#94716=AXIS2_PLACEMENT_3D('',#137167,#106702,#106703);
#94717=AXIS2_PLACEMENT_3D('',#137170,#106705,#106706);
#94718=AXIS2_PLACEMENT_3D('',#137184,#106707,#106708);
#94719=AXIS2_PLACEMENT_3D('',#137185,#106709,#106710);
#94720=AXIS2_PLACEMENT_3D('',#137186,#106711,#106712);
#94721=AXIS2_PLACEMENT_3D('',#137190,#106714,#106715);
#94722=AXIS2_PLACEMENT_3D('',#137193,#106717,#106718);
#94723=AXIS2_PLACEMENT_3D('',#137237,#106720,#106721);
#94724=AXIS2_PLACEMENT_3D('',#137238,#106722,#106723);
#94725=AXIS2_PLACEMENT_3D('',#137269,#106724,#106725);
#94726=AXIS2_PLACEMENT_3D('',#137270,#106726,#106727);
#94727=AXIS2_PLACEMENT_3D('',#137271,#106728,#106729);
#94728=AXIS2_PLACEMENT_3D('',#137275,#106731,#106732);
#94729=AXIS2_PLACEMENT_3D('',#137279,#106734,#106735);
#94730=AXIS2_PLACEMENT_3D('',#137282,#106737,#106738);
#94731=AXIS2_PLACEMENT_3D('',#137340,#106740,#106741);
#94732=AXIS2_PLACEMENT_3D('',#137341,#106742,#106743);
#94733=AXIS2_PLACEMENT_3D('',#137342,#106744,#106745);
#94734=AXIS2_PLACEMENT_3D('',#137345,#106746,#106747);
#94735=AXIS2_PLACEMENT_3D('',#137354,#106748,#106749);
#94736=AXIS2_PLACEMENT_3D('',#137368,#106750,#106751);
#94737=AXIS2_PLACEMENT_3D('',#137369,#106752,#106753);
#94738=AXIS2_PLACEMENT_3D('',#137370,#106754,#106755);
#94739=AXIS2_PLACEMENT_3D('',#137374,#106757,#106758);
#94740=AXIS2_PLACEMENT_3D('',#137377,#106760,#106761);
#94741=AXIS2_PLACEMENT_3D('',#137402,#106763,#106764);
#94742=AXIS2_PLACEMENT_3D('',#137403,#106765,#106766);
#94743=AXIS2_PLACEMENT_3D('',#137406,#106768,#106769);
#94744=AXIS2_PLACEMENT_3D('',#137407,#106770,#106771);
#94745=AXIS2_PLACEMENT_3D('',#137411,#106774,#106775);
#94746=AXIS2_PLACEMENT_3D('',#137414,#106777,#106778);
#94747=AXIS2_PLACEMENT_3D('',#137415,#106779,#106780);
#94748=AXIS2_PLACEMENT_3D('',#137417,#106781,#106782);
#94749=AXIS2_PLACEMENT_3D('',#137434,#106784,#106785);
#94750=AXIS2_PLACEMENT_3D('',#137437,#106787,#106788);
#94751=AXIS2_PLACEMENT_3D('',#137450,#106789,#106790);
#94752=AXIS2_PLACEMENT_3D('',#137451,#106791,#106792);
#94753=AXIS2_PLACEMENT_3D('',#137481,#106793,#106794);
#94754=AXIS2_PLACEMENT_3D('',#137482,#106795,#106796);
#94755=AXIS2_PLACEMENT_3D('',#137483,#106797,#106798);
#94756=AXIS2_PLACEMENT_3D('',#137551,#106800,#106801);
#94757=AXIS2_PLACEMENT_3D('',#137653,#106802,#106803);
#94758=AXIS2_PLACEMENT_3D('',#137679,#106804,#106805);
#94759=AXIS2_PLACEMENT_3D('',#137778,#106806,#106807);
#94760=AXIS2_PLACEMENT_3D('',#137792,#106808,#106809);
#94761=AXIS2_PLACEMENT_3D('',#137793,#106810,#106811);
#94762=AXIS2_PLACEMENT_3D('',#137794,#106812,#106813);
#94763=AXIS2_PLACEMENT_3D('',#137835,#106815,#106816);
#94764=AXIS2_PLACEMENT_3D('',#137857,#106817,#106818);
#94765=AXIS2_PLACEMENT_3D('',#137858,#106819,#106820);
#94766=AXIS2_PLACEMENT_3D('',#137859,#106821,#106822);
#94767=AXIS2_PLACEMENT_3D('',#137953,#106824,#106825);
#94768=AXIS2_PLACEMENT_3D('',#138040,#106826,#106827);
#94769=AXIS2_PLACEMENT_3D('',#138041,#106828,#106829);
#94770=AXIS2_PLACEMENT_3D('',#138043,#106831,#106832);
#94771=AXIS2_PLACEMENT_3D('',#138047,#106834,#106835);
#94772=AXIS2_PLACEMENT_3D('',#138049,#106837,#106838);
#94773=AXIS2_PLACEMENT_3D('',#138053,#106841,#106842);
#94774=AXIS2_PLACEMENT_3D('',#138056,#106844,#106845);
#94775=AXIS2_PLACEMENT_3D('',#138057,#106846,#106847);
#94776=AXIS2_PLACEMENT_3D('',#138061,#106849,#106850);
#94777=AXIS2_PLACEMENT_3D('',#138063,#106852,#106853);
#94778=AXIS2_PLACEMENT_3D('',#138067,#106856,#106857);
#94779=AXIS2_PLACEMENT_3D('',#138070,#106859,#106860);
#94780=AXIS2_PLACEMENT_3D('',#138071,#106861,#106862);
#94781=AXIS2_PLACEMENT_3D('',#138076,#106864,#106865);
#94782=AXIS2_PLACEMENT_3D('',#138079,#106867,#106868);
#94783=AXIS2_PLACEMENT_3D('',#138081,#106869,#106870);
#94784=AXIS2_PLACEMENT_3D('',#138150,#106872,#106873);
#94785=AXIS2_PLACEMENT_3D('',#138164,#106875,#106876);
#94786=AXIS2_PLACEMENT_3D('',#138165,#106877,#106878);
#94787=AXIS2_PLACEMENT_3D('',#138200,#106879,#106880);
#94788=AXIS2_PLACEMENT_3D('',#138201,#106881,#106882);
#94789=AXIS2_PLACEMENT_3D('',#138202,#106883,#106884);
#94790=AXIS2_PLACEMENT_3D('',#138206,#106886,#106887);
#94791=AXIS2_PLACEMENT_3D('',#138210,#106889,#106890);
#94792=AXIS2_PLACEMENT_3D('',#138216,#106893,#106894);
#94793=AXIS2_PLACEMENT_3D('',#138260,#106896,#106897);
#94794=AXIS2_PLACEMENT_3D('',#138263,#106899,#106900);
#94795=AXIS2_PLACEMENT_3D('',#138264,#106901,#106902);
#94796=AXIS2_PLACEMENT_3D('',#138268,#106905,#106906);
#94797=AXIS2_PLACEMENT_3D('',#138271,#106908,#106909);
#94798=AXIS2_PLACEMENT_3D('',#138285,#106910,#106911);
#94799=AXIS2_PLACEMENT_3D('',#138286,#106912,#106913);
#94800=AXIS2_PLACEMENT_3D('',#138287,#106914,#106915);
#94801=AXIS2_PLACEMENT_3D('',#138338,#106917,#106918);
#94802=AXIS2_PLACEMENT_3D('',#138342,#106920,#106921);
#94803=AXIS2_PLACEMENT_3D('',#138345,#106923,#106924);
#94804=AXIS2_PLACEMENT_3D('',#138346,#106925,#106926);
#94805=AXIS2_PLACEMENT_3D('',#138382,#106927,#106928);
#94806=AXIS2_PLACEMENT_3D('',#138383,#106929,#106930);
#94807=AXIS2_PLACEMENT_3D('',#138384,#106931,#106932);
#94808=AXIS2_PLACEMENT_3D('',#138481,#106935,#106936);
#94809=AXIS2_PLACEMENT_3D('',#138578,#106938,#106939);
#94810=AXIS2_PLACEMENT_3D('',#138690,#106940,#106941);
#94811=AXIS2_PLACEMENT_3D('',#138704,#106942,#106943);
#94812=AXIS2_PLACEMENT_3D('',#138705,#106944,#106945);
#94813=AXIS2_PLACEMENT_3D('',#138706,#106946,#106947);
#94814=AXIS2_PLACEMENT_3D('',#138785,#106950,#106951);
#94815=AXIS2_PLACEMENT_3D('',#138787,#106953,#106954);
#94816=AXIS2_PLACEMENT_3D('',#138817,#106955,#106956);
#94817=AXIS2_PLACEMENT_3D('',#138818,#106957,#106958);
#94818=AXIS2_PLACEMENT_3D('',#138819,#106959,#106960);
#94819=AXIS2_PLACEMENT_3D('',#138880,#106963,#106964);
#94820=AXIS2_PLACEMENT_3D('',#138887,#106965,#106966);
#94821=AXIS2_PLACEMENT_3D('',#138891,#106968,#106969);
#94822=AXIS2_PLACEMENT_3D('',#138937,#106970,#106971);
#94823=AXIS2_PLACEMENT_3D('',#138961,#106972,#106973);
#94824=AXIS2_PLACEMENT_3D('',#139021,#106974,#106975);
#94825=AXIS2_PLACEMENT_3D('',#139035,#106976,#106977);
#94826=AXIS2_PLACEMENT_3D('',#139036,#106978,#106979);
#94827=AXIS2_PLACEMENT_3D('',#139037,#106980,#106981);
#94828=AXIS2_PLACEMENT_3D('',#139044,#106982,#106983);
#94829=AXIS2_PLACEMENT_3D('',#139048,#106985,#106986);
#94830=AXIS2_PLACEMENT_3D('',#139055,#106987,#106988);
#94831=AXIS2_PLACEMENT_3D('',#139085,#106991,#106992);
#94832=AXIS2_PLACEMENT_3D('',#139117,#106993,#106994);
#94833=AXIS2_PLACEMENT_3D('',#139118,#106995,#106996);
#94834=AXIS2_PLACEMENT_3D('',#139119,#106997,#106998);
#94835=AXIS2_PLACEMENT_3D('',#139201,#107001,#107002);
#94836=AXIS2_PLACEMENT_3D('',#139298,#107004,#107005);
#94837=AXIS2_PLACEMENT_3D('',#139410,#107006,#107007);
#94838=AXIS2_PLACEMENT_3D('',#139424,#107008,#107009);
#94839=AXIS2_PLACEMENT_3D('',#139425,#107010,#107011);
#94840=AXIS2_PLACEMENT_3D('',#139426,#107012,#107013);
#94841=AXIS2_PLACEMENT_3D('',#139468,#107015,#107016);
#94842=AXIS2_PLACEMENT_3D('',#139513,#107019,#107020);
#94843=AXIS2_PLACEMENT_3D('',#139547,#107021,#107022);
#94844=AXIS2_PLACEMENT_3D('',#139548,#107023,#107024);
#94845=AXIS2_PLACEMENT_3D('',#139549,#107025,#107026);
#94846=AXIS2_PLACEMENT_3D('',#139553,#107028,#107029);
#94847=AXIS2_PLACEMENT_3D('',#139557,#107031,#107032);
#94848=AXIS2_PLACEMENT_3D('',#139561,#107034,#107035);
#94849=AXIS2_PLACEMENT_3D('',#139610,#107037,#107038);
#94850=AXIS2_PLACEMENT_3D('',#139613,#107040,#107041);
#94851=AXIS2_PLACEMENT_3D('',#139614,#107042,#107043);
#94852=AXIS2_PLACEMENT_3D('',#139618,#107046,#107047);
#94853=AXIS2_PLACEMENT_3D('',#139621,#107049,#107050);
#94854=AXIS2_PLACEMENT_3D('',#139635,#107051,#107052);
#94855=AXIS2_PLACEMENT_3D('',#139636,#107053,#107054);
#94856=AXIS2_PLACEMENT_3D('',#139637,#107055,#107056);
#94857=AXIS2_PLACEMENT_3D('',#139683,#107058,#107059);
#94858=AXIS2_PLACEMENT_3D('',#139689,#107062,#107063);
#94859=AXIS2_PLACEMENT_3D('',#139692,#107065,#107066);
#94860=AXIS2_PLACEMENT_3D('',#139693,#107067,#107068);
#94861=AXIS2_PLACEMENT_3D('',#139728,#107069,#107070);
#94862=AXIS2_PLACEMENT_3D('',#139729,#107071,#107072);
#94863=AXIS2_PLACEMENT_3D('',#139730,#107073,#107074);
#94864=AXIS2_PLACEMENT_3D('',#139733,#107075,#107076);
#94865=AXIS2_PLACEMENT_3D('',#139801,#107078,#107079);
#94866=AXIS2_PLACEMENT_3D('',#139805,#107081,#107082);
#94867=AXIS2_PLACEMENT_3D('',#139809,#107085,#107086);
#94868=AXIS2_PLACEMENT_3D('',#139817,#107087,#107088);
#94869=AXIS2_PLACEMENT_3D('',#139851,#107091,#107092);
#94870=AXIS2_PLACEMENT_3D('',#139893,#107093,#107094);
#94871=AXIS2_PLACEMENT_3D('',#139904,#107095,#107096);
#94872=AXIS2_PLACEMENT_3D('',#140007,#107101,#107102);
#94873=AXIS2_PLACEMENT_3D('',#140011,#107104,#107105);
#94874=AXIS2_PLACEMENT_3D('',#140015,#107108,#107109);
#94875=AXIS2_PLACEMENT_3D('',#140018,#107111,#107112);
#94876=AXIS2_PLACEMENT_3D('',#140019,#107113,#107114);
#94877=AXIS2_PLACEMENT_3D('',#140023,#107117,#107118);
#94878=AXIS2_PLACEMENT_3D('',#140026,#107120,#107121);
#94879=AXIS2_PLACEMENT_3D('',#140027,#107122,#107123);
#94880=AXIS2_PLACEMENT_3D('',#140079,#107127,#107128);
#94881=AXIS2_PLACEMENT_3D('',#140082,#107130,#107131);
#94882=AXIS2_PLACEMENT_3D('',#140169,#107136,#107137);
#94883=AXIS2_PLACEMENT_3D('',#140189,#107138,#107139);
#94884=AXIS2_PLACEMENT_3D('',#140221,#107140,#107141);
#94885=AXIS2_PLACEMENT_3D('',#140226,#107143,#107144);
#94886=AXIS2_PLACEMENT_3D('',#140229,#107146,#107147);
#94887=AXIS2_PLACEMENT_3D('',#140231,#107148,#107149);
#94888=AXIS2_PLACEMENT_3D('',#140301,#107152,#107153);
#94889=AXIS2_PLACEMENT_3D('',#140304,#107154,#107155);
#94890=AXIS2_PLACEMENT_3D('',#140305,#107156,#107157);
#94891=AXIS2_PLACEMENT_3D('',#140307,#107158,#107159);
#94892=AXIS2_PLACEMENT_3D('',#140316,#107160,#107161);
#94893=AXIS2_PLACEMENT_3D('',#140349,#107163,#107164);
#94894=AXIS2_PLACEMENT_3D('',#140360,#107165,#107166);
#94895=AXIS2_PLACEMENT_3D('',#140364,#107168,#107169);
#94896=AXIS2_PLACEMENT_3D('',#140368,#107171,#107172);
#94897=AXIS2_PLACEMENT_3D('',#140464,#107178,#107179);
#94898=AXIS2_PLACEMENT_3D('',#140467,#107181,#107182);
#94899=AXIS2_PLACEMENT_3D('',#140468,#107183,#107184);
#94900=AXIS2_PLACEMENT_3D('',#140472,#107187,#107188);
#94901=AXIS2_PLACEMENT_3D('',#140475,#107190,#107191);
#94902=AXIS2_PLACEMENT_3D('',#140476,#107192,#107193);
#94903=AXIS2_PLACEMENT_3D('',#140481,#107195,#107196);
#94904=AXIS2_PLACEMENT_3D('',#140484,#107198,#107199);
#94905=AXIS2_PLACEMENT_3D('',#140596,#107204,#107205);
#94906=AXIS2_PLACEMENT_3D('',#140599,#107206,#107207);
#94907=AXIS2_PLACEMENT_3D('',#140643,#107210,#107211);
#94908=AXIS2_PLACEMENT_3D('',#140675,#107212,#107213);
#94909=AXIS2_PLACEMENT_3D('',#140686,#107214,#107215);
#94910=AXIS2_PLACEMENT_3D('',#140690,#107217,#107218);
#94911=AXIS2_PLACEMENT_3D('',#140693,#107220,#107221);
#94912=AXIS2_PLACEMENT_3D('',#140736,#107224,#107225);
#94913=AXIS2_PLACEMENT_3D('',#140739,#107227,#107228);
#94914=AXIS2_PLACEMENT_3D('',#140740,#107229,#107230);
#94915=AXIS2_PLACEMENT_3D('',#140744,#107233,#107234);
#94916=AXIS2_PLACEMENT_3D('',#140747,#107236,#107237);
#94917=AXIS2_PLACEMENT_3D('',#140748,#107238,#107239);
#94918=AXIS2_PLACEMENT_3D('',#140831,#107241,#107242);
#94919=AXIS2_PLACEMENT_3D('',#140834,#107244,#107245);
#94920=AXIS2_PLACEMENT_3D('',#140871,#107246,#107247);
#94921=AXIS2_PLACEMENT_3D('',#140903,#107248,#107249);
#94922=AXIS2_PLACEMENT_3D('',#140917,#107250,#107251);
#94923=AXIS2_PLACEMENT_3D('',#140925,#107255,#107256);
#94924=AXIS2_PLACEMENT_3D('',#140929,#107259,#107260);
#94925=AXIS2_PLACEMENT_3D('',#140932,#107262,#107263);
#94926=AXIS2_PLACEMENT_3D('',#140933,#107264,#107265);
#94927=AXIS2_PLACEMENT_3D('',#140937,#107268,#107269);
#94928=AXIS2_PLACEMENT_3D('',#140940,#107271,#107272);
#94929=AXIS2_PLACEMENT_3D('',#140941,#107273,#107274);
#94930=AXIS2_PLACEMENT_3D('',#140944,#107276,#107277);
#94931=AXIS2_PLACEMENT_3D('',#140991,#107280,#107281);
#94932=AXIS2_PLACEMENT_3D('',#140992,#107282,#107283);
#94933=AXIS2_PLACEMENT_3D('',#140995,#107284,#107285);
#94934=AXIS2_PLACEMENT_3D('',#141039,#107288,#107289);
#94935=AXIS2_PLACEMENT_3D('',#141071,#107290,#107291);
#94936=AXIS2_PLACEMENT_3D('',#141082,#107292,#107293);
#94937=AXIS2_PLACEMENT_3D('',#141184,#107298,#107299);
#94938=AXIS2_PLACEMENT_3D('',#141188,#107301,#107302);
#94939=AXIS2_PLACEMENT_3D('',#141192,#107305,#107306);
#94940=AXIS2_PLACEMENT_3D('',#141195,#107308,#107309);
#94941=AXIS2_PLACEMENT_3D('',#141196,#107310,#107311);
#94942=AXIS2_PLACEMENT_3D('',#141200,#107314,#107315);
#94943=AXIS2_PLACEMENT_3D('',#141203,#107317,#107318);
#94944=AXIS2_PLACEMENT_3D('',#141235,#107319,#107320);
#94945=AXIS2_PLACEMENT_3D('',#141246,#107321,#107322);
#94946=AXIS2_PLACEMENT_3D('',#141290,#107328,#107329);
#94947=AXIS2_PLACEMENT_3D('',#141293,#107331,#107332);
#94948=AXIS2_PLACEMENT_3D('',#141320,#107336,#107337);
#94949=AXIS2_PLACEMENT_3D('',#141321,#107338,#107339);
#94950=AXIS2_PLACEMENT_3D('',#141326,#107341,#107342);
#94951=AXIS2_PLACEMENT_3D('',#141329,#107344,#107345);
#94952=AXIS2_PLACEMENT_3D('',#141331,#107346,#107347);
#94953=AXIS2_PLACEMENT_3D('',#141333,#107348,#107349);
#94954=AXIS2_PLACEMENT_3D('',#141335,#107350,#107351);
#94955=AXIS2_PLACEMENT_3D('',#141429,#107354,#107355);
#94956=AXIS2_PLACEMENT_3D('',#141451,#107356,#107357);
#94957=AXIS2_PLACEMENT_3D('',#141454,#107358,#107359);
#94958=AXIS2_PLACEMENT_3D('',#141455,#107360,#107361);
#94959=AXIS2_PLACEMENT_3D('',#141457,#107362,#107363);
#94960=AXIS2_PLACEMENT_3D('',#141466,#107364,#107365);
#94961=AXIS2_PLACEMENT_3D('',#141499,#107367,#107368);
#94962=AXIS2_PLACEMENT_3D('',#141510,#107369,#107370);
#94963=AXIS2_PLACEMENT_3D('',#141514,#107372,#107373);
#94964=AXIS2_PLACEMENT_3D('',#141518,#107375,#107376);
#94965=AXIS2_PLACEMENT_3D('',#141617,#107382,#107383);
#94966=AXIS2_PLACEMENT_3D('',#141620,#107385,#107386);
#94967=AXIS2_PLACEMENT_3D('',#141621,#107387,#107388);
#94968=AXIS2_PLACEMENT_3D('',#141625,#107391,#107392);
#94969=AXIS2_PLACEMENT_3D('',#141628,#107394,#107395);
#94970=AXIS2_PLACEMENT_3D('',#141629,#107396,#107397);
#94971=AXIS2_PLACEMENT_3D('',#141634,#107399,#107400);
#94972=AXIS2_PLACEMENT_3D('',#141637,#107402,#107403);
#94973=AXIS2_PLACEMENT_3D('',#141743,#107408,#107409);
#94974=AXIS2_PLACEMENT_3D('',#141746,#107410,#107411);
#94975=AXIS2_PLACEMENT_3D('',#141758,#107412,#107413);
#94976=AXIS2_PLACEMENT_3D('',#141759,#107414,#107415);
#94977=AXIS2_PLACEMENT_3D('',#141810,#107416,#107417);
#94978=AXIS2_PLACEMENT_3D('',#141811,#107418,#107419);
#94979=AXIS2_PLACEMENT_3D('',#141893,#107421,#107422);
#94980=AXIS2_PLACEMENT_3D('',#141895,#107423,#107424);
#94981=AXIS2_PLACEMENT_3D('',#141899,#107426,#107427);
#94982=AXIS2_PLACEMENT_3D('',#141934,#107430,#107431);
#94983=AXIS2_PLACEMENT_3D('',#141945,#107432,#107433);
#94984=AXIS2_PLACEMENT_3D('',#142031,#107440,#107441);
#94985=AXIS2_PLACEMENT_3D('',#142035,#107443,#107444);
#94986=AXIS2_PLACEMENT_3D('',#142039,#107447,#107448);
#94987=AXIS2_PLACEMENT_3D('',#142042,#107450,#107451);
#94988=AXIS2_PLACEMENT_3D('',#142043,#107452,#107453);
#94989=AXIS2_PLACEMENT_3D('',#142047,#107456,#107457);
#94990=AXIS2_PLACEMENT_3D('',#142050,#107459,#107460);
#94991=AXIS2_PLACEMENT_3D('',#142051,#107461,#107462);
#94992=AXIS2_PLACEMENT_3D('',#142056,#107464,#107465);
#94993=AXIS2_PLACEMENT_3D('',#142059,#107467,#107468);
#94994=AXIS2_PLACEMENT_3D('',#142200,#107473,#107474);
#94995=AXIS2_PLACEMENT_3D('',#142201,#107475,#107476);
#94996=AXIS2_PLACEMENT_3D('',#142204,#107477,#107478);
#94997=AXIS2_PLACEMENT_3D('',#142238,#107481,#107482);
#94998=AXIS2_PLACEMENT_3D('',#142252,#107483,#107484);
#94999=AXIS2_PLACEMENT_3D('',#142256,#107486,#107487);
#95000=AXIS2_PLACEMENT_3D('',#142260,#107489,#107490);
#95001=AXIS2_PLACEMENT_3D('',#142368,#107496,#107497);
#95002=AXIS2_PLACEMENT_3D('',#142371,#107499,#107500);
#95003=AXIS2_PLACEMENT_3D('',#142372,#107501,#107502);
#95004=AXIS2_PLACEMENT_3D('',#142376,#107505,#107506);
#95005=AXIS2_PLACEMENT_3D('',#142379,#107508,#107509);
#95006=AXIS2_PLACEMENT_3D('',#142411,#107510,#107511);
#95007=AXIS2_PLACEMENT_3D('',#142422,#107512,#107513);
#95008=AXIS2_PLACEMENT_3D('',#142427,#107515,#107516);
#95009=AXIS2_PLACEMENT_3D('',#142430,#107518,#107519);
#95010=AXIS2_PLACEMENT_3D('',#142539,#107524,#107525);
#95011=AXIS2_PLACEMENT_3D('',#142541,#107527,#107528);
#95012=AXIS2_PLACEMENT_3D('',#142542,#107529,#107530);
#95013=AXIS2_PLACEMENT_3D('',#142543,#107531,#107532);
#95014=AXIS2_PLACEMENT_3D('',#142545,#107533,#107534);
#95015=AXIS2_PLACEMENT_3D('',#142548,#107536,#107537);
#95016=AXIS2_PLACEMENT_3D('',#142549,#107538,#107539);
#95017=AXIS2_PLACEMENT_3D('',#142551,#107540,#107541);
#95018=AXIS2_PLACEMENT_3D('',#142552,#107542,#107543);
#95019=AXIS2_PLACEMENT_3D('',#142571,#107545,#107546);
#95020=AXIS2_PLACEMENT_3D('',#142572,#107547,#107548);
#95021=AXIS2_PLACEMENT_3D('',#142573,#107549,#107550);
#95022=AXIS2_PLACEMENT_3D('',#142584,#107551,#107552);
#95023=AXIS2_PLACEMENT_3D('',#142585,#107553,#107554);
#95024=AXIS2_PLACEMENT_3D('',#142586,#107555,#107556);
#95025=AXIS2_PLACEMENT_3D('',#142588,#107557,#107558);
#95026=AXIS2_PLACEMENT_3D('',#142589,#107559,#107560);
#95027=AXIS2_PLACEMENT_3D('',#142599,#107561,#107562);
#95028=AXIS2_PLACEMENT_3D('',#142600,#107563,#107564);
#95029=AXIS2_PLACEMENT_3D('',#142601,#107565,#107566);
#95030=AXIS2_PLACEMENT_3D('',#142602,#107567,#107568);
#95031=AXIS2_PLACEMENT_3D('',#142603,#107569,#107570);
#95032=AXIS2_PLACEMENT_3D('',#142604,#107571,#107572);
#95033=AXIS2_PLACEMENT_3D('',#142606,#107573,#107574);
#95034=AXIS2_PLACEMENT_3D('',#142609,#107576,#107577);
#95035=AXIS2_PLACEMENT_3D('',#142610,#107578,#107579);
#95036=AXIS2_PLACEMENT_3D('',#142612,#107580,#107581);
#95037=AXIS2_PLACEMENT_3D('',#142613,#107582,#107583);
#95038=AXIS2_PLACEMENT_3D('',#142643,#107585,#107586);
#95039=AXIS2_PLACEMENT_3D('',#142662,#107587,#107588);
#95040=AXIS2_PLACEMENT_3D('',#142663,#107589,#107590);
#95041=AXIS2_PLACEMENT_3D('',#142664,#107591,#107592);
#95042=AXIS2_PLACEMENT_3D('',#142666,#107593,#107594);
#95043=AXIS2_PLACEMENT_3D('',#142669,#107596,#107597);
#95044=AXIS2_PLACEMENT_3D('',#142670,#107598,#107599);
#95045=AXIS2_PLACEMENT_3D('',#142671,#107600,#107601);
#95046=AXIS2_PLACEMENT_3D('',#142672,#107602,#107603);
#95047=AXIS2_PLACEMENT_3D('',#142675,#107605,#107606);
#95048=AXIS2_PLACEMENT_3D('',#142676,#107607,#107608);
#95049=AXIS2_PLACEMENT_3D('',#142710,#107611,#107612);
#95050=AXIS2_PLACEMENT_3D('',#142740,#107613,#107614);
#95051=AXIS2_PLACEMENT_3D('',#142741,#107615,#107616);
#95052=AXIS2_PLACEMENT_3D('',#142748,#107617,#107618);
#95053=AXIS2_PLACEMENT_3D('',#142749,#107619,#107620);
#95054=AXIS2_PLACEMENT_3D('',#142750,#107621,#107622);
#95055=AXIS2_PLACEMENT_3D('',#142751,#107623,#107624);
#95056=AXIS2_PLACEMENT_3D('',#142765,#107625,#107626);
#95057=AXIS2_PLACEMENT_3D('',#142794,#107627,#107628);
#95058=AXIS2_PLACEMENT_3D('',#142796,#107630,#107631);
#95059=AXIS2_PLACEMENT_3D('',#142798,#107633,#107634);
#95060=AXIS2_PLACEMENT_3D('',#142835,#107635,#107636);
#95061=AXIS2_PLACEMENT_3D('',#142872,#107637,#107638);
#95062=AXIS2_PLACEMENT_3D('',#142873,#107639,#107640);
#95063=AXIS2_PLACEMENT_3D('',#142875,#107642,#107643);
#95064=AXIS2_PLACEMENT_3D('',#142877,#107645,#107646);
#95065=AXIS2_PLACEMENT_3D('',#142890,#107647,#107648);
#95066=AXIS2_PLACEMENT_3D('',#142921,#107649,#107650);
#95067=AXIS2_PLACEMENT_3D('',#142941,#107651,#107652);
#95068=AXIS2_PLACEMENT_3D('',#142970,#107653,#107654);
#95069=AXIS2_PLACEMENT_3D('',#142971,#107655,#107656);
#95070=AXIS2_PLACEMENT_3D('',#142982,#107658,#107659);
#95071=AXIS2_PLACEMENT_3D('',#142983,#107660,#107661);
#95072=AXIS2_PLACEMENT_3D('',#142986,#107663,#107664);
#95073=AXIS2_PLACEMENT_3D('',#142987,#107665,#107666);
#95074=AXIS2_PLACEMENT_3D('',#142991,#107669,#107670);
#95075=AXIS2_PLACEMENT_3D('',#142992,#107671,#107672);
#95076=AXIS2_PLACEMENT_3D('',#143002,#107673,#107674);
#95077=AXIS2_PLACEMENT_3D('',#143003,#107675,#107676);
#95078=AXIS2_PLACEMENT_3D('',#143033,#107679,#107680);
#95079=AXIS2_PLACEMENT_3D('',#143034,#107681,#107682);
#95080=AXIS2_PLACEMENT_3D('',#143037,#107684,#107685);
#95081=AXIS2_PLACEMENT_3D('',#143038,#107686,#107687);
#95082=AXIS2_PLACEMENT_3D('',#143042,#107690,#107691);
#95083=AXIS2_PLACEMENT_3D('',#143043,#107692,#107693);
#95084=AXIS2_PLACEMENT_3D('',#143053,#107694,#107695);
#95085=AXIS2_PLACEMENT_3D('',#143054,#107696,#107697);
#95086=AXIS2_PLACEMENT_3D('',#143081,#107700,#107701);
#95087=AXIS2_PLACEMENT_3D('',#143082,#107702,#107703);
#95088=AXIS2_PLACEMENT_3D('',#143083,#107704,#107705);
#95089=AXIS2_PLACEMENT_3D('',#143084,#107706,#107707);
#95090=AXIS2_PLACEMENT_3D('',#143086,#107708,#107709);
#95091=AXIS2_PLACEMENT_3D('',#143087,#107710,#107711);
#95092=AXIS2_PLACEMENT_3D('',#143119,#107713,#107714);
#95093=AXIS2_PLACEMENT_3D('',#143120,#107715,#107716);
#95094=AXIS2_PLACEMENT_3D('',#143122,#107717,#107718);
#95095=AXIS2_PLACEMENT_3D('',#143155,#107720,#107721);
#95096=AXIS2_PLACEMENT_3D('',#143166,#107722,#107723);
#95097=AXIS2_PLACEMENT_3D('',#143168,#107724,#107725);
#95098=AXIS2_PLACEMENT_3D('',#143213,#107727,#107728);
#95099=AXIS2_PLACEMENT_3D('',#143217,#107731,#107732);
#95100=AXIS2_PLACEMENT_3D('',#143220,#107734,#107735);
#95101=AXIS2_PLACEMENT_3D('',#143221,#107736,#107737);
#95102=AXIS2_PLACEMENT_3D('',#143224,#107739,#107740);
#95103=AXIS2_PLACEMENT_3D('',#143225,#107741,#107742);
#95104=AXIS2_PLACEMENT_3D('',#143228,#107744,#107745);
#95105=AXIS2_PLACEMENT_3D('',#143229,#107746,#107747);
#95106=AXIS2_PLACEMENT_3D('',#143295,#107758,#107759);
#95107=AXIS2_PLACEMENT_3D('',#143311,#107762,#107763);
#95108=AXIS2_PLACEMENT_3D('',#143315,#107765,#107766);
#95109=AXIS2_PLACEMENT_3D('',#143317,#107767,#107768);
#95110=AXIS2_PLACEMENT_3D('',#143368,#107770,#107771);
#95111=AXIS2_PLACEMENT_3D('',#143381,#107773,#107774);
#95112=AXIS2_PLACEMENT_3D('',#143390,#107775,#107776);
#95113=AXIS2_PLACEMENT_3D('',#143394,#107778,#107779);
#95114=AXIS2_PLACEMENT_3D('',#143442,#107781,#107782);
#95115=AXIS2_PLACEMENT_3D('',#143455,#107784,#107785);
#95116=AXIS2_PLACEMENT_3D('',#143468,#107787,#107788);
#95117=AXIS2_PLACEMENT_3D('',#143513,#107790,#107791);
#95118=AXIS2_PLACEMENT_3D('',#143567,#107793,#107794);
#95119=AXIS2_PLACEMENT_3D('',#143578,#107796,#107797);
#95120=AXIS2_PLACEMENT_3D('',#143592,#107799,#107800);
#95121=AXIS2_PLACEMENT_3D('',#143643,#107802,#107803);
#95122=AXIS2_PLACEMENT_3D('',#143691,#107805,#107806);
#95123=AXIS2_PLACEMENT_3D('',#143696,#107807,#107808);
#95124=AXIS2_PLACEMENT_3D('',#143712,#107811,#107812);
#95125=AXIS2_PLACEMENT_3D('',#143778,#107823,#107824);
#95126=AXIS2_PLACEMENT_3D('',#143781,#107826,#107827);
#95127=AXIS2_PLACEMENT_3D('',#143782,#107828,#107829);
#95128=AXIS2_PLACEMENT_3D('',#143785,#107831,#107832);
#95129=AXIS2_PLACEMENT_3D('',#143786,#107833,#107834);
#95130=AXIS2_PLACEMENT_3D('',#143789,#107836,#107837);
#95131=AXIS2_PLACEMENT_3D('',#143790,#107838,#107839);
#95132=AXIS2_PLACEMENT_3D('',#143884,#107849,#107850);
#95133=AXIS2_PLACEMENT_3D('',#143885,#107851,#107852);
#95134=AXIS2_PLACEMENT_3D('',#143886,#107853,#107854);
#95135=AXIS2_PLACEMENT_3D('',#143891,#107856,#107857);
#95136=AXIS2_PLACEMENT_3D('',#143893,#107858,#107859);
#95137=AXIS2_PLACEMENT_3D('',#143895,#107860,#107861);
#95138=AXIS2_PLACEMENT_3D('',#143930,#107865,#107866);
#95139=AXIS2_PLACEMENT_3D('',#143931,#107867,#107868);
#95140=AXIS2_PLACEMENT_3D('',#143932,#107869,#107870);
#95141=AXIS2_PLACEMENT_3D('',#143936,#107872,#107873);
#95142=AXIS2_PLACEMENT_3D('',#143968,#107875,#107876);
#95143=AXIS2_PLACEMENT_3D('',#143969,#107877,#107878);
#95144=AXIS2_PLACEMENT_3D('',#143970,#107879,#107880);
#95145=AXIS2_PLACEMENT_3D('',#143974,#107882,#107883);
#95146=AXIS2_PLACEMENT_3D('',#143976,#107884,#107885);
#95147=AXIS2_PLACEMENT_3D('',#143978,#107886,#107887);
#95148=AXIS2_PLACEMENT_3D('',#143982,#107890,#107891);
#95149=AXIS2_PLACEMENT_3D('',#143984,#107893,#107894);
#95150=AXIS2_PLACEMENT_3D('',#143986,#107895,#107896);
#95151=AXIS2_PLACEMENT_3D('',#144000,#107898,#107899);
#95152=AXIS2_PLACEMENT_3D('',#144001,#107900,#107901);
#95153=AXIS2_PLACEMENT_3D('',#144031,#107902,#107903);
#95154=AXIS2_PLACEMENT_3D('',#144032,#107904,#107905);
#95155=AXIS2_PLACEMENT_3D('',#144035,#107907,#107908);
#95156=AXIS2_PLACEMENT_3D('',#144036,#107909,#107910);
#95157=AXIS2_PLACEMENT_3D('',#144040,#107913,#107914);
#95158=AXIS2_PLACEMENT_3D('',#144041,#107915,#107916);
#95159=AXIS2_PLACEMENT_3D('',#144054,#107917,#107918);
#95160=AXIS2_PLACEMENT_3D('',#144055,#107919,#107920);
#95161=AXIS2_PLACEMENT_3D('',#144084,#107921,#107922);
#95162=AXIS2_PLACEMENT_3D('',#144142,#107923,#107924);
#95163=AXIS2_PLACEMENT_3D('',#144216,#107925,#107926);
#95164=AXIS2_PLACEMENT_3D('',#144229,#107927,#107928);
#95165=AXIS2_PLACEMENT_3D('',#144230,#107929,#107930);
#95166=AXIS2_PLACEMENT_3D('',#144269,#107931,#107932);
#95167=AXIS2_PLACEMENT_3D('',#144270,#107933,#107934);
#95168=AXIS2_PLACEMENT_3D('',#144271,#107935,#107936);
#95169=AXIS2_PLACEMENT_3D('',#144272,#107937,#107938);
#95170=AXIS2_PLACEMENT_3D('',#144315,#107939,#107940);
#95171=AXIS2_PLACEMENT_3D('',#144322,#107941,#107942);
#95172=AXIS2_PLACEMENT_3D('',#144325,#107944,#107945);
#95173=AXIS2_PLACEMENT_3D('',#144326,#107946,#107947);
#95174=AXIS2_PLACEMENT_3D('',#144340,#107949,#107950);
#95175=AXIS2_PLACEMENT_3D('',#144353,#107951,#107952);
#95176=AXIS2_PLACEMENT_3D('',#144367,#107953,#107954);
#95177=AXIS2_PLACEMENT_3D('',#144368,#107955,#107956);
#95178=AXIS2_PLACEMENT_3D('',#144369,#107957,#107958);
#95179=AXIS2_PLACEMENT_3D('',#144371,#107959,#107960);
#95180=AXIS2_PLACEMENT_3D('',#144385,#107962,#107963);
#95181=AXIS2_PLACEMENT_3D('',#144449,#107964,#107965);
#95182=AXIS2_PLACEMENT_3D('',#144468,#107966,#107967);
#95183=AXIS2_PLACEMENT_3D('',#144469,#107968,#107969);
#95184=AXIS2_PLACEMENT_3D('',#144471,#107970,#107971);
#95185=AXIS2_PLACEMENT_3D('',#144491,#107973,#107974);
#95186=AXIS2_PLACEMENT_3D('',#144529,#107975,#107976);
#95187=AXIS2_PLACEMENT_3D('',#144531,#107978,#107979);
#95188=AXIS2_PLACEMENT_3D('',#144533,#107981,#107982);
#95189=AXIS2_PLACEMENT_3D('',#144546,#107983,#107984);
#95190=AXIS2_PLACEMENT_3D('',#144559,#107985,#107986);
#95191=AXIS2_PLACEMENT_3D('',#144579,#107987,#107988);
#95192=AXIS2_PLACEMENT_3D('',#144605,#107989,#107990);
#95193=AXIS2_PLACEMENT_3D('',#144607,#107991,#107992);
#95194=AXIS2_PLACEMENT_3D('',#144686,#107994,#107995);
#95195=AXIS2_PLACEMENT_3D('',#144705,#107996,#107997);
#95196=AXIS2_PLACEMENT_3D('',#144706,#107998,#107999);
#95197=AXIS2_PLACEMENT_3D('',#144708,#108000,#108001);
#95198=AXIS2_PLACEMENT_3D('',#144728,#108003,#108004);
#95199=AXIS2_PLACEMENT_3D('',#144769,#108005,#108006);
#95200=AXIS2_PLACEMENT_3D('',#144771,#108007,#108008);
#95201=AXIS2_PLACEMENT_3D('',#144772,#108009,#108010);
#95202=AXIS2_PLACEMENT_3D('',#144773,#108011,#108012);
#95203=AXIS2_PLACEMENT_3D('',#144775,#108013,#108014);
#95204=AXIS2_PLACEMENT_3D('',#144777,#108016,#108017);
#95205=AXIS2_PLACEMENT_3D('',#144778,#108018,#108019);
#95206=AXIS2_PLACEMENT_3D('',#144779,#108020,#108021);
#95207=AXIS2_PLACEMENT_3D('',#144781,#108022,#108023);
#95208=AXIS2_PLACEMENT_3D('',#144783,#108025,#108026);
#95209=AXIS2_PLACEMENT_3D('',#144784,#108027,#108028);
#95210=AXIS2_PLACEMENT_3D('',#144797,#108029,#108030);
#95211=AXIS2_PLACEMENT_3D('',#144810,#108031,#108032);
#95212=AXIS2_PLACEMENT_3D('',#144830,#108033,#108034);
#95213=AXIS2_PLACEMENT_3D('',#144859,#108035,#108036);
#95214=AXIS2_PLACEMENT_3D('',#144861,#108037,#108038);
#95215=AXIS2_PLACEMENT_3D('',#144887,#108040,#108041);
#95216=AXIS2_PLACEMENT_3D('',#144889,#108042,#108043);
#95217=AXIS2_PLACEMENT_3D('',#144891,#108045,#108046);
#95218=AXIS2_PLACEMENT_3D('',#144892,#108047,#108048);
#95219=AXIS2_PLACEMENT_3D('',#144946,#108049,#108050);
#95220=AXIS2_PLACEMENT_3D('',#144965,#108051,#108052);
#95221=AXIS2_PLACEMENT_3D('',#144966,#108053,#108054);
#95222=AXIS2_PLACEMENT_3D('',#144968,#108055,#108056);
#95223=AXIS2_PLACEMENT_3D('',#144988,#108058,#108059);
#95224=AXIS2_PLACEMENT_3D('',#145032,#108060,#108061);
#95225=AXIS2_PLACEMENT_3D('',#145034,#108062,#108063);
#95226=AXIS2_PLACEMENT_3D('',#145035,#108064,#108065);
#95227=AXIS2_PLACEMENT_3D('',#145036,#108066,#108067);
#95228=AXIS2_PLACEMENT_3D('',#145037,#108068,#108069);
#95229=AXIS2_PLACEMENT_3D('',#145039,#108071,#108072);
#95230=AXIS2_PLACEMENT_3D('',#145040,#108073,#108074);
#95231=AXIS2_PLACEMENT_3D('',#145070,#108075,#108076);
#95232=AXIS2_PLACEMENT_3D('',#145095,#108077,#108078);
#95233=AXIS2_PLACEMENT_3D('',#145108,#108079,#108080);
#95234=AXIS2_PLACEMENT_3D('',#145127,#108081,#108082);
#95235=AXIS2_PLACEMENT_3D('',#145159,#108083,#108084);
#95236=AXIS2_PLACEMENT_3D('',#145160,#108085,#108086);
#95237=AXIS2_PLACEMENT_3D('',#145161,#108087,#108088);
#95238=AXIS2_PLACEMENT_3D('',#145162,#108089,#108090);
#95239=AXIS2_PLACEMENT_3D('',#145163,#108091,#108092);
#95240=AXIS2_PLACEMENT_3D('',#145164,#108093,#108094);
#95241=AXIS2_PLACEMENT_3D('',#145165,#108095,#108096);
#95242=AXIS2_PLACEMENT_3D('',#145166,#108097,#108098);
#95243=AXIS2_PLACEMENT_3D('',#145185,#108099,#108100);
#95244=AXIS2_PLACEMENT_3D('',#145210,#108101,#108102);
#95245=AXIS2_PLACEMENT_3D('',#145247,#108103,#108104);
#95246=AXIS2_PLACEMENT_3D('',#145249,#108105,#108106);
#95247=AXIS2_PLACEMENT_3D('',#145250,#108107,#108108);
#95248=AXIS2_PLACEMENT_3D('',#145251,#108109,#108110);
#95249=AXIS2_PLACEMENT_3D('',#145253,#108111,#108112);
#95250=AXIS2_PLACEMENT_3D('',#145255,#108114,#108115);
#95251=AXIS2_PLACEMENT_3D('',#145256,#108116,#108117);
#95252=AXIS2_PLACEMENT_3D('',#145257,#108118,#108119);
#95253=AXIS2_PLACEMENT_3D('',#145259,#108120,#108121);
#95254=AXIS2_PLACEMENT_3D('',#145260,#108122,#108123);
#95255=AXIS2_PLACEMENT_3D('',#145261,#108124,#108125);
#95256=AXIS2_PLACEMENT_3D('',#145263,#108126,#108127);
#95257=AXIS2_PLACEMENT_3D('',#145265,#108129,#108130);
#95258=AXIS2_PLACEMENT_3D('',#145266,#108131,#108132);
#95259=AXIS2_PLACEMENT_3D('',#145267,#108133,#108134);
#95260=AXIS2_PLACEMENT_3D('',#145271,#108136,#108137);
#95261=AXIS2_PLACEMENT_3D('',#145282,#108138,#108139);
#95262=AXIS2_PLACEMENT_3D('',#145283,#108140,#108141);
#95263=AXIS2_PLACEMENT_3D('',#145284,#108142,#108143);
#95264=AXIS2_PLACEMENT_3D('',#145298,#108144,#108145);
#95265=AXIS2_PLACEMENT_3D('',#145299,#108146,#108147);
#95266=AXIS2_PLACEMENT_3D('',#145319,#108148,#108149);
#95267=AXIS2_PLACEMENT_3D('',#145345,#108150,#108151);
#95268=AXIS2_PLACEMENT_3D('',#145352,#108152,#108153);
#95269=AXIS2_PLACEMENT_3D('',#145354,#108154,#108155);
#95270=AXIS2_PLACEMENT_3D('',#145374,#108157,#108158);
#95271=AXIS2_PLACEMENT_3D('',#145424,#108159,#108160);
#95272=AXIS2_PLACEMENT_3D('',#145426,#108161,#108162);
#95273=AXIS2_PLACEMENT_3D('',#145428,#108164,#108165);
#95274=AXIS2_PLACEMENT_3D('',#145429,#108166,#108167);
#95275=AXIS2_PLACEMENT_3D('',#145517,#108168,#108169);
#95276=AXIS2_PLACEMENT_3D('',#145536,#108170,#108171);
#95277=AXIS2_PLACEMENT_3D('',#145537,#108172,#108173);
#95278=AXIS2_PLACEMENT_3D('',#145539,#108174,#108175);
#95279=AXIS2_PLACEMENT_3D('',#145560,#108177,#108178);
#95280=AXIS2_PLACEMENT_3D('',#145586,#108179,#108180);
#95281=AXIS2_PLACEMENT_3D('',#145605,#108181,#108182);
#95282=AXIS2_PLACEMENT_3D('',#145606,#108183,#108184);
#95283=AXIS2_PLACEMENT_3D('',#145607,#108185,#108186);
#95284=AXIS2_PLACEMENT_3D('',#145608,#108187,#108188);
#95285=AXIS2_PLACEMENT_3D('',#145609,#108189,#108190);
#95286=AXIS2_PLACEMENT_3D('',#145611,#108191,#108192);
#95287=AXIS2_PLACEMENT_3D('',#145622,#108194,#108195);
#95288=AXIS2_PLACEMENT_3D('',#145624,#108196,#108197);
#95289=AXIS2_PLACEMENT_3D('',#145625,#108198,#108199);
#95290=AXIS2_PLACEMENT_3D('',#145626,#108200,#108201);
#95291=AXIS2_PLACEMENT_3D('',#145628,#108202,#108203);
#95292=AXIS2_PLACEMENT_3D('',#145630,#108205,#108206);
#95293=AXIS2_PLACEMENT_3D('',#145631,#108207,#108208);
#95294=AXIS2_PLACEMENT_3D('',#145632,#108209,#108210);
#95295=AXIS2_PLACEMENT_3D('',#145634,#108211,#108212);
#95296=AXIS2_PLACEMENT_3D('',#145636,#108214,#108215);
#95297=AXIS2_PLACEMENT_3D('',#145637,#108216,#108217);
#95298=AXIS2_PLACEMENT_3D('',#145656,#108218,#108219);
#95299=AXIS2_PLACEMENT_3D('',#145657,#108220,#108221);
#95300=AXIS2_PLACEMENT_3D('',#145659,#108222,#108223);
#95301=AXIS2_PLACEMENT_3D('',#145661,#108225,#108226);
#95302=AXIS2_PLACEMENT_3D('',#145664,#108227,#108228);
#95303=AXIS2_PLACEMENT_3D('',#145665,#108229,#108230);
#95304=AXIS2_PLACEMENT_3D('',#145670,#108231,#108232);
#95305=AXIS2_PLACEMENT_3D('',#145671,#108233,#108234);
#95306=AXIS2_PLACEMENT_3D('',#145672,#108235,#108236);
#95307=AXIS2_PLACEMENT_3D('',#145686,#108237,#108238);
#95308=AXIS2_PLACEMENT_3D('',#145687,#108239,#108240);
#95309=AXIS2_PLACEMENT_3D('',#145707,#108241,#108242);
#95310=AXIS2_PLACEMENT_3D('',#145733,#108243,#108244);
#95311=AXIS2_PLACEMENT_3D('',#145740,#108245,#108246);
#95312=AXIS2_PLACEMENT_3D('',#145742,#108247,#108248);
#95313=AXIS2_PLACEMENT_3D('',#145871,#108250,#108251);
#95314=AXIS2_PLACEMENT_3D('',#145890,#108252,#108253);
#95315=AXIS2_PLACEMENT_3D('',#145891,#108254,#108255);
#95316=AXIS2_PLACEMENT_3D('',#145893,#108256,#108257);
#95317=AXIS2_PLACEMENT_3D('',#145914,#108259,#108260);
#95318=AXIS2_PLACEMENT_3D('',#145934,#108261,#108262);
#95319=AXIS2_PLACEMENT_3D('',#145951,#108263,#108264);
#95320=AXIS2_PLACEMENT_3D('',#145952,#108265,#108266);
#95321=AXIS2_PLACEMENT_3D('',#145953,#108267,#108268);
#95322=AXIS2_PLACEMENT_3D('',#145954,#108269,#108270);
#95323=AXIS2_PLACEMENT_3D('',#145998,#108271,#108272);
#95324=AXIS2_PLACEMENT_3D('',#146024,#108273,#108274);
#95325=AXIS2_PLACEMENT_3D('',#146026,#108276,#108277);
#95326=AXIS2_PLACEMENT_3D('',#146033,#108279,#108280);
#95327=AXIS2_PLACEMENT_3D('',#146034,#108281,#108282);
#95328=AXIS2_PLACEMENT_3D('',#146047,#108283,#108284);
#95329=AXIS2_PLACEMENT_3D('',#146148,#108285,#108286);
#95330=AXIS2_PLACEMENT_3D('',#146149,#108287,#108288);
#95331=AXIS2_PLACEMENT_3D('',#146150,#108289,#108290);
#95332=AXIS2_PLACEMENT_3D('',#146164,#108291,#108292);
#95333=AXIS2_PLACEMENT_3D('',#146165,#108293,#108294);
#95334=AXIS2_PLACEMENT_3D('',#146179,#108295,#108296);
#95335=AXIS2_PLACEMENT_3D('',#146203,#108297,#108298);
#95336=AXIS2_PLACEMENT_3D('',#146211,#108299,#108300);
#95337=AXIS2_PLACEMENT_3D('',#146213,#108301,#108302);
#95338=AXIS2_PLACEMENT_3D('',#146299,#108304,#108305);
#95339=AXIS2_PLACEMENT_3D('',#146312,#108306,#108307);
#95340=AXIS2_PLACEMENT_3D('',#146325,#108308,#108309);
#95341=AXIS2_PLACEMENT_3D('',#146326,#108310,#108311);
#95342=AXIS2_PLACEMENT_3D('',#146328,#108312,#108313);
#95343=AXIS2_PLACEMENT_3D('',#146343,#108315,#108316);
#95344=AXIS2_PLACEMENT_3D('',#146344,#108317,#108318);
#95345=AXIS2_PLACEMENT_3D('',#146358,#108319,#108320);
#95346=AXIS2_PLACEMENT_3D('',#146375,#108321,#108322);
#95347=AXIS2_PLACEMENT_3D('',#146376,#108323,#108324);
#95348=AXIS2_PLACEMENT_3D('',#146377,#108325,#108326);
#95349=AXIS2_PLACEMENT_3D('',#146378,#108327,#108328);
#95350=AXIS2_PLACEMENT_3D('',#146410,#108329,#108330);
#95351=AXIS2_PLACEMENT_3D('',#146468,#108331,#108332);
#95352=AXIS2_PLACEMENT_3D('',#146470,#108334,#108335);
#95353=AXIS2_PLACEMENT_3D('',#146473,#108337,#108338);
#95354=AXIS2_PLACEMENT_3D('',#146474,#108339,#108340);
#95355=AXIS2_PLACEMENT_3D('',#146475,#108341,#108342);
#95356=AXIS2_PLACEMENT_3D('',#146488,#108343,#108344);
#95357=AXIS2_PLACEMENT_3D('',#146542,#108345,#108346);
#95358=AXIS2_PLACEMENT_3D('',#146543,#108347,#108348);
#95359=AXIS2_PLACEMENT_3D('',#146544,#108349,#108350);
#95360=AXIS2_PLACEMENT_3D('',#146558,#108351,#108352);
#95361=AXIS2_PLACEMENT_3D('',#146559,#108353,#108354);
#95362=AXIS2_PLACEMENT_3D('',#146573,#108355,#108356);
#95363=AXIS2_PLACEMENT_3D('',#146591,#108357,#108358);
#95364=AXIS2_PLACEMENT_3D('',#146592,#108359,#108360);
#95365=AXIS2_PLACEMENT_3D('',#146593,#108361,#108362);
#95366=AXIS2_PLACEMENT_3D('',#146595,#108363,#108364);
#95367=AXIS2_PLACEMENT_3D('',#146609,#108366,#108367);
#95368=AXIS2_PLACEMENT_3D('',#146679,#108368,#108369);
#95369=AXIS2_PLACEMENT_3D('',#146698,#108370,#108371);
#95370=AXIS2_PLACEMENT_3D('',#146699,#108372,#108373);
#95371=AXIS2_PLACEMENT_3D('',#146701,#108374,#108375);
#95372=AXIS2_PLACEMENT_3D('',#146722,#108377,#108378);
#95373=AXIS2_PLACEMENT_3D('',#146761,#108379,#108380);
#95374=AXIS2_PLACEMENT_3D('',#146778,#108381,#108382);
#95375=AXIS2_PLACEMENT_3D('',#146779,#108383,#108384);
#95376=AXIS2_PLACEMENT_3D('',#146780,#108385,#108386);
#95377=AXIS2_PLACEMENT_3D('',#146781,#108387,#108388);
#95378=AXIS2_PLACEMENT_3D('',#146825,#108389,#108390);
#95379=AXIS2_PLACEMENT_3D('',#146884,#108391,#108392);
#95380=AXIS2_PLACEMENT_3D('',#146886,#108394,#108395);
#95381=AXIS2_PLACEMENT_3D('',#146893,#108397,#108398);
#95382=AXIS2_PLACEMENT_3D('',#146894,#108399,#108400);
#95383=AXIS2_PLACEMENT_3D('',#146907,#108401,#108402);
#95384=AXIS2_PLACEMENT_3D('',#146971,#108403,#108404);
#95385=AXIS2_PLACEMENT_3D('',#146972,#108405,#108406);
#95386=AXIS2_PLACEMENT_3D('',#146973,#108407,#108408);
#95387=AXIS2_PLACEMENT_3D('',#146987,#108409,#108410);
#95388=AXIS2_PLACEMENT_3D('',#146988,#108411,#108412);
#95389=AXIS2_PLACEMENT_3D('',#147002,#108413,#108414);
#95390=AXIS2_PLACEMENT_3D('',#147026,#108415,#108416);
#95391=AXIS2_PLACEMENT_3D('',#147052,#108417,#108418);
#95392=AXIS2_PLACEMENT_3D('',#147054,#108419,#108420);
#95393=AXIS2_PLACEMENT_3D('',#147148,#108422,#108423);
#95394=AXIS2_PLACEMENT_3D('',#147167,#108424,#108425);
#95395=AXIS2_PLACEMENT_3D('',#147168,#108426,#108427);
#95396=AXIS2_PLACEMENT_3D('',#147170,#108428,#108429);
#95397=AXIS2_PLACEMENT_3D('',#147191,#108431,#108432);
#95398=AXIS2_PLACEMENT_3D('',#147239,#108433,#108434);
#95399=AXIS2_PLACEMENT_3D('',#147258,#108435,#108436);
#95400=AXIS2_PLACEMENT_3D('',#147259,#108437,#108438);
#95401=AXIS2_PLACEMENT_3D('',#147260,#108439,#108440);
#95402=AXIS2_PLACEMENT_3D('',#147261,#108441,#108442);
#95403=AXIS2_PLACEMENT_3D('',#147262,#108443,#108444);
#95404=AXIS2_PLACEMENT_3D('',#147264,#108445,#108446);
#95405=AXIS2_PLACEMENT_3D('',#147266,#108447,#108448);
#95406=AXIS2_PLACEMENT_3D('',#147268,#108449,#108450);
#95407=AXIS2_PLACEMENT_3D('',#147273,#108451,#108452);
#95408=AXIS2_PLACEMENT_3D('',#147275,#108453,#108454);
#95409=AXIS2_PLACEMENT_3D('',#147277,#108456,#108457);
#95410=AXIS2_PLACEMENT_3D('',#147278,#108458,#108459);
#95411=AXIS2_PLACEMENT_3D('',#147279,#108460,#108461);
#95412=AXIS2_PLACEMENT_3D('',#147281,#108462,#108463);
#95413=AXIS2_PLACEMENT_3D('',#147283,#108465,#108466);
#95414=AXIS2_PLACEMENT_3D('',#147284,#108467,#108468);
#95415=AXIS2_PLACEMENT_3D('',#147303,#108469,#108470);
#95416=AXIS2_PLACEMENT_3D('',#147304,#108471,#108472);
#95417=AXIS2_PLACEMENT_3D('',#147306,#108473,#108474);
#95418=AXIS2_PLACEMENT_3D('',#147308,#108476,#108477);
#95419=AXIS2_PLACEMENT_3D('',#147310,#108478,#108479);
#95420=AXIS2_PLACEMENT_3D('',#147311,#108480,#108481);
#95421=AXIS2_PLACEMENT_3D('',#147312,#108482,#108483);
#95422=AXIS2_PLACEMENT_3D('',#147352,#108485,#108486);
#95423=AXIS2_PLACEMENT_3D('',#147353,#108487,#108488);
#95424=AXIS2_PLACEMENT_3D('',#147354,#108489,#108490);
#95425=AXIS2_PLACEMENT_3D('',#147368,#108491,#108492);
#95426=AXIS2_PLACEMENT_3D('',#147369,#108493,#108494);
#95427=AXIS2_PLACEMENT_3D('',#147389,#108495,#108496);
#95428=AXIS2_PLACEMENT_3D('',#147415,#108497,#108498);
#95429=AXIS2_PLACEMENT_3D('',#147444,#108499,#108500);
#95430=AXIS2_PLACEMENT_3D('',#147446,#108501,#108502);
#95431=AXIS2_PLACEMENT_3D('',#147535,#108504,#108505);
#95432=AXIS2_PLACEMENT_3D('',#147549,#108506,#108507);
#95433=AXIS2_PLACEMENT_3D('',#147550,#108508,#108509);
#95434=AXIS2_PLACEMENT_3D('',#147551,#108510,#108511);
#95435=AXIS2_PLACEMENT_3D('',#147552,#108512,#108513);
#95436=AXIS2_PLACEMENT_3D('',#147553,#108514,#108515);
#95437=AXIS2_PLACEMENT_3D('',#147554,#108516,#108517);
#95438=AXIS2_PLACEMENT_3D('',#147556,#108518,#108519);
#95439=AXIS2_PLACEMENT_3D('',#147569,#108521,#108522);
#95440=AXIS2_PLACEMENT_3D('',#147571,#108523,#108524);
#95441=AXIS2_PLACEMENT_3D('',#147572,#108525,#108526);
#95442=AXIS2_PLACEMENT_3D('',#147573,#108527,#108528);
#95443=AXIS2_PLACEMENT_3D('',#147593,#108530,#108531);
#95444=AXIS2_PLACEMENT_3D('',#147594,#108532,#108533);
#95445=AXIS2_PLACEMENT_3D('',#147596,#108534,#108535);
#95446=AXIS2_PLACEMENT_3D('',#147617,#108537,#108538);
#95447=AXIS2_PLACEMENT_3D('',#147691,#108539,#108540);
#95448=AXIS2_PLACEMENT_3D('',#147702,#108541,#108542);
#95449=AXIS2_PLACEMENT_3D('',#147703,#108543,#108544);
#95450=AXIS2_PLACEMENT_3D('',#147704,#108545,#108546);
#95451=AXIS2_PLACEMENT_3D('',#147705,#108547,#108548);
#95452=AXIS2_PLACEMENT_3D('',#147706,#108549,#108550);
#95453=AXIS2_PLACEMENT_3D('',#147708,#108551,#108552);
#95454=AXIS2_PLACEMENT_3D('',#147746,#108553,#108554);
#95455=AXIS2_PLACEMENT_3D('',#147748,#108555,#108556);
#95456=AXIS2_PLACEMENT_3D('',#147749,#108557,#108558);
#95457=AXIS2_PLACEMENT_3D('',#147760,#108559,#108560);
#95458=AXIS2_PLACEMENT_3D('',#147761,#108561,#108562);
#95459=AXIS2_PLACEMENT_3D('',#147762,#108563,#108564);
#95460=AXIS2_PLACEMENT_3D('',#147764,#108565,#108566);
#95461=AXIS2_PLACEMENT_3D('',#147773,#108568,#108569);
#95462=AXIS2_PLACEMENT_3D('',#147775,#108570,#108571);
#95463=AXIS2_PLACEMENT_3D('',#147776,#108572,#108573);
#95464=AXIS2_PLACEMENT_3D('',#147777,#108574,#108575);
#95465=AXIS2_PLACEMENT_3D('',#147779,#108576,#108577);
#95466=AXIS2_PLACEMENT_3D('',#147781,#108579,#108580);
#95467=AXIS2_PLACEMENT_3D('',#147782,#108581,#108582);
#95468=AXIS2_PLACEMENT_3D('',#147813,#108583,#108584);
#95469=AXIS2_PLACEMENT_3D('',#147839,#108585,#108586);
#95470=AXIS2_PLACEMENT_3D('',#147850,#108587,#108588);
#95471=AXIS2_PLACEMENT_3D('',#147852,#108589,#108590);
#95472=AXIS2_PLACEMENT_3D('',#147885,#108592,#108593);
#95473=AXIS2_PLACEMENT_3D('',#147948,#108594,#108595);
#95474=AXIS2_PLACEMENT_3D('',#147968,#108596,#108597);
#95475=AXIS2_PLACEMENT_3D('',#147969,#108598,#108599);
#95476=AXIS2_PLACEMENT_3D('',#147970,#108600,#108601);
#95477=AXIS2_PLACEMENT_3D('',#147972,#108603,#108604);
#95478=AXIS2_PLACEMENT_3D('',#147975,#108606,#108607);
#95479=AXIS2_PLACEMENT_3D('',#147976,#108608,#108609);
#95480=AXIS2_PLACEMENT_3D('',#147977,#108610,#108611);
#95481=AXIS2_PLACEMENT_3D('',#147978,#108612,#108613);
#95482=AXIS2_PLACEMENT_3D('',#147979,#108614,#108615);
#95483=AXIS2_PLACEMENT_3D('',#147980,#108616,#108617);
#95484=AXIS2_PLACEMENT_3D('',#147981,#108618,#108619);
#95485=AXIS2_PLACEMENT_3D('',#147982,#108620,#108621);
#95486=AXIS2_PLACEMENT_3D('',#147983,#108622,#108623);
#95487=AXIS2_PLACEMENT_3D('',#147984,#108624,#108625);
#95488=AXIS2_PLACEMENT_3D('',#147987,#108627,#108628);
#95489=AXIS2_PLACEMENT_3D('',#148018,#108629,#108630);
#95490=AXIS2_PLACEMENT_3D('',#148020,#108631,#108632);
#95491=AXIS2_PLACEMENT_3D('',#148022,#108634,#108635);
#95492=AXIS2_PLACEMENT_3D('',#148024,#108636,#108637);
#95493=AXIS2_PLACEMENT_3D('',#148025,#108638,#108639);
#95494=AXIS2_PLACEMENT_3D('',#148026,#108640,#108641);
#95495=AXIS2_PLACEMENT_3D('',#148035,#108643,#108644);
#95496=AXIS2_PLACEMENT_3D('',#148036,#108645,#108646);
#95497=AXIS2_PLACEMENT_3D('',#148037,#108647,#108648);
#95498=AXIS2_PLACEMENT_3D('',#148068,#108649,#108650);
#95499=AXIS2_PLACEMENT_3D('',#148079,#108651,#108652);
#95500=AXIS2_PLACEMENT_3D('',#148092,#108653,#108654);
#95501=AXIS2_PLACEMENT_3D('',#148111,#108655,#108656);
#95502=AXIS2_PLACEMENT_3D('',#148125,#108657,#108658);
#95503=AXIS2_PLACEMENT_3D('',#148126,#108659,#108660);
#95504=AXIS2_PLACEMENT_3D('',#148140,#108661,#108662);
#95505=AXIS2_PLACEMENT_3D('',#148164,#108663,#108664);
#95506=AXIS2_PLACEMENT_3D('',#148196,#108665,#108666);
#95507=AXIS2_PLACEMENT_3D('',#148198,#108667,#108668);
#95508=AXIS2_PLACEMENT_3D('',#148225,#108670,#108671);
#95509=AXIS2_PLACEMENT_3D('',#148250,#108672,#108673);
#95510=AXIS2_PLACEMENT_3D('',#148252,#108674,#108675);
#95511=AXIS2_PLACEMENT_3D('',#148254,#108677,#108678);
#95512=AXIS2_PLACEMENT_3D('',#148255,#108679,#108680);
#95513=AXIS2_PLACEMENT_3D('',#148256,#108681,#108682);
#95514=AXIS2_PLACEMENT_3D('',#148290,#108683,#108684);
#95515=AXIS2_PLACEMENT_3D('',#148291,#108685,#108686);
#95516=AXIS2_PLACEMENT_3D('',#148292,#108687,#108688);
#95517=AXIS2_PLACEMENT_3D('',#148305,#108689,#108690);
#95518=AXIS2_PLACEMENT_3D('',#148331,#108691,#108692);
#95519=AXIS2_PLACEMENT_3D('',#148342,#108693,#108694);
#95520=AXIS2_PLACEMENT_3D('',#148344,#108695,#108696);
#95521=AXIS2_PLACEMENT_3D('',#148377,#108698,#108699);
#95522=AXIS2_PLACEMENT_3D('',#148431,#108700,#108701);
#95523=AXIS2_PLACEMENT_3D('',#148467,#108702,#108703);
#95524=AXIS2_PLACEMENT_3D('',#148478,#108704,#108705);
#95525=AXIS2_PLACEMENT_3D('',#148480,#108706,#108707);
#95526=AXIS2_PLACEMENT_3D('',#148512,#108709,#108710);
#95527=AXIS2_PLACEMENT_3D('',#148523,#108711,#108712);
#95528=AXIS2_PLACEMENT_3D('',#148524,#108713,#108714);
#95529=AXIS2_PLACEMENT_3D('',#148525,#108715,#108716);
#95530=AXIS2_PLACEMENT_3D('',#148527,#108717,#108718);
#95531=AXIS2_PLACEMENT_3D('',#148536,#108720,#108721);
#95532=AXIS2_PLACEMENT_3D('',#148538,#108722,#108723);
#95533=AXIS2_PLACEMENT_3D('',#148539,#108724,#108725);
#95534=AXIS2_PLACEMENT_3D('',#148540,#108726,#108727);
#95535=AXIS2_PLACEMENT_3D('',#148542,#108728,#108729);
#95536=AXIS2_PLACEMENT_3D('',#148544,#108731,#108732);
#95537=AXIS2_PLACEMENT_3D('',#148545,#108733,#108734);
#95538=AXIS2_PLACEMENT_3D('',#148546,#108735,#108736);
#95539=AXIS2_PLACEMENT_3D('',#148548,#108737,#108738);
#95540=AXIS2_PLACEMENT_3D('',#148550,#108740,#108741);
#95541=AXIS2_PLACEMENT_3D('',#148551,#108742,#108743);
#95542=AXIS2_PLACEMENT_3D('',#148552,#108744,#108745);
#95543=AXIS2_PLACEMENT_3D('',#148556,#108747,#108748);
#95544=AXIS2_PLACEMENT_3D('',#148563,#108749,#108750);
#95545=AXIS2_PLACEMENT_3D('',#148564,#108751,#108752);
#95546=AXIS2_PLACEMENT_3D('',#148565,#108753,#108754);
#95547=AXIS2_PLACEMENT_3D('',#148597,#108755,#108756);
#95548=AXIS2_PLACEMENT_3D('',#148608,#108757,#108758);
#95549=AXIS2_PLACEMENT_3D('',#148610,#108759,#108760);
#95550=AXIS2_PLACEMENT_3D('',#148631,#108762,#108763);
#95551=AXIS2_PLACEMENT_3D('',#148651,#108764,#108765);
#95552=AXIS2_PLACEMENT_3D('',#148681,#108766,#108767);
#95553=AXIS2_PLACEMENT_3D('',#148722,#108768,#108769);
#95554=AXIS2_PLACEMENT_3D('',#148724,#108770,#108771);
#95555=AXIS2_PLACEMENT_3D('',#148751,#108773,#108774);
#95556=AXIS2_PLACEMENT_3D('',#148772,#108775,#108776);
#95557=AXIS2_PLACEMENT_3D('',#148795,#108777,#108778);
#95558=AXIS2_PLACEMENT_3D('',#148797,#108779,#108780);
#95559=AXIS2_PLACEMENT_3D('',#148799,#108782,#108783);
#95560=AXIS2_PLACEMENT_3D('',#148800,#108784,#108785);
#95561=AXIS2_PLACEMENT_3D('',#148801,#108786,#108787);
#95562=AXIS2_PLACEMENT_3D('',#148804,#108788,#108789);
#95563=AXIS2_PLACEMENT_3D('',#148819,#108790,#108791);
#95564=AXIS2_PLACEMENT_3D('',#148820,#108792,#108793);
#95565=AXIS2_PLACEMENT_3D('',#148821,#108794,#108795);
#95566=AXIS2_PLACEMENT_3D('',#148822,#108796,#108797);
#95567=AXIS2_PLACEMENT_3D('',#148841,#108798,#108799);
#95568=AXIS2_PLACEMENT_3D('',#148855,#108800,#108801);
#95569=AXIS2_PLACEMENT_3D('',#148884,#108802,#108803);
#95570=AXIS2_PLACEMENT_3D('',#148925,#108804,#108805);
#95571=AXIS2_PLACEMENT_3D('',#148926,#108806,#108807);
#95572=AXIS2_PLACEMENT_3D('',#148927,#108808,#108809);
#95573=AXIS2_PLACEMENT_3D('',#148928,#108810,#108811);
#95574=AXIS2_PLACEMENT_3D('',#148929,#108812,#108813);
#95575=AXIS2_PLACEMENT_3D('',#148930,#108814,#108815);
#95576=AXIS2_PLACEMENT_3D('',#148931,#108816,#108817);
#95577=AXIS2_PLACEMENT_3D('',#148932,#108818,#108819);
#95578=AXIS2_PLACEMENT_3D('',#148963,#108820,#108821);
#95579=AXIS2_PLACEMENT_3D('',#149016,#108822,#108823);
#95580=AXIS2_PLACEMENT_3D('',#149018,#108825,#108826);
#95581=AXIS2_PLACEMENT_3D('',#149019,#108827,#108828);
#95582=AXIS2_PLACEMENT_3D('',#149020,#108829,#108830);
#95583=AXIS2_PLACEMENT_3D('',#149021,#108831,#108832);
#95584=AXIS2_PLACEMENT_3D('',#149022,#108833,#108834);
#95585=AXIS2_PLACEMENT_3D('',#149023,#108835,#108836);
#95586=AXIS2_PLACEMENT_3D('',#149024,#108837,#108838);
#95587=AXIS2_PLACEMENT_3D('',#149025,#108839,#108840);
#95588=AXIS2_PLACEMENT_3D('',#149026,#108841,#108842);
#95589=AXIS2_PLACEMENT_3D('',#149052,#108843,#108844);
#95590=AXIS2_PLACEMENT_3D('',#149073,#108845,#108846);
#95591=AXIS2_PLACEMENT_3D('',#149102,#108847,#108848);
#95592=AXIS2_PLACEMENT_3D('',#149105,#108849,#108850);
#95593=AXIS2_PLACEMENT_3D('',#149122,#108851,#108852);
#95594=AXIS2_PLACEMENT_3D('',#149123,#108853,#108854);
#95595=AXIS2_PLACEMENT_3D('',#149124,#108855,#108856);
#95596=AXIS2_PLACEMENT_3D('',#149125,#108857,#108858);
#95597=AXIS2_PLACEMENT_3D('',#149157,#108859,#108860);
#95598=AXIS2_PLACEMENT_3D('',#149159,#108861,#108862);
#95599=AXIS2_PLACEMENT_3D('',#149160,#108863,#108864);
#95600=AXIS2_PLACEMENT_3D('',#149171,#108865,#108866);
#95601=AXIS2_PLACEMENT_3D('',#149172,#108867,#108868);
#95602=AXIS2_PLACEMENT_3D('',#149173,#108869,#108870);
#95603=AXIS2_PLACEMENT_3D('',#149175,#108871,#108872);
#95604=AXIS2_PLACEMENT_3D('',#149184,#108874,#108875);
#95605=AXIS2_PLACEMENT_3D('',#149186,#108876,#108877);
#95606=AXIS2_PLACEMENT_3D('',#149187,#108878,#108879);
#95607=AXIS2_PLACEMENT_3D('',#149188,#108880,#108881);
#95608=AXIS2_PLACEMENT_3D('',#149190,#108882,#108883);
#95609=AXIS2_PLACEMENT_3D('',#149192,#108885,#108886);
#95610=AXIS2_PLACEMENT_3D('',#149193,#108887,#108888);
#95611=AXIS2_PLACEMENT_3D('',#149224,#108889,#108890);
#95612=AXIS2_PLACEMENT_3D('',#149238,#108891,#108892);
#95613=AXIS2_PLACEMENT_3D('',#149274,#108893,#108894);
#95614=AXIS2_PLACEMENT_3D('',#149324,#108895,#108896);
#95615=AXIS2_PLACEMENT_3D('',#149326,#108897,#108898);
#95616=AXIS2_PLACEMENT_3D('',#149365,#108900,#108901);
#95617=AXIS2_PLACEMENT_3D('',#149428,#108902,#108903);
#95618=AXIS2_PLACEMENT_3D('',#149458,#108904,#108905);
#95619=AXIS2_PLACEMENT_3D('',#149467,#108906,#108907);
#95620=AXIS2_PLACEMENT_3D('',#149469,#108909,#108910);
#95621=AXIS2_PLACEMENT_3D('',#149472,#108912,#108913);
#95622=AXIS2_PLACEMENT_3D('',#149473,#108914,#108915);
#95623=AXIS2_PLACEMENT_3D('',#149474,#108916,#108917);
#95624=AXIS2_PLACEMENT_3D('',#149475,#108918,#108919);
#95625=AXIS2_PLACEMENT_3D('',#149507,#108921,#108922);
#95626=AXIS2_PLACEMENT_3D('',#149509,#108923,#108924);
#95627=AXIS2_PLACEMENT_3D('',#149511,#108926,#108927);
#95628=AXIS2_PLACEMENT_3D('',#149513,#108928,#108929);
#95629=AXIS2_PLACEMENT_3D('',#149514,#108930,#108931);
#95630=AXIS2_PLACEMENT_3D('',#149515,#108932,#108933);
#95631=AXIS2_PLACEMENT_3D('',#149524,#108935,#108936);
#95632=AXIS2_PLACEMENT_3D('',#149525,#108937,#108938);
#95633=AXIS2_PLACEMENT_3D('',#149526,#108939,#108940);
#95634=AXIS2_PLACEMENT_3D('',#149557,#108941,#108942);
#95635=AXIS2_PLACEMENT_3D('',#149568,#108943,#108944);
#95636=AXIS2_PLACEMENT_3D('',#149569,#108945,#108946);
#95637=AXIS2_PLACEMENT_3D('',#149570,#108947,#108948);
#95638=AXIS2_PLACEMENT_3D('',#149571,#108949,#108950);
#95639=AXIS2_PLACEMENT_3D('',#149586,#108952,#108953);
#95640=AXIS2_PLACEMENT_3D('',#149593,#108954,#108955);
#95641=AXIS2_PLACEMENT_3D('',#149594,#108956,#108957);
#95642=AXIS2_PLACEMENT_3D('',#149595,#108958,#108959);
#95643=AXIS2_PLACEMENT_3D('',#149615,#108960,#108961);
#95644=AXIS2_PLACEMENT_3D('',#149654,#108962,#108963);
#95645=AXIS2_PLACEMENT_3D('',#149655,#108964,#108965);
#95646=AXIS2_PLACEMENT_3D('',#149675,#108966,#108967);
#95647=AXIS2_PLACEMENT_3D('',#149701,#108968,#108969);
#95648=AXIS2_PLACEMENT_3D('',#149739,#108970,#108971);
#95649=AXIS2_PLACEMENT_3D('',#149741,#108972,#108973);
#95650=AXIS2_PLACEMENT_3D('',#149768,#108975,#108976);
#95651=AXIS2_PLACEMENT_3D('',#149797,#108977,#108978);
#95652=AXIS2_PLACEMENT_3D('',#149816,#108979,#108980);
#95653=AXIS2_PLACEMENT_3D('',#149829,#108981,#108982);
#95654=AXIS2_PLACEMENT_3D('',#149831,#108983,#108984);
#95655=AXIS2_PLACEMENT_3D('',#149833,#108986,#108987);
#95656=AXIS2_PLACEMENT_3D('',#149834,#108988,#108989);
#95657=AXIS2_PLACEMENT_3D('',#149835,#108990,#108991);
#95658=AXIS2_PLACEMENT_3D('',#149872,#108992,#108993);
#95659=AXIS2_PLACEMENT_3D('',#149873,#108994,#108995);
#95660=AXIS2_PLACEMENT_3D('',#149874,#108996,#108997);
#95661=AXIS2_PLACEMENT_3D('',#149887,#108998,#108999);
#95662=AXIS2_PLACEMENT_3D('',#149913,#109000,#109001);
#95663=AXIS2_PLACEMENT_3D('',#149924,#109002,#109003);
#95664=AXIS2_PLACEMENT_3D('',#149926,#109004,#109005);
#95665=AXIS2_PLACEMENT_3D('',#149959,#109007,#109008);
#95666=AXIS2_PLACEMENT_3D('',#149983,#109009,#109010);
#95667=AXIS2_PLACEMENT_3D('',#150019,#109011,#109012);
#95668=AXIS2_PLACEMENT_3D('',#150030,#109013,#109014);
#95669=AXIS2_PLACEMENT_3D('',#150032,#109015,#109016);
#95670=AXIS2_PLACEMENT_3D('',#150064,#109018,#109019);
#95671=AXIS2_PLACEMENT_3D('',#150075,#109020,#109021);
#95672=AXIS2_PLACEMENT_3D('',#150076,#109022,#109023);
#95673=AXIS2_PLACEMENT_3D('',#150077,#109024,#109025);
#95674=AXIS2_PLACEMENT_3D('',#150079,#109026,#109027);
#95675=AXIS2_PLACEMENT_3D('',#150088,#109029,#109030);
#95676=AXIS2_PLACEMENT_3D('',#150090,#109031,#109032);
#95677=AXIS2_PLACEMENT_3D('',#150091,#109033,#109034);
#95678=AXIS2_PLACEMENT_3D('',#150092,#109035,#109036);
#95679=AXIS2_PLACEMENT_3D('',#150094,#109037,#109038);
#95680=AXIS2_PLACEMENT_3D('',#150096,#109040,#109041);
#95681=AXIS2_PLACEMENT_3D('',#150097,#109042,#109043);
#95682=AXIS2_PLACEMENT_3D('',#150098,#109044,#109045);
#95683=AXIS2_PLACEMENT_3D('',#150100,#109046,#109047);
#95684=AXIS2_PLACEMENT_3D('',#150102,#109049,#109050);
#95685=AXIS2_PLACEMENT_3D('',#150103,#109051,#109052);
#95686=AXIS2_PLACEMENT_3D('',#150104,#109053,#109054);
#95687=AXIS2_PLACEMENT_3D('',#150108,#109056,#109057);
#95688=AXIS2_PLACEMENT_3D('',#150115,#109058,#109059);
#95689=AXIS2_PLACEMENT_3D('',#150116,#109060,#109061);
#95690=AXIS2_PLACEMENT_3D('',#150117,#109062,#109063);
#95691=AXIS2_PLACEMENT_3D('',#150149,#109064,#109065);
#95692=AXIS2_PLACEMENT_3D('',#150160,#109066,#109067);
#95693=AXIS2_PLACEMENT_3D('',#150162,#109068,#109069);
#95694=AXIS2_PLACEMENT_3D('',#150183,#109071,#109072);
#95695=AXIS2_PLACEMENT_3D('',#150203,#109073,#109074);
#95696=AXIS2_PLACEMENT_3D('',#150233,#109075,#109076);
#95697=AXIS2_PLACEMENT_3D('',#150274,#109077,#109078);
#95698=AXIS2_PLACEMENT_3D('',#150276,#109079,#109080);
#95699=AXIS2_PLACEMENT_3D('',#150303,#109082,#109083);
#95700=AXIS2_PLACEMENT_3D('',#150362,#109084,#109085);
#95701=AXIS2_PLACEMENT_3D('',#150385,#109086,#109087);
#95702=AXIS2_PLACEMENT_3D('',#150387,#109088,#109089);
#95703=AXIS2_PLACEMENT_3D('',#150389,#109091,#109092);
#95704=AXIS2_PLACEMENT_3D('',#150390,#109093,#109094);
#95705=AXIS2_PLACEMENT_3D('',#150391,#109095,#109096);
#95706=AXIS2_PLACEMENT_3D('',#150423,#109097,#109098);
#95707=AXIS2_PLACEMENT_3D('',#150454,#109099,#109100);
#95708=AXIS2_PLACEMENT_3D('',#150455,#109101,#109102);
#95709=AXIS2_PLACEMENT_3D('',#150475,#109103,#109104);
#95710=AXIS2_PLACEMENT_3D('',#150476,#109105,#109106);
#95711=AXIS2_PLACEMENT_3D('',#150483,#109107,#109108);
#95712=AXIS2_PLACEMENT_3D('',#150484,#109109,#109110);
#95713=AXIS2_PLACEMENT_3D('',#150485,#109111,#109112);
#95714=AXIS2_PLACEMENT_3D('',#150494,#109113,#109114);
#95715=AXIS2_PLACEMENT_3D('',#150497,#109116,#109117);
#95716=AXIS2_PLACEMENT_3D('',#150498,#109118,#109119);
#95717=AXIS2_PLACEMENT_3D('',#150500,#109120,#109121);
#95718=AXIS2_PLACEMENT_3D('',#150501,#109122,#109123);
#95719=AXIS2_PLACEMENT_3D('',#150502,#109124,#109125);
#95720=AXIS2_PLACEMENT_3D('',#150522,#109127,#109128);
#95721=AXIS2_PLACEMENT_3D('',#150542,#109129,#109130);
#95722=AXIS2_PLACEMENT_3D('',#150580,#109131,#109132);
#95723=AXIS2_PLACEMENT_3D('',#150582,#109133,#109134);
#95724=AXIS2_PLACEMENT_3D('',#150609,#109136,#109137);
#95725=AXIS2_PLACEMENT_3D('',#150639,#109138,#109139);
#95726=AXIS2_PLACEMENT_3D('',#150658,#109140,#109141);
#95727=AXIS2_PLACEMENT_3D('',#150689,#109142,#109143);
#95728=AXIS2_PLACEMENT_3D('',#150690,#109144,#109145);
#95729=AXIS2_PLACEMENT_3D('',#150701,#109146,#109147);
#95730=AXIS2_PLACEMENT_3D('',#150702,#109148,#109149);
#95731=AXIS2_PLACEMENT_3D('',#150703,#109150,#109151);
#95732=AXIS2_PLACEMENT_3D('',#150705,#109152,#109153);
#95733=AXIS2_PLACEMENT_3D('',#150714,#109155,#109156);
#95734=AXIS2_PLACEMENT_3D('',#150716,#109157,#109158);
#95735=AXIS2_PLACEMENT_3D('',#150717,#109159,#109160);
#95736=AXIS2_PLACEMENT_3D('',#150718,#109161,#109162);
#95737=AXIS2_PLACEMENT_3D('',#150720,#109163,#109164);
#95738=AXIS2_PLACEMENT_3D('',#150722,#109166,#109167);
#95739=AXIS2_PLACEMENT_3D('',#150723,#109168,#109169);
#95740=AXIS2_PLACEMENT_3D('',#150754,#109170,#109171);
#95741=AXIS2_PLACEMENT_3D('',#150755,#109172,#109173);
#95742=AXIS2_PLACEMENT_3D('',#150757,#109174,#109175);
#95743=AXIS2_PLACEMENT_3D('',#150759,#109177,#109178);
#95744=AXIS2_PLACEMENT_3D('',#150760,#109179,#109180);
#95745=AXIS2_PLACEMENT_3D('',#150761,#109181,#109182);
#95746=AXIS2_PLACEMENT_3D('',#150762,#109183,#109184);
#95747=AXIS2_PLACEMENT_3D('',#150764,#109185,#109186);
#95748=AXIS2_PLACEMENT_3D('',#150766,#109188,#109189);
#95749=AXIS2_PLACEMENT_3D('',#150767,#109190,#109191);
#95750=AXIS2_PLACEMENT_3D('',#150768,#109192,#109193);
#95751=AXIS2_PLACEMENT_3D('',#150772,#109195,#109196);
#95752=AXIS2_PLACEMENT_3D('',#150779,#109197,#109198);
#95753=AXIS2_PLACEMENT_3D('',#150781,#109199,#109200);
#95754=AXIS2_PLACEMENT_3D('',#150782,#109201,#109202);
#95755=AXIS2_PLACEMENT_3D('',#150783,#109203,#109204);
#95756=AXIS2_PLACEMENT_3D('',#150815,#109205,#109206);
#95757=AXIS2_PLACEMENT_3D('',#150826,#109207,#109208);
#95758=AXIS2_PLACEMENT_3D('',#150828,#109209,#109210);
#95759=AXIS2_PLACEMENT_3D('',#150861,#109212,#109213);
#95760=AXIS2_PLACEMENT_3D('',#150885,#109214,#109215);
#95761=AXIS2_PLACEMENT_3D('',#150921,#109216,#109217);
#95762=AXIS2_PLACEMENT_3D('',#150971,#109218,#109219);
#95763=AXIS2_PLACEMENT_3D('',#150973,#109220,#109221);
#95764=AXIS2_PLACEMENT_3D('',#151012,#109223,#109224);
#95765=AXIS2_PLACEMENT_3D('',#151075,#109225,#109226);
#95766=AXIS2_PLACEMENT_3D('',#151104,#109227,#109228);
#95767=AXIS2_PLACEMENT_3D('',#151113,#109229,#109230);
#95768=AXIS2_PLACEMENT_3D('',#151114,#109231,#109232);
#95769=AXIS2_PLACEMENT_3D('',#151116,#109233,#109234);
#95770=AXIS2_PLACEMENT_3D('',#151118,#109236,#109237);
#95771=AXIS2_PLACEMENT_3D('',#151119,#109238,#109239);
#95772=AXIS2_PLACEMENT_3D('',#151120,#109240,#109241);
#95773=AXIS2_PLACEMENT_3D('',#151122,#109242,#109243);
#95774=AXIS2_PLACEMENT_3D('',#151129,#109244,#109245);
#95775=AXIS2_PLACEMENT_3D('',#151130,#109246,#109247);
#95776=AXIS2_PLACEMENT_3D('',#151149,#109248,#109249);
#95777=AXIS2_PLACEMENT_3D('',#151163,#109250,#109251);
#95778=AXIS2_PLACEMENT_3D('',#151193,#109252,#109253);
#95779=AXIS2_PLACEMENT_3D('',#151237,#109254,#109255);
#95780=AXIS2_PLACEMENT_3D('',#151239,#109256,#109257);
#95781=AXIS2_PLACEMENT_3D('',#151266,#109259,#109260);
#95782=AXIS2_PLACEMENT_3D('',#151326,#109261,#109262);
#95783=AXIS2_PLACEMENT_3D('',#151350,#109263,#109264);
#95784=AXIS2_PLACEMENT_3D('',#151357,#109265,#109266);
#95785=AXIS2_PLACEMENT_3D('',#151359,#109267,#109268);
#95786=AXIS2_PLACEMENT_3D('',#151391,#109270,#109271);
#95787=AXIS2_PLACEMENT_3D('',#151402,#109272,#109273);
#95788=AXIS2_PLACEMENT_3D('',#151403,#109274,#109275);
#95789=AXIS2_PLACEMENT_3D('',#151404,#109276,#109277);
#95790=AXIS2_PLACEMENT_3D('',#151406,#109278,#109279);
#95791=AXIS2_PLACEMENT_3D('',#151415,#109281,#109282);
#95792=AXIS2_PLACEMENT_3D('',#151417,#109283,#109284);
#95793=AXIS2_PLACEMENT_3D('',#151418,#109285,#109286);
#95794=AXIS2_PLACEMENT_3D('',#151419,#109287,#109288);
#95795=AXIS2_PLACEMENT_3D('',#151421,#109289,#109290);
#95796=AXIS2_PLACEMENT_3D('',#151423,#109292,#109293);
#95797=AXIS2_PLACEMENT_3D('',#151424,#109294,#109295);
#95798=AXIS2_PLACEMENT_3D('',#151425,#109296,#109297);
#95799=AXIS2_PLACEMENT_3D('',#151427,#109298,#109299);
#95800=AXIS2_PLACEMENT_3D('',#151429,#109301,#109302);
#95801=AXIS2_PLACEMENT_3D('',#151430,#109303,#109304);
#95802=AXIS2_PLACEMENT_3D('',#151431,#109305,#109306);
#95803=AXIS2_PLACEMENT_3D('',#151432,#109307,#109308);
#95804=AXIS2_PLACEMENT_3D('',#151436,#109310,#109311);
#95805=AXIS2_PLACEMENT_3D('',#151443,#109312,#109313);
#95806=AXIS2_PLACEMENT_3D('',#151445,#109314,#109315);
#95807=AXIS2_PLACEMENT_3D('',#151446,#109316,#109317);
#95808=AXIS2_PLACEMENT_3D('',#151447,#109318,#109319);
#95809=AXIS2_PLACEMENT_3D('',#151479,#109320,#109321);
#95810=AXIS2_PLACEMENT_3D('',#151490,#109322,#109323);
#95811=AXIS2_PLACEMENT_3D('',#151492,#109324,#109325);
#95812=AXIS2_PLACEMENT_3D('',#151519,#109327,#109328);
#95813=AXIS2_PLACEMENT_3D('',#151541,#109329,#109330);
#95814=AXIS2_PLACEMENT_3D('',#151571,#109331,#109332);
#95815=AXIS2_PLACEMENT_3D('',#151582,#109333,#109334);
#95816=AXIS2_PLACEMENT_3D('',#151584,#109335,#109336);
#95817=AXIS2_PLACEMENT_3D('',#151610,#109338,#109339);
#95818=AXIS2_PLACEMENT_3D('',#151666,#109340,#109341);
#95819=AXIS2_PLACEMENT_3D('',#151668,#109342,#109343);
#95820=AXIS2_PLACEMENT_3D('',#151670,#109345,#109346);
#95821=AXIS2_PLACEMENT_3D('',#151671,#109347,#109348);
#95822=AXIS2_PLACEMENT_3D('',#151672,#109349,#109350);
#95823=AXIS2_PLACEMENT_3D('',#151673,#109351,#109352);
#95824=AXIS2_PLACEMENT_3D('',#151674,#109353,#109354);
#95825=AXIS2_PLACEMENT_3D('',#151675,#109355,#109356);
#95826=AXIS2_PLACEMENT_3D('',#151720,#109358,#109359);
#95827=AXIS2_PLACEMENT_3D('',#151721,#109360,#109361);
#95828=AXIS2_PLACEMENT_3D('',#151722,#109362,#109363);
#95829=AXIS2_PLACEMENT_3D('',#151723,#109364,#109365);
#95830=AXIS2_PLACEMENT_3D('',#151724,#109366,#109367);
#95831=AXIS2_PLACEMENT_3D('',#151725,#109368,#109369);
#95832=AXIS2_PLACEMENT_3D('',#151726,#109370,#109371);
#95833=AXIS2_PLACEMENT_3D('',#151727,#109372,#109373);
#95834=AXIS2_PLACEMENT_3D('',#151728,#109374,#109375);
#95835=AXIS2_PLACEMENT_3D('',#151729,#109376,#109377);
#95836=AXIS2_PLACEMENT_3D('',#151748,#109378,#109379);
#95837=AXIS2_PLACEMENT_3D('',#151749,#109380,#109381);
#95838=AXIS2_PLACEMENT_3D('',#151750,#109382,#109383);
#95839=AXIS2_PLACEMENT_3D('',#151770,#109385,#109386);
#95840=AXIS2_PLACEMENT_3D('',#151790,#109388,#109389);
#95841=AXIS2_PLACEMENT_3D('',#151791,#109390,#109391);
#95842=AXIS2_PLACEMENT_3D('',#151792,#109392,#109393);
#95843=AXIS2_PLACEMENT_3D('',#151812,#109395,#109396);
#95844=AXIS2_PLACEMENT_3D('',#151814,#109397,#109398);
#95845=AXIS2_PLACEMENT_3D('',#151835,#109400,#109401);
#95846=AXIS2_PLACEMENT_3D('',#151860,#109402,#109403);
#95847=AXIS2_PLACEMENT_3D('',#151889,#109404,#109405);
#95848=AXIS2_PLACEMENT_3D('',#151890,#109406,#109407);
#95849=AXIS2_PLACEMENT_3D('',#151891,#109408,#109409);
#95850=AXIS2_PLACEMENT_3D('',#151892,#109410,#109411);
#95851=AXIS2_PLACEMENT_3D('',#151923,#109412,#109413);
#95852=AXIS2_PLACEMENT_3D('',#151924,#109414,#109415);
#95853=AXIS2_PLACEMENT_3D('',#151955,#109416,#109417);
#95854=AXIS2_PLACEMENT_3D('',#151956,#109418,#109419);
#95855=AXIS2_PLACEMENT_3D('',#151958,#109420,#109421);
#95856=AXIS2_PLACEMENT_3D('',#151959,#109422,#109423);
#95857=AXIS2_PLACEMENT_3D('',#151972,#109424,#109425);
#95858=AXIS2_PLACEMENT_3D('',#151989,#109426,#109427);
#95859=AXIS2_PLACEMENT_3D('',#151990,#109428,#109429);
#95860=AXIS2_PLACEMENT_3D('',#152009,#109430,#109431);
#95861=AXIS2_PLACEMENT_3D('',#152022,#109432,#109433);
#95862=AXIS2_PLACEMENT_3D('',#152023,#109434,#109435);
#95863=AXIS2_PLACEMENT_3D('',#152054,#109436,#109437);
#95864=AXIS2_PLACEMENT_3D('',#152055,#109438,#109439);
#95865=AXIS2_PLACEMENT_3D('',#152092,#109440,#109441);
#95866=AXIS2_PLACEMENT_3D('',#152105,#109442,#109443);
#95867=AXIS2_PLACEMENT_3D('',#152106,#109444,#109445);
#95868=AXIS2_PLACEMENT_3D('',#152131,#109446,#109447);
#95869=AXIS2_PLACEMENT_3D('',#152132,#109448,#109449);
#95870=AXIS2_PLACEMENT_3D('',#152157,#109450,#109451);
#95871=AXIS2_PLACEMENT_3D('',#152170,#109452,#109453);
#95872=AXIS2_PLACEMENT_3D('',#152171,#109454,#109455);
#95873=AXIS2_PLACEMENT_3D('',#152202,#109456,#109457);
#95874=AXIS2_PLACEMENT_3D('',#152203,#109458,#109459);
#95875=AXIS2_PLACEMENT_3D('',#152216,#109460,#109461);
#95876=AXIS2_PLACEMENT_3D('',#152236,#109462,#109463);
#95877=AXIS2_PLACEMENT_3D('',#152243,#109464,#109465);
#95878=AXIS2_PLACEMENT_3D('',#152244,#109466,#109467);
#95879=AXIS2_PLACEMENT_3D('',#152245,#109468,#109469);
#95880=AXIS2_PLACEMENT_3D('',#152270,#109470,#109471);
#95881=AXIS2_PLACEMENT_3D('',#152271,#109472,#109473);
#95882=AXIS2_PLACEMENT_3D('',#152302,#109474,#109475);
#95883=AXIS2_PLACEMENT_3D('',#152303,#109476,#109477);
#95884=AXIS2_PLACEMENT_3D('',#152304,#109478,#109479);
#95885=AXIS2_PLACEMENT_3D('',#152305,#109480,#109481);
#95886=AXIS2_PLACEMENT_3D('',#152318,#109482,#109483);
#95887=AXIS2_PLACEMENT_3D('',#152350,#109484,#109485);
#95888=AXIS2_PLACEMENT_3D('',#152355,#109486,#109487);
#95889=AXIS2_PLACEMENT_3D('',#152375,#109489,#109490);
#95890=AXIS2_PLACEMENT_3D('',#152376,#109491,#109492);
#95891=AXIS2_PLACEMENT_3D('',#152377,#109493,#109494);
#95892=AXIS2_PLACEMENT_3D('',#152397,#109496,#109497);
#95893=AXIS2_PLACEMENT_3D('',#152398,#109498,#109499);
#95894=AXIS2_PLACEMENT_3D('',#152418,#109500,#109501);
#95895=AXIS2_PLACEMENT_3D('',#152425,#109502,#109503);
#95896=AXIS2_PLACEMENT_3D('',#152445,#109505,#109506);
#95897=AXIS2_PLACEMENT_3D('',#152446,#109507,#109508);
#95898=AXIS2_PLACEMENT_3D('',#152447,#109509,#109510);
#95899=AXIS2_PLACEMENT_3D('',#152467,#109512,#109513);
#95900=AXIS2_PLACEMENT_3D('',#152468,#109514,#109515);
#95901=AXIS2_PLACEMENT_3D('',#152469,#109516,#109517);
#95902=AXIS2_PLACEMENT_3D('',#152470,#109518,#109519);
#95903=AXIS2_PLACEMENT_3D('',#152471,#109520,#109521);
#95904=AXIS2_PLACEMENT_3D('',#152472,#109522,#109523);
#95905=AXIS2_PLACEMENT_3D('',#152473,#109524,#109525);
#95906=AXIS2_PLACEMENT_3D('',#152492,#109526,#109527);
#95907=AXIS2_PLACEMENT_3D('',#152493,#109528,#109529);
#95908=AXIS2_PLACEMENT_3D('',#152494,#109530,#109531);
#95909=AXIS2_PLACEMENT_3D('',#152514,#109533,#109534);
#95910=AXIS2_PLACEMENT_3D('',#152534,#109536,#109537);
#95911=AXIS2_PLACEMENT_3D('',#152535,#109538,#109539);
#95912=AXIS2_PLACEMENT_3D('',#152536,#109540,#109541);
#95913=AXIS2_PLACEMENT_3D('',#152556,#109543,#109544);
#95914=AXIS2_PLACEMENT_3D('',#152558,#109545,#109546);
#95915=AXIS2_PLACEMENT_3D('',#152638,#109548,#109549);
#95916=AXIS2_PLACEMENT_3D('',#152723,#109551,#109552);
#95917=AXIS2_PLACEMENT_3D('',#152724,#109553,#109554);
#95918=AXIS2_PLACEMENT_3D('',#152725,#109555,#109556);
#95919=AXIS2_PLACEMENT_3D('',#152726,#109557,#109558);
#95920=AXIS2_PLACEMENT_3D('',#152727,#109559,#109560);
#95921=AXIS2_PLACEMENT_3D('',#152728,#109561,#109562);
#95922=AXIS2_PLACEMENT_3D('',#152729,#109563,#109564);
#95923=AXIS2_PLACEMENT_3D('',#152730,#109565,#109566);
#95924=AXIS2_PLACEMENT_3D('',#152731,#109567,#109568);
#95925=AXIS2_PLACEMENT_3D('',#152733,#109570,#109571);
#95926=AXIS2_PLACEMENT_3D('',#152735,#109573,#109574);
#95927=AXIS2_PLACEMENT_3D('',#152737,#109576,#109577);
#95928=AXIS2_PLACEMENT_3D('',#152782,#109578,#109579);
#95929=AXIS2_PLACEMENT_3D('',#152783,#109580,#109581);
#95930=AXIS2_PLACEMENT_3D('',#152784,#109582,#109583);
#95931=AXIS2_PLACEMENT_3D('',#152787,#109586,#109587);
#95932=AXIS2_PLACEMENT_3D('',#152789,#109589,#109590);
#95933=AXIS2_PLACEMENT_3D('',#152790,#109591,#109592);
#95934=AXIS2_PLACEMENT_3D('',#152791,#109593,#109594);
#95935=AXIS2_PLACEMENT_3D('',#152832,#109595,#109596);
#95936=AXIS2_PLACEMENT_3D('',#152845,#109597,#109598);
#95937=AXIS2_PLACEMENT_3D('',#152903,#109599,#109600);
#95938=AXIS2_PLACEMENT_3D('',#152916,#109601,#109602);
#95939=AXIS2_PLACEMENT_3D('',#152960,#109603,#109604);
#95940=AXIS2_PLACEMENT_3D('',#152973,#109605,#109606);
#95941=AXIS2_PLACEMENT_3D('',#153025,#109607,#109608);
#95942=AXIS2_PLACEMENT_3D('',#153026,#109609,#109610);
#95943=AXIS2_PLACEMENT_3D('',#153028,#109612,#109613);
#95944=AXIS2_PLACEMENT_3D('',#153031,#109616,#109617);
#95945=AXIS2_PLACEMENT_3D('',#153032,#109618,#109619);
#95946=AXIS2_PLACEMENT_3D('',#153033,#109620,#109621);
#95947=AXIS2_PLACEMENT_3D('',#153078,#109622,#109623);
#95948=AXIS2_PLACEMENT_3D('',#153079,#109624,#109625);
#95949=AXIS2_PLACEMENT_3D('',#153081,#109627,#109628);
#95950=AXIS2_PLACEMENT_3D('',#153102,#109629,#109630);
#95951=AXIS2_PLACEMENT_3D('',#153103,#109631,#109632);
#95952=AXIS2_PLACEMENT_3D('',#153105,#109634,#109635);
#95953=AXIS2_PLACEMENT_3D('',#153107,#109637,#109638);
#95954=AXIS2_PLACEMENT_3D('',#153108,#109639,#109640);
#95955=AXIS2_PLACEMENT_3D('',#153126,#109641,#109642);
#95956=AXIS2_PLACEMENT_3D('',#153143,#109643,#109644);
#95957=AXIS2_PLACEMENT_3D('',#153144,#109645,#109646);
#95958=AXIS2_PLACEMENT_3D('',#153145,#109647,#109648);
#95959=AXIS2_PLACEMENT_3D('',#153146,#109649,#109650);
#95960=AXIS2_PLACEMENT_3D('',#153147,#109651,#109652);
#95961=AXIS2_PLACEMENT_3D('',#153157,#109653,#109654);
#95962=AXIS2_PLACEMENT_3D('',#153178,#109655,#109656);
#95963=AXIS2_PLACEMENT_3D('',#153195,#109657,#109658);
#95964=AXIS2_PLACEMENT_3D('',#153196,#109659,#109660);
#95965=AXIS2_PLACEMENT_3D('',#153198,#109662,#109663);
#95966=AXIS2_PLACEMENT_3D('',#153200,#109665,#109666);
#95967=AXIS2_PLACEMENT_3D('',#153201,#109667,#109668);
#95968=AXIS2_PLACEMENT_3D('',#153202,#109669,#109670);
#95969=AXIS2_PLACEMENT_3D('',#153203,#109671,#109672);
#95970=AXIS2_PLACEMENT_3D('',#153208,#109673,#109674);
#95971=AXIS2_PLACEMENT_3D('',#153210,#109676,#109677);
#95972=AXIS2_PLACEMENT_3D('',#153212,#109679,#109680);
#95973=AXIS2_PLACEMENT_3D('',#153229,#109681,#109682);
#95974=AXIS2_PLACEMENT_3D('',#153250,#109683,#109684);
#95975=AXIS2_PLACEMENT_3D('',#153251,#109685,#109686);
#95976=AXIS2_PLACEMENT_3D('',#153252,#109687,#109688);
#95977=AXIS2_PLACEMENT_3D('',#153253,#109689,#109690);
#95978=AXIS2_PLACEMENT_3D('',#153254,#109691,#109692);
#95979=AXIS2_PLACEMENT_3D('',#153255,#109693,#109694);
#95980=AXIS2_PLACEMENT_3D('',#153256,#109695,#109696);
#95981=AXIS2_PLACEMENT_3D('',#153257,#109697,#109698);
#95982=AXIS2_PLACEMENT_3D('',#153258,#109699,#109700);
#95983=AXIS2_PLACEMENT_3D('',#153297,#109701,#109702);
#95984=AXIS2_PLACEMENT_3D('',#153329,#109703,#109704);
#95985=AXIS2_PLACEMENT_3D('',#153330,#109705,#109706);
#95986=AXIS2_PLACEMENT_3D('',#153332,#109708,#109709);
#95987=AXIS2_PLACEMENT_3D('',#153334,#109711,#109712);
#95988=AXIS2_PLACEMENT_3D('',#153366,#109713,#109714);
#95989=AXIS2_PLACEMENT_3D('',#153405,#109715,#109716);
#95990=AXIS2_PLACEMENT_3D('',#153406,#109717,#109718);
#95991=AXIS2_PLACEMENT_3D('',#153407,#109719,#109720);
#95992=AXIS2_PLACEMENT_3D('',#153408,#109721,#109722);
#95993=AXIS2_PLACEMENT_3D('',#153409,#109723,#109724);
#95994=AXIS2_PLACEMENT_3D('',#153411,#109726,#109727);
#95995=AXIS2_PLACEMENT_3D('',#153413,#109729,#109730);
#95996=AXIS2_PLACEMENT_3D('',#153414,#109731,#109732);
#95997=AXIS2_PLACEMENT_3D('',#153415,#109733,#109734);
#95998=AXIS2_PLACEMENT_3D('',#153416,#109735,#109736);
#95999=AXIS2_PLACEMENT_3D('',#153417,#109737,#109738);
#96000=AXIS2_PLACEMENT_3D('',#153418,#109739,#109740);
#96001=AXIS2_PLACEMENT_3D('',#153439,#109741,#109742);
#96002=AXIS2_PLACEMENT_3D('',#153460,#109743,#109744);
#96003=AXIS2_PLACEMENT_3D('',#153461,#109745,#109746);
#96004=AXIS2_PLACEMENT_3D('',#153463,#109748,#109749);
#96005=AXIS2_PLACEMENT_3D('',#153465,#109751,#109752);
#96006=AXIS2_PLACEMENT_3D('',#153466,#109753,#109754);
#96007=AXIS2_PLACEMENT_3D('',#153467,#109755,#109756);
#96008=AXIS2_PLACEMENT_3D('',#153470,#109757,#109758);
#96009=AXIS2_PLACEMENT_3D('',#153474,#109761,#109762);
#96010=AXIS2_PLACEMENT_3D('',#153483,#109767,#109768);
#96011=AXIS2_PLACEMENT_3D('',#153485,#109769,#109770);
#96012=AXIS2_PLACEMENT_3D('',#153488,#109772,#109773);
#96013=AXIS2_PLACEMENT_3D('',#153489,#109774,#109775);
#96014=AXIS2_PLACEMENT_3D('',#153495,#109779,#109780);
#96015=AXIS2_PLACEMENT_3D('',#153532,#109781,#109782);
#96016=AXIS2_PLACEMENT_3D('',#153791,#109783,#109784);
#96017=AXIS2_PLACEMENT_3D('',#154066,#109787,#109788);
#96018=AXIS2_PLACEMENT_3D('',#154069,#109789,#109790);
#96019=AXIS2_PLACEMENT_3D('',#154090,#109791,#109792);
#96020=AXIS2_PLACEMENT_3D('',#154093,#109793,#109794);
#96021=AXIS2_PLACEMENT_3D('',#154228,#109795,#109796);
#96022=AXIS2_PLACEMENT_3D('',#154234,#109800,#109801);
#96023=AXIS2_PLACEMENT_3D('',#154243,#109806,#109807);
#96024=AXIS2_PLACEMENT_3D('',#154245,#109808,#109809);
#96025=AXIS2_PLACEMENT_3D('',#154248,#109811,#109812);
#96026=AXIS2_PLACEMENT_3D('',#154249,#109813,#109814);
#96027=AXIS2_PLACEMENT_3D('',#154255,#109818,#109819);
#96028=AXIS2_PLACEMENT_3D('',#154272,#109820,#109821);
#96029=AXIS2_PLACEMENT_3D('',#154274,#109822,#109823);
#96030=AXIS2_PLACEMENT_3D('',#154368,#109824,#109825);
#96031=AXIS2_PLACEMENT_3D('',#154601,#109826,#109827);
#96032=AXIS2_PLACEMENT_3D('',#154807,#109830,#109831);
#96033=AXIS2_PLACEMENT_3D('',#154816,#109836,#109837);
#96034=AXIS2_PLACEMENT_3D('',#154818,#109838,#109839);
#96035=AXIS2_PLACEMENT_3D('',#154821,#109841,#109842);
#96036=AXIS2_PLACEMENT_3D('',#154822,#109843,#109844);
#96037=AXIS2_PLACEMENT_3D('',#154828,#109848,#109849);
#96038=AXIS2_PLACEMENT_3D('',#154834,#109852,#109853);
#96039=AXIS2_PLACEMENT_3D('',#154981,#109854,#109855);
#96040=AXIS2_PLACEMENT_3D('',#155238,#109858,#109859);
#96041=AXIS2_PLACEMENT_3D('',#155241,#109860,#109861);
#96042=AXIS2_PLACEMENT_3D('',#155289,#109862,#109863);
#96043=AXIS2_PLACEMENT_3D('',#155307,#109864,#109865);
#96044=AXIS2_PLACEMENT_3D('',#155368,#109866,#109867);
#96045=AXIS2_PLACEMENT_3D('',#155375,#109870,#109871);
#96046=AXIS2_PLACEMENT_3D('',#155377,#109873,#109874);
#96047=AXIS2_PLACEMENT_3D('',#155450,#109875,#109876);
#96048=AXIS2_PLACEMENT_3D('',#155518,#109877,#109878);
#96049=AXIS2_PLACEMENT_3D('',#155808,#109879,#109880);
#96050=AXIS2_PLACEMENT_3D('',#156125,#109883,#109884);
#96051=AXIS2_PLACEMENT_3D('',#156134,#109889,#109890);
#96052=AXIS2_PLACEMENT_3D('',#156138,#109892,#109893);
#96053=AXIS2_PLACEMENT_3D('',#156139,#109894,#109895);
#96054=AXIS2_PLACEMENT_3D('',#156140,#109896,#109897);
#96055=AXIS2_PLACEMENT_3D('',#156146,#109901,#109902);
#96056=AXIS2_PLACEMENT_3D('',#156153,#109903,#109904);
#96057=AXIS2_PLACEMENT_3D('',#156170,#109905,#109906);
#96058=AXIS2_PLACEMENT_3D('',#156204,#109907,#109908);
#96059=AXIS2_PLACEMENT_3D('',#156209,#109909,#109910);
#96060=AXIS2_PLACEMENT_3D('',#156236,#109911,#109912);
#96061=AXIS2_PLACEMENT_3D('',#156237,#109913,#109914);
#96062=AXIS2_PLACEMENT_3D('',#156246,#109919,#109920);
#96063=AXIS2_PLACEMENT_3D('',#156248,#109921,#109922);
#96064=AXIS2_PLACEMENT_3D('',#156251,#109924,#109925);
#96065=AXIS2_PLACEMENT_3D('',#156252,#109926,#109927);
#96066=AXIS2_PLACEMENT_3D('',#156258,#109931,#109932);
#96067=AXIS2_PLACEMENT_3D('',#156264,#109935,#109936);
#96068=AXIS2_PLACEMENT_3D('',#156420,#109937,#109938);
#96069=AXIS2_PLACEMENT_3D('',#156656,#109941,#109942);
#96070=AXIS2_PLACEMENT_3D('',#156659,#109943,#109944);
#96071=AXIS2_PLACEMENT_3D('',#156700,#109945,#109946);
#96072=AXIS2_PLACEMENT_3D('',#156702,#109947,#109948);
#96073=AXIS2_PLACEMENT_3D('',#156704,#109949,#109950);
#96074=AXIS2_PLACEMENT_3D('',#156705,#109951,#109952);
#96075=AXIS2_PLACEMENT_3D('',#156706,#109953,#109954);
#96076=AXIS2_PLACEMENT_3D('',#156713,#109957,#109958);
#96077=AXIS2_PLACEMENT_3D('',#156715,#109960,#109961);
#96078=AXIS2_PLACEMENT_3D('',#156717,#109962,#109963);
#96079=AXIS2_PLACEMENT_3D('',#156718,#109964,#109965);
#96080=AXIS2_PLACEMENT_3D('',#156851,#109966,#109967);
#96081=AXIS2_PLACEMENT_3D('',#157088,#109968,#109969);
#96082=AXIS2_PLACEMENT_3D('',#157097,#109972,#109973);
#96083=AXIS2_PLACEMENT_3D('',#157106,#109978,#109979);
#96084=AXIS2_PLACEMENT_3D('',#157110,#109981,#109982);
#96085=AXIS2_PLACEMENT_3D('',#157111,#109983,#109984);
#96086=AXIS2_PLACEMENT_3D('',#157112,#109985,#109986);
#96087=AXIS2_PLACEMENT_3D('',#157118,#109990,#109991);
#96088=AXIS2_PLACEMENT_3D('',#157121,#109992,#109993);
#96089=AXIS2_PLACEMENT_3D('',#157341,#109994,#109995);
#96090=AXIS2_PLACEMENT_3D('',#157346,#109997,#109998);
#96091=AXIS2_PLACEMENT_3D('',#157349,#110000,#110001);
#96092=AXIS2_PLACEMENT_3D('',#157350,#110002,#110003);
#96093=AXIS2_PLACEMENT_3D('',#157354,#110005,#110006);
#96094=AXIS2_PLACEMENT_3D('',#157356,#110008,#110009);
#96095=AXIS2_PLACEMENT_3D('',#157569,#110012,#110013);
#96096=AXIS2_PLACEMENT_3D('',#157572,#110014,#110015);
#96097=AXIS2_PLACEMENT_3D('',#157644,#110016,#110017);
#96098=AXIS2_PLACEMENT_3D('',#157649,#110019,#110020);
#96099=AXIS2_PLACEMENT_3D('',#157653,#110023,#110024);
#96100=AXIS2_PLACEMENT_3D('',#157662,#110029,#110030);
#96101=AXIS2_PLACEMENT_3D('',#157663,#110031,#110032);
#96102=AXIS2_PLACEMENT_3D('',#157664,#110033,#110034);
#96103=AXIS2_PLACEMENT_3D('',#157665,#110035,#110036);
#96104=AXIS2_PLACEMENT_3D('',#157667,#110037,#110038);
#96105=AXIS2_PLACEMENT_3D('',#157699,#110039,#110040);
#96106=AXIS2_PLACEMENT_3D('',#157935,#110043,#110044);
#96107=AXIS2_PLACEMENT_3D('',#157938,#110045,#110046);
#96108=AXIS2_PLACEMENT_3D('',#158125,#110047,#110048);
#96109=AXIS2_PLACEMENT_3D('',#158231,#110049,#110050);
#96110=AXIS2_PLACEMENT_3D('',#158391,#110053,#110054);
#96111=AXIS2_PLACEMENT_3D('',#158392,#110055,#110056);
#96112=AXIS2_PLACEMENT_3D('',#158395,#110057,#110058);
#96113=AXIS2_PLACEMENT_3D('',#158497,#110059,#110060);
#96114=AXIS2_PLACEMENT_3D('',#158539,#110061,#110062);
#96115=AXIS2_PLACEMENT_3D('',#158540,#110063,#110064);
#96116=AXIS2_PLACEMENT_3D('',#158663,#110067,#110068);
#96117=AXIS2_PLACEMENT_3D('',#158725,#110069,#110070);
#96118=AXIS2_PLACEMENT_3D('',#158728,#110071,#110072);
#96119=AXIS2_PLACEMENT_3D('',#158818,#110073,#110074);
#96120=AXIS2_PLACEMENT_3D('',#158954,#110075,#110076);
#96121=AXIS2_PLACEMENT_3D('',#159211,#110079,#110080);
#96122=AXIS2_PLACEMENT_3D('',#159214,#110081,#110082);
#96123=AXIS2_PLACEMENT_3D('',#159247,#110083,#110084);
#96124=AXIS2_PLACEMENT_3D('',#159266,#110086,#110087);
#96125=AXIS2_PLACEMENT_3D('',#159267,#110088,#110089);
#96126=AXIS2_PLACEMENT_3D('',#159276,#110094,#110095);
#96127=AXIS2_PLACEMENT_3D('',#159278,#110096,#110097);
#96128=AXIS2_PLACEMENT_3D('',#159280,#110099,#110100);
#96129=AXIS2_PLACEMENT_3D('',#159281,#110101,#110102);
#96130=AXIS2_PLACEMENT_3D('',#159284,#110104,#110105);
#96131=AXIS2_PLACEMENT_3D('',#159285,#110106,#110107);
#96132=AXIS2_PLACEMENT_3D('',#159290,#110109,#110110);
#96133=AXIS2_PLACEMENT_3D('',#159293,#110112,#110113);
#96134=AXIS2_PLACEMENT_3D('',#159294,#110114,#110115);
#96135=AXIS2_PLACEMENT_3D('',#159500,#110118,#110119);
#96136=AXIS2_PLACEMENT_3D('',#159503,#110120,#110121);
#96137=AXIS2_PLACEMENT_3D('',#159551,#110122,#110123);
#96138=AXIS2_PLACEMENT_3D('',#159555,#110125,#110126);
#96139=AXIS2_PLACEMENT_3D('',#159557,#110128,#110129);
#96140=AXIS2_PLACEMENT_3D('',#159563,#110133,#110134);
#96141=AXIS2_PLACEMENT_3D('',#159569,#110138,#110139);
#96142=AXIS2_PLACEMENT_3D('',#159611,#110142,#110143);
#96143=AXIS2_PLACEMENT_3D('',#159620,#110148,#110149);
#96144=AXIS2_PLACEMENT_3D('',#159659,#110152,#110153);
#96145=AXIS2_PLACEMENT_3D('',#159716,#110156,#110157);
#96146=AXIS2_PLACEMENT_3D('',#159721,#110159,#110160);
#96147=AXIS2_PLACEMENT_3D('',#159724,#110162,#110163);
#96148=AXIS2_PLACEMENT_3D('',#159725,#110164,#110165);
#96149=AXIS2_PLACEMENT_3D('',#159743,#110166,#110167);
#96150=AXIS2_PLACEMENT_3D('',#159909,#110168,#110169);
#96151=AXIS2_PLACEMENT_3D('',#160101,#110170,#110171);
#96152=AXIS2_PLACEMENT_3D('',#160103,#110172,#110173);
#96153=AXIS2_PLACEMENT_3D('',#160106,#110175,#110176);
#96154=AXIS2_PLACEMENT_3D('',#160366,#110177,#110178);
#96155=AXIS2_PLACEMENT_3D('',#160368,#110179,#110180);
#96156=AXIS2_PLACEMENT_3D('',#160370,#110181,#110182);
#96157=AXIS2_PLACEMENT_3D('',#160371,#110183,#110184);
#96158=AXIS2_PLACEMENT_3D('',#160397,#110185,#110186);
#96159=AXIS2_PLACEMENT_3D('',#160399,#110187,#110188);
#96160=AXIS2_PLACEMENT_3D('',#160413,#110189,#110190);
#96161=AXIS2_PLACEMENT_3D('',#160508,#110192,#110193);
#96162=AXIS2_PLACEMENT_3D('',#160566,#110194,#110195);
#96163=AXIS2_PLACEMENT_3D('',#160574,#110196,#110197);
#96164=AXIS2_PLACEMENT_3D('',#160577,#110199,#110200);
#96165=AXIS2_PLACEMENT_3D('',#160605,#110201,#110202);
#96166=AXIS2_PLACEMENT_3D('',#160652,#110203,#110204);
#96167=AXIS2_PLACEMENT_3D('',#160819,#110206,#110207);
#96168=AXIS2_PLACEMENT_3D('',#160828,#110208,#110209);
#96169=AXIS2_PLACEMENT_3D('',#160884,#110210,#110211);
#96170=AXIS2_PLACEMENT_3D('',#160887,#110213,#110214);
#96171=AXIS2_PLACEMENT_3D('',#160915,#110215,#110216);
#96172=AXIS2_PLACEMENT_3D('',#160962,#110217,#110218);
#96173=AXIS2_PLACEMENT_3D('',#161039,#110221,#110222);
#96174=AXIS2_PLACEMENT_3D('',#161040,#110223,#110224);
#96175=AXIS2_PLACEMENT_3D('',#161042,#110225,#110226);
#96176=AXIS2_PLACEMENT_3D('',#161044,#110227,#110228);
#96177=AXIS2_PLACEMENT_3D('',#161045,#110229,#110230);
#96178=AXIS2_PLACEMENT_3D('',#161046,#110231,#110232);
#96179=AXIS2_PLACEMENT_3D('',#161048,#110233,#110234);
#96180=AXIS2_PLACEMENT_3D('',#161050,#110235,#110236);
#96181=AXIS2_PLACEMENT_3D('',#161051,#110237,#110238);
#96182=AXIS2_PLACEMENT_3D('',#161052,#110239,#110240);
#96183=AXIS2_PLACEMENT_3D('',#161054,#110241,#110242);
#96184=AXIS2_PLACEMENT_3D('',#161056,#110243,#110244);
#96185=AXIS2_PLACEMENT_3D('',#161057,#110245,#110246);
#96186=AXIS2_PLACEMENT_3D('',#161077,#110247,#110248);
#96187=AXIS2_PLACEMENT_3D('',#161129,#110249,#110250);
#96188=AXIS2_PLACEMENT_3D('',#161137,#110251,#110252);
#96189=AXIS2_PLACEMENT_3D('',#161140,#110254,#110255);
#96190=AXIS2_PLACEMENT_3D('',#161168,#110256,#110257);
#96191=AXIS2_PLACEMENT_3D('',#161221,#110258,#110259);
#96192=AXIS2_PLACEMENT_3D('',#161301,#110261,#110262);
#96193=AXIS2_PLACEMENT_3D('',#161334,#110263,#110264);
#96194=AXIS2_PLACEMENT_3D('',#161335,#110265,#110266);
#96195=AXIS2_PLACEMENT_3D('',#161430,#110269,#110270);
#96196=AXIS2_PLACEMENT_3D('',#161439,#110271,#110272);
#96197=AXIS2_PLACEMENT_3D('',#161489,#110273,#110274);
#96198=AXIS2_PLACEMENT_3D('',#161492,#110276,#110277);
#96199=AXIS2_PLACEMENT_3D('',#161520,#110278,#110279);
#96200=AXIS2_PLACEMENT_3D('',#161573,#110280,#110281);
#96201=AXIS2_PLACEMENT_3D('',#161827,#110283,#110284);
#96202=AXIS2_PLACEMENT_3D('',#161844,#110285,#110286);
#96203=AXIS2_PLACEMENT_3D('',#161886,#110287,#110288);
#96204=AXIS2_PLACEMENT_3D('',#161887,#110289,#110290);
#96205=AXIS2_PLACEMENT_3D('',#161888,#110291,#110292);
#96206=AXIS2_PLACEMENT_3D('',#161889,#110293,#110294);
#96207=AXIS2_PLACEMENT_3D('',#161891,#110295,#110296);
#96208=AXIS2_PLACEMENT_3D('',#161892,#110297,#110298);
#96209=AXIS2_PLACEMENT_3D('',#161925,#110299,#110300);
#96210=AXIS2_PLACEMENT_3D('',#162033,#110301,#110302);
#96211=AXIS2_PLACEMENT_3D('',#162036,#110303,#110304);
#96212=AXIS2_PLACEMENT_3D('',#162037,#110305,#110306);
#96213=AXIS2_PLACEMENT_3D('',#162038,#110307,#110308);
#96214=AXIS2_PLACEMENT_3D('',#162064,#110309,#110310);
#96215=AXIS2_PLACEMENT_3D('',#162140,#110311,#110312);
#96216=AXIS2_PLACEMENT_3D('',#162151,#110313,#110314);
#96217=AXIS2_PLACEMENT_3D('',#162153,#110315,#110316);
#96218=AXIS2_PLACEMENT_3D('',#162154,#110317,#110318);
#96219=AXIS2_PLACEMENT_3D('',#162174,#110319,#110320);
#96220=AXIS2_PLACEMENT_3D('',#162220,#110321,#110322);
#96221=AXIS2_PLACEMENT_3D('',#162231,#110323,#110324);
#96222=AXIS2_PLACEMENT_3D('',#162232,#110325,#110326);
#96223=AXIS2_PLACEMENT_3D('',#162235,#110327,#110328);
#96224=AXIS2_PLACEMENT_3D('',#162236,#110329,#110330);
#96225=AXIS2_PLACEMENT_3D('',#162237,#110331,#110332);
#96226=AXIS2_PLACEMENT_3D('',#162269,#110333,#110334);
#96227=AXIS2_PLACEMENT_3D('',#162336,#110335,#110336);
#96228=AXIS2_PLACEMENT_3D('',#162393,#110337,#110338);
#96229=AXIS2_PLACEMENT_3D('',#162394,#110339,#110340);
#96230=AXIS2_PLACEMENT_3D('',#162503,#110341,#110342);
#96231=AXIS2_PLACEMENT_3D('',#162519,#110343,#110344);
#96232=AXIS2_PLACEMENT_3D('',#162522,#110345,#110346);
#96233=AXIS2_PLACEMENT_3D('',#162523,#110347,#110348);
#96234=AXIS2_PLACEMENT_3D('',#162524,#110349,#110350);
#96235=AXIS2_PLACEMENT_3D('',#162550,#110351,#110352);
#96236=AXIS2_PLACEMENT_3D('',#162629,#110353,#110354);
#96237=AXIS2_PLACEMENT_3D('',#162660,#110355,#110356);
#96238=AXIS2_PLACEMENT_3D('',#162661,#110357,#110358);
#96239=AXIS2_PLACEMENT_3D('',#162740,#110359,#110360);
#96240=AXIS2_PLACEMENT_3D('',#162829,#110361,#110362);
#96241=AXIS2_PLACEMENT_3D('',#162832,#110363,#110364);
#96242=AXIS2_PLACEMENT_3D('',#162833,#110365,#110366);
#96243=AXIS2_PLACEMENT_3D('',#162834,#110367,#110368);
#96244=AXIS2_PLACEMENT_3D('',#162866,#110369,#110370);
#96245=AXIS2_PLACEMENT_3D('',#162939,#110371,#110372);
#96246=AXIS2_PLACEMENT_3D('',#163002,#110373,#110374);
#96247=AXIS2_PLACEMENT_3D('',#163003,#110375,#110376);
#96248=AXIS2_PLACEMENT_3D('',#163052,#110377,#110378);
#96249=AXIS2_PLACEMENT_3D('',#163102,#110379,#110380);
#96250=AXIS2_PLACEMENT_3D('',#163105,#110381,#110382);
#96251=AXIS2_PLACEMENT_3D('',#163106,#110383,#110384);
#96252=AXIS2_PLACEMENT_3D('',#163107,#110385,#110386);
#96253=AXIS2_PLACEMENT_3D('',#163121,#110387,#110388);
#96254=AXIS2_PLACEMENT_3D('',#163130,#110389,#110390);
#96255=AXIS2_PLACEMENT_3D('',#163181,#110391,#110392);
#96256=AXIS2_PLACEMENT_3D('',#163210,#110393,#110394);
#96257=AXIS2_PLACEMENT_3D('',#163212,#110395,#110396);
#96258=AXIS2_PLACEMENT_3D('',#163213,#110397,#110398);
#96259=AXIS2_PLACEMENT_3D('',#163246,#110399,#110400);
#96260=AXIS2_PLACEMENT_3D('',#163309,#110401,#110402);
#96261=AXIS2_PLACEMENT_3D('',#163312,#110403,#110404);
#96262=AXIS2_PLACEMENT_3D('',#163313,#110405,#110406);
#96263=AXIS2_PLACEMENT_3D('',#163314,#110407,#110408);
#96264=AXIS2_PLACEMENT_3D('',#163347,#110409,#110410);
#96265=AXIS2_PLACEMENT_3D('',#163392,#110411,#110412);
#96266=AXIS2_PLACEMENT_3D('',#163463,#110413,#110414);
#96267=AXIS2_PLACEMENT_3D('',#163465,#110415,#110416);
#96268=AXIS2_PLACEMENT_3D('',#163466,#110417,#110418);
#96269=AXIS2_PLACEMENT_3D('',#163488,#110419,#110420);
#96270=AXIS2_PLACEMENT_3D('',#163611,#110421,#110422);
#96271=AXIS2_PLACEMENT_3D('',#163632,#110423,#110424);
#96272=AXIS2_PLACEMENT_3D('',#163670,#110425,#110426);
#96273=AXIS2_PLACEMENT_3D('',#163684,#110427,#110428);
#96274=AXIS2_PLACEMENT_3D('',#163779,#110430,#110431);
#96275=AXIS2_PLACEMENT_3D('',#163837,#110432,#110433);
#96276=AXIS2_PLACEMENT_3D('',#163845,#110434,#110435);
#96277=AXIS2_PLACEMENT_3D('',#163848,#110437,#110438);
#96278=AXIS2_PLACEMENT_3D('',#163876,#110439,#110440);
#96279=AXIS2_PLACEMENT_3D('',#163923,#110441,#110442);
#96280=AXIS2_PLACEMENT_3D('',#164090,#110444,#110445);
#96281=AXIS2_PLACEMENT_3D('',#164099,#110446,#110447);
#96282=AXIS2_PLACEMENT_3D('',#164155,#110448,#110449);
#96283=AXIS2_PLACEMENT_3D('',#164158,#110451,#110452);
#96284=AXIS2_PLACEMENT_3D('',#164186,#110453,#110454);
#96285=AXIS2_PLACEMENT_3D('',#164233,#110455,#110456);
#96286=AXIS2_PLACEMENT_3D('',#164310,#110459,#110460);
#96287=AXIS2_PLACEMENT_3D('',#164311,#110461,#110462);
#96288=AXIS2_PLACEMENT_3D('',#164313,#110463,#110464);
#96289=AXIS2_PLACEMENT_3D('',#164315,#110465,#110466);
#96290=AXIS2_PLACEMENT_3D('',#164316,#110467,#110468);
#96291=AXIS2_PLACEMENT_3D('',#164317,#110469,#110470);
#96292=AXIS2_PLACEMENT_3D('',#164319,#110471,#110472);
#96293=AXIS2_PLACEMENT_3D('',#164321,#110473,#110474);
#96294=AXIS2_PLACEMENT_3D('',#164322,#110475,#110476);
#96295=AXIS2_PLACEMENT_3D('',#164323,#110477,#110478);
#96296=AXIS2_PLACEMENT_3D('',#164325,#110479,#110480);
#96297=AXIS2_PLACEMENT_3D('',#164327,#110481,#110482);
#96298=AXIS2_PLACEMENT_3D('',#164328,#110483,#110484);
#96299=AXIS2_PLACEMENT_3D('',#164329,#110485,#110486);
#96300=AXIS2_PLACEMENT_3D('',#164404,#110489,#110490);
#96301=AXIS2_PLACEMENT_3D('',#164407,#110491,#110492);
#96302=AXIS2_PLACEMENT_3D('',#164409,#110493,#110494);
#96303=AXIS2_PLACEMENT_3D('',#164410,#110495,#110496);
#96304=AXIS2_PLACEMENT_3D('',#164889,#110497,#110498);
#96305=AXIS2_PLACEMENT_3D('',#164895,#110502,#110503);
#96306=AXIS2_PLACEMENT_3D('',#164942,#110506,#110507);
#96307=AXIS2_PLACEMENT_3D('',#164943,#110508,#110509);
#96308=AXIS2_PLACEMENT_3D('',#164946,#110510,#110511);
#96309=AXIS2_PLACEMENT_3D('',#164949,#110514,#110515);
#96310=AXIS2_PLACEMENT_3D('',#164951,#110516,#110517);
#96311=AXIS2_PLACEMENT_3D('',#164953,#110518,#110519);
#96312=AXIS2_PLACEMENT_3D('',#164954,#110520,#110521);
#96313=AXIS2_PLACEMENT_3D('',#164955,#110522,#110523);
#96314=AXIS2_PLACEMENT_3D('',#164958,#110525,#110526);
#96315=AXIS2_PLACEMENT_3D('',#164972,#110527,#110528);
#96316=AXIS2_PLACEMENT_3D('',#164991,#110529,#110530);
#96317=AXIS2_PLACEMENT_3D('',#165021,#110531,#110532);
#96318=AXIS2_PLACEMENT_3D('',#165050,#110533,#110534);
#96319=AXIS2_PLACEMENT_3D('',#165052,#110535,#110536);
#96320=AXIS2_PLACEMENT_3D('',#165079,#110538,#110539);
#96321=AXIS2_PLACEMENT_3D('',#165109,#110540,#110541);
#96322=AXIS2_PLACEMENT_3D('',#165139,#110542,#110543);
#96323=AXIS2_PLACEMENT_3D('',#165153,#110544,#110545);
#96324=AXIS2_PLACEMENT_3D('',#165155,#110546,#110547);
#96325=AXIS2_PLACEMENT_3D('',#165189,#110549,#110550);
#96326=AXIS2_PLACEMENT_3D('',#165190,#110551,#110552);
#96327=AXIS2_PLACEMENT_3D('',#165201,#110553,#110554);
#96328=AXIS2_PLACEMENT_3D('',#165204,#110557,#110558);
#96329=AXIS2_PLACEMENT_3D('',#165206,#110560,#110561);
#96330=AXIS2_PLACEMENT_3D('',#165209,#110562,#110563);
#96331=AXIS2_PLACEMENT_3D('',#165213,#110565,#110566);
#96332=AXIS2_PLACEMENT_3D('',#165215,#110568,#110569);
#96333=AXIS2_PLACEMENT_3D('',#165217,#110570,#110571);
#96334=AXIS2_PLACEMENT_3D('',#165219,#110572,#110573);
#96335=AXIS2_PLACEMENT_3D('',#165220,#110574,#110575);
#96336=AXIS2_PLACEMENT_3D('',#165221,#110576,#110577);
#96337=AXIS2_PLACEMENT_3D('',#165224,#110579,#110580);
#96338=AXIS2_PLACEMENT_3D('',#165225,#110581,#110582);
#96339=AXIS2_PLACEMENT_3D('',#165227,#110583,#110584);
#96340=AXIS2_PLACEMENT_3D('',#165229,#110585,#110586);
#96341=AXIS2_PLACEMENT_3D('',#165230,#110587,#110588);
#96342=AXIS2_PLACEMENT_3D('',#165231,#110589,#110590);
#96343=AXIS2_PLACEMENT_3D('',#165234,#110592,#110593);
#96344=AXIS2_PLACEMENT_3D('',#165235,#110594,#110595);
#96345=AXIS2_PLACEMENT_3D('',#165237,#110596,#110597);
#96346=AXIS2_PLACEMENT_3D('',#165238,#110598,#110599);
#96347=AXIS2_PLACEMENT_3D('',#165239,#110600,#110601);
#96348=AXIS2_PLACEMENT_3D('',#165241,#110603,#110604);
#96349=AXIS2_PLACEMENT_3D('',#165244,#110606,#110607);
#96350=AXIS2_PLACEMENT_3D('',#165287,#110609,#110610);
#96351=AXIS2_PLACEMENT_3D('',#165288,#110611,#110612);
#96352=AXIS2_PLACEMENT_3D('',#165291,#110614,#110615);
#96353=AXIS2_PLACEMENT_3D('',#165333,#110616,#110617);
#96354=AXIS2_PLACEMENT_3D('',#165351,#110618,#110619);
#96355=AXIS2_PLACEMENT_3D('',#165396,#110620,#110621);
#96356=AXIS2_PLACEMENT_3D('',#165397,#110622,#110623);
#96357=AXIS2_PLACEMENT_3D('',#165400,#110625,#110626);
#96358=AXIS2_PLACEMENT_3D('',#165442,#110627,#110628);
#96359=AXIS2_PLACEMENT_3D('',#165460,#110629,#110630);
#96360=AXIS2_PLACEMENT_3D('',#165497,#110631,#110632);
#96361=AXIS2_PLACEMENT_3D('',#165574,#110633,#110634);
#96362=AXIS2_PLACEMENT_3D('',#165578,#110636,#110637);
#96363=AXIS2_PLACEMENT_3D('',#165580,#110639,#110640);
#96364=AXIS2_PLACEMENT_3D('',#165582,#110641,#110642);
#96365=AXIS2_PLACEMENT_3D('',#165653,#110643,#110644);
#96366=AXIS2_PLACEMENT_3D('',#165655,#110645,#110646);
#96367=AXIS2_PLACEMENT_3D('',#165657,#110647,#110648);
#96368=AXIS2_PLACEMENT_3D('',#165658,#110649,#110650);
#96369=AXIS2_PLACEMENT_3D('',#165659,#110651,#110652);
#96370=AXIS2_PLACEMENT_3D('',#165662,#110654,#110655);
#96371=AXIS2_PLACEMENT_3D('',#165663,#110656,#110657);
#96372=AXIS2_PLACEMENT_3D('',#165666,#110658,#110659);
#96373=AXIS2_PLACEMENT_3D('',#165669,#110661,#110662);
#96374=AXIS2_PLACEMENT_3D('',#165715,#110664,#110665);
#96375=AXIS2_PLACEMENT_3D('',#165733,#110666,#110667);
#96376=AXIS2_PLACEMENT_3D('',#165790,#110668,#110669);
#96377=AXIS2_PLACEMENT_3D('',#165791,#110670,#110671);
#96378=AXIS2_PLACEMENT_3D('',#165794,#110673,#110674);
#96379=AXIS2_PLACEMENT_3D('',#165826,#110675,#110676);
#96380=AXIS2_PLACEMENT_3D('',#165856,#110677,#110678);
#96381=AXIS2_PLACEMENT_3D('',#165892,#110679,#110680);
#96382=AXIS2_PLACEMENT_3D('',#165906,#110681,#110682);
#96383=AXIS2_PLACEMENT_3D('',#165908,#110683,#110684);
#96384=AXIS2_PLACEMENT_3D('',#165942,#110686,#110687);
#96385=AXIS2_PLACEMENT_3D('',#165943,#110688,#110689);
#96386=AXIS2_PLACEMENT_3D('',#165954,#110690,#110691);
#96387=AXIS2_PLACEMENT_3D('',#165957,#110694,#110695);
#96388=AXIS2_PLACEMENT_3D('',#165959,#110697,#110698);
#96389=AXIS2_PLACEMENT_3D('',#165961,#110699,#110700);
#96390=AXIS2_PLACEMENT_3D('',#165963,#110701,#110702);
#96391=AXIS2_PLACEMENT_3D('',#165964,#110703,#110704);
#96392=AXIS2_PLACEMENT_3D('',#165965,#110705,#110706);
#96393=AXIS2_PLACEMENT_3D('',#165968,#110708,#110709);
#96394=AXIS2_PLACEMENT_3D('',#165969,#110710,#110711);
#96395=AXIS2_PLACEMENT_3D('',#165972,#110712,#110713);
#96396=AXIS2_PLACEMENT_3D('',#165975,#110715,#110716);
#96397=AXIS2_PLACEMENT_3D('',#165977,#110718,#110719);
#96398=AXIS2_PLACEMENT_3D('',#165981,#110721,#110722);
#96399=AXIS2_PLACEMENT_3D('',#165983,#110724,#110725);
#96400=AXIS2_PLACEMENT_3D('',#165986,#110727,#110728);
#96401=AXIS2_PLACEMENT_3D('',#166047,#110729,#110730);
#96402=AXIS2_PLACEMENT_3D('',#166074,#110731,#110732);
#96403=AXIS2_PLACEMENT_3D('',#166076,#110733,#110734);
#96404=AXIS2_PLACEMENT_3D('',#166078,#110735,#110736);
#96405=AXIS2_PLACEMENT_3D('',#166079,#110737,#110738);
#96406=AXIS2_PLACEMENT_3D('',#166080,#110739,#110740);
#96407=AXIS2_PLACEMENT_3D('',#166082,#110741,#110742);
#96408=AXIS2_PLACEMENT_3D('',#166084,#110744,#110745);
#96409=AXIS2_PLACEMENT_3D('',#166086,#110746,#110747);
#96410=AXIS2_PLACEMENT_3D('',#166087,#110748,#110749);
#96411=AXIS2_PLACEMENT_3D('',#166088,#110750,#110751);
#96412=AXIS2_PLACEMENT_3D('',#166090,#110753,#110754);
#96413=AXIS2_PLACEMENT_3D('',#166092,#110755,#110756);
#96414=AXIS2_PLACEMENT_3D('',#166148,#110759,#110760);
#96415=AXIS2_PLACEMENT_3D('',#166150,#110761,#110762);
#96416=AXIS2_PLACEMENT_3D('',#166174,#110763,#110764);
#96417=AXIS2_PLACEMENT_3D('',#166207,#110765,#110766);
#96418=AXIS2_PLACEMENT_3D('',#166224,#110767,#110768);
#96419=AXIS2_PLACEMENT_3D('',#166226,#110769,#110770);
#96420=AXIS2_PLACEMENT_3D('',#166247,#110772,#110773);
#96421=AXIS2_PLACEMENT_3D('',#166293,#110774,#110775);
#96422=AXIS2_PLACEMENT_3D('',#166329,#110776,#110777);
#96423=AXIS2_PLACEMENT_3D('',#166331,#110778,#110779);
#96424=AXIS2_PLACEMENT_3D('',#166334,#110781,#110782);
#96425=AXIS2_PLACEMENT_3D('',#166335,#110783,#110784);
#96426=AXIS2_PLACEMENT_3D('',#166337,#110785,#110786);
#96427=AXIS2_PLACEMENT_3D('',#166338,#110787,#110788);
#96428=AXIS2_PLACEMENT_3D('',#166339,#110789,#110790);
#96429=AXIS2_PLACEMENT_3D('',#166341,#110792,#110793);
#96430=AXIS2_PLACEMENT_3D('',#166343,#110794,#110795);
#96431=AXIS2_PLACEMENT_3D('',#166456,#110798,#110799);
#96432=AXIS2_PLACEMENT_3D('',#166457,#110800,#110801);
#96433=AXIS2_PLACEMENT_3D('',#166458,#110802,#110803);
#96434=AXIS2_PLACEMENT_3D('',#166459,#110804,#110805);
#96435=AXIS2_PLACEMENT_3D('',#166460,#110806,#110807);
#96436=AXIS2_PLACEMENT_3D('',#166461,#110808,#110809);
#96437=AXIS2_PLACEMENT_3D('',#166463,#110810,#110811);
#96438=AXIS2_PLACEMENT_3D('',#166465,#110812,#110813);
#96439=AXIS2_PLACEMENT_3D('',#166466,#110814,#110815);
#96440=AXIS2_PLACEMENT_3D('',#166467,#110816,#110817);
#96441=AXIS2_PLACEMENT_3D('',#166470,#110819,#110820);
#96442=AXIS2_PLACEMENT_3D('',#166490,#110821,#110822);
#96443=AXIS2_PLACEMENT_3D('',#166548,#110823,#110824);
#96444=AXIS2_PLACEMENT_3D('',#166584,#110825,#110826);
#96445=AXIS2_PLACEMENT_3D('',#166614,#110827,#110828);
#96446=AXIS2_PLACEMENT_3D('',#166634,#110829,#110830);
#96447=AXIS2_PLACEMENT_3D('',#166636,#110831,#110832);
#96448=AXIS2_PLACEMENT_3D('',#166663,#110834,#110835);
#96449=AXIS2_PLACEMENT_3D('',#166693,#110836,#110837);
#96450=AXIS2_PLACEMENT_3D('',#166717,#110838,#110839);
#96451=AXIS2_PLACEMENT_3D('',#166734,#110840,#110841);
#96452=AXIS2_PLACEMENT_3D('',#166736,#110842,#110843);
#96453=AXIS2_PLACEMENT_3D('',#166769,#110845,#110846);
#96454=AXIS2_PLACEMENT_3D('',#166780,#110847,#110848);
#96455=AXIS2_PLACEMENT_3D('',#166783,#110851,#110852);
#96456=AXIS2_PLACEMENT_3D('',#166785,#110854,#110855);
#96457=AXIS2_PLACEMENT_3D('',#166787,#110856,#110857);
#96458=AXIS2_PLACEMENT_3D('',#166789,#110858,#110859);
#96459=AXIS2_PLACEMENT_3D('',#166790,#110860,#110861);
#96460=AXIS2_PLACEMENT_3D('',#166791,#110862,#110863);
#96461=AXIS2_PLACEMENT_3D('',#166794,#110865,#110866);
#96462=AXIS2_PLACEMENT_3D('',#166795,#110867,#110868);
#96463=AXIS2_PLACEMENT_3D('',#166797,#110869,#110870);
#96464=AXIS2_PLACEMENT_3D('',#166799,#110871,#110872);
#96465=AXIS2_PLACEMENT_3D('',#166800,#110873,#110874);
#96466=AXIS2_PLACEMENT_3D('',#166801,#110875,#110876);
#96467=AXIS2_PLACEMENT_3D('',#166804,#110878,#110879);
#96468=AXIS2_PLACEMENT_3D('',#166805,#110880,#110881);
#96469=AXIS2_PLACEMENT_3D('',#166807,#110882,#110883);
#96470=AXIS2_PLACEMENT_3D('',#166808,#110884,#110885);
#96471=AXIS2_PLACEMENT_3D('',#166809,#110886,#110887);
#96472=AXIS2_PLACEMENT_3D('',#166811,#110889,#110890);
#96473=AXIS2_PLACEMENT_3D('',#166814,#110892,#110893);
#96474=AXIS2_PLACEMENT_3D('',#166857,#110895,#110896);
#96475=AXIS2_PLACEMENT_3D('',#166858,#110897,#110898);
#96476=AXIS2_PLACEMENT_3D('',#166861,#110900,#110901);
#96477=AXIS2_PLACEMENT_3D('',#166912,#110902,#110903);
#96478=AXIS2_PLACEMENT_3D('',#166930,#110904,#110905);
#96479=AXIS2_PLACEMENT_3D('',#166978,#110906,#110907);
#96480=AXIS2_PLACEMENT_3D('',#166979,#110908,#110909);
#96481=AXIS2_PLACEMENT_3D('',#166982,#110911,#110912);
#96482=AXIS2_PLACEMENT_3D('',#167024,#110913,#110914);
#96483=AXIS2_PLACEMENT_3D('',#167043,#110915,#110916);
#96484=AXIS2_PLACEMENT_3D('',#167063,#110917,#110918);
#96485=AXIS2_PLACEMENT_3D('',#167066,#110919,#110920);
#96486=AXIS2_PLACEMENT_3D('',#167070,#110922,#110923);
#96487=AXIS2_PLACEMENT_3D('',#167185,#110925,#110926);
#96488=AXIS2_PLACEMENT_3D('',#167187,#110927,#110928);
#96489=AXIS2_PLACEMENT_3D('',#167216,#110929,#110930);
#96490=AXIS2_PLACEMENT_3D('',#167218,#110931,#110932);
#96491=AXIS2_PLACEMENT_3D('',#167220,#110933,#110934);
#96492=AXIS2_PLACEMENT_3D('',#167221,#110935,#110936);
#96493=AXIS2_PLACEMENT_3D('',#167222,#110937,#110938);
#96494=AXIS2_PLACEMENT_3D('',#167225,#110940,#110941);
#96495=AXIS2_PLACEMENT_3D('',#167240,#110942,#110943);
#96496=AXIS2_PLACEMENT_3D('',#167242,#110944,#110945);
#96497=AXIS2_PLACEMENT_3D('',#167244,#110946,#110947);
#96498=AXIS2_PLACEMENT_3D('',#167271,#110948,#110949);
#96499=AXIS2_PLACEMENT_3D('',#167272,#110950,#110951);
#96500=AXIS2_PLACEMENT_3D('',#167273,#110952,#110953);
#96501=AXIS2_PLACEMENT_3D('',#167300,#110954,#110955);
#96502=AXIS2_PLACEMENT_3D('',#167342,#110956,#110957);
#96503=AXIS2_PLACEMENT_3D('',#167343,#110958,#110959);
#96504=AXIS2_PLACEMENT_3D('',#167346,#110961,#110962);
#96505=AXIS2_PLACEMENT_3D('',#167391,#110963,#110964);
#96506=AXIS2_PLACEMENT_3D('',#167418,#110965,#110966);
#96507=AXIS2_PLACEMENT_3D('',#167436,#110967,#110968);
#96508=AXIS2_PLACEMENT_3D('',#167469,#110969,#110970);
#96509=AXIS2_PLACEMENT_3D('',#167470,#110971,#110972);
#96510=AXIS2_PLACEMENT_3D('',#167473,#110975,#110976);
#96511=AXIS2_PLACEMENT_3D('',#167475,#110978,#110979);
#96512=AXIS2_PLACEMENT_3D('',#167480,#110982,#110983);
#96513=AXIS2_PLACEMENT_3D('',#167481,#110984,#110985);
#96514=AXIS2_PLACEMENT_3D('',#167483,#110986,#110987);
#96515=AXIS2_PLACEMENT_3D('',#167487,#110989,#110990);
#96516=AXIS2_PLACEMENT_3D('',#167520,#110992,#110993);
#96517=AXIS2_PLACEMENT_3D('',#167531,#110994,#110995);
#96518=AXIS2_PLACEMENT_3D('',#167534,#110998,#110999);
#96519=AXIS2_PLACEMENT_3D('',#167537,#111001,#111002);
#96520=AXIS2_PLACEMENT_3D('',#167538,#111003,#111004);
#96521=AXIS2_PLACEMENT_3D('',#167540,#111005,#111006);
#96522=AXIS2_PLACEMENT_3D('',#167541,#111007,#111008);
#96523=AXIS2_PLACEMENT_3D('',#167542,#111009,#111010);
#96524=AXIS2_PLACEMENT_3D('',#167545,#111012,#111013);
#96525=AXIS2_PLACEMENT_3D('',#167578,#111014,#111015);
#96526=AXIS2_PLACEMENT_3D('',#167600,#111016,#111017);
#96527=AXIS2_PLACEMENT_3D('',#167618,#111018,#111019);
#96528=AXIS2_PLACEMENT_3D('',#167659,#111021,#111022);
#96529=AXIS2_PLACEMENT_3D('',#167660,#111023,#111024);
#96530=AXIS2_PLACEMENT_3D('',#167662,#111025,#111026);
#96531=AXIS2_PLACEMENT_3D('',#167664,#111027,#111028);
#96532=AXIS2_PLACEMENT_3D('',#167665,#111029,#111030);
#96533=AXIS2_PLACEMENT_3D('',#167666,#111031,#111032);
#96534=AXIS2_PLACEMENT_3D('',#167669,#111034,#111035);
#96535=AXIS2_PLACEMENT_3D('',#167670,#111036,#111037);
#96536=AXIS2_PLACEMENT_3D('',#167672,#111038,#111039);
#96537=AXIS2_PLACEMENT_3D('',#167674,#111040,#111041);
#96538=AXIS2_PLACEMENT_3D('',#167701,#111043,#111044);
#96539=AXIS2_PLACEMENT_3D('',#167734,#111045,#111046);
#96540=AXIS2_PLACEMENT_3D('',#167776,#111047,#111048);
#96541=AXIS2_PLACEMENT_3D('',#167796,#111049,#111050);
#96542=AXIS2_PLACEMENT_3D('',#167798,#111051,#111052);
#96543=AXIS2_PLACEMENT_3D('',#167831,#111054,#111055);
#96544=AXIS2_PLACEMENT_3D('',#167861,#111056,#111057);
#96545=AXIS2_PLACEMENT_3D('',#167898,#111058,#111059);
#96546=AXIS2_PLACEMENT_3D('',#167991,#111060,#111061);
#96547=AXIS2_PLACEMENT_3D('',#167993,#111062,#111063);
#96548=AXIS2_PLACEMENT_3D('',#167995,#111064,#111065);
#96549=AXIS2_PLACEMENT_3D('',#167996,#111066,#111067);
#96550=AXIS2_PLACEMENT_3D('',#167997,#111068,#111069);
#96551=AXIS2_PLACEMENT_3D('',#168000,#111071,#111072);
#96552=AXIS2_PLACEMENT_3D('',#168001,#111073,#111074);
#96553=AXIS2_PLACEMENT_3D('',#168003,#111075,#111076);
#96554=AXIS2_PLACEMENT_3D('',#168004,#111077,#111078);
#96555=AXIS2_PLACEMENT_3D('',#168005,#111079,#111080);
#96556=AXIS2_PLACEMENT_3D('',#168007,#111082,#111083);
#96557=AXIS2_PLACEMENT_3D('',#168009,#111084,#111085);
#96558=AXIS2_PLACEMENT_3D('',#168013,#111088,#111089);
#96559=AXIS2_PLACEMENT_3D('',#168054,#111090,#111091);
#96560=AXIS2_PLACEMENT_3D('',#168058,#111093,#111094);
#96561=AXIS2_PLACEMENT_3D('',#168060,#111096,#111097);
#96562=AXIS2_PLACEMENT_3D('',#168063,#111098,#111099);
#96563=AXIS2_PLACEMENT_3D('',#168066,#111102,#111103);
#96564=AXIS2_PLACEMENT_3D('',#168067,#111104,#111105);
#96565=AXIS2_PLACEMENT_3D('',#168094,#111106,#111107);
#96566=AXIS2_PLACEMENT_3D('',#168115,#111108,#111109);
#96567=AXIS2_PLACEMENT_3D('',#168206,#111110,#111111);
#96568=AXIS2_PLACEMENT_3D('',#168248,#111112,#111113);
#96569=AXIS2_PLACEMENT_3D('',#168249,#111114,#111115);
#96570=AXIS2_PLACEMENT_3D('',#168253,#111117,#111118);
#96571=AXIS2_PLACEMENT_3D('',#168255,#111120,#111121);
#96572=AXIS2_PLACEMENT_3D('',#168258,#111122,#111123);
#96573=AXIS2_PLACEMENT_3D('',#168260,#111124,#111125);
#96574=AXIS2_PLACEMENT_3D('',#168262,#111126,#111127);
#96575=AXIS2_PLACEMENT_3D('',#168263,#111128,#111129);
#96576=AXIS2_PLACEMENT_3D('',#168264,#111130,#111131);
#96577=AXIS2_PLACEMENT_3D('',#168268,#111133,#111134);
#96578=AXIS2_PLACEMENT_3D('',#168270,#111136,#111137);
#96579=AXIS2_PLACEMENT_3D('',#168272,#111138,#111139);
#96580=AXIS2_PLACEMENT_3D('',#168274,#111140,#111141);
#96581=AXIS2_PLACEMENT_3D('',#168275,#111142,#111143);
#96582=AXIS2_PLACEMENT_3D('',#168276,#111144,#111145);
#96583=AXIS2_PLACEMENT_3D('',#168375,#111148,#111149);
#96584=AXIS2_PLACEMENT_3D('',#168398,#111151,#111152);
#96585=AXIS2_PLACEMENT_3D('',#168413,#111153,#111154);
#96586=AXIS2_PLACEMENT_3D('',#168419,#111155,#111156);
#96587=AXIS2_PLACEMENT_3D('',#168480,#111157,#111158);
#96588=AXIS2_PLACEMENT_3D('',#168481,#111159,#111160);
#96589=AXIS2_PLACEMENT_3D('',#168485,#111162,#111163);
#96590=AXIS2_PLACEMENT_3D('',#168487,#111165,#111166);
#96591=AXIS2_PLACEMENT_3D('',#168490,#111167,#111168);
#96592=AXIS2_PLACEMENT_3D('',#168492,#111169,#111170);
#96593=AXIS2_PLACEMENT_3D('',#168494,#111171,#111172);
#96594=AXIS2_PLACEMENT_3D('',#168495,#111173,#111174);
#96595=AXIS2_PLACEMENT_3D('',#168496,#111175,#111176);
#96596=AXIS2_PLACEMENT_3D('',#168501,#111179,#111180);
#96597=AXIS2_PLACEMENT_3D('',#168502,#111181,#111182);
#96598=AXIS2_PLACEMENT_3D('',#168504,#111183,#111184);
#96599=AXIS2_PLACEMENT_3D('',#168506,#111185,#111186);
#96600=AXIS2_PLACEMENT_3D('',#168507,#111187,#111188);
#96601=AXIS2_PLACEMENT_3D('',#168508,#111189,#111190);
#96602=AXIS2_PLACEMENT_3D('',#168510,#111191,#111192);
#96603=AXIS2_PLACEMENT_3D('',#168514,#111194,#111195);
#96604=AXIS2_PLACEMENT_3D('',#168541,#111197,#111198);
#96605=AXIS2_PLACEMENT_3D('',#168568,#111199,#111200);
#96606=AXIS2_PLACEMENT_3D('',#168593,#111201,#111202);
#96607=AXIS2_PLACEMENT_3D('',#168689,#111203,#111204);
#96608=AXIS2_PLACEMENT_3D('',#168692,#111205,#111206);
#96609=AXIS2_PLACEMENT_3D('',#168695,#111209,#111210);
#96610=AXIS2_PLACEMENT_3D('',#168698,#111211,#111212);
#96611=AXIS2_PLACEMENT_3D('',#168701,#111215,#111216);
#96612=AXIS2_PLACEMENT_3D('',#168702,#111217,#111218);
#96613=AXIS2_PLACEMENT_3D('',#168703,#111219,#111220);
#96614=AXIS2_PLACEMENT_3D('',#168705,#111221,#111222);
#96615=AXIS2_PLACEMENT_3D('',#168707,#111223,#111224);
#96616=AXIS2_PLACEMENT_3D('',#168708,#111225,#111226);
#96617=AXIS2_PLACEMENT_3D('',#168709,#111227,#111228);
#96618=AXIS2_PLACEMENT_3D('',#168712,#111230,#111231);
#96619=AXIS2_PLACEMENT_3D('',#168732,#111232,#111233);
#96620=AXIS2_PLACEMENT_3D('',#168790,#111234,#111235);
#96621=AXIS2_PLACEMENT_3D('',#168826,#111236,#111237);
#96622=AXIS2_PLACEMENT_3D('',#168856,#111238,#111239);
#96623=AXIS2_PLACEMENT_3D('',#168882,#111240,#111241);
#96624=AXIS2_PLACEMENT_3D('',#168884,#111242,#111243);
#96625=AXIS2_PLACEMENT_3D('',#168911,#111245,#111246);
#96626=AXIS2_PLACEMENT_3D('',#168941,#111247,#111248);
#96627=AXIS2_PLACEMENT_3D('',#168965,#111249,#111250);
#96628=AXIS2_PLACEMENT_3D('',#168982,#111251,#111252);
#96629=AXIS2_PLACEMENT_3D('',#168984,#111253,#111254);
#96630=AXIS2_PLACEMENT_3D('',#169017,#111256,#111257);
#96631=AXIS2_PLACEMENT_3D('',#169028,#111258,#111259);
#96632=AXIS2_PLACEMENT_3D('',#169031,#111262,#111263);
#96633=AXIS2_PLACEMENT_3D('',#169033,#111265,#111266);
#96634=AXIS2_PLACEMENT_3D('',#169035,#111267,#111268);
#96635=AXIS2_PLACEMENT_3D('',#169037,#111269,#111270);
#96636=AXIS2_PLACEMENT_3D('',#169038,#111271,#111272);
#96637=AXIS2_PLACEMENT_3D('',#169039,#111273,#111274);
#96638=AXIS2_PLACEMENT_3D('',#169042,#111276,#111277);
#96639=AXIS2_PLACEMENT_3D('',#169043,#111278,#111279);
#96640=AXIS2_PLACEMENT_3D('',#169045,#111280,#111281);
#96641=AXIS2_PLACEMENT_3D('',#169047,#111282,#111283);
#96642=AXIS2_PLACEMENT_3D('',#169048,#111284,#111285);
#96643=AXIS2_PLACEMENT_3D('',#169049,#111286,#111287);
#96644=AXIS2_PLACEMENT_3D('',#169052,#111289,#111290);
#96645=AXIS2_PLACEMENT_3D('',#169053,#111291,#111292);
#96646=AXIS2_PLACEMENT_3D('',#169055,#111293,#111294);
#96647=AXIS2_PLACEMENT_3D('',#169056,#111295,#111296);
#96648=AXIS2_PLACEMENT_3D('',#169057,#111297,#111298);
#96649=AXIS2_PLACEMENT_3D('',#169059,#111300,#111301);
#96650=AXIS2_PLACEMENT_3D('',#169062,#111303,#111304);
#96651=AXIS2_PLACEMENT_3D('',#169105,#111306,#111307);
#96652=AXIS2_PLACEMENT_3D('',#169106,#111308,#111309);
#96653=AXIS2_PLACEMENT_3D('',#169109,#111311,#111312);
#96654=AXIS2_PLACEMENT_3D('',#169160,#111313,#111314);
#96655=AXIS2_PLACEMENT_3D('',#169178,#111315,#111316);
#96656=AXIS2_PLACEMENT_3D('',#169226,#111317,#111318);
#96657=AXIS2_PLACEMENT_3D('',#169227,#111319,#111320);
#96658=AXIS2_PLACEMENT_3D('',#169230,#111322,#111323);
#96659=AXIS2_PLACEMENT_3D('',#169269,#111324,#111325);
#96660=AXIS2_PLACEMENT_3D('',#169288,#111326,#111327);
#96661=AXIS2_PLACEMENT_3D('',#169302,#111328,#111329);
#96662=AXIS2_PLACEMENT_3D('',#169305,#111330,#111331);
#96663=AXIS2_PLACEMENT_3D('',#169309,#111333,#111334);
#96664=AXIS2_PLACEMENT_3D('',#169424,#111336,#111337);
#96665=AXIS2_PLACEMENT_3D('',#169426,#111338,#111339);
#96666=AXIS2_PLACEMENT_3D('',#169443,#111340,#111341);
#96667=AXIS2_PLACEMENT_3D('',#169445,#111342,#111343);
#96668=AXIS2_PLACEMENT_3D('',#169447,#111344,#111345);
#96669=AXIS2_PLACEMENT_3D('',#169448,#111346,#111347);
#96670=AXIS2_PLACEMENT_3D('',#169449,#111348,#111349);
#96671=AXIS2_PLACEMENT_3D('',#169452,#111351,#111352);
#96672=AXIS2_PLACEMENT_3D('',#169466,#111353,#111354);
#96673=AXIS2_PLACEMENT_3D('',#169468,#111355,#111356);
#96674=AXIS2_PLACEMENT_3D('',#169498,#111357,#111358);
#96675=AXIS2_PLACEMENT_3D('',#169512,#111359,#111360);
#96676=AXIS2_PLACEMENT_3D('',#169514,#111361,#111362);
#96677=AXIS2_PLACEMENT_3D('',#169535,#111364,#111365);
#96678=AXIS2_PLACEMENT_3D('',#169571,#111366,#111367);
#96679=AXIS2_PLACEMENT_3D('',#169589,#111368,#111369);
#96680=AXIS2_PLACEMENT_3D('',#169614,#111370,#111371);
#96681=AXIS2_PLACEMENT_3D('',#169689,#111372,#111373);
#96682=AXIS2_PLACEMENT_3D('',#169690,#111374,#111375);
#96683=AXIS2_PLACEMENT_3D('',#169691,#111376,#111377);
#96684=AXIS2_PLACEMENT_3D('',#169693,#111378,#111379);
#96685=AXIS2_PLACEMENT_3D('',#169697,#111381,#111382);
#96686=AXIS2_PLACEMENT_3D('',#169730,#111384,#111385);
#96687=AXIS2_PLACEMENT_3D('',#169741,#111386,#111387);
#96688=AXIS2_PLACEMENT_3D('',#169744,#111390,#111391);
#96689=AXIS2_PLACEMENT_3D('',#169747,#111393,#111394);
#96690=AXIS2_PLACEMENT_3D('',#169748,#111395,#111396);
#96691=AXIS2_PLACEMENT_3D('',#169750,#111397,#111398);
#96692=AXIS2_PLACEMENT_3D('',#169751,#111399,#111400);
#96693=AXIS2_PLACEMENT_3D('',#169752,#111401,#111402);
#96694=AXIS2_PLACEMENT_3D('',#169754,#111403,#111404);
#96695=AXIS2_PLACEMENT_3D('',#169788,#111406,#111407);
#96696=AXIS2_PLACEMENT_3D('',#169827,#111408,#111409);
#96697=AXIS2_PLACEMENT_3D('',#169846,#111410,#111411);
#96698=AXIS2_PLACEMENT_3D('',#169848,#111413,#111414);
#96699=AXIS2_PLACEMENT_3D('',#169851,#111417,#111418);
#96700=AXIS2_PLACEMENT_3D('',#169854,#111419,#111420);
#96701=AXIS2_PLACEMENT_3D('',#169857,#111423,#111424);
#96702=AXIS2_PLACEMENT_3D('',#169860,#111425,#111426);
#96703=AXIS2_PLACEMENT_3D('',#169861,#111427,#111428);
#96704=AXIS2_PLACEMENT_3D('',#169862,#111429,#111430);
#96705=AXIS2_PLACEMENT_3D('',#169863,#111431,#111432);
#96706=AXIS2_PLACEMENT_3D('',#169866,#111434,#111435);
#96707=AXIS2_PLACEMENT_3D('',#169867,#111436,#111437);
#96708=AXIS2_PLACEMENT_3D('',#169869,#111438,#111439);
#96709=AXIS2_PLACEMENT_3D('',#169871,#111440,#111441);
#96710=AXIS2_PLACEMENT_3D('',#169886,#111443,#111444);
#96711=AXIS2_PLACEMENT_3D('',#169910,#111445,#111446);
#96712=AXIS2_PLACEMENT_3D('',#169967,#111447,#111448);
#96713=AXIS2_PLACEMENT_3D('',#169984,#111449,#111450);
#96714=AXIS2_PLACEMENT_3D('',#169987,#111452,#111453);
#96715=AXIS2_PLACEMENT_3D('',#170026,#111454,#111455);
#96716=AXIS2_PLACEMENT_3D('',#170078,#111456,#111457);
#96717=AXIS2_PLACEMENT_3D('',#170104,#111458,#111459);
#96718=AXIS2_PLACEMENT_3D('',#170106,#111460,#111461);
#96719=AXIS2_PLACEMENT_3D('',#170108,#111462,#111463);
#96720=AXIS2_PLACEMENT_3D('',#170109,#111464,#111465);
#96721=AXIS2_PLACEMENT_3D('',#170110,#111466,#111467);
#96722=AXIS2_PLACEMENT_3D('',#170113,#111469,#111470);
#96723=AXIS2_PLACEMENT_3D('',#170114,#111471,#111472);
#96724=AXIS2_PLACEMENT_3D('',#170116,#111473,#111474);
#96725=AXIS2_PLACEMENT_3D('',#170117,#111475,#111476);
#96726=AXIS2_PLACEMENT_3D('',#170118,#111477,#111478);
#96727=AXIS2_PLACEMENT_3D('',#170120,#111480,#111481);
#96728=AXIS2_PLACEMENT_3D('',#170122,#111482,#111483);
#96729=AXIS2_PLACEMENT_3D('',#170126,#111486,#111487);
#96730=AXIS2_PLACEMENT_3D('',#170167,#111488,#111489);
#96731=AXIS2_PLACEMENT_3D('',#170169,#111490,#111491);
#96732=AXIS2_PLACEMENT_3D('',#170170,#111492,#111493);
#96733=AXIS2_PLACEMENT_3D('',#170171,#111494,#111495);
#96734=AXIS2_PLACEMENT_3D('',#170175,#111497,#111498);
#96735=AXIS2_PLACEMENT_3D('',#170177,#111500,#111501);
#96736=AXIS2_PLACEMENT_3D('',#170181,#111503,#111504);
#96737=AXIS2_PLACEMENT_3D('',#170218,#111506,#111507);
#96738=AXIS2_PLACEMENT_3D('',#170220,#111508,#111509);
#96739=AXIS2_PLACEMENT_3D('',#170247,#111510,#111511);
#96740=AXIS2_PLACEMENT_3D('',#170273,#111512,#111513);
#96741=AXIS2_PLACEMENT_3D('',#170275,#111514,#111515);
#96742=AXIS2_PLACEMENT_3D('',#170297,#111517,#111518);
#96743=AXIS2_PLACEMENT_3D('',#170359,#111519,#111520);
#96744=AXIS2_PLACEMENT_3D('',#170361,#111521,#111522);
#96745=AXIS2_PLACEMENT_3D('',#170364,#111524,#111525);
#96746=AXIS2_PLACEMENT_3D('',#170365,#111526,#111527);
#96747=AXIS2_PLACEMENT_3D('',#170367,#111528,#111529);
#96748=AXIS2_PLACEMENT_3D('',#170368,#111530,#111531);
#96749=AXIS2_PLACEMENT_3D('',#170369,#111532,#111533);
#96750=AXIS2_PLACEMENT_3D('',#170371,#111535,#111536);
#96751=AXIS2_PLACEMENT_3D('',#170373,#111537,#111538);
#96752=AXIS2_PLACEMENT_3D('',#170388,#111541,#111542);
#96753=AXIS2_PLACEMENT_3D('',#170409,#111543,#111544);
#96754=AXIS2_PLACEMENT_3D('',#170569,#111545,#111546);
#96755=AXIS2_PLACEMENT_3D('',#170571,#111547,#111548);
#96756=AXIS2_PLACEMENT_3D('',#170580,#111549,#111550);
#96757=AXIS2_PLACEMENT_3D('',#170582,#111551,#111552);
#96758=AXIS2_PLACEMENT_3D('',#170619,#111554,#111555);
#96759=AXIS2_PLACEMENT_3D('',#170646,#111556,#111557);
#96760=AXIS2_PLACEMENT_3D('',#170660,#111558,#111559);
#96761=AXIS2_PLACEMENT_3D('',#170661,#111560,#111561);
#96762=AXIS2_PLACEMENT_3D('',#170662,#111562,#111563);
#96763=AXIS2_PLACEMENT_3D('',#170665,#111566,#111567);
#96764=AXIS2_PLACEMENT_3D('',#170668,#111569,#111570);
#96765=AXIS2_PLACEMENT_3D('',#170669,#111571,#111572);
#96766=AXIS2_PLACEMENT_3D('',#170671,#111573,#111574);
#96767=AXIS2_PLACEMENT_3D('',#170672,#111575,#111576);
#96768=AXIS2_PLACEMENT_3D('',#170673,#111577,#111578);
#96769=AXIS2_PLACEMENT_3D('',#170676,#111580,#111581);
#96770=AXIS2_PLACEMENT_3D('',#170728,#111582,#111583);
#96771=AXIS2_PLACEMENT_3D('',#170736,#111584,#111585);
#96772=AXIS2_PLACEMENT_3D('',#170738,#111586,#111587);
#96773=AXIS2_PLACEMENT_3D('',#170740,#111588,#111589);
#96774=AXIS2_PLACEMENT_3D('',#170741,#111590,#111591);
#96775=AXIS2_PLACEMENT_3D('',#170742,#111592,#111593);
#96776=AXIS2_PLACEMENT_3D('',#170745,#111595,#111596);
#96777=AXIS2_PLACEMENT_3D('',#170746,#111597,#111598);
#96778=AXIS2_PLACEMENT_3D('',#170748,#111599,#111600);
#96779=AXIS2_PLACEMENT_3D('',#170750,#111601,#111602);
#96780=AXIS2_PLACEMENT_3D('',#170751,#111603,#111604);
#96781=AXIS2_PLACEMENT_3D('',#170752,#111605,#111606);
#96782=AXIS2_PLACEMENT_3D('',#170755,#111608,#111609);
#96783=AXIS2_PLACEMENT_3D('',#170756,#111610,#111611);
#96784=AXIS2_PLACEMENT_3D('',#170757,#111612,#111613);
#96785=AXIS2_PLACEMENT_3D('',#170758,#111614,#111615);
#96786=AXIS2_PLACEMENT_3D('',#170761,#111617,#111618);
#96787=AXIS2_PLACEMENT_3D('',#170776,#111620,#111621);
#96788=AXIS2_PLACEMENT_3D('',#170777,#111622,#111623);
#96789=AXIS2_PLACEMENT_3D('',#170804,#111624,#111625);
#96790=AXIS2_PLACEMENT_3D('',#170840,#111626,#111627);
#96791=AXIS2_PLACEMENT_3D('',#170841,#111628,#111629);
#96792=AXIS2_PLACEMENT_3D('',#170844,#111631,#111632);
#96793=AXIS2_PLACEMENT_3D('',#170865,#111633,#111634);
#96794=AXIS2_PLACEMENT_3D('',#171002,#111635,#111636);
#96795=AXIS2_PLACEMENT_3D('',#171174,#111637,#111638);
#96796=AXIS2_PLACEMENT_3D('',#171176,#111639,#111640);
#96797=AXIS2_PLACEMENT_3D('',#171190,#111641,#111642);
#96798=AXIS2_PLACEMENT_3D('',#171192,#111643,#111644);
#96799=AXIS2_PLACEMENT_3D('',#171213,#111646,#111647);
#96800=AXIS2_PLACEMENT_3D('',#171240,#111648,#111649);
#96801=AXIS2_PLACEMENT_3D('',#171258,#111650,#111651);
#96802=AXIS2_PLACEMENT_3D('',#171259,#111652,#111653);
#96803=AXIS2_PLACEMENT_3D('',#171260,#111654,#111655);
#96804=AXIS2_PLACEMENT_3D('',#171346,#111658,#111659);
#96805=AXIS2_PLACEMENT_3D('',#171377,#111660,#111661);
#96806=AXIS2_PLACEMENT_3D('',#171382,#111662,#111663);
#96807=AXIS2_PLACEMENT_3D('',#171385,#111664,#111665);
#96808=AXIS2_PLACEMENT_3D('',#171388,#111668,#111669);
#96809=AXIS2_PLACEMENT_3D('',#171395,#111671,#111672);
#96810=AXIS2_PLACEMENT_3D('',#171397,#111673,#111674);
#96811=AXIS2_PLACEMENT_3D('',#171400,#111676,#111677);
#96812=AXIS2_PLACEMENT_3D('',#171480,#111678,#111679);
#96813=AXIS2_PLACEMENT_3D('',#171483,#111681,#111682);
#96814=AXIS2_PLACEMENT_3D('',#171498,#111684,#111685);
#96815=AXIS2_PLACEMENT_3D('',#171499,#111686,#111687);
#96816=AXIS2_PLACEMENT_3D('',#171517,#111688,#111689);
#96817=AXIS2_PLACEMENT_3D('',#171550,#111690,#111691);
#96818=AXIS2_PLACEMENT_3D('',#171551,#111692,#111693);
#96819=AXIS2_PLACEMENT_3D('',#171554,#111695,#111696);
#96820=AXIS2_PLACEMENT_3D('',#171588,#111697,#111698);
#96821=AXIS2_PLACEMENT_3D('',#171671,#111699,#111700);
#96822=AXIS2_PLACEMENT_3D('',#171753,#111701,#111702);
#96823=AXIS2_PLACEMENT_3D('',#171767,#111703,#111704);
#96824=AXIS2_PLACEMENT_3D('',#171769,#111705,#111706);
#96825=AXIS2_PLACEMENT_3D('',#171770,#111707,#111708);
#96826=AXIS2_PLACEMENT_3D('',#171771,#111709,#111710);
#96827=AXIS2_PLACEMENT_3D('',#171773,#111711,#111712);
#96828=AXIS2_PLACEMENT_3D('',#171788,#111714,#111715);
#96829=AXIS2_PLACEMENT_3D('',#171789,#111716,#111717);
#96830=AXIS2_PLACEMENT_3D('',#171803,#111718,#111719);
#96831=AXIS2_PLACEMENT_3D('',#171821,#111720,#111721);
#96832=AXIS2_PLACEMENT_3D('',#171822,#111722,#111723);
#96833=AXIS2_PLACEMENT_3D('',#171823,#111724,#111725);
#96834=AXIS2_PLACEMENT_3D('',#171882,#111728,#111729);
#96835=AXIS2_PLACEMENT_3D('',#171907,#111730,#111731);
#96836=AXIS2_PLACEMENT_3D('',#171912,#111732,#111733);
#96837=AXIS2_PLACEMENT_3D('',#171915,#111734,#111735);
#96838=AXIS2_PLACEMENT_3D('',#171918,#111738,#111739);
#96839=AXIS2_PLACEMENT_3D('',#171920,#111740,#111741);
#96840=AXIS2_PLACEMENT_3D('',#171922,#111743,#111744);
#96841=AXIS2_PLACEMENT_3D('',#171924,#111745,#111746);
#96842=AXIS2_PLACEMENT_3D('',#171927,#111748,#111749);
#96843=AXIS2_PLACEMENT_3D('',#171983,#111750,#111751);
#96844=AXIS2_PLACEMENT_3D('',#171986,#111753,#111754);
#96845=AXIS2_PLACEMENT_3D('',#172001,#111756,#111757);
#96846=AXIS2_PLACEMENT_3D('',#172002,#111758,#111759);
#96847=AXIS2_PLACEMENT_3D('',#172020,#111760,#111761);
#96848=AXIS2_PLACEMENT_3D('',#172034,#111762,#111763);
#96849=AXIS2_PLACEMENT_3D('',#172035,#111764,#111765);
#96850=AXIS2_PLACEMENT_3D('',#172036,#111766,#111767);
#96851=AXIS2_PLACEMENT_3D('',#172039,#111769,#111770);
#96852=AXIS2_PLACEMENT_3D('',#172053,#111771,#111772);
#96853=AXIS2_PLACEMENT_3D('',#172055,#111773,#111774);
#96854=AXIS2_PLACEMENT_3D('',#172056,#111775,#111776);
#96855=AXIS2_PLACEMENT_3D('',#172075,#111777,#111778);
#96856=AXIS2_PLACEMENT_3D('',#172228,#111779,#111780);
#96857=AXIS2_PLACEMENT_3D('',#172230,#111781,#111782);
#96858=AXIS2_PLACEMENT_3D('',#172244,#111783,#111784);
#96859=AXIS2_PLACEMENT_3D('',#172246,#111785,#111786);
#96860=AXIS2_PLACEMENT_3D('',#172267,#111788,#111789);
#96861=AXIS2_PLACEMENT_3D('',#172294,#111790,#111791);
#96862=AXIS2_PLACEMENT_3D('',#172312,#111792,#111793);
#96863=AXIS2_PLACEMENT_3D('',#172313,#111794,#111795);
#96864=AXIS2_PLACEMENT_3D('',#172314,#111796,#111797);
#96865=AXIS2_PLACEMENT_3D('',#172394,#111800,#111801);
#96866=AXIS2_PLACEMENT_3D('',#172424,#111802,#111803);
#96867=AXIS2_PLACEMENT_3D('',#172429,#111804,#111805);
#96868=AXIS2_PLACEMENT_3D('',#172433,#111807,#111808);
#96869=AXIS2_PLACEMENT_3D('',#172435,#111810,#111811);
#96870=AXIS2_PLACEMENT_3D('',#172442,#111813,#111814);
#96871=AXIS2_PLACEMENT_3D('',#172444,#111815,#111816);
#96872=AXIS2_PLACEMENT_3D('',#172447,#111818,#111819);
#96873=AXIS2_PLACEMENT_3D('',#172527,#111820,#111821);
#96874=AXIS2_PLACEMENT_3D('',#172530,#111823,#111824);
#96875=AXIS2_PLACEMENT_3D('',#172545,#111826,#111827);
#96876=AXIS2_PLACEMENT_3D('',#172546,#111828,#111829);
#96877=AXIS2_PLACEMENT_3D('',#172564,#111830,#111831);
#96878=AXIS2_PLACEMENT_3D('',#172597,#111832,#111833);
#96879=AXIS2_PLACEMENT_3D('',#172598,#111834,#111835);
#96880=AXIS2_PLACEMENT_3D('',#172601,#111837,#111838);
#96881=AXIS2_PLACEMENT_3D('',#172635,#111839,#111840);
#96882=AXIS2_PLACEMENT_3D('',#172718,#111841,#111842);
#96883=AXIS2_PLACEMENT_3D('',#172883,#111843,#111844);
#96884=AXIS2_PLACEMENT_3D('',#172885,#111845,#111846);
#96885=AXIS2_PLACEMENT_3D('',#172902,#111847,#111848);
#96886=AXIS2_PLACEMENT_3D('',#172904,#111849,#111850);
#96887=AXIS2_PLACEMENT_3D('',#172938,#111852,#111853);
#96888=AXIS2_PLACEMENT_3D('',#172965,#111854,#111855);
#96889=AXIS2_PLACEMENT_3D('',#172979,#111856,#111857);
#96890=AXIS2_PLACEMENT_3D('',#172980,#111858,#111859);
#96891=AXIS2_PLACEMENT_3D('',#172981,#111860,#111861);
#96892=AXIS2_PLACEMENT_3D('',#172984,#111864,#111865);
#96893=AXIS2_PLACEMENT_3D('',#172986,#111866,#111867);
#96894=AXIS2_PLACEMENT_3D('',#172987,#111868,#111869);
#96895=AXIS2_PLACEMENT_3D('',#172988,#111870,#111871);
#96896=AXIS2_PLACEMENT_3D('',#172991,#111873,#111874);
#96897=AXIS2_PLACEMENT_3D('',#173055,#111875,#111876);
#96898=AXIS2_PLACEMENT_3D('',#173063,#111877,#111878);
#96899=AXIS2_PLACEMENT_3D('',#173065,#111879,#111880);
#96900=AXIS2_PLACEMENT_3D('',#173067,#111881,#111882);
#96901=AXIS2_PLACEMENT_3D('',#173068,#111883,#111884);
#96902=AXIS2_PLACEMENT_3D('',#173069,#111885,#111886);
#96903=AXIS2_PLACEMENT_3D('',#173072,#111888,#111889);
#96904=AXIS2_PLACEMENT_3D('',#173073,#111890,#111891);
#96905=AXIS2_PLACEMENT_3D('',#173075,#111892,#111893);
#96906=AXIS2_PLACEMENT_3D('',#173077,#111894,#111895);
#96907=AXIS2_PLACEMENT_3D('',#173078,#111896,#111897);
#96908=AXIS2_PLACEMENT_3D('',#173079,#111898,#111899);
#96909=AXIS2_PLACEMENT_3D('',#173082,#111901,#111902);
#96910=AXIS2_PLACEMENT_3D('',#173083,#111903,#111904);
#96911=AXIS2_PLACEMENT_3D('',#173085,#111905,#111906);
#96912=AXIS2_PLACEMENT_3D('',#173086,#111907,#111908);
#96913=AXIS2_PLACEMENT_3D('',#173087,#111909,#111910);
#96914=AXIS2_PLACEMENT_3D('',#173089,#111912,#111913);
#96915=AXIS2_PLACEMENT_3D('',#173092,#111915,#111916);
#96916=AXIS2_PLACEMENT_3D('',#173107,#111918,#111919);
#96917=AXIS2_PLACEMENT_3D('',#173108,#111920,#111921);
#96918=AXIS2_PLACEMENT_3D('',#173135,#111922,#111923);
#96919=AXIS2_PLACEMENT_3D('',#173163,#111924,#111925);
#96920=AXIS2_PLACEMENT_3D('',#173164,#111926,#111927);
#96921=AXIS2_PLACEMENT_3D('',#173167,#111929,#111930);
#96922=AXIS2_PLACEMENT_3D('',#173188,#111931,#111932);
#96923=AXIS2_PLACEMENT_3D('',#173322,#111933,#111934);
#96924=AXIS2_PLACEMENT_3D('',#173502,#111935,#111936);
#96925=AXIS2_PLACEMENT_3D('',#173504,#111937,#111938);
#96926=AXIS2_PLACEMENT_3D('',#173506,#111939,#111940);
#96927=AXIS2_PLACEMENT_3D('',#173507,#111941,#111942);
#96928=AXIS2_PLACEMENT_3D('',#173508,#111943,#111944);
#96929=AXIS2_PLACEMENT_3D('',#173511,#111946,#111947);
#96930=AXIS2_PLACEMENT_3D('',#173532,#111948,#111949);
#96931=AXIS2_PLACEMENT_3D('',#173541,#111950,#111951);
#96932=AXIS2_PLACEMENT_3D('',#173626,#111952,#111953);
#96933=AXIS2_PLACEMENT_3D('',#173627,#111954,#111955);
#96934=AXIS2_PLACEMENT_3D('',#173630,#111957,#111958);
#96935=AXIS2_PLACEMENT_3D('',#173672,#111959,#111960);
#96936=AXIS2_PLACEMENT_3D('',#173699,#111961,#111962);
#96937=AXIS2_PLACEMENT_3D('',#173713,#111963,#111964);
#96938=AXIS2_PLACEMENT_3D('',#173714,#111965,#111966);
#96939=AXIS2_PLACEMENT_3D('',#173715,#111967,#111968);
#96940=AXIS2_PLACEMENT_3D('',#173718,#111971,#111972);
#96941=AXIS2_PLACEMENT_3D('',#173720,#111974,#111975);
#96942=AXIS2_PLACEMENT_3D('',#173722,#111976,#111977);
#96943=AXIS2_PLACEMENT_3D('',#173724,#111978,#111979);
#96944=AXIS2_PLACEMENT_3D('',#173725,#111980,#111981);
#96945=AXIS2_PLACEMENT_3D('',#173726,#111982,#111983);
#96946=AXIS2_PLACEMENT_3D('',#173729,#111985,#111986);
#96947=AXIS2_PLACEMENT_3D('',#173730,#111987,#111988);
#96948=AXIS2_PLACEMENT_3D('',#173732,#111989,#111990);
#96949=AXIS2_PLACEMENT_3D('',#173733,#111991,#111992);
#96950=AXIS2_PLACEMENT_3D('',#173734,#111993,#111994);
#96951=AXIS2_PLACEMENT_3D('',#173736,#111995,#111996);
#96952=AXIS2_PLACEMENT_3D('',#173738,#111997,#111998);
#96953=AXIS2_PLACEMENT_3D('',#173739,#111999,#112000);
#96954=AXIS2_PLACEMENT_3D('',#173740,#112001,#112002);
#96955=AXIS2_PLACEMENT_3D('',#173743,#112004,#112005);
#96956=AXIS2_PLACEMENT_3D('',#173744,#112006,#112007);
#96957=AXIS2_PLACEMENT_3D('',#173746,#112008,#112009);
#96958=AXIS2_PLACEMENT_3D('',#173747,#112010,#112011);
#96959=AXIS2_PLACEMENT_3D('',#173762,#112012,#112013);
#96960=AXIS2_PLACEMENT_3D('',#173779,#112014,#112015);
#96961=AXIS2_PLACEMENT_3D('',#173798,#112016,#112017);
#96962=AXIS2_PLACEMENT_3D('',#173805,#112018,#112019);
#96963=AXIS2_PLACEMENT_3D('',#173834,#112020,#112021);
#96964=AXIS2_PLACEMENT_3D('',#173836,#112022,#112023);
#96965=AXIS2_PLACEMENT_3D('',#173838,#112024,#112025);
#96966=AXIS2_PLACEMENT_3D('',#173857,#112026,#112027);
#96967=AXIS2_PLACEMENT_3D('',#173895,#112028,#112029);
#96968=AXIS2_PLACEMENT_3D('',#173902,#112030,#112031);
#96969=AXIS2_PLACEMENT_3D('',#173950,#112032,#112033);
#96970=AXIS2_PLACEMENT_3D('',#174054,#112034,#112035);
#96971=AXIS2_PLACEMENT_3D('',#174058,#112037,#112038);
#96972=AXIS2_PLACEMENT_3D('',#174060,#112040,#112041);
#96973=AXIS2_PLACEMENT_3D('',#174063,#112042,#112043);
#96974=AXIS2_PLACEMENT_3D('',#174065,#112044,#112045);
#96975=AXIS2_PLACEMENT_3D('',#174067,#112046,#112047);
#96976=AXIS2_PLACEMENT_3D('',#174068,#112048,#112049);
#96977=AXIS2_PLACEMENT_3D('',#174069,#112050,#112051);
#96978=AXIS2_PLACEMENT_3D('',#174074,#112054,#112055);
#96979=AXIS2_PLACEMENT_3D('',#174075,#112056,#112057);
#96980=AXIS2_PLACEMENT_3D('',#174077,#112058,#112059);
#96981=AXIS2_PLACEMENT_3D('',#174079,#112060,#112061);
#96982=AXIS2_PLACEMENT_3D('',#174080,#112062,#112063);
#96983=AXIS2_PLACEMENT_3D('',#174081,#112064,#112065);
#96984=AXIS2_PLACEMENT_3D('',#174083,#112066,#112067);
#96985=AXIS2_PLACEMENT_3D('',#174087,#112069,#112070);
#96986=AXIS2_PLACEMENT_3D('',#174108,#112072,#112073);
#96987=AXIS2_PLACEMENT_3D('',#174139,#112074,#112075);
#96988=AXIS2_PLACEMENT_3D('',#174189,#112076,#112077);
#96989=AXIS2_PLACEMENT_3D('',#174278,#112078,#112079);
#96990=AXIS2_PLACEMENT_3D('',#174279,#112080,#112081);
#96991=AXIS2_PLACEMENT_3D('',#174280,#112082,#112083);
#96992=AXIS2_PLACEMENT_3D('',#174281,#112084,#112085);
#96993=AXIS2_PLACEMENT_3D('',#174282,#112086,#112087);
#96994=AXIS2_PLACEMENT_3D('',#174283,#112088,#112089);
#96995=AXIS2_PLACEMENT_3D('',#174286,#112090,#112091);
#96996=AXIS2_PLACEMENT_3D('',#174288,#112092,#112093);
#96997=AXIS2_PLACEMENT_3D('',#174289,#112094,#112095);
#96998=AXIS2_PLACEMENT_3D('',#174290,#112096,#112097);
#96999=AXIS2_PLACEMENT_3D('',#174291,#112098,#112099);
#97000=AXIS2_PLACEMENT_3D('',#174294,#112101,#112102);
#97001=AXIS2_PLACEMENT_3D('',#174295,#112103,#112104);
#97002=AXIS2_PLACEMENT_3D('',#174297,#112105,#112106);
#97003=AXIS2_PLACEMENT_3D('',#174298,#112107,#112108);
#97004=AXIS2_PLACEMENT_3D('',#174313,#112109,#112110);
#97005=AXIS2_PLACEMENT_3D('',#174319,#112111,#112112);
#97006=AXIS2_PLACEMENT_3D('',#174383,#112113,#112114);
#97007=AXIS2_PLACEMENT_3D('',#174384,#112115,#112116);
#97008=AXIS2_PLACEMENT_3D('',#174387,#112118,#112119);
#97009=AXIS2_PLACEMENT_3D('',#174427,#112120,#112121);
#97010=AXIS2_PLACEMENT_3D('',#174485,#112122,#112123);
#97011=AXIS2_PLACEMENT_3D('',#174579,#112124,#112125);
#97012=AXIS2_PLACEMENT_3D('',#174581,#112126,#112127);
#97013=AXIS2_PLACEMENT_3D('',#174583,#112128,#112129);
#97014=AXIS2_PLACEMENT_3D('',#174584,#112130,#112131);
#97015=AXIS2_PLACEMENT_3D('',#174585,#112132,#112133);
#97016=AXIS2_PLACEMENT_3D('',#174588,#112135,#112136);
#97017=AXIS2_PLACEMENT_3D('',#174608,#112137,#112138);
#97018=AXIS2_PLACEMENT_3D('',#174610,#112139,#112140);
#97019=AXIS2_PLACEMENT_3D('',#174627,#112141,#112142);
#97020=AXIS2_PLACEMENT_3D('',#174629,#112143,#112144);
#97021=AXIS2_PLACEMENT_3D('',#174650,#112146,#112147);
#97022=AXIS2_PLACEMENT_3D('',#174678,#112148,#112149);
#97023=AXIS2_PLACEMENT_3D('',#174735,#112150,#112151);
#97024=AXIS2_PLACEMENT_3D('',#174740,#112152,#112153);
#97025=AXIS2_PLACEMENT_3D('',#174742,#112154,#112155);
#97026=AXIS2_PLACEMENT_3D('',#174744,#112156,#112157);
#97027=AXIS2_PLACEMENT_3D('',#174745,#112158,#112159);
#97028=AXIS2_PLACEMENT_3D('',#174746,#112160,#112161);
#97029=AXIS2_PLACEMENT_3D('',#174749,#112163,#112164);
#97030=AXIS2_PLACEMENT_3D('',#174750,#112165,#112166);
#97031=AXIS2_PLACEMENT_3D('',#174752,#112167,#112168);
#97032=AXIS2_PLACEMENT_3D('',#174754,#112169,#112170);
#97033=AXIS2_PLACEMENT_3D('',#174755,#112171,#112172);
#97034=AXIS2_PLACEMENT_3D('',#174756,#112173,#112174);
#97035=AXIS2_PLACEMENT_3D('',#174759,#112176,#112177);
#97036=AXIS2_PLACEMENT_3D('',#174760,#112178,#112179);
#97037=AXIS2_PLACEMENT_3D('',#174762,#112180,#112181);
#97038=AXIS2_PLACEMENT_3D('',#174763,#112182,#112183);
#97039=AXIS2_PLACEMENT_3D('',#174778,#112184,#112185);
#97040=AXIS2_PLACEMENT_3D('',#174784,#112186,#112187);
#97041=AXIS2_PLACEMENT_3D('',#174839,#112188,#112189);
#97042=AXIS2_PLACEMENT_3D('',#174840,#112190,#112191);
#97043=AXIS2_PLACEMENT_3D('',#174843,#112193,#112194);
#97044=AXIS2_PLACEMENT_3D('',#174877,#112195,#112196);
#97045=AXIS2_PLACEMENT_3D('',#174993,#112197,#112198);
#97046=AXIS2_PLACEMENT_3D('',#175152,#112199,#112200);
#97047=AXIS2_PLACEMENT_3D('',#175154,#112201,#112202);
#97048=AXIS2_PLACEMENT_3D('',#175168,#112203,#112204);
#97049=AXIS2_PLACEMENT_3D('',#175170,#112205,#112206);
#97050=AXIS2_PLACEMENT_3D('',#175191,#112208,#112209);
#97051=AXIS2_PLACEMENT_3D('',#175219,#112210,#112211);
#97052=AXIS2_PLACEMENT_3D('',#175269,#112212,#112213);
#97053=AXIS2_PLACEMENT_3D('',#175274,#112214,#112215);
#97054=AXIS2_PLACEMENT_3D('',#175277,#112216,#112217);
#97055=AXIS2_PLACEMENT_3D('',#175281,#112219,#112220);
#97056=AXIS2_PLACEMENT_3D('',#175283,#112222,#112223);
#97057=AXIS2_PLACEMENT_3D('',#175295,#112225,#112226);
#97058=AXIS2_PLACEMENT_3D('',#175297,#112227,#112228);
#97059=AXIS2_PLACEMENT_3D('',#175300,#112230,#112231);
#97060=AXIS2_PLACEMENT_3D('',#175315,#112232,#112233);
#97061=AXIS2_PLACEMENT_3D('',#175321,#112234,#112235);
#97062=AXIS2_PLACEMENT_3D('',#175368,#112236,#112237);
#97063=AXIS2_PLACEMENT_3D('',#175369,#112238,#112239);
#97064=AXIS2_PLACEMENT_3D('',#175372,#112241,#112242);
#97065=AXIS2_PLACEMENT_3D('',#175406,#112243,#112244);
#97066=AXIS2_PLACEMENT_3D('',#175495,#112245,#112246);
#97067=AXIS2_PLACEMENT_3D('',#175586,#112247,#112248);
#97068=AXIS2_PLACEMENT_3D('',#175600,#112249,#112250);
#97069=AXIS2_PLACEMENT_3D('',#175602,#112251,#112252);
#97070=AXIS2_PLACEMENT_3D('',#175603,#112253,#112254);
#97071=AXIS2_PLACEMENT_3D('',#175604,#112255,#112256);
#97072=AXIS2_PLACEMENT_3D('',#175606,#112257,#112258);
#97073=AXIS2_PLACEMENT_3D('',#175621,#112260,#112261);
#97074=AXIS2_PLACEMENT_3D('',#175622,#112262,#112263);
#97075=AXIS2_PLACEMENT_3D('',#175637,#112264,#112265);
#97076=AXIS2_PLACEMENT_3D('',#175680,#112266,#112267);
#97077=AXIS2_PLACEMENT_3D('',#175685,#112268,#112269);
#97078=AXIS2_PLACEMENT_3D('',#175689,#112271,#112272);
#97079=AXIS2_PLACEMENT_3D('',#175691,#112274,#112275);
#97080=AXIS2_PLACEMENT_3D('',#175789,#112277,#112278);
#97081=AXIS2_PLACEMENT_3D('',#175803,#112279,#112280);
#97082=AXIS2_PLACEMENT_3D('',#175804,#112281,#112282);
#97083=AXIS2_PLACEMENT_3D('',#175821,#112285,#112286);
#97084=AXIS2_PLACEMENT_3D('',#175822,#112287,#112288);
#97085=AXIS2_PLACEMENT_3D('',#175823,#112289,#112290);
#97086=AXIS2_PLACEMENT_3D('',#175824,#112291,#112292);
#97087=AXIS2_PLACEMENT_3D('',#175825,#112293,#112294);
#97088=AXIS2_PLACEMENT_3D('',#175840,#112295,#112296);
#97089=AXIS2_PLACEMENT_3D('',#175841,#112297,#112298);
#97090=AXIS2_PLACEMENT_3D('',#175842,#112299,#112300);
#97091=AXIS2_PLACEMENT_3D('',#176037,#112301,#112302);
#97092=AXIS2_PLACEMENT_3D('',#176225,#112303,#112304);
#97093=AXIS2_PLACEMENT_3D('',#176226,#112305,#112306);
#97094=AXIS2_PLACEMENT_3D('',#176227,#112307,#112308);
#97095=AXIS2_PLACEMENT_3D('',#176228,#112309,#112310);
#97096=AXIS2_PLACEMENT_3D('',#176229,#112311,#112312);
#97097=AXIS2_PLACEMENT_3D('',#176244,#112313,#112314);
#97098=AXIS2_PLACEMENT_3D('',#176245,#112315,#112316);
#97099=AXIS2_PLACEMENT_3D('',#176246,#112317,#112318);
#97100=AXIS2_PLACEMENT_3D('',#176247,#112319,#112320);
#97101=AXIS2_PLACEMENT_3D('',#176268,#112323,#112324);
#97102=AXIS2_PLACEMENT_3D('',#176270,#112325,#112326);
#97103=AXIS2_PLACEMENT_3D('',#176272,#112328,#112329);
#97104=AXIS2_PLACEMENT_3D('',#176305,#112331,#112332);
#97105=AXIS2_PLACEMENT_3D('',#176306,#112333,#112334);
#97106=AXIS2_PLACEMENT_3D('',#176307,#112335,#112336);
#97107=AXIS2_PLACEMENT_3D('',#176308,#112337,#112338);
#97108=AXIS2_PLACEMENT_3D('',#176309,#112339,#112340);
#97109=AXIS2_PLACEMENT_3D('',#176324,#112341,#112342);
#97110=AXIS2_PLACEMENT_3D('',#176325,#112343,#112344);
#97111=AXIS2_PLACEMENT_3D('',#176326,#112345,#112346);
#97112=AXIS2_PLACEMENT_3D('',#176327,#112347,#112348);
#97113=AXIS2_PLACEMENT_3D('',#176400,#112350,#112351);
#97114=AXIS2_PLACEMENT_3D('',#176402,#112352,#112353);
#97115=AXIS2_PLACEMENT_3D('',#176404,#112355,#112356);
#97116=AXIS2_PLACEMENT_3D('',#176407,#112358,#112359);
#97117=AXIS2_PLACEMENT_3D('',#176474,#112360,#112361);
#97118=AXIS2_PLACEMENT_3D('',#176475,#112362,#112363);
#97119=AXIS2_PLACEMENT_3D('',#176563,#112364,#112365);
#97120=AXIS2_PLACEMENT_3D('',#176565,#112366,#112367);
#97121=AXIS2_PLACEMENT_3D('',#176566,#112368,#112369);
#97122=AXIS2_PLACEMENT_3D('',#176646,#112370,#112371);
#97123=AXIS2_PLACEMENT_3D('',#176652,#112375,#112376);
#97124=AXIS2_PLACEMENT_3D('',#176654,#112377,#112378);
#97125=AXIS2_PLACEMENT_3D('',#176656,#112380,#112381);
#97126=AXIS2_PLACEMENT_3D('',#176658,#112382,#112383);
#97127=AXIS2_PLACEMENT_3D('',#176660,#112385,#112386);
#97128=AXIS2_PLACEMENT_3D('',#176662,#112387,#112388);
#97129=AXIS2_PLACEMENT_3D('',#176664,#112390,#112391);
#97130=AXIS2_PLACEMENT_3D('',#176668,#112394,#112395);
#97131=AXIS2_PLACEMENT_3D('',#176671,#112397,#112398);
#97132=AXIS2_PLACEMENT_3D('',#176672,#112399,#112400);
#97133=AXIS2_PLACEMENT_3D('',#176675,#112402,#112403);
#97134=AXIS2_PLACEMENT_3D('',#176676,#112404,#112405);
#97135=AXIS2_PLACEMENT_3D('',#176678,#112406,#112407);
#97136=AXIS2_PLACEMENT_3D('',#176680,#112409,#112410);
#97137=AXIS2_PLACEMENT_3D('',#176684,#112413,#112414);
#97138=AXIS2_PLACEMENT_3D('',#176686,#112415,#112416);
#97139=AXIS2_PLACEMENT_3D('',#176688,#112418,#112419);
#97140=AXIS2_PLACEMENT_3D('',#176690,#112420,#112421);
#97141=AXIS2_PLACEMENT_3D('',#176692,#112423,#112424);
#97142=AXIS2_PLACEMENT_3D('',#176694,#112425,#112426);
#97143=AXIS2_PLACEMENT_3D('',#176696,#112428,#112429);
#97144=AXIS2_PLACEMENT_3D('',#176749,#112434,#112435);
#97145=AXIS2_PLACEMENT_3D('',#176751,#112436,#112437);
#97146=AXIS2_PLACEMENT_3D('',#176846,#112438,#112439);
#97147=AXIS2_PLACEMENT_3D('',#176848,#112440,#112441);
#97148=AXIS2_PLACEMENT_3D('',#176881,#112443,#112444);
#97149=AXIS2_PLACEMENT_3D('',#176892,#112445,#112446);
#97150=AXIS2_PLACEMENT_3D('',#176894,#112447,#112448);
#97151=AXIS2_PLACEMENT_3D('',#176927,#112450,#112451);
#97152=AXIS2_PLACEMENT_3D('',#176977,#112452,#112453);
#97153=AXIS2_PLACEMENT_3D('',#176979,#112455,#112456);
#97154=AXIS2_PLACEMENT_3D('',#176984,#112459,#112460);
#97155=AXIS2_PLACEMENT_3D('',#176995,#112461,#112462);
#97156=AXIS2_PLACEMENT_3D('',#176997,#112463,#112464);
#97157=AXIS2_PLACEMENT_3D('',#176998,#112465,#112466);
#97158=AXIS2_PLACEMENT_3D('',#176999,#112467,#112468);
#97159=AXIS2_PLACEMENT_3D('',#177011,#112470,#112471);
#97160=AXIS2_PLACEMENT_3D('',#177013,#112472,#112473);
#97161=AXIS2_PLACEMENT_3D('',#177014,#112474,#112475);
#97162=AXIS2_PLACEMENT_3D('',#177015,#112476,#112477);
#97163=AXIS2_PLACEMENT_3D('',#177019,#112479,#112480);
#97164=AXIS2_PLACEMENT_3D('',#177021,#112482,#112483);
#97165=AXIS2_PLACEMENT_3D('',#177025,#112486,#112487);
#97166=AXIS2_PLACEMENT_3D('',#177027,#112488,#112489);
#97167=AXIS2_PLACEMENT_3D('',#177039,#112491,#112492);
#97168=AXIS2_PLACEMENT_3D('',#177041,#112493,#112494);
#97169=AXIS2_PLACEMENT_3D('',#177042,#112495,#112496);
#97170=AXIS2_PLACEMENT_3D('',#177043,#112497,#112498);
#97171=AXIS2_PLACEMENT_3D('',#177055,#112500,#112501);
#97172=AXIS2_PLACEMENT_3D('',#177057,#112502,#112503);
#97173=AXIS2_PLACEMENT_3D('',#177058,#112504,#112505);
#97174=AXIS2_PLACEMENT_3D('',#177059,#112506,#112507);
#97175=AXIS2_PLACEMENT_3D('',#177063,#112509,#112510);
#97176=AXIS2_PLACEMENT_3D('',#177065,#112512,#112513);
#97177=AXIS2_PLACEMENT_3D('',#177069,#112516,#112517);
#97178=AXIS2_PLACEMENT_3D('',#177071,#112518,#112519);
#97179=AXIS2_PLACEMENT_3D('',#177083,#112521,#112522);
#97180=AXIS2_PLACEMENT_3D('',#177085,#112523,#112524);
#97181=AXIS2_PLACEMENT_3D('',#177086,#112525,#112526);
#97182=AXIS2_PLACEMENT_3D('',#177087,#112527,#112528);
#97183=AXIS2_PLACEMENT_3D('',#177089,#112529,#112530);
#97184=AXIS2_PLACEMENT_3D('',#177312,#112532,#112533);
#97185=AXIS2_PLACEMENT_3D('',#177361,#112534,#112535);
#97186=AXIS2_PLACEMENT_3D('',#177362,#112536,#112537);
#97187=AXIS2_PLACEMENT_3D('',#177363,#112538,#112539);
#97188=AXIS2_PLACEMENT_3D('',#177364,#112540,#112541);
#97189=AXIS2_PLACEMENT_3D('',#177369,#112543,#112544);
#97190=AXIS2_PLACEMENT_3D('',#177372,#112546,#112547);
#97191=AXIS2_PLACEMENT_3D('',#177373,#112548,#112549);
#97192=AXIS2_PLACEMENT_3D('',#177378,#112552,#112553);
#97193=AXIS2_PLACEMENT_3D('',#177379,#112554,#112555);
#97194=AXIS2_PLACEMENT_3D('',#177381,#112556,#112557);
#97195=AXIS2_PLACEMENT_3D('',#177384,#112559,#112560);
#97196=AXIS2_PLACEMENT_3D('',#177457,#112561,#112562);
#97197=AXIS2_PLACEMENT_3D('',#177477,#112563,#112564);
#97198=AXIS2_PLACEMENT_3D('',#177515,#112565,#112566);
#97199=AXIS2_PLACEMENT_3D('',#177579,#112567,#112568);
#97200=AXIS2_PLACEMENT_3D('',#177586,#112569,#112570);
#97201=AXIS2_PLACEMENT_3D('',#177591,#112572,#112573);
#97202=AXIS2_PLACEMENT_3D('',#177594,#112575,#112576);
#97203=AXIS2_PLACEMENT_3D('',#177595,#112577,#112578);
#97204=AXIS2_PLACEMENT_3D('',#177604,#112581,#112582);
#97205=AXIS2_PLACEMENT_3D('',#177606,#112583,#112584);
#97206=AXIS2_PLACEMENT_3D('',#177609,#112586,#112587);
#97207=AXIS2_PLACEMENT_3D('',#177629,#112588,#112589);
#97208=AXIS2_PLACEMENT_3D('',#177631,#112590,#112591);
#97209=AXIS2_PLACEMENT_3D('',#177691,#112592,#112593);
#97210=AXIS2_PLACEMENT_3D('',#177726,#112594,#112595);
#97211=AXIS2_PLACEMENT_3D('',#177728,#112596,#112597);
#97212=AXIS2_PLACEMENT_3D('',#177731,#112600,#112601);
#97213=AXIS2_PLACEMENT_3D('',#177733,#112602,#112603);
#97214=AXIS2_PLACEMENT_3D('',#177734,#112604,#112605);
#97215=AXIS2_PLACEMENT_3D('',#177735,#112606,#112607);
#97216=AXIS2_PLACEMENT_3D('',#177819,#112608,#112609);
#97217=AXIS2_PLACEMENT_3D('',#177836,#112610,#112611);
#97218=AXIS2_PLACEMENT_3D('',#177840,#112614,#112615);
#97219=AXIS2_PLACEMENT_3D('',#177842,#112616,#112617);
#97220=AXIS2_PLACEMENT_3D('',#177844,#112619,#112620);
#97221=AXIS2_PLACEMENT_3D('',#177846,#112621,#112622);
#97222=AXIS2_PLACEMENT_3D('',#177848,#112623,#112624);
#97223=AXIS2_PLACEMENT_3D('',#177849,#112625,#112626);
#97224=AXIS2_PLACEMENT_3D('',#177850,#112627,#112628);
#97225=AXIS2_PLACEMENT_3D('',#177852,#112630,#112631);
#97226=AXIS2_PLACEMENT_3D('',#177856,#112633,#112634);
#97227=AXIS2_PLACEMENT_3D('',#177858,#112636,#112637);
#97228=AXIS2_PLACEMENT_3D('',#177860,#112638,#112639);
#97229=AXIS2_PLACEMENT_3D('',#177863,#112641,#112642);
#97230=AXIS2_PLACEMENT_3D('',#177864,#112643,#112644);
#97231=AXIS2_PLACEMENT_3D('',#177865,#112645,#112646);
#97232=AXIS2_PLACEMENT_3D('',#177867,#112647,#112648);
#97233=AXIS2_PLACEMENT_3D('',#177868,#112649,#112650);
#97234=AXIS2_PLACEMENT_3D('',#177870,#112651,#112652);
#97235=AXIS2_PLACEMENT_3D('',#177872,#112654,#112655);
#97236=AXIS2_PLACEMENT_3D('',#177875,#112656,#112657);
#97237=AXIS2_PLACEMENT_3D('',#177878,#112660,#112661);
#97238=AXIS2_PLACEMENT_3D('',#177880,#112662,#112663);
#97239=AXIS2_PLACEMENT_3D('',#177884,#112665,#112666);
#97240=AXIS2_PLACEMENT_3D('',#177896,#112668,#112669);
#97241=AXIS2_PLACEMENT_3D('',#177897,#112670,#112671);
#97242=AXIS2_PLACEMENT_3D('',#177898,#112672,#112673);
#97243=AXIS2_PLACEMENT_3D('',#177900,#112674,#112675);
#97244=AXIS2_PLACEMENT_3D('',#177901,#112676,#112677);
#97245=AXIS2_PLACEMENT_3D('',#177912,#112678,#112679);
#97246=AXIS2_PLACEMENT_3D('',#177913,#112680,#112681);
#97247=AXIS2_PLACEMENT_3D('',#177914,#112682,#112683);
#97248=AXIS2_PLACEMENT_3D('',#177917,#112686,#112687);
#97249=AXIS2_PLACEMENT_3D('',#177919,#112688,#112689);
#97250=AXIS2_PLACEMENT_3D('',#177921,#112691,#112692);
#97251=AXIS2_PLACEMENT_3D('',#177922,#112693,#112694);
#97252=AXIS2_PLACEMENT_3D('',#177924,#112695,#112696);
#97253=AXIS2_PLACEMENT_3D('',#177925,#112697,#112698);
#97254=AXIS2_PLACEMENT_3D('',#177927,#112699,#112700);
#97255=AXIS2_PLACEMENT_3D('',#177929,#112702,#112703);
#97256=AXIS2_PLACEMENT_3D('',#177933,#112705,#112706);
#97257=AXIS2_PLACEMENT_3D('',#177935,#112708,#112709);
#97258=AXIS2_PLACEMENT_3D('',#177938,#112711,#112712);
#97259=AXIS2_PLACEMENT_3D('',#177939,#112713,#112714);
#97260=AXIS2_PLACEMENT_3D('',#178059,#112717,#112718);
#97261=AXIS2_PLACEMENT_3D('',#178060,#112719,#112720);
#97262=AXIS2_PLACEMENT_3D('',#178061,#112721,#112722);
#97263=AXIS2_PLACEMENT_3D('',#178119,#112724,#112725);
#97264=AXIS2_PLACEMENT_3D('',#178123,#112728,#112729);
#97265=AXIS2_PLACEMENT_3D('',#178172,#112731,#112732);
#97266=AXIS2_PLACEMENT_3D('',#178219,#112734,#112735);
#97267=AXIS2_PLACEMENT_3D('',#178290,#112736,#112737);
#97268=AXIS2_PLACEMENT_3D('',#178324,#112739,#112740);
#97269=AXIS2_PLACEMENT_3D('',#178408,#112741,#112742);
#97270=AXIS2_PLACEMENT_3D('',#178412,#112745,#112746);
#97271=AXIS2_PLACEMENT_3D('',#178470,#112748,#112749);
#97272=AXIS2_PLACEMENT_3D('',#178474,#112752,#112753);
#97273=AXIS2_PLACEMENT_3D('',#178523,#112755,#112756);
#97274=AXIS2_PLACEMENT_3D('',#178567,#112758,#112759);
#97275=AXIS2_PLACEMENT_3D('',#178638,#112760,#112761);
#97276=AXIS2_PLACEMENT_3D('',#178693,#112764,#112765);
#97277=AXIS2_PLACEMENT_3D('',#178764,#112766,#112767);
#97278=AXIS2_PLACEMENT_3D('',#178820,#112768,#112769);
#97279=AXIS2_PLACEMENT_3D('',#178835,#112772,#112773);
#97280=AXIS2_PLACEMENT_3D('',#178887,#112775,#112776);
#97281=AXIS2_PLACEMENT_3D('',#178891,#112779,#112780);
#97282=AXIS2_PLACEMENT_3D('',#178946,#112782,#112783);
#97283=AXIS2_PLACEMENT_3D('',#178990,#112785,#112786);
#97284=AXIS2_PLACEMENT_3D('',#179067,#112787,#112788);
#97285=AXIS2_PLACEMENT_3D('',#179069,#112789,#112790);
#97286=AXIS2_PLACEMENT_3D('',#179071,#112792,#112793);
#97287=AXIS2_PLACEMENT_3D('',#179110,#112794,#112795);
#97288=AXIS2_PLACEMENT_3D('',#179125,#112796,#112797);
#97289=AXIS2_PLACEMENT_3D('',#179126,#112798,#112799);
#97290=AXIS2_PLACEMENT_3D('',#179170,#112800,#112801);
#97291=AXIS2_PLACEMENT_3D('',#179174,#112804,#112805);
#97292=AXIS2_PLACEMENT_3D('',#179290,#112808,#112809);
#97293=AXIS2_PLACEMENT_3D('',#179291,#112810,#112811);
#97294=AXIS2_PLACEMENT_3D('',#179343,#112813,#112814);
#97295=AXIS2_PLACEMENT_3D('',#179347,#112817,#112818);
#97296=AXIS2_PLACEMENT_3D('',#179402,#112820,#112821);
#97297=AXIS2_PLACEMENT_3D('',#179516,#112823,#112824);
#97298=AXIS2_PLACEMENT_3D('',#179548,#112825,#112826);
#97299=AXIS2_PLACEMENT_3D('',#179625,#112827,#112828);
#97300=AXIS2_PLACEMENT_3D('',#179627,#112830,#112831);
#97301=AXIS2_PLACEMENT_3D('',#179643,#112835,#112836);
#97302=AXIS2_PLACEMENT_3D('',#179701,#112838,#112839);
#97303=AXIS2_PLACEMENT_3D('',#179705,#112842,#112843);
#97304=AXIS2_PLACEMENT_3D('',#179754,#112845,#112846);
#97305=AXIS2_PLACEMENT_3D('',#179801,#112848,#112849);
#97306=AXIS2_PLACEMENT_3D('',#179910,#112850,#112851);
#97307=AXIS2_PLACEMENT_3D('',#180021,#112852,#112853);
#97308=AXIS2_PLACEMENT_3D('',#180026,#112857,#112858);
#97309=AXIS2_PLACEMENT_3D('',#180084,#112860,#112861);
#97310=AXIS2_PLACEMENT_3D('',#180088,#112864,#112865);
#97311=AXIS2_PLACEMENT_3D('',#180137,#112867,#112868);
#97312=AXIS2_PLACEMENT_3D('',#180182,#112871,#112872);
#97313=AXIS2_PLACEMENT_3D('',#180287,#112873,#112874);
#97314=AXIS2_PLACEMENT_3D('',#180358,#112875,#112876);
#97315=AXIS2_PLACEMENT_3D('',#180360,#112878,#112879);
#97316=AXIS2_PLACEMENT_3D('',#180375,#112882,#112883);
#97317=AXIS2_PLACEMENT_3D('',#180427,#112885,#112886);
#97318=AXIS2_PLACEMENT_3D('',#180431,#112889,#112890);
#97319=AXIS2_PLACEMENT_3D('',#180486,#112892,#112893);
#97320=AXIS2_PLACEMENT_3D('',#180530,#112895,#112896);
#97321=AXIS2_PLACEMENT_3D('',#180607,#112897,#112898);
#97322=AXIS2_PLACEMENT_3D('',#180609,#112899,#112900);
#97323=AXIS2_PLACEMENT_3D('',#180611,#112902,#112903);
#97324=AXIS2_PLACEMENT_3D('',#180633,#112904,#112905);
#97325=AXIS2_PLACEMENT_3D('',#180704,#112908,#112909);
#97326=AXIS2_PLACEMENT_3D('',#180737,#112910,#112911);
#97327=AXIS2_PLACEMENT_3D('',#180818,#112912,#112913);
#97328=AXIS2_PLACEMENT_3D('',#180822,#112916,#112917);
#97329=AXIS2_PLACEMENT_3D('',#180874,#112919,#112920);
#97330=AXIS2_PLACEMENT_3D('',#180878,#112923,#112924);
#97331=AXIS2_PLACEMENT_3D('',#180933,#112926,#112927);
#97332=AXIS2_PLACEMENT_3D('',#181047,#112929,#112930);
#97333=AXIS2_PLACEMENT_3D('',#181079,#112931,#112932);
#97334=AXIS2_PLACEMENT_3D('',#181156,#112933,#112934);
#97335=AXIS2_PLACEMENT_3D('',#181158,#112936,#112937);
#97336=AXIS2_PLACEMENT_3D('',#181163,#112940,#112941);
#97337=AXIS2_PLACEMENT_3D('',#181177,#112942,#112943);
#97338=AXIS2_PLACEMENT_3D('',#181178,#112944,#112945);
#97339=AXIS2_PLACEMENT_3D('',#181179,#112946,#112947);
#97340=AXIS2_PLACEMENT_3D('',#181180,#112948,#112949);
#97341=AXIS2_PLACEMENT_3D('',#181181,#112950,#112951);
#97342=AXIS2_PLACEMENT_3D('',#181183,#112952,#112953);
#97343=AXIS2_PLACEMENT_3D('',#181200,#112956,#112957);
#97344=AXIS2_PLACEMENT_3D('',#181201,#112958,#112959);
#97345=AXIS2_PLACEMENT_3D('',#181202,#112960,#112961);
#97346=AXIS2_PLACEMENT_3D('',#181223,#112963,#112964);
#97347=AXIS2_PLACEMENT_3D('',#181225,#112965,#112966);
#97348=AXIS2_PLACEMENT_3D('',#181227,#112968,#112969);
#97349=AXIS2_PLACEMENT_3D('',#181282,#112971,#112972);
#97350=AXIS2_PLACEMENT_3D('',#181285,#112974,#112975);
#97351=AXIS2_PLACEMENT_3D('',#181299,#112976,#112977);
#97352=AXIS2_PLACEMENT_3D('',#181300,#112978,#112979);
#97353=AXIS2_PLACEMENT_3D('',#181301,#112980,#112981);
#97354=AXIS2_PLACEMENT_3D('',#181302,#112982,#112983);
#97355=AXIS2_PLACEMENT_3D('',#181303,#112984,#112985);
#97356=AXIS2_PLACEMENT_3D('',#181305,#112986,#112987);
#97357=AXIS2_PLACEMENT_3D('',#181358,#112989,#112990);
#97358=AXIS2_PLACEMENT_3D('',#181359,#112991,#112992);
#97359=AXIS2_PLACEMENT_3D('',#181460,#112993,#112994);
#97360=AXIS2_PLACEMENT_3D('',#181729,#112995,#112996);
#97361=AXIS2_PLACEMENT_3D('',#181732,#112998,#112999);
#97362=AXIS2_PLACEMENT_3D('',#181746,#113000,#113001);
#97363=AXIS2_PLACEMENT_3D('',#181747,#113002,#113003);
#97364=AXIS2_PLACEMENT_3D('',#181748,#113004,#113005);
#97365=AXIS2_PLACEMENT_3D('',#181749,#113006,#113007);
#97366=AXIS2_PLACEMENT_3D('',#181750,#113008,#113009);
#97367=AXIS2_PLACEMENT_3D('',#181752,#113010,#113011);
#97368=AXIS2_PLACEMENT_3D('',#181796,#113013,#113014);
#97369=AXIS2_PLACEMENT_3D('',#181797,#113015,#113016);
#97370=AXIS2_PLACEMENT_3D('',#181955,#113017,#113018);
#97371=AXIS2_PLACEMENT_3D('',#182146,#113019,#113020);
#97372=AXIS2_PLACEMENT_3D('',#182149,#113022,#113023);
#97373=AXIS2_PLACEMENT_3D('',#182163,#113024,#113025);
#97374=AXIS2_PLACEMENT_3D('',#182164,#113026,#113027);
#97375=AXIS2_PLACEMENT_3D('',#182165,#113028,#113029);
#97376=AXIS2_PLACEMENT_3D('',#182166,#113030,#113031);
#97377=AXIS2_PLACEMENT_3D('',#182167,#113032,#113033);
#97378=AXIS2_PLACEMENT_3D('',#182169,#113034,#113035);
#97379=AXIS2_PLACEMENT_3D('',#182222,#113037,#113038);
#97380=AXIS2_PLACEMENT_3D('',#182223,#113039,#113040);
#97381=AXIS2_PLACEMENT_3D('',#182386,#113041,#113042);
#97382=AXIS2_PLACEMENT_3D('',#182578,#113043,#113044);
#97383=AXIS2_PLACEMENT_3D('',#182581,#113046,#113047);
#97384=AXIS2_PLACEMENT_3D('',#182595,#113048,#113049);
#97385=AXIS2_PLACEMENT_3D('',#182596,#113050,#113051);
#97386=AXIS2_PLACEMENT_3D('',#182597,#113052,#113053);
#97387=AXIS2_PLACEMENT_3D('',#182598,#113054,#113055);
#97388=AXIS2_PLACEMENT_3D('',#182599,#113056,#113057);
#97389=AXIS2_PLACEMENT_3D('',#182601,#113058,#113059);
#97390=AXIS2_PLACEMENT_3D('',#182618,#113062,#113063);
#97391=AXIS2_PLACEMENT_3D('',#182619,#113064,#113065);
#97392=AXIS2_PLACEMENT_3D('',#182620,#113066,#113067);
#97393=AXIS2_PLACEMENT_3D('',#182672,#113069,#113070);
#97394=AXIS2_PLACEMENT_3D('',#182674,#113071,#113072);
#97395=AXIS2_PLACEMENT_3D('',#182676,#113074,#113075);
#97396=AXIS2_PLACEMENT_3D('',#182755,#113077,#113078);
#97397=AXIS2_PLACEMENT_3D('',#182758,#113080,#113081);
#97398=AXIS2_PLACEMENT_3D('',#182772,#113082,#113083);
#97399=AXIS2_PLACEMENT_3D('',#182773,#113084,#113085);
#97400=AXIS2_PLACEMENT_3D('',#182774,#113086,#113087);
#97401=AXIS2_PLACEMENT_3D('',#182775,#113088,#113089);
#97402=AXIS2_PLACEMENT_3D('',#182790,#113090,#113091);
#97403=AXIS2_PLACEMENT_3D('',#182791,#113092,#113093);
#97404=AXIS2_PLACEMENT_3D('',#182805,#113094,#113095);
#97405=AXIS2_PLACEMENT_3D('',#182809,#113098,#113099);
#97406=AXIS2_PLACEMENT_3D('',#182860,#113101,#113102);
#97407=AXIS2_PLACEMENT_3D('',#182862,#113103,#113104);
#97408=AXIS2_PLACEMENT_3D('',#182864,#113106,#113107);
#97409=AXIS2_PLACEMENT_3D('',#182879,#113108,#113109);
#97410=AXIS2_PLACEMENT_3D('',#182880,#113110,#113111);
#97411=AXIS2_PLACEMENT_3D('',#182882,#113112,#113113);
#97412=AXIS2_PLACEMENT_3D('',#182919,#113115,#113116);
#97413=AXIS2_PLACEMENT_3D('',#182921,#113117,#113118);
#97414=AXIS2_PLACEMENT_3D('',#182923,#113120,#113121);
#97415=AXIS2_PLACEMENT_3D('',#182978,#113122,#113123);
#97416=AXIS2_PLACEMENT_3D('',#182981,#113124,#113125);
#97417=AXIS2_PLACEMENT_3D('',#183224,#113128,#113129);
#97418=AXIS2_PLACEMENT_3D('',#183457,#113130,#113131);
#97419=AXIS2_PLACEMENT_3D('',#183460,#113133,#113134);
#97420=AXIS2_PLACEMENT_3D('',#183475,#113136,#113137);
#97421=AXIS2_PLACEMENT_3D('',#183476,#113138,#113139);
#97422=AXIS2_PLACEMENT_3D('',#183477,#113140,#113141);
#97423=AXIS2_PLACEMENT_3D('',#183478,#113142,#113143);
#97424=AXIS2_PLACEMENT_3D('',#183479,#113144,#113145);
#97425=AXIS2_PLACEMENT_3D('',#183480,#113146,#113147);
#97426=AXIS2_PLACEMENT_3D('',#183482,#113148,#113149);
#97427=AXIS2_PLACEMENT_3D('',#183560,#113152,#113153);
#97428=AXIS2_PLACEMENT_3D('',#183561,#113154,#113155);
#97429=AXIS2_PLACEMENT_3D('',#183782,#113156,#113157);
#97430=AXIS2_PLACEMENT_3D('',#184036,#113158,#113159);
#97431=AXIS2_PLACEMENT_3D('',#184039,#113161,#113162);
#97432=AXIS2_PLACEMENT_3D('',#184054,#113164,#113165);
#97433=AXIS2_PLACEMENT_3D('',#184055,#113166,#113167);
#97434=AXIS2_PLACEMENT_3D('',#184056,#113168,#113169);
#97435=AXIS2_PLACEMENT_3D('',#184057,#113170,#113171);
#97436=AXIS2_PLACEMENT_3D('',#184072,#113172,#113173);
#97437=AXIS2_PLACEMENT_3D('',#184073,#113174,#113175);
#97438=AXIS2_PLACEMENT_3D('',#184074,#113176,#113177);
#97439=AXIS2_PLACEMENT_3D('',#184075,#113178,#113179);
#97440=AXIS2_PLACEMENT_3D('',#184080,#113183,#113184);
#97441=AXIS2_PLACEMENT_3D('',#184165,#113186,#113187);
#97442=AXIS2_PLACEMENT_3D('',#184167,#113188,#113189);
#97443=AXIS2_PLACEMENT_3D('',#184169,#113191,#113192);
#97444=AXIS2_PLACEMENT_3D('',#184188,#113194,#113195);
#97445=AXIS2_PLACEMENT_3D('',#184191,#113197,#113198);
#97446=AXIS2_PLACEMENT_3D('',#184206,#113200,#113201);
#97447=AXIS2_PLACEMENT_3D('',#184223,#113202,#113203);
#97448=AXIS2_PLACEMENT_3D('',#184225,#113204,#113205);
#97449=AXIS2_PLACEMENT_3D('',#184292,#113206,#113207);
#97450=AXIS2_PLACEMENT_3D('',#184367,#113210,#113211);
#97451=AXIS2_PLACEMENT_3D('',#184370,#113213,#113214);
#97452=AXIS2_PLACEMENT_3D('',#184385,#113216,#113217);
#97453=AXIS2_PLACEMENT_3D('',#184386,#113218,#113219);
#97454=AXIS2_PLACEMENT_3D('',#184387,#113220,#113221);
#97455=AXIS2_PLACEMENT_3D('',#184388,#113222,#113223);
#97456=AXIS2_PLACEMENT_3D('',#184389,#113224,#113225);
#97457=AXIS2_PLACEMENT_3D('',#184392,#113227,#113228);
#97458=AXIS2_PLACEMENT_3D('',#184409,#113231,#113232);
#97459=AXIS2_PLACEMENT_3D('',#184410,#113233,#113234);
#97460=AXIS2_PLACEMENT_3D('',#184411,#113235,#113236);
#97461=AXIS2_PLACEMENT_3D('',#184432,#113238,#113239);
#97462=AXIS2_PLACEMENT_3D('',#184434,#113240,#113241);
#97463=AXIS2_PLACEMENT_3D('',#184436,#113243,#113244);
#97464=AXIS2_PLACEMENT_3D('',#184491,#113246,#113247);
#97465=AXIS2_PLACEMENT_3D('',#184494,#113249,#113250);
#97466=AXIS2_PLACEMENT_3D('',#184509,#113252,#113253);
#97467=AXIS2_PLACEMENT_3D('',#184511,#113254,#113255);
#97468=AXIS2_PLACEMENT_3D('',#184512,#113256,#113257);
#97469=AXIS2_PLACEMENT_3D('',#184513,#113258,#113259);
#97470=AXIS2_PLACEMENT_3D('',#184514,#113260,#113261);
#97471=AXIS2_PLACEMENT_3D('',#184515,#113262,#113263);
#97472=AXIS2_PLACEMENT_3D('',#184518,#113265,#113266);
#97473=AXIS2_PLACEMENT_3D('',#184580,#113268,#113269);
#97474=AXIS2_PLACEMENT_3D('',#184581,#113270,#113271);
#97475=AXIS2_PLACEMENT_3D('',#184778,#113272,#113273);
#97476=AXIS2_PLACEMENT_3D('',#185011,#113274,#113275);
#97477=AXIS2_PLACEMENT_3D('',#185014,#113277,#113278);
#97478=AXIS2_PLACEMENT_3D('',#185029,#113280,#113281);
#97479=AXIS2_PLACEMENT_3D('',#185031,#113282,#113283);
#97480=AXIS2_PLACEMENT_3D('',#185032,#113284,#113285);
#97481=AXIS2_PLACEMENT_3D('',#185033,#113286,#113287);
#97482=AXIS2_PLACEMENT_3D('',#185034,#113288,#113289);
#97483=AXIS2_PLACEMENT_3D('',#185035,#113290,#113291);
#97484=AXIS2_PLACEMENT_3D('',#185068,#113293,#113294);
#97485=AXIS2_PLACEMENT_3D('',#185123,#113297,#113298);
#97486=AXIS2_PLACEMENT_3D('',#185124,#113299,#113300);
#97487=AXIS2_PLACEMENT_3D('',#185270,#113301,#113302);
#97488=AXIS2_PLACEMENT_3D('',#185271,#113303,#113304);
#97489=AXIS2_PLACEMENT_3D('',#185273,#113305,#113306);
#97490=AXIS2_PLACEMENT_3D('',#185419,#113308,#113309);
#97491=AXIS2_PLACEMENT_3D('',#185421,#113310,#113311);
#97492=AXIS2_PLACEMENT_3D('',#185423,#113312,#113313);
#97493=AXIS2_PLACEMENT_3D('',#185424,#113314,#113315);
#97494=AXIS2_PLACEMENT_3D('',#185468,#113316,#113317);
#97495=AXIS2_PLACEMENT_3D('',#185471,#113319,#113320);
#97496=AXIS2_PLACEMENT_3D('',#185503,#113321,#113322);
#97497=AXIS2_PLACEMENT_3D('',#185523,#113323,#113324);
#97498=AXIS2_PLACEMENT_3D('',#185524,#113325,#113326);
#97499=AXIS2_PLACEMENT_3D('',#185526,#113328,#113329);
#97500=AXIS2_PLACEMENT_3D('',#185527,#113330,#113331);
#97501=AXIS2_PLACEMENT_3D('',#185528,#113332,#113333);
#97502=AXIS2_PLACEMENT_3D('',#185530,#113334,#113335);
#97503=AXIS2_PLACEMENT_3D('',#185563,#113337,#113338);
#97504=AXIS2_PLACEMENT_3D('',#185629,#113339,#113340);
#97505=AXIS2_PLACEMENT_3D('',#185630,#113341,#113342);
#97506=AXIS2_PLACEMENT_3D('',#185681,#113343,#113344);
#97507=AXIS2_PLACEMENT_3D('',#185682,#113345,#113346);
#97508=AXIS2_PLACEMENT_3D('',#185684,#113348,#113349);
#97509=AXIS2_PLACEMENT_3D('',#185685,#113350,#113351);
#97510=AXIS2_PLACEMENT_3D('',#185686,#113352,#113353);
#97511=AXIS2_PLACEMENT_3D('',#185688,#113354,#113355);
#97512=AXIS2_PLACEMENT_3D('',#185709,#113357,#113358);
#97513=AXIS2_PLACEMENT_3D('',#185732,#113359,#113360);
#97514=AXIS2_PLACEMENT_3D('',#185734,#113361,#113362);
#97515=AXIS2_PLACEMENT_3D('',#185735,#113363,#113364);
#97516=AXIS2_PLACEMENT_3D('',#185813,#113365,#113366);
#97517=AXIS2_PLACEMENT_3D('',#185814,#113367,#113368);
#97518=AXIS2_PLACEMENT_3D('',#185816,#113370,#113371);
#97519=AXIS2_PLACEMENT_3D('',#185817,#113372,#113373);
#97520=AXIS2_PLACEMENT_3D('',#185818,#113374,#113375);
#97521=AXIS2_PLACEMENT_3D('',#185820,#113376,#113377);
#97522=AXIS2_PLACEMENT_3D('',#185895,#113379,#113380);
#97523=AXIS2_PLACEMENT_3D('',#185898,#113382,#113383);
#97524=AXIS2_PLACEMENT_3D('',#185899,#113384,#113385);
#97525=AXIS2_PLACEMENT_3D('',#185902,#113387,#113388);
#97526=AXIS2_PLACEMENT_3D('',#185903,#113389,#113390);
#97527=AXIS2_PLACEMENT_3D('',#185905,#113391,#113392);
#97528=AXIS2_PLACEMENT_3D('',#185907,#113393,#113394);
#97529=AXIS2_PLACEMENT_3D('',#185908,#113395,#113396);
#97530=AXIS2_PLACEMENT_3D('',#185909,#113397,#113398);
#97531=AXIS2_PLACEMENT_3D('',#185912,#113400,#113401);
#97532=AXIS2_PLACEMENT_3D('',#185913,#113402,#113403);
#97533=AXIS2_PLACEMENT_3D('',#185915,#113404,#113405);
#97534=AXIS2_PLACEMENT_3D('',#185916,#113406,#113407);
#97535=AXIS2_PLACEMENT_3D('',#185917,#113408,#113409);
#97536=AXIS2_PLACEMENT_3D('',#185919,#113410,#113411);
#97537=AXIS2_PLACEMENT_3D('',#185920,#113412,#113413);
#97538=AXIS2_PLACEMENT_3D('',#185921,#113414,#113415);
#97539=AXIS2_PLACEMENT_3D('',#185923,#113416,#113417);
#97540=AXIS2_PLACEMENT_3D('',#185924,#113418,#113419);
#97541=AXIS2_PLACEMENT_3D('',#185925,#113420,#113421);
#97542=AXIS2_PLACEMENT_3D('',#185928,#113423,#113424);
#97543=AXIS2_PLACEMENT_3D('',#185929,#113425,#113426);
#97544=AXIS2_PLACEMENT_3D('',#185931,#113427,#113428);
#97545=AXIS2_PLACEMENT_3D('',#185932,#113429,#113430);
#97546=AXIS2_PLACEMENT_3D('',#185933,#113431,#113432);
#97547=AXIS2_PLACEMENT_3D('',#185935,#113433,#113434);
#97548=AXIS2_PLACEMENT_3D('',#185936,#113435,#113436);
#97549=AXIS2_PLACEMENT_3D('',#185937,#113437,#113438);
#97550=AXIS2_PLACEMENT_3D('',#185939,#113439,#113440);
#97551=AXIS2_PLACEMENT_3D('',#185940,#113441,#113442);
#97552=AXIS2_PLACEMENT_3D('',#185941,#113443,#113444);
#97553=AXIS2_PLACEMENT_3D('',#185944,#113446,#113447);
#97554=AXIS2_PLACEMENT_3D('',#185945,#113448,#113449);
#97555=AXIS2_PLACEMENT_3D('',#185947,#113450,#113451);
#97556=AXIS2_PLACEMENT_3D('',#185948,#113452,#113453);
#97557=AXIS2_PLACEMENT_3D('',#185949,#113454,#113455);
#97558=AXIS2_PLACEMENT_3D('',#185951,#113456,#113457);
#97559=AXIS2_PLACEMENT_3D('',#185952,#113458,#113459);
#97560=AXIS2_PLACEMENT_3D('',#185953,#113460,#113461);
#97561=AXIS2_PLACEMENT_3D('',#185955,#113462,#113463);
#97562=AXIS2_PLACEMENT_3D('',#185956,#113464,#113465);
#97563=AXIS2_PLACEMENT_3D('',#185957,#113466,#113467);
#97564=AXIS2_PLACEMENT_3D('',#185960,#113469,#113470);
#97565=AXIS2_PLACEMENT_3D('',#185961,#113471,#113472);
#97566=AXIS2_PLACEMENT_3D('',#185963,#113473,#113474);
#97567=AXIS2_PLACEMENT_3D('',#185965,#113475,#113476);
#97568=AXIS2_PLACEMENT_3D('',#185966,#113477,#113478);
#97569=AXIS2_PLACEMENT_3D('',#185967,#113479,#113480);
#97570=AXIS2_PLACEMENT_3D('',#185970,#113482,#113483);
#97571=AXIS2_PLACEMENT_3D('',#185971,#113484,#113485);
#97572=AXIS2_PLACEMENT_3D('',#185973,#113486,#113487);
#97573=AXIS2_PLACEMENT_3D('',#185975,#113489,#113490);
#97574=AXIS2_PLACEMENT_3D('',#185977,#113491,#113492);
#97575=AXIS2_PLACEMENT_3D('',#185978,#113493,#113494);
#97576=AXIS2_PLACEMENT_3D('',#185979,#113495,#113496);
#97577=AXIS2_PLACEMENT_3D('',#185984,#113499,#113500);
#97578=AXIS2_PLACEMENT_3D('',#185985,#113501,#113502);
#97579=AXIS2_PLACEMENT_3D('',#185989,#113505,#113506);
#97580=AXIS2_PLACEMENT_3D('',#185991,#113507,#113508);
#97581=AXIS2_PLACEMENT_3D('',#185993,#113510,#113511);
#97582=AXIS2_PLACEMENT_3D('',#185995,#113513,#113514);
#97583=AXIS2_PLACEMENT_3D('',#185997,#113515,#113516);
#97584=AXIS2_PLACEMENT_3D('',#185999,#113518,#113519);
#97585=AXIS2_PLACEMENT_3D('',#186001,#113520,#113521);
#97586=AXIS2_PLACEMENT_3D('',#186002,#113522,#113523);
#97587=AXIS2_PLACEMENT_3D('',#186003,#113524,#113525);
#97588=AXIS2_PLACEMENT_3D('',#186005,#113526,#113527);
#97589=AXIS2_PLACEMENT_3D('',#186007,#113529,#113530);
#97590=AXIS2_PLACEMENT_3D('',#186009,#113531,#113532);
#97591=AXIS2_PLACEMENT_3D('',#186010,#113533,#113534);
#97592=AXIS2_PLACEMENT_3D('',#186011,#113535,#113536);
#97593=AXIS2_PLACEMENT_3D('',#186013,#113538,#113539);
#97594=AXIS2_PLACEMENT_3D('',#186015,#113541,#113542);
#97595=AXIS2_PLACEMENT_3D('',#186017,#113543,#113544);
#97596=AXIS2_PLACEMENT_3D('',#186019,#113546,#113547);
#97597=AXIS2_PLACEMENT_3D('',#186021,#113548,#113549);
#97598=AXIS2_PLACEMENT_3D('',#186022,#113550,#113551);
#97599=AXIS2_PLACEMENT_3D('',#186023,#113552,#113553);
#97600=AXIS2_PLACEMENT_3D('',#186025,#113554,#113555);
#97601=AXIS2_PLACEMENT_3D('',#186027,#113557,#113558);
#97602=AXIS2_PLACEMENT_3D('',#186029,#113559,#113560);
#97603=AXIS2_PLACEMENT_3D('',#186030,#113561,#113562);
#97604=AXIS2_PLACEMENT_3D('',#186031,#113563,#113564);
#97605=AXIS2_PLACEMENT_3D('',#186033,#113566,#113567);
#97606=AXIS2_PLACEMENT_3D('',#186036,#113569,#113570);
#97607=AXIS2_PLACEMENT_3D('',#186056,#113571,#113572);
#97608=AXIS2_PLACEMENT_3D('',#186063,#113573,#113574);
#97609=AXIS2_PLACEMENT_3D('',#186064,#113575,#113576);
#97610=AXIS2_PLACEMENT_3D('',#186065,#113577,#113578);
#97611=AXIS2_PLACEMENT_3D('',#186067,#113579,#113580);
#97612=AXIS2_PLACEMENT_3D('',#186069,#113582,#113583);
#97613=AXIS2_PLACEMENT_3D('',#186071,#113584,#113585);
#97614=AXIS2_PLACEMENT_3D('',#186072,#113586,#113587);
#97615=AXIS2_PLACEMENT_3D('',#186073,#113588,#113589);
#97616=AXIS2_PLACEMENT_3D('',#186075,#113590,#113591);
#97617=AXIS2_PLACEMENT_3D('',#186077,#113593,#113594);
#97618=AXIS2_PLACEMENT_3D('',#186079,#113595,#113596);
#97619=AXIS2_PLACEMENT_3D('',#186080,#113597,#113598);
#97620=AXIS2_PLACEMENT_3D('',#186081,#113599,#113600);
#97621=AXIS2_PLACEMENT_3D('',#186083,#113602,#113603);
#97622=AXIS2_PLACEMENT_3D('',#186084,#113604,#113605);
#97623=AXIS2_PLACEMENT_3D('',#186085,#113606,#113607);
#97624=AXIS2_PLACEMENT_3D('',#186087,#113608,#113609);
#97625=AXIS2_PLACEMENT_3D('',#186089,#113611,#113612);
#97626=AXIS2_PLACEMENT_3D('',#186091,#113613,#113614);
#97627=AXIS2_PLACEMENT_3D('',#186092,#113615,#113616);
#97628=AXIS2_PLACEMENT_3D('',#186093,#113617,#113618);
#97629=AXIS2_PLACEMENT_3D('',#186095,#113619,#113620);
#97630=AXIS2_PLACEMENT_3D('',#186097,#113622,#113623);
#97631=AXIS2_PLACEMENT_3D('',#186099,#113624,#113625);
#97632=AXIS2_PLACEMENT_3D('',#186100,#113626,#113627);
#97633=AXIS2_PLACEMENT_3D('',#186101,#113628,#113629);
#97634=AXIS2_PLACEMENT_3D('',#186103,#113630,#113631);
#97635=AXIS2_PLACEMENT_3D('',#186105,#113633,#113634);
#97636=AXIS2_PLACEMENT_3D('',#186107,#113635,#113636);
#97637=AXIS2_PLACEMENT_3D('',#186109,#113638,#113639);
#97638=AXIS2_PLACEMENT_3D('',#186111,#113640,#113641);
#97639=AXIS2_PLACEMENT_3D('',#186113,#113643,#113644);
#97640=AXIS2_PLACEMENT_3D('',#186114,#113645,#113646);
#97641=AXIS2_PLACEMENT_3D('',#186158,#113647,#113648);
#97642=AXIS2_PLACEMENT_3D('',#186233,#113649,#113650);
#97643=AXIS2_PLACEMENT_3D('',#186247,#113651,#113652);
#97644=AXIS2_PLACEMENT_3D('',#186271,#113653,#113654);
#97645=AXIS2_PLACEMENT_3D('',#186272,#113655,#113656);
#97646=AXIS2_PLACEMENT_3D('',#186273,#113657,#113658);
#97647=AXIS2_PLACEMENT_3D('',#186327,#113660,#113661);
#97648=AXIS2_PLACEMENT_3D('',#186329,#113662,#113663);
#97649=AXIS2_PLACEMENT_3D('',#186330,#113664,#113665);
#97650=AXIS2_PLACEMENT_3D('',#186331,#113666,#113667);
#97651=AXIS2_PLACEMENT_3D('',#186337,#113670,#113671);
#97652=AXIS2_PLACEMENT_3D('',#186340,#113673,#113674);
#97653=AXIS2_PLACEMENT_3D('',#186341,#113675,#113676);
#97654=AXIS2_PLACEMENT_3D('',#186347,#113679,#113680);
#97655=AXIS2_PLACEMENT_3D('',#186350,#113682,#113683);
#97656=AXIS2_PLACEMENT_3D('',#186351,#113684,#113685);
#97657=AXIS2_PLACEMENT_3D('',#186354,#113687,#113688);
#97658=AXIS2_PLACEMENT_3D('',#186355,#113689,#113690);
#97659=AXIS2_PLACEMENT_3D('',#186357,#113691,#113692);
#97660=AXIS2_PLACEMENT_3D('',#186360,#113694,#113695);
#97661=AXIS2_PLACEMENT_3D('',#186380,#113696,#113697);
#97662=AXIS2_PLACEMENT_3D('',#186388,#113698,#113699);
#97663=AXIS2_PLACEMENT_3D('',#186390,#113700,#113701);
#97664=AXIS2_PLACEMENT_3D('',#186411,#113703,#113704);
#97665=AXIS2_PLACEMENT_3D('',#186419,#113705,#113706);
#97666=AXIS2_PLACEMENT_3D('',#186421,#113708,#113709);
#97667=AXIS2_PLACEMENT_3D('',#186423,#113711,#113712);
#97668=AXIS2_PLACEMENT_3D('',#186425,#113713,#113714);
#97669=AXIS2_PLACEMENT_3D('',#186446,#113716,#113717);
#97670=AXIS2_PLACEMENT_3D('',#186454,#113718,#113719);
#97671=AXIS2_PLACEMENT_3D('',#186456,#113720,#113721);
#97672=AXIS2_PLACEMENT_3D('',#186477,#113723,#113724);
#97673=AXIS2_PLACEMENT_3D('',#186485,#113725,#113726);
#97674=AXIS2_PLACEMENT_3D('',#186487,#113728,#113729);
#97675=AXIS2_PLACEMENT_3D('',#186490,#113731,#113732);
#97676=AXIS2_PLACEMENT_3D('',#186504,#113733,#113734);
#97677=AXIS2_PLACEMENT_3D('',#186506,#113735,#113736);
#97678=AXIS2_PLACEMENT_3D('',#186507,#113737,#113738);
#97679=AXIS2_PLACEMENT_3D('',#186508,#113739,#113740);
#97680=AXIS2_PLACEMENT_3D('',#186547,#113742,#113743);
#97681=AXIS2_PLACEMENT_3D('',#186550,#113745,#113746);
#97682=AXIS2_PLACEMENT_3D('',#186570,#113747,#113748);
#97683=AXIS2_PLACEMENT_3D('',#186578,#113749,#113750);
#97684=AXIS2_PLACEMENT_3D('',#186580,#113751,#113752);
#97685=AXIS2_PLACEMENT_3D('',#186601,#113754,#113755);
#97686=AXIS2_PLACEMENT_3D('',#186609,#113756,#113757);
#97687=AXIS2_PLACEMENT_3D('',#186611,#113759,#113760);
#97688=AXIS2_PLACEMENT_3D('',#186614,#113762,#113763);
#97689=AXIS2_PLACEMENT_3D('',#186652,#113764,#113765);
#97690=AXIS2_PLACEMENT_3D('',#186654,#113766,#113767);
#97691=AXIS2_PLACEMENT_3D('',#186669,#113769,#113770);
#97692=AXIS2_PLACEMENT_3D('',#186670,#113771,#113772);
#97693=AXIS2_PLACEMENT_3D('',#186671,#113773,#113774);
#97694=AXIS2_PLACEMENT_3D('',#186674,#113776,#113777);
#97695=AXIS2_PLACEMENT_3D('',#186675,#113778,#113779);
#97696=AXIS2_PLACEMENT_3D('',#186678,#113781,#113782);
#97697=AXIS2_PLACEMENT_3D('',#186705,#113783,#113784);
#97698=AXIS2_PLACEMENT_3D('',#186706,#113785,#113786);
#97699=AXIS2_PLACEMENT_3D('',#186709,#113788,#113789);
#97700=AXIS2_PLACEMENT_3D('',#186736,#113790,#113791);
#97701=AXIS2_PLACEMENT_3D('',#186737,#113792,#113793);
#97702=AXIS2_PLACEMENT_3D('',#186739,#113795,#113796);
#97703=AXIS2_PLACEMENT_3D('',#186741,#113798,#113799);
#97704=AXIS2_PLACEMENT_3D('',#186743,#113800,#113801);
#97705=AXIS2_PLACEMENT_3D('',#186745,#113802,#113803);
#97706=AXIS2_PLACEMENT_3D('',#186747,#113805,#113806);
#97707=AXIS2_PLACEMENT_3D('',#186749,#113807,#113808);
#97708=AXIS2_PLACEMENT_3D('',#186770,#113810,#113811);
#97709=AXIS2_PLACEMENT_3D('',#186778,#113812,#113813);
#97710=AXIS2_PLACEMENT_3D('',#186780,#113814,#113815);
#97711=AXIS2_PLACEMENT_3D('',#186801,#113817,#113818);
#97712=AXIS2_PLACEMENT_3D('',#186809,#113819,#113820);
#97713=AXIS2_PLACEMENT_3D('',#186811,#113822,#113823);
#97714=AXIS2_PLACEMENT_3D('',#186814,#113825,#113826);
#97715=AXIS2_PLACEMENT_3D('',#186850,#113827,#113828);
#97716=AXIS2_PLACEMENT_3D('',#186851,#113829,#113830);
#97717=AXIS2_PLACEMENT_3D('',#186853,#113831,#113832);
#97718=AXIS2_PLACEMENT_3D('',#186881,#113834,#113835);
#97719=AXIS2_PLACEMENT_3D('',#186882,#113836,#113837);
#97720=AXIS2_PLACEMENT_3D('',#186885,#113839,#113840);
#97721=AXIS2_PLACEMENT_3D('',#186912,#113841,#113842);
#97722=AXIS2_PLACEMENT_3D('',#186913,#113843,#113844);
#97723=AXIS2_PLACEMENT_3D('',#186915,#113846,#113847);
#97724=AXIS2_PLACEMENT_3D('',#186936,#113849,#113850);
#97725=AXIS2_PLACEMENT_3D('',#186995,#113851,#113852);
#97726=AXIS2_PLACEMENT_3D('',#186997,#113853,#113854);
#97727=AXIS2_PLACEMENT_3D('',#186999,#113855,#113856);
#97728=AXIS2_PLACEMENT_3D('',#187001,#113858,#113859);
#97729=AXIS2_PLACEMENT_3D('',#187004,#113861,#113862);
#97730=AXIS2_PLACEMENT_3D('',#187024,#113863,#113864);
#97731=AXIS2_PLACEMENT_3D('',#187032,#113865,#113866);
#97732=AXIS2_PLACEMENT_3D('',#187034,#113867,#113868);
#97733=AXIS2_PLACEMENT_3D('',#187055,#113870,#113871);
#97734=AXIS2_PLACEMENT_3D('',#187063,#113872,#113873);
#97735=AXIS2_PLACEMENT_3D('',#187065,#113875,#113876);
#97736=AXIS2_PLACEMENT_3D('',#187068,#113878,#113879);
#97737=AXIS2_PLACEMENT_3D('',#187106,#113880,#113881);
#97738=AXIS2_PLACEMENT_3D('',#187109,#113883,#113884);
#97739=AXIS2_PLACEMENT_3D('',#187129,#113885,#113886);
#97740=AXIS2_PLACEMENT_3D('',#187167,#113887,#113888);
#97741=AXIS2_PLACEMENT_3D('',#187170,#113890,#113891);
#97742=AXIS2_PLACEMENT_3D('',#187171,#113892,#113893);
#97743=AXIS2_PLACEMENT_3D('',#187173,#113894,#113895);
#97744=AXIS2_PLACEMENT_3D('',#187194,#113897,#113898);
#97745=AXIS2_PLACEMENT_3D('',#187202,#113899,#113900);
#97746=AXIS2_PLACEMENT_3D('',#187204,#113901,#113902);
#97747=AXIS2_PLACEMENT_3D('',#187225,#113904,#113905);
#97748=AXIS2_PLACEMENT_3D('',#187233,#113906,#113907);
#97749=AXIS2_PLACEMENT_3D('',#187235,#113909,#113910);
#97750=AXIS2_PLACEMENT_3D('',#187262,#113912,#113913);
#97751=AXIS2_PLACEMENT_3D('',#187331,#113914,#113915);
#97752=AXIS2_PLACEMENT_3D('',#187332,#113916,#113917);
#97753=AXIS2_PLACEMENT_3D('',#187334,#113919,#113920);
#97754=AXIS2_PLACEMENT_3D('',#187335,#113921,#113922);
#97755=AXIS2_PLACEMENT_3D('',#187336,#113923,#113924);
#97756=AXIS2_PLACEMENT_3D('',#187339,#113926,#113927);
#97757=AXIS2_PLACEMENT_3D('',#187414,#113928,#113929);
#97758=AXIS2_PLACEMENT_3D('',#187415,#113930,#113931);
#97759=AXIS2_PLACEMENT_3D('',#187417,#113932,#113933);
#97760=AXIS2_PLACEMENT_3D('',#187418,#113934,#113935);
#97761=AXIS2_PLACEMENT_3D('',#187457,#113936,#113937);
#97762=AXIS2_PLACEMENT_3D('',#187458,#113938,#113939);
#97763=AXIS2_PLACEMENT_3D('',#187460,#113941,#113942);
#97764=AXIS2_PLACEMENT_3D('',#187461,#113943,#113944);
#97765=AXIS2_PLACEMENT_3D('',#187462,#113945,#113946);
#97766=AXIS2_PLACEMENT_3D('',#187465,#113948,#113949);
#97767=AXIS2_PLACEMENT_3D('',#187491,#113950,#113951);
#97768=AXIS2_PLACEMENT_3D('',#187533,#113952,#113953);
#97769=AXIS2_PLACEMENT_3D('',#187534,#113954,#113955);
#97770=AXIS2_PLACEMENT_3D('',#187566,#113956,#113957);
#97771=AXIS2_PLACEMENT_3D('',#187619,#113958,#113959);
#97772=AXIS2_PLACEMENT_3D('',#187621,#113961,#113962);
#97773=AXIS2_PLACEMENT_3D('',#187622,#113963,#113964);
#97774=AXIS2_PLACEMENT_3D('',#187623,#113965,#113966);
#97775=AXIS2_PLACEMENT_3D('',#187626,#113968,#113969);
#97776=AXIS2_PLACEMENT_3D('',#187658,#113970,#113971);
#97777=AXIS2_PLACEMENT_3D('',#187689,#113972,#113973);
#97778=AXIS2_PLACEMENT_3D('',#187690,#113974,#113975);
#97779=AXIS2_PLACEMENT_3D('',#187722,#113976,#113977);
#97780=AXIS2_PLACEMENT_3D('',#187745,#113978,#113979);
#97781=AXIS2_PLACEMENT_3D('',#187747,#113981,#113982);
#97782=AXIS2_PLACEMENT_3D('',#187748,#113983,#113984);
#97783=AXIS2_PLACEMENT_3D('',#187749,#113985,#113986);
#97784=AXIS2_PLACEMENT_3D('',#187752,#113988,#113989);
#97785=AXIS2_PLACEMENT_3D('',#187790,#113990,#113991);
#97786=AXIS2_PLACEMENT_3D('',#187847,#113992,#113993);
#97787=AXIS2_PLACEMENT_3D('',#187848,#113994,#113995);
#97788=AXIS2_PLACEMENT_3D('',#187880,#113996,#113997);
#97789=AXIS2_PLACEMENT_3D('',#187927,#113998,#113999);
#97790=AXIS2_PLACEMENT_3D('',#187929,#114001,#114002);
#97791=AXIS2_PLACEMENT_3D('',#187930,#114003,#114004);
#97792=AXIS2_PLACEMENT_3D('',#187931,#114005,#114006);
#97793=AXIS2_PLACEMENT_3D('',#187934,#114008,#114009);
#97794=AXIS2_PLACEMENT_3D('',#188009,#114010,#114011);
#97795=AXIS2_PLACEMENT_3D('',#188010,#114012,#114013);
#97796=AXIS2_PLACEMENT_3D('',#188012,#114014,#114015);
#97797=AXIS2_PLACEMENT_3D('',#188013,#114016,#114017);
#97798=AXIS2_PLACEMENT_3D('',#188100,#114018,#114019);
#97799=AXIS2_PLACEMENT_3D('',#188101,#114020,#114021);
#97800=AXIS2_PLACEMENT_3D('',#188103,#114023,#114024);
#97801=AXIS2_PLACEMENT_3D('',#188104,#114025,#114026);
#97802=AXIS2_PLACEMENT_3D('',#188105,#114027,#114028);
#97803=AXIS2_PLACEMENT_3D('',#188107,#114029,#114030);
#97804=AXIS2_PLACEMENT_3D('',#188128,#114032,#114033);
#97805=AXIS2_PLACEMENT_3D('',#188181,#114034,#114035);
#97806=AXIS2_PLACEMENT_3D('',#188187,#114039,#114040);
#97807=AXIS2_PLACEMENT_3D('',#188188,#114041,#114042);
#97808=AXIS2_PLACEMENT_3D('',#188189,#114043,#114044);
#97809=AXIS2_PLACEMENT_3D('',#188195,#114048,#114049);
#97810=AXIS2_PLACEMENT_3D('',#188196,#114050,#114051);
#97811=AXIS2_PLACEMENT_3D('',#188197,#114052,#114053);
#97812=AXIS2_PLACEMENT_3D('',#188198,#114054,#114055);
#97813=AXIS2_PLACEMENT_3D('',#188199,#114056,#114057);
#97814=AXIS2_PLACEMENT_3D('',#188205,#114061,#114062);
#97815=AXIS2_PLACEMENT_3D('',#188206,#114063,#114064);
#97816=AXIS2_PLACEMENT_3D('',#188226,#114065,#114066);
#97817=AXIS2_PLACEMENT_3D('',#188238,#114067,#114068);
#97818=AXIS2_PLACEMENT_3D('',#188240,#114069,#114070);
#97819=AXIS2_PLACEMENT_3D('',#188241,#114071,#114072);
#97820=AXIS2_PLACEMENT_3D('',#188254,#114073,#114074);
#97821=AXIS2_PLACEMENT_3D('',#188255,#114075,#114076);
#97822=AXIS2_PLACEMENT_3D('',#188258,#114077,#114078);
#97823=AXIS2_PLACEMENT_3D('',#188261,#114081,#114082);
#97824=AXIS2_PLACEMENT_3D('',#188262,#114083,#114084);
#97825=AXIS2_PLACEMENT_3D('',#188276,#114085,#114086);
#97826=AXIS2_PLACEMENT_3D('',#188284,#114087,#114088);
#97827=AXIS2_PLACEMENT_3D('',#188286,#114089,#114090);
#97828=AXIS2_PLACEMENT_3D('',#188287,#114091,#114092);
#97829=AXIS2_PLACEMENT_3D('',#188331,#114093,#114094);
#97830=AXIS2_PLACEMENT_3D('',#188334,#114096,#114097);
#97831=AXIS2_PLACEMENT_3D('',#188415,#114098,#114099);
#97832=AXIS2_PLACEMENT_3D('',#188429,#114100,#114101);
#97833=AXIS2_PLACEMENT_3D('',#188430,#114102,#114103);
#97834=AXIS2_PLACEMENT_3D('',#188474,#114104,#114105);
#97835=AXIS2_PLACEMENT_3D('',#188475,#114106,#114107);
#97836=AXIS2_PLACEMENT_3D('',#188477,#114109,#114110);
#97837=AXIS2_PLACEMENT_3D('',#188478,#114111,#114112);
#97838=AXIS2_PLACEMENT_3D('',#188479,#114113,#114114);
#97839=AXIS2_PLACEMENT_3D('',#188482,#114116,#114117);
#97840=AXIS2_PLACEMENT_3D('',#188514,#114118,#114119);
#97841=AXIS2_PLACEMENT_3D('',#188528,#114120,#114121);
#97842=AXIS2_PLACEMENT_3D('',#188529,#114122,#114123);
#97843=AXIS2_PLACEMENT_3D('',#188604,#114124,#114125);
#97844=AXIS2_PLACEMENT_3D('',#188605,#114126,#114127);
#97845=AXIS2_PLACEMENT_3D('',#188607,#114129,#114130);
#97846=AXIS2_PLACEMENT_3D('',#188608,#114131,#114132);
#97847=AXIS2_PLACEMENT_3D('',#188609,#114133,#114134);
#97848=AXIS2_PLACEMENT_3D('',#188611,#114135,#114136);
#97849=AXIS2_PLACEMENT_3D('',#188690,#114138,#114139);
#97850=AXIS2_PLACEMENT_3D('',#188691,#114140,#114141);
#97851=AXIS2_PLACEMENT_3D('',#188693,#114142,#114143);
#97852=AXIS2_PLACEMENT_3D('',#188694,#114144,#114145);
#97853=AXIS2_PLACEMENT_3D('',#188728,#114146,#114147);
#97854=AXIS2_PLACEMENT_3D('',#188729,#114148,#114149);
#97855=AXIS2_PLACEMENT_3D('',#188731,#114151,#114152);
#97856=AXIS2_PLACEMENT_3D('',#188732,#114153,#114154);
#97857=AXIS2_PLACEMENT_3D('',#188733,#114155,#114156);
#97858=AXIS2_PLACEMENT_3D('',#188736,#114158,#114159);
#97859=AXIS2_PLACEMENT_3D('',#188737,#114160,#114161);
#97860=AXIS2_PLACEMENT_3D('',#188739,#114162,#114163);
#97861=AXIS2_PLACEMENT_3D('',#188741,#114164,#114165);
#97862=AXIS2_PLACEMENT_3D('',#188742,#114166,#114167);
#97863=AXIS2_PLACEMENT_3D('',#188774,#114168,#114169);
#97864=AXIS2_PLACEMENT_3D('',#188818,#114170,#114171);
#97865=AXIS2_PLACEMENT_3D('',#188820,#114173,#114174);
#97866=AXIS2_PLACEMENT_3D('',#188821,#114175,#114176);
#97867=AXIS2_PLACEMENT_3D('',#188822,#114177,#114178);
#97868=AXIS2_PLACEMENT_3D('',#188825,#114180,#114181);
#97869=AXIS2_PLACEMENT_3D('',#188857,#114182,#114183);
#97870=AXIS2_PLACEMENT_3D('',#188901,#114184,#114185);
#97871=AXIS2_PLACEMENT_3D('',#188903,#114186,#114187);
#97872=AXIS2_PLACEMENT_3D('',#188904,#114188,#114189);
#97873=AXIS2_PLACEMENT_3D('',#188924,#114190,#114191);
#97874=AXIS2_PLACEMENT_3D('',#188944,#114192,#114193);
#97875=AXIS2_PLACEMENT_3D('',#188946,#114195,#114196);
#97876=AXIS2_PLACEMENT_3D('',#188947,#114197,#114198);
#97877=AXIS2_PLACEMENT_3D('',#188948,#114199,#114200);
#97878=AXIS2_PLACEMENT_3D('',#188951,#114202,#114203);
#97879=AXIS2_PLACEMENT_3D('',#188983,#114204,#114205);
#97880=AXIS2_PLACEMENT_3D('',#189034,#114206,#114207);
#97881=AXIS2_PLACEMENT_3D('',#189035,#114208,#114209);
#97882=AXIS2_PLACEMENT_3D('',#189068,#114210,#114211);
#97883=AXIS2_PLACEMENT_3D('',#189069,#114212,#114213);
#97884=AXIS2_PLACEMENT_3D('',#189116,#114214,#114215);
#97885=AXIS2_PLACEMENT_3D('',#189118,#114217,#114218);
#97886=AXIS2_PLACEMENT_3D('',#189119,#114219,#114220);
#97887=AXIS2_PLACEMENT_3D('',#189120,#114221,#114222);
#97888=AXIS2_PLACEMENT_3D('',#189123,#114224,#114225);
#97889=AXIS2_PLACEMENT_3D('',#189164,#114226,#114227);
#97890=AXIS2_PLACEMENT_3D('',#189165,#114228,#114229);
#97891=AXIS2_PLACEMENT_3D('',#189167,#114230,#114231);
#97892=AXIS2_PLACEMENT_3D('',#189168,#114232,#114233);
#97893=AXIS2_PLACEMENT_3D('',#189170,#114235,#114236);
#97894=AXIS2_PLACEMENT_3D('',#189176,#114240,#114241);
#97895=AXIS2_PLACEMENT_3D('',#189177,#114242,#114243);
#97896=AXIS2_PLACEMENT_3D('',#189178,#114244,#114245);
#97897=AXIS2_PLACEMENT_3D('',#189184,#114249,#114250);
#97898=AXIS2_PLACEMENT_3D('',#189185,#114251,#114252);
#97899=AXIS2_PLACEMENT_3D('',#189186,#114253,#114254);
#97900=AXIS2_PLACEMENT_3D('',#189187,#114255,#114256);
#97901=AXIS2_PLACEMENT_3D('',#189188,#114257,#114258);
#97902=AXIS2_PLACEMENT_3D('',#189194,#114262,#114263);
#97903=AXIS2_PLACEMENT_3D('',#189195,#114264,#114265);
#97904=AXIS2_PLACEMENT_3D('',#189209,#114266,#114267);
#97905=AXIS2_PLACEMENT_3D('',#189223,#114268,#114269);
#97906=AXIS2_PLACEMENT_3D('',#189224,#114270,#114271);
#97907=AXIS2_PLACEMENT_3D('',#189225,#114272,#114273);
#97908=AXIS2_PLACEMENT_3D('',#189226,#114274,#114275);
#97909=AXIS2_PLACEMENT_3D('',#189239,#114276,#114277);
#97910=AXIS2_PLACEMENT_3D('',#189252,#114278,#114279);
#97911=AXIS2_PLACEMENT_3D('',#189253,#114280,#114281);
#97912=AXIS2_PLACEMENT_3D('',#189254,#114282,#114283);
#97913=AXIS2_PLACEMENT_3D('',#189267,#114284,#114285);
#97914=AXIS2_PLACEMENT_3D('',#189280,#114286,#114287);
#97915=AXIS2_PLACEMENT_3D('',#189281,#114288,#114289);
#97916=AXIS2_PLACEMENT_3D('',#189282,#114290,#114291);
#97917=AXIS2_PLACEMENT_3D('',#189283,#114292,#114293);
#97918=AXIS2_PLACEMENT_3D('',#189284,#114294,#114295);
#97919=AXIS2_PLACEMENT_3D('',#189285,#114296,#114297);
#97920=AXIS2_PLACEMENT_3D('',#189286,#114298,#114299);
#97921=AXIS2_PLACEMENT_3D('',#189287,#114300,#114301);
#97922=AXIS2_PLACEMENT_3D('',#189288,#114302,#114303);
#97923=AXIS2_PLACEMENT_3D('',#189289,#114304,#114305);
#97924=AXIS2_PLACEMENT_3D('',#189290,#114306,#114307);
#97925=AXIS2_PLACEMENT_3D('',#189291,#114308,#114309);
#97926=AXIS2_PLACEMENT_3D('',#189292,#114310,#114311);
#97927=AXIS2_PLACEMENT_3D('',#189293,#114312,#114313);
#97928=AXIS2_PLACEMENT_3D('',#189295,#114315,#114316);
#97929=AXIS2_PLACEMENT_3D('',#189297,#114318,#114319);
#97930=AXIS2_PLACEMENT_3D('',#189298,#114320,#114321);
#97931=AXIS2_PLACEMENT_3D('',#189299,#114322,#114323);
#97932=AXIS2_PLACEMENT_3D('',#189300,#114324,#114325);
#97933=AXIS2_PLACEMENT_3D('',#189301,#114326,#114327);
#97934=AXIS2_PLACEMENT_3D('',#189302,#114328,#114329);
#97935=AXIS2_PLACEMENT_3D('',#189303,#114330,#114331);
#97936=AXIS2_PLACEMENT_3D('',#189304,#114332,#114333);
#97937=AXIS2_PLACEMENT_3D('',#189305,#114334,#114335);
#97938=AXIS2_PLACEMENT_3D('',#189306,#114336,#114337);
#97939=AXIS2_PLACEMENT_3D('',#189307,#114338,#114339);
#97940=AXIS2_PLACEMENT_3D('',#189308,#114340,#114341);
#97941=AXIS2_PLACEMENT_3D('',#189309,#114342,#114343);
#97942=AXIS2_PLACEMENT_3D('',#189310,#114344,#114345);
#97943=AXIS2_PLACEMENT_3D('',#189323,#114348,#114349);
#97944=AXIS2_PLACEMENT_3D('',#189333,#114351,#114352);
#97945=AXIS2_PLACEMENT_3D('',#189343,#114354,#114355);
#97946=AXIS2_PLACEMENT_3D('',#189353,#114357,#114358);
#97947=AXIS2_PLACEMENT_3D('',#189363,#114360,#114361);
#97948=AXIS2_PLACEMENT_3D('',#189370,#114362,#114363);
#97949=AXIS2_PLACEMENT_3D('',#189373,#114365,#114366);
#97950=AXIS2_PLACEMENT_3D('',#189374,#114367,#114368);
#97951=AXIS2_PLACEMENT_3D('',#189375,#114369,#114370);
#97952=AXIS2_PLACEMENT_3D('',#189376,#114371,#114372);
#97953=AXIS2_PLACEMENT_3D('',#189377,#114373,#114374);
#97954=AXIS2_PLACEMENT_3D('',#189378,#114375,#114376);
#97955=AXIS2_PLACEMENT_3D('',#189379,#114377,#114378);
#97956=AXIS2_PLACEMENT_3D('',#189380,#114379,#114380);
#97957=AXIS2_PLACEMENT_3D('',#189381,#114381,#114382);
#97958=AXIS2_PLACEMENT_3D('',#189382,#114383,#114384);
#97959=AXIS2_PLACEMENT_3D('',#189383,#114385,#114386);
#97960=AXIS2_PLACEMENT_3D('',#189384,#114387,#114388);
#97961=AXIS2_PLACEMENT_3D('',#189385,#114389,#114390);
#97962=AXIS2_PLACEMENT_3D('',#189387,#114391,#114392);
#97963=AXIS2_PLACEMENT_3D('',#189389,#114393,#114394);
#97964=AXIS2_PLACEMENT_3D('',#189391,#114395,#114396);
#97965=AXIS2_PLACEMENT_3D('',#189392,#114397,#114398);
#97966=AXIS2_PLACEMENT_3D('',#189393,#114399,#114400);
#97967=AXIS2_PLACEMENT_3D('',#189395,#114401,#114402);
#97968=AXIS2_PLACEMENT_3D('',#189396,#114403,#114404);
#97969=AXIS2_PLACEMENT_3D('',#189397,#114405,#114406);
#97970=AXIS2_PLACEMENT_3D('',#189399,#114408,#114409);
#97971=AXIS2_PLACEMENT_3D('',#189401,#114410,#114411);
#97972=AXIS2_PLACEMENT_3D('',#189404,#114413,#114414);
#97973=AXIS2_PLACEMENT_3D('',#189405,#114415,#114416);
#97974=AXIS2_PLACEMENT_3D('',#189406,#114417,#114418);
#97975=AXIS2_PLACEMENT_3D('',#189408,#114419,#114420);
#97976=AXIS2_PLACEMENT_3D('',#189410,#114422,#114423);
#97977=AXIS2_PLACEMENT_3D('',#189412,#114424,#114425);
#97978=AXIS2_PLACEMENT_3D('',#189413,#114426,#114427);
#97979=AXIS2_PLACEMENT_3D('',#189415,#114428,#114429);
#97980=AXIS2_PLACEMENT_3D('',#189417,#114431,#114432);
#97981=AXIS2_PLACEMENT_3D('',#189438,#114433,#114434);
#97982=AXIS2_PLACEMENT_3D('',#189447,#114435,#114436);
#97983=AXIS2_PLACEMENT_3D('',#189454,#114437,#114438);
#97984=AXIS2_PLACEMENT_3D('',#189456,#114439,#114440);
#97985=AXIS2_PLACEMENT_3D('',#189458,#114441,#114442);
#97986=AXIS2_PLACEMENT_3D('',#189460,#114443,#114444);
#97987=AXIS2_PLACEMENT_3D('',#189461,#114445,#114446);
#97988=AXIS2_PLACEMENT_3D('',#189494,#114447,#114448);
#97989=AXIS2_PLACEMENT_3D('',#189528,#114449,#114450);
#97990=AXIS2_PLACEMENT_3D('',#189553,#114451,#114452);
#97991=AXIS2_PLACEMENT_3D('',#189577,#114453,#114454);
#97992=AXIS2_PLACEMENT_3D('',#189579,#114455,#114456);
#97993=AXIS2_PLACEMENT_3D('',#189580,#114457,#114458);
#97994=AXIS2_PLACEMENT_3D('',#189613,#114459,#114460);
#97995=AXIS2_PLACEMENT_3D('',#189676,#114461,#114462);
#97996=AXIS2_PLACEMENT_3D('',#189679,#114463,#114464);
#97997=AXIS2_PLACEMENT_3D('',#189680,#114465,#114466);
#97998=AXIS2_PLACEMENT_3D('',#189681,#114467,#114468);
#97999=AXIS2_PLACEMENT_3D('',#189702,#114469,#114470);
#98000=AXIS2_PLACEMENT_3D('',#189716,#114471,#114472);
#98001=AXIS2_PLACEMENT_3D('',#189719,#114473,#114474);
#98002=AXIS2_PLACEMENT_3D('',#189720,#114475,#114476);
#98003=AXIS2_PLACEMENT_3D('',#189721,#114477,#114478);
#98004=AXIS2_PLACEMENT_3D('',#189754,#114479,#114480);
#98005=AXIS2_PLACEMENT_3D('',#189814,#114481,#114482);
#98006=AXIS2_PLACEMENT_3D('',#189817,#114483,#114484);
#98007=AXIS2_PLACEMENT_3D('',#189818,#114485,#114486);
#98008=AXIS2_PLACEMENT_3D('',#189819,#114487,#114488);
#98009=AXIS2_PLACEMENT_3D('',#189834,#114489,#114490);
#98010=AXIS2_PLACEMENT_3D('',#189857,#114491,#114492);
#98011=AXIS2_PLACEMENT_3D('',#189885,#114493,#114494);
#98012=AXIS2_PLACEMENT_3D('',#189887,#114495,#114496);
#98013=AXIS2_PLACEMENT_3D('',#189919,#114497,#114498);
#98014=AXIS2_PLACEMENT_3D('',#189920,#114499,#114500);
#98015=AXIS2_PLACEMENT_3D('',#189959,#114501,#114502);
#98016=AXIS2_PLACEMENT_3D('',#189974,#114503,#114504);
#98017=AXIS2_PLACEMENT_3D('',#190044,#114505,#114506);
#98018=AXIS2_PLACEMENT_3D('',#190082,#114507,#114508);
#98019=AXIS2_PLACEMENT_3D('',#190135,#114509,#114510);
#98020=AXIS2_PLACEMENT_3D('',#190180,#114511,#114512);
#98021=AXIS2_PLACEMENT_3D('',#190243,#114513,#114514);
#98022=AXIS2_PLACEMENT_3D('',#190245,#114515,#114516);
#98023=AXIS2_PLACEMENT_3D('',#190246,#114517,#114518);
#98024=AXIS2_PLACEMENT_3D('',#190261,#114519,#114520);
#98025=AXIS2_PLACEMENT_3D('',#190299,#114521,#114522);
#98026=AXIS2_PLACEMENT_3D('',#190334,#114523,#114524);
#98027=AXIS2_PLACEMENT_3D('',#190351,#114525,#114526);
#98028=AXIS2_PLACEMENT_3D('',#190354,#114527,#114528);
#98029=AXIS2_PLACEMENT_3D('',#190355,#114529,#114530);
#98030=AXIS2_PLACEMENT_3D('',#190356,#114531,#114532);
#98031=AXIS2_PLACEMENT_3D('',#190357,#114533,#114534);
#98032=AXIS2_PLACEMENT_3D('',#190359,#114535,#114536);
#98033=AXIS2_PLACEMENT_3D('',#190360,#114537,#114538);
#98034=AXIS2_PLACEMENT_3D('',#190361,#114539,#114540);
#98035=AXIS2_PLACEMENT_3D('',#190364,#114541,#114542);
#98036=AXIS2_PLACEMENT_3D('',#190365,#114543,#114544);
#98037=AXIS2_PLACEMENT_3D('',#190366,#114545,#114546);
#98038=AXIS2_PLACEMENT_3D('',#190381,#114547,#114548);
#98039=AXIS2_PLACEMENT_3D('',#190390,#114549,#114550);
#98040=AXIS2_PLACEMENT_3D('',#190391,#114551,#114552);
#98041=AXIS2_PLACEMENT_3D('',#190392,#114553,#114554);
#98042=AXIS2_PLACEMENT_3D('',#190393,#114555,#114556);
#98043=AXIS2_PLACEMENT_3D('',#190396,#114557,#114558);
#98044=AXIS2_PLACEMENT_3D('',#190398,#114559,#114560);
#98045=AXIS2_PLACEMENT_3D('',#190400,#114561,#114562);
#98046=AXIS2_PLACEMENT_3D('',#190401,#114563,#114564);
#98047=AXIS2_PLACEMENT_3D('',#190402,#114565,#114566);
#98048=AXIS2_PLACEMENT_3D('',#190405,#114567,#114568);
#98049=AXIS2_PLACEMENT_3D('',#190406,#114569,#114570);
#98050=AXIS2_PLACEMENT_3D('',#190407,#114571,#114572);
#98051=AXIS2_PLACEMENT_3D('',#190408,#114573,#114574);
#98052=AXIS2_PLACEMENT_3D('',#190411,#114575,#114576);
#98053=AXIS2_PLACEMENT_3D('',#190412,#114577,#114578);
#98054=AXIS2_PLACEMENT_3D('',#190413,#114579,#114580);
#98055=AXIS2_PLACEMENT_3D('',#190414,#114581,#114582);
#98056=AXIS2_PLACEMENT_3D('',#190417,#114583,#114584);
#98057=AXIS2_PLACEMENT_3D('',#190418,#114585,#114586);
#98058=AXIS2_PLACEMENT_3D('',#190419,#114587,#114588);
#98059=AXIS2_PLACEMENT_3D('',#190420,#114589,#114590);
#98060=AXIS2_PLACEMENT_3D('',#190423,#114591,#114592);
#98061=AXIS2_PLACEMENT_3D('',#190424,#114593,#114594);
#98062=AXIS2_PLACEMENT_3D('',#190425,#114595,#114596);
#98063=AXIS2_PLACEMENT_3D('',#190426,#114597,#114598);
#98064=AXIS2_PLACEMENT_3D('',#190429,#114599,#114600);
#98065=AXIS2_PLACEMENT_3D('',#190430,#114601,#114602);
#98066=AXIS2_PLACEMENT_3D('',#190431,#114603,#114604);
#98067=AXIS2_PLACEMENT_3D('',#190432,#114605,#114606);
#98068=AXIS2_PLACEMENT_3D('',#190435,#114607,#114608);
#98069=AXIS2_PLACEMENT_3D('',#190436,#114609,#114610);
#98070=AXIS2_PLACEMENT_3D('',#190437,#114611,#114612);
#98071=AXIS2_PLACEMENT_3D('',#190451,#114613,#114614);
#98072=AXIS2_PLACEMENT_3D('',#190453,#114615,#114616);
#98073=AXIS2_PLACEMENT_3D('',#190454,#114617,#114618);
#98074=AXIS2_PLACEMENT_3D('',#190469,#114619,#114620);
#98075=AXIS2_PLACEMENT_3D('',#190470,#114621,#114622);
#98076=AXIS2_PLACEMENT_3D('',#190525,#114623,#114624);
#98077=AXIS2_PLACEMENT_3D('',#190576,#114625,#114626);
#98078=AXIS2_PLACEMENT_3D('',#190637,#114627,#114628);
#98079=AXIS2_PLACEMENT_3D('',#190638,#114629,#114630);
#98080=AXIS2_PLACEMENT_3D('',#190639,#114631,#114632);
#98081=AXIS2_PLACEMENT_3D('',#190654,#114633,#114634);
#98082=AXIS2_PLACEMENT_3D('',#190655,#114635,#114636);
#98083=AXIS2_PLACEMENT_3D('',#190656,#114637,#114638);
#98084=AXIS2_PLACEMENT_3D('',#190671,#114639,#114640);
#98085=AXIS2_PLACEMENT_3D('',#190709,#114641,#114642);
#98086=AXIS2_PLACEMENT_3D('',#190759,#114643,#114644);
#98087=AXIS2_PLACEMENT_3D('',#190802,#114645,#114646);
#98088=AXIS2_PLACEMENT_3D('',#190875,#114647,#114648);
#98089=AXIS2_PLACEMENT_3D('',#190968,#114649,#114650);
#98090=AXIS2_PLACEMENT_3D('',#191012,#114651,#114652);
#98091=AXIS2_PLACEMENT_3D('',#191013,#114653,#114654);
#98092=AXIS2_PLACEMENT_3D('',#191014,#114655,#114656);
#98093=AXIS2_PLACEMENT_3D('',#191071,#114657,#114658);
#98094=AXIS2_PLACEMENT_3D('',#191092,#114659,#114660);
#98095=AXIS2_PLACEMENT_3D('',#191111,#114661,#114662);
#98096=AXIS2_PLACEMENT_3D('',#191114,#114663,#114664);
#98097=AXIS2_PLACEMENT_3D('',#191115,#114665,#114666);
#98098=AXIS2_PLACEMENT_3D('',#191116,#114667,#114668);
#98099=AXIS2_PLACEMENT_3D('',#191143,#114669,#114670);
#98100=AXIS2_PLACEMENT_3D('',#191216,#114671,#114672);
#98101=AXIS2_PLACEMENT_3D('',#191274,#114673,#114674);
#98102=AXIS2_PLACEMENT_3D('',#191321,#114675,#114676);
#98103=AXIS2_PLACEMENT_3D('',#191362,#114677,#114678);
#98104=AXIS2_PLACEMENT_3D('',#191363,#114679,#114680);
#98105=AXIS2_PLACEMENT_3D('',#191364,#114681,#114682);
#98106=AXIS2_PLACEMENT_3D('',#191379,#114683,#114684);
#98107=AXIS2_PLACEMENT_3D('',#191551,#114685,#114686);
#98108=AXIS2_PLACEMENT_3D('',#191552,#114687,#114688);
#98109=AXIS2_PLACEMENT_3D('',#191553,#114689,#114690);
#98110=AXIS2_PLACEMENT_3D('',#191636,#114691,#114692);
#98111=AXIS2_PLACEMENT_3D('',#191640,#114694,#114695);
#98112=AXIS2_PLACEMENT_3D('',#191652,#114697,#114698);
#98113=AXIS2_PLACEMENT_3D('',#191654,#114699,#114700);
#98114=AXIS2_PLACEMENT_3D('',#191655,#114701,#114702);
#98115=AXIS2_PLACEMENT_3D('',#191656,#114703,#114704);
#98116=AXIS2_PLACEMENT_3D('',#191658,#114705,#114706);
#98117=AXIS2_PLACEMENT_3D('',#191660,#114707,#114708);
#98118=AXIS2_PLACEMENT_3D('',#191661,#114709,#114710);
#98119=AXIS2_PLACEMENT_3D('',#191662,#114711,#114712);
#98120=AXIS2_PLACEMENT_3D('',#191674,#114713,#114714);
#98121=AXIS2_PLACEMENT_3D('',#191675,#114715,#114716);
#98122=AXIS2_PLACEMENT_3D('',#191676,#114717,#114718);
#98123=AXIS2_PLACEMENT_3D('',#191677,#114719,#114720);
#98124=AXIS2_PLACEMENT_3D('',#191680,#114723,#114724);
#98125=AXIS2_PLACEMENT_3D('',#191684,#114726,#114727);
#98126=AXIS2_PLACEMENT_3D('',#191696,#114729,#114730);
#98127=AXIS2_PLACEMENT_3D('',#191698,#114731,#114732);
#98128=AXIS2_PLACEMENT_3D('',#191699,#114733,#114734);
#98129=AXIS2_PLACEMENT_3D('',#191700,#114735,#114736);
#98130=AXIS2_PLACEMENT_3D('',#191703,#114737,#114738);
#98131=AXIS2_PLACEMENT_3D('',#191704,#114739,#114740);
#98132=AXIS2_PLACEMENT_3D('',#191705,#114741,#114742);
#98133=AXIS2_PLACEMENT_3D('',#191717,#114743,#114744);
#98134=AXIS2_PLACEMENT_3D('',#191718,#114745,#114746);
#98135=AXIS2_PLACEMENT_3D('',#191719,#114747,#114748);
#98136=AXIS2_PLACEMENT_3D('',#191720,#114749,#114750);
#98137=AXIS2_PLACEMENT_3D('',#191723,#114753,#114754);
#98138=AXIS2_PLACEMENT_3D('',#191727,#114756,#114757);
#98139=AXIS2_PLACEMENT_3D('',#191740,#114759,#114760);
#98140=AXIS2_PLACEMENT_3D('',#191741,#114761,#114762);
#98141=AXIS2_PLACEMENT_3D('',#191742,#114763,#114764);
#98142=AXIS2_PLACEMENT_3D('',#191743,#114765,#114766);
#98143=AXIS2_PLACEMENT_3D('',#191746,#114767,#114768);
#98144=AXIS2_PLACEMENT_3D('',#191747,#114769,#114770);
#98145=AXIS2_PLACEMENT_3D('',#191748,#114771,#114772);
#98146=AXIS2_PLACEMENT_3D('',#191759,#114773,#114774);
#98147=AXIS2_PLACEMENT_3D('',#191761,#114775,#114776);
#98148=AXIS2_PLACEMENT_3D('',#191762,#114777,#114778);
#98149=AXIS2_PLACEMENT_3D('',#191763,#114779,#114780);
#98150=AXIS2_PLACEMENT_3D('',#191766,#114783,#114784);
#98151=AXIS2_PLACEMENT_3D('',#191770,#114786,#114787);
#98152=AXIS2_PLACEMENT_3D('',#191783,#114789,#114790);
#98153=AXIS2_PLACEMENT_3D('',#191784,#114791,#114792);
#98154=AXIS2_PLACEMENT_3D('',#191785,#114793,#114794);
#98155=AXIS2_PLACEMENT_3D('',#191786,#114795,#114796);
#98156=AXIS2_PLACEMENT_3D('',#191789,#114797,#114798);
#98157=AXIS2_PLACEMENT_3D('',#191790,#114799,#114800);
#98158=AXIS2_PLACEMENT_3D('',#191791,#114801,#114802);
#98159=AXIS2_PLACEMENT_3D('',#191802,#114803,#114804);
#98160=AXIS2_PLACEMENT_3D('',#191804,#114805,#114806);
#98161=AXIS2_PLACEMENT_3D('',#191805,#114807,#114808);
#98162=AXIS2_PLACEMENT_3D('',#191806,#114809,#114810);
#98163=AXIS2_PLACEMENT_3D('',#191809,#114813,#114814);
#98164=AXIS2_PLACEMENT_3D('',#191812,#114817,#114818);
#98165=AXIS2_PLACEMENT_3D('',#191815,#114821,#114822);
#98166=AXIS2_PLACEMENT_3D('',#191818,#114825,#114826);
#98167=AXIS2_PLACEMENT_3D('',#191821,#114829,#114830);
#98168=AXIS2_PLACEMENT_3D('',#191824,#114833,#114834);
#98169=AXIS2_PLACEMENT_3D('',#191827,#114837,#114838);
#98170=AXIS2_PLACEMENT_3D('',#191830,#114841,#114842);
#98171=AXIS2_PLACEMENT_3D('',#191833,#114845,#114846);
#98172=AXIS2_PLACEMENT_3D('',#191836,#114847,#114848);
#98173=AXIS2_PLACEMENT_3D('',#191838,#114849,#114850);
#98174=AXIS2_PLACEMENT_3D('',#191840,#114851,#114852);
#98175=AXIS2_PLACEMENT_3D('',#191841,#114853,#114854);
#98176=AXIS2_PLACEMENT_3D('',#191842,#114855,#114856);
#98177=AXIS2_PLACEMENT_3D('',#191845,#114857,#114858);
#98178=AXIS2_PLACEMENT_3D('',#191848,#114861,#114862);
#98179=AXIS2_PLACEMENT_3D('',#191851,#114863,#114864);
#98180=AXIS2_PLACEMENT_3D('',#191852,#114865,#114866);
#98181=AXIS2_PLACEMENT_3D('',#191853,#114867,#114868);
#98182=AXIS2_PLACEMENT_3D('',#191854,#114869,#114870);
#98183=AXIS2_PLACEMENT_3D('',#191857,#114871,#114872);
#98184=AXIS2_PLACEMENT_3D('',#191858,#114873,#114874);
#98185=AXIS2_PLACEMENT_3D('',#191859,#114875,#114876);
#98186=AXIS2_PLACEMENT_3D('',#191860,#114877,#114878);
#98187=AXIS2_PLACEMENT_3D('',#191863,#114879,#114880);
#98188=AXIS2_PLACEMENT_3D('',#191864,#114881,#114882);
#98189=AXIS2_PLACEMENT_3D('',#191865,#114883,#114884);
#98190=AXIS2_PLACEMENT_3D('',#191866,#114885,#114886);
#98191=AXIS2_PLACEMENT_3D('',#191869,#114887,#114888);
#98192=AXIS2_PLACEMENT_3D('',#191872,#114891,#114892);
#98193=AXIS2_PLACEMENT_3D('',#191875,#114893,#114894);
#98194=AXIS2_PLACEMENT_3D('',#191876,#114895,#114896);
#98195=AXIS2_PLACEMENT_3D('',#191877,#114897,#114898);
#98196=AXIS2_PLACEMENT_3D('',#191878,#114899,#114900);
#98197=AXIS2_PLACEMENT_3D('',#191881,#114901,#114902);
#98198=AXIS2_PLACEMENT_3D('',#191882,#114903,#114904);
#98199=AXIS2_PLACEMENT_3D('',#191883,#114905,#114906);
#98200=AXIS2_PLACEMENT_3D('',#191884,#114907,#114908);
#98201=AXIS2_PLACEMENT_3D('',#191887,#114909,#114910);
#98202=AXIS2_PLACEMENT_3D('',#191888,#114911,#114912);
#98203=AXIS2_PLACEMENT_3D('',#191889,#114913,#114914);
#98204=AXIS2_PLACEMENT_3D('',#191890,#114915,#114916);
#98205=AXIS2_PLACEMENT_3D('',#191893,#114919,#114920);
#98206=AXIS2_PLACEMENT_3D('',#191896,#114921,#114922);
#98207=AXIS2_PLACEMENT_3D('',#191898,#114923,#114924);
#98208=AXIS2_PLACEMENT_3D('',#191900,#114925,#114926);
#98209=AXIS2_PLACEMENT_3D('',#191901,#114927,#114928);
#98210=AXIS2_PLACEMENT_3D('',#191902,#114929,#114930);
#98211=AXIS2_PLACEMENT_3D('',#191905,#114931,#114932);
#98212=AXIS2_PLACEMENT_3D('',#191908,#114935,#114936);
#98213=AXIS2_PLACEMENT_3D('',#191911,#114937,#114938);
#98214=AXIS2_PLACEMENT_3D('',#191912,#114939,#114940);
#98215=AXIS2_PLACEMENT_3D('',#191913,#114941,#114942);
#98216=AXIS2_PLACEMENT_3D('',#191914,#114943,#114944);
#98217=AXIS2_PLACEMENT_3D('',#191917,#114945,#114946);
#98218=AXIS2_PLACEMENT_3D('',#191918,#114947,#114948);
#98219=AXIS2_PLACEMENT_3D('',#191919,#114949,#114950);
#98220=AXIS2_PLACEMENT_3D('',#191920,#114951,#114952);
#98221=AXIS2_PLACEMENT_3D('',#191923,#114953,#114954);
#98222=AXIS2_PLACEMENT_3D('',#191924,#114955,#114956);
#98223=AXIS2_PLACEMENT_3D('',#191925,#114957,#114958);
#98224=AXIS2_PLACEMENT_3D('',#191926,#114959,#114960);
#98225=AXIS2_PLACEMENT_3D('',#191929,#114961,#114962);
#98226=AXIS2_PLACEMENT_3D('',#191932,#114965,#114966);
#98227=AXIS2_PLACEMENT_3D('',#191935,#114967,#114968);
#98228=AXIS2_PLACEMENT_3D('',#191938,#114971,#114972);
#98229=AXIS2_PLACEMENT_3D('',#191939,#114973,#114974);
#98230=AXIS2_PLACEMENT_3D('',#191940,#114975,#114976);
#98231=AXIS2_PLACEMENT_3D('',#191941,#114977,#114978);
#98232=AXIS2_PLACEMENT_3D('',#191944,#114979,#114980);
#98233=AXIS2_PLACEMENT_3D('',#191946,#114981,#114982);
#98234=AXIS2_PLACEMENT_3D('',#191948,#114983,#114984);
#98235=AXIS2_PLACEMENT_3D('',#191949,#114985,#114986);
#98236=AXIS2_PLACEMENT_3D('',#191950,#114987,#114988);
#98237=AXIS2_PLACEMENT_3D('',#191953,#114989,#114990);
#98238=AXIS2_PLACEMENT_3D('',#191956,#114993,#114994);
#98239=AXIS2_PLACEMENT_3D('',#191959,#114995,#114996);
#98240=AXIS2_PLACEMENT_3D('',#191960,#114997,#114998);
#98241=AXIS2_PLACEMENT_3D('',#191961,#114999,#115000);
#98242=AXIS2_PLACEMENT_3D('',#191962,#115001,#115002);
#98243=AXIS2_PLACEMENT_3D('',#191965,#115003,#115004);
#98244=AXIS2_PLACEMENT_3D('',#191966,#115005,#115006);
#98245=AXIS2_PLACEMENT_3D('',#191967,#115007,#115008);
#98246=AXIS2_PLACEMENT_3D('',#191968,#115009,#115010);
#98247=AXIS2_PLACEMENT_3D('',#191971,#115011,#115012);
#98248=AXIS2_PLACEMENT_3D('',#191972,#115013,#115014);
#98249=AXIS2_PLACEMENT_3D('',#191973,#115015,#115016);
#98250=AXIS2_PLACEMENT_3D('',#191974,#115017,#115018);
#98251=AXIS2_PLACEMENT_3D('',#191977,#115019,#115020);
#98252=AXIS2_PLACEMENT_3D('',#191980,#115023,#115024);
#98253=AXIS2_PLACEMENT_3D('',#191983,#115025,#115026);
#98254=AXIS2_PLACEMENT_3D('',#191986,#115029,#115030);
#98255=AXIS2_PLACEMENT_3D('',#191987,#115031,#115032);
#98256=AXIS2_PLACEMENT_3D('',#191988,#115033,#115034);
#98257=AXIS2_PLACEMENT_3D('',#191989,#115035,#115036);
#98258=AXIS2_PLACEMENT_3D('',#191992,#115037,#115038);
#98259=AXIS2_PLACEMENT_3D('',#191994,#115039,#115040);
#98260=AXIS2_PLACEMENT_3D('',#191996,#115041,#115042);
#98261=AXIS2_PLACEMENT_3D('',#191997,#115043,#115044);
#98262=AXIS2_PLACEMENT_3D('',#191998,#115045,#115046);
#98263=AXIS2_PLACEMENT_3D('',#192001,#115047,#115048);
#98264=AXIS2_PLACEMENT_3D('',#192004,#115051,#115052);
#98265=AXIS2_PLACEMENT_3D('',#192007,#115053,#115054);
#98266=AXIS2_PLACEMENT_3D('',#192010,#115057,#115058);
#98267=AXIS2_PLACEMENT_3D('',#192013,#115059,#115060);
#98268=AXIS2_PLACEMENT_3D('',#192014,#115061,#115062);
#98269=AXIS2_PLACEMENT_3D('',#192015,#115063,#115064);
#98270=AXIS2_PLACEMENT_3D('',#192016,#115065,#115066);
#98271=AXIS2_PLACEMENT_3D('',#192019,#115067,#115068);
#98272=AXIS2_PLACEMENT_3D('',#192020,#115069,#115070);
#98273=AXIS2_PLACEMENT_3D('',#192021,#115071,#115072);
#98274=AXIS2_PLACEMENT_3D('',#192022,#115073,#115074);
#98275=AXIS2_PLACEMENT_3D('',#192025,#115075,#115076);
#98276=AXIS2_PLACEMENT_3D('',#192028,#115079,#115080);
#98277=AXIS2_PLACEMENT_3D('',#192031,#115081,#115082);
#98278=AXIS2_PLACEMENT_3D('',#192034,#115085,#115086);
#98279=AXIS2_PLACEMENT_3D('',#192035,#115087,#115088);
#98280=AXIS2_PLACEMENT_3D('',#192036,#115089,#115090);
#98281=AXIS2_PLACEMENT_3D('',#192037,#115091,#115092);
#98282=AXIS2_PLACEMENT_3D('',#192040,#115093,#115094);
#98283=AXIS2_PLACEMENT_3D('',#192042,#115095,#115096);
#98284=AXIS2_PLACEMENT_3D('',#192044,#115097,#115098);
#98285=AXIS2_PLACEMENT_3D('',#192045,#115099,#115100);
#98286=AXIS2_PLACEMENT_3D('',#192046,#115101,#115102);
#98287=AXIS2_PLACEMENT_3D('',#192049,#115103,#115104);
#98288=AXIS2_PLACEMENT_3D('',#192052,#115107,#115108);
#98289=AXIS2_PLACEMENT_3D('',#192055,#115109,#115110);
#98290=AXIS2_PLACEMENT_3D('',#192058,#115113,#115114);
#98291=AXIS2_PLACEMENT_3D('',#192061,#115115,#115116);
#98292=AXIS2_PLACEMENT_3D('',#192062,#115117,#115118);
#98293=AXIS2_PLACEMENT_3D('',#192063,#115119,#115120);
#98294=AXIS2_PLACEMENT_3D('',#192064,#115121,#115122);
#98295=AXIS2_PLACEMENT_3D('',#192067,#115123,#115124);
#98296=AXIS2_PLACEMENT_3D('',#192068,#115125,#115126);
#98297=AXIS2_PLACEMENT_3D('',#192069,#115127,#115128);
#98298=AXIS2_PLACEMENT_3D('',#192070,#115129,#115130);
#98299=AXIS2_PLACEMENT_3D('',#192073,#115131,#115132);
#98300=AXIS2_PLACEMENT_3D('',#192074,#115133,#115134);
#98301=AXIS2_PLACEMENT_3D('',#192075,#115135,#115136);
#98302=AXIS2_PLACEMENT_3D('',#192076,#115137,#115138);
#98303=AXIS2_PLACEMENT_3D('',#192079,#115139,#115140);
#98304=AXIS2_PLACEMENT_3D('',#192082,#115143,#115144);
#98305=AXIS2_PLACEMENT_3D('',#192085,#115145,#115146);
#98306=AXIS2_PLACEMENT_3D('',#192086,#115147,#115148);
#98307=AXIS2_PLACEMENT_3D('',#192087,#115149,#115150);
#98308=AXIS2_PLACEMENT_3D('',#192088,#115151,#115152);
#98309=AXIS2_PLACEMENT_3D('',#192089,#115153,#115154);
#98310=AXIS2_PLACEMENT_3D('',#192090,#115155,#115156);
#98311=AXIS2_PLACEMENT_3D('',#192091,#115157,#115158);
#98312=AXIS2_PLACEMENT_3D('',#192094,#115159,#115160);
#98313=AXIS2_PLACEMENT_3D('',#192096,#115161,#115162);
#98314=AXIS2_PLACEMENT_3D('',#192098,#115163,#115164);
#98315=AXIS2_PLACEMENT_3D('',#192099,#115165,#115166);
#98316=AXIS2_PLACEMENT_3D('',#192100,#115167,#115168);
#98317=AXIS2_PLACEMENT_3D('',#192103,#115169,#115170);
#98318=AXIS2_PLACEMENT_3D('',#192106,#115173,#115174);
#98319=AXIS2_PLACEMENT_3D('',#192109,#115175,#115176);
#98320=AXIS2_PLACEMENT_3D('',#192112,#115179,#115180);
#98321=AXIS2_PLACEMENT_3D('',#192115,#115181,#115182);
#98322=AXIS2_PLACEMENT_3D('',#192116,#115183,#115184);
#98323=AXIS2_PLACEMENT_3D('',#192117,#115185,#115186);
#98324=AXIS2_PLACEMENT_3D('',#192118,#115187,#115188);
#98325=AXIS2_PLACEMENT_3D('',#192121,#115189,#115190);
#98326=AXIS2_PLACEMENT_3D('',#192122,#115191,#115192);
#98327=AXIS2_PLACEMENT_3D('',#192123,#115193,#115194);
#98328=AXIS2_PLACEMENT_3D('',#192124,#115195,#115196);
#98329=AXIS2_PLACEMENT_3D('',#192127,#115197,#115198);
#98330=AXIS2_PLACEMENT_3D('',#192130,#115201,#115202);
#98331=AXIS2_PLACEMENT_3D('',#192133,#115203,#115204);
#98332=AXIS2_PLACEMENT_3D('',#192136,#115207,#115208);
#98333=AXIS2_PLACEMENT_3D('',#192137,#115209,#115210);
#98334=AXIS2_PLACEMENT_3D('',#192138,#115211,#115212);
#98335=AXIS2_PLACEMENT_3D('',#192139,#115213,#115214);
#98336=AXIS2_PLACEMENT_3D('',#192142,#115215,#115216);
#98337=AXIS2_PLACEMENT_3D('',#192144,#115217,#115218);
#98338=AXIS2_PLACEMENT_3D('',#192146,#115219,#115220);
#98339=AXIS2_PLACEMENT_3D('',#192147,#115221,#115222);
#98340=AXIS2_PLACEMENT_3D('',#192148,#115223,#115224);
#98341=AXIS2_PLACEMENT_3D('',#192151,#115225,#115226);
#98342=AXIS2_PLACEMENT_3D('',#192154,#115229,#115230);
#98343=AXIS2_PLACEMENT_3D('',#192157,#115231,#115232);
#98344=AXIS2_PLACEMENT_3D('',#192160,#115235,#115236);
#98345=AXIS2_PLACEMENT_3D('',#192163,#115237,#115238);
#98346=AXIS2_PLACEMENT_3D('',#192164,#115239,#115240);
#98347=AXIS2_PLACEMENT_3D('',#192165,#115241,#115242);
#98348=AXIS2_PLACEMENT_3D('',#192166,#115243,#115244);
#98349=AXIS2_PLACEMENT_3D('',#192169,#115245,#115246);
#98350=AXIS2_PLACEMENT_3D('',#192170,#115247,#115248);
#98351=AXIS2_PLACEMENT_3D('',#192171,#115249,#115250);
#98352=AXIS2_PLACEMENT_3D('',#192172,#115251,#115252);
#98353=AXIS2_PLACEMENT_3D('',#192175,#115253,#115254);
#98354=AXIS2_PLACEMENT_3D('',#192178,#115257,#115258);
#98355=AXIS2_PLACEMENT_3D('',#192181,#115259,#115260);
#98356=AXIS2_PLACEMENT_3D('',#192184,#115263,#115264);
#98357=AXIS2_PLACEMENT_3D('',#192185,#115265,#115266);
#98358=AXIS2_PLACEMENT_3D('',#192186,#115267,#115268);
#98359=AXIS2_PLACEMENT_3D('',#192187,#115269,#115270);
#98360=AXIS2_PLACEMENT_3D('',#192190,#115271,#115272);
#98361=AXIS2_PLACEMENT_3D('',#192192,#115273,#115274);
#98362=AXIS2_PLACEMENT_3D('',#192194,#115275,#115276);
#98363=AXIS2_PLACEMENT_3D('',#192195,#115277,#115278);
#98364=AXIS2_PLACEMENT_3D('',#192196,#115279,#115280);
#98365=AXIS2_PLACEMENT_3D('',#192199,#115281,#115282);
#98366=AXIS2_PLACEMENT_3D('',#192202,#115285,#115286);
#98367=AXIS2_PLACEMENT_3D('',#192205,#115287,#115288);
#98368=AXIS2_PLACEMENT_3D('',#192208,#115291,#115292);
#98369=AXIS2_PLACEMENT_3D('',#192211,#115293,#115294);
#98370=AXIS2_PLACEMENT_3D('',#192212,#115295,#115296);
#98371=AXIS2_PLACEMENT_3D('',#192213,#115297,#115298);
#98372=AXIS2_PLACEMENT_3D('',#192214,#115299,#115300);
#98373=AXIS2_PLACEMENT_3D('',#192217,#115301,#115302);
#98374=AXIS2_PLACEMENT_3D('',#192218,#115303,#115304);
#98375=AXIS2_PLACEMENT_3D('',#192219,#115305,#115306);
#98376=AXIS2_PLACEMENT_3D('',#192220,#115307,#115308);
#98377=AXIS2_PLACEMENT_3D('',#192223,#115309,#115310);
#98378=AXIS2_PLACEMENT_3D('',#192226,#115313,#115314);
#98379=AXIS2_PLACEMENT_3D('',#192229,#115315,#115316);
#98380=AXIS2_PLACEMENT_3D('',#192232,#115319,#115320);
#98381=AXIS2_PLACEMENT_3D('',#192233,#115321,#115322);
#98382=AXIS2_PLACEMENT_3D('',#192234,#115323,#115324);
#98383=AXIS2_PLACEMENT_3D('',#192235,#115325,#115326);
#98384=AXIS2_PLACEMENT_3D('',#192238,#115327,#115328);
#98385=AXIS2_PLACEMENT_3D('',#192240,#115329,#115330);
#98386=AXIS2_PLACEMENT_3D('',#192242,#115331,#115332);
#98387=AXIS2_PLACEMENT_3D('',#192243,#115333,#115334);
#98388=AXIS2_PLACEMENT_3D('',#192244,#115335,#115336);
#98389=AXIS2_PLACEMENT_3D('',#192247,#115337,#115338);
#98390=AXIS2_PLACEMENT_3D('',#192250,#115341,#115342);
#98391=AXIS2_PLACEMENT_3D('',#192253,#115343,#115344);
#98392=AXIS2_PLACEMENT_3D('',#192256,#115347,#115348);
#98393=AXIS2_PLACEMENT_3D('',#192259,#115349,#115350);
#98394=AXIS2_PLACEMENT_3D('',#192260,#115351,#115352);
#98395=AXIS2_PLACEMENT_3D('',#192261,#115353,#115354);
#98396=AXIS2_PLACEMENT_3D('',#192262,#115355,#115356);
#98397=AXIS2_PLACEMENT_3D('',#192265,#115357,#115358);
#98398=AXIS2_PLACEMENT_3D('',#192266,#115359,#115360);
#98399=AXIS2_PLACEMENT_3D('',#192267,#115361,#115362);
#98400=AXIS2_PLACEMENT_3D('',#192268,#115363,#115364);
#98401=AXIS2_PLACEMENT_3D('',#192271,#115365,#115366);
#98402=AXIS2_PLACEMENT_3D('',#192274,#115369,#115370);
#98403=AXIS2_PLACEMENT_3D('',#192277,#115371,#115372);
#98404=AXIS2_PLACEMENT_3D('',#192280,#115375,#115376);
#98405=AXIS2_PLACEMENT_3D('',#192281,#115377,#115378);
#98406=AXIS2_PLACEMENT_3D('',#192282,#115379,#115380);
#98407=AXIS2_PLACEMENT_3D('',#192283,#115381,#115382);
#98408=AXIS2_PLACEMENT_3D('',#192286,#115383,#115384);
#98409=AXIS2_PLACEMENT_3D('',#192288,#115385,#115386);
#98410=AXIS2_PLACEMENT_3D('',#192290,#115387,#115388);
#98411=AXIS2_PLACEMENT_3D('',#192291,#115389,#115390);
#98412=AXIS2_PLACEMENT_3D('',#192292,#115391,#115392);
#98413=AXIS2_PLACEMENT_3D('',#192295,#115393,#115394);
#98414=AXIS2_PLACEMENT_3D('',#192298,#115397,#115398);
#98415=AXIS2_PLACEMENT_3D('',#192301,#115399,#115400);
#98416=AXIS2_PLACEMENT_3D('',#192304,#115403,#115404);
#98417=AXIS2_PLACEMENT_3D('',#192307,#115405,#115406);
#98418=AXIS2_PLACEMENT_3D('',#192308,#115407,#115408);
#98419=AXIS2_PLACEMENT_3D('',#192309,#115409,#115410);
#98420=AXIS2_PLACEMENT_3D('',#192310,#115411,#115412);
#98421=AXIS2_PLACEMENT_3D('',#192313,#115413,#115414);
#98422=AXIS2_PLACEMENT_3D('',#192314,#115415,#115416);
#98423=AXIS2_PLACEMENT_3D('',#192315,#115417,#115418);
#98424=AXIS2_PLACEMENT_3D('',#192316,#115419,#115420);
#98425=AXIS2_PLACEMENT_3D('',#192319,#115421,#115422);
#98426=AXIS2_PLACEMENT_3D('',#192322,#115425,#115426);
#98427=AXIS2_PLACEMENT_3D('',#192325,#115427,#115428);
#98428=AXIS2_PLACEMENT_3D('',#192326,#115429,#115430);
#98429=AXIS2_PLACEMENT_3D('',#192327,#115431,#115432);
#98430=AXIS2_PLACEMENT_3D('',#192328,#115433,#115434);
#98431=AXIS2_PLACEMENT_3D('',#192329,#115435,#115436);
#98432=AXIS2_PLACEMENT_3D('',#192330,#115437,#115438);
#98433=AXIS2_PLACEMENT_3D('',#192331,#115439,#115440);
#98434=AXIS2_PLACEMENT_3D('',#192334,#115441,#115442);
#98435=AXIS2_PLACEMENT_3D('',#192336,#115443,#115444);
#98436=AXIS2_PLACEMENT_3D('',#192338,#115445,#115446);
#98437=AXIS2_PLACEMENT_3D('',#192339,#115447,#115448);
#98438=AXIS2_PLACEMENT_3D('',#192340,#115449,#115450);
#98439=AXIS2_PLACEMENT_3D('',#192343,#115451,#115452);
#98440=AXIS2_PLACEMENT_3D('',#192346,#115455,#115456);
#98441=AXIS2_PLACEMENT_3D('',#192349,#115457,#115458);
#98442=AXIS2_PLACEMENT_3D('',#192352,#115461,#115462);
#98443=AXIS2_PLACEMENT_3D('',#192355,#115463,#115464);
#98444=AXIS2_PLACEMENT_3D('',#192356,#115465,#115466);
#98445=AXIS2_PLACEMENT_3D('',#192357,#115467,#115468);
#98446=AXIS2_PLACEMENT_3D('',#192358,#115469,#115470);
#98447=AXIS2_PLACEMENT_3D('',#192361,#115471,#115472);
#98448=AXIS2_PLACEMENT_3D('',#192362,#115473,#115474);
#98449=AXIS2_PLACEMENT_3D('',#192363,#115475,#115476);
#98450=AXIS2_PLACEMENT_3D('',#192364,#115477,#115478);
#98451=AXIS2_PLACEMENT_3D('',#192367,#115479,#115480);
#98452=AXIS2_PLACEMENT_3D('',#192370,#115483,#115484);
#98453=AXIS2_PLACEMENT_3D('',#192373,#115485,#115486);
#98454=AXIS2_PLACEMENT_3D('',#192374,#115487,#115488);
#98455=AXIS2_PLACEMENT_3D('',#192375,#115489,#115490);
#98456=AXIS2_PLACEMENT_3D('',#192376,#115491,#115492);
#98457=AXIS2_PLACEMENT_3D('',#192379,#115493,#115494);
#98458=AXIS2_PLACEMENT_3D('',#192380,#115495,#115496);
#98459=AXIS2_PLACEMENT_3D('',#192381,#115497,#115498);
#98460=AXIS2_PLACEMENT_3D('',#192382,#115499,#115500);
#98461=AXIS2_PLACEMENT_3D('',#192385,#115501,#115502);
#98462=AXIS2_PLACEMENT_3D('',#192386,#115503,#115504);
#98463=AXIS2_PLACEMENT_3D('',#192387,#115505,#115506);
#98464=AXIS2_PLACEMENT_3D('',#192388,#115507,#115508);
#98465=AXIS2_PLACEMENT_3D('',#192389,#115509,#115510);
#98466=AXIS2_PLACEMENT_3D('',#192390,#115511,#115512);
#98467=AXIS2_PLACEMENT_3D('',#192391,#115513,#115514);
#98468=AXIS2_PLACEMENT_3D('',#192394,#115515,#115516);
#98469=AXIS2_PLACEMENT_3D('',#192396,#115517,#115518);
#98470=AXIS2_PLACEMENT_3D('',#192398,#115519,#115520);
#98471=AXIS2_PLACEMENT_3D('',#192399,#115521,#115522);
#98472=AXIS2_PLACEMENT_3D('',#192400,#115523,#115524);
#98473=AXIS2_PLACEMENT_3D('',#192403,#115525,#115526);
#98474=AXIS2_PLACEMENT_3D('',#192406,#115529,#115530);
#98475=AXIS2_PLACEMENT_3D('',#192409,#115531,#115532);
#98476=AXIS2_PLACEMENT_3D('',#192412,#115535,#115536);
#98477=AXIS2_PLACEMENT_3D('',#192415,#115537,#115538);
#98478=AXIS2_PLACEMENT_3D('',#192416,#115539,#115540);
#98479=AXIS2_PLACEMENT_3D('',#192417,#115541,#115542);
#98480=AXIS2_PLACEMENT_3D('',#192418,#115543,#115544);
#98481=AXIS2_PLACEMENT_3D('',#192421,#115545,#115546);
#98482=AXIS2_PLACEMENT_3D('',#192422,#115547,#115548);
#98483=AXIS2_PLACEMENT_3D('',#192423,#115549,#115550);
#98484=AXIS2_PLACEMENT_3D('',#192424,#115551,#115552);
#98485=AXIS2_PLACEMENT_3D('',#192427,#115553,#115554);
#98486=AXIS2_PLACEMENT_3D('',#192430,#115557,#115558);
#98487=AXIS2_PLACEMENT_3D('',#192433,#115559,#115560);
#98488=AXIS2_PLACEMENT_3D('',#192434,#115561,#115562);
#98489=AXIS2_PLACEMENT_3D('',#192435,#115563,#115564);
#98490=AXIS2_PLACEMENT_3D('',#192436,#115565,#115566);
#98491=AXIS2_PLACEMENT_3D('',#192437,#115567,#115568);
#98492=AXIS2_PLACEMENT_3D('',#192438,#115569,#115570);
#98493=AXIS2_PLACEMENT_3D('',#192439,#115571,#115572);
#98494=AXIS2_PLACEMENT_3D('',#192442,#115573,#115574);
#98495=AXIS2_PLACEMENT_3D('',#192444,#115575,#115576);
#98496=AXIS2_PLACEMENT_3D('',#192446,#115577,#115578);
#98497=AXIS2_PLACEMENT_3D('',#192447,#115579,#115580);
#98498=AXIS2_PLACEMENT_3D('',#192448,#115581,#115582);
#98499=AXIS2_PLACEMENT_3D('',#192451,#115583,#115584);
#98500=AXIS2_PLACEMENT_3D('',#192454,#115587,#115588);
#98501=AXIS2_PLACEMENT_3D('',#192457,#115589,#115590);
#98502=AXIS2_PLACEMENT_3D('',#192460,#115593,#115594);
#98503=AXIS2_PLACEMENT_3D('',#192463,#115595,#115596);
#98504=AXIS2_PLACEMENT_3D('',#192464,#115597,#115598);
#98505=AXIS2_PLACEMENT_3D('',#192465,#115599,#115600);
#98506=AXIS2_PLACEMENT_3D('',#192466,#115601,#115602);
#98507=AXIS2_PLACEMENT_3D('',#192469,#115603,#115604);
#98508=AXIS2_PLACEMENT_3D('',#192470,#115605,#115606);
#98509=AXIS2_PLACEMENT_3D('',#192471,#115607,#115608);
#98510=AXIS2_PLACEMENT_3D('',#192472,#115609,#115610);
#98511=AXIS2_PLACEMENT_3D('',#192475,#115611,#115612);
#98512=AXIS2_PLACEMENT_3D('',#192478,#115615,#115616);
#98513=AXIS2_PLACEMENT_3D('',#192481,#115617,#115618);
#98514=AXIS2_PLACEMENT_3D('',#192484,#115621,#115622);
#98515=AXIS2_PLACEMENT_3D('',#192485,#115623,#115624);
#98516=AXIS2_PLACEMENT_3D('',#192486,#115625,#115626);
#98517=AXIS2_PLACEMENT_3D('',#192487,#115627,#115628);
#98518=AXIS2_PLACEMENT_3D('',#192490,#115629,#115630);
#98519=AXIS2_PLACEMENT_3D('',#192492,#115631,#115632);
#98520=AXIS2_PLACEMENT_3D('',#192494,#115633,#115634);
#98521=AXIS2_PLACEMENT_3D('',#192495,#115635,#115636);
#98522=AXIS2_PLACEMENT_3D('',#192496,#115637,#115638);
#98523=AXIS2_PLACEMENT_3D('',#192499,#115639,#115640);
#98524=AXIS2_PLACEMENT_3D('',#192502,#115643,#115644);
#98525=AXIS2_PLACEMENT_3D('',#192505,#115645,#115646);
#98526=AXIS2_PLACEMENT_3D('',#192506,#115647,#115648);
#98527=AXIS2_PLACEMENT_3D('',#192507,#115649,#115650);
#98528=AXIS2_PLACEMENT_3D('',#192508,#115651,#115652);
#98529=AXIS2_PLACEMENT_3D('',#192511,#115653,#115654);
#98530=AXIS2_PLACEMENT_3D('',#192512,#115655,#115656);
#98531=AXIS2_PLACEMENT_3D('',#192513,#115657,#115658);
#98532=AXIS2_PLACEMENT_3D('',#192514,#115659,#115660);
#98533=AXIS2_PLACEMENT_3D('',#192517,#115661,#115662);
#98534=AXIS2_PLACEMENT_3D('',#192518,#115663,#115664);
#98535=AXIS2_PLACEMENT_3D('',#192519,#115665,#115666);
#98536=AXIS2_PLACEMENT_3D('',#192520,#115667,#115668);
#98537=AXIS2_PLACEMENT_3D('',#192523,#115669,#115670);
#98538=AXIS2_PLACEMENT_3D('',#192526,#115673,#115674);
#98539=AXIS2_PLACEMENT_3D('',#192529,#115675,#115676);
#98540=AXIS2_PLACEMENT_3D('',#192532,#115679,#115680);
#98541=AXIS2_PLACEMENT_3D('',#192535,#115681,#115682);
#98542=AXIS2_PLACEMENT_3D('',#192536,#115683,#115684);
#98543=AXIS2_PLACEMENT_3D('',#192537,#115685,#115686);
#98544=AXIS2_PLACEMENT_3D('',#192538,#115687,#115688);
#98545=AXIS2_PLACEMENT_3D('',#192541,#115689,#115690);
#98546=AXIS2_PLACEMENT_3D('',#192542,#115691,#115692);
#98547=AXIS2_PLACEMENT_3D('',#192543,#115693,#115694);
#98548=AXIS2_PLACEMENT_3D('',#192544,#115695,#115696);
#98549=AXIS2_PLACEMENT_3D('',#192547,#115699,#115700);
#98550=AXIS2_PLACEMENT_3D('',#192550,#115701,#115702);
#98551=AXIS2_PLACEMENT_3D('',#192552,#115703,#115704);
#98552=AXIS2_PLACEMENT_3D('',#192554,#115705,#115706);
#98553=AXIS2_PLACEMENT_3D('',#192555,#115707,#115708);
#98554=AXIS2_PLACEMENT_3D('',#192556,#115709,#115710);
#98555=AXIS2_PLACEMENT_3D('',#192559,#115711,#115712);
#98556=AXIS2_PLACEMENT_3D('',#192562,#115715,#115716);
#98557=AXIS2_PLACEMENT_3D('',#192565,#115717,#115718);
#98558=AXIS2_PLACEMENT_3D('',#192568,#115721,#115722);
#98559=AXIS2_PLACEMENT_3D('',#192571,#115723,#115724);
#98560=AXIS2_PLACEMENT_3D('',#192572,#115725,#115726);
#98561=AXIS2_PLACEMENT_3D('',#192573,#115727,#115728);
#98562=AXIS2_PLACEMENT_3D('',#192574,#115729,#115730);
#98563=AXIS2_PLACEMENT_3D('',#192577,#115731,#115732);
#98564=AXIS2_PLACEMENT_3D('',#192578,#115733,#115734);
#98565=AXIS2_PLACEMENT_3D('',#192579,#115735,#115736);
#98566=AXIS2_PLACEMENT_3D('',#192580,#115737,#115738);
#98567=AXIS2_PLACEMENT_3D('',#192583,#115739,#115740);
#98568=AXIS2_PLACEMENT_3D('',#192586,#115743,#115744);
#98569=AXIS2_PLACEMENT_3D('',#192589,#115745,#115746);
#98570=AXIS2_PLACEMENT_3D('',#192590,#115747,#115748);
#98571=AXIS2_PLACEMENT_3D('',#192591,#115749,#115750);
#98572=AXIS2_PLACEMENT_3D('',#192592,#115751,#115752);
#98573=AXIS2_PLACEMENT_3D('',#192595,#115753,#115754);
#98574=AXIS2_PLACEMENT_3D('',#192596,#115755,#115756);
#98575=AXIS2_PLACEMENT_3D('',#192597,#115757,#115758);
#98576=AXIS2_PLACEMENT_3D('',#192598,#115759,#115760);
#98577=AXIS2_PLACEMENT_3D('',#192601,#115761,#115762);
#98578=AXIS2_PLACEMENT_3D('',#192602,#115763,#115764);
#98579=AXIS2_PLACEMENT_3D('',#192603,#115765,#115766);
#98580=AXIS2_PLACEMENT_3D('',#192604,#115767,#115768);
#98581=AXIS2_PLACEMENT_3D('',#192607,#115771,#115772);
#98582=AXIS2_PLACEMENT_3D('',#192610,#115773,#115774);
#98583=AXIS2_PLACEMENT_3D('',#192612,#115775,#115776);
#98584=AXIS2_PLACEMENT_3D('',#192614,#115777,#115778);
#98585=AXIS2_PLACEMENT_3D('',#192615,#115779,#115780);
#98586=AXIS2_PLACEMENT_3D('',#192616,#115781,#115782);
#98587=AXIS2_PLACEMENT_3D('',#192619,#115783,#115784);
#98588=AXIS2_PLACEMENT_3D('',#192622,#115787,#115788);
#98589=AXIS2_PLACEMENT_3D('',#192625,#115789,#115790);
#98590=AXIS2_PLACEMENT_3D('',#192628,#115793,#115794);
#98591=AXIS2_PLACEMENT_3D('',#192631,#115795,#115796);
#98592=AXIS2_PLACEMENT_3D('',#192632,#115797,#115798);
#98593=AXIS2_PLACEMENT_3D('',#192633,#115799,#115800);
#98594=AXIS2_PLACEMENT_3D('',#192634,#115801,#115802);
#98595=AXIS2_PLACEMENT_3D('',#192637,#115803,#115804);
#98596=AXIS2_PLACEMENT_3D('',#192638,#115805,#115806);
#98597=AXIS2_PLACEMENT_3D('',#192639,#115807,#115808);
#98598=AXIS2_PLACEMENT_3D('',#192640,#115809,#115810);
#98599=AXIS2_PLACEMENT_3D('',#192643,#115811,#115812);
#98600=AXIS2_PLACEMENT_3D('',#192646,#115815,#115816);
#98601=AXIS2_PLACEMENT_3D('',#192649,#115817,#115818);
#98602=AXIS2_PLACEMENT_3D('',#192652,#115821,#115822);
#98603=AXIS2_PLACEMENT_3D('',#192653,#115823,#115824);
#98604=AXIS2_PLACEMENT_3D('',#192654,#115825,#115826);
#98605=AXIS2_PLACEMENT_3D('',#192655,#115827,#115828);
#98606=AXIS2_PLACEMENT_3D('',#192658,#115829,#115830);
#98607=AXIS2_PLACEMENT_3D('',#192660,#115831,#115832);
#98608=AXIS2_PLACEMENT_3D('',#192662,#115833,#115834);
#98609=AXIS2_PLACEMENT_3D('',#192663,#115835,#115836);
#98610=AXIS2_PLACEMENT_3D('',#192664,#115837,#115838);
#98611=AXIS2_PLACEMENT_3D('',#192667,#115839,#115840);
#98612=AXIS2_PLACEMENT_3D('',#192670,#115843,#115844);
#98613=AXIS2_PLACEMENT_3D('',#192673,#115845,#115846);
#98614=AXIS2_PLACEMENT_3D('',#192676,#115849,#115850);
#98615=AXIS2_PLACEMENT_3D('',#192679,#115851,#115852);
#98616=AXIS2_PLACEMENT_3D('',#192680,#115853,#115854);
#98617=AXIS2_PLACEMENT_3D('',#192681,#115855,#115856);
#98618=AXIS2_PLACEMENT_3D('',#192682,#115857,#115858);
#98619=AXIS2_PLACEMENT_3D('',#192685,#115859,#115860);
#98620=AXIS2_PLACEMENT_3D('',#192686,#115861,#115862);
#98621=AXIS2_PLACEMENT_3D('',#192687,#115863,#115864);
#98622=AXIS2_PLACEMENT_3D('',#192688,#115865,#115866);
#98623=AXIS2_PLACEMENT_3D('',#192691,#115867,#115868);
#98624=AXIS2_PLACEMENT_3D('',#192692,#115869,#115870);
#98625=AXIS2_PLACEMENT_3D('',#192693,#115871,#115872);
#98626=AXIS2_PLACEMENT_3D('',#192694,#115873,#115874);
#98627=AXIS2_PLACEMENT_3D('',#192697,#115875,#115876);
#98628=AXIS2_PLACEMENT_3D('',#192700,#115879,#115880);
#98629=AXIS2_PLACEMENT_3D('',#192701,#115881,#115882);
#98630=AXIS2_PLACEMENT_3D('',#192702,#115883,#115884);
#98631=AXIS2_PLACEMENT_3D('',#192703,#115885,#115886);
#98632=AXIS2_PLACEMENT_3D('',#192706,#115887,#115888);
#98633=AXIS2_PLACEMENT_3D('',#192708,#115889,#115890);
#98634=AXIS2_PLACEMENT_3D('',#192710,#115891,#115892);
#98635=AXIS2_PLACEMENT_3D('',#192711,#115893,#115894);
#98636=AXIS2_PLACEMENT_3D('',#192712,#115895,#115896);
#98637=AXIS2_PLACEMENT_3D('',#192715,#115897,#115898);
#98638=AXIS2_PLACEMENT_3D('',#192718,#115901,#115902);
#98639=AXIS2_PLACEMENT_3D('',#192721,#115903,#115904);
#98640=AXIS2_PLACEMENT_3D('',#192724,#115907,#115908);
#98641=AXIS2_PLACEMENT_3D('',#192727,#115909,#115910);
#98642=AXIS2_PLACEMENT_3D('',#192728,#115911,#115912);
#98643=AXIS2_PLACEMENT_3D('',#192729,#115913,#115914);
#98644=AXIS2_PLACEMENT_3D('',#192730,#115915,#115916);
#98645=AXIS2_PLACEMENT_3D('',#192733,#115917,#115918);
#98646=AXIS2_PLACEMENT_3D('',#192734,#115919,#115920);
#98647=AXIS2_PLACEMENT_3D('',#192735,#115921,#115922);
#98648=AXIS2_PLACEMENT_3D('',#192736,#115923,#115924);
#98649=AXIS2_PLACEMENT_3D('',#192739,#115925,#115926);
#98650=AXIS2_PLACEMENT_3D('',#192742,#115929,#115930);
#98651=AXIS2_PLACEMENT_3D('',#192745,#115931,#115932);
#98652=AXIS2_PLACEMENT_3D('',#192748,#115935,#115936);
#98653=AXIS2_PLACEMENT_3D('',#192749,#115937,#115938);
#98654=AXIS2_PLACEMENT_3D('',#192750,#115939,#115940);
#98655=AXIS2_PLACEMENT_3D('',#192751,#115941,#115942);
#98656=AXIS2_PLACEMENT_3D('',#192754,#115943,#115944);
#98657=AXIS2_PLACEMENT_3D('',#192756,#115945,#115946);
#98658=AXIS2_PLACEMENT_3D('',#192758,#115947,#115948);
#98659=AXIS2_PLACEMENT_3D('',#192759,#115949,#115950);
#98660=AXIS2_PLACEMENT_3D('',#192760,#115951,#115952);
#98661=AXIS2_PLACEMENT_3D('',#192763,#115953,#115954);
#98662=AXIS2_PLACEMENT_3D('',#192766,#115957,#115958);
#98663=AXIS2_PLACEMENT_3D('',#192769,#115959,#115960);
#98664=AXIS2_PLACEMENT_3D('',#192772,#115963,#115964);
#98665=AXIS2_PLACEMENT_3D('',#192775,#115965,#115966);
#98666=AXIS2_PLACEMENT_3D('',#192776,#115967,#115968);
#98667=AXIS2_PLACEMENT_3D('',#192777,#115969,#115970);
#98668=AXIS2_PLACEMENT_3D('',#192778,#115971,#115972);
#98669=AXIS2_PLACEMENT_3D('',#192781,#115973,#115974);
#98670=AXIS2_PLACEMENT_3D('',#192782,#115975,#115976);
#98671=AXIS2_PLACEMENT_3D('',#192783,#115977,#115978);
#98672=AXIS2_PLACEMENT_3D('',#192784,#115979,#115980);
#98673=AXIS2_PLACEMENT_3D('',#192787,#115981,#115982);
#98674=AXIS2_PLACEMENT_3D('',#192790,#115985,#115986);
#98675=AXIS2_PLACEMENT_3D('',#192793,#115987,#115988);
#98676=AXIS2_PLACEMENT_3D('',#192796,#115991,#115992);
#98677=AXIS2_PLACEMENT_3D('',#192797,#115993,#115994);
#98678=AXIS2_PLACEMENT_3D('',#192798,#115995,#115996);
#98679=AXIS2_PLACEMENT_3D('',#192799,#115997,#115998);
#98680=AXIS2_PLACEMENT_3D('',#192802,#115999,#116000);
#98681=AXIS2_PLACEMENT_3D('',#192804,#116001,#116002);
#98682=AXIS2_PLACEMENT_3D('',#192806,#116003,#116004);
#98683=AXIS2_PLACEMENT_3D('',#192807,#116005,#116006);
#98684=AXIS2_PLACEMENT_3D('',#192808,#116007,#116008);
#98685=AXIS2_PLACEMENT_3D('',#192811,#116009,#116010);
#98686=AXIS2_PLACEMENT_3D('',#192814,#116013,#116014);
#98687=AXIS2_PLACEMENT_3D('',#192817,#116015,#116016);
#98688=AXIS2_PLACEMENT_3D('',#192820,#116019,#116020);
#98689=AXIS2_PLACEMENT_3D('',#192823,#116021,#116022);
#98690=AXIS2_PLACEMENT_3D('',#192824,#116023,#116024);
#98691=AXIS2_PLACEMENT_3D('',#192825,#116025,#116026);
#98692=AXIS2_PLACEMENT_3D('',#192826,#116027,#116028);
#98693=AXIS2_PLACEMENT_3D('',#192829,#116029,#116030);
#98694=AXIS2_PLACEMENT_3D('',#192830,#116031,#116032);
#98695=AXIS2_PLACEMENT_3D('',#192831,#116033,#116034);
#98696=AXIS2_PLACEMENT_3D('',#192832,#116035,#116036);
#98697=AXIS2_PLACEMENT_3D('',#192835,#116037,#116038);
#98698=AXIS2_PLACEMENT_3D('',#192838,#116041,#116042);
#98699=AXIS2_PLACEMENT_3D('',#192841,#116043,#116044);
#98700=AXIS2_PLACEMENT_3D('',#192842,#116045,#116046);
#98701=AXIS2_PLACEMENT_3D('',#192843,#116047,#116048);
#98702=AXIS2_PLACEMENT_3D('',#192844,#116049,#116050);
#98703=AXIS2_PLACEMENT_3D('',#192846,#116051,#116052);
#98704=AXIS2_PLACEMENT_3D('',#192848,#116053,#116054);
#98705=AXIS2_PLACEMENT_3D('',#192849,#116055,#116056);
#98706=AXIS2_PLACEMENT_3D('',#192850,#116057,#116058);
#98707=AXIS2_PLACEMENT_3D('',#192851,#116059,#116060);
#98708=AXIS2_PLACEMENT_3D('',#192852,#116061,#116062);
#98709=AXIS2_PLACEMENT_3D('',#192853,#116063,#116064);
#98710=AXIS2_PLACEMENT_3D('',#192856,#116065,#116066);
#98711=AXIS2_PLACEMENT_3D('',#192858,#116067,#116068);
#98712=AXIS2_PLACEMENT_3D('',#192860,#116069,#116070);
#98713=AXIS2_PLACEMENT_3D('',#192861,#116071,#116072);
#98714=AXIS2_PLACEMENT_3D('',#192862,#116073,#116074);
#98715=AXIS2_PLACEMENT_3D('',#192865,#116075,#116076);
#98716=AXIS2_PLACEMENT_3D('',#192868,#116079,#116080);
#98717=AXIS2_PLACEMENT_3D('',#192871,#116081,#116082);
#98718=AXIS2_PLACEMENT_3D('',#192874,#116085,#116086);
#98719=AXIS2_PLACEMENT_3D('',#192877,#116087,#116088);
#98720=AXIS2_PLACEMENT_3D('',#192878,#116089,#116090);
#98721=AXIS2_PLACEMENT_3D('',#192879,#116091,#116092);
#98722=AXIS2_PLACEMENT_3D('',#192880,#116093,#116094);
#98723=AXIS2_PLACEMENT_3D('',#192883,#116095,#116096);
#98724=AXIS2_PLACEMENT_3D('',#192884,#116097,#116098);
#98725=AXIS2_PLACEMENT_3D('',#192885,#116099,#116100);
#98726=AXIS2_PLACEMENT_3D('',#192886,#116101,#116102);
#98727=AXIS2_PLACEMENT_3D('',#192889,#116103,#116104);
#98728=AXIS2_PLACEMENT_3D('',#192890,#116105,#116106);
#98729=AXIS2_PLACEMENT_3D('',#192891,#116107,#116108);
#98730=AXIS2_PLACEMENT_3D('',#192892,#116109,#116110);
#98731=AXIS2_PLACEMENT_3D('',#192895,#116111,#116112);
#98732=AXIS2_PLACEMENT_3D('',#192898,#116115,#116116);
#98733=AXIS2_PLACEMENT_3D('',#192899,#116117,#116118);
#98734=AXIS2_PLACEMENT_3D('',#192900,#116119,#116120);
#98735=AXIS2_PLACEMENT_3D('',#192901,#116121,#116122);
#98736=AXIS2_PLACEMENT_3D('',#192904,#116123,#116124);
#98737=AXIS2_PLACEMENT_3D('',#192906,#116125,#116126);
#98738=AXIS2_PLACEMENT_3D('',#192908,#116127,#116128);
#98739=AXIS2_PLACEMENT_3D('',#192909,#116129,#116130);
#98740=AXIS2_PLACEMENT_3D('',#192910,#116131,#116132);
#98741=AXIS2_PLACEMENT_3D('',#192913,#116133,#116134);
#98742=AXIS2_PLACEMENT_3D('',#192916,#116137,#116138);
#98743=AXIS2_PLACEMENT_3D('',#192919,#116139,#116140);
#98744=AXIS2_PLACEMENT_3D('',#192922,#116143,#116144);
#98745=AXIS2_PLACEMENT_3D('',#192925,#116145,#116146);
#98746=AXIS2_PLACEMENT_3D('',#192926,#116147,#116148);
#98747=AXIS2_PLACEMENT_3D('',#192927,#116149,#116150);
#98748=AXIS2_PLACEMENT_3D('',#192928,#116151,#116152);
#98749=AXIS2_PLACEMENT_3D('',#192931,#116153,#116154);
#98750=AXIS2_PLACEMENT_3D('',#192932,#116155,#116156);
#98751=AXIS2_PLACEMENT_3D('',#192933,#116157,#116158);
#98752=AXIS2_PLACEMENT_3D('',#192934,#116159,#116160);
#98753=AXIS2_PLACEMENT_3D('',#192937,#116161,#116162);
#98754=AXIS2_PLACEMENT_3D('',#192938,#116163,#116164);
#98755=AXIS2_PLACEMENT_3D('',#192939,#116165,#116166);
#98756=AXIS2_PLACEMENT_3D('',#192940,#116167,#116168);
#98757=AXIS2_PLACEMENT_3D('',#192943,#116169,#116170);
#98758=AXIS2_PLACEMENT_3D('',#192946,#116173,#116174);
#98759=AXIS2_PLACEMENT_3D('',#192949,#116175,#116176);
#98760=AXIS2_PLACEMENT_3D('',#192950,#116177,#116178);
#98761=AXIS2_PLACEMENT_3D('',#192951,#116179,#116180);
#98762=AXIS2_PLACEMENT_3D('',#192952,#116181,#116182);
#98763=AXIS2_PLACEMENT_3D('',#192955,#116183,#116184);
#98764=AXIS2_PLACEMENT_3D('',#192956,#116185,#116186);
#98765=AXIS2_PLACEMENT_3D('',#192957,#116187,#116188);
#98766=AXIS2_PLACEMENT_3D('',#192958,#116189,#116190);
#98767=AXIS2_PLACEMENT_3D('',#192959,#116191,#116192);
#98768=AXIS2_PLACEMENT_3D('',#192960,#116193,#116194);
#98769=AXIS2_PLACEMENT_3D('',#192961,#116195,#116196);
#98770=AXIS2_PLACEMENT_3D('',#192964,#116197,#116198);
#98771=AXIS2_PLACEMENT_3D('',#192966,#116199,#116200);
#98772=AXIS2_PLACEMENT_3D('',#192968,#116201,#116202);
#98773=AXIS2_PLACEMENT_3D('',#192969,#116203,#116204);
#98774=AXIS2_PLACEMENT_3D('',#192970,#116205,#116206);
#98775=AXIS2_PLACEMENT_3D('',#192973,#116207,#116208);
#98776=AXIS2_PLACEMENT_3D('',#192976,#116211,#116212);
#98777=AXIS2_PLACEMENT_3D('',#192979,#116213,#116214);
#98778=AXIS2_PLACEMENT_3D('',#192982,#116217,#116218);
#98779=AXIS2_PLACEMENT_3D('',#192985,#116219,#116220);
#98780=AXIS2_PLACEMENT_3D('',#192986,#116221,#116222);
#98781=AXIS2_PLACEMENT_3D('',#192987,#116223,#116224);
#98782=AXIS2_PLACEMENT_3D('',#192988,#116225,#116226);
#98783=AXIS2_PLACEMENT_3D('',#192991,#116227,#116228);
#98784=AXIS2_PLACEMENT_3D('',#192992,#116229,#116230);
#98785=AXIS2_PLACEMENT_3D('',#192993,#116231,#116232);
#98786=AXIS2_PLACEMENT_3D('',#192994,#116233,#116234);
#98787=AXIS2_PLACEMENT_3D('',#192997,#116235,#116236);
#98788=AXIS2_PLACEMENT_3D('',#193000,#116239,#116240);
#98789=AXIS2_PLACEMENT_3D('',#193003,#116241,#116242);
#98790=AXIS2_PLACEMENT_3D('',#193006,#116245,#116246);
#98791=AXIS2_PLACEMENT_3D('',#193007,#116247,#116248);
#98792=AXIS2_PLACEMENT_3D('',#193008,#116249,#116250);
#98793=AXIS2_PLACEMENT_3D('',#193009,#116251,#116252);
#98794=AXIS2_PLACEMENT_3D('',#193012,#116253,#116254);
#98795=AXIS2_PLACEMENT_3D('',#193014,#116255,#116256);
#98796=AXIS2_PLACEMENT_3D('',#193016,#116257,#116258);
#98797=AXIS2_PLACEMENT_3D('',#193017,#116259,#116260);
#98798=AXIS2_PLACEMENT_3D('',#193018,#116261,#116262);
#98799=AXIS2_PLACEMENT_3D('',#193021,#116263,#116264);
#98800=AXIS2_PLACEMENT_3D('',#193024,#116267,#116268);
#98801=AXIS2_PLACEMENT_3D('',#193027,#116269,#116270);
#98802=AXIS2_PLACEMENT_3D('',#193030,#116273,#116274);
#98803=AXIS2_PLACEMENT_3D('',#193033,#116275,#116276);
#98804=AXIS2_PLACEMENT_3D('',#193034,#116277,#116278);
#98805=AXIS2_PLACEMENT_3D('',#193035,#116279,#116280);
#98806=AXIS2_PLACEMENT_3D('',#193036,#116281,#116282);
#98807=AXIS2_PLACEMENT_3D('',#193039,#116283,#116284);
#98808=AXIS2_PLACEMENT_3D('',#193040,#116285,#116286);
#98809=AXIS2_PLACEMENT_3D('',#193041,#116287,#116288);
#98810=AXIS2_PLACEMENT_3D('',#193042,#116289,#116290);
#98811=AXIS2_PLACEMENT_3D('',#193045,#116291,#116292);
#98812=AXIS2_PLACEMENT_3D('',#193048,#116295,#116296);
#98813=AXIS2_PLACEMENT_3D('',#193051,#116297,#116298);
#98814=AXIS2_PLACEMENT_3D('',#193052,#116299,#116300);
#98815=AXIS2_PLACEMENT_3D('',#193053,#116301,#116302);
#98816=AXIS2_PLACEMENT_3D('',#193054,#116303,#116304);
#98817=AXIS2_PLACEMENT_3D('',#193057,#116305,#116306);
#98818=AXIS2_PLACEMENT_3D('',#193058,#116307,#116308);
#98819=AXIS2_PLACEMENT_3D('',#193059,#116309,#116310);
#98820=AXIS2_PLACEMENT_3D('',#193060,#116311,#116312);
#98821=AXIS2_PLACEMENT_3D('',#193063,#116313,#116314);
#98822=AXIS2_PLACEMENT_3D('',#193064,#116315,#116316);
#98823=AXIS2_PLACEMENT_3D('',#193065,#116317,#116318);
#98824=AXIS2_PLACEMENT_3D('',#193066,#116319,#116320);
#98825=AXIS2_PLACEMENT_3D('',#193067,#116321,#116322);
#98826=AXIS2_PLACEMENT_3D('',#193068,#116323,#116324);
#98827=AXIS2_PLACEMENT_3D('',#193069,#116325,#116326);
#98828=AXIS2_PLACEMENT_3D('',#193072,#116327,#116328);
#98829=AXIS2_PLACEMENT_3D('',#193074,#116329,#116330);
#98830=AXIS2_PLACEMENT_3D('',#193076,#116331,#116332);
#98831=AXIS2_PLACEMENT_3D('',#193077,#116333,#116334);
#98832=AXIS2_PLACEMENT_3D('',#193078,#116335,#116336);
#98833=AXIS2_PLACEMENT_3D('',#193081,#116337,#116338);
#98834=AXIS2_PLACEMENT_3D('',#193084,#116341,#116342);
#98835=AXIS2_PLACEMENT_3D('',#193087,#116343,#116344);
#98836=AXIS2_PLACEMENT_3D('',#193090,#116347,#116348);
#98837=AXIS2_PLACEMENT_3D('',#193093,#116349,#116350);
#98838=AXIS2_PLACEMENT_3D('',#193094,#116351,#116352);
#98839=AXIS2_PLACEMENT_3D('',#193095,#116353,#116354);
#98840=AXIS2_PLACEMENT_3D('',#193096,#116355,#116356);
#98841=AXIS2_PLACEMENT_3D('',#193099,#116357,#116358);
#98842=AXIS2_PLACEMENT_3D('',#193100,#116359,#116360);
#98843=AXIS2_PLACEMENT_3D('',#193101,#116361,#116362);
#98844=AXIS2_PLACEMENT_3D('',#193102,#116363,#116364);
#98845=AXIS2_PLACEMENT_3D('',#193105,#116365,#116366);
#98846=AXIS2_PLACEMENT_3D('',#193108,#116369,#116370);
#98847=AXIS2_PLACEMENT_3D('',#193111,#116371,#116372);
#98848=AXIS2_PLACEMENT_3D('',#193112,#116373,#116374);
#98849=AXIS2_PLACEMENT_3D('',#193113,#116375,#116376);
#98850=AXIS2_PLACEMENT_3D('',#193114,#116377,#116378);
#98851=AXIS2_PLACEMENT_3D('',#193115,#116379,#116380);
#98852=AXIS2_PLACEMENT_3D('',#193116,#116381,#116382);
#98853=AXIS2_PLACEMENT_3D('',#193117,#116383,#116384);
#98854=AXIS2_PLACEMENT_3D('',#193120,#116385,#116386);
#98855=AXIS2_PLACEMENT_3D('',#193122,#116387,#116388);
#98856=AXIS2_PLACEMENT_3D('',#193124,#116389,#116390);
#98857=AXIS2_PLACEMENT_3D('',#193125,#116391,#116392);
#98858=AXIS2_PLACEMENT_3D('',#193126,#116393,#116394);
#98859=AXIS2_PLACEMENT_3D('',#193129,#116395,#116396);
#98860=AXIS2_PLACEMENT_3D('',#193132,#116399,#116400);
#98861=AXIS2_PLACEMENT_3D('',#193135,#116401,#116402);
#98862=AXIS2_PLACEMENT_3D('',#193138,#116405,#116406);
#98863=AXIS2_PLACEMENT_3D('',#193141,#116407,#116408);
#98864=AXIS2_PLACEMENT_3D('',#193142,#116409,#116410);
#98865=AXIS2_PLACEMENT_3D('',#193143,#116411,#116412);
#98866=AXIS2_PLACEMENT_3D('',#193144,#116413,#116414);
#98867=AXIS2_PLACEMENT_3D('',#193147,#116415,#116416);
#98868=AXIS2_PLACEMENT_3D('',#193148,#116417,#116418);
#98869=AXIS2_PLACEMENT_3D('',#193149,#116419,#116420);
#98870=AXIS2_PLACEMENT_3D('',#193150,#116421,#116422);
#98871=AXIS2_PLACEMENT_3D('',#193153,#116423,#116424);
#98872=AXIS2_PLACEMENT_3D('',#193156,#116427,#116428);
#98873=AXIS2_PLACEMENT_3D('',#193159,#116429,#116430);
#98874=AXIS2_PLACEMENT_3D('',#193162,#116433,#116434);
#98875=AXIS2_PLACEMENT_3D('',#193163,#116435,#116436);
#98876=AXIS2_PLACEMENT_3D('',#193164,#116437,#116438);
#98877=AXIS2_PLACEMENT_3D('',#193165,#116439,#116440);
#98878=AXIS2_PLACEMENT_3D('',#193168,#116441,#116442);
#98879=AXIS2_PLACEMENT_3D('',#193170,#116443,#116444);
#98880=AXIS2_PLACEMENT_3D('',#193172,#116445,#116446);
#98881=AXIS2_PLACEMENT_3D('',#193173,#116447,#116448);
#98882=AXIS2_PLACEMENT_3D('',#193174,#116449,#116450);
#98883=AXIS2_PLACEMENT_3D('',#193177,#116451,#116452);
#98884=AXIS2_PLACEMENT_3D('',#193180,#116455,#116456);
#98885=AXIS2_PLACEMENT_3D('',#193183,#116457,#116458);
#98886=AXIS2_PLACEMENT_3D('',#193186,#116461,#116462);
#98887=AXIS2_PLACEMENT_3D('',#193189,#116463,#116464);
#98888=AXIS2_PLACEMENT_3D('',#193190,#116465,#116466);
#98889=AXIS2_PLACEMENT_3D('',#193191,#116467,#116468);
#98890=AXIS2_PLACEMENT_3D('',#193192,#116469,#116470);
#98891=AXIS2_PLACEMENT_3D('',#193195,#116471,#116472);
#98892=AXIS2_PLACEMENT_3D('',#193196,#116473,#116474);
#98893=AXIS2_PLACEMENT_3D('',#193197,#116475,#116476);
#98894=AXIS2_PLACEMENT_3D('',#193198,#116477,#116478);
#98895=AXIS2_PLACEMENT_3D('',#193201,#116479,#116480);
#98896=AXIS2_PLACEMENT_3D('',#193204,#116483,#116484);
#98897=AXIS2_PLACEMENT_3D('',#193207,#116485,#116486);
#98898=AXIS2_PLACEMENT_3D('',#193208,#116487,#116488);
#98899=AXIS2_PLACEMENT_3D('',#193209,#116489,#116490);
#98900=AXIS2_PLACEMENT_3D('',#193210,#116491,#116492);
#98901=AXIS2_PLACEMENT_3D('',#193211,#116493,#116494);
#98902=AXIS2_PLACEMENT_3D('',#193212,#116495,#116496);
#98903=AXIS2_PLACEMENT_3D('',#193213,#116497,#116498);
#98904=AXIS2_PLACEMENT_3D('',#193216,#116499,#116500);
#98905=AXIS2_PLACEMENT_3D('',#193218,#116501,#116502);
#98906=AXIS2_PLACEMENT_3D('',#193220,#116503,#116504);
#98907=AXIS2_PLACEMENT_3D('',#193221,#116505,#116506);
#98908=AXIS2_PLACEMENT_3D('',#193222,#116507,#116508);
#98909=AXIS2_PLACEMENT_3D('',#193225,#116509,#116510);
#98910=AXIS2_PLACEMENT_3D('',#193228,#116513,#116514);
#98911=AXIS2_PLACEMENT_3D('',#193231,#116515,#116516);
#98912=AXIS2_PLACEMENT_3D('',#193234,#116519,#116520);
#98913=AXIS2_PLACEMENT_3D('',#193237,#116521,#116522);
#98914=AXIS2_PLACEMENT_3D('',#193238,#116523,#116524);
#98915=AXIS2_PLACEMENT_3D('',#193239,#116525,#116526);
#98916=AXIS2_PLACEMENT_3D('',#193240,#116527,#116528);
#98917=AXIS2_PLACEMENT_3D('',#193243,#116529,#116530);
#98918=AXIS2_PLACEMENT_3D('',#193244,#116531,#116532);
#98919=AXIS2_PLACEMENT_3D('',#193245,#116533,#116534);
#98920=AXIS2_PLACEMENT_3D('',#193246,#116535,#116536);
#98921=AXIS2_PLACEMENT_3D('',#193249,#116537,#116538);
#98922=AXIS2_PLACEMENT_3D('',#193252,#116541,#116542);
#98923=AXIS2_PLACEMENT_3D('',#193255,#116543,#116544);
#98924=AXIS2_PLACEMENT_3D('',#193258,#116547,#116548);
#98925=AXIS2_PLACEMENT_3D('',#193259,#116549,#116550);
#98926=AXIS2_PLACEMENT_3D('',#193260,#116551,#116552);
#98927=AXIS2_PLACEMENT_3D('',#193261,#116553,#116554);
#98928=AXIS2_PLACEMENT_3D('',#193264,#116555,#116556);
#98929=AXIS2_PLACEMENT_3D('',#193266,#116557,#116558);
#98930=AXIS2_PLACEMENT_3D('',#193268,#116559,#116560);
#98931=AXIS2_PLACEMENT_3D('',#193269,#116561,#116562);
#98932=AXIS2_PLACEMENT_3D('',#193270,#116563,#116564);
#98933=AXIS2_PLACEMENT_3D('',#193273,#116565,#116566);
#98934=AXIS2_PLACEMENT_3D('',#193276,#116569,#116570);
#98935=AXIS2_PLACEMENT_3D('',#193279,#116571,#116572);
#98936=AXIS2_PLACEMENT_3D('',#193280,#116573,#116574);
#98937=AXIS2_PLACEMENT_3D('',#193281,#116575,#116576);
#98938=AXIS2_PLACEMENT_3D('',#193282,#116577,#116578);
#98939=AXIS2_PLACEMENT_3D('',#193285,#116579,#116580);
#98940=AXIS2_PLACEMENT_3D('',#193286,#116581,#116582);
#98941=AXIS2_PLACEMENT_3D('',#193287,#116583,#116584);
#98942=AXIS2_PLACEMENT_3D('',#193288,#116585,#116586);
#98943=AXIS2_PLACEMENT_3D('',#193291,#116587,#116588);
#98944=AXIS2_PLACEMENT_3D('',#193292,#116589,#116590);
#98945=AXIS2_PLACEMENT_3D('',#193293,#116591,#116592);
#98946=AXIS2_PLACEMENT_3D('',#193294,#116593,#116594);
#98947=AXIS2_PLACEMENT_3D('',#193297,#116597,#116598);
#98948=AXIS2_PLACEMENT_3D('',#193300,#116599,#116600);
#98949=AXIS2_PLACEMENT_3D('',#193302,#116601,#116602);
#98950=AXIS2_PLACEMENT_3D('',#193304,#116603,#116604);
#98951=AXIS2_PLACEMENT_3D('',#193305,#116605,#116606);
#98952=AXIS2_PLACEMENT_3D('',#193306,#116607,#116608);
#98953=AXIS2_PLACEMENT_3D('',#193309,#116609,#116610);
#98954=AXIS2_PLACEMENT_3D('',#193312,#116613,#116614);
#98955=AXIS2_PLACEMENT_3D('',#193315,#116615,#116616);
#98956=AXIS2_PLACEMENT_3D('',#193316,#116617,#116618);
#98957=AXIS2_PLACEMENT_3D('',#193317,#116619,#116620);
#98958=AXIS2_PLACEMENT_3D('',#193318,#116621,#116622);
#98959=AXIS2_PLACEMENT_3D('',#193321,#116623,#116624);
#98960=AXIS2_PLACEMENT_3D('',#193322,#116625,#116626);
#98961=AXIS2_PLACEMENT_3D('',#193323,#116627,#116628);
#98962=AXIS2_PLACEMENT_3D('',#193324,#116629,#116630);
#98963=AXIS2_PLACEMENT_3D('',#193327,#116631,#116632);
#98964=AXIS2_PLACEMENT_3D('',#193328,#116633,#116634);
#98965=AXIS2_PLACEMENT_3D('',#193329,#116635,#116636);
#98966=AXIS2_PLACEMENT_3D('',#193330,#116637,#116638);
#98967=AXIS2_PLACEMENT_3D('',#193333,#116641,#116642);
#98968=AXIS2_PLACEMENT_3D('',#193336,#116643,#116644);
#98969=AXIS2_PLACEMENT_3D('',#193338,#116645,#116646);
#98970=AXIS2_PLACEMENT_3D('',#193340,#116647,#116648);
#98971=AXIS2_PLACEMENT_3D('',#193341,#116649,#116650);
#98972=AXIS2_PLACEMENT_3D('',#193342,#116651,#116652);
#98973=AXIS2_PLACEMENT_3D('',#193345,#116653,#116654);
#98974=AXIS2_PLACEMENT_3D('',#193346,#116655,#116656);
#98975=AXIS2_PLACEMENT_3D('',#193347,#116657,#116658);
#98976=AXIS2_PLACEMENT_3D('',#193348,#116659,#116660);
#98977=AXIS2_PLACEMENT_3D('',#193351,#116661,#116662);
#98978=AXIS2_PLACEMENT_3D('',#193352,#116663,#116664);
#98979=AXIS2_PLACEMENT_3D('',#193353,#116665,#116666);
#98980=AXIS2_PLACEMENT_3D('',#193354,#116667,#116668);
#98981=AXIS2_PLACEMENT_3D('',#193357,#116669,#116670);
#98982=AXIS2_PLACEMENT_3D('',#193358,#116671,#116672);
#98983=AXIS2_PLACEMENT_3D('',#193359,#116673,#116674);
#98984=AXIS2_PLACEMENT_3D('',#193360,#116675,#116676);
#98985=AXIS2_PLACEMENT_3D('',#193363,#116677,#116678);
#98986=AXIS2_PLACEMENT_3D('',#193364,#116679,#116680);
#98987=AXIS2_PLACEMENT_3D('',#193365,#116681,#116682);
#98988=AXIS2_PLACEMENT_3D('',#193366,#116683,#116684);
#98989=AXIS2_PLACEMENT_3D('',#193369,#116685,#116686);
#98990=AXIS2_PLACEMENT_3D('',#193370,#116687,#116688);
#98991=AXIS2_PLACEMENT_3D('',#193371,#116689,#116690);
#98992=AXIS2_PLACEMENT_3D('',#193372,#116691,#116692);
#98993=AXIS2_PLACEMENT_3D('',#193375,#116693,#116694);
#98994=AXIS2_PLACEMENT_3D('',#193376,#116695,#116696);
#98995=AXIS2_PLACEMENT_3D('',#193377,#116697,#116698);
#98996=AXIS2_PLACEMENT_3D('',#193378,#116699,#116700);
#98997=AXIS2_PLACEMENT_3D('',#193381,#116701,#116702);
#98998=AXIS2_PLACEMENT_3D('',#193383,#116703,#116704);
#98999=AXIS2_PLACEMENT_3D('',#193385,#116705,#116706);
#99000=AXIS2_PLACEMENT_3D('',#193386,#116707,#116708);
#99001=AXIS2_PLACEMENT_3D('',#193387,#116709,#116710);
#99002=AXIS2_PLACEMENT_3D('',#193390,#116711,#116712);
#99003=AXIS2_PLACEMENT_3D('',#193391,#116713,#116714);
#99004=AXIS2_PLACEMENT_3D('',#193392,#116715,#116716);
#99005=AXIS2_PLACEMENT_3D('',#193393,#116717,#116718);
#99006=AXIS2_PLACEMENT_3D('',#193396,#116719,#116720);
#99007=AXIS2_PLACEMENT_3D('',#193397,#116721,#116722);
#99008=AXIS2_PLACEMENT_3D('',#193398,#116723,#116724);
#99009=AXIS2_PLACEMENT_3D('',#193399,#116725,#116726);
#99010=AXIS2_PLACEMENT_3D('',#193402,#116727,#116728);
#99011=AXIS2_PLACEMENT_3D('',#193403,#116729,#116730);
#99012=AXIS2_PLACEMENT_3D('',#193404,#116731,#116732);
#99013=AXIS2_PLACEMENT_3D('',#193405,#116733,#116734);
#99014=AXIS2_PLACEMENT_3D('',#193408,#116735,#116736);
#99015=AXIS2_PLACEMENT_3D('',#193409,#116737,#116738);
#99016=AXIS2_PLACEMENT_3D('',#193410,#116739,#116740);
#99017=AXIS2_PLACEMENT_3D('',#193411,#116741,#116742);
#99018=AXIS2_PLACEMENT_3D('',#193414,#116743,#116744);
#99019=AXIS2_PLACEMENT_3D('',#193415,#116745,#116746);
#99020=AXIS2_PLACEMENT_3D('',#193416,#116747,#116748);
#99021=AXIS2_PLACEMENT_3D('',#193417,#116749,#116750);
#99022=AXIS2_PLACEMENT_3D('',#193420,#116751,#116752);
#99023=AXIS2_PLACEMENT_3D('',#193421,#116753,#116754);
#99024=AXIS2_PLACEMENT_3D('',#193422,#116755,#116756);
#99025=AXIS2_PLACEMENT_3D('',#193423,#116757,#116758);
#99026=AXIS2_PLACEMENT_3D('',#193426,#116759,#116760);
#99027=AXIS2_PLACEMENT_3D('',#193428,#116761,#116762);
#99028=AXIS2_PLACEMENT_3D('',#193440,#116763,#116764);
#99029=AXIS2_PLACEMENT_3D('',#193441,#116765,#116766);
#99030=AXIS2_PLACEMENT_3D('',#193444,#116767,#116768);
#99031=AXIS2_PLACEMENT_3D('',#193447,#116771,#116772);
#99032=AXIS2_PLACEMENT_3D('',#193449,#116773,#116774);
#99033=AXIS2_PLACEMENT_3D('',#193451,#116775,#116776);
#99034=AXIS2_PLACEMENT_3D('',#193452,#116777,#116778);
#99035=AXIS2_PLACEMENT_3D('',#193453,#116779,#116780);
#99036=AXIS2_PLACEMENT_3D('',#193456,#116781,#116782);
#99037=AXIS2_PLACEMENT_3D('',#193457,#116783,#116784);
#99038=AXIS2_PLACEMENT_3D('',#193458,#116785,#116786);
#99039=AXIS2_PLACEMENT_3D('',#193459,#116787,#116788);
#99040=AXIS2_PLACEMENT_3D('',#193462,#116789,#116790);
#99041=AXIS2_PLACEMENT_3D('',#193463,#116791,#116792);
#99042=AXIS2_PLACEMENT_3D('',#193464,#116793,#116794);
#99043=AXIS2_PLACEMENT_3D('',#193465,#116795,#116796);
#99044=AXIS2_PLACEMENT_3D('',#193468,#116797,#116798);
#99045=AXIS2_PLACEMENT_3D('',#193471,#116801,#116802);
#99046=AXIS2_PLACEMENT_3D('',#193484,#116803,#116804);
#99047=AXIS2_PLACEMENT_3D('',#193485,#116805,#116806);
#99048=AXIS2_PLACEMENT_3D('',#193486,#116807,#116808);
#99049=AXIS2_PLACEMENT_3D('',#193489,#116809,#116810);
#99050=AXIS2_PLACEMENT_3D('',#193491,#116811,#116812);
#99051=AXIS2_PLACEMENT_3D('',#193503,#116813,#116814);
#99052=AXIS2_PLACEMENT_3D('',#193504,#116815,#116816);
#99053=AXIS2_PLACEMENT_3D('',#193507,#116817,#116818);
#99054=AXIS2_PLACEMENT_3D('',#193510,#116821,#116822);
#99055=AXIS2_PLACEMENT_3D('',#193513,#116823,#116824);
#99056=AXIS2_PLACEMENT_3D('',#193514,#116825,#116826);
#99057=AXIS2_PLACEMENT_3D('',#193515,#116827,#116828);
#99058=AXIS2_PLACEMENT_3D('',#193516,#116829,#116830);
#99059=AXIS2_PLACEMENT_3D('',#193519,#116831,#116832);
#99060=AXIS2_PLACEMENT_3D('',#193520,#116833,#116834);
#99061=AXIS2_PLACEMENT_3D('',#193521,#116835,#116836);
#99062=AXIS2_PLACEMENT_3D('',#193522,#116837,#116838);
#99063=AXIS2_PLACEMENT_3D('',#193525,#116839,#116840);
#99064=AXIS2_PLACEMENT_3D('',#193526,#116841,#116842);
#99065=AXIS2_PLACEMENT_3D('',#193527,#116843,#116844);
#99066=AXIS2_PLACEMENT_3D('',#193528,#116845,#116846);
#99067=AXIS2_PLACEMENT_3D('',#193531,#116847,#116848);
#99068=AXIS2_PLACEMENT_3D('',#193534,#116851,#116852);
#99069=AXIS2_PLACEMENT_3D('',#193547,#116853,#116854);
#99070=AXIS2_PLACEMENT_3D('',#193548,#116855,#116856);
#99071=AXIS2_PLACEMENT_3D('',#193549,#116857,#116858);
#99072=AXIS2_PLACEMENT_3D('',#193552,#116859,#116860);
#99073=AXIS2_PLACEMENT_3D('',#193554,#116861,#116862);
#99074=AXIS2_PLACEMENT_3D('',#193566,#116863,#116864);
#99075=AXIS2_PLACEMENT_3D('',#193567,#116865,#116866);
#99076=AXIS2_PLACEMENT_3D('',#193570,#116867,#116868);
#99077=AXIS2_PLACEMENT_3D('',#193573,#116871,#116872);
#99078=AXIS2_PLACEMENT_3D('',#193575,#116873,#116874);
#99079=AXIS2_PLACEMENT_3D('',#193577,#116875,#116876);
#99080=AXIS2_PLACEMENT_3D('',#193578,#116877,#116878);
#99081=AXIS2_PLACEMENT_3D('',#193579,#116879,#116880);
#99082=AXIS2_PLACEMENT_3D('',#193582,#116881,#116882);
#99083=AXIS2_PLACEMENT_3D('',#193583,#116883,#116884);
#99084=AXIS2_PLACEMENT_3D('',#193584,#116885,#116886);
#99085=AXIS2_PLACEMENT_3D('',#193585,#116887,#116888);
#99086=AXIS2_PLACEMENT_3D('',#193588,#116889,#116890);
#99087=AXIS2_PLACEMENT_3D('',#193589,#116891,#116892);
#99088=AXIS2_PLACEMENT_3D('',#193590,#116893,#116894);
#99089=AXIS2_PLACEMENT_3D('',#193591,#116895,#116896);
#99090=AXIS2_PLACEMENT_3D('',#193594,#116897,#116898);
#99091=AXIS2_PLACEMENT_3D('',#193597,#116901,#116902);
#99092=AXIS2_PLACEMENT_3D('',#193610,#116903,#116904);
#99093=AXIS2_PLACEMENT_3D('',#193611,#116905,#116906);
#99094=AXIS2_PLACEMENT_3D('',#193612,#116907,#116908);
#99095=AXIS2_PLACEMENT_3D('',#193626,#116909,#116910);
#99096=AXIS2_PLACEMENT_3D('',#193628,#116911,#116912);
#99097=AXIS2_PLACEMENT_3D('',#193629,#116913,#116914);
#99098=AXIS2_PLACEMENT_3D('',#193630,#116915,#116916);
#99099=AXIS2_PLACEMENT_3D('',#193633,#116917,#116918);
#99100=AXIS2_PLACEMENT_3D('',#193636,#116921,#116922);
#99101=AXIS2_PLACEMENT_3D('',#193639,#116923,#116924);
#99102=AXIS2_PLACEMENT_3D('',#193640,#116925,#116926);
#99103=AXIS2_PLACEMENT_3D('',#193641,#116927,#116928);
#99104=AXIS2_PLACEMENT_3D('',#193642,#116929,#116930);
#99105=AXIS2_PLACEMENT_3D('',#193645,#116931,#116932);
#99106=AXIS2_PLACEMENT_3D('',#193646,#116933,#116934);
#99107=AXIS2_PLACEMENT_3D('',#193647,#116935,#116936);
#99108=AXIS2_PLACEMENT_3D('',#193648,#116937,#116938);
#99109=AXIS2_PLACEMENT_3D('',#193651,#116939,#116940);
#99110=AXIS2_PLACEMENT_3D('',#193652,#116941,#116942);
#99111=AXIS2_PLACEMENT_3D('',#193653,#116943,#116944);
#99112=AXIS2_PLACEMENT_3D('',#193654,#116945,#116946);
#99113=AXIS2_PLACEMENT_3D('',#193657,#116947,#116948);
#99114=AXIS2_PLACEMENT_3D('',#193660,#116951,#116952);
#99115=AXIS2_PLACEMENT_3D('',#193673,#116953,#116954);
#99116=AXIS2_PLACEMENT_3D('',#193674,#116955,#116956);
#99117=AXIS2_PLACEMENT_3D('',#193675,#116957,#116958);
#99118=AXIS2_PLACEMENT_3D('',#193678,#116959,#116960);
#99119=AXIS2_PLACEMENT_3D('',#193680,#116961,#116962);
#99120=AXIS2_PLACEMENT_3D('',#193682,#116963,#116964);
#99121=AXIS2_PLACEMENT_3D('',#193683,#116965,#116966);
#99122=AXIS2_PLACEMENT_3D('',#193684,#116967,#116968);
#99123=AXIS2_PLACEMENT_3D('',#193687,#116969,#116970);
#99124=AXIS2_PLACEMENT_3D('',#193688,#116971,#116972);
#99125=AXIS2_PLACEMENT_3D('',#193689,#116973,#116974);
#99126=AXIS2_PLACEMENT_3D('',#193690,#116975,#116976);
#99127=AXIS2_PLACEMENT_3D('',#193693,#116977,#116978);
#99128=AXIS2_PLACEMENT_3D('',#193694,#116979,#116980);
#99129=AXIS2_PLACEMENT_3D('',#193695,#116981,#116982);
#99130=AXIS2_PLACEMENT_3D('',#193696,#116983,#116984);
#99131=AXIS2_PLACEMENT_3D('',#193699,#116985,#116986);
#99132=AXIS2_PLACEMENT_3D('',#193700,#116987,#116988);
#99133=AXIS2_PLACEMENT_3D('',#193701,#116989,#116990);
#99134=AXIS2_PLACEMENT_3D('',#193702,#116991,#116992);
#99135=AXIS2_PLACEMENT_3D('',#193705,#116993,#116994);
#99136=AXIS2_PLACEMENT_3D('',#193706,#116995,#116996);
#99137=AXIS2_PLACEMENT_3D('',#193707,#116997,#116998);
#99138=AXIS2_PLACEMENT_3D('',#193708,#116999,#117000);
#99139=AXIS2_PLACEMENT_3D('',#193711,#117001,#117002);
#99140=AXIS2_PLACEMENT_3D('',#193712,#117003,#117004);
#99141=AXIS2_PLACEMENT_3D('',#193713,#117005,#117006);
#99142=AXIS2_PLACEMENT_3D('',#193714,#117007,#117008);
#99143=AXIS2_PLACEMENT_3D('',#193717,#117009,#117010);
#99144=AXIS2_PLACEMENT_3D('',#193718,#117011,#117012);
#99145=AXIS2_PLACEMENT_3D('',#193719,#117013,#117014);
#99146=AXIS2_PLACEMENT_3D('',#193916,#117015,#117016);
#99147=AXIS2_PLACEMENT_3D('',#194031,#117017,#117018);
#99148=AXIS2_PLACEMENT_3D('',#194057,#117019,#117020);
#99149=AXIS2_PLACEMENT_3D('',#194080,#117021,#117022);
#99150=AXIS2_PLACEMENT_3D('',#194081,#117023,#117024);
#99151=AXIS2_PLACEMENT_3D('',#194082,#117025,#117026);
#99152=AXIS2_PLACEMENT_3D('',#194163,#117027,#117028);
#99153=AXIS2_PLACEMENT_3D('',#194265,#117029,#117030);
#99154=AXIS2_PLACEMENT_3D('',#194471,#117031,#117032);
#99155=AXIS2_PLACEMENT_3D('',#194569,#117033,#117034);
#99156=AXIS2_PLACEMENT_3D('',#194570,#117035,#117036);
#99157=AXIS2_PLACEMENT_3D('',#194571,#117037,#117038);
#99158=AXIS2_PLACEMENT_3D('',#194586,#117039,#117040);
#99159=AXIS2_PLACEMENT_3D('',#194909,#117041,#117042);
#99160=AXIS2_PLACEMENT_3D('',#195312,#117043,#117044);
#99161=AXIS2_PLACEMENT_3D('',#195335,#117045,#117046);
#99162=AXIS2_PLACEMENT_3D('',#195336,#117047,#117048);
#99163=AXIS2_PLACEMENT_3D('',#195337,#117049,#117050);
#99164=AXIS2_PLACEMENT_3D('',#195436,#117051,#117052);
#99165=AXIS2_PLACEMENT_3D('',#195553,#117053,#117054);
#99166=AXIS2_PLACEMENT_3D('',#195768,#117055,#117056);
#99167=AXIS2_PLACEMENT_3D('',#195866,#117057,#117058);
#99168=AXIS2_PLACEMENT_3D('',#195867,#117059,#117060);
#99169=AXIS2_PLACEMENT_3D('',#195868,#117061,#117062);
#99170=AXIS2_PLACEMENT_3D('',#195883,#117063,#117064);
#99171=AXIS2_PLACEMENT_3D('',#195910,#117065,#117066);
#99172=AXIS2_PLACEMENT_3D('',#195911,#117067,#117068);
#99173=AXIS2_PLACEMENT_3D('',#195926,#117069,#117070);
#99174=AXIS2_PLACEMENT_3D('',#195927,#117071,#117072);
#99175=AXIS2_PLACEMENT_3D('',#195928,#117073,#117074);
#99176=AXIS2_PLACEMENT_3D('',#196009,#117075,#117076);
#99177=AXIS2_PLACEMENT_3D('',#196088,#117077,#117078);
#99178=AXIS2_PLACEMENT_3D('',#196160,#117079,#117080);
#99179=AXIS2_PLACEMENT_3D('',#196161,#117081,#117082);
#99180=AXIS2_PLACEMENT_3D('',#196186,#117083,#117084);
#99181=AXIS2_PLACEMENT_3D('',#196187,#117085,#117086);
#99182=AXIS2_PLACEMENT_3D('',#197288,#117087,#117088);
#99183=AXIS2_PLACEMENT_3D('',#197317,#117089,#117090);
#99184=AXIS2_PLACEMENT_3D('',#197342,#117091,#117092);
#99185=AXIS2_PLACEMENT_3D('',#197344,#117093,#117094);
#99186=AXIS2_PLACEMENT_3D('',#197345,#117095,#117096);
#99187=AXIS2_PLACEMENT_3D('',#197366,#117097,#117098);
#99188=AXIS2_PLACEMENT_3D('',#197460,#117099,#117100);
#99189=AXIS2_PLACEMENT_3D('',#197634,#117101,#117102);
#99190=AXIS2_PLACEMENT_3D('',#197635,#117103,#117104);
#99191=AXIS2_PLACEMENT_3D('',#197636,#117105,#117106);
#99192=AXIS2_PLACEMENT_3D('',#197649,#117107,#117108);
#99193=AXIS2_PLACEMENT_3D('',#197668,#117109,#117110);
#99194=AXIS2_PLACEMENT_3D('',#197749,#117111,#117112);
#99195=AXIS2_PLACEMENT_3D('',#197750,#117113,#117114);
#99196=AXIS2_PLACEMENT_3D('',#197751,#117115,#117116);
#99197=AXIS2_PLACEMENT_3D('',#197765,#117117,#117118);
#99198=AXIS2_PLACEMENT_3D('',#197767,#117119,#117120);
#99199=AXIS2_PLACEMENT_3D('',#197768,#117121,#117122);
#99200=AXIS2_PLACEMENT_3D('',#197801,#117123,#117124);
#99201=AXIS2_PLACEMENT_3D('',#197905,#117125,#117126);
#99202=AXIS2_PLACEMENT_3D('',#197972,#117127,#117128);
#99203=AXIS2_PLACEMENT_3D('',#197983,#117129,#117130);
#99204=AXIS2_PLACEMENT_3D('',#197996,#117131,#117132);
#99205=AXIS2_PLACEMENT_3D('',#198001,#117133,#117134);
#99206=AXIS2_PLACEMENT_3D('',#198004,#117135,#117136);
#99207=AXIS2_PLACEMENT_3D('',#198006,#117137,#117138);
#99208=AXIS2_PLACEMENT_3D('',#198008,#117139,#117140);
#99209=AXIS2_PLACEMENT_3D('',#198009,#117141,#117142);
#99210=AXIS2_PLACEMENT_3D('',#198530,#117143,#117144);
#99211=AXIS2_PLACEMENT_3D('',#198550,#117145,#117146);
#99212=AXIS2_PLACEMENT_3D('',#198551,#117147,#117148);
#99213=AXIS2_PLACEMENT_3D('',#198552,#117149,#117150);
#99214=AXIS2_PLACEMENT_3D('',#198573,#117151,#117152);
#99215=AXIS2_PLACEMENT_3D('',#198606,#117153,#117154);
#99216=AXIS2_PLACEMENT_3D('',#198764,#117155,#117156);
#99217=AXIS2_PLACEMENT_3D('',#198926,#117157,#117158);
#99218=AXIS2_PLACEMENT_3D('',#198927,#117159,#117160);
#99219=AXIS2_PLACEMENT_3D('',#198928,#117161,#117162);
#99220=AXIS2_PLACEMENT_3D('',#199108,#117163,#117164);
#99221=AXIS2_PLACEMENT_3D('',#199111,#117165,#117166);
#99222=AXIS2_PLACEMENT_3D('',#199114,#117169,#117170);
#99223=AXIS2_PLACEMENT_3D('',#199118,#117172,#117173);
#99224=AXIS2_PLACEMENT_3D('',#199120,#117175,#117176);
#99225=AXIS2_PLACEMENT_3D('',#199124,#117178,#117179);
#99226=AXIS2_PLACEMENT_3D('',#199126,#117181,#117182);
#99227=AXIS2_PLACEMENT_3D('',#199130,#117184,#117185);
#99228=AXIS2_PLACEMENT_3D('',#199132,#117187,#117188);
#99229=AXIS2_PLACEMENT_3D('',#199136,#117190,#117191);
#99230=AXIS2_PLACEMENT_3D('',#199138,#117193,#117194);
#99231=AXIS2_PLACEMENT_3D('',#199142,#117196,#117197);
#99232=AXIS2_PLACEMENT_3D('',#199144,#117199,#117200);
#99233=AXIS2_PLACEMENT_3D('',#199148,#117202,#117203);
#99234=AXIS2_PLACEMENT_3D('',#199150,#117205,#117206);
#99235=AXIS2_PLACEMENT_3D('',#199154,#117208,#117209);
#99236=AXIS2_PLACEMENT_3D('',#199156,#117211,#117212);
#99237=AXIS2_PLACEMENT_3D('',#199160,#117214,#117215);
#99238=AXIS2_PLACEMENT_3D('',#199162,#117217,#117218);
#99239=AXIS2_PLACEMENT_3D('',#199165,#117219,#117220);
#99240=AXIS2_PLACEMENT_3D('',#199168,#117223,#117224);
#99241=AXIS2_PLACEMENT_3D('',#199172,#117226,#117227);
#99242=AXIS2_PLACEMENT_3D('',#199174,#117229,#117230);
#99243=AXIS2_PLACEMENT_3D('',#199178,#117232,#117233);
#99244=AXIS2_PLACEMENT_3D('',#199180,#117235,#117236);
#99245=AXIS2_PLACEMENT_3D('',#199184,#117238,#117239);
#99246=AXIS2_PLACEMENT_3D('',#199186,#117241,#117242);
#99247=AXIS2_PLACEMENT_3D('',#199190,#117244,#117245);
#99248=AXIS2_PLACEMENT_3D('',#199192,#117247,#117248);
#99249=AXIS2_PLACEMENT_3D('',#199196,#117250,#117251);
#99250=AXIS2_PLACEMENT_3D('',#199198,#117253,#117254);
#99251=AXIS2_PLACEMENT_3D('',#199202,#117256,#117257);
#99252=AXIS2_PLACEMENT_3D('',#199204,#117259,#117260);
#99253=AXIS2_PLACEMENT_3D('',#199208,#117262,#117263);
#99254=AXIS2_PLACEMENT_3D('',#199210,#117265,#117266);
#99255=AXIS2_PLACEMENT_3D('',#199214,#117268,#117269);
#99256=AXIS2_PLACEMENT_3D('',#199216,#117271,#117272);
#99257=AXIS2_PLACEMENT_3D('',#199220,#117274,#117275);
#99258=AXIS2_PLACEMENT_3D('',#199222,#117277,#117278);
#99259=AXIS2_PLACEMENT_3D('',#199226,#117280,#117281);
#99260=AXIS2_PLACEMENT_3D('',#199228,#117283,#117284);
#99261=AXIS2_PLACEMENT_3D('',#199232,#117286,#117287);
#99262=AXIS2_PLACEMENT_3D('',#199234,#117289,#117290);
#99263=AXIS2_PLACEMENT_3D('',#199238,#117292,#117293);
#99264=AXIS2_PLACEMENT_3D('',#199240,#117295,#117296);
#99265=AXIS2_PLACEMENT_3D('',#199244,#117298,#117299);
#99266=AXIS2_PLACEMENT_3D('',#199246,#117301,#117302);
#99267=AXIS2_PLACEMENT_3D('',#199250,#117304,#117305);
#99268=AXIS2_PLACEMENT_3D('',#199252,#117307,#117308);
#99269=AXIS2_PLACEMENT_3D('',#199256,#117310,#117311);
#99270=AXIS2_PLACEMENT_3D('',#199258,#117313,#117314);
#99271=AXIS2_PLACEMENT_3D('',#199262,#117316,#117317);
#99272=AXIS2_PLACEMENT_3D('',#199264,#117319,#117320);
#99273=AXIS2_PLACEMENT_3D('',#199268,#117322,#117323);
#99274=AXIS2_PLACEMENT_3D('',#199270,#117325,#117326);
#99275=AXIS2_PLACEMENT_3D('',#199273,#117327,#117328);
#99276=AXIS2_PLACEMENT_3D('',#199276,#117331,#117332);
#99277=AXIS2_PLACEMENT_3D('',#199280,#117334,#117335);
#99278=AXIS2_PLACEMENT_3D('',#199282,#117337,#117338);
#99279=AXIS2_PLACEMENT_3D('',#199286,#117340,#117341);
#99280=AXIS2_PLACEMENT_3D('',#199288,#117343,#117344);
#99281=AXIS2_PLACEMENT_3D('',#199292,#117346,#117347);
#99282=AXIS2_PLACEMENT_3D('',#199294,#117349,#117350);
#99283=AXIS2_PLACEMENT_3D('',#199298,#117352,#117353);
#99284=AXIS2_PLACEMENT_3D('',#199300,#117355,#117356);
#99285=AXIS2_PLACEMENT_3D('',#199304,#117358,#117359);
#99286=AXIS2_PLACEMENT_3D('',#199306,#117361,#117362);
#99287=AXIS2_PLACEMENT_3D('',#199310,#117364,#117365);
#99288=AXIS2_PLACEMENT_3D('',#199312,#117367,#117368);
#99289=AXIS2_PLACEMENT_3D('',#199316,#117370,#117371);
#99290=AXIS2_PLACEMENT_3D('',#199318,#117373,#117374);
#99291=AXIS2_PLACEMENT_3D('',#199322,#117376,#117377);
#99292=AXIS2_PLACEMENT_3D('',#199324,#117379,#117380);
#99293=AXIS2_PLACEMENT_3D('',#199328,#117382,#117383);
#99294=AXIS2_PLACEMENT_3D('',#199330,#117385,#117386);
#99295=AXIS2_PLACEMENT_3D('',#199334,#117388,#117389);
#99296=AXIS2_PLACEMENT_3D('',#199336,#117391,#117392);
#99297=AXIS2_PLACEMENT_3D('',#199340,#117394,#117395);
#99298=AXIS2_PLACEMENT_3D('',#199342,#117397,#117398);
#99299=AXIS2_PLACEMENT_3D('',#199346,#117400,#117401);
#99300=AXIS2_PLACEMENT_3D('',#199348,#117403,#117404);
#99301=AXIS2_PLACEMENT_3D('',#199352,#117406,#117407);
#99302=AXIS2_PLACEMENT_3D('',#199354,#117409,#117410);
#99303=AXIS2_PLACEMENT_3D('',#199358,#117412,#117413);
#99304=AXIS2_PLACEMENT_3D('',#199360,#117415,#117416);
#99305=AXIS2_PLACEMENT_3D('',#199364,#117418,#117419);
#99306=AXIS2_PLACEMENT_3D('',#199366,#117421,#117422);
#99307=AXIS2_PLACEMENT_3D('',#199370,#117424,#117425);
#99308=AXIS2_PLACEMENT_3D('',#199372,#117427,#117428);
#99309=AXIS2_PLACEMENT_3D('',#199376,#117430,#117431);
#99310=AXIS2_PLACEMENT_3D('',#199378,#117433,#117434);
#99311=AXIS2_PLACEMENT_3D('',#199382,#117436,#117437);
#99312=AXIS2_PLACEMENT_3D('',#199384,#117439,#117440);
#99313=AXIS2_PLACEMENT_3D('',#199388,#117442,#117443);
#99314=AXIS2_PLACEMENT_3D('',#199390,#117445,#117446);
#99315=AXIS2_PLACEMENT_3D('',#199394,#117448,#117449);
#99316=AXIS2_PLACEMENT_3D('',#199396,#117451,#117452);
#99317=AXIS2_PLACEMENT_3D('',#199400,#117454,#117455);
#99318=AXIS2_PLACEMENT_3D('',#199402,#117457,#117458);
#99319=AXIS2_PLACEMENT_3D('',#199406,#117460,#117461);
#99320=AXIS2_PLACEMENT_3D('',#199408,#117463,#117464);
#99321=AXIS2_PLACEMENT_3D('',#199412,#117466,#117467);
#99322=AXIS2_PLACEMENT_3D('',#199414,#117469,#117470);
#99323=AXIS2_PLACEMENT_3D('',#199418,#117472,#117473);
#99324=AXIS2_PLACEMENT_3D('',#199420,#117475,#117476);
#99325=AXIS2_PLACEMENT_3D('',#199424,#117478,#117479);
#99326=AXIS2_PLACEMENT_3D('',#199426,#117481,#117482);
#99327=AXIS2_PLACEMENT_3D('',#199430,#117484,#117485);
#99328=AXIS2_PLACEMENT_3D('',#199432,#117487,#117488);
#99329=AXIS2_PLACEMENT_3D('',#199436,#117490,#117491);
#99330=AXIS2_PLACEMENT_3D('',#199438,#117493,#117494);
#99331=AXIS2_PLACEMENT_3D('',#199442,#117496,#117497);
#99332=AXIS2_PLACEMENT_3D('',#199444,#117499,#117500);
#99333=AXIS2_PLACEMENT_3D('',#199448,#117502,#117503);
#99334=AXIS2_PLACEMENT_3D('',#199450,#117505,#117506);
#99335=AXIS2_PLACEMENT_3D('',#199454,#117508,#117509);
#99336=AXIS2_PLACEMENT_3D('',#199456,#117511,#117512);
#99337=AXIS2_PLACEMENT_3D('',#199460,#117514,#117515);
#99338=AXIS2_PLACEMENT_3D('',#199462,#117517,#117518);
#99339=AXIS2_PLACEMENT_3D('',#199466,#117520,#117521);
#99340=AXIS2_PLACEMENT_3D('',#199468,#117523,#117524);
#99341=AXIS2_PLACEMENT_3D('',#199472,#117526,#117527);
#99342=AXIS2_PLACEMENT_3D('',#199474,#117529,#117530);
#99343=AXIS2_PLACEMENT_3D('',#199478,#117532,#117533);
#99344=AXIS2_PLACEMENT_3D('',#199480,#117535,#117536);
#99345=AXIS2_PLACEMENT_3D('',#199484,#117538,#117539);
#99346=AXIS2_PLACEMENT_3D('',#199486,#117541,#117542);
#99347=AXIS2_PLACEMENT_3D('',#199490,#117544,#117545);
#99348=AXIS2_PLACEMENT_3D('',#199492,#117547,#117548);
#99349=AXIS2_PLACEMENT_3D('',#199496,#117550,#117551);
#99350=AXIS2_PLACEMENT_3D('',#199498,#117553,#117554);
#99351=AXIS2_PLACEMENT_3D('',#199502,#117556,#117557);
#99352=AXIS2_PLACEMENT_3D('',#199504,#117559,#117560);
#99353=AXIS2_PLACEMENT_3D('',#199508,#117562,#117563);
#99354=AXIS2_PLACEMENT_3D('',#199510,#117565,#117566);
#99355=AXIS2_PLACEMENT_3D('',#199514,#117568,#117569);
#99356=AXIS2_PLACEMENT_3D('',#199516,#117571,#117572);
#99357=AXIS2_PLACEMENT_3D('',#199520,#117574,#117575);
#99358=AXIS2_PLACEMENT_3D('',#199522,#117577,#117578);
#99359=AXIS2_PLACEMENT_3D('',#199526,#117580,#117581);
#99360=AXIS2_PLACEMENT_3D('',#199528,#117583,#117584);
#99361=AXIS2_PLACEMENT_3D('',#199532,#117586,#117587);
#99362=AXIS2_PLACEMENT_3D('',#199534,#117589,#117590);
#99363=AXIS2_PLACEMENT_3D('',#199538,#117592,#117593);
#99364=AXIS2_PLACEMENT_3D('',#199540,#117595,#117596);
#99365=AXIS2_PLACEMENT_3D('',#199544,#117598,#117599);
#99366=AXIS2_PLACEMENT_3D('',#199546,#117601,#117602);
#99367=AXIS2_PLACEMENT_3D('',#199550,#117604,#117605);
#99368=AXIS2_PLACEMENT_3D('',#199552,#117607,#117608);
#99369=AXIS2_PLACEMENT_3D('',#199556,#117610,#117611);
#99370=AXIS2_PLACEMENT_3D('',#199558,#117613,#117614);
#99371=AXIS2_PLACEMENT_3D('',#199562,#117616,#117617);
#99372=AXIS2_PLACEMENT_3D('',#199564,#117619,#117620);
#99373=AXIS2_PLACEMENT_3D('',#199568,#117622,#117623);
#99374=AXIS2_PLACEMENT_3D('',#199570,#117625,#117626);
#99375=AXIS2_PLACEMENT_3D('',#199574,#117628,#117629);
#99376=AXIS2_PLACEMENT_3D('',#199576,#117631,#117632);
#99377=AXIS2_PLACEMENT_3D('',#199580,#117634,#117635);
#99378=AXIS2_PLACEMENT_3D('',#199582,#117637,#117638);
#99379=AXIS2_PLACEMENT_3D('',#199586,#117640,#117641);
#99380=AXIS2_PLACEMENT_3D('',#199588,#117643,#117644);
#99381=AXIS2_PLACEMENT_3D('',#199592,#117646,#117647);
#99382=AXIS2_PLACEMENT_3D('',#199594,#117649,#117650);
#99383=AXIS2_PLACEMENT_3D('',#199598,#117652,#117653);
#99384=AXIS2_PLACEMENT_3D('',#199600,#117655,#117656);
#99385=AXIS2_PLACEMENT_3D('',#199604,#117658,#117659);
#99386=AXIS2_PLACEMENT_3D('',#199606,#117661,#117662);
#99387=AXIS2_PLACEMENT_3D('',#199610,#117664,#117665);
#99388=AXIS2_PLACEMENT_3D('',#199612,#117667,#117668);
#99389=AXIS2_PLACEMENT_3D('',#199616,#117670,#117671);
#99390=AXIS2_PLACEMENT_3D('',#199618,#117673,#117674);
#99391=AXIS2_PLACEMENT_3D('',#199621,#117675,#117676);
#99392=AXIS2_PLACEMENT_3D('',#199624,#117679,#117680);
#99393=AXIS2_PLACEMENT_3D('',#199628,#117682,#117683);
#99394=AXIS2_PLACEMENT_3D('',#199630,#117685,#117686);
#99395=AXIS2_PLACEMENT_3D('',#199634,#117688,#117689);
#99396=AXIS2_PLACEMENT_3D('',#199636,#117691,#117692);
#99397=AXIS2_PLACEMENT_3D('',#199640,#117694,#117695);
#99398=AXIS2_PLACEMENT_3D('',#199642,#117697,#117698);
#99399=AXIS2_PLACEMENT_3D('',#199646,#117700,#117701);
#99400=AXIS2_PLACEMENT_3D('',#199648,#117703,#117704);
#99401=AXIS2_PLACEMENT_3D('',#199652,#117706,#117707);
#99402=AXIS2_PLACEMENT_3D('',#199654,#117709,#117710);
#99403=AXIS2_PLACEMENT_3D('',#199658,#117712,#117713);
#99404=AXIS2_PLACEMENT_3D('',#199660,#117715,#117716);
#99405=AXIS2_PLACEMENT_3D('',#199664,#117718,#117719);
#99406=AXIS2_PLACEMENT_3D('',#199666,#117721,#117722);
#99407=AXIS2_PLACEMENT_3D('',#199670,#117724,#117725);
#99408=AXIS2_PLACEMENT_3D('',#199672,#117727,#117728);
#99409=AXIS2_PLACEMENT_3D('',#199676,#117730,#117731);
#99410=AXIS2_PLACEMENT_3D('',#199678,#117733,#117734);
#99411=AXIS2_PLACEMENT_3D('',#199682,#117736,#117737);
#99412=AXIS2_PLACEMENT_3D('',#199684,#117739,#117740);
#99413=AXIS2_PLACEMENT_3D('',#199688,#117742,#117743);
#99414=AXIS2_PLACEMENT_3D('',#199690,#117745,#117746);
#99415=AXIS2_PLACEMENT_3D('',#199694,#117748,#117749);
#99416=AXIS2_PLACEMENT_3D('',#199696,#117751,#117752);
#99417=AXIS2_PLACEMENT_3D('',#199700,#117754,#117755);
#99418=AXIS2_PLACEMENT_3D('',#199702,#117757,#117758);
#99419=AXIS2_PLACEMENT_3D('',#199706,#117760,#117761);
#99420=AXIS2_PLACEMENT_3D('',#199708,#117763,#117764);
#99421=AXIS2_PLACEMENT_3D('',#199712,#117766,#117767);
#99422=AXIS2_PLACEMENT_3D('',#199714,#117769,#117770);
#99423=AXIS2_PLACEMENT_3D('',#199718,#117772,#117773);
#99424=AXIS2_PLACEMENT_3D('',#199720,#117775,#117776);
#99425=AXIS2_PLACEMENT_3D('',#199724,#117778,#117779);
#99426=AXIS2_PLACEMENT_3D('',#199726,#117781,#117782);
#99427=AXIS2_PLACEMENT_3D('',#199730,#117784,#117785);
#99428=AXIS2_PLACEMENT_3D('',#199732,#117787,#117788);
#99429=AXIS2_PLACEMENT_3D('',#199736,#117790,#117791);
#99430=AXIS2_PLACEMENT_3D('',#199738,#117793,#117794);
#99431=AXIS2_PLACEMENT_3D('',#199742,#117796,#117797);
#99432=AXIS2_PLACEMENT_3D('',#199744,#117799,#117800);
#99433=AXIS2_PLACEMENT_3D('',#199748,#117802,#117803);
#99434=AXIS2_PLACEMENT_3D('',#199750,#117805,#117806);
#99435=AXIS2_PLACEMENT_3D('',#199754,#117808,#117809);
#99436=AXIS2_PLACEMENT_3D('',#199756,#117811,#117812);
#99437=AXIS2_PLACEMENT_3D('',#199760,#117814,#117815);
#99438=AXIS2_PLACEMENT_3D('',#199762,#117817,#117818);
#99439=AXIS2_PLACEMENT_3D('',#199765,#117819,#117820);
#99440=AXIS2_PLACEMENT_3D('',#199768,#117823,#117824);
#99441=AXIS2_PLACEMENT_3D('',#199772,#117826,#117827);
#99442=AXIS2_PLACEMENT_3D('',#199774,#117829,#117830);
#99443=AXIS2_PLACEMENT_3D('',#199778,#117832,#117833);
#99444=AXIS2_PLACEMENT_3D('',#199780,#117835,#117836);
#99445=AXIS2_PLACEMENT_3D('',#199784,#117838,#117839);
#99446=AXIS2_PLACEMENT_3D('',#199786,#117841,#117842);
#99447=AXIS2_PLACEMENT_3D('',#199790,#117844,#117845);
#99448=AXIS2_PLACEMENT_3D('',#199792,#117847,#117848);
#99449=AXIS2_PLACEMENT_3D('',#199796,#117850,#117851);
#99450=AXIS2_PLACEMENT_3D('',#199798,#117853,#117854);
#99451=AXIS2_PLACEMENT_3D('',#199802,#117856,#117857);
#99452=AXIS2_PLACEMENT_3D('',#199804,#117859,#117860);
#99453=AXIS2_PLACEMENT_3D('',#199808,#117862,#117863);
#99454=AXIS2_PLACEMENT_3D('',#199810,#117865,#117866);
#99455=AXIS2_PLACEMENT_3D('',#199814,#117868,#117869);
#99456=AXIS2_PLACEMENT_3D('',#199816,#117871,#117872);
#99457=AXIS2_PLACEMENT_3D('',#199820,#117874,#117875);
#99458=AXIS2_PLACEMENT_3D('',#199822,#117877,#117878);
#99459=AXIS2_PLACEMENT_3D('',#199826,#117880,#117881);
#99460=AXIS2_PLACEMENT_3D('',#199828,#117883,#117884);
#99461=AXIS2_PLACEMENT_3D('',#199832,#117886,#117887);
#99462=AXIS2_PLACEMENT_3D('',#199834,#117889,#117890);
#99463=AXIS2_PLACEMENT_3D('',#199838,#117892,#117893);
#99464=AXIS2_PLACEMENT_3D('',#199840,#117895,#117896);
#99465=AXIS2_PLACEMENT_3D('',#199844,#117898,#117899);
#99466=AXIS2_PLACEMENT_3D('',#199846,#117901,#117902);
#99467=AXIS2_PLACEMENT_3D('',#199850,#117904,#117905);
#99468=AXIS2_PLACEMENT_3D('',#199852,#117907,#117908);
#99469=AXIS2_PLACEMENT_3D('',#199856,#117910,#117911);
#99470=AXIS2_PLACEMENT_3D('',#199858,#117913,#117914);
#99471=AXIS2_PLACEMENT_3D('',#199861,#117915,#117916);
#99472=AXIS2_PLACEMENT_3D('',#199864,#117919,#117920);
#99473=AXIS2_PLACEMENT_3D('',#199868,#117922,#117923);
#99474=AXIS2_PLACEMENT_3D('',#199870,#117925,#117926);
#99475=AXIS2_PLACEMENT_3D('',#199874,#117928,#117929);
#99476=AXIS2_PLACEMENT_3D('',#199876,#117931,#117932);
#99477=AXIS2_PLACEMENT_3D('',#199880,#117934,#117935);
#99478=AXIS2_PLACEMENT_3D('',#199882,#117937,#117938);
#99479=AXIS2_PLACEMENT_3D('',#199886,#117940,#117941);
#99480=AXIS2_PLACEMENT_3D('',#199888,#117943,#117944);
#99481=AXIS2_PLACEMENT_3D('',#199891,#117945,#117946);
#99482=AXIS2_PLACEMENT_3D('',#199894,#117949,#117950);
#99483=AXIS2_PLACEMENT_3D('',#199898,#117952,#117953);
#99484=AXIS2_PLACEMENT_3D('',#199900,#117955,#117956);
#99485=AXIS2_PLACEMENT_3D('',#199903,#117957,#117958);
#99486=AXIS2_PLACEMENT_3D('',#199906,#117961,#117962);
#99487=AXIS2_PLACEMENT_3D('',#199910,#117964,#117965);
#99488=AXIS2_PLACEMENT_3D('',#199912,#117967,#117968);
#99489=AXIS2_PLACEMENT_3D('',#199916,#117970,#117971);
#99490=AXIS2_PLACEMENT_3D('',#199918,#117973,#117974);
#99491=AXIS2_PLACEMENT_3D('',#199922,#117976,#117977);
#99492=AXIS2_PLACEMENT_3D('',#199924,#117979,#117980);
#99493=AXIS2_PLACEMENT_3D('',#199927,#117982,#117983);
#99494=AXIS2_PLACEMENT_3D('',#199928,#117984,#117985);
#99495=AXIS2_PLACEMENT_3D('',#199930,#117986,#117987);
#99496=AXIS2_PLACEMENT_3D('',#199932,#117989,#117990);
#99497=AXIS2_PLACEMENT_3D('',#199933,#117991,#117992);
#99498=AXIS2_PLACEMENT_3D('',#199934,#117993,#117994);
#99499=AXIS2_PLACEMENT_3D('',#199935,#117995,#117996);
#99500=AXIS2_PLACEMENT_3D('',#199936,#117997,#117998);
#99501=AXIS2_PLACEMENT_3D('',#199937,#117999,#118000);
#99502=AXIS2_PLACEMENT_3D('',#199938,#118001,#118002);
#99503=AXIS2_PLACEMENT_3D('',#199940,#118004,#118005);
#99504=AXIS2_PLACEMENT_3D('',#199942,#118007,#118008);
#99505=AXIS2_PLACEMENT_3D('',#199943,#118009,#118010);
#99506=AXIS2_PLACEMENT_3D('',#199944,#118011,#118012);
#99507=AXIS2_PLACEMENT_3D('',#199945,#118013,#118014);
#99508=AXIS2_PLACEMENT_3D('',#199946,#118015,#118016);
#99509=AXIS2_PLACEMENT_3D('',#199947,#118017,#118018);
#99510=AXIS2_PLACEMENT_3D('',#199948,#118019,#118020);
#99511=AXIS2_PLACEMENT_3D('',#199950,#118022,#118023);
#99512=AXIS2_PLACEMENT_3D('',#199952,#118025,#118026);
#99513=AXIS2_PLACEMENT_3D('',#199953,#118027,#118028);
#99514=AXIS2_PLACEMENT_3D('',#199954,#118029,#118030);
#99515=AXIS2_PLACEMENT_3D('',#199955,#118031,#118032);
#99516=AXIS2_PLACEMENT_3D('',#199956,#118033,#118034);
#99517=AXIS2_PLACEMENT_3D('',#199958,#118036,#118037);
#99518=AXIS2_PLACEMENT_3D('',#199960,#118039,#118040);
#99519=AXIS2_PLACEMENT_3D('',#199962,#118042,#118043);
#99520=AXIS2_PLACEMENT_3D('',#199964,#118045,#118046);
#99521=AXIS2_PLACEMENT_3D('',#199966,#118048,#118049);
#99522=AXIS2_PLACEMENT_3D('',#199968,#118051,#118052);
#99523=AXIS2_PLACEMENT_3D('',#199970,#118054,#118055);
#99524=AXIS2_PLACEMENT_3D('',#199972,#118057,#118058);
#99525=AXIS2_PLACEMENT_3D('',#199974,#118060,#118061);
#99526=AXIS2_PLACEMENT_3D('',#199976,#118063,#118064);
#99527=AXIS2_PLACEMENT_3D('',#199978,#118066,#118067);
#99528=AXIS2_PLACEMENT_3D('',#199980,#118069,#118070);
#99529=AXIS2_PLACEMENT_3D('',#199982,#118072,#118073);
#99530=AXIS2_PLACEMENT_3D('',#199984,#118075,#118076);
#99531=AXIS2_PLACEMENT_3D('',#199986,#118078,#118079);
#99532=AXIS2_PLACEMENT_3D('',#199988,#118081,#118082);
#99533=AXIS2_PLACEMENT_3D('',#199990,#118084,#118085);
#99534=AXIS2_PLACEMENT_3D('',#199992,#118087,#118088);
#99535=AXIS2_PLACEMENT_3D('',#199994,#118090,#118091);
#99536=AXIS2_PLACEMENT_3D('',#199996,#118093,#118094);
#99537=AXIS2_PLACEMENT_3D('',#199998,#118096,#118097);
#99538=AXIS2_PLACEMENT_3D('',#200000,#118099,#118100);
#99539=AXIS2_PLACEMENT_3D('',#200002,#118102,#118103);
#99540=AXIS2_PLACEMENT_3D('',#200004,#118105,#118106);
#99541=AXIS2_PLACEMENT_3D('',#200006,#118108,#118109);
#99542=AXIS2_PLACEMENT_3D('',#200008,#118111,#118112);
#99543=AXIS2_PLACEMENT_3D('',#200010,#118114,#118115);
#99544=AXIS2_PLACEMENT_3D('',#200012,#118117,#118118);
#99545=AXIS2_PLACEMENT_3D('',#200014,#118120,#118121);
#99546=AXIS2_PLACEMENT_3D('',#200016,#118123,#118124);
#99547=AXIS2_PLACEMENT_3D('',#200018,#118126,#118127);
#99548=AXIS2_PLACEMENT_3D('',#200020,#118129,#118130);
#99549=AXIS2_PLACEMENT_3D('',#200029,#118135,#118136);
#99550=AXIS2_PLACEMENT_3D('',#200035,#118140,#118141);
#99551=AXIS2_PLACEMENT_3D('',#200041,#118145,#118146);
#99552=AXIS2_PLACEMENT_3D('',#200043,#118148,#118149);
#99553=AXIS2_PLACEMENT_3D('',#200045,#118151,#118152);
#99554=AXIS2_PLACEMENT_3D('',#200047,#118154,#118155);
#99555=AXIS2_PLACEMENT_3D('',#200049,#118157,#118158);
#99556=AXIS2_PLACEMENT_3D('',#200051,#118160,#118161);
#99557=AXIS2_PLACEMENT_3D('',#200053,#118163,#118164);
#99558=AXIS2_PLACEMENT_3D('',#200055,#118166,#118167);
#99559=AXIS2_PLACEMENT_3D('',#200057,#118169,#118170);
#99560=AXIS2_PLACEMENT_3D('',#200059,#118172,#118173);
#99561=AXIS2_PLACEMENT_3D('',#200061,#118175,#118176);
#99562=AXIS2_PLACEMENT_3D('',#200063,#118178,#118179);
#99563=AXIS2_PLACEMENT_3D('',#200065,#118181,#118182);
#99564=AXIS2_PLACEMENT_3D('',#200067,#118184,#118185);
#99565=AXIS2_PLACEMENT_3D('',#200069,#118187,#118188);
#99566=AXIS2_PLACEMENT_3D('',#200071,#118190,#118191);
#99567=AXIS2_PLACEMENT_3D('',#200073,#118193,#118194);
#99568=AXIS2_PLACEMENT_3D('',#200075,#118196,#118197);
#99569=AXIS2_PLACEMENT_3D('',#200077,#118199,#118200);
#99570=AXIS2_PLACEMENT_3D('',#200079,#118202,#118203);
#99571=AXIS2_PLACEMENT_3D('',#200081,#118205,#118206);
#99572=AXIS2_PLACEMENT_3D('',#200083,#118208,#118209);
#99573=AXIS2_PLACEMENT_3D('',#200085,#118211,#118212);
#99574=AXIS2_PLACEMENT_3D('',#200090,#118214,#118215);
#99575=AXIS2_PLACEMENT_3D('',#200093,#118217,#118218);
#99576=AXIS2_PLACEMENT_3D('',#200094,#118219,#118220);
#99577=AXIS2_PLACEMENT_3D('',#200096,#118221,#118222);
#99578=AXIS2_PLACEMENT_3D('',#200099,#118224,#118225);
#99579=AXIS2_PLACEMENT_3D('',#200100,#118226,#118227);
#99580=AXIS2_PLACEMENT_3D('',#200102,#118228,#118229);
#99581=AXIS2_PLACEMENT_3D('',#200105,#118231,#118232);
#99582=AXIS2_PLACEMENT_3D('',#200106,#118233,#118234);
#99583=AXIS2_PLACEMENT_3D('',#200108,#118235,#118236);
#99584=AXIS2_PLACEMENT_3D('',#200111,#118238,#118239);
#99585=AXIS2_PLACEMENT_3D('',#200112,#118240,#118241);
#99586=AXIS2_PLACEMENT_3D('',#200114,#118242,#118243);
#99587=AXIS2_PLACEMENT_3D('',#200117,#118245,#118246);
#99588=AXIS2_PLACEMENT_3D('',#200118,#118247,#118248);
#99589=AXIS2_PLACEMENT_3D('',#200120,#118249,#118250);
#99590=AXIS2_PLACEMENT_3D('',#200123,#118252,#118253);
#99591=AXIS2_PLACEMENT_3D('',#200124,#118254,#118255);
#99592=AXIS2_PLACEMENT_3D('',#200126,#118256,#118257);
#99593=AXIS2_PLACEMENT_3D('',#200129,#118259,#118260);
#99594=AXIS2_PLACEMENT_3D('',#200130,#118261,#118262);
#99595=AXIS2_PLACEMENT_3D('',#200135,#118264,#118265);
#99596=AXIS2_PLACEMENT_3D('',#200144,#118267,#118268);
#99597=AXIS2_PLACEMENT_3D('',#200153,#118270,#118271);
#99598=AXIS2_PLACEMENT_3D('',#200156,#118272,#118273);
#99599=AXIS2_PLACEMENT_3D('',#200165,#118275,#118276);
#99600=AXIS2_PLACEMENT_3D('',#200174,#118278,#118279);
#99601=AXIS2_PLACEMENT_3D('',#200190,#118282,#118283);
#99602=AXIS2_PLACEMENT_3D('',#200206,#118286,#118287);
#99603=AXIS2_PLACEMENT_3D('',#200207,#118288,#118289);
#99604=AXIS2_PLACEMENT_3D('',#200208,#118290,#118291);
#99605=AXIS2_PLACEMENT_3D('',#200209,#118292,#118293);
#99606=AXIS2_PLACEMENT_3D('',#200225,#118296,#118297);
#99607=AXIS2_PLACEMENT_3D('',#200241,#118300,#118301);
#99608=AXIS2_PLACEMENT_3D('',#200242,#118302,#118303);
#99609=AXIS2_PLACEMENT_3D('',#200243,#118304,#118305);
#99610=AXIS2_PLACEMENT_3D('',#200244,#118306,#118307);
#99611=AXIS2_PLACEMENT_3D('',#200247,#118308,#118309);
#99612=AXIS2_PLACEMENT_3D('',#200251,#118311,#118312);
#99613=AXIS2_PLACEMENT_3D('',#200253,#118314,#118315);
#99614=AXIS2_PLACEMENT_3D('',#200256,#118316,#118317);
#99615=AXIS2_PLACEMENT_3D('',#200260,#118319,#118320);
#99616=AXIS2_PLACEMENT_3D('',#200262,#118322,#118323);
#99617=AXIS2_PLACEMENT_3D('',#200264,#118324,#118325);
#99618=AXIS2_PLACEMENT_3D('',#200267,#118327,#118328);
#99619=AXIS2_PLACEMENT_3D('',#200268,#118329,#118330);
#99620=AXIS2_PLACEMENT_3D('',#200270,#118331,#118332);
#99621=AXIS2_PLACEMENT_3D('',#200273,#118334,#118335);
#99622=AXIS2_PLACEMENT_3D('',#200274,#118336,#118337);
#99623=AXIS2_PLACEMENT_3D('',#200283,#118338,#118339);
#99624=AXIS2_PLACEMENT_3D('',#200284,#118340,#118341);
#99625=AXIS2_PLACEMENT_3D('',#200285,#118342,#118343);
#99626=AXIS2_PLACEMENT_3D('',#200288,#118344,#118345);
#99627=AXIS2_PLACEMENT_3D('',#200292,#118347,#118348);
#99628=AXIS2_PLACEMENT_3D('',#200294,#118350,#118351);
#99629=AXIS2_PLACEMENT_3D('',#200295,#118352,#118353);
#99630=AXIS2_PLACEMENT_3D('',#200296,#118354,#118355);
#99631=AXIS2_PLACEMENT_3D('',#202382,#118356,#118357);
#99632=AXIS2_PLACEMENT_3D('',#202385,#118358,#118359);
#99633=AXIS2_PLACEMENT_3D('',#202395,#118362,#118363);
#99634=AXIS2_PLACEMENT_3D('',#202413,#118365,#118366);
#99635=AXIS2_PLACEMENT_3D('',#202414,#118367,#118368);
#99636=AXIS2_PLACEMENT_3D('',#202416,#118369,#118370);
#99637=AXIS2_PLACEMENT_3D('',#202417,#118371,#118372);
#99638=AXIS2_PLACEMENT_3D('',#202419,#118374,#118375);
#99639=AXIS2_PLACEMENT_3D('',#202422,#118376,#118377);
#99640=AXIS2_PLACEMENT_3D('',#202425,#118379,#118380);
#99641=AXIS2_PLACEMENT_3D('',#202427,#118382,#118383);
#99642=AXIS2_PLACEMENT_3D('',#202439,#118385,#118386);
#99643=AXIS2_PLACEMENT_3D('',#202448,#118387,#118388);
#99644=AXIS2_PLACEMENT_3D('',#202450,#118389,#118390);
#99645=AXIS2_PLACEMENT_3D('',#202451,#118391,#118392);
#99646=AXIS2_PLACEMENT_3D('',#202453,#118394,#118395);
#99647=AXIS2_PLACEMENT_3D('',#202456,#118396,#118397);
#99648=AXIS2_PLACEMENT_3D('',#202460,#118399,#118400);
#99649=AXIS2_PLACEMENT_3D('',#202462,#118402,#118403);
#99650=AXIS2_PLACEMENT_3D('',#202464,#118404,#118405);
#99651=AXIS2_PLACEMENT_3D('',#202466,#118406,#118407);
#99652=AXIS2_PLACEMENT_3D('',#202468,#118409,#118410);
#99653=AXIS2_PLACEMENT_3D('',#202470,#118411,#118412);
#99654=AXIS2_PLACEMENT_3D('',#202472,#118413,#118414);
#99655=AXIS2_PLACEMENT_3D('',#202474,#118416,#118417);
#99656=AXIS2_PLACEMENT_3D('',#202476,#118418,#118419);
#99657=AXIS2_PLACEMENT_3D('',#202478,#118420,#118421);
#99658=AXIS2_PLACEMENT_3D('',#202480,#118423,#118424);
#99659=AXIS2_PLACEMENT_3D('',#202483,#118425,#118426);
#99660=AXIS2_PLACEMENT_3D('',#202487,#118428,#118429);
#99661=AXIS2_PLACEMENT_3D('',#202489,#118431,#118432);
#99662=AXIS2_PLACEMENT_3D('',#202491,#118433,#118434);
#99663=AXIS2_PLACEMENT_3D('',#202493,#118435,#118436);
#99664=AXIS2_PLACEMENT_3D('',#202495,#118438,#118439);
#99665=AXIS2_PLACEMENT_3D('',#202496,#118440,#118441);
#99666=AXIS2_PLACEMENT_3D('',#202497,#118442,#118443);
#99667=AXIS2_PLACEMENT_3D('',#202570,#118444,#118445);
#99668=AXIS2_PLACEMENT_3D('',#202752,#118446,#118447);
#99669=AXIS2_PLACEMENT_3D('',#202770,#118448,#118449);
#99670=AXIS2_PLACEMENT_3D('',#202854,#118450,#118451);
#99671=AXIS2_PLACEMENT_3D('',#202856,#118452,#118453);
#99672=AXIS2_PLACEMENT_3D('',#202880,#118454,#118455);
#99673=AXIS2_PLACEMENT_3D('',#202888,#118456,#118457);
#99674=AXIS2_PLACEMENT_3D('',#202952,#118458,#118459);
#99675=AXIS2_PLACEMENT_3D('',#202967,#118460,#118461);
#99676=AXIS2_PLACEMENT_3D('',#203229,#118462,#118463);
#99677=AXIS2_PLACEMENT_3D('',#203238,#118464,#118465);
#99678=AXIS2_PLACEMENT_3D('',#203562,#118466,#118467);
#99679=AXIS2_PLACEMENT_3D('',#203565,#118468,#118469);
#99680=AXIS2_PLACEMENT_3D('',#203572,#118470,#118471);
#99681=AXIS2_PLACEMENT_3D('',#203580,#118472,#118473);
#99682=AXIS2_PLACEMENT_3D('',#203587,#118474,#118475);
#99683=AXIS2_PLACEMENT_3D('',#203590,#118476,#118477);
#99684=AXIS2_PLACEMENT_3D('',#203597,#118478,#118479);
#99685=AXIS2_PLACEMENT_3D('',#203600,#118480,#118481);
#99686=AXIS2_PLACEMENT_3D('',#203607,#118482,#118483);
#99687=AXIS2_PLACEMENT_3D('',#203610,#118484,#118485);
#99688=AXIS2_PLACEMENT_3D('',#203617,#118486,#118487);
#99689=AXIS2_PLACEMENT_3D('',#203626,#118488,#118489);
#99690=AXIS2_PLACEMENT_3D('',#203627,#118490,#118491);
#99691=AXIS2_PLACEMENT_3D('',#203629,#118492,#118493);
#99692=AXIS2_PLACEMENT_3D('',#203631,#118495,#118496);
#99693=AXIS2_PLACEMENT_3D('',#203642,#118497,#118498);
#99694=AXIS2_PLACEMENT_3D('',#203651,#118499,#118500);
#99695=AXIS2_PLACEMENT_3D('',#203654,#118501,#118502);
#99696=AXIS2_PLACEMENT_3D('',#203669,#118503,#118504);
#99697=AXIS2_PLACEMENT_3D('',#203671,#118505,#118506);
#99698=AXIS2_PLACEMENT_3D('',#203678,#118507,#118508);
#99699=AXIS2_PLACEMENT_3D('',#203681,#118509,#118510);
#99700=AXIS2_PLACEMENT_3D('',#203698,#118511,#118512);
#99701=AXIS2_PLACEMENT_3D('',#203726,#118513,#118514);
#99702=AXIS2_PLACEMENT_3D('',#203727,#118515,#118516);
#99703=AXIS2_PLACEMENT_3D('',#203729,#118518,#118519);
#99704=AXIS2_PLACEMENT_3D('',#203731,#118521,#118522);
#99705=AXIS2_PLACEMENT_3D('',#204865,#118523,#118524);
#99706=AXIS2_PLACEMENT_3D('',#204866,#118525,#118526);
#99707=AXIS2_PLACEMENT_3D('',#204870,#118528,#118529);
#99708=AXIS2_PLACEMENT_3D('',#204872,#118531,#118532);
#99709=AXIS2_PLACEMENT_3D('',#204874,#118533,#118534);
#99710=AXIS2_PLACEMENT_3D('',#204876,#118536,#118537);
#99711=AXIS2_PLACEMENT_3D('',#204878,#118538,#118539);
#99712=AXIS2_PLACEMENT_3D('',#204880,#118541,#118542);
#99713=AXIS2_PLACEMENT_3D('',#204881,#118543,#118544);
#99714=AXIS2_PLACEMENT_3D('',#204882,#118545,#118546);
#99715=AXIS2_PLACEMENT_3D('',#204886,#118548,#118549);
#99716=AXIS2_PLACEMENT_3D('',#204888,#118551,#118552);
#99717=AXIS2_PLACEMENT_3D('',#204889,#118553,#118554);
#99718=AXIS2_PLACEMENT_3D('',#204890,#118555,#118556);
#99719=AXIS2_PLACEMENT_3D('',#204894,#118558,#118559);
#99720=AXIS2_PLACEMENT_3D('',#204896,#118561,#118562);
#99721=AXIS2_PLACEMENT_3D('',#204898,#118563,#118564);
#99722=AXIS2_PLACEMENT_3D('',#204899,#118565,#118566);
#99723=AXIS2_PLACEMENT_3D('',#204902,#118568,#118569);
#99724=AXIS2_PLACEMENT_3D('',#204903,#118570,#118571);
#99725=AXIS2_PLACEMENT_3D('',#204904,#118572,#118573);
#99726=AXIS2_PLACEMENT_3D('',#204906,#118574,#118575);
#99727=AXIS2_PLACEMENT_3D('',#204907,#118576,#118577);
#99728=AXIS2_PLACEMENT_3D('',#204909,#118579,#118580);
#99729=AXIS2_PLACEMENT_3D('',#204910,#118581,#118582);
#99730=AXIS2_PLACEMENT_3D('',#204911,#118583,#118584);
#99731=AXIS2_PLACEMENT_3D('',#204912,#118585,#118586);
#99732=AXIS2_PLACEMENT_3D('',#204913,#118587,#118588);
#99733=AXIS2_PLACEMENT_3D('',#204914,#118589,#118590);
#99734=AXIS2_PLACEMENT_3D('',#204915,#118591,#118592);
#99735=AXIS2_PLACEMENT_3D('',#204916,#118593,#118594);
#99736=AXIS2_PLACEMENT_3D('',#204917,#118595,#118596);
#99737=AXIS2_PLACEMENT_3D('',#204918,#118597,#118598);
#99738=AXIS2_PLACEMENT_3D('',#204919,#118599,#118600);
#99739=AXIS2_PLACEMENT_3D('',#204920,#118601,#118602);
#99740=AXIS2_PLACEMENT_3D('',#204921,#118603,#118604);
#99741=AXIS2_PLACEMENT_3D('',#204922,#118605,#118606);
#99742=AXIS2_PLACEMENT_3D('',#204923,#118607,#118608);
#99743=AXIS2_PLACEMENT_3D('',#205008,#118609,#118610);
#99744=AXIS2_PLACEMENT_3D('',#205012,#118612,#118613);
#99745=AXIS2_PLACEMENT_3D('',#205014,#118615,#118616);
#99746=AXIS2_PLACEMENT_3D('',#205017,#118618,#118619);
#99747=AXIS2_PLACEMENT_3D('',#205018,#118620,#118621);
#99748=AXIS2_PLACEMENT_3D('',#205021,#118623,#118624);
#99749=AXIS2_PLACEMENT_3D('',#205022,#118625,#118626);
#99750=AXIS2_PLACEMENT_3D('',#205025,#118628,#118629);
#99751=AXIS2_PLACEMENT_3D('',#205026,#118630,#118631);
#99752=AXIS2_PLACEMENT_3D('',#205029,#118633,#118634);
#99753=AXIS2_PLACEMENT_3D('',#205030,#118635,#118636);
#99754=AXIS2_PLACEMENT_3D('',#205033,#118638,#118639);
#99755=AXIS2_PLACEMENT_3D('',#205034,#118640,#118641);
#99756=AXIS2_PLACEMENT_3D('',#205036,#118642,#118643);
#99757=AXIS2_PLACEMENT_3D('',#205038,#118645,#118646);
#99758=AXIS2_PLACEMENT_3D('',#205042,#118648,#118649);
#99759=AXIS2_PLACEMENT_3D('',#205044,#118651,#118652);
#99760=AXIS2_PLACEMENT_3D('',#205048,#118654,#118655);
#99761=AXIS2_PLACEMENT_3D('',#205050,#118657,#118658);
#99762=AXIS2_PLACEMENT_3D('',#205052,#118659,#118660);
#99763=AXIS2_PLACEMENT_3D('',#205054,#118662,#118663);
#99764=AXIS2_PLACEMENT_3D('',#205056,#118664,#118665);
#99765=AXIS2_PLACEMENT_3D('',#205058,#118667,#118668);
#99766=AXIS2_PLACEMENT_3D('',#205060,#118669,#118670);
#99767=AXIS2_PLACEMENT_3D('',#205062,#118672,#118673);
#99768=AXIS2_PLACEMENT_3D('',#205064,#118674,#118675);
#99769=AXIS2_PLACEMENT_3D('',#205066,#118677,#118678);
#99770=AXIS2_PLACEMENT_3D('',#205067,#118679,#118680);
#99771=AXIS2_PLACEMENT_3D('',#205459,#118685,#118686);
#99772=AXIS2_PLACEMENT_3D('',#205462,#118689,#118690);
#99773=AXIS2_PLACEMENT_3D('',#205464,#118692,#118693);
#99774=AXIS2_PLACEMENT_3D('',#205466,#118695,#118696);
#99775=AXIS2_PLACEMENT_3D('',#205469,#118699,#118700);
#99776=AXIS2_PLACEMENT_3D('',#205471,#118702,#118703);
#99777=AXIS2_PLACEMENT_3D('',#205473,#118705,#118706);
#99778=AXIS2_PLACEMENT_3D('',#205477,#118708,#118709);
#99779=AXIS2_PLACEMENT_3D('',#205479,#118711,#118712);
#99780=AXIS2_PLACEMENT_3D('',#205481,#118713,#118714);
#99781=AXIS2_PLACEMENT_3D('',#205483,#118716,#118717);
#99782=AXIS2_PLACEMENT_3D('',#205485,#118718,#118719);
#99783=AXIS2_PLACEMENT_3D('',#205487,#118721,#118722);
#99784=AXIS2_PLACEMENT_3D('',#205489,#118723,#118724);
#99785=AXIS2_PLACEMENT_3D('',#205491,#118726,#118727);
#99786=AXIS2_PLACEMENT_3D('',#205495,#118729,#118730);
#99787=AXIS2_PLACEMENT_3D('',#205497,#118732,#118733);
#99788=AXIS2_PLACEMENT_3D('',#205499,#118734,#118735);
#99789=AXIS2_PLACEMENT_3D('',#205501,#118737,#118738);
#99790=AXIS2_PLACEMENT_3D('',#205502,#118739,#118740);
#99791=AXIS2_PLACEMENT_3D('',#205580,#118741,#118742);
#99792=AXIS2_PLACEMENT_3D('',#205679,#118743,#118744);
#99793=AXIS2_PLACEMENT_3D('',#206368,#118745,#118746);
#99794=AXIS2_PLACEMENT_3D('',#206961,#118747,#118748);
#99795=AXIS2_PLACEMENT_3D('',#206962,#118749,#118750);
#99796=AXIS2_PLACEMENT_3D('',#206963,#118751,#118752);
#99797=AXIS2_PLACEMENT_3D('',#206964,#118753,#118754);
#99798=AXIS2_PLACEMENT_3D('',#206965,#118755,#118756);
#99799=AXIS2_PLACEMENT_3D('',#206966,#118757,#118758);
#99800=AXIS2_PLACEMENT_3D('',#206967,#118759,#118760);
#99801=AXIS2_PLACEMENT_3D('',#206968,#118761,#118762);
#99802=AXIS2_PLACEMENT_3D('',#206969,#118763,#118764);
#99803=AXIS2_PLACEMENT_3D('',#206970,#118765,#118766);
#99804=AXIS2_PLACEMENT_3D('',#206971,#118767,#118768);
#99805=AXIS2_PLACEMENT_3D('',#206973,#118770,#118771);
#99806=AXIS2_PLACEMENT_3D('',#206975,#118773,#118774);
#99807=AXIS2_PLACEMENT_3D('',#206977,#118776,#118777);
#99808=AXIS2_PLACEMENT_3D('',#206979,#118779,#118780);
#99809=AXIS2_PLACEMENT_3D('',#206981,#118782,#118783);
#99810=AXIS2_PLACEMENT_3D('',#206983,#118785,#118786);
#99811=AXIS2_PLACEMENT_3D('',#206985,#118788,#118789);
#99812=AXIS2_PLACEMENT_3D('',#206987,#118791,#118792);
#99813=AXIS2_PLACEMENT_3D('',#206989,#118794,#118795);
#99814=AXIS2_PLACEMENT_3D('',#206991,#118797,#118798);
#99815=AXIS2_PLACEMENT_3D('',#206992,#118799,#118800);
#99816=AXIS2_PLACEMENT_3D('',#206993,#118801,#118802);
#99817=AXIS2_PLACEMENT_3D('',#206994,#118803,#118804);
#99818=AXIS2_PLACEMENT_3D('',#206995,#118805,#118806);
#99819=AXIS2_PLACEMENT_3D('',#206996,#118807,#118808);
#99820=AXIS2_PLACEMENT_3D('',#206997,#118809,#118810);
#99821=AXIS2_PLACEMENT_3D('',#206998,#118811,#118812);
#99822=AXIS2_PLACEMENT_3D('',#207000,#118814,#118815);
#99823=AXIS2_PLACEMENT_3D('',#207002,#118817,#118818);
#99824=AXIS2_PLACEMENT_3D('',#207004,#118820,#118821);
#99825=AXIS2_PLACEMENT_3D('',#207006,#118823,#118824);
#99826=AXIS2_PLACEMENT_3D('',#207008,#118826,#118827);
#99827=AXIS2_PLACEMENT_3D('',#207010,#118829,#118830);
#99828=AXIS2_PLACEMENT_3D('',#207012,#118832,#118833);
#99829=AXIS2_PLACEMENT_3D('',#207014,#118835,#118836);
#99830=AXIS2_PLACEMENT_3D('',#207016,#118838,#118839);
#99831=AXIS2_PLACEMENT_3D('',#207018,#118841,#118842);
#99832=AXIS2_PLACEMENT_3D('',#207020,#118844,#118845);
#99833=AXIS2_PLACEMENT_3D('',#207022,#118847,#118848);
#99834=AXIS2_PLACEMENT_3D('',#207024,#118850,#118851);
#99835=AXIS2_PLACEMENT_3D('',#207026,#118853,#118854);
#99836=AXIS2_PLACEMENT_3D('',#207027,#118855,#118856);
#99837=AXIS2_PLACEMENT_3D('',#207028,#118857,#118858);
#99838=AXIS2_PLACEMENT_3D('',#207029,#118859,#118860);
#99839=AXIS2_PLACEMENT_3D('',#207030,#118861,#118862);
#99840=AXIS2_PLACEMENT_3D('',#207031,#118863,#118864);
#99841=AXIS2_PLACEMENT_3D('',#207032,#118865,#118866);
#99842=AXIS2_PLACEMENT_3D('',#207033,#118867,#118868);
#99843=AXIS2_PLACEMENT_3D('',#207034,#118869,#118870);
#99844=AXIS2_PLACEMENT_3D('',#207035,#118871,#118872);
#99845=AXIS2_PLACEMENT_3D('',#207036,#118873,#118874);
#99846=AXIS2_PLACEMENT_3D('',#207037,#118875,#118876);
#99847=AXIS2_PLACEMENT_3D('',#207038,#118877,#118878);
#99848=AXIS2_PLACEMENT_3D('',#207039,#118879,#118880);
#99849=AXIS2_PLACEMENT_3D('',#207040,#118881,#118882);
#99850=AXIS2_PLACEMENT_3D('',#207041,#118883,#118884);
#99851=AXIS2_PLACEMENT_3D('',#207042,#118885,#118886);
#99852=AXIS2_PLACEMENT_3D('',#207044,#118888,#118889);
#99853=AXIS2_PLACEMENT_3D('',#207046,#118891,#118892);
#99854=AXIS2_PLACEMENT_3D('',#207048,#118894,#118895);
#99855=AXIS2_PLACEMENT_3D('',#207050,#118897,#118898);
#99856=AXIS2_PLACEMENT_3D('',#207052,#118900,#118901);
#99857=AXIS2_PLACEMENT_3D('',#207054,#118903,#118904);
#99858=AXIS2_PLACEMENT_3D('',#207056,#118906,#118907);
#99859=AXIS2_PLACEMENT_3D('',#207058,#118909,#118910);
#99860=AXIS2_PLACEMENT_3D('',#207060,#118912,#118913);
#99861=AXIS2_PLACEMENT_3D('',#207062,#118915,#118916);
#99862=AXIS2_PLACEMENT_3D('',#207064,#118918,#118919);
#99863=AXIS2_PLACEMENT_3D('',#207066,#118921,#118922);
#99864=AXIS2_PLACEMENT_3D('',#207068,#118924,#118925);
#99865=AXIS2_PLACEMENT_3D('',#207070,#118927,#118928);
#99866=AXIS2_PLACEMENT_3D('',#207072,#118930,#118931);
#99867=AXIS2_PLACEMENT_3D('',#207074,#118933,#118934);
#99868=AXIS2_PLACEMENT_3D('',#207076,#118936,#118937);
#99869=AXIS2_PLACEMENT_3D('',#207078,#118939,#118940);
#99870=AXIS2_PLACEMENT_3D('',#207080,#118942,#118943);
#99871=AXIS2_PLACEMENT_3D('',#207082,#118945,#118946);
#99872=AXIS2_PLACEMENT_3D('',#207084,#118948,#118949);
#99873=AXIS2_PLACEMENT_3D('',#207086,#118951,#118952);
#99874=AXIS2_PLACEMENT_3D('',#207088,#118954,#118955);
#99875=AXIS2_PLACEMENT_3D('',#207090,#118957,#118958);
#99876=AXIS2_PLACEMENT_3D('',#207092,#118960,#118961);
#99877=AXIS2_PLACEMENT_3D('',#207094,#118963,#118964);
#99878=AXIS2_PLACEMENT_3D('',#207096,#118966,#118967);
#99879=AXIS2_PLACEMENT_3D('',#207118,#118969,#118970);
#99880=AXIS2_PLACEMENT_3D('',#207173,#118971,#118972);
#99881=AXIS2_PLACEMENT_3D('',#207199,#118973,#118974);
#99882=AXIS2_PLACEMENT_3D('',#207200,#118975,#118976);
#99883=AXIS2_PLACEMENT_3D('',#207202,#118977,#118978);
#99884=AXIS2_PLACEMENT_3D('',#207203,#118979,#118980);
#99885=AXIS2_PLACEMENT_3D('',#207204,#118981,#118982);
#99886=AXIS2_PLACEMENT_3D('',#207206,#118983,#118984);
#99887=AXIS2_PLACEMENT_3D('',#207208,#118985,#118986);
#99888=AXIS2_PLACEMENT_3D('',#207210,#118987,#118988);
#99889=AXIS2_PLACEMENT_3D('',#207211,#118989,#118990);
#99890=AXIS2_PLACEMENT_3D('',#207244,#118991,#118992);
#99891=AXIS2_PLACEMENT_3D('',#207326,#118993,#118994);
#99892=AXIS2_PLACEMENT_3D('',#207372,#118995,#118996);
#99893=AXIS2_PLACEMENT_3D('',#207423,#118997,#118998);
#99894=AXIS2_PLACEMENT_3D('',#207425,#118999,#119000);
#99895=AXIS2_PLACEMENT_3D('',#207426,#119001,#119002);
#99896=AXIS2_PLACEMENT_3D('',#207459,#119003,#119004);
#99897=AXIS2_PLACEMENT_3D('',#207523,#119005,#119006);
#99898=AXIS2_PLACEMENT_3D('',#207526,#119007,#119008);
#99899=AXIS2_PLACEMENT_3D('',#207527,#119009,#119010);
#99900=AXIS2_PLACEMENT_3D('',#207528,#119011,#119012);
#99901=AXIS2_PLACEMENT_3D('',#207549,#119013,#119014);
#99902=AXIS2_PLACEMENT_3D('',#207582,#119015,#119016);
#99903=AXIS2_PLACEMENT_3D('',#207585,#119017,#119018);
#99904=AXIS2_PLACEMENT_3D('',#207586,#119019,#119020);
#99905=AXIS2_PLACEMENT_3D('',#207587,#119021,#119022);
#99906=AXIS2_PLACEMENT_3D('',#207620,#119023,#119024);
#99907=AXIS2_PLACEMENT_3D('',#207743,#119025,#119026);
#99908=AXIS2_PLACEMENT_3D('',#207746,#119027,#119028);
#99909=AXIS2_PLACEMENT_3D('',#207747,#119029,#119030);
#99910=AXIS2_PLACEMENT_3D('',#207748,#119031,#119032);
#99911=AXIS2_PLACEMENT_3D('',#207763,#119033,#119034);
#99912=AXIS2_PLACEMENT_3D('',#207797,#119035,#119036);
#99913=AXIS2_PLACEMENT_3D('',#207855,#119037,#119038);
#99914=AXIS2_PLACEMENT_3D('',#207961,#119039,#119040);
#99915=AXIS2_PLACEMENT_3D('',#207962,#119041,#119042);
#99916=AXIS2_PLACEMENT_3D('',#207963,#119043,#119044);
#99917=AXIS2_PLACEMENT_3D('',#208002,#119045,#119046);
#99918=AXIS2_PLACEMENT_3D('',#208039,#119047,#119048);
#99919=AXIS2_PLACEMENT_3D('',#208081,#119049,#119050);
#99920=AXIS2_PLACEMENT_3D('',#208110,#119051,#119052);
#99921=AXIS2_PLACEMENT_3D('',#208160,#119053,#119054);
#99922=AXIS2_PLACEMENT_3D('',#208333,#119055,#119056);
#99923=AXIS2_PLACEMENT_3D('',#208397,#119057,#119058);
#99924=AXIS2_PLACEMENT_3D('',#208399,#119059,#119060);
#99925=AXIS2_PLACEMENT_3D('',#208400,#119061,#119062);
#99926=AXIS2_PLACEMENT_3D('',#208415,#119063,#119064);
#99927=AXIS2_PLACEMENT_3D('',#208449,#119065,#119066);
#99928=AXIS2_PLACEMENT_3D('',#208484,#119067,#119068);
#99929=AXIS2_PLACEMENT_3D('',#208589,#119069,#119070);
#99930=AXIS2_PLACEMENT_3D('',#208592,#119071,#119072);
#99931=AXIS2_PLACEMENT_3D('',#208593,#119073,#119074);
#99932=AXIS2_PLACEMENT_3D('',#208594,#119075,#119076);
#99933=AXIS2_PLACEMENT_3D('',#208595,#119077,#119078);
#99934=AXIS2_PLACEMENT_3D('',#208597,#119079,#119080);
#99935=AXIS2_PLACEMENT_3D('',#208598,#119081,#119082);
#99936=AXIS2_PLACEMENT_3D('',#208599,#119083,#119084);
#99937=AXIS2_PLACEMENT_3D('',#208602,#119085,#119086);
#99938=AXIS2_PLACEMENT_3D('',#208603,#119087,#119088);
#99939=AXIS2_PLACEMENT_3D('',#208604,#119089,#119090);
#99940=AXIS2_PLACEMENT_3D('',#208619,#119091,#119092);
#99941=AXIS2_PLACEMENT_3D('',#208628,#119093,#119094);
#99942=AXIS2_PLACEMENT_3D('',#208629,#119095,#119096);
#99943=AXIS2_PLACEMENT_3D('',#208630,#119097,#119098);
#99944=AXIS2_PLACEMENT_3D('',#208631,#119099,#119100);
#99945=AXIS2_PLACEMENT_3D('',#208633,#119101,#119102);
#99946=AXIS2_PLACEMENT_3D('',#208635,#119103,#119104);
#99947=AXIS2_PLACEMENT_3D('',#208636,#119105,#119106);
#99948=AXIS2_PLACEMENT_3D('',#208637,#119107,#119108);
#99949=AXIS2_PLACEMENT_3D('',#208640,#119109,#119110);
#99950=AXIS2_PLACEMENT_3D('',#208641,#119111,#119112);
#99951=AXIS2_PLACEMENT_3D('',#208642,#119113,#119114);
#99952=AXIS2_PLACEMENT_3D('',#208643,#119115,#119116);
#99953=AXIS2_PLACEMENT_3D('',#208646,#119117,#119118);
#99954=AXIS2_PLACEMENT_3D('',#208647,#119119,#119120);
#99955=AXIS2_PLACEMENT_3D('',#208648,#119121,#119122);
#99956=AXIS2_PLACEMENT_3D('',#208649,#119123,#119124);
#99957=AXIS2_PLACEMENT_3D('',#208652,#119125,#119126);
#99958=AXIS2_PLACEMENT_3D('',#208653,#119127,#119128);
#99959=AXIS2_PLACEMENT_3D('',#208654,#119129,#119130);
#99960=AXIS2_PLACEMENT_3D('',#208655,#119131,#119132);
#99961=AXIS2_PLACEMENT_3D('',#208658,#119133,#119134);
#99962=AXIS2_PLACEMENT_3D('',#208659,#119135,#119136);
#99963=AXIS2_PLACEMENT_3D('',#208660,#119137,#119138);
#99964=AXIS2_PLACEMENT_3D('',#208661,#119139,#119140);
#99965=AXIS2_PLACEMENT_3D('',#208664,#119141,#119142);
#99966=AXIS2_PLACEMENT_3D('',#208665,#119143,#119144);
#99967=AXIS2_PLACEMENT_3D('',#208666,#119145,#119146);
#99968=AXIS2_PLACEMENT_3D('',#208667,#119147,#119148);
#99969=AXIS2_PLACEMENT_3D('',#208670,#119149,#119150);
#99970=AXIS2_PLACEMENT_3D('',#208671,#119151,#119152);
#99971=AXIS2_PLACEMENT_3D('',#208672,#119153,#119154);
#99972=AXIS2_PLACEMENT_3D('',#208673,#119155,#119156);
#99973=AXIS2_PLACEMENT_3D('',#208676,#119157,#119158);
#99974=AXIS2_PLACEMENT_3D('',#208677,#119159,#119160);
#99975=AXIS2_PLACEMENT_3D('',#208678,#119161,#119162);
#99976=AXIS2_PLACEMENT_3D('',#208679,#119163,#119164);
#99977=AXIS2_PLACEMENT_3D('',#208680,#119165,#119166);
#99978=AXIS2_PLACEMENT_3D('',#208681,#119167,#119168);
#99979=AXIS2_PLACEMENT_3D('',#208695,#119169,#119170);
#99980=AXIS2_PLACEMENT_3D('',#208697,#119171,#119172);
#99981=AXIS2_PLACEMENT_3D('',#208698,#119173,#119174);
#99982=AXIS2_PLACEMENT_3D('',#208713,#119175,#119176);
#99983=AXIS2_PLACEMENT_3D('',#208718,#119177,#119178);
#99984=AXIS2_PLACEMENT_3D('',#208812,#119179,#119180);
#99985=AXIS2_PLACEMENT_3D('',#208851,#119181,#119182);
#99986=AXIS2_PLACEMENT_3D('',#209013,#119183,#119184);
#99987=AXIS2_PLACEMENT_3D('',#209014,#119185,#119186);
#99988=AXIS2_PLACEMENT_3D('',#209015,#119187,#119188);
#99989=AXIS2_PLACEMENT_3D('',#209030,#119189,#119190);
#99990=AXIS2_PLACEMENT_3D('',#209031,#119191,#119192);
#99991=AXIS2_PLACEMENT_3D('',#209032,#119193,#119194);
#99992=AXIS2_PLACEMENT_3D('',#209047,#119195,#119196);
#99993=AXIS2_PLACEMENT_3D('',#209121,#119197,#119198);
#99994=AXIS2_PLACEMENT_3D('',#209210,#119199,#119200);
#99995=AXIS2_PLACEMENT_3D('',#209379,#119201,#119202);
#99996=AXIS2_PLACEMENT_3D('',#209565,#119203,#119204);
#99997=AXIS2_PLACEMENT_3D('',#209737,#119205,#119206);
#99998=AXIS2_PLACEMENT_3D('',#209857,#119207,#119208);
#99999=AXIS2_PLACEMENT_3D('',#209858,#119209,#119210);
#100000=AXIS2_PLACEMENT_3D('',#209859,#119211,#119212);
#100001=AXIS2_PLACEMENT_3D('',#209916,#119213,#119214);
#100002=AXIS2_PLACEMENT_3D('',#210016,#119215,#119216);
#100003=AXIS2_PLACEMENT_3D('',#210035,#119217,#119218);
#100004=AXIS2_PLACEMENT_3D('',#210038,#119219,#119220);
#100005=AXIS2_PLACEMENT_3D('',#210039,#119221,#119222);
#100006=AXIS2_PLACEMENT_3D('',#210040,#119223,#119224);
#100007=AXIS2_PLACEMENT_3D('',#210067,#119225,#119226);
#100008=AXIS2_PLACEMENT_3D('',#210259,#119227,#119228);
#100009=AXIS2_PLACEMENT_3D('',#210393,#119229,#119230);
#100010=AXIS2_PLACEMENT_3D('',#210473,#119231,#119232);
#100011=AXIS2_PLACEMENT_3D('',#210556,#119233,#119234);
#100012=AXIS2_PLACEMENT_3D('',#210557,#119235,#119236);
#100013=AXIS2_PLACEMENT_3D('',#210558,#119237,#119238);
#100014=AXIS2_PLACEMENT_3D('',#210573,#119239,#119240);
#100015=AXIS2_PLACEMENT_3D('',#210734,#119241,#119242);
#100016=AXIS2_PLACEMENT_3D('',#210735,#119243,#119244);
#100017=AXIS2_PLACEMENT_3D('',#210736,#119245,#119246);
#100018=AXIS2_PLACEMENT_3D('',#210829,#119247,#119248);
#100019=AXIS2_PLACEMENT_3D('',#210834,#119251,#119252);
#100020=AXIS2_PLACEMENT_3D('',#210845,#119253,#119254);
#100021=AXIS2_PLACEMENT_3D('',#210847,#119255,#119256);
#100022=AXIS2_PLACEMENT_3D('',#210848,#119257,#119258);
#100023=AXIS2_PLACEMENT_3D('',#210849,#119259,#119260);
#100024=AXIS2_PLACEMENT_3D('',#210851,#119261,#119262);
#100025=AXIS2_PLACEMENT_3D('',#210852,#119263,#119264);
#100026=AXIS2_PLACEMENT_3D('',#210854,#119265,#119266);
#100027=AXIS2_PLACEMENT_3D('',#210855,#119267,#119268);
#100028=AXIS2_PLACEMENT_3D('',#210867,#119269,#119270);
#100029=AXIS2_PLACEMENT_3D('',#210868,#119271,#119272);
#100030=AXIS2_PLACEMENT_3D('',#210869,#119273,#119274);
#100031=AXIS2_PLACEMENT_3D('',#210870,#119275,#119276);
#100032=AXIS2_PLACEMENT_3D('',#210873,#119279,#119280);
#100033=AXIS2_PLACEMENT_3D('',#210878,#119283,#119284);
#100034=AXIS2_PLACEMENT_3D('',#210889,#119285,#119286);
#100035=AXIS2_PLACEMENT_3D('',#210891,#119287,#119288);
#100036=AXIS2_PLACEMENT_3D('',#210892,#119289,#119290);
#100037=AXIS2_PLACEMENT_3D('',#210893,#119291,#119292);
#100038=AXIS2_PLACEMENT_3D('',#210896,#119293,#119294);
#100039=AXIS2_PLACEMENT_3D('',#210897,#119295,#119296);
#100040=AXIS2_PLACEMENT_3D('',#210898,#119297,#119298);
#100041=AXIS2_PLACEMENT_3D('',#210910,#119299,#119300);
#100042=AXIS2_PLACEMENT_3D('',#210911,#119301,#119302);
#100043=AXIS2_PLACEMENT_3D('',#210912,#119303,#119304);
#100044=AXIS2_PLACEMENT_3D('',#210913,#119305,#119306);
#100045=AXIS2_PLACEMENT_3D('',#210916,#119309,#119310);
#100046=AXIS2_PLACEMENT_3D('',#210921,#119313,#119314);
#100047=AXIS2_PLACEMENT_3D('',#210933,#119315,#119316);
#100048=AXIS2_PLACEMENT_3D('',#210934,#119317,#119318);
#100049=AXIS2_PLACEMENT_3D('',#210935,#119319,#119320);
#100050=AXIS2_PLACEMENT_3D('',#210936,#119321,#119322);
#100051=AXIS2_PLACEMENT_3D('',#210939,#119323,#119324);
#100052=AXIS2_PLACEMENT_3D('',#210940,#119325,#119326);
#100053=AXIS2_PLACEMENT_3D('',#210941,#119327,#119328);
#100054=AXIS2_PLACEMENT_3D('',#210952,#119329,#119330);
#100055=AXIS2_PLACEMENT_3D('',#210954,#119331,#119332);
#100056=AXIS2_PLACEMENT_3D('',#210955,#119333,#119334);
#100057=AXIS2_PLACEMENT_3D('',#210956,#119335,#119336);
#100058=AXIS2_PLACEMENT_3D('',#210959,#119339,#119340);
#100059=AXIS2_PLACEMENT_3D('',#210964,#119343,#119344);
#100060=AXIS2_PLACEMENT_3D('',#210976,#119345,#119346);
#100061=AXIS2_PLACEMENT_3D('',#210977,#119347,#119348);
#100062=AXIS2_PLACEMENT_3D('',#210978,#119349,#119350);
#100063=AXIS2_PLACEMENT_3D('',#210979,#119351,#119352);
#100064=AXIS2_PLACEMENT_3D('',#210982,#119353,#119354);
#100065=AXIS2_PLACEMENT_3D('',#210983,#119355,#119356);
#100066=AXIS2_PLACEMENT_3D('',#210984,#119357,#119358);
#100067=AXIS2_PLACEMENT_3D('',#210995,#119359,#119360);
#100068=AXIS2_PLACEMENT_3D('',#210997,#119361,#119362);
#100069=AXIS2_PLACEMENT_3D('',#210998,#119363,#119364);
#100070=AXIS2_PLACEMENT_3D('',#210999,#119365,#119366);
#100071=AXIS2_PLACEMENT_3D('',#211002,#119369,#119370);
#100072=AXIS2_PLACEMENT_3D('',#211005,#119373,#119374);
#100073=AXIS2_PLACEMENT_3D('',#211008,#119377,#119378);
#100074=AXIS2_PLACEMENT_3D('',#211011,#119381,#119382);
#100075=AXIS2_PLACEMENT_3D('',#211014,#119385,#119386);
#100076=AXIS2_PLACEMENT_3D('',#211017,#119389,#119390);
#100077=AXIS2_PLACEMENT_3D('',#211020,#119393,#119394);
#100078=AXIS2_PLACEMENT_3D('',#211023,#119397,#119398);
#100079=AXIS2_PLACEMENT_3D('',#211026,#119401,#119402);
#100080=AXIS2_PLACEMENT_3D('',#211029,#119403,#119404);
#100081=AXIS2_PLACEMENT_3D('',#211031,#119405,#119406);
#100082=AXIS2_PLACEMENT_3D('',#211033,#119407,#119408);
#100083=AXIS2_PLACEMENT_3D('',#211034,#119409,#119410);
#100084=AXIS2_PLACEMENT_3D('',#211035,#119411,#119412);
#100085=AXIS2_PLACEMENT_3D('',#211038,#119413,#119414);
#100086=AXIS2_PLACEMENT_3D('',#211041,#119417,#119418);
#100087=AXIS2_PLACEMENT_3D('',#211044,#119419,#119420);
#100088=AXIS2_PLACEMENT_3D('',#211045,#119421,#119422);
#100089=AXIS2_PLACEMENT_3D('',#211046,#119423,#119424);
#100090=AXIS2_PLACEMENT_3D('',#211047,#119425,#119426);
#100091=AXIS2_PLACEMENT_3D('',#211050,#119427,#119428);
#100092=AXIS2_PLACEMENT_3D('',#211051,#119429,#119430);
#100093=AXIS2_PLACEMENT_3D('',#211052,#119431,#119432);
#100094=AXIS2_PLACEMENT_3D('',#211053,#119433,#119434);
#100095=AXIS2_PLACEMENT_3D('',#211056,#119435,#119436);
#100096=AXIS2_PLACEMENT_3D('',#211057,#119437,#119438);
#100097=AXIS2_PLACEMENT_3D('',#211058,#119439,#119440);
#100098=AXIS2_PLACEMENT_3D('',#211059,#119441,#119442);
#100099=AXIS2_PLACEMENT_3D('',#211062,#119443,#119444);
#100100=AXIS2_PLACEMENT_3D('',#211065,#119447,#119448);
#100101=AXIS2_PLACEMENT_3D('',#211068,#119449,#119450);
#100102=AXIS2_PLACEMENT_3D('',#211069,#119451,#119452);
#100103=AXIS2_PLACEMENT_3D('',#211070,#119453,#119454);
#100104=AXIS2_PLACEMENT_3D('',#211071,#119455,#119456);
#100105=AXIS2_PLACEMENT_3D('',#211074,#119457,#119458);
#100106=AXIS2_PLACEMENT_3D('',#211075,#119459,#119460);
#100107=AXIS2_PLACEMENT_3D('',#211076,#119461,#119462);
#100108=AXIS2_PLACEMENT_3D('',#211077,#119463,#119464);
#100109=AXIS2_PLACEMENT_3D('',#211080,#119465,#119466);
#100110=AXIS2_PLACEMENT_3D('',#211081,#119467,#119468);
#100111=AXIS2_PLACEMENT_3D('',#211082,#119469,#119470);
#100112=AXIS2_PLACEMENT_3D('',#211083,#119471,#119472);
#100113=AXIS2_PLACEMENT_3D('',#211086,#119475,#119476);
#100114=AXIS2_PLACEMENT_3D('',#211089,#119477,#119478);
#100115=AXIS2_PLACEMENT_3D('',#211091,#119479,#119480);
#100116=AXIS2_PLACEMENT_3D('',#211093,#119481,#119482);
#100117=AXIS2_PLACEMENT_3D('',#211094,#119483,#119484);
#100118=AXIS2_PLACEMENT_3D('',#211095,#119485,#119486);
#100119=AXIS2_PLACEMENT_3D('',#211098,#119487,#119488);
#100120=AXIS2_PLACEMENT_3D('',#211101,#119491,#119492);
#100121=AXIS2_PLACEMENT_3D('',#211104,#119493,#119494);
#100122=AXIS2_PLACEMENT_3D('',#211105,#119495,#119496);
#100123=AXIS2_PLACEMENT_3D('',#211106,#119497,#119498);
#100124=AXIS2_PLACEMENT_3D('',#211107,#119499,#119500);
#100125=AXIS2_PLACEMENT_3D('',#211110,#119501,#119502);
#100126=AXIS2_PLACEMENT_3D('',#211111,#119503,#119504);
#100127=AXIS2_PLACEMENT_3D('',#211112,#119505,#119506);
#100128=AXIS2_PLACEMENT_3D('',#211113,#119507,#119508);
#100129=AXIS2_PLACEMENT_3D('',#211116,#119509,#119510);
#100130=AXIS2_PLACEMENT_3D('',#211117,#119511,#119512);
#100131=AXIS2_PLACEMENT_3D('',#211118,#119513,#119514);
#100132=AXIS2_PLACEMENT_3D('',#211119,#119515,#119516);
#100133=AXIS2_PLACEMENT_3D('',#211122,#119517,#119518);
#100134=AXIS2_PLACEMENT_3D('',#211125,#119521,#119522);
#100135=AXIS2_PLACEMENT_3D('',#211128,#119523,#119524);
#100136=AXIS2_PLACEMENT_3D('',#211131,#119527,#119528);
#100137=AXIS2_PLACEMENT_3D('',#211132,#119529,#119530);
#100138=AXIS2_PLACEMENT_3D('',#211133,#119531,#119532);
#100139=AXIS2_PLACEMENT_3D('',#211134,#119533,#119534);
#100140=AXIS2_PLACEMENT_3D('',#211137,#119535,#119536);
#100141=AXIS2_PLACEMENT_3D('',#211139,#119537,#119538);
#100142=AXIS2_PLACEMENT_3D('',#211141,#119539,#119540);
#100143=AXIS2_PLACEMENT_3D('',#211142,#119541,#119542);
#100144=AXIS2_PLACEMENT_3D('',#211143,#119543,#119544);
#100145=AXIS2_PLACEMENT_3D('',#211146,#119545,#119546);
#100146=AXIS2_PLACEMENT_3D('',#211149,#119549,#119550);
#100147=AXIS2_PLACEMENT_3D('',#211152,#119551,#119552);
#100148=AXIS2_PLACEMENT_3D('',#211153,#119553,#119554);
#100149=AXIS2_PLACEMENT_3D('',#211154,#119555,#119556);
#100150=AXIS2_PLACEMENT_3D('',#211155,#119557,#119558);
#100151=AXIS2_PLACEMENT_3D('',#211158,#119559,#119560);
#100152=AXIS2_PLACEMENT_3D('',#211159,#119561,#119562);
#100153=AXIS2_PLACEMENT_3D('',#211160,#119563,#119564);
#100154=AXIS2_PLACEMENT_3D('',#211161,#119565,#119566);
#100155=AXIS2_PLACEMENT_3D('',#211164,#119567,#119568);
#100156=AXIS2_PLACEMENT_3D('',#211165,#119569,#119570);
#100157=AXIS2_PLACEMENT_3D('',#211166,#119571,#119572);
#100158=AXIS2_PLACEMENT_3D('',#211167,#119573,#119574);
#100159=AXIS2_PLACEMENT_3D('',#211170,#119575,#119576);
#100160=AXIS2_PLACEMENT_3D('',#211173,#119579,#119580);
#100161=AXIS2_PLACEMENT_3D('',#211176,#119581,#119582);
#100162=AXIS2_PLACEMENT_3D('',#211179,#119585,#119586);
#100163=AXIS2_PLACEMENT_3D('',#211180,#119587,#119588);
#100164=AXIS2_PLACEMENT_3D('',#211181,#119589,#119590);
#100165=AXIS2_PLACEMENT_3D('',#211182,#119591,#119592);
#100166=AXIS2_PLACEMENT_3D('',#211185,#119593,#119594);
#100167=AXIS2_PLACEMENT_3D('',#211187,#119595,#119596);
#100168=AXIS2_PLACEMENT_3D('',#211189,#119597,#119598);
#100169=AXIS2_PLACEMENT_3D('',#211190,#119599,#119600);
#100170=AXIS2_PLACEMENT_3D('',#211191,#119601,#119602);
#100171=AXIS2_PLACEMENT_3D('',#211194,#119603,#119604);
#100172=AXIS2_PLACEMENT_3D('',#211197,#119607,#119608);
#100173=AXIS2_PLACEMENT_3D('',#211200,#119609,#119610);
#100174=AXIS2_PLACEMENT_3D('',#211203,#119613,#119614);
#100175=AXIS2_PLACEMENT_3D('',#211206,#119615,#119616);
#100176=AXIS2_PLACEMENT_3D('',#211207,#119617,#119618);
#100177=AXIS2_PLACEMENT_3D('',#211208,#119619,#119620);
#100178=AXIS2_PLACEMENT_3D('',#211209,#119621,#119622);
#100179=AXIS2_PLACEMENT_3D('',#211212,#119623,#119624);
#100180=AXIS2_PLACEMENT_3D('',#211213,#119625,#119626);
#100181=AXIS2_PLACEMENT_3D('',#211214,#119627,#119628);
#100182=AXIS2_PLACEMENT_3D('',#211215,#119629,#119630);
#100183=AXIS2_PLACEMENT_3D('',#211218,#119631,#119632);
#100184=AXIS2_PLACEMENT_3D('',#211221,#119635,#119636);
#100185=AXIS2_PLACEMENT_3D('',#211224,#119637,#119638);
#100186=AXIS2_PLACEMENT_3D('',#211227,#119641,#119642);
#100187=AXIS2_PLACEMENT_3D('',#211228,#119643,#119644);
#100188=AXIS2_PLACEMENT_3D('',#211229,#119645,#119646);
#100189=AXIS2_PLACEMENT_3D('',#211230,#119647,#119648);
#100190=AXIS2_PLACEMENT_3D('',#211233,#119649,#119650);
#100191=AXIS2_PLACEMENT_3D('',#211235,#119651,#119652);
#100192=AXIS2_PLACEMENT_3D('',#211237,#119653,#119654);
#100193=AXIS2_PLACEMENT_3D('',#211238,#119655,#119656);
#100194=AXIS2_PLACEMENT_3D('',#211239,#119657,#119658);
#100195=AXIS2_PLACEMENT_3D('',#211242,#119659,#119660);
#100196=AXIS2_PLACEMENT_3D('',#211245,#119663,#119664);
#100197=AXIS2_PLACEMENT_3D('',#211248,#119665,#119666);
#100198=AXIS2_PLACEMENT_3D('',#211251,#119669,#119670);
#100199=AXIS2_PLACEMENT_3D('',#211254,#119671,#119672);
#100200=AXIS2_PLACEMENT_3D('',#211255,#119673,#119674);
#100201=AXIS2_PLACEMENT_3D('',#211256,#119675,#119676);
#100202=AXIS2_PLACEMENT_3D('',#211257,#119677,#119678);
#100203=AXIS2_PLACEMENT_3D('',#211260,#119679,#119680);
#100204=AXIS2_PLACEMENT_3D('',#211261,#119681,#119682);
#100205=AXIS2_PLACEMENT_3D('',#211262,#119683,#119684);
#100206=AXIS2_PLACEMENT_3D('',#211263,#119685,#119686);
#100207=AXIS2_PLACEMENT_3D('',#211266,#119687,#119688);
#100208=AXIS2_PLACEMENT_3D('',#211267,#119689,#119690);
#100209=AXIS2_PLACEMENT_3D('',#211268,#119691,#119692);
#100210=AXIS2_PLACEMENT_3D('',#211269,#119693,#119694);
#100211=AXIS2_PLACEMENT_3D('',#211272,#119695,#119696);
#100212=AXIS2_PLACEMENT_3D('',#211275,#119699,#119700);
#100213=AXIS2_PLACEMENT_3D('',#211278,#119701,#119702);
#100214=AXIS2_PLACEMENT_3D('',#211279,#119703,#119704);
#100215=AXIS2_PLACEMENT_3D('',#211280,#119705,#119706);
#100216=AXIS2_PLACEMENT_3D('',#211281,#119707,#119708);
#100217=AXIS2_PLACEMENT_3D('',#211282,#119709,#119710);
#100218=AXIS2_PLACEMENT_3D('',#211283,#119711,#119712);
#100219=AXIS2_PLACEMENT_3D('',#211284,#119713,#119714);
#100220=AXIS2_PLACEMENT_3D('',#211287,#119715,#119716);
#100221=AXIS2_PLACEMENT_3D('',#211289,#119717,#119718);
#100222=AXIS2_PLACEMENT_3D('',#211291,#119719,#119720);
#100223=AXIS2_PLACEMENT_3D('',#211292,#119721,#119722);
#100224=AXIS2_PLACEMENT_3D('',#211293,#119723,#119724);
#100225=AXIS2_PLACEMENT_3D('',#211296,#119725,#119726);
#100226=AXIS2_PLACEMENT_3D('',#211299,#119729,#119730);
#100227=AXIS2_PLACEMENT_3D('',#211302,#119731,#119732);
#100228=AXIS2_PLACEMENT_3D('',#211305,#119735,#119736);
#100229=AXIS2_PLACEMENT_3D('',#211308,#119737,#119738);
#100230=AXIS2_PLACEMENT_3D('',#211309,#119739,#119740);
#100231=AXIS2_PLACEMENT_3D('',#211310,#119741,#119742);
#100232=AXIS2_PLACEMENT_3D('',#211311,#119743,#119744);
#100233=AXIS2_PLACEMENT_3D('',#211314,#119745,#119746);
#100234=AXIS2_PLACEMENT_3D('',#211315,#119747,#119748);
#100235=AXIS2_PLACEMENT_3D('',#211316,#119749,#119750);
#100236=AXIS2_PLACEMENT_3D('',#211317,#119751,#119752);
#100237=AXIS2_PLACEMENT_3D('',#211320,#119753,#119754);
#100238=AXIS2_PLACEMENT_3D('',#211323,#119757,#119758);
#100239=AXIS2_PLACEMENT_3D('',#211326,#119759,#119760);
#100240=AXIS2_PLACEMENT_3D('',#211329,#119763,#119764);
#100241=AXIS2_PLACEMENT_3D('',#211330,#119765,#119766);
#100242=AXIS2_PLACEMENT_3D('',#211331,#119767,#119768);
#100243=AXIS2_PLACEMENT_3D('',#211332,#119769,#119770);
#100244=AXIS2_PLACEMENT_3D('',#211335,#119771,#119772);
#100245=AXIS2_PLACEMENT_3D('',#211337,#119773,#119774);
#100246=AXIS2_PLACEMENT_3D('',#211339,#119775,#119776);
#100247=AXIS2_PLACEMENT_3D('',#211340,#119777,#119778);
#100248=AXIS2_PLACEMENT_3D('',#211341,#119779,#119780);
#100249=AXIS2_PLACEMENT_3D('',#211344,#119781,#119782);
#100250=AXIS2_PLACEMENT_3D('',#211347,#119785,#119786);
#100251=AXIS2_PLACEMENT_3D('',#211350,#119787,#119788);
#100252=AXIS2_PLACEMENT_3D('',#211353,#119791,#119792);
#100253=AXIS2_PLACEMENT_3D('',#211356,#119793,#119794);
#100254=AXIS2_PLACEMENT_3D('',#211357,#119795,#119796);
#100255=AXIS2_PLACEMENT_3D('',#211358,#119797,#119798);
#100256=AXIS2_PLACEMENT_3D('',#211359,#119799,#119800);
#100257=AXIS2_PLACEMENT_3D('',#211362,#119801,#119802);
#100258=AXIS2_PLACEMENT_3D('',#211363,#119803,#119804);
#100259=AXIS2_PLACEMENT_3D('',#211364,#119805,#119806);
#100260=AXIS2_PLACEMENT_3D('',#211365,#119807,#119808);
#100261=AXIS2_PLACEMENT_3D('',#211368,#119809,#119810);
#100262=AXIS2_PLACEMENT_3D('',#211371,#119813,#119814);
#100263=AXIS2_PLACEMENT_3D('',#211374,#119815,#119816);
#100264=AXIS2_PLACEMENT_3D('',#211377,#119819,#119820);
#100265=AXIS2_PLACEMENT_3D('',#211378,#119821,#119822);
#100266=AXIS2_PLACEMENT_3D('',#211379,#119823,#119824);
#100267=AXIS2_PLACEMENT_3D('',#211380,#119825,#119826);
#100268=AXIS2_PLACEMENT_3D('',#211383,#119827,#119828);
#100269=AXIS2_PLACEMENT_3D('',#211385,#119829,#119830);
#100270=AXIS2_PLACEMENT_3D('',#211387,#119831,#119832);
#100271=AXIS2_PLACEMENT_3D('',#211388,#119833,#119834);
#100272=AXIS2_PLACEMENT_3D('',#211389,#119835,#119836);
#100273=AXIS2_PLACEMENT_3D('',#211392,#119837,#119838);
#100274=AXIS2_PLACEMENT_3D('',#211395,#119841,#119842);
#100275=AXIS2_PLACEMENT_3D('',#211398,#119843,#119844);
#100276=AXIS2_PLACEMENT_3D('',#211401,#119847,#119848);
#100277=AXIS2_PLACEMENT_3D('',#211404,#119849,#119850);
#100278=AXIS2_PLACEMENT_3D('',#211405,#119851,#119852);
#100279=AXIS2_PLACEMENT_3D('',#211406,#119853,#119854);
#100280=AXIS2_PLACEMENT_3D('',#211407,#119855,#119856);
#100281=AXIS2_PLACEMENT_3D('',#211410,#119857,#119858);
#100282=AXIS2_PLACEMENT_3D('',#211411,#119859,#119860);
#100283=AXIS2_PLACEMENT_3D('',#211412,#119861,#119862);
#100284=AXIS2_PLACEMENT_3D('',#211413,#119863,#119864);
#100285=AXIS2_PLACEMENT_3D('',#211416,#119865,#119866);
#100286=AXIS2_PLACEMENT_3D('',#211419,#119869,#119870);
#100287=AXIS2_PLACEMENT_3D('',#211422,#119871,#119872);
#100288=AXIS2_PLACEMENT_3D('',#211425,#119875,#119876);
#100289=AXIS2_PLACEMENT_3D('',#211426,#119877,#119878);
#100290=AXIS2_PLACEMENT_3D('',#211427,#119879,#119880);
#100291=AXIS2_PLACEMENT_3D('',#211428,#119881,#119882);
#100292=AXIS2_PLACEMENT_3D('',#211431,#119883,#119884);
#100293=AXIS2_PLACEMENT_3D('',#211433,#119885,#119886);
#100294=AXIS2_PLACEMENT_3D('',#211435,#119887,#119888);
#100295=AXIS2_PLACEMENT_3D('',#211436,#119889,#119890);
#100296=AXIS2_PLACEMENT_3D('',#211437,#119891,#119892);
#100297=AXIS2_PLACEMENT_3D('',#211440,#119893,#119894);
#100298=AXIS2_PLACEMENT_3D('',#211443,#119897,#119898);
#100299=AXIS2_PLACEMENT_3D('',#211446,#119899,#119900);
#100300=AXIS2_PLACEMENT_3D('',#211449,#119903,#119904);
#100301=AXIS2_PLACEMENT_3D('',#211452,#119905,#119906);
#100302=AXIS2_PLACEMENT_3D('',#211453,#119907,#119908);
#100303=AXIS2_PLACEMENT_3D('',#211454,#119909,#119910);
#100304=AXIS2_PLACEMENT_3D('',#211455,#119911,#119912);
#100305=AXIS2_PLACEMENT_3D('',#211458,#119913,#119914);
#100306=AXIS2_PLACEMENT_3D('',#211459,#119915,#119916);
#100307=AXIS2_PLACEMENT_3D('',#211460,#119917,#119918);
#100308=AXIS2_PLACEMENT_3D('',#211461,#119919,#119920);
#100309=AXIS2_PLACEMENT_3D('',#211464,#119921,#119922);
#100310=AXIS2_PLACEMENT_3D('',#211467,#119925,#119926);
#100311=AXIS2_PLACEMENT_3D('',#211470,#119927,#119928);
#100312=AXIS2_PLACEMENT_3D('',#211473,#119931,#119932);
#100313=AXIS2_PLACEMENT_3D('',#211474,#119933,#119934);
#100314=AXIS2_PLACEMENT_3D('',#211475,#119935,#119936);
#100315=AXIS2_PLACEMENT_3D('',#211476,#119937,#119938);
#100316=AXIS2_PLACEMENT_3D('',#211479,#119939,#119940);
#100317=AXIS2_PLACEMENT_3D('',#211481,#119941,#119942);
#100318=AXIS2_PLACEMENT_3D('',#211483,#119943,#119944);
#100319=AXIS2_PLACEMENT_3D('',#211484,#119945,#119946);
#100320=AXIS2_PLACEMENT_3D('',#211485,#119947,#119948);
#100321=AXIS2_PLACEMENT_3D('',#211488,#119949,#119950);
#100322=AXIS2_PLACEMENT_3D('',#211491,#119953,#119954);
#100323=AXIS2_PLACEMENT_3D('',#211494,#119955,#119956);
#100324=AXIS2_PLACEMENT_3D('',#211497,#119959,#119960);
#100325=AXIS2_PLACEMENT_3D('',#211500,#119961,#119962);
#100326=AXIS2_PLACEMENT_3D('',#211501,#119963,#119964);
#100327=AXIS2_PLACEMENT_3D('',#211502,#119965,#119966);
#100328=AXIS2_PLACEMENT_3D('',#211503,#119967,#119968);
#100329=AXIS2_PLACEMENT_3D('',#211506,#119969,#119970);
#100330=AXIS2_PLACEMENT_3D('',#211507,#119971,#119972);
#100331=AXIS2_PLACEMENT_3D('',#211508,#119973,#119974);
#100332=AXIS2_PLACEMENT_3D('',#211509,#119975,#119976);
#100333=AXIS2_PLACEMENT_3D('',#211512,#119977,#119978);
#100334=AXIS2_PLACEMENT_3D('',#211515,#119981,#119982);
#100335=AXIS2_PLACEMENT_3D('',#211518,#119983,#119984);
#100336=AXIS2_PLACEMENT_3D('',#211519,#119985,#119986);
#100337=AXIS2_PLACEMENT_3D('',#211520,#119987,#119988);
#100338=AXIS2_PLACEMENT_3D('',#211521,#119989,#119990);
#100339=AXIS2_PLACEMENT_3D('',#211522,#119991,#119992);
#100340=AXIS2_PLACEMENT_3D('',#211523,#119993,#119994);
#100341=AXIS2_PLACEMENT_3D('',#211524,#119995,#119996);
#100342=AXIS2_PLACEMENT_3D('',#211527,#119997,#119998);
#100343=AXIS2_PLACEMENT_3D('',#211529,#119999,#120000);
#100344=AXIS2_PLACEMENT_3D('',#211531,#120001,#120002);
#100345=AXIS2_PLACEMENT_3D('',#211532,#120003,#120004);
#100346=AXIS2_PLACEMENT_3D('',#211533,#120005,#120006);
#100347=AXIS2_PLACEMENT_3D('',#211536,#120007,#120008);
#100348=AXIS2_PLACEMENT_3D('',#211539,#120011,#120012);
#100349=AXIS2_PLACEMENT_3D('',#211542,#120013,#120014);
#100350=AXIS2_PLACEMENT_3D('',#211545,#120017,#120018);
#100351=AXIS2_PLACEMENT_3D('',#211548,#120019,#120020);
#100352=AXIS2_PLACEMENT_3D('',#211549,#120021,#120022);
#100353=AXIS2_PLACEMENT_3D('',#211550,#120023,#120024);
#100354=AXIS2_PLACEMENT_3D('',#211551,#120025,#120026);
#100355=AXIS2_PLACEMENT_3D('',#211554,#120027,#120028);
#100356=AXIS2_PLACEMENT_3D('',#211555,#120029,#120030);
#100357=AXIS2_PLACEMENT_3D('',#211556,#120031,#120032);
#100358=AXIS2_PLACEMENT_3D('',#211557,#120033,#120034);
#100359=AXIS2_PLACEMENT_3D('',#211560,#120035,#120036);
#100360=AXIS2_PLACEMENT_3D('',#211563,#120039,#120040);
#100361=AXIS2_PLACEMENT_3D('',#211566,#120041,#120042);
#100362=AXIS2_PLACEMENT_3D('',#211567,#120043,#120044);
#100363=AXIS2_PLACEMENT_3D('',#211568,#120045,#120046);
#100364=AXIS2_PLACEMENT_3D('',#211569,#120047,#120048);
#100365=AXIS2_PLACEMENT_3D('',#211572,#120049,#120050);
#100366=AXIS2_PLACEMENT_3D('',#211573,#120051,#120052);
#100367=AXIS2_PLACEMENT_3D('',#211574,#120053,#120054);
#100368=AXIS2_PLACEMENT_3D('',#211575,#120055,#120056);
#100369=AXIS2_PLACEMENT_3D('',#211578,#120057,#120058);
#100370=AXIS2_PLACEMENT_3D('',#211579,#120059,#120060);
#100371=AXIS2_PLACEMENT_3D('',#211580,#120061,#120062);
#100372=AXIS2_PLACEMENT_3D('',#211581,#120063,#120064);
#100373=AXIS2_PLACEMENT_3D('',#211582,#120065,#120066);
#100374=AXIS2_PLACEMENT_3D('',#211583,#120067,#120068);
#100375=AXIS2_PLACEMENT_3D('',#211584,#120069,#120070);
#100376=AXIS2_PLACEMENT_3D('',#211587,#120071,#120072);
#100377=AXIS2_PLACEMENT_3D('',#211589,#120073,#120074);
#100378=AXIS2_PLACEMENT_3D('',#211591,#120075,#120076);
#100379=AXIS2_PLACEMENT_3D('',#211592,#120077,#120078);
#100380=AXIS2_PLACEMENT_3D('',#211593,#120079,#120080);
#100381=AXIS2_PLACEMENT_3D('',#211596,#120081,#120082);
#100382=AXIS2_PLACEMENT_3D('',#211599,#120085,#120086);
#100383=AXIS2_PLACEMENT_3D('',#211602,#120087,#120088);
#100384=AXIS2_PLACEMENT_3D('',#211605,#120091,#120092);
#100385=AXIS2_PLACEMENT_3D('',#211608,#120093,#120094);
#100386=AXIS2_PLACEMENT_3D('',#211609,#120095,#120096);
#100387=AXIS2_PLACEMENT_3D('',#211610,#120097,#120098);
#100388=AXIS2_PLACEMENT_3D('',#211611,#120099,#120100);
#100389=AXIS2_PLACEMENT_3D('',#211614,#120101,#120102);
#100390=AXIS2_PLACEMENT_3D('',#211615,#120103,#120104);
#100391=AXIS2_PLACEMENT_3D('',#211616,#120105,#120106);
#100392=AXIS2_PLACEMENT_3D('',#211617,#120107,#120108);
#100393=AXIS2_PLACEMENT_3D('',#211620,#120109,#120110);
#100394=AXIS2_PLACEMENT_3D('',#211623,#120113,#120114);
#100395=AXIS2_PLACEMENT_3D('',#211626,#120115,#120116);
#100396=AXIS2_PLACEMENT_3D('',#211627,#120117,#120118);
#100397=AXIS2_PLACEMENT_3D('',#211628,#120119,#120120);
#100398=AXIS2_PLACEMENT_3D('',#211629,#120121,#120122);
#100399=AXIS2_PLACEMENT_3D('',#211630,#120123,#120124);
#100400=AXIS2_PLACEMENT_3D('',#211631,#120125,#120126);
#100401=AXIS2_PLACEMENT_3D('',#211632,#120127,#120128);
#100402=AXIS2_PLACEMENT_3D('',#211635,#120129,#120130);
#100403=AXIS2_PLACEMENT_3D('',#211637,#120131,#120132);
#100404=AXIS2_PLACEMENT_3D('',#211639,#120133,#120134);
#100405=AXIS2_PLACEMENT_3D('',#211640,#120135,#120136);
#100406=AXIS2_PLACEMENT_3D('',#211641,#120137,#120138);
#100407=AXIS2_PLACEMENT_3D('',#211644,#120139,#120140);
#100408=AXIS2_PLACEMENT_3D('',#211647,#120143,#120144);
#100409=AXIS2_PLACEMENT_3D('',#211650,#120145,#120146);
#100410=AXIS2_PLACEMENT_3D('',#211653,#120149,#120150);
#100411=AXIS2_PLACEMENT_3D('',#211656,#120151,#120152);
#100412=AXIS2_PLACEMENT_3D('',#211657,#120153,#120154);
#100413=AXIS2_PLACEMENT_3D('',#211658,#120155,#120156);
#100414=AXIS2_PLACEMENT_3D('',#211659,#120157,#120158);
#100415=AXIS2_PLACEMENT_3D('',#211662,#120159,#120160);
#100416=AXIS2_PLACEMENT_3D('',#211663,#120161,#120162);
#100417=AXIS2_PLACEMENT_3D('',#211664,#120163,#120164);
#100418=AXIS2_PLACEMENT_3D('',#211665,#120165,#120166);
#100419=AXIS2_PLACEMENT_3D('',#211668,#120167,#120168);
#100420=AXIS2_PLACEMENT_3D('',#211671,#120171,#120172);
#100421=AXIS2_PLACEMENT_3D('',#211674,#120173,#120174);
#100422=AXIS2_PLACEMENT_3D('',#211677,#120177,#120178);
#100423=AXIS2_PLACEMENT_3D('',#211678,#120179,#120180);
#100424=AXIS2_PLACEMENT_3D('',#211679,#120181,#120182);
#100425=AXIS2_PLACEMENT_3D('',#211680,#120183,#120184);
#100426=AXIS2_PLACEMENT_3D('',#211683,#120185,#120186);
#100427=AXIS2_PLACEMENT_3D('',#211685,#120187,#120188);
#100428=AXIS2_PLACEMENT_3D('',#211687,#120189,#120190);
#100429=AXIS2_PLACEMENT_3D('',#211688,#120191,#120192);
#100430=AXIS2_PLACEMENT_3D('',#211689,#120193,#120194);
#100431=AXIS2_PLACEMENT_3D('',#211692,#120195,#120196);
#100432=AXIS2_PLACEMENT_3D('',#211695,#120199,#120200);
#100433=AXIS2_PLACEMENT_3D('',#211698,#120201,#120202);
#100434=AXIS2_PLACEMENT_3D('',#211699,#120203,#120204);
#100435=AXIS2_PLACEMENT_3D('',#211700,#120205,#120206);
#100436=AXIS2_PLACEMENT_3D('',#211701,#120207,#120208);
#100437=AXIS2_PLACEMENT_3D('',#211704,#120209,#120210);
#100438=AXIS2_PLACEMENT_3D('',#211705,#120211,#120212);
#100439=AXIS2_PLACEMENT_3D('',#211706,#120213,#120214);
#100440=AXIS2_PLACEMENT_3D('',#211707,#120215,#120216);
#100441=AXIS2_PLACEMENT_3D('',#211710,#120217,#120218);
#100442=AXIS2_PLACEMENT_3D('',#211711,#120219,#120220);
#100443=AXIS2_PLACEMENT_3D('',#211712,#120221,#120222);
#100444=AXIS2_PLACEMENT_3D('',#211713,#120223,#120224);
#100445=AXIS2_PLACEMENT_3D('',#211716,#120225,#120226);
#100446=AXIS2_PLACEMENT_3D('',#211719,#120229,#120230);
#100447=AXIS2_PLACEMENT_3D('',#211722,#120231,#120232);
#100448=AXIS2_PLACEMENT_3D('',#211725,#120235,#120236);
#100449=AXIS2_PLACEMENT_3D('',#211728,#120237,#120238);
#100450=AXIS2_PLACEMENT_3D('',#211729,#120239,#120240);
#100451=AXIS2_PLACEMENT_3D('',#211730,#120241,#120242);
#100452=AXIS2_PLACEMENT_3D('',#211731,#120243,#120244);
#100453=AXIS2_PLACEMENT_3D('',#211734,#120245,#120246);
#100454=AXIS2_PLACEMENT_3D('',#211735,#120247,#120248);
#100455=AXIS2_PLACEMENT_3D('',#211736,#120249,#120250);
#100456=AXIS2_PLACEMENT_3D('',#211737,#120251,#120252);
#100457=AXIS2_PLACEMENT_3D('',#211740,#120255,#120256);
#100458=AXIS2_PLACEMENT_3D('',#211743,#120257,#120258);
#100459=AXIS2_PLACEMENT_3D('',#211745,#120259,#120260);
#100460=AXIS2_PLACEMENT_3D('',#211747,#120261,#120262);
#100461=AXIS2_PLACEMENT_3D('',#211748,#120263,#120264);
#100462=AXIS2_PLACEMENT_3D('',#211749,#120265,#120266);
#100463=AXIS2_PLACEMENT_3D('',#211752,#120267,#120268);
#100464=AXIS2_PLACEMENT_3D('',#211755,#120271,#120272);
#100465=AXIS2_PLACEMENT_3D('',#211758,#120273,#120274);
#100466=AXIS2_PLACEMENT_3D('',#211761,#120277,#120278);
#100467=AXIS2_PLACEMENT_3D('',#211764,#120279,#120280);
#100468=AXIS2_PLACEMENT_3D('',#211765,#120281,#120282);
#100469=AXIS2_PLACEMENT_3D('',#211766,#120283,#120284);
#100470=AXIS2_PLACEMENT_3D('',#211767,#120285,#120286);
#100471=AXIS2_PLACEMENT_3D('',#211770,#120287,#120288);
#100472=AXIS2_PLACEMENT_3D('',#211771,#120289,#120290);
#100473=AXIS2_PLACEMENT_3D('',#211772,#120291,#120292);
#100474=AXIS2_PLACEMENT_3D('',#211773,#120293,#120294);
#100475=AXIS2_PLACEMENT_3D('',#211776,#120295,#120296);
#100476=AXIS2_PLACEMENT_3D('',#211779,#120299,#120300);
#100477=AXIS2_PLACEMENT_3D('',#211782,#120301,#120302);
#100478=AXIS2_PLACEMENT_3D('',#211783,#120303,#120304);
#100479=AXIS2_PLACEMENT_3D('',#211784,#120305,#120306);
#100480=AXIS2_PLACEMENT_3D('',#211785,#120307,#120308);
#100481=AXIS2_PLACEMENT_3D('',#211788,#120309,#120310);
#100482=AXIS2_PLACEMENT_3D('',#211789,#120311,#120312);
#100483=AXIS2_PLACEMENT_3D('',#211790,#120313,#120314);
#100484=AXIS2_PLACEMENT_3D('',#211791,#120315,#120316);
#100485=AXIS2_PLACEMENT_3D('',#211794,#120317,#120318);
#100486=AXIS2_PLACEMENT_3D('',#211795,#120319,#120320);
#100487=AXIS2_PLACEMENT_3D('',#211796,#120321,#120322);
#100488=AXIS2_PLACEMENT_3D('',#211797,#120323,#120324);
#100489=AXIS2_PLACEMENT_3D('',#211800,#120327,#120328);
#100490=AXIS2_PLACEMENT_3D('',#211803,#120329,#120330);
#100491=AXIS2_PLACEMENT_3D('',#211805,#120331,#120332);
#100492=AXIS2_PLACEMENT_3D('',#211807,#120333,#120334);
#100493=AXIS2_PLACEMENT_3D('',#211808,#120335,#120336);
#100494=AXIS2_PLACEMENT_3D('',#211809,#120337,#120338);
#100495=AXIS2_PLACEMENT_3D('',#211812,#120339,#120340);
#100496=AXIS2_PLACEMENT_3D('',#211815,#120343,#120344);
#100497=AXIS2_PLACEMENT_3D('',#211818,#120345,#120346);
#100498=AXIS2_PLACEMENT_3D('',#211821,#120349,#120350);
#100499=AXIS2_PLACEMENT_3D('',#211824,#120351,#120352);
#100500=AXIS2_PLACEMENT_3D('',#211825,#120353,#120354);
#100501=AXIS2_PLACEMENT_3D('',#211826,#120355,#120356);
#100502=AXIS2_PLACEMENT_3D('',#211827,#120357,#120358);
#100503=AXIS2_PLACEMENT_3D('',#211830,#120359,#120360);
#100504=AXIS2_PLACEMENT_3D('',#211831,#120361,#120362);
#100505=AXIS2_PLACEMENT_3D('',#211832,#120363,#120364);
#100506=AXIS2_PLACEMENT_3D('',#211833,#120365,#120366);
#100507=AXIS2_PLACEMENT_3D('',#211836,#120367,#120368);
#100508=AXIS2_PLACEMENT_3D('',#211839,#120371,#120372);
#100509=AXIS2_PLACEMENT_3D('',#211842,#120373,#120374);
#100510=AXIS2_PLACEMENT_3D('',#211845,#120377,#120378);
#100511=AXIS2_PLACEMENT_3D('',#211846,#120379,#120380);
#100512=AXIS2_PLACEMENT_3D('',#211847,#120381,#120382);
#100513=AXIS2_PLACEMENT_3D('',#211848,#120383,#120384);
#100514=AXIS2_PLACEMENT_3D('',#211851,#120385,#120386);
#100515=AXIS2_PLACEMENT_3D('',#211853,#120387,#120388);
#100516=AXIS2_PLACEMENT_3D('',#211855,#120389,#120390);
#100517=AXIS2_PLACEMENT_3D('',#211856,#120391,#120392);
#100518=AXIS2_PLACEMENT_3D('',#211857,#120393,#120394);
#100519=AXIS2_PLACEMENT_3D('',#211860,#120395,#120396);
#100520=AXIS2_PLACEMENT_3D('',#211863,#120399,#120400);
#100521=AXIS2_PLACEMENT_3D('',#211866,#120401,#120402);
#100522=AXIS2_PLACEMENT_3D('',#211869,#120405,#120406);
#100523=AXIS2_PLACEMENT_3D('',#211872,#120407,#120408);
#100524=AXIS2_PLACEMENT_3D('',#211873,#120409,#120410);
#100525=AXIS2_PLACEMENT_3D('',#211874,#120411,#120412);
#100526=AXIS2_PLACEMENT_3D('',#211875,#120413,#120414);
#100527=AXIS2_PLACEMENT_3D('',#211878,#120415,#120416);
#100528=AXIS2_PLACEMENT_3D('',#211879,#120417,#120418);
#100529=AXIS2_PLACEMENT_3D('',#211880,#120419,#120420);
#100530=AXIS2_PLACEMENT_3D('',#211881,#120421,#120422);
#100531=AXIS2_PLACEMENT_3D('',#211884,#120423,#120424);
#100532=AXIS2_PLACEMENT_3D('',#211885,#120425,#120426);
#100533=AXIS2_PLACEMENT_3D('',#211886,#120427,#120428);
#100534=AXIS2_PLACEMENT_3D('',#211887,#120429,#120430);
#100535=AXIS2_PLACEMENT_3D('',#211890,#120431,#120432);
#100536=AXIS2_PLACEMENT_3D('',#211893,#120435,#120436);
#100537=AXIS2_PLACEMENT_3D('',#211894,#120437,#120438);
#100538=AXIS2_PLACEMENT_3D('',#211895,#120439,#120440);
#100539=AXIS2_PLACEMENT_3D('',#211896,#120441,#120442);
#100540=AXIS2_PLACEMENT_3D('',#211899,#120443,#120444);
#100541=AXIS2_PLACEMENT_3D('',#211901,#120445,#120446);
#100542=AXIS2_PLACEMENT_3D('',#211903,#120447,#120448);
#100543=AXIS2_PLACEMENT_3D('',#211904,#120449,#120450);
#100544=AXIS2_PLACEMENT_3D('',#211905,#120451,#120452);
#100545=AXIS2_PLACEMENT_3D('',#211908,#120453,#120454);
#100546=AXIS2_PLACEMENT_3D('',#211911,#120457,#120458);
#100547=AXIS2_PLACEMENT_3D('',#211914,#120459,#120460);
#100548=AXIS2_PLACEMENT_3D('',#211917,#120463,#120464);
#100549=AXIS2_PLACEMENT_3D('',#211920,#120465,#120466);
#100550=AXIS2_PLACEMENT_3D('',#211921,#120467,#120468);
#100551=AXIS2_PLACEMENT_3D('',#211922,#120469,#120470);
#100552=AXIS2_PLACEMENT_3D('',#211923,#120471,#120472);
#100553=AXIS2_PLACEMENT_3D('',#211926,#120473,#120474);
#100554=AXIS2_PLACEMENT_3D('',#211927,#120475,#120476);
#100555=AXIS2_PLACEMENT_3D('',#211928,#120477,#120478);
#100556=AXIS2_PLACEMENT_3D('',#211929,#120479,#120480);
#100557=AXIS2_PLACEMENT_3D('',#211932,#120481,#120482);
#100558=AXIS2_PLACEMENT_3D('',#211935,#120485,#120486);
#100559=AXIS2_PLACEMENT_3D('',#211938,#120487,#120488);
#100560=AXIS2_PLACEMENT_3D('',#211941,#120491,#120492);
#100561=AXIS2_PLACEMENT_3D('',#211942,#120493,#120494);
#100562=AXIS2_PLACEMENT_3D('',#211943,#120495,#120496);
#100563=AXIS2_PLACEMENT_3D('',#211944,#120497,#120498);
#100564=AXIS2_PLACEMENT_3D('',#211947,#120499,#120500);
#100565=AXIS2_PLACEMENT_3D('',#211949,#120501,#120502);
#100566=AXIS2_PLACEMENT_3D('',#211951,#120503,#120504);
#100567=AXIS2_PLACEMENT_3D('',#211952,#120505,#120506);
#100568=AXIS2_PLACEMENT_3D('',#211953,#120507,#120508);
#100569=AXIS2_PLACEMENT_3D('',#211956,#120509,#120510);
#100570=AXIS2_PLACEMENT_3D('',#211959,#120513,#120514);
#100571=AXIS2_PLACEMENT_3D('',#211962,#120515,#120516);
#100572=AXIS2_PLACEMENT_3D('',#211965,#120519,#120520);
#100573=AXIS2_PLACEMENT_3D('',#211968,#120521,#120522);
#100574=AXIS2_PLACEMENT_3D('',#211969,#120523,#120524);
#100575=AXIS2_PLACEMENT_3D('',#211970,#120525,#120526);
#100576=AXIS2_PLACEMENT_3D('',#211971,#120527,#120528);
#100577=AXIS2_PLACEMENT_3D('',#211974,#120529,#120530);
#100578=AXIS2_PLACEMENT_3D('',#211975,#120531,#120532);
#100579=AXIS2_PLACEMENT_3D('',#211976,#120533,#120534);
#100580=AXIS2_PLACEMENT_3D('',#211977,#120535,#120536);
#100581=AXIS2_PLACEMENT_3D('',#211980,#120537,#120538);
#100582=AXIS2_PLACEMENT_3D('',#211983,#120541,#120542);
#100583=AXIS2_PLACEMENT_3D('',#211986,#120543,#120544);
#100584=AXIS2_PLACEMENT_3D('',#211989,#120547,#120548);
#100585=AXIS2_PLACEMENT_3D('',#211990,#120549,#120550);
#100586=AXIS2_PLACEMENT_3D('',#211991,#120551,#120552);
#100587=AXIS2_PLACEMENT_3D('',#211992,#120553,#120554);
#100588=AXIS2_PLACEMENT_3D('',#211995,#120555,#120556);
#100589=AXIS2_PLACEMENT_3D('',#211997,#120557,#120558);
#100590=AXIS2_PLACEMENT_3D('',#211999,#120559,#120560);
#100591=AXIS2_PLACEMENT_3D('',#212000,#120561,#120562);
#100592=AXIS2_PLACEMENT_3D('',#212001,#120563,#120564);
#100593=AXIS2_PLACEMENT_3D('',#212004,#120565,#120566);
#100594=AXIS2_PLACEMENT_3D('',#212007,#120569,#120570);
#100595=AXIS2_PLACEMENT_3D('',#212010,#120571,#120572);
#100596=AXIS2_PLACEMENT_3D('',#212013,#120575,#120576);
#100597=AXIS2_PLACEMENT_3D('',#212016,#120577,#120578);
#100598=AXIS2_PLACEMENT_3D('',#212017,#120579,#120580);
#100599=AXIS2_PLACEMENT_3D('',#212018,#120581,#120582);
#100600=AXIS2_PLACEMENT_3D('',#212019,#120583,#120584);
#100601=AXIS2_PLACEMENT_3D('',#212022,#120585,#120586);
#100602=AXIS2_PLACEMENT_3D('',#212023,#120587,#120588);
#100603=AXIS2_PLACEMENT_3D('',#212024,#120589,#120590);
#100604=AXIS2_PLACEMENT_3D('',#212025,#120591,#120592);
#100605=AXIS2_PLACEMENT_3D('',#212028,#120593,#120594);
#100606=AXIS2_PLACEMENT_3D('',#212031,#120597,#120598);
#100607=AXIS2_PLACEMENT_3D('',#212034,#120599,#120600);
#100608=AXIS2_PLACEMENT_3D('',#212035,#120601,#120602);
#100609=AXIS2_PLACEMENT_3D('',#212036,#120603,#120604);
#100610=AXIS2_PLACEMENT_3D('',#212037,#120605,#120606);
#100611=AXIS2_PLACEMENT_3D('',#212039,#120607,#120608);
#100612=AXIS2_PLACEMENT_3D('',#212041,#120609,#120610);
#100613=AXIS2_PLACEMENT_3D('',#212042,#120611,#120612);
#100614=AXIS2_PLACEMENT_3D('',#212043,#120613,#120614);
#100615=AXIS2_PLACEMENT_3D('',#212044,#120615,#120616);
#100616=AXIS2_PLACEMENT_3D('',#212045,#120617,#120618);
#100617=AXIS2_PLACEMENT_3D('',#212046,#120619,#120620);
#100618=AXIS2_PLACEMENT_3D('',#212049,#120621,#120622);
#100619=AXIS2_PLACEMENT_3D('',#212051,#120623,#120624);
#100620=AXIS2_PLACEMENT_3D('',#212053,#120625,#120626);
#100621=AXIS2_PLACEMENT_3D('',#212054,#120627,#120628);
#100622=AXIS2_PLACEMENT_3D('',#212055,#120629,#120630);
#100623=AXIS2_PLACEMENT_3D('',#212058,#120631,#120632);
#100624=AXIS2_PLACEMENT_3D('',#212061,#120635,#120636);
#100625=AXIS2_PLACEMENT_3D('',#212064,#120637,#120638);
#100626=AXIS2_PLACEMENT_3D('',#212067,#120641,#120642);
#100627=AXIS2_PLACEMENT_3D('',#212070,#120643,#120644);
#100628=AXIS2_PLACEMENT_3D('',#212071,#120645,#120646);
#100629=AXIS2_PLACEMENT_3D('',#212072,#120647,#120648);
#100630=AXIS2_PLACEMENT_3D('',#212073,#120649,#120650);
#100631=AXIS2_PLACEMENT_3D('',#212076,#120651,#120652);
#100632=AXIS2_PLACEMENT_3D('',#212077,#120653,#120654);
#100633=AXIS2_PLACEMENT_3D('',#212078,#120655,#120656);
#100634=AXIS2_PLACEMENT_3D('',#212079,#120657,#120658);
#100635=AXIS2_PLACEMENT_3D('',#212082,#120659,#120660);
#100636=AXIS2_PLACEMENT_3D('',#212083,#120661,#120662);
#100637=AXIS2_PLACEMENT_3D('',#212084,#120663,#120664);
#100638=AXIS2_PLACEMENT_3D('',#212085,#120665,#120666);
#100639=AXIS2_PLACEMENT_3D('',#212088,#120667,#120668);
#100640=AXIS2_PLACEMENT_3D('',#212091,#120671,#120672);
#100641=AXIS2_PLACEMENT_3D('',#212092,#120673,#120674);
#100642=AXIS2_PLACEMENT_3D('',#212093,#120675,#120676);
#100643=AXIS2_PLACEMENT_3D('',#212094,#120677,#120678);
#100644=AXIS2_PLACEMENT_3D('',#212097,#120679,#120680);
#100645=AXIS2_PLACEMENT_3D('',#212099,#120681,#120682);
#100646=AXIS2_PLACEMENT_3D('',#212101,#120683,#120684);
#100647=AXIS2_PLACEMENT_3D('',#212102,#120685,#120686);
#100648=AXIS2_PLACEMENT_3D('',#212103,#120687,#120688);
#100649=AXIS2_PLACEMENT_3D('',#212106,#120689,#120690);
#100650=AXIS2_PLACEMENT_3D('',#212109,#120693,#120694);
#100651=AXIS2_PLACEMENT_3D('',#212112,#120695,#120696);
#100652=AXIS2_PLACEMENT_3D('',#212115,#120699,#120700);
#100653=AXIS2_PLACEMENT_3D('',#212118,#120701,#120702);
#100654=AXIS2_PLACEMENT_3D('',#212119,#120703,#120704);
#100655=AXIS2_PLACEMENT_3D('',#212120,#120705,#120706);
#100656=AXIS2_PLACEMENT_3D('',#212121,#120707,#120708);
#100657=AXIS2_PLACEMENT_3D('',#212124,#120709,#120710);
#100658=AXIS2_PLACEMENT_3D('',#212125,#120711,#120712);
#100659=AXIS2_PLACEMENT_3D('',#212126,#120713,#120714);
#100660=AXIS2_PLACEMENT_3D('',#212127,#120715,#120716);
#100661=AXIS2_PLACEMENT_3D('',#212130,#120717,#120718);
#100662=AXIS2_PLACEMENT_3D('',#212131,#120719,#120720);
#100663=AXIS2_PLACEMENT_3D('',#212132,#120721,#120722);
#100664=AXIS2_PLACEMENT_3D('',#212133,#120723,#120724);
#100665=AXIS2_PLACEMENT_3D('',#212136,#120725,#120726);
#100666=AXIS2_PLACEMENT_3D('',#212139,#120729,#120730);
#100667=AXIS2_PLACEMENT_3D('',#212142,#120731,#120732);
#100668=AXIS2_PLACEMENT_3D('',#212143,#120733,#120734);
#100669=AXIS2_PLACEMENT_3D('',#212144,#120735,#120736);
#100670=AXIS2_PLACEMENT_3D('',#212145,#120737,#120738);
#100671=AXIS2_PLACEMENT_3D('',#212148,#120739,#120740);
#100672=AXIS2_PLACEMENT_3D('',#212149,#120741,#120742);
#100673=AXIS2_PLACEMENT_3D('',#212150,#120743,#120744);
#100674=AXIS2_PLACEMENT_3D('',#212151,#120745,#120746);
#100675=AXIS2_PLACEMENT_3D('',#212152,#120747,#120748);
#100676=AXIS2_PLACEMENT_3D('',#212153,#120749,#120750);
#100677=AXIS2_PLACEMENT_3D('',#212154,#120751,#120752);
#100678=AXIS2_PLACEMENT_3D('',#212157,#120753,#120754);
#100679=AXIS2_PLACEMENT_3D('',#212159,#120755,#120756);
#100680=AXIS2_PLACEMENT_3D('',#212161,#120757,#120758);
#100681=AXIS2_PLACEMENT_3D('',#212162,#120759,#120760);
#100682=AXIS2_PLACEMENT_3D('',#212163,#120761,#120762);
#100683=AXIS2_PLACEMENT_3D('',#212166,#120763,#120764);
#100684=AXIS2_PLACEMENT_3D('',#212169,#120767,#120768);
#100685=AXIS2_PLACEMENT_3D('',#212172,#120769,#120770);
#100686=AXIS2_PLACEMENT_3D('',#212175,#120773,#120774);
#100687=AXIS2_PLACEMENT_3D('',#212178,#120775,#120776);
#100688=AXIS2_PLACEMENT_3D('',#212179,#120777,#120778);
#100689=AXIS2_PLACEMENT_3D('',#212180,#120779,#120780);
#100690=AXIS2_PLACEMENT_3D('',#212181,#120781,#120782);
#100691=AXIS2_PLACEMENT_3D('',#212184,#120783,#120784);
#100692=AXIS2_PLACEMENT_3D('',#212185,#120785,#120786);
#100693=AXIS2_PLACEMENT_3D('',#212186,#120787,#120788);
#100694=AXIS2_PLACEMENT_3D('',#212187,#120789,#120790);
#100695=AXIS2_PLACEMENT_3D('',#212190,#120791,#120792);
#100696=AXIS2_PLACEMENT_3D('',#212193,#120795,#120796);
#100697=AXIS2_PLACEMENT_3D('',#212196,#120797,#120798);
#100698=AXIS2_PLACEMENT_3D('',#212199,#120801,#120802);
#100699=AXIS2_PLACEMENT_3D('',#212200,#120803,#120804);
#100700=AXIS2_PLACEMENT_3D('',#212201,#120805,#120806);
#100701=AXIS2_PLACEMENT_3D('',#212202,#120807,#120808);
#100702=AXIS2_PLACEMENT_3D('',#212205,#120809,#120810);
#100703=AXIS2_PLACEMENT_3D('',#212207,#120811,#120812);
#100704=AXIS2_PLACEMENT_3D('',#212209,#120813,#120814);
#100705=AXIS2_PLACEMENT_3D('',#212210,#120815,#120816);
#100706=AXIS2_PLACEMENT_3D('',#212211,#120817,#120818);
#100707=AXIS2_PLACEMENT_3D('',#212214,#120819,#120820);
#100708=AXIS2_PLACEMENT_3D('',#212217,#120823,#120824);
#100709=AXIS2_PLACEMENT_3D('',#212220,#120825,#120826);
#100710=AXIS2_PLACEMENT_3D('',#212223,#120829,#120830);
#100711=AXIS2_PLACEMENT_3D('',#212226,#120831,#120832);
#100712=AXIS2_PLACEMENT_3D('',#212227,#120833,#120834);
#100713=AXIS2_PLACEMENT_3D('',#212228,#120835,#120836);
#100714=AXIS2_PLACEMENT_3D('',#212229,#120837,#120838);
#100715=AXIS2_PLACEMENT_3D('',#212232,#120839,#120840);
#100716=AXIS2_PLACEMENT_3D('',#212233,#120841,#120842);
#100717=AXIS2_PLACEMENT_3D('',#212234,#120843,#120844);
#100718=AXIS2_PLACEMENT_3D('',#212235,#120845,#120846);
#100719=AXIS2_PLACEMENT_3D('',#212238,#120847,#120848);
#100720=AXIS2_PLACEMENT_3D('',#212241,#120851,#120852);
#100721=AXIS2_PLACEMENT_3D('',#212244,#120853,#120854);
#100722=AXIS2_PLACEMENT_3D('',#212245,#120855,#120856);
#100723=AXIS2_PLACEMENT_3D('',#212246,#120857,#120858);
#100724=AXIS2_PLACEMENT_3D('',#212247,#120859,#120860);
#100725=AXIS2_PLACEMENT_3D('',#212250,#120861,#120862);
#100726=AXIS2_PLACEMENT_3D('',#212251,#120863,#120864);
#100727=AXIS2_PLACEMENT_3D('',#212252,#120865,#120866);
#100728=AXIS2_PLACEMENT_3D('',#212253,#120867,#120868);
#100729=AXIS2_PLACEMENT_3D('',#212256,#120869,#120870);
#100730=AXIS2_PLACEMENT_3D('',#212257,#120871,#120872);
#100731=AXIS2_PLACEMENT_3D('',#212258,#120873,#120874);
#100732=AXIS2_PLACEMENT_3D('',#212259,#120875,#120876);
#100733=AXIS2_PLACEMENT_3D('',#212260,#120877,#120878);
#100734=AXIS2_PLACEMENT_3D('',#212261,#120879,#120880);
#100735=AXIS2_PLACEMENT_3D('',#212262,#120881,#120882);
#100736=AXIS2_PLACEMENT_3D('',#212265,#120883,#120884);
#100737=AXIS2_PLACEMENT_3D('',#212267,#120885,#120886);
#100738=AXIS2_PLACEMENT_3D('',#212269,#120887,#120888);
#100739=AXIS2_PLACEMENT_3D('',#212270,#120889,#120890);
#100740=AXIS2_PLACEMENT_3D('',#212271,#120891,#120892);
#100741=AXIS2_PLACEMENT_3D('',#212274,#120893,#120894);
#100742=AXIS2_PLACEMENT_3D('',#212277,#120897,#120898);
#100743=AXIS2_PLACEMENT_3D('',#212280,#120899,#120900);
#100744=AXIS2_PLACEMENT_3D('',#212283,#120903,#120904);
#100745=AXIS2_PLACEMENT_3D('',#212286,#120905,#120906);
#100746=AXIS2_PLACEMENT_3D('',#212287,#120907,#120908);
#100747=AXIS2_PLACEMENT_3D('',#212288,#120909,#120910);
#100748=AXIS2_PLACEMENT_3D('',#212289,#120911,#120912);
#100749=AXIS2_PLACEMENT_3D('',#212292,#120913,#120914);
#100750=AXIS2_PLACEMENT_3D('',#212293,#120915,#120916);
#100751=AXIS2_PLACEMENT_3D('',#212294,#120917,#120918);
#100752=AXIS2_PLACEMENT_3D('',#212295,#120919,#120920);
#100753=AXIS2_PLACEMENT_3D('',#212298,#120921,#120922);
#100754=AXIS2_PLACEMENT_3D('',#212301,#120925,#120926);
#100755=AXIS2_PLACEMENT_3D('',#212304,#120927,#120928);
#100756=AXIS2_PLACEMENT_3D('',#212305,#120929,#120930);
#100757=AXIS2_PLACEMENT_3D('',#212306,#120931,#120932);
#100758=AXIS2_PLACEMENT_3D('',#212307,#120933,#120934);
#100759=AXIS2_PLACEMENT_3D('',#212308,#120935,#120936);
#100760=AXIS2_PLACEMENT_3D('',#212309,#120937,#120938);
#100761=AXIS2_PLACEMENT_3D('',#212310,#120939,#120940);
#100762=AXIS2_PLACEMENT_3D('',#212313,#120941,#120942);
#100763=AXIS2_PLACEMENT_3D('',#212315,#120943,#120944);
#100764=AXIS2_PLACEMENT_3D('',#212317,#120945,#120946);
#100765=AXIS2_PLACEMENT_3D('',#212318,#120947,#120948);
#100766=AXIS2_PLACEMENT_3D('',#212319,#120949,#120950);
#100767=AXIS2_PLACEMENT_3D('',#212322,#120951,#120952);
#100768=AXIS2_PLACEMENT_3D('',#212325,#120955,#120956);
#100769=AXIS2_PLACEMENT_3D('',#212328,#120957,#120958);
#100770=AXIS2_PLACEMENT_3D('',#212331,#120961,#120962);
#100771=AXIS2_PLACEMENT_3D('',#212334,#120963,#120964);
#100772=AXIS2_PLACEMENT_3D('',#212335,#120965,#120966);
#100773=AXIS2_PLACEMENT_3D('',#212336,#120967,#120968);
#100774=AXIS2_PLACEMENT_3D('',#212337,#120969,#120970);
#100775=AXIS2_PLACEMENT_3D('',#212340,#120971,#120972);
#100776=AXIS2_PLACEMENT_3D('',#212341,#120973,#120974);
#100777=AXIS2_PLACEMENT_3D('',#212342,#120975,#120976);
#100778=AXIS2_PLACEMENT_3D('',#212343,#120977,#120978);
#100779=AXIS2_PLACEMENT_3D('',#212346,#120979,#120980);
#100780=AXIS2_PLACEMENT_3D('',#212349,#120983,#120984);
#100781=AXIS2_PLACEMENT_3D('',#212352,#120985,#120986);
#100782=AXIS2_PLACEMENT_3D('',#212355,#120989,#120990);
#100783=AXIS2_PLACEMENT_3D('',#212356,#120991,#120992);
#100784=AXIS2_PLACEMENT_3D('',#212357,#120993,#120994);
#100785=AXIS2_PLACEMENT_3D('',#212358,#120995,#120996);
#100786=AXIS2_PLACEMENT_3D('',#212361,#120997,#120998);
#100787=AXIS2_PLACEMENT_3D('',#212363,#120999,#121000);
#100788=AXIS2_PLACEMENT_3D('',#212365,#121001,#121002);
#100789=AXIS2_PLACEMENT_3D('',#212366,#121003,#121004);
#100790=AXIS2_PLACEMENT_3D('',#212367,#121005,#121006);
#100791=AXIS2_PLACEMENT_3D('',#212370,#121007,#121008);
#100792=AXIS2_PLACEMENT_3D('',#212373,#121011,#121012);
#100793=AXIS2_PLACEMENT_3D('',#212376,#121013,#121014);
#100794=AXIS2_PLACEMENT_3D('',#212379,#121017,#121018);
#100795=AXIS2_PLACEMENT_3D('',#212382,#121019,#121020);
#100796=AXIS2_PLACEMENT_3D('',#212383,#121021,#121022);
#100797=AXIS2_PLACEMENT_3D('',#212384,#121023,#121024);
#100798=AXIS2_PLACEMENT_3D('',#212385,#121025,#121026);
#100799=AXIS2_PLACEMENT_3D('',#212388,#121027,#121028);
#100800=AXIS2_PLACEMENT_3D('',#212389,#121029,#121030);
#100801=AXIS2_PLACEMENT_3D('',#212390,#121031,#121032);
#100802=AXIS2_PLACEMENT_3D('',#212391,#121033,#121034);
#100803=AXIS2_PLACEMENT_3D('',#212394,#121035,#121036);
#100804=AXIS2_PLACEMENT_3D('',#212397,#121039,#121040);
#100805=AXIS2_PLACEMENT_3D('',#212400,#121041,#121042);
#100806=AXIS2_PLACEMENT_3D('',#212401,#121043,#121044);
#100807=AXIS2_PLACEMENT_3D('',#212402,#121045,#121046);
#100808=AXIS2_PLACEMENT_3D('',#212403,#121047,#121048);
#100809=AXIS2_PLACEMENT_3D('',#212404,#121049,#121050);
#100810=AXIS2_PLACEMENT_3D('',#212405,#121051,#121052);
#100811=AXIS2_PLACEMENT_3D('',#212406,#121053,#121054);
#100812=AXIS2_PLACEMENT_3D('',#212409,#121055,#121056);
#100813=AXIS2_PLACEMENT_3D('',#212411,#121057,#121058);
#100814=AXIS2_PLACEMENT_3D('',#212413,#121059,#121060);
#100815=AXIS2_PLACEMENT_3D('',#212414,#121061,#121062);
#100816=AXIS2_PLACEMENT_3D('',#212415,#121063,#121064);
#100817=AXIS2_PLACEMENT_3D('',#212418,#121065,#121066);
#100818=AXIS2_PLACEMENT_3D('',#212421,#121069,#121070);
#100819=AXIS2_PLACEMENT_3D('',#212424,#121071,#121072);
#100820=AXIS2_PLACEMENT_3D('',#212427,#121075,#121076);
#100821=AXIS2_PLACEMENT_3D('',#212430,#121077,#121078);
#100822=AXIS2_PLACEMENT_3D('',#212431,#121079,#121080);
#100823=AXIS2_PLACEMENT_3D('',#212432,#121081,#121082);
#100824=AXIS2_PLACEMENT_3D('',#212433,#121083,#121084);
#100825=AXIS2_PLACEMENT_3D('',#212436,#121085,#121086);
#100826=AXIS2_PLACEMENT_3D('',#212437,#121087,#121088);
#100827=AXIS2_PLACEMENT_3D('',#212438,#121089,#121090);
#100828=AXIS2_PLACEMENT_3D('',#212439,#121091,#121092);
#100829=AXIS2_PLACEMENT_3D('',#212442,#121093,#121094);
#100830=AXIS2_PLACEMENT_3D('',#212445,#121097,#121098);
#100831=AXIS2_PLACEMENT_3D('',#212448,#121099,#121100);
#100832=AXIS2_PLACEMENT_3D('',#212451,#121103,#121104);
#100833=AXIS2_PLACEMENT_3D('',#212452,#121105,#121106);
#100834=AXIS2_PLACEMENT_3D('',#212453,#121107,#121108);
#100835=AXIS2_PLACEMENT_3D('',#212454,#121109,#121110);
#100836=AXIS2_PLACEMENT_3D('',#212457,#121111,#121112);
#100837=AXIS2_PLACEMENT_3D('',#212459,#121113,#121114);
#100838=AXIS2_PLACEMENT_3D('',#212461,#121115,#121116);
#100839=AXIS2_PLACEMENT_3D('',#212462,#121117,#121118);
#100840=AXIS2_PLACEMENT_3D('',#212463,#121119,#121120);
#100841=AXIS2_PLACEMENT_3D('',#212466,#121121,#121122);
#100842=AXIS2_PLACEMENT_3D('',#212469,#121125,#121126);
#100843=AXIS2_PLACEMENT_3D('',#212472,#121127,#121128);
#100844=AXIS2_PLACEMENT_3D('',#212473,#121129,#121130);
#100845=AXIS2_PLACEMENT_3D('',#212474,#121131,#121132);
#100846=AXIS2_PLACEMENT_3D('',#212475,#121133,#121134);
#100847=AXIS2_PLACEMENT_3D('',#212478,#121135,#121136);
#100848=AXIS2_PLACEMENT_3D('',#212479,#121137,#121138);
#100849=AXIS2_PLACEMENT_3D('',#212480,#121139,#121140);
#100850=AXIS2_PLACEMENT_3D('',#212481,#121141,#121142);
#100851=AXIS2_PLACEMENT_3D('',#212484,#121143,#121144);
#100852=AXIS2_PLACEMENT_3D('',#212485,#121145,#121146);
#100853=AXIS2_PLACEMENT_3D('',#212486,#121147,#121148);
#100854=AXIS2_PLACEMENT_3D('',#212487,#121149,#121150);
#100855=AXIS2_PLACEMENT_3D('',#212490,#121153,#121154);
#100856=AXIS2_PLACEMENT_3D('',#212493,#121155,#121156);
#100857=AXIS2_PLACEMENT_3D('',#212495,#121157,#121158);
#100858=AXIS2_PLACEMENT_3D('',#212497,#121159,#121160);
#100859=AXIS2_PLACEMENT_3D('',#212498,#121161,#121162);
#100860=AXIS2_PLACEMENT_3D('',#212499,#121163,#121164);
#100861=AXIS2_PLACEMENT_3D('',#212502,#121165,#121166);
#100862=AXIS2_PLACEMENT_3D('',#212505,#121169,#121170);
#100863=AXIS2_PLACEMENT_3D('',#212508,#121171,#121172);
#100864=AXIS2_PLACEMENT_3D('',#212509,#121173,#121174);
#100865=AXIS2_PLACEMENT_3D('',#212510,#121175,#121176);
#100866=AXIS2_PLACEMENT_3D('',#212511,#121177,#121178);
#100867=AXIS2_PLACEMENT_3D('',#212514,#121179,#121180);
#100868=AXIS2_PLACEMENT_3D('',#212515,#121181,#121182);
#100869=AXIS2_PLACEMENT_3D('',#212516,#121183,#121184);
#100870=AXIS2_PLACEMENT_3D('',#212517,#121185,#121186);
#100871=AXIS2_PLACEMENT_3D('',#212520,#121187,#121188);
#100872=AXIS2_PLACEMENT_3D('',#212521,#121189,#121190);
#100873=AXIS2_PLACEMENT_3D('',#212522,#121191,#121192);
#100874=AXIS2_PLACEMENT_3D('',#212523,#121193,#121194);
#100875=AXIS2_PLACEMENT_3D('',#212526,#121197,#121198);
#100876=AXIS2_PLACEMENT_3D('',#212528,#121199,#121200);
#100877=AXIS2_PLACEMENT_3D('',#212530,#121201,#121202);
#100878=AXIS2_PLACEMENT_3D('',#212531,#121203,#121204);
#100879=AXIS2_PLACEMENT_3D('',#212532,#121205,#121206);
#100880=AXIS2_PLACEMENT_3D('',#212534,#121207,#121208);
#100881=AXIS2_PLACEMENT_3D('',#212536,#121209,#121210);
#100882=AXIS2_PLACEMENT_3D('',#212537,#121211,#121212);
#100883=AXIS2_PLACEMENT_3D('',#212538,#121213,#121214);
#100884=AXIS2_PLACEMENT_3D('',#212541,#121215,#121216);
#100885=AXIS2_PLACEMENT_3D('',#212542,#121217,#121218);
#100886=AXIS2_PLACEMENT_3D('',#212543,#121219,#121220);
#100887=AXIS2_PLACEMENT_3D('',#212544,#121221,#121222);
#100888=AXIS2_PLACEMENT_3D('',#212547,#121223,#121224);
#100889=AXIS2_PLACEMENT_3D('',#212548,#121225,#121226);
#100890=AXIS2_PLACEMENT_3D('',#212549,#121227,#121228);
#100891=AXIS2_PLACEMENT_3D('',#212550,#121229,#121230);
#100892=AXIS2_PLACEMENT_3D('',#212553,#121231,#121232);
#100893=AXIS2_PLACEMENT_3D('',#212554,#121233,#121234);
#100894=AXIS2_PLACEMENT_3D('',#212555,#121235,#121236);
#100895=AXIS2_PLACEMENT_3D('',#212556,#121237,#121238);
#100896=AXIS2_PLACEMENT_3D('',#212559,#121239,#121240);
#100897=AXIS2_PLACEMENT_3D('',#212560,#121241,#121242);
#100898=AXIS2_PLACEMENT_3D('',#212561,#121243,#121244);
#100899=AXIS2_PLACEMENT_3D('',#212562,#121245,#121246);
#100900=AXIS2_PLACEMENT_3D('',#212565,#121247,#121248);
#100901=AXIS2_PLACEMENT_3D('',#212566,#121249,#121250);
#100902=AXIS2_PLACEMENT_3D('',#212567,#121251,#121252);
#100903=AXIS2_PLACEMENT_3D('',#212568,#121253,#121254);
#100904=AXIS2_PLACEMENT_3D('',#212571,#121255,#121256);
#100905=AXIS2_PLACEMENT_3D('',#212572,#121257,#121258);
#100906=AXIS2_PLACEMENT_3D('',#212573,#121259,#121260);
#100907=AXIS2_PLACEMENT_3D('',#212574,#121261,#121262);
#100908=AXIS2_PLACEMENT_3D('',#212577,#121263,#121264);
#100909=AXIS2_PLACEMENT_3D('',#212578,#121265,#121266);
#100910=AXIS2_PLACEMENT_3D('',#212579,#121267,#121268);
#100911=AXIS2_PLACEMENT_3D('',#212580,#121269,#121270);
#100912=AXIS2_PLACEMENT_3D('',#212583,#121271,#121272);
#100913=AXIS2_PLACEMENT_3D('',#212584,#121273,#121274);
#100914=AXIS2_PLACEMENT_3D('',#212585,#121275,#121276);
#100915=AXIS2_PLACEMENT_3D('',#212586,#121277,#121278);
#100916=AXIS2_PLACEMENT_3D('',#212587,#121279,#121280);
#100917=AXIS2_PLACEMENT_3D('',#212588,#121281,#121282);
#100918=AXIS2_PLACEMENT_3D('',#212589,#121283,#121284);
#100919=AXIS2_PLACEMENT_3D('',#212592,#121285,#121286);
#100920=AXIS2_PLACEMENT_3D('',#212593,#121287,#121288);
#100921=AXIS2_PLACEMENT_3D('',#212594,#121289,#121290);
#100922=AXIS2_PLACEMENT_3D('',#212595,#121291,#121292);
#100923=AXIS2_PLACEMENT_3D('',#212598,#121293,#121294);
#100924=AXIS2_PLACEMENT_3D('',#212599,#121295,#121296);
#100925=AXIS2_PLACEMENT_3D('',#212600,#121297,#121298);
#100926=AXIS2_PLACEMENT_3D('',#212601,#121299,#121300);
#100927=AXIS2_PLACEMENT_3D('',#212604,#121301,#121302);
#100928=AXIS2_PLACEMENT_3D('',#212605,#121303,#121304);
#100929=AXIS2_PLACEMENT_3D('',#212606,#121305,#121306);
#100930=AXIS2_PLACEMENT_3D('',#212607,#121307,#121308);
#100931=AXIS2_PLACEMENT_3D('',#212610,#121309,#121310);
#100932=AXIS2_PLACEMENT_3D('',#212611,#121311,#121312);
#100933=AXIS2_PLACEMENT_3D('',#212612,#121313,#121314);
#100934=AXIS2_PLACEMENT_3D('',#212613,#121315,#121316);
#100935=AXIS2_PLACEMENT_3D('',#212616,#121317,#121318);
#100936=AXIS2_PLACEMENT_3D('',#212617,#121319,#121320);
#100937=AXIS2_PLACEMENT_3D('',#212618,#121321,#121322);
#100938=AXIS2_PLACEMENT_3D('',#212619,#121323,#121324);
#100939=AXIS2_PLACEMENT_3D('',#212622,#121325,#121326);
#100940=AXIS2_PLACEMENT_3D('',#212623,#121327,#121328);
#100941=AXIS2_PLACEMENT_3D('',#212624,#121329,#121330);
#100942=AXIS2_PLACEMENT_3D('',#212625,#121331,#121332);
#100943=AXIS2_PLACEMENT_3D('',#212628,#121333,#121334);
#100944=AXIS2_PLACEMENT_3D('',#212629,#121335,#121336);
#100945=AXIS2_PLACEMENT_3D('',#212630,#121337,#121338);
#100946=AXIS2_PLACEMENT_3D('',#212631,#121339,#121340);
#100947=AXIS2_PLACEMENT_3D('',#212634,#121341,#121342);
#100948=AXIS2_PLACEMENT_3D('',#212635,#121343,#121344);
#100949=AXIS2_PLACEMENT_3D('',#212636,#121345,#121346);
#100950=AXIS2_PLACEMENT_3D('',#212637,#121347,#121348);
#100951=AXIS2_PLACEMENT_3D('',#212638,#121349,#121350);
#100952=AXIS2_PLACEMENT_3D('',#212639,#121351,#121352);
#100953=AXIS2_PLACEMENT_3D('',#212640,#121353,#121354);
#100954=AXIS2_PLACEMENT_3D('',#212643,#121355,#121356);
#100955=AXIS2_PLACEMENT_3D('',#212645,#121357,#121358);
#100956=AXIS2_PLACEMENT_3D('',#212657,#121359,#121360);
#100957=AXIS2_PLACEMENT_3D('',#212658,#121361,#121362);
#100958=AXIS2_PLACEMENT_3D('',#212661,#121363,#121364);
#100959=AXIS2_PLACEMENT_3D('',#212664,#121367,#121368);
#100960=AXIS2_PLACEMENT_3D('',#212666,#121369,#121370);
#100961=AXIS2_PLACEMENT_3D('',#212668,#121371,#121372);
#100962=AXIS2_PLACEMENT_3D('',#212669,#121373,#121374);
#100963=AXIS2_PLACEMENT_3D('',#212670,#121375,#121376);
#100964=AXIS2_PLACEMENT_3D('',#212673,#121377,#121378);
#100965=AXIS2_PLACEMENT_3D('',#212674,#121379,#121380);
#100966=AXIS2_PLACEMENT_3D('',#212675,#121381,#121382);
#100967=AXIS2_PLACEMENT_3D('',#212676,#121383,#121384);
#100968=AXIS2_PLACEMENT_3D('',#212679,#121385,#121386);
#100969=AXIS2_PLACEMENT_3D('',#212680,#121387,#121388);
#100970=AXIS2_PLACEMENT_3D('',#212681,#121389,#121390);
#100971=AXIS2_PLACEMENT_3D('',#212682,#121391,#121392);
#100972=AXIS2_PLACEMENT_3D('',#212685,#121393,#121394);
#100973=AXIS2_PLACEMENT_3D('',#212688,#121397,#121398);
#100974=AXIS2_PLACEMENT_3D('',#212701,#121399,#121400);
#100975=AXIS2_PLACEMENT_3D('',#212702,#121401,#121402);
#100976=AXIS2_PLACEMENT_3D('',#212703,#121403,#121404);
#100977=AXIS2_PLACEMENT_3D('',#212706,#121405,#121406);
#100978=AXIS2_PLACEMENT_3D('',#212708,#121407,#121408);
#100979=AXIS2_PLACEMENT_3D('',#212720,#121409,#121410);
#100980=AXIS2_PLACEMENT_3D('',#212721,#121411,#121412);
#100981=AXIS2_PLACEMENT_3D('',#212724,#121413,#121414);
#100982=AXIS2_PLACEMENT_3D('',#212727,#121417,#121418);
#100983=AXIS2_PLACEMENT_3D('',#212730,#121419,#121420);
#100984=AXIS2_PLACEMENT_3D('',#212731,#121421,#121422);
#100985=AXIS2_PLACEMENT_3D('',#212732,#121423,#121424);
#100986=AXIS2_PLACEMENT_3D('',#212733,#121425,#121426);
#100987=AXIS2_PLACEMENT_3D('',#212736,#121427,#121428);
#100988=AXIS2_PLACEMENT_3D('',#212737,#121429,#121430);
#100989=AXIS2_PLACEMENT_3D('',#212738,#121431,#121432);
#100990=AXIS2_PLACEMENT_3D('',#212739,#121433,#121434);
#100991=AXIS2_PLACEMENT_3D('',#212742,#121435,#121436);
#100992=AXIS2_PLACEMENT_3D('',#212743,#121437,#121438);
#100993=AXIS2_PLACEMENT_3D('',#212744,#121439,#121440);
#100994=AXIS2_PLACEMENT_3D('',#212745,#121441,#121442);
#100995=AXIS2_PLACEMENT_3D('',#212748,#121443,#121444);
#100996=AXIS2_PLACEMENT_3D('',#212751,#121447,#121448);
#100997=AXIS2_PLACEMENT_3D('',#212764,#121449,#121450);
#100998=AXIS2_PLACEMENT_3D('',#212765,#121451,#121452);
#100999=AXIS2_PLACEMENT_3D('',#212766,#121453,#121454);
#101000=AXIS2_PLACEMENT_3D('',#212769,#121455,#121456);
#101001=AXIS2_PLACEMENT_3D('',#212771,#121457,#121458);
#101002=AXIS2_PLACEMENT_3D('',#212783,#121459,#121460);
#101003=AXIS2_PLACEMENT_3D('',#212784,#121461,#121462);
#101004=AXIS2_PLACEMENT_3D('',#212787,#121463,#121464);
#101005=AXIS2_PLACEMENT_3D('',#212790,#121467,#121468);
#101006=AXIS2_PLACEMENT_3D('',#212792,#121469,#121470);
#101007=AXIS2_PLACEMENT_3D('',#212794,#121471,#121472);
#101008=AXIS2_PLACEMENT_3D('',#212795,#121473,#121474);
#101009=AXIS2_PLACEMENT_3D('',#212796,#121475,#121476);
#101010=AXIS2_PLACEMENT_3D('',#212799,#121477,#121478);
#101011=AXIS2_PLACEMENT_3D('',#212800,#121479,#121480);
#101012=AXIS2_PLACEMENT_3D('',#212801,#121481,#121482);
#101013=AXIS2_PLACEMENT_3D('',#212802,#121483,#121484);
#101014=AXIS2_PLACEMENT_3D('',#212805,#121485,#121486);
#101015=AXIS2_PLACEMENT_3D('',#212806,#121487,#121488);
#101016=AXIS2_PLACEMENT_3D('',#212807,#121489,#121490);
#101017=AXIS2_PLACEMENT_3D('',#212808,#121491,#121492);
#101018=AXIS2_PLACEMENT_3D('',#212811,#121493,#121494);
#101019=AXIS2_PLACEMENT_3D('',#212814,#121497,#121498);
#101020=AXIS2_PLACEMENT_3D('',#212827,#121499,#121500);
#101021=AXIS2_PLACEMENT_3D('',#212828,#121501,#121502);
#101022=AXIS2_PLACEMENT_3D('',#212829,#121503,#121504);
#101023=AXIS2_PLACEMENT_3D('',#212843,#121505,#121506);
#101024=AXIS2_PLACEMENT_3D('',#212845,#121507,#121508);
#101025=AXIS2_PLACEMENT_3D('',#212846,#121509,#121510);
#101026=AXIS2_PLACEMENT_3D('',#212847,#121511,#121512);
#101027=AXIS2_PLACEMENT_3D('',#212850,#121513,#121514);
#101028=AXIS2_PLACEMENT_3D('',#212853,#121517,#121518);
#101029=AXIS2_PLACEMENT_3D('',#212856,#121519,#121520);
#101030=AXIS2_PLACEMENT_3D('',#212857,#121521,#121522);
#101031=AXIS2_PLACEMENT_3D('',#212858,#121523,#121524);
#101032=AXIS2_PLACEMENT_3D('',#212859,#121525,#121526);
#101033=AXIS2_PLACEMENT_3D('',#212862,#121527,#121528);
#101034=AXIS2_PLACEMENT_3D('',#212863,#121529,#121530);
#101035=AXIS2_PLACEMENT_3D('',#212864,#121531,#121532);
#101036=AXIS2_PLACEMENT_3D('',#212865,#121533,#121534);
#101037=AXIS2_PLACEMENT_3D('',#212868,#121535,#121536);
#101038=AXIS2_PLACEMENT_3D('',#212869,#121537,#121538);
#101039=AXIS2_PLACEMENT_3D('',#212870,#121539,#121540);
#101040=AXIS2_PLACEMENT_3D('',#212871,#121541,#121542);
#101041=AXIS2_PLACEMENT_3D('',#212874,#121543,#121544);
#101042=AXIS2_PLACEMENT_3D('',#212877,#121547,#121548);
#101043=AXIS2_PLACEMENT_3D('',#212890,#121549,#121550);
#101044=AXIS2_PLACEMENT_3D('',#212891,#121551,#121552);
#101045=AXIS2_PLACEMENT_3D('',#212892,#121553,#121554);
#101046=AXIS2_PLACEMENT_3D('',#212894,#121555,#121556);
#101047=AXIS2_PLACEMENT_3D('',#212896,#121557,#121558);
#101048=AXIS2_PLACEMENT_3D('',#212897,#121559,#121560);
#101049=AXIS2_PLACEMENT_3D('',#212898,#121561,#121562);
#101050=AXIS2_PLACEMENT_3D('',#212901,#121563,#121564);
#101051=AXIS2_PLACEMENT_3D('',#212902,#121565,#121566);
#101052=AXIS2_PLACEMENT_3D('',#212903,#121567,#121568);
#101053=AXIS2_PLACEMENT_3D('',#212904,#121569,#121570);
#101054=AXIS2_PLACEMENT_3D('',#212907,#121571,#121572);
#101055=AXIS2_PLACEMENT_3D('',#212908,#121573,#121574);
#101056=AXIS2_PLACEMENT_3D('',#212909,#121575,#121576);
#101057=AXIS2_PLACEMENT_3D('',#212910,#121577,#121578);
#101058=AXIS2_PLACEMENT_3D('',#212913,#121579,#121580);
#101059=AXIS2_PLACEMENT_3D('',#212914,#121581,#121582);
#101060=AXIS2_PLACEMENT_3D('',#212915,#121583,#121584);
#101061=AXIS2_PLACEMENT_3D('',#212916,#121585,#121586);
#101062=AXIS2_PLACEMENT_3D('',#212919,#121587,#121588);
#101063=AXIS2_PLACEMENT_3D('',#212920,#121589,#121590);
#101064=AXIS2_PLACEMENT_3D('',#212921,#121591,#121592);
#101065=AXIS2_PLACEMENT_3D('',#212922,#121593,#121594);
#101066=AXIS2_PLACEMENT_3D('',#212925,#121595,#121596);
#101067=AXIS2_PLACEMENT_3D('',#212926,#121597,#121598);
#101068=AXIS2_PLACEMENT_3D('',#212927,#121599,#121600);
#101069=AXIS2_PLACEMENT_3D('',#212928,#121601,#121602);
#101070=AXIS2_PLACEMENT_3D('',#212931,#121603,#121604);
#101071=AXIS2_PLACEMENT_3D('',#212932,#121605,#121606);
#101072=AXIS2_PLACEMENT_3D('',#212933,#121607,#121608);
#101073=AXIS2_PLACEMENT_3D('',#212934,#121609,#121610);
#101074=AXIS2_PLACEMENT_3D('',#212937,#121611,#121612);
#101075=AXIS2_PLACEMENT_3D('',#212938,#121613,#121614);
#101076=AXIS2_PLACEMENT_3D('',#212939,#121615,#121616);
#101077=AXIS2_PLACEMENT_3D('',#212940,#121617,#121618);
#101078=AXIS2_PLACEMENT_3D('',#212941,#121619,#121620);
#101079=AXIS2_PLACEMENT_3D('',#212942,#121621,#121622);
#101080=AXIS2_PLACEMENT_3D('',#213177,#121623,#121624);
#101081=AXIS2_PLACEMENT_3D('',#213410,#121625,#121626);
#101082=AXIS2_PLACEMENT_3D('',#213415,#121627,#121628);
#101083=AXIS2_PLACEMENT_3D('',#213430,#121629,#121630);
#101084=AXIS2_PLACEMENT_3D('',#213431,#121631,#121632);
#101085=AXIS2_PLACEMENT_3D('',#213432,#121633,#121634);
#101086=AXIS2_PLACEMENT_3D('',#213513,#121635,#121636);
#101087=AXIS2_PLACEMENT_3D('',#213664,#121637,#121638);
#101088=AXIS2_PLACEMENT_3D('',#213897,#121639,#121640);
#101089=AXIS2_PLACEMENT_3D('',#214054,#121641,#121642);
#101090=AXIS2_PLACEMENT_3D('',#214055,#121643,#121644);
#101091=AXIS2_PLACEMENT_3D('',#214056,#121645,#121646);
#101092=AXIS2_PLACEMENT_3D('',#214071,#121647,#121648);
#101093=AXIS2_PLACEMENT_3D('',#214403,#121649,#121650);
#101094=AXIS2_PLACEMENT_3D('',#214927,#121651,#121652);
#101095=AXIS2_PLACEMENT_3D('',#214962,#121653,#121654);
#101096=AXIS2_PLACEMENT_3D('',#214963,#121655,#121656);
#101097=AXIS2_PLACEMENT_3D('',#214964,#121657,#121658);
#101098=AXIS2_PLACEMENT_3D('',#215063,#121659,#121660);
#101099=AXIS2_PLACEMENT_3D('',#215392,#121661,#121662);
#101100=AXIS2_PLACEMENT_3D('',#215637,#121663,#121664);
#101101=AXIS2_PLACEMENT_3D('',#215775,#121665,#121666);
#101102=AXIS2_PLACEMENT_3D('',#215776,#121667,#121668);
#101103=AXIS2_PLACEMENT_3D('',#215777,#121669,#121670);
#101104=AXIS2_PLACEMENT_3D('',#215792,#121671,#121672);
#101105=AXIS2_PLACEMENT_3D('',#216763,#121673,#121674);
#101106=AXIS2_PLACEMENT_3D('',#216764,#121675,#121676);
#101107=AXIS2_PLACEMENT_3D('',#216779,#121677,#121678);
#101108=AXIS2_PLACEMENT_3D('',#216780,#121679,#121680);
#101109=AXIS2_PLACEMENT_3D('',#216781,#121681,#121682);
#101110=AXIS2_PLACEMENT_3D('',#216862,#121683,#121684);
#101111=AXIS2_PLACEMENT_3D('',#217215,#121685,#121686);
#101112=AXIS2_PLACEMENT_3D('',#217277,#121687,#121688);
#101113=AXIS2_PLACEMENT_3D('',#217279,#121689,#121690);
#101114=AXIS2_PLACEMENT_3D('',#217280,#121691,#121692);
#101115=AXIS2_PLACEMENT_3D('',#217305,#121693,#121694);
#101116=AXIS2_PLACEMENT_3D('',#217306,#121695,#121696);
#101117=AXIS2_PLACEMENT_3D('',#218572,#121697,#121698);
#101118=AXIS2_PLACEMENT_3D('',#218593,#121699,#121700);
#101119=AXIS2_PLACEMENT_3D('',#218618,#121701,#121702);
#101120=AXIS2_PLACEMENT_3D('',#218620,#121703,#121704);
#101121=AXIS2_PLACEMENT_3D('',#218621,#121705,#121706);
#101122=AXIS2_PLACEMENT_3D('',#218642,#121707,#121708);
#101123=AXIS2_PLACEMENT_3D('',#218743,#121709,#121710);
#101124=AXIS2_PLACEMENT_3D('',#219018,#121711,#121712);
#101125=AXIS2_PLACEMENT_3D('',#219019,#121713,#121714);
#101126=AXIS2_PLACEMENT_3D('',#219020,#121715,#121716);
#101127=AXIS2_PLACEMENT_3D('',#219067,#121717,#121718);
#101128=AXIS2_PLACEMENT_3D('',#220115,#121719,#121720);
#101129=AXIS2_PLACEMENT_3D('',#220116,#121721,#121722);
#101130=AXIS2_PLACEMENT_3D('',#220131,#121723,#121724);
#101131=AXIS2_PLACEMENT_3D('',#220132,#121725,#121726);
#101132=AXIS2_PLACEMENT_3D('',#220133,#121727,#121728);
#101133=AXIS2_PLACEMENT_3D('',#220147,#121729,#121730);
#101134=AXIS2_PLACEMENT_3D('',#220149,#121731,#121732);
#101135=AXIS2_PLACEMENT_3D('',#220150,#121733,#121734);
#101136=AXIS2_PLACEMENT_3D('',#220183,#121735,#121736);
#101137=AXIS2_PLACEMENT_3D('',#220398,#121737,#121738);
#101138=AXIS2_PLACEMENT_3D('',#220608,#121739,#121740);
#101139=AXIS2_PLACEMENT_3D('',#220609,#121741,#121742);
#101140=AXIS2_PLACEMENT_3D('',#220632,#121743,#121744);
#101141=AXIS2_PLACEMENT_3D('',#220643,#121745,#121746);
#101142=AXIS2_PLACEMENT_3D('',#220645,#121747,#121748);
#101143=AXIS2_PLACEMENT_3D('',#220647,#121749,#121750);
#101144=AXIS2_PLACEMENT_3D('',#220648,#121751,#121752);
#101145=AXIS2_PLACEMENT_3D('',#221316,#121753,#121754);
#101146=AXIS2_PLACEMENT_3D('',#221341,#121755,#121756);
#101147=AXIS2_PLACEMENT_3D('',#221343,#121757,#121758);
#101148=AXIS2_PLACEMENT_3D('',#221344,#121759,#121760);
#101149=AXIS2_PLACEMENT_3D('',#221358,#121761,#121762);
#101150=AXIS2_PLACEMENT_3D('',#221398,#121763,#121764);
#101151=AXIS2_PLACEMENT_3D('',#221501,#121765,#121766);
#101152=AXIS2_PLACEMENT_3D('',#221827,#121767,#121768);
#101153=AXIS2_PLACEMENT_3D('',#221841,#121769,#121770);
#101154=AXIS2_PLACEMENT_3D('',#222188,#121771,#121772);
#101155=AXIS2_PLACEMENT_3D('',#222191,#121773,#121774);
#101156=AXIS2_PLACEMENT_3D('',#222194,#121777,#121778);
#101157=AXIS2_PLACEMENT_3D('',#222199,#121781,#121782);
#101158=AXIS2_PLACEMENT_3D('',#222200,#121783,#121784);
#101159=AXIS2_PLACEMENT_3D('',#222205,#121787,#121788);
#101160=AXIS2_PLACEMENT_3D('',#222206,#121789,#121790);
#101161=AXIS2_PLACEMENT_3D('',#222211,#121793,#121794);
#101162=AXIS2_PLACEMENT_3D('',#222212,#121795,#121796);
#101163=AXIS2_PLACEMENT_3D('',#222217,#121799,#121800);
#101164=AXIS2_PLACEMENT_3D('',#222218,#121801,#121802);
#101165=AXIS2_PLACEMENT_3D('',#222223,#121805,#121806);
#101166=AXIS2_PLACEMENT_3D('',#222224,#121807,#121808);
#101167=AXIS2_PLACEMENT_3D('',#222229,#121811,#121812);
#101168=AXIS2_PLACEMENT_3D('',#222230,#121813,#121814);
#101169=AXIS2_PLACEMENT_3D('',#222235,#121817,#121818);
#101170=AXIS2_PLACEMENT_3D('',#222236,#121819,#121820);
#101171=AXIS2_PLACEMENT_3D('',#222241,#121823,#121824);
#101172=AXIS2_PLACEMENT_3D('',#222242,#121825,#121826);
#101173=AXIS2_PLACEMENT_3D('',#222245,#121827,#121828);
#101174=AXIS2_PLACEMENT_3D('',#222248,#121831,#121832);
#101175=AXIS2_PLACEMENT_3D('',#222253,#121835,#121836);
#101176=AXIS2_PLACEMENT_3D('',#222254,#121837,#121838);
#101177=AXIS2_PLACEMENT_3D('',#222259,#121841,#121842);
#101178=AXIS2_PLACEMENT_3D('',#222260,#121843,#121844);
#101179=AXIS2_PLACEMENT_3D('',#222265,#121847,#121848);
#101180=AXIS2_PLACEMENT_3D('',#222266,#121849,#121850);
#101181=AXIS2_PLACEMENT_3D('',#222271,#121853,#121854);
#101182=AXIS2_PLACEMENT_3D('',#222272,#121855,#121856);
#101183=AXIS2_PLACEMENT_3D('',#222277,#121859,#121860);
#101184=AXIS2_PLACEMENT_3D('',#222278,#121861,#121862);
#101185=AXIS2_PLACEMENT_3D('',#222283,#121865,#121866);
#101186=AXIS2_PLACEMENT_3D('',#222284,#121867,#121868);
#101187=AXIS2_PLACEMENT_3D('',#222289,#121871,#121872);
#101188=AXIS2_PLACEMENT_3D('',#222290,#121873,#121874);
#101189=AXIS2_PLACEMENT_3D('',#222295,#121877,#121878);
#101190=AXIS2_PLACEMENT_3D('',#222296,#121879,#121880);
#101191=AXIS2_PLACEMENT_3D('',#222301,#121883,#121884);
#101192=AXIS2_PLACEMENT_3D('',#222302,#121885,#121886);
#101193=AXIS2_PLACEMENT_3D('',#222307,#121889,#121890);
#101194=AXIS2_PLACEMENT_3D('',#222308,#121891,#121892);
#101195=AXIS2_PLACEMENT_3D('',#222313,#121895,#121896);
#101196=AXIS2_PLACEMENT_3D('',#222314,#121897,#121898);
#101197=AXIS2_PLACEMENT_3D('',#222319,#121901,#121902);
#101198=AXIS2_PLACEMENT_3D('',#222320,#121903,#121904);
#101199=AXIS2_PLACEMENT_3D('',#222325,#121907,#121908);
#101200=AXIS2_PLACEMENT_3D('',#222326,#121909,#121910);
#101201=AXIS2_PLACEMENT_3D('',#222331,#121913,#121914);
#101202=AXIS2_PLACEMENT_3D('',#222332,#121915,#121916);
#101203=AXIS2_PLACEMENT_3D('',#222337,#121919,#121920);
#101204=AXIS2_PLACEMENT_3D('',#222338,#121921,#121922);
#101205=AXIS2_PLACEMENT_3D('',#222343,#121925,#121926);
#101206=AXIS2_PLACEMENT_3D('',#222344,#121927,#121928);
#101207=AXIS2_PLACEMENT_3D('',#222349,#121931,#121932);
#101208=AXIS2_PLACEMENT_3D('',#222350,#121933,#121934);
#101209=AXIS2_PLACEMENT_3D('',#222353,#121935,#121936);
#101210=AXIS2_PLACEMENT_3D('',#222356,#121939,#121940);
#101211=AXIS2_PLACEMENT_3D('',#222361,#121943,#121944);
#101212=AXIS2_PLACEMENT_3D('',#222362,#121945,#121946);
#101213=AXIS2_PLACEMENT_3D('',#222367,#121949,#121950);
#101214=AXIS2_PLACEMENT_3D('',#222368,#121951,#121952);
#101215=AXIS2_PLACEMENT_3D('',#222373,#121955,#121956);
#101216=AXIS2_PLACEMENT_3D('',#222374,#121957,#121958);
#101217=AXIS2_PLACEMENT_3D('',#222379,#121961,#121962);
#101218=AXIS2_PLACEMENT_3D('',#222380,#121963,#121964);
#101219=AXIS2_PLACEMENT_3D('',#222385,#121967,#121968);
#101220=AXIS2_PLACEMENT_3D('',#222386,#121969,#121970);
#101221=AXIS2_PLACEMENT_3D('',#222391,#121973,#121974);
#101222=AXIS2_PLACEMENT_3D('',#222392,#121975,#121976);
#101223=AXIS2_PLACEMENT_3D('',#222397,#121979,#121980);
#101224=AXIS2_PLACEMENT_3D('',#222398,#121981,#121982);
#101225=AXIS2_PLACEMENT_3D('',#222403,#121985,#121986);
#101226=AXIS2_PLACEMENT_3D('',#222404,#121987,#121988);
#101227=AXIS2_PLACEMENT_3D('',#222409,#121991,#121992);
#101228=AXIS2_PLACEMENT_3D('',#222410,#121993,#121994);
#101229=AXIS2_PLACEMENT_3D('',#222415,#121997,#121998);
#101230=AXIS2_PLACEMENT_3D('',#222416,#121999,#122000);
#101231=AXIS2_PLACEMENT_3D('',#222421,#122003,#122004);
#101232=AXIS2_PLACEMENT_3D('',#222422,#122005,#122006);
#101233=AXIS2_PLACEMENT_3D('',#222427,#122009,#122010);
#101234=AXIS2_PLACEMENT_3D('',#222428,#122011,#122012);
#101235=AXIS2_PLACEMENT_3D('',#222433,#122015,#122016);
#101236=AXIS2_PLACEMENT_3D('',#222434,#122017,#122018);
#101237=AXIS2_PLACEMENT_3D('',#222439,#122021,#122022);
#101238=AXIS2_PLACEMENT_3D('',#222440,#122023,#122024);
#101239=AXIS2_PLACEMENT_3D('',#222445,#122027,#122028);
#101240=AXIS2_PLACEMENT_3D('',#222446,#122029,#122030);
#101241=AXIS2_PLACEMENT_3D('',#222451,#122033,#122034);
#101242=AXIS2_PLACEMENT_3D('',#222452,#122035,#122036);
#101243=AXIS2_PLACEMENT_3D('',#222457,#122039,#122040);
#101244=AXIS2_PLACEMENT_3D('',#222458,#122041,#122042);
#101245=AXIS2_PLACEMENT_3D('',#222463,#122045,#122046);
#101246=AXIS2_PLACEMENT_3D('',#222464,#122047,#122048);
#101247=AXIS2_PLACEMENT_3D('',#222469,#122051,#122052);
#101248=AXIS2_PLACEMENT_3D('',#222470,#122053,#122054);
#101249=AXIS2_PLACEMENT_3D('',#222475,#122057,#122058);
#101250=AXIS2_PLACEMENT_3D('',#222476,#122059,#122060);
#101251=AXIS2_PLACEMENT_3D('',#222481,#122063,#122064);
#101252=AXIS2_PLACEMENT_3D('',#222482,#122065,#122066);
#101253=AXIS2_PLACEMENT_3D('',#222487,#122069,#122070);
#101254=AXIS2_PLACEMENT_3D('',#222488,#122071,#122072);
#101255=AXIS2_PLACEMENT_3D('',#222493,#122075,#122076);
#101256=AXIS2_PLACEMENT_3D('',#222494,#122077,#122078);
#101257=AXIS2_PLACEMENT_3D('',#222499,#122081,#122082);
#101258=AXIS2_PLACEMENT_3D('',#222500,#122083,#122084);
#101259=AXIS2_PLACEMENT_3D('',#222505,#122087,#122088);
#101260=AXIS2_PLACEMENT_3D('',#222506,#122089,#122090);
#101261=AXIS2_PLACEMENT_3D('',#222511,#122093,#122094);
#101262=AXIS2_PLACEMENT_3D('',#222512,#122095,#122096);
#101263=AXIS2_PLACEMENT_3D('',#222517,#122099,#122100);
#101264=AXIS2_PLACEMENT_3D('',#222518,#122101,#122102);
#101265=AXIS2_PLACEMENT_3D('',#222523,#122105,#122106);
#101266=AXIS2_PLACEMENT_3D('',#222524,#122107,#122108);
#101267=AXIS2_PLACEMENT_3D('',#222529,#122111,#122112);
#101268=AXIS2_PLACEMENT_3D('',#222530,#122113,#122114);
#101269=AXIS2_PLACEMENT_3D('',#222535,#122117,#122118);
#101270=AXIS2_PLACEMENT_3D('',#222536,#122119,#122120);
#101271=AXIS2_PLACEMENT_3D('',#222541,#122123,#122124);
#101272=AXIS2_PLACEMENT_3D('',#222542,#122125,#122126);
#101273=AXIS2_PLACEMENT_3D('',#222547,#122129,#122130);
#101274=AXIS2_PLACEMENT_3D('',#222548,#122131,#122132);
#101275=AXIS2_PLACEMENT_3D('',#222553,#122135,#122136);
#101276=AXIS2_PLACEMENT_3D('',#222554,#122137,#122138);
#101277=AXIS2_PLACEMENT_3D('',#222559,#122141,#122142);
#101278=AXIS2_PLACEMENT_3D('',#222560,#122143,#122144);
#101279=AXIS2_PLACEMENT_3D('',#222565,#122147,#122148);
#101280=AXIS2_PLACEMENT_3D('',#222566,#122149,#122150);
#101281=AXIS2_PLACEMENT_3D('',#222571,#122153,#122154);
#101282=AXIS2_PLACEMENT_3D('',#222572,#122155,#122156);
#101283=AXIS2_PLACEMENT_3D('',#222577,#122159,#122160);
#101284=AXIS2_PLACEMENT_3D('',#222578,#122161,#122162);
#101285=AXIS2_PLACEMENT_3D('',#222583,#122165,#122166);
#101286=AXIS2_PLACEMENT_3D('',#222584,#122167,#122168);
#101287=AXIS2_PLACEMENT_3D('',#222589,#122171,#122172);
#101288=AXIS2_PLACEMENT_3D('',#222590,#122173,#122174);
#101289=AXIS2_PLACEMENT_3D('',#222595,#122177,#122178);
#101290=AXIS2_PLACEMENT_3D('',#222596,#122179,#122180);
#101291=AXIS2_PLACEMENT_3D('',#222601,#122183,#122184);
#101292=AXIS2_PLACEMENT_3D('',#222602,#122185,#122186);
#101293=AXIS2_PLACEMENT_3D('',#222607,#122189,#122190);
#101294=AXIS2_PLACEMENT_3D('',#222608,#122191,#122192);
#101295=AXIS2_PLACEMENT_3D('',#222613,#122195,#122196);
#101296=AXIS2_PLACEMENT_3D('',#222614,#122197,#122198);
#101297=AXIS2_PLACEMENT_3D('',#222619,#122201,#122202);
#101298=AXIS2_PLACEMENT_3D('',#222620,#122203,#122204);
#101299=AXIS2_PLACEMENT_3D('',#222625,#122207,#122208);
#101300=AXIS2_PLACEMENT_3D('',#222626,#122209,#122210);
#101301=AXIS2_PLACEMENT_3D('',#222631,#122213,#122214);
#101302=AXIS2_PLACEMENT_3D('',#222632,#122215,#122216);
#101303=AXIS2_PLACEMENT_3D('',#222637,#122219,#122220);
#101304=AXIS2_PLACEMENT_3D('',#222638,#122221,#122222);
#101305=AXIS2_PLACEMENT_3D('',#222643,#122225,#122226);
#101306=AXIS2_PLACEMENT_3D('',#222644,#122227,#122228);
#101307=AXIS2_PLACEMENT_3D('',#222649,#122231,#122232);
#101308=AXIS2_PLACEMENT_3D('',#222650,#122233,#122234);
#101309=AXIS2_PLACEMENT_3D('',#222655,#122237,#122238);
#101310=AXIS2_PLACEMENT_3D('',#222656,#122239,#122240);
#101311=AXIS2_PLACEMENT_3D('',#222661,#122243,#122244);
#101312=AXIS2_PLACEMENT_3D('',#222662,#122245,#122246);
#101313=AXIS2_PLACEMENT_3D('',#222667,#122249,#122250);
#101314=AXIS2_PLACEMENT_3D('',#222668,#122251,#122252);
#101315=AXIS2_PLACEMENT_3D('',#222673,#122255,#122256);
#101316=AXIS2_PLACEMENT_3D('',#222674,#122257,#122258);
#101317=AXIS2_PLACEMENT_3D('',#222679,#122261,#122262);
#101318=AXIS2_PLACEMENT_3D('',#222680,#122263,#122264);
#101319=AXIS2_PLACEMENT_3D('',#222685,#122267,#122268);
#101320=AXIS2_PLACEMENT_3D('',#222686,#122269,#122270);
#101321=AXIS2_PLACEMENT_3D('',#222691,#122273,#122274);
#101322=AXIS2_PLACEMENT_3D('',#222692,#122275,#122276);
#101323=AXIS2_PLACEMENT_3D('',#222697,#122279,#122280);
#101324=AXIS2_PLACEMENT_3D('',#222698,#122281,#122282);
#101325=AXIS2_PLACEMENT_3D('',#222701,#122283,#122284);
#101326=AXIS2_PLACEMENT_3D('',#222704,#122287,#122288);
#101327=AXIS2_PLACEMENT_3D('',#222709,#122291,#122292);
#101328=AXIS2_PLACEMENT_3D('',#222710,#122293,#122294);
#101329=AXIS2_PLACEMENT_3D('',#222715,#122297,#122298);
#101330=AXIS2_PLACEMENT_3D('',#222716,#122299,#122300);
#101331=AXIS2_PLACEMENT_3D('',#222721,#122303,#122304);
#101332=AXIS2_PLACEMENT_3D('',#222722,#122305,#122306);
#101333=AXIS2_PLACEMENT_3D('',#222727,#122309,#122310);
#101334=AXIS2_PLACEMENT_3D('',#222728,#122311,#122312);
#101335=AXIS2_PLACEMENT_3D('',#222733,#122315,#122316);
#101336=AXIS2_PLACEMENT_3D('',#222734,#122317,#122318);
#101337=AXIS2_PLACEMENT_3D('',#222739,#122321,#122322);
#101338=AXIS2_PLACEMENT_3D('',#222740,#122323,#122324);
#101339=AXIS2_PLACEMENT_3D('',#222745,#122327,#122328);
#101340=AXIS2_PLACEMENT_3D('',#222746,#122329,#122330);
#101341=AXIS2_PLACEMENT_3D('',#222751,#122333,#122334);
#101342=AXIS2_PLACEMENT_3D('',#222752,#122335,#122336);
#101343=AXIS2_PLACEMENT_3D('',#222757,#122339,#122340);
#101344=AXIS2_PLACEMENT_3D('',#222758,#122341,#122342);
#101345=AXIS2_PLACEMENT_3D('',#222763,#122345,#122346);
#101346=AXIS2_PLACEMENT_3D('',#222764,#122347,#122348);
#101347=AXIS2_PLACEMENT_3D('',#222769,#122351,#122352);
#101348=AXIS2_PLACEMENT_3D('',#222770,#122353,#122354);
#101349=AXIS2_PLACEMENT_3D('',#222775,#122357,#122358);
#101350=AXIS2_PLACEMENT_3D('',#222776,#122359,#122360);
#101351=AXIS2_PLACEMENT_3D('',#222781,#122363,#122364);
#101352=AXIS2_PLACEMENT_3D('',#222782,#122365,#122366);
#101353=AXIS2_PLACEMENT_3D('',#222787,#122369,#122370);
#101354=AXIS2_PLACEMENT_3D('',#222788,#122371,#122372);
#101355=AXIS2_PLACEMENT_3D('',#222793,#122375,#122376);
#101356=AXIS2_PLACEMENT_3D('',#222794,#122377,#122378);
#101357=AXIS2_PLACEMENT_3D('',#222799,#122381,#122382);
#101358=AXIS2_PLACEMENT_3D('',#222800,#122383,#122384);
#101359=AXIS2_PLACEMENT_3D('',#222805,#122387,#122388);
#101360=AXIS2_PLACEMENT_3D('',#222806,#122389,#122390);
#101361=AXIS2_PLACEMENT_3D('',#222811,#122393,#122394);
#101362=AXIS2_PLACEMENT_3D('',#222812,#122395,#122396);
#101363=AXIS2_PLACEMENT_3D('',#222817,#122399,#122400);
#101364=AXIS2_PLACEMENT_3D('',#222818,#122401,#122402);
#101365=AXIS2_PLACEMENT_3D('',#222823,#122405,#122406);
#101366=AXIS2_PLACEMENT_3D('',#222824,#122407,#122408);
#101367=AXIS2_PLACEMENT_3D('',#222829,#122411,#122412);
#101368=AXIS2_PLACEMENT_3D('',#222830,#122413,#122414);
#101369=AXIS2_PLACEMENT_3D('',#222835,#122417,#122418);
#101370=AXIS2_PLACEMENT_3D('',#222836,#122419,#122420);
#101371=AXIS2_PLACEMENT_3D('',#222841,#122423,#122424);
#101372=AXIS2_PLACEMENT_3D('',#222842,#122425,#122426);
#101373=AXIS2_PLACEMENT_3D('',#222845,#122427,#122428);
#101374=AXIS2_PLACEMENT_3D('',#222848,#122431,#122432);
#101375=AXIS2_PLACEMENT_3D('',#222853,#122435,#122436);
#101376=AXIS2_PLACEMENT_3D('',#222854,#122437,#122438);
#101377=AXIS2_PLACEMENT_3D('',#222859,#122441,#122442);
#101378=AXIS2_PLACEMENT_3D('',#222860,#122443,#122444);
#101379=AXIS2_PLACEMENT_3D('',#222865,#122447,#122448);
#101380=AXIS2_PLACEMENT_3D('',#222866,#122449,#122450);
#101381=AXIS2_PLACEMENT_3D('',#222871,#122453,#122454);
#101382=AXIS2_PLACEMENT_3D('',#222872,#122455,#122456);
#101383=AXIS2_PLACEMENT_3D('',#222877,#122459,#122460);
#101384=AXIS2_PLACEMENT_3D('',#222878,#122461,#122462);
#101385=AXIS2_PLACEMENT_3D('',#222883,#122465,#122466);
#101386=AXIS2_PLACEMENT_3D('',#222884,#122467,#122468);
#101387=AXIS2_PLACEMENT_3D('',#222889,#122471,#122472);
#101388=AXIS2_PLACEMENT_3D('',#222890,#122473,#122474);
#101389=AXIS2_PLACEMENT_3D('',#222895,#122477,#122478);
#101390=AXIS2_PLACEMENT_3D('',#222896,#122479,#122480);
#101391=AXIS2_PLACEMENT_3D('',#222901,#122483,#122484);
#101392=AXIS2_PLACEMENT_3D('',#222902,#122485,#122486);
#101393=AXIS2_PLACEMENT_3D('',#222907,#122489,#122490);
#101394=AXIS2_PLACEMENT_3D('',#222908,#122491,#122492);
#101395=AXIS2_PLACEMENT_3D('',#222913,#122495,#122496);
#101396=AXIS2_PLACEMENT_3D('',#222914,#122497,#122498);
#101397=AXIS2_PLACEMENT_3D('',#222919,#122501,#122502);
#101398=AXIS2_PLACEMENT_3D('',#222920,#122503,#122504);
#101399=AXIS2_PLACEMENT_3D('',#222925,#122507,#122508);
#101400=AXIS2_PLACEMENT_3D('',#222926,#122509,#122510);
#101401=AXIS2_PLACEMENT_3D('',#222931,#122513,#122514);
#101402=AXIS2_PLACEMENT_3D('',#222932,#122515,#122516);
#101403=AXIS2_PLACEMENT_3D('',#222937,#122519,#122520);
#101404=AXIS2_PLACEMENT_3D('',#222938,#122521,#122522);
#101405=AXIS2_PLACEMENT_3D('',#222941,#122523,#122524);
#101406=AXIS2_PLACEMENT_3D('',#222944,#122527,#122528);
#101407=AXIS2_PLACEMENT_3D('',#222949,#122531,#122532);
#101408=AXIS2_PLACEMENT_3D('',#222950,#122533,#122534);
#101409=AXIS2_PLACEMENT_3D('',#222955,#122537,#122538);
#101410=AXIS2_PLACEMENT_3D('',#222956,#122539,#122540);
#101411=AXIS2_PLACEMENT_3D('',#222961,#122543,#122544);
#101412=AXIS2_PLACEMENT_3D('',#222962,#122545,#122546);
#101413=AXIS2_PLACEMENT_3D('',#222967,#122549,#122550);
#101414=AXIS2_PLACEMENT_3D('',#222968,#122551,#122552);
#101415=AXIS2_PLACEMENT_3D('',#222971,#122553,#122554);
#101416=AXIS2_PLACEMENT_3D('',#222974,#122557,#122558);
#101417=AXIS2_PLACEMENT_3D('',#222979,#122561,#122562);
#101418=AXIS2_PLACEMENT_3D('',#222980,#122563,#122564);
#101419=AXIS2_PLACEMENT_3D('',#222983,#122565,#122566);
#101420=AXIS2_PLACEMENT_3D('',#222986,#122569,#122570);
#101421=AXIS2_PLACEMENT_3D('',#222991,#122573,#122574);
#101422=AXIS2_PLACEMENT_3D('',#222992,#122575,#122576);
#101423=AXIS2_PLACEMENT_3D('',#222997,#122579,#122580);
#101424=AXIS2_PLACEMENT_3D('',#222998,#122581,#122582);
#101425=AXIS2_PLACEMENT_3D('',#223003,#122585,#122586);
#101426=AXIS2_PLACEMENT_3D('',#223004,#122587,#122588);
#101427=AXIS2_PLACEMENT_3D('',#223007,#122590,#122591);
#101428=AXIS2_PLACEMENT_3D('',#223008,#122592,#122593);
#101429=AXIS2_PLACEMENT_3D('',#223011,#122595,#122596);
#101430=AXIS2_PLACEMENT_3D('',#223012,#122597,#122598);
#101431=AXIS2_PLACEMENT_3D('',#223014,#122599,#122600);
#101432=AXIS2_PLACEMENT_3D('',#223015,#122601,#122602);
#101433=AXIS2_PLACEMENT_3D('',#223017,#122604,#122605);
#101434=AXIS2_PLACEMENT_3D('',#223018,#122606,#122607);
#101435=AXIS2_PLACEMENT_3D('',#223019,#122608,#122609);
#101436=AXIS2_PLACEMENT_3D('',#223020,#122610,#122611);
#101437=AXIS2_PLACEMENT_3D('',#223021,#122612,#122613);
#101438=AXIS2_PLACEMENT_3D('',#223022,#122614,#122615);
#101439=AXIS2_PLACEMENT_3D('',#223025,#122617,#122618);
#101440=AXIS2_PLACEMENT_3D('',#223026,#122619,#122620);
#101441=AXIS2_PLACEMENT_3D('',#223027,#122621,#122622);
#101442=AXIS2_PLACEMENT_3D('',#223028,#122623,#122624);
#101443=AXIS2_PLACEMENT_3D('',#223029,#122625,#122626);
#101444=AXIS2_PLACEMENT_3D('',#223030,#122627,#122628);
#101445=AXIS2_PLACEMENT_3D('',#223031,#122629,#122630);
#101446=AXIS2_PLACEMENT_3D('',#223032,#122631,#122632);
#101447=AXIS2_PLACEMENT_3D('',#223033,#122633,#122634);
#101448=AXIS2_PLACEMENT_3D('',#223034,#122635,#122636);
#101449=AXIS2_PLACEMENT_3D('',#223035,#122637,#122638);
#101450=AXIS2_PLACEMENT_3D('',#223036,#122639,#122640);
#101451=AXIS2_PLACEMENT_3D('',#223037,#122641,#122642);
#101452=AXIS2_PLACEMENT_3D('',#223038,#122643,#122644);
#101453=AXIS2_PLACEMENT_3D('',#223039,#122645,#122646);
#101454=AXIS2_PLACEMENT_3D('',#223040,#122647,#122648);
#101455=AXIS2_PLACEMENT_3D('',#223041,#122649,#122650);
#101456=AXIS2_PLACEMENT_3D('',#223042,#122651,#122652);
#101457=AXIS2_PLACEMENT_3D('',#223043,#122653,#122654);
#101458=AXIS2_PLACEMENT_3D('',#223044,#122655,#122656);
#101459=AXIS2_PLACEMENT_3D('',#223046,#122658,#122659);
#101460=AXIS2_PLACEMENT_3D('',#223048,#122661,#122662);
#101461=AXIS2_PLACEMENT_3D('',#223049,#122663,#122664);
#101462=AXIS2_PLACEMENT_3D('',#223050,#122665,#122666);
#101463=AXIS2_PLACEMENT_3D('',#223051,#122667,#122668);
#101464=AXIS2_PLACEMENT_3D('',#223052,#122669,#122670);
#101465=AXIS2_PLACEMENT_3D('',#223053,#122671,#122672);
#101466=AXIS2_PLACEMENT_3D('',#223054,#122673,#122674);
#101467=AXIS2_PLACEMENT_3D('',#223056,#122676,#122677);
#101468=AXIS2_PLACEMENT_3D('',#223058,#122679,#122680);
#101469=AXIS2_PLACEMENT_3D('',#223059,#122681,#122682);
#101470=AXIS2_PLACEMENT_3D('',#223060,#122683,#122684);
#101471=AXIS2_PLACEMENT_3D('',#223061,#122685,#122686);
#101472=AXIS2_PLACEMENT_3D('',#223062,#122687,#122688);
#101473=AXIS2_PLACEMENT_3D('',#223064,#122690,#122691);
#101474=AXIS2_PLACEMENT_3D('',#223066,#122693,#122694);
#101475=AXIS2_PLACEMENT_3D('',#223068,#122696,#122697);
#101476=AXIS2_PLACEMENT_3D('',#223070,#122699,#122700);
#101477=AXIS2_PLACEMENT_3D('',#223072,#122702,#122703);
#101478=AXIS2_PLACEMENT_3D('',#223074,#122705,#122706);
#101479=AXIS2_PLACEMENT_3D('',#223076,#122708,#122709);
#101480=AXIS2_PLACEMENT_3D('',#223078,#122711,#122712);
#101481=AXIS2_PLACEMENT_3D('',#223080,#122714,#122715);
#101482=AXIS2_PLACEMENT_3D('',#223082,#122717,#122718);
#101483=AXIS2_PLACEMENT_3D('',#223084,#122720,#122721);
#101484=AXIS2_PLACEMENT_3D('',#223086,#122723,#122724);
#101485=AXIS2_PLACEMENT_3D('',#223088,#122726,#122727);
#101486=AXIS2_PLACEMENT_3D('',#223090,#122729,#122730);
#101487=AXIS2_PLACEMENT_3D('',#223092,#122732,#122733);
#101488=AXIS2_PLACEMENT_3D('',#223094,#122735,#122736);
#101489=AXIS2_PLACEMENT_3D('',#223096,#122738,#122739);
#101490=AXIS2_PLACEMENT_3D('',#223098,#122741,#122742);
#101491=AXIS2_PLACEMENT_3D('',#223100,#122744,#122745);
#101492=AXIS2_PLACEMENT_3D('',#223102,#122747,#122748);
#101493=AXIS2_PLACEMENT_3D('',#223104,#122750,#122751);
#101494=AXIS2_PLACEMENT_3D('',#223106,#122753,#122754);
#101495=AXIS2_PLACEMENT_3D('',#223108,#122756,#122757);
#101496=AXIS2_PLACEMENT_3D('',#223110,#122759,#122760);
#101497=AXIS2_PLACEMENT_3D('',#223112,#122762,#122763);
#101498=AXIS2_PLACEMENT_3D('',#223114,#122765,#122766);
#101499=AXIS2_PLACEMENT_3D('',#223116,#122768,#122769);
#101500=AXIS2_PLACEMENT_3D('',#223118,#122771,#122772);
#101501=AXIS2_PLACEMENT_3D('',#223120,#122774,#122775);
#101502=AXIS2_PLACEMENT_3D('',#223122,#122777,#122778);
#101503=AXIS2_PLACEMENT_3D('',#223124,#122780,#122781);
#101504=AXIS2_PLACEMENT_3D('',#223126,#122783,#122784);
#101505=AXIS2_PLACEMENT_3D('',#223135,#122789,#122790);
#101506=AXIS2_PLACEMENT_3D('',#223141,#122794,#122795);
#101507=AXIS2_PLACEMENT_3D('',#223147,#122799,#122800);
#101508=AXIS2_PLACEMENT_3D('',#223149,#122802,#122803);
#101509=AXIS2_PLACEMENT_3D('',#223151,#122805,#122806);
#101510=AXIS2_PLACEMENT_3D('',#223153,#122808,#122809);
#101511=AXIS2_PLACEMENT_3D('',#223155,#122811,#122812);
#101512=AXIS2_PLACEMENT_3D('',#223157,#122814,#122815);
#101513=AXIS2_PLACEMENT_3D('',#223159,#122817,#122818);
#101514=AXIS2_PLACEMENT_3D('',#223161,#122820,#122821);
#101515=AXIS2_PLACEMENT_3D('',#223163,#122823,#122824);
#101516=AXIS2_PLACEMENT_3D('',#223165,#122826,#122827);
#101517=AXIS2_PLACEMENT_3D('',#223167,#122829,#122830);
#101518=AXIS2_PLACEMENT_3D('',#223169,#122832,#122833);
#101519=AXIS2_PLACEMENT_3D('',#223171,#122835,#122836);
#101520=AXIS2_PLACEMENT_3D('',#223173,#122838,#122839);
#101521=AXIS2_PLACEMENT_3D('',#223175,#122841,#122842);
#101522=AXIS2_PLACEMENT_3D('',#223177,#122844,#122845);
#101523=AXIS2_PLACEMENT_3D('',#223179,#122847,#122848);
#101524=AXIS2_PLACEMENT_3D('',#223181,#122850,#122851);
#101525=AXIS2_PLACEMENT_3D('',#223183,#122853,#122854);
#101526=AXIS2_PLACEMENT_3D('',#223185,#122856,#122857);
#101527=AXIS2_PLACEMENT_3D('',#223187,#122859,#122860);
#101528=AXIS2_PLACEMENT_3D('',#223189,#122862,#122863);
#101529=AXIS2_PLACEMENT_3D('',#223191,#122865,#122866);
#101530=AXIS2_PLACEMENT_3D('',#223192,#122867,#122868);
#101531=AXIS2_PLACEMENT_3D('',#223194,#122869,#122870);
#101532=AXIS2_PLACEMENT_3D('',#223196,#122871,#122872);
#101533=AXIS2_PLACEMENT_3D('',#223198,#122873,#122874);
#101534=AXIS2_PLACEMENT_3D('',#223200,#122875,#122876);
#101535=AXIS2_PLACEMENT_3D('',#223202,#122877,#122878);
#101536=AXIS2_PLACEMENT_3D('',#223204,#122879,#122880);
#101537=AXIS2_PLACEMENT_3D('',#223206,#122881,#122882);
#101538=AXIS2_PLACEMENT_3D('',#223208,#122883,#122884);
#101539=AXIS2_PLACEMENT_3D('',#223209,#122885,#122886);
#101540=AXIS2_PLACEMENT_3D('',#223210,#122887,#122888);
#101541=AXIS2_PLACEMENT_3D('',#223220,#122898,#122899);
#101542=AXIS2_PLACEMENT_3D('',#223222,#122901,#122902);
#101543=AXIS2_PLACEMENT_3D('',#223228,#122908,#122909);
#101544=AXIS2_PLACEMENT_3D('',#223232,#122912,#122913);
#101545=AXIS2_PLACEMENT_3D('',#223234,#122914,#122915);
#101546=AXIS2_PLACEMENT_3D('',#223235,#122916,#122917);
#101547=AXIS2_PLACEMENT_3D('',#223239,#122920,#122921);
#101548=AXIS2_PLACEMENT_3D('',#223241,#122922,#122923);
#101549=AXIS2_PLACEMENT_3D('',#223242,#122924,#122925);
#101550=AXIS2_PLACEMENT_3D('',#223245,#122928,#122929);
#101551=AXIS2_PLACEMENT_3D('',#223248,#122932,#122933);
#101552=AXIS2_PLACEMENT_3D('',#223251,#122936,#122937);
#101553=AXIS2_PLACEMENT_3D('',#223254,#122940,#122941);
#101554=AXIS2_PLACEMENT_3D('',#223258,#122945,#122946);
#101555=AXIS2_PLACEMENT_3D('',#223268,#122955,#122956);
#101556=AXIS2_PLACEMENT_3D('',#223270,#122957,#122958);
#101557=AXIS2_PLACEMENT_3D('',#223271,#122959,#122960);
#101558=AXIS2_PLACEMENT_3D('',#223274,#122962,#122963);
#101559=AXIS2_PLACEMENT_3D('',#223276,#122964,#122965);
#101560=AXIS2_PLACEMENT_3D('',#223277,#122966,#122967);
#101561=AXIS2_PLACEMENT_3D('',#223283,#122973,#122974);
#101562=AXIS2_PLACEMENT_3D('',#223292,#122983,#122984);
#101563=AXIS2_PLACEMENT_3D('',#223297,#122987,#122988);
#101564=AXIS2_PLACEMENT_3D('',#223298,#122989,#122990);
#101565=AXIS2_PLACEMENT_3D('',#223300,#122991,#122992);
#101566=AXIS2_PLACEMENT_3D('',#223302,#122994,#122995);
#101567=AXIS2_PLACEMENT_3D('',#223305,#122997,#122998);
#101568=AXIS2_PLACEMENT_3D('',#223306,#122999,#123000);
#101569=AXIS2_PLACEMENT_3D('',#223309,#123002,#123003);
#101570=AXIS2_PLACEMENT_3D('',#223310,#123004,#123005);
#101571=AXIS2_PLACEMENT_3D('',#223313,#123007,#123008);
#101572=AXIS2_PLACEMENT_3D('',#223314,#123009,#123010);
#101573=AXIS2_PLACEMENT_3D('',#223316,#123011,#123012);
#101574=AXIS2_PLACEMENT_3D('',#223318,#123014,#123015);
#101575=AXIS2_PLACEMENT_3D('',#223321,#123017,#123018);
#101576=AXIS2_PLACEMENT_3D('',#223322,#123019,#123020);
#101577=AXIS2_PLACEMENT_3D('',#223323,#123021,#123022);
#101578=AXIS2_PLACEMENT_3D('',#223324,#123023,#123024);
#101579=AXIS2_PLACEMENT_3D('',#223337,#123027,#123028);
#101580=AXIS2_PLACEMENT_3D('',#223338,#123029,#123030);
#101581=AXIS2_PLACEMENT_3D('',#223342,#123033,#123034);
#101582=AXIS2_PLACEMENT_3D('',#223345,#123035,#123036);
#101583=AXIS2_PLACEMENT_3D('',#223354,#123038,#123039);
#101584=AXIS2_PLACEMENT_3D('',#223363,#123041,#123042);
#101585=AXIS2_PLACEMENT_3D('',#223379,#123045,#123046);
#101586=AXIS2_PLACEMENT_3D('',#223395,#123049,#123050);
#101587=AXIS2_PLACEMENT_3D('',#223396,#123051,#123052);
#101588=AXIS2_PLACEMENT_3D('',#223397,#123053,#123054);
#101589=AXIS2_PLACEMENT_3D('',#223398,#123055,#123056);
#101590=AXIS2_PLACEMENT_3D('',#223414,#123059,#123060);
#101591=AXIS2_PLACEMENT_3D('',#223430,#123063,#123064);
#101592=AXIS2_PLACEMENT_3D('',#223431,#123065,#123066);
#101593=AXIS2_PLACEMENT_3D('',#223432,#123067,#123068);
#101594=AXIS2_PLACEMENT_3D('',#225923,#123069,#123070);
#101595=AXIS2_PLACEMENT_3D('',#225926,#123071,#123072);
#101596=AXIS2_PLACEMENT_3D('',#225930,#123074,#123075);
#101597=AXIS2_PLACEMENT_3D('',#225932,#123077,#123078);
#101598=AXIS2_PLACEMENT_3D('',#225933,#123079,#123080);
#101599=AXIS2_PLACEMENT_3D('',#225934,#123081,#123082);
#101600=AXIS2_PLACEMENT_3D('',#225935,#123083,#123084);
#101601=AXIS2_PLACEMENT_3D('',#225937,#123085,#123086);
#101602=AXIS2_PLACEMENT_3D('',#225940,#123088,#123089);
#101603=AXIS2_PLACEMENT_3D('',#225941,#123090,#123091);
#101604=AXIS2_PLACEMENT_3D('',#225942,#123092,#123093);
#101605=AXIS2_PLACEMENT_3D('',#225943,#123094,#123095);
#101606=AXIS2_PLACEMENT_3D('',#225945,#123096,#123097);
#101607=AXIS2_PLACEMENT_3D('',#225947,#123098,#123099);
#101608=AXIS2_PLACEMENT_3D('',#225949,#123101,#123102);
#101609=AXIS2_PLACEMENT_3D('',#225951,#123103,#123104);
#101610=AXIS2_PLACEMENT_3D('',#225953,#123105,#123106);
#101611=AXIS2_PLACEMENT_3D('',#225955,#123108,#123109);
#101612=AXIS2_PLACEMENT_3D('',#225957,#123110,#123111);
#101613=AXIS2_PLACEMENT_3D('',#225959,#123112,#123113);
#101614=AXIS2_PLACEMENT_3D('',#225961,#123115,#123116);
#101615=AXIS2_PLACEMENT_3D('',#225963,#123117,#123118);
#101616=AXIS2_PLACEMENT_3D('',#225971,#123119,#123120);
#101617=AXIS2_PLACEMENT_3D('',#225972,#123121,#123122);
#101618=AXIS2_PLACEMENT_3D('',#225975,#123123,#123124);
#101619=AXIS2_PLACEMENT_3D('',#225979,#123126,#123127);
#101620=AXIS2_PLACEMENT_3D('',#225981,#123129,#123130);
#101621=AXIS2_PLACEMENT_3D('',#225982,#123131,#123132);
#101622=AXIS2_PLACEMENT_3D('',#225983,#123133,#123134);
#101623=AXIS2_PLACEMENT_3D('',#228076,#123135,#123136);
#101624=AXIS2_PLACEMENT_3D('',#228079,#123137,#123138);
#101625=AXIS2_PLACEMENT_3D('',#228089,#123141,#123142);
#101626=AXIS2_PLACEMENT_3D('',#228099,#123143,#123144);
#101627=AXIS2_PLACEMENT_3D('',#228108,#123146,#123147);
#101628=AXIS2_PLACEMENT_3D('',#228110,#123148,#123149);
#101629=AXIS2_PLACEMENT_3D('',#228112,#123151,#123152);
#101630=AXIS2_PLACEMENT_3D('',#228113,#123153,#123154);
#101631=AXIS2_PLACEMENT_3D('',#228116,#123155,#123156);
#101632=AXIS2_PLACEMENT_3D('',#228119,#123158,#123159);
#101633=AXIS2_PLACEMENT_3D('',#228121,#123161,#123162);
#101634=AXIS2_PLACEMENT_3D('',#228129,#123163,#123164);
#101635=AXIS2_PLACEMENT_3D('',#228140,#123166,#123167);
#101636=AXIS2_PLACEMENT_3D('',#228142,#123168,#123169);
#101637=AXIS2_PLACEMENT_3D('',#228144,#123171,#123172);
#101638=AXIS2_PLACEMENT_3D('',#228145,#123173,#123174);
#101639=AXIS2_PLACEMENT_3D('',#228146,#123175,#123176);
#101640=AXIS2_PLACEMENT_3D('',#228153,#123177,#123178);
#101641=AXIS2_PLACEMENT_3D('',#228155,#123179,#123180);
#101642=AXIS2_PLACEMENT_3D('',#228157,#123181,#123182);
#101643=AXIS2_PLACEMENT_3D('',#228159,#123183,#123184);
#101644=AXIS2_PLACEMENT_3D('',#228161,#123185,#123186);
#101645=AXIS2_PLACEMENT_3D('',#228163,#123187,#123188);
#101646=AXIS2_PLACEMENT_3D('',#228165,#123189,#123190);
#101647=AXIS2_PLACEMENT_3D('',#228167,#123191,#123192);
#101648=AXIS2_PLACEMENT_3D('',#228169,#123193,#123194);
#101649=AXIS2_PLACEMENT_3D('',#228170,#123195,#123196);
#101650=AXIS2_PLACEMENT_3D('',#228171,#123197,#123198);
#101651=AXIS2_PLACEMENT_3D('',#228172,#123199,#123200);
#101652=AXIS2_PLACEMENT_3D('',#228173,#123201,#123202);
#101653=AXIS2_PLACEMENT_3D('',#228176,#123203,#123204);
#101654=AXIS2_PLACEMENT_3D('',#228179,#123207,#123208);
#101655=AXIS2_PLACEMENT_3D('',#228181,#123209,#123210);
#101656=AXIS2_PLACEMENT_3D('',#228183,#123212,#123213);
#101657=AXIS2_PLACEMENT_3D('',#228185,#123214,#123215);
#101658=AXIS2_PLACEMENT_3D('',#228187,#123217,#123218);
#101659=AXIS2_PLACEMENT_3D('',#228189,#123219,#123220);
#101660=AXIS2_PLACEMENT_3D('',#228191,#123222,#123223);
#101661=AXIS2_PLACEMENT_3D('',#228192,#123224,#123225);
#101662=AXIS2_PLACEMENT_3D('',#228193,#123226,#123227);
#101663=AXIS2_PLACEMENT_3D('',#228195,#123228,#123229);
#101664=AXIS2_PLACEMENT_3D('',#228197,#123231,#123232);
#101665=AXIS2_PLACEMENT_3D('',#228199,#123233,#123234);
#101666=AXIS2_PLACEMENT_3D('',#228201,#123236,#123237);
#101667=AXIS2_PLACEMENT_3D('',#228203,#123238,#123239);
#101668=AXIS2_PLACEMENT_3D('',#228205,#123241,#123242);
#101669=AXIS2_PLACEMENT_3D('',#228206,#123243,#123244);
#101670=AXIS2_PLACEMENT_3D('',#228279,#123245,#123246);
#101671=AXIS2_PLACEMENT_3D('',#228477,#123247,#123248);
#101672=AXIS2_PLACEMENT_3D('',#228484,#123249,#123250);
#101673=AXIS2_PLACEMENT_3D('',#228485,#123251,#123252);
#101674=AXIS2_PLACEMENT_3D('',#228487,#123253,#123254);
#101675=AXIS2_PLACEMENT_3D('',#228488,#123255,#123256);
#101676=AXIS2_PLACEMENT_3D('',#228489,#123257,#123258);
#101677=AXIS2_PLACEMENT_3D('',#228528,#123259,#123260);
#101678=AXIS2_PLACEMENT_3D('',#228537,#123261,#123262);
#101679=AXIS2_PLACEMENT_3D('',#228805,#123263,#123264);
#101680=AXIS2_PLACEMENT_3D('',#228814,#123265,#123266);
#101681=AXIS2_PLACEMENT_3D('',#229138,#123267,#123268);
#101682=AXIS2_PLACEMENT_3D('',#229139,#123269,#123270);
#101683=AXIS2_PLACEMENT_3D('',#229140,#123271,#123272);
#101684=AXIS2_PLACEMENT_3D('',#229147,#123273,#123274);
#101685=AXIS2_PLACEMENT_3D('',#229150,#123275,#123276);
#101686=AXIS2_PLACEMENT_3D('',#229157,#123277,#123278);
#101687=AXIS2_PLACEMENT_3D('',#229160,#123279,#123280);
#101688=AXIS2_PLACEMENT_3D('',#229167,#123281,#123282);
#101689=AXIS2_PLACEMENT_3D('',#229170,#123283,#123284);
#101690=AXIS2_PLACEMENT_3D('',#229177,#123285,#123286);
#101691=AXIS2_PLACEMENT_3D('',#229178,#123287,#123288);
#101692=AXIS2_PLACEMENT_3D('',#229179,#123289,#123290);
#101693=AXIS2_PLACEMENT_3D('',#229180,#123291,#123292);
#101694=AXIS2_PLACEMENT_3D('',#229183,#123294,#123295);
#101695=AXIS2_PLACEMENT_3D('',#229184,#123296,#123297);
#101696=AXIS2_PLACEMENT_3D('',#229203,#123298,#123299);
#101697=AXIS2_PLACEMENT_3D('',#229204,#123300,#123301);
#101698=AXIS2_PLACEMENT_3D('',#229207,#123302,#123303);
#101699=AXIS2_PLACEMENT_3D('',#229222,#123304,#123305);
#101700=AXIS2_PLACEMENT_3D('',#229230,#123306,#123307);
#101701=AXIS2_PLACEMENT_3D('',#229231,#123308,#123309);
#101702=AXIS2_PLACEMENT_3D('',#229234,#123310,#123311);
#101703=AXIS2_PLACEMENT_3D('',#229251,#123312,#123313);
#101704=AXIS2_PLACEMENT_3D('',#229252,#123314,#123315);
#101705=AXIS2_PLACEMENT_3D('',#229253,#123316,#123317);
#101706=AXIS2_PLACEMENT_3D('',#229255,#123319,#123320);
#101707=AXIS2_PLACEMENT_3D('',#229257,#123322,#123323);
#101708=AXIS2_PLACEMENT_3D('',#230391,#123324,#123325);
#101709=AXIS2_PLACEMENT_3D('',#230392,#123326,#123327);
#101710=AXIS2_PLACEMENT_3D('',#230395,#123330,#123331);
#101711=AXIS2_PLACEMENT_3D('',#230397,#123333,#123334);
#101712=AXIS2_PLACEMENT_3D('',#230399,#123336,#123337);
#101713=AXIS2_PLACEMENT_3D('',#230400,#123338,#123339);
#101714=AXIS2_PLACEMENT_3D('',#230403,#123342,#123343);
#101715=AXIS2_PLACEMENT_3D('',#230404,#123344,#123345);
#101716=AXIS2_PLACEMENT_3D('',#230407,#123348,#123349);
#101717=AXIS2_PLACEMENT_3D('',#230409,#123350,#123351);
#101718=AXIS2_PLACEMENT_3D('',#230410,#123352,#123353);
#101719=AXIS2_PLACEMENT_3D('',#230412,#123355,#123356);
#101720=AXIS2_PLACEMENT_3D('',#230414,#123357,#123358);
#101721=AXIS2_PLACEMENT_3D('',#230415,#123359,#123360);
#101722=AXIS2_PLACEMENT_3D('',#230417,#123362,#123363);
#101723=AXIS2_PLACEMENT_3D('',#230418,#123364,#123365);
#101724=AXIS2_PLACEMENT_3D('',#230419,#123366,#123367);
#101725=AXIS2_PLACEMENT_3D('',#230420,#123368,#123369);
#101726=AXIS2_PLACEMENT_3D('',#230421,#123370,#123371);
#101727=AXIS2_PLACEMENT_3D('',#230422,#123372,#123373);
#101728=AXIS2_PLACEMENT_3D('',#230423,#123374,#123375);
#101729=AXIS2_PLACEMENT_3D('',#230424,#123376,#123377);
#101730=AXIS2_PLACEMENT_3D('',#230425,#123378,#123379);
#101731=AXIS2_PLACEMENT_3D('',#230426,#123380,#123381);
#101732=AXIS2_PLACEMENT_3D('',#230427,#123382,#123383);
#101733=AXIS2_PLACEMENT_3D('',#230428,#123384,#123385);
#101734=AXIS2_PLACEMENT_3D('',#230429,#123386,#123387);
#101735=AXIS2_PLACEMENT_3D('',#230430,#123388,#123389);
#101736=AXIS2_PLACEMENT_3D('',#230767,#123390,#123391);
#101737=AXIS2_PLACEMENT_3D('',#230768,#123392,#123393);
#101738=AXIS2_PLACEMENT_3D('',#230773,#123396,#123397);
#101739=AXIS2_PLACEMENT_3D('',#230774,#123398,#123399);
#101740=AXIS2_PLACEMENT_3D('',#230777,#123401,#123402);
#101741=AXIS2_PLACEMENT_3D('',#230778,#123403,#123404);
#101742=AXIS2_PLACEMENT_3D('',#230781,#123406,#123407);
#101743=AXIS2_PLACEMENT_3D('',#230782,#123408,#123409);
#101744=AXIS2_PLACEMENT_3D('',#230785,#123411,#123412);
#101745=AXIS2_PLACEMENT_3D('',#230786,#123413,#123414);
#101746=AXIS2_PLACEMENT_3D('',#230789,#123416,#123417);
#101747=AXIS2_PLACEMENT_3D('',#230790,#123418,#123419);
#101748=AXIS2_PLACEMENT_3D('',#230793,#123421,#123422);
#101749=AXIS2_PLACEMENT_3D('',#230794,#123423,#123424);
#101750=AXIS2_PLACEMENT_3D('',#230795,#123425,#123426);
#101751=AXIS2_PLACEMENT_3D('',#230796,#123427,#123428);
#101752=AXIS2_PLACEMENT_3D('',#230798,#123429,#123430);
#101753=AXIS2_PLACEMENT_3D('',#230800,#123432,#123433);
#101754=AXIS2_PLACEMENT_3D('',#230801,#123434,#123435);
#101755=AXIS2_PLACEMENT_3D('',#230802,#123436,#123437);
#101756=AXIS2_PLACEMENT_3D('',#230804,#123438,#123439);
#101757=AXIS2_PLACEMENT_3D('',#230806,#123440,#123441);
#101758=AXIS2_PLACEMENT_3D('',#230808,#123442,#123443);
#101759=AXIS2_PLACEMENT_3D('',#230810,#123444,#123445);
#101760=AXIS2_PLACEMENT_3D('',#230812,#123446,#123447);
#101761=AXIS2_PLACEMENT_3D('',#230814,#123448,#123449);
#101762=AXIS2_PLACEMENT_3D('',#230816,#123450,#123451);
#101763=AXIS2_PLACEMENT_3D('',#230818,#123452,#123453);
#101764=AXIS2_PLACEMENT_3D('',#230819,#123454,#123455);
#101765=AXIS2_PLACEMENT_3D('',#230820,#123456,#123457);
#101766=AXIS2_PLACEMENT_3D('',#230823,#123460,#123461);
#101767=AXIS2_PLACEMENT_3D('',#230824,#123462,#123463);
#101768=AXIS2_PLACEMENT_3D('',#230826,#123465,#123466);
#101769=AXIS2_PLACEMENT_3D('',#230828,#123468,#123469);
#101770=AXIS2_PLACEMENT_3D('',#230830,#123471,#123472);
#101771=AXIS2_PLACEMENT_3D('',#230832,#123474,#123475);
#101772=AXIS2_PLACEMENT_3D('',#230834,#123477,#123478);
#101773=AXIS2_PLACEMENT_3D('',#230836,#123480,#123481);
#101774=AXIS2_PLACEMENT_3D('',#231228,#123486,#123487);
#101775=AXIS2_PLACEMENT_3D('',#231231,#123490,#123491);
#101776=AXIS2_PLACEMENT_3D('',#231233,#123493,#123494);
#101777=AXIS2_PLACEMENT_3D('',#231235,#123496,#123497);
#101778=AXIS2_PLACEMENT_3D('',#231238,#123500,#123501);
#101779=AXIS2_PLACEMENT_3D('',#231240,#123503,#123504);
#101780=AXIS2_PLACEMENT_3D('',#231242,#123506,#123507);
#101781=AXIS2_PLACEMENT_3D('',#231243,#123508,#123509);
#101782=AXIS2_PLACEMENT_3D('',#231245,#123510,#123511);
#101783=AXIS2_PLACEMENT_3D('',#231247,#123512,#123513);
#101784=AXIS2_PLACEMENT_3D('',#231249,#123514,#123515);
#101785=AXIS2_PLACEMENT_3D('',#231251,#123516,#123517);
#101786=AXIS2_PLACEMENT_3D('',#231253,#123518,#123519);
#101787=AXIS2_PLACEMENT_3D('',#231255,#123520,#123521);
#101788=AXIS2_PLACEMENT_3D('',#231257,#123522,#123523);
#101789=AXIS2_PLACEMENT_3D('',#231259,#123524,#123525);
#101790=AXIS2_PLACEMENT_3D('',#231260,#123526,#123527);
#101791=AXIS2_PLACEMENT_3D('',#231261,#123528,#123529);
#101792=AXIS2_PLACEMENT_3D('',#231262,#123530,#123531);
#101793=AXIS2_PLACEMENT_3D('',#231265,#123534,#123535);
#101794=AXIS2_PLACEMENT_3D('',#231267,#123537,#123538);
#101795=AXIS2_PLACEMENT_3D('',#231269,#123540,#123541);
#101796=AXIS2_PLACEMENT_3D('',#231271,#123543,#123544);
#101797=AXIS2_PLACEMENT_3D('',#231272,#123545,#123546);
#101798=AXIS2_PLACEMENT_3D('',#231274,#123548,#123549);
#101799=AXIS2_PLACEMENT_3D('',#231276,#123551,#123552);
#101800=AXIS2_PLACEMENT_3D('',#231278,#123554,#123555);
#101801=AXIS2_PLACEMENT_3D('',#231356,#123556,#123557);
#101802=AXIS2_PLACEMENT_3D('',#231406,#123558,#123559);
#101803=AXIS2_PLACEMENT_3D('',#231407,#123560,#123561);
#101804=AXIS2_PLACEMENT_3D('',#231457,#123562,#123563);
#101805=AXIS2_PLACEMENT_3D('',#232146,#123564,#123565);
#101806=AXIS2_PLACEMENT_3D('',#232739,#123566,#123567);
#101807=AXIS2_PLACEMENT_3D('',#232740,#123568,#123569);
#101808=AXIS2_PLACEMENT_3D('',#232741,#123570,#123571);
#101809=AXIS2_PLACEMENT_3D('',#232742,#123572,#123573);
#101810=AXIS2_PLACEMENT_3D('',#232743,#123574,#123575);
#101811=AXIS2_PLACEMENT_3D('',#232744,#123576,#123577);
#101812=AXIS2_PLACEMENT_3D('',#232745,#123578,#123579);
#101813=AXIS2_PLACEMENT_3D('',#232746,#123580,#123581);
#101814=AXIS2_PLACEMENT_3D('',#232747,#123582,#123583);
#101815=AXIS2_PLACEMENT_3D('',#232748,#123584,#123585);
#101816=AXIS2_PLACEMENT_3D('',#232749,#123586,#123587);
#101817=AXIS2_PLACEMENT_3D('',#232750,#123588,#123589);
#101818=AXIS2_PLACEMENT_3D('',#232751,#123590,#123591);
#101819=AXIS2_PLACEMENT_3D('',#232752,#123592,#123593);
#101820=AXIS2_PLACEMENT_3D('',#232753,#123594,#123595);
#101821=AXIS2_PLACEMENT_3D('',#232754,#123596,#123597);
#101822=AXIS2_PLACEMENT_3D('',#232755,#123598,#123599);
#101823=AXIS2_PLACEMENT_3D('',#232756,#123600,#123601);
#101824=AXIS2_PLACEMENT_3D('',#232757,#123602,#123603);
#101825=AXIS2_PLACEMENT_3D('',#232758,#123604,#123605);
#101826=AXIS2_PLACEMENT_3D('',#232759,#123606,#123607);
#101827=AXIS2_PLACEMENT_3D('',#232760,#123608,#123609);
#101828=AXIS2_PLACEMENT_3D('',#232761,#123610,#123611);
#101829=AXIS2_PLACEMENT_3D('',#232762,#123612,#123613);
#101830=AXIS2_PLACEMENT_3D('',#232763,#123614,#123615);
#101831=AXIS2_PLACEMENT_3D('',#232764,#123616,#123617);
#101832=AXIS2_PLACEMENT_3D('',#232765,#123618,#123619);
#101833=AXIS2_PLACEMENT_3D('',#232766,#123620,#123621);
#101834=AXIS2_PLACEMENT_3D('',#232767,#123622,#123623);
#101835=AXIS2_PLACEMENT_3D('',#232768,#123624,#123625);
#101836=AXIS2_PLACEMENT_3D('',#232769,#123626,#123627);
#101837=AXIS2_PLACEMENT_3D('',#232770,#123628,#123629);
#101838=AXIS2_PLACEMENT_3D('',#232771,#123630,#123631);
#101839=AXIS2_PLACEMENT_3D('',#232772,#123632,#123633);
#101840=AXIS2_PLACEMENT_3D('',#232773,#123634,#123635);
#101841=AXIS2_PLACEMENT_3D('',#232774,#123636,#123637);
#101842=AXIS2_PLACEMENT_3D('',#232775,#123638,#123639);
#101843=AXIS2_PLACEMENT_3D('',#232776,#123640,#123641);
#101844=AXIS2_PLACEMENT_3D('',#232777,#123642,#123643);
#101845=AXIS2_PLACEMENT_3D('',#232778,#123644,#123645);
#101846=AXIS2_PLACEMENT_3D('',#232779,#123646,#123647);
#101847=AXIS2_PLACEMENT_3D('',#232780,#123648,#123649);
#101848=AXIS2_PLACEMENT_3D('',#232781,#123650,#123651);
#101849=AXIS2_PLACEMENT_3D('',#232782,#123652,#123653);
#101850=AXIS2_PLACEMENT_3D('',#232783,#123654,#123655);
#101851=AXIS2_PLACEMENT_3D('',#232784,#123656,#123657);
#101852=AXIS2_PLACEMENT_3D('',#232785,#123658,#123659);
#101853=AXIS2_PLACEMENT_3D('',#232786,#123660,#123661);
#101854=AXIS2_PLACEMENT_3D('',#232787,#123662,#123663);
#101855=AXIS2_PLACEMENT_3D('',#232788,#123664,#123665);
#101856=AXIS2_PLACEMENT_3D('',#232789,#123666,#123667);
#101857=AXIS2_PLACEMENT_3D('',#232790,#123668,#123669);
#101858=AXIS2_PLACEMENT_3D('',#232791,#123670,#123671);
#101859=AXIS2_PLACEMENT_3D('',#232792,#123672,#123673);
#101860=AXIS2_PLACEMENT_3D('',#232793,#123674,#123675);
#101861=AXIS2_PLACEMENT_3D('',#232794,#123676,#123677);
#101862=AXIS2_PLACEMENT_3D('',#232795,#123678,#123679);
#101863=AXIS2_PLACEMENT_3D('',#232796,#123680,#123681);
#101864=AXIS2_PLACEMENT_3D('',#232797,#123682,#123683);
#101865=AXIS2_PLACEMENT_3D('',#232798,#123684,#123685);
#101866=AXIS2_PLACEMENT_3D('',#232799,#123686,#123687);
#101867=AXIS2_PLACEMENT_3D('',#232800,#123688,#123689);
#101868=AXIS2_PLACEMENT_3D('',#232801,#123690,#123691);
#101869=AXIS2_PLACEMENT_3D('',#232802,#123692,#123693);
#101870=AXIS2_PLACEMENT_3D('',#232803,#123694,#123695);
#101871=AXIS2_PLACEMENT_3D('',#232804,#123696,#123697);
#101872=AXIS2_PLACEMENT_3D('',#232805,#123698,#123699);
#101873=AXIS2_PLACEMENT_3D('',#232806,#123700,#123701);
#101874=AXIS2_PLACEMENT_3D('',#232807,#123702,#123703);
#101875=AXIS2_PLACEMENT_3D('',#232808,#123704,#123705);
#101876=AXIS2_PLACEMENT_3D('',#232809,#123706,#123707);
#101877=AXIS2_PLACEMENT_3D('',#232810,#123708,#123709);
#101878=AXIS2_PLACEMENT_3D('',#232811,#123710,#123711);
#101879=AXIS2_PLACEMENT_3D('',#232812,#123712,#123713);
#101880=AXIS2_PLACEMENT_3D('',#232825,#123716,#123717);
#101881=AXIS2_PLACEMENT_3D('',#232835,#123719,#123720);
#101882=AXIS2_PLACEMENT_3D('',#232845,#123722,#123723);
#101883=AXIS2_PLACEMENT_3D('',#232855,#123725,#123726);
#101884=AXIS2_PLACEMENT_3D('',#232865,#123728,#123729);
#101885=AXIS2_PLACEMENT_3D('',#232872,#123730,#123731);
#101886=AXIS2_PLACEMENT_3D('',#232875,#123733,#123734);
#101887=AXIS2_PLACEMENT_3D('',#232876,#123735,#123736);
#101888=AXIS2_PLACEMENT_3D('',#232877,#123737,#123738);
#101889=AXIS2_PLACEMENT_3D('',#232878,#123739,#123740);
#101890=AXIS2_PLACEMENT_3D('',#232879,#123741,#123742);
#101891=AXIS2_PLACEMENT_3D('',#232880,#123743,#123744);
#101892=AXIS2_PLACEMENT_3D('',#232881,#123745,#123746);
#101893=AXIS2_PLACEMENT_3D('',#232882,#123747,#123748);
#101894=AXIS2_PLACEMENT_3D('',#232883,#123749,#123750);
#101895=AXIS2_PLACEMENT_3D('',#232884,#123751,#123752);
#101896=AXIS2_PLACEMENT_3D('',#232885,#123753,#123754);
#101897=AXIS2_PLACEMENT_3D('',#232886,#123755,#123756);
#101898=AXIS2_PLACEMENT_3D('',#232887,#123757,#123758);
#101899=AXIS2_PLACEMENT_3D('',#232889,#123759,#123760);
#101900=AXIS2_PLACEMENT_3D('',#232891,#123761,#123762);
#101901=AXIS2_PLACEMENT_3D('',#232893,#123763,#123764);
#101902=AXIS2_PLACEMENT_3D('',#232894,#123765,#123766);
#101903=AXIS2_PLACEMENT_3D('',#232895,#123767,#123768);
#101904=AXIS2_PLACEMENT_3D('',#232897,#123769,#123770);
#101905=AXIS2_PLACEMENT_3D('',#232898,#123771,#123772);
#101906=AXIS2_PLACEMENT_3D('',#232899,#123773,#123774);
#101907=AXIS2_PLACEMENT_3D('',#232901,#123776,#123777);
#101908=AXIS2_PLACEMENT_3D('',#232904,#123778,#123779);
#101909=AXIS2_PLACEMENT_3D('',#232906,#123780,#123781);
#101910=AXIS2_PLACEMENT_3D('',#232908,#123782,#123783);
#101911=AXIS2_PLACEMENT_3D('',#232910,#123784,#123785);
#101912=AXIS2_PLACEMENT_3D('',#232912,#123786,#123787);
#101913=AXIS2_PLACEMENT_3D('',#232913,#123788,#123789);
#101914=AXIS2_PLACEMENT_3D('',#232914,#123790,#123791);
#101915=AXIS2_PLACEMENT_3D('',#232922,#123792,#123793);
#101916=AXIS2_PLACEMENT_3D('',#232930,#123794,#123795);
#101917=AXIS2_PLACEMENT_3D('',#232938,#123796,#123797);
#101918=AXIS2_PLACEMENT_3D('',#232946,#123798,#123799);
#101919=AXIS2_PLACEMENT_3D('',#232954,#123800,#123801);
#101920=AXIS2_PLACEMENT_3D('',#232962,#123802,#123803);
#101921=AXIS2_PLACEMENT_3D('',#232965,#123804,#123805);
#101922=AXIS2_PLACEMENT_3D('',#232967,#123806,#123807);
#101923=AXIS2_PLACEMENT_3D('',#232969,#123808,#123809);
#101924=AXIS2_PLACEMENT_3D('',#232971,#123810,#123811);
#101925=AXIS2_PLACEMENT_3D('',#232973,#123812,#123813);
#101926=AXIS2_PLACEMENT_3D('',#232974,#123814,#123815);
#101927=AXIS2_PLACEMENT_3D('',#232975,#123816,#123817);
#101928=AXIS2_PLACEMENT_3D('',#232983,#123818,#123819);
#101929=AXIS2_PLACEMENT_3D('',#232991,#123820,#123821);
#101930=AXIS2_PLACEMENT_3D('',#232999,#123822,#123823);
#101931=AXIS2_PLACEMENT_3D('',#233007,#123824,#123825);
#101932=AXIS2_PLACEMENT_3D('',#233015,#123826,#123827);
#101933=AXIS2_PLACEMENT_3D('',#233023,#123828,#123829);
#101934=AXIS2_PLACEMENT_3D('',#233026,#123832,#123833);
#101935=AXIS2_PLACEMENT_3D('',#233028,#123835,#123836);
#101936=AXIS2_PLACEMENT_3D('',#233030,#123838,#123839);
#101937=AXIS2_PLACEMENT_3D('',#233032,#123841,#123842);
#101938=AXIS2_PLACEMENT_3D('',#233034,#123844,#123845);
#101939=AXIS2_PLACEMENT_3D('',#233035,#123846,#123847);
#101940=AXIS2_PLACEMENT_3D('',#233038,#123848,#123849);
#101941=AXIS2_PLACEMENT_3D('',#233040,#123850,#123851);
#101942=AXIS2_PLACEMENT_3D('',#233042,#123852,#123853);
#101943=AXIS2_PLACEMENT_3D('',#233044,#123854,#123855);
#101944=AXIS2_PLACEMENT_3D('',#233046,#123856,#123857);
#101945=AXIS2_PLACEMENT_3D('',#233047,#123858,#123859);
#101946=AXIS2_PLACEMENT_3D('',#233048,#123860,#123861);
#101947=AXIS2_PLACEMENT_3D('',#233056,#123862,#123863);
#101948=AXIS2_PLACEMENT_3D('',#233064,#123864,#123865);
#101949=AXIS2_PLACEMENT_3D('',#233072,#123866,#123867);
#101950=AXIS2_PLACEMENT_3D('',#233080,#123868,#123869);
#101951=AXIS2_PLACEMENT_3D('',#233088,#123870,#123871);
#101952=AXIS2_PLACEMENT_3D('',#233096,#123872,#123873);
#101953=AXIS2_PLACEMENT_3D('',#233099,#123874,#123875);
#101954=AXIS2_PLACEMENT_3D('',#233101,#123876,#123877);
#101955=AXIS2_PLACEMENT_3D('',#233103,#123878,#123879);
#101956=AXIS2_PLACEMENT_3D('',#233105,#123880,#123881);
#101957=AXIS2_PLACEMENT_3D('',#233107,#123882,#123883);
#101958=AXIS2_PLACEMENT_3D('',#233108,#123884,#123885);
#101959=AXIS2_PLACEMENT_3D('',#233109,#123886,#123887);
#101960=AXIS2_PLACEMENT_3D('',#233117,#123888,#123889);
#101961=AXIS2_PLACEMENT_3D('',#233125,#123890,#123891);
#101962=AXIS2_PLACEMENT_3D('',#233133,#123892,#123893);
#101963=AXIS2_PLACEMENT_3D('',#233141,#123894,#123895);
#101964=AXIS2_PLACEMENT_3D('',#233149,#123896,#123897);
#101965=AXIS2_PLACEMENT_3D('',#233157,#123898,#123899);
#101966=AXIS2_PLACEMENT_3D('',#233160,#123902,#123903);
#101967=AXIS2_PLACEMENT_3D('',#233162,#123905,#123906);
#101968=AXIS2_PLACEMENT_3D('',#233164,#123908,#123909);
#101969=AXIS2_PLACEMENT_3D('',#233166,#123911,#123912);
#101970=AXIS2_PLACEMENT_3D('',#233168,#123914,#123915);
#101971=AXIS2_PLACEMENT_3D('',#233169,#123916,#123917);
#101972=AXIS2_PLACEMENT_3D('',#233182,#123920,#123921);
#101973=AXIS2_PLACEMENT_3D('',#233192,#123923,#123924);
#101974=AXIS2_PLACEMENT_3D('',#233202,#123926,#123927);
#101975=AXIS2_PLACEMENT_3D('',#233212,#123929,#123930);
#101976=AXIS2_PLACEMENT_3D('',#233222,#123932,#123933);
#101977=AXIS2_PLACEMENT_3D('',#233229,#123934,#123935);
#101978=AXIS2_PLACEMENT_3D('',#233232,#123937,#123938);
#101979=AXIS2_PLACEMENT_3D('',#233233,#123939,#123940);
#101980=AXIS2_PLACEMENT_3D('',#233234,#123941,#123942);
#101981=AXIS2_PLACEMENT_3D('',#233235,#123943,#123944);
#101982=AXIS2_PLACEMENT_3D('',#233236,#123945,#123946);
#101983=AXIS2_PLACEMENT_3D('',#233237,#123947,#123948);
#101984=AXIS2_PLACEMENT_3D('',#233238,#123949,#123950);
#101985=AXIS2_PLACEMENT_3D('',#233239,#123951,#123952);
#101986=AXIS2_PLACEMENT_3D('',#233240,#123953,#123954);
#101987=AXIS2_PLACEMENT_3D('',#233241,#123955,#123956);
#101988=AXIS2_PLACEMENT_3D('',#233242,#123957,#123958);
#101989=AXIS2_PLACEMENT_3D('',#233243,#123959,#123960);
#101990=AXIS2_PLACEMENT_3D('',#233244,#123961,#123962);
#101991=AXIS2_PLACEMENT_3D('',#233246,#123963,#123964);
#101992=AXIS2_PLACEMENT_3D('',#233248,#123965,#123966);
#101993=AXIS2_PLACEMENT_3D('',#233250,#123967,#123968);
#101994=AXIS2_PLACEMENT_3D('',#233251,#123969,#123970);
#101995=AXIS2_PLACEMENT_3D('',#233252,#123971,#123972);
#101996=AXIS2_PLACEMENT_3D('',#233254,#123973,#123974);
#101997=AXIS2_PLACEMENT_3D('',#233255,#123975,#123976);
#101998=AXIS2_PLACEMENT_3D('',#233256,#123977,#123978);
#101999=AXIS2_PLACEMENT_3D('',#233258,#123980,#123981);
#102000=AXIS2_PLACEMENT_3D('',#233260,#123982,#123983);
#102001=AXIS2_PLACEMENT_3D('',#233263,#123984,#123985);
#102002=AXIS2_PLACEMENT_3D('',#233284,#123986,#123987);
#102003=AXIS2_PLACEMENT_3D('',#233303,#123988,#123989);
#102004=AXIS2_PLACEMENT_3D('',#233306,#123990,#123991);
#102005=AXIS2_PLACEMENT_3D('',#233307,#123992,#123993);
#102006=AXIS2_PLACEMENT_3D('',#233308,#123994,#123995);
#102007=AXIS2_PLACEMENT_3D('',#233309,#123996,#123997);
#102008=AXIS2_PLACEMENT_3D('',#233311,#123998,#123999);
#102009=AXIS2_PLACEMENT_3D('',#233313,#124000,#124001);
#102010=AXIS2_PLACEMENT_3D('',#233315,#124002,#124003);
#102011=AXIS2_PLACEMENT_3D('',#233316,#124004,#124005);
#102012=AXIS2_PLACEMENT_3D('',#233317,#124006,#124007);
#102013=AXIS2_PLACEMENT_3D('',#233320,#124008,#124009);
#102014=AXIS2_PLACEMENT_3D('',#233324,#124011,#124012);
#102015=AXIS2_PLACEMENT_3D('',#233326,#124014,#124015);
#102016=AXIS2_PLACEMENT_3D('',#233329,#124018,#124019);
#102017=AXIS2_PLACEMENT_3D('',#233331,#124021,#124022);
#102018=AXIS2_PLACEMENT_3D('',#233333,#124024,#124025);
#102019=AXIS2_PLACEMENT_3D('',#233334,#124026,#124027);
#102020=AXIS2_PLACEMENT_3D('',#233336,#124028,#124029);
#102021=AXIS2_PLACEMENT_3D('',#233337,#124030,#124031);
#102022=AXIS2_PLACEMENT_3D('',#233339,#124032,#124033);
#102023=AXIS2_PLACEMENT_3D('',#233341,#124035,#124036);
#102024=AXIS2_PLACEMENT_3D('',#233343,#124038,#124039);
#102025=AXIS2_PLACEMENT_3D('',#233344,#124040,#124041);
#102026=AXIS2_PLACEMENT_3D('',#233346,#124042,#124043);
#102027=AXIS2_PLACEMENT_3D('',#233349,#124045,#124046);
#102028=AXIS2_PLACEMENT_3D('',#233350,#124047,#124048);
#102029=AXIS2_PLACEMENT_3D('',#233351,#124049,#124050);
#102030=AXIS2_PLACEMENT_3D('',#233353,#124051,#124052);
#102031=AXIS2_PLACEMENT_3D('',#233355,#124054,#124055);
#102032=AXIS2_PLACEMENT_3D('',#233357,#124056,#124057);
#102033=AXIS2_PLACEMENT_3D('',#233358,#124058,#124059);
#102034=AXIS2_PLACEMENT_3D('',#233360,#124060,#124061);
#102035=AXIS2_PLACEMENT_3D('',#233362,#124063,#124064);
#102036=AXIS2_PLACEMENT_3D('',#233363,#124065,#124066);
#102037=AXIS2_PLACEMENT_3D('',#233366,#124067,#124068);
#102038=AXIS2_PLACEMENT_3D('',#233368,#124069,#124070);
#102039=AXIS2_PLACEMENT_3D('',#233370,#124071,#124072);
#102040=AXIS2_PLACEMENT_3D('',#233371,#124073,#124074);
#102041=AXIS2_PLACEMENT_3D('',#233372,#124075,#124076);
#102042=AXIS2_PLACEMENT_3D('',#233375,#124077,#124078);
#102043=AXIS2_PLACEMENT_3D('',#233378,#124081,#124082);
#102044=AXIS2_PLACEMENT_3D('',#233381,#124083,#124084);
#102045=AXIS2_PLACEMENT_3D('',#233384,#124087,#124088);
#102046=AXIS2_PLACEMENT_3D('',#233387,#124089,#124090);
#102047=AXIS2_PLACEMENT_3D('',#233388,#124091,#124092);
#102048=AXIS2_PLACEMENT_3D('',#233389,#124093,#124094);
#102049=AXIS2_PLACEMENT_3D('',#233390,#124095,#124096);
#102050=AXIS2_PLACEMENT_3D('',#233393,#124097,#124098);
#102051=AXIS2_PLACEMENT_3D('',#233394,#124099,#124100);
#102052=AXIS2_PLACEMENT_3D('',#233395,#124101,#124102);
#102053=AXIS2_PLACEMENT_3D('',#233396,#124103,#124104);
#102054=AXIS2_PLACEMENT_3D('',#233399,#124105,#124106);
#102055=AXIS2_PLACEMENT_3D('',#233402,#124109,#124110);
#102056=AXIS2_PLACEMENT_3D('',#233405,#124111,#124112);
#102057=AXIS2_PLACEMENT_3D('',#233408,#124115,#124116);
#102058=AXIS2_PLACEMENT_3D('',#233409,#124117,#124118);
#102059=AXIS2_PLACEMENT_3D('',#233410,#124119,#124120);
#102060=AXIS2_PLACEMENT_3D('',#233411,#124121,#124122);
#102061=AXIS2_PLACEMENT_3D('',#233417,#124126,#124127);
#102062=AXIS2_PLACEMENT_3D('',#233420,#124129,#124130);
#102063=AXIS2_PLACEMENT_3D('',#233421,#124131,#124132);
#102064=AXIS2_PLACEMENT_3D('',#233424,#124134,#124135);
#102065=AXIS2_PLACEMENT_3D('',#233425,#124136,#124137);
#102066=AXIS2_PLACEMENT_3D('',#233435,#124142,#124143);
#102067=AXIS2_PLACEMENT_3D('',#233437,#124144,#124145);
#102068=AXIS2_PLACEMENT_3D('',#233438,#124146,#124147);
#102069=AXIS2_PLACEMENT_3D('',#233440,#124148,#124149);
#102070=AXIS2_PLACEMENT_3D('',#233442,#124150,#124151);
#102071=AXIS2_PLACEMENT_3D('',#233444,#124152,#124153);
#102072=AXIS2_PLACEMENT_3D('',#233445,#124154,#124155);
#102073=AXIS2_PLACEMENT_3D('',#233446,#124156,#124157);
#102074=AXIS2_PLACEMENT_3D('',#233448,#124158,#124159);
#102075=AXIS2_PLACEMENT_3D('',#233450,#124161,#124162);
#102076=AXIS2_PLACEMENT_3D('',#233453,#124163,#124164);
#102077=AXIS2_PLACEMENT_3D('',#233454,#124165,#124166);
#102078=AXIS2_PLACEMENT_3D('',#233455,#124167,#124168);
#102079=AXIS2_PLACEMENT_3D('',#233456,#124169,#124170);
#102080=AXIS2_PLACEMENT_3D('',#233459,#124172,#124173);
#102081=AXIS2_PLACEMENT_3D('',#233460,#124174,#124175);
#102082=AXIS2_PLACEMENT_3D('',#233462,#124176,#124177);
#102083=AXIS2_PLACEMENT_3D('',#233464,#124178,#124179);
#102084=AXIS2_PLACEMENT_3D('',#233465,#124180,#124181);
#102085=AXIS2_PLACEMENT_3D('',#233466,#124182,#124183);
#102086=AXIS2_PLACEMENT_3D('',#233468,#124184,#124185);
#102087=AXIS2_PLACEMENT_3D('',#233470,#124186,#124187);
#102088=AXIS2_PLACEMENT_3D('',#233472,#124188,#124189);
#102089=AXIS2_PLACEMENT_3D('',#233473,#124190,#124191);
#102090=AXIS2_PLACEMENT_3D('',#233474,#124192,#124193);
#102091=AXIS2_PLACEMENT_3D('',#233476,#124195,#124196);
#102092=AXIS2_PLACEMENT_3D('',#233478,#124198,#124199);
#102093=AXIS2_PLACEMENT_3D('',#233483,#124201,#124202);
#102094=AXIS2_PLACEMENT_3D('',#233486,#124204,#124205);
#102095=AXIS2_PLACEMENT_3D('',#233487,#124206,#124207);
#102096=AXIS2_PLACEMENT_3D('',#233490,#124208,#124209);
#102097=AXIS2_PLACEMENT_3D('',#233493,#124211,#124212);
#102098=AXIS2_PLACEMENT_3D('',#233495,#124214,#124215);
#102099=AXIS2_PLACEMENT_3D('',#233497,#124216,#124217);
#102100=AXIS2_PLACEMENT_3D('',#233498,#124218,#124219);
#102101=AXIS2_PLACEMENT_3D('',#233499,#124220,#124221);
#102102=AXIS2_PLACEMENT_3D('',#233502,#124222,#124223);
#102103=AXIS2_PLACEMENT_3D('',#233503,#124224,#124225);
#102104=AXIS2_PLACEMENT_3D('',#233504,#124226,#124227);
#102105=AXIS2_PLACEMENT_3D('',#233505,#124228,#124229);
#102106=AXIS2_PLACEMENT_3D('',#233510,#124232,#124233);
#102107=AXIS2_PLACEMENT_3D('',#233511,#124234,#124235);
#102108=AXIS2_PLACEMENT_3D('',#233513,#124236,#124237);
#102109=AXIS2_PLACEMENT_3D('',#233515,#124238,#124239);
#102110=AXIS2_PLACEMENT_3D('',#233516,#124240,#124241);
#102111=AXIS2_PLACEMENT_3D('',#233517,#124242,#124243);
#102112=AXIS2_PLACEMENT_3D('',#233520,#124245,#124246);
#102113=AXIS2_PLACEMENT_3D('',#233522,#124248,#124249);
#102114=AXIS2_PLACEMENT_3D('',#233524,#124250,#124251);
#102115=AXIS2_PLACEMENT_3D('',#233525,#124252,#124253);
#102116=AXIS2_PLACEMENT_3D('',#233526,#124254,#124255);
#102117=AXIS2_PLACEMENT_3D('',#233528,#124256,#124257);
#102118=AXIS2_PLACEMENT_3D('',#233530,#124258,#124259);
#102119=AXIS2_PLACEMENT_3D('',#233531,#124260,#124261);
#102120=AXIS2_PLACEMENT_3D('',#233536,#124264,#124265);
#102121=AXIS2_PLACEMENT_3D('',#233537,#124266,#124267);
#102122=AXIS2_PLACEMENT_3D('',#233542,#124270,#124271);
#102123=AXIS2_PLACEMENT_3D('',#233543,#124272,#124273);
#102124=AXIS2_PLACEMENT_3D('',#233546,#124276,#124277);
#102125=AXIS2_PLACEMENT_3D('',#233548,#124279,#124280);
#102126=AXIS2_PLACEMENT_3D('',#233550,#124282,#124283);
#102127=AXIS2_PLACEMENT_3D('',#233552,#124285,#124286);
#102128=AXIS2_PLACEMENT_3D('',#233554,#124288,#124289);
#102129=AXIS2_PLACEMENT_3D('',#233556,#124291,#124292);
#102130=AXIS2_PLACEMENT_3D('',#233558,#124294,#124295);
#102131=AXIS2_PLACEMENT_3D('',#233559,#124296,#124297);
#102132=AXIS2_PLACEMENT_3D('',#233561,#124299,#124300);
#102133=AXIS2_PLACEMENT_3D('',#233563,#124302,#124303);
#102134=AXIS2_PLACEMENT_3D('',#233565,#124305,#124306);
#102135=AXIS2_PLACEMENT_3D('',#233567,#124308,#124309);
#102136=AXIS2_PLACEMENT_3D('',#233569,#124311,#124312);
#102137=AXIS2_PLACEMENT_3D('',#233570,#124313,#124314);
#102138=AXIS2_PLACEMENT_3D('',#233572,#124315,#124316);
#102139=AXIS2_PLACEMENT_3D('',#233575,#124317,#124318);
#102140=AXIS2_PLACEMENT_3D('',#233596,#124319,#124320);
#102141=AXIS2_PLACEMENT_3D('',#233615,#124321,#124322);
#102142=AXIS2_PLACEMENT_3D('',#233618,#124323,#124324);
#102143=AXIS2_PLACEMENT_3D('',#233619,#124325,#124326);
#102144=AXIS2_PLACEMENT_3D('',#233620,#124327,#124328);
#102145=AXIS2_PLACEMENT_3D('',#233621,#124329,#124330);
#102146=AXIS2_PLACEMENT_3D('',#233623,#124331,#124332);
#102147=AXIS2_PLACEMENT_3D('',#233625,#124333,#124334);
#102148=AXIS2_PLACEMENT_3D('',#233627,#124335,#124336);
#102149=AXIS2_PLACEMENT_3D('',#233628,#124337,#124338);
#102150=AXIS2_PLACEMENT_3D('',#233629,#124339,#124340);
#102151=AXIS2_PLACEMENT_3D('',#233632,#124341,#124342);
#102152=AXIS2_PLACEMENT_3D('',#233636,#124344,#124345);
#102153=AXIS2_PLACEMENT_3D('',#233638,#124347,#124348);
#102154=AXIS2_PLACEMENT_3D('',#233641,#124351,#124352);
#102155=AXIS2_PLACEMENT_3D('',#233643,#124354,#124355);
#102156=AXIS2_PLACEMENT_3D('',#233645,#124357,#124358);
#102157=AXIS2_PLACEMENT_3D('',#233646,#124359,#124360);
#102158=AXIS2_PLACEMENT_3D('',#233648,#124361,#124362);
#102159=AXIS2_PLACEMENT_3D('',#233649,#124363,#124364);
#102160=AXIS2_PLACEMENT_3D('',#233651,#124365,#124366);
#102161=AXIS2_PLACEMENT_3D('',#233653,#124368,#124369);
#102162=AXIS2_PLACEMENT_3D('',#233655,#124371,#124372);
#102163=AXIS2_PLACEMENT_3D('',#233656,#124373,#124374);
#102164=AXIS2_PLACEMENT_3D('',#233659,#124375,#124376);
#102165=AXIS2_PLACEMENT_3D('',#233674,#124379,#124380);
#102166=AXIS2_PLACEMENT_3D('',#233677,#124381,#124382);
#102167=AXIS2_PLACEMENT_3D('',#233678,#124383,#124384);
#102168=AXIS2_PLACEMENT_3D('',#233679,#124385,#124386);
#102169=AXIS2_PLACEMENT_3D('',#233680,#124387,#124388);
#102170=AXIS2_PLACEMENT_3D('',#233683,#124389,#124390);
#102171=AXIS2_PLACEMENT_3D('',#233686,#124393,#124394);
#102172=AXIS2_PLACEMENT_3D('',#233689,#124395,#124396);
#102173=AXIS2_PLACEMENT_3D('',#233690,#124397,#124398);
#102174=AXIS2_PLACEMENT_3D('',#233691,#124399,#124400);
#102175=AXIS2_PLACEMENT_3D('',#233692,#124401,#124402);
#102176=AXIS2_PLACEMENT_3D('',#233707,#124405,#124406);
#102177=AXIS2_PLACEMENT_3D('',#233710,#124407,#124408);
#102178=AXIS2_PLACEMENT_3D('',#233714,#124410,#124411);
#102179=AXIS2_PLACEMENT_3D('',#233716,#124413,#124414);
#102180=AXIS2_PLACEMENT_3D('',#233719,#124415,#124416);
#102181=AXIS2_PLACEMENT_3D('',#233720,#124417,#124418);
#102182=AXIS2_PLACEMENT_3D('',#233721,#124419,#124420);
#102183=AXIS2_PLACEMENT_3D('',#233722,#124421,#124422);
#102184=AXIS2_PLACEMENT_3D('',#233725,#124423,#124424);
#102185=AXIS2_PLACEMENT_3D('',#233728,#124427,#124428);
#102186=AXIS2_PLACEMENT_3D('',#233731,#124429,#124430);
#102187=AXIS2_PLACEMENT_3D('',#233732,#124431,#124432);
#102188=AXIS2_PLACEMENT_3D('',#233733,#124433,#124434);
#102189=AXIS2_PLACEMENT_3D('',#233734,#124435,#124436);
#102190=AXIS2_PLACEMENT_3D('',#233749,#124439,#124440);
#102191=AXIS2_PLACEMENT_3D('',#233752,#124441,#124442);
#102192=AXIS2_PLACEMENT_3D('',#233756,#124444,#124445);
#102193=AXIS2_PLACEMENT_3D('',#233758,#124447,#124448);
#102194=AXIS2_PLACEMENT_3D('',#233761,#124449,#124450);
#102195=AXIS2_PLACEMENT_3D('',#233762,#124451,#124452);
#102196=AXIS2_PLACEMENT_3D('',#233763,#124453,#124454);
#102197=AXIS2_PLACEMENT_3D('',#233764,#124455,#124456);
#102198=AXIS2_PLACEMENT_3D('',#233767,#124457,#124458);
#102199=AXIS2_PLACEMENT_3D('',#233770,#124461,#124462);
#102200=AXIS2_PLACEMENT_3D('',#233773,#124463,#124464);
#102201=AXIS2_PLACEMENT_3D('',#233774,#124465,#124466);
#102202=AXIS2_PLACEMENT_3D('',#233775,#124467,#124468);
#102203=AXIS2_PLACEMENT_3D('',#233776,#124469,#124470);
#102204=AXIS2_PLACEMENT_3D('',#233779,#124471,#124472);
#102205=AXIS2_PLACEMENT_3D('',#233782,#124475,#124476);
#102206=AXIS2_PLACEMENT_3D('',#233785,#124477,#124478);
#102207=AXIS2_PLACEMENT_3D('',#233786,#124479,#124480);
#102208=AXIS2_PLACEMENT_3D('',#233787,#124481,#124482);
#102209=AXIS2_PLACEMENT_3D('',#233788,#124483,#124484);
#102210=AXIS2_PLACEMENT_3D('',#233791,#124485,#124486);
#102211=AXIS2_PLACEMENT_3D('',#233794,#124489,#124490);
#102212=AXIS2_PLACEMENT_3D('',#233797,#124491,#124492);
#102213=AXIS2_PLACEMENT_3D('',#233798,#124493,#124494);
#102214=AXIS2_PLACEMENT_3D('',#233799,#124495,#124496);
#102215=AXIS2_PLACEMENT_3D('',#233800,#124497,#124498);
#102216=AXIS2_PLACEMENT_3D('',#233803,#124499,#124500);
#102217=AXIS2_PLACEMENT_3D('',#233806,#124503,#124504);
#102218=AXIS2_PLACEMENT_3D('',#233809,#124505,#124506);
#102219=AXIS2_PLACEMENT_3D('',#233813,#124508,#124509);
#102220=AXIS2_PLACEMENT_3D('',#233815,#124511,#124512);
#102221=AXIS2_PLACEMENT_3D('',#233818,#124513,#124514);
#102222=AXIS2_PLACEMENT_3D('',#233819,#124515,#124516);
#102223=AXIS2_PLACEMENT_3D('',#233820,#124517,#124518);
#102224=AXIS2_PLACEMENT_3D('',#233821,#124519,#124520);
#102225=AXIS2_PLACEMENT_3D('',#233824,#124521,#124522);
#102226=AXIS2_PLACEMENT_3D('',#233827,#124525,#124526);
#102227=AXIS2_PLACEMENT_3D('',#233830,#124527,#124528);
#102228=AXIS2_PLACEMENT_3D('',#233831,#124529,#124530);
#102229=AXIS2_PLACEMENT_3D('',#233832,#124531,#124532);
#102230=AXIS2_PLACEMENT_3D('',#233833,#124533,#124534);
#102231=AXIS2_PLACEMENT_3D('',#233848,#124537,#124538);
#102232=AXIS2_PLACEMENT_3D('',#233851,#124539,#124540);
#102233=AXIS2_PLACEMENT_3D('',#233855,#124542,#124543);
#102234=AXIS2_PLACEMENT_3D('',#233857,#124545,#124546);
#102235=AXIS2_PLACEMENT_3D('',#233860,#124547,#124548);
#102236=AXIS2_PLACEMENT_3D('',#233861,#124549,#124550);
#102237=AXIS2_PLACEMENT_3D('',#233862,#124551,#124552);
#102238=AXIS2_PLACEMENT_3D('',#233863,#124553,#124554);
#102239=AXIS2_PLACEMENT_3D('',#233866,#124555,#124556);
#102240=AXIS2_PLACEMENT_3D('',#233869,#124559,#124560);
#102241=AXIS2_PLACEMENT_3D('',#233872,#124561,#124562);
#102242=AXIS2_PLACEMENT_3D('',#233873,#124563,#124564);
#102243=AXIS2_PLACEMENT_3D('',#233874,#124565,#124566);
#102244=AXIS2_PLACEMENT_3D('',#233875,#124567,#124568);
#102245=AXIS2_PLACEMENT_3D('',#233878,#124569,#124570);
#102246=AXIS2_PLACEMENT_3D('',#233879,#124571,#124572);
#102247=AXIS2_PLACEMENT_3D('',#233880,#124573,#124574);
#102248=AXIS2_PLACEMENT_3D('',#233881,#124575,#124576);
#102249=AXIS2_PLACEMENT_3D('',#233884,#124577,#124578);
#102250=AXIS2_PLACEMENT_3D('',#233887,#124581,#124582);
#102251=AXIS2_PLACEMENT_3D('',#233890,#124583,#124584);
#102252=AXIS2_PLACEMENT_3D('',#233891,#124585,#124586);
#102253=AXIS2_PLACEMENT_3D('',#233892,#124587,#124588);
#102254=AXIS2_PLACEMENT_3D('',#233893,#124589,#124590);
#102255=AXIS2_PLACEMENT_3D('',#233896,#124591,#124592);
#102256=AXIS2_PLACEMENT_3D('',#233899,#124595,#124596);
#102257=AXIS2_PLACEMENT_3D('',#233902,#124597,#124598);
#102258=AXIS2_PLACEMENT_3D('',#233903,#124599,#124600);
#102259=AXIS2_PLACEMENT_3D('',#233904,#124601,#124602);
#102260=AXIS2_PLACEMENT_3D('',#233905,#124603,#124604);
#102261=AXIS2_PLACEMENT_3D('',#233908,#124605,#124606);
#102262=AXIS2_PLACEMENT_3D('',#233911,#124609,#124610);
#102263=AXIS2_PLACEMENT_3D('',#233914,#124611,#124612);
#102264=AXIS2_PLACEMENT_3D('',#233918,#124614,#124615);
#102265=AXIS2_PLACEMENT_3D('',#233920,#124617,#124618);
#102266=AXIS2_PLACEMENT_3D('',#233923,#124619,#124620);
#102267=AXIS2_PLACEMENT_3D('',#233924,#124621,#124622);
#102268=AXIS2_PLACEMENT_3D('',#233925,#124623,#124624);
#102269=AXIS2_PLACEMENT_3D('',#233926,#124625,#124626);
#102270=AXIS2_PLACEMENT_3D('',#233929,#124627,#124628);
#102271=AXIS2_PLACEMENT_3D('',#233932,#124631,#124632);
#102272=AXIS2_PLACEMENT_3D('',#233935,#124633,#124634);
#102273=AXIS2_PLACEMENT_3D('',#233936,#124635,#124636);
#102274=AXIS2_PLACEMENT_3D('',#233937,#124637,#124638);
#102275=AXIS2_PLACEMENT_3D('',#233938,#124639,#124640);
#102276=AXIS2_PLACEMENT_3D('',#233941,#124641,#124642);
#102277=AXIS2_PLACEMENT_3D('',#233942,#124643,#124644);
#102278=AXIS2_PLACEMENT_3D('',#233943,#124645,#124646);
#102279=AXIS2_PLACEMENT_3D('',#233944,#124647,#124648);
#102280=AXIS2_PLACEMENT_3D('',#233947,#124649,#124650);
#102281=AXIS2_PLACEMENT_3D('',#233948,#124651,#124652);
#102282=AXIS2_PLACEMENT_3D('',#233949,#124653,#124654);
#102283=AXIS2_PLACEMENT_3D('',#233950,#124655,#124656);
#102284=AXIS2_PLACEMENT_3D('',#233953,#124657,#124658);
#102285=AXIS2_PLACEMENT_3D('',#233956,#124661,#124662);
#102286=AXIS2_PLACEMENT_3D('',#233959,#124663,#124664);
#102287=AXIS2_PLACEMENT_3D('',#233960,#124665,#124666);
#102288=AXIS2_PLACEMENT_3D('',#233961,#124667,#124668);
#102289=AXIS2_PLACEMENT_3D('',#233962,#124669,#124670);
#102290=AXIS2_PLACEMENT_3D('',#233965,#124671,#124672);
#102291=AXIS2_PLACEMENT_3D('',#233968,#124675,#124676);
#102292=AXIS2_PLACEMENT_3D('',#233971,#124677,#124678);
#102293=AXIS2_PLACEMENT_3D('',#233975,#124680,#124681);
#102294=AXIS2_PLACEMENT_3D('',#233977,#124683,#124684);
#102295=AXIS2_PLACEMENT_3D('',#233980,#124685,#124686);
#102296=AXIS2_PLACEMENT_3D('',#233981,#124687,#124688);
#102297=AXIS2_PLACEMENT_3D('',#233982,#124689,#124690);
#102298=AXIS2_PLACEMENT_3D('',#233983,#124691,#124692);
#102299=AXIS2_PLACEMENT_3D('',#233986,#124693,#124694);
#102300=AXIS2_PLACEMENT_3D('',#233989,#124697,#124698);
#102301=AXIS2_PLACEMENT_3D('',#233992,#124699,#124700);
#102302=AXIS2_PLACEMENT_3D('',#233993,#124701,#124702);
#102303=AXIS2_PLACEMENT_3D('',#233994,#124703,#124704);
#102304=AXIS2_PLACEMENT_3D('',#233995,#124705,#124706);
#102305=AXIS2_PLACEMENT_3D('',#233998,#124707,#124708);
#102306=AXIS2_PLACEMENT_3D('',#233999,#124709,#124710);
#102307=AXIS2_PLACEMENT_3D('',#234000,#124711,#124712);
#102308=AXIS2_PLACEMENT_3D('',#234001,#124713,#124714);
#102309=AXIS2_PLACEMENT_3D('',#234004,#124715,#124716);
#102310=AXIS2_PLACEMENT_3D('',#234005,#124717,#124718);
#102311=AXIS2_PLACEMENT_3D('',#234006,#124719,#124720);
#102312=AXIS2_PLACEMENT_3D('',#234007,#124721,#124722);
#102313=AXIS2_PLACEMENT_3D('',#234010,#124723,#124724);
#102314=AXIS2_PLACEMENT_3D('',#234013,#124727,#124728);
#102315=AXIS2_PLACEMENT_3D('',#234016,#124729,#124730);
#102316=AXIS2_PLACEMENT_3D('',#234017,#124731,#124732);
#102317=AXIS2_PLACEMENT_3D('',#234018,#124733,#124734);
#102318=AXIS2_PLACEMENT_3D('',#234019,#124735,#124736);
#102319=AXIS2_PLACEMENT_3D('',#234022,#124737,#124738);
#102320=AXIS2_PLACEMENT_3D('',#234025,#124741,#124742);
#102321=AXIS2_PLACEMENT_3D('',#234028,#124743,#124744);
#102322=AXIS2_PLACEMENT_3D('',#234032,#124746,#124747);
#102323=AXIS2_PLACEMENT_3D('',#234034,#124749,#124750);
#102324=AXIS2_PLACEMENT_3D('',#234037,#124751,#124752);
#102325=AXIS2_PLACEMENT_3D('',#234038,#124753,#124754);
#102326=AXIS2_PLACEMENT_3D('',#234039,#124755,#124756);
#102327=AXIS2_PLACEMENT_3D('',#234040,#124757,#124758);
#102328=AXIS2_PLACEMENT_3D('',#234043,#124759,#124760);
#102329=AXIS2_PLACEMENT_3D('',#234046,#124763,#124764);
#102330=AXIS2_PLACEMENT_3D('',#234049,#124765,#124766);
#102331=AXIS2_PLACEMENT_3D('',#234050,#124767,#124768);
#102332=AXIS2_PLACEMENT_3D('',#234051,#124769,#124770);
#102333=AXIS2_PLACEMENT_3D('',#234052,#124771,#124772);
#102334=AXIS2_PLACEMENT_3D('',#234055,#124773,#124774);
#102335=AXIS2_PLACEMENT_3D('',#234056,#124775,#124776);
#102336=AXIS2_PLACEMENT_3D('',#234057,#124777,#124778);
#102337=AXIS2_PLACEMENT_3D('',#234058,#124779,#124780);
#102338=AXIS2_PLACEMENT_3D('',#234061,#124781,#124782);
#102339=AXIS2_PLACEMENT_3D('',#234062,#124783,#124784);
#102340=AXIS2_PLACEMENT_3D('',#234063,#124785,#124786);
#102341=AXIS2_PLACEMENT_3D('',#234064,#124787,#124788);
#102342=AXIS2_PLACEMENT_3D('',#234067,#124789,#124790);
#102343=AXIS2_PLACEMENT_3D('',#234070,#124793,#124794);
#102344=AXIS2_PLACEMENT_3D('',#234073,#124795,#124796);
#102345=AXIS2_PLACEMENT_3D('',#234074,#124797,#124798);
#102346=AXIS2_PLACEMENT_3D('',#234075,#124799,#124800);
#102347=AXIS2_PLACEMENT_3D('',#234076,#124801,#124802);
#102348=AXIS2_PLACEMENT_3D('',#234079,#124803,#124804);
#102349=AXIS2_PLACEMENT_3D('',#234082,#124807,#124808);
#102350=AXIS2_PLACEMENT_3D('',#234085,#124809,#124810);
#102351=AXIS2_PLACEMENT_3D('',#234089,#124812,#124813);
#102352=AXIS2_PLACEMENT_3D('',#234091,#124815,#124816);
#102353=AXIS2_PLACEMENT_3D('',#234094,#124817,#124818);
#102354=AXIS2_PLACEMENT_3D('',#234095,#124819,#124820);
#102355=AXIS2_PLACEMENT_3D('',#234096,#124821,#124822);
#102356=AXIS2_PLACEMENT_3D('',#234097,#124823,#124824);
#102357=AXIS2_PLACEMENT_3D('',#234100,#124825,#124826);
#102358=AXIS2_PLACEMENT_3D('',#234103,#124829,#124830);
#102359=AXIS2_PLACEMENT_3D('',#234106,#124831,#124832);
#102360=AXIS2_PLACEMENT_3D('',#234107,#124833,#124834);
#102361=AXIS2_PLACEMENT_3D('',#234108,#124835,#124836);
#102362=AXIS2_PLACEMENT_3D('',#234109,#124837,#124838);
#102363=AXIS2_PLACEMENT_3D('',#234112,#124839,#124840);
#102364=AXIS2_PLACEMENT_3D('',#234113,#124841,#124842);
#102365=AXIS2_PLACEMENT_3D('',#234114,#124843,#124844);
#102366=AXIS2_PLACEMENT_3D('',#234115,#124845,#124846);
#102367=AXIS2_PLACEMENT_3D('',#234118,#124847,#124848);
#102368=AXIS2_PLACEMENT_3D('',#234119,#124849,#124850);
#102369=AXIS2_PLACEMENT_3D('',#234120,#124851,#124852);
#102370=AXIS2_PLACEMENT_3D('',#234121,#124853,#124854);
#102371=AXIS2_PLACEMENT_3D('',#234124,#124855,#124856);
#102372=AXIS2_PLACEMENT_3D('',#234127,#124859,#124860);
#102373=AXIS2_PLACEMENT_3D('',#234130,#124861,#124862);
#102374=AXIS2_PLACEMENT_3D('',#234131,#124863,#124864);
#102375=AXIS2_PLACEMENT_3D('',#234132,#124865,#124866);
#102376=AXIS2_PLACEMENT_3D('',#234133,#124867,#124868);
#102377=AXIS2_PLACEMENT_3D('',#234136,#124869,#124870);
#102378=AXIS2_PLACEMENT_3D('',#234139,#124873,#124874);
#102379=AXIS2_PLACEMENT_3D('',#234142,#124875,#124876);
#102380=AXIS2_PLACEMENT_3D('',#234146,#124878,#124879);
#102381=AXIS2_PLACEMENT_3D('',#234148,#124881,#124882);
#102382=AXIS2_PLACEMENT_3D('',#234151,#124883,#124884);
#102383=AXIS2_PLACEMENT_3D('',#234152,#124885,#124886);
#102384=AXIS2_PLACEMENT_3D('',#234153,#124887,#124888);
#102385=AXIS2_PLACEMENT_3D('',#234154,#124889,#124890);
#102386=AXIS2_PLACEMENT_3D('',#234157,#124891,#124892);
#102387=AXIS2_PLACEMENT_3D('',#234160,#124895,#124896);
#102388=AXIS2_PLACEMENT_3D('',#234163,#124897,#124898);
#102389=AXIS2_PLACEMENT_3D('',#234164,#124899,#124900);
#102390=AXIS2_PLACEMENT_3D('',#234165,#124901,#124902);
#102391=AXIS2_PLACEMENT_3D('',#234166,#124903,#124904);
#102392=AXIS2_PLACEMENT_3D('',#234169,#124905,#124906);
#102393=AXIS2_PLACEMENT_3D('',#234170,#124907,#124908);
#102394=AXIS2_PLACEMENT_3D('',#234171,#124909,#124910);
#102395=AXIS2_PLACEMENT_3D('',#234172,#124911,#124912);
#102396=AXIS2_PLACEMENT_3D('',#234175,#124913,#124914);
#102397=AXIS2_PLACEMENT_3D('',#234176,#124915,#124916);
#102398=AXIS2_PLACEMENT_3D('',#234177,#124917,#124918);
#102399=AXIS2_PLACEMENT_3D('',#234178,#124919,#124920);
#102400=AXIS2_PLACEMENT_3D('',#234181,#124921,#124922);
#102401=AXIS2_PLACEMENT_3D('',#234184,#124925,#124926);
#102402=AXIS2_PLACEMENT_3D('',#234187,#124927,#124928);
#102403=AXIS2_PLACEMENT_3D('',#234188,#124929,#124930);
#102404=AXIS2_PLACEMENT_3D('',#234189,#124931,#124932);
#102405=AXIS2_PLACEMENT_3D('',#234190,#124933,#124934);
#102406=AXIS2_PLACEMENT_3D('',#234193,#124935,#124936);
#102407=AXIS2_PLACEMENT_3D('',#234196,#124939,#124940);
#102408=AXIS2_PLACEMENT_3D('',#234199,#124941,#124942);
#102409=AXIS2_PLACEMENT_3D('',#234203,#124944,#124945);
#102410=AXIS2_PLACEMENT_3D('',#234205,#124947,#124948);
#102411=AXIS2_PLACEMENT_3D('',#234208,#124949,#124950);
#102412=AXIS2_PLACEMENT_3D('',#234209,#124951,#124952);
#102413=AXIS2_PLACEMENT_3D('',#234210,#124953,#124954);
#102414=AXIS2_PLACEMENT_3D('',#234211,#124955,#124956);
#102415=AXIS2_PLACEMENT_3D('',#234214,#124957,#124958);
#102416=AXIS2_PLACEMENT_3D('',#234217,#124961,#124962);
#102417=AXIS2_PLACEMENT_3D('',#234220,#124963,#124964);
#102418=AXIS2_PLACEMENT_3D('',#234221,#124965,#124966);
#102419=AXIS2_PLACEMENT_3D('',#234222,#124967,#124968);
#102420=AXIS2_PLACEMENT_3D('',#234223,#124969,#124970);
#102421=AXIS2_PLACEMENT_3D('',#234226,#124971,#124972);
#102422=AXIS2_PLACEMENT_3D('',#234227,#124973,#124974);
#102423=AXIS2_PLACEMENT_3D('',#234228,#124975,#124976);
#102424=AXIS2_PLACEMENT_3D('',#234229,#124977,#124978);
#102425=AXIS2_PLACEMENT_3D('',#234232,#124979,#124980);
#102426=AXIS2_PLACEMENT_3D('',#234233,#124981,#124982);
#102427=AXIS2_PLACEMENT_3D('',#234234,#124983,#124984);
#102428=AXIS2_PLACEMENT_3D('',#234235,#124985,#124986);
#102429=AXIS2_PLACEMENT_3D('',#234238,#124987,#124988);
#102430=AXIS2_PLACEMENT_3D('',#234241,#124991,#124992);
#102431=AXIS2_PLACEMENT_3D('',#234244,#124993,#124994);
#102432=AXIS2_PLACEMENT_3D('',#234245,#124995,#124996);
#102433=AXIS2_PLACEMENT_3D('',#234246,#124997,#124998);
#102434=AXIS2_PLACEMENT_3D('',#234247,#124999,#125000);
#102435=AXIS2_PLACEMENT_3D('',#234250,#125001,#125002);
#102436=AXIS2_PLACEMENT_3D('',#234253,#125005,#125006);
#102437=AXIS2_PLACEMENT_3D('',#234256,#125007,#125008);
#102438=AXIS2_PLACEMENT_3D('',#234260,#125010,#125011);
#102439=AXIS2_PLACEMENT_3D('',#234262,#125013,#125014);
#102440=AXIS2_PLACEMENT_3D('',#234265,#125015,#125016);
#102441=AXIS2_PLACEMENT_3D('',#234266,#125017,#125018);
#102442=AXIS2_PLACEMENT_3D('',#234267,#125019,#125020);
#102443=AXIS2_PLACEMENT_3D('',#234268,#125021,#125022);
#102444=AXIS2_PLACEMENT_3D('',#234271,#125023,#125024);
#102445=AXIS2_PLACEMENT_3D('',#234274,#125027,#125028);
#102446=AXIS2_PLACEMENT_3D('',#234277,#125029,#125030);
#102447=AXIS2_PLACEMENT_3D('',#234278,#125031,#125032);
#102448=AXIS2_PLACEMENT_3D('',#234279,#125033,#125034);
#102449=AXIS2_PLACEMENT_3D('',#234280,#125035,#125036);
#102450=AXIS2_PLACEMENT_3D('',#234283,#125037,#125038);
#102451=AXIS2_PLACEMENT_3D('',#234286,#125041,#125042);
#102452=AXIS2_PLACEMENT_3D('',#234289,#125043,#125044);
#102453=AXIS2_PLACEMENT_3D('',#234290,#125045,#125046);
#102454=AXIS2_PLACEMENT_3D('',#234291,#125047,#125048);
#102455=AXIS2_PLACEMENT_3D('',#234292,#125049,#125050);
#102456=AXIS2_PLACEMENT_3D('',#234295,#125051,#125052);
#102457=AXIS2_PLACEMENT_3D('',#234296,#125053,#125054);
#102458=AXIS2_PLACEMENT_3D('',#234297,#125055,#125056);
#102459=AXIS2_PLACEMENT_3D('',#234298,#125057,#125058);
#102460=AXIS2_PLACEMENT_3D('',#234301,#125059,#125060);
#102461=AXIS2_PLACEMENT_3D('',#234304,#125063,#125064);
#102462=AXIS2_PLACEMENT_3D('',#234307,#125065,#125066);
#102463=AXIS2_PLACEMENT_3D('',#234308,#125067,#125068);
#102464=AXIS2_PLACEMENT_3D('',#234309,#125069,#125070);
#102465=AXIS2_PLACEMENT_3D('',#234310,#125071,#125072);
#102466=AXIS2_PLACEMENT_3D('',#234313,#125073,#125074);
#102467=AXIS2_PLACEMENT_3D('',#234316,#125077,#125078);
#102468=AXIS2_PLACEMENT_3D('',#234319,#125079,#125080);
#102469=AXIS2_PLACEMENT_3D('',#234323,#125082,#125083);
#102470=AXIS2_PLACEMENT_3D('',#234325,#125085,#125086);
#102471=AXIS2_PLACEMENT_3D('',#234328,#125087,#125088);
#102472=AXIS2_PLACEMENT_3D('',#234329,#125089,#125090);
#102473=AXIS2_PLACEMENT_3D('',#234330,#125091,#125092);
#102474=AXIS2_PLACEMENT_3D('',#234331,#125093,#125094);
#102475=AXIS2_PLACEMENT_3D('',#234334,#125095,#125096);
#102476=AXIS2_PLACEMENT_3D('',#234337,#125099,#125100);
#102477=AXIS2_PLACEMENT_3D('',#234340,#125101,#125102);
#102478=AXIS2_PLACEMENT_3D('',#234341,#125103,#125104);
#102479=AXIS2_PLACEMENT_3D('',#234342,#125105,#125106);
#102480=AXIS2_PLACEMENT_3D('',#234343,#125107,#125108);
#102481=AXIS2_PLACEMENT_3D('',#234346,#125109,#125110);
#102482=AXIS2_PLACEMENT_3D('',#234349,#125113,#125114);
#102483=AXIS2_PLACEMENT_3D('',#234352,#125115,#125116);
#102484=AXIS2_PLACEMENT_3D('',#234353,#125117,#125118);
#102485=AXIS2_PLACEMENT_3D('',#234354,#125119,#125120);
#102486=AXIS2_PLACEMENT_3D('',#234355,#125121,#125122);
#102487=AXIS2_PLACEMENT_3D('',#234358,#125123,#125124);
#102488=AXIS2_PLACEMENT_3D('',#234361,#125127,#125128);
#102489=AXIS2_PLACEMENT_3D('',#234364,#125129,#125130);
#102490=AXIS2_PLACEMENT_3D('',#234365,#125131,#125132);
#102491=AXIS2_PLACEMENT_3D('',#234366,#125133,#125134);
#102492=AXIS2_PLACEMENT_3D('',#234367,#125135,#125136);
#102493=AXIS2_PLACEMENT_3D('',#234370,#125137,#125138);
#102494=AXIS2_PLACEMENT_3D('',#234373,#125141,#125142);
#102495=AXIS2_PLACEMENT_3D('',#234389,#125144,#125145);
#102496=AXIS2_PLACEMENT_3D('',#234391,#125147,#125148);
#102497=AXIS2_PLACEMENT_3D('',#234394,#125149,#125150);
#102498=AXIS2_PLACEMENT_3D('',#234395,#125151,#125152);
#102499=AXIS2_PLACEMENT_3D('',#234396,#125153,#125154);
#102500=AXIS2_PLACEMENT_3D('',#234397,#125155,#125156);
#102501=AXIS2_PLACEMENT_3D('',#234400,#125157,#125158);
#102502=AXIS2_PLACEMENT_3D('',#234403,#125161,#125162);
#102503=AXIS2_PLACEMENT_3D('',#234406,#125163,#125164);
#102504=AXIS2_PLACEMENT_3D('',#234407,#125165,#125166);
#102505=AXIS2_PLACEMENT_3D('',#234408,#125167,#125168);
#102506=AXIS2_PLACEMENT_3D('',#234409,#125169,#125170);
#102507=AXIS2_PLACEMENT_3D('',#234412,#125171,#125172);
#102508=AXIS2_PLACEMENT_3D('',#234415,#125175,#125176);
#102509=AXIS2_PLACEMENT_3D('',#234420,#125179,#125180);
#102510=AXIS2_PLACEMENT_3D('',#234421,#125181,#125182);
#102511=AXIS2_PLACEMENT_3D('',#234426,#125185,#125186);
#102512=AXIS2_PLACEMENT_3D('',#234427,#125187,#125188);
#102513=AXIS2_PLACEMENT_3D('',#234432,#125191,#125192);
#102514=AXIS2_PLACEMENT_3D('',#234433,#125193,#125194);
#102515=AXIS2_PLACEMENT_3D('',#234438,#125197,#125198);
#102516=AXIS2_PLACEMENT_3D('',#234439,#125199,#125200);
#102517=AXIS2_PLACEMENT_3D('',#234444,#125203,#125204);
#102518=AXIS2_PLACEMENT_3D('',#234445,#125205,#125206);
#102519=AXIS2_PLACEMENT_3D('',#234450,#125209,#125210);
#102520=AXIS2_PLACEMENT_3D('',#234451,#125211,#125212);
#102521=AXIS2_PLACEMENT_3D('',#234456,#125215,#125216);
#102522=AXIS2_PLACEMENT_3D('',#234457,#125217,#125218);
#102523=AXIS2_PLACEMENT_3D('',#234462,#125221,#125222);
#102524=AXIS2_PLACEMENT_3D('',#234463,#125223,#125224);
#102525=AXIS2_PLACEMENT_3D('',#234468,#125227,#125228);
#102526=AXIS2_PLACEMENT_3D('',#234469,#125229,#125230);
#102527=AXIS2_PLACEMENT_3D('',#234474,#125233,#125234);
#102528=AXIS2_PLACEMENT_3D('',#234475,#125235,#125236);
#102529=AXIS2_PLACEMENT_3D('',#234480,#125239,#125240);
#102530=AXIS2_PLACEMENT_3D('',#234481,#125241,#125242);
#102531=AXIS2_PLACEMENT_3D('',#234486,#125245,#125246);
#102532=AXIS2_PLACEMENT_3D('',#234487,#125247,#125248);
#102533=AXIS2_PLACEMENT_3D('',#234492,#125251,#125252);
#102534=AXIS2_PLACEMENT_3D('',#234493,#125253,#125254);
#102535=AXIS2_PLACEMENT_3D('',#234498,#125257,#125258);
#102536=AXIS2_PLACEMENT_3D('',#234499,#125259,#125260);
#102537=AXIS2_PLACEMENT_3D('',#234504,#125263,#125264);
#102538=AXIS2_PLACEMENT_3D('',#234505,#125265,#125266);
#102539=AXIS2_PLACEMENT_3D('',#234510,#125269,#125270);
#102540=AXIS2_PLACEMENT_3D('',#234511,#125271,#125272);
#102541=AXIS2_PLACEMENT_3D('',#234516,#125275,#125276);
#102542=AXIS2_PLACEMENT_3D('',#234517,#125277,#125278);
#102543=AXIS2_PLACEMENT_3D('',#234522,#125281,#125282);
#102544=AXIS2_PLACEMENT_3D('',#234523,#125283,#125284);
#102545=AXIS2_PLACEMENT_3D('',#234528,#125287,#125288);
#102546=AXIS2_PLACEMENT_3D('',#234529,#125289,#125290);
#102547=AXIS2_PLACEMENT_3D('',#234534,#125293,#125294);
#102548=AXIS2_PLACEMENT_3D('',#234535,#125295,#125296);
#102549=AXIS2_PLACEMENT_3D('',#234540,#125299,#125300);
#102550=AXIS2_PLACEMENT_3D('',#234541,#125301,#125302);
#102551=AXIS2_PLACEMENT_3D('',#234546,#125305,#125306);
#102552=AXIS2_PLACEMENT_3D('',#234547,#125307,#125308);
#102553=AXIS2_PLACEMENT_3D('',#234552,#125311,#125312);
#102554=AXIS2_PLACEMENT_3D('',#234553,#125313,#125314);
#102555=AXIS2_PLACEMENT_3D('',#234558,#125317,#125318);
#102556=AXIS2_PLACEMENT_3D('',#234559,#125319,#125320);
#102557=AXIS2_PLACEMENT_3D('',#234564,#125323,#125324);
#102558=AXIS2_PLACEMENT_3D('',#234565,#125325,#125326);
#102559=AXIS2_PLACEMENT_3D('',#234570,#125329,#125330);
#102560=AXIS2_PLACEMENT_3D('',#234571,#125331,#125332);
#102561=AXIS2_PLACEMENT_3D('',#234572,#125333,#125334);
#102562=AXIS2_PLACEMENT_3D('',#234574,#125335,#125336);
#102563=AXIS2_PLACEMENT_3D('',#234578,#125339,#125340);
#102564=AXIS2_PLACEMENT_3D('',#234590,#125352,#125353);
#102565=AXIS2_PLACEMENT_3D('',#234592,#125355,#125356);
#102566=AXIS2_PLACEMENT_3D('',#234596,#125358,#125359);
#102567=AXIS2_PLACEMENT_3D('',#234598,#125361,#125362);
#102568=AXIS2_PLACEMENT_3D('',#234600,#125364,#125365);
#102569=AXIS2_PLACEMENT_3D('',#234602,#125367,#125368);
#102570=AXIS2_PLACEMENT_3D('',#234606,#125371,#125372);
#102571=AXIS2_PLACEMENT_3D('',#234608,#125374,#125375);
#102572=AXIS2_PLACEMENT_3D('',#234610,#125377,#125378);
#102573=AXIS2_PLACEMENT_3D('',#234612,#125380,#125381);
#102574=AXIS2_PLACEMENT_3D('',#234614,#125383,#125384);
#102575=AXIS2_PLACEMENT_3D('',#234616,#125386,#125387);
#102576=AXIS2_PLACEMENT_3D('',#234618,#125389,#125390);
#102577=AXIS2_PLACEMENT_3D('',#234620,#125392,#125393);
#102578=AXIS2_PLACEMENT_3D('',#234622,#125395,#125396);
#102579=AXIS2_PLACEMENT_3D('',#234624,#125398,#125399);
#102580=AXIS2_PLACEMENT_3D('',#234626,#125401,#125402);
#102581=AXIS2_PLACEMENT_3D('',#234629,#125405,#125406);
#102582=AXIS2_PLACEMENT_3D('',#234630,#125407,#125408);
#102583=AXIS2_PLACEMENT_3D('',#234631,#125409,#125410);
#102584=AXIS2_PLACEMENT_3D('',#234632,#125411,#125412);
#102585=AXIS2_PLACEMENT_3D('',#234634,#125414,#125415);
#102586=AXIS2_PLACEMENT_3D('',#234636,#125417,#125418);
#102587=AXIS2_PLACEMENT_3D('',#234639,#125421,#125422);
#102588=AXIS2_PLACEMENT_3D('',#234640,#125423,#125424);
#102589=AXIS2_PLACEMENT_3D('',#234641,#125425,#125426);
#102590=AXIS2_PLACEMENT_3D('',#234642,#125427,#125428);
#102591=AXIS2_PLACEMENT_3D('',#234644,#125430,#125431);
#102592=AXIS2_PLACEMENT_3D('',#234646,#125433,#125434);
#102593=AXIS2_PLACEMENT_3D('',#234649,#125437,#125438);
#102594=AXIS2_PLACEMENT_3D('',#234650,#125439,#125440);
#102595=AXIS2_PLACEMENT_3D('',#234651,#125441,#125442);
#102596=AXIS2_PLACEMENT_3D('',#234652,#125443,#125444);
#102597=AXIS2_PLACEMENT_3D('',#234654,#125446,#125447);
#102598=AXIS2_PLACEMENT_3D('',#234656,#125449,#125450);
#102599=AXIS2_PLACEMENT_3D('',#234659,#125453,#125454);
#102600=AXIS2_PLACEMENT_3D('',#234660,#125455,#125456);
#102601=AXIS2_PLACEMENT_3D('',#234661,#125457,#125458);
#102602=AXIS2_PLACEMENT_3D('',#234662,#125459,#125460);
#102603=AXIS2_PLACEMENT_3D('',#234664,#125462,#125463);
#102604=AXIS2_PLACEMENT_3D('',#234666,#125465,#125466);
#102605=AXIS2_PLACEMENT_3D('',#234669,#125469,#125470);
#102606=AXIS2_PLACEMENT_3D('',#234670,#125471,#125472);
#102607=AXIS2_PLACEMENT_3D('',#234672,#125474,#125475);
#102608=AXIS2_PLACEMENT_3D('',#234675,#125477,#125478);
#102609=AXIS2_PLACEMENT_3D('',#234676,#125479,#125480);
#102610=AXIS2_PLACEMENT_3D('',#234678,#125482,#125483);
#102611=AXIS2_PLACEMENT_3D('',#234681,#125485,#125486);
#102612=AXIS2_PLACEMENT_3D('',#234682,#125487,#125488);
#102613=AXIS2_PLACEMENT_3D('',#234684,#125490,#125491);
#102614=AXIS2_PLACEMENT_3D('',#234689,#125496,#125497);
#102615=AXIS2_PLACEMENT_3D('',#234691,#125499,#125500);
#102616=AXIS2_PLACEMENT_3D('',#234700,#125507,#125508);
#102617=AXIS2_PLACEMENT_3D('',#234709,#125514,#125515);
#102618=AXIS2_PLACEMENT_3D('',#234711,#125517,#125518);
#102619=AXIS2_PLACEMENT_3D('',#234712,#125519,#125520);
#102620=AXIS2_PLACEMENT_3D('',#234713,#125521,#125522);
#102621=AXIS2_PLACEMENT_3D('',#234715,#125524,#125525);
#102622=AXIS2_PLACEMENT_3D('',#234716,#125526,#125527);
#102623=AXIS2_PLACEMENT_3D('',#234718,#125529,#125530);
#102624=AXIS2_PLACEMENT_3D('',#234719,#125531,#125532);
#102625=AXIS2_PLACEMENT_3D('',#234721,#125534,#125535);
#102626=AXIS2_PLACEMENT_3D('',#234722,#125536,#125537);
#102627=AXIS2_PLACEMENT_3D('',#234724,#125539,#125540);
#102628=AXIS2_PLACEMENT_3D('',#234725,#125541,#125542);
#102629=AXIS2_PLACEMENT_3D('',#234726,#125543,#125544);
#102630=AXIS2_PLACEMENT_3D('',#234728,#125546,#125547);
#102631=AXIS2_PLACEMENT_3D('',#234729,#125548,#125549);
#102632=AXIS2_PLACEMENT_3D('',#234730,#125550,#125551);
#102633=AXIS2_PLACEMENT_3D('',#234731,#125552,#125553);
#102634=AXIS2_PLACEMENT_3D('',#234733,#125555,#125556);
#102635=AXIS2_PLACEMENT_3D('',#234734,#125557,#125558);
#102636=AXIS2_PLACEMENT_3D('',#234736,#125560,#125561);
#102637=AXIS2_PLACEMENT_3D('',#234738,#125563,#125564);
#102638=AXIS2_PLACEMENT_3D('',#234739,#125565,#125566);
#102639=AXIS2_PLACEMENT_3D('',#234740,#125567,#125568);
#102640=AXIS2_PLACEMENT_3D('',#234742,#125570,#125571);
#102641=AXIS2_PLACEMENT_3D('',#234744,#125573,#125574);
#102642=AXIS2_PLACEMENT_3D('',#234745,#125575,#125576);
#102643=AXIS2_PLACEMENT_3D('',#234746,#125577,#125578);
#102644=AXIS2_PLACEMENT_3D('',#234748,#125580,#125581);
#102645=AXIS2_PLACEMENT_3D('',#234749,#125582,#125583);
#102646=AXIS2_PLACEMENT_3D('',#234752,#125584,#125585);
#102647=AXIS2_PLACEMENT_3D('',#234754,#125586,#125587);
#102648=AXIS2_PLACEMENT_3D('',#234756,#125588,#125589);
#102649=AXIS2_PLACEMENT_3D('',#234758,#125590,#125591);
#102650=AXIS2_PLACEMENT_3D('',#234760,#125592,#125593);
#102651=AXIS2_PLACEMENT_3D('',#234761,#125594,#125595);
#102652=AXIS2_PLACEMENT_3D('',#234762,#125596,#125597);
#102653=AXIS2_PLACEMENT_3D('',#234770,#125598,#125599);
#102654=AXIS2_PLACEMENT_3D('',#234778,#125600,#125601);
#102655=AXIS2_PLACEMENT_3D('',#234786,#125602,#125603);
#102656=AXIS2_PLACEMENT_3D('',#234794,#125604,#125605);
#102657=AXIS2_PLACEMENT_3D('',#234802,#125606,#125607);
#102658=AXIS2_PLACEMENT_3D('',#234810,#125608,#125609);
#102659=AXIS2_PLACEMENT_3D('',#234813,#125610,#125611);
#102660=AXIS2_PLACEMENT_3D('',#234815,#125612,#125613);
#102661=AXIS2_PLACEMENT_3D('',#234817,#125614,#125615);
#102662=AXIS2_PLACEMENT_3D('',#234819,#125616,#125617);
#102663=AXIS2_PLACEMENT_3D('',#234821,#125618,#125619);
#102664=AXIS2_PLACEMENT_3D('',#234822,#125620,#125621);
#102665=AXIS2_PLACEMENT_3D('',#234823,#125622,#125623);
#102666=AXIS2_PLACEMENT_3D('',#234831,#125624,#125625);
#102667=AXIS2_PLACEMENT_3D('',#234839,#125626,#125627);
#102668=AXIS2_PLACEMENT_3D('',#234847,#125628,#125629);
#102669=AXIS2_PLACEMENT_3D('',#234855,#125630,#125631);
#102670=AXIS2_PLACEMENT_3D('',#234863,#125632,#125633);
#102671=AXIS2_PLACEMENT_3D('',#234871,#125634,#125635);
#102672=AXIS2_PLACEMENT_3D('',#234874,#125638,#125639);
#102673=AXIS2_PLACEMENT_3D('',#234876,#125641,#125642);
#102674=AXIS2_PLACEMENT_3D('',#234878,#125644,#125645);
#102675=AXIS2_PLACEMENT_3D('',#234880,#125647,#125648);
#102676=AXIS2_PLACEMENT_3D('',#234882,#125650,#125651);
#102677=AXIS2_PLACEMENT_3D('',#234883,#125652,#125653);
#102678=AXIS2_PLACEMENT_3D('',#234886,#125654,#125655);
#102679=AXIS2_PLACEMENT_3D('',#234888,#125656,#125657);
#102680=AXIS2_PLACEMENT_3D('',#234890,#125658,#125659);
#102681=AXIS2_PLACEMENT_3D('',#234892,#125660,#125661);
#102682=AXIS2_PLACEMENT_3D('',#234894,#125662,#125663);
#102683=AXIS2_PLACEMENT_3D('',#234895,#125664,#125665);
#102684=AXIS2_PLACEMENT_3D('',#234896,#125666,#125667);
#102685=AXIS2_PLACEMENT_3D('',#234904,#125668,#125669);
#102686=AXIS2_PLACEMENT_3D('',#234912,#125670,#125671);
#102687=AXIS2_PLACEMENT_3D('',#234920,#125672,#125673);
#102688=AXIS2_PLACEMENT_3D('',#234928,#125674,#125675);
#102689=AXIS2_PLACEMENT_3D('',#234936,#125676,#125677);
#102690=AXIS2_PLACEMENT_3D('',#234944,#125678,#125679);
#102691=AXIS2_PLACEMENT_3D('',#234947,#125680,#125681);
#102692=AXIS2_PLACEMENT_3D('',#234949,#125682,#125683);
#102693=AXIS2_PLACEMENT_3D('',#234951,#125684,#125685);
#102694=AXIS2_PLACEMENT_3D('',#234953,#125686,#125687);
#102695=AXIS2_PLACEMENT_3D('',#234955,#125688,#125689);
#102696=AXIS2_PLACEMENT_3D('',#234956,#125690,#125691);
#102697=AXIS2_PLACEMENT_3D('',#234957,#125692,#125693);
#102698=AXIS2_PLACEMENT_3D('',#234965,#125694,#125695);
#102699=AXIS2_PLACEMENT_3D('',#234973,#125696,#125697);
#102700=AXIS2_PLACEMENT_3D('',#234981,#125698,#125699);
#102701=AXIS2_PLACEMENT_3D('',#234989,#125700,#125701);
#102702=AXIS2_PLACEMENT_3D('',#234997,#125702,#125703);
#102703=AXIS2_PLACEMENT_3D('',#235005,#125704,#125705);
#102704=AXIS2_PLACEMENT_3D('',#235008,#125708,#125709);
#102705=AXIS2_PLACEMENT_3D('',#235010,#125711,#125712);
#102706=AXIS2_PLACEMENT_3D('',#235012,#125714,#125715);
#102707=AXIS2_PLACEMENT_3D('',#235014,#125717,#125718);
#102708=AXIS2_PLACEMENT_3D('',#235016,#125720,#125721);
#102709=AXIS2_PLACEMENT_3D('',#235017,#125722,#125723);
#102710=AXIS2_PLACEMENT_3D('',#235030,#125726,#125727);
#102711=AXIS2_PLACEMENT_3D('',#235040,#125729,#125730);
#102712=AXIS2_PLACEMENT_3D('',#235050,#125732,#125733);
#102713=AXIS2_PLACEMENT_3D('',#235060,#125735,#125736);
#102714=AXIS2_PLACEMENT_3D('',#235070,#125738,#125739);
#102715=AXIS2_PLACEMENT_3D('',#235077,#125740,#125741);
#102716=AXIS2_PLACEMENT_3D('',#235080,#125743,#125744);
#102717=AXIS2_PLACEMENT_3D('',#235081,#125745,#125746);
#102718=AXIS2_PLACEMENT_3D('',#235082,#125747,#125748);
#102719=AXIS2_PLACEMENT_3D('',#235083,#125749,#125750);
#102720=AXIS2_PLACEMENT_3D('',#235084,#125751,#125752);
#102721=AXIS2_PLACEMENT_3D('',#235085,#125753,#125754);
#102722=AXIS2_PLACEMENT_3D('',#235086,#125755,#125756);
#102723=AXIS2_PLACEMENT_3D('',#235087,#125757,#125758);
#102724=AXIS2_PLACEMENT_3D('',#235088,#125759,#125760);
#102725=AXIS2_PLACEMENT_3D('',#235089,#125761,#125762);
#102726=AXIS2_PLACEMENT_3D('',#235090,#125763,#125764);
#102727=AXIS2_PLACEMENT_3D('',#235091,#125765,#125766);
#102728=AXIS2_PLACEMENT_3D('',#235092,#125767,#125768);
#102729=AXIS2_PLACEMENT_3D('',#235094,#125769,#125770);
#102730=AXIS2_PLACEMENT_3D('',#235096,#125771,#125772);
#102731=AXIS2_PLACEMENT_3D('',#235098,#125773,#125774);
#102732=AXIS2_PLACEMENT_3D('',#235099,#125775,#125776);
#102733=AXIS2_PLACEMENT_3D('',#235100,#125777,#125778);
#102734=AXIS2_PLACEMENT_3D('',#235102,#125779,#125780);
#102735=AXIS2_PLACEMENT_3D('',#235103,#125781,#125782);
#102736=AXIS2_PLACEMENT_3D('',#235104,#125783,#125784);
#102737=AXIS2_PLACEMENT_3D('',#235106,#125786,#125787);
#102738=AXIS2_PLACEMENT_3D('',#235109,#125788,#125789);
#102739=AXIS2_PLACEMENT_3D('',#235111,#125790,#125791);
#102740=AXIS2_PLACEMENT_3D('',#235113,#125793,#125794);
#102741=AXIS2_PLACEMENT_3D('',#235118,#125796,#125797);
#102742=AXIS2_PLACEMENT_3D('',#235119,#125798,#125799);
#102743=AXIS2_PLACEMENT_3D('',#235120,#125800,#125801);
#102744=AXIS2_PLACEMENT_3D('',#235122,#125802,#125803);
#102745=AXIS2_PLACEMENT_3D('',#235124,#125804,#125805);
#102746=AXIS2_PLACEMENT_3D('',#235125,#125806,#125807);
#102747=AXIS2_PLACEMENT_3D('',#235126,#125808,#125809);
#102748=AXIS2_PLACEMENT_3D('',#235130,#125811,#125812);
#102749=AXIS2_PLACEMENT_3D('',#235132,#125814,#125815);
#102750=AXIS2_PLACEMENT_3D('',#235134,#125816,#125817);
#102751=AXIS2_PLACEMENT_3D('',#235135,#125818,#125819);
#102752=AXIS2_PLACEMENT_3D('',#235136,#125820,#125821);
#102753=AXIS2_PLACEMENT_3D('',#235139,#125822,#125823);
#102754=AXIS2_PLACEMENT_3D('',#235146,#125824,#125825);
#102755=AXIS2_PLACEMENT_3D('',#235147,#125826,#125827);
#102756=AXIS2_PLACEMENT_3D('',#235148,#125828,#125829);
#102757=AXIS2_PLACEMENT_3D('',#235150,#125830,#125831);
#102758=AXIS2_PLACEMENT_3D('',#235151,#125832,#125833);
#102759=AXIS2_PLACEMENT_3D('',#235152,#125834,#125835);
#102760=AXIS2_PLACEMENT_3D('',#235154,#125836,#125837);
#102761=AXIS2_PLACEMENT_3D('',#235161,#125838,#125839);
#102762=AXIS2_PLACEMENT_3D('',#235164,#125840,#125841);
#102763=AXIS2_PLACEMENT_3D('',#235172,#125842,#125843);
#102764=AXIS2_PLACEMENT_3D('',#235173,#125844,#125845);
#102765=AXIS2_PLACEMENT_3D('',#235175,#125846,#125847);
#102766=AXIS2_PLACEMENT_3D('',#235176,#125848,#125849);
#102767=AXIS2_PLACEMENT_3D('',#235177,#125850,#125851);
#102768=AXIS2_PLACEMENT_3D('',#235180,#125852,#125853);
#102769=AXIS2_PLACEMENT_3D('',#235185,#125854,#125855);
#102770=AXIS2_PLACEMENT_3D('',#235186,#125856,#125857);
#102771=AXIS2_PLACEMENT_3D('',#235189,#125858,#125859);
#102772=AXIS2_PLACEMENT_3D('',#235197,#125860,#125861);
#102773=AXIS2_PLACEMENT_3D('',#235198,#125862,#125863);
#102774=AXIS2_PLACEMENT_3D('',#235205,#125864,#125865);
#102775=AXIS2_PLACEMENT_3D('',#235206,#125866,#125867);
#102776=AXIS2_PLACEMENT_3D('',#235207,#125868,#125869);
#102777=AXIS2_PLACEMENT_3D('',#235210,#125870,#125871);
#102778=AXIS2_PLACEMENT_3D('',#235214,#125873,#125874);
#102779=AXIS2_PLACEMENT_3D('',#235216,#125876,#125877);
#102780=AXIS2_PLACEMENT_3D('',#235219,#125878,#125879);
#102781=AXIS2_PLACEMENT_3D('',#235234,#125882,#125883);
#102782=AXIS2_PLACEMENT_3D('',#235237,#125886,#125887);
#102783=AXIS2_PLACEMENT_3D('',#235240,#125890,#125891);
#102784=AXIS2_PLACEMENT_3D('',#235251,#125898,#125899);
#102785=AXIS2_PLACEMENT_3D('',#235256,#125901,#125902);
#102786=AXIS2_PLACEMENT_3D('',#235257,#125903,#125904);
#102787=AXIS2_PLACEMENT_3D('',#235258,#125905,#125906);
#102788=AXIS2_PLACEMENT_3D('',#235261,#125907,#125908);
#102789=AXIS2_PLACEMENT_3D('',#235263,#125909,#125910);
#102790=AXIS2_PLACEMENT_3D('',#235265,#125912,#125913);
#102791=AXIS2_PLACEMENT_3D('',#235268,#125914,#125915);
#102792=AXIS2_PLACEMENT_3D('',#235269,#125916,#125917);
#102793=AXIS2_PLACEMENT_3D('',#235270,#125918,#125919);
#102794=AXIS2_PLACEMENT_3D('',#235271,#125920,#125921);
#102795=AXIS2_PLACEMENT_3D('',#235274,#125922,#125923);
#102796=AXIS2_PLACEMENT_3D('',#235277,#125926,#125927);
#102797=AXIS2_PLACEMENT_3D('',#235279,#125928,#125929);
#102798=AXIS2_PLACEMENT_3D('',#235280,#125930,#125931);
#102799=AXIS2_PLACEMENT_3D('',#235281,#125932,#125933);
#102800=AXIS2_PLACEMENT_3D('',#235284,#125934,#125935);
#102801=AXIS2_PLACEMENT_3D('',#235291,#125936,#125937);
#102802=AXIS2_PLACEMENT_3D('',#235292,#125938,#125939);
#102803=AXIS2_PLACEMENT_3D('',#235293,#125940,#125941);
#102804=AXIS2_PLACEMENT_3D('',#235295,#125942,#125943);
#102805=AXIS2_PLACEMENT_3D('',#235296,#125944,#125945);
#102806=AXIS2_PLACEMENT_3D('',#235297,#125946,#125947);
#102807=AXIS2_PLACEMENT_3D('',#235305,#125948,#125949);
#102808=AXIS2_PLACEMENT_3D('',#235306,#125950,#125951);
#102809=AXIS2_PLACEMENT_3D('',#235309,#125952,#125953);
#102810=AXIS2_PLACEMENT_3D('',#235317,#125954,#125955);
#102811=AXIS2_PLACEMENT_3D('',#235318,#125956,#125957);
#102812=AXIS2_PLACEMENT_3D('',#235320,#125958,#125959);
#102813=AXIS2_PLACEMENT_3D('',#235321,#125960,#125961);
#102814=AXIS2_PLACEMENT_3D('',#235322,#125962,#125963);
#102815=AXIS2_PLACEMENT_3D('',#235329,#125964,#125965);
#102816=AXIS2_PLACEMENT_3D('',#235330,#125966,#125967);
#102817=AXIS2_PLACEMENT_3D('',#235331,#125968,#125969);
#102818=AXIS2_PLACEMENT_3D('',#235334,#125970,#125971);
#102819=AXIS2_PLACEMENT_3D('',#235342,#125972,#125973);
#102820=AXIS2_PLACEMENT_3D('',#235343,#125974,#125975);
#102821=AXIS2_PLACEMENT_3D('',#235346,#125976,#125977);
#102822=AXIS2_PLACEMENT_3D('',#235351,#125978,#125979);
#102823=AXIS2_PLACEMENT_3D('',#235352,#125980,#125981);
#102824=AXIS2_PLACEMENT_3D('',#235355,#125982,#125983);
#102825=AXIS2_PLACEMENT_3D('',#235359,#125985,#125986);
#102826=AXIS2_PLACEMENT_3D('',#235361,#125988,#125989);
#102827=AXIS2_PLACEMENT_3D('',#235364,#125990,#125991);
#102828=AXIS2_PLACEMENT_3D('',#235445,#125994,#125995);
#102829=AXIS2_PLACEMENT_3D('',#235448,#125998,#125999);
#102830=AXIS2_PLACEMENT_3D('',#235451,#126002,#126003);
#102831=AXIS2_PLACEMENT_3D('',#235454,#126006,#126007);
#102832=AXIS2_PLACEMENT_3D('',#235457,#126010,#126011);
#102833=AXIS2_PLACEMENT_3D('',#235468,#126018,#126019);
#102834=AXIS2_PLACEMENT_3D('',#235470,#126020,#126021);
#102835=AXIS2_PLACEMENT_3D('',#235503,#126023,#126024);
#102836=AXIS2_PLACEMENT_3D('',#235514,#126025,#126026);
#102837=AXIS2_PLACEMENT_3D('',#235516,#126027,#126028);
#102838=AXIS2_PLACEMENT_3D('',#235518,#126030,#126031);
#102839=AXIS2_PLACEMENT_3D('',#235521,#126032,#126033);
#102840=AXIS2_PLACEMENT_3D('',#235522,#126034,#126035);
#102841=AXIS2_PLACEMENT_3D('',#235523,#126036,#126037);
#102842=AXIS2_PLACEMENT_3D('',#235524,#126038,#126039);
#102843=AXIS2_PLACEMENT_3D('',#235527,#126042,#126043);
#102844=AXIS2_PLACEMENT_3D('',#235529,#126044,#126045);
#102845=AXIS2_PLACEMENT_3D('',#235531,#126047,#126048);
#102846=AXIS2_PLACEMENT_3D('',#235534,#126049,#126050);
#102847=AXIS2_PLACEMENT_3D('',#235535,#126051,#126052);
#102848=AXIS2_PLACEMENT_3D('',#235536,#126053,#126054);
#102849=AXIS2_PLACEMENT_3D('',#235537,#126055,#126056);
#102850=AXIS2_PLACEMENT_3D('',#235540,#126059,#126060);
#102851=AXIS2_PLACEMENT_3D('',#235542,#126061,#126062);
#102852=AXIS2_PLACEMENT_3D('',#235544,#126064,#126065);
#102853=AXIS2_PLACEMENT_3D('',#235546,#126066,#126067);
#102854=AXIS2_PLACEMENT_3D('',#235548,#126069,#126070);
#102855=AXIS2_PLACEMENT_3D('',#235551,#126072,#126073);
#102856=AXIS2_PLACEMENT_3D('',#235553,#126074,#126075);
#102857=AXIS2_PLACEMENT_3D('',#235555,#126077,#126078);
#102858=AXIS2_PLACEMENT_3D('',#235557,#126079,#126080);
#102859=AXIS2_PLACEMENT_3D('',#235590,#126082,#126083);
#102860=AXIS2_PLACEMENT_3D('',#235601,#126084,#126085);
#102861=AXIS2_PLACEMENT_3D('',#235603,#126087,#126088);
#102862=AXIS2_PLACEMENT_3D('',#235605,#126089,#126090);
#102863=AXIS2_PLACEMENT_3D('',#235607,#126092,#126093);
#102864=AXIS2_PLACEMENT_3D('',#235610,#126094,#126095);
#102865=AXIS2_PLACEMENT_3D('',#235611,#126096,#126097);
#102866=AXIS2_PLACEMENT_3D('',#235612,#126098,#126099);
#102867=AXIS2_PLACEMENT_3D('',#235613,#126100,#126101);
#102868=AXIS2_PLACEMENT_3D('',#235616,#126104,#126105);
#102869=AXIS2_PLACEMENT_3D('',#235618,#126106,#126107);
#102870=AXIS2_PLACEMENT_3D('',#235620,#126109,#126110);
#102871=AXIS2_PLACEMENT_3D('',#235623,#126111,#126112);
#102872=AXIS2_PLACEMENT_3D('',#235624,#126113,#126114);
#102873=AXIS2_PLACEMENT_3D('',#235625,#126115,#126116);
#102874=AXIS2_PLACEMENT_3D('',#235626,#126117,#126118);
#102875=AXIS2_PLACEMENT_3D('',#235629,#126121,#126122);
#102876=AXIS2_PLACEMENT_3D('',#235632,#126125,#126126);
#102877=AXIS2_PLACEMENT_3D('',#235634,#126128,#126129);
#102878=AXIS2_PLACEMENT_3D('',#235636,#126131,#126132);
#102879=AXIS2_PLACEMENT_3D('',#235637,#126133,#126134);
#102880=AXIS2_PLACEMENT_3D('',#235638,#126135,#126136);
#102881=AXIS2_PLACEMENT_3D('',#235664,#126138,#126139);
#102882=AXIS2_PLACEMENT_3D('',#235693,#126140,#126141);
#102883=AXIS2_PLACEMENT_3D('',#235769,#126143,#126144);
#102884=AXIS2_PLACEMENT_3D('',#235847,#126146,#126147);
#102885=AXIS2_PLACEMENT_3D('',#235925,#126149,#126150);
#102886=AXIS2_PLACEMENT_3D('',#236001,#126152,#126153);
#102887=AXIS2_PLACEMENT_3D('',#236077,#126155,#126156);
#102888=AXIS2_PLACEMENT_3D('',#236153,#126158,#126159);
#102889=AXIS2_PLACEMENT_3D('',#236229,#126161,#126162);
#102890=AXIS2_PLACEMENT_3D('',#236307,#126164,#126165);
#102891=AXIS2_PLACEMENT_3D('',#236385,#126167,#126168);
#102892=AXIS2_PLACEMENT_3D('',#236461,#126170,#126171);
#102893=AXIS2_PLACEMENT_3D('',#236537,#126173,#126174);
#102894=AXIS2_PLACEMENT_3D('',#236613,#126176,#126177);
#102895=AXIS2_PLACEMENT_3D('',#236689,#126179,#126180);
#102896=AXIS2_PLACEMENT_3D('',#236765,#126182,#126183);
#102897=AXIS2_PLACEMENT_3D('',#236843,#126185,#126186);
#102898=AXIS2_PLACEMENT_3D('',#236921,#126188,#126189);
#102899=AXIS2_PLACEMENT_3D('',#236997,#126191,#126192);
#102900=AXIS2_PLACEMENT_3D('',#237025,#126194,#126195);
#102901=AXIS2_PLACEMENT_3D('',#237043,#126197,#126198);
#102902=AXIS2_PLACEMENT_3D('',#237062,#126199,#126200);
#102903=AXIS2_PLACEMENT_3D('',#237138,#126202,#126203);
#102904=AXIS2_PLACEMENT_3D('',#237216,#126205,#126206);
#102905=AXIS2_PLACEMENT_3D('',#237292,#126208,#126209);
#102906=AXIS2_PLACEMENT_3D('',#237368,#126211,#126212);
#102907=AXIS2_PLACEMENT_3D('',#237444,#126214,#126215);
#102908=AXIS2_PLACEMENT_3D('',#237520,#126217,#126218);
#102909=AXIS2_PLACEMENT_3D('',#237598,#126220,#126221);
#102910=AXIS2_PLACEMENT_3D('',#237674,#126223,#126224);
#102911=AXIS2_PLACEMENT_3D('',#237752,#126226,#126227);
#102912=AXIS2_PLACEMENT_3D('',#237828,#126229,#126230);
#102913=AXIS2_PLACEMENT_3D('',#237904,#126232,#126233);
#102914=AXIS2_PLACEMENT_3D('',#237980,#126235,#126236);
#102915=AXIS2_PLACEMENT_3D('',#238056,#126238,#126239);
#102916=AXIS2_PLACEMENT_3D('',#238134,#126241,#126242);
#102917=AXIS2_PLACEMENT_3D('',#238210,#126244,#126245);
#102918=AXIS2_PLACEMENT_3D('',#238288,#126247,#126248);
#102919=AXIS2_PLACEMENT_3D('',#238364,#126250,#126251);
#102920=AXIS2_PLACEMENT_3D('',#238410,#126253,#126254);
#102921=AXIS2_PLACEMENT_3D('',#238428,#126256,#126257);
#102922=AXIS2_PLACEMENT_3D('',#238473,#126259,#126260);
#102923=AXIS2_PLACEMENT_3D('',#238503,#126262,#126263);
#102924=AXIS2_PLACEMENT_3D('',#238533,#126265,#126266);
#102925=AXIS2_PLACEMENT_3D('',#238563,#126268,#126269);
#102926=AXIS2_PLACEMENT_3D('',#238593,#126271,#126272);
#102927=AXIS2_PLACEMENT_3D('',#238623,#126274,#126275);
#102928=AXIS2_PLACEMENT_3D('',#238653,#126277,#126278);
#102929=AXIS2_PLACEMENT_3D('',#238683,#126280,#126281);
#102930=AXIS2_PLACEMENT_3D('',#238713,#126283,#126284);
#102931=AXIS2_PLACEMENT_3D('',#238743,#126286,#126287);
#102932=AXIS2_PLACEMENT_3D('',#238773,#126289,#126290);
#102933=AXIS2_PLACEMENT_3D('',#238803,#126292,#126293);
#102934=AXIS2_PLACEMENT_3D('',#238833,#126295,#126296);
#102935=AXIS2_PLACEMENT_3D('',#238863,#126298,#126299);
#102936=AXIS2_PLACEMENT_3D('',#238893,#126301,#126302);
#102937=AXIS2_PLACEMENT_3D('',#238923,#126304,#126305);
#102938=AXIS2_PLACEMENT_3D('',#238953,#126307,#126308);
#102939=AXIS2_PLACEMENT_3D('',#238958,#126310,#126311);
#102940=AXIS2_PLACEMENT_3D('',#238964,#126312,#126313);
#102941=AXIS2_PLACEMENT_3D('',#238998,#126315,#126316);
#102942=AXIS2_PLACEMENT_3D('',#239035,#126317,#126318);
#102943=AXIS2_PLACEMENT_3D('',#239111,#126320,#126321);
#102944=AXIS2_PLACEMENT_3D('',#239187,#126323,#126324);
#102945=AXIS2_PLACEMENT_3D('',#239265,#126326,#126327);
#102946=AXIS2_PLACEMENT_3D('',#239341,#126329,#126330);
#102947=AXIS2_PLACEMENT_3D('',#239417,#126332,#126333);
#102948=AXIS2_PLACEMENT_3D('',#239495,#126335,#126336);
#102949=AXIS2_PLACEMENT_3D('',#239571,#126338,#126339);
#102950=AXIS2_PLACEMENT_3D('',#239647,#126341,#126342);
#102951=AXIS2_PLACEMENT_3D('',#239723,#126344,#126345);
#102952=AXIS2_PLACEMENT_3D('',#239801,#126347,#126348);
#102953=AXIS2_PLACEMENT_3D('',#239877,#126350,#126351);
#102954=AXIS2_PLACEMENT_3D('',#239953,#126353,#126354);
#102955=AXIS2_PLACEMENT_3D('',#240031,#126356,#126357);
#102956=AXIS2_PLACEMENT_3D('',#240107,#126359,#126360);
#102957=AXIS2_PLACEMENT_3D('',#240183,#126362,#126363);
#102958=AXIS2_PLACEMENT_3D('',#240259,#126365,#126366);
#102959=AXIS2_PLACEMENT_3D('',#240309,#126368,#126369);
#102960=AXIS2_PLACEMENT_3D('',#240344,#126370,#126371);
#102961=AXIS2_PLACEMENT_3D('',#240372,#126373,#126374);
#102962=AXIS2_PLACEMENT_3D('',#240417,#126376,#126377);
#102963=AXIS2_PLACEMENT_3D('',#240447,#126379,#126380);
#102964=AXIS2_PLACEMENT_3D('',#240477,#126382,#126383);
#102965=AXIS2_PLACEMENT_3D('',#240507,#126385,#126386);
#102966=AXIS2_PLACEMENT_3D('',#240537,#126388,#126389);
#102967=AXIS2_PLACEMENT_3D('',#240567,#126391,#126392);
#102968=AXIS2_PLACEMENT_3D('',#240597,#126394,#126395);
#102969=AXIS2_PLACEMENT_3D('',#240627,#126397,#126398);
#102970=AXIS2_PLACEMENT_3D('',#240657,#126400,#126401);
#102971=AXIS2_PLACEMENT_3D('',#240687,#126403,#126404);
#102972=AXIS2_PLACEMENT_3D('',#240717,#126406,#126407);
#102973=AXIS2_PLACEMENT_3D('',#240747,#126409,#126410);
#102974=AXIS2_PLACEMENT_3D('',#240777,#126412,#126413);
#102975=AXIS2_PLACEMENT_3D('',#240807,#126415,#126416);
#102976=AXIS2_PLACEMENT_3D('',#240837,#126418,#126419);
#102977=AXIS2_PLACEMENT_3D('',#240867,#126421,#126422);
#102978=AXIS2_PLACEMENT_3D('',#240897,#126424,#126425);
#102979=AXIS2_PLACEMENT_3D('',#240902,#126427,#126428);
#102980=AXIS2_PLACEMENT_3D('',#240908,#126429,#126430);
#102981=AXIS2_PLACEMENT_3D('',#240913,#126432,#126433);
#102982=AXIS2_PLACEMENT_3D('',#240924,#126434,#126435);
#102983=AXIS2_PLACEMENT_3D('',#241002,#126437,#126438);
#102984=AXIS2_PLACEMENT_3D('',#241078,#126440,#126441);
#102985=AXIS2_PLACEMENT_3D('',#241154,#126443,#126444);
#102986=AXIS2_PLACEMENT_3D('',#241230,#126446,#126447);
#102987=AXIS2_PLACEMENT_3D('',#241306,#126449,#126450);
#102988=AXIS2_PLACEMENT_3D('',#241382,#126452,#126453);
#102989=AXIS2_PLACEMENT_3D('',#241460,#126455,#126456);
#102990=AXIS2_PLACEMENT_3D('',#241538,#126458,#126459);
#102991=AXIS2_PLACEMENT_3D('',#241614,#126461,#126462);
#102992=AXIS2_PLACEMENT_3D('',#241690,#126464,#126465);
#102993=AXIS2_PLACEMENT_3D('',#241766,#126467,#126468);
#102994=AXIS2_PLACEMENT_3D('',#241842,#126470,#126471);
#102995=AXIS2_PLACEMENT_3D('',#241918,#126473,#126474);
#102996=AXIS2_PLACEMENT_3D('',#241998,#126476,#126477);
#102997=AXIS2_PLACEMENT_3D('',#242074,#126479,#126480);
#102998=AXIS2_PLACEMENT_3D('',#242150,#126482,#126483);
#102999=AXIS2_PLACEMENT_3D('',#242226,#126485,#126486);
#103000=AXIS2_PLACEMENT_3D('',#242290,#126488,#126489);
#103001=AXIS2_PLACEMENT_3D('',#242308,#126491,#126492);
#103002=AXIS2_PLACEMENT_3D('',#242353,#126494,#126495);
#103003=AXIS2_PLACEMENT_3D('',#242383,#126497,#126498);
#103004=AXIS2_PLACEMENT_3D('',#242413,#126500,#126501);
#103005=AXIS2_PLACEMENT_3D('',#242443,#126503,#126504);
#103006=AXIS2_PLACEMENT_3D('',#242473,#126506,#126507);
#103007=AXIS2_PLACEMENT_3D('',#242503,#126509,#126510);
#103008=AXIS2_PLACEMENT_3D('',#242533,#126512,#126513);
#103009=AXIS2_PLACEMENT_3D('',#242563,#126515,#126516);
#103010=AXIS2_PLACEMENT_3D('',#242593,#126518,#126519);
#103011=AXIS2_PLACEMENT_3D('',#242623,#126521,#126522);
#103012=AXIS2_PLACEMENT_3D('',#242653,#126524,#126525);
#103013=AXIS2_PLACEMENT_3D('',#242683,#126527,#126528);
#103014=AXIS2_PLACEMENT_3D('',#242713,#126530,#126531);
#103015=AXIS2_PLACEMENT_3D('',#242743,#126533,#126534);
#103016=AXIS2_PLACEMENT_3D('',#242773,#126536,#126537);
#103017=AXIS2_PLACEMENT_3D('',#242803,#126539,#126540);
#103018=AXIS2_PLACEMENT_3D('',#242833,#126542,#126543);
#103019=AXIS2_PLACEMENT_3D('',#242838,#126545,#126546);
#103020=AXIS2_PLACEMENT_3D('',#242844,#126547,#126548);
#103021=AXIS2_PLACEMENT_3D('',#242862,#126550,#126551);
#103022=AXIS2_PLACEMENT_3D('',#242907,#126553,#126554);
#103023=AXIS2_PLACEMENT_3D('',#242937,#126556,#126557);
#103024=AXIS2_PLACEMENT_3D('',#242967,#126559,#126560);
#103025=AXIS2_PLACEMENT_3D('',#242997,#126562,#126563);
#103026=AXIS2_PLACEMENT_3D('',#243027,#126565,#126566);
#103027=AXIS2_PLACEMENT_3D('',#243057,#126568,#126569);
#103028=AXIS2_PLACEMENT_3D('',#243087,#126571,#126572);
#103029=AXIS2_PLACEMENT_3D('',#243117,#126574,#126575);
#103030=AXIS2_PLACEMENT_3D('',#243147,#126577,#126578);
#103031=AXIS2_PLACEMENT_3D('',#243177,#126580,#126581);
#103032=AXIS2_PLACEMENT_3D('',#243207,#126583,#126584);
#103033=AXIS2_PLACEMENT_3D('',#243237,#126586,#126587);
#103034=AXIS2_PLACEMENT_3D('',#243267,#126589,#126590);
#103035=AXIS2_PLACEMENT_3D('',#243297,#126592,#126593);
#103036=AXIS2_PLACEMENT_3D('',#243327,#126595,#126596);
#103037=AXIS2_PLACEMENT_3D('',#243357,#126598,#126599);
#103038=AXIS2_PLACEMENT_3D('',#243387,#126601,#126602);
#103039=AXIS2_PLACEMENT_3D('',#243392,#126604,#126605);
#103040=AXIS2_PLACEMENT_3D('',#243398,#126606,#126607);
#103041=AXIS2_PLACEMENT_3D('',#243415,#126616,#126617);
#103042=AXIS2_PLACEMENT_3D('',#243420,#126619,#126620);
#103043=AXIS2_PLACEMENT_3D('',#243424,#126623,#126624);
#103044=AXIS2_PLACEMENT_3D('',#243425,#126625,#126626);
#103045=AXIS2_PLACEMENT_3D('',#243518,#126631,#126632);
#103046=AXIS2_PLACEMENT_3D('',#243527,#126637,#126638);
#103047=AXIS2_PLACEMENT_3D('',#243533,#126642,#126643);
#103048=AXIS2_PLACEMENT_3D('',#243539,#126647,#126648);
#103049=AXIS2_PLACEMENT_3D('',#243542,#126651,#126652);
#103050=AXIS2_PLACEMENT_3D('',#243546,#126654,#126655);
#103051=AXIS2_PLACEMENT_3D('',#243552,#126658,#126659);
#103052=AXIS2_PLACEMENT_3D('',#243555,#126661,#126662);
#103053=AXIS2_PLACEMENT_3D('',#243557,#126663,#126664);
#103054=AXIS2_PLACEMENT_3D('',#243727,#126667,#126668);
#103055=AXIS2_PLACEMENT_3D('',#243832,#126671,#126672);
#103056=AXIS2_PLACEMENT_3D('',#243833,#126673,#126674);
#103057=AXIS2_PLACEMENT_3D('',#243835,#126675,#126676);
#103058=AXIS2_PLACEMENT_3D('',#243837,#126677,#126678);
#103059=AXIS2_PLACEMENT_3D('',#243838,#126679,#126680);
#103060=AXIS2_PLACEMENT_3D('',#243841,#126682,#126683);
#103061=AXIS2_PLACEMENT_3D('',#243842,#126684,#126685);
#103062=AXIS2_PLACEMENT_3D('',#243844,#126687,#126688);
#103063=AXIS2_PLACEMENT_3D('',#243845,#126689,#126690);
#103064=AXIS2_PLACEMENT_3D('',#243847,#126691,#126692);
#103065=AXIS2_PLACEMENT_3D('',#243849,#126693,#126694);
#103066=AXIS2_PLACEMENT_3D('',#243850,#126695,#126696);
#103067=AXIS2_PLACEMENT_3D('',#243853,#126698,#126699);
#103068=AXIS2_PLACEMENT_3D('',#243854,#126700,#126701);
#103069=AXIS2_PLACEMENT_3D('',#243856,#126703,#126704);
#103070=AXIS2_PLACEMENT_3D('',#243857,#126705,#126706);
#103071=AXIS2_PLACEMENT_3D('',#243859,#126707,#126708);
#103072=AXIS2_PLACEMENT_3D('',#243861,#126709,#126710);
#103073=AXIS2_PLACEMENT_3D('',#243862,#126711,#126712);
#103074=AXIS2_PLACEMENT_3D('',#243865,#126714,#126715);
#103075=AXIS2_PLACEMENT_3D('',#243866,#126716,#126717);
#103076=AXIS2_PLACEMENT_3D('',#243905,#126719,#126720);
#103077=AXIS2_PLACEMENT_3D('',#243906,#126721,#126722);
#103078=AXIS2_PLACEMENT_3D('',#243908,#126723,#126724);
#103079=AXIS2_PLACEMENT_3D('',#243910,#126725,#126726);
#103080=AXIS2_PLACEMENT_3D('',#243911,#126727,#126728);
#103081=AXIS2_PLACEMENT_3D('',#243914,#126730,#126731);
#103082=AXIS2_PLACEMENT_3D('',#243915,#126732,#126733);
#103083=AXIS2_PLACEMENT_3D('',#243917,#126734,#126735);
#103084=AXIS2_PLACEMENT_3D('',#243919,#126737,#126738);
#103085=AXIS2_PLACEMENT_3D('',#243920,#126739,#126740);
#103086=AXIS2_PLACEMENT_3D('',#243921,#126741,#126742);
#103087=AXIS2_PLACEMENT_3D('',#243923,#126743,#126744);
#103088=AXIS2_PLACEMENT_3D('',#243924,#126745,#126746);
#103089=AXIS2_PLACEMENT_3D('',#243925,#126747,#126748);
#103090=AXIS2_PLACEMENT_3D('',#243926,#126749,#126750);
#103091=AXIS2_PLACEMENT_3D('',#243928,#126751,#126752);
#103092=AXIS2_PLACEMENT_3D('',#243930,#126753,#126754);
#103093=AXIS2_PLACEMENT_3D('',#243932,#126755,#126756);
#103094=AXIS2_PLACEMENT_3D('',#243933,#126757,#126758);
#103095=AXIS2_PLACEMENT_3D('',#243934,#126759,#126760);
#103096=AXIS2_PLACEMENT_3D('',#243937,#126761,#126762);
#103097=AXIS2_PLACEMENT_3D('',#243938,#126763,#126764);
#103098=AXIS2_PLACEMENT_3D('',#243940,#126765,#126766);
#103099=AXIS2_PLACEMENT_3D('',#243942,#126767,#126768);
#103100=AXIS2_PLACEMENT_3D('',#243943,#126769,#126770);
#103101=AXIS2_PLACEMENT_3D('',#243944,#126771,#126772);
#103102=AXIS2_PLACEMENT_3D('',#243957,#126775,#126776);
#103103=AXIS2_PLACEMENT_3D('',#243967,#126778,#126779);
#103104=AXIS2_PLACEMENT_3D('',#243977,#126781,#126782);
#103105=AXIS2_PLACEMENT_3D('',#243987,#126784,#126785);
#103106=AXIS2_PLACEMENT_3D('',#243997,#126787,#126788);
#103107=AXIS2_PLACEMENT_3D('',#244004,#126789,#126790);
#103108=AXIS2_PLACEMENT_3D('',#244007,#126792,#126793);
#103109=AXIS2_PLACEMENT_3D('',#244008,#126794,#126795);
#103110=AXIS2_PLACEMENT_3D('',#244009,#126796,#126797);
#103111=AXIS2_PLACEMENT_3D('',#244010,#126798,#126799);
#103112=AXIS2_PLACEMENT_3D('',#244011,#126800,#126801);
#103113=AXIS2_PLACEMENT_3D('',#244012,#126802,#126803);
#103114=AXIS2_PLACEMENT_3D('',#244013,#126804,#126805);
#103115=AXIS2_PLACEMENT_3D('',#244014,#126806,#126807);
#103116=AXIS2_PLACEMENT_3D('',#244015,#126808,#126809);
#103117=AXIS2_PLACEMENT_3D('',#244016,#126810,#126811);
#103118=AXIS2_PLACEMENT_3D('',#244017,#126812,#126813);
#103119=AXIS2_PLACEMENT_3D('',#244018,#126814,#126815);
#103120=AXIS2_PLACEMENT_3D('',#244019,#126816,#126817);
#103121=AXIS2_PLACEMENT_3D('',#244021,#126819,#126820);
#103122=AXIS2_PLACEMENT_3D('',#244022,#126821,#126822);
#103123=AXIS2_PLACEMENT_3D('',#246035,#126824,#126825);
#103124=AXIS2_PLACEMENT_3D('',#246037,#126826,#126827);
#103125=AXIS2_PLACEMENT_3D('',#246038,#126828,#126829);
#103126=AXIS2_PLACEMENT_3D('',#246083,#126830,#126831);
#103127=AXIS2_PLACEMENT_3D('',#246250,#126832,#126833);
#103128=AXIS2_PLACEMENT_3D('',#246251,#126834,#126835);
#103129=AXIS2_PLACEMENT_3D('',#246252,#126836,#126837);
#103130=AXIS2_PLACEMENT_3D('',#246267,#126838,#126839);
#103131=AXIS2_PLACEMENT_3D('',#246329,#126840,#126841);
#103132=AXIS2_PLACEMENT_3D('',#246600,#126842,#126843);
#103133=AXIS2_PLACEMENT_3D('',#246620,#126844,#126845);
#103134=AXIS2_PLACEMENT_3D('',#246703,#126848,#126849);
#103135=AXIS2_PLACEMENT_3D('',#246723,#126850,#126851);
#103136=AXIS2_PLACEMENT_3D('',#246928,#126853,#126854);
#103137=AXIS2_PLACEMENT_3D('',#247109,#126855,#126856);
#103138=AXIS2_PLACEMENT_3D('',#247110,#126857,#126858);
#103139=AXIS2_PLACEMENT_3D('',#247113,#126859,#126860);
#103140=AXIS2_PLACEMENT_3D('',#247117,#126863,#126864);
#103141=AXIS2_PLACEMENT_3D('',#247476,#126865,#126866);
#103142=AXIS2_PLACEMENT_3D('',#247478,#126867,#126868);
#103143=AXIS2_PLACEMENT_3D('',#247485,#126869,#126870);
#103144=AXIS2_PLACEMENT_3D('',#247488,#126871,#126872);
#103145=AXIS2_PLACEMENT_3D('',#247644,#126875,#126876);
#103146=AXIS2_PLACEMENT_3D('',#247646,#126877,#126878);
#103147=AXIS2_PLACEMENT_3D('',#247647,#126879,#126880);
#103148=AXIS2_PLACEMENT_3D('',#247662,#126881,#126882);
#103149=AXIS2_PLACEMENT_3D('',#247663,#126883,#126884);
#103150=AXIS2_PLACEMENT_3D('',#247664,#126885,#126886);
#103151=AXIS2_PLACEMENT_3D('',#247665,#126887,#126888);
#103152=AXIS2_PLACEMENT_3D('',#247667,#126889,#126890);
#103153=AXIS2_PLACEMENT_3D('',#247668,#126891,#126892);
#103154=AXIS2_PLACEMENT_3D('',#247669,#126893,#126894);
#103155=AXIS2_PLACEMENT_3D('',#247672,#126895,#126896);
#103156=AXIS2_PLACEMENT_3D('',#247712,#126899,#126900);
#103157=AXIS2_PLACEMENT_3D('',#247838,#126901,#126902);
#103158=AXIS2_PLACEMENT_3D('',#247853,#126904,#126905);
#103159=AXIS2_PLACEMENT_3D('',#247855,#126906,#126907);
#103160=AXIS2_PLACEMENT_3D('',#247856,#126908,#126909);
#103161=AXIS2_PLACEMENT_3D('',#247857,#126910,#126911);
#103162=AXIS2_PLACEMENT_3D('',#247859,#126912,#126913);
#103163=AXIS2_PLACEMENT_3D('',#247860,#126914,#126915);
#103164=AXIS2_PLACEMENT_3D('',#247861,#126916,#126917);
#103165=AXIS2_PLACEMENT_3D('',#247864,#126918,#126919);
#103166=AXIS2_PLACEMENT_3D('',#247904,#126922,#126923);
#103167=AXIS2_PLACEMENT_3D('',#247961,#126924,#126925);
#103168=AXIS2_PLACEMENT_3D('',#247963,#126927,#126928);
#103169=AXIS2_PLACEMENT_3D('',#247967,#126929,#126930);
#103170=AXIS2_PLACEMENT_3D('',#247968,#126931,#126932);
#103171=AXIS2_PLACEMENT_3D('',#247969,#126933,#126934);
#103172=AXIS2_PLACEMENT_3D('',#247970,#126935,#126936);
#103173=AXIS2_PLACEMENT_3D('',#247971,#126937,#126938);
#103174=AXIS2_PLACEMENT_3D('',#247972,#126939,#126940);
#103175=AXIS2_PLACEMENT_3D('',#247977,#126942,#126943);
#103176=AXIS2_PLACEMENT_3D('',#247996,#126945,#126946);
#103177=AXIS2_PLACEMENT_3D('',#248001,#126948,#126949);
#103178=AXIS2_PLACEMENT_3D('',#248020,#126951,#126952);
#103179=AXIS2_PLACEMENT_3D('',#248025,#126954,#126955);
#103180=AXIS2_PLACEMENT_3D('',#248057,#126957,#126958);
#103181=AXIS2_PLACEMENT_3D('',#248059,#126959,#126960);
#103182=AXIS2_PLACEMENT_3D('',#248073,#126961,#126962);
#103183=AXIS2_PLACEMENT_3D('',#248078,#126964,#126965);
#103184=AXIS2_PLACEMENT_3D('',#248087,#126967,#126968);
#103185=AXIS2_PLACEMENT_3D('',#248092,#126970,#126971);
#103186=AXIS2_PLACEMENT_3D('',#248101,#126973,#126974);
#103187=AXIS2_PLACEMENT_3D('',#248126,#126976,#126977);
#103188=AXIS2_PLACEMENT_3D('',#248128,#126978,#126979);
#103189=AXIS2_PLACEMENT_3D('',#248145,#126980,#126981);
#103190=AXIS2_PLACEMENT_3D('',#248146,#126982,#126983);
#103191=AXIS2_PLACEMENT_3D('',#248147,#126984,#126985);
#103192=AXIS2_PLACEMENT_3D('',#248167,#126986,#126987);
#103193=AXIS2_PLACEMENT_3D('',#248169,#126988,#126989);
#103194=AXIS2_PLACEMENT_3D('',#248186,#126990,#126991);
#103195=AXIS2_PLACEMENT_3D('',#248205,#126993,#126994);
#103196=AXIS2_PLACEMENT_3D('',#248207,#126995,#126996);
#103197=AXIS2_PLACEMENT_3D('',#248221,#126997,#126998);
#103198=AXIS2_PLACEMENT_3D('',#248226,#127000,#127001);
#103199=AXIS2_PLACEMENT_3D('',#248235,#127003,#127004);
#103200=AXIS2_PLACEMENT_3D('',#248240,#127006,#127007);
#103201=AXIS2_PLACEMENT_3D('',#248249,#127009,#127010);
#103202=AXIS2_PLACEMENT_3D('',#248276,#127013,#127014);
#103203=AXIS2_PLACEMENT_3D('',#248278,#127015,#127016);
#103204=AXIS2_PLACEMENT_3D('',#248295,#127017,#127018);
#103205=AXIS2_PLACEMENT_3D('',#248296,#127019,#127020);
#103206=AXIS2_PLACEMENT_3D('',#248297,#127021,#127022);
#103207=AXIS2_PLACEMENT_3D('',#248317,#127023,#127024);
#103208=AXIS2_PLACEMENT_3D('',#248319,#127025,#127026);
#103209=AXIS2_PLACEMENT_3D('',#248336,#127027,#127028);
#103210=AXIS2_PLACEMENT_3D('',#248355,#127030,#127031);
#103211=AXIS2_PLACEMENT_3D('',#248357,#127032,#127033);
#103212=AXIS2_PLACEMENT_3D('',#248411,#127034,#127035);
#103213=AXIS2_PLACEMENT_3D('',#248412,#127036,#127037);
#103214=AXIS2_PLACEMENT_3D('',#248453,#127038,#127039);
#103215=AXIS2_PLACEMENT_3D('',#248454,#127040,#127041);
#103216=AXIS2_PLACEMENT_3D('',#248495,#127042,#127043);
#103217=AXIS2_PLACEMENT_3D('',#248521,#127046,#127047);
#103218=AXIS2_PLACEMENT_3D('',#248522,#127048,#127049);
#103219=AXIS2_PLACEMENT_3D('',#248548,#127052,#127053);
#103220=AXIS2_PLACEMENT_3D('',#248549,#127054,#127055);
#103221=AXIS2_PLACEMENT_3D('',#248575,#127058,#127059);
#103222=AXIS2_PLACEMENT_3D('',#248576,#127060,#127061);
#103223=AXIS2_PLACEMENT_3D('',#248602,#127064,#127065);
#103224=AXIS2_PLACEMENT_3D('',#248603,#127066,#127067);
#103225=AXIS2_PLACEMENT_3D('',#248604,#127068,#127069);
#103226=AXIS2_PLACEMENT_3D('',#248605,#127070,#127071);
#103227=AXIS2_PLACEMENT_3D('',#248619,#127072,#127073);
#103228=AXIS2_PLACEMENT_3D('',#248634,#127074,#127075);
#103229=AXIS2_PLACEMENT_3D('',#248635,#127076,#127077);
#103230=AXIS2_PLACEMENT_3D('',#248664,#127080,#127081);
#103231=AXIS2_PLACEMENT_3D('',#248665,#127082,#127083);
#103232=AXIS2_PLACEMENT_3D('',#248694,#127086,#127087);
#103233=AXIS2_PLACEMENT_3D('',#248695,#127088,#127089);
#103234=AXIS2_PLACEMENT_3D('',#248720,#127091,#127092);
#103235=AXIS2_PLACEMENT_3D('',#248738,#127093,#127094);
#103236=AXIS2_PLACEMENT_3D('',#248739,#127095,#127096);
#103237=AXIS2_PLACEMENT_3D('',#248740,#127097,#127098);
#103238=AXIS2_PLACEMENT_3D('',#248741,#127099,#127100);
#103239=AXIS2_PLACEMENT_3D('',#248761,#127101,#127102);
#103240=AXIS2_PLACEMENT_3D('',#248779,#127103,#127104);
#103241=AXIS2_PLACEMENT_3D('',#248780,#127105,#127106);
#103242=AXIS2_PLACEMENT_3D('',#248799,#127108,#127109);
#103243=AXIS2_PLACEMENT_3D('',#248814,#127110,#127111);
#103244=AXIS2_PLACEMENT_3D('',#248815,#127112,#127113);
#103245=AXIS2_PLACEMENT_3D('',#248816,#127114,#127115);
#103246=AXIS2_PLACEMENT_3D('',#248817,#127116,#127117);
#103247=AXIS2_PLACEMENT_3D('',#248831,#127118,#127119);
#103248=AXIS2_PLACEMENT_3D('',#248846,#127120,#127121);
#103249=AXIS2_PLACEMENT_3D('',#248847,#127122,#127123);
#103250=AXIS2_PLACEMENT_3D('',#248876,#127126,#127127);
#103251=AXIS2_PLACEMENT_3D('',#248877,#127128,#127129);
#103252=AXIS2_PLACEMENT_3D('',#248906,#127132,#127133);
#103253=AXIS2_PLACEMENT_3D('',#248907,#127134,#127135);
#103254=AXIS2_PLACEMENT_3D('',#248932,#127137,#127138);
#103255=AXIS2_PLACEMENT_3D('',#248950,#127139,#127140);
#103256=AXIS2_PLACEMENT_3D('',#248951,#127141,#127142);
#103257=AXIS2_PLACEMENT_3D('',#248952,#127143,#127144);
#103258=AXIS2_PLACEMENT_3D('',#248953,#127145,#127146);
#103259=AXIS2_PLACEMENT_3D('',#248973,#127147,#127148);
#103260=AXIS2_PLACEMENT_3D('',#248991,#127149,#127150);
#103261=AXIS2_PLACEMENT_3D('',#248992,#127151,#127152);
#103262=AXIS2_PLACEMENT_3D('',#249011,#127154,#127155);
#103263=AXIS2_PLACEMENT_3D('',#249026,#127156,#127157);
#103264=AXIS2_PLACEMENT_3D('',#249027,#127158,#127159);
#103265=AXIS2_PLACEMENT_3D('',#249028,#127160,#127161);
#103266=AXIS2_PLACEMENT_3D('',#249029,#127162,#127163);
#103267=AXIS2_PLACEMENT_3D('',#249030,#127164,#127165);
#103268=AXIS2_PLACEMENT_3D('',#249031,#127166,#127167);
#103269=AXIS2_PLACEMENT_3D('',#249032,#127168,#127169);
#103270=AXIS2_PLACEMENT_3D('',#249033,#127170,#127171);
#103271=AXIS2_PLACEMENT_3D('',#249034,#127172,#127173);
#103272=AXIS2_PLACEMENT_3D('',#249035,#127174,#127175);
#103273=AXIS2_PLACEMENT_3D('',#249036,#127176,#127177);
#103274=AXIS2_PLACEMENT_3D('',#249037,#127178,#127179);
#103275=AXIS2_PLACEMENT_3D('',#249038,#127180,#127181);
#103276=AXIS2_PLACEMENT_3D('',#249039,#127182,#127183);
#103277=AXIS2_PLACEMENT_3D('',#249040,#127184,#127185);
#103278=AXIS2_PLACEMENT_3D('',#249069,#127186,#127187);
#103279=AXIS2_PLACEMENT_3D('',#249070,#127188,#127189);
#103280=AXIS2_PLACEMENT_3D('',#249130,#127190,#127191);
#103281=AXIS2_PLACEMENT_3D('',#249131,#127192,#127193);
#103282=AXIS2_PLACEMENT_3D('',#249163,#127194,#127195);
#103283=AXIS2_PLACEMENT_3D('',#249166,#127197,#127198);
#103284=AXIS2_PLACEMENT_3D('',#249167,#127199,#127200);
#103285=AXIS2_PLACEMENT_3D('',#249168,#127201,#127202);
#103286=AXIS2_PLACEMENT_3D('',#249169,#127203,#127204);
#103287=AXIS2_PLACEMENT_3D('',#249170,#127205,#127206);
#103288=AXIS2_PLACEMENT_3D('',#249171,#127207,#127208);
#103289=AXIS2_PLACEMENT_3D('',#250187,#127209,#127210);
#103290=AXIS2_PLACEMENT_3D('',#251467,#127213,#127214);
#103291=AXIS2_PLACEMENT_3D('',#252037,#127217,#127218);
#103292=AXIS2_PLACEMENT_3D('',#252038,#127219,#127220);
#103293=AXIS2_PLACEMENT_3D('',#254404,#127221,#127222);
#103294=AXIS2_PLACEMENT_3D('',#255719,#127224,#127225);
#103295=AXIS2_PLACEMENT_3D('',#256139,#127228,#127229);
#103296=AXIS2_PLACEMENT_3D('',#258537,#127230,#127231);
#103297=AXIS2_PLACEMENT_3D('',#258652,#127232,#127233);
#103298=AXIS2_PLACEMENT_3D('',#259889,#127235,#127236);
#103299=AXIS2_PLACEMENT_3D('',#260277,#127239,#127240);
#103300=AXIS2_PLACEMENT_3D('',#262605,#127241,#127242);
#103301=AXIS2_PLACEMENT_3D('',#262658,#127243,#127244);
#103302=AXIS2_PLACEMENT_3D('',#263854,#127247,#127248);
#103303=AXIS2_PLACEMENT_3D('',#264398,#127251,#127252);
#103304=AXIS2_PLACEMENT_3D('',#264399,#127253,#127254);
#103305=AXIS2_PLACEMENT_3D('',#264428,#127255,#127256);
#103306=AXIS2_PLACEMENT_3D('',#266693,#127257,#127258);
#103307=AXIS2_PLACEMENT_3D('',#266694,#127259,#127260);
#103308=AXIS2_PLACEMENT_3D('',#266705,#127261,#127262);
#103309=AXIS2_PLACEMENT_3D('',#266970,#127263,#127264);
#103310=AXIS2_PLACEMENT_3D('',#271074,#127267,#127268);
#103311=AXIS2_PLACEMENT_3D('',#271075,#127269,#127270);
#103312=AXIS2_PLACEMENT_3D('',#271079,#127273,#127274);
#103313=AXIS2_PLACEMENT_3D('',#271080,#127275,#127276);
#103314=AXIS2_PLACEMENT_3D('',#271129,#127277,#127278);
#103315=AXIS2_PLACEMENT_3D('',#271178,#127279,#127280);
#103316=AXIS2_PLACEMENT_3D('',#271179,#127281,#127282);
#103317=AXIS2_PLACEMENT_3D('',#271180,#127283,#127284);
#103318=AXIS2_PLACEMENT_3D('',#271181,#127285,#127286);
#103319=AXIS2_PLACEMENT_3D('',#271182,#127287,#127288);
#103320=AXIS2_PLACEMENT_3D('',#271183,#127289,#127290);
#103321=AXIS2_PLACEMENT_3D('',#271184,#127291,#127292);
#103322=AXIS2_PLACEMENT_3D('',#271185,#127293,#127294);
#103323=AXIS2_PLACEMENT_3D('',#271186,#127295,#127296);
#103324=AXIS2_PLACEMENT_3D('',#271187,#127297,#127298);
#103325=AXIS2_PLACEMENT_3D('',#271188,#127299,#127300);
#103326=AXIS2_PLACEMENT_3D('',#271189,#127301,#127302);
#103327=AXIS2_PLACEMENT_3D('',#271190,#127303,#127304);
#103328=AXIS2_PLACEMENT_3D('',#271191,#127305,#127306);
#103329=AXIS2_PLACEMENT_3D('',#271192,#127307,#127308);
#103330=AXIS2_PLACEMENT_3D('',#271193,#127309,#127310);
#103331=AXIS2_PLACEMENT_3D('',#271194,#127311,#127312);
#105182=DIRECTION('axis',(0.,0.,1.));
#105183=DIRECTION('refdir',(1.,0.,0.));
#105184=DIRECTION('center_axis',(0.,0.,-1.));
#105185=DIRECTION('ref_axis',(1.,0.,0.));
#105186=DIRECTION('center_axis',(0.,0.,1.));
#105187=DIRECTION('ref_axis',(-1.,0.,0.));
#105188=DIRECTION('',(0.707106781186552,-8.65956056235499E-17,0.707106781186543));
#105189=DIRECTION('center_axis',(0.,0.,-1.));
#105190=DIRECTION('ref_axis',(-1.,0.,0.));
#105191=DIRECTION('center_axis',(0.,0.,1.));
#105192=DIRECTION('ref_axis',(1.,0.,0.));
#105193=DIRECTION('center_axis',(0.,0.,-1.));
#105194=DIRECTION('ref_axis',(1.,0.,0.));
#105195=DIRECTION('center_axis',(0.,0.,-1.));
#105196=DIRECTION('ref_axis',(-1.,0.,0.));
#105197=DIRECTION('',(0.,0.,1.));
#105198=DIRECTION('center_axis',(0.,1.23467863058847E-16,-1.));
#105199=DIRECTION('ref_axis',(-1.,0.,0.));
#105200=DIRECTION('center_axis',(0.,0.,1.));
#105201=DIRECTION('ref_axis',(0.,1.,0.));
#105202=DIRECTION('center_axis',(0.,0.,-1.));
#105203=DIRECTION('ref_axis',(1.,0.,0.));
#105204=DIRECTION('center_axis',(0.,0.,-1.));
#105205=DIRECTION('ref_axis',(-1.,0.,0.));
#105206=DIRECTION('',(0.,0.,1.));
#105207=DIRECTION('center_axis',(0.,0.,1.));
#105208=DIRECTION('ref_axis',(1.,0.,0.));
#105209=DIRECTION('center_axis',(0.,0.,-1.));
#105210=DIRECTION('ref_axis',(-1.,0.,0.));
#105211=DIRECTION('center_axis',(0.,0.,-1.));
#105212=DIRECTION('ref_axis',(1.,0.,0.));
#105213=DIRECTION('',(-0.707106781186552,8.65956056235499E-17,0.707106781186543));
#105214=DIRECTION('center_axis',(0.,0.,1.));
#105215=DIRECTION('ref_axis',(1.,0.,0.));
#105216=DIRECTION('center_axis',(0.,0.,1.));
#105217=DIRECTION('ref_axis',(1.,0.,0.));
#105218=DIRECTION('center_axis',(0.,0.,-1.));
#105219=DIRECTION('ref_axis',(-1.,0.,0.));
#105220=DIRECTION('center_axis',(0.,0.,1.));
#105221=DIRECTION('ref_axis',(1.,0.,0.));
#105222=DIRECTION('',(0.,0.,1.));
#105223=DIRECTION('center_axis',(0.,1.23467863058847E-16,-1.));
#105224=DIRECTION('ref_axis',(-1.,0.,0.));
#105225=DIRECTION('center_axis',(0.,0.,-1.));
#105226=DIRECTION('ref_axis',(0.,1.,0.));
#105227=DIRECTION('center_axis',(0.,0.,-1.));
#105228=DIRECTION('ref_axis',(-1.,0.,0.));
#105229=DIRECTION('center_axis',(0.,0.,1.));
#105230=DIRECTION('ref_axis',(1.,0.,0.));
#105231=DIRECTION('',(0.,0.,1.));
#105232=DIRECTION('center_axis',(0.,0.,1.));
#105233=DIRECTION('ref_axis',(1.,0.,0.));
#105234=DIRECTION('center_axis',(0.,0.,-1.));
#105235=DIRECTION('ref_axis',(0.,1.,0.));
#105236=DIRECTION('',(-1.54660695142382E-33,-1.23467863058847E-16,1.));
#105237=DIRECTION('center_axis',(0.,0.,1.));
#105238=DIRECTION('ref_axis',(0.,1.,0.));
#105239=DIRECTION('',(0.,1.23467863058847E-16,-1.));
#105240=DIRECTION('center_axis',(0.,0.,1.));
#105241=DIRECTION('ref_axis',(1.,0.,0.));
#105242=DIRECTION('center_axis',(0.,0.,-1.));
#105243=DIRECTION('ref_axis',(0.,1.,0.));
#105244=DIRECTION('center_axis',(0.,0.,1.));
#105245=DIRECTION('ref_axis',(1.,0.,0.));
#105246=DIRECTION('',(0.,-1.23467863058847E-16,1.));
#105247=DIRECTION('center_axis',(0.,0.,1.));
#105248=DIRECTION('ref_axis',(0.,1.,0.));
#105249=DIRECTION('',(-5.86299591403052E-36,1.23467863058847E-16,-1.));
#105250=DIRECTION('center_axis',(0.,0.,-1.));
#105251=DIRECTION('ref_axis',(1.,0.,0.));
#105252=DIRECTION('center_axis',(-0.911086081553275,0.412216147184822,0.));
#105253=DIRECTION('ref_axis',(-0.412216147184823,-0.911086081553275,0.));
#105254=DIRECTION('center_axis',(-0.970284356147939,0.241967494127993,-1.34486472837252E-14));
#105255=DIRECTION('ref_axis',(-0.241967494127993,-0.970284356147939,-2.62269727666659E-30));
#105256=DIRECTION('center_axis',(0.,0.,-1.));
#105257=DIRECTION('ref_axis',(1.,-5.55111512312579E-15,0.));
#105258=DIRECTION('center_axis',(-0.919081670180344,0.0804092269952343,
-0.385776152389619));
#105259=DIRECTION('ref_axis',(-0.387029378450866,1.43097488374089E-17,0.922067383771889));
#105260=DIRECTION('center_axis',(5.61645494961161E-33,0.,-1.));
#105261=DIRECTION('ref_axis',(0.,1.,0.));
#105262=DIRECTION('',(-6.15711282612512E-33,-1.23467863058847E-16,1.));
#105263=DIRECTION('center_axis',(0.,0.,-1.));
#105264=DIRECTION('ref_axis',(0.,1.,0.));
#105265=DIRECTION('',(1.23259516440783E-32,1.23467863058847E-16,-1.));
#105266=DIRECTION('center_axis',(0.,0.,-1.));
#105267=DIRECTION('ref_axis',(0.,1.,0.));
#105268=DIRECTION('center_axis',(-0.0871557427476402,-0.996194698091747,
-1.22998030563942E-16));
#105269=DIRECTION('ref_axis',(-0.996194698091747,0.0871557427476402,1.12142775393191E-33));
#105270=DIRECTION('',(-0.996194698091747,0.0871557427476402,1.07609333103578E-17));
#105271=DIRECTION('',(-6.16356212163056E-32,1.23467863058847E-16,-1.));
#105272=DIRECTION('',(-0.996194698091747,0.0871557427476402,1.54074395550979E-33));
#105273=DIRECTION('',(6.16356212163056E-32,-1.23467863058847E-16,1.));
#105274=DIRECTION('',(-0.996194698091747,0.0871557427476402,1.07609333103578E-17));
#105275=DIRECTION('',(-6.16356212163056E-32,1.23467863058847E-16,-1.));
#105276=DIRECTION('',(0.996194698091747,-0.0871557427476402,0.));
#105277=DIRECTION('',(-0.996194698091747,0.0871557427476402,1.07609333103578E-17));
#105278=DIRECTION('',(1.13659195805196E-16,1.13523971920422E-16,-1.));
#105279=DIRECTION('',(-0.996194698091747,0.0871557427476402,1.54074395550979E-33));
#105280=DIRECTION('',(1.13659195805196E-16,-1.33411754197273E-16,1.));
#105281=DIRECTION('center_axis',(0.,1.23467863058847E-16,-1.));
#105282=DIRECTION('ref_axis',(0.,1.,0.));
#105283=DIRECTION('center_axis',(0.996194698091747,-0.0871557427476394,
-1.20952890408421E-15));
#105284=DIRECTION('ref_axis',(0.0871557427476394,0.996194698091747,1.39857739234396E-32));
#105285=DIRECTION('center_axis',(0.707106781186544,-0.707106781186551,0.));
#105286=DIRECTION('ref_axis',(0.707106781186551,0.707106781186544,0.));
#105287=DIRECTION('center_axis',(0.,0.,1.));
#105288=DIRECTION('ref_axis',(0.,1.,0.));
#105289=DIRECTION('center_axis',(-1.35502005093696E-32,0.,-1.));
#105290=DIRECTION('ref_axis',(0.,1.,0.));
#105291=DIRECTION('',(8.71576399210526E-33,-1.23467863058847E-16,1.));
#105292=DIRECTION('center_axis',(-2.85576800769162E-31,6.6052904065149E-46,
-1.));
#105293=DIRECTION('ref_axis',(2.31296463463574E-15,1.,3.11150763893057E-61));
#105294=DIRECTION('',(1.54660695142382E-33,1.23467863058847E-16,-1.));
#105295=DIRECTION('center_axis',(-2.85576800769162E-31,6.6052904065149E-46,
-1.));
#105296=DIRECTION('ref_axis',(2.31296463463574E-15,1.,3.11150763893057E-61));
#105297=DIRECTION('center_axis',(-0.707106781186548,-0.707106781186547,
-8.7304963227523E-17));
#105298=DIRECTION('ref_axis',(-0.707106781186547,0.707106781186548,3.47167550285579E-33));
#105299=DIRECTION('',(0.707106781186547,-0.707106781186548,0.));
#105300=DIRECTION('',(-0.707106781186547,0.707106781186548,8.73049632275231E-17));
#105301=DIRECTION('center_axis',(0.,1.23467863058847E-16,-1.));
#105302=DIRECTION('ref_axis',(0.,1.,0.));
#105303=DIRECTION('center_axis',(0.707106781186548,-0.707106781186548,0.));
#105304=DIRECTION('ref_axis',(0.707106781186548,0.707106781186548,0.));
#105305=DIRECTION('center_axis',(0.0871557427476394,-0.996194698091747,
0.));
#105306=DIRECTION('ref_axis',(0.996194698091747,0.0871557427476394,0.));
#105307=DIRECTION('center_axis',(0.,0.,1.));
#105308=DIRECTION('ref_axis',(0.,1.,0.));
#105309=DIRECTION('center_axis',(-0.996194698091747,-0.0871557427476402,
-1.07609333103578E-17));
#105310=DIRECTION('ref_axis',(-0.0871557427476402,0.996194698091747,1.81609423396931E-34));
#105311=DIRECTION('',(-0.0871557427476402,0.996194698091747,1.22998030563942E-16));
#105312=DIRECTION('',(1.08020383274181E-17,4.42963887209064E-33,-1.));
#105313=DIRECTION('',(-0.0871557427476402,0.996194698091747,0.));
#105314=DIRECTION('',(-1.08020383274181E-17,-4.42963887209064E-33,1.));
#105315=DIRECTION('',(-0.0871557427476402,0.996194698091747,1.22998030563942E-16));
#105316=DIRECTION('',(1.08020383274181E-17,4.42963887209064E-33,-1.));
#105317=DIRECTION('',(-0.0871557427476402,0.996194698091747,0.));
#105318=DIRECTION('',(-1.08020383274181E-17,-4.62223186652937E-33,1.));
#105319=DIRECTION('',(-0.0871557427476402,0.996194698091747,1.22998030563942E-16));
#105320=DIRECTION('',(0.0871557427476402,-0.996194698091747,0.));
#105321=DIRECTION('center_axis',(-0.996194698091748,-0.0871557427476319,
-1.23112093893486E-14));
#105322=DIRECTION('ref_axis',(0.0399152964550247,-0.45623392616117,-0.888964213975159));
#105323=DIRECTION('',(-1.08020383274181E-17,-4.42963887209064E-33,1.));
#105324=DIRECTION('center_axis',(0.,-1.38777878078144E-14,1.));
#105325=DIRECTION('ref_axis',(0.,1.,1.38777878078144E-14));
#105326=DIRECTION('center_axis',(0.999990739418254,-0.00427492665558239,
-0.00049606433434234));
#105327=DIRECTION('ref_axis',(0.00427492718156908,0.999990862457049,1.90763185875202E-22));
#105328=DIRECTION('center_axis',(0.,0.,-1.));
#105329=DIRECTION('ref_axis',(0.,1.,0.));
#105330=DIRECTION('center_axis',(0.,0.,1.));
#105331=DIRECTION('ref_axis',(1.,0.,0.));
#105332=DIRECTION('',(6.19323182390956E-32,-1.23467863058847E-16,1.));
#105333=DIRECTION('',(0.,1.23467863058847E-16,-1.));
#105334=DIRECTION('center_axis',(0.,-1.23467863058847E-16,1.));
#105335=DIRECTION('ref_axis',(0.,-1.,-1.21694324257719E-16));
#105336=DIRECTION('center_axis',(-1.73309037721552E-31,-1.19033121480991E-16,
1.));
#105337=DIRECTION('ref_axis',(3.90798504668055E-14,-1.,-1.19033121480991E-16));
#105338=DIRECTION('center_axis',(0.999944632572398,0.0105228573644618,3.55322387352642E-5));
#105339=DIRECTION('ref_axis',(0.00955105836032764,-0.906170827987028,-0.422803982702979));
#105340=DIRECTION('center_axis',(0.,1.18842113532929E-16,-1.));
#105341=DIRECTION('ref_axis',(0.,-1.,-1.18842113532929E-16));
#105342=DIRECTION('center_axis',(-0.998402993028371,-0.0564930323058765,
-2.85110252341697E-5));
#105343=DIRECTION('ref_axis',(0.0553356758873256,-0.977847117549328,-0.201873667610621));
#105344=DIRECTION('center_axis',(0.,0.,-1.));
#105345=DIRECTION('ref_axis',(0.,1.,0.));
#105346=DIRECTION('center_axis',(-5.55111512312579E-13,6.5495003047383E-14,
1.));
#105347=DIRECTION('ref_axis',(1.,7.99467207819295E-41,5.55111512312579E-13));
#105348=DIRECTION('',(-6.19323182390956E-32,1.23467863058847E-16,-1.));
#105349=DIRECTION('center_axis',(0.,0.,1.));
#105350=DIRECTION('ref_axis',(1.,0.,0.));
#105351=DIRECTION('center_axis',(0.,0.,1.));
#105352=DIRECTION('ref_axis',(1.,0.,0.));
#105353=DIRECTION('',(0.,-1.23467863058847E-16,1.));
#105354=DIRECTION('center_axis',(-5.55111512312579E-13,6.5495003047383E-14,
1.));
#105355=DIRECTION('ref_axis',(1.,7.99467207819295E-41,5.55111512312579E-13));
#105356=DIRECTION('center_axis',(-0.99074835547853,0.134685218959648,0.0166609696710313));
#105357=DIRECTION('ref_axis',(-0.13470391634661,-0.99088589399632,2.11341644556228E-18));
#105358=DIRECTION('center_axis',(0.003518046819505,0.149207652782245,-0.988799625656174));
#105359=DIRECTION('ref_axis',(-0.14424605496163,-0.978388820119907,-0.148149898050531));
#105360=DIRECTION('center_axis',(-0.989538255790606,0.14315195982541,0.0179320028170335));
#105361=DIRECTION('ref_axis',(-0.143174981115239,-0.989697390510176,-2.48873089681965E-18));
#105362=DIRECTION('center_axis',(-0.0109903293950669,-0.174043205665198,
0.98467668562913));
#105363=DIRECTION('ref_axis',(-0.115491862188353,-0.977924987362897,-0.174138878081674));
#105364=DIRECTION('center_axis',(0.,-1.38777878078144E-14,1.));
#105365=DIRECTION('ref_axis',(0.,1.,1.38777878078144E-14));
#105366=DIRECTION('center_axis',(0.,0.,-1.));
#105367=DIRECTION('ref_axis',(0.,1.,0.));
#105368=DIRECTION('center_axis',(0.,0.,1.));
#105369=DIRECTION('ref_axis',(1.,0.,0.));
#105370=DIRECTION('',(6.19323182390956E-32,-1.23467863058847E-16,1.));
#105371=DIRECTION('',(0.,1.23467863058847E-16,-1.));
#105372=DIRECTION('center_axis',(0.,-1.23467863058847E-16,1.));
#105373=DIRECTION('ref_axis',(0.,-1.,-1.21694324257719E-16));
#105374=DIRECTION('center_axis',(-6.69603100287811E-32,-1.19033121480991E-16,
1.));
#105375=DIRECTION('ref_axis',(1.50990331349022E-14,-1.,-1.19033121480991E-16));
#105376=DIRECTION('center_axis',(0.997043106246102,0.0768439138394239,0.00023915050274134));
#105377=DIRECTION('ref_axis',(0.0767329141488397,-0.995425758077136,-0.0569176602012574));
#105378=DIRECTION('center_axis',(0.,1.18842113532929E-16,-1.));
#105379=DIRECTION('ref_axis',(0.,-1.,-1.18842113532929E-16));
#105380=DIRECTION('center_axis',(-0.993203928613398,-0.116387082026082,
-5.76573235384675E-5));
#105381=DIRECTION('ref_axis',(0.115222785780397,-0.983198120721487,-0.141580948742201));
#105382=DIRECTION('center_axis',(0.,0.,-1.));
#105383=DIRECTION('ref_axis',(0.,1.,0.));
#105384=DIRECTION('center_axis',(0.,0.,1.));
#105385=DIRECTION('ref_axis',(1.,0.,0.));
#105386=DIRECTION('',(-6.19323182390956E-32,1.23467863058847E-16,-1.));
#105387=DIRECTION('center_axis',(0.,0.,1.));
#105388=DIRECTION('ref_axis',(1.,0.,0.));
#105389=DIRECTION('center_axis',(0.,0.,1.));
#105390=DIRECTION('ref_axis',(1.,0.,0.));
#105391=DIRECTION('',(0.,-1.23467863058847E-16,1.));
#105392=DIRECTION('center_axis',(-0.962140601075499,0.272553597962085,-1.24636926569648E-14));
#105393=DIRECTION('ref_axis',(-0.272553597962085,-0.962140601075499,-4.52904126028793E-31));
#105394=DIRECTION('center_axis',(0.,0.,-1.));
#105395=DIRECTION('ref_axis',(1.,0.,0.));
#105396=DIRECTION('center_axis',(0.,0.,-1.));
#105397=DIRECTION('ref_axis',(1.,0.,0.));
#105398=DIRECTION('center_axis',(-0.959694777166788,0.28104436425374,1.95400042656926E-13));
#105399=DIRECTION('ref_axis',(-0.28104436425374,-0.959694777166788,-3.56742184214581E-30));
#105400=DIRECTION('center_axis',(0.,0.,1.));
#105401=DIRECTION('ref_axis',(1.,0.,0.));
#105402=DIRECTION('center_axis',(0.,0.,1.));
#105403=DIRECTION('ref_axis',(1.,0.,0.));
#105404=DIRECTION('center_axis',(0.,0.,-1.));
#105405=DIRECTION('ref_axis',(0.,1.,0.));
#105406=DIRECTION('center_axis',(0.,0.,1.));
#105407=DIRECTION('ref_axis',(1.,0.,0.));
#105408=DIRECTION('',(6.19323182390956E-32,-1.23467863058847E-16,1.));
#105409=DIRECTION('',(0.,1.23467863058847E-16,-1.));
#105410=DIRECTION('center_axis',(0.,-1.23467863058847E-16,1.));
#105411=DIRECTION('ref_axis',(0.,-1.,-1.21694324257719E-16));
#105412=DIRECTION('center_axis',(-5.51437847295852E-32,-1.19033121480991E-16,
1.));
#105413=DIRECTION('ref_axis',(1.24344978758017E-14,-1.,-1.19033121480991E-16));
#105414=DIRECTION('center_axis',(0.991081580819709,0.133256151528742,0.000313432060176465));
#105415=DIRECTION('ref_axis',(0.133155408522202,-0.990235223988547,-0.0412775768866911));
#105416=DIRECTION('center_axis',(0.,1.18842113532929E-16,-1.));
#105417=DIRECTION('ref_axis',(0.,-1.,-1.18842113532929E-16));
#105418=DIRECTION('center_axis',(-0.986714641503604,-0.162462950731673,
-7.66940215737917E-5));
#105419=DIRECTION('ref_axis',(0.162365053105111,-0.986103455739161,-0.0351790293990564));
#105420=DIRECTION('center_axis',(0.,0.,-1.));
#105421=DIRECTION('ref_axis',(0.,1.,0.));
#105422=DIRECTION('center_axis',(0.,0.,1.));
#105423=DIRECTION('ref_axis',(1.,0.,0.));
#105424=DIRECTION('',(-6.19323182390956E-32,1.23467863058847E-16,-1.));
#105425=DIRECTION('center_axis',(0.,0.,1.));
#105426=DIRECTION('ref_axis',(1.,0.,0.));
#105427=DIRECTION('',(0.,-1.23467863058847E-16,1.));
#105428=DIRECTION('center_axis',(-0.911656491798923,0.41095308851605,-5.08035184938228E-15));
#105429=DIRECTION('ref_axis',(-0.41095308851605,-0.911656491798923,7.81754519040083E-31));
#105430=DIRECTION('center_axis',(0.,0.,-1.));
#105431=DIRECTION('ref_axis',(1.,0.,0.));
#105432=DIRECTION('center_axis',(0.,0.,-1.));
#105433=DIRECTION('ref_axis',(1.,0.,0.));
#105434=DIRECTION('center_axis',(0.,0.,1.));
#105435=DIRECTION('ref_axis',(1.,0.,0.));
#105436=DIRECTION('center_axis',(0.,0.,-1.));
#105437=DIRECTION('ref_axis',(0.,1.,0.));
#105438=DIRECTION('',(-1.54074395550979E-33,-1.23467863058847E-16,1.));
#105439=DIRECTION('center_axis',(0.,0.,1.));
#105440=DIRECTION('ref_axis',(0.,1.,0.));
#105441=DIRECTION('',(0.,1.23467863058847E-16,-1.));
#105442=DIRECTION('center_axis',(0.,1.23467863058847E-16,-1.));
#105443=DIRECTION('ref_axis',(0.,1.,1.21694324257719E-16));
#105444=DIRECTION('center_axis',(0.,-1.19212619247436E-16,1.));
#105445=DIRECTION('ref_axis',(0.,1.,1.19212619247436E-16));
#105446=DIRECTION('center_axis',(-0.913306614095669,-0.407272671129681,
-2.94898912583324E-15));
#105447=DIRECTION('ref_axis',(0.407272671129681,-0.913306614095669,-7.93980541862816E-31));
#105448=DIRECTION('center_axis',(4.39608526712911E-31,1.18842113532929E-16,
-1.));
#105449=DIRECTION('ref_axis',(-9.50350909079134E-14,1.,1.18842113532929E-16));
#105450=DIRECTION('center_axis',(0.,0.,-1.));
#105451=DIRECTION('ref_axis',(0.,1.,0.));
#105452=DIRECTION('center_axis',(0.,0.,-1.));
#105453=DIRECTION('ref_axis',(-1.,0.,0.));
#105454=DIRECTION('',(0.,1.23467863058847E-16,-1.));
#105455=DIRECTION('center_axis',(0.,0.,-1.));
#105456=DIRECTION('ref_axis',(-1.,0.,0.));
#105457=DIRECTION('',(0.,-1.23467863058847E-16,1.));
#105458=DIRECTION('center_axis',(-0.930967150605313,-0.365102950541111,
0.));
#105459=DIRECTION('ref_axis',(0.365102950541111,-0.930967150605313,0.));
#105460=DIRECTION('center_axis',(0.,0.,1.));
#105461=DIRECTION('ref_axis',(-1.,0.,0.));
#105462=DIRECTION('center_axis',(-0.934252508717439,-0.356612184249462,
0.));
#105463=DIRECTION('ref_axis',(0.356612184249462,-0.934252508717439,0.));
#105464=DIRECTION('center_axis',(0.,0.,1.));
#105465=DIRECTION('ref_axis',(-1.,-1.23459581198307E-13,0.));
#105466=DIRECTION('center_axis',(0.,0.,-1.));
#105467=DIRECTION('ref_axis',(-1.,0.,0.));
#105468=DIRECTION('center_axis',(0.,0.,1.));
#105469=DIRECTION('ref_axis',(1.,0.,0.));
#105470=DIRECTION('center_axis',(0.,0.,-1.));
#105471=DIRECTION('ref_axis',(-0.574616980402509,-0.818422461711006,0.));
#105472=DIRECTION('',(0.,1.23467863058847E-16,-1.));
#105473=DIRECTION('center_axis',(0.,0.,-1.));
#105474=DIRECTION('ref_axis',(-1.,0.,0.));
#105475=DIRECTION('',(1.87032180698308E-16,-1.23467863058847E-16,1.));
#105476=DIRECTION('center_axis',(0.,-1.23467863058847E-16,1.));
#105477=DIRECTION('ref_axis',(0.,-1.,-1.21694324257719E-16));
#105478=DIRECTION('center_axis',(0.,-1.19033121480991E-16,1.));
#105479=DIRECTION('ref_axis',(0.,-1.,-1.19033121480991E-16));
#105480=DIRECTION('center_axis',(-0.989231081512618,0.146362093675256,-7.00312215489063E-5));
#105481=DIRECTION('ref_axis',(0.145905880903543,0.986109658115763,-0.0793676010004968));
#105482=DIRECTION('center_axis',(0.,1.18842113532929E-16,-1.));
#105483=DIRECTION('ref_axis',(0.,-1.,-1.18842113532929E-16));
#105484=DIRECTION('center_axis',(0.993897575431132,-0.11030651249529,0.000287842394383403));
#105485=DIRECTION('ref_axis',(0.11019840995775,0.99280107613086,-0.0469290280763431));
#105486=DIRECTION('center_axis',(0.,0.,-1.));
#105487=DIRECTION('ref_axis',(0.,1.,0.));
#105488=DIRECTION('center_axis',(2.7755575615626E-13,-5.13478148889134E-13,
-1.));
#105489=DIRECTION('ref_axis',(1.14794370197489E-40,-1.,5.13478148889134E-13));
#105490=DIRECTION('',(0.,1.23467863058847E-16,-1.));
#105491=DIRECTION('center_axis',(0.,0.,-1.));
#105492=DIRECTION('ref_axis',(-1.,0.,0.));
#105493=DIRECTION('',(0.,-1.23467863058847E-16,1.));
#105494=DIRECTION('center_axis',(-0.974807460973989,-0.220687770576049,
0.0323623538639763));
#105495=DIRECTION('ref_axis',(0.220803427003966,-0.975318330917298,-7.28333184199878E-18));
#105496=DIRECTION('center_axis',(-0.976728808322011,-0.212349635823786,
0.0301407889639504));
#105497=DIRECTION('ref_axis',(0.212446157929364,-0.977172773863994,-1.17576428045677E-20));
#105498=DIRECTION('center_axis',(-0.049502590584409,0.39010562996265,0.91943846504096));
#105499=DIRECTION('ref_axis',(-0.184301157644048,0.901190701629574,-0.392286123368467));
#105500=DIRECTION('center_axis',(0.0251527414239362,-0.254018072308455,
-0.966872358969661));
#105501=DIRECTION('ref_axis',(-0.21303056621937,0.943601106365043,-0.253446108518006));
#105502=DIRECTION('center_axis',(0.,1.38777878078144E-14,1.));
#105503=DIRECTION('ref_axis',(0.,1.,-1.38777878078144E-14));
#105504=DIRECTION('center_axis',(0.,0.,-1.));
#105505=DIRECTION('ref_axis',(-0.634315526883886,-0.773074260568814,0.));
#105506=DIRECTION('center_axis',(0.,0.,1.));
#105507=DIRECTION('ref_axis',(1.,0.,0.));
#105508=DIRECTION('',(1.87032180698308E-16,-1.23467863058847E-16,1.));
#105509=DIRECTION('',(0.,1.23467863058847E-16,-1.));
#105510=DIRECTION('center_axis',(0.,-1.23467863058847E-16,1.));
#105511=DIRECTION('ref_axis',(0.,-1.,-1.21694324257719E-16));
#105512=DIRECTION('center_axis',(0.,-1.19033121480991E-16,1.));
#105513=DIRECTION('ref_axis',(0.,-1.,-1.19033121480991E-16));
#105514=DIRECTION('center_axis',(-0.995792071114552,0.0916414155502236,
-4.54020018912243E-5));
#105515=DIRECTION('ref_axis',(0.0902737810735944,0.980845595415019,-0.172605221258321));
#105516=DIRECTION('center_axis',(0.,1.18842113532929E-16,-1.));
#105517=DIRECTION('ref_axis',(0.,-1.,-1.18842113532929E-16));
#105518=DIRECTION('center_axis',(0.99894947983821,-0.0458248384975214,0.000144594765933473));
#105519=DIRECTION('ref_axis',(0.0458248568623928,0.998949481468877,-0.000126359025533782));
#105520=DIRECTION('center_axis',(0.,0.,-1.));
#105521=DIRECTION('ref_axis',(0.,1.,0.));
#105522=DIRECTION('center_axis',(0.,0.,-1.));
#105523=DIRECTION('ref_axis',(-1.,0.,0.));
#105524=DIRECTION('',(0.,1.23467863058847E-16,-1.));
#105525=DIRECTION('center_axis',(0.,0.,-1.));
#105526=DIRECTION('ref_axis',(-1.,0.,0.));
#105527=DIRECTION('',(0.,-1.23467863058847E-16,1.));
#105528=DIRECTION('center_axis',(-0.996993498376656,-0.0769676640255834,
0.00894107874490511));
#105529=DIRECTION('ref_axis',(0.07697074071877,-0.997033352036532,7.99587428479913E-19));
#105530=DIRECTION('center_axis',(-0.997624402707396,-0.0684293228260734,
0.00793592466417746));
#105531=DIRECTION('ref_axis',(0.0684314777296081,-0.997655818835204,-3.0788904879186E-19));
#105532=DIRECTION('center_axis',(-0.00150472629281886,0.0576832079807129,
0.998333803552618));
#105533=DIRECTION('ref_axis',(-0.0662281834101546,0.996137339756707,-0.0576561190561847));
#105534=DIRECTION('center_axis',(0.000120245183265025,-0.117893637115676,
-0.993026221138562));
#105535=DIRECTION('ref_axis',(-0.0688956039870738,0.990665697053924,-0.117621734521805));
#105536=DIRECTION('center_axis',(0.,-4.63518112781003E-12,1.));
#105537=DIRECTION('ref_axis',(0.,1.,4.63518112781003E-12));
#105538=DIRECTION('center_axis',(0.,0.,-1.));
#105539=DIRECTION('ref_axis',(-0.688859710772107,-0.724894681229604,0.));
#105540=DIRECTION('center_axis',(0.,0.,1.));
#105541=DIRECTION('ref_axis',(1.,0.,0.));
#105542=DIRECTION('',(1.87032180698308E-16,-1.23467863058847E-16,1.));
#105543=DIRECTION('',(0.,1.23467863058847E-16,-1.));
#105544=DIRECTION('center_axis',(-0.0690733635565107,0.78951215817867,0.609835570080205));
#105545=DIRECTION('ref_axis',(-3.95541556389227E-18,0.611295598907861,-0.791402357057319));
#105546=DIRECTION('center_axis',(-0.222999209171599,0.974818625544692,0.));
#105547=DIRECTION('ref_axis',(-0.974818625544692,-0.222999209171599,0.));
#105548=DIRECTION('center_axis',(0.,0.,-1.));
#105549=DIRECTION('ref_axis',(1.,0.,0.));
#105550=DIRECTION('center_axis',(-0.334110320282714,0.942533974921107,0.));
#105551=DIRECTION('ref_axis',(-0.942533974921107,-0.334110320282714,0.));
#105552=DIRECTION('center_axis',(0.,0.,-1.));
#105553=DIRECTION('ref_axis',(1.,-1.5419764230905E-14,0.));
#105554=DIRECTION('center_axis',(-0.388071473886494,0.870248040119286,-0.303428541544968));
#105555=DIRECTION('ref_axis',(-0.913306614096678,-0.407272671127417,-4.84423453041484E-17));
#105556=DIRECTION('center_axis',(0.,0.,-1.));
#105557=DIRECTION('ref_axis',(0.,1.,0.));
#105558=DIRECTION('',(0.,-1.23467863058847E-16,1.));
#105559=DIRECTION('center_axis',(0.,0.,1.));
#105560=DIRECTION('ref_axis',(0.,1.,0.));
#105561=DIRECTION('',(0.,1.23467863058847E-16,-1.));
#105562=DIRECTION('center_axis',(0.,0.,1.));
#105563=DIRECTION('ref_axis',(1.,0.,0.));
#105564=DIRECTION('center_axis',(-0.886046769573674,0.368569282539184,0.281207763222511));
#105565=DIRECTION('ref_axis',(0.259553330905099,-0.108212392885459,0.959646886329587));
#105566=DIRECTION('center_axis',(0.,1.18842113532929E-16,-1.));
#105567=DIRECTION('ref_axis',(0.,1.,1.18842113532929E-16));
#105568=DIRECTION('center_axis',(0.,0.,-1.));
#105569=DIRECTION('ref_axis',(1.,1.78263170299393E-15,0.));
#105570=DIRECTION('',(0.,-1.23467863058847E-16,1.));
#105571=DIRECTION('center_axis',(0.,1.18842113532929E-16,-1.));
#105572=DIRECTION('ref_axis',(0.,-1.,-1.18842113532929E-16));
#105573=DIRECTION('',(0.,1.23467863058847E-16,-1.));
#105574=DIRECTION('center_axis',(0.,0.,-1.));
#105575=DIRECTION('ref_axis',(1.,0.,0.));
#105576=DIRECTION('',(0.,-1.23467863058847E-16,1.));
#105577=DIRECTION('center_axis',(0.,1.18842113532929E-16,-1.));
#105578=DIRECTION('ref_axis',(0.,-1.,-1.18842113532929E-16));
#105579=DIRECTION('',(0.,1.23467863058847E-16,-1.));
#105580=DIRECTION('center_axis',(0.14258112270268,-0.00286725800189432,
-0.989778966376026));
#105581=DIRECTION('ref_axis',(-0.97964031348631,0.142384138292289,-0.141533082193549));
#105582=DIRECTION('',(0.,-1.23467863058847E-16,1.));
#105583=DIRECTION('center_axis',(0.,1.18842113532929E-16,-1.));
#105584=DIRECTION('ref_axis',(0.,-1.,-1.18842113532929E-16));
#105585=DIRECTION('',(0.,1.23467863058847E-16,-1.));
#105586=DIRECTION('center_axis',(0.115833335784744,6.92921622240005E-10,
-0.993268663716408));
#105587=DIRECTION('ref_axis',(-0.99326587756307,0.00236855704116508,-0.115833010866533));
#105588=DIRECTION('',(0.,-1.23467863058847E-16,1.));
#105589=DIRECTION('center_axis',(0.,1.18842113532929E-16,-1.));
#105590=DIRECTION('ref_axis',(0.,-1.,-1.18842113532929E-16));
#105591=DIRECTION('',(0.,1.23467863058847E-16,-1.));
#105592=DIRECTION('center_axis',(0.145269618857488,0.00325155863830722,
-0.989386762193341));
#105593=DIRECTION('ref_axis',(-0.979906495318529,-0.13766658060369,-0.144330083549635));
#105594=DIRECTION('',(0.,-1.23467863058847E-16,1.));
#105595=DIRECTION('center_axis',(0.,1.18842113532929E-16,-1.));
#105596=DIRECTION('ref_axis',(0.,-1.,-1.18842113532929E-16));
#105597=DIRECTION('',(0.,1.23467863058847E-16,-1.));
#105598=DIRECTION('center_axis',(0.,0.,-1.));
#105599=DIRECTION('ref_axis',(1.,0.,0.));
#105600=DIRECTION('',(0.,-1.23467863058847E-16,1.));
#105601=DIRECTION('center_axis',(0.,1.18842113532929E-16,-1.));
#105602=DIRECTION('ref_axis',(0.,-1.,-1.18842113532929E-16));
#105603=DIRECTION('',(0.,1.23467863058847E-16,-1.));
#105604=DIRECTION('center_axis',(-0.384110320270104,-0.923287204428827,
0.));
#105605=DIRECTION('ref_axis',(0.923287204428827,-0.384110320270104,0.));
#105606=DIRECTION('center_axis',(-0.405419774737912,-0.90915150463265,-0.0952803645860425));
#105607=DIRECTION('ref_axis',(0.913306614095667,-0.407272671129684,-4.7539503937481E-18));
#105608=DIRECTION('center_axis',(0.,0.,-1.));
#105609=DIRECTION('ref_axis',(1.,0.,0.));
#105610=DIRECTION('center_axis',(0.272999209159005,0.962014257585904,0.));
#105611=DIRECTION('ref_axis',(-0.962014257585904,0.272999209159004,0.));
#105612=DIRECTION('center_axis',(0.,0.,-1.));
#105613=DIRECTION('ref_axis',(1.,2.69845874040837E-15,0.));
#105614=DIRECTION('center_axis',(0.0479130906931042,0.547649132616206,-0.835335120346889));
#105615=DIRECTION('ref_axis',(-2.39380283931159E-17,-0.836295598856108,
-0.54827882626808));
#105616=DIRECTION('center_axis',(4.26141870503966E-34,0.,-1.));
#105617=DIRECTION('ref_axis',(0.,1.,0.));
#105618=DIRECTION('',(0.,-1.23467863058847E-16,1.));
#105619=DIRECTION('center_axis',(-2.85576800769162E-31,6.6052904065149E-46,
-1.));
#105620=DIRECTION('ref_axis',(2.31296463463574E-15,1.,3.11150763893057E-61));
#105621=DIRECTION('',(-1.23259516440783E-32,1.23467863058847E-16,-1.));
#105622=DIRECTION('center_axis',(-2.85576800769162E-31,6.6052904065149E-46,
-1.));
#105623=DIRECTION('ref_axis',(2.31296463463574E-15,1.,3.11150763893057E-61));
#105624=DIRECTION('center_axis',(-0.996194698091746,0.0871557427476566,
1.07609333103598E-17));
#105625=DIRECTION('ref_axis',(1.08020383274202E-17,1.24308539071746E-35,
1.));
#105626=DIRECTION('',(0.0871557427476566,0.996194698091746,1.22998030563941E-16));
#105627=DIRECTION('',(-1.08020383274202E-17,-4.37133056147834E-33,-1.));
#105628=DIRECTION('',(0.0871557427476566,0.996194698091746,0.));
#105629=DIRECTION('',(1.08020383274202E-17,4.37133056147834E-33,1.));
#105630=DIRECTION('',(0.0871557427476566,0.996194698091746,1.22998030563941E-16));
#105631=DIRECTION('',(-1.08020383274202E-17,-4.37133056147834E-33,-1.));
#105632=DIRECTION('center_axis',(-0.996194698091723,0.0871557427479135,
1.21464724749175E-13));
#105633=DIRECTION('ref_axis',(-0.0257890725821804,-0.294770448454491,0.955220030387392));
#105634=DIRECTION('',(-0.0871557427476566,-0.996194698091746,-3.51482972517089E-16));
#105635=DIRECTION('',(0.0871557427476566,0.996194698091746,1.22998030563941E-16));
#105636=DIRECTION('',(-1.08020383274202E-17,-4.56392355591706E-33,-1.));
#105637=DIRECTION('',(0.0871557427476566,0.996194698091746,0.));
#105638=DIRECTION('',(1.08020383274202E-17,4.37133056147834E-33,1.));
#105639=DIRECTION('center_axis',(0.,1.23467863058847E-16,-1.));
#105640=DIRECTION('ref_axis',(0.,1.,0.));
#105641=DIRECTION('center_axis',(-0.0871557427476572,-0.996194698091746,
0.));
#105642=DIRECTION('ref_axis',(0.996194698091746,-0.0871557427476572,0.));
#105643=DIRECTION('center_axis',(-0.707106781186544,-0.707106781186551,
0.));
#105644=DIRECTION('ref_axis',(0.707106781186551,-0.707106781186544,0.));
#105645=DIRECTION('center_axis',(0.,0.,1.));
#105646=DIRECTION('ref_axis',(0.,1.,0.));
#105647=DIRECTION('center_axis',(1.67127905768941E-33,0.,-1.));
#105648=DIRECTION('ref_axis',(0.,1.,0.));
#105649=DIRECTION('',(1.23259516440783E-32,-1.23467863058847E-16,1.));
#105650=DIRECTION('center_axis',(5.71153601538325E-31,2.64211616260596E-45,
-1.));
#105651=DIRECTION('ref_axis',(-4.62592926927148E-15,1.,1.24460305557223E-60));
#105652=DIRECTION('',(3.08148791101958E-33,1.23467863058847E-16,-1.));
#105653=DIRECTION('center_axis',(5.71153601538325E-31,2.64211616260596E-45,
-1.));
#105654=DIRECTION('ref_axis',(-4.62592926927148E-15,1.,1.24460305557223E-60));
#105655=DIRECTION('center_axis',(-0.707106781186548,0.707106781186547,8.73049632275231E-17));
#105656=DIRECTION('ref_axis',(1.23467863058847E-16,2.16153073061992E-33,
1.));
#105657=DIRECTION('',(-0.707106781186547,-0.707106781186548,0.));
#105658=DIRECTION('',(0.707106781186547,0.707106781186548,8.73049632275231E-17));
#105659=DIRECTION('center_axis',(0.,1.23467863058847E-16,-1.));
#105660=DIRECTION('ref_axis',(0.,1.,0.));
#105661=DIRECTION('center_axis',(-0.707106781186548,-0.707106781186548,
0.));
#105662=DIRECTION('ref_axis',(0.707106781186548,-0.707106781186548,0.));
#105663=DIRECTION('center_axis',(-0.996194698091746,-0.0871557427476538,
0.));
#105664=DIRECTION('ref_axis',(0.0871557427476538,-0.996194698091746,0.));
#105665=DIRECTION('center_axis',(0.,0.,1.));
#105666=DIRECTION('ref_axis',(0.,1.,0.));
#105667=DIRECTION('center_axis',(-0.0871557427476569,0.996194698091746,
1.22998030563941E-16));
#105668=DIRECTION('ref_axis',(1.41124413247282E-15,-4.52989727324155E-33,
1.));
#105669=DIRECTION('',(0.996194698091746,0.0871557427476568,1.07609333103598E-17));
#105670=DIRECTION('',(-1.87032180698308E-16,1.07104667533214E-16,-1.));
#105671=DIRECTION('',(0.996194698091746,0.0871557427476568,1.54074395550979E-33));
#105672=DIRECTION('',(5.23852944873328E-32,-1.23467863058847E-16,1.));
#105673=DIRECTION('',(0.996194698091746,0.0871557427476568,1.07609333103598E-17));
#105674=DIRECTION('',(-0.996194698091746,-0.0871557427476568,0.));
#105675=DIRECTION('',(-1.87032180698308E-16,1.07104667533214E-16,-1.));
#105676=DIRECTION('',(0.996194698091746,0.0871557427476568,1.54074395550979E-33));
#105677=DIRECTION('',(-1.54074395550979E-33,-1.23467863058847E-16,1.));
#105678=DIRECTION('center_axis',(0.,0.,-1.));
#105679=DIRECTION('ref_axis',(-1.,0.,0.));
#105680=DIRECTION('center_axis',(0.,0.,-1.));
#105681=DIRECTION('ref_axis',(0.,1.,0.));
#105682=DIRECTION('center_axis',(0.,0.,-1.));
#105683=DIRECTION('ref_axis',(-1.,0.,0.));
#105684=DIRECTION('',(-5.16102651992463E-32,-2.15733828054269E-47,1.));
#105685=DIRECTION('center_axis',(0.,-1.23467863058847E-16,1.));
#105686=DIRECTION('ref_axis',(0.,-1.,-1.21694324257719E-16));
#105687=DIRECTION('center_axis',(9.84710441599736E-32,-1.19033121480991E-16,
1.));
#105688=DIRECTION('ref_axis',(-2.22044604925031E-14,-1.,-1.19033121480991E-16));
#105689=DIRECTION('center_axis',(-0.162977314581735,-0.986629813581626,
-7.67047044552073E-5));
#105690=DIRECTION('ref_axis',(0.982479968620953,-0.162284694779714,-0.0916339953228362));
#105691=DIRECTION('center_axis',(0.133849112401615,0.991001679892255,0.000292506460560356));
#105692=DIRECTION('ref_axis',(0.990279721870948,-0.133762854809558,0.0381257278539607));
#105693=DIRECTION('center_axis',(0.,0.,-1.));
#105694=DIRECTION('ref_axis',(0.,1.,0.));
#105695=DIRECTION('center_axis',(0.,0.,-1.));
#105696=DIRECTION('ref_axis',(-1.,0.,0.));
#105697=DIRECTION('',(5.16102651992463E-32,2.15733828054269E-47,-1.));
#105698=DIRECTION('center_axis',(0.,0.,-1.));
#105699=DIRECTION('ref_axis',(-1.,0.,0.));
#105700=DIRECTION('center_axis',(0.282954786668892,-0.959133248668381,0.));
#105701=DIRECTION('ref_axis',(0.959133248668381,0.282954786668892,0.));
#105702=DIRECTION('center_axis',(0.,0.,-1.));
#105703=DIRECTION('ref_axis',(1.,0.,0.));
#105704=DIRECTION('center_axis',(0.274464020377229,-0.96159736975429,0.));
#105705=DIRECTION('ref_axis',(0.96159736975429,0.274464020377229,0.));
#105706=DIRECTION('center_axis',(0.,0.,1.));
#105707=DIRECTION('ref_axis',(1.,0.,0.));
#105708=DIRECTION('center_axis',(0.,0.,1.));
#105709=DIRECTION('ref_axis',(1.,0.,0.));
#105710=DIRECTION('center_axis',(0.,0.,-1.));
#105711=DIRECTION('ref_axis',(0.,1.,0.));
#105712=DIRECTION('center_axis',(0.,0.,1.));
#105713=DIRECTION('ref_axis',(1.,0.,0.));
#105714=DIRECTION('',(-5.16102651992463E-32,-2.15733828054269E-47,1.));
#105715=DIRECTION('center_axis',(0.,-1.23467863058847E-16,1.));
#105716=DIRECTION('ref_axis',(0.,-1.,-1.21694324257719E-16));
#105717=DIRECTION('center_axis',(0.,-1.19033121480991E-16,1.));
#105718=DIRECTION('ref_axis',(0.,-1.,-1.19033121480991E-16));
#105719=DIRECTION('center_axis',(-0.117127826816072,-0.99311684553817,-5.73904025634227E-5));
#105720=DIRECTION('ref_axis',(0.983475565813904,-0.115998770283216,0.138996750824625));
#105721=DIRECTION('center_axis',(0.0776595476784529,0.996979910344055,0.000230271010090371));
#105722=DIRECTION('ref_axis',(0.995508289094979,-0.0775574567760436,0.05429629123265));
#105723=DIRECTION('center_axis',(0.,0.,-1.));
#105724=DIRECTION('ref_axis',(0.,1.,0.));
#105725=DIRECTION('center_axis',(0.,0.,1.));
#105726=DIRECTION('ref_axis',(1.,0.,0.));
#105727=DIRECTION('center_axis',(1.18805075949821E-12,-7.25808302348696E-12,
1.));
#105728=DIRECTION('ref_axis',(5.87747175411144E-39,1.,7.25808302348696E-12));
#105729=DIRECTION('',(5.16102651992463E-32,2.15733828054269E-47,-1.));
#105730=DIRECTION('center_axis',(-0.14514509610524,0.989248239790814,-0.0179114808817288));
#105731=DIRECTION('ref_axis',(-0.989406963861029,-0.145168384517086,-1.21343959465114E-18));
#105732=DIRECTION('center_axis',(-0.136675079747296,0.990475586151279,-0.0166744059669382));
#105733=DIRECTION('ref_axis',(-0.990613308713893,-0.136694083993833,9.06110283290218E-19));
#105734=DIRECTION('center_axis',(-0.16767237013086,-0.0112896091060275,
0.98577812971324));
#105735=DIRECTION('ref_axis',(-0.977934730745161,-0.124494525481806,-0.167764047183683));
#105736=DIRECTION('center_axis',(6.61970478432749E-12,0.,1.));
#105737=DIRECTION('ref_axis',(1.,0.,-6.61970478432749E-12));
#105738=DIRECTION('center_axis',(0.,0.,-1.));
#105739=DIRECTION('ref_axis',(0.,1.,0.));
#105740=DIRECTION('center_axis',(0.,0.,1.));
#105741=DIRECTION('ref_axis',(1.,0.,0.));
#105742=DIRECTION('',(-5.16102651992463E-32,-2.15733828054269E-47,1.));
#105743=DIRECTION('center_axis',(0.,-1.23467863058847E-16,1.));
#105744=DIRECTION('ref_axis',(0.,-1.,-1.21694324257719E-16));
#105745=DIRECTION('center_axis',(-1.96942088319945E-31,-1.19033121480991E-16,
1.));
#105746=DIRECTION('ref_axis',(4.44089209850063E-14,-1.,-1.19033121480991E-16));
#105747=DIRECTION('center_axis',(-0.0573840568526241,-0.998352176938356,
-2.86632424776913E-5));
#105748=DIRECTION('ref_axis',(0.978156398817009,-0.0562289739133945,0.200120868342077));
#105749=DIRECTION('center_axis',(0.0114617529384933,0.99993431126188,3.71591962562455E-5));
#105750=DIRECTION('ref_axis',(-0.999934311920365,0.0114617532273491,-7.56982004799599E-6));
#105751=DIRECTION('center_axis',(0.,0.,-1.));
#105752=DIRECTION('ref_axis',(0.,1.,0.));
#105753=DIRECTION('center_axis',(0.,0.,1.));
#105754=DIRECTION('ref_axis',(1.,0.,0.));
#105755=DIRECTION('center_axis',(0.,0.,1.));
#105756=DIRECTION('ref_axis',(1.,0.,0.));
#105757=DIRECTION('',(5.16102651992463E-32,2.15733828054269E-47,-1.));
#105758=DIRECTION('center_axis',(-0.00620231251671424,0.999980508301815,
-0.000717172147678158));
#105759=DIRECTION('ref_axis',(-0.999980765464846,-0.00620231411175082,5.84684475171815E-22));
#105760=DIRECTION('center_axis',(0.00235261362124023,0.999997195602435,
0.000272022820600068));
#105761=DIRECTION('ref_axis',(-0.999997232600541,0.00235261370828272,8.12493746167259E-22));
#105762=DIRECTION('center_axis',(-0.0305144215778958,-2.78804702901659E-8,
0.999534326612031));
#105763=DIRECTION('ref_axis',(-0.99952008198814,-0.00533875532879332,-0.0305139868578466));
#105764=DIRECTION('center_axis',(3.91353616180368E-12,0.,1.));
#105765=DIRECTION('ref_axis',(1.,0.,-3.91353616180368E-12));
#105766=DIRECTION('center_axis',(0.,0.,-1.));
#105767=DIRECTION('ref_axis',(0.,1.,0.));
#105768=DIRECTION('center_axis',(0.,0.,1.));
#105769=DIRECTION('ref_axis',(1.,0.,0.));
#105770=DIRECTION('',(-5.16102651992463E-32,-2.15733828054269E-47,1.));
#105771=DIRECTION('center_axis',(0.,-1.23467863058847E-16,1.));
#105772=DIRECTION('ref_axis',(0.,-1.,-1.21694324257719E-16));
#105773=DIRECTION('center_axis',(0.,-1.19033121480991E-16,1.));
#105774=DIRECTION('ref_axis',(0.,-1.,-1.19033121480991E-16));
#105775=DIRECTION('center_axis',(0.00957667179610246,-0.999954142104087,
3.23448419023486E-5));
#105776=DIRECTION('ref_axis',(-0.906194367619744,-0.0086923991525787,-0.422772054766189));
#105777=DIRECTION('center_axis',(-0.055599347306662,0.998453159538039,-2.80638595116041E-5));
#105778=DIRECTION('ref_axis',(0.977793822426841,0.0544546102272507,0.202370789020812));
#105779=DIRECTION('center_axis',(0.,0.,-1.));
#105780=DIRECTION('ref_axis',(0.,1.,0.));
#105781=DIRECTION('center_axis',(0.,0.,1.));
#105782=DIRECTION('ref_axis',(1.,0.,0.));
#105783=DIRECTION('center_axis',(0.,0.,1.));
#105784=DIRECTION('ref_axis',(1.,0.,0.));
#105785=DIRECTION('',(5.16102651992463E-32,2.15733828054269E-47,-1.));
#105786=DIRECTION('center_axis',(0.132860127107541,0.991003467296,0.0161342626814395));
#105787=DIRECTION('ref_axis',(-0.991132478736687,0.132877423188709,7.57324997548269E-19));
#105788=DIRECTION('center_axis',(0.141334929101325,0.989809819863889,0.0173481502454526));
#105789=DIRECTION('ref_axis',(-0.989958799240908,0.1413562018643,-1.53957070961197E-18));
#105790=DIRECTION('center_axis',(-0.159896444557162,0.0103428845664614,
0.987079607608638));
#105791=DIRECTION('ref_axis',(-0.980515938222932,0.113929190724357,-0.16002698019927));
#105792=DIRECTION('center_axis',(0.,0.,1.));
#105793=DIRECTION('ref_axis',(1.,0.,0.));
#105794=DIRECTION('center_axis',(0.,0.,-1.));
#105795=DIRECTION('ref_axis',(0.,1.,0.));
#105796=DIRECTION('center_axis',(0.,0.,1.));
#105797=DIRECTION('ref_axis',(1.,0.,0.));
#105798=DIRECTION('',(-5.16102651992463E-32,-2.15733828054269E-47,1.));
#105799=DIRECTION('center_axis',(0.,-1.23467863058847E-16,1.));
#105800=DIRECTION('ref_axis',(0.,-1.,-1.21694324257719E-16));
#105801=DIRECTION('center_axis',(-4.72661011967866E-32,-1.19033121480991E-16,
1.));
#105802=DIRECTION('ref_axis',(1.06581410364015E-14,-1.,-1.19033121480991E-16));
#105803=DIRECTION('center_axis',(0.0759780984300171,-0.997109458589618,
0.000236960074453804));
#105804=DIRECTION('ref_axis',(0.995484288532962,0.0758678217481024,0.0570535266852247));
#105805=DIRECTION('center_axis',(-0.115641121459685,0.993291058926343,-5.73108184457433E-5));
#105806=DIRECTION('ref_axis',(0.983116729805053,0.114464840497617,0.142756071209856));
#105807=DIRECTION('center_axis',(0.,0.,-1.));
#105808=DIRECTION('ref_axis',(0.,1.,0.));
#105809=DIRECTION('center_axis',(0.,0.,-1.));
#105810=DIRECTION('ref_axis',(-1.,0.,0.));
#105811=DIRECTION('',(5.16102651992463E-32,2.15733828054269E-47,-1.));
#105812=DIRECTION('center_axis',(0.,0.,-1.));
#105813=DIRECTION('ref_axis',(-1.,0.,0.));
#105814=DIRECTION('center_axis',(-0.270643175546941,-0.962679734662503,
0.));
#105815=DIRECTION('ref_axis',(0.962679734662504,-0.270643175546941,0.));
#105816=DIRECTION('center_axis',(0.,0.,-1.));
#105817=DIRECTION('ref_axis',(1.,0.,0.));
#105818=DIRECTION('center_axis',(-0.279133941838593,-0.960252176521172,
-2.49865799020366E-15));
#105819=DIRECTION('ref_axis',(0.960252176521172,-0.279133941838593,3.84227067759201E-30));
#105820=DIRECTION('center_axis',(0.,0.,1.));
#105821=DIRECTION('ref_axis',(1.,0.,0.));
#105822=DIRECTION('center_axis',(0.,0.,1.));
#105823=DIRECTION('ref_axis',(1.,0.,0.));
#105824=DIRECTION('center_axis',(0.,0.,-1.));
#105825=DIRECTION('ref_axis',(0.,1.,0.));
#105826=DIRECTION('center_axis',(0.,0.,1.));
#105827=DIRECTION('ref_axis',(1.,0.,0.));
#105828=DIRECTION('',(-5.16102651992463E-32,-2.15733828054269E-47,1.));
#105829=DIRECTION('center_axis',(0.,-1.23467863058847E-16,1.));
#105830=DIRECTION('ref_axis',(0.,-1.,-1.21694324257719E-16));
#105831=DIRECTION('center_axis',(0.,-1.19033121480991E-16,1.));
#105832=DIRECTION('ref_axis',(0.,-1.,-1.19033121480991E-16));
#105833=DIRECTION('center_axis',(0.132576902561935,-0.991172672369243,0.000313776189307544));
#105834=DIRECTION('ref_axis',(0.99031382809775,0.132475188409534,0.0415793979542594));
#105835=DIRECTION('center_axis',(-0.161944455651288,0.986799872024417,-7.65271292523058E-5));
#105836=DIRECTION('ref_axis',(0.98612977255929,0.161837341642917,0.0368340402632872));
#105837=DIRECTION('center_axis',(0.,0.,-1.));
#105838=DIRECTION('ref_axis',(0.,1.,0.));
#105839=DIRECTION('center_axis',(0.,0.,-1.));
#105840=DIRECTION('ref_axis',(-1.,0.,0.));
#105841=DIRECTION('',(5.16102651992463E-32,2.15733828054269E-47,-1.));
#105842=DIRECTION('center_axis',(0.,0.,-1.));
#105843=DIRECTION('ref_axis',(-1.,0.,0.));
#105844=DIRECTION('center_axis',(0.996194698091747,-0.0871557427476409,
-1.07609333103578E-17));
#105845=DIRECTION('ref_axis',(-0.0871557427476409,-0.996194698091747,2.79703111108876E-34));
#105846=DIRECTION('',(0.996194698091747,-0.0871557427476402,-1.07609333103578E-17));
#105847=DIRECTION('center_axis',(1.13659195805196E-16,0.,1.));
#105848=DIRECTION('ref_axis',(-0.675590207615648,0.737277336810136,7.678703969146E-17));
#105849=DIRECTION('center_axis',(0.,0.,1.));
#105850=DIRECTION('ref_axis',(1.,0.,0.));
#105851=DIRECTION('center_axis',(0.,0.,1.));
#105852=DIRECTION('ref_axis',(1.,0.,0.));
#105853=DIRECTION('',(-1.13659195805196E-16,1.33411754197273E-16,-1.));
#105854=DIRECTION('center_axis',(-0.996194698091747,0.0871557427476457,
0.));
#105855=DIRECTION('ref_axis',(-0.0871557427476457,-0.996194698091747,0.));
#105856=DIRECTION('center_axis',(-0.996194698091747,0.0871557427476457,
0.));
#105857=DIRECTION('ref_axis',(0.0871557427476457,0.996194698091747,0.));
#105858=DIRECTION('center_axis',(-0.996194698091747,0.0871557427476457,
-1.3824978635387E-14));
#105859=DIRECTION('ref_axis',(-0.0871557427476457,-0.996194698091747,6.24837364119099E-31));
#105860=DIRECTION('',(0.996194698091747,-0.0871557427476402,0.));
#105861=DIRECTION('center_axis',(0.,0.,-1.));
#105862=DIRECTION('ref_axis',(-1.,0.,0.));
#105863=DIRECTION('center_axis',(0.,1.13523971920422E-16,-1.));
#105864=DIRECTION('ref_axis',(1.,0.,0.));
#105865=DIRECTION('center_axis',(0.,0.,-1.));
#105866=DIRECTION('ref_axis',(-1.,0.,0.));
#105867=DIRECTION('',(-1.13659195805196E-16,-1.13523971920422E-16,1.));
#105868=DIRECTION('center_axis',(0.996194698091747,-0.0871557427476409,
-1.07609333103578E-17));
#105869=DIRECTION('ref_axis',(-0.0871557427476409,-0.996194698091747,2.79703111108876E-34));
#105870=DIRECTION('',(0.996194698091747,-0.0871557427476402,-1.07609333103578E-17));
#105871=DIRECTION('center_axis',(0.,0.,1.));
#105872=DIRECTION('ref_axis',(1.,0.,0.));
#105873=DIRECTION('center_axis',(-6.19323182390956E-32,0.,-1.));
#105874=DIRECTION('ref_axis',(0.,1.,0.));
#105875=DIRECTION('center_axis',(0.,0.,1.));
#105876=DIRECTION('ref_axis',(1.,0.,0.));
#105877=DIRECTION('',(6.19323182390956E-32,-1.23467863058847E-16,1.));
#105878=DIRECTION('center_axis',(-0.996194698091747,0.08715574274764,0.));
#105879=DIRECTION('ref_axis',(-0.08715574274764,-0.996194698091747,0.));
#105880=DIRECTION('center_axis',(0.996194698091747,-0.0871557427476409,
-1.07609333103578E-17));
#105881=DIRECTION('ref_axis',(-0.0871557427476409,-0.996194698091747,2.79703111108876E-34));
#105882=DIRECTION('',(0.996194698091747,-0.0871557427476402,-1.07609333103578E-17));
#105883=DIRECTION('center_axis',(6.19323182390956E-32,0.,1.));
#105884=DIRECTION('ref_axis',(-0.675590207615642,0.737277336810141,4.18408677372686E-32));
#105885=DIRECTION('center_axis',(0.,0.,1.));
#105886=DIRECTION('ref_axis',(1.,0.,0.));
#105887=DIRECTION('center_axis',(0.,0.,1.));
#105888=DIRECTION('ref_axis',(1.,0.,0.));
#105889=DIRECTION('',(-6.19323182390956E-32,1.23467863058847E-16,-1.));
#105890=DIRECTION('center_axis',(-0.996194698091747,0.0871557427476457,
0.));
#105891=DIRECTION('ref_axis',(-0.0871557427476457,-0.996194698091747,0.));
#105892=DIRECTION('center_axis',(-0.996194698091747,0.0871557427476457,
0.));
#105893=DIRECTION('ref_axis',(0.0871557427476457,0.996194698091747,0.));
#105894=DIRECTION('center_axis',(-0.996194698091747,0.0871557427476457,
-3.00690150789426E-14));
#105895=DIRECTION('ref_axis',(-0.0871557427476457,-0.996194698091747,1.22577679051452E-30));
#105896=DIRECTION('',(0.996194698091747,-0.0871557427476402,0.));
#105897=DIRECTION('center_axis',(0.,0.,1.));
#105898=DIRECTION('ref_axis',(1.,0.,0.));
#105899=DIRECTION('center_axis',(-6.19323182390956E-32,0.,-1.));
#105900=DIRECTION('ref_axis',(0.,1.,0.));
#105901=DIRECTION('center_axis',(0.,0.,1.));
#105902=DIRECTION('ref_axis',(1.,0.,0.));
#105903=DIRECTION('',(6.19323182390956E-32,-1.23467863058847E-16,1.));
#105904=DIRECTION('center_axis',(0.707106781186548,-0.707106781186548,-8.7304963227523E-17));
#105905=DIRECTION('ref_axis',(-0.707106781186548,-0.707106781186548,-2.5701266908181E-33));
#105906=DIRECTION('',(0.707106781186547,-0.707106781186548,-8.73049632275231E-17));
#105907=DIRECTION('center_axis',(-0.955086750882198,-0.0835592633859996,
0.284301156859545));
#105908=DIRECTION('ref_axis',(0.28529890144429,-2.70823414235005E-19,0.958438593147564));
#105909=DIRECTION('center_axis',(-0.996194698091746,-0.0871557427476572,
-1.07609333103598E-17));
#105910=DIRECTION('ref_axis',(-0.0871557427476572,0.996194698091746,-1.48387871229006E-34));
#105911=DIRECTION('',(-0.996194698091746,-0.0871557427476568,-1.07609333103598E-17));
#105912=DIRECTION('center_axis',(0.,0.,1.));
#105913=DIRECTION('ref_axis',(0.,-1.,0.));
#105914=DIRECTION('center_axis',(0.,0.,-1.));
#105915=DIRECTION('ref_axis',(-1.,0.,0.));
#105916=DIRECTION('',(0.,1.23467863058847E-16,-1.));
#105917=DIRECTION('center_axis',(0.,0.,-1.));
#105918=DIRECTION('ref_axis',(-1.,0.,0.));
#105919=DIRECTION('center_axis',(-0.996194698091746,-0.0871557427476538,
0.));
#105920=DIRECTION('ref_axis',(0.0871557427476538,-0.996194698091746,0.));
#105921=DIRECTION('center_axis',(0.996194698091746,0.0871557427476572,0.));
#105922=DIRECTION('ref_axis',(0.0871557427476572,-0.996194698091746,0.));
#105923=DIRECTION('center_axis',(-0.996194698091745,-0.0871557427476607,
0.));
#105924=DIRECTION('ref_axis',(0.0871557427476607,-0.996194698091745,0.));
#105925=DIRECTION('',(-0.996194698091746,-0.0871557427476568,0.));
#105926=DIRECTION('center_axis',(0.,0.,1.));
#105927=DIRECTION('ref_axis',(1.,0.,0.));
#105928=DIRECTION('center_axis',(0.,1.07104667533214E-16,-1.));
#105929=DIRECTION('ref_axis',(1.,0.,0.));
#105930=DIRECTION('center_axis',(0.,0.,-1.));
#105931=DIRECTION('ref_axis',(-1.,0.,0.));
#105932=DIRECTION('',(1.87032180698308E-16,-1.07104667533214E-16,1.));
#105933=DIRECTION('center_axis',(-0.996194698091746,-0.0871557427476572,
-1.07609333103598E-17));
#105934=DIRECTION('ref_axis',(-0.0871557427476572,0.996194698091746,-1.48387871229006E-34));
#105935=DIRECTION('',(-0.996194698091746,-0.0871557427476568,-1.07609333103598E-17));
#105936=DIRECTION('center_axis',(5.40794518211031E-32,0.,1.));
#105937=DIRECTION('ref_axis',(0.,-1.,0.));
#105938=DIRECTION('center_axis',(0.,0.,1.));
#105939=DIRECTION('ref_axis',(1.,0.,0.));
#105940=DIRECTION('center_axis',(0.,0.,1.));
#105941=DIRECTION('ref_axis',(1.,0.,0.));
#105942=DIRECTION('',(-5.40794518211031E-32,1.23467863058847E-16,-1.));
#105943=DIRECTION('center_axis',(0.996194698091745,0.0871557427476607,0.));
#105944=DIRECTION('ref_axis',(-0.0871557427476607,0.996194698091745,0.));
#105945=DIRECTION('center_axis',(0.996194698091746,0.0871557427476572,0.));
#105946=DIRECTION('ref_axis',(0.0871557427476572,-0.996194698091746,0.));
#105947=DIRECTION('center_axis',(0.996194698091745,0.0871557427476607,1.2095289040845E-15));
#105948=DIRECTION('ref_axis',(-0.0871557427476607,0.996194698091745,-5.51367835803032E-32));
#105949=DIRECTION('',(-0.996194698091746,-0.0871557427476568,0.));
#105950=DIRECTION('center_axis',(0.,0.,-1.));
#105951=DIRECTION('ref_axis',(-1.,0.,0.));
#105952=DIRECTION('center_axis',(0.,-1.07104667533214E-16,1.));
#105953=DIRECTION('ref_axis',(-1.,0.,0.));
#105954=DIRECTION('center_axis',(0.,0.,-1.));
#105955=DIRECTION('ref_axis',(-1.,0.,0.));
#105956=DIRECTION('',(1.87032180698308E-16,-1.07104667533214E-16,1.));
#105957=DIRECTION('center_axis',(-0.707106781186548,-0.707106781186548,
-8.7304963227523E-17));
#105958=DIRECTION('ref_axis',(-0.707106781186548,0.707106781186548,2.5701266908181E-33));
#105959=DIRECTION('',(-0.707106781186547,-0.707106781186548,-8.73049632275231E-17));
#105960=DIRECTION('center_axis',(-0.0871557427476572,-0.996194698091746,
-1.22998030563942E-16));
#105961=DIRECTION('ref_axis',(-0.996194698091746,0.0871557427476572,1.44426287624373E-33));
#105962=DIRECTION('',(-0.0871557427476566,-0.996194698091746,-1.22998030563941E-16));
#105963=DIRECTION('center_axis',(0.,4.51531312650048E-33,1.));
#105964=DIRECTION('ref_axis',(0.737277336810104,0.675590207615682,-3.05050133258228E-33));
#105965=DIRECTION('center_axis',(0.,0.,-1.));
#105966=DIRECTION('ref_axis',(-1.,0.,0.));
#105967=DIRECTION('',(-1.08020383274202E-17,-4.51531312650048E-33,-1.));
#105968=DIRECTION('center_axis',(0.,0.,-1.));
#105969=DIRECTION('ref_axis',(-1.,0.,0.));
#105970=DIRECTION('center_axis',(-0.0871557427476538,-0.996194698091746,
0.));
#105971=DIRECTION('ref_axis',(0.996194698091746,-0.0871557427476538,0.));
#105972=DIRECTION('center_axis',(0.0871557427476538,0.996194698091746,0.));
#105973=DIRECTION('ref_axis',(0.996194698091746,-0.0871557427476538,0.));
#105974=DIRECTION('center_axis',(-0.0871557427476538,-0.996194698091746,
0.));
#105975=DIRECTION('ref_axis',(0.996194698091746,-0.0871557427476538,0.));
#105976=DIRECTION('',(-0.0871557427476566,-0.996194698091746,0.));
#105977=DIRECTION('center_axis',(0.,0.,1.));
#105978=DIRECTION('ref_axis',(1.,0.,0.));
#105979=DIRECTION('center_axis',(0.,-4.73133896404282E-33,-1.));
#105980=DIRECTION('ref_axis',(1.,0.,0.));
#105981=DIRECTION('center_axis',(0.,0.,1.));
#105982=DIRECTION('ref_axis',(1.,0.,0.));
#105983=DIRECTION('',(1.08020383274202E-17,4.73133896404282E-33,1.));
#105984=DIRECTION('center_axis',(-0.0871557427476572,-0.996194698091746,
-1.22998030563942E-16));
#105985=DIRECTION('ref_axis',(-0.996194698091746,0.0871557427476572,1.44426287624373E-33));
#105986=DIRECTION('',(-0.0871557427476566,-0.996194698091746,-1.22998030563941E-16));
#105987=DIRECTION('center_axis',(0.,0.,-1.));
#105988=DIRECTION('ref_axis',(-1.,0.,0.));
#105989=DIRECTION('center_axis',(0.985034259191114,-0.172358661574676,4.57699418854155E-11));
#105990=DIRECTION('ref_axis',(0.0566495632167467,0.323753735284747,-0.944443934744951));
#105991=DIRECTION('center_axis',(0.,4.51531312650048E-33,1.));
#105992=DIRECTION('ref_axis',(-1.,0.,0.));
#105993=DIRECTION('center_axis',(0.,0.,-1.));
#105994=DIRECTION('ref_axis',(-1.,0.,0.));
#105995=DIRECTION('',(1.08020383274202E-17,4.51531312650048E-33,1.));
#105996=DIRECTION('center_axis',(0.0871557427476607,0.996194698091745,0.));
#105997=DIRECTION('ref_axis',(-0.996194698091745,0.0871557427476607,0.));
#105998=DIRECTION('center_axis',(0.0835592633859915,0.955086750882199,0.284301156859544));
#105999=DIRECTION('ref_axis',(-2.48475885091778E-18,0.285298901444289,-0.958438593147564));
#106000=DIRECTION('center_axis',(-0.0871557427476572,-0.996194698091746,
-1.22998030563942E-16));
#106001=DIRECTION('ref_axis',(-0.996194698091746,0.0871557427476572,1.44426287624373E-33));
#106002=DIRECTION('',(-0.0871557427476566,-0.996194698091746,-1.22998030563941E-16));
#106003=DIRECTION('center_axis',(0.,4.51531312650048E-33,1.));
#106004=DIRECTION('ref_axis',(0.737277336810102,0.675590207615684,-3.05050133258228E-33));
#106005=DIRECTION('center_axis',(0.,0.,1.));
#106006=DIRECTION('ref_axis',(1.,0.,0.));
#106007=DIRECTION('center_axis',(0.,0.,1.));
#106008=DIRECTION('ref_axis',(1.,0.,0.));
#106009=DIRECTION('',(-1.08020383274202E-17,-4.51531312650048E-33,-1.));
#106010=DIRECTION('center_axis',(0.0871557427476538,0.996194698091746,6.91248931769351E-15));
#106011=DIRECTION('ref_axis',(-0.996194698091746,0.0871557427476538,2.78649888037662E-32));
#106012=DIRECTION('center_axis',(0.0871557427476538,0.996194698091746,0.));
#106013=DIRECTION('ref_axis',(0.996194698091746,-0.0871557427476538,0.));
#106014=DIRECTION('center_axis',(0.0871557427476538,0.996194698091746,6.91248931769351E-15));
#106015=DIRECTION('ref_axis',(-0.996194698091746,0.0871557427476538,2.78649888037662E-32));
#106016=DIRECTION('',(-0.0871557427476566,-0.996194698091746,0.));
#106017=DIRECTION('center_axis',(0.,0.,1.));
#106018=DIRECTION('ref_axis',(1.,0.,0.));
#106019=DIRECTION('center_axis',(0.,-4.51531312650048E-33,-1.));
#106020=DIRECTION('ref_axis',(1.,0.,0.));
#106021=DIRECTION('center_axis',(0.,0.,1.));
#106022=DIRECTION('ref_axis',(1.,0.,0.));
#106023=DIRECTION('',(1.08020383274202E-17,4.51531312650048E-33,1.));
#106024=DIRECTION('center_axis',(0.0871557427476394,-0.996194698091747,
0.));
#106025=DIRECTION('ref_axis',(0.996194698091747,0.0871557427476394,0.));
#106026=DIRECTION('center_axis',(0.,4.51531312649963E-33,-1.));
#106027=DIRECTION('ref_axis',(1.,0.,0.));
#106028=DIRECTION('center_axis',(0.,0.,-1.));
#106029=DIRECTION('ref_axis',(-1.,0.,0.));
#106030=DIRECTION('',(1.08020383274181E-17,4.51531312649963E-33,-1.));
#106031=DIRECTION('center_axis',(1.38777878078144E-14,0.,-1.));
#106032=DIRECTION('ref_axis',(-1.,0.,-1.38777878078144E-14));
#106033=DIRECTION('center_axis',(0.985034259178149,0.172358661648767,3.69403275210692E-11));
#106034=DIRECTION('ref_axis',(-0.0885145471782662,0.505862951942684,0.858060515808564));
#106035=DIRECTION('center_axis',(0.0871557427476394,-0.996194698091747,
-1.22998030563942E-16));
#106036=DIRECTION('ref_axis',(-0.996194698091747,-0.0871557427476394,8.16488070285074E-35));
#106037=DIRECTION('',(0.0871557427476402,-0.996194698091747,-1.22998030563942E-16));
#106038=DIRECTION('center_axis',(0.,-4.73133896404192E-33,1.));
#106039=DIRECTION('ref_axis',(-1.,0.,0.));
#106040=DIRECTION('center_axis',(0.,0.,1.));
#106041=DIRECTION('ref_axis',(1.,0.,0.));
#106042=DIRECTION('center_axis',(0.,0.,1.));
#106043=DIRECTION('ref_axis',(1.,0.,0.));
#106044=DIRECTION('',(1.08020383274181E-17,4.73133896404192E-33,-1.));
#106045=DIRECTION('center_axis',(-0.0871557427476469,0.996194698091747,
-1.3824978635387E-14));
#106046=DIRECTION('ref_axis',(-0.996194698091747,-0.0871557427476469,-9.13671722807069E-31));
#106047=DIRECTION('center_axis',(-0.0871557427476469,0.996194698091747,
0.));
#106048=DIRECTION('ref_axis',(0.996194698091747,0.0871557427476469,0.));
#106049=DIRECTION('center_axis',(-0.0871557427476469,0.996194698091747,
0.));
#106050=DIRECTION('ref_axis',(-0.996194698091747,-0.0871557427476469,0.));
#106051=DIRECTION('',(0.0871557427476402,-0.996194698091747,0.));
#106052=DIRECTION('center_axis',(0.,0.,-1.));
#106053=DIRECTION('ref_axis',(-1.,0.,0.));
#106054=DIRECTION('center_axis',(0.,-4.51531312649963E-33,1.));
#106055=DIRECTION('ref_axis',(0.737277336810104,-0.675590207615683,-3.0505013325817E-33));
#106056=DIRECTION('center_axis',(0.,0.,-1.));
#106057=DIRECTION('ref_axis',(-1.,0.,0.));
#106058=DIRECTION('',(-1.08020383274181E-17,-4.51531312649963E-33,1.));
#106059=DIRECTION('center_axis',(0.0871557427476394,-0.996194698091747,
-1.22998030563942E-16));
#106060=DIRECTION('ref_axis',(-0.996194698091747,-0.0871557427476394,8.16488070285074E-35));
#106061=DIRECTION('',(0.0871557427476402,-0.996194698091747,-1.22998030563942E-16));
#106062=DIRECTION('center_axis',(0.,-4.51531312649963E-33,1.));
#106063=DIRECTION('ref_axis',(-1.,0.,0.));
#106064=DIRECTION('center_axis',(0.,0.,1.));
#106065=DIRECTION('ref_axis',(1.,0.,0.));
#106066=DIRECTION('center_axis',(0.,0.,1.));
#106067=DIRECTION('ref_axis',(1.,0.,0.));
#106068=DIRECTION('',(1.08020383274181E-17,4.51531312649963E-33,-1.));
#106069=DIRECTION('center_axis',(-0.0871557427476469,0.996194698091747,
0.));
#106070=DIRECTION('ref_axis',(-0.996194698091747,-0.0871557427476469,0.));
#106071=DIRECTION('center_axis',(-0.0871557427476469,0.996194698091747,
0.));
#106072=DIRECTION('ref_axis',(0.996194698091747,0.0871557427476469,0.));
#106073=DIRECTION('center_axis',(-0.0871557427476469,0.996194698091747,
-1.3824978635387E-14));
#106074=DIRECTION('ref_axis',(-0.996194698091747,-0.0871557427476469,-9.13671722807069E-31));
#106075=DIRECTION('',(0.0871557427476402,-0.996194698091747,0.));
#106076=DIRECTION('center_axis',(0.,0.,1.));
#106077=DIRECTION('ref_axis',(1.,0.,0.));
#106078=DIRECTION('center_axis',(0.,0.,1.));
#106079=DIRECTION('ref_axis',(1.,0.,0.));
#106080=DIRECTION('center_axis',(0.,4.51531312649963E-33,-1.));
#106081=DIRECTION('ref_axis',(1.,0.,0.));
#106082=DIRECTION('center_axis',(0.,0.,1.));
#106083=DIRECTION('ref_axis',(1.,0.,0.));
#106084=DIRECTION('center_axis',(0.,0.,1.));
#106085=DIRECTION('ref_axis',(1.,0.,0.));
#106086=DIRECTION('',(-1.08020383274181E-17,-4.51531312649963E-33,1.));
#106087=DIRECTION('center_axis',(0.0871557427476394,-0.996194698091747,
-1.22998030563942E-16));
#106088=DIRECTION('ref_axis',(-0.996194698091747,-0.0871557427476394,8.16488070285074E-35));
#106089=DIRECTION('',(0.0871557427476402,-0.996194698091747,-1.22998030563942E-16));
#106090=DIRECTION('center_axis',(0.,1.23467863058847E-16,-1.));
#106091=DIRECTION('ref_axis',(-1.,0.,0.));
#106092=DIRECTION('',(-4.38004274807345E-16,1.,1.23467863058847E-16));
#106093=DIRECTION('center_axis',(0.,0.,1.));
#106094=DIRECTION('ref_axis',(0.,1.,0.));
#106095=DIRECTION('center_axis',(1.76945321870477E-31,1.17608371252665E-16,
-1.));
#106096=DIRECTION('ref_axis',(-3.01980662698042E-14,1.,1.17608371252665E-16));
#106097=DIRECTION('center_axis',(0.,0.,1.));
#106098=DIRECTION('ref_axis',(0.,1.,0.));
#106099=DIRECTION('',(1.,4.38004274807345E-16,5.40794518211031E-32));
#106100=DIRECTION('center_axis',(0.,0.,1.));
#106101=DIRECTION('ref_axis',(0.,1.,0.));
#106102=DIRECTION('',(1.,4.38004274807345E-16,5.40794518211031E-32));
#106103=DIRECTION('center_axis',(0.,1.23467863058847E-16,-1.));
#106104=DIRECTION('ref_axis',(-1.,0.,0.));
#106105=DIRECTION('',(-1.,-4.38004274807345E-16,-5.40794518211031E-32));
#106106=DIRECTION('center_axis',(0.,0.,1.));
#106107=DIRECTION('ref_axis',(0.,1.,0.));
#106108=DIRECTION('center_axis',(0.,0.,1.));
#106109=DIRECTION('ref_axis',(0.,1.,0.));
#106110=DIRECTION('',(-4.38004274807345E-16,1.,1.23467863058847E-16));
#106111=DIRECTION('center_axis',(0.,0.,-1.));
#106112=DIRECTION('ref_axis',(0.,-1.,0.));
#106113=DIRECTION('',(-5.01606788234257E-16,1.,0.));
#106114=DIRECTION('',(-1.,-5.01606788234257E-16,0.));
#106115=DIRECTION('',(5.01606788234257E-16,-1.,0.));
#106116=DIRECTION('center_axis',(0.,-1.,0.));
#106117=DIRECTION('ref_axis',(-1.,0.,0.));
#106118=DIRECTION('',(5.01606788234257E-16,-1.,0.));
#106119=DIRECTION('center_axis',(0.,-1.,0.));
#106120=DIRECTION('ref_axis',(0.,0.,1.));
#106121=DIRECTION('center_axis',(6.703313282803E-15,-0.423071618151431,
-0.90609624539269));
#106122=DIRECTION('ref_axis',(9.44993610611347E-31,-0.90609624539269,0.423071618151431));
#106123=DIRECTION('center_axis',(1.,0.,0.));
#106124=DIRECTION('ref_axis',(0.,0.97671957347062,-0.214520103485359));
#106125=DIRECTION('center_axis',(-0.999690759108302,0.0248673681371606,
-1.24658621679628E-5));
#106126=DIRECTION('ref_axis',(0.0242993767343897,0.976750214327029,-0.212998965026647));
#106127=DIRECTION('center_axis',(0.,-0.423401464461212,-0.905942161449671));
#106128=DIRECTION('ref_axis',(0.,-0.905942161449671,0.423401464461211));
#106129=DIRECTION('center_axis',(0.,1.,0.));
#106130=DIRECTION('ref_axis',(0.,0.,-1.));
#106131=DIRECTION('center_axis',(0.,0.,-1.));
#106132=DIRECTION('ref_axis',(1.,0.,0.));
#106133=DIRECTION('center_axis',(0.,1.,0.));
#106134=DIRECTION('ref_axis',(0.,0.,-1.));
#106135=DIRECTION('center_axis',(0.,0.,1.));
#106136=DIRECTION('ref_axis',(1.,0.,0.));
#106137=DIRECTION('center_axis',(-1.,0.,0.));
#106138=DIRECTION('ref_axis',(0.,0.,1.));
#106139=DIRECTION('center_axis',(0.,0.,-1.));
#106140=DIRECTION('ref_axis',(1.,0.,0.));
#106141=DIRECTION('center_axis',(-1.,0.,0.));
#106142=DIRECTION('ref_axis',(0.,0.,-1.));
#106143=DIRECTION('',(-1.,0.,0.));
#106144=DIRECTION('center_axis',(-1.,0.,0.));
#106145=DIRECTION('ref_axis',(0.,0.,1.));
#106146=DIRECTION('',(1.,0.,0.));
#106147=DIRECTION('center_axis',(0.,-1.,0.));
#106148=DIRECTION('ref_axis',(0.,0.,-1.));
#106149=DIRECTION('',(0.,-1.,0.));
#106150=DIRECTION('',(0.,1.,0.));
#106151=DIRECTION('center_axis',(0.,-1.,0.));
#106152=DIRECTION('ref_axis',(0.,0.,-1.));
#106153=DIRECTION('',(0.,-1.,0.));
#106154=DIRECTION('center_axis',(9.37295054023422E-45,-1.,2.02617679489732E-30));
#106155=DIRECTION('ref_axis',(-1.,-4.97841222228891E-60,4.62592926927148E-15));
#106156=DIRECTION('center_axis',(0.,-1.,0.));
#106157=DIRECTION('ref_axis',(0.,0.,-1.));
#106158=DIRECTION('',(0.,1.,0.));
#106159=DIRECTION('center_axis',(0.,1.,0.));
#106160=DIRECTION('ref_axis',(0.,0.,-1.));
#106161=DIRECTION('',(0.,-1.,0.));
#106162=DIRECTION('center_axis',(0.,0.,-1.));
#106163=DIRECTION('ref_axis',(1.,0.,0.));
#106164=DIRECTION('center_axis',(0.,0.,1.));
#106165=DIRECTION('ref_axis',(1.,0.,0.));
#106166=DIRECTION('center_axis',(-1.,0.,0.));
#106167=DIRECTION('ref_axis',(0.,0.,1.));
#106168=DIRECTION('center_axis',(0.,0.,-1.));
#106169=DIRECTION('ref_axis',(1.,0.,0.));
#106170=DIRECTION('center_axis',(-1.,0.,0.));
#106171=DIRECTION('ref_axis',(0.,0.,-1.));
#106172=DIRECTION('',(-1.,0.,0.));
#106173=DIRECTION('center_axis',(-1.,0.,0.));
#106174=DIRECTION('ref_axis',(0.,0.,1.));
#106175=DIRECTION('',(1.,0.,0.));
#106176=DIRECTION('center_axis',(0.,0.,-1.));
#106177=DIRECTION('ref_axis',(1.,0.,0.));
#106178=DIRECTION('center_axis',(0.,0.,1.));
#106179=DIRECTION('ref_axis',(1.,0.,0.));
#106180=DIRECTION('center_axis',(0.,-1.,0.));
#106181=DIRECTION('ref_axis',(0.,0.,1.));
#106182=DIRECTION('center_axis',(0.,0.,-1.));
#106183=DIRECTION('ref_axis',(1.,0.,0.));
#106184=DIRECTION('center_axis',(0.,-1.,0.));
#106185=DIRECTION('ref_axis',(0.,0.,-1.));
#106186=DIRECTION('',(0.,-1.,0.));
#106187=DIRECTION('center_axis',(0.,-1.,0.));
#106188=DIRECTION('ref_axis',(0.,0.,1.));
#106189=DIRECTION('',(0.,1.,0.));
#106190=DIRECTION('center_axis',(0.,0.,-1.));
#106191=DIRECTION('ref_axis',(1.,0.,0.));
#106192=DIRECTION('center_axis',(0.991696083061511,0.128603555318137,6.6332437503331E-5));
#106193=DIRECTION('ref_axis',(-0.0239412820628473,0.184110745713541,0.982613885677376));
#106194=DIRECTION('center_axis',(0.,0.,-1.));
#106195=DIRECTION('ref_axis',(0.,-1.,0.));
#106196=DIRECTION('center_axis',(-0.998076762506053,-0.0619901273296905,
-1.60961186456236E-5));
#106197=DIRECTION('ref_axis',(0.0113170760680052,-0.181956139738737,-0.983241520177341));
#106198=DIRECTION('center_axis',(0.,0.,1.));
#106199=DIRECTION('ref_axis',(1.,0.,0.));
#106200=DIRECTION('center_axis',(0.,-1.,0.));
#106201=DIRECTION('ref_axis',(0.,0.,-1.));
#106202=DIRECTION('center_axis',(0.,1.,0.));
#106203=DIRECTION('ref_axis',(0.,0.,-1.));
#106204=DIRECTION('',(0.,1.,0.));
#106205=DIRECTION('center_axis',(0.,1.,0.));
#106206=DIRECTION('ref_axis',(0.,0.,-1.));
#106207=DIRECTION('',(0.,-1.,0.));
#106208=DIRECTION('center_axis',(0.,0.,-1.));
#106209=DIRECTION('ref_axis',(1.,0.,0.));
#106210=DIRECTION('center_axis',(0.,0.,1.));
#106211=DIRECTION('ref_axis',(1.,0.,0.));
#106212=DIRECTION('center_axis',(-1.,0.,0.));
#106213=DIRECTION('ref_axis',(0.,0.,1.));
#106214=DIRECTION('center_axis',(0.,0.,-1.));
#106215=DIRECTION('ref_axis',(1.,0.,0.));
#106216=DIRECTION('center_axis',(-1.,0.,0.));
#106217=DIRECTION('ref_axis',(0.,0.,-1.));
#106218=DIRECTION('',(-1.,0.,0.));
#106219=DIRECTION('center_axis',(-1.,0.,0.));
#106220=DIRECTION('ref_axis',(0.,0.,1.));
#106221=DIRECTION('',(1.,0.,0.));
#106222=DIRECTION('center_axis',(0.,0.,-1.));
#106223=DIRECTION('ref_axis',(1.,0.,0.));
#106224=DIRECTION('center_axis',(0.,0.,1.));
#106225=DIRECTION('ref_axis',(1.,0.,0.));
#106226=DIRECTION('center_axis',(0.,-1.,0.));
#106227=DIRECTION('ref_axis',(0.,0.,1.));
#106228=DIRECTION('center_axis',(0.,0.,-1.));
#106229=DIRECTION('ref_axis',(1.,0.,0.));
#106230=DIRECTION('center_axis',(0.,-1.,0.));
#106231=DIRECTION('ref_axis',(0.,0.,-1.));
#106232=DIRECTION('',(0.,-1.,0.));
#106233=DIRECTION('center_axis',(0.,-1.,0.));
#106234=DIRECTION('ref_axis',(0.,0.,1.));
#106235=DIRECTION('',(0.,1.,0.));
#106236=DIRECTION('center_axis',(0.,0.,-1.));
#106237=DIRECTION('ref_axis',(1.,0.,0.));
#106238=DIRECTION('center_axis',(0.,0.,1.));
#106239=DIRECTION('ref_axis',(1.,0.,0.));
#106240=DIRECTION('center_axis',(0.950554487276066,0.310557831521497,-3.79371153572051E-14));
#106241=DIRECTION('ref_axis',(-0.310557831521497,0.950554487276066,1.69736969313821E-30));
#106242=DIRECTION('center_axis',(-0.988230180462193,-0.15293610778742,0.00341428740686027));
#106243=DIRECTION('ref_axis',(0.0254252921822052,-0.186218180898005,-0.982179384644418));
#106244=DIRECTION('center_axis',(1.,0.,1.73472347597681E-14));
#106245=DIRECTION('ref_axis',(1.73472347597681E-14,0.,-1.));
#106246=DIRECTION('center_axis',(-1.,0.,0.));
#106247=DIRECTION('ref_axis',(0.,1.,0.));
#106248=DIRECTION('',(1.,4.38004274807345E-16,0.));
#106249=DIRECTION('',(-1.,-4.38004274807345E-16,0.));
#106250=DIRECTION('center_axis',(1.,0.,0.));
#106251=DIRECTION('ref_axis',(0.,0.,-1.));
#106252=DIRECTION('center_axis',(0.,-1.,0.));
#106253=DIRECTION('ref_axis',(0.,0.,-1.));
#106254=DIRECTION('center_axis',(0.,1.,0.));
#106255=DIRECTION('ref_axis',(0.,0.,-1.));
#106256=DIRECTION('',(0.,1.,0.));
#106257=DIRECTION('center_axis',(0.,1.,0.));
#106258=DIRECTION('ref_axis',(0.,0.,-1.));
#106259=DIRECTION('',(0.,-1.,0.));
#106260=DIRECTION('center_axis',(0.,0.,-1.));
#106261=DIRECTION('ref_axis',(1.,0.,0.));
#106262=DIRECTION('center_axis',(0.,0.,1.));
#106263=DIRECTION('ref_axis',(1.,0.,0.));
#106264=DIRECTION('center_axis',(-1.,0.,0.));
#106265=DIRECTION('ref_axis',(0.,0.,1.));
#106266=DIRECTION('center_axis',(0.,0.,-1.));
#106267=DIRECTION('ref_axis',(1.,0.,0.));
#106268=DIRECTION('center_axis',(-1.,0.,0.));
#106269=DIRECTION('ref_axis',(0.,0.,-1.));
#106270=DIRECTION('',(-1.,0.,0.));
#106271=DIRECTION('center_axis',(-1.,0.,0.));
#106272=DIRECTION('ref_axis',(0.,0.,1.));
#106273=DIRECTION('',(1.,0.,0.));
#106274=DIRECTION('center_axis',(0.,0.,-1.));
#106275=DIRECTION('ref_axis',(1.,0.,0.));
#106276=DIRECTION('center_axis',(0.,0.,1.));
#106277=DIRECTION('ref_axis',(1.,0.,0.));
#106278=DIRECTION('center_axis',(0.,-1.,0.));
#106279=DIRECTION('ref_axis',(0.,0.,1.));
#106280=DIRECTION('center_axis',(0.,0.,-1.));
#106281=DIRECTION('ref_axis',(1.,0.,0.));
#106282=DIRECTION('center_axis',(0.,-1.,0.));
#106283=DIRECTION('ref_axis',(0.,0.,-1.));
#106284=DIRECTION('',(0.,-1.,0.));
#106285=DIRECTION('center_axis',(0.,-1.,0.));
#106286=DIRECTION('ref_axis',(0.,0.,1.));
#106287=DIRECTION('',(0.,1.,0.));
#106288=DIRECTION('center_axis',(-1.,0.,0.));
#106289=DIRECTION('ref_axis',(0.,1.,0.));
#106290=DIRECTION('',(-1.,-4.38004274807345E-16,0.));
#106291=DIRECTION('center_axis',(1.,0.,0.));
#106292=DIRECTION('ref_axis',(0.,0.,-1.));
#106293=DIRECTION('',(1.,4.38004274807345E-16,0.));
#106294=DIRECTION('center_axis',(-1.,0.,0.));
#106295=DIRECTION('ref_axis',(0.,0.,1.));
#106296=DIRECTION('center_axis',(0.,-1.,0.));
#106297=DIRECTION('ref_axis',(0.,0.,-1.));
#106298=DIRECTION('center_axis',(0.,1.,0.));
#106299=DIRECTION('ref_axis',(0.,0.,-1.));
#106300=DIRECTION('',(0.,1.,0.));
#106301=DIRECTION('center_axis',(0.,1.,0.));
#106302=DIRECTION('ref_axis',(0.,0.,-1.));
#106303=DIRECTION('',(0.,-1.,0.));
#106304=DIRECTION('center_axis',(0.,0.,-1.));
#106305=DIRECTION('ref_axis',(1.,0.,0.));
#106306=DIRECTION('center_axis',(0.,0.,1.));
#106307=DIRECTION('ref_axis',(1.,0.,0.));
#106308=DIRECTION('center_axis',(-1.,0.,0.));
#106309=DIRECTION('ref_axis',(0.,0.,1.));
#106310=DIRECTION('center_axis',(0.,0.,-1.));
#106311=DIRECTION('ref_axis',(1.,0.,0.));
#106312=DIRECTION('center_axis',(-1.,0.,0.));
#106313=DIRECTION('ref_axis',(0.,0.,-1.));
#106314=DIRECTION('',(-1.,0.,0.));
#106315=DIRECTION('center_axis',(-1.,0.,0.));
#106316=DIRECTION('ref_axis',(0.,0.,1.));
#106317=DIRECTION('',(1.,0.,0.));
#106318=DIRECTION('center_axis',(0.,0.,-1.));
#106319=DIRECTION('ref_axis',(1.,0.,0.));
#106320=DIRECTION('center_axis',(0.,0.,1.));
#106321=DIRECTION('ref_axis',(1.,0.,0.));
#106322=DIRECTION('center_axis',(0.,-1.,0.));
#106323=DIRECTION('ref_axis',(0.,0.,1.));
#106324=DIRECTION('center_axis',(0.,0.,-1.));
#106325=DIRECTION('ref_axis',(1.,0.,0.));
#106326=DIRECTION('center_axis',(0.,-1.,0.));
#106327=DIRECTION('ref_axis',(0.,0.,-1.));
#106328=DIRECTION('',(0.,-1.,0.));
#106329=DIRECTION('center_axis',(0.,-1.,0.));
#106330=DIRECTION('ref_axis',(0.,0.,1.));
#106331=DIRECTION('',(0.,1.,0.));
#106332=DIRECTION('center_axis',(-1.,0.,0.));
#106333=DIRECTION('ref_axis',(0.,1.,0.));
#106334=DIRECTION('',(-1.,-4.38004274807345E-16,0.));
#106335=DIRECTION('center_axis',(1.,0.,0.));
#106336=DIRECTION('ref_axis',(0.,0.,-1.));
#106337=DIRECTION('',(1.,4.38004274807345E-16,0.));
#106338=DIRECTION('center_axis',(-1.,0.,0.));
#106339=DIRECTION('ref_axis',(0.,0.,1.));
#106340=DIRECTION('center_axis',(0.,-1.,0.));
#106341=DIRECTION('ref_axis',(0.,0.,-1.));
#106342=DIRECTION('center_axis',(0.,1.,0.));
#106343=DIRECTION('ref_axis',(0.,0.,-1.));
#106344=DIRECTION('',(0.,1.,0.));
#106345=DIRECTION('',(0.,-1.,0.));
#106346=DIRECTION('center_axis',(1.,0.,-1.6326809185664E-16));
#106347=DIRECTION('ref_axis',(-1.6326809185664E-16,0.,-1.));
#106348=DIRECTION('',(-1.6326809185664E-16,-7.15121221728469E-32,-1.));
#106349=DIRECTION('',(-1.6326809185664E-16,0.,-1.));
#106350=DIRECTION('',(0.,1.,0.));
#106351=DIRECTION('',(-1.6326809185664E-16,1.00522029149049E-16,-1.));
#106352=DIRECTION('',(2.0158362407235E-32,1.,1.23467863058847E-16));
#106353=DIRECTION('',(2.0158362407235E-32,1.,1.23467863058847E-16));
#106354=DIRECTION('center_axis',(0.,-1.,0.));
#106355=DIRECTION('ref_axis',(0.,0.,-1.));
#106356=DIRECTION('center_axis',(0.,-1.,0.));
#106357=DIRECTION('ref_axis',(0.,0.,-1.));
#106358=DIRECTION('',(0.,-1.,0.));
#106359=DIRECTION('center_axis',(0.,0.,1.));
#106360=DIRECTION('ref_axis',(-1.,0.,0.));
#106361=DIRECTION('center_axis',(0.990268068741571,0.139173100960059,0.));
#106362=DIRECTION('ref_axis',(-0.139173100960059,0.990268068741571,0.));
#106363=DIRECTION('center_axis',(0.,0.,1.));
#106364=DIRECTION('ref_axis',(-1.,-1.5419764230905E-15,0.));
#106365=DIRECTION('center_axis',(0.904824724134427,0.425784239486454,0.));
#106366=DIRECTION('ref_axis',(-0.425784239486454,0.904824724134427,0.));
#106367=DIRECTION('center_axis',(0.,0.,-1.));
#106368=DIRECTION('ref_axis',(-1.,0.,0.));
#106369=DIRECTION('center_axis',(-0.990268068741572,-0.139173100960052,
0.));
#106370=DIRECTION('ref_axis',(-0.139173100960052,0.990268068741572,0.));
#106371=DIRECTION('center_axis',(0.990268068741572,0.139173100960052,0.));
#106372=DIRECTION('ref_axis',(-0.139173100960052,0.990268068741572,0.));
#106373=DIRECTION('',(0.990268068741571,0.139173100960059,0.));
#106374=DIRECTION('',(-0.990268068741571,-0.139173100960059,0.));
#106375=DIRECTION('center_axis',(0.,0.,1.));
#106376=DIRECTION('ref_axis',(0.,-1.,0.));
#106377=DIRECTION('',(0.,1.23467863058847E-16,-1.));
#106378=DIRECTION('center_axis',(0.,0.,1.));
#106379=DIRECTION('ref_axis',(0.,-1.,0.));
#106380=DIRECTION('',(3.43088182518023E-33,-1.23467863058847E-16,1.));
#106381=DIRECTION('center_axis',(0.,-1.23467863058847E-16,1.));
#106382=DIRECTION('ref_axis',(0.,-1.,0.));
#106383=DIRECTION('center_axis',(-0.990268068741572,-0.139173100960051,
-1.7605559658208E-14));
#106384=DIRECTION('ref_axis',(0.139173100960051,-0.990268068741572,2.08829111071605E-30));
#106385=DIRECTION('center_axis',(-0.904824724134424,-0.42578423948646,0.));
#106386=DIRECTION('ref_axis',(0.42578423948646,-0.904824724134424,0.));
#106387=DIRECTION('center_axis',(0.,0.,-1.));
#106388=DIRECTION('ref_axis',(0.,-1.,0.));
#106389=DIRECTION('center_axis',(0.990268068741571,0.139173100960064,1.71834053708117E-17));
#106390=DIRECTION('ref_axis',(0.139173100960064,-0.990268068741571,7.54967553857625E-35));
#106391=DIRECTION('center_axis',(-0.990268068741571,-0.139173100960064,
-3.86282952735861E-15));
#106392=DIRECTION('ref_axis',(0.139173100960064,-0.990268068741571,3.33751075060364E-33));
#106393=DIRECTION('',(0.990268068741571,0.139173100960059,1.71834053708117E-17));
#106394=DIRECTION('',(-0.990268068741571,-0.139173100960059,-1.71834053708117E-17));
#106395=DIRECTION('center_axis',(0.,-1.23467863058847E-16,1.));
#106396=DIRECTION('ref_axis',(0.,-1.,0.));
#106397=DIRECTION('center_axis',(-0.728126055379271,-0.685443248911113,
1.18468586241421E-15));
#106398=DIRECTION('ref_axis',(0.685443248911113,-0.728126055379271,2.48798705504199E-31));
#106399=DIRECTION('center_axis',(0.,0.,-1.));
#106400=DIRECTION('ref_axis',(0.,-1.,0.));
#106401=DIRECTION('center_axis',(3.11538328111815E-31,-7.86084147552189E-46,
1.));
#106402=DIRECTION('ref_axis',(-2.52323414687536E-15,-1.,3.11150763893057E-61));
#106403=DIRECTION('center_axis',(0.,-1.23467863058847E-16,1.));
#106404=DIRECTION('ref_axis',(0.,-1.,0.));
#106405=DIRECTION('center_axis',(-0.685443248911113,-0.728126055379271,
-1.18468586241421E-15));
#106406=DIRECTION('ref_axis',(0.728126055379271,-0.685443248911113,2.6468713136043E-31));
#106407=DIRECTION('center_axis',(0.,0.,-1.));
#106408=DIRECTION('ref_axis',(0.,-1.,0.));
#106409=DIRECTION('center_axis',(0.,0.,1.));
#106410=DIRECTION('ref_axis',(0.,-1.,0.));
#106411=DIRECTION('center_axis',(0.,-1.23467863058847E-16,1.));
#106412=DIRECTION('ref_axis',(0.,-1.,0.));
#106413=DIRECTION('center_axis',(-0.139173100960068,-0.99026806874157,-2.36226307343407E-14));
#106414=DIRECTION('ref_axis',(0.99026806874157,-0.139173100960068,-1.46728138438144E-30));
#106415=DIRECTION('center_axis',(0.,0.,-1.));
#106416=DIRECTION('ref_axis',(0.,-1.,0.));
#106417=DIRECTION('center_axis',(-6.23076656223629E-31,-3.14433659020876E-45,
1.));
#106418=DIRECTION('ref_axis',(5.04646829375071E-15,-1.,1.86690458335834E-60));
#106419=DIRECTION('center_axis',(0.139173100960068,0.99026806874157,1.22266282302933E-16));
#106420=DIRECTION('ref_axis',(0.99026806874157,-0.139173100960068,-6.9848527780828E-33));
#106421=DIRECTION('center_axis',(-0.139173100960068,-0.99026806874157,0.));
#106422=DIRECTION('ref_axis',(0.99026806874157,-0.139173100960068,0.));
#106423=DIRECTION('',(0.139173100960067,0.99026806874157,1.22266282302933E-16));
#106424=DIRECTION('',(-0.139173100960067,-0.99026806874157,-1.22266282302933E-16));
#106425=DIRECTION('center_axis',(0.,-1.23467863058847E-16,1.));
#106426=DIRECTION('ref_axis',(0.,-1.,0.));
#106427=DIRECTION('center_axis',(-0.425784239486454,-0.904824724134427,
0.));
#106428=DIRECTION('ref_axis',(0.904824724134427,-0.425784239486454,0.));
#106429=DIRECTION('center_axis',(0.,0.,1.));
#106430=DIRECTION('ref_axis',(0.,-1.,0.));
#106431=DIRECTION('center_axis',(0.,0.,-1.));
#106432=DIRECTION('ref_axis',(0.,-1.,0.));
#106433=DIRECTION('center_axis',(0.,-1.23467863058847E-16,1.));
#106434=DIRECTION('ref_axis',(0.,-1.,0.));
#106435=DIRECTION('center_axis',(0.425784239486448,-0.90482472413443,1.18178866550092E-14));
#106436=DIRECTION('ref_axis',(0.90482472413443,0.425784239486448,3.74967935723291E-30));
#106437=DIRECTION('center_axis',(0.,0.,-1.));
#106438=DIRECTION('ref_axis',(0.,-1.,0.));
#106439=DIRECTION('center_axis',(-2.19322982990717E-31,-3.89595880873225E-46,
1.));
#106440=DIRECTION('ref_axis',(1.77635683940025E-15,-1.,-5.4451383681285E-61));
#106441=DIRECTION('center_axis',(0.,-1.23467863058847E-16,1.));
#106442=DIRECTION('ref_axis',(0.,-1.,0.));
#106443=DIRECTION('center_axis',(0.139173100960068,-0.99026806874157,0.));
#106444=DIRECTION('ref_axis',(0.99026806874157,0.139173100960068,0.));
#106445=DIRECTION('center_axis',(0.,0.,1.));
#106446=DIRECTION('ref_axis',(0.,-1.,0.));
#106447=DIRECTION('center_axis',(0.,0.,-1.));
#106448=DIRECTION('ref_axis',(0.,-1.,0.));
#106449=DIRECTION('center_axis',(-0.139173100960064,0.990268068741571,1.22266282302934E-16));
#106450=DIRECTION('ref_axis',(0.990268068741571,0.139173100960064,-6.46427645420959E-34));
#106451=DIRECTION('center_axis',(0.139173100960064,-0.990268068741571,-3.86282952735861E-15));
#106452=DIRECTION('ref_axis',(0.990268068741571,0.139173100960064,3.00533800087463E-32));
#106453=DIRECTION('',(-0.139173100960065,0.99026806874157,1.22266282302933E-16));
#106454=DIRECTION('',(0.139173100960065,-0.99026806874157,-1.22266282302933E-16));
#106455=DIRECTION('center_axis',(0.,-1.23467863058847E-16,1.));
#106456=DIRECTION('ref_axis',(0.,-1.,0.));
#106457=DIRECTION('center_axis',(0.685443248911113,-0.728126055379271,-1.18468586241421E-15));
#106458=DIRECTION('ref_axis',(0.728126055379271,0.685443248911113,-2.6468713136043E-31));
#106459=DIRECTION('center_axis',(0.,0.,-1.));
#106460=DIRECTION('ref_axis',(0.,-1.,0.));
#106461=DIRECTION('center_axis',(-1.24615331244726E-30,-1.2577346360835E-44,
1.));
#106462=DIRECTION('ref_axis',(1.00929365875014E-14,-1.,-9.95682444457783E-60));
#106463=DIRECTION('center_axis',(0.,-1.23467863058847E-16,1.));
#106464=DIRECTION('ref_axis',(0.,-1.,0.));
#106465=DIRECTION('center_axis',(0.728126055379271,-0.685443248911113,0.));
#106466=DIRECTION('ref_axis',(0.685443248911113,0.728126055379271,0.));
#106467=DIRECTION('center_axis',(0.,0.,-1.));
#106468=DIRECTION('ref_axis',(0.,-1.,0.));
#106469=DIRECTION('center_axis',(0.,0.,1.));
#106470=DIRECTION('ref_axis',(0.,-1.,0.));
#106471=DIRECTION('center_axis',(0.,-1.23467863058847E-16,1.));
#106472=DIRECTION('ref_axis',(0.,-1.,0.));
#106473=DIRECTION('center_axis',(0.990268068741571,-0.139173100960064,-7.72565905471723E-15));
#106474=DIRECTION('ref_axis',(0.139173100960064,0.990268068741571,-6.67502150120727E-33));
#106475=DIRECTION('center_axis',(0.,0.,-1.));
#106476=DIRECTION('ref_axis',(0.,-1.,0.));
#106477=DIRECTION('center_axis',(3.11538328111815E-31,-7.86084147552191E-46,
1.));
#106478=DIRECTION('ref_axis',(-2.52323414687536E-15,-1.,-6.22301527786114E-61));
#106479=DIRECTION('center_axis',(-0.990268068741571,0.139173100960064,1.71834053708117E-17));
#106480=DIRECTION('ref_axis',(0.139173100960064,0.990268068741571,-7.54967553857625E-35));
#106481=DIRECTION('center_axis',(0.990268068741571,-0.139173100960064,0.));
#106482=DIRECTION('ref_axis',(0.139173100960064,0.990268068741571,0.));
#106483=DIRECTION('',(-0.990268068741571,0.139173100960059,1.71834053708117E-17));
#106484=DIRECTION('',(0.990268068741571,-0.139173100960059,-1.71834053708117E-17));
#106485=DIRECTION('center_axis',(0.,-1.23467863058847E-16,1.));
#106486=DIRECTION('ref_axis',(0.,-1.,0.));
#106487=DIRECTION('center_axis',(0.902736181373369,-0.430194591829591,1.25279811715363E-14));
#106488=DIRECTION('ref_axis',(0.430194591829591,0.902736181373369,2.66752875008673E-30));
#106489=DIRECTION('center_axis',(1.5706724042304E-30,-1.99810034797076E-44,
1.));
#106490=DIRECTION('ref_axis',(-1.27213054904966E-14,-1.,2.98704733337335E-59));
#106491=DIRECTION('center_axis',(0.,0.,-1.));
#106492=DIRECTION('ref_axis',(0.,-1.,0.));
#106493=DIRECTION('center_axis',(0.,0.,-1.));
#106494=DIRECTION('ref_axis',(0.,1.,0.));
#106495=DIRECTION('center_axis',(0.,0.,1.));
#106496=DIRECTION('ref_axis',(0.,-1.,0.));
#106497=DIRECTION('',(0.,0.,-1.));
#106498=DIRECTION('center_axis',(0.,0.,1.));
#106499=DIRECTION('ref_axis',(0.,-1.,0.));
#106500=DIRECTION('center_axis',(0.,0.,1.));
#106501=DIRECTION('ref_axis',(0.,-1.,0.));
#106502=DIRECTION('center_axis',(0.,0.,1.));
#106503=DIRECTION('ref_axis',(0.,-1.,0.));
#106504=DIRECTION('center_axis',(0.,0.,-1.));
#106505=DIRECTION('ref_axis',(0.,1.,0.));
#106506=DIRECTION('center_axis',(0.,0.,1.));
#106507=DIRECTION('ref_axis',(0.,1.,0.));
#106508=DIRECTION('',(0.,0.,-1.));
#106509=DIRECTION('center_axis',(0.,0.,1.));
#106510=DIRECTION('ref_axis',(0.,1.,0.));
#106511=DIRECTION('center_axis',(0.,0.,1.));
#106512=DIRECTION('ref_axis',(0.,1.,0.));
#106513=DIRECTION('center_axis',(0.,0.,1.));
#106514=DIRECTION('ref_axis',(1.,0.,0.));
#106515=DIRECTION('center_axis',(-0.91200931366711,0.410169491533009,5.52463721181358E-12));
#106516=DIRECTION('ref_axis',(-0.410169491533009,-0.91200931366711,-2.38205677224627E-27));
#106517=DIRECTION('center_axis',(0.,0.,1.));
#106518=DIRECTION('ref_axis',(-0.550808342809401,0.834631756819474,0.));
#106519=DIRECTION('',(0.,-1.23467863058847E-16,1.));
#106520=DIRECTION('center_axis',(0.,0.,1.));
#106521=DIRECTION('ref_axis',(1.,0.,0.));
#106522=DIRECTION('',(-6.19323182390956E-32,1.23467863058847E-16,-1.));
#106523=DIRECTION('center_axis',(0.,-6.17339315294237E-17,1.));
#106524=DIRECTION('ref_axis',(0.,-1.,0.));
#106525=DIRECTION('center_axis',(1.37076864369198E-30,-3.04371781932207E-44,
1.));
#106526=DIRECTION('ref_axis',(-2.22044604925031E-14,-1.,3.98272977783113E-59));
#106527=DIRECTION('center_axis',(0.991119122260598,0.132976688396752,-0.000292971696495811));
#106528=DIRECTION('ref_axis',(0.132889234509439,-0.990382454371073,0.0385103288147991));
#106529=DIRECTION('center_axis',(0.,0.,-1.));
#106530=DIRECTION('ref_axis',(0.,-1.,0.));
#106531=DIRECTION('center_axis',(-0.98674762086852,-0.162262524904213,7.56440721780465E-5));
#106532=DIRECTION('ref_axis',(0.162172283364071,-0.986183084450869,0.0338093840738556));
#106533=DIRECTION('center_axis',(0.,0.,1.));
#106534=DIRECTION('ref_axis',(0.,-1.,0.));
#106535=DIRECTION('center_axis',(0.,0.,1.));
#106536=DIRECTION('ref_axis',(1.,0.,0.));
#106537=DIRECTION('',(6.19323182390956E-32,-1.23467863058847E-16,1.));
#106538=DIRECTION('center_axis',(0.,0.,1.));
#106539=DIRECTION('ref_axis',(1.,0.,0.));
#106540=DIRECTION('',(0.,1.23467863058847E-16,-1.));
#106541=DIRECTION('center_axis',(-0.959851548777671,0.280508474576272,0.));
#106542=DIRECTION('ref_axis',(-0.280508474576272,-0.959851548777671,0.));
#106543=DIRECTION('center_axis',(0.,0.,1.));
#106544=DIRECTION('ref_axis',(-1.,0.,0.));
#106545=DIRECTION('center_axis',(-0.962287669136798,0.272033898305467,2.53734057564779E-13));
#106546=DIRECTION('ref_axis',(-0.272033898305467,-0.962287669136798,2.03523668564842E-29));
#106547=DIRECTION('center_axis',(0.,0.,-1.));
#106548=DIRECTION('ref_axis',(-1.,0.,0.));
#106549=DIRECTION('center_axis',(0.,0.,1.));
#106550=DIRECTION('ref_axis',(-1.,0.,0.));
#106551=DIRECTION('center_axis',(0.,0.,1.));
#106552=DIRECTION('ref_axis',(1.,0.,0.));
#106553=DIRECTION('center_axis',(0.,0.,1.));
#106554=DIRECTION('ref_axis',(-0.610293066582434,0.792175720961838,0.));
#106555=DIRECTION('',(0.,-1.23467863058847E-16,1.));
#106556=DIRECTION('center_axis',(0.,0.,1.));
#106557=DIRECTION('ref_axis',(1.,0.,0.));
#106558=DIRECTION('',(-6.19323182390956E-32,1.23467863058847E-16,-1.));
#106559=DIRECTION('center_axis',(0.,-6.17339315294237E-17,1.));
#106560=DIRECTION('ref_axis',(0.,-1.,0.));
#106561=DIRECTION('center_axis',(2.19322982990717E-31,-7.79191761746451E-46,
1.));
#106562=DIRECTION('ref_axis',(-3.5527136788005E-15,-1.,-1.0890276736257E-60));
#106563=DIRECTION('center_axis',(0.997057160474908,0.0766613778272904,-0.000227805474783485));
#106564=DIRECTION('ref_axis',(0.0765600400510118,-0.995577374783063,0.0544449362884298));
#106565=DIRECTION('center_axis',(0.,0.,-1.));
#106566=DIRECTION('ref_axis',(0.,-1.,0.));
#106567=DIRECTION('center_axis',(-0.993225936104905,-0.116199124850017,
5.68561820310259E-5));
#106568=DIRECTION('ref_axis',(0.115054757945929,-0.983375585734681,0.140480817391474));
#106569=DIRECTION('center_axis',(0.,0.,1.));
#106570=DIRECTION('ref_axis',(0.,-1.,0.));
#106571=DIRECTION('center_axis',(0.,0.,1.));
#106572=DIRECTION('ref_axis',(1.,0.,0.));
#106573=DIRECTION('',(6.19323182390956E-32,-1.23467863058847E-16,1.));
#106574=DIRECTION('center_axis',(0.,0.,1.));
#106575=DIRECTION('ref_axis',(1.,0.,0.));
#106576=DIRECTION('',(0.,1.23467863058847E-16,-1.));
#106577=DIRECTION('center_axis',(-0.989571111262359,0.142966967401199,-0.017591531686721));
#106578=DIRECTION('ref_axis',(-0.142989093957737,-0.989724264130745,-6.72869096378782E-19));
#106579=DIRECTION('center_axis',(-0.99077695153738,0.134510490459868,-0.0163694917007939));
#106580=DIRECTION('ref_axis',(-0.134528515815408,-0.990909722645057,-8.11100475129765E-19));
#106581=DIRECTION('center_axis',(-0.0107641901120226,-0.163472360314363,
-0.986489188802636));
#106582=DIRECTION('ref_axis',(-0.12265200609037,-0.978880947255001,0.163549920523247));
#106583=DIRECTION('center_axis',(0.00303671056267577,0.143796114116046,
0.989602675801801));
#106584=DIRECTION('ref_axis',(-0.135485018598508,-0.980423214391085,0.142878026366596));
#106585=DIRECTION('center_axis',(-1.66533453693774E-13,1.96105155259282E-14,
1.));
#106586=DIRECTION('ref_axis',(1.,3.15330219577248E-42,1.66533453693774E-13));
#106587=DIRECTION('center_axis',(0.,0.,1.));
#106588=DIRECTION('ref_axis',(-0.664473794614039,0.747311565728258,0.));
#106589=DIRECTION('',(0.,-1.23467863058847E-16,1.));
#106590=DIRECTION('center_axis',(0.,0.,1.));
#106591=DIRECTION('ref_axis',(1.,0.,0.));
#106592=DIRECTION('',(-6.19323182390956E-32,1.23467863058847E-16,-1.));
#106593=DIRECTION('center_axis',(0.,-6.17339315294237E-17,1.));
#106594=DIRECTION('ref_axis',(0.,-1.,0.));
#106595=DIRECTION('center_axis',(-8.2246118621519E-31,-1.09573841495595E-44,
1.));
#106596=DIRECTION('ref_axis',(1.33226762955019E-14,-1.,1.36906336112945E-59));
#106597=DIRECTION('center_axis',(0.999944906622129,0.0104967882139315,-3.40243194832232E-5));
#106598=DIRECTION('ref_axis',(0.0104967884357142,-0.99994490717852,6.34634886399102E-6));
#106599=DIRECTION('center_axis',(0.,0.,-1.));
#106600=DIRECTION('ref_axis',(0.,-1.,0.));
#106601=DIRECTION('center_axis',(-0.998408840407527,-0.0563895966071302,
2.81172984632072E-5));
#106602=DIRECTION('ref_axis',(0.0552480255757205,-0.978096630168846,0.20068541980506));
#106603=DIRECTION('center_axis',(0.,0.,1.));
#106604=DIRECTION('ref_axis',(0.,-1.,0.));
#106605=DIRECTION('center_axis',(0.,0.,1.));
#106606=DIRECTION('ref_axis',(1.,0.,0.));
#106607=DIRECTION('',(6.19323182390956E-32,-1.23467863058847E-16,1.));
#106608=DIRECTION('center_axis',(0.,0.,1.));
#106609=DIRECTION('ref_axis',(1.,0.,0.));
#106610=DIRECTION('',(0.,1.23467863058847E-16,-1.));
#106611=DIRECTION('center_axis',(-0.999990764844661,0.00426925256430225,
-0.000493667835992639));
#106612=DIRECTION('ref_axis',(-0.00426925308452771,-0.999990886697524,1.74890393922737E-21));
#106613=DIRECTION('center_axis',(0.,0.,1.));
#106614=DIRECTION('ref_axis',(0.,-1.,0.));
#106615=DIRECTION('',(0.,1.23467863058847E-16,-1.));
#106616=DIRECTION('',(3.43088182518023E-33,1.23467863058847E-16,-1.));
#106617=DIRECTION('',(0.,-1.23467863058847E-16,1.));
#106618=DIRECTION('center_axis',(-0.908150397510606,0.418644067796653,0.));
#106619=DIRECTION('ref_axis',(-0.418644067796653,-0.908150397510606,0.));
#106620=DIRECTION('center_axis',(-0.691017694403315,0.329301163645224,0.643471281133376));
#106621=DIRECTION('ref_axis',(0.681480917945783,1.81728452038657E-16,0.731835882200219));
#106622=DIRECTION('center_axis',(0.,0.,1.));
#106623=DIRECTION('ref_axis',(-1.,0.,0.));
#106624=DIRECTION('center_axis',(0.,0.,-1.));
#106625=DIRECTION('ref_axis',(-1.,0.,0.));
#106626=DIRECTION('center_axis',(0.,0.,1.));
#106627=DIRECTION('ref_axis',(-1.,0.,0.));
#106628=DIRECTION('center_axis',(1.0547118733939E-12,0.,-1.));
#106629=DIRECTION('ref_axis',(-1.,0.,-1.0547118733939E-12));
#106630=DIRECTION('center_axis',(-2.85977186515575E-47,0.,1.));
#106631=DIRECTION('ref_axis',(0.,-1.,0.));
#106632=DIRECTION('',(-2.85977186515575E-47,5.70122241611331E-32,1.));
#106633=DIRECTION('center_axis',(0.,0.,-1.));
#106634=DIRECTION('ref_axis',(-1.,0.,0.));
#106635=DIRECTION('',(2.85977186515575E-47,-5.70122241611331E-32,-1.));
#106636=DIRECTION('center_axis',(0.,-0.422696864907095,0.906271129628277));
#106637=DIRECTION('ref_axis',(0.,0.906271129628277,0.422696864907095));
#106638=DIRECTION('center_axis',(-1.,0.,0.));
#106639=DIRECTION('ref_axis',(0.,0.976478786201388,0.215613497023408));
#106640=DIRECTION('center_axis',(1.,5.01606788234257E-16,0.));
#106641=DIRECTION('ref_axis',(-5.01606788234257E-16,1.,0.));
#106642=DIRECTION('center_axis',(1.,0.,0.));
#106643=DIRECTION('ref_axis',(0.,0.976373434674102,0.216090064701498));
#106644=DIRECTION('',(0.,0.,1.));
#106645=DIRECTION('center_axis',(1.,-6.16404235248998E-16,2.09401852497606E-16));
#106646=DIRECTION('ref_axis',(6.47177887660072E-16,0.976105817825534,-0.21729572569921));
#106647=DIRECTION('center_axis',(-1.,0.,0.));
#106648=DIRECTION('ref_axis',(0.,0.976212736710707,-0.216814881140091));
#106649=DIRECTION('center_axis',(0.,-1.18842113532926E-16,1.));
#106650=DIRECTION('ref_axis',(0.,1.,1.18842113532926E-16));
#106651=DIRECTION('center_axis',(-1.25618648527741E-14,-0.425033206427438,
0.905177757920515));
#106652=DIRECTION('ref_axis',(-2.68759262534439E-30,0.905177757920515,0.425033206427438));
#106653=DIRECTION('center_axis',(1.,0.,0.));
#106654=DIRECTION('ref_axis',(0.,0.97773854081723,0.20982694250404));
#106655=DIRECTION('center_axis',(-1.,-5.01606788234257E-16,0.));
#106656=DIRECTION('ref_axis',(-5.01606788234257E-16,1.,0.));
#106657=DIRECTION('',(-2.85977186515575E-47,5.70122241611331E-32,1.));
#106658=DIRECTION('center_axis',(1.,0.,0.));
#106659=DIRECTION('ref_axis',(0.,0.978009404010872,-0.20856079609145));
#106660=DIRECTION('',(0.,0.,-1.));
#106661=DIRECTION('center_axis',(0.,0.,1.));
#106662=DIRECTION('ref_axis',(1.,0.,0.));
#106663=DIRECTION('center_axis',(0.,0.,-1.));
#106664=DIRECTION('ref_axis',(-1.,0.,0.));
#106665=DIRECTION('center_axis',(0.,-0.427133403156944,0.904188617439729));
#106666=DIRECTION('ref_axis',(0.,0.904188617439729,0.427133403156944));
#106667=DIRECTION('center_axis',(-0.999999999999896,4.44492331285301E-7,
9.98246615501751E-8));
#106668=DIRECTION('ref_axis',(-3.30569704855731E-8,-0.289344971701435,0.957224888597812));
#106669=DIRECTION('center_axis',(1.,5.01606788234257E-16,0.));
#106670=DIRECTION('ref_axis',(-5.01606788234257E-16,1.,0.));
#106671=DIRECTION('',(2.85977186515575E-47,-5.70122241611331E-32,-1.));
#106672=DIRECTION('',(0.,0.,1.));
#106673=DIRECTION('center_axis',(-1.,0.,0.));
#106674=DIRECTION('ref_axis',(0.,0.979170381919184,-0.203040299379802));
#106675=DIRECTION('center_axis',(0.,-1.18842113532926E-16,1.));
#106676=DIRECTION('ref_axis',(0.,1.,1.18842113532926E-16));
#106677=DIRECTION('center_axis',(4.39817443652073E-16,-0.434491800625061,
0.900675788055609));
#106678=DIRECTION('ref_axis',(9.63119795361041E-32,0.900675788055609,0.434491800625061));
#106679=DIRECTION('center_axis',(0.999999999999961,2.70500792618992E-7,
6.20337317877928E-8));
#106680=DIRECTION('ref_axis',(1.37645772676246E-7,-0.677526578069449,0.735498290962993));
#106681=DIRECTION('center_axis',(-1.,-5.01606788234257E-16,0.));
#106682=DIRECTION('ref_axis',(-5.01606788234257E-16,1.,0.));
#106683=DIRECTION('',(-5.01606788234257E-16,1.,0.));
#106684=DIRECTION('center_axis',(-1.,-6.93889390390722E-16,0.));
#106685=DIRECTION('ref_axis',(-6.93889390390722E-16,1.,0.));
#106686=DIRECTION('',(-2.85977186515575E-47,5.70122241611331E-32,1.));
#106687=DIRECTION('center_axis',(-1.,-6.93889390390722E-16,0.));
#106688=DIRECTION('ref_axis',(-6.93889390390722E-16,1.,0.));
#106689=DIRECTION('',(5.01606788234257E-16,-1.,0.));
#106690=DIRECTION('center_axis',(0.999999999999962,2.70358791824049E-7,
-6.1992890822951E-8));
#106691=DIRECTION('ref_axis',(-1.37951269970466E-7,0.678661255727541,0.734451427920388));
#106692=DIRECTION('',(0.,0.,-1.));
#106693=DIRECTION('center_axis',(0.,-1.,0.));
#106694=DIRECTION('ref_axis',(-1.,0.,0.));
#106695=DIRECTION('',(5.01606788234257E-16,-1.,0.));
#106696=DIRECTION('center_axis',(0.,1.,0.));
#106697=DIRECTION('ref_axis',(0.,0.,-1.));
#106698=DIRECTION('center_axis',(0.,0.,-1.));
#106699=DIRECTION('ref_axis',(0.,-1.,0.));
#106700=DIRECTION('',(-5.01606788234257E-16,1.,0.));
#106701=DIRECTION('',(-1.,-5.01606788234257E-16,0.));
#106702=DIRECTION('center_axis',(0.,-1.,0.));
#106703=DIRECTION('ref_axis',(-1.,0.,0.));
#106704=DIRECTION('',(5.01606788234257E-16,-1.,0.));
#106705=DIRECTION('center_axis',(0.,-1.,0.));
#106706=DIRECTION('ref_axis',(0.,0.,1.));
#106707=DIRECTION('center_axis',(0.,-0.439015545441723,0.898479466020513));
#106708=DIRECTION('ref_axis',(0.,0.898479466020513,0.439015545441723));
#106709=DIRECTION('center_axis',(-0.999999999999983,1.80161300130019E-7,
4.18470807107139E-8));
#106710=DIRECTION('ref_axis',(1.57783577724163E-7,0.949012697225746,-0.315237847512461));
#106711=DIRECTION('center_axis',(1.,5.01606788234257E-16,0.));
#106712=DIRECTION('ref_axis',(-5.01606788234257E-16,1.,0.));
#106713=DIRECTION('',(-5.01606788234257E-16,1.,0.));
#106714=DIRECTION('center_axis',(1.,0.,0.));
#106715=DIRECTION('ref_axis',(0.,-1.,0.));
#106716=DIRECTION('',(2.85977186515575E-47,-5.70122241611331E-32,-1.));
#106717=DIRECTION('center_axis',(1.,0.,0.));
#106718=DIRECTION('ref_axis',(0.,-1.,0.));
#106719=DIRECTION('',(0.,0.,1.));
#106720=DIRECTION('center_axis',(-0.999999999999982,1.83115484047939E-7,
-4.25253431652647E-8));
#106721=DIRECTION('ref_axis',(1.60098072209542E-7,0.948126339374677,0.317893763046633));
#106722=DIRECTION('center_axis',(0.,-1.18842113532926E-16,1.));
#106723=DIRECTION('ref_axis',(0.,1.,1.18842113532926E-16));
#106724=DIRECTION('center_axis',(-1.87193934265674E-16,-0.452600956351886,
0.8917131681821));
#106725=DIRECTION('ref_axis',(4.92064035297146E-32,0.8917131681821,0.452600956351886));
#106726=DIRECTION('center_axis',(1.,2.12837658787934E-8,5.13482592661443E-9));
#106727=DIRECTION('ref_axis',(2.11054534386375E-8,-0.99947069068166,0.0325321144152161));
#106728=DIRECTION('center_axis',(-1.,-5.01606788234257E-16,0.));
#106729=DIRECTION('ref_axis',(-5.01606788234257E-16,1.,0.));
#106730=DIRECTION('',(-5.01606788234257E-16,1.,0.));
#106731=DIRECTION('center_axis',(-1.,0.,0.));
#106732=DIRECTION('ref_axis',(0.,1.,0.));
#106733=DIRECTION('',(-2.85977186515575E-47,5.70122241611331E-32,1.));
#106734=DIRECTION('center_axis',(-1.,0.,0.));
#106735=DIRECTION('ref_axis',(0.,1.,0.));
#106736=DIRECTION('',(5.01606788234257E-16,-1.,0.));
#106737=DIRECTION('center_axis',(1.,2.01124692837111E-8,-4.85055393716843E-9));
#106738=DIRECTION('ref_axis',(1.99358965914732E-8,-0.999421676179656,-0.0340046053093633));
#106739=DIRECTION('',(0.,0.,-1.));
#106740=DIRECTION('center_axis',(0.,-1.,0.));
#106741=DIRECTION('ref_axis',(-1.,0.,0.));
#106742=DIRECTION('center_axis',(0.,1.,0.));
#106743=DIRECTION('ref_axis',(0.,0.,-1.));
#106744=DIRECTION('center_axis',(0.,1.23467863058847E-16,-1.));
#106745=DIRECTION('ref_axis',(0.,1.,1.1837531408762E-16));
#106746=DIRECTION('center_axis',(0.,-1.19392659184112E-16,1.));
#106747=DIRECTION('ref_axis',(0.,1.,1.19392659184112E-16));
#106748=DIRECTION('center_axis',(-0.982083847990974,-0.18844354663646,-0.00058757664438451));
#106749=DIRECTION('ref_axis',(0.152822052410976,-0.798257081809623,0.582607116020463));
#106750=DIRECTION('center_axis',(-1.,0.,0.));
#106751=DIRECTION('ref_axis',(0.,-0.558140143889771,-0.829746696154137));
#106752=DIRECTION('center_axis',(0.,-0.605101105507222,-0.796148636947862));
#106753=DIRECTION('ref_axis',(0.,-0.796148636947862,0.605101105507222));
#106754=DIRECTION('center_axis',(1.,0.,0.));
#106755=DIRECTION('ref_axis',(0.,1.,0.));
#106756=DIRECTION('',(0.,-1.,0.));
#106757=DIRECTION('center_axis',(1.,0.,0.));
#106758=DIRECTION('ref_axis',(0.,0.,1.));
#106759=DIRECTION('',(0.,0.,1.));
#106760=DIRECTION('center_axis',(1.,0.,0.));
#106761=DIRECTION('ref_axis',(0.,0.,1.));
#106762=DIRECTION('',(0.,0.,-1.));
#106763=DIRECTION('center_axis',(1.,0.,0.));
#106764=DIRECTION('ref_axis',(0.,-0.892435299537675,0.45117539398675));
#106765=DIRECTION('center_axis',(0.,-1.,0.));
#106766=DIRECTION('ref_axis',(0.,0.,-1.));
#106767=DIRECTION('',(0.,1.,0.));
#106768=DIRECTION('center_axis',(0.,-1.,0.));
#106769=DIRECTION('ref_axis',(0.,0.,1.));
#106770=DIRECTION('center_axis',(0.,0.,1.));
#106771=DIRECTION('ref_axis',(1.,0.,0.));
#106772=DIRECTION('',(0.,-1.,0.));
#106773=DIRECTION('',(1.,0.,0.));
#106774=DIRECTION('center_axis',(0.,-1.,0.));
#106775=DIRECTION('ref_axis',(0.,0.,-1.));
#106776=DIRECTION('',(0.,1.,0.));
#106777=DIRECTION('center_axis',(0.,1.,0.));
#106778=DIRECTION('ref_axis',(0.,0.,-1.));
#106779=DIRECTION('center_axis',(-1.,0.,1.87032180698308E-16));
#106780=DIRECTION('ref_axis',(0.,1.,0.));
#106781=DIRECTION('center_axis',(0.999999999999995,-9.86470856182844E-8,
2.32552699791497E-8));
#106782=DIRECTION('ref_axis',(9.49367918032427E-8,0.992051753940111,0.125830511023124));
#106783=DIRECTION('',(1.87032180698308E-16,8.19208946723987E-32,1.));
#106784=DIRECTION('center_axis',(-1.,0.,0.));
#106785=DIRECTION('ref_axis',(0.,0.,-1.));
#106786=DIRECTION('',(-1.87032180698308E-16,0.,-1.));
#106787=DIRECTION('center_axis',(-1.,0.,0.));
#106788=DIRECTION('ref_axis',(0.,0.,-1.));
#106789=DIRECTION('center_axis',(-1.85986770746484E-14,-0.444295746197836,
-0.895880176089698));
#106790=DIRECTION('ref_axis',(8.37014173169963E-31,-0.895880176089698,0.444295746197836));
#106791=DIRECTION('center_axis',(0.,-1.18842113532926E-16,1.));
#106792=DIRECTION('ref_axis',(0.,1.,1.18842113532926E-16));
#106793=DIRECTION('center_axis',(-0.999999999999951,-3.06438046744071E-7,
6.9946007058117E-8));
#106794=DIRECTION('ref_axis',(1.06561695484496E-7,-0.539875486220256,-0.841744889725165));
#106795=DIRECTION('center_axis',(0.,-0.432834338283548,-0.901473480254768));
#106796=DIRECTION('ref_axis',(0.,-0.901473480254768,0.432834338283548));
#106797=DIRECTION('center_axis',(1.,0.,0.));
#106798=DIRECTION('ref_axis',(0.,1.,0.));
#106799=DIRECTION('',(0.,0.,1.));
#106800=DIRECTION('center_axis',(1.,0.,0.));
#106801=DIRECTION('ref_axis',(0.,0.000252653767746131,-0.999999968083036));
#106802=DIRECTION('center_axis',(0.,0.,1.));
#106803=DIRECTION('ref_axis',(1.,0.,0.));
#106804=DIRECTION('center_axis',(3.552570199055E-14,1.,2.23044154114413E-16));
#106805=DIRECTION('ref_axis',(0.00256148703537234,1.37530068325002E-16,
-0.999996719386703));
#106806=DIRECTION('center_axis',(0.,0.,1.));
#106807=DIRECTION('ref_axis',(1.,0.,0.));
#106808=DIRECTION('center_axis',(0.,-0.429430624963615,-0.903099849597684));
#106809=DIRECTION('ref_axis',(0.,-0.903099849597684,0.429430624963615));
#106810=DIRECTION('center_axis',(0.999999999999922,-3.86396202578527E-7,
8.73478327237184E-8));
#106811=DIRECTION('ref_axis',(-5.51687521210774E-8,-0.354181556455975,-0.935176681203301));
#106812=DIRECTION('center_axis',(-1.,0.,1.87032180698308E-16));
#106813=DIRECTION('ref_axis',(0.,1.,0.));
#106814=DIRECTION('',(-1.87032180698308E-16,0.,-1.));
#106815=DIRECTION('center_axis',(0.,-1.18842113532926E-16,1.));
#106816=DIRECTION('ref_axis',(0.,1.,1.18842113532926E-16));
#106817=DIRECTION('center_axis',(-1.,1.54885822040769E-14,-1.69750672317071E-15));
#106818=DIRECTION('ref_axis',(1.54954772622702E-14,0.977150339649803,-0.212549320681755));
#106819=DIRECTION('center_axis',(0.,-0.424147858891027,-0.905592951495404));
#106820=DIRECTION('ref_axis',(0.,-0.905592951495404,0.424147858891027));
#106821=DIRECTION('center_axis',(1.,0.,0.));
#106822=DIRECTION('ref_axis',(0.,1.,0.));
#106823=DIRECTION('',(0.,0.,1.));
#106824=DIRECTION('center_axis',(0.,0.,1.));
#106825=DIRECTION('ref_axis',(1.,0.,0.));
#106826=DIRECTION('center_axis',(0.,0.,1.));
#106827=DIRECTION('ref_axis',(1.,0.,0.));
#106828=DIRECTION('center_axis',(-1.,0.,1.87032180698308E-16));
#106829=DIRECTION('ref_axis',(0.,1.,0.));
#106830=DIRECTION('',(-1.87032180698308E-16,0.,-1.));
#106831=DIRECTION('center_axis',(-1.,0.,0.));
#106832=DIRECTION('ref_axis',(0.,1.,0.));
#106833=DIRECTION('',(-1.,-4.18005656861881E-16,0.));
#106834=DIRECTION('center_axis',(1.,0.,0.));
#106835=DIRECTION('ref_axis',(0.,0.,-1.));
#106836=DIRECTION('',(1.,4.18005656861881E-16,0.));
#106837=DIRECTION('center_axis',(0.,0.,-1.));
#106838=DIRECTION('ref_axis',(0.,-1.,0.));
#106839=DIRECTION('',(1.,4.18005656861881E-16,0.));
#106840=DIRECTION('',(-4.18005656861881E-16,1.,0.));
#106841=DIRECTION('center_axis',(-1.,0.,0.));
#106842=DIRECTION('ref_axis',(0.,1.,0.));
#106843=DIRECTION('',(-1.,-4.18005656861881E-16,0.));
#106844=DIRECTION('center_axis',(-1.,0.,0.));
#106845=DIRECTION('ref_axis',(0.,0.,1.));
#106846=DIRECTION('center_axis',(-1.,0.,0.));
#106847=DIRECTION('ref_axis',(0.,1.,0.));
#106848=DIRECTION('',(-1.,-4.18005656861881E-16,0.));
#106849=DIRECTION('center_axis',(1.,0.,0.));
#106850=DIRECTION('ref_axis',(0.,0.,-1.));
#106851=DIRECTION('',(1.,4.18005656861881E-16,0.));
#106852=DIRECTION('center_axis',(0.,0.,-1.));
#106853=DIRECTION('ref_axis',(0.,-1.,0.));
#106854=DIRECTION('',(1.,4.18005656861881E-16,0.));
#106855=DIRECTION('',(-4.18005656861881E-16,1.,0.));
#106856=DIRECTION('center_axis',(-1.,0.,0.));
#106857=DIRECTION('ref_axis',(0.,1.,0.));
#106858=DIRECTION('',(-1.,-4.18005656861881E-16,0.));
#106859=DIRECTION('center_axis',(-1.,0.,0.));
#106860=DIRECTION('ref_axis',(0.,0.,1.));
#106861=DIRECTION('center_axis',(4.18005656861882E-16,-1.,0.));
#106862=DIRECTION('ref_axis',(0.,0.,-1.));
#106863=DIRECTION('',(1.,4.18005656861881E-16,0.));
#106864=DIRECTION('center_axis',(0.,-1.,0.));
#106865=DIRECTION('ref_axis',(-1.,0.,0.));
#106866=DIRECTION('',(0.,0.,-1.));
#106867=DIRECTION('center_axis',(0.,-1.,0.));
#106868=DIRECTION('ref_axis',(-1.,0.,0.));
#106869=DIRECTION('center_axis',(0.,1.,0.));
#106870=DIRECTION('ref_axis',(0.949353414912971,0.,-0.314210269712943));
#106871=DIRECTION('',(0.,0.,1.));
#106872=DIRECTION('center_axis',(2.01185813448618E-8,1.,-4.85634575709083E-9));
#106873=DIRECTION('ref_axis',(0.999508172274741,-1.99563942566965E-8,0.0313594253136996));
#106874=DIRECTION('',(-5.16102651992463E-32,-2.15733828054269E-47,1.));
#106875=DIRECTION('center_axis',(0.452924541251067,-1.8658316499269E-14,
-0.891548854484436));
#106876=DIRECTION('ref_axis',(-0.891548854484436,-1.10243984483832E-29,
-0.452924541251067));
#106877=DIRECTION('center_axis',(0.,-1.18842113532926E-16,1.));
#106878=DIRECTION('ref_axis',(0.,1.,1.18842113532926E-16));
#106879=DIRECTION('center_axis',(1.78035353894022E-7,-0.999999999999983,
4.13792904095341E-8));
#106880=DIRECTION('ref_axis',(0.953984227728196,1.57435058485391E-7,-0.299856787893509));
#106881=DIRECTION('center_axis',(0.439239043992112,0.,-0.898370225593489));
#106882=DIRECTION('ref_axis',(-0.898370225593489,0.,-0.439239043992112));
#106883=DIRECTION('center_axis',(-4.18005656861882E-16,1.,0.));
#106884=DIRECTION('ref_axis',(1.,4.18005656861882E-16,0.));
#106885=DIRECTION('',(1.,4.18005656861881E-16,0.));
#106886=DIRECTION('center_axis',(0.,1.,0.));
#106887=DIRECTION('ref_axis',(1.,0.,0.));
#106888=DIRECTION('',(0.,0.,1.));
#106889=DIRECTION('center_axis',(0.,1.,0.));
#106890=DIRECTION('ref_axis',(1.,0.,0.));
#106891=DIRECTION('',(-1.,-4.18005656861881E-16,0.));
#106892=DIRECTION('',(5.16102651992463E-32,2.15733828054269E-47,-1.));
#106893=DIRECTION('center_axis',(1.77394867447905E-7,-0.999999999999983,
-4.1222642628058E-8));
#106894=DIRECTION('ref_axis',(0.952173814166433,1.56314884088295E-7,0.305556913873213));
#106895=DIRECTION('',(0.,0.,-1.));
#106896=DIRECTION('center_axis',(-1.,0.,0.));
#106897=DIRECTION('ref_axis',(0.,1.,0.));
#106898=DIRECTION('',(-1.,-4.18005656861881E-16,0.));
#106899=DIRECTION('center_axis',(1.,0.,0.));
#106900=DIRECTION('ref_axis',(0.,0.,-1.));
#106901=DIRECTION('center_axis',(0.,0.,-1.));
#106902=DIRECTION('ref_axis',(0.,-1.,0.));
#106903=DIRECTION('',(1.,4.18005656861881E-16,0.));
#106904=DIRECTION('',(-4.18005656861881E-16,1.,0.));
#106905=DIRECTION('center_axis',(-1.,0.,0.));
#106906=DIRECTION('ref_axis',(0.,1.,0.));
#106907=DIRECTION('',(-1.,-4.18005656861881E-16,0.));
#106908=DIRECTION('center_axis',(-1.,0.,0.));
#106909=DIRECTION('ref_axis',(0.,0.,1.));
#106910=DIRECTION('center_axis',(-0.434677673768106,0.,0.900586098009262));
#106911=DIRECTION('ref_axis',(0.900586098009262,0.,0.434677673768106));
#106912=DIRECTION('center_axis',(2.65375153024716E-7,0.999999999999963,
6.08903066929881E-8));
#106913=DIRECTION('ref_axis',(-0.69985050026065,1.42229635936985E-7,0.714289351233027));
#106914=DIRECTION('center_axis',(4.18005656861882E-16,-1.,0.));
#106915=DIRECTION('ref_axis',(0.,0.,-1.));
#106916=DIRECTION('',(0.,0.,1.));
#106917=DIRECTION('center_axis',(2.67568067369228E-7,0.999999999999962,
-6.13851229161734E-8));
#106918=DIRECTION('ref_axis',(0.690330185099942,-1.40298517037424E-7,0.723494461305586));
#106919=DIRECTION('',(-5.16102651992463E-32,-2.15733828054269E-47,1.));
#106920=DIRECTION('center_axis',(0.,-1.,0.));
#106921=DIRECTION('ref_axis',(-1.,0.,0.));
#106922=DIRECTION('',(0.,0.,-1.));
#106923=DIRECTION('center_axis',(0.,-1.,0.));
#106924=DIRECTION('ref_axis',(-1.,0.,0.));
#106925=DIRECTION('center_axis',(0.,-1.18842113532926E-16,1.));
#106926=DIRECTION('ref_axis',(0.,1.,1.18842113532926E-16));
#106927=DIRECTION('center_axis',(-0.427243916491378,0.,0.904136403327014));
#106928=DIRECTION('ref_axis',(0.904136403327014,0.,0.427243916491378));
#106929=DIRECTION('center_axis',(0.,-1.,0.));
#106930=DIRECTION('ref_axis',(0.979260396969467,0.,0.202605712967828));
#106931=DIRECTION('center_axis',(-4.18005656861882E-16,1.,0.));
#106932=DIRECTION('ref_axis',(1.,4.18005656861882E-16,0.));
#106933=DIRECTION('',(0.,0.,1.));
#106934=DIRECTION('',(5.16102651992463E-32,2.15733828054269E-47,-1.));
#106935=DIRECTION('center_axis',(4.42078072401712E-7,-0.999999999999897,
-9.93087227438785E-8));
#106936=DIRECTION('ref_axis',(-0.291484561136116,-3.38626385168455E-8,-0.956575533148995));
#106937=DIRECTION('',(0.,0.,-1.));
#106938=DIRECTION('center_axis',(0.,0.,1.));
#106939=DIRECTION('ref_axis',(1.,0.,0.));
#106940=DIRECTION('center_axis',(0.,0.,-1.));
#106941=DIRECTION('ref_axis',(-1.,0.,0.));
#106942=DIRECTION('center_axis',(-0.425113301005477,0.,0.905140144567805));
#106943=DIRECTION('ref_axis',(0.905140144567805,0.,0.425113301005477));
#106944=DIRECTION('center_axis',(0.,1.,0.));
#106945=DIRECTION('ref_axis',(0.978069789124882,0.,0.208277429408972));
#106946=DIRECTION('center_axis',(4.18005656861882E-16,-1.,0.));
#106947=DIRECTION('ref_axis',(0.,0.,-1.));
#106948=DIRECTION('',(0.,0.,-1.));
#106949=DIRECTION('',(0.,0.,1.));
#106950=DIRECTION('center_axis',(0.,1.,0.));
#106951=DIRECTION('ref_axis',(0.977785987053698,0.,-0.209605733512769));
#106952=DIRECTION('',(-5.16102651992463E-32,-2.15733828054269E-47,1.));
#106953=DIRECTION('center_axis',(0.,-1.18842113532926E-16,1.));
#106954=DIRECTION('ref_axis',(0.,1.,1.18842113532926E-16));
#106955=DIRECTION('center_axis',(-0.422711655064036,-5.86630265286877E-15,
0.906264231156137));
#106956=DIRECTION('ref_axis',(0.906264231156137,8.13850067779198E-31,0.422711655064036));
#106957=DIRECTION('center_axis',(0.,-1.,0.));
#106958=DIRECTION('ref_axis',(0.976222312485803,0.,0.216771761548571));
#106959=DIRECTION('center_axis',(-4.18005656861882E-16,1.,0.));
#106960=DIRECTION('ref_axis',(1.,4.18005656861882E-16,0.));
#106961=DIRECTION('',(0.,0.,1.));
#106962=DIRECTION('',(5.16102651992463E-32,2.15733828054269E-47,-1.));
#106963=DIRECTION('center_axis',(0.,-1.,0.));
#106964=DIRECTION('ref_axis',(0.976488023107232,0.,-0.21557166030842));
#106965=DIRECTION('center_axis',(0.,1.,0.));
#106966=DIRECTION('ref_axis',(0.976392755984516,0.,-0.216002745494037));
#106967=DIRECTION('',(0.,0.,-1.));
#106968=DIRECTION('center_axis',(0.,1.,0.));
#106969=DIRECTION('ref_axis',(0.976124389191499,0.,0.217212285162516));
#106970=DIRECTION('center_axis',(0.,0.,1.));
#106971=DIRECTION('ref_axis',(1.,0.,0.));
#106972=DIRECTION('center_axis',(1.,0.,0.));
#106973=DIRECTION('ref_axis',(0.,-0.0033149217825888,0.999994505631694));
#106974=DIRECTION('center_axis',(0.,0.,1.));
#106975=DIRECTION('ref_axis',(1.,0.,0.));
#106976=DIRECTION('center_axis',(-0.422683349901129,0.,0.906277433083468));
#106977=DIRECTION('ref_axis',(0.906277433083468,0.,0.422683349901129));
#106978=DIRECTION('center_axis',(0.,1.,0.));
#106979=DIRECTION('ref_axis',(0.976470143643405,0.,0.215652634050752));
#106980=DIRECTION('center_axis',(4.18005656861882E-16,-1.,0.));
#106981=DIRECTION('ref_axis',(0.,0.,-1.));
#106982=DIRECTION('center_axis',(0.,-1.,0.));
#106983=DIRECTION('ref_axis',(0.976404651458869,0.,0.21594896760458));
#106984=DIRECTION('',(0.,0.,1.));
#106985=DIRECTION('center_axis',(0.,-1.,0.));
#106986=DIRECTION('ref_axis',(0.976137352210661,0.,-0.217154022802156));
#106987=DIRECTION('center_axis',(0.,1.,0.));
#106988=DIRECTION('ref_axis',(0.976204192855077,0.,-0.216853346416809));
#106989=DIRECTION('',(-5.16102651992463E-32,-2.15733828054269E-47,1.));
#106990=DIRECTION('',(0.,0.,-1.));
#106991=DIRECTION('center_axis',(0.,-1.18842113532926E-16,1.));
#106992=DIRECTION('ref_axis',(0.,1.,1.18842113532926E-16));
#106993=DIRECTION('center_axis',(-0.424954451342053,5.8974277037113E-15,
0.905214733797774));
#106994=DIRECTION('ref_axis',(0.905214733797774,1.745344269554E-30,0.424954451342053));
#106995=DIRECTION('center_axis',(0.,-1.,0.));
#106996=DIRECTION('ref_axis',(0.977685721591009,0.,0.210072915429545));
#106997=DIRECTION('center_axis',(-4.18005656861882E-16,1.,0.));
#106998=DIRECTION('ref_axis',(1.,4.18005656861882E-16,0.));
#106999=DIRECTION('',(0.,0.,1.));
#107000=DIRECTION('',(5.16102651992463E-32,2.15733828054269E-47,-1.));
#107001=DIRECTION('center_axis',(0.,-1.,0.));
#107002=DIRECTION('ref_axis',(0.977956433447826,0.,-0.208809037826448));
#107003=DIRECTION('',(0.,0.,-1.));
#107004=DIRECTION('center_axis',(0.,0.,1.));
#107005=DIRECTION('ref_axis',(1.,0.,0.));
#107006=DIRECTION('center_axis',(0.,0.,1.));
#107007=DIRECTION('ref_axis',(1.,0.,0.));
#107008=DIRECTION('center_axis',(-0.427024288778512,0.,0.904240154380022));
#107009=DIRECTION('ref_axis',(0.904240154380022,0.,0.427024288778512));
#107010=DIRECTION('center_axis',(4.47342289204968E-7,0.999999999999895,
1.00433397542106E-7));
#107011=DIRECTION('ref_axis',(-0.286876404864124,3.21200065696789E-8,0.957967602965901));
#107012=DIRECTION('center_axis',(4.18005656861882E-16,-1.,0.));
#107013=DIRECTION('ref_axis',(0.,0.,-1.));
#107014=DIRECTION('',(0.,0.,1.));
#107015=DIRECTION('center_axis',(0.,1.,0.));
#107016=DIRECTION('ref_axis',(0.979094017787432,0.,-0.203408220907771));
#107017=DIRECTION('',(-5.16102651992463E-32,-2.15733828054269E-47,1.));
#107018=DIRECTION('',(0.,0.,-1.));
#107019=DIRECTION('center_axis',(0.,-1.18842113532926E-16,1.));
#107020=DIRECTION('ref_axis',(0.,1.,1.18842113532926E-16));
#107021=DIRECTION('center_axis',(2.74436147249853E-7,-0.99999999999996,
6.29034153387369E-8));
#107022=DIRECTION('ref_axis',(0.660475707126984,1.34027541627577E-7,-0.750847414788845));
#107023=DIRECTION('center_axis',(0.434307547312743,0.,-0.900764649809921));
#107024=DIRECTION('ref_axis',(-0.900764649809921,0.,-0.434307547312743));
#107025=DIRECTION('center_axis',(-4.18005656861882E-16,1.,0.));
#107026=DIRECTION('ref_axis',(1.,4.18005656861882E-16,0.));
#107027=DIRECTION('',(1.,4.18005656861881E-16,0.));
#107028=DIRECTION('center_axis',(-3.46944695195361E-16,1.,0.));
#107029=DIRECTION('ref_axis',(1.,3.46944695195361E-16,0.));
#107030=DIRECTION('',(0.,0.,1.));
#107031=DIRECTION('center_axis',(-3.46944695195361E-16,1.,0.));
#107032=DIRECTION('ref_axis',(1.,3.46944695195361E-16,0.));
#107033=DIRECTION('',(5.16102651992463E-32,2.15733828054269E-47,-1.));
#107034=DIRECTION('center_axis',(2.74310940053038E-7,-0.99999999999996,
-6.28664519205214E-8));
#107035=DIRECTION('ref_axis',(-0.661953171072186,-1.34459749665864E-7,-0.749545194973231));
#107036=DIRECTION('',(0.,0.,-1.));
#107037=DIRECTION('center_axis',(-1.,0.,0.));
#107038=DIRECTION('ref_axis',(0.,1.,0.));
#107039=DIRECTION('',(-1.,-4.18005656861881E-16,0.));
#107040=DIRECTION('center_axis',(1.,0.,0.));
#107041=DIRECTION('ref_axis',(0.,0.,-1.));
#107042=DIRECTION('center_axis',(0.,0.,-1.));
#107043=DIRECTION('ref_axis',(0.,-1.,0.));
#107044=DIRECTION('',(1.,4.18005656861881E-16,0.));
#107045=DIRECTION('',(-4.18005656861881E-16,1.,0.));
#107046=DIRECTION('center_axis',(-1.,0.,0.));
#107047=DIRECTION('ref_axis',(0.,1.,0.));
#107048=DIRECTION('',(-1.,-4.18005656861881E-16,0.));
#107049=DIRECTION('center_axis',(-1.,0.,0.));
#107050=DIRECTION('ref_axis',(0.,0.,1.));
#107051=DIRECTION('center_axis',(-0.438793812561498,0.,0.898587775377423));
#107052=DIRECTION('ref_axis',(0.898587775377423,0.,0.438793812561498));
#107053=DIRECTION('center_axis',(1.84116539076111E-7,0.999999999999982,
4.27391046394982E-8));
#107054=DIRECTION('ref_axis',(0.944128962664186,-1.59743963387227E-7,-0.329576245895577));
#107055=DIRECTION('center_axis',(4.18005656861882E-16,-1.,0.));
#107056=DIRECTION('ref_axis',(0.,0.,-1.));
#107057=DIRECTION('',(0.,0.,1.));
#107058=DIRECTION('center_axis',(1.87037537959256E-7,0.999999999999982,
-4.3409180827419E-8));
#107059=DIRECTION('ref_axis',(0.943089040549533,-1.61957749522192E-7,0.332540315744325));
#107060=DIRECTION('',(-5.16102651992463E-32,-2.15733828054269E-47,1.));
#107061=DIRECTION('',(1.,4.18005656861881E-16,0.));
#107062=DIRECTION('center_axis',(3.46944695195361E-16,-1.,0.));
#107063=DIRECTION('ref_axis',(-1.,-3.46944695195361E-16,0.));
#107064=DIRECTION('',(0.,0.,-1.));
#107065=DIRECTION('center_axis',(3.46944695195361E-16,-1.,0.));
#107066=DIRECTION('ref_axis',(-1.,-3.46944695195361E-16,0.));
#107067=DIRECTION('center_axis',(0.,-1.18842113532926E-16,1.));
#107068=DIRECTION('ref_axis',(0.,1.,1.18842113532926E-16));
#107069=DIRECTION('center_axis',(2.32689124945317E-8,-1.,5.60875666134475E-9));
#107070=DIRECTION('ref_axis',(0.999404101599166,2.30614476367381E-8,-0.0345172667916152));
#107071=DIRECTION('center_axis',(0.452279624303263,0.,-0.891876191766604));
#107072=DIRECTION('ref_axis',(-0.891876191766604,0.,-0.452279624303263));
#107073=DIRECTION('center_axis',(-4.18005656861882E-16,1.,0.));
#107074=DIRECTION('ref_axis',(1.,4.18005656861882E-16,0.));
#107075=DIRECTION('center_axis',(2.20735454691794E-8,-1.,-5.3187770880344E-9));
#107076=DIRECTION('ref_axis',(0.999350588277669,2.18675573381274E-8,0.0360333416307286));
#107077=DIRECTION('',(0.,0.,-1.));
#107078=DIRECTION('center_axis',(-6.93889390390722E-16,1.,0.));
#107079=DIRECTION('ref_axis',(1.,6.93889390390722E-16,0.));
#107080=DIRECTION('',(0.,0.,1.));
#107081=DIRECTION('center_axis',(-6.93889390390722E-16,1.,0.));
#107082=DIRECTION('ref_axis',(1.,6.93889390390722E-16,0.));
#107083=DIRECTION('',(-1.,-4.18005656861881E-16,0.));
#107084=DIRECTION('',(5.16102651992463E-32,2.15733828054269E-47,-1.));
#107085=DIRECTION('center_axis',(0.,1.23467863058847E-16,-1.));
#107086=DIRECTION('ref_axis',(-1.,0.,0.));
#107087=DIRECTION('center_axis',(0.,1.17559414210783E-16,-1.));
#107088=DIRECTION('ref_axis',(0.,1.,1.17559414210783E-16));
#107089=DIRECTION('',(-5.01606788234257E-16,1.,1.23467863058847E-16));
#107090=DIRECTION('',(5.01606788234257E-16,-1.,-1.23467863058847E-16));
#107091=DIRECTION('center_axis',(0.,-1.,0.));
#107092=DIRECTION('ref_axis',(0.,0.,1.));
#107093=DIRECTION('center_axis',(0.,-1.,0.));
#107094=DIRECTION('ref_axis',(0.,0.,1.));
#107095=DIRECTION('center_axis',(-1.,-5.01606788234257E-16,1.13659195805196E-16));
#107096=DIRECTION('ref_axis',(-5.01606788234257E-16,1.,5.42661491374937E-48));
#107097=DIRECTION('',(5.01606788234257E-16,-1.,-1.23467863058847E-16));
#107098=DIRECTION('',(-1.13659195805196E-16,-4.9783213633841E-32,-1.));
#107099=DIRECTION('',(-5.01606788234257E-16,1.,1.23467863058847E-16));
#107100=DIRECTION('',(-5.01606788234257E-16,1.,0.));
#107101=DIRECTION('center_axis',(-1.,0.,1.13659195805196E-16));
#107102=DIRECTION('ref_axis',(0.,1.,0.));
#107103=DIRECTION('',(1.13659195805196E-16,1.14024448322266E-31,1.));
#107104=DIRECTION('center_axis',(-1.,0.,1.13659195805196E-16));
#107105=DIRECTION('ref_axis',(0.,1.,0.));
#107106=DIRECTION('',(5.01606788234257E-16,-1.,0.));
#107107=DIRECTION('',(-1.13659195805196E-16,1.39441621308911E-16,-1.));
#107108=DIRECTION('center_axis',(0.,-1.,0.));
#107109=DIRECTION('ref_axis',(-1.,0.,0.));
#107110=DIRECTION('',(5.01606788234257E-16,-1.,0.));
#107111=DIRECTION('center_axis',(0.,1.,0.));
#107112=DIRECTION('ref_axis',(0.,0.,-1.));
#107113=DIRECTION('center_axis',(0.,0.,-1.));
#107114=DIRECTION('ref_axis',(0.,-1.,0.));
#107115=DIRECTION('',(-4.38004274807345E-16,1.,0.));
#107116=DIRECTION('',(-1.,-5.01606788234257E-16,0.));
#107117=DIRECTION('center_axis',(0.,1.,0.));
#107118=DIRECTION('ref_axis',(1.,0.,0.));
#107119=DIRECTION('',(4.38004274807345E-16,-1.,0.));
#107120=DIRECTION('center_axis',(0.,1.,0.));
#107121=DIRECTION('ref_axis',(0.,0.,-1.));
#107122=DIRECTION('center_axis',(1.,4.38004274807345E-16,1.13659195805196E-16));
#107123=DIRECTION('ref_axis',(-4.38004274807345E-16,1.,-1.29211895128087E-48));
#107124=DIRECTION('',(-4.38004274807345E-16,1.,1.23467863058847E-16));
#107125=DIRECTION('',(-1.13659195805196E-16,-1.07494104808783E-16,1.));
#107126=DIRECTION('',(-4.38004274807345E-16,1.,0.));
#107127=DIRECTION('center_axis',(1.,0.,1.13659195805196E-16));
#107128=DIRECTION('ref_axis',(0.,-1.,0.));
#107129=DIRECTION('',(1.13659195805196E-16,0.,-1.));
#107130=DIRECTION('center_axis',(1.,0.,1.13659195805196E-16));
#107131=DIRECTION('ref_axis',(0.,-1.,0.));
#107132=DIRECTION('',(4.38004274807345E-16,-1.,-1.23467863058847E-16));
#107133=DIRECTION('',(4.38004274807345E-16,-1.,-1.23467863058847E-16));
#107134=DIRECTION('',(-1.13659195805196E-16,-4.9783213633841E-32,1.));
#107135=DIRECTION('',(-4.38004274807345E-16,1.,1.23467863058847E-16));
#107136=DIRECTION('center_axis',(0.,1.,2.77555756156289E-14));
#107137=DIRECTION('ref_axis',(0.,2.77555756156289E-14,-1.));
#107138=DIRECTION('center_axis',(0.,-0.800147951883018,0.599802680135236));
#107139=DIRECTION('ref_axis',(0.,0.599802680135236,0.800147951883018));
#107140=DIRECTION('center_axis',(1.,5.01606788234257E-16,0.));
#107141=DIRECTION('ref_axis',(-5.01606788234257E-16,1.,0.));
#107142=DIRECTION('',(-5.01606788234257E-16,1.,0.));
#107143=DIRECTION('center_axis',(1.,0.,0.));
#107144=DIRECTION('ref_axis',(0.,-1.,0.));
#107145=DIRECTION('',(2.85977186515575E-47,-5.70122241611331E-32,-1.));
#107146=DIRECTION('center_axis',(1.,0.,0.));
#107147=DIRECTION('ref_axis',(0.,-1.,0.));
#107148=DIRECTION('center_axis',(1.,0.,0.));
#107149=DIRECTION('ref_axis',(0.,0.919361469721465,0.393413888915463));
#107150=DIRECTION('',(0.,0.,1.));
#107151=DIRECTION('',(6.19323182390956E-32,-1.23467863058847E-16,1.));
#107152=DIRECTION('center_axis',(0.,1.23467863058847E-16,-1.));
#107153=DIRECTION('ref_axis',(0.,1.,1.1837531408762E-16));
#107154=DIRECTION('center_axis',(0.,-1.19392659184112E-16,1.));
#107155=DIRECTION('ref_axis',(0.,1.,1.19392659184112E-16));
#107156=DIRECTION('center_axis',(-0.976975053597396,0.213351911799271,-0.000840464134822775));
#107157=DIRECTION('ref_axis',(0.178869337010668,0.821208026530106,0.541870037407396));
#107158=DIRECTION('center_axis',(0.,1.17559414210783E-16,-1.));
#107159=DIRECTION('ref_axis',(0.,1.,1.17559414210783E-16));
#107160=DIRECTION('center_axis',(0.,1.23467863058847E-16,-1.));
#107161=DIRECTION('ref_axis',(-1.,0.,0.));
#107162=DIRECTION('',(5.01606788234257E-16,-1.,-1.23467863058847E-16));
#107163=DIRECTION('center_axis',(0.,-1.,0.));
#107164=DIRECTION('ref_axis',(0.,0.,1.));
#107165=DIRECTION('center_axis',(-1.,-5.01606788234257E-16,0.));
#107166=DIRECTION('ref_axis',(-5.01606788234257E-16,1.,0.));
#107167=DIRECTION('',(-5.01606788234257E-16,1.,0.));
#107168=DIRECTION('center_axis',(-1.,0.,0.));
#107169=DIRECTION('ref_axis',(0.,1.,0.));
#107170=DIRECTION('',(-2.85977186515575E-47,5.70122241611331E-32,1.));
#107171=DIRECTION('center_axis',(-1.,0.,0.));
#107172=DIRECTION('ref_axis',(0.,1.,0.));
#107173=DIRECTION('',(5.01606788234257E-16,-1.,0.));
#107174=DIRECTION('',(-6.19323182390956E-32,1.23467863058847E-16,-1.));
#107175=DIRECTION('',(5.01606788234257E-16,-1.,-1.23467863058847E-16));
#107176=DIRECTION('',(0.,0.,-1.));
#107177=DIRECTION('',(-5.01606788234257E-16,1.,1.23467863058847E-16));
#107178=DIRECTION('center_axis',(0.,-1.,0.));
#107179=DIRECTION('ref_axis',(-1.,0.,0.));
#107180=DIRECTION('',(5.01606788234257E-16,-1.,0.));
#107181=DIRECTION('center_axis',(0.,1.,0.));
#107182=DIRECTION('ref_axis',(0.,0.,-1.));
#107183=DIRECTION('center_axis',(0.,0.,-1.));
#107184=DIRECTION('ref_axis',(0.,-1.,0.));
#107185=DIRECTION('',(-5.01606788234257E-16,1.,0.));
#107186=DIRECTION('',(-1.,-5.01606788234257E-16,0.));
#107187=DIRECTION('center_axis',(0.,-1.,0.));
#107188=DIRECTION('ref_axis',(-1.,0.,0.));
#107189=DIRECTION('',(5.01606788234257E-16,-1.,0.));
#107190=DIRECTION('center_axis',(0.,-1.,0.));
#107191=DIRECTION('ref_axis',(0.,0.,1.));
#107192=DIRECTION('center_axis',(1.,5.01606788234257E-16,0.));
#107193=DIRECTION('ref_axis',(-5.01606788234257E-16,1.,0.));
#107194=DIRECTION('',(-5.01606788234257E-16,1.,0.));
#107195=DIRECTION('center_axis',(1.,0.,0.));
#107196=DIRECTION('ref_axis',(0.,-1.,0.));
#107197=DIRECTION('',(2.85977186515575E-47,-5.70122241611331E-32,-1.));
#107198=DIRECTION('center_axis',(1.,0.,0.));
#107199=DIRECTION('ref_axis',(0.,-1.,0.));
#107200=DIRECTION('',(5.01606788234257E-16,-1.,-1.23467863058847E-16));
#107201=DIRECTION('',(0.,0.,1.));
#107202=DIRECTION('',(-5.01606788234257E-16,1.,1.23467863058847E-16));
#107203=DIRECTION('',(6.19323182390956E-32,-1.23467863058847E-16,1.));
#107204=DIRECTION('center_axis',(0.,1.23467863058847E-16,-1.));
#107205=DIRECTION('ref_axis',(-1.,0.,0.));
#107206=DIRECTION('center_axis',(2.62387838037626E-32,1.17559414210783E-16,
-1.));
#107207=DIRECTION('ref_axis',(-4.44089209850062E-15,1.,1.17559414210783E-16));
#107208=DIRECTION('',(-2.30924636740563E-32,-1.,-1.23467863058847E-16));
#107209=DIRECTION('',(0.,1.,1.23467863058847E-16));
#107210=DIRECTION('center_axis',(0.,-1.,0.));
#107211=DIRECTION('ref_axis',(0.,0.,1.));
#107212=DIRECTION('center_axis',(0.,-1.,0.));
#107213=DIRECTION('ref_axis',(0.,0.,1.));
#107214=DIRECTION('center_axis',(1.,0.,0.));
#107215=DIRECTION('ref_axis',(0.,1.,0.));
#107216=DIRECTION('',(0.,-1.,0.));
#107217=DIRECTION('center_axis',(1.,0.,0.));
#107218=DIRECTION('ref_axis',(0.,0.,1.));
#107219=DIRECTION('',(0.,0.,1.));
#107220=DIRECTION('center_axis',(1.,0.,0.));
#107221=DIRECTION('ref_axis',(0.,0.,1.));
#107222=DIRECTION('',(0.,0.,-1.));
#107223=DIRECTION('',(0.,-1.,-1.23467863058847E-16));
#107224=DIRECTION('center_axis',(0.,-1.,0.));
#107225=DIRECTION('ref_axis',(0.,0.,-1.));
#107226=DIRECTION('',(0.,1.,0.));
#107227=DIRECTION('center_axis',(0.,-1.,0.));
#107228=DIRECTION('ref_axis',(0.,0.,1.));
#107229=DIRECTION('center_axis',(0.,0.,1.));
#107230=DIRECTION('ref_axis',(1.,0.,0.));
#107231=DIRECTION('',(0.,-1.,0.));
#107232=DIRECTION('',(1.,0.,0.));
#107233=DIRECTION('center_axis',(0.,-1.,0.));
#107234=DIRECTION('ref_axis',(0.,0.,-1.));
#107235=DIRECTION('',(0.,1.,0.));
#107236=DIRECTION('center_axis',(0.,1.,0.));
#107237=DIRECTION('ref_axis',(0.,0.,-1.));
#107238=DIRECTION('center_axis',(-1.,0.,1.87032180698308E-16));
#107239=DIRECTION('ref_axis',(0.,1.,0.));
#107240=DIRECTION('',(1.87032180698308E-16,8.19208946723987E-32,1.));
#107241=DIRECTION('center_axis',(-1.,0.,0.));
#107242=DIRECTION('ref_axis',(0.,0.,-1.));
#107243=DIRECTION('',(-1.87032180698308E-16,0.,-1.));
#107244=DIRECTION('center_axis',(-1.,0.,0.));
#107245=DIRECTION('ref_axis',(0.,0.,-1.));
#107246=DIRECTION('center_axis',(3.33932916167122E-16,-0.999710458475598,
-0.0240624025090732));
#107247=DIRECTION('ref_axis',(2.2263435019713E-33,-0.0240624025090732,0.999710458475598));
#107248=DIRECTION('center_axis',(0.,1.,0.));
#107249=DIRECTION('ref_axis',(0.,0.,-1.));
#107250=DIRECTION('center_axis',(-1.,-4.38004274807345E-16,0.));
#107251=DIRECTION('ref_axis',(-4.38004274807345E-16,1.,0.));
#107252=DIRECTION('',(-5.40794518211031E-32,1.23467863058847E-16,-1.));
#107253=DIRECTION('',(4.38004274807345E-16,-1.,-1.23467863058847E-16));
#107254=DIRECTION('',(4.38004274807345E-16,-1.,0.));
#107255=DIRECTION('center_axis',(1.,0.,0.));
#107256=DIRECTION('ref_axis',(0.,1.,0.));
#107257=DIRECTION('',(0.,0.,1.));
#107258=DIRECTION('',(-4.38004274807345E-16,1.,0.));
#107259=DIRECTION('center_axis',(-4.38004274807346E-16,1.,0.));
#107260=DIRECTION('ref_axis',(1.,4.38004274807346E-16,0.));
#107261=DIRECTION('',(-4.38004274807345E-16,1.,0.));
#107262=DIRECTION('center_axis',(0.,-1.,0.));
#107263=DIRECTION('ref_axis',(0.,0.,1.));
#107264=DIRECTION('center_axis',(0.,0.,1.));
#107265=DIRECTION('ref_axis',(1.,0.,0.));
#107266=DIRECTION('',(0.,-1.,0.));
#107267=DIRECTION('',(1.,0.,0.));
#107268=DIRECTION('center_axis',(0.,-1.,0.));
#107269=DIRECTION('ref_axis',(0.,0.,-1.));
#107270=DIRECTION('',(0.,1.,0.));
#107271=DIRECTION('center_axis',(0.,1.,0.));
#107272=DIRECTION('ref_axis',(0.,0.,-1.));
#107273=DIRECTION('center_axis',(-1.,0.,1.87032180698308E-16));
#107274=DIRECTION('ref_axis',(0.,1.,0.));
#107275=DIRECTION('',(-1.87032180698308E-16,0.,-1.));
#107276=DIRECTION('center_axis',(-1.,0.,0.));
#107277=DIRECTION('ref_axis',(0.,0.,-1.));
#107278=DIRECTION('',(2.30924636740563E-32,1.,1.23467863058847E-16));
#107279=DIRECTION('',(1.87032180698308E-16,8.19208946723987E-32,1.));
#107280=DIRECTION('center_axis',(-1.,0.,0.));
#107281=DIRECTION('ref_axis',(0.,0.,-1.));
#107282=DIRECTION('center_axis',(0.,1.23467863058847E-16,-1.));
#107283=DIRECTION('ref_axis',(-1.,0.,0.));
#107284=DIRECTION('center_axis',(5.24775676075252E-32,1.17559414210783E-16,
-1.));
#107285=DIRECTION('ref_axis',(-8.88178419700125E-15,1.,1.17559414210783E-16));
#107286=DIRECTION('',(1.,4.18005656861881E-16,5.16102651992463E-32));
#107287=DIRECTION('',(-1.,-4.18005656861881E-16,-5.16102651992463E-32));
#107288=DIRECTION('center_axis',(1.,0.,0.));
#107289=DIRECTION('ref_axis',(0.,0.,-1.));
#107290=DIRECTION('center_axis',(-1.,0.,0.));
#107291=DIRECTION('ref_axis',(0.,0.,1.));
#107292=DIRECTION('center_axis',(-4.18005656861882E-16,1.,0.));
#107293=DIRECTION('ref_axis',(1.,4.18005656861882E-16,0.));
#107294=DIRECTION('',(-1.,-4.18005656861881E-16,-5.16102651992463E-32));
#107295=DIRECTION('',(0.,0.,-1.));
#107296=DIRECTION('',(1.,4.18005656861881E-16,5.16102651992463E-32));
#107297=DIRECTION('',(1.,4.18005656861881E-16,0.));
#107298=DIRECTION('center_axis',(0.,1.,0.));
#107299=DIRECTION('ref_axis',(1.,0.,0.));
#107300=DIRECTION('',(0.,0.,1.));
#107301=DIRECTION('center_axis',(0.,1.,0.));
#107302=DIRECTION('ref_axis',(1.,0.,0.));
#107303=DIRECTION('',(-1.,-4.18005656861881E-16,0.));
#107304=DIRECTION('',(-1.73522765332111E-17,-7.25334975031394E-33,-1.));
#107305=DIRECTION('center_axis',(-1.,0.,0.));
#107306=DIRECTION('ref_axis',(0.,1.,0.));
#107307=DIRECTION('',(-1.,-4.18005656861881E-16,0.));
#107308=DIRECTION('center_axis',(1.,0.,0.));
#107309=DIRECTION('ref_axis',(0.,0.,-1.));
#107310=DIRECTION('center_axis',(0.,0.,-1.));
#107311=DIRECTION('ref_axis',(0.,-1.,0.));
#107312=DIRECTION('',(1.,4.38004274807345E-16,0.));
#107313=DIRECTION('',(-4.18005656861881E-16,1.,0.));
#107314=DIRECTION('center_axis',(1.,0.,0.));
#107315=DIRECTION('ref_axis',(0.,-1.,0.));
#107316=DIRECTION('',(-1.,-4.38004274807345E-16,0.));
#107317=DIRECTION('center_axis',(-1.,0.,0.));
#107318=DIRECTION('ref_axis',(0.,0.,1.));
#107319=DIRECTION('center_axis',(-1.,0.,0.));
#107320=DIRECTION('ref_axis',(0.,0.,1.));
#107321=DIRECTION('center_axis',(4.38004274807345E-16,-1.,0.));
#107322=DIRECTION('ref_axis',(0.,0.,-1.));
#107323=DIRECTION('',(1.6326809185664E-16,7.15121221728469E-32,1.));
#107324=DIRECTION('',(1.,4.38004274807345E-16,5.40794518211031E-32));
#107325=DIRECTION('',(1.,4.38004274807345E-16,5.40794518211031E-32));
#107326=DIRECTION('',(1.73522765332111E-17,7.60037129918566E-33,1.));
#107327=DIRECTION('',(1.,4.38004274807345E-16,0.));
#107328=DIRECTION('center_axis',(0.,-1.,0.));
#107329=DIRECTION('ref_axis',(-1.,0.,0.));
#107330=DIRECTION('',(0.,0.,-1.));
#107331=DIRECTION('center_axis',(0.,-1.,0.));
#107332=DIRECTION('ref_axis',(-1.,0.,0.));
#107333=DIRECTION('',(-1.,-4.38004274807345E-16,-5.40794518211031E-32));
#107334=DIRECTION('',(-1.,-4.38004274807345E-16,-5.40794518211031E-32));
#107335=DIRECTION('',(-5.40794518211031E-32,-2.3687031076881E-47,1.));
#107336=DIRECTION('center_axis',(0.,1.,0.));
#107337=DIRECTION('ref_axis',(-1.,0.,0.));
#107338=DIRECTION('center_axis',(4.18005656861882E-16,-1.,0.));
#107339=DIRECTION('ref_axis',(0.,0.,-1.));
#107340=DIRECTION('',(1.,4.18005656861881E-16,0.));
#107341=DIRECTION('center_axis',(6.93889390390722E-16,-1.,0.));
#107342=DIRECTION('ref_axis',(-1.,-6.93889390390722E-16,0.));
#107343=DIRECTION('',(0.,0.,-1.));
#107344=DIRECTION('center_axis',(6.93889390390722E-16,-1.,0.));
#107345=DIRECTION('ref_axis',(-1.,-6.93889390390722E-16,0.));
#107346=DIRECTION('center_axis',(0.,1.,0.));
#107347=DIRECTION('ref_axis',(0.964920734332925,0.,0.262541380461079));
#107348=DIRECTION('center_axis',(0.,1.,0.));
#107349=DIRECTION('ref_axis',(-0.285513244926914,0.,0.958374763321376));
#107350=DIRECTION('center_axis',(0.,-1.,0.));
#107351=DIRECTION('ref_axis',(0.882822386976779,0.,0.469706965088471));
#107352=DIRECTION('',(0.,0.,1.));
#107353=DIRECTION('',(-5.16102651992463E-32,-2.15733828054269E-47,1.));
#107354=DIRECTION('center_axis',(0.403600920616143,-3.09956391918065E-14,
-0.91493513260657));
#107355=DIRECTION('ref_axis',(-0.91493513260657,-7.63177238048844E-30,-0.403600920616143));
#107356=DIRECTION('center_axis',(0.,1.23467863058847E-16,-1.));
#107357=DIRECTION('ref_axis',(0.,1.,1.1837531408762E-16));
#107358=DIRECTION('center_axis',(0.,-1.19392659184112E-16,1.));
#107359=DIRECTION('ref_axis',(0.,1.,1.19392659184112E-16));
#107360=DIRECTION('center_axis',(0.212543372582222,0.977151310604023,-0.000794327523214365));
#107361=DIRECTION('ref_axis',(0.808607924198044,-0.175426436275447,0.561585959920498));
#107362=DIRECTION('center_axis',(-3.98829513817191E-31,1.17559414210783E-16,
-1.));
#107363=DIRECTION('ref_axis',(6.75015598972095E-14,1.,1.17559414210783E-16));
#107364=DIRECTION('center_axis',(0.,1.23467863058847E-16,-1.));
#107365=DIRECTION('ref_axis',(-1.,0.,0.));
#107366=DIRECTION('',(-1.,-4.18005656861881E-16,-5.16102651992463E-32));
#107367=DIRECTION('center_axis',(-1.,0.,0.));
#107368=DIRECTION('ref_axis',(0.,0.,1.));
#107369=DIRECTION('center_axis',(-4.18005656861882E-16,1.,0.));
#107370=DIRECTION('ref_axis',(1.,4.18005656861882E-16,0.));
#107371=DIRECTION('',(1.,4.18005656861881E-16,0.));
#107372=DIRECTION('center_axis',(0.,1.,0.));
#107373=DIRECTION('ref_axis',(1.,0.,0.));
#107374=DIRECTION('',(0.,0.,1.));
#107375=DIRECTION('center_axis',(0.,1.,0.));
#107376=DIRECTION('ref_axis',(1.,0.,0.));
#107377=DIRECTION('',(-1.,-4.18005656861881E-16,0.));
#107378=DIRECTION('',(-1.73522765332111E-17,-7.25334975031394E-33,-1.));
#107379=DIRECTION('',(-1.,-4.18005656861881E-16,-5.16102651992463E-32));
#107380=DIRECTION('',(0.,0.,-1.));
#107381=DIRECTION('',(1.,4.18005656861881E-16,5.16102651992463E-32));
#107382=DIRECTION('center_axis',(-1.,0.,0.));
#107383=DIRECTION('ref_axis',(0.,1.,0.));
#107384=DIRECTION('',(-1.,-4.18005656861881E-16,0.));
#107385=DIRECTION('center_axis',(1.,0.,0.));
#107386=DIRECTION('ref_axis',(0.,0.,-1.));
#107387=DIRECTION('center_axis',(0.,0.,-1.));
#107388=DIRECTION('ref_axis',(0.,-1.,0.));
#107389=DIRECTION('',(1.,4.18005656861881E-16,0.));
#107390=DIRECTION('',(-4.18005656861881E-16,1.,0.));
#107391=DIRECTION('center_axis',(-1.,0.,0.));
#107392=DIRECTION('ref_axis',(0.,1.,0.));
#107393=DIRECTION('',(-1.,-4.18005656861881E-16,0.));
#107394=DIRECTION('center_axis',(-1.,0.,0.));
#107395=DIRECTION('ref_axis',(0.,0.,1.));
#107396=DIRECTION('center_axis',(4.18005656861882E-16,-1.,0.));
#107397=DIRECTION('ref_axis',(0.,0.,-1.));
#107398=DIRECTION('',(1.,4.18005656861881E-16,0.));
#107399=DIRECTION('center_axis',(0.,-1.,0.));
#107400=DIRECTION('ref_axis',(-1.,0.,0.));
#107401=DIRECTION('',(0.,0.,-1.));
#107402=DIRECTION('center_axis',(0.,-1.,0.));
#107403=DIRECTION('ref_axis',(-1.,0.,0.));
#107404=DIRECTION('',(-1.,-4.18005656861881E-16,-5.16102651992463E-32));
#107405=DIRECTION('',(0.,0.,1.));
#107406=DIRECTION('',(1.,4.18005656861881E-16,5.16102651992463E-32));
#107407=DIRECTION('',(1.73522765332111E-17,7.25334975031394E-33,1.));
#107408=DIRECTION('center_axis',(0.,1.23467863058847E-16,-1.));
#107409=DIRECTION('ref_axis',(0.,1.,1.1837531408762E-16));
#107410=DIRECTION('center_axis',(0.,-1.19392659184112E-16,1.));
#107411=DIRECTION('ref_axis',(0.,1.,1.19392659184112E-16));
#107412=DIRECTION('center_axis',(0.,1.17559414210783E-16,-1.));
#107413=DIRECTION('ref_axis',(0.,1.,1.17559414210783E-16));
#107414=DIRECTION('center_axis',(0.214155640377145,-0.97679914458343,-0.000890413238434334));
#107415=DIRECTION('ref_axis',(0.833617683430173,0.18323919483608,-0.52106137387868));
#107416=DIRECTION('center_axis',(0.817080261705548,0.,-0.576523933528517));
#107417=DIRECTION('ref_axis',(-0.576523933528517,0.,-0.817080261705548));
#107418=DIRECTION('center_axis',(-4.18005656861882E-16,1.,0.));
#107419=DIRECTION('ref_axis',(1.,4.18005656861882E-16,0.));
#107420=DIRECTION('',(0.,0.,-1.));
#107421=DIRECTION('center_axis',(0.,1.,0.));
#107422=DIRECTION('ref_axis',(0.979462303582526,0.,-0.201627368828764));
#107423=DIRECTION('center_axis',(0.,1.,0.));
#107424=DIRECTION('ref_axis',(1.,0.,0.));
#107425=DIRECTION('',(0.,0.,1.));
#107426=DIRECTION('center_axis',(0.,1.,0.));
#107427=DIRECTION('ref_axis',(1.,0.,0.));
#107428=DIRECTION('',(-1.,-4.18005656861881E-16,0.));
#107429=DIRECTION('',(5.16102651992463E-32,2.15733828054269E-47,-1.));
#107430=DIRECTION('center_axis',(-1.,0.,0.));
#107431=DIRECTION('ref_axis',(0.,0.,1.));
#107432=DIRECTION('center_axis',(-4.38004274807345E-16,1.,0.));
#107433=DIRECTION('ref_axis',(1.,4.38004274807345E-16,0.));
#107434=DIRECTION('',(-1.,-4.38004274807345E-16,-5.40794518211031E-32));
#107435=DIRECTION('',(-1.,-4.38004274807345E-16,-5.40794518211031E-32));
#107436=DIRECTION('',(1.13659195805196E-16,4.9783213633841E-32,-1.));
#107437=DIRECTION('',(1.,4.38004274807345E-16,5.40794518211031E-32));
#107438=DIRECTION('',(1.,4.38004274807345E-16,5.40794518211031E-32));
#107439=DIRECTION('',(1.,4.38004274807345E-16,0.));
#107440=DIRECTION('center_axis',(0.,1.,0.));
#107441=DIRECTION('ref_axis',(1.,0.,0.));
#107442=DIRECTION('',(0.,0.,1.));
#107443=DIRECTION('center_axis',(0.,1.,0.));
#107444=DIRECTION('ref_axis',(1.,0.,0.));
#107445=DIRECTION('',(-1.,-4.38004274807345E-16,0.));
#107446=DIRECTION('',(1.73522765332109E-17,7.60037129918555E-33,-1.));
#107447=DIRECTION('center_axis',(1.,0.,0.));
#107448=DIRECTION('ref_axis',(0.,-1.,0.));
#107449=DIRECTION('',(-1.,-4.38004274807345E-16,0.));
#107450=DIRECTION('center_axis',(-1.,0.,0.));
#107451=DIRECTION('ref_axis',(0.,0.,1.));
#107452=DIRECTION('center_axis',(0.,0.,-1.));
#107453=DIRECTION('ref_axis',(0.,-1.,0.));
#107454=DIRECTION('',(1.,4.18005656861881E-16,0.));
#107455=DIRECTION('',(-4.18005656861881E-16,1.,0.));
#107456=DIRECTION('center_axis',(-1.,0.,0.));
#107457=DIRECTION('ref_axis',(0.,1.,0.));
#107458=DIRECTION('',(-1.,-4.18005656861881E-16,0.));
#107459=DIRECTION('center_axis',(-1.,0.,0.));
#107460=DIRECTION('ref_axis',(0.,0.,1.));
#107461=DIRECTION('center_axis',(4.18005656861882E-16,-1.,0.));
#107462=DIRECTION('ref_axis',(0.,0.,-1.));
#107463=DIRECTION('',(1.,4.18005656861881E-16,0.));
#107464=DIRECTION('center_axis',(0.,-1.,0.));
#107465=DIRECTION('ref_axis',(-1.,0.,0.));
#107466=DIRECTION('',(0.,0.,-1.));
#107467=DIRECTION('center_axis',(0.,-1.,0.));
#107468=DIRECTION('ref_axis',(-1.,0.,0.));
#107469=DIRECTION('',(-1.,-4.18005656861881E-16,-5.16102651992463E-32));
#107470=DIRECTION('',(0.,0.,1.));
#107471=DIRECTION('',(1.,4.18005656861881E-16,5.16102651992463E-32));
#107472=DIRECTION('',(-1.73522765332109E-17,-7.25334975031383E-33,1.));
#107473=DIRECTION('center_axis',(1.,-1.38777878078144E-14,1.38777878078144E-14));
#107474=DIRECTION('ref_axis',(1.38777878078144E-14,4.48415508583941E-44,
-1.));
#107475=DIRECTION('center_axis',(0.,1.23467863058847E-16,-1.));
#107476=DIRECTION('ref_axis',(-1.,0.,0.));
#107477=DIRECTION('center_axis',(8.39641081720404E-32,1.17559414210783E-16,
-1.));
#107478=DIRECTION('ref_axis',(-1.4210854715202E-14,1.,1.17559414210783E-16));
#107479=DIRECTION('',(1.,4.18005656861881E-16,5.16102651992463E-32));
#107480=DIRECTION('',(-1.,-4.18005656861881E-16,-5.16102651992463E-32));
#107481=DIRECTION('center_axis',(-1.,0.,0.));
#107482=DIRECTION('ref_axis',(0.,0.,1.));
#107483=DIRECTION('center_axis',(-4.18005656861882E-16,1.,0.));
#107484=DIRECTION('ref_axis',(1.,4.18005656861882E-16,0.));
#107485=DIRECTION('',(1.,4.18005656861881E-16,0.));
#107486=DIRECTION('center_axis',(0.,1.,0.));
#107487=DIRECTION('ref_axis',(1.,0.,0.));
#107488=DIRECTION('',(0.,0.,1.));
#107489=DIRECTION('center_axis',(0.,1.,0.));
#107490=DIRECTION('ref_axis',(1.,0.,0.));
#107491=DIRECTION('',(-1.,-4.18005656861881E-16,0.));
#107492=DIRECTION('',(1.73522765332109E-17,7.25334975031383E-33,-1.));
#107493=DIRECTION('',(-1.,-4.18005656861881E-16,-5.16102651992463E-32));
#107494=DIRECTION('',(0.,0.,-1.));
#107495=DIRECTION('',(1.,4.18005656861881E-16,5.16102651992463E-32));
#107496=DIRECTION('center_axis',(-1.,0.,0.));
#107497=DIRECTION('ref_axis',(0.,1.,0.));
#107498=DIRECTION('',(-1.,-4.18005656861881E-16,0.));
#107499=DIRECTION('center_axis',(1.,0.,0.));
#107500=DIRECTION('ref_axis',(0.,0.,-1.));
#107501=DIRECTION('center_axis',(0.,0.,-1.));
#107502=DIRECTION('ref_axis',(0.,-1.,0.));
#107503=DIRECTION('',(1.,4.18005656861881E-16,0.));
#107504=DIRECTION('',(-4.18005656861881E-16,1.,0.));
#107505=DIRECTION('center_axis',(-1.,0.,0.));
#107506=DIRECTION('ref_axis',(0.,1.,0.));
#107507=DIRECTION('',(-1.,-4.18005656861881E-16,0.));
#107508=DIRECTION('center_axis',(-1.,0.,0.));
#107509=DIRECTION('ref_axis',(0.,0.,1.));
#107510=DIRECTION('center_axis',(-1.,0.,0.));
#107511=DIRECTION('ref_axis',(0.,0.,1.));
#107512=DIRECTION('center_axis',(4.18005656861882E-16,-1.,0.));
#107513=DIRECTION('ref_axis',(0.,0.,-1.));
#107514=DIRECTION('',(1.,4.18005656861881E-16,0.));
#107515=DIRECTION('center_axis',(0.,-1.,0.));
#107516=DIRECTION('ref_axis',(-1.,0.,0.));
#107517=DIRECTION('',(0.,0.,-1.));
#107518=DIRECTION('center_axis',(0.,-1.,0.));
#107519=DIRECTION('ref_axis',(-1.,0.,0.));
#107520=DIRECTION('',(-1.,-4.18005656861881E-16,-5.16102651992463E-32));
#107521=DIRECTION('',(0.,0.,1.));
#107522=DIRECTION('',(1.,4.18005656861881E-16,5.16102651992463E-32));
#107523=DIRECTION('',(-1.73522765332109E-17,-7.25334975031383E-33,1.));
#107524=DIRECTION('center_axis',(0.,1.23467863058847E-16,-1.));
#107525=DIRECTION('ref_axis',(-1.,0.,0.));
#107526=DIRECTION('',(1.,4.18005656861881E-16,5.16102651992463E-32));
#107527=DIRECTION('center_axis',(1.,4.38004274807346E-16,5.40794518211031E-32));
#107528=DIRECTION('ref_axis',(4.38004274807346E-16,-1.,-5.80597460094347E-63));
#107529=DIRECTION('center_axis',(-1.,-4.38004274807345E-16,0.));
#107530=DIRECTION('ref_axis',(0.,0.,-1.));
#107531=DIRECTION('center_axis',(0.,0.,-1.));
#107532=DIRECTION('ref_axis',(0.,1.,0.));
#107533=DIRECTION('center_axis',(0.,0.,-1.));
#107534=DIRECTION('ref_axis',(1.,0.,0.));
#107535=DIRECTION('',(0.,0.,-1.));
#107536=DIRECTION('center_axis',(0.,0.,1.));
#107537=DIRECTION('ref_axis',(0.,1.,0.));
#107538=DIRECTION('center_axis',(0.,1.23467863058847E-16,-1.));
#107539=DIRECTION('ref_axis',(-1.,0.,0.));
#107540=DIRECTION('center_axis',(0.,0.,1.));
#107541=DIRECTION('ref_axis',(0.,1.,0.));
#107542=DIRECTION('center_axis',(0.,0.,-1.));
#107543=DIRECTION('ref_axis',(0.,1.,0.));
#107544=DIRECTION('',(0.,0.,-1.));
#107545=DIRECTION('center_axis',(1.,4.38004274807346E-16,5.40794518211031E-32));
#107546=DIRECTION('ref_axis',(4.38004274807346E-16,-1.,-5.80597460094347E-63));
#107547=DIRECTION('center_axis',(1.,4.38004274807345E-16,-4.02455846426619E-13));
#107548=DIRECTION('ref_axis',(-4.02455846426619E-13,-4.48415508583941E-44,
-1.));
#107549=DIRECTION('center_axis',(1.,0.,0.));
#107550=DIRECTION('ref_axis',(0.,0.,-1.));
#107551=DIRECTION('center_axis',(0.71239495798367,0.701778757044872,0.));
#107552=DIRECTION('ref_axis',(-0.701778757044872,0.71239495798367,0.));
#107553=DIRECTION('center_axis',(-1.71346080461497E-30,2.37790454634537E-44,
-1.));
#107554=DIRECTION('ref_axis',(1.38777878078144E-14,1.,2.48920611114446E-59));
#107555=DIRECTION('center_axis',(0.,1.23467863058847E-16,-1.));
#107556=DIRECTION('ref_axis',(0.,1.,1.19418947186571E-16));
#107557=DIRECTION('center_axis',(0.740307041655026,0.672268907563025,0.));
#107558=DIRECTION('ref_axis',(-0.672268907563025,0.740307041655026,0.));
#107559=DIRECTION('center_axis',(0.,-1.18613571006961E-16,1.));
#107560=DIRECTION('ref_axis',(0.,1.,1.18613571006961E-16));
#107561=DIRECTION('center_axis',(0.,1.,0.));
#107562=DIRECTION('ref_axis',(0.,0.,-1.));
#107563=DIRECTION('center_axis',(-8.56730402307488E-31,5.94476136586342E-45,
-1.));
#107564=DIRECTION('ref_axis',(6.93889390390722E-15,1.,9.95682444457783E-60));
#107565=DIRECTION('center_axis',(0.,1.,1.23467863058847E-16));
#107566=DIRECTION('ref_axis',(1.,0.,0.));
#107567=DIRECTION('center_axis',(0.,1.,1.23467863058847E-16));
#107568=DIRECTION('ref_axis',(1.,0.,0.));
#107569=DIRECTION('center_axis',(0.,1.,0.));
#107570=DIRECTION('ref_axis',(0.,0.,-1.));
#107571=DIRECTION('center_axis',(0.,0.,-1.));
#107572=DIRECTION('ref_axis',(0.,1.,0.));
#107573=DIRECTION('center_axis',(0.,0.,-1.));
#107574=DIRECTION('ref_axis',(1.,0.,0.));
#107575=DIRECTION('',(0.,0.,-1.));
#107576=DIRECTION('center_axis',(0.,0.,1.));
#107577=DIRECTION('ref_axis',(0.,1.,0.));
#107578=DIRECTION('center_axis',(0.,1.23467863058847E-16,-1.));
#107579=DIRECTION('ref_axis',(-1.,0.,0.));
#107580=DIRECTION('center_axis',(0.,0.,1.));
#107581=DIRECTION('ref_axis',(0.,1.,0.));
#107582=DIRECTION('center_axis',(0.,0.,-1.));
#107583=DIRECTION('ref_axis',(0.,1.,0.));
#107584=DIRECTION('',(0.,0.,-1.));
#107585=DIRECTION('center_axis',(0.,0.,1.));
#107586=DIRECTION('ref_axis',(0.,1.,0.));
#107587=DIRECTION('center_axis',(-1.,-4.38004274807346E-16,-5.40794518211031E-32));
#107588=DIRECTION('ref_axis',(-4.38004274807346E-16,1.,5.80597460094347E-63));
#107589=DIRECTION('center_axis',(-1.,-4.38004274807345E-16,0.));
#107590=DIRECTION('ref_axis',(0.,0.,1.));
#107591=DIRECTION('center_axis',(-1.,-5.01606788234257E-16,0.));
#107592=DIRECTION('ref_axis',(-5.01606788234257E-16,1.,0.));
#107593=DIRECTION('center_axis',(-1.,0.,0.));
#107594=DIRECTION('ref_axis',(0.,-1.,0.));
#107595=DIRECTION('',(1.,5.01606788234257E-16,0.));
#107596=DIRECTION('center_axis',(1.,0.,0.));
#107597=DIRECTION('ref_axis',(0.,1.,0.));
#107598=DIRECTION('center_axis',(1.,5.01606788234257E-16,0.));
#107599=DIRECTION('ref_axis',(0.,-1.,0.));
#107600=DIRECTION('center_axis',(0.,0.,-1.));
#107601=DIRECTION('ref_axis',(-1.,0.,0.));
#107602=DIRECTION('center_axis',(0.,0.,1.));
#107603=DIRECTION('ref_axis',(-1.,0.,0.));
#107604=DIRECTION('',(1.87032180698308E-16,0.,1.));
#107605=DIRECTION('center_axis',(0.,0.,-1.));
#107606=DIRECTION('ref_axis',(-1.,0.,0.));
#107607=DIRECTION('center_axis',(0.,1.,0.));
#107608=DIRECTION('ref_axis',(1.,0.,0.));
#107609=DIRECTION('',(0.,0.,-1.));
#107610=DIRECTION('',(-1.,0.,0.));
#107611=DIRECTION('center_axis',(0.,-1.,0.));
#107612=DIRECTION('ref_axis',(0.,0.,1.));
#107613=DIRECTION('center_axis',(-0.488849591387095,-0.481564692142823,
-0.727407399111432));
#107614=DIRECTION('ref_axis',(-0.82998476161361,2.33877977530395E-17,0.557786066058662));
#107615=DIRECTION('center_axis',(-0.366954554655378,-9.16653140031321E-14,
-0.930238869762855));
#107616=DIRECTION('ref_axis',(-0.930238869762855,-2.79622788237931E-29,
0.366954554655378));
#107617=DIRECTION('center_axis',(4.38004274807345E-16,-1.,0.));
#107618=DIRECTION('ref_axis',(-1.,0.,0.));
#107619=DIRECTION('center_axis',(0.,0.,-1.));
#107620=DIRECTION('ref_axis',(-1.,0.,0.));
#107621=DIRECTION('center_axis',(0.,-1.,0.));
#107622=DIRECTION('ref_axis',(0.,0.,-1.));
#107623=DIRECTION('center_axis',(0.,-1.,0.));
#107624=DIRECTION('ref_axis',(0.,0.,1.));
#107625=DIRECTION('center_axis',(-0.716305556970081,-0.650473286312467,
-0.252568511195758));
#107626=DIRECTION('ref_axis',(0.672268907563029,-0.740307041655023,-6.62280424422414E-17));
#107627=DIRECTION('center_axis',(0.,0.,1.));
#107628=DIRECTION('ref_axis',(-1.,0.,0.));
#107629=DIRECTION('',(1.87032180698308E-16,0.,1.));
#107630=DIRECTION('center_axis',(0.,1.,0.));
#107631=DIRECTION('ref_axis',(1.,0.,0.));
#107632=DIRECTION('',(0.,0.,-1.));
#107633=DIRECTION('center_axis',(0.,0.,-1.));
#107634=DIRECTION('ref_axis',(1.,0.,0.));
#107635=DIRECTION('center_axis',(0.,-0.425268108821871,-0.905067420482623));
#107636=DIRECTION('ref_axis',(0.,-0.905067420482623,0.425268108821871));
#107637=DIRECTION('center_axis',(0.,-0.434584798675586,-0.900630919278314));
#107638=DIRECTION('ref_axis',(0.,-0.900630919278314,0.434584798675586));
#107639=DIRECTION('center_axis',(0.,0.,1.));
#107640=DIRECTION('ref_axis',(-1.,0.,0.));
#107641=DIRECTION('',(1.87032180698308E-16,0.,1.));
#107642=DIRECTION('center_axis',(0.,1.,0.));
#107643=DIRECTION('ref_axis',(1.,0.,0.));
#107644=DIRECTION('',(0.,0.,-1.));
#107645=DIRECTION('center_axis',(0.,0.,-1.));
#107646=DIRECTION('ref_axis',(1.,0.,0.));
#107647=DIRECTION('center_axis',(1.79937481368581E-15,-0.983475799774124,
0.181039640020212));
#107648=DIRECTION('ref_axis',(3.24346588047852E-31,0.181039640020212,0.983475799774124));
#107649=DIRECTION('center_axis',(0.,-0.425920949091245,-0.904760379948864));
#107650=DIRECTION('ref_axis',(0.,-0.904760379948864,0.425920949091245));
#107651=DIRECTION('center_axis',(-6.15557891118828E-9,1.,-7.98957508368948E-9));
#107652=DIRECTION('ref_axis',(0.717962811307083,-1.14191836379562E-9,-0.696081461885051));
#107653=DIRECTION('center_axis',(-0.998868362320773,0.00644281759551,0.0471220209249073));
#107654=DIRECTION('ref_axis',(0.0465471507530001,0.335857313107545,0.940762046422451));
#107655=DIRECTION('center_axis',(4.38004274807345E-16,-1.,0.));
#107656=DIRECTION('ref_axis',(0.,0.,-1.));
#107657=DIRECTION('',(-1.87032180698308E-16,-8.19208946723987E-32,-1.));
#107658=DIRECTION('center_axis',(0.,0.,-1.));
#107659=DIRECTION('ref_axis',(-1.,0.,0.));
#107660=DIRECTION('center_axis',(0.,0.,1.));
#107661=DIRECTION('ref_axis',(-1.,0.,0.));
#107662=DIRECTION('',(1.87032180698308E-16,0.,1.));
#107663=DIRECTION('center_axis',(0.,0.,-1.));
#107664=DIRECTION('ref_axis',(-1.,0.,0.));
#107665=DIRECTION('center_axis',(0.,1.,0.));
#107666=DIRECTION('ref_axis',(1.,0.,0.));
#107667=DIRECTION('',(0.,0.,-1.));
#107668=DIRECTION('',(-1.,0.,0.));
#107669=DIRECTION('center_axis',(0.,0.,-1.));
#107670=DIRECTION('ref_axis',(1.,0.,0.));
#107671=DIRECTION('center_axis',(0.,0.,1.));
#107672=DIRECTION('ref_axis',(1.,0.,0.));
#107673=DIRECTION('center_axis',(0.,0.,-1.));
#107674=DIRECTION('ref_axis',(-1.,0.,0.));
#107675=DIRECTION('center_axis',(4.38004274807345E-16,-1.,0.));
#107676=DIRECTION('ref_axis',(0.,0.,-1.));
#107677=DIRECTION('',(-1.87032180698308E-16,-8.19208946723987E-32,-1.));
#107678=DIRECTION('',(0.,0.,1.));
#107679=DIRECTION('center_axis',(0.,0.,-1.));
#107680=DIRECTION('ref_axis',(-1.,0.,0.));
#107681=DIRECTION('center_axis',(0.,0.,1.));
#107682=DIRECTION('ref_axis',(-1.,0.,0.));
#107683=DIRECTION('',(1.87032180698308E-16,0.,1.));
#107684=DIRECTION('center_axis',(0.,0.,-1.));
#107685=DIRECTION('ref_axis',(-1.,0.,0.));
#107686=DIRECTION('center_axis',(0.,1.,0.));
#107687=DIRECTION('ref_axis',(1.,0.,0.));
#107688=DIRECTION('',(0.,0.,-1.));
#107689=DIRECTION('',(-1.,0.,0.));
#107690=DIRECTION('center_axis',(0.,0.,-1.));
#107691=DIRECTION('ref_axis',(1.,0.,0.));
#107692=DIRECTION('center_axis',(0.,0.,1.));
#107693=DIRECTION('ref_axis',(1.,0.,0.));
#107694=DIRECTION('center_axis',(0.,0.,-1.));
#107695=DIRECTION('ref_axis',(-1.,0.,0.));
#107696=DIRECTION('center_axis',(4.38004274807345E-16,-1.,0.));
#107697=DIRECTION('ref_axis',(0.,0.,-1.));
#107698=DIRECTION('',(-1.87032180698308E-16,-8.19208946723987E-32,-1.));
#107699=DIRECTION('',(0.,0.,1.));
#107700=DIRECTION('center_axis',(0.,0.,-1.));
#107701=DIRECTION('ref_axis',(-1.,0.,0.));
#107702=DIRECTION('center_axis',(0.,7.15121221728469E-32,1.));
#107703=DIRECTION('ref_axis',(-1.,0.,0.));
#107704=DIRECTION('center_axis',(0.,7.15121221728469E-32,1.));
#107705=DIRECTION('ref_axis',(-1.,0.,0.));
#107706=DIRECTION('center_axis',(-2.0158362407235E-32,-1.,0.));
#107707=DIRECTION('ref_axis',(0.,0.,-1.));
#107708=DIRECTION('center_axis',(0.,1.,0.));
#107709=DIRECTION('ref_axis',(0.,0.,-1.));
#107710=DIRECTION('center_axis',(0.,1.,0.));
#107711=DIRECTION('ref_axis',(0.,0.,-1.));
#107712=DIRECTION('',(-2.0158362407235E-32,-1.,-1.23467863058847E-16));
#107713=DIRECTION('center_axis',(-1.41612495910826E-31,1.,0.));
#107714=DIRECTION('ref_axis',(0.,0.,-1.));
#107715=DIRECTION('center_axis',(-2.0158362407235E-32,-1.,0.));
#107716=DIRECTION('ref_axis',(0.,0.,-1.));
#107717=DIRECTION('center_axis',(0.,1.,0.));
#107718=DIRECTION('ref_axis',(0.,0.,-1.));
#107719=DIRECTION('',(-2.0158362407235E-32,-1.,-1.23467863058847E-16));
#107720=DIRECTION('center_axis',(0.,0.,-1.));
#107721=DIRECTION('ref_axis',(-1.,0.,0.));
#107722=DIRECTION('center_axis',(0.,-1.0052202914905E-16,1.));
#107723=DIRECTION('ref_axis',(-1.,0.,0.));
#107724=DIRECTION('center_axis',(0.,0.,-1.));
#107725=DIRECTION('ref_axis',(-1.,0.,0.));
#107726=DIRECTION('',(1.6326809185664E-16,-1.0052202914905E-16,1.));
#107727=DIRECTION('center_axis',(-0.139173100960059,0.990268068741571,1.22266282302934E-16));
#107728=DIRECTION('ref_axis',(8.78519494496445E-16,-5.20658772030138E-33,
1.));
#107729=DIRECTION('',(-3.43088182518023E-33,1.23467863058847E-16,-1.));
#107730=DIRECTION('',(-0.990268068741571,-0.139173100960059,-1.71834053708117E-17));
#107731=DIRECTION('center_axis',(0.,0.,-1.));
#107732=DIRECTION('ref_axis',(0.,1.,0.));
#107733=DIRECTION('',(0.,-1.23467863058847E-16,1.));
#107734=DIRECTION('center_axis',(0.,0.,1.));
#107735=DIRECTION('ref_axis',(0.,1.,0.));
#107736=DIRECTION('center_axis',(0.,0.,-1.));
#107737=DIRECTION('ref_axis',(0.,1.,0.));
#107738=DIRECTION('',(0.,1.23467863058847E-16,-1.));
#107739=DIRECTION('center_axis',(0.,0.,1.));
#107740=DIRECTION('ref_axis',(0.,1.,0.));
#107741=DIRECTION('center_axis',(0.,0.,-1.));
#107742=DIRECTION('ref_axis',(0.,1.,0.));
#107743=DIRECTION('',(3.05149908249585E-33,-1.23467863058847E-16,1.));
#107744=DIRECTION('center_axis',(0.,0.,1.));
#107745=DIRECTION('ref_axis',(0.,1.,0.));
#107746=DIRECTION('center_axis',(-0.99026806874157,0.139173100960067,1.71834053708127E-17));
#107747=DIRECTION('ref_axis',(1.73522765332111E-17,-1.01418524800046E-34,
1.));
#107748=DIRECTION('',(-0.139173100960067,-0.99026806874157,-1.22266282302933E-16));
#107749=DIRECTION('',(-3.05149908249585E-33,1.23467863058847E-16,-1.));
#107750=DIRECTION('',(-0.139173100960067,-0.99026806874157,-1.22266282302933E-16));
#107751=DIRECTION('',(1.73522765332111E-17,6.55191041448207E-33,1.));
#107752=DIRECTION('',(-0.139173100960067,-0.99026806874157,0.));
#107753=DIRECTION('',(-1.73522765332111E-17,-6.55191041448207E-33,-1.));
#107754=DIRECTION('',(-0.139173100960067,-0.99026806874157,-1.22266282302933E-16));
#107755=DIRECTION('',(1.73522765332111E-17,6.93709640335951E-33,1.));
#107756=DIRECTION('',(-0.139173100960067,-0.99026806874157,0.));
#107757=DIRECTION('',(-1.73522765332111E-17,-6.93709640335951E-33,-1.));
#107758=DIRECTION('center_axis',(0.,0.,1.));
#107759=DIRECTION('ref_axis',(0.,-1.,0.));
#107760=DIRECTION('',(0.,1.23467863058847E-16,-1.));
#107761=DIRECTION('',(0.,-1.23467863058847E-16,1.));
#107762=DIRECTION('center_axis',(0.,0.,1.));
#107763=DIRECTION('ref_axis',(0.,-1.,0.));
#107764=DIRECTION('',(0.,1.23467863058847E-16,-1.));
#107765=DIRECTION('center_axis',(-0.907068166518068,-0.420531768759975,
0.0195031472628737));
#107766=DIRECTION('ref_axis',(0.0518039117125095,-0.157474353828549,-0.986163365075769));
#107767=DIRECTION('center_axis',(0.,0.,1.));
#107768=DIRECTION('ref_axis',(-1.,0.,0.));
#107769=DIRECTION('',(0.,1.23467863058847E-16,-1.));
#107770=DIRECTION('center_axis',(1.3159378979443E-30,-2.80509034228723E-44,
1.));
#107771=DIRECTION('ref_axis',(-2.1316282072803E-14,-1.,-5.4762534445178E-59));
#107772=DIRECTION('',(0.,-1.23467863058847E-16,1.));
#107773=DIRECTION('center_axis',(0.,0.,1.));
#107774=DIRECTION('ref_axis',(-1.,-1.77920356510442E-15,0.));
#107775=DIRECTION('center_axis',(-0.966107498808678,-0.25814005491211,0.000113117697403614));
#107776=DIRECTION('ref_axis',(0.25388184709702,-0.950091406535467,0.181301756588465));
#107777=DIRECTION('',(0.,1.23467863058847E-16,-1.));
#107778=DIRECTION('center_axis',(0.,0.,1.));
#107779=DIRECTION('ref_axis',(0.,-1.,0.));
#107780=DIRECTION('',(0.,-1.23467863058847E-16,1.));
#107781=DIRECTION('center_axis',(0.14008961833327,0.00275771348606123,0.990134987691864));
#107782=DIRECTION('ref_axis',(-0.979470506182107,-0.146013776318751,0.13898742621009));
#107783=DIRECTION('',(0.,1.23467863058847E-16,-1.));
#107784=DIRECTION('center_axis',(-6.57968948972152E-31,-7.01272585571806E-45,
1.));
#107785=DIRECTION('ref_axis',(1.06581410364015E-14,-1.,0.));
#107786=DIRECTION('',(0.,-1.23467863058847E-16,1.));
#107787=DIRECTION('center_axis',(0.115800998570926,-7.45156346442165E-10,
0.99327243429483));
#107788=DIRECTION('ref_axis',(-0.993253120969688,-0.00623601609274104,0.115798746915784));
#107789=DIRECTION('',(0.,1.23467863058847E-16,-1.));
#107790=DIRECTION('center_axis',(0.,0.,1.));
#107791=DIRECTION('ref_axis',(0.,-1.,0.));
#107792=DIRECTION('',(0.,-1.23467863058847E-16,1.));
#107793=DIRECTION('center_axis',(0.137684637338237,-0.0024146994890512,
0.990473174733882));
#107794=DIRECTION('ref_axis',(-0.981548350661306,0.133629566375757,0.136769785787277));
#107795=DIRECTION('',(0.,1.23467863058847E-16,-1.));
#107796=DIRECTION('center_axis',(-1.8642453554211E-30,-5.62966047861811E-44,
1.));
#107797=DIRECTION('ref_axis',(3.01980662698043E-14,-1.,-9.95682444457782E-59));
#107798=DIRECTION('',(0.,-1.23467863058847E-16,1.));
#107799=DIRECTION('center_axis',(0.,0.,1.));
#107800=DIRECTION('ref_axis',(-1.,1.13691107810172E-13,0.));
#107801=DIRECTION('',(0.,1.23467863058847E-16,-1.));
#107802=DIRECTION('center_axis',(1.15144566070127E-30,-2.14764729331365E-44,
1.));
#107803=DIRECTION('ref_axis',(-1.86517468137027E-14,-1.,3.73380916671668E-59));
#107804=DIRECTION('',(0.,-1.23467863058847E-16,1.));
#107805=DIRECTION('center_axis',(0.,0.,1.));
#107806=DIRECTION('ref_axis',(-1.,-1.0479508998465E-13,0.));
#107807=DIRECTION('center_axis',(0.,0.,1.));
#107808=DIRECTION('ref_axis',(0.,-1.,0.));
#107809=DIRECTION('',(3.79382742684518E-34,-1.23467863058847E-16,1.));
#107810=DIRECTION('',(0.,-1.23467863058847E-16,1.));
#107811=DIRECTION('center_axis',(-0.99026806874157,-0.139173100960065,-1.71834053708124E-17));
#107812=DIRECTION('ref_axis',(-0.139173100960065,0.99026806874157,2.95927408114303E-34));
#107813=DIRECTION('',(0.139173100960065,-0.99026806874157,-1.22266282302933E-16));
#107814=DIRECTION('',(-1.73522765332109E-17,-6.98077064262961E-33,1.));
#107815=DIRECTION('',(0.139173100960065,-0.99026806874157,-3.85185988877447E-34));
#107816=DIRECTION('',(1.73522765332109E-17,6.98077064262961E-33,-1.));
#107817=DIRECTION('',(0.139173100960065,-0.99026806874157,-1.22266282302933E-16));
#107818=DIRECTION('',(-3.79382742684518E-34,1.23467863058847E-16,-1.));
#107819=DIRECTION('',(0.139173100960065,-0.99026806874157,-1.22266282302933E-16));
#107820=DIRECTION('',(-1.73522765332109E-17,-7.36595663150706E-33,1.));
#107821=DIRECTION('',(0.139173100960065,-0.99026806874157,-3.85185988877447E-34));
#107822=DIRECTION('',(1.73522765332109E-17,6.98077064262961E-33,-1.));
#107823=DIRECTION('center_axis',(0.,0.,-1.));
#107824=DIRECTION('ref_axis',(0.,1.,0.));
#107825=DIRECTION('',(0.,-1.23467863058847E-16,1.));
#107826=DIRECTION('center_axis',(0.,0.,1.));
#107827=DIRECTION('ref_axis',(0.,1.,0.));
#107828=DIRECTION('center_axis',(0.,0.,-1.));
#107829=DIRECTION('ref_axis',(0.,1.,0.));
#107830=DIRECTION('',(0.,1.23467863058847E-16,-1.));
#107831=DIRECTION('center_axis',(0.,0.,1.));
#107832=DIRECTION('ref_axis',(0.,1.,0.));
#107833=DIRECTION('center_axis',(0.,0.,-1.));
#107834=DIRECTION('ref_axis',(0.,1.,0.));
#107835=DIRECTION('',(-3.43088182518023E-33,-1.23467863058847E-16,1.));
#107836=DIRECTION('center_axis',(0.,0.,1.));
#107837=DIRECTION('ref_axis',(0.,1.,0.));
#107838=DIRECTION('center_axis',(-0.139173100960059,-0.990268068741571,
-1.22266282302934E-16));
#107839=DIRECTION('ref_axis',(-0.990268068741571,0.139173100960059,3.29749813286563E-34));
#107840=DIRECTION('',(0.990268068741571,-0.139173100960059,-1.71834053708117E-17));
#107841=DIRECTION('',(0.990268068741571,-0.139173100960059,-1.71834053708117E-17));
#107842=DIRECTION('',(5.85782591378957E-32,-1.23467863058847E-16,1.));
#107843=DIRECTION('',(0.990268068741571,-0.139173100960059,0.));
#107844=DIRECTION('',(-5.85782591378957E-32,1.23467863058847E-16,-1.));
#107845=DIRECTION('',(0.990268068741571,-0.139173100960059,-1.71834053708117E-17));
#107846=DIRECTION('',(1.13659195805196E-16,-1.39441621308911E-16,1.));
#107847=DIRECTION('',(0.990268068741571,-0.139173100960059,0.));
#107848=DIRECTION('',(1.13659195805196E-16,1.07494104808783E-16,-1.));
#107849=DIRECTION('center_axis',(0.,1.,0.));
#107850=DIRECTION('ref_axis',(0.,0.,-1.));
#107851=DIRECTION('center_axis',(-4.38004274807345E-16,1.,0.));
#107852=DIRECTION('ref_axis',(0.,0.,-1.));
#107853=DIRECTION('center_axis',(0.,1.23467863058847E-16,-1.));
#107854=DIRECTION('ref_axis',(-1.,0.,0.));
#107855=DIRECTION('',(-0.139173100960065,0.99026806874157,1.22266282302933E-16));
#107856=DIRECTION('center_axis',(4.28365201153744E-31,1.48619034146585E-45,
-1.));
#107857=DIRECTION('ref_axis',(-3.46944695195361E-15,1.,1.24460305557223E-60));
#107858=DIRECTION('center_axis',(0.,0.,-1.));
#107859=DIRECTION('ref_axis',(0.,1.,0.));
#107860=DIRECTION('center_axis',(0.,0.,-1.));
#107861=DIRECTION('ref_axis',(0.,1.,0.));
#107862=DIRECTION('',(-0.990268068741571,0.139173100960059,1.71834053708117E-17));
#107863=DIRECTION('',(4.38004274807345E-16,-1.,-1.23467863058847E-16));
#107864=DIRECTION('',(1.,4.38004274807345E-16,5.40794518211031E-32));
#107865=DIRECTION('center_axis',(-1.,0.,0.));
#107866=DIRECTION('ref_axis',(0.,0.,1.));
#107867=DIRECTION('center_axis',(-1.,-4.38004274807345E-16,0.));
#107868=DIRECTION('ref_axis',(0.,0.,1.));
#107869=DIRECTION('center_axis',(0.,1.23467863058847E-16,-1.));
#107870=DIRECTION('ref_axis',(-1.,0.,0.));
#107871=DIRECTION('',(4.38004274807345E-16,-1.,-1.23467863058847E-16));
#107872=DIRECTION('center_axis',(0.,0.,-1.));
#107873=DIRECTION('ref_axis',(0.,1.,0.));
#107874=DIRECTION('',(1.,4.38004274807345E-16,5.40794518211031E-32));
#107875=DIRECTION('center_axis',(1.,0.,0.));
#107876=DIRECTION('ref_axis',(0.,0.,-1.));
#107877=DIRECTION('center_axis',(1.,0.,4.33680868994201E-16));
#107878=DIRECTION('ref_axis',(0.,1.,0.));
#107879=DIRECTION('center_axis',(0.,1.23467863058847E-16,-1.));
#107880=DIRECTION('ref_axis',(-1.,0.,0.));
#107881=DIRECTION('',(0.990268068741571,0.139173100960059,1.71834053708117E-17));
#107882=DIRECTION('center_axis',(0.,0.,-1.));
#107883=DIRECTION('ref_axis',(0.,1.,0.));
#107884=DIRECTION('center_axis',(-6.14104352374008E-30,3.05443170604608E-43,
-1.));
#107885=DIRECTION('ref_axis',(4.9737991503207E-14,1.,0.));
#107886=DIRECTION('center_axis',(-4.28365201153744E-31,1.48619034146585E-45,
-1.));
#107887=DIRECTION('ref_axis',(3.46944695195361E-15,1.,1.24460305557223E-60));
#107888=DIRECTION('',(0.139173100960067,0.99026806874157,1.22266282302933E-16));
#107889=DIRECTION('',(-1.,-4.38004274807345E-16,-5.40794518211031E-32));
#107890=DIRECTION('center_axis',(0.,1.23467863058847E-16,-1.));
#107891=DIRECTION('ref_axis',(-1.,0.,0.));
#107892=DIRECTION('',(-1.,-4.38004274807345E-16,-5.40794518211031E-32));
#107893=DIRECTION('center_axis',(0.,-1.,0.));
#107894=DIRECTION('ref_axis',(-1.,0.,0.));
#107895=DIRECTION('center_axis',(0.,-1.,0.));
#107896=DIRECTION('ref_axis',(0.,0.,1.));
#107897=DIRECTION('',(-5.01606788234257E-16,1.,0.));
#107898=DIRECTION('center_axis',(0.,0.452474032063612,0.891777578944491));
#107899=DIRECTION('ref_axis',(0.,0.891777578944491,-0.452474032063612));
#107900=DIRECTION('center_axis',(0.,0.,-1.));
#107901=DIRECTION('ref_axis',(-1.,0.,0.));
#107902=DIRECTION('center_axis',(0.,0.438949247410394,0.898511857572202));
#107903=DIRECTION('ref_axis',(0.,0.898511857572202,-0.438949247410394));
#107904=DIRECTION('center_axis',(0.,-1.,0.));
#107905=DIRECTION('ref_axis',(-1.,0.,0.));
#107906=DIRECTION('',(5.01606788234257E-16,-1.,0.));
#107907=DIRECTION('center_axis',(0.,1.,0.));
#107908=DIRECTION('ref_axis',(0.,0.,-1.));
#107909=DIRECTION('center_axis',(0.,0.,1.));
#107910=DIRECTION('ref_axis',(1.,0.,0.));
#107911=DIRECTION('',(-5.01606788234257E-16,1.,0.));
#107912=DIRECTION('',(1.,5.01606788234257E-16,0.));
#107913=DIRECTION('center_axis',(0.,-1.,0.));
#107914=DIRECTION('ref_axis',(-1.,0.,0.));
#107915=DIRECTION('center_axis',(0.,-1.,0.));
#107916=DIRECTION('ref_axis',(0.,0.,1.));
#107917=DIRECTION('center_axis',(0.,0.434444534286154,0.900698588113075));
#107918=DIRECTION('ref_axis',(0.,0.900698588113075,-0.434444534286154));
#107919=DIRECTION('center_axis',(0.,0.,-1.));
#107920=DIRECTION('ref_axis',(-1.,0.,0.));
#107921=DIRECTION('center_axis',(0.,0.427115883537276,0.904196893397767));
#107922=DIRECTION('ref_axis',(0.,0.904196893397767,-0.427115883537276));
#107923=DIRECTION('center_axis',(0.,0.,-1.));
#107924=DIRECTION('ref_axis',(-1.,0.,0.));
#107925=DIRECTION('center_axis',(0.,0.,1.));
#107926=DIRECTION('ref_axis',(1.,0.,0.));
#107927=DIRECTION('center_axis',(0.,0.425023904828957,0.905182125499585));
#107928=DIRECTION('ref_axis',(0.,0.905182125499585,-0.425023904828957));
#107929=DIRECTION('center_axis',(0.,0.,-1.));
#107930=DIRECTION('ref_axis',(-1.,0.,0.));
#107931=DIRECTION('center_axis',(0.,0.422696564637279,0.906271269678038));
#107932=DIRECTION('ref_axis',(0.,0.906271269678038,-0.422696564637279));
#107933=DIRECTION('center_axis',(0.,0.,1.));
#107934=DIRECTION('ref_axis',(0.,-1.,0.));
#107935=DIRECTION('center_axis',(0.,0.,1.));
#107936=DIRECTION('ref_axis',(1.,0.,0.));
#107937=DIRECTION('center_axis',(0.,-4.38538094726937E-12,1.));
#107938=DIRECTION('ref_axis',(0.,1.,4.38538094726937E-12));
#107939=DIRECTION('center_axis',(-0.939797023107103,0.132079858078289,-0.315176881209658));
#107940=DIRECTION('ref_axis',(-0.317962525883615,-4.30796627806664E-16,
0.948103281364278));
#107941=DIRECTION('center_axis',(0.,-1.,0.));
#107942=DIRECTION('ref_axis',(-1.,0.,0.));
#107943=DIRECTION('',(5.01606788234257E-16,-1.,0.));
#107944=DIRECTION('center_axis',(0.,1.,0.));
#107945=DIRECTION('ref_axis',(0.,0.,-1.));
#107946=DIRECTION('center_axis',(0.,0.,1.));
#107947=DIRECTION('ref_axis',(1.,0.,0.));
#107948=DIRECTION('',(1.,5.01606788234257E-16,0.));
#107949=DIRECTION('center_axis',(0.,-0.422768104239746,0.906237899250264));
#107950=DIRECTION('ref_axis',(0.,0.906237899250264,0.422768104239746));
#107951=DIRECTION('center_axis',(0.,0.422768104239797,0.90623789925024));
#107952=DIRECTION('ref_axis',(0.,0.90623789925024,-0.422768104239797));
#107953=DIRECTION('center_axis',(0.,0.,1.));
#107954=DIRECTION('ref_axis',(1.,0.,0.));
#107955=DIRECTION('center_axis',(-0.999980556584797,-0.00245118997350333,
-0.0057339445474203));
#107956=DIRECTION('ref_axis',(-0.00114511081840959,0.976049495468532,-0.217545561013868));
#107957=DIRECTION('center_axis',(0.,0.,1.));
#107958=DIRECTION('ref_axis',(-1.,0.,0.));
#107959=DIRECTION('center_axis',(0.,0.,1.));
#107960=DIRECTION('ref_axis',(1.,0.,0.));
#107961=DIRECTION('',(0.,0.,-1.));
#107962=DIRECTION('center_axis',(-0.99998055646326,-0.00245129305198786,
0.00573392167742329));
#107963=DIRECTION('ref_axis',(0.00115277299597243,-0.976316950640099,-0.216342050945344));
#107964=DIRECTION('center_axis',(5.9276100702047E-15,-0.42712932005395,
0.904190546262374));
#107965=DIRECTION('ref_axis',(-3.36279389150844E-29,0.904190546262374,0.42712932005395));
#107966=DIRECTION('center_axis',(0.,0.,1.));
#107967=DIRECTION('ref_axis',(1.,0.,0.));
#107968=DIRECTION('center_axis',(0.,0.,-1.));
#107969=DIRECTION('ref_axis',(1.,0.,0.));
#107970=DIRECTION('center_axis',(0.,0.,1.));
#107971=DIRECTION('ref_axis',(1.,0.,0.));
#107972=DIRECTION('',(0.,0.,1.));
#107973=DIRECTION('center_axis',(-5.01926581554439E-14,0.427129320053956,
0.904190546262371));
#107974=DIRECTION('ref_axis',(3.44539770291064E-30,0.904190546262371,-0.427129320053956));
#107975=DIRECTION('center_axis',(2.85977186515575E-47,0.,-1.));
#107976=DIRECTION('ref_axis',(0.,1.,0.));
#107977=DIRECTION('',(2.85977186515575E-47,-5.70122241611331E-32,-1.));
#107978=DIRECTION('center_axis',(5.01606788234257E-16,-1.,5.70122241611331E-32));
#107979=DIRECTION('ref_axis',(-4.59816715307009E-64,-5.70122241611331E-32,
-1.));
#107980=DIRECTION('',(-2.85977186515575E-47,5.70122241611331E-32,1.));
#107981=DIRECTION('center_axis',(-2.85977186515575E-47,0.,1.));
#107982=DIRECTION('ref_axis',(0.,-1.,0.));
#107983=DIRECTION('center_axis',(0.,-0.430903547306764,0.902397990311618));
#107984=DIRECTION('ref_axis',(0.,0.902397990311618,0.430903547306764));
#107985=DIRECTION('center_axis',(0.,0.430903547308298,0.902397990310886));
#107986=DIRECTION('ref_axis',(0.,0.902397990310886,-0.430903547308298));
#107987=DIRECTION('center_axis',(0.,0.,1.));
#107988=DIRECTION('ref_axis',(1.,0.,0.));
#107989=DIRECTION('center_axis',(0.,0.,1.));
#107990=DIRECTION('ref_axis',(-1.,0.,0.));
#107991=DIRECTION('center_axis',(0.,0.,1.));
#107992=DIRECTION('ref_axis',(1.,0.,0.));
#107993=DIRECTION('',(0.,0.,-1.));
#107994=DIRECTION('center_axis',(3.10313574260842E-14,-0.443150313610309,
0.896447321122153));
#107995=DIRECTION('ref_axis',(1.13003852554043E-30,0.896447321122153,0.443150313610309));
#107996=DIRECTION('center_axis',(0.,0.,1.));
#107997=DIRECTION('ref_axis',(1.,0.,0.));
#107998=DIRECTION('center_axis',(0.,0.,-1.));
#107999=DIRECTION('ref_axis',(1.,0.,0.));
#108000=DIRECTION('center_axis',(0.,0.,1.));
#108001=DIRECTION('ref_axis',(1.,0.,0.));
#108002=DIRECTION('',(0.,0.,1.));
#108003=DIRECTION('center_axis',(6.14994601925012E-15,0.443150313610303,
0.896447321122156));
#108004=DIRECTION('ref_axis',(3.80752501607971E-29,0.896447321122156,-0.443150313610303));
#108005=DIRECTION('center_axis',(-1.,-5.01606788234257E-16,0.));
#108006=DIRECTION('ref_axis',(0.,1.,0.));
#108007=DIRECTION('center_axis',(0.,0.,1.));
#108008=DIRECTION('ref_axis',(1.,0.,0.));
#108009=DIRECTION('center_axis',(1.,0.,0.));
#108010=DIRECTION('ref_axis',(0.,1.,0.));
#108011=DIRECTION('center_axis',(2.85977186515575E-47,0.,-1.));
#108012=DIRECTION('ref_axis',(0.,1.,0.));
#108013=DIRECTION('center_axis',(0.,0.,1.));
#108014=DIRECTION('ref_axis',(1.,0.,0.));
#108015=DIRECTION('',(2.85977186515575E-47,-5.70122241611331E-32,-1.));
#108016=DIRECTION('center_axis',(-1.,-5.01606788234257E-16,0.));
#108017=DIRECTION('ref_axis',(0.,1.,0.));
#108018=DIRECTION('center_axis',(1.,0.,0.));
#108019=DIRECTION('ref_axis',(0.,1.,0.));
#108020=DIRECTION('center_axis',(-1.,-5.01606788234257E-16,0.));
#108021=DIRECTION('ref_axis',(-5.01606788234257E-16,1.,0.));
#108022=DIRECTION('center_axis',(-1.,0.,0.));
#108023=DIRECTION('ref_axis',(0.,-1.,0.));
#108024=DIRECTION('',(1.,5.01606788234257E-16,0.));
#108025=DIRECTION('center_axis',(1.,5.01606788234257E-16,0.));
#108026=DIRECTION('ref_axis',(0.,-1.,0.));
#108027=DIRECTION('center_axis',(0.,0.,-1.));
#108028=DIRECTION('ref_axis',(-1.,0.,0.));
#108029=DIRECTION('center_axis',(0.,-0.450013465461336,0.893021769557427));
#108030=DIRECTION('ref_axis',(0.,0.893021769557427,0.450013465461336));
#108031=DIRECTION('center_axis',(0.,0.450013465459867,0.893021769558168));
#108032=DIRECTION('ref_axis',(0.,0.893021769558168,-0.450013465459867));
#108033=DIRECTION('center_axis',(0.,0.,1.));
#108034=DIRECTION('ref_axis',(1.,0.,0.));
#108035=DIRECTION('center_axis',(0.,0.,1.));
#108036=DIRECTION('ref_axis',(-1.,0.,0.));
#108037=DIRECTION('center_axis',(0.,0.,1.));
#108038=DIRECTION('ref_axis',(1.,0.,0.));
#108039=DIRECTION('',(0.,0.,-1.));
#108040=DIRECTION('center_axis',(-2.85977186515575E-47,0.,1.));
#108041=DIRECTION('ref_axis',(0.,-1.,0.));
#108042=DIRECTION('center_axis',(0.,0.,-1.));
#108043=DIRECTION('ref_axis',(-1.,0.,0.));
#108044=DIRECTION('',(-2.85977186515575E-47,5.70122241611331E-32,1.));
#108045=DIRECTION('center_axis',(1.,5.01606788234257E-16,0.));
#108046=DIRECTION('ref_axis',(0.,-1.,0.));
#108047=DIRECTION('center_axis',(-1.,0.,0.));
#108048=DIRECTION('ref_axis',(0.,-1.,0.));
#108049=DIRECTION('center_axis',(6.4968286789753E-15,-0.468145843483567,
0.883651214693365));
#108050=DIRECTION('ref_axis',(8.06613026210763E-31,0.883651214693365,0.468145843483567));
#108051=DIRECTION('center_axis',(0.,0.,1.));
#108052=DIRECTION('ref_axis',(1.,0.,0.));
#108053=DIRECTION('center_axis',(0.,0.,-1.));
#108054=DIRECTION('ref_axis',(1.,0.,0.));
#108055=DIRECTION('center_axis',(0.,0.,1.));
#108056=DIRECTION('ref_axis',(1.,0.,0.));
#108057=DIRECTION('',(0.,0.,1.));
#108058=DIRECTION('center_axis',(6.4968286789756E-15,0.468145843483589,
0.883651214693354));
#108059=DIRECTION('ref_axis',(-1.16233255777344E-30,0.883651214693354,-0.468145843483589));
#108060=DIRECTION('center_axis',(-1.,-5.01606788234257E-16,0.));
#108061=DIRECTION('ref_axis',(0.,1.,0.));
#108062=DIRECTION('center_axis',(0.,0.,1.));
#108063=DIRECTION('ref_axis',(1.,0.,0.));
#108064=DIRECTION('center_axis',(1.,0.,0.));
#108065=DIRECTION('ref_axis',(0.,1.,0.));
#108066=DIRECTION('center_axis',(2.85977186515575E-47,0.,-1.));
#108067=DIRECTION('ref_axis',(0.,1.,0.));
#108068=DIRECTION('center_axis',(0.,0.,1.));
#108069=DIRECTION('ref_axis',(1.,0.,0.));
#108070=DIRECTION('',(2.85977186515575E-47,-5.70122241611331E-32,-1.));
#108071=DIRECTION('center_axis',(-1.,-5.01606788234257E-16,0.));
#108072=DIRECTION('ref_axis',(0.,1.,0.));
#108073=DIRECTION('center_axis',(0.,-1.18842113532926E-16,1.));
#108074=DIRECTION('ref_axis',(0.,1.,1.18842113532926E-16));
#108075=DIRECTION('center_axis',(0.,-0.450823097219337,-0.892613317743783));
#108076=DIRECTION('ref_axis',(0.,-0.892613317743783,0.450823097219337));
#108077=DIRECTION('center_axis',(-1.22429528305785E-14,-0.470879150309884,
-0.882197724891332));
#108078=DIRECTION('ref_axis',(-1.13789948105108E-30,-0.882197724891332,
0.470879150309884));
#108079=DIRECTION('center_axis',(0.,-0.466134040541469,-0.884714109895668));
#108080=DIRECTION('ref_axis',(0.,-0.884714109895668,0.466134040541469));
#108081=DIRECTION('center_axis',(0.,0.,-1.));
#108082=DIRECTION('ref_axis',(-1.,0.,0.));
#108083=DIRECTION('center_axis',(0.,0.,-1.));
#108084=DIRECTION('ref_axis',(1.,0.,0.));
#108085=DIRECTION('center_axis',(1.,0.,0.));
#108086=DIRECTION('ref_axis',(0.,0.,1.));
#108087=DIRECTION('center_axis',(-1.,0.,0.));
#108088=DIRECTION('ref_axis',(0.,0.,1.));
#108089=DIRECTION('center_axis',(1.,0.,0.));
#108090=DIRECTION('ref_axis',(0.,0.,1.));
#108091=DIRECTION('center_axis',(1.,0.,0.));
#108092=DIRECTION('ref_axis',(0.,0.,-1.));
#108093=DIRECTION('center_axis',(-1.,0.,1.87032180698308E-16));
#108094=DIRECTION('ref_axis',(0.,0.,-1.));
#108095=DIRECTION('center_axis',(0.,8.19208946723988E-32,1.));
#108096=DIRECTION('ref_axis',(-1.,0.,0.));
#108097=DIRECTION('center_axis',(0.,0.,-1.));
#108098=DIRECTION('ref_axis',(-1.,0.,0.));
#108099=DIRECTION('center_axis',(0.,-0.457805146562934,-0.88905255625328));
#108100=DIRECTION('ref_axis',(0.,-0.88905255625328,0.457805146562934));
#108101=DIRECTION('center_axis',(0.,-0.440696042277477,-0.89765639212394));
#108102=DIRECTION('ref_axis',(0.,-0.89765639212394,0.440696042277477));
#108103=DIRECTION('center_axis',(-4.18005656861882E-16,1.,0.));
#108104=DIRECTION('ref_axis',(1.,5.9211894646675E-16,0.));
#108105=DIRECTION('center_axis',(5.78241158658935E-16,-1.,0.));
#108106=DIRECTION('ref_axis',(1.,5.78241158658935E-16,0.));
#108107=DIRECTION('center_axis',(0.,0.,1.));
#108108=DIRECTION('ref_axis',(1.,0.,0.));
#108109=DIRECTION('center_axis',(-4.18005656861881E-16,1.,0.));
#108110=DIRECTION('ref_axis',(1.,4.18005656861881E-16,0.));
#108111=DIRECTION('center_axis',(-5.78241158658935E-16,1.,0.));
#108112=DIRECTION('ref_axis',(-1.,-5.78241158658935E-16,0.));
#108113=DIRECTION('',(4.18005656861881E-16,-1.,0.));
#108114=DIRECTION('center_axis',(4.18005656861882E-16,-1.,0.));
#108115=DIRECTION('ref_axis',(-1.,-5.9211894646675E-16,0.));
#108116=DIRECTION('center_axis',(0.,0.,-1.));
#108117=DIRECTION('ref_axis',(-1.,0.,0.));
#108118=DIRECTION('center_axis',(-4.18005656861882E-16,1.,0.));
#108119=DIRECTION('ref_axis',(1.,0.,0.));
#108120=DIRECTION('center_axis',(0.,-1.,0.));
#108121=DIRECTION('ref_axis',(1.,0.,0.));
#108122=DIRECTION('center_axis',(0.,0.,1.));
#108123=DIRECTION('ref_axis',(1.,0.,0.));
#108124=DIRECTION('center_axis',(-4.18005656861881E-16,1.,0.));
#108125=DIRECTION('ref_axis',(1.,4.18005656861881E-16,0.));
#108126=DIRECTION('center_axis',(0.,1.,0.));
#108127=DIRECTION('ref_axis',(-1.,0.,0.));
#108128=DIRECTION('',(4.18005656861881E-16,-1.,0.));
#108129=DIRECTION('center_axis',(4.18005656861882E-16,-1.,0.));
#108130=DIRECTION('ref_axis',(-1.,0.,0.));
#108131=DIRECTION('center_axis',(0.,0.,-1.));
#108132=DIRECTION('ref_axis',(-1.,0.,0.));
#108133=DIRECTION('center_axis',(-1.,0.,0.));
#108134=DIRECTION('ref_axis',(0.,1.,0.));
#108135=DIRECTION('',(-1.,-4.18005656861881E-16,0.));
#108136=DIRECTION('center_axis',(1.,0.,0.));
#108137=DIRECTION('ref_axis',(0.,0.,-1.));
#108138=DIRECTION('center_axis',(0.,0.,1.));
#108139=DIRECTION('ref_axis',(0.,-1.,0.));
#108140=DIRECTION('center_axis',(0.,0.,-1.));
#108141=DIRECTION('ref_axis',(-1.,0.,0.));
#108142=DIRECTION('center_axis',(0.,0.,-1.));
#108143=DIRECTION('ref_axis',(-1.,0.,0.));
#108144=DIRECTION('center_axis',(-0.452796108559755,-6.28380831479673E-15,
-0.891614089207401));
#108145=DIRECTION('ref_axis',(-0.891614089207401,-8.65475050140857E-31,
0.452796108559755));
#108146=DIRECTION('center_axis',(-0.162781055433294,-0.986662212774382,
7.66497430181043E-5));
#108147=DIRECTION('ref_axis',(0.986085660689183,-0.162688589397824,-0.0341685917609087));
#108148=DIRECTION('center_axis',(-0.473890079491229,-6.57654596740791E-15,
-0.880584006531913));
#108149=DIRECTION('ref_axis',(-0.880584006531913,4.48746122839123E-29,0.473890079491229));
#108150=DIRECTION('center_axis',(0.,0.,-1.));
#108151=DIRECTION('ref_axis',(-1.,0.,0.));
#108152=DIRECTION('center_axis',(0.,0.,1.));
#108153=DIRECTION('ref_axis',(-1.,0.,0.));
#108154=DIRECTION('center_axis',(0.,0.,-1.));
#108155=DIRECTION('ref_axis',(-1.,0.,0.));
#108156=DIRECTION('',(0.,0.,-1.));
#108157=DIRECTION('center_axis',(0.473890079491223,6.57654596740749E-15,
-0.880584006531917));
#108158=DIRECTION('ref_axis',(-0.880584006531917,-2.59399416170326E-30,
-0.473890079491223));
#108159=DIRECTION('center_axis',(0.,0.,1.));
#108160=DIRECTION('ref_axis',(-1.,0.,0.));
#108161=DIRECTION('center_axis',(0.,0.,-1.));
#108162=DIRECTION('ref_axis',(-1.,0.,0.));
#108163=DIRECTION('',(0.,0.,1.));
#108164=DIRECTION('center_axis',(4.18005656861882E-16,-1.,0.));
#108165=DIRECTION('ref_axis',(-1.,0.,0.));
#108166=DIRECTION('center_axis',(0.,1.,0.));
#108167=DIRECTION('ref_axis',(-1.,0.,0.));
#108168=DIRECTION('center_axis',(0.453758938247698,0.,-0.891124472764788));
#108169=DIRECTION('ref_axis',(-0.891124472764788,0.,-0.453758938247698));
#108170=DIRECTION('center_axis',(0.,0.,1.));
#108171=DIRECTION('ref_axis',(1.,0.,0.));
#108172=DIRECTION('center_axis',(0.,0.,-1.));
#108173=DIRECTION('ref_axis',(1.,0.,0.));
#108174=DIRECTION('center_axis',(0.,0.,1.));
#108175=DIRECTION('ref_axis',(1.,0.,0.));
#108176=DIRECTION('',(0.,0.,1.));
#108177=DIRECTION('center_axis',(0.453758938247726,-6.29717026090114E-15,
0.891124472764774));
#108178=DIRECTION('ref_axis',(0.891124472764774,1.97126653384901E-30,-0.453758938247726));
#108179=DIRECTION('center_axis',(0.439171790863778,-6.20608564480709E-14,
0.898403104463415));
#108180=DIRECTION('ref_axis',(0.898403104463415,-1.60954096059593E-29,-0.439171790863778));
#108181=DIRECTION('center_axis',(0.,0.,1.));
#108182=DIRECTION('ref_axis',(1.,0.,0.));
#108183=DIRECTION('center_axis',(0.133735125220376,0.991017062579732,-0.000312982633993186));
#108184=DIRECTION('ref_axis',(0.990180089850999,-0.133635142118712,-0.0410492198900214));
#108185=DIRECTION('center_axis',(0.,0.,1.));
#108186=DIRECTION('ref_axis',(0.,-1.,0.));
#108187=DIRECTION('center_axis',(0.,0.,1.));
#108188=DIRECTION('ref_axis',(1.,0.,0.));
#108189=DIRECTION('center_axis',(-1.,0.,0.));
#108190=DIRECTION('ref_axis',(0.,1.,0.));
#108191=DIRECTION('center_axis',(-1.,0.,0.));
#108192=DIRECTION('ref_axis',(0.,0.,1.));
#108193=DIRECTION('',(1.,4.18005656861881E-16,0.));
#108194=DIRECTION('center_axis',(-4.18005656861882E-16,1.,0.));
#108195=DIRECTION('ref_axis',(1.,0.,0.));
#108196=DIRECTION('center_axis',(0.,0.,1.));
#108197=DIRECTION('ref_axis',(1.,0.,0.));
#108198=DIRECTION('center_axis',(0.,-1.,0.));
#108199=DIRECTION('ref_axis',(1.,0.,0.));
#108200=DIRECTION('center_axis',(0.,0.,-1.));
#108201=DIRECTION('ref_axis',(1.,0.,0.));
#108202=DIRECTION('center_axis',(0.,0.,1.));
#108203=DIRECTION('ref_axis',(1.,0.,0.));
#108204=DIRECTION('',(0.,0.,-1.));
#108205=DIRECTION('center_axis',(-4.18005656861882E-16,1.,0.));
#108206=DIRECTION('ref_axis',(1.,0.,0.));
#108207=DIRECTION('center_axis',(0.,-1.,0.));
#108208=DIRECTION('ref_axis',(1.,0.,0.));
#108209=DIRECTION('center_axis',(-4.18005656861881E-16,1.,0.));
#108210=DIRECTION('ref_axis',(1.,4.18005656861881E-16,0.));
#108211=DIRECTION('center_axis',(0.,1.,0.));
#108212=DIRECTION('ref_axis',(-1.,0.,0.));
#108213=DIRECTION('',(4.18005656861881E-16,-1.,0.));
#108214=DIRECTION('center_axis',(4.18005656861882E-16,-1.,0.));
#108215=DIRECTION('ref_axis',(-1.,0.,0.));
#108216=DIRECTION('center_axis',(0.,0.,-1.));
#108217=DIRECTION('ref_axis',(-1.,0.,0.));
#108218=DIRECTION('center_axis',(-0.446066534667472,0.,0.894999802597606));
#108219=DIRECTION('ref_axis',(0.894999802597606,0.,0.446066534667472));
#108220=DIRECTION('center_axis',(0.,0.,1.));
#108221=DIRECTION('ref_axis',(-1.,0.,0.));
#108222=DIRECTION('center_axis',(0.,0.,-1.));
#108223=DIRECTION('ref_axis',(-1.,0.,0.));
#108224=DIRECTION('',(0.,0.,1.));
#108225=DIRECTION('center_axis',(4.18005656861882E-16,-1.,0.));
#108226=DIRECTION('ref_axis',(-1.,0.,0.));
#108227=DIRECTION('center_axis',(1.,0.,0.));
#108228=DIRECTION('ref_axis',(0.,0.,-1.));
#108229=DIRECTION('center_axis',(0.,1.,0.));
#108230=DIRECTION('ref_axis',(-1.,0.,0.));
#108231=DIRECTION('center_axis',(0.,0.,1.));
#108232=DIRECTION('ref_axis',(0.,-1.,0.));
#108233=DIRECTION('center_axis',(0.,0.,-1.));
#108234=DIRECTION('ref_axis',(-1.,0.,0.));
#108235=DIRECTION('center_axis',(0.,0.,-1.));
#108236=DIRECTION('ref_axis',(-1.,0.,0.));
#108237=DIRECTION('center_axis',(-0.434629636675507,0.,-0.90060928205483));
#108238=DIRECTION('ref_axis',(-0.90060928205483,0.,0.434629636675507));
#108239=DIRECTION('center_axis',(-0.116944233518957,-0.993138481232708,
5.78053165623419E-5));
#108240=DIRECTION('ref_axis',(0.983258715661079,-0.115789058593805,-0.140695387225332));
#108241=DIRECTION('center_axis',(-0.446066534667672,4.96824693939355E-14,
-0.894999802597506));
#108242=DIRECTION('ref_axis',(-0.894999802597506,-9.63397512853712E-30,
0.446066534667672));
#108243=DIRECTION('center_axis',(0.,0.,1.));
#108244=DIRECTION('ref_axis',(1.,0.,0.));
#108245=DIRECTION('center_axis',(0.,0.,1.));
#108246=DIRECTION('ref_axis',(-1.,0.,0.));
#108247=DIRECTION('center_axis',(0.,0.,1.));
#108248=DIRECTION('ref_axis',(1.,0.,0.));
#108249=DIRECTION('',(0.,0.,-1.));
#108250=DIRECTION('center_axis',(-0.432211889750627,1.54100116546287E-13,
0.901772078941343));
#108251=DIRECTION('ref_axis',(0.901772078941343,9.67025840811756E-28,0.432211889750627));
#108252=DIRECTION('center_axis',(0.,0.,1.));
#108253=DIRECTION('ref_axis',(1.,0.,0.));
#108254=DIRECTION('center_axis',(0.,0.,-1.));
#108255=DIRECTION('ref_axis',(1.,0.,0.));
#108256=DIRECTION('center_axis',(0.,0.,1.));
#108257=DIRECTION('ref_axis',(1.,0.,0.));
#108258=DIRECTION('',(0.,0.,1.));
#108259=DIRECTION('center_axis',(0.432211889750627,-1.1996289787948E-14,
0.901772078941343));
#108260=DIRECTION('ref_axis',(0.901772078941343,7.55282579686682E-29,-0.432211889750627));
#108261=DIRECTION('center_axis',(0.42722596110711,0.,0.904144887811741));
#108262=DIRECTION('ref_axis',(0.904144887811741,0.,-0.42722596110711));
#108263=DIRECTION('center_axis',(0.,0.,1.));
#108264=DIRECTION('ref_axis',(1.,0.,0.));
#108265=DIRECTION('center_axis',(0.0775715986932,0.996986754706871,-0.000240863536308724));
#108266=DIRECTION('ref_axis',(0.995376869740143,-0.0774600592983714,-0.0567875549729645));
#108267=DIRECTION('center_axis',(0.,0.,1.));
#108268=DIRECTION('ref_axis',(0.,-1.,0.));
#108269=DIRECTION('center_axis',(0.,0.,1.));
#108270=DIRECTION('ref_axis',(1.,0.,0.));
#108271=DIRECTION('center_axis',(0.,0.,1.));
#108272=DIRECTION('ref_axis',(1.,0.,0.));
#108273=DIRECTION('center_axis',(0.,0.,-1.));
#108274=DIRECTION('ref_axis',(1.,0.,0.));
#108275=DIRECTION('',(0.,0.,-1.));
#108276=DIRECTION('center_axis',(-1.,-4.18005656861882E-16,0.));
#108277=DIRECTION('ref_axis',(-4.18005656861882E-16,1.,0.));
#108278=DIRECTION('',(0.,0.,1.));
#108279=DIRECTION('center_axis',(0.,0.,1.));
#108280=DIRECTION('ref_axis',(-1.,0.,0.));
#108281=DIRECTION('center_axis',(0.,0.,-1.));
#108282=DIRECTION('ref_axis',(-1.,0.,0.));
#108283=DIRECTION('center_axis',(-0.427895220819097,0.,0.903828346534991));
#108284=DIRECTION('ref_axis',(0.903828346534991,0.,0.427895220819097));
#108285=DIRECTION('center_axis',(0.,0.,1.));
#108286=DIRECTION('ref_axis',(0.,-1.,0.));
#108287=DIRECTION('center_axis',(0.,0.,1.));
#108288=DIRECTION('ref_axis',(1.,0.,0.));
#108289=DIRECTION('center_axis',(0.,0.,1.));
#108290=DIRECTION('ref_axis',(1.,0.,0.));
#108291=DIRECTION('center_axis',(0.425103688199478,0.,0.905144659310986));
#108292=DIRECTION('ref_axis',(0.905144659310986,0.,-0.425103688199478));
#108293=DIRECTION('center_axis',(-0.0572816986700422,-0.998358055091024,
2.88503434636003E-5));
#108294=DIRECTION('ref_axis',(0.977894907203397,-0.0561134278004395,-0.20142699343967));
#108295=DIRECTION('center_axis',(0.427895220819092,0.,0.903828346534994));
#108296=DIRECTION('ref_axis',(0.903828346534994,0.,-0.427895220819092));
#108297=DIRECTION('center_axis',(0.,0.,1.));
#108298=DIRECTION('ref_axis',(1.,0.,0.));
#108299=DIRECTION('center_axis',(0.,0.,1.));
#108300=DIRECTION('ref_axis',(-1.,0.,0.));
#108301=DIRECTION('center_axis',(0.,0.,1.));
#108302=DIRECTION('ref_axis',(1.,0.,0.));
#108303=DIRECTION('',(0.,0.,-1.));
#108304=DIRECTION('center_axis',(-0.00301258321928094,-0.999973601321737,
0.00661218587031605));
#108305=DIRECTION('ref_axis',(0.976036390081241,-0.00150160440505745,0.217602183861723));
#108306=DIRECTION('center_axis',(-0.422820321921619,0.,0.906213537401698));
#108307=DIRECTION('ref_axis',(0.906213537401698,0.,0.422820321921619));
#108308=DIRECTION('center_axis',(0.,0.,1.));
#108309=DIRECTION('ref_axis',(1.,0.,0.));
#108310=DIRECTION('center_axis',(0.,0.,-1.));
#108311=DIRECTION('ref_axis',(1.,0.,0.));
#108312=DIRECTION('center_axis',(0.,0.,1.));
#108313=DIRECTION('ref_axis',(1.,0.,0.));
#108314=DIRECTION('',(0.,0.,1.));
#108315=DIRECTION('center_axis',(0.422820321921648,-5.86781070846046E-15,
0.906213537401685));
#108316=DIRECTION('ref_axis',(0.906213537401684,-2.1653413854129E-31,-0.422820321921648));
#108317=DIRECTION('center_axis',(-0.00301263259095615,-0.999973601245449,
-0.0066121749130267));
#108318=DIRECTION('ref_axis',(0.976304654845778,-0.00151044331358758,-0.216395331482594));
#108319=DIRECTION('center_axis',(0.422711298276089,-5.8662977014411E-15,
0.906264397573767));
#108320=DIRECTION('ref_axis',(0.906264397573767,-1.10286040862995E-31,-0.422711298276089));
#108321=DIRECTION('center_axis',(0.,0.,1.));
#108322=DIRECTION('ref_axis',(1.,0.,0.));
#108323=DIRECTION('center_axis',(0.0114473717304193,0.999934475947494,-3.86273995495549E-5));
#108324=DIRECTION('ref_axis',(-0.906145684596772,0.0103900004240839,0.422838085060741));
#108325=DIRECTION('center_axis',(0.,0.,1.));
#108326=DIRECTION('ref_axis',(0.,-1.,0.));
#108327=DIRECTION('center_axis',(8.20654853338604E-14,-3.5527136788005E-12,
1.));
#108328=DIRECTION('ref_axis',(1.83670992315982E-40,1.,3.5527136788005E-12));
#108329=DIRECTION('center_axis',(0.,5.55111512312578E-14,1.));
#108330=DIRECTION('ref_axis',(0.,1.,-5.55111512312578E-14));
#108331=DIRECTION('center_axis',(0.,0.,-1.));
#108332=DIRECTION('ref_axis',(1.,0.,0.));
#108333=DIRECTION('',(0.,0.,-1.));
#108334=DIRECTION('center_axis',(-1.,-4.18005656861882E-16,0.));
#108335=DIRECTION('ref_axis',(-4.18005656861882E-16,1.,0.));
#108336=DIRECTION('',(0.,0.,1.));
#108337=DIRECTION('center_axis',(1.,0.,0.));
#108338=DIRECTION('ref_axis',(0.,0.00139138517159681,-0.999999032023184));
#108339=DIRECTION('center_axis',(0.,0.,1.));
#108340=DIRECTION('ref_axis',(-1.,0.,0.));
#108341=DIRECTION('center_axis',(4.44089209850062E-13,0.,1.));
#108342=DIRECTION('ref_axis',(1.,0.,-4.44089209850062E-13));
#108343=DIRECTION('center_axis',(-0.422759120858735,0.,0.906242090023824));
#108344=DIRECTION('ref_axis',(0.906242090023824,0.,0.422759120858735));
#108345=DIRECTION('center_axis',(0.,0.,1.));
#108346=DIRECTION('ref_axis',(0.,-1.,0.));
#108347=DIRECTION('center_axis',(0.,0.,1.));
#108348=DIRECTION('ref_axis',(1.,0.,0.));
#108349=DIRECTION('center_axis',(0.,0.,1.));
#108350=DIRECTION('ref_axis',(1.,0.,0.));
#108351=DIRECTION('center_axis',(0.422683101271474,0.,0.906277549043078));
#108352=DIRECTION('ref_axis',(0.906277549043078,0.,-0.422683101271474));
#108353=DIRECTION('center_axis',(0.00955294373602,-0.999954369112247,-3.0972651916074E-5));
#108354=DIRECTION('ref_axis',(-0.99995436957652,-0.0095529439031991,5.25421246130079E-6));
#108355=DIRECTION('center_axis',(0.422759120858763,0.,0.906242090023811));
#108356=DIRECTION('ref_axis',(0.906242090023811,0.,-0.422759120858763));
#108357=DIRECTION('center_axis',(0.,0.,1.));
#108358=DIRECTION('ref_axis',(1.,0.,0.));
#108359=DIRECTION('center_axis',(-0.00252660201784237,0.999981531120523,
-0.0055275401488527));
#108360=DIRECTION('ref_axis',(0.976075629574813,0.00126433814704904,-0.217427612779938));
#108361=DIRECTION('center_axis',(0.,0.,1.));
#108362=DIRECTION('ref_axis',(-1.,0.,0.));
#108363=DIRECTION('center_axis',(0.,0.,1.));
#108364=DIRECTION('ref_axis',(1.,0.,0.));
#108365=DIRECTION('',(0.,0.,-1.));
#108366=DIRECTION('center_axis',(-0.00252663505004111,0.999981531077572,
0.0055275328202581));
#108367=DIRECTION('ref_axis',(0.976342845954299,0.00127169757905682,0.21622448968405));
#108368=DIRECTION('center_axis',(-0.427566573571512,0.,0.903983863331817));
#108369=DIRECTION('ref_axis',(0.903983863331817,0.,0.427566573571512));
#108370=DIRECTION('center_axis',(0.,0.,1.));
#108371=DIRECTION('ref_axis',(1.,0.,0.));
#108372=DIRECTION('center_axis',(0.,0.,-1.));
#108373=DIRECTION('ref_axis',(1.,0.,0.));
#108374=DIRECTION('center_axis',(0.,0.,1.));
#108375=DIRECTION('ref_axis',(1.,0.,0.));
#108376=DIRECTION('',(0.,0.,1.));
#108377=DIRECTION('center_axis',(0.427566573571518,4.42475067662884E-14,
0.903983863331814));
#108378=DIRECTION('ref_axis',(0.903983863331814,-2.72495173441675E-28,-0.427566573571518));
#108379=DIRECTION('center_axis',(0.424945455576639,5.89730286238743E-15,
0.905218956819157));
#108380=DIRECTION('ref_axis',(0.905218956819157,3.24660130849529E-29,-0.424945455576639));
#108381=DIRECTION('center_axis',(0.,0.,1.));
#108382=DIRECTION('ref_axis',(1.,0.,0.));
#108383=DIRECTION('center_axis',(-0.0554974440951108,0.998458828862227,
2.76763464500059E-5));
#108384=DIRECTION('ref_axis',(0.978043885168222,0.0543682946724248,-0.201182124502805));
#108385=DIRECTION('center_axis',(0.,0.,1.));
#108386=DIRECTION('ref_axis',(0.,-1.,0.));
#108387=DIRECTION('center_axis',(3.85729088923276E-14,3.33066907387548E-13,
1.));
#108388=DIRECTION('ref_axis',(-1.00445073922803E-41,1.,-3.33066907387547E-13));
#108389=DIRECTION('center_axis',(0.,0.,1.));
#108390=DIRECTION('ref_axis',(1.,0.,0.));
#108391=DIRECTION('center_axis',(0.,0.,-1.));
#108392=DIRECTION('ref_axis',(1.,0.,0.));
#108393=DIRECTION('',(0.,0.,-1.));
#108394=DIRECTION('center_axis',(-1.,-4.18005656861882E-16,0.));
#108395=DIRECTION('ref_axis',(-4.18005656861882E-16,1.,0.));
#108396=DIRECTION('',(0.,0.,1.));
#108397=DIRECTION('center_axis',(0.,0.,1.));
#108398=DIRECTION('ref_axis',(-1.,0.,0.));
#108399=DIRECTION('center_axis',(0.,0.,1.));
#108400=DIRECTION('ref_axis',(1.,0.,0.));
#108401=DIRECTION('center_axis',(-0.431774610811204,0.,0.901981532770396));
#108402=DIRECTION('ref_axis',(0.901981532770396,0.,0.431774610811205));
#108403=DIRECTION('center_axis',(0.,0.,1.));
#108404=DIRECTION('ref_axis',(0.,-1.,0.));
#108405=DIRECTION('center_axis',(0.,0.,1.));
#108406=DIRECTION('ref_axis',(1.,0.,0.));
#108407=DIRECTION('center_axis',(0.,0.,1.));
#108408=DIRECTION('ref_axis',(1.,0.,0.));
#108409=DIRECTION('center_axis',(0.427007199080172,0.,0.904248224733511));
#108410=DIRECTION('ref_axis',(0.904248224733511,0.,-0.427007199080172));
#108411=DIRECTION('center_axis',(0.0757974280411721,-0.997123211513648,
-0.000225749977414995));
#108412=DIRECTION('ref_axis',(0.995635758500845,0.0756967156000945,-0.054584280171167));
#108413=DIRECTION('center_axis',(0.43177461081284,0.,0.901981532769613));
#108414=DIRECTION('ref_axis',(0.901981532769613,0.,-0.43177461081284));
#108415=DIRECTION('center_axis',(0.,0.,1.));
#108416=DIRECTION('ref_axis',(1.,0.,0.));
#108417=DIRECTION('center_axis',(0.,0.,1.));
#108418=DIRECTION('ref_axis',(-1.,0.,0.));
#108419=DIRECTION('center_axis',(0.,0.,1.));
#108420=DIRECTION('ref_axis',(1.,0.,0.));
#108421=DIRECTION('',(0.,0.,-1.));
#108422=DIRECTION('center_axis',(0.44541715199073,0.,-0.895323159933031));
#108423=DIRECTION('ref_axis',(-0.895323159933031,0.,-0.44541715199073));
#108424=DIRECTION('center_axis',(0.,0.,1.));
#108425=DIRECTION('ref_axis',(1.,0.,0.));
#108426=DIRECTION('center_axis',(0.,0.,-1.));
#108427=DIRECTION('ref_axis',(1.,0.,0.));
#108428=DIRECTION('center_axis',(0.,0.,1.));
#108429=DIRECTION('ref_axis',(1.,0.,0.));
#108430=DIRECTION('',(0.,0.,1.));
#108431=DIRECTION('center_axis',(0.445417151990703,0.,0.895323159933044));
#108432=DIRECTION('ref_axis',(0.895323159933044,0.,-0.445417151990703));
#108433=DIRECTION('center_axis',(0.434261044064412,6.0265826227258E-15,
0.90078707007155));
#108434=DIRECTION('ref_axis',(0.90078707007155,1.10802520916158E-30,-0.434261044064412));
#108435=DIRECTION('center_axis',(0.,0.,1.));
#108436=DIRECTION('ref_axis',(1.,0.,0.));
#108437=DIRECTION('center_axis',(-0.115453898308443,0.993312838018061,5.65145097326706E-5));
#108438=DIRECTION('ref_axis',(0.983295509889155,0.114297632119478,-0.141654479363368));
#108439=DIRECTION('center_axis',(0.,0.,1.));
#108440=DIRECTION('ref_axis',(0.,-1.,0.));
#108441=DIRECTION('center_axis',(0.,0.,1.));
#108442=DIRECTION('ref_axis',(1.,0.,0.));
#108443=DIRECTION('center_axis',(-4.18005656861882E-16,1.,0.));
#108444=DIRECTION('ref_axis',(1.,2.96059473233375E-16,0.));
#108445=DIRECTION('center_axis',(0.,0.,1.));
#108446=DIRECTION('ref_axis',(1.,0.,0.));
#108447=DIRECTION('center_axis',(4.33680868994202E-16,-1.,0.));
#108448=DIRECTION('ref_axis',(1.,4.33680868994202E-16,0.));
#108449=DIRECTION('center_axis',(-1.,0.,0.));
#108450=DIRECTION('ref_axis',(0.,0.,1.));
#108451=DIRECTION('center_axis',(0.,0.,-1.));
#108452=DIRECTION('ref_axis',(1.,0.,0.));
#108453=DIRECTION('center_axis',(0.,0.,1.));
#108454=DIRECTION('ref_axis',(1.,0.,0.));
#108455=DIRECTION('',(0.,0.,-1.));
#108456=DIRECTION('center_axis',(-4.18005656861882E-16,1.,0.));
#108457=DIRECTION('ref_axis',(1.,2.96059473233375E-16,0.));
#108458=DIRECTION('center_axis',(4.33680868994202E-16,-1.,0.));
#108459=DIRECTION('ref_axis',(1.,4.33680868994202E-16,0.));
#108460=DIRECTION('center_axis',(-4.18005656861881E-16,1.,0.));
#108461=DIRECTION('ref_axis',(1.,4.18005656861881E-16,0.));
#108462=DIRECTION('center_axis',(-4.33680868994202E-16,1.,0.));
#108463=DIRECTION('ref_axis',(-1.,-4.33680868994202E-16,0.));
#108464=DIRECTION('',(4.18005656861881E-16,-1.,0.));
#108465=DIRECTION('center_axis',(4.18005656861882E-16,-1.,0.));
#108466=DIRECTION('ref_axis',(-1.,-2.96059473233375E-16,0.));
#108467=DIRECTION('center_axis',(0.,0.,-1.));
#108468=DIRECTION('ref_axis',(-1.,0.,0.));
#108469=DIRECTION('center_axis',(-0.453032377894844,0.,0.891494063120413));
#108470=DIRECTION('ref_axis',(0.891494063120413,0.,0.453032377894844));
#108471=DIRECTION('center_axis',(0.,0.,1.));
#108472=DIRECTION('ref_axis',(-1.,0.,0.));
#108473=DIRECTION('center_axis',(0.,0.,-1.));
#108474=DIRECTION('ref_axis',(-1.,0.,0.));
#108475=DIRECTION('',(0.,0.,1.));
#108476=DIRECTION('center_axis',(4.18005656861882E-16,-1.,0.));
#108477=DIRECTION('ref_axis',(-1.,-2.96059473233375E-16,0.));
#108478=DIRECTION('center_axis',(1.,0.,0.));
#108479=DIRECTION('ref_axis',(0.,0.,-1.));
#108480=DIRECTION('center_axis',(-4.33680868994202E-16,1.,0.));
#108481=DIRECTION('ref_axis',(-1.,-4.33680868994202E-16,0.));
#108482=DIRECTION('center_axis',(-1.,0.,0.));
#108483=DIRECTION('ref_axis',(0.,1.,0.));
#108484=DIRECTION('',(-1.,-4.18005656861881E-16,0.));
#108485=DIRECTION('center_axis',(0.,0.,1.));
#108486=DIRECTION('ref_axis',(0.,-1.,0.));
#108487=DIRECTION('center_axis',(0.,0.,-1.));
#108488=DIRECTION('ref_axis',(-1.,0.,0.));
#108489=DIRECTION('center_axis',(0.,0.,-1.));
#108490=DIRECTION('ref_axis',(-1.,0.,0.));
#108491=DIRECTION('center_axis',(-0.438728460697982,-6.08858048281589E-15,
-0.898619684724066));
#108492=DIRECTION('ref_axis',(-0.898619684724066,-1.57717257184587E-30,
0.438728460697982));
#108493=DIRECTION('center_axis',(0.132298166463164,-0.991209921788581,-0.000293425222152531));
#108494=DIRECTION('ref_axis',(0.990461456417794,0.132209758351032,-0.0388160166362208));
#108495=DIRECTION('center_axis',(-0.45303237789485,-6.28708721049444E-15,
-0.89149406312041));
#108496=DIRECTION('ref_axis',(-0.89149406312041,3.90721898735751E-30,0.45303237789485));
#108497=DIRECTION('center_axis',(0.,0.,1.));
#108498=DIRECTION('ref_axis',(1.,0.,0.));
#108499=DIRECTION('center_axis',(0.,0.,1.));
#108500=DIRECTION('ref_axis',(-1.,0.,0.));
#108501=DIRECTION('center_axis',(0.,0.,1.));
#108502=DIRECTION('ref_axis',(1.,0.,0.));
#108503=DIRECTION('',(0.,0.,-1.));
#108504=DIRECTION('center_axis',(0.473027330271434,0.,-0.881047753993096));
#108505=DIRECTION('ref_axis',(-0.881047753993096,0.,-0.473027330271434));
#108506=DIRECTION('center_axis',(-0.452154194923616,0.,-0.891939787212666));
#108507=DIRECTION('ref_axis',(-0.891939787212666,0.,0.452154194923616));
#108508=DIRECTION('center_axis',(0.,0.,-1.));
#108509=DIRECTION('ref_axis',(-1.,0.,0.));
#108510=DIRECTION('center_axis',(-0.16174361462519,0.986832811286145,7.54788824122006E-5));
#108511=DIRECTION('ref_axis',(0.98621116070404,0.16164443851147,-0.0354770630281384));
#108512=DIRECTION('center_axis',(0.,0.,1.));
#108513=DIRECTION('ref_axis',(0.,-1.,0.));
#108514=DIRECTION('center_axis',(0.,0.,-1.));
#108515=DIRECTION('ref_axis',(-1.,0.,0.));
#108516=DIRECTION('center_axis',(-1.,0.,0.));
#108517=DIRECTION('ref_axis',(0.,1.,0.));
#108518=DIRECTION('center_axis',(-1.,0.,0.));
#108519=DIRECTION('ref_axis',(0.,0.,1.));
#108520=DIRECTION('',(1.,4.18005656861881E-16,0.));
#108521=DIRECTION('center_axis',(-4.18005656861882E-16,1.,0.));
#108522=DIRECTION('ref_axis',(1.,5.9211894646675E-16,0.));
#108523=DIRECTION('center_axis',(0.,0.,1.));
#108524=DIRECTION('ref_axis',(1.,0.,0.));
#108525=DIRECTION('center_axis',(5.78241158658935E-16,-1.,0.));
#108526=DIRECTION('ref_axis',(1.,5.78241158658935E-16,0.));
#108527=DIRECTION('center_axis',(0.,0.,-1.));
#108528=DIRECTION('ref_axis',(1.,0.,0.));
#108529=DIRECTION('',(0.,0.,-1.));
#108530=DIRECTION('center_axis',(0.,0.,-1.));
#108531=DIRECTION('ref_axis',(-1.,0.,0.));
#108532=DIRECTION('center_axis',(0.,0.,-1.));
#108533=DIRECTION('ref_axis',(1.,0.,0.));
#108534=DIRECTION('center_axis',(0.,0.,-1.));
#108535=DIRECTION('ref_axis',(-1.,0.,0.));
#108536=DIRECTION('',(0.,0.,1.));
#108537=DIRECTION('center_axis',(-0.473027330271494,0.,-0.881047753993064));
#108538=DIRECTION('ref_axis',(-0.881047753993064,0.,0.473027330271494));
#108539=DIRECTION('center_axis',(-0.744016723942684,0.668160994441905,0.));
#108540=DIRECTION('ref_axis',(-0.668160994441905,-0.744016723942684,0.));
#108541=DIRECTION('center_axis',(0.,-1.,-1.23467863058847E-16));
#108542=DIRECTION('ref_axis',(-1.,0.,0.));
#108543=DIRECTION('center_axis',(0.,-1.,0.));
#108544=DIRECTION('ref_axis',(0.,0.,1.));
#108545=DIRECTION('center_axis',(0.,-1.,-1.23467863058847E-16));
#108546=DIRECTION('ref_axis',(-1.,0.,0.));
#108547=DIRECTION('center_axis',(0.,-1.,0.));
#108548=DIRECTION('ref_axis',(0.,0.,1.));
#108549=DIRECTION('center_axis',(0.,1.23467863058847E-16,-1.));
#108550=DIRECTION('ref_axis',(0.,1.,1.1837531408762E-16));
#108551=DIRECTION('center_axis',(0.,-1.19392659184112E-16,1.));
#108552=DIRECTION('ref_axis',(0.,1.,1.19392659184112E-16));
#108553=DIRECTION('center_axis',(0.,-1.,0.));
#108554=DIRECTION('ref_axis',(0.,0.,1.));
#108555=DIRECTION('center_axis',(0.,0.,-1.));
#108556=DIRECTION('ref_axis',(-1.,0.,0.));
#108557=DIRECTION('center_axis',(0.,0.,-1.));
#108558=DIRECTION('ref_axis',(-1.,0.,0.));
#108559=DIRECTION('center_axis',(-1.13659195805196E-16,0.,-1.));
#108560=DIRECTION('ref_axis',(0.,1.,0.));
#108561=DIRECTION('center_axis',(0.,0.,-1.));
#108562=DIRECTION('ref_axis',(-1.,0.,0.));
#108563=DIRECTION('center_axis',(0.,-1.,0.));
#108564=DIRECTION('ref_axis',(-1.,0.,0.));
#108565=DIRECTION('center_axis',(0.,-1.,0.));
#108566=DIRECTION('ref_axis',(0.,0.,1.));
#108567=DIRECTION('',(-5.01606788234257E-16,1.,0.));
#108568=DIRECTION('center_axis',(-1.,-5.01606788234257E-16,1.13659195805196E-16));
#108569=DIRECTION('ref_axis',(0.,1.,0.));
#108570=DIRECTION('center_axis',(0.,0.,1.));
#108571=DIRECTION('ref_axis',(1.,0.,0.));
#108572=DIRECTION('center_axis',(1.,0.,-1.13659195805196E-16));
#108573=DIRECTION('ref_axis',(0.,1.,0.));
#108574=DIRECTION('center_axis',(0.,-1.14024448322266E-31,-1.));
#108575=DIRECTION('ref_axis',(1.,0.,0.));
#108576=DIRECTION('center_axis',(0.,0.,1.));
#108577=DIRECTION('ref_axis',(1.,0.,0.));
#108578=DIRECTION('',(-1.13659195805196E-16,-1.14024448322266E-31,-1.));
#108579=DIRECTION('center_axis',(-1.,-5.01606788234257E-16,1.13659195805196E-16));
#108580=DIRECTION('ref_axis',(0.,1.,0.));
#108581=DIRECTION('center_axis',(1.,0.,-1.13659195805196E-16));
#108582=DIRECTION('ref_axis',(0.,1.,0.));
#108583=DIRECTION('center_axis',(-6.24334907322839E-14,-0.457979853752065,
0.888962571516505));
#108584=DIRECTION('ref_axis',(-1.27562203883084E-29,0.888962571516505,0.457979853752065));
#108585=DIRECTION('center_axis',(0.,0.,1.));
#108586=DIRECTION('ref_axis',(1.,0.,0.));
#108587=DIRECTION('center_axis',(0.,-4.9783213633841E-32,-1.));
#108588=DIRECTION('ref_axis',(1.,0.,0.));
#108589=DIRECTION('center_axis',(0.,1.11022302462516E-13,-1.));
#108590=DIRECTION('ref_axis',(0.,-1.,-1.11022302462516E-13));
#108591=DIRECTION('',(1.13659195805196E-16,4.9783213633841E-32,1.));
#108592=DIRECTION('center_axis',(0.,-0.489712654585584,-0.871883889023499));
#108593=DIRECTION('ref_axis',(0.,-0.871883889023499,0.489712654585584));
#108594=DIRECTION('center_axis',(0.,-0.973635916817664,-0.228107653274998));
#108595=DIRECTION('ref_axis',(0.,-0.228107653274998,0.973635916817664));
#108596=DIRECTION('center_axis',(0.,-1.,0.));
#108597=DIRECTION('ref_axis',(0.,0.,1.));
#108598=DIRECTION('center_axis',(0.952431113365324,-0.30470794606498,-0.00529546018307552));
#108599=DIRECTION('ref_axis',(0.0463072011468755,0.161873964053018,-0.985724334123747));
#108600=DIRECTION('center_axis',(0.,1.,1.23467863058847E-16));
#108601=DIRECTION('ref_axis',(1.,0.,0.));
#108602=DIRECTION('',(-5.01606788234257E-16,1.,1.23467863058847E-16));
#108603=DIRECTION('center_axis',(-1.,-5.01606788234257E-16,0.));
#108604=DIRECTION('ref_axis',(-5.01606788234257E-16,1.,0.));
#108605=DIRECTION('',(1.,5.01606788234257E-16,0.));
#108606=DIRECTION('center_axis',(-1.,0.,-1.13659195805196E-16));
#108607=DIRECTION('ref_axis',(0.,-1.,0.));
#108608=DIRECTION('center_axis',(1.,4.38004274807345E-16,1.13659195805196E-16));
#108609=DIRECTION('ref_axis',(0.,-1.,0.));
#108610=DIRECTION('center_axis',(0.,0.,1.));
#108611=DIRECTION('ref_axis',(1.,0.,0.));
#108612=DIRECTION('center_axis',(0.,-1.,-1.23467863058847E-16));
#108613=DIRECTION('ref_axis',(-1.,0.,0.));
#108614=DIRECTION('center_axis',(0.,1.,0.));
#108615=DIRECTION('ref_axis',(0.,0.,-1.));
#108616=DIRECTION('center_axis',(0.,4.9783213633841E-32,-1.));
#108617=DIRECTION('ref_axis',(1.,0.,0.));
#108618=DIRECTION('center_axis',(0.,0.,-1.));
#108619=DIRECTION('ref_axis',(0.,1.,0.));
#108620=DIRECTION('center_axis',(0.,0.,1.));
#108621=DIRECTION('ref_axis',(0.,1.,0.));
#108622=DIRECTION('center_axis',(0.,1.,1.23467863058847E-16));
#108623=DIRECTION('ref_axis',(1.,0.,0.));
#108624=DIRECTION('center_axis',(-4.38004274807345E-16,1.,0.));
#108625=DIRECTION('ref_axis',(0.,0.,-1.));
#108626=DIRECTION('',(-4.38004274807345E-16,1.,1.23467863058847E-16));
#108627=DIRECTION('center_axis',(0.,1.,0.));
#108628=DIRECTION('ref_axis',(0.,0.,-1.));
#108629=DIRECTION('center_axis',(1.13659195805195E-16,0.,-1.));
#108630=DIRECTION('ref_axis',(1.,0.,1.13659195805195E-16));
#108631=DIRECTION('center_axis',(0.,0.,1.));
#108632=DIRECTION('ref_axis',(1.,0.,0.));
#108633=DIRECTION('',(-1.13659195805196E-16,0.,1.));
#108634=DIRECTION('center_axis',(1.,4.38004274807345E-16,1.13659195805196E-16));
#108635=DIRECTION('ref_axis',(0.,-1.,0.));
#108636=DIRECTION('center_axis',(0.,-1.,0.));
#108637=DIRECTION('ref_axis',(0.,0.,1.));
#108638=DIRECTION('center_axis',(-1.,0.,-1.13659195805196E-16));
#108639=DIRECTION('ref_axis',(0.,-1.,0.));
#108640=DIRECTION('center_axis',(0.,1.,0.));
#108641=DIRECTION('ref_axis',(1.,0.,0.));
#108642=DIRECTION('',(4.38004274807345E-16,-1.,0.));
#108643=DIRECTION('center_axis',(0.,1.07494104808783E-16,-1.));
#108644=DIRECTION('ref_axis',(1.,0.,0.));
#108645=DIRECTION('center_axis',(0.,0.,1.));
#108646=DIRECTION('ref_axis',(1.,0.,0.));
#108647=DIRECTION('center_axis',(0.,0.,1.));
#108648=DIRECTION('ref_axis',(1.,0.,0.));
#108649=DIRECTION('center_axis',(0.,1.,0.));
#108650=DIRECTION('ref_axis',(0.,0.,-1.));
#108651=DIRECTION('center_axis',(0.,-1.,-1.23467863058847E-16));
#108652=DIRECTION('ref_axis',(-1.,0.,0.));
#108653=DIRECTION('center_axis',(0.,-0.460605100635463,0.887605171947863));
#108654=DIRECTION('ref_axis',(0.,0.887605171947863,0.460605100635463));
#108655=DIRECTION('center_axis',(0.,0.635616055211064,0.772005330524295));
#108656=DIRECTION('ref_axis',(0.,0.772005330524295,-0.635616055211064));
#108657=DIRECTION('center_axis',(0.,0.46043947842117,0.887691098700016));
#108658=DIRECTION('ref_axis',(0.,0.887691098700016,-0.46043947842117));
#108659=DIRECTION('center_axis',(-0.976945182380867,0.213489703311671,0.000507151563339024));
#108660=DIRECTION('ref_axis',(0.169470879268944,0.776952017533326,-0.606321023493912));
#108661=DIRECTION('center_axis',(0.,0.477110018651024,0.878843575446063));
#108662=DIRECTION('ref_axis',(0.,0.878843575446063,-0.477110018651024));
#108663=DIRECTION('center_axis',(0.,0.,1.));
#108664=DIRECTION('ref_axis',(1.,0.,0.));
#108665=DIRECTION('center_axis',(0.,0.,1.));
#108666=DIRECTION('ref_axis',(-1.,0.,0.));
#108667=DIRECTION('center_axis',(0.,0.,1.));
#108668=DIRECTION('ref_axis',(1.,0.,0.));
#108669=DIRECTION('',(0.,0.,-1.));
#108670=DIRECTION('center_axis',(0.,-0.477110018651003,0.878843575446074));
#108671=DIRECTION('ref_axis',(0.,0.878843575446074,0.477110018651003));
#108672=DIRECTION('center_axis',(-2.85977186515575E-47,0.,1.));
#108673=DIRECTION('ref_axis',(0.,-1.,0.));
#108674=DIRECTION('center_axis',(0.,0.,-1.));
#108675=DIRECTION('ref_axis',(-1.,0.,0.));
#108676=DIRECTION('',(-2.85977186515575E-47,5.70122241611331E-32,1.));
#108677=DIRECTION('center_axis',(1.,5.01606788234257E-16,0.));
#108678=DIRECTION('ref_axis',(0.,-1.,0.));
#108679=DIRECTION('center_axis',(-1.,0.,0.));
#108680=DIRECTION('ref_axis',(0.,-1.,0.));
#108681=DIRECTION('center_axis',(0.,-1.18842113532926E-16,1.));
#108682=DIRECTION('ref_axis',(0.,1.,1.18842113532926E-16));
#108683=DIRECTION('center_axis',(1.88564486786379E-14,-0.483290003559882,
0.875460320322451));
#108684=DIRECTION('ref_axis',(-3.50034193199929E-30,0.875460320322451,0.483290003559882));
#108685=DIRECTION('center_axis',(0.,-1.,0.));
#108686=DIRECTION('ref_axis',(0.,0.,1.));
#108687=DIRECTION('center_axis',(0.,1.,1.23467863058847E-16));
#108688=DIRECTION('ref_axis',(1.,0.,0.));
#108689=DIRECTION('center_axis',(0.,-0.498898715136559,0.866660297945562));
#108690=DIRECTION('ref_axis',(0.,0.866660297945562,0.498898715136559));
#108691=DIRECTION('center_axis',(-1.60982338570647E-12,0.,1.));
#108692=DIRECTION('ref_axis',(1.,0.,1.60982338570648E-12));
#108693=DIRECTION('center_axis',(0.,0.,-1.));
#108694=DIRECTION('ref_axis',(1.,0.,0.));
#108695=DIRECTION('center_axis',(0.,0.,1.));
#108696=DIRECTION('ref_axis',(1.,0.,0.));
#108697=DIRECTION('',(0.,0.,1.));
#108698=DIRECTION('center_axis',(6.92361050625672E-15,0.498898715136586,
0.866660297945547));
#108699=DIRECTION('ref_axis',(-2.25138771964303E-30,0.866660297945547,-0.498898715136586));
#108700=DIRECTION('center_axis',(6.20126212581678E-14,0.483005416470283,
0.875617363727084));
#108701=DIRECTION('ref_axis',(-9.99028424960391E-30,0.875617363727084,-0.483005416470283));
#108702=DIRECTION('center_axis',(0.,1.,0.));
#108703=DIRECTION('ref_axis',(0.,0.,-1.));
#108704=DIRECTION('center_axis',(0.,-1.,-1.23467863058847E-16));
#108705=DIRECTION('ref_axis',(-1.,0.,0.));
#108706=DIRECTION('center_axis',(0.,1.,0.));
#108707=DIRECTION('ref_axis',(0.,0.,-1.));
#108708=DIRECTION('',(-5.01606788234257E-16,1.,1.23467863058847E-16));
#108709=DIRECTION('center_axis',(0.,0.,1.));
#108710=DIRECTION('ref_axis',(1.,0.,0.));
#108711=DIRECTION('center_axis',(6.19323182390956E-32,0.,1.));
#108712=DIRECTION('ref_axis',(-0.656059028990495,0.754709580222783,4.06312565670714E-32));
#108713=DIRECTION('center_axis',(0.,0.,1.));
#108714=DIRECTION('ref_axis',(1.,0.,0.));
#108715=DIRECTION('center_axis',(0.,-1.,0.));
#108716=DIRECTION('ref_axis',(-1.,0.,0.));
#108717=DIRECTION('center_axis',(0.,-1.,0.));
#108718=DIRECTION('ref_axis',(0.,0.,1.));
#108719=DIRECTION('',(-5.01606788234257E-16,1.,0.));
#108720=DIRECTION('center_axis',(-1.,-5.01606788234257E-16,0.));
#108721=DIRECTION('ref_axis',(0.,1.,0.));
#108722=DIRECTION('center_axis',(0.,0.,1.));
#108723=DIRECTION('ref_axis',(1.,0.,0.));
#108724=DIRECTION('center_axis',(1.,0.,0.));
#108725=DIRECTION('ref_axis',(0.,1.,0.));
#108726=DIRECTION('center_axis',(2.85977186515575E-47,0.,-1.));
#108727=DIRECTION('ref_axis',(0.,1.,0.));
#108728=DIRECTION('center_axis',(0.,0.,1.));
#108729=DIRECTION('ref_axis',(1.,0.,0.));
#108730=DIRECTION('',(2.85977186515575E-47,-5.70122241611331E-32,-1.));
#108731=DIRECTION('center_axis',(-1.,-5.01606788234257E-16,0.));
#108732=DIRECTION('ref_axis',(0.,1.,0.));
#108733=DIRECTION('center_axis',(1.,0.,0.));
#108734=DIRECTION('ref_axis',(0.,1.,0.));
#108735=DIRECTION('center_axis',(-1.,-5.01606788234257E-16,0.));
#108736=DIRECTION('ref_axis',(-5.01606788234257E-16,1.,0.));
#108737=DIRECTION('center_axis',(-1.,0.,0.));
#108738=DIRECTION('ref_axis',(0.,-1.,0.));
#108739=DIRECTION('',(1.,5.01606788234257E-16,0.));
#108740=DIRECTION('center_axis',(1.,5.01606788234257E-16,0.));
#108741=DIRECTION('ref_axis',(0.,-1.,0.));
#108742=DIRECTION('center_axis',(0.,0.,-1.));
#108743=DIRECTION('ref_axis',(-1.,0.,0.));
#108744=DIRECTION('center_axis',(0.,-1.,0.));
#108745=DIRECTION('ref_axis',(-1.,0.,0.));
#108746=DIRECTION('',(5.01606788234257E-16,-1.,0.));
#108747=DIRECTION('center_axis',(0.,1.,0.));
#108748=DIRECTION('ref_axis',(0.,0.,-1.));
#108749=DIRECTION('center_axis',(-6.19323182390956E-32,0.,-1.));
#108750=DIRECTION('ref_axis',(0.,1.,0.));
#108751=DIRECTION('center_axis',(0.,0.,1.));
#108752=DIRECTION('ref_axis',(1.,0.,0.));
#108753=DIRECTION('center_axis',(0.,0.,1.));
#108754=DIRECTION('ref_axis',(1.,0.,0.));
#108755=DIRECTION('center_axis',(0.,1.,0.));
#108756=DIRECTION('ref_axis',(0.,0.,-1.));
#108757=DIRECTION('center_axis',(0.,1.,1.23467863058847E-16));
#108758=DIRECTION('ref_axis',(1.,0.,0.));
#108759=DIRECTION('center_axis',(0.,1.,0.));
#108760=DIRECTION('ref_axis',(0.,0.,-1.));
#108761=DIRECTION('',(5.01606788234257E-16,-1.,-1.23467863058847E-16));
#108762=DIRECTION('center_axis',(0.,0.495757141593727,0.86846120037617));
#108763=DIRECTION('ref_axis',(0.,0.86846120037617,-0.495757141593727));
#108764=DIRECTION('center_axis',(0.,0.509034676478003,0.860746012562902));
#108765=DIRECTION('ref_axis',(0.,0.860746012562902,-0.509034676478003));
#108766=DIRECTION('center_axis',(0.,0.,1.));
#108767=DIRECTION('ref_axis',(1.,0.,0.));
#108768=DIRECTION('center_axis',(0.,0.,1.));
#108769=DIRECTION('ref_axis',(-1.,0.,0.));
#108770=DIRECTION('center_axis',(0.,-1.9151347174784E-12,1.));
#108771=DIRECTION('ref_axis',(0.,1.,1.9151347174784E-12));
#108772=DIRECTION('',(0.,0.,-1.));
#108773=DIRECTION('center_axis',(0.,-0.509034676477531,0.860746012563181));
#108774=DIRECTION('ref_axis',(0.,0.860746012563181,0.509034676477531));
#108775=DIRECTION('center_axis',(0.,-0.496115977596257,0.868256262156346));
#108776=DIRECTION('ref_axis',(0.,0.868256262156346,0.496115977596257));
#108777=DIRECTION('center_axis',(-2.85977186515575E-47,0.,1.));
#108778=DIRECTION('ref_axis',(0.,-1.,0.));
#108779=DIRECTION('center_axis',(0.,0.,-1.));
#108780=DIRECTION('ref_axis',(-1.,0.,0.));
#108781=DIRECTION('',(-2.85977186515575E-47,5.70122241611331E-32,1.));
#108782=DIRECTION('center_axis',(1.,5.01606788234257E-16,0.));
#108783=DIRECTION('ref_axis',(0.,-1.,0.));
#108784=DIRECTION('center_axis',(-1.,0.,0.));
#108785=DIRECTION('ref_axis',(0.,-1.,0.));
#108786=DIRECTION('center_axis',(0.,1.23467863058847E-16,-1.));
#108787=DIRECTION('ref_axis',(0.,1.,1.1837531408762E-16));
#108788=DIRECTION('center_axis',(0.,-1.19392659184112E-16,1.));
#108789=DIRECTION('ref_axis',(0.,1.,1.19392659184112E-16));
#108790=DIRECTION('center_axis',(0.,-1.,0.));
#108791=DIRECTION('ref_axis',(0.,0.,-1.));
#108792=DIRECTION('center_axis',(0.,-1.,0.));
#108793=DIRECTION('ref_axis',(0.,0.,1.));
#108794=DIRECTION('center_axis',(-2.30924636740563E-32,-1.,0.));
#108795=DIRECTION('ref_axis',(0.,0.,-1.));
#108796=DIRECTION('center_axis',(0.,-1.,0.));
#108797=DIRECTION('ref_axis',(0.,0.,1.));
#108798=DIRECTION('center_axis',(0.,-0.481647286662901,-0.876365158624112));
#108799=DIRECTION('ref_axis',(0.,-0.876365158624112,0.481647286662901));
#108800=DIRECTION('center_axis',(0.,-0.498146280733357,-0.867093007117186));
#108801=DIRECTION('ref_axis',(0.,-0.867093007117186,0.498146280733357));
#108802=DIRECTION('center_axis',(0.,0.,-1.));
#108803=DIRECTION('ref_axis',(-1.,0.,0.));
#108804=DIRECTION('center_axis',(0.,0.,-1.));
#108805=DIRECTION('ref_axis',(1.,0.,0.));
#108806=DIRECTION('center_axis',(1.,0.,0.));
#108807=DIRECTION('ref_axis',(0.,0.,1.));
#108808=DIRECTION('center_axis',(-1.,0.,0.));
#108809=DIRECTION('ref_axis',(0.,0.,1.));
#108810=DIRECTION('center_axis',(1.,0.,0.));
#108811=DIRECTION('ref_axis',(0.,0.,1.));
#108812=DIRECTION('center_axis',(1.,0.,0.));
#108813=DIRECTION('ref_axis',(0.,0.,-1.));
#108814=DIRECTION('center_axis',(-1.,0.,1.87032180698308E-16));
#108815=DIRECTION('ref_axis',(0.,0.,-1.));
#108816=DIRECTION('center_axis',(0.,8.19208946723987E-32,1.));
#108817=DIRECTION('ref_axis',(-1.,0.,0.));
#108818=DIRECTION('center_axis',(0.,0.,-1.));
#108819=DIRECTION('ref_axis',(-1.,0.,0.));
#108820=DIRECTION('center_axis',(0.,-0.488256551855887,-0.872700142987154));
#108821=DIRECTION('ref_axis',(0.,-0.872700142987154,0.488256551855887));
#108822=DIRECTION('center_axis',(0.,0.,1.));
#108823=DIRECTION('ref_axis',(0.,-1.,0.));
#108824=DIRECTION('',(0.,-1.23467863058847E-16,1.));
#108825=DIRECTION('center_axis',(0.,0.,1.));
#108826=DIRECTION('ref_axis',(-1.,0.,0.));
#108827=DIRECTION('center_axis',(0.,0.,1.));
#108828=DIRECTION('ref_axis',(1.,0.,0.));
#108829=DIRECTION('center_axis',(-1.,-4.38004274807345E-16,0.));
#108830=DIRECTION('ref_axis',(0.,1.,0.));
#108831=DIRECTION('center_axis',(-1.,0.,0.));
#108832=DIRECTION('ref_axis',(0.,1.,0.));
#108833=DIRECTION('center_axis',(1.,0.,0.));
#108834=DIRECTION('ref_axis',(0.,0.,1.));
#108835=DIRECTION('center_axis',(1.,0.,0.));
#108836=DIRECTION('ref_axis',(0.,0.,-1.));
#108837=DIRECTION('center_axis',(-1.,0.,1.87032180698308E-16));
#108838=DIRECTION('ref_axis',(0.,0.,-1.));
#108839=DIRECTION('center_axis',(0.,8.19208946723988E-32,1.));
#108840=DIRECTION('ref_axis',(-1.,0.,0.));
#108841=DIRECTION('center_axis',(0.,0.,-1.));
#108842=DIRECTION('ref_axis',(-1.,0.,0.));
#108843=DIRECTION('center_axis',(-1.44372869288582E-12,-0.522894079854115,
-0.852397666147391));
#108844=DIRECTION('ref_axis',(-4.54659658509035E-27,-0.852397666147391,
0.522894079854115));
#108845=DIRECTION('center_axis',(-1.90454958189083E-14,-0.515457402104623,
-0.856915203865326));
#108846=DIRECTION('ref_axis',(-1.04773227122123E-29,-0.856915203865326,
0.515457402104623));
#108847=DIRECTION('center_axis',(0.,1.23467863058847E-16,-1.));
#108848=DIRECTION('ref_axis',(0.,1.,1.1837531408762E-16));
#108849=DIRECTION('center_axis',(0.,-1.19392659184112E-16,1.));
#108850=DIRECTION('ref_axis',(0.,1.,1.19392659184112E-16));
#108851=DIRECTION('center_axis',(-1.,-4.1800565686188E-16,-5.16102651992463E-32));
#108852=DIRECTION('ref_axis',(-4.1800565686188E-16,1.,-8.08534226092968E-63));
#108853=DIRECTION('center_axis',(1.,0.,0.));
#108854=DIRECTION('ref_axis',(0.,0.,-1.));
#108855=DIRECTION('center_axis',(-1.,0.,-5.16102651992463E-32));
#108856=DIRECTION('ref_axis',(0.,1.,0.));
#108857=DIRECTION('center_axis',(-1.,0.,0.));
#108858=DIRECTION('ref_axis',(0.,0.,1.));
#108859=DIRECTION('center_axis',(-1.,0.,0.));
#108860=DIRECTION('ref_axis',(0.,0.,1.));
#108861=DIRECTION('center_axis',(0.,0.,-1.));
#108862=DIRECTION('ref_axis',(-1.,0.,0.));
#108863=DIRECTION('center_axis',(0.,0.,-1.));
#108864=DIRECTION('ref_axis',(-1.,0.,0.));
#108865=DIRECTION('center_axis',(0.,-7.68642463345396E-33,-1.));
#108866=DIRECTION('ref_axis',(1.,0.,0.));
#108867=DIRECTION('center_axis',(0.,0.,-1.));
#108868=DIRECTION('ref_axis',(-1.,0.,0.));
#108869=DIRECTION('center_axis',(-1.,0.,0.));
#108870=DIRECTION('ref_axis',(0.,1.,0.));
#108871=DIRECTION('center_axis',(-1.,0.,0.));
#108872=DIRECTION('ref_axis',(0.,0.,1.));
#108873=DIRECTION('',(1.,4.18005656861881E-16,0.));
#108874=DIRECTION('center_axis',(-4.18005656861882E-16,1.,0.));
#108875=DIRECTION('ref_axis',(1.,0.,0.));
#108876=DIRECTION('center_axis',(0.,0.,1.));
#108877=DIRECTION('ref_axis',(1.,0.,0.));
#108878=DIRECTION('center_axis',(0.,-1.,0.));
#108879=DIRECTION('ref_axis',(1.,0.,0.));
#108880=DIRECTION('center_axis',(0.,0.,-1.));
#108881=DIRECTION('ref_axis',(1.,0.,0.));
#108882=DIRECTION('center_axis',(0.,0.,1.));
#108883=DIRECTION('ref_axis',(1.,0.,0.));
#108884=DIRECTION('',(0.,0.,-1.));
#108885=DIRECTION('center_axis',(-4.18005656861882E-16,1.,0.));
#108886=DIRECTION('ref_axis',(1.,0.,0.));
#108887=DIRECTION('center_axis',(0.,-1.,0.));
#108888=DIRECTION('ref_axis',(1.,0.,0.));
#108889=DIRECTION('center_axis',(0.533061469511947,0.,-0.846076515287928));
#108890=DIRECTION('ref_axis',(-0.846076515287928,0.,-0.533061469511947));
#108891=DIRECTION('center_axis',(0.542737080693052,0.,-0.839902649859366));
#108892=DIRECTION('ref_axis',(-0.839902649859366,0.,-0.542737080693052));
#108893=DIRECTION('center_axis',(-1.11022302462516E-13,0.,-1.));
#108894=DIRECTION('ref_axis',(-1.,0.,1.11022302462516E-13));
#108895=DIRECTION('center_axis',(0.,0.,-1.));
#108896=DIRECTION('ref_axis',(1.,0.,0.));
#108897=DIRECTION('center_axis',(0.,0.,-1.));
#108898=DIRECTION('ref_axis',(-1.,0.,0.));
#108899=DIRECTION('',(0.,0.,1.));
#108900=DIRECTION('center_axis',(-0.542737080693356,0.,-0.839902649859169));
#108901=DIRECTION('ref_axis',(-0.839902649859169,0.,0.542737080693356));
#108902=DIRECTION('center_axis',(-0.532459169918176,0.,-0.846455688367706));
#108903=DIRECTION('ref_axis',(-0.846455688367706,0.,0.532459169918176));
#108904=DIRECTION('center_axis',(-1.,0.,0.));
#108905=DIRECTION('ref_axis',(0.,0.,1.));
#108906=DIRECTION('center_axis',(1.,0.,5.16102651992463E-32));
#108907=DIRECTION('ref_axis',(0.,-1.,0.));
#108908=DIRECTION('',(1.,4.18005656861881E-16,5.16102651992463E-32));
#108909=DIRECTION('center_axis',(-4.18005656861881E-16,1.,0.));
#108910=DIRECTION('ref_axis',(1.,4.18005656861881E-16,0.));
#108911=DIRECTION('',(4.18005656861881E-16,-1.,0.));
#108912=DIRECTION('center_axis',(0.,1.,0.));
#108913=DIRECTION('ref_axis',(-1.,0.,0.));
#108914=DIRECTION('center_axis',(4.38004274807345E-16,-1.,0.));
#108915=DIRECTION('ref_axis',(-1.,0.,0.));
#108916=DIRECTION('center_axis',(0.,0.,-1.));
#108917=DIRECTION('ref_axis',(-1.,0.,0.));
#108918=DIRECTION('center_axis',(0.,0.,1.));
#108919=DIRECTION('ref_axis',(0.,-1.,0.));
#108920=DIRECTION('',(0.,1.23467863058847E-16,-1.));
#108921=DIRECTION('center_axis',(0.,0.,-1.));
#108922=DIRECTION('ref_axis',(1.,0.,0.));
#108923=DIRECTION('center_axis',(0.,0.,-1.));
#108924=DIRECTION('ref_axis',(-1.,0.,0.));
#108925=DIRECTION('',(0.,0.,1.));
#108926=DIRECTION('center_axis',(4.38004274807345E-16,-1.,0.));
#108927=DIRECTION('ref_axis',(-1.,0.,0.));
#108928=DIRECTION('center_axis',(1.,0.,0.));
#108929=DIRECTION('ref_axis',(0.,0.,-1.));
#108930=DIRECTION('center_axis',(0.,1.,0.));
#108931=DIRECTION('ref_axis',(-1.,0.,0.));
#108932=DIRECTION('center_axis',(1.,0.,0.));
#108933=DIRECTION('ref_axis',(0.,-1.,0.));
#108934=DIRECTION('',(-1.,-4.38004274807345E-16,0.));
#108935=DIRECTION('center_axis',(0.,-7.60037129918566E-33,-1.));
#108936=DIRECTION('ref_axis',(1.,0.,0.));
#108937=DIRECTION('center_axis',(0.,0.,1.));
#108938=DIRECTION('ref_axis',(1.,0.,0.));
#108939=DIRECTION('center_axis',(0.,0.,1.));
#108940=DIRECTION('ref_axis',(1.,0.,0.));
#108941=DIRECTION('center_axis',(1.,0.,0.));
#108942=DIRECTION('ref_axis',(0.,0.,-1.));
#108943=DIRECTION('center_axis',(-1.,0.,-5.40794518211031E-32));
#108944=DIRECTION('ref_axis',(0.,1.,0.));
#108945=DIRECTION('center_axis',(-1.,0.,-5.40794518211031E-32));
#108946=DIRECTION('ref_axis',(0.,1.,0.));
#108947=DIRECTION('center_axis',(-1.,0.,-5.40794518211031E-32));
#108948=DIRECTION('ref_axis',(0.,1.,0.));
#108949=DIRECTION('center_axis',(-1.,0.,0.));
#108950=DIRECTION('ref_axis',(0.,1.,0.));
#108951=DIRECTION('',(-1.,-4.18005656861881E-16,0.));
#108952=DIRECTION('center_axis',(1.,0.,0.));
#108953=DIRECTION('ref_axis',(0.,0.,-1.));
#108954=DIRECTION('center_axis',(0.,0.,1.));
#108955=DIRECTION('ref_axis',(0.,-1.,0.));
#108956=DIRECTION('center_axis',(0.,0.,-1.));
#108957=DIRECTION('ref_axis',(-1.,0.,0.));
#108958=DIRECTION('center_axis',(0.,0.,-1.));
#108959=DIRECTION('ref_axis',(-1.,0.,0.));
#108960=DIRECTION('center_axis',(-0.639652375806928,0.,-0.768664320834884));
#108961=DIRECTION('ref_axis',(-0.768664320834884,0.,0.639652375806928));
#108962=DIRECTION('center_axis',(-0.460063868749635,-6.3846687485495E-15,
-0.887885824118799));
#108963=DIRECTION('ref_axis',(-0.887885824118799,1.45303619130616E-30,0.460063868749635));
#108964=DIRECTION('center_axis',(0.212606354611556,0.977137797844532,0.000511861626231249));
#108965=DIRECTION('ref_axis',(0.773811164394419,-0.168046480235339,-0.610718152947059));
#108966=DIRECTION('center_axis',(-0.482846004727867,-1.73271215008562E-12,
-0.875705279028473));
#108967=DIRECTION('ref_axis',(-0.875705279028473,2.53817490248555E-28,0.482846004727867));
#108968=DIRECTION('center_axis',(0.,0.,-1.));
#108969=DIRECTION('ref_axis',(-1.,0.,0.));
#108970=DIRECTION('center_axis',(0.,0.,1.));
#108971=DIRECTION('ref_axis',(-1.,0.,0.));
#108972=DIRECTION('center_axis',(0.,0.,-1.));
#108973=DIRECTION('ref_axis',(-1.,0.,0.));
#108974=DIRECTION('',(0.,0.,-1.));
#108975=DIRECTION('center_axis',(0.482846004726866,0.,-0.875705279029025));
#108976=DIRECTION('ref_axis',(-0.875705279029025,0.,-0.482846004726866));
#108977=DIRECTION('center_axis',(0.460227641765603,-1.23207131288176E-14,
-0.887800944894108));
#108978=DIRECTION('ref_axis',(-0.887800944894108,7.43200893707752E-29,-0.460227641765603));
#108979=DIRECTION('center_axis',(0.782801330915055,-1.71942202750291E-12,
-0.622271706184379));
#108980=DIRECTION('ref_axis',(-0.622271706184379,-5.64324648533862E-28,
-0.782801330915055));
#108981=DIRECTION('center_axis',(0.,0.,1.));
#108982=DIRECTION('ref_axis',(-1.,0.,0.));
#108983=DIRECTION('center_axis',(0.,0.,-1.));
#108984=DIRECTION('ref_axis',(-1.,0.,0.));
#108985=DIRECTION('',(0.,0.,1.));
#108986=DIRECTION('center_axis',(4.18005656861882E-16,-1.,0.));
#108987=DIRECTION('ref_axis',(-1.,-5.9211894646675E-16,0.));
#108988=DIRECTION('center_axis',(-5.78241158658935E-16,1.,0.));
#108989=DIRECTION('ref_axis',(-1.,-5.78241158658935E-16,0.));
#108990=DIRECTION('center_axis',(0.,-1.18842113532926E-16,1.));
#108991=DIRECTION('ref_axis',(0.,1.,1.18842113532926E-16));
#108992=DIRECTION('center_axis',(-0.482758140724685,-1.88531393333386E-14,
0.875753719697522));
#108993=DIRECTION('ref_axis',(0.875753719697522,-7.73315028487173E-30,0.482758140724685));
#108994=DIRECTION('center_axis',(-1.,0.,0.));
#108995=DIRECTION('ref_axis',(0.,0.,1.));
#108996=DIRECTION('center_axis',(1.,0.,5.16102651992463E-32));
#108997=DIRECTION('ref_axis',(0.,-1.,0.));
#108998=DIRECTION('center_axis',(-0.506538210354814,0.,0.862217514001277));
#108999=DIRECTION('ref_axis',(0.862217514001277,0.,0.506538210354814));
#109000=DIRECTION('center_axis',(0.,1.77635683940025E-12,1.));
#109001=DIRECTION('ref_axis',(0.,1.,-1.77635683940025E-12));
#109002=DIRECTION('center_axis',(0.,0.,-1.));
#109003=DIRECTION('ref_axis',(1.,0.,0.));
#109004=DIRECTION('center_axis',(0.,0.,1.));
#109005=DIRECTION('ref_axis',(1.,0.,0.));
#109006=DIRECTION('',(0.,0.,1.));
#109007=DIRECTION('center_axis',(0.50653821035484,0.,0.862217514001262));
#109008=DIRECTION('ref_axis',(0.862217514001262,0.,-0.50653821035484));
#109009=DIRECTION('center_axis',(0.482476521947278,-1.33914135876736E-14,
0.875908902666058));
#109010=DIRECTION('ref_axis',(0.875908902666058,-3.49403168495695E-30,-0.482476521947278));
#109011=DIRECTION('center_axis',(1.,0.,0.));
#109012=DIRECTION('ref_axis',(0.,0.,-1.));
#109013=DIRECTION('center_axis',(-1.,-4.1800565686188E-16,-5.16102651992463E-32));
#109014=DIRECTION('ref_axis',(-4.1800565686188E-16,1.,-8.08534226092968E-63));
#109015=DIRECTION('center_axis',(1.,0.,0.));
#109016=DIRECTION('ref_axis',(0.,0.,-1.));
#109017=DIRECTION('',(1.,4.18005656861881E-16,5.16102651992463E-32));
#109018=DIRECTION('center_axis',(0.,0.,1.));
#109019=DIRECTION('ref_axis',(1.,0.,0.));
#109020=DIRECTION('center_axis',(0.,7.25334975031394E-33,1.));
#109021=DIRECTION('ref_axis',(0.754709580222751,0.656059028990531,-4.75862559411968E-33));
#109022=DIRECTION('center_axis',(0.,0.,1.));
#109023=DIRECTION('ref_axis',(1.,0.,0.));
#109024=DIRECTION('center_axis',(-1.,0.,0.));
#109025=DIRECTION('ref_axis',(0.,1.,0.));
#109026=DIRECTION('center_axis',(-1.,0.,0.));
#109027=DIRECTION('ref_axis',(0.,0.,1.));
#109028=DIRECTION('',(1.,4.18005656861881E-16,0.));
#109029=DIRECTION('center_axis',(-4.18005656861882E-16,1.,0.));
#109030=DIRECTION('ref_axis',(1.,0.,0.));
#109031=DIRECTION('center_axis',(0.,0.,1.));
#109032=DIRECTION('ref_axis',(1.,0.,0.));
#109033=DIRECTION('center_axis',(0.,-1.,0.));
#109034=DIRECTION('ref_axis',(1.,0.,0.));
#109035=DIRECTION('center_axis',(0.,0.,-1.));
#109036=DIRECTION('ref_axis',(1.,0.,0.));
#109037=DIRECTION('center_axis',(0.,0.,1.));
#109038=DIRECTION('ref_axis',(1.,0.,0.));
#109039=DIRECTION('',(0.,0.,-1.));
#109040=DIRECTION('center_axis',(-4.18005656861882E-16,1.,0.));
#109041=DIRECTION('ref_axis',(1.,0.,0.));
#109042=DIRECTION('center_axis',(0.,-1.,0.));
#109043=DIRECTION('ref_axis',(1.,0.,0.));
#109044=DIRECTION('center_axis',(-4.18005656861881E-16,1.,0.));
#109045=DIRECTION('ref_axis',(1.,4.18005656861881E-16,0.));
#109046=DIRECTION('center_axis',(0.,1.,0.));
#109047=DIRECTION('ref_axis',(-1.,0.,0.));
#109048=DIRECTION('',(4.18005656861881E-16,-1.,0.));
#109049=DIRECTION('center_axis',(4.18005656861882E-16,-1.,0.));
#109050=DIRECTION('ref_axis',(-1.,0.,0.));
#109051=DIRECTION('center_axis',(0.,0.,-1.));
#109052=DIRECTION('ref_axis',(-1.,0.,0.));
#109053=DIRECTION('center_axis',(-1.,0.,0.));
#109054=DIRECTION('ref_axis',(0.,1.,0.));
#109055=DIRECTION('',(-1.,-4.18005656861881E-16,0.));
#109056=DIRECTION('center_axis',(1.,0.,0.));
#109057=DIRECTION('ref_axis',(0.,0.,-1.));
#109058=DIRECTION('center_axis',(0.,-7.25334975031394E-33,-1.));
#109059=DIRECTION('ref_axis',(1.,0.,0.));
#109060=DIRECTION('center_axis',(0.,0.,1.));
#109061=DIRECTION('ref_axis',(1.,0.,0.));
#109062=DIRECTION('center_axis',(0.,0.,1.));
#109063=DIRECTION('ref_axis',(1.,0.,0.));
#109064=DIRECTION('center_axis',(1.,0.,0.));
#109065=DIRECTION('ref_axis',(0.,0.,-1.));
#109066=DIRECTION('center_axis',(1.,4.1800565686188E-16,5.16102651992463E-32));
#109067=DIRECTION('ref_axis',(4.1800565686188E-16,-1.,8.08534226092968E-63));
#109068=DIRECTION('center_axis',(1.,0.,0.));
#109069=DIRECTION('ref_axis',(0.,0.,-1.));
#109070=DIRECTION('',(-1.,-4.18005656861881E-16,-5.16102651992463E-32));
#109071=DIRECTION('center_axis',(0.495139693244723,0.,0.868813377068702));
#109072=DIRECTION('ref_axis',(0.868813377068702,0.,-0.495139693244723));
#109073=DIRECTION('center_axis',(0.517480097907924,0.,0.855695242635604));
#109074=DIRECTION('ref_axis',(0.855695242635604,0.,-0.517480097907924));
#109075=DIRECTION('center_axis',(0.,0.,1.));
#109076=DIRECTION('ref_axis',(1.,0.,0.));
#109077=DIRECTION('center_axis',(0.,0.,1.));
#109078=DIRECTION('ref_axis',(-1.,0.,0.));
#109079=DIRECTION('center_axis',(-1.11022302462516E-12,0.,1.));
#109080=DIRECTION('ref_axis',(1.,0.,1.11022302462516E-12));
#109081=DIRECTION('',(0.,0.,-1.));
#109082=DIRECTION('center_axis',(-0.517480097905755,0.,0.855695242636916));
#109083=DIRECTION('ref_axis',(0.855695242636916,0.,0.517480097905755));
#109084=DIRECTION('center_axis',(-0.49549481432688,0.,0.868610896187223));
#109085=DIRECTION('ref_axis',(0.868610896187223,0.,0.49549481432688));
#109086=DIRECTION('center_axis',(0.,0.,1.));
#109087=DIRECTION('ref_axis',(-1.,0.,0.));
#109088=DIRECTION('center_axis',(0.,0.,-1.));
#109089=DIRECTION('ref_axis',(-1.,0.,0.));
#109090=DIRECTION('',(0.,0.,1.));
#109091=DIRECTION('center_axis',(4.18005656861882E-16,-1.,0.));
#109092=DIRECTION('ref_axis',(-1.,0.,0.));
#109093=DIRECTION('center_axis',(0.,1.,0.));
#109094=DIRECTION('ref_axis',(-1.,0.,0.));
#109095=DIRECTION('center_axis',(0.,-1.18842113532926E-16,1.));
#109096=DIRECTION('ref_axis',(0.,1.,1.18842113532926E-16));
#109097=DIRECTION('center_axis',(0.460985151818831,0.,-0.887407848625743));
#109098=DIRECTION('ref_axis',(-0.887407848625743,0.,-0.460985151818831));
#109099=DIRECTION('center_axis',(-0.483825549717016,0.,0.87516446308167));
#109100=DIRECTION('ref_axis',(0.87516446308167,0.,0.483825549717016));
#109101=DIRECTION('center_axis',(-1.,0.,0.));
#109102=DIRECTION('ref_axis',(0.,0.,1.));
#109103=DIRECTION('center_axis',(-0.661718432379332,0.,-0.749752436641215));
#109104=DIRECTION('ref_axis',(-0.749752436641215,0.,0.661718432379332));
#109105=DIRECTION('center_axis',(0.,0.,-1.));
#109106=DIRECTION('ref_axis',(-1.,0.,0.));
#109107=DIRECTION('center_axis',(0.,0.,1.));
#109108=DIRECTION('ref_axis',(0.,-1.,0.));
#109109=DIRECTION('center_axis',(0.,0.,-1.));
#109110=DIRECTION('ref_axis',(-1.,0.,0.));
#109111=DIRECTION('center_axis',(-1.,0.,0.));
#109112=DIRECTION('ref_axis',(0.,1.,0.));
#109113=DIRECTION('center_axis',(-1.,0.,0.));
#109114=DIRECTION('ref_axis',(0.,0.,1.));
#109115=DIRECTION('',(1.,4.18005656861881E-16,0.));
#109116=DIRECTION('center_axis',(0.732878068742756,0.679645439025561,-0.0311739244825062));
#109117=DIRECTION('ref_axis',(0.680359513835124,-0.732052760892824,0.0347805578337564));
#109118=DIRECTION('center_axis',(-4.18005656861882E-16,1.,0.));
#109119=DIRECTION('ref_axis',(1.,0.,0.));
#109120=DIRECTION('center_axis',(0.,0.,1.));
#109121=DIRECTION('ref_axis',(1.,0.,0.));
#109122=DIRECTION('center_axis',(0.,-1.,0.));
#109123=DIRECTION('ref_axis',(1.,0.,0.));
#109124=DIRECTION('center_axis',(0.,0.,-1.));
#109125=DIRECTION('ref_axis',(1.,0.,0.));
#109126=DIRECTION('',(0.,0.,-1.));
#109127=DIRECTION('center_axis',(0.483753083973024,0.,-0.875204521095834));
#109128=DIRECTION('ref_axis',(-0.875204521095834,0.,-0.483753083973024));
#109129=DIRECTION('center_axis',(0.,0.,-1.));
#109130=DIRECTION('ref_axis',(-1.,0.,0.));
#109131=DIRECTION('center_axis',(0.,0.,-1.));
#109132=DIRECTION('ref_axis',(1.,0.,0.));
#109133=DIRECTION('center_axis',(0.,0.,-1.));
#109134=DIRECTION('ref_axis',(-1.,0.,0.));
#109135=DIRECTION('',(0.,0.,1.));
#109136=DIRECTION('center_axis',(-0.48375308397303,0.,-0.875204521095831));
#109137=DIRECTION('ref_axis',(-0.875204521095831,0.,0.48375308397303));
#109138=DIRECTION('center_axis',(-0.460817663464343,0.,-0.887494834373285));
#109139=DIRECTION('ref_axis',(-0.887494834373285,0.,0.460817663464343));
#109140=DIRECTION('center_axis',(0.214288672238559,-0.976770219107516,0.000551375454002857));
#109141=DIRECTION('ref_axis',(0.837939441759682,0.183541158169798,-0.513974839074017));
#109142=DIRECTION('center_axis',(-1.,0.,0.));
#109143=DIRECTION('ref_axis',(0.,0.,1.));
#109144=DIRECTION('center_axis',(0.,0.,-1.));
#109145=DIRECTION('ref_axis',(-1.,0.,0.));
#109146=DIRECTION('center_axis',(0.,-7.60037129918555E-33,1.));
#109147=DIRECTION('ref_axis',(-1.,0.,0.));
#109148=DIRECTION('center_axis',(0.,0.,-1.));
#109149=DIRECTION('ref_axis',(-1.,0.,0.));
#109150=DIRECTION('center_axis',(1.,0.,0.));
#109151=DIRECTION('ref_axis',(0.,-1.,0.));
#109152=DIRECTION('center_axis',(1.,0.,0.));
#109153=DIRECTION('ref_axis',(0.,0.,-1.));
#109154=DIRECTION('',(1.,4.38004274807345E-16,0.));
#109155=DIRECTION('center_axis',(-4.38004274807345E-16,1.,0.));
#109156=DIRECTION('ref_axis',(1.,0.,0.));
#109157=DIRECTION('center_axis',(0.,0.,-1.));
#109158=DIRECTION('ref_axis',(-1.,0.,0.));
#109159=DIRECTION('center_axis',(0.,-1.,0.));
#109160=DIRECTION('ref_axis',(1.,0.,0.));
#109161=DIRECTION('center_axis',(0.,0.,1.));
#109162=DIRECTION('ref_axis',(-1.,0.,0.));
#109163=DIRECTION('center_axis',(0.,0.,-1.));
#109164=DIRECTION('ref_axis',(-1.,0.,0.));
#109165=DIRECTION('',(0.,0.,-1.));
#109166=DIRECTION('center_axis',(-4.38004274807345E-16,1.,0.));
#109167=DIRECTION('ref_axis',(1.,0.,0.));
#109168=DIRECTION('center_axis',(0.,-1.,0.));
#109169=DIRECTION('ref_axis',(1.,0.,0.));
#109170=DIRECTION('center_axis',(-1.,0.,0.));
#109171=DIRECTION('ref_axis',(0.,0.,1.));
#109172=DIRECTION('center_axis',(-1.,-4.38004274807346E-16,-5.40794518211031E-32));
#109173=DIRECTION('ref_axis',(-4.38004274807346E-16,1.,5.80597460094347E-63));
#109174=DIRECTION('center_axis',(-1.,0.,0.));
#109175=DIRECTION('ref_axis',(0.,0.,1.));
#109176=DIRECTION('',(-1.,-4.38004274807345E-16,-5.40794518211031E-32));
#109177=DIRECTION('center_axis',(1.,0.,5.40794518211031E-32));
#109178=DIRECTION('ref_axis',(0.,-1.,0.));
#109179=DIRECTION('center_axis',(-1.,0.,0.));
#109180=DIRECTION('ref_axis',(0.,0.,1.));
#109181=DIRECTION('center_axis',(1.,0.,5.40794518211031E-32));
#109182=DIRECTION('ref_axis',(0.,-1.,0.));
#109183=DIRECTION('center_axis',(-4.18005656861881E-16,1.,0.));
#109184=DIRECTION('ref_axis',(1.,4.18005656861881E-16,0.));
#109185=DIRECTION('center_axis',(0.,1.,0.));
#109186=DIRECTION('ref_axis',(-1.,0.,0.));
#109187=DIRECTION('',(4.18005656861881E-16,-1.,0.));
#109188=DIRECTION('center_axis',(4.18005656861882E-16,-1.,0.));
#109189=DIRECTION('ref_axis',(-1.,0.,0.));
#109190=DIRECTION('center_axis',(0.,0.,-1.));
#109191=DIRECTION('ref_axis',(-1.,0.,0.));
#109192=DIRECTION('center_axis',(-1.,0.,0.));
#109193=DIRECTION('ref_axis',(0.,1.,0.));
#109194=DIRECTION('',(-1.,-4.18005656861881E-16,0.));
#109195=DIRECTION('center_axis',(1.,0.,0.));
#109196=DIRECTION('ref_axis',(0.,0.,-1.));
#109197=DIRECTION('center_axis',(0.,7.25334975031382E-33,-1.));
#109198=DIRECTION('ref_axis',(1.,0.,0.));
#109199=DIRECTION('center_axis',(0.,0.,1.));
#109200=DIRECTION('ref_axis',(1.,0.,0.));
#109201=DIRECTION('center_axis',(0.,0.,1.));
#109202=DIRECTION('ref_axis',(1.,0.,0.));
#109203=DIRECTION('center_axis',(0.,0.,1.));
#109204=DIRECTION('ref_axis',(1.,0.,0.));
#109205=DIRECTION('center_axis',(1.,0.,0.));
#109206=DIRECTION('ref_axis',(0.,0.,-1.));
#109207=DIRECTION('center_axis',(-1.,0.,-5.16102651992463E-32));
#109208=DIRECTION('ref_axis',(0.,1.,0.));
#109209=DIRECTION('center_axis',(1.,0.,-1.38777878078144E-14));
#109210=DIRECTION('ref_axis',(-1.38777878078144E-14,0.,-1.));
#109211=DIRECTION('',(-1.,-4.18005656861881E-16,-5.16102651992463E-32));
#109212=DIRECTION('center_axis',(0.534259922646944,0.,0.845320255910907));
#109213=DIRECTION('ref_axis',(0.845320255910907,0.,-0.534259922646944));
#109214=DIRECTION('center_axis',(0.543750575738856,0.,0.839246871536417));
#109215=DIRECTION('ref_axis',(0.839246871536417,0.,-0.543750575738856));
#109216=DIRECTION('center_axis',(0.,-1.66533453693774E-12,-1.));
#109217=DIRECTION('ref_axis',(0.,-1.,1.66533453693774E-12));
#109218=DIRECTION('center_axis',(0.,0.,1.));
#109219=DIRECTION('ref_axis',(-1.,0.,0.));
#109220=DIRECTION('center_axis',(0.,0.,-1.));
#109221=DIRECTION('ref_axis',(-1.,0.,0.));
#109222=DIRECTION('',(0.,0.,-1.));
#109223=DIRECTION('center_axis',(0.543750575738856,0.,-0.839246871536417));
#109224=DIRECTION('ref_axis',(-0.839246871536417,0.,-0.543750575738856));
#109225=DIRECTION('center_axis',(0.534875344054122,-1.17257728967007E-14,
-0.844930983171398));
#109226=DIRECTION('ref_axis',(-0.844930983171398,-8.89670234612257E-31,
-0.534875344054122));
#109227=DIRECTION('center_axis',(1.,0.,0.));
#109228=DIRECTION('ref_axis',(0.,0.,-1.));
#109229=DIRECTION('center_axis',(1.,4.1800565686188E-16,5.16102651992463E-32));
#109230=DIRECTION('ref_axis',(4.1800565686188E-16,-1.,8.08534226092968E-63));
#109231=DIRECTION('center_axis',(0.,0.,1.));
#109232=DIRECTION('ref_axis',(-1.,0.,0.));
#109233=DIRECTION('center_axis',(0.,0.,-1.));
#109234=DIRECTION('ref_axis',(-1.,0.,0.));
#109235=DIRECTION('',(0.,0.,1.));
#109236=DIRECTION('center_axis',(4.18005656861882E-16,-1.,0.));
#109237=DIRECTION('ref_axis',(-1.,0.,0.));
#109238=DIRECTION('center_axis',(0.,1.,0.));
#109239=DIRECTION('ref_axis',(-1.,0.,0.));
#109240=DIRECTION('center_axis',(0.,1.23467863058847E-16,-1.));
#109241=DIRECTION('ref_axis',(0.,1.,1.1837531408762E-16));
#109242=DIRECTION('center_axis',(0.,-1.19392659184112E-16,1.));
#109243=DIRECTION('ref_axis',(0.,1.,1.19392659184112E-16));
#109244=DIRECTION('center_axis',(1.,0.,5.16102651992463E-32));
#109245=DIRECTION('ref_axis',(0.,-1.,0.));
#109246=DIRECTION('center_axis',(-1.,0.,0.));
#109247=DIRECTION('ref_axis',(0.,0.,1.));
#109248=DIRECTION('center_axis',(-0.496741562438066,-1.20445113324067E-14,
0.867898507975782));
#109249=DIRECTION('ref_axis',(0.867898507975782,5.70559822356712E-31,0.496741562438066));
#109250=DIRECTION('center_axis',(-0.518474310548575,0.,0.855093205037428));
#109251=DIRECTION('ref_axis',(0.855093205037428,0.,0.518474310548575));
#109252=DIRECTION('center_axis',(0.,0.,1.));
#109253=DIRECTION('ref_axis',(1.,0.,0.));
#109254=DIRECTION('center_axis',(0.,0.,-1.));
#109255=DIRECTION('ref_axis',(1.,0.,0.));
#109256=DIRECTION('center_axis',(-2.72711680125255E-25,-1.11022302462516E-13,
1.));
#109257=DIRECTION('ref_axis',(-1.56607307231965E-53,1.,1.11022302462516E-13));
#109258=DIRECTION('',(0.,0.,1.));
#109259=DIRECTION('center_axis',(0.518474310548581,-7.19527646559628E-15,
0.855093205037424));
#109260=DIRECTION('ref_axis',(0.855093205037424,3.43699106634736E-31,-0.518474310548581));
#109261=DIRECTION('center_axis',(0.496378972716316,-6.19668439877561E-14,
0.868105935612178));
#109262=DIRECTION('ref_axis',(0.868105935612178,3.44724486393529E-29,-0.496378972716316));
#109263=DIRECTION('center_axis',(1.,0.,0.));
#109264=DIRECTION('ref_axis',(0.,0.,-1.));
#109265=DIRECTION('center_axis',(-1.,-4.1800565686188E-16,-5.16102651992463E-32));
#109266=DIRECTION('ref_axis',(-4.1800565686188E-16,1.,-8.08534226092968E-63));
#109267=DIRECTION('center_axis',(1.,0.,0.));
#109268=DIRECTION('ref_axis',(0.,0.,-1.));
#109269=DIRECTION('',(1.,4.18005656861881E-16,5.16102651992463E-32));
#109270=DIRECTION('center_axis',(0.,0.,1.));
#109271=DIRECTION('ref_axis',(1.,0.,0.));
#109272=DIRECTION('center_axis',(0.,-7.25334975031382E-33,1.));
#109273=DIRECTION('ref_axis',(-1.,0.,0.));
#109274=DIRECTION('center_axis',(0.,0.,1.));
#109275=DIRECTION('ref_axis',(1.,0.,0.));
#109276=DIRECTION('center_axis',(-1.,0.,0.));
#109277=DIRECTION('ref_axis',(0.,1.,0.));
#109278=DIRECTION('center_axis',(-1.,0.,0.));
#109279=DIRECTION('ref_axis',(0.,0.,1.));
#109280=DIRECTION('',(1.,4.18005656861881E-16,0.));
#109281=DIRECTION('center_axis',(-4.18005656861882E-16,1.,0.));
#109282=DIRECTION('ref_axis',(1.,0.,0.));
#109283=DIRECTION('center_axis',(0.,0.,1.));
#109284=DIRECTION('ref_axis',(1.,0.,0.));
#109285=DIRECTION('center_axis',(0.,-1.,0.));
#109286=DIRECTION('ref_axis',(1.,0.,0.));
#109287=DIRECTION('center_axis',(0.,0.,-1.));
#109288=DIRECTION('ref_axis',(1.,0.,0.));
#109289=DIRECTION('center_axis',(0.,0.,1.));
#109290=DIRECTION('ref_axis',(1.,0.,0.));
#109291=DIRECTION('',(0.,0.,-1.));
#109292=DIRECTION('center_axis',(-4.18005656861882E-16,1.,0.));
#109293=DIRECTION('ref_axis',(1.,0.,0.));
#109294=DIRECTION('center_axis',(0.,-1.,0.));
#109295=DIRECTION('ref_axis',(1.,0.,0.));
#109296=DIRECTION('center_axis',(-4.18005656861881E-16,1.,0.));
#109297=DIRECTION('ref_axis',(1.,4.18005656861881E-16,0.));
#109298=DIRECTION('center_axis',(0.,1.,0.));
#109299=DIRECTION('ref_axis',(-1.,0.,0.));
#109300=DIRECTION('',(4.18005656861881E-16,-1.,0.));
#109301=DIRECTION('center_axis',(4.18005656861882E-16,-1.,0.));
#109302=DIRECTION('ref_axis',(-1.,0.,0.));
#109303=DIRECTION('center_axis',(0.,0.,-1.));
#109304=DIRECTION('ref_axis',(-1.,0.,0.));
#109305=DIRECTION('center_axis',(-1.,0.,-5.16102651992463E-32));
#109306=DIRECTION('ref_axis',(0.,1.,0.));
#109307=DIRECTION('center_axis',(-1.,0.,0.));
#109308=DIRECTION('ref_axis',(0.,1.,0.));
#109309=DIRECTION('',(-1.,-4.18005656861881E-16,0.));
#109310=DIRECTION('center_axis',(1.,0.,0.));
#109311=DIRECTION('ref_axis',(0.,0.,-1.));
#109312=DIRECTION('center_axis',(0.,7.25334975031382E-33,-1.));
#109313=DIRECTION('ref_axis',(1.,0.,0.));
#109314=DIRECTION('center_axis',(0.,0.,1.));
#109315=DIRECTION('ref_axis',(1.,0.,0.));
#109316=DIRECTION('center_axis',(0.,0.,1.));
#109317=DIRECTION('ref_axis',(1.,0.,0.));
#109318=DIRECTION('center_axis',(0.,0.,1.));
#109319=DIRECTION('ref_axis',(1.,0.,0.));
#109320=DIRECTION('center_axis',(1.,0.,0.));
#109321=DIRECTION('ref_axis',(0.,0.,-1.));
#109322=DIRECTION('center_axis',(1.,4.1800565686188E-16,5.16102651992463E-32));
#109323=DIRECTION('ref_axis',(4.1800565686188E-16,-1.,8.08534226092968E-63));
#109324=DIRECTION('center_axis',(1.,0.,0.));
#109325=DIRECTION('ref_axis',(0.,0.,-1.));
#109326=DIRECTION('',(-1.,-4.18005656861881E-16,-5.16102651992463E-32));
#109327=DIRECTION('center_axis',(0.483537964931496,0.,0.875323389650881));
#109328=DIRECTION('ref_axis',(0.875323389650881,0.,-0.483537964931496));
#109329=DIRECTION('center_axis',(0.507514080295474,0.,0.861643463563578));
#109330=DIRECTION('ref_axis',(0.861643463563578,0.,-0.507514080295474));
#109331=DIRECTION('center_axis',(1.11022302462516E-13,0.,1.));
#109332=DIRECTION('ref_axis',(1.,0.,-1.11022302462516E-13));
#109333=DIRECTION('center_axis',(0.,0.,1.));
#109334=DIRECTION('ref_axis',(-1.,0.,0.));
#109335=DIRECTION('center_axis',(0.,0.,1.));
#109336=DIRECTION('ref_axis',(1.,0.,0.));
#109337=DIRECTION('',(0.,0.,-1.));
#109338=DIRECTION('center_axis',(-0.507514080295481,0.,0.861643463563574));
#109339=DIRECTION('ref_axis',(0.861643463563574,0.,0.507514080295481));
#109340=DIRECTION('center_axis',(0.,0.,1.));
#109341=DIRECTION('ref_axis',(-1.,0.,0.));
#109342=DIRECTION('center_axis',(0.,0.,-1.));
#109343=DIRECTION('ref_axis',(-1.,0.,0.));
#109344=DIRECTION('',(0.,0.,1.));
#109345=DIRECTION('center_axis',(4.18005656861882E-16,-1.,0.));
#109346=DIRECTION('ref_axis',(-1.,0.,0.));
#109347=DIRECTION('center_axis',(0.,1.,0.));
#109348=DIRECTION('ref_axis',(-1.,0.,0.));
#109349=DIRECTION('center_axis',(0.,1.23467863058847E-16,-1.));
#109350=DIRECTION('ref_axis',(-1.,0.,0.));
#109351=DIRECTION('center_axis',(0.,0.,1.));
#109352=DIRECTION('ref_axis',(0.,1.,0.));
#109353=DIRECTION('center_axis',(0.,0.,1.));
#109354=DIRECTION('ref_axis',(0.,-1.,0.));
#109355=DIRECTION('center_axis',(5.01606788234257E-16,-1.,5.70122241611331E-32));
#109356=DIRECTION('ref_axis',(-4.59816715307009E-64,-5.70122241611331E-32,
-1.));
#109357=DIRECTION('',(-1.,-5.01606788234257E-16,0.));
#109358=DIRECTION('center_axis',(0.,0.,-1.));
#109359=DIRECTION('ref_axis',(-1.,0.,0.));
#109360=DIRECTION('center_axis',(0.990268068741571,0.139173100960059,1.71834053708117E-17));
#109361=DIRECTION('ref_axis',(0.139173100960059,-0.990268068741571,4.14246685971564E-34));
#109362=DIRECTION('center_axis',(-0.990268068741571,-0.139173100960059,
0.));
#109363=DIRECTION('ref_axis',(0.139173100960059,-0.990268068741571,0.));
#109364=DIRECTION('center_axis',(0.,1.23467863058847E-16,-1.));
#109365=DIRECTION('ref_axis',(0.,1.,0.));
#109366=DIRECTION('center_axis',(-0.728126055379271,-0.685443248911113,
0.));
#109367=DIRECTION('ref_axis',(0.685443248911113,-0.728126055379271,0.));
#109368=DIRECTION('center_axis',(0.,1.23467863058847E-16,-1.));
#109369=DIRECTION('ref_axis',(0.,1.,0.));
#109370=DIRECTION('center_axis',(-0.685443248911109,-0.728126055379275,
0.));
#109371=DIRECTION('ref_axis',(0.728126055379275,-0.685443248911109,0.));
#109372=DIRECTION('center_axis',(0.,1.23467863058847E-16,-1.));
#109373=DIRECTION('ref_axis',(0.,1.,0.));
#109374=DIRECTION('center_axis',(-0.139173100960066,-0.99026806874157,0.));
#109375=DIRECTION('ref_axis',(0.99026806874157,-0.139173100960066,0.));
#109376=DIRECTION('center_axis',(0.139173100960066,0.99026806874157,1.22266282302933E-16));
#109377=DIRECTION('ref_axis',(0.99026806874157,-0.139173100960066,-9.57340194962255E-34));
#109378=DIRECTION('center_axis',(0.139173100960066,0.99026806874157,0.));
#109379=DIRECTION('ref_axis',(-0.99026806874157,0.139173100960066,0.));
#109380=DIRECTION('center_axis',(-0.139173100960066,-0.99026806874157,0.));
#109381=DIRECTION('ref_axis',(-0.99026806874157,0.139173100960066,0.));
#109382=DIRECTION('center_axis',(0.139173100960066,0.99026806874157,0.));
#109383=DIRECTION('ref_axis',(-0.99026806874157,0.139173100960066,0.));
#109384=DIRECTION('',(0.139173100960067,0.99026806874157,0.));
#109385=DIRECTION('center_axis',(0.139173100960066,0.99026806874157,1.22266282302933E-16));
#109386=DIRECTION('ref_axis',(0.99026806874157,-0.139173100960066,-9.57340194962255E-34));
#109387=DIRECTION('',(0.139173100960067,0.99026806874157,1.22266282302933E-16));
#109388=DIRECTION('center_axis',(0.139173100960066,0.99026806874157,0.));
#109389=DIRECTION('ref_axis',(-0.99026806874157,0.139173100960066,0.));
#109390=DIRECTION('center_axis',(-0.139173100960066,-0.99026806874157,0.));
#109391=DIRECTION('ref_axis',(-0.99026806874157,0.139173100960066,0.));
#109392=DIRECTION('center_axis',(0.139173100960066,0.99026806874157,0.));
#109393=DIRECTION('ref_axis',(-0.99026806874157,0.139173100960066,0.));
#109394=DIRECTION('',(0.139173100960067,0.99026806874157,0.));
#109395=DIRECTION('center_axis',(0.139173100960066,0.99026806874157,1.22266282302933E-16));
#109396=DIRECTION('ref_axis',(0.99026806874157,-0.139173100960066,-9.57340194962255E-34));
#109397=DIRECTION('center_axis',(0.139173100960066,0.99026806874157,0.));
#109398=DIRECTION('ref_axis',(-0.99026806874157,0.139173100960066,0.));
#109399=DIRECTION('',(0.139173100960067,0.99026806874157,1.22266282302933E-16));
#109400=DIRECTION('center_axis',(0.133528512868191,0.950104737537312,-0.281906232567436));
#109401=DIRECTION('ref_axis',(2.32560161936155E-16,-0.284453521859895,-0.958689831958962));
#109402=DIRECTION('center_axis',(0.369731042763204,0.785707308414229,0.495946551073502));
#109403=DIRECTION('ref_axis',(-1.91361720426385E-15,0.533770129672178,-0.845629616717477));
#109404=DIRECTION('center_axis',(0.416737288136069,0.909026970269307,0.));
#109405=DIRECTION('ref_axis',(-0.909026970269307,0.416737288136069,0.));
#109406=DIRECTION('center_axis',(0.,0.,1.));
#109407=DIRECTION('ref_axis',(-1.,0.,0.));
#109408=DIRECTION('center_axis',(0.40826271186488,0.912864479591979,-3.16713488626711E-15));
#109409=DIRECTION('ref_axis',(-0.912864479591979,0.40826271186488,6.04208104977424E-31));
#109410=DIRECTION('center_axis',(0.,0.,-1.));
#109411=DIRECTION('ref_axis',(-1.,0.,0.));
#109412=DIRECTION('center_axis',(0.,-6.17339315294237E-17,1.));
#109413=DIRECTION('ref_axis',(0.,-1.,0.));
#109414=DIRECTION('center_axis',(0.,0.,-1.));
#109415=DIRECTION('ref_axis',(0.,-1.,0.));
#109416=DIRECTION('center_axis',(-0.278601694915732,-0.960406734456856,
8.33020054374265E-16));
#109417=DIRECTION('ref_axis',(0.960406734456856,-0.278601694915732,-5.45700864471184E-31));
#109418=DIRECTION('center_axis',(0.,0.,1.));
#109419=DIRECTION('ref_axis',(-1.,0.,0.));
#109420=DIRECTION('center_axis',(-0.270127118644541,-0.962824667202081,
4.0829772679528E-16));
#109421=DIRECTION('ref_axis',(0.962824667202081,-0.270127118644541,5.77560433057458E-31));
#109422=DIRECTION('center_axis',(0.,0.,-1.));
#109423=DIRECTION('ref_axis',(-1.,0.,0.));
#109424=DIRECTION('center_axis',(-0.185959552881302,-0.695904038033425,
0.693640118895209));
#109425=DIRECTION('ref_axis',(-3.15382046976506E-16,0.705953788300242,0.708257897085897));
#109426=DIRECTION('center_axis',(0.,-6.17339315294237E-17,1.));
#109427=DIRECTION('ref_axis',(0.,-1.,0.));
#109428=DIRECTION('center_axis',(0.,0.,-1.));
#109429=DIRECTION('ref_axis',(0.,-1.,0.));
#109430=DIRECTION('center_axis',(0.141151402782332,0.989840911569284,-0.0170660855578596));
#109431=DIRECTION('ref_axis',(-0.989985089278404,0.141171962536586,2.4318092123443E-19));
#109432=DIRECTION('center_axis',(0.1326869973619,0.991030504325029,-0.0158965476868861));
#109433=DIRECTION('ref_axis',(-0.991155744879145,0.132703765557229,-2.90070390844182E-17));
#109434=DIRECTION('center_axis',(-0.1499957800683,0.0101893565027498,-0.988634129987308));
#109435=DIRECTION('ref_axis',(-0.981224439714038,0.121089666642347,0.150119590794534));
#109436=DIRECTION('center_axis',(0.,-6.17339315294237E-17,1.));
#109437=DIRECTION('ref_axis',(0.,-1.,0.));
#109438=DIRECTION('center_axis',(0.,0.,-1.));
#109439=DIRECTION('ref_axis',(0.,-1.,0.));
#109440=DIRECTION('center_axis',(0.00234948403731584,0.999997203076769,
-0.000271594180011335));
#109441=DIRECTION('ref_axis',(-0.999997239958367,0.00234948412396881,6.81083076705817E-23));
#109442=DIRECTION('center_axis',(-0.00619406208384126,0.999980560265093,
0.000716021516796888));
#109443=DIRECTION('ref_axis',(-0.999980816603614,-0.00619406367164884,-2.43997512021813E-21));
#109444=DIRECTION('center_axis',(-0.0216109392502409,-2.83714134350443E-8,
-0.99976645638105));
#109445=DIRECTION('ref_axis',(-0.999764411688039,0.00202245879910768,0.021610894994789));
#109446=DIRECTION('center_axis',(0.,-6.17339315294237E-17,1.));
#109447=DIRECTION('ref_axis',(0.,-1.,0.));
#109448=DIRECTION('center_axis',(0.,0.,-1.));
#109449=DIRECTION('ref_axis',(0.,-1.,0.));
#109450=DIRECTION('center_axis',(-0.136497250965888,0.990504401193308,0.0164174204868685));
#109451=DIRECTION('ref_axis',(-0.990637914348733,-0.136515649853022,4.14575077332242E-19));
#109452=DIRECTION('center_axis',(-0.144956948347396,0.989281282708723,0.017607578141073));
#109453=DIRECTION('ref_axis',(-0.989434670234472,-0.144979423843532,1.06064347286242E-18));
#109454=DIRECTION('center_axis',(-0.157548218657054,-0.0111059690216339,
-0.98744884234581));
#109455=DIRECTION('ref_axis',(-0.980524532402052,-0.11697738133772,0.157759099937552));
#109456=DIRECTION('center_axis',(0.,-6.17339315294237E-17,1.));
#109457=DIRECTION('ref_axis',(0.,-1.,0.));
#109458=DIRECTION('center_axis',(0.,0.,-1.));
#109459=DIRECTION('ref_axis',(0.,-1.,0.));
#109460=DIRECTION('center_axis',(0.0971107883155516,-0.363411229368455,
-0.926553707650906));
#109461=DIRECTION('ref_axis',(-3.86068458172679E-17,-0.930953788243945,
0.365137021067773));
#109462=DIRECTION('center_axis',(0.273940677965627,-0.961746590820957,0.));
#109463=DIRECTION('ref_axis',(0.961746590820957,0.273940677965627,0.));
#109464=DIRECTION('center_axis',(0.,0.,1.));
#109465=DIRECTION('ref_axis',(-1.,0.,0.));
#109466=DIRECTION('center_axis',(0.282415254236812,-0.959292251701408,0.));
#109467=DIRECTION('ref_axis',(0.959292251701408,0.282415254236812,0.));
#109468=DIRECTION('center_axis',(0.,0.,-1.));
#109469=DIRECTION('ref_axis',(-1.,0.,0.));
#109470=DIRECTION('center_axis',(0.,-6.17339315294237E-17,1.));
#109471=DIRECTION('ref_axis',(0.,-1.,0.));
#109472=DIRECTION('center_axis',(0.,0.,-1.));
#109473=DIRECTION('ref_axis',(0.,-1.,0.));
#109474=DIRECTION('center_axis',(-0.412076271185962,0.911149354785193,0.));
#109475=DIRECTION('ref_axis',(-0.911149354785193,-0.412076271185962,0.));
#109476=DIRECTION('center_axis',(0.,0.,1.));
#109477=DIRECTION('ref_axis',(-1.,0.,0.));
#109478=DIRECTION('center_axis',(-0.42055084745715,0.907268970428876,0.));
#109479=DIRECTION('ref_axis',(-0.907268970428876,-0.42055084745715,0.));
#109480=DIRECTION('center_axis',(0.,0.,-1.));
#109481=DIRECTION('ref_axis',(-1.,0.,0.));
#109482=DIRECTION('center_axis',(-0.408524918701489,0.868147321075037,-0.281829061152641));
#109483=DIRECTION('ref_axis',(-0.904824724134437,-0.425784239486432,-2.46811619432984E-17));
#109484=DIRECTION('center_axis',(0.133528512868198,-0.950104737537311,-0.281906232567435));
#109485=DIRECTION('ref_axis',(-1.78830809785603E-17,-0.284453521859893,
0.958689831958962));
#109486=DIRECTION('center_axis',(-0.139173100960066,0.99026806874157,1.22266282302934E-16));
#109487=DIRECTION('ref_axis',(0.99026806874157,0.139173100960066,1.22723965167578E-33));
#109488=DIRECTION('',(-0.139173100960065,0.99026806874157,1.22266282302933E-16));
#109489=DIRECTION('center_axis',(-0.139173100960066,0.99026806874157,0.));
#109490=DIRECTION('ref_axis',(-0.99026806874157,-0.139173100960066,0.));
#109491=DIRECTION('center_axis',(0.139173100960066,-0.99026806874157,0.));
#109492=DIRECTION('ref_axis',(-0.99026806874157,-0.139173100960066,0.));
#109493=DIRECTION('center_axis',(-0.139173100960039,0.990268068741574,2.74854602616996E-14));
#109494=DIRECTION('ref_axis',(-0.990268068741574,-0.139173100960039,-5.80135260633727E-30));
#109495=DIRECTION('',(-0.139173100960065,0.99026806874157,0.));
#109496=DIRECTION('center_axis',(-0.139173100960066,0.99026806874157,1.22266282302934E-16));
#109497=DIRECTION('ref_axis',(0.99026806874157,0.139173100960066,1.22723965167578E-33));
#109498=DIRECTION('center_axis',(0.139173100960066,-0.99026806874157,0.));
#109499=DIRECTION('ref_axis',(0.99026806874157,0.139173100960066,0.));
#109500=DIRECTION('center_axis',(0.139173100960073,-0.990268068741569,0.));
#109501=DIRECTION('ref_axis',(0.990268068741569,0.139173100960073,0.));
#109502=DIRECTION('center_axis',(-0.139173100960066,0.99026806874157,1.22266282302934E-16));
#109503=DIRECTION('ref_axis',(0.99026806874157,0.139173100960066,1.22723965167578E-33));
#109504=DIRECTION('',(-0.139173100960065,0.99026806874157,1.22266282302933E-16));
#109505=DIRECTION('center_axis',(-0.139173100960066,0.99026806874157,0.));
#109506=DIRECTION('ref_axis',(-0.99026806874157,-0.139173100960066,0.));
#109507=DIRECTION('center_axis',(0.139173100960066,-0.99026806874157,0.));
#109508=DIRECTION('ref_axis',(-0.99026806874157,-0.139173100960066,0.));
#109509=DIRECTION('center_axis',(-0.139173100960066,0.99026806874157,0.));
#109510=DIRECTION('ref_axis',(-0.99026806874157,-0.139173100960066,0.));
#109511=DIRECTION('',(-0.139173100960065,0.99026806874157,0.));
#109512=DIRECTION('center_axis',(0.,1.23467863058847E-16,-1.));
#109513=DIRECTION('ref_axis',(0.,1.,0.));
#109514=DIRECTION('center_axis',(0.685443248911109,-0.728126055379275,0.));
#109515=DIRECTION('ref_axis',(0.728126055379275,0.685443248911109,0.));
#109516=DIRECTION('center_axis',(0.,1.23467863058847E-16,-1.));
#109517=DIRECTION('ref_axis',(0.,1.,0.));
#109518=DIRECTION('center_axis',(0.728126055379271,-0.685443248911113,0.));
#109519=DIRECTION('ref_axis',(0.685443248911113,0.728126055379271,0.));
#109520=DIRECTION('center_axis',(0.,1.23467863058847E-16,-1.));
#109521=DIRECTION('ref_axis',(0.,1.,0.));
#109522=DIRECTION('center_axis',(0.990268068741571,-0.139173100960059,0.));
#109523=DIRECTION('ref_axis',(0.139173100960059,0.990268068741571,0.));
#109524=DIRECTION('center_axis',(-0.990268068741571,0.139173100960059,1.71834053708117E-17));
#109525=DIRECTION('ref_axis',(0.139173100960059,0.990268068741571,-4.14246685971564E-34));
#109526=DIRECTION('center_axis',(-0.990268068741571,0.139173100960064,0.));
#109527=DIRECTION('ref_axis',(-0.139173100960064,-0.990268068741571,0.));
#109528=DIRECTION('center_axis',(0.990268068741572,-0.139173100960051,0.));
#109529=DIRECTION('ref_axis',(-0.139173100960051,-0.990268068741572,0.));
#109530=DIRECTION('center_axis',(-0.990268068741572,0.139173100960051,0.));
#109531=DIRECTION('ref_axis',(-0.139173100960051,-0.990268068741572,0.));
#109532=DIRECTION('',(-0.990268068741571,0.139173100960059,0.));
#109533=DIRECTION('center_axis',(-0.990268068741571,0.139173100960059,1.71834053708117E-17));
#109534=DIRECTION('ref_axis',(0.139173100960059,0.990268068741571,-4.14246685971564E-34));
#109535=DIRECTION('',(-0.990268068741571,0.139173100960059,1.71834053708117E-17));
#109536=DIRECTION('center_axis',(-0.990268068741572,0.139173100960051,0.));
#109537=DIRECTION('ref_axis',(-0.139173100960051,-0.990268068741572,0.));
#109538=DIRECTION('center_axis',(0.990268068741572,-0.139173100960051,0.));
#109539=DIRECTION('ref_axis',(-0.139173100960051,-0.990268068741572,0.));
#109540=DIRECTION('center_axis',(-0.990268068741572,0.139173100960051,1.37427301308497E-14));
#109541=DIRECTION('ref_axis',(-0.139173100960051,-0.990268068741572,1.93598700157835E-30));
#109542=DIRECTION('',(-0.990268068741571,0.139173100960059,0.));
#109543=DIRECTION('center_axis',(-0.990268068741571,0.139173100960059,1.71834053708117E-17));
#109544=DIRECTION('ref_axis',(0.139173100960059,0.990268068741571,-4.14246685971564E-34));
#109545=DIRECTION('center_axis',(-0.990268068741571,0.139173100960059,0.));
#109546=DIRECTION('ref_axis',(-0.139173100960059,-0.990268068741571,0.));
#109547=DIRECTION('',(-0.990268068741571,0.139173100960059,1.71834053708117E-17));
#109548=DIRECTION('center_axis',(1.,5.01606788234257E-16,0.));
#109549=DIRECTION('ref_axis',(5.01606788234257E-16,-1.,0.));
#109550=DIRECTION('',(-1.,-5.01606788234257E-16,0.));
#109551=DIRECTION('center_axis',(0.,1.23467863058847E-16,-1.));
#109552=DIRECTION('ref_axis',(0.,1.,0.));
#109553=DIRECTION('center_axis',(0.,0.,1.));
#109554=DIRECTION('ref_axis',(0.,1.,0.));
#109555=DIRECTION('center_axis',(0.,0.,-1.));
#109556=DIRECTION('ref_axis',(1.,8.87756872621991E-15,0.));
#109557=DIRECTION('center_axis',(1.,5.01606788234257E-16,0.));
#109558=DIRECTION('ref_axis',(5.01606788234257E-16,-1.,0.));
#109559=DIRECTION('center_axis',(-4.38004274807345E-16,1.,0.));
#109560=DIRECTION('ref_axis',(1.,4.38004274807345E-16,0.));
#109561=DIRECTION('center_axis',(-4.38004274807345E-16,1.,0.));
#109562=DIRECTION('ref_axis',(1.,4.38004274807345E-16,0.));
#109563=DIRECTION('center_axis',(5.01606788234257E-16,-1.,5.70122241611331E-32));
#109564=DIRECTION('ref_axis',(-4.59816715307009E-64,-5.70122241611331E-32,
-1.));
#109565=DIRECTION('center_axis',(-4.38004274807345E-16,1.,0.));
#109566=DIRECTION('ref_axis',(1.,4.38004274807345E-16,0.));
#109567=DIRECTION('center_axis',(-1.,-4.18005656861882E-16,0.));
#109568=DIRECTION('ref_axis',(-4.18005656861882E-16,1.,0.));
#109569=DIRECTION('',(-4.18005656861881E-16,1.,0.));
#109570=DIRECTION('center_axis',(-1.,-4.18005656861882E-16,0.));
#109571=DIRECTION('ref_axis',(-4.18005656861882E-16,1.,0.));
#109572=DIRECTION('',(-4.18005656861881E-16,1.,0.));
#109573=DIRECTION('center_axis',(0.,0.,1.));
#109574=DIRECTION('ref_axis',(1.,0.,0.));
#109575=DIRECTION('',(4.18005656861881E-16,-1.,0.));
#109576=DIRECTION('center_axis',(0.,0.,-1.));
#109577=DIRECTION('ref_axis',(-1.,0.,0.));
#109578=DIRECTION('center_axis',(-1.,-4.38004274807345E-16,0.));
#109579=DIRECTION('ref_axis',(-4.38004274807345E-16,1.,0.));
#109580=DIRECTION('center_axis',(4.18005656861881E-16,-1.,0.));
#109581=DIRECTION('ref_axis',(-1.,-4.18005656861881E-16,0.));
#109582=DIRECTION('center_axis',(0.,0.,1.));
#109583=DIRECTION('ref_axis',(1.,0.,0.));
#109584=DIRECTION('',(4.18005656861881E-16,-1.,0.));
#109585=DIRECTION('',(-1.,-4.18005656861881E-16,0.));
#109586=DIRECTION('center_axis',(4.18005656861881E-16,-1.,0.));
#109587=DIRECTION('ref_axis',(-1.,-4.18005656861881E-16,0.));
#109588=DIRECTION('',(-4.18005656861881E-16,1.,0.));
#109589=DIRECTION('center_axis',(-1.,-4.18005656861882E-16,0.));
#109590=DIRECTION('ref_axis',(-4.18005656861882E-16,1.,0.));
#109591=DIRECTION('center_axis',(-1.,0.,0.));
#109592=DIRECTION('ref_axis',(0.,1.,0.));
#109593=DIRECTION('center_axis',(0.,0.,-1.));
#109594=DIRECTION('ref_axis',(-1.,0.,0.));
#109595=DIRECTION('center_axis',(-1.,-4.38004274807345E-16,0.));
#109596=DIRECTION('ref_axis',(-4.38004274807345E-16,1.,0.));
#109597=DIRECTION('center_axis',(0.,0.,-1.));
#109598=DIRECTION('ref_axis',(-1.,0.,0.));
#109599=DIRECTION('center_axis',(-1.,-4.38004274807345E-16,0.));
#109600=DIRECTION('ref_axis',(-4.38004274807345E-16,1.,0.));
#109601=DIRECTION('center_axis',(0.,0.,-1.));
#109602=DIRECTION('ref_axis',(-1.,0.,0.));
#109603=DIRECTION('center_axis',(-1.,-4.38004274807345E-16,0.));
#109604=DIRECTION('ref_axis',(-4.38004274807345E-16,1.,0.));
#109605=DIRECTION('center_axis',(0.,0.,-1.));
#109606=DIRECTION('ref_axis',(-1.,0.,0.));
#109607=DIRECTION('center_axis',(-1.,-4.38004274807345E-16,0.));
#109608=DIRECTION('ref_axis',(-4.38004274807345E-16,1.,0.));
#109609=DIRECTION('center_axis',(-1.,0.,0.));
#109610=DIRECTION('ref_axis',(0.,1.,0.));
#109611=DIRECTION('',(1.,4.18005656861881E-16,0.));
#109612=DIRECTION('center_axis',(4.18005656861881E-16,-1.,0.));
#109613=DIRECTION('ref_axis',(-1.,-4.18005656861881E-16,0.));
#109614=DIRECTION('',(-4.18005656861881E-16,1.,0.));
#109615=DIRECTION('',(4.18005656861881E-16,-1.,0.));
#109616=DIRECTION('center_axis',(-1.,-4.18005656861882E-16,0.));
#109617=DIRECTION('ref_axis',(-4.18005656861882E-16,1.,0.));
#109618=DIRECTION('center_axis',(0.,0.,1.));
#109619=DIRECTION('ref_axis',(1.,0.,0.));
#109620=DIRECTION('center_axis',(0.,0.,-1.));
#109621=DIRECTION('ref_axis',(-1.,0.,0.));
#109622=DIRECTION('center_axis',(-1.,-4.38004274807345E-16,0.));
#109623=DIRECTION('ref_axis',(-4.38004274807345E-16,1.,0.));
#109624=DIRECTION('center_axis',(0.,0.,1.));
#109625=DIRECTION('ref_axis',(1.,0.,0.));
#109626=DIRECTION('',(4.18005656861881E-16,-1.,0.));
#109627=DIRECTION('center_axis',(4.18005656861881E-16,-1.,0.));
#109628=DIRECTION('ref_axis',(-1.,-4.18005656861881E-16,0.));
#109629=DIRECTION('center_axis',(0.,-1.18842113532926E-16,1.));
#109630=DIRECTION('ref_axis',(0.,1.,1.18842113532926E-16));
#109631=DIRECTION('center_axis',(0.,0.,1.));
#109632=DIRECTION('ref_axis',(1.,0.,0.));
#109633=DIRECTION('',(1.,5.01606788234257E-16,0.));
#109634=DIRECTION('center_axis',(1.,5.01606788234257E-16,0.));
#109635=DIRECTION('ref_axis',(5.01606788234257E-16,-1.,0.));
#109636=DIRECTION('',(-1.,-5.01606788234257E-16,0.));
#109637=DIRECTION('center_axis',(5.01606788234257E-16,-1.,5.70122241611331E-32));
#109638=DIRECTION('ref_axis',(-4.59816715307009E-64,-5.70122241611331E-32,
-1.));
#109639=DIRECTION('center_axis',(-4.38004274807345E-16,1.,0.));
#109640=DIRECTION('ref_axis',(1.,4.38004274807345E-16,0.));
#109641=DIRECTION('center_axis',(0.0999814467122865,-0.00101927549405267,
0.994988779530094));
#109642=DIRECTION('ref_axis',(0.648676516536244,0.758334173982988,-0.0644054148650803));
#109643=DIRECTION('center_axis',(-0.742683090861321,0.669643059061075,-1.01363406279984E-15));
#109644=DIRECTION('ref_axis',(-0.669643059061075,-0.742683090861321,-3.71575034000761E-31));
#109645=DIRECTION('center_axis',(0.,1.23467863058847E-16,-1.));
#109646=DIRECTION('ref_axis',(0.,1.,0.));
#109647=DIRECTION('center_axis',(0.,0.,1.));
#109648=DIRECTION('ref_axis',(0.,1.,0.));
#109649=DIRECTION('center_axis',(0.,0.,-1.));
#109650=DIRECTION('ref_axis',(1.,-7.98385375378166E-15,0.));
#109651=DIRECTION('center_axis',(0.,1.23467863058847E-16,-1.));
#109652=DIRECTION('ref_axis',(-1.,0.,0.));
#109653=DIRECTION('center_axis',(0.,0.,-1.));
#109654=DIRECTION('ref_axis',(-1.,0.,0.));
#109655=DIRECTION('center_axis',(-4.38004274807345E-16,1.,0.));
#109656=DIRECTION('ref_axis',(1.,4.38004274807345E-16,0.));
#109657=DIRECTION('center_axis',(0.,1.23467863058847E-16,-1.));
#109658=DIRECTION('ref_axis',(-1.,0.,0.));
#109659=DIRECTION('center_axis',(0.,0.,1.));
#109660=DIRECTION('ref_axis',(1.,0.,0.));
#109661=DIRECTION('',(1.,5.01606788234257E-16,0.));
#109662=DIRECTION('center_axis',(1.,5.01606788234257E-16,0.));
#109663=DIRECTION('ref_axis',(5.01606788234257E-16,-1.,0.));
#109664=DIRECTION('',(-1.,-5.01606788234257E-16,0.));
#109665=DIRECTION('center_axis',(5.01606788234257E-16,-1.,5.70122241611331E-32));
#109666=DIRECTION('ref_axis',(-4.59816715307009E-64,-5.70122241611331E-32,
-1.));
#109667=DIRECTION('center_axis',(0.,0.,-1.));
#109668=DIRECTION('ref_axis',(-1.,0.,0.));
#109669=DIRECTION('center_axis',(0.,-1.18842113532926E-16,1.));
#109670=DIRECTION('ref_axis',(0.,1.,1.18842113532926E-16));
#109671=DIRECTION('center_axis',(0.,-1.18842113532926E-16,1.));
#109672=DIRECTION('ref_axis',(0.,1.,1.18842113532926E-16));
#109673=DIRECTION('center_axis',(0.,0.,1.));
#109674=DIRECTION('ref_axis',(1.,0.,0.));
#109675=DIRECTION('',(4.18005656861881E-16,-1.,0.));
#109676=DIRECTION('center_axis',(4.18005656861881E-16,-1.,0.));
#109677=DIRECTION('ref_axis',(-1.,-4.18005656861881E-16,0.));
#109678=DIRECTION('',(-4.18005656861881E-16,1.,0.));
#109679=DIRECTION('center_axis',(-1.,-4.18005656861882E-16,0.));
#109680=DIRECTION('ref_axis',(-4.18005656861882E-16,1.,0.));
#109681=DIRECTION('center_axis',(-1.,-4.38004274807345E-16,0.));
#109682=DIRECTION('ref_axis',(-4.38004274807345E-16,1.,0.));
#109683=DIRECTION('center_axis',(0.,0.,-1.));
#109684=DIRECTION('ref_axis',(-1.,0.,0.));
#109685=DIRECTION('center_axis',(0.,0.,-1.));
#109686=DIRECTION('ref_axis',(1.,0.,0.));
#109687=DIRECTION('center_axis',(0.,1.23467863058847E-16,-1.));
#109688=DIRECTION('ref_axis',(0.,1.,0.));
#109689=DIRECTION('center_axis',(0.,0.,1.));
#109690=DIRECTION('ref_axis',(0.,1.,0.));
#109691=DIRECTION('center_axis',(0.,1.23467863058847E-16,-1.));
#109692=DIRECTION('ref_axis',(-1.,0.,0.));
#109693=DIRECTION('center_axis',(0.,1.23467863058847E-16,-1.));
#109694=DIRECTION('ref_axis',(0.,1.,0.));
#109695=DIRECTION('center_axis',(0.,0.,1.));
#109696=DIRECTION('ref_axis',(0.,1.,0.));
#109697=DIRECTION('center_axis',(0.,0.,-1.));
#109698=DIRECTION('ref_axis',(1.,0.,0.));
#109699=DIRECTION('center_axis',(0.,0.,-1.));
#109700=DIRECTION('ref_axis',(-1.,0.,0.));
#109701=DIRECTION('center_axis',(-1.,-4.38004274807345E-16,0.));
#109702=DIRECTION('ref_axis',(-4.38004274807345E-16,1.,0.));
#109703=DIRECTION('center_axis',(0.,1.23467863058847E-16,-1.));
#109704=DIRECTION('ref_axis',(-1.,0.,0.));
#109705=DIRECTION('center_axis',(0.,0.,1.));
#109706=DIRECTION('ref_axis',(1.,0.,0.));
#109707=DIRECTION('',(4.18005656861881E-16,-1.,0.));
#109708=DIRECTION('center_axis',(4.18005656861881E-16,-1.,0.));
#109709=DIRECTION('ref_axis',(-1.,-4.18005656861881E-16,0.));
#109710=DIRECTION('',(-4.18005656861881E-16,1.,0.));
#109711=DIRECTION('center_axis',(-1.,-4.18005656861882E-16,0.));
#109712=DIRECTION('ref_axis',(-4.18005656861882E-16,1.,0.));
#109713=DIRECTION('center_axis',(-1.,-4.38004274807345E-16,0.));
#109714=DIRECTION('ref_axis',(-4.38004274807345E-16,1.,0.));
#109715=DIRECTION('center_axis',(0.,0.,-1.));
#109716=DIRECTION('ref_axis',(-1.,0.,0.));
#109717=DIRECTION('center_axis',(0.,0.,-1.));
#109718=DIRECTION('ref_axis',(1.,-1.06649986710964E-14,0.));
#109719=DIRECTION('center_axis',(0.,1.23467863058847E-16,-1.));
#109720=DIRECTION('ref_axis',(0.,1.,0.));
#109721=DIRECTION('center_axis',(0.,0.,1.));
#109722=DIRECTION('ref_axis',(0.,1.,0.));
#109723=DIRECTION('center_axis',(0.,0.,1.));
#109724=DIRECTION('ref_axis',(1.,0.,0.));
#109725=DIRECTION('',(4.18005656861881E-16,-1.,0.));
#109726=DIRECTION('center_axis',(4.18005656861881E-16,-1.,0.));
#109727=DIRECTION('ref_axis',(-1.,-4.18005656861881E-16,0.));
#109728=DIRECTION('',(-4.18005656861881E-16,1.,0.));
#109729=DIRECTION('center_axis',(-1.,-4.18005656861882E-16,0.));
#109730=DIRECTION('ref_axis',(-4.18005656861882E-16,1.,0.));
#109731=DIRECTION('center_axis',(0.,1.23467863058847E-16,-1.));
#109732=DIRECTION('ref_axis',(-1.,0.,0.));
#109733=DIRECTION('center_axis',(0.,0.,1.));
#109734=DIRECTION('ref_axis',(0.,1.,0.));
#109735=DIRECTION('center_axis',(0.,1.23467863058847E-16,-1.));
#109736=DIRECTION('ref_axis',(0.,1.,0.));
#109737=DIRECTION('center_axis',(0.,0.,-1.));
#109738=DIRECTION('ref_axis',(1.,0.,0.));
#109739=DIRECTION('center_axis',(0.,0.,-1.));
#109740=DIRECTION('ref_axis',(-1.,0.,0.));
#109741=DIRECTION('center_axis',(-1.,-4.38004274807345E-16,0.));
#109742=DIRECTION('ref_axis',(-4.38004274807345E-16,1.,0.));
#109743=DIRECTION('center_axis',(0.,-1.18842113532926E-16,1.));
#109744=DIRECTION('ref_axis',(0.,1.,1.18842113532926E-16));
#109745=DIRECTION('center_axis',(0.,0.,1.));
#109746=DIRECTION('ref_axis',(1.,0.,0.));
#109747=DIRECTION('',(4.18005656861881E-16,-1.,0.));
#109748=DIRECTION('center_axis',(4.18005656861881E-16,-1.,0.));
#109749=DIRECTION('ref_axis',(-1.,-4.18005656861881E-16,0.));
#109750=DIRECTION('',(-4.18005656861881E-16,1.,0.));
#109751=DIRECTION('center_axis',(-1.,-4.18005656861882E-16,0.));
#109752=DIRECTION('ref_axis',(-4.18005656861882E-16,1.,0.));
#109753=DIRECTION('center_axis',(0.,1.23467863058847E-16,-1.));
#109754=DIRECTION('ref_axis',(-1.,0.,0.));
#109755=DIRECTION('center_axis',(0.,1.23467863058847E-16,-1.));
#109756=DIRECTION('ref_axis',(-1.,0.,0.));
#109757=DIRECTION('center_axis',(0.,0.,-1.));
#109758=DIRECTION('ref_axis',(0.,1.,0.));
#109759=DIRECTION('',(1.,-4.18005656861881E-16,-5.16102651992463E-32));
#109760=DIRECTION('',(0.139173100960065,0.99026806874157,1.22266282302933E-16));
#109761=DIRECTION('center_axis',(1.,-4.18005656861882E-16,0.));
#109762=DIRECTION('ref_axis',(-4.18005656861882E-16,-1.,0.));
#109763=DIRECTION('',(-4.18005656861881E-16,-1.,0.));
#109764=DIRECTION('',(0.,0.,-1.));
#109765=DIRECTION('',(4.18005656861881E-16,1.,0.));
#109766=DIRECTION('',(0.,0.,1.));
#109767=DIRECTION('center_axis',(-4.18005656861881E-16,-1.,0.));
#109768=DIRECTION('ref_axis',(1.,-4.18005656861881E-16,0.));
#109769=DIRECTION('center_axis',(0.,1.,0.));
#109770=DIRECTION('ref_axis',(-1.,0.,0.));
#109771=DIRECTION('',(-4.18005656861881E-16,-1.,0.));
#109772=DIRECTION('center_axis',(0.,-1.,0.));
#109773=DIRECTION('ref_axis',(1.,0.,0.));
#109774=DIRECTION('center_axis',(0.,0.,1.));
#109775=DIRECTION('ref_axis',(1.,0.,0.));
#109776=DIRECTION('',(-1.,4.18005656861881E-16,0.));
#109777=DIRECTION('',(0.139173100960065,0.99026806874157,0.));
#109778=DIRECTION('',(1.,-4.18005656861881E-16,0.));
#109779=DIRECTION('center_axis',(0.,-1.18842113532926E-16,1.));
#109780=DIRECTION('ref_axis',(0.,1.,1.18842113532926E-16));
#109781=DIRECTION('center_axis',(0.,1.19392659184112E-16,-1.));
#109782=DIRECTION('ref_axis',(0.,1.,1.19392659184112E-16));
#109783=DIRECTION('center_axis',(1.,-4.38004274807345E-16,0.));
#109784=DIRECTION('ref_axis',(-4.38004274807345E-16,-1.,0.));
#109785=DIRECTION('',(0.,0.,1.));
#109786=DIRECTION('',(0.,0.,-1.));
#109787=DIRECTION('center_axis',(0.,0.,-1.));
#109788=DIRECTION('ref_axis',(1.,0.,0.));
#109789=DIRECTION('center_axis',(0.,0.,1.));
#109790=DIRECTION('ref_axis',(-1.,0.,0.));
#109791=DIRECTION('center_axis',(0.,1.23467863058847E-16,-1.));
#109792=DIRECTION('ref_axis',(0.,1.,0.));
#109793=DIRECTION('center_axis',(0.,0.,-1.));
#109794=DIRECTION('ref_axis',(0.,1.,0.));
#109795=DIRECTION('center_axis',(0.,1.23467863058847E-16,-1.));
#109796=DIRECTION('ref_axis',(-1.,0.,0.));
#109797=DIRECTION('',(0.139173100960065,0.99026806874157,1.22266282302933E-16));
#109798=DIRECTION('',(-1.,4.18005656861881E-16,5.16102651992463E-32));
#109799=DIRECTION('',(1.,-4.18005656861881E-16,-5.16102651992463E-32));
#109800=DIRECTION('center_axis',(1.,-4.18005656861882E-16,0.));
#109801=DIRECTION('ref_axis',(-4.18005656861882E-16,-1.,0.));
#109802=DIRECTION('',(-4.18005656861881E-16,-1.,0.));
#109803=DIRECTION('',(0.,0.,-1.));
#109804=DIRECTION('',(4.18005656861881E-16,1.,0.));
#109805=DIRECTION('',(0.,0.,1.));
#109806=DIRECTION('center_axis',(-4.18005656861881E-16,-1.,0.));
#109807=DIRECTION('ref_axis',(1.,-4.18005656861881E-16,0.));
#109808=DIRECTION('center_axis',(0.,1.,0.));
#109809=DIRECTION('ref_axis',(-1.,0.,0.));
#109810=DIRECTION('',(-4.18005656861881E-16,-1.,0.));
#109811=DIRECTION('center_axis',(0.,-1.,0.));
#109812=DIRECTION('ref_axis',(1.,0.,0.));
#109813=DIRECTION('center_axis',(0.,0.,1.));
#109814=DIRECTION('ref_axis',(1.,0.,0.));
#109815=DIRECTION('',(-1.,4.38004274807345E-16,0.));
#109816=DIRECTION('',(0.139173100960065,0.99026806874157,0.));
#109817=DIRECTION('',(1.,-4.18005656861881E-16,0.));
#109818=DIRECTION('center_axis',(0.,1.23467863058847E-16,-1.));
#109819=DIRECTION('ref_axis',(0.,1.,0.));
#109820=DIRECTION('center_axis',(0.214612320896177,0.976699255456037,-0.000340750905301442));
#109821=DIRECTION('ref_axis',(-0.880441023637846,0.193310232164562,-0.432960457820371));
#109822=DIRECTION('center_axis',(0.,0.,1.));
#109823=DIRECTION('ref_axis',(-1.,-1.06649986710964E-14,0.));
#109824=DIRECTION('center_axis',(0.,0.,-1.));
#109825=DIRECTION('ref_axis',(1.,0.,0.));
#109826=DIRECTION('center_axis',(1.,-4.38004274807345E-16,0.));
#109827=DIRECTION('ref_axis',(-4.38004274807345E-16,-1.,0.));
#109828=DIRECTION('',(0.,0.,1.));
#109829=DIRECTION('',(0.,0.,-1.));
#109830=DIRECTION('center_axis',(1.,-4.18005656861882E-16,0.));
#109831=DIRECTION('ref_axis',(-4.18005656861882E-16,-1.,0.));
#109832=DIRECTION('',(-4.18005656861881E-16,-1.,0.));
#109833=DIRECTION('',(0.,0.,-1.));
#109834=DIRECTION('',(4.18005656861881E-16,1.,0.));
#109835=DIRECTION('',(0.,0.,1.));
#109836=DIRECTION('center_axis',(-4.18005656861881E-16,-1.,0.));
#109837=DIRECTION('ref_axis',(1.,-4.18005656861881E-16,0.));
#109838=DIRECTION('center_axis',(0.,1.,0.));
#109839=DIRECTION('ref_axis',(-1.,0.,0.));
#109840=DIRECTION('',(-4.18005656861881E-16,-1.,0.));
#109841=DIRECTION('center_axis',(0.,-1.,0.));
#109842=DIRECTION('ref_axis',(1.,0.,0.));
#109843=DIRECTION('center_axis',(0.,0.,1.));
#109844=DIRECTION('ref_axis',(1.,0.,0.));
#109845=DIRECTION('',(-1.,4.18005656861881E-16,0.));
#109846=DIRECTION('',(-0.139173100960067,0.99026806874157,0.));
#109847=DIRECTION('',(1.,-4.18005656861881E-16,0.));
#109848=DIRECTION('center_axis',(0.,1.23467863058847E-16,-1.));
#109849=DIRECTION('ref_axis',(-1.,0.,0.));
#109850=DIRECTION('',(-0.139173100960067,0.99026806874157,1.22266282302933E-16));
#109851=DIRECTION('',(-1.,4.18005656861881E-16,5.16102651992463E-32));
#109852=DIRECTION('center_axis',(0.,0.,-1.));
#109853=DIRECTION('ref_axis',(0.,1.,0.));
#109854=DIRECTION('center_axis',(1.,-4.38004274807345E-16,0.));
#109855=DIRECTION('ref_axis',(-4.38004274807345E-16,-1.,0.));
#109856=DIRECTION('',(0.,0.,1.));
#109857=DIRECTION('',(0.,0.,-1.));
#109858=DIRECTION('center_axis',(0.,0.,-1.));
#109859=DIRECTION('ref_axis',(1.,0.,0.));
#109860=DIRECTION('center_axis',(0.,0.,1.));
#109861=DIRECTION('ref_axis',(-1.,0.,0.));
#109862=DIRECTION('center_axis',(0.,1.23467863058847E-16,-1.));
#109863=DIRECTION('ref_axis',(0.,1.,0.));
#109864=DIRECTION('center_axis',(0.212854559998133,-0.977083829553736,-0.000355404849016026));
#109865=DIRECTION('ref_axis',(-0.773913504202019,-0.168372497077826,-0.610498640654939));
#109866=DIRECTION('center_axis',(0.,1.23467863058847E-16,-1.));
#109867=DIRECTION('ref_axis',(-1.,0.,0.));
#109868=DIRECTION('',(-0.139173100960067,0.99026806874157,1.22266282302933E-16));
#109869=DIRECTION('',(-1.,4.18005656861881E-16,5.16102651992463E-32));
#109870=DIRECTION('center_axis',(0.,0.,-1.));
#109871=DIRECTION('ref_axis',(0.,1.,0.));
#109872=DIRECTION('',(1.,-4.18005656861881E-16,-5.16102651992463E-32));
#109873=DIRECTION('center_axis',(0.,1.23467863058847E-16,-1.));
#109874=DIRECTION('ref_axis',(0.,1.,0.));
#109875=DIRECTION('center_axis',(0.,0.,1.));
#109876=DIRECTION('ref_axis',(-1.,0.,0.));
#109877=DIRECTION('center_axis',(0.,0.,-1.));
#109878=DIRECTION('ref_axis',(1.,0.,0.));
#109879=DIRECTION('center_axis',(1.,-4.38004274807345E-16,0.));
#109880=DIRECTION('ref_axis',(-4.38004274807345E-16,-1.,0.));
#109881=DIRECTION('',(0.,0.,1.));
#109882=DIRECTION('',(0.,0.,-1.));
#109883=DIRECTION('center_axis',(1.,-4.18005656861882E-16,0.));
#109884=DIRECTION('ref_axis',(-4.18005656861882E-16,-1.,0.));
#109885=DIRECTION('',(4.18005656861881E-16,1.,0.));
#109886=DIRECTION('',(0.,0.,1.));
#109887=DIRECTION('',(-4.18005656861881E-16,-1.,0.));
#109888=DIRECTION('',(0.,0.,-1.));
#109889=DIRECTION('center_axis',(-4.18005656861881E-16,-1.,0.));
#109890=DIRECTION('ref_axis',(1.,-4.18005656861881E-16,0.));
#109891=DIRECTION('',(-4.18005656861881E-16,-1.,0.));
#109892=DIRECTION('center_axis',(0.,-1.,0.));
#109893=DIRECTION('ref_axis',(1.,0.,0.));
#109894=DIRECTION('center_axis',(0.,1.,0.));
#109895=DIRECTION('ref_axis',(-1.,0.,0.));
#109896=DIRECTION('center_axis',(0.,0.,1.));
#109897=DIRECTION('ref_axis',(1.,0.,0.));
#109898=DIRECTION('',(-1.,4.18005656861881E-16,0.));
#109899=DIRECTION('',(-0.139173100960067,0.99026806874157,0.));
#109900=DIRECTION('',(1.,-4.38004274807345E-16,0.));
#109901=DIRECTION('center_axis',(0.,-1.18842113532926E-16,1.));
#109902=DIRECTION('ref_axis',(0.,1.,1.18842113532926E-16));
#109903=DIRECTION('center_axis',(0.,1.19392659184112E-16,-1.));
#109904=DIRECTION('ref_axis',(0.,1.,1.19392659184112E-16));
#109905=DIRECTION('center_axis',(0.,-1.18842113532926E-16,1.));
#109906=DIRECTION('ref_axis',(0.,1.,1.18842113532926E-16));
#109907=DIRECTION('center_axis',(0.,1.19392659184112E-16,-1.));
#109908=DIRECTION('ref_axis',(0.,1.,1.19392659184112E-16));
#109909=DIRECTION('center_axis',(0.,0.,-1.));
#109910=DIRECTION('ref_axis',(1.,0.,0.));
#109911=DIRECTION('center_axis',(0.,0.,1.));
#109912=DIRECTION('ref_axis',(-1.,-7.98385375378166E-15,0.));
#109913=DIRECTION('center_axis',(-5.01606788234257E-16,-1.,5.70122241611331E-32));
#109914=DIRECTION('ref_axis',(-1.,5.01606788234257E-16,0.));
#109915=DIRECTION('',(-1.,5.01606788234257E-16,0.));
#109916=DIRECTION('',(-2.85977186515575E-47,-5.70122241611331E-32,-1.));
#109917=DIRECTION('',(1.,-5.01606788234257E-16,0.));
#109918=DIRECTION('',(2.85977186515575E-47,5.70122241611331E-32,1.));
#109919=DIRECTION('center_axis',(-1.,5.01606788234257E-16,0.));
#109920=DIRECTION('ref_axis',(-5.01606788234257E-16,-1.,0.));
#109921=DIRECTION('center_axis',(1.,0.,0.));
#109922=DIRECTION('ref_axis',(0.,1.,0.));
#109923=DIRECTION('',(-1.,5.01606788234257E-16,0.));
#109924=DIRECTION('center_axis',(-1.,0.,0.));
#109925=DIRECTION('ref_axis',(0.,-1.,0.));
#109926=DIRECTION('center_axis',(0.,0.,1.));
#109927=DIRECTION('ref_axis',(1.,0.,0.));
#109928=DIRECTION('',(5.01606788234257E-16,1.,0.));
#109929=DIRECTION('',(0.990268068741571,0.139173100960059,0.));
#109930=DIRECTION('',(-5.01606788234257E-16,-1.,0.));
#109931=DIRECTION('center_axis',(0.,1.23467863058847E-16,-1.));
#109932=DIRECTION('ref_axis',(-1.,0.,0.));
#109933=DIRECTION('',(0.990268068741571,0.139173100960059,1.71834053708117E-17));
#109934=DIRECTION('',(5.01606788234257E-16,1.,1.23467863058847E-16));
#109935=DIRECTION('center_axis',(0.,0.,-1.));
#109936=DIRECTION('ref_axis',(0.,1.,0.));
#109937=DIRECTION('center_axis',(4.38004274807345E-16,1.,0.));
#109938=DIRECTION('ref_axis',(1.,-4.38004274807345E-16,0.));
#109939=DIRECTION('',(0.,0.,1.));
#109940=DIRECTION('',(0.,0.,-1.));
#109941=DIRECTION('center_axis',(0.,0.,-1.));
#109942=DIRECTION('ref_axis',(1.,0.,0.));
#109943=DIRECTION('center_axis',(0.,0.,1.));
#109944=DIRECTION('ref_axis',(-1.,8.87756872621991E-15,0.));
#109945=DIRECTION('center_axis',(0.,-1.,0.));
#109946=DIRECTION('ref_axis',(0.,0.,-1.));
#109947=DIRECTION('center_axis',(0.,0.,1.));
#109948=DIRECTION('ref_axis',(0.,1.,0.));
#109949=DIRECTION('center_axis',(-1.,0.,0.));
#109950=DIRECTION('ref_axis',(0.,0.,1.));
#109951=DIRECTION('center_axis',(0.,0.,-1.));
#109952=DIRECTION('ref_axis',(0.,1.,0.));
#109953=DIRECTION('center_axis',(0.,1.23467863058847E-16,-1.));
#109954=DIRECTION('ref_axis',(-1.,0.,0.));
#109955=DIRECTION('',(0.990268068741571,0.139173100960059,1.71834053708117E-17));
#109956=DIRECTION('',(5.01606788234257E-16,1.,1.23467863058847E-16));
#109957=DIRECTION('center_axis',(0.,0.,-1.));
#109958=DIRECTION('ref_axis',(0.,1.,0.));
#109959=DIRECTION('',(-5.01606788234257E-16,-1.,-1.23467863058847E-16));
#109960=DIRECTION('center_axis',(0.,1.23467863058847E-16,-1.));
#109961=DIRECTION('ref_axis',(0.,1.,0.));
#109962=DIRECTION('center_axis',(0.952430221804268,0.304711142119182,0.00527185567859643));
#109963=DIRECTION('ref_axis',(0.0463243094405771,-0.161849302626711,0.985727579807982));
#109964=DIRECTION('center_axis',(-0.742683090861321,-0.669643059061075,
1.01363406279984E-15));
#109965=DIRECTION('ref_axis',(0.669643059061075,-0.742683090861321,-3.71575034000761E-31));
#109966=DIRECTION('center_axis',(0.0999814466925417,0.0010192755153814,
-0.994988779532056));
#109967=DIRECTION('ref_axis',(-0.648676516538678,0.75833417398337,-0.0644054148360687));
#109968=DIRECTION('center_axis',(4.38004274807345E-16,1.,0.));
#109969=DIRECTION('ref_axis',(1.,-4.38004274807345E-16,0.));
#109970=DIRECTION('',(-1.13659195805196E-16,4.9783213633841E-32,1.));
#109971=DIRECTION('',(0.,0.,-1.));
#109972=DIRECTION('center_axis',(-5.01606788234257E-16,-1.,5.70122241611331E-32));
#109973=DIRECTION('ref_axis',(-1.,5.01606788234257E-16,0.));
#109974=DIRECTION('',(1.,-5.01606788234257E-16,0.));
#109975=DIRECTION('',(1.13659195805196E-16,0.,1.));
#109976=DIRECTION('',(-1.,5.01606788234257E-16,0.));
#109977=DIRECTION('',(1.13659195805196E-16,-1.14024448322266E-31,-1.));
#109978=DIRECTION('center_axis',(-1.,5.01606788234257E-16,0.));
#109979=DIRECTION('ref_axis',(-5.01606788234257E-16,-1.,0.));
#109980=DIRECTION('',(-1.,5.01606788234257E-16,0.));
#109981=DIRECTION('center_axis',(-1.,0.,1.13659195805196E-16));
#109982=DIRECTION('ref_axis',(0.,-1.,0.));
#109983=DIRECTION('center_axis',(1.,0.,1.13659195805196E-16));
#109984=DIRECTION('ref_axis',(0.,1.,0.));
#109985=DIRECTION('center_axis',(0.,0.,1.));
#109986=DIRECTION('ref_axis',(1.,0.,0.));
#109987=DIRECTION('',(5.01606788234257E-16,1.,0.));
#109988=DIRECTION('',(0.990268068741571,0.139173100960059,0.));
#109989=DIRECTION('',(-4.38004274807345E-16,-1.,0.));
#109990=DIRECTION('center_axis',(0.,-1.18842113532926E-16,1.));
#109991=DIRECTION('ref_axis',(0.,1.,1.18842113532926E-16));
#109992=DIRECTION('center_axis',(0.,1.19392659184112E-16,-1.));
#109993=DIRECTION('ref_axis',(0.,1.,1.19392659184112E-16));
#109994=DIRECTION('center_axis',(-4.18005656861881E-16,-1.,0.));
#109995=DIRECTION('ref_axis',(1.,-4.18005656861881E-16,0.));
#109996=DIRECTION('',(4.18005656861881E-16,1.,0.));
#109997=DIRECTION('center_axis',(5.78241158658935E-16,1.,0.));
#109998=DIRECTION('ref_axis',(-1.,5.78241158658935E-16,0.));
#109999=DIRECTION('',(-4.18005656861881E-16,-1.,0.));
#110000=DIRECTION('center_axis',(-5.78241158658935E-16,-1.,0.));
#110001=DIRECTION('ref_axis',(1.,-5.78241158658935E-16,0.));
#110002=DIRECTION('center_axis',(0.,0.,1.));
#110003=DIRECTION('ref_axis',(1.,0.,0.));
#110004=DIRECTION('',(-1.,4.18005656861881E-16,0.));
#110005=DIRECTION('center_axis',(0.,0.,1.));
#110006=DIRECTION('ref_axis',(1.,0.,0.));
#110007=DIRECTION('',(1.,-4.18005656861881E-16,0.));
#110008=DIRECTION('center_axis',(1.,-4.38004274807345E-16,0.));
#110009=DIRECTION('ref_axis',(-4.38004274807345E-16,-1.,0.));
#110010=DIRECTION('',(0.,0.,1.));
#110011=DIRECTION('',(0.,0.,-1.));
#110012=DIRECTION('center_axis',(0.,0.,-1.));
#110013=DIRECTION('ref_axis',(1.,0.,0.));
#110014=DIRECTION('center_axis',(0.,0.,1.));
#110015=DIRECTION('ref_axis',(0.,-1.,0.));
#110016=DIRECTION('center_axis',(0.,0.,1.));
#110017=DIRECTION('ref_axis',(1.,0.,0.));
#110018=DIRECTION('',(-1.,4.18005656861881E-16,0.));
#110019=DIRECTION('center_axis',(0.,0.,1.));
#110020=DIRECTION('ref_axis',(1.,0.,0.));
#110021=DIRECTION('',(1.,-4.18005656861881E-16,0.));
#110022=DIRECTION('',(-4.18005656861881E-16,-1.,0.));
#110023=DIRECTION('center_axis',(1.,-4.18005656861882E-16,0.));
#110024=DIRECTION('ref_axis',(-4.18005656861882E-16,-1.,0.));
#110025=DIRECTION('',(-4.18005656861881E-16,-1.,0.));
#110026=DIRECTION('',(0.,0.,-1.));
#110027=DIRECTION('',(4.18005656861881E-16,1.,0.));
#110028=DIRECTION('',(0.,0.,1.));
#110029=DIRECTION('center_axis',(-4.18005656861881E-16,-1.,0.));
#110030=DIRECTION('ref_axis',(1.,-4.18005656861881E-16,0.));
#110031=DIRECTION('center_axis',(4.33680868994202E-16,1.,0.));
#110032=DIRECTION('ref_axis',(-1.,4.33680868994202E-16,0.));
#110033=DIRECTION('center_axis',(-4.33680868994202E-16,-1.,0.));
#110034=DIRECTION('ref_axis',(1.,-4.33680868994202E-16,0.));
#110035=DIRECTION('center_axis',(1.,0.,0.));
#110036=DIRECTION('ref_axis',(0.,1.,0.));
#110037=DIRECTION('center_axis',(-1.,0.,0.));
#110038=DIRECTION('ref_axis',(0.,0.,1.));
#110039=DIRECTION('center_axis',(1.,-4.38004274807345E-16,0.));
#110040=DIRECTION('ref_axis',(-4.38004274807345E-16,-1.,0.));
#110041=DIRECTION('',(0.,0.,-1.));
#110042=DIRECTION('',(0.,0.,1.));
#110043=DIRECTION('center_axis',(0.,0.,-1.));
#110044=DIRECTION('ref_axis',(1.,0.,0.));
#110045=DIRECTION('center_axis',(0.,0.,1.));
#110046=DIRECTION('ref_axis',(0.,-1.,0.));
#110047=DIRECTION('center_axis',(-0.149968574026289,-0.0101861056380938,
0.988638290810371));
#110048=DIRECTION('ref_axis',(0.981228608534593,0.121089848369309,0.150092193052014));
#110049=DIRECTION('center_axis',(1.,-4.38004274807345E-16,0.));
#110050=DIRECTION('ref_axis',(-4.38004274807345E-16,-1.,0.));
#110051=DIRECTION('',(0.,0.,1.));
#110052=DIRECTION('',(0.,0.,-1.));
#110053=DIRECTION('center_axis',(-0.00252744588198969,-0.999981530022895,
0.00552735292733838));
#110054=DIRECTION('ref_axis',(0.976049181036949,-0.00126447960099768,0.217546310675312));
#110055=DIRECTION('center_axis',(0.,0.,-1.));
#110056=DIRECTION('ref_axis',(1.,0.,0.));
#110057=DIRECTION('center_axis',(0.,0.,1.));
#110058=DIRECTION('ref_axis',(0.,-1.,0.));
#110059=DIRECTION('center_axis',(-0.0216109392502409,2.83714134350443E-8,
0.99976645638105));
#110060=DIRECTION('ref_axis',(0.999764411688039,0.00202245879910768,0.021610894994789));
#110061=DIRECTION('center_axis',(1.,0.,0.));
#110062=DIRECTION('ref_axis',(0.,0.00139138517159681,-0.999999032023184));
#110063=DIRECTION('center_axis',(1.,-4.38004274807345E-16,0.));
#110064=DIRECTION('ref_axis',(-4.38004274807345E-16,-1.,0.));
#110065=DIRECTION('',(0.,0.,1.));
#110066=DIRECTION('',(0.,0.,-1.));
#110067=DIRECTION('center_axis',(-0.00301392117783963,0.999973599253448,
0.00661188893112461));
#110068=DIRECTION('ref_axis',(0.976327184229521,0.00151250353879502,0.216293646849601));
#110069=DIRECTION('center_axis',(0.,0.,-1.));
#110070=DIRECTION('ref_axis',(1.,0.,0.));
#110071=DIRECTION('center_axis',(0.,0.,1.));
#110072=DIRECTION('ref_axis',(0.,-1.,0.));
#110073=DIRECTION('center_axis',(-0.157518537373542,0.0111023184919509,
0.987453618610922));
#110074=DIRECTION('ref_axis',(0.98052929088236,-0.116977821119357,0.157729195420202));
#110075=DIRECTION('center_axis',(1.,-4.38004274807345E-16,0.));
#110076=DIRECTION('ref_axis',(-4.38004274807345E-16,-1.,0.));
#110077=DIRECTION('',(0.,0.,1.));
#110078=DIRECTION('',(0.,0.,-1.));
#110079=DIRECTION('center_axis',(0.,0.,-1.));
#110080=DIRECTION('ref_axis',(1.,0.,0.));
#110081=DIRECTION('center_axis',(0.,0.,1.));
#110082=DIRECTION('ref_axis',(0.,-1.,0.));
#110083=DIRECTION('center_axis',(1.,0.,0.));
#110084=DIRECTION('ref_axis',(0.,1.,0.));
#110085=DIRECTION('',(1.,-4.18005656861881E-16,0.));
#110086=DIRECTION('center_axis',(1.,0.,0.));
#110087=DIRECTION('ref_axis',(0.,0.,-1.));
#110088=DIRECTION('center_axis',(1.,-4.18005656861882E-16,0.));
#110089=DIRECTION('ref_axis',(-4.18005656861882E-16,-1.,0.));
#110090=DIRECTION('',(-4.18005656861881E-16,-1.,0.));
#110091=DIRECTION('',(0.,0.,-1.));
#110092=DIRECTION('',(4.18005656861881E-16,1.,0.));
#110093=DIRECTION('',(0.,0.,1.));
#110094=DIRECTION('center_axis',(-4.18005656861881E-16,-1.,0.));
#110095=DIRECTION('ref_axis',(1.,-4.18005656861881E-16,0.));
#110096=DIRECTION('center_axis',(0.,1.,0.));
#110097=DIRECTION('ref_axis',(-1.,0.,0.));
#110098=DIRECTION('',(-4.18005656861881E-16,-1.,0.));
#110099=DIRECTION('center_axis',(0.,-1.,0.));
#110100=DIRECTION('ref_axis',(1.,0.,0.));
#110101=DIRECTION('center_axis',(0.,0.,1.));
#110102=DIRECTION('ref_axis',(1.,0.,0.));
#110103=DIRECTION('',(-1.,4.18005656861881E-16,0.));
#110104=DIRECTION('center_axis',(0.,0.,1.));
#110105=DIRECTION('ref_axis',(1.,0.,0.));
#110106=DIRECTION('center_axis',(-4.18005656861881E-16,-1.,0.));
#110107=DIRECTION('ref_axis',(1.,-4.18005656861881E-16,0.));
#110108=DIRECTION('',(4.18005656861881E-16,1.,0.));
#110109=DIRECTION('center_axis',(0.,1.,0.));
#110110=DIRECTION('ref_axis',(-1.,0.,0.));
#110111=DIRECTION('',(-4.18005656861881E-16,-1.,0.));
#110112=DIRECTION('center_axis',(0.,-1.,0.));
#110113=DIRECTION('ref_axis',(1.,0.,0.));
#110114=DIRECTION('center_axis',(1.,-4.38004274807345E-16,0.));
#110115=DIRECTION('ref_axis',(-4.38004274807345E-16,-1.,0.));
#110116=DIRECTION('',(0.,0.,-1.));
#110117=DIRECTION('',(0.,0.,1.));
#110118=DIRECTION('center_axis',(0.,0.,-1.));
#110119=DIRECTION('ref_axis',(1.,0.,0.));
#110120=DIRECTION('center_axis',(0.,0.,1.));
#110121=DIRECTION('ref_axis',(0.,-1.,0.));
#110122=DIRECTION('center_axis',(0.,0.,1.));
#110123=DIRECTION('ref_axis',(1.,0.,0.));
#110124=DIRECTION('',(-1.,4.18005656861881E-16,0.));
#110125=DIRECTION('center_axis',(0.,0.,1.));
#110126=DIRECTION('ref_axis',(1.,0.,0.));
#110127=DIRECTION('',(1.,-4.18005656861881E-16,0.));
#110128=DIRECTION('center_axis',(1.,-4.18005656861882E-16,0.));
#110129=DIRECTION('ref_axis',(-4.18005656861882E-16,-1.,0.));
#110130=DIRECTION('',(-4.18005656861881E-16,-1.,0.));
#110131=DIRECTION('',(0.,0.,-1.));
#110132=DIRECTION('',(0.,0.,1.));
#110133=DIRECTION('center_axis',(1.,-4.18005656861882E-16,0.));
#110134=DIRECTION('ref_axis',(-4.18005656861882E-16,-1.,0.));
#110135=DIRECTION('',(-4.18005656861881E-16,-1.,0.));
#110136=DIRECTION('',(0.,0.,-1.));
#110137=DIRECTION('',(0.,0.,1.));
#110138=DIRECTION('center_axis',(4.38004274807345E-16,1.,0.));
#110139=DIRECTION('ref_axis',(1.,-4.38004274807345E-16,0.));
#110140=DIRECTION('',(0.,0.,1.));
#110141=DIRECTION('',(0.,0.,-1.));
#110142=DIRECTION('center_axis',(-5.01606788234257E-16,-1.,5.70122241611331E-32));
#110143=DIRECTION('ref_axis',(-1.,5.01606788234257E-16,0.));
#110144=DIRECTION('',(-1.,5.01606788234257E-16,0.));
#110145=DIRECTION('',(-2.85977186515575E-47,-5.70122241611331E-32,-1.));
#110146=DIRECTION('',(1.,-5.01606788234257E-16,0.));
#110147=DIRECTION('',(2.85977186515575E-47,5.70122241611331E-32,1.));
#110148=DIRECTION('center_axis',(4.38004274807345E-16,1.,0.));
#110149=DIRECTION('ref_axis',(1.,-4.38004274807345E-16,0.));
#110150=DIRECTION('',(0.,0.,1.));
#110151=DIRECTION('',(0.,0.,-1.));
#110152=DIRECTION('center_axis',(4.38004274807345E-16,1.,0.));
#110153=DIRECTION('ref_axis',(1.,-4.38004274807345E-16,0.));
#110154=DIRECTION('',(0.,0.,1.));
#110155=DIRECTION('',(0.,0.,-1.));
#110156=DIRECTION('center_axis',(-1.,5.01606788234257E-16,0.));
#110157=DIRECTION('ref_axis',(-5.01606788234257E-16,-1.,0.));
#110158=DIRECTION('',(1.,-5.01606788234257E-16,0.));
#110159=DIRECTION('center_axis',(1.,0.,0.));
#110160=DIRECTION('ref_axis',(0.,1.,0.));
#110161=DIRECTION('',(-1.,5.01606788234257E-16,0.));
#110162=DIRECTION('center_axis',(-1.,0.,0.));
#110163=DIRECTION('ref_axis',(0.,-1.,0.));
#110164=DIRECTION('center_axis',(0.,1.23467863058847E-16,-1.));
#110165=DIRECTION('ref_axis',(0.,1.,0.));
#110166=DIRECTION('center_axis',(-0.976893716583792,-0.213725378195426,
-0.000359463945942464));
#110167=DIRECTION('ref_axis',(-0.169779058278416,0.777043764862974,-0.606117198945607));
#110168=DIRECTION('center_axis',(-0.999980560004511,0.00244828575950157,
0.00573458890456878));
#110169=DIRECTION('ref_axis',(-0.00114118854494862,-0.976015867166676,0.217696404948694));
#110170=DIRECTION('center_axis',(-1.,5.01606788234257E-16,0.));
#110171=DIRECTION('ref_axis',(-5.01606788234257E-16,-1.,0.));
#110172=DIRECTION('center_axis',(1.,0.,0.));
#110173=DIRECTION('ref_axis',(0.,1.,0.));
#110174=DIRECTION('',(-1.,5.01606788234257E-16,0.));
#110175=DIRECTION('center_axis',(-1.,0.,0.));
#110176=DIRECTION('ref_axis',(0.,-1.,0.));
#110177=DIRECTION('center_axis',(0.,-1.,0.));
#110178=DIRECTION('ref_axis',(0.,0.,-1.));
#110179=DIRECTION('center_axis',(0.,0.,1.));
#110180=DIRECTION('ref_axis',(0.,1.,0.));
#110181=DIRECTION('center_axis',(-1.,0.,0.));
#110182=DIRECTION('ref_axis',(0.,0.,1.));
#110183=DIRECTION('center_axis',(0.,0.,-1.));
#110184=DIRECTION('ref_axis',(0.,1.,0.));
#110185=DIRECTION('center_axis',(-0.990268068741571,-0.139173100960059,
0.));
#110186=DIRECTION('ref_axis',(0.139173100960059,-0.990268068741571,0.));
#110187=DIRECTION('center_axis',(-0.939797023107103,-0.132079858078289,
0.315176881209658));
#110188=DIRECTION('ref_axis',(0.317962525883615,-4.30796627806664E-16,0.948103281364278));
#110189=DIRECTION('center_axis',(0.990268068741571,0.139173100960059,1.71834053708117E-17));
#110190=DIRECTION('ref_axis',(-0.139173100960059,0.990268068741571,-4.14246685971564E-34));
#110191=DIRECTION('',(-0.990268068741571,-0.139173100960059,-1.71834053708117E-17));
#110192=DIRECTION('center_axis',(-0.990268068741572,-0.139173100960051,
-1.37427301308497E-14));
#110193=DIRECTION('ref_axis',(0.139173100960051,-0.990268068741572,1.93598700157835E-30));
#110194=DIRECTION('center_axis',(0.,0.,-1.));
#110195=DIRECTION('ref_axis',(-1.,0.,0.));
#110196=DIRECTION('center_axis',(-0.990268068741572,-0.139173100960051,
0.));
#110197=DIRECTION('ref_axis',(0.139173100960051,-0.990268068741572,0.));
#110198=DIRECTION('',(-0.990268068741571,-0.139173100960059,0.));
#110199=DIRECTION('center_axis',(-0.990268068741572,-0.139173100960051,
0.));
#110200=DIRECTION('ref_axis',(0.139173100960051,-0.990268068741572,0.));
#110201=DIRECTION('center_axis',(0.,0.,-1.));
#110202=DIRECTION('ref_axis',(-1.,0.,0.));
#110203=DIRECTION('center_axis',(0.990268068741571,0.139173100960059,1.71834053708117E-17));
#110204=DIRECTION('ref_axis',(-0.139173100960059,0.990268068741571,-4.14246685971564E-34));
#110205=DIRECTION('',(-0.990268068741571,-0.139173100960059,-1.71834053708117E-17));
#110206=DIRECTION('center_axis',(0.,0.,1.));
#110207=DIRECTION('ref_axis',(1.,0.,0.));
#110208=DIRECTION('center_axis',(-0.990268068741572,-0.139173100960051,
0.));
#110209=DIRECTION('ref_axis',(0.139173100960051,-0.990268068741572,0.));
#110210=DIRECTION('center_axis',(-0.990268068741572,-0.139173100960051,
0.));
#110211=DIRECTION('ref_axis',(0.139173100960051,-0.990268068741572,0.));
#110212=DIRECTION('',(-0.990268068741571,-0.139173100960059,0.));
#110213=DIRECTION('center_axis',(-0.990268068741571,-0.139173100960064,
0.));
#110214=DIRECTION('ref_axis',(0.139173100960064,-0.990268068741571,0.));
#110215=DIRECTION('center_axis',(0.,0.,-1.));
#110216=DIRECTION('ref_axis',(-1.,0.,0.));
#110217=DIRECTION('center_axis',(0.990268068741571,0.139173100960059,1.71834053708117E-17));
#110218=DIRECTION('ref_axis',(-0.139173100960059,0.990268068741571,-4.14246685971564E-34));
#110219=DIRECTION('',(0.990268068741571,0.139173100960059,1.71834053708117E-17));
#110220=DIRECTION('',(-0.990268068741571,-0.139173100960059,-1.71834053708117E-17));
#110221=DIRECTION('center_axis',(0.990268068741571,0.139173100960059,0.));
#110222=DIRECTION('ref_axis',(-0.139173100960059,0.990268068741571,0.));
#110223=DIRECTION('center_axis',(0.,1.23467863058847E-16,-1.));
#110224=DIRECTION('ref_axis',(0.,1.,0.));
#110225=DIRECTION('center_axis',(0.,0.,-1.));
#110226=DIRECTION('ref_axis',(0.,1.,0.));
#110227=DIRECTION('center_axis',(0.728126055379271,0.685443248911113,0.));
#110228=DIRECTION('ref_axis',(-0.685443248911113,0.728126055379271,0.));
#110229=DIRECTION('center_axis',(0.,0.,1.));
#110230=DIRECTION('ref_axis',(0.,1.,0.));
#110231=DIRECTION('center_axis',(0.,1.23467863058847E-16,-1.));
#110232=DIRECTION('ref_axis',(0.,1.,0.));
#110233=DIRECTION('center_axis',(0.,0.,-1.));
#110234=DIRECTION('ref_axis',(0.,1.,0.));
#110235=DIRECTION('center_axis',(0.685443248911109,0.728126055379275,0.));
#110236=DIRECTION('ref_axis',(-0.728126055379275,0.685443248911109,0.));
#110237=DIRECTION('center_axis',(0.,0.,1.));
#110238=DIRECTION('ref_axis',(0.,1.,0.));
#110239=DIRECTION('center_axis',(0.,1.23467863058847E-16,-1.));
#110240=DIRECTION('ref_axis',(0.,1.,0.));
#110241=DIRECTION('center_axis',(0.,0.,-1.));
#110242=DIRECTION('ref_axis',(0.,1.,0.));
#110243=DIRECTION('center_axis',(0.139173100960066,0.99026806874157,0.));
#110244=DIRECTION('ref_axis',(-0.99026806874157,0.139173100960066,0.));
#110245=DIRECTION('center_axis',(4.28365201153744E-31,-1.48619034146585E-45,
1.));
#110246=DIRECTION('ref_axis',(3.46944695195361E-15,1.,1.24460305557223E-60));
#110247=DIRECTION('center_axis',(-0.139173100960066,-0.99026806874157,0.));
#110248=DIRECTION('ref_axis',(0.99026806874157,-0.139173100960066,0.));
#110249=DIRECTION('center_axis',(0.,0.,-1.));
#110250=DIRECTION('ref_axis',(-1.,0.,0.));
#110251=DIRECTION('center_axis',(-0.139173100960066,-0.99026806874157,0.));
#110252=DIRECTION('ref_axis',(0.99026806874157,-0.139173100960066,0.));
#110253=DIRECTION('',(-0.139173100960065,-0.99026806874157,-3.85185988877447E-34));
#110254=DIRECTION('center_axis',(-0.139173100960066,-0.99026806874157,0.));
#110255=DIRECTION('ref_axis',(0.99026806874157,-0.139173100960066,0.));
#110256=DIRECTION('center_axis',(0.,0.,-1.));
#110257=DIRECTION('ref_axis',(-1.,0.,0.));
#110258=DIRECTION('center_axis',(0.139173100960066,0.99026806874157,1.22266282302934E-16));
#110259=DIRECTION('ref_axis',(-0.99026806874157,0.139173100960066,1.22723965167578E-33));
#110260=DIRECTION('',(-0.139173100960065,-0.99026806874157,-1.22266282302933E-16));
#110261=DIRECTION('center_axis',(0.139173100960073,0.990268068741569,0.));
#110262=DIRECTION('ref_axis',(-0.990268068741569,0.139173100960073,0.));
#110263=DIRECTION('center_axis',(0.133528512868198,0.950104737537311,0.281906232567435));
#110264=DIRECTION('ref_axis',(1.78830809785603E-17,-0.284453521859893,0.958689831958962));
#110265=DIRECTION('center_axis',(0.139173100960066,0.99026806874157,1.22266282302934E-16));
#110266=DIRECTION('ref_axis',(-0.99026806874157,0.139173100960066,1.22723965167578E-33));
#110267=DIRECTION('',(-0.139173100960065,-0.99026806874157,-1.22266282302933E-16));
#110268=DIRECTION('',(0.139173100960065,0.99026806874157,1.22266282302933E-16));
#110269=DIRECTION('center_axis',(0.,0.,1.));
#110270=DIRECTION('ref_axis',(1.,0.,0.));
#110271=DIRECTION('center_axis',(-0.139173100960039,-0.990268068741574,
-2.74854602616996E-14));
#110272=DIRECTION('ref_axis',(0.990268068741574,-0.139173100960039,-5.80135260633727E-30));
#110273=DIRECTION('center_axis',(-0.139173100960066,-0.99026806874157,0.));
#110274=DIRECTION('ref_axis',(0.99026806874157,-0.139173100960066,0.));
#110275=DIRECTION('',(-0.139173100960065,-0.99026806874157,-3.85185988877447E-34));
#110276=DIRECTION('center_axis',(-0.139173100960066,-0.99026806874157,0.));
#110277=DIRECTION('ref_axis',(0.99026806874157,-0.139173100960066,0.));
#110278=DIRECTION('center_axis',(0.,0.,-1.));
#110279=DIRECTION('ref_axis',(-1.,0.,0.));
#110280=DIRECTION('center_axis',(0.139173100960066,0.99026806874157,1.22266282302934E-16));
#110281=DIRECTION('ref_axis',(-0.99026806874157,0.139173100960066,1.22723965167578E-33));
#110282=DIRECTION('',(-0.139173100960065,-0.99026806874157,-1.22266282302933E-16));
#110283=DIRECTION('center_axis',(0.,0.,1.));
#110284=DIRECTION('ref_axis',(1.,0.,0.));
#110285=DIRECTION('center_axis',(-0.408524918701489,-0.868147321075037,
0.281829061152641));
#110286=DIRECTION('ref_axis',(0.904824724134437,-0.425784239486432,-2.46811619432984E-17));
#110287=DIRECTION('center_axis',(-0.907068166518068,0.420531768759975,-0.0195031472628737));
#110288=DIRECTION('ref_axis',(0.0518039117125095,0.157474353828549,0.986163365075769));
#110289=DIRECTION('center_axis',(-0.42055084745715,-0.907268970428876,0.));
#110290=DIRECTION('ref_axis',(0.907268970428876,-0.42055084745715,0.));
#110291=DIRECTION('center_axis',(0.732902040696953,-0.679599705515257,0.0316044143406873));
#110292=DIRECTION('ref_axis',(-0.11008573061797,-0.164305835944245,-0.980247277062768));
#110293=DIRECTION('center_axis',(0.,0.,1.));
#110294=DIRECTION('ref_axis',(1.,0.,0.));
#110295=DIRECTION('center_axis',(0.,0.,-1.));
#110296=DIRECTION('ref_axis',(1.,0.,0.));
#110297=DIRECTION('center_axis',(-0.412076271185962,-0.911149354785193,
0.));
#110298=DIRECTION('ref_axis',(0.911149354785193,-0.412076271185962,0.));
#110299=DIRECTION('center_axis',(0.,0.,1.));
#110300=DIRECTION('ref_axis',(1.,0.,0.));
#110301=DIRECTION('center_axis',(0.,-6.17339315294237E-17,1.));
#110302=DIRECTION('ref_axis',(0.,-1.,0.));
#110303=DIRECTION('center_axis',(1.3159378979443E-30,2.80509034228723E-44,
-1.));
#110304=DIRECTION('ref_axis',(2.1316282072803E-14,-1.,-5.4762534445178E-59));
#110305=DIRECTION('center_axis',(0.132724703727513,-0.991152939252941,6.34877946761353E-5));
#110306=DIRECTION('ref_axis',(0.985065037121742,0.131916564409429,0.1106566431569));
#110307=DIRECTION('center_axis',(-0.162778679587413,0.986662604791219,-7.60156866848099E-5));
#110308=DIRECTION('ref_axis',(0.986084783174683,0.162685986477531,0.0342062888248791));
#110309=DIRECTION('center_axis',(0.282415254236812,0.959292251701408,0.));
#110310=DIRECTION('ref_axis',(-0.959292251701408,0.282415254236812,0.));
#110311=DIRECTION('center_axis',(0.,0.,-1.));
#110312=DIRECTION('ref_axis',(-1.,0.,0.));
#110313=DIRECTION('center_axis',(0.,0.,1.));
#110314=DIRECTION('ref_axis',(1.,0.,0.));
#110315=DIRECTION('center_axis',(0.273940677965627,0.961746590820957,0.));
#110316=DIRECTION('ref_axis',(-0.961746590820957,0.273940677965627,0.));
#110317=DIRECTION('center_axis',(0.,0.,-1.));
#110318=DIRECTION('ref_axis',(1.,-1.77920356510442E-15,0.));
#110319=DIRECTION('center_axis',(0.0971107883155516,0.363411229368455,0.926553707650906));
#110320=DIRECTION('ref_axis',(3.86068458172679E-17,-0.930953788243945,0.365137021067773));
#110321=DIRECTION('center_axis',(0.,0.,1.));
#110322=DIRECTION('ref_axis',(1.,0.,0.));
#110323=DIRECTION('center_axis',(-0.966107498808678,0.25814005491211,-0.000113117697403614));
#110324=DIRECTION('ref_axis',(0.25388184709702,0.950091406535467,-0.181301756588465));
#110325=DIRECTION('center_axis',(0.,-6.17339315294237E-17,1.));
#110326=DIRECTION('ref_axis',(0.,-1.,0.));
#110327=DIRECTION('center_axis',(0.,0.,-1.));
#110328=DIRECTION('ref_axis',(0.,-1.,0.));
#110329=DIRECTION('center_axis',(0.0766838736637995,-0.997055455878901,
3.77098383583762E-5));
#110330=DIRECTION('ref_axis',(0.97952184613108,0.0753424193663023,0.186709594815031));
#110331=DIRECTION('center_axis',(-0.116942841787273,0.993138645130569,-5.74711537241093E-5));
#110332=DIRECTION('ref_axis',(0.983260089651775,0.115787775552541,0.140686840644664));
#110333=DIRECTION('center_axis',(-0.144956948347396,-0.989281282708723,
-0.017607578141073));
#110334=DIRECTION('ref_axis',(0.989434670234472,-0.144979423843532,1.06064347286242E-18));
#110335=DIRECTION('center_axis',(0.,0.,-1.));
#110336=DIRECTION('ref_axis',(-1.,0.,0.));
#110337=DIRECTION('center_axis',(0.140089618365222,-0.00275771349061114,
-0.990134987687331));
#110338=DIRECTION('ref_axis',(0.979470506177534,-0.146013776318709,0.138987426242359));
#110339=DIRECTION('center_axis',(-0.136497250965888,-0.990504401193308,
-0.0164174204868685));
#110340=DIRECTION('ref_axis',(0.990637914348733,-0.136515649853022,4.14575077332242E-19));
#110341=DIRECTION('center_axis',(0.,0.,-1.));
#110342=DIRECTION('ref_axis',(-1.,0.,0.));
#110343=DIRECTION('center_axis',(0.,-6.17339315294237E-17,1.));
#110344=DIRECTION('ref_axis',(0.,-1.,0.));
#110345=DIRECTION('center_axis',(-6.57968948972152E-31,7.01272585571806E-45,
-1.));
#110346=DIRECTION('ref_axis',(-1.06581410364015E-14,-1.,0.));
#110347=DIRECTION('center_axis',(0.0112985155260908,-0.999936169720593,
5.60510491874375E-6));
#110348=DIRECTION('ref_axis',(0.976494079513853,0.0110348444394294,0.2152615731676));
#110349=DIRECTION('center_axis',(-0.0572811109810715,0.99835808881386,-2.87177830595105E-5));
#110350=DIRECTION('ref_axis',(0.977895626960296,0.0561128647169375,0.201423655972154));
#110351=DIRECTION('center_axis',(-0.00619406208384126,-0.999980560265093,
-0.000716021516796888));
#110352=DIRECTION('ref_axis',(0.999980816603614,-0.00619406367164884,-2.43997512021813E-21));
#110353=DIRECTION('center_axis',(8.20654853338604E-14,3.5527136788005E-12,
-1.));
#110354=DIRECTION('ref_axis',(-1.83670992315982E-40,1.,3.5527136788005E-12));
#110355=DIRECTION('center_axis',(0.115801534012589,-2.98133654443904E-10,
-0.993272371870038));
#110356=DIRECTION('ref_axis',(0.99325305842217,-0.00623603598024155,0.115799282339136));
#110357=DIRECTION('center_axis',(0.00234948403731584,-0.999997203076769,
0.000271594180011335));
#110358=DIRECTION('ref_axis',(0.999997239958367,0.00234948412396881,6.81083076705817E-23));
#110359=DIRECTION('center_axis',(0.,0.,-1.));
#110360=DIRECTION('ref_axis',(-1.,0.,0.));
#110361=DIRECTION('center_axis',(0.,-6.17339315294237E-17,1.));
#110362=DIRECTION('ref_axis',(0.,-1.,0.));
#110363=DIRECTION('center_axis',(0.,0.,-1.));
#110364=DIRECTION('ref_axis',(0.,-1.,0.));
#110365=DIRECTION('center_axis',(-0.0554962509005653,-0.998458895190388,
-2.74074994885905E-5));
#110366=DIRECTION('ref_axis',(0.978041961940448,-0.0543669614620168,0.201191834290228));
#110367=DIRECTION('center_axis',(0.00943472545585777,0.999955491976012,
4.75229707891771E-6));
#110368=DIRECTION('ref_axis',(0.976210029853252,-0.00921171311038235,0.216631304190978));
#110369=DIRECTION('center_axis',(0.1326869973619,-0.991030504325029,0.0158965476868861));
#110370=DIRECTION('ref_axis',(0.991155744879145,0.132703765557229,-2.90070390844182E-17));
#110371=DIRECTION('center_axis',(3.85729088923276E-14,-3.33066907387548E-13,
-1.));
#110372=DIRECTION('ref_axis',(1.00445073922803E-41,1.,-3.33066907387547E-13));
#110373=DIRECTION('center_axis',(0.137685287328068,0.00241479086434434,
-0.99047308415649));
#110374=DIRECTION('ref_axis',(0.981548262063148,0.133629545123289,0.136770442387809));
#110375=DIRECTION('center_axis',(0.141151402782332,-0.989840911569284,0.0170660855578596));
#110376=DIRECTION('ref_axis',(0.989985089278404,0.141171962536586,2.4318092123443E-19));
#110377=DIRECTION('center_axis',(0.,0.,-1.));
#110378=DIRECTION('ref_axis',(-1.,0.,0.));
#110379=DIRECTION('center_axis',(0.,-6.17339315294237E-17,1.));
#110380=DIRECTION('ref_axis',(0.,-1.,0.));
#110381=DIRECTION('center_axis',(-1.8642453554211E-30,5.62966047861811E-44,
-1.));
#110382=DIRECTION('ref_axis',(-3.01980662698043E-14,-1.,-9.95682444457782E-59));
#110383=DIRECTION('center_axis',(-0.115451282615198,-0.993313142075069,
-5.58879192006845E-5));
#110384=DIRECTION('ref_axis',(0.983286165238662,-0.114293836168303,0.14172239154128));
#110385=DIRECTION('center_axis',(0.0749734441413244,0.997185530014467,3.74613657666356E-5));
#110386=DIRECTION('ref_axis',(0.979143860919972,-0.0736240940087581,0.189358898402267));
#110387=DIRECTION('center_axis',(-0.185959552881302,0.695904038033425,-0.693640118895209));
#110388=DIRECTION('ref_axis',(3.15382046976506E-16,0.705953788300242,0.708257897085897));
#110389=DIRECTION('center_axis',(0.,0.,-1.));
#110390=DIRECTION('ref_axis',(-1.,0.,0.));
#110391=DIRECTION('center_axis',(-0.270127118644541,0.962824667202081,-4.0829772679528E-16));
#110392=DIRECTION('ref_axis',(-0.962824667202081,-0.270127118644541,5.77560433057458E-31));
#110393=DIRECTION('center_axis',(0.,0.,1.));
#110394=DIRECTION('ref_axis',(1.,0.,0.));
#110395=DIRECTION('center_axis',(-0.278601694915732,0.960406734456856,-8.33020054374265E-16));
#110396=DIRECTION('ref_axis',(-0.960406734456856,-0.278601694915732,-5.45700864471184E-31));
#110397=DIRECTION('center_axis',(0.,0.,-1.));
#110398=DIRECTION('ref_axis',(1.,1.13691107810172E-13,0.));
#110399=DIRECTION('center_axis',(0.,0.,1.));
#110400=DIRECTION('ref_axis',(1.,0.,0.));
#110401=DIRECTION('center_axis',(0.,-6.17339315294237E-17,1.));
#110402=DIRECTION('ref_axis',(0.,-1.,0.));
#110403=DIRECTION('center_axis',(1.15144566070127E-30,2.14764729331365E-44,
-1.));
#110404=DIRECTION('ref_axis',(1.86517468137027E-14,-1.,3.73380916671668E-59));
#110405=DIRECTION('center_axis',(-0.161739700498652,-0.986833452889392,
-7.44379325117182E-5));
#110406=DIRECTION('ref_axis',(0.986200813837069,-0.161638712068232,0.0357894055276974));
#110407=DIRECTION('center_axis',(0.131366277566232,0.991333897851926,6.39382359252622E-5));
#110408=DIRECTION('ref_axis',(0.984780382030639,-0.130505244040753,0.114786673640506));
#110409=DIRECTION('center_axis',(0.,0.,1.));
#110410=DIRECTION('ref_axis',(1.,0.,0.));
#110411=DIRECTION('center_axis',(0.40826271186488,-0.912864479591979,3.16713488626711E-15));
#110412=DIRECTION('ref_axis',(0.912864479591979,0.40826271186488,6.04208104977424E-31));
#110413=DIRECTION('center_axis',(0.,0.,1.));
#110414=DIRECTION('ref_axis',(1.,0.,0.));
#110415=DIRECTION('center_axis',(0.,0.,-1.));
#110416=DIRECTION('ref_axis',(1.,-1.0479508998465E-13,0.));
#110417=DIRECTION('center_axis',(0.416737288136069,-0.909026970269307,0.));
#110418=DIRECTION('ref_axis',(0.909026970269307,0.416737288136069,0.));
#110419=DIRECTION('center_axis',(0.369731042763204,-0.785707308414229,-0.495946551073502));
#110420=DIRECTION('ref_axis',(1.91361720426385E-15,0.533770129672178,-0.845629616717477));
#110421=DIRECTION('center_axis',(0.133528512868191,-0.950104737537312,0.281906232567436));
#110422=DIRECTION('ref_axis',(-2.32560161936155E-16,-0.284453521859895,
-0.958689831958962));
#110423=DIRECTION('center_axis',(0.,0.,1.));
#110424=DIRECTION('ref_axis',(1.,0.,0.));
#110425=DIRECTION('center_axis',(0.139173100960066,-0.99026806874157,0.));
#110426=DIRECTION('ref_axis',(0.99026806874157,0.139173100960066,0.));
#110427=DIRECTION('center_axis',(-0.139173100960066,0.99026806874157,1.22266282302933E-16));
#110428=DIRECTION('ref_axis',(-0.99026806874157,-0.139173100960066,-9.57340194962255E-34));
#110429=DIRECTION('',(0.139173100960067,-0.99026806874157,-1.22266282302933E-16));
#110430=DIRECTION('center_axis',(0.139173100960066,-0.99026806874157,0.));
#110431=DIRECTION('ref_axis',(0.99026806874157,0.139173100960066,0.));
#110432=DIRECTION('center_axis',(0.,0.,-1.));
#110433=DIRECTION('ref_axis',(-1.,0.,0.));
#110434=DIRECTION('center_axis',(0.139173100960066,-0.99026806874157,0.));
#110435=DIRECTION('ref_axis',(0.99026806874157,0.139173100960066,0.));
#110436=DIRECTION('',(0.139173100960067,-0.99026806874157,0.));
#110437=DIRECTION('center_axis',(0.139173100960066,-0.99026806874157,0.));
#110438=DIRECTION('ref_axis',(0.99026806874157,0.139173100960066,0.));
#110439=DIRECTION('center_axis',(0.,0.,-1.));
#110440=DIRECTION('ref_axis',(-1.,0.,0.));
#110441=DIRECTION('center_axis',(-0.139173100960066,0.99026806874157,1.22266282302933E-16));
#110442=DIRECTION('ref_axis',(-0.99026806874157,-0.139173100960066,-9.57340194962255E-34));
#110443=DIRECTION('',(0.139173100960067,-0.99026806874157,-1.22266282302933E-16));
#110444=DIRECTION('center_axis',(0.,0.,1.));
#110445=DIRECTION('ref_axis',(1.,0.,0.));
#110446=DIRECTION('center_axis',(0.139173100960066,-0.99026806874157,0.));
#110447=DIRECTION('ref_axis',(0.99026806874157,0.139173100960066,0.));
#110448=DIRECTION('center_axis',(0.139173100960066,-0.99026806874157,0.));
#110449=DIRECTION('ref_axis',(0.99026806874157,0.139173100960066,0.));
#110450=DIRECTION('',(0.139173100960067,-0.99026806874157,0.));
#110451=DIRECTION('center_axis',(0.139173100960066,-0.99026806874157,0.));
#110452=DIRECTION('ref_axis',(0.99026806874157,0.139173100960066,0.));
#110453=DIRECTION('center_axis',(0.,0.,-1.));
#110454=DIRECTION('ref_axis',(-1.,0.,0.));
#110455=DIRECTION('center_axis',(-0.139173100960066,0.99026806874157,1.22266282302933E-16));
#110456=DIRECTION('ref_axis',(-0.99026806874157,-0.139173100960066,-9.57340194962255E-34));
#110457=DIRECTION('',(-0.139173100960067,0.99026806874157,1.22266282302933E-16));
#110458=DIRECTION('',(0.139173100960067,-0.99026806874157,-1.22266282302933E-16));
#110459=DIRECTION('center_axis',(-0.139173100960066,0.99026806874157,0.));
#110460=DIRECTION('ref_axis',(-0.99026806874157,-0.139173100960066,0.));
#110461=DIRECTION('center_axis',(0.,1.23467863058847E-16,-1.));
#110462=DIRECTION('ref_axis',(0.,1.,0.));
#110463=DIRECTION('center_axis',(0.,0.,-1.));
#110464=DIRECTION('ref_axis',(0.,1.,0.));
#110465=DIRECTION('center_axis',(-0.685443248911109,0.728126055379275,0.));
#110466=DIRECTION('ref_axis',(-0.728126055379275,-0.685443248911109,0.));
#110467=DIRECTION('center_axis',(-4.28365201153744E-31,-1.48619034146585E-45,
1.));
#110468=DIRECTION('ref_axis',(-3.46944695195361E-15,1.,1.24460305557223E-60));
#110469=DIRECTION('center_axis',(0.,1.23467863058847E-16,-1.));
#110470=DIRECTION('ref_axis',(0.,1.,0.));
#110471=DIRECTION('center_axis',(0.,0.,-1.));
#110472=DIRECTION('ref_axis',(0.,1.,0.));
#110473=DIRECTION('center_axis',(-0.728126055379271,0.685443248911113,0.));
#110474=DIRECTION('ref_axis',(-0.685443248911113,-0.728126055379271,0.));
#110475=DIRECTION('center_axis',(-6.14104352374008E-30,-3.05443170604608E-43,
1.));
#110476=DIRECTION('ref_axis',(-4.9737991503207E-14,1.,0.));
#110477=DIRECTION('center_axis',(0.,1.23467863058847E-16,-1.));
#110478=DIRECTION('ref_axis',(0.,1.,0.));
#110479=DIRECTION('center_axis',(0.,0.,-1.));
#110480=DIRECTION('ref_axis',(0.,1.,0.));
#110481=DIRECTION('center_axis',(-0.990268068741571,0.139173100960059,0.));
#110482=DIRECTION('ref_axis',(-0.139173100960059,-0.990268068741571,0.));
#110483=DIRECTION('center_axis',(0.,0.,1.));
#110484=DIRECTION('ref_axis',(0.,1.,0.));
#110485=DIRECTION('center_axis',(-0.990268068741571,0.139173100960059,1.71834053708117E-17));
#110486=DIRECTION('ref_axis',(-0.139173100960059,-0.990268068741571,4.14246685971564E-34));
#110487=DIRECTION('',(0.990268068741571,-0.139173100960059,-1.71834053708117E-17));
#110488=DIRECTION('',(-0.990268068741571,0.139173100960059,1.71834053708117E-17));
#110489=DIRECTION('center_axis',(0.,0.,-1.));
#110490=DIRECTION('ref_axis',(1.,0.,0.));
#110491=DIRECTION('center_axis',(0.,-7.15121221728469E-32,-1.));
#110492=DIRECTION('ref_axis',(1.,0.,0.));
#110493=DIRECTION('center_axis',(-1.,0.,5.40794518211031E-32));
#110494=DIRECTION('ref_axis',(0.,1.,0.));
#110495=DIRECTION('center_axis',(0.,-1.,0.));
#110496=DIRECTION('ref_axis',(0.,0.,-1.));
#110497=DIRECTION('center_axis',(-5.01606788234257E-16,-1.,5.70122241611331E-32));
#110498=DIRECTION('ref_axis',(-1.,5.01606788234257E-16,0.));
#110499=DIRECTION('',(-1.,5.01606788234257E-16,0.));
#110500=DIRECTION('',(-2.85977186515575E-47,-5.70122241611331E-32,-1.));
#110501=DIRECTION('',(2.85977186515575E-47,5.70122241611331E-32,1.));
#110502=DIRECTION('center_axis',(0.,0.,1.));
#110503=DIRECTION('ref_axis',(0.,-1.,0.));
#110504=DIRECTION('',(0.,1.23467863058847E-16,-1.));
#110505=DIRECTION('',(0.,-1.23467863058847E-16,1.));
#110506=DIRECTION('center_axis',(0.,1.18613571006961E-16,-1.));
#110507=DIRECTION('ref_axis',(0.,1.,1.18613571006961E-16));
#110508=DIRECTION('center_axis',(0.,1.23467863058847E-16,-1.));
#110509=DIRECTION('ref_axis',(-1.,0.,0.));
#110510=DIRECTION('center_axis',(0.,0.,-1.));
#110511=DIRECTION('ref_axis',(0.,1.,0.));
#110512=DIRECTION('',(4.38004274807345E-16,1.,1.23467863058847E-16));
#110513=DIRECTION('',(1.,-4.38004274807345E-16,-5.40794518211031E-32));
#110514=DIRECTION('center_axis',(-4.18005656861882E-16,-1.,0.));
#110515=DIRECTION('ref_axis',(1.,0.,0.));
#110516=DIRECTION('center_axis',(1.,0.,0.));
#110517=DIRECTION('ref_axis',(0.,0.,-1.));
#110518=DIRECTION('center_axis',(0.,1.,0.));
#110519=DIRECTION('ref_axis',(1.,0.,0.));
#110520=DIRECTION('center_axis',(0.,0.,1.));
#110521=DIRECTION('ref_axis',(1.,0.,0.));
#110522=DIRECTION('center_axis',(0.,0.,1.));
#110523=DIRECTION('ref_axis',(1.,0.,0.));
#110524=DIRECTION('',(0.,0.,-1.));
#110525=DIRECTION('center_axis',(0.,0.,1.));
#110526=DIRECTION('ref_axis',(1.,0.,0.));
#110527=DIRECTION('center_axis',(-0.507514080295481,0.,-0.861643463563574));
#110528=DIRECTION('ref_axis',(-0.861643463563574,0.,0.507514080295481));
#110529=DIRECTION('center_axis',(-0.483825549717016,0.,-0.87516446308167));
#110530=DIRECTION('ref_axis',(-0.87516446308167,0.,0.483825549717016));
#110531=DIRECTION('center_axis',(0.,0.,-1.));
#110532=DIRECTION('ref_axis',(-1.,0.,0.));
#110533=DIRECTION('center_axis',(0.,0.,1.));
#110534=DIRECTION('ref_axis',(-0.707106781193192,-0.707106781179903,0.));
#110535=DIRECTION('center_axis',(1.11022302462516E-13,0.,-1.));
#110536=DIRECTION('ref_axis',(-1.,0.,-1.11022302462516E-13));
#110537=DIRECTION('',(0.,0.,1.));
#110538=DIRECTION('center_axis',(0.507514080295474,0.,-0.861643463563578));
#110539=DIRECTION('ref_axis',(-0.861643463563578,0.,-0.507514080295474));
#110540=DIRECTION('center_axis',(0.483537964931496,0.,-0.875323389650881));
#110541=DIRECTION('ref_axis',(-0.875323389650881,0.,-0.483537964931496));
#110542=DIRECTION('center_axis',(1.,0.,0.));
#110543=DIRECTION('ref_axis',(0.,0.,-1.));
#110544=DIRECTION('center_axis',(-1.,4.1800565686188E-16,5.16102651992463E-32));
#110545=DIRECTION('ref_axis',(-4.1800565686188E-16,-1.,8.08534226092968E-63));
#110546=DIRECTION('center_axis',(1.,0.,0.));
#110547=DIRECTION('ref_axis',(0.,0.,-1.));
#110548=DIRECTION('',(-1.,4.18005656861881E-16,5.16102651992463E-32));
#110549=DIRECTION('center_axis',(0.,0.,-1.));
#110550=DIRECTION('ref_axis',(-1.,0.,0.));
#110551=DIRECTION('center_axis',(0.,0.,-1.));
#110552=DIRECTION('ref_axis',(-1.,0.,0.));
#110553=DIRECTION('center_axis',(0.,7.25334975031382E-33,-1.));
#110554=DIRECTION('ref_axis',(-1.,0.,0.));
#110555=DIRECTION('',(1.73522765332109E-17,-7.25334975031383E-33,1.));
#110556=DIRECTION('',(-1.73522765332109E-17,6.98077064262961E-33,-1.));
#110557=DIRECTION('center_axis',(1.,0.,0.));
#110558=DIRECTION('ref_axis',(0.,1.,0.));
#110559=DIRECTION('',(-1.,4.18005656861881E-16,0.));
#110560=DIRECTION('center_axis',(1.,0.,-5.16102651992463E-32));
#110561=DIRECTION('ref_axis',(0.,1.,0.));
#110562=DIRECTION('center_axis',(-1.,0.,0.));
#110563=DIRECTION('ref_axis',(0.,0.,1.));
#110564=DIRECTION('',(-1.,4.18005656861881E-16,5.16102651992463E-32));
#110565=DIRECTION('center_axis',(-1.,0.,0.));
#110566=DIRECTION('ref_axis',(0.,0.,1.));
#110567=DIRECTION('',(1.,-4.18005656861881E-16,-5.16102651992463E-32));
#110568=DIRECTION('center_axis',(-4.18005656861882E-16,-1.,0.));
#110569=DIRECTION('ref_axis',(1.,0.,0.));
#110570=DIRECTION('center_axis',(0.,1.,0.));
#110571=DIRECTION('ref_axis',(1.,0.,0.));
#110572=DIRECTION('center_axis',(-1.,0.,0.));
#110573=DIRECTION('ref_axis',(0.,0.,1.));
#110574=DIRECTION('center_axis',(0.,-1.,0.));
#110575=DIRECTION('ref_axis',(1.,0.,0.));
#110576=DIRECTION('center_axis',(4.18005656861881E-16,1.,0.));
#110577=DIRECTION('ref_axis',(-1.,4.18005656861881E-16,0.));
#110578=DIRECTION('',(4.18005656861881E-16,1.,0.));
#110579=DIRECTION('center_axis',(0.,1.,0.));
#110580=DIRECTION('ref_axis',(-1.,0.,0.));
#110581=DIRECTION('center_axis',(4.18005656861882E-16,1.,0.));
#110582=DIRECTION('ref_axis',(-1.,0.,0.));
#110583=DIRECTION('center_axis',(1.,0.,0.));
#110584=DIRECTION('ref_axis',(0.,0.,-1.));
#110585=DIRECTION('center_axis',(0.,-1.,0.));
#110586=DIRECTION('ref_axis',(-1.,0.,0.));
#110587=DIRECTION('center_axis',(0.,0.,-1.));
#110588=DIRECTION('ref_axis',(-1.,0.,0.));
#110589=DIRECTION('center_axis',(0.,0.,-1.));
#110590=DIRECTION('ref_axis',(-1.,0.,0.));
#110591=DIRECTION('',(0.,0.,1.));
#110592=DIRECTION('center_axis',(0.,0.,-1.));
#110593=DIRECTION('ref_axis',(-1.,0.,0.));
#110594=DIRECTION('center_axis',(4.18005656861882E-16,1.,0.));
#110595=DIRECTION('ref_axis',(-1.,0.,0.));
#110596=DIRECTION('center_axis',(0.,-1.,0.));
#110597=DIRECTION('ref_axis',(-1.,0.,0.));
#110598=DIRECTION('center_axis',(-1.,0.,0.));
#110599=DIRECTION('ref_axis',(0.,0.,1.));
#110600=DIRECTION('center_axis',(1.,0.,0.));
#110601=DIRECTION('ref_axis',(0.,1.,0.));
#110602=DIRECTION('',(1.,-4.18005656861881E-16,0.));
#110603=DIRECTION('center_axis',(0.,-7.25334975031382E-33,1.));
#110604=DIRECTION('ref_axis',(1.,0.,0.));
#110605=DIRECTION('',(-1.73522765332109E-17,7.25334975031383E-33,-1.));
#110606=DIRECTION('center_axis',(0.,0.,-1.));
#110607=DIRECTION('ref_axis',(-1.,0.,0.));
#110608=DIRECTION('',(1.73522765332109E-17,-6.98077064262961E-33,1.));
#110609=DIRECTION('center_axis',(1.,0.,0.));
#110610=DIRECTION('ref_axis',(0.,0.,-1.));
#110611=DIRECTION('center_axis',(1.,-4.1800565686188E-16,-5.16102651992463E-32));
#110612=DIRECTION('ref_axis',(4.1800565686188E-16,1.,-8.08534226092968E-63));
#110613=DIRECTION('',(1.,-4.18005656861881E-16,-5.16102651992463E-32));
#110614=DIRECTION('center_axis',(1.,0.,0.));
#110615=DIRECTION('ref_axis',(0.,0.,-1.));
#110616=DIRECTION('center_axis',(0.496378972716316,6.19668439877561E-14,
-0.868105935612178));
#110617=DIRECTION('ref_axis',(-0.868105935612178,3.44724486393529E-29,-0.496378972716316));
#110618=DIRECTION('center_axis',(0.518474310548581,7.19527646559628E-15,
-0.855093205037424));
#110619=DIRECTION('ref_axis',(-0.855093205037424,3.43699106634736E-31,-0.518474310548581));
#110620=DIRECTION('center_axis',(-2.72711680125255E-25,1.11022302462516E-13,
-1.));
#110621=DIRECTION('ref_axis',(1.56607307231965E-53,1.,1.11022302462516E-13));
#110622=DIRECTION('center_axis',(0.,0.,-1.));
#110623=DIRECTION('ref_axis',(-1.,0.,0.));
#110624=DIRECTION('',(0.,0.,-1.));
#110625=DIRECTION('center_axis',(0.,0.,-1.));
#110626=DIRECTION('ref_axis',(-1.,0.,0.));
#110627=DIRECTION('center_axis',(-0.518474310548575,0.,-0.855093205037428));
#110628=DIRECTION('ref_axis',(-0.855093205037428,0.,0.518474310548575));
#110629=DIRECTION('center_axis',(-0.496741562438066,1.20445113324067E-14,
-0.867898507975782));
#110630=DIRECTION('ref_axis',(-0.867898507975782,5.70559822356712E-31,0.496741562438066));
#110631=DIRECTION('center_axis',(-1.,0.,0.));
#110632=DIRECTION('ref_axis',(0.,0.,1.));
#110633=DIRECTION('center_axis',(-1.,0.,5.16102651992463E-32));
#110634=DIRECTION('ref_axis',(0.,-1.,0.));
#110635=DIRECTION('',(-1.,4.18005656861881E-16,5.16102651992463E-32));
#110636=DIRECTION('center_axis',(-1.,0.,0.));
#110637=DIRECTION('ref_axis',(0.,0.,1.));
#110638=DIRECTION('',(1.,-4.18005656861881E-16,-5.16102651992463E-32));
#110639=DIRECTION('center_axis',(0.,1.23467863058847E-16,-1.));
#110640=DIRECTION('ref_axis',(0.,1.,1.1837531408762E-16));
#110641=DIRECTION('center_axis',(8.39641081720404E-32,-1.17559414210783E-16,
1.));
#110642=DIRECTION('ref_axis',(1.4210854715202E-14,1.,1.17559414210783E-16));
#110643=DIRECTION('center_axis',(-4.18005656861882E-16,-1.,0.));
#110644=DIRECTION('ref_axis',(1.,0.,0.));
#110645=DIRECTION('center_axis',(1.,0.,0.));
#110646=DIRECTION('ref_axis',(0.,0.,-1.));
#110647=DIRECTION('center_axis',(0.,1.,0.));
#110648=DIRECTION('ref_axis',(1.,0.,0.));
#110649=DIRECTION('center_axis',(0.,0.,1.));
#110650=DIRECTION('ref_axis',(1.,0.,0.));
#110651=DIRECTION('center_axis',(0.,0.,1.));
#110652=DIRECTION('ref_axis',(1.,0.,0.));
#110653=DIRECTION('',(0.,0.,-1.));
#110654=DIRECTION('center_axis',(0.,0.,1.));
#110655=DIRECTION('ref_axis',(1.,0.,0.));
#110656=DIRECTION('center_axis',(-1.,4.1800565686188E-16,5.16102651992463E-32));
#110657=DIRECTION('ref_axis',(-4.1800565686188E-16,-1.,8.08534226092968E-63));
#110658=DIRECTION('center_axis',(1.,1.38777878078144E-14,-1.38777878078144E-14));
#110659=DIRECTION('ref_axis',(-1.38777878078144E-14,4.48415508583941E-44,
-1.));
#110660=DIRECTION('',(1.,-4.18005656861881E-16,-5.16102651992463E-32));
#110661=DIRECTION('center_axis',(1.,0.,0.));
#110662=DIRECTION('ref_axis',(0.,0.,-1.));
#110663=DIRECTION('',(-1.,4.18005656861881E-16,5.16102651992463E-32));
#110664=DIRECTION('center_axis',(0.534875344054122,1.17257728967007E-14,
0.844930983171398));
#110665=DIRECTION('ref_axis',(0.844930983171398,-8.89670234612257E-31,-0.534875344054122));
#110666=DIRECTION('center_axis',(0.543750575738856,0.,0.839246871536417));
#110667=DIRECTION('ref_axis',(0.839246871536417,0.,-0.543750575738856));
#110668=DIRECTION('center_axis',(0.,0.,1.));
#110669=DIRECTION('ref_axis',(1.,0.,0.));
#110670=DIRECTION('center_axis',(0.,0.,1.));
#110671=DIRECTION('ref_axis',(1.,0.,0.));
#110672=DIRECTION('',(0.,0.,1.));
#110673=DIRECTION('center_axis',(0.,1.66533453693774E-12,1.));
#110674=DIRECTION('ref_axis',(0.,-1.,1.66533453693774E-12));
#110675=DIRECTION('center_axis',(0.543750575738856,0.,-0.839246871536417));
#110676=DIRECTION('ref_axis',(-0.839246871536417,0.,-0.543750575738856));
#110677=DIRECTION('center_axis',(0.534259922646944,0.,-0.845320255910907));
#110678=DIRECTION('ref_axis',(-0.845320255910907,0.,-0.534259922646944));
#110679=DIRECTION('center_axis',(1.,0.,1.38777878078144E-14));
#110680=DIRECTION('ref_axis',(1.38777878078144E-14,0.,-1.));
#110681=DIRECTION('center_axis',(1.,0.,-5.16102651992463E-32));
#110682=DIRECTION('ref_axis',(0.,1.,0.));
#110683=DIRECTION('center_axis',(1.,0.,0.));
#110684=DIRECTION('ref_axis',(0.,0.,-1.));
#110685=DIRECTION('',(-1.,4.18005656861881E-16,5.16102651992463E-32));
#110686=DIRECTION('center_axis',(0.,0.,-1.));
#110687=DIRECTION('ref_axis',(-1.,0.,0.));
#110688=DIRECTION('center_axis',(0.,0.,-1.));
#110689=DIRECTION('ref_axis',(-1.,0.,0.));
#110690=DIRECTION('center_axis',(0.,7.25334975031382E-33,-1.));
#110691=DIRECTION('ref_axis',(-1.,0.,0.));
#110692=DIRECTION('',(1.73522765332109E-17,-7.25334975031383E-33,1.));
#110693=DIRECTION('',(-1.73522765332109E-17,6.98077064262961E-33,-1.));
#110694=DIRECTION('center_axis',(1.,0.,0.));
#110695=DIRECTION('ref_axis',(0.,1.,0.));
#110696=DIRECTION('',(-1.,4.18005656861881E-16,0.));
#110697=DIRECTION('center_axis',(-4.18005656861882E-16,-1.,0.));
#110698=DIRECTION('ref_axis',(1.,0.,0.));
#110699=DIRECTION('center_axis',(0.,1.,0.));
#110700=DIRECTION('ref_axis',(1.,0.,0.));
#110701=DIRECTION('center_axis',(-1.,0.,0.));
#110702=DIRECTION('ref_axis',(0.,0.,1.));
#110703=DIRECTION('center_axis',(0.,-1.,0.));
#110704=DIRECTION('ref_axis',(1.,0.,0.));
#110705=DIRECTION('center_axis',(4.18005656861881E-16,1.,0.));
#110706=DIRECTION('ref_axis',(-1.,4.18005656861881E-16,0.));
#110707=DIRECTION('',(4.18005656861881E-16,1.,0.));
#110708=DIRECTION('center_axis',(0.,1.,0.));
#110709=DIRECTION('ref_axis',(-1.,0.,0.));
#110710=DIRECTION('center_axis',(-1.,0.,5.40794518211031E-32));
#110711=DIRECTION('ref_axis',(0.,-1.,0.));
#110712=DIRECTION('center_axis',(-1.,4.38004274807345E-16,0.));
#110713=DIRECTION('ref_axis',(0.,0.,1.));
#110714=DIRECTION('',(-1.,4.38004274807345E-16,5.40794518211031E-32));
#110715=DIRECTION('center_axis',(-1.,0.,0.));
#110716=DIRECTION('ref_axis',(0.,0.,1.));
#110717=DIRECTION('',(1.,-4.38004274807345E-16,-5.40794518211031E-32));
#110718=DIRECTION('center_axis',(-1.,0.,5.40794518211031E-32));
#110719=DIRECTION('ref_axis',(0.,-1.,0.));
#110720=DIRECTION('',(-1.,4.38004274807345E-16,5.40794518211031E-32));
#110721=DIRECTION('center_axis',(-1.,0.,0.));
#110722=DIRECTION('ref_axis',(0.,0.,1.));
#110723=DIRECTION('',(1.,-4.38004274807345E-16,-5.40794518211031E-32));
#110724=DIRECTION('center_axis',(1.,-4.38004274807346E-16,-5.40794518211031E-32));
#110725=DIRECTION('ref_axis',(4.38004274807346E-16,1.,5.80597460094347E-63));
#110726=DIRECTION('',(-1.,4.38004274807345E-16,5.40794518211031E-32));
#110727=DIRECTION('center_axis',(-1.,0.,0.));
#110728=DIRECTION('ref_axis',(0.,0.,1.));
#110729=DIRECTION('center_axis',(-1.,4.38004274807345E-16,0.));
#110730=DIRECTION('ref_axis',(0.,0.,1.));
#110731=DIRECTION('center_axis',(4.38004274807345E-16,1.,0.));
#110732=DIRECTION('ref_axis',(-1.,0.,0.));
#110733=DIRECTION('center_axis',(0.,0.,1.));
#110734=DIRECTION('ref_axis',(1.,0.,0.));
#110735=DIRECTION('center_axis',(-1.,0.,0.));
#110736=DIRECTION('ref_axis',(0.,0.,1.));
#110737=DIRECTION('center_axis',(0.,-1.,0.));
#110738=DIRECTION('ref_axis',(-1.,0.,0.));
#110739=DIRECTION('center_axis',(0.,0.,1.));
#110740=DIRECTION('ref_axis',(1.,0.,0.));
#110741=DIRECTION('center_axis',(0.,0.,1.));
#110742=DIRECTION('ref_axis',(1.,0.,0.));
#110743=DIRECTION('',(0.,0.,1.));
#110744=DIRECTION('center_axis',(4.38004274807345E-16,1.,0.));
#110745=DIRECTION('ref_axis',(-1.,0.,0.));
#110746=DIRECTION('center_axis',(1.,0.,0.));
#110747=DIRECTION('ref_axis',(0.,0.,-1.));
#110748=DIRECTION('center_axis',(0.,-1.,0.));
#110749=DIRECTION('ref_axis',(-1.,0.,0.));
#110750=DIRECTION('center_axis',(-1.,0.,0.));
#110751=DIRECTION('ref_axis',(0.,-1.,0.));
#110752=DIRECTION('',(1.,-4.38004274807345E-16,0.));
#110753=DIRECTION('center_axis',(0.,-7.60037129918555E-33,1.));
#110754=DIRECTION('ref_axis',(1.,0.,0.));
#110755=DIRECTION('center_axis',(0.,0.,1.));
#110756=DIRECTION('ref_axis',(1.,0.,0.));
#110757=DIRECTION('',(1.73522765332109E-17,-7.36595663150706E-33,1.));
#110758=DIRECTION('',(-1.73522765332109E-17,7.60037129918555E-33,-1.));
#110759=DIRECTION('center_axis',(-0.460817663464343,0.,0.887494834373285));
#110760=DIRECTION('ref_axis',(0.887494834373285,0.,0.460817663464343));
#110761=DIRECTION('center_axis',(-0.661718432379332,0.,0.749752436641215));
#110762=DIRECTION('ref_axis',(0.749752436641215,0.,0.661718432379332));
#110763=DIRECTION('center_axis',(-0.48375308397303,0.,0.875204521095831));
#110764=DIRECTION('ref_axis',(0.875204521095831,0.,0.48375308397303));
#110765=DIRECTION('center_axis',(0.,0.,1.));
#110766=DIRECTION('ref_axis',(1.,0.,0.));
#110767=DIRECTION('center_axis',(0.,0.,-1.));
#110768=DIRECTION('ref_axis',(-1.,0.,0.));
#110769=DIRECTION('center_axis',(0.,0.,1.));
#110770=DIRECTION('ref_axis',(1.,0.,0.));
#110771=DIRECTION('',(0.,0.,-1.));
#110772=DIRECTION('center_axis',(0.483753083973024,0.,0.875204521095834));
#110773=DIRECTION('ref_axis',(0.875204521095834,0.,-0.483753083973024));
#110774=DIRECTION('center_axis',(0.460985151818831,0.,0.887407848625743));
#110775=DIRECTION('ref_axis',(0.887407848625743,0.,-0.460985151818831));
#110776=DIRECTION('center_axis',(0.,0.,-1.));
#110777=DIRECTION('ref_axis',(-1.,0.,0.));
#110778=DIRECTION('center_axis',(0.,0.,-1.));
#110779=DIRECTION('ref_axis',(-1.,0.,0.));
#110780=DIRECTION('',(0.,0.,1.));
#110781=DIRECTION('center_axis',(0.,0.,-1.));
#110782=DIRECTION('ref_axis',(-1.,0.,0.));
#110783=DIRECTION('center_axis',(4.18005656861882E-16,1.,0.));
#110784=DIRECTION('ref_axis',(-1.,0.,0.));
#110785=DIRECTION('center_axis',(0.,-1.,0.));
#110786=DIRECTION('ref_axis',(-1.,0.,0.));
#110787=DIRECTION('center_axis',(-1.,0.,0.));
#110788=DIRECTION('ref_axis',(0.,0.,1.));
#110789=DIRECTION('center_axis',(1.,0.,0.));
#110790=DIRECTION('ref_axis',(0.,1.,0.));
#110791=DIRECTION('',(1.,-4.18005656861881E-16,0.));
#110792=DIRECTION('center_axis',(0.,0.,1.));
#110793=DIRECTION('ref_axis',(0.,-1.,0.));
#110794=DIRECTION('center_axis',(0.,0.,1.));
#110795=DIRECTION('ref_axis',(1.,0.,0.));
#110796=DIRECTION('',(0.,-1.23467863058847E-16,1.));
#110797=DIRECTION('',(-5.16102651992463E-32,2.15733828054269E-47,-1.));
#110798=DIRECTION('center_axis',(0.817080261705548,0.,0.576523933528517));
#110799=DIRECTION('ref_axis',(0.576523933528517,0.,-0.817080261705548));
#110800=DIRECTION('center_axis',(0.214170029765708,0.976796000598309,0.000878387901143853));
#110801=DIRECTION('ref_axis',(0.840875521369131,-0.184825863749487,0.50869220325404));
#110802=DIRECTION('center_axis',(0.,-1.,0.));
#110803=DIRECTION('ref_axis',(0.979462303532354,0.,0.201627369072492));
#110804=DIRECTION('center_axis',(0.,-1.18842113532926E-16,1.));
#110805=DIRECTION('ref_axis',(0.,1.,1.18842113532926E-16));
#110806=DIRECTION('center_axis',(0.,1.19392659184112E-16,-1.));
#110807=DIRECTION('ref_axis',(0.,1.,1.19392659184112E-16));
#110808=DIRECTION('center_axis',(-4.18005656861882E-16,-1.,0.));
#110809=DIRECTION('ref_axis',(1.,0.,0.));
#110810=DIRECTION('center_axis',(1.,0.,0.));
#110811=DIRECTION('ref_axis',(0.,0.,-1.));
#110812=DIRECTION('center_axis',(0.,1.,0.));
#110813=DIRECTION('ref_axis',(1.,0.,0.));
#110814=DIRECTION('center_axis',(0.,0.,1.));
#110815=DIRECTION('ref_axis',(1.,0.,0.));
#110816=DIRECTION('center_axis',(0.,0.,1.));
#110817=DIRECTION('ref_axis',(1.,0.,0.));
#110818=DIRECTION('',(0.,0.,-1.));
#110819=DIRECTION('center_axis',(0.,0.,1.));
#110820=DIRECTION('ref_axis',(1.,0.,0.));
#110821=DIRECTION('center_axis',(-0.49549481432688,0.,-0.868610896187223));
#110822=DIRECTION('ref_axis',(-0.868610896187223,0.,0.49549481432688));
#110823=DIRECTION('center_axis',(-1.,0.,0.));
#110824=DIRECTION('ref_axis',(0.,0.,1.));
#110825=DIRECTION('center_axis',(-0.517480097905755,0.,-0.855695242636916));
#110826=DIRECTION('ref_axis',(-0.855695242636916,0.,0.517480097905755));
#110827=DIRECTION('center_axis',(-1.11022302462516E-12,0.,-1.));
#110828=DIRECTION('ref_axis',(-1.,0.,1.11022302462516E-12));
#110829=DIRECTION('center_axis',(0.,0.,1.));
#110830=DIRECTION('ref_axis',(1.,0.,0.));
#110831=DIRECTION('center_axis',(0.,0.,-1.));
#110832=DIRECTION('ref_axis',(-1.,0.,0.));
#110833=DIRECTION('',(0.,0.,1.));
#110834=DIRECTION('center_axis',(0.517480097907924,0.,-0.855695242635604));
#110835=DIRECTION('ref_axis',(-0.855695242635604,0.,-0.517480097907924));
#110836=DIRECTION('center_axis',(0.495139693244723,0.,-0.868813377068702));
#110837=DIRECTION('ref_axis',(-0.868813377068702,0.,-0.495139693244723));
#110838=DIRECTION('center_axis',(1.,0.,0.));
#110839=DIRECTION('ref_axis',(0.,0.,-1.));
#110840=DIRECTION('center_axis',(-1.,4.1800565686188E-16,5.16102651992463E-32));
#110841=DIRECTION('ref_axis',(-4.1800565686188E-16,-1.,8.08534226092968E-63));
#110842=DIRECTION('center_axis',(1.,0.,0.));
#110843=DIRECTION('ref_axis',(0.,0.,-1.));
#110844=DIRECTION('',(-1.,4.18005656861881E-16,5.16102651992463E-32));
#110845=DIRECTION('center_axis',(0.,0.,-1.));
#110846=DIRECTION('ref_axis',(-1.,0.,0.));
#110847=DIRECTION('center_axis',(0.,-7.25334975031394E-33,-1.));
#110848=DIRECTION('ref_axis',(-1.,0.,0.));
#110849=DIRECTION('',(1.73522765332111E-17,-6.55191041448207E-33,-1.));
#110850=DIRECTION('',(-1.73522765332111E-17,7.25334975031394E-33,1.));
#110851=DIRECTION('center_axis',(1.,0.,0.));
#110852=DIRECTION('ref_axis',(0.,1.,0.));
#110853=DIRECTION('',(-1.,4.18005656861881E-16,0.));
#110854=DIRECTION('center_axis',(-4.18005656861882E-16,-1.,0.));
#110855=DIRECTION('ref_axis',(1.,0.,0.));
#110856=DIRECTION('center_axis',(0.,1.,0.));
#110857=DIRECTION('ref_axis',(1.,0.,0.));
#110858=DIRECTION('center_axis',(-1.,0.,0.));
#110859=DIRECTION('ref_axis',(0.,0.,1.));
#110860=DIRECTION('center_axis',(0.,-1.,0.));
#110861=DIRECTION('ref_axis',(1.,0.,0.));
#110862=DIRECTION('center_axis',(4.18005656861881E-16,1.,0.));
#110863=DIRECTION('ref_axis',(-1.,4.18005656861881E-16,0.));
#110864=DIRECTION('',(4.18005656861881E-16,1.,0.));
#110865=DIRECTION('center_axis',(0.,1.,0.));
#110866=DIRECTION('ref_axis',(-1.,0.,0.));
#110867=DIRECTION('center_axis',(4.18005656861882E-16,1.,0.));
#110868=DIRECTION('ref_axis',(-1.,0.,0.));
#110869=DIRECTION('center_axis',(1.,0.,0.));
#110870=DIRECTION('ref_axis',(0.,0.,-1.));
#110871=DIRECTION('center_axis',(0.,-1.,0.));
#110872=DIRECTION('ref_axis',(-1.,0.,0.));
#110873=DIRECTION('center_axis',(0.,0.,-1.));
#110874=DIRECTION('ref_axis',(-1.,0.,0.));
#110875=DIRECTION('center_axis',(0.,0.,-1.));
#110876=DIRECTION('ref_axis',(-1.,0.,0.));
#110877=DIRECTION('',(0.,0.,1.));
#110878=DIRECTION('center_axis',(0.,0.,-1.));
#110879=DIRECTION('ref_axis',(-1.,0.,0.));
#110880=DIRECTION('center_axis',(4.18005656861882E-16,1.,0.));
#110881=DIRECTION('ref_axis',(-1.,0.,0.));
#110882=DIRECTION('center_axis',(0.,-1.,0.));
#110883=DIRECTION('ref_axis',(-1.,0.,0.));
#110884=DIRECTION('center_axis',(-1.,0.,0.));
#110885=DIRECTION('ref_axis',(0.,0.,1.));
#110886=DIRECTION('center_axis',(1.,0.,0.));
#110887=DIRECTION('ref_axis',(0.,1.,0.));
#110888=DIRECTION('',(1.,-4.18005656861881E-16,0.));
#110889=DIRECTION('center_axis',(0.,7.25334975031394E-33,1.));
#110890=DIRECTION('ref_axis',(-0.754709580222751,0.656059028990531,-4.75862559411968E-33));
#110891=DIRECTION('',(1.73522765332111E-17,-7.25334975031394E-33,-1.));
#110892=DIRECTION('center_axis',(0.,0.,-1.));
#110893=DIRECTION('ref_axis',(-1.,0.,0.));
#110894=DIRECTION('',(-1.73522765332111E-17,6.55191041448207E-33,1.));
#110895=DIRECTION('center_axis',(1.,0.,0.));
#110896=DIRECTION('ref_axis',(0.,0.,-1.));
#110897=DIRECTION('center_axis',(1.,-4.1800565686188E-16,-5.16102651992463E-32));
#110898=DIRECTION('ref_axis',(4.1800565686188E-16,1.,-8.08534226092968E-63));
#110899=DIRECTION('',(1.,-4.18005656861881E-16,-5.16102651992463E-32));
#110900=DIRECTION('center_axis',(1.,0.,0.));
#110901=DIRECTION('ref_axis',(0.,0.,-1.));
#110902=DIRECTION('center_axis',(0.482476521947278,1.33914135876736E-14,
-0.875908902666058));
#110903=DIRECTION('ref_axis',(-0.875908902666058,-3.49403168495695E-30,
-0.482476521947278));
#110904=DIRECTION('center_axis',(0.50653821035484,0.,-0.862217514001262));
#110905=DIRECTION('ref_axis',(-0.862217514001262,0.,-0.50653821035484));
#110906=DIRECTION('center_axis',(0.,0.,-1.));
#110907=DIRECTION('ref_axis',(-1.,0.,0.));
#110908=DIRECTION('center_axis',(0.,0.,-1.));
#110909=DIRECTION('ref_axis',(-1.,0.,0.));
#110910=DIRECTION('',(0.,0.,-1.));
#110911=DIRECTION('center_axis',(0.,-1.77635683940025E-12,-1.));
#110912=DIRECTION('ref_axis',(0.,1.,-1.77635683940025E-12));
#110913=DIRECTION('center_axis',(-0.506538210354814,0.,-0.862217514001277));
#110914=DIRECTION('ref_axis',(-0.862217514001277,0.,0.506538210354814));
#110915=DIRECTION('center_axis',(-0.482758140724685,1.88531393333386E-14,
-0.875753719697522));
#110916=DIRECTION('ref_axis',(-0.875753719697522,-7.73315028487173E-30,
0.482758140724685));
#110917=DIRECTION('center_axis',(-1.,0.,5.16102651992463E-32));
#110918=DIRECTION('ref_axis',(0.,-1.,0.));
#110919=DIRECTION('center_axis',(-1.,0.,0.));
#110920=DIRECTION('ref_axis',(0.,0.,1.));
#110921=DIRECTION('',(-1.,4.18005656861881E-16,5.16102651992463E-32));
#110922=DIRECTION('center_axis',(-1.,0.,0.));
#110923=DIRECTION('ref_axis',(0.,0.,1.));
#110924=DIRECTION('',(1.,-4.18005656861881E-16,-5.16102651992463E-32));
#110925=DIRECTION('center_axis',(0.,-1.18842113532926E-16,1.));
#110926=DIRECTION('ref_axis',(0.,1.,1.18842113532926E-16));
#110927=DIRECTION('center_axis',(0.,1.19392659184112E-16,-1.));
#110928=DIRECTION('ref_axis',(0.,1.,1.19392659184112E-16));
#110929=DIRECTION('center_axis',(-4.18005656861882E-16,-1.,0.));
#110930=DIRECTION('ref_axis',(1.,-5.9211894646675E-16,0.));
#110931=DIRECTION('center_axis',(1.,0.,0.));
#110932=DIRECTION('ref_axis',(0.,0.,-1.));
#110933=DIRECTION('center_axis',(6.93889390390722E-16,1.,0.));
#110934=DIRECTION('ref_axis',(1.,-6.93889390390722E-16,0.));
#110935=DIRECTION('center_axis',(0.,0.,1.));
#110936=DIRECTION('ref_axis',(1.,0.,0.));
#110937=DIRECTION('center_axis',(0.,0.,1.));
#110938=DIRECTION('ref_axis',(1.,0.,0.));
#110939=DIRECTION('',(0.,0.,-1.));
#110940=DIRECTION('center_axis',(0.,0.,1.));
#110941=DIRECTION('ref_axis',(1.,0.,0.));
#110942=DIRECTION('center_axis',(0.403600920616143,3.09956391918065E-14,
0.91493513260657));
#110943=DIRECTION('ref_axis',(0.91493513260657,-7.63177238048844E-30,-0.403600920616143));
#110944=DIRECTION('center_axis',(0.,-1.,0.));
#110945=DIRECTION('ref_axis',(-0.285513245062781,0.,-0.9583747632809));
#110946=DIRECTION('center_axis',(0.782801330915055,1.71942202750291E-12,
0.622271706184379));
#110947=DIRECTION('ref_axis',(0.622271706184379,-5.64324648533862E-28,-0.782801330915055));
#110948=DIRECTION('center_axis',(0.,1.,0.));
#110949=DIRECTION('ref_axis',(0.882822386979436,0.,-0.469706965083476));
#110950=DIRECTION('center_axis',(0.460227641765603,1.23207131288176E-14,
0.887800944894108));
#110951=DIRECTION('ref_axis',(0.887800944894108,7.43200893707752E-29,-0.460227641765603));
#110952=DIRECTION('center_axis',(0.213575684387547,-0.976926520634823,-1.78530135123478E-5));
#110953=DIRECTION('ref_axis',(0.953391643317273,0.20842650212588,0.218180584984919));
#110954=DIRECTION('center_axis',(0.482846004726866,0.,0.875705279029025));
#110955=DIRECTION('ref_axis',(0.875705279029025,0.,-0.482846004726866));
#110956=DIRECTION('center_axis',(0.,0.,1.));
#110957=DIRECTION('ref_axis',(1.,0.,0.));
#110958=DIRECTION('center_axis',(0.,0.,1.));
#110959=DIRECTION('ref_axis',(1.,0.,0.));
#110960=DIRECTION('',(0.,0.,1.));
#110961=DIRECTION('center_axis',(0.,0.,1.));
#110962=DIRECTION('ref_axis',(1.,0.,0.));
#110963=DIRECTION('center_axis',(-0.482846004727867,1.73271215008562E-12,
0.875705279028473));
#110964=DIRECTION('ref_axis',(0.875705279028473,2.53817490248555E-28,0.482846004727867));
#110965=DIRECTION('center_axis',(-0.460063868749635,6.3846687485495E-15,
0.887885824118799));
#110966=DIRECTION('ref_axis',(0.887885824118799,1.45303619130616E-30,0.460063868749635));
#110967=DIRECTION('center_axis',(-0.639652375806928,0.,0.768664320834884));
#110968=DIRECTION('ref_axis',(0.768664320834884,0.,0.639652375806928));
#110969=DIRECTION('center_axis',(0.,0.,1.));
#110970=DIRECTION('ref_axis',(1.,0.,0.));
#110971=DIRECTION('center_axis',(0.,0.,1.));
#110972=DIRECTION('ref_axis',(0.,-1.,0.));
#110973=DIRECTION('',(5.16102651992463E-32,-2.15733828054269E-47,1.));
#110974=DIRECTION('',(0.,1.23467863058847E-16,-1.));
#110975=DIRECTION('center_axis',(1.,0.,0.));
#110976=DIRECTION('ref_axis',(0.,1.,0.));
#110977=DIRECTION('',(-1.,4.18005656861881E-16,0.));
#110978=DIRECTION('center_axis',(1.,0.,-5.40794518211031E-32));
#110979=DIRECTION('ref_axis',(0.,1.,0.));
#110980=DIRECTION('',(1.,-4.38004274807345E-16,-5.40794518211031E-32));
#110981=DIRECTION('',(-1.,4.38004274807345E-16,5.40794518211031E-32));
#110982=DIRECTION('center_axis',(1.,0.,-4.33680868994201E-16));
#110983=DIRECTION('ref_axis',(0.,1.,0.));
#110984=DIRECTION('center_axis',(1.,0.,-5.40794518211031E-32));
#110985=DIRECTION('ref_axis',(0.,1.,0.));
#110986=DIRECTION('center_axis',(1.,0.,0.));
#110987=DIRECTION('ref_axis',(0.,0.,-1.));
#110988=DIRECTION('',(1.,-4.38004274807345E-16,-5.40794518211031E-32));
#110989=DIRECTION('center_axis',(1.,0.,0.));
#110990=DIRECTION('ref_axis',(0.,0.,-1.));
#110991=DIRECTION('',(-1.,4.38004274807345E-16,5.40794518211031E-32));
#110992=DIRECTION('center_axis',(0.,0.,-1.));
#110993=DIRECTION('ref_axis',(-1.,0.,0.));
#110994=DIRECTION('center_axis',(0.,-7.60037129918566E-33,-1.));
#110995=DIRECTION('ref_axis',(-1.,0.,0.));
#110996=DIRECTION('',(1.73522765332111E-17,-6.93709640335951E-33,-1.));
#110997=DIRECTION('',(-1.73522765332111E-17,7.60037129918566E-33,1.));
#110998=DIRECTION('center_axis',(-1.,0.,0.));
#110999=DIRECTION('ref_axis',(0.,-1.,0.));
#111000=DIRECTION('',(-1.,4.38004274807345E-16,0.));
#111001=DIRECTION('center_axis',(1.,0.,0.));
#111002=DIRECTION('ref_axis',(0.,0.,-1.));
#111003=DIRECTION('center_axis',(-4.38004274807345E-16,-1.,0.));
#111004=DIRECTION('ref_axis',(1.,0.,0.));
#111005=DIRECTION('center_axis',(0.,1.,0.));
#111006=DIRECTION('ref_axis',(1.,0.,0.));
#111007=DIRECTION('center_axis',(0.,0.,1.));
#111008=DIRECTION('ref_axis',(1.,0.,0.));
#111009=DIRECTION('center_axis',(0.,0.,-1.));
#111010=DIRECTION('ref_axis',(-1.,0.,0.));
#111011=DIRECTION('',(0.,0.,-1.));
#111012=DIRECTION('center_axis',(0.,0.,1.));
#111013=DIRECTION('ref_axis',(1.,0.,0.));
#111014=DIRECTION('center_axis',(-1.,4.38004274807345E-16,0.));
#111015=DIRECTION('ref_axis',(0.,0.,-1.));
#111016=DIRECTION('center_axis',(1.,-4.38004274807345E-16,4.02455846426619E-13));
#111017=DIRECTION('ref_axis',(4.02455846426619E-13,-4.48415508583941E-44,
-1.));
#111018=DIRECTION('center_axis',(0.,0.,1.));
#111019=DIRECTION('ref_axis',(0.,-1.,0.));
#111020=DIRECTION('',(5.40794518211031E-32,-2.3687031076881E-47,1.));
#111021=DIRECTION('center_axis',(-1.71346080461497E-30,-2.37790454634537E-44,
1.));
#111022=DIRECTION('ref_axis',(-1.38777878078144E-14,1.,2.48920611114446E-59));
#111023=DIRECTION('center_axis',(-4.38004274807345E-16,-1.,0.));
#111024=DIRECTION('ref_axis',(1.,0.,0.));
#111025=DIRECTION('center_axis',(0.,1.,0.));
#111026=DIRECTION('ref_axis',(1.,0.,0.));
#111027=DIRECTION('center_axis',(-1.,0.,0.));
#111028=DIRECTION('ref_axis',(0.,0.,1.));
#111029=DIRECTION('center_axis',(0.,-1.,0.));
#111030=DIRECTION('ref_axis',(1.,0.,0.));
#111031=DIRECTION('center_axis',(4.18005656861881E-16,1.,0.));
#111032=DIRECTION('ref_axis',(-1.,4.18005656861881E-16,0.));
#111033=DIRECTION('',(4.18005656861881E-16,1.,0.));
#111034=DIRECTION('center_axis',(0.,1.,0.));
#111035=DIRECTION('ref_axis',(-1.,0.,0.));
#111036=DIRECTION('center_axis',(-1.,0.,5.16102651992463E-32));
#111037=DIRECTION('ref_axis',(0.,-1.,0.));
#111038=DIRECTION('center_axis',(-1.,0.,0.));
#111039=DIRECTION('ref_axis',(0.,0.,1.));
#111040=DIRECTION('center_axis',(-1.,0.,0.));
#111041=DIRECTION('ref_axis',(0.,0.,1.));
#111042=DIRECTION('',(1.,-4.18005656861881E-16,-5.16102651992463E-32));
#111043=DIRECTION('center_axis',(-0.532459169918176,0.,0.846455688367706));
#111044=DIRECTION('ref_axis',(0.846455688367706,0.,0.532459169918176));
#111045=DIRECTION('center_axis',(-0.542737080693356,0.,0.839902649859169));
#111046=DIRECTION('ref_axis',(0.839902649859169,0.,0.542737080693356));
#111047=DIRECTION('center_axis',(0.,0.,1.));
#111048=DIRECTION('ref_axis',(1.,0.,0.));
#111049=DIRECTION('center_axis',(0.,0.,-1.));
#111050=DIRECTION('ref_axis',(-1.,0.,0.));
#111051=DIRECTION('center_axis',(-1.11022302462516E-13,0.,1.));
#111052=DIRECTION('ref_axis',(1.,0.,1.11022302462516E-13));
#111053=DIRECTION('',(0.,0.,-1.));
#111054=DIRECTION('center_axis',(0.542737080693052,0.,0.839902649859366));
#111055=DIRECTION('ref_axis',(0.839902649859366,0.,-0.542737080693052));
#111056=DIRECTION('center_axis',(0.533061469511947,0.,0.846076515287928));
#111057=DIRECTION('ref_axis',(0.846076515287928,0.,-0.533061469511947));
#111058=DIRECTION('center_axis',(1.,0.,0.));
#111059=DIRECTION('ref_axis',(0.,0.,-1.));
#111060=DIRECTION('center_axis',(4.18005656861882E-16,1.,0.));
#111061=DIRECTION('ref_axis',(-1.,0.,0.));
#111062=DIRECTION('center_axis',(1.,0.,0.));
#111063=DIRECTION('ref_axis',(0.,0.,-1.));
#111064=DIRECTION('center_axis',(0.,-1.,0.));
#111065=DIRECTION('ref_axis',(-1.,0.,0.));
#111066=DIRECTION('center_axis',(0.,0.,-1.));
#111067=DIRECTION('ref_axis',(-1.,0.,0.));
#111068=DIRECTION('center_axis',(0.,0.,-1.));
#111069=DIRECTION('ref_axis',(-1.,0.,0.));
#111070=DIRECTION('',(0.,0.,1.));
#111071=DIRECTION('center_axis',(0.,0.,-1.));
#111072=DIRECTION('ref_axis',(-1.,0.,0.));
#111073=DIRECTION('center_axis',(4.18005656861882E-16,1.,0.));
#111074=DIRECTION('ref_axis',(-1.,0.,0.));
#111075=DIRECTION('center_axis',(0.,-1.,0.));
#111076=DIRECTION('ref_axis',(-1.,0.,0.));
#111077=DIRECTION('center_axis',(-1.,0.,0.));
#111078=DIRECTION('ref_axis',(0.,0.,1.));
#111079=DIRECTION('center_axis',(1.,0.,0.));
#111080=DIRECTION('ref_axis',(0.,1.,0.));
#111081=DIRECTION('',(1.,-4.18005656861881E-16,0.));
#111082=DIRECTION('center_axis',(0.,-7.68642463345396E-33,-1.));
#111083=DIRECTION('ref_axis',(-1.,0.,0.));
#111084=DIRECTION('center_axis',(0.,0.,1.));
#111085=DIRECTION('ref_axis',(1.,0.,0.));
#111086=DIRECTION('',(-1.73522765332111E-17,6.93709640335951E-33,1.));
#111087=DIRECTION('',(1.73522765332111E-17,-7.25334975031394E-33,-1.));
#111088=DIRECTION('center_axis',(0.,0.,1.));
#111089=DIRECTION('ref_axis',(1.,0.,0.));
#111090=DIRECTION('center_axis',(1.,0.,-5.16102651992463E-32));
#111091=DIRECTION('ref_axis',(0.,1.,0.));
#111092=DIRECTION('',(-1.,4.18005656861881E-16,5.16102651992463E-32));
#111093=DIRECTION('center_axis',(-1.,0.,0.));
#111094=DIRECTION('ref_axis',(0.,0.,1.));
#111095=DIRECTION('',(1.,-4.18005656861881E-16,-5.16102651992463E-32));
#111096=DIRECTION('center_axis',(1.,-4.1800565686188E-16,-5.16102651992463E-32));
#111097=DIRECTION('ref_axis',(4.1800565686188E-16,1.,-8.08534226092968E-63));
#111098=DIRECTION('center_axis',(1.,0.,0.));
#111099=DIRECTION('ref_axis',(0.,0.,-1.));
#111100=DIRECTION('',(1.,-4.18005656861881E-16,-5.16102651992463E-32));
#111101=DIRECTION('',(-1.,4.18005656861881E-16,5.16102651992463E-32));
#111102=DIRECTION('center_axis',(0.,1.23467863058847E-16,-1.));
#111103=DIRECTION('ref_axis',(0.,1.,1.1837531408762E-16));
#111104=DIRECTION('center_axis',(5.24775676075252E-32,-1.17559414210783E-16,
1.));
#111105=DIRECTION('ref_axis',(8.88178419700125E-15,1.,1.17559414210783E-16));
#111106=DIRECTION('center_axis',(0.,1.,0.));
#111107=DIRECTION('ref_axis',(0.,0.,1.));
#111108=DIRECTION('center_axis',(-1.90454958189083E-14,0.515457402104623,
0.856915203865326));
#111109=DIRECTION('ref_axis',(1.04773227122123E-29,-0.856915203865326,0.515457402104623));
#111110=DIRECTION('center_axis',(-1.44372869288582E-12,0.522894079854115,
0.852397666147391));
#111111=DIRECTION('ref_axis',(4.54659658509035E-27,-0.852397666147391,0.522894079854115));
#111112=DIRECTION('center_axis',(0.,0.,1.));
#111113=DIRECTION('ref_axis',(1.,0.,0.));
#111114=DIRECTION('center_axis',(0.,8.19208946723988E-32,1.));
#111115=DIRECTION('ref_axis',(1.,0.,0.));
#111116=DIRECTION('',(-1.87032180698308E-16,8.19208946723987E-32,1.));
#111117=DIRECTION('center_axis',(0.,0.,1.));
#111118=DIRECTION('ref_axis',(1.,0.,0.));
#111119=DIRECTION('',(1.87032180698308E-16,-8.19208946723987E-32,-1.));
#111120=DIRECTION('center_axis',(1.,0.,1.87032180698308E-16));
#111121=DIRECTION('ref_axis',(0.,0.,-1.));
#111122=DIRECTION('center_axis',(0.,0.,1.));
#111123=DIRECTION('ref_axis',(1.,0.,0.));
#111124=DIRECTION('center_axis',(-1.,0.,0.));
#111125=DIRECTION('ref_axis',(0.,0.,-1.));
#111126=DIRECTION('center_axis',(0.,-1.,0.));
#111127=DIRECTION('ref_axis',(0.,0.,-1.));
#111128=DIRECTION('center_axis',(1.,0.,0.));
#111129=DIRECTION('ref_axis',(0.,0.,-1.));
#111130=DIRECTION('center_axis',(-1.,0.,0.));
#111131=DIRECTION('ref_axis',(0.,0.,1.));
#111132=DIRECTION('',(-1.,0.,0.));
#111133=DIRECTION('center_axis',(-1.,0.,0.));
#111134=DIRECTION('ref_axis',(0.,1.,0.));
#111135=DIRECTION('',(1.,0.,0.));
#111136=DIRECTION('center_axis',(1.,-4.38004274807345E-16,0.));
#111137=DIRECTION('ref_axis',(0.,1.,0.));
#111138=DIRECTION('center_axis',(0.,1.,0.));
#111139=DIRECTION('ref_axis',(0.,0.,1.));
#111140=DIRECTION('center_axis',(1.,0.,0.));
#111141=DIRECTION('ref_axis',(0.,1.,0.));
#111142=DIRECTION('center_axis',(0.,0.,-1.));
#111143=DIRECTION('ref_axis',(-1.,0.,0.));
#111144=DIRECTION('center_axis',(0.,0.,1.));
#111145=DIRECTION('ref_axis',(1.,0.,0.));
#111146=DIRECTION('',(0.,0.,1.));
#111147=DIRECTION('',(0.,0.,-1.));
#111148=DIRECTION('center_axis',(0.,0.,1.));
#111149=DIRECTION('ref_axis',(0.,-1.,0.));
#111150=DIRECTION('',(5.40794518211031E-32,1.23467863058847E-16,-1.));
#111151=DIRECTION('center_axis',(-8.56730402307488E-31,-5.94476136586342E-45,
1.));
#111152=DIRECTION('ref_axis',(-6.93889390390722E-15,1.,9.95682444457783E-60));
#111153=DIRECTION('center_axis',(-1.22429528305785E-14,0.470879150309884,
0.882197724891332));
#111154=DIRECTION('ref_axis',(1.13789948105108E-30,-0.882197724891332,0.470879150309884));
#111155=DIRECTION('center_axis',(0.,0.488256551855887,0.872700142987154));
#111156=DIRECTION('ref_axis',(0.,-0.872700142987154,0.488256551855887));
#111157=DIRECTION('center_axis',(0.,0.,1.));
#111158=DIRECTION('ref_axis',(1.,0.,0.));
#111159=DIRECTION('center_axis',(0.,8.19208946723987E-32,1.));
#111160=DIRECTION('ref_axis',(1.,0.,0.));
#111161=DIRECTION('',(-1.87032180698308E-16,8.19208946723987E-32,1.));
#111162=DIRECTION('center_axis',(0.,0.,1.));
#111163=DIRECTION('ref_axis',(1.,0.,0.));
#111164=DIRECTION('',(1.87032180698308E-16,-8.19208946723987E-32,-1.));
#111165=DIRECTION('center_axis',(1.,0.,1.87032180698308E-16));
#111166=DIRECTION('ref_axis',(0.,0.,-1.));
#111167=DIRECTION('center_axis',(0.,0.,1.));
#111168=DIRECTION('ref_axis',(1.,0.,0.));
#111169=DIRECTION('center_axis',(-1.,0.,0.));
#111170=DIRECTION('ref_axis',(0.,0.,-1.));
#111171=DIRECTION('center_axis',(0.,-1.,0.));
#111172=DIRECTION('ref_axis',(0.,0.,-1.));
#111173=DIRECTION('center_axis',(1.,0.,0.));
#111174=DIRECTION('ref_axis',(0.,0.,-1.));
#111175=DIRECTION('center_axis',(-1.,0.,0.));
#111176=DIRECTION('ref_axis',(0.,0.,1.));
#111177=DIRECTION('',(1.,0.,0.));
#111178=DIRECTION('',(-1.,0.,0.));
#111179=DIRECTION('center_axis',(-1.,0.,0.));
#111180=DIRECTION('ref_axis',(0.,0.,1.));
#111181=DIRECTION('center_axis',(-1.,0.,0.));
#111182=DIRECTION('ref_axis',(0.,0.,1.));
#111183=DIRECTION('center_axis',(0.,1.,0.));
#111184=DIRECTION('ref_axis',(0.,0.,1.));
#111185=DIRECTION('center_axis',(1.,0.,0.));
#111186=DIRECTION('ref_axis',(0.,0.,1.));
#111187=DIRECTION('center_axis',(0.,0.,-1.));
#111188=DIRECTION('ref_axis',(-1.,0.,0.));
#111189=DIRECTION('center_axis',(0.,0.,-1.));
#111190=DIRECTION('ref_axis',(-1.,0.,0.));
#111191=DIRECTION('center_axis',(0.,0.,1.));
#111192=DIRECTION('ref_axis',(1.,0.,0.));
#111193=DIRECTION('',(0.,0.,1.));
#111194=DIRECTION('center_axis',(0.,0.,1.));
#111195=DIRECTION('ref_axis',(1.,0.,0.));
#111196=DIRECTION('',(0.,0.,-1.));
#111197=DIRECTION('center_axis',(0.,0.498146280733357,0.867093007117186));
#111198=DIRECTION('ref_axis',(0.,-0.867093007117186,0.498146280733357));
#111199=DIRECTION('center_axis',(0.,0.481647286662901,0.876365158624112));
#111200=DIRECTION('ref_axis',(0.,-0.876365158624112,0.481647286662901));
#111201=DIRECTION('center_axis',(0.,1.,0.));
#111202=DIRECTION('ref_axis',(0.,0.,1.));
#111203=DIRECTION('center_axis',(2.30924636740563E-32,-1.,0.));
#111204=DIRECTION('ref_axis',(0.,0.,-1.));
#111205=DIRECTION('center_axis',(0.,1.,0.));
#111206=DIRECTION('ref_axis',(0.,0.,1.));
#111207=DIRECTION('',(-2.30924636740563E-32,1.,1.23467863058847E-16));
#111208=DIRECTION('',(2.30924636740563E-32,-1.,-1.23467863058847E-16));
#111209=DIRECTION('center_axis',(0.,-1.,0.));
#111210=DIRECTION('ref_axis',(0.,0.,-1.));
#111211=DIRECTION('center_axis',(0.,1.,0.));
#111212=DIRECTION('ref_axis',(0.,0.,1.));
#111213=DIRECTION('',(0.,1.,1.23467863058847E-16));
#111214=DIRECTION('',(0.,-1.,-1.23467863058847E-16));
#111215=DIRECTION('center_axis',(0.,1.23467863058847E-16,-1.));
#111216=DIRECTION('ref_axis',(0.,1.,1.1837531408762E-16));
#111217=DIRECTION('center_axis',(2.62387838037626E-32,-1.17559414210783E-16,
1.));
#111218=DIRECTION('ref_axis',(4.44089209850062E-15,1.,1.17559414210783E-16));
#111219=DIRECTION('center_axis',(-1.,5.01606788234257E-16,0.));
#111220=DIRECTION('ref_axis',(0.,-1.,0.));
#111221=DIRECTION('center_axis',(0.,-1.,0.));
#111222=DIRECTION('ref_axis',(0.,0.,-1.));
#111223=DIRECTION('center_axis',(1.,0.,0.));
#111224=DIRECTION('ref_axis',(0.,-1.,0.));
#111225=DIRECTION('center_axis',(0.,0.,1.));
#111226=DIRECTION('ref_axis',(1.,0.,0.));
#111227=DIRECTION('center_axis',(2.85977186515575E-47,0.,1.));
#111228=DIRECTION('ref_axis',(0.,-1.,0.));
#111229=DIRECTION('',(-2.85977186515575E-47,-5.70122241611331E-32,-1.));
#111230=DIRECTION('center_axis',(0.,0.,1.));
#111231=DIRECTION('ref_axis',(1.,0.,0.));
#111232=DIRECTION('center_axis',(0.,0.496115977596257,-0.868256262156346));
#111233=DIRECTION('ref_axis',(0.,0.868256262156346,0.496115977596257));
#111234=DIRECTION('center_axis',(0.,1.,0.));
#111235=DIRECTION('ref_axis',(0.,0.,1.));
#111236=DIRECTION('center_axis',(0.,0.509034676477531,-0.860746012563181));
#111237=DIRECTION('ref_axis',(0.,0.860746012563181,0.509034676477531));
#111238=DIRECTION('center_axis',(0.,1.9151347174784E-12,-1.));
#111239=DIRECTION('ref_axis',(0.,1.,1.9151347174784E-12));
#111240=DIRECTION('center_axis',(0.,0.,1.));
#111241=DIRECTION('ref_axis',(1.,0.,0.));
#111242=DIRECTION('center_axis',(0.,0.,-1.));
#111243=DIRECTION('ref_axis',(-1.,0.,0.));
#111244=DIRECTION('',(0.,0.,1.));
#111245=DIRECTION('center_axis',(0.,-0.509034676478003,-0.860746012562902));
#111246=DIRECTION('ref_axis',(0.,0.860746012562902,-0.509034676478003));
#111247=DIRECTION('center_axis',(0.,-0.495757141593727,-0.86846120037617));
#111248=DIRECTION('ref_axis',(0.,0.86846120037617,-0.495757141593727));
#111249=DIRECTION('center_axis',(0.,-1.,0.));
#111250=DIRECTION('ref_axis',(0.,0.,-1.));
#111251=DIRECTION('center_axis',(0.,1.,1.23467863058847E-16));
#111252=DIRECTION('ref_axis',(-1.,0.,0.));
#111253=DIRECTION('center_axis',(0.,-1.,0.));
#111254=DIRECTION('ref_axis',(0.,0.,-1.));
#111255=DIRECTION('',(5.01606788234257E-16,1.,1.23467863058847E-16));
#111256=DIRECTION('center_axis',(0.,0.,-1.));
#111257=DIRECTION('ref_axis',(-1.,0.,0.));
#111258=DIRECTION('center_axis',(6.19323182390956E-32,0.,-1.));
#111259=DIRECTION('ref_axis',(0.,1.,0.));
#111260=DIRECTION('',(5.85782591378957E-32,1.23467863058847E-16,-1.));
#111261=DIRECTION('',(-6.19323182390956E-32,-1.23467863058847E-16,1.));
#111262=DIRECTION('center_axis',(0.,-1.,0.));
#111263=DIRECTION('ref_axis',(1.,0.,0.));
#111264=DIRECTION('',(5.01606788234257E-16,1.,0.));
#111265=DIRECTION('center_axis',(-1.,5.01606788234257E-16,0.));
#111266=DIRECTION('ref_axis',(0.,-1.,0.));
#111267=DIRECTION('center_axis',(1.,0.,0.));
#111268=DIRECTION('ref_axis',(0.,-1.,0.));
#111269=DIRECTION('center_axis',(0.,1.,0.));
#111270=DIRECTION('ref_axis',(0.,0.,1.));
#111271=DIRECTION('center_axis',(-1.,0.,0.));
#111272=DIRECTION('ref_axis',(0.,-1.,0.));
#111273=DIRECTION('center_axis',(1.,-5.01606788234257E-16,0.));
#111274=DIRECTION('ref_axis',(5.01606788234257E-16,1.,0.));
#111275=DIRECTION('',(1.,-5.01606788234257E-16,0.));
#111276=DIRECTION('center_axis',(1.,0.,0.));
#111277=DIRECTION('ref_axis',(0.,1.,0.));
#111278=DIRECTION('center_axis',(1.,-5.01606788234257E-16,0.));
#111279=DIRECTION('ref_axis',(0.,1.,0.));
#111280=DIRECTION('center_axis',(0.,-1.,0.));
#111281=DIRECTION('ref_axis',(0.,0.,-1.));
#111282=DIRECTION('center_axis',(-1.,0.,0.));
#111283=DIRECTION('ref_axis',(0.,1.,0.));
#111284=DIRECTION('center_axis',(0.,0.,-1.));
#111285=DIRECTION('ref_axis',(-1.,0.,0.));
#111286=DIRECTION('center_axis',(-2.85977186515575E-47,0.,-1.));
#111287=DIRECTION('ref_axis',(0.,1.,0.));
#111288=DIRECTION('',(2.85977186515575E-47,5.70122241611331E-32,1.));
#111289=DIRECTION('center_axis',(0.,0.,-1.));
#111290=DIRECTION('ref_axis',(-1.,0.,0.));
#111291=DIRECTION('center_axis',(1.,-5.01606788234257E-16,0.));
